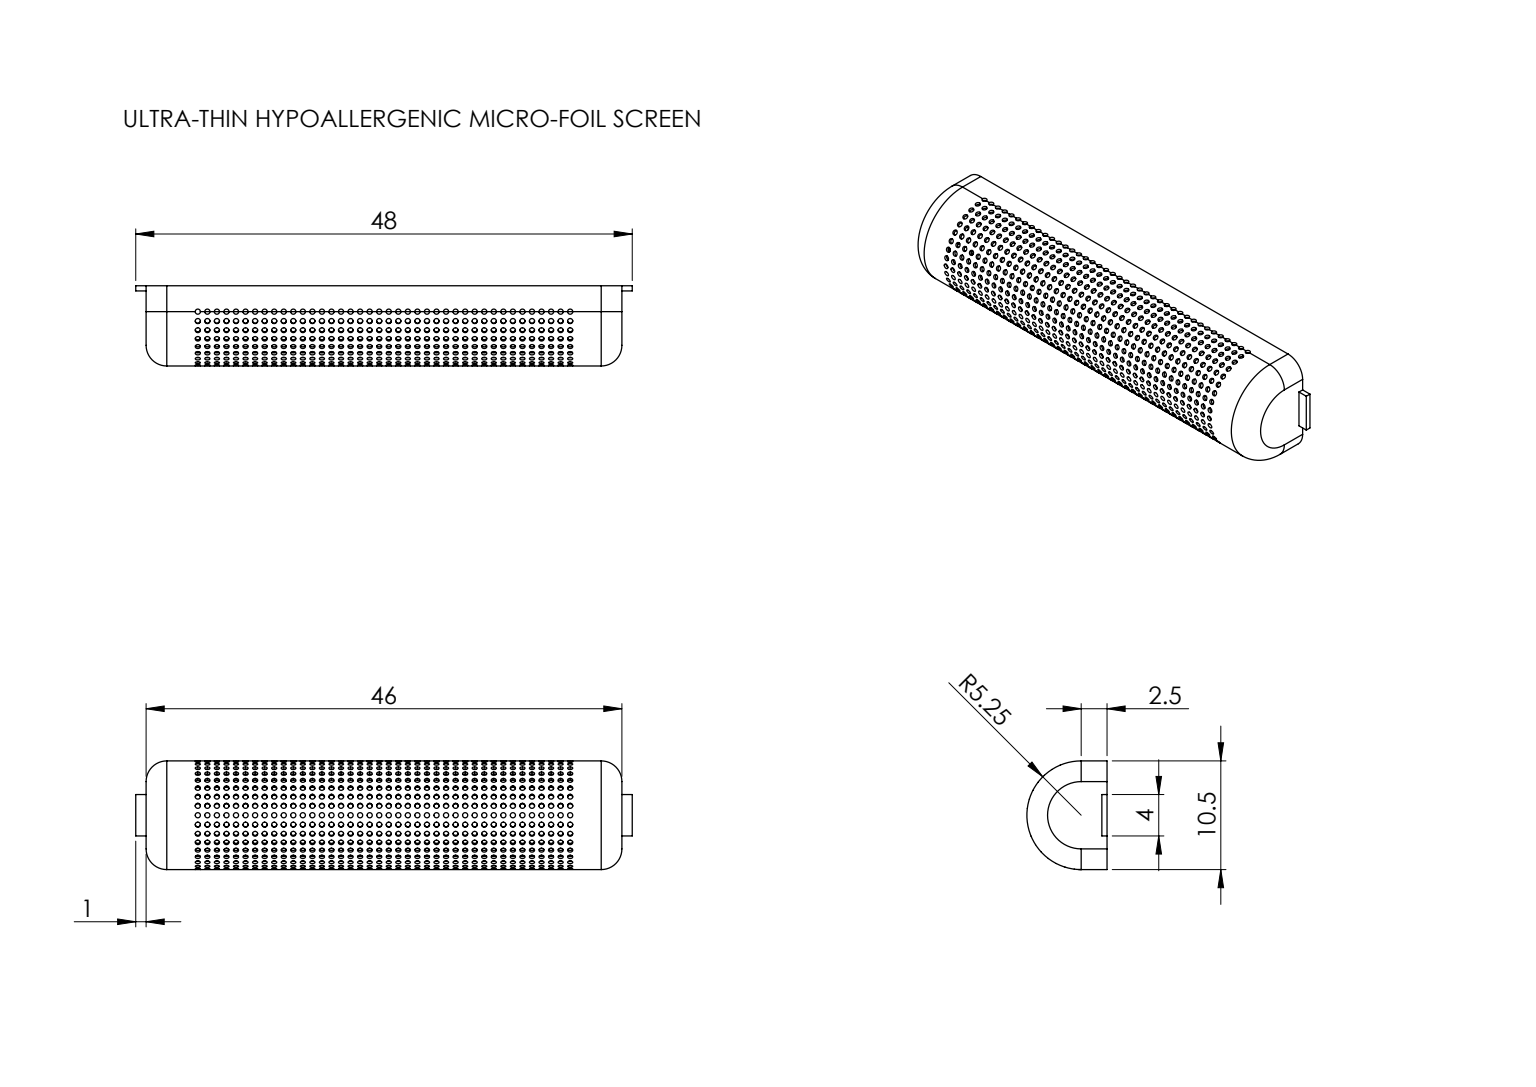
ISO-10303-21;
HEADER;
FILE_DESCRIPTION (('STEP AP214'),
    '1' );
FILE_NAME ('Ultra-Thin Hypoallergenic Micro-Foil Screen.step',
    '2026-10-05T05:16:24',
    ( '' ),
    ( '' ),
    'SwSTEP 2.0',
    'SolidWorks 2026',
    '' );
FILE_SCHEMA (( 'AUTOMOTIVE_DESIGN' ));
ENDSEC;

DATA;
#1=ORIENTED_EDGE ( 'NONE', *, *, #60678, .F. ) ;
#2=CARTESIAN_POINT ( 'NONE',  ( 7.173131342990376247, -12.65882529074907126, 30.72640787790839312 ) ) ;
#3=VERTEX_POINT ( 'NONE', #26210 ) ;
#4=CARTESIAN_POINT ( 'NONE',  ( -5.143005456283213483, -4.661471528628507777, 34.16647553114621871 ) ) ;
#5=CARTESIAN_POINT ( 'NONE',  ( -13.13461538461396394, -7.500000000000154543, 35.00000000000007105 ) ) ;
#6=CARTESIAN_POINT ( 'NONE',  ( 9.561616225640134914, -4.809359713505814149, 33.96456829005828837 ) ) ;
#7=EDGE_LOOP ( 'NONE', ( #52254, #76310 ) ) ;
#8=CARTESIAN_POINT ( 'NONE',  ( -3.230769230769352962, -3.643525952248796163, 33.31231777344771672 ) ) ;
#10=VERTEX_POINT ( 'NONE', #55017 ) ;
#11=CARTESIAN_POINT ( 'NONE',  ( 8.096099255531889582, -12.68172785388650681, 30.59649109432439218 ) ) ;
#12=ORIENTED_EDGE ( 'NONE', *, *, #66253, .T. ) ;
#13=CARTESIAN_POINT ( 'NONE',  ( -14.17690186672535901, -11.93129842949671726, 32.56571108434900452 ) ) ;
#14=ORIENTED_EDGE ( 'NONE', *, *, #40073, .T. ) ;
#15=CARTESIAN_POINT ( 'NONE',  ( 1.634669696253701288, -6.567000820036038355, 34.66262288849541306 ) ) ;
#16=AXIS2_PLACEMENT_3D ( 'NONE', #36065, #63514, #64832 ) ;
#17=CARTESIAN_POINT ( 'NONE',  ( 12.46153846153846168, -2.292212530054420494, 30.41441678777542634 ) ) ;
#18=FACE_BOUND ( 'NONE', #68088, .T. ) ;
#19=CARTESIAN_POINT ( 'NONE',  ( -17.93480601821664777, -2.506253911140446711, 29.99999999999985434 ) ) ;
#20=CARTESIAN_POINT ( 'NONE',  ( 16.08776377448601735, -3.322132147404559976, 32.92929555188719348 ) ) ;
#21=CARTESIAN_POINT ( 'NONE',  ( 9.562159722575998444, -2.373036134822904319, 30.88089517874952250 ) ) ;
#22=CARTESIAN_POINT ( 'NONE',  ( 10.36540787133602493, -10.06842814019191401, 34.32929386961144758 ) ) ;
#23=CARTESIAN_POINT ( 'NONE',  ( -3.230769230769351186, -3.300289026999228881, 32.46337939537708905 ) ) ;
#24=CARTESIAN_POINT ( 'NONE',  ( -8.096177070375302876, -9.356822207818506598, 34.66110646841856635 ) ) ;
#25=DIRECTION ( 'NONE',  ( -0.000000000000000000, 1.000000000000000000, 3.491481338843133355E-15 ) ) ;
#26=ORIENTED_EDGE ( 'NONE', *, *, #20674, .T. ) ;
#27=ORIENTED_EDGE ( 'NONE', *, *, #74196, .T. ) ;
#28=CARTESIAN_POINT ( 'NONE',  ( -17.07692307692307665, -9.780366693483667717, 34.19971097300155094 ) ) ;
#29=CYLINDRICAL_SURFACE ( 'NONE', #7462, 0.2499999999999994726 ) ;
#30=FACE_OUTER_BOUND ( 'NONE', #56324, .T. ) ;
#31=CARTESIAN_POINT ( 'NONE',  ( 3.453548772037640990, -10.81320215134717344, 33.49497208177562868 ) ) ;
#32=CARTESIAN_POINT ( 'NONE',  ( 9.019230769230707878, -7.565270000091922853, 34.99999999999999289 ) ) ;
#33=CARTESIAN_POINT ( 'NONE',  ( 11.53846153846153832, -12.09954503811598769, 35.62045528018868623 ) ) ;
#34=ORIENTED_EDGE ( 'NONE', *, *, #66033, .T. ) ;
#35=CARTESIAN_POINT ( 'NONE',  ( 2.057669070399343436, -9.271318131107980420, 34.42618302367067429 ) ) ;
#36=CARTESIAN_POINT ( 'NONE',  ( 3.453548772037639214, -11.41317474335729187, 32.86274602512330034 ) ) ;
#37=CARTESIAN_POINT ( 'NONE',  ( -14.08491263871424160, -12.47679350104403007, 31.42216943046555855 ) ) ;
#38=CARTESIAN_POINT ( 'NONE',  ( -7.053224892808619195, -6.809168938359898782, 34.95455904226513866 ) ) ;
#40=EDGE_LOOP ( 'NONE', ( #88640, #57937, #33954, #2221 ) ) ;
#41=VECTOR ( 'NONE', #83929, 1000.000000000000000 ) ;
#42=VECTOR ( 'NONE', #62583, 1000.000000000000114 ) ;
#44=CARTESIAN_POINT ( 'NONE',  ( -4.153846153846274980, -8.656820664282941280, 34.87096338111179961 ) ) ;
#45=VERTEX_POINT ( 'NONE', #81605 ) ;
#46=DIRECTION ( 'NONE',  ( -0.000000000000000000, 1.000000000000000000, 3.491481338843133355E-15 ) ) ;
#47=CARTESIAN_POINT ( 'NONE',  ( 15.45378207486262667, -4.026326845037962343, 33.68677907613344047 ) ) ;
#48=CARTESIAN_POINT ( 'NONE',  ( 4.946775867484856093, -6.852621066184267029, 34.70813303252209181 ) ) ;
#50=CIRCLE ( 'NONE', #37444, 0.2500000000000002220 ) ;
#51=CIRCLE ( 'NONE', #79120, 0.2500000000000002220 ) ;
#52=DIRECTION ( 'NONE',  ( 0.000000000000000000, 0.9848077530122072432, 0.1736481776669354937 ) ) ;
#53=VERTEX_POINT ( 'NONE', #13143 ) ;
#55=CARTESIAN_POINT ( 'NONE',  ( -15.23076923076922995, -2.486705287966279876, 31.30864560766543647 ) ) ;
#56=CARTESIAN_POINT ( 'NONE',  ( -0.5276208408985970655, -5.471508081941601986, 34.59228464037088457 ) ) ;
#57=VERTEX_POINT ( 'NONE', #40625 ) ;
#58=CARTESIAN_POINT ( 'NONE',  ( -6.923076923076922462, -2.499999999999998668, 29.50000000000001066 ) ) ;
#59=CYLINDRICAL_SURFACE ( 'NONE', #2416, 0.2500000000000002220 ) ;
#60=CARTESIAN_POINT ( 'NONE',  ( -13.60754160213153163, -4.887634598454295265, 34.01352882383564946 ) ) ;
#61=CARTESIAN_POINT ( 'NONE',  ( 11.53846153846153832, -9.905515769479276145, 34.41647553114623292 ) ) ;
#62=CARTESIAN_POINT ( 'NONE',  ( 2.438482748659261290, -2.494656445102013453, 31.33466734024120015 ) ) ;
#64=CARTESIAN_POINT ( 'NONE',  ( -3.454254174493178287, -6.760086850603068243, 34.69517049084099369 ) ) ;
#67=CARTESIAN_POINT ( 'NONE',  ( 15.00784301325308157, -8.239355502252617924, 34.69524867566427417 ) ) ;
#68=CARTESIAN_POINT ( 'NONE',  ( -14.17716686945866122, -3.625058011473228703, 33.29252011169590020 ) ) ;
#69=EDGE_CURVE ( 'NONE', #39109, #41438, #13798, .T. ) ;
#70=CARTESIAN_POINT ( 'NONE',  ( 9.692307692307695177, -10.67929555188718282, 33.92786785259544047 ) ) ;
#71=ORIENTED_EDGE ( 'NONE', *, *, #84593, .F. ) ;
#72=ORIENTED_EDGE ( 'NONE', *, *, #88944, .T. ) ;
#73=CARTESIAN_POINT ( 'NONE',  ( 20.74999999999998224, -2.499999999999999556, 27.25000000000000000 ) ) ;
#74=CARTESIAN_POINT ( 'NONE',  ( -3.100243529005668019, -6.001044277235011215, 34.52024696741798948 ) ) ;
#75=CARTESIAN_POINT ( 'NONE',  ( -16.15384615384627409, -3.835265460704628815, 33.15142922262033665 ) ) ;
#76=CARTESIAN_POINT ( 'NONE',  ( 8.769230769230768274, -1.466349020453238561, 30.81389545987213907 ) ) ;
#77=CARTESIAN_POINT ( 'NONE',  ( 17.86985203026830504, -2.647304123082329763, 31.75400227202886683 ) ) ;
#78=ORIENTED_EDGE ( 'NONE', *, *, #41184, .T. ) ;
#79=DIRECTION ( 'NONE',  ( 0.000000000000000000, 0.000000000000000000, 1.000000000000000000 ) ) ;
#81=CARTESIAN_POINT ( 'NONE',  ( -14.53117725141625094, -2.847400154188067578, 31.58180166144859058 ) ) ;
#82=LINE ( 'NONE', #529, #19231 ) ;
#83=AXIS2_PLACEMENT_3D ( 'NONE', #55221, #39954, #48454 ) ;
#84=ORIENTED_EDGE ( 'NONE', *, *, #75949, .F. ) ;
#86=EDGE_LOOP ( 'NONE', ( #15345, #5769, #84477, #70207 ) ) ;
#87=CARTESIAN_POINT ( 'NONE',  ( -16.28453762051371712, -5.582088688514999397, 34.36776431015576350 ) ) ;
#88=CYLINDRICAL_SURFACE ( 'NONE', #13871, 0.2499999999999997502 ) ;
#90=B_SPLINE_CURVE_WITH_KNOTS ( 'NONE', 3,
 ( #88183, #40422, #6186, #26896, #54800, #20574, #33653, #54355, #75089, #55682 ),
 .UNSPECIFIED., .F., .F.,
 ( 4, 2, 2, 2, 4 ),
 ( 0.000000000000000000, 0.0001954311564186868202, 0.0003908623128373736404, 0.0005862934692560604335, 0.0007817246256747472808 ),
 .UNSPECIFIED. ) ;
#91=CARTESIAN_POINT ( 'NONE',  ( 10.74591005361826035, -11.66157788607254098, 32.95092075102925833 ) ) ;
#92=CYLINDRICAL_SURFACE ( 'NONE', #79519, 0.2499999999999986955 ) ;
#93=CARTESIAN_POINT ( 'NONE',  ( 1.319344938654610333, -4.481592998940161721, 33.73612834413957984 ) ) ;
#94=CARTESIAN_POINT ( 'NONE',  ( -8.096177070375304652, -4.931416488878822335, 34.32920672191015399 ) ) ;
#95=DIRECTION ( 'NONE',  ( -0.000000000000000000, -0.7660444431189791237, -0.6427876096865379196 ) ) ;
#96=EDGE_CURVE ( 'NONE', #40194, #70315, #60434, .T. ) ;
#97=ORIENTED_EDGE ( 'NONE', *, *, #11144, .F. ) ;
#98=AXIS2_PLACEMENT_3D ( 'NONE', #21974, #77793, #7575 ) ;
#99=FACE_BOUND ( 'NONE', #31817, .T. ) ;
#100=ORIENTED_EDGE ( 'NONE', *, *, #35787, .T. ) ;
#101=CYLINDRICAL_SURFACE ( 'NONE', #51513, 0.2499999999999973355 ) ;
#102=VECTOR ( 'NONE', #77496, 999.9999999999998863 ) ;
#105=EDGE_CURVE ( 'NONE', #4412, #9551, #46022, .T. ) ;
#106=CARTESIAN_POINT ( 'NONE',  ( 4.853996859406928266, -11.76352882383564769, 32.36236540154569497 ) ) ;
#107=CARTESIAN_POINT ( 'NONE',  ( 5.999999999999878320, -5.941354392335915335, 34.76329471203413846 ) ) ;
#108=CARTESIAN_POINT ( 'NONE',  ( 7.145856464345329506, -10.11255958852956027, 34.01340905677048454 ) ) ;
#109=VECTOR ( 'NONE', #52522, 1000.000000000000227 ) ;
#110=EDGE_LOOP ( 'NONE', ( #30011, #23876 ) ) ;
#112=EDGE_LOOP ( 'NONE', ( #70272, #77319 ) ) ;
#113=FACE_OUTER_BOUND ( 'NONE', #58827, .T. ) ;
#114=ORIENTED_EDGE ( 'NONE', *, *, #66071, .T. ) ;
#115=CARTESIAN_POINT ( 'NONE',  ( 4.219913487196229163, -9.905515769479277921, 34.41647553114623292 ) ) ;
#116=B_SPLINE_CURVE_WITH_KNOTS ( 'NONE', 3,
 ( #3209, #77983, #15855, #1446, #43753, #43319, #9097, #77545, #29810, #58146 ),
 .UNSPECIFIED., .F., .F.,
 ( 4, 2, 2, 2, 4 ),
 ( 0.000000000000000000, 0.0001954311564186862239, 0.0003908623128373724478, 0.0005862934692560586988, 0.0007817246256747448956 ),
 .UNSPECIFIED. ) ;
#117=CARTESIAN_POINT ( 'NONE',  ( -11.76138849736838488, -5.582147617184174848, 34.63737895849758530 ) ) ;
#118=DIRECTION ( 'NONE',  ( 0.000000000000000000, 0.8660254037844377084, 0.5000000000000015543 ) ) ;
#119=B_SPLINE_CURVE_WITH_KNOTS ( 'NONE', 3,
 ( #65439, #64982, #64535, #3731, #23563, #51451, #79408, #16806, #85720, #17710 ),
 .UNSPECIFIED., .F., .F.,
 ( 4, 2, 2, 2, 4 ),
 ( 0.000000000000000000, 0.0001954311564186878773, 0.0003908623128373757546, 0.0005862934692560635777, 0.0007817246256747515092 ),
 .UNSPECIFIED. ) ;
#120=CARTESIAN_POINT ( 'NONE',  ( 3.361294669002876656, -9.503571793651733657, 34.60286762892837942 ) ) ;
#122=CARTESIAN_POINT ( 'NONE',  ( 5.207448778686637247, -11.46989282347013095, 32.79007818306219946 ) ) ;
#123=FACE_OUTER_BOUND ( 'NONE', #61461, .T. ) ;
#124=CARTESIAN_POINT ( 'NONE',  ( 17.29970261819148902, -2.600157965045223563, 30.74683119005207033 ) ) ;
#126=VERTEX_POINT ( 'NONE', #50456 ) ;
#127=ORIENTED_EDGE ( 'NONE', *, *, #9186, .F. ) ;
#128=CARTESIAN_POINT ( 'NONE',  ( -11.76194648218548622, -12.44517049084099725, 30.48991314939691932 ) ) ;
#129=DIRECTION ( 'NONE',  ( -0.000000000000000000, -0.1736481776669307198, -0.9848077530122080203 ) ) ;
#131=VECTOR ( 'NONE', #1295, 1000.000000000000000 ) ;
#132=CARTESIAN_POINT ( 'NONE',  ( -9.692307692307691624, -13.75783147151868846, 33.36296068462461051 ) ) ;
#133=FACE_OUTER_BOUND ( 'NONE', #80352, .T. ) ;
#134=FACE_BOUND ( 'NONE', #49727, .T. ) ;
#135=CARTESIAN_POINT ( 'NONE',  ( 7.976679547917409963, -11.46989282347013095, 32.79007818306219946 ) ) ;
#136=ORIENTED_EDGE ( 'NONE', *, *, #30561, .F. ) ;
#137=LINE ( 'NONE', #38123, #5695 ) ;
#138=LINE ( 'NONE', #88449, #37538 ) ;
#139=CARTESIAN_POINT ( 'NONE',  ( -1.515305987725692694, -3.338472653186242756, 32.95098750199972670 ) ) ;
#141=EDGE_LOOP ( 'NONE', ( #49067, #42517 ) ) ;
#142=DIRECTION ( 'NONE',  ( -1.000000000000000000, 0.000000000000000000, 0.000000000000000000 ) ) ;
#143=ORIENTED_EDGE ( 'NONE', *, *, #6318, .F. ) ;
#144=FACE_BOUND ( 'NONE', #88806, .T. ) ;
#145=CARTESIAN_POINT ( 'NONE',  ( -17.14219307747939425, -4.320704448112772766, 33.92786785259540494 ) ) ;
#146=CARTESIAN_POINT ( 'NONE',  ( -6.249999999999997335, -7.433931650972300353, 34.75000000000000711 ) ) ;
#147=CARTESIAN_POINT ( 'NONE',  ( -12.46153846153846168, -11.91647553114624181, 32.58852847137148245 ) ) ;
#148=VERTEX_POINT ( 'NONE', #49138 ) ;
#149=CARTESIAN_POINT ( 'NONE',  ( -1.384615384615383471, -12.29105614889573062, 35.45975837776705220 ) ) ;
#150=CARTESIAN_POINT ( 'NONE',  ( 4.153846153846154188, -1.367168528481310208, 33.57946703557072254 ) ) ;
#151=DIRECTION ( 'NONE',  ( -0.000000000000000000, -0.7660444431189791237, -0.6427876096865379196 ) ) ;
#152=CYLINDRICAL_SURFACE ( 'NONE', #86329, 0.2499999999999979738 ) ;
#153=ORIENTED_EDGE ( 'NONE', *, *, #56606, .F. ) ;
#154=ADVANCED_FACE ( 'NONE', ( #8609 ), #21669, .F. ) ;
#155=CARTESIAN_POINT ( 'NONE',  ( 17.99999999999987566, -5.219633306517616589, 34.19971097300220464 ) ) ;
#157=CYLINDRICAL_SURFACE ( 'NONE', #25456, 0.2499999999999997502 ) ;
#158=EDGE_LOOP ( 'NONE', ( #23871, #73123 ) ) ;
#159=DIRECTION ( 'NONE',  ( -0.000000000000000000, -0.000000000000000000, -1.000000000000000000 ) ) ;
#160=CARTESIAN_POINT ( 'NONE',  ( 0.7114838709165050012, -10.92531984108285670, 33.72920026020278073 ) ) ;
#161=CARTESIAN_POINT ( 'NONE',  ( -4.946397375159514276, -8.586989748646452369, 34.63063291749215011 ) ) ;
#162=CARTESIAN_POINT ( 'NONE',  ( -13.16183584334697265, -3.755027918224367323, 33.06320215134714857 ) ) ;
#163=LINE ( 'NONE', #28079, #50987 ) ;
#164=CARTESIAN_POINT ( 'NONE',  ( 9.019230769230768274, -2.249999999999998668, 29.75000000000000355 ) ) ;
#165=CARTESIAN_POINT ( 'NONE',  ( 6.923076923076802558, -6.026961402154118908, 34.52809138561165270 ) ) ;
#166=B_SPLINE_CURVE_WITH_KNOTS ( 'NONE', 3,
 ( #17891, #45348, #37256, #46689, #46249, #54325, #5263, #80940, #74167, #26867 ),
 .UNSPECIFIED., .F., .F.,
 ( 4, 2, 2, 2, 4 ),
 ( 0.0007817359430256306564, 0.0009771253907249969738, 0.001172514838424363291, 0.001367904286123729826, 0.001563293733823096143 ),
 .UNSPECIFIED. ) ;
#167=CARTESIAN_POINT ( 'NONE',  ( 7.976945653978636308, -4.118422570099831148, 33.43335022499816489 ) ) ;
#170=B_SPLINE_CURVE_WITH_KNOTS ( 'NONE', 3,
 ( #23736, #63848, #16993, #84585, #2145, #85454, #30936, #70611, #58864, #78697 ),
 .UNSPECIFIED., .F., .F.,
 ( 4, 2, 2, 2, 4 ),
 ( 0.000000000000000000, 0.0001954339857564080165, 0.0003908679715128160329, 0.0005863019572692240765, 0.0007817359430256320659 ),
 .UNSPECIFIED. ) ;
#171=CARTESIAN_POINT ( 'NONE',  ( -17.86947429823644029, -9.417988943895561960, 34.36773134775778260 ) ) ;
#172=ORIENTED_EDGE ( 'NONE', *, *, #13053, .F. ) ;
#173=AXIS2_PLACEMENT_3D ( 'NONE', #50512, #36570, #71672 ) ;
#174=EDGE_CURVE ( 'NONE', #81993, #52360, #48073, .T. ) ;
#175=ORIENTED_EDGE ( 'NONE', *, *, #79367, .F. ) ;
#178=CARTESIAN_POINT ( 'NONE',  ( -5.326946301144536378, -11.56360843649121861, 33.07473185843129926 ) ) ;
#180=CARTESIAN_POINT ( 'NONE',  ( 14.37376065869474751, -11.16473453929635440, 33.15142922261926373 ) ) ;
#182=CARTESIAN_POINT ( 'NONE',  ( 16.15384615384603251, -12.46129190930018460, 30.37095296980731973 ) ) ;
#183=CYLINDRICAL_SURFACE ( 'NONE', #47613, 0.2499999999999986955 ) ;
#184=AXIS2_PLACEMENT_3D ( 'NONE', #19967, #48769, #88028 ) ;
#185=DIRECTION ( 'NONE',  ( -0.000000000000000000, 0.1736481776669307198, -0.9848077530122080203 ) ) ;
#186=CARTESIAN_POINT ( 'NONE',  ( -1.384615384615383471, -4.098570777380720287, 33.41473453929634729 ) ) ;
#189=CARTESIAN_POINT ( 'NONE',  ( 10.55011416942384272, -2.625532179533445198, 30.86335684631481513 ) ) ;
#190=CARTESIAN_POINT ( 'NONE',  ( -16.94613263595612906, -10.70102852606553157, 33.91149625220312913 ) ) ;
#191=EDGE_CURVE ( 'NONE', #15565, #57014, #22554, .T. ) ;
#192=FACE_OUTER_BOUND ( 'NONE', #7478, .T. ) ;
#193=CARTESIAN_POINT ( 'NONE',  ( 11.53846153846141753, -5.219633306517616589, 34.19971097300220464 ) ) ;
#194=EDGE_CURVE ( 'NONE', #29769, #50046, #28803, .T. ) ;
#196=ORIENTED_EDGE ( 'NONE', *, *, #14784, .T. ) ;
#197=CARTESIAN_POINT ( 'NONE',  ( -7.173076923076921574, -2.249999999999998668, 29.75000000000000355 ) ) ;
#198=CARTESIAN_POINT ( 'NONE',  ( 1.515140822849032176, -3.625058011473228259, 33.29252011169590020 ) ) ;
#199=CARTESIAN_POINT ( 'NONE',  ( -6.792286482109973988, -11.93129842949671726, 32.56571108434900452 ) ) ;
#200=CARTESIAN_POINT ( 'NONE',  ( 0.3954560821783253965, -9.905515769479277921, 34.41647553114623292 ) ) ;
#202=CARTESIAN_POINT ( 'NONE',  ( 9.823098133274644539, -11.37503395064541678, 33.29242100308974273 ) ) ;
#203=FACE_OUTER_BOUND ( 'NONE', #61905, .T. ) ;
#204=AXIS2_PLACEMENT_3D ( 'NONE', #81774, #26380, #5659 ) ;
#205=CARTESIAN_POINT ( 'NONE',  ( -12.46153846153858247, -10.90142922262034020, 33.41473453929536674 ) ) ;
#206=B_SPLINE_CURVE_WITH_KNOTS ( 'NONE', 3,
 ( #5381, #32848, #40069, #18451, #4487, #53554, #45461, #67081, #59870, #45907 ),
 .UNSPECIFIED., .F., .F.,
 ( 4, 2, 2, 2, 4 ),
 ( 0.000000000000000000, 0.0001954311564186865763, 0.0003908623128373731525, 0.0005862934692560596746, 0.0007817246256747463051 ),
 .UNSPECIFIED. ) ;
#207=EDGE_CURVE ( 'NONE', #60261, #51867, #35183, .T. ) ;
#208=ORIENTED_EDGE ( 'NONE', *, *, #85819, .F. ) ;
#209=FACE_OUTER_BOUND ( 'NONE', #38454, .T. ) ;
#210=EDGE_CURVE ( 'NONE', #70883, #82406, #15810, .T. ) ;
#211=ORIENTED_EDGE ( 'NONE', *, *, #69069, .F. ) ;
#212=CARTESIAN_POINT ( 'NONE',  ( 16.15384615384603251, -9.528491918059723176, 34.59228464037033035 ) ) ;
#213=CARTESIAN_POINT ( 'NONE',  ( 8.769230769230645706, -9.528491918059723176, 34.59228464037033035 ) ) ;
#214=EDGE_CURVE ( 'NONE', #41163, #3816, #38532, .T. ) ;
#215=CARTESIAN_POINT ( 'NONE',  ( 14.05771557674995442, -4.943428324936578910, 34.04746400365624481 ) ) ;
#216=EDGE_CURVE ( 'NONE', #29227, #38893, #56032, .T. ) ;
#217=CARTESIAN_POINT ( 'NONE',  ( 16.15384615384615330, -13.63283147151868846, 33.57946703557072254 ) ) ;
#219=VERTEX_POINT ( 'NONE', #73411 ) ;
#220=ORIENTED_EDGE ( 'NONE', *, *, #40538, .F. ) ;
#221=VERTEX_POINT ( 'NONE', #52233 ) ;
#222=ORIENTED_EDGE ( 'NONE', *, *, #80830, .F. ) ;
#223=CARTESIAN_POINT ( 'NONE',  ( -10.68065461594093257, -12.51329471203370325, 31.30864560766548976 ) ) ;
#224=CARTESIAN_POINT ( 'NONE',  ( 7.596130608860882205, -3.711651800289232916, 33.01384336483936011 ) ) ;
#225=CARTESIAN_POINT ( 'NONE',  ( 4.153846153846030731, -12.16647553114689728, 32.15551576947799362 ) ) ;
#226=AXIS2_PLACEMENT_3D ( 'NONE', #60512, #52858, #32161 ) ;
#228=CARTESIAN_POINT ( 'NONE',  ( -7.846153846153844924, -4.786620604624113540, 33.94971097300155094 ) ) ;
#229=CARTESIAN_POINT ( 'NONE',  ( -15.23076923076922995, -2.486705287966279876, 31.30864560766543647 ) ) ;
#230=ORIENTED_EDGE ( 'NONE', *, *, #73529, .T. ) ;
#232=AXIS2_PLACEMENT_3D ( 'NONE', #57713, #64451, #65352 ) ;
#233=ORIENTED_EDGE ( 'NONE', *, *, #46432, .F. ) ;
#234=CARTESIAN_POINT ( 'NONE',  ( 8.769230769230647482, -9.442884908241554243, 34.35708131394783038 ) ) ;
#236=CARTESIAN_POINT ( 'NONE',  ( 17.29970274590113632, -10.97394488606063589, 33.68653795673696294 ) ) ;
#237=CARTESIAN_POINT ( 'NONE',  ( -5.010854725920638408, -11.16473453929635440, 33.15142922261926373 ) ) ;
#238=EDGE_CURVE ( 'NONE', #50121, #11896, #56698, .T. ) ;
#240=ORIENTED_EDGE ( 'NONE', *, *, #48332, .T. ) ;
#241=EDGE_CURVE ( 'NONE', #37535, #9541, #20178, .T. ) ;
#242=ORIENTED_EDGE ( 'NONE', *, *, #19023, .F. ) ;
#243=ADVANCED_FACE ( 'NONE', ( #11714 ), #66194, .F. ) ;
#244=CARTESIAN_POINT ( 'NONE',  ( 7.846153846153846700, -12.10708131394839349, 31.69288490824020244 ) ) ;
#245=FACE_BOUND ( 'NONE', #29215, .T. ) ;
#246=CARTESIAN_POINT ( 'NONE',  ( 5.076923076922953193, -5.094484230521993062, 34.41647553114689373 ) ) ;
#247=EDGE_CURVE ( 'NONE', #52855, #6141, #63243, .T. ) ;
#248=CARTESIAN_POINT ( 'NONE',  ( -4.376773112753002515, -10.01117774369187252, 34.36070679894347535 ) ) ;
#249=ORIENTED_EDGE ( 'NONE', *, *, #43935, .F. ) ;
#250=CARTESIAN_POINT ( 'NONE',  ( 8.769230769230768274, -11.91647553114624181, 32.58852847137148245 ) ) ;
#251=CARTESIAN_POINT ( 'NONE',  ( 6.923076923076800782, -12.16647553114689728, 32.15551576947799362 ) ) ;
#252=CARTESIAN_POINT ( 'NONE',  ( 16.37685750545900376, -2.554770724473668597, 30.48948780036025852 ) ) ;
#253=CARTESIAN_POINT ( 'NONE',  ( 1.384615384615386802, -10.51840700105979565, 33.73612834413961536 ) ) ;
#254=ORIENTED_EDGE ( 'NONE', *, *, #43401, .T. ) ;
#255=EDGE_CURVE ( 'NONE', #87291, #13888, #15871, .T. ) ;
#256=VECTOR ( 'NONE', #26612, 1000.000000000000227 ) ;
#257=CARTESIAN_POINT ( 'NONE',  ( -0.5268613770306369570, -7.749976743299138882, 34.99404534957040624 ) ) ;
#258=CARTESIAN_POINT ( 'NONE',  ( 1.634560902963528184, -8.433404298154336232, 34.66254593164985920 ) ) ;
#259=CARTESIAN_POINT ( 'NONE',  ( -12.68446467905460473, -12.15238873228292071, 31.58232369045353849 ) ) ;
#260=CARTESIAN_POINT ( 'NONE',  ( -2.557715544985271094, -10.76384336483936011, 33.53834819971076087 ) ) ;
#261=LINE ( 'NONE', #27723, #60185 ) ;
#262=FACE_BOUND ( 'NONE', #7058, .T. ) ;
#263=CARTESIAN_POINT ( 'NONE',  ( 17.07692307692295586, -3.835265460704628815, 33.15142922262033665 ) ) ;
#264=CARTESIAN_POINT ( 'NONE',  ( 16.82694633287448838, -2.920706130388546651, 32.31842814019191223 ) ) ;
#265=CARTESIAN_POINT ( 'NONE',  ( 5.326868486301119532, -9.357781135181031829, 34.66075350412533851 ) ) ;
#266=DIRECTION ( 'NONE',  ( 0.000000000000000000, 0.9848077530122072432, 0.1736481776669354937 ) ) ;
#267=CARTESIAN_POINT ( 'NONE',  ( -11.47239420511146513, -10.67929555188718282, 33.92786785259544757 ) ) ;
#268=AXIS2_PLACEMENT_3D ( 'NONE', #2934, #72732, #79505 ) ;
#269=CARTESIAN_POINT ( 'NONE',  ( -10.86540783960607115, -6.652501968072648708, 34.93155406624980941 ) ) ;
#271=ORIENTED_EDGE ( 'NONE', *, *, #6399, .T. ) ;
#272=DIRECTION ( 'NONE',  ( -0.000000000000000000, -0.7660444431189791237, -0.6427876096865379196 ) ) ;
#273=VERTEX_POINT ( 'NONE', #30632 ) ;
#274=CARTESIAN_POINT ( 'NONE',  ( 0.5915836243732391919, -2.504778602574659896, 29.97347330155780298 ) ) ;
#275=VERTEX_POINT ( 'NONE', #24313 ) ;
#276=CARTESIAN_POINT ( 'NONE',  ( -11.28840722682322451, -2.779044189368095275, 31.39831045268885745 ) ) ;
#277=CARTESIAN_POINT ( 'NONE',  ( -7.846153846153844924, -9.780366693483667717, 34.19971097300155094 ) ) ;
#278=CARTESIAN_POINT ( 'NONE',  ( 5.999999999999878320, -8.656820664282941280, 34.87096338111179961 ) ) ;
#279=EDGE_LOOP ( 'NONE', ( #7724, #29052, #33264, #45854 ) ) ;
#280=CARTESIAN_POINT ( 'NONE',  ( 5.299935921016470708, -11.98016756924215009, 32.48728574198911190 ) ) ;
#283=CARTESIAN_POINT ( 'NONE',  ( 3.903822916553188804, -9.271318131107980420, 34.42618302367067429 ) ) ;
#285=CARTESIAN_POINT ( 'NONE',  ( 12.21156173059611127, -2.779195860258146578, 31.39871582349836032 ) ) ;
#287=CARTESIAN_POINT ( 'NONE',  ( -0.2114841499001467451, -4.235687564193446164, 33.53795663066793509 ) ) ;
#288=CARTESIAN_POINT ( 'NONE',  ( 11.60452988946397745, -3.513871655860379306, 32.76840700105978499 ) ) ;
#290=DIRECTION ( 'NONE',  ( 0.000000000000000000, 0.9396926207859126468, 0.3420201433256571111 ) ) ;
#291=CARTESIAN_POINT ( 'NONE',  ( -1.384615384615383471, -12.78798330534102945, 29.74999999999997868 ) ) ;
#292=VERTEX_POINT ( 'NONE', #79277 ) ;
#295=AXIS2_PLACEMENT_3D ( 'NONE', #58758, #37145, #86253 ) ;
#296=LINE ( 'NONE', #12484, #72000 ) ;
#297=CARTESIAN_POINT ( 'NONE',  ( -8.769230769230892619, -3.643525952248795718, 33.31231777344771672 ) ) ;
#300=CARTESIAN_POINT ( 'NONE',  ( 17.07692307692307665, -12.78798330534102767, 29.49999999999997868 ) ) ;
#301=CARTESIAN_POINT ( 'NONE',  ( 16.15384615384603251, -2.657715359629662544, 31.77849191805970364 ) ) ;
#302=CARTESIAN_POINT ( 'NONE',  ( 4.023698184114458343, -9.504002272028875709, 34.60269587691767867 ) ) ;
#303=ORIENTED_EDGE ( 'NONE', *, *, #59543, .T. ) ;
#304=CYLINDRICAL_SURFACE ( 'NONE', #8160, 0.2500000000000009437 ) ;
#305=CARTESIAN_POINT ( 'NONE',  ( -11.53846153846153655, -2.517432740324522911, 35.29906147534542527 ) ) ;
#306=VECTOR ( 'NONE', #74624, 1000.000000000000000 ) ;
#307=MANIFOLD_SOLID_BREP ( 'Mirror3', #61571 ) ;
#308=CARTESIAN_POINT ( 'NONE',  ( 7.053867364043872712, -11.93129842949671726, 32.56571108434900452 ) ) ;
#309=CARTESIAN_POINT ( 'NONE',  ( -11.53846153846153655, -9.905515769479276145, 34.41647553114623292 ) ) ;
#310=CARTESIAN_POINT ( 'NONE',  ( -13.38461538461550582, -11.94971097300221174, 32.03036669348237098 ) ) ;
#311=ADVANCED_FACE ( 'NONE', ( #54905 ), #17579, .F. ) ;
#313=VERTEX_POINT ( 'NONE', #40952 ) ;
#314=VERTEX_POINT ( 'NONE', #12156 ) ;
#315=EDGE_CURVE ( 'NONE', #65909, #14846, #33750, .T. ) ;
#316=ORIENTED_EDGE ( 'NONE', *, *, #59548, .F. ) ;
#317=CARTESIAN_POINT ( 'NONE',  ( -16.40382289789474513, -3.436278759898155677, 33.07459398097509506 ) ) ;
#318=CARTESIAN_POINT ( 'NONE',  ( 6.673100192134572950, -2.779195860258147022, 31.39871582349836743 ) ) ;
#319=ADVANCED_FACE ( 'NONE', ( #87382 ), #67987, .F. ) ;
#320=CARTESIAN_POINT ( 'NONE',  ( -16.15384615384615330, -11.11383981884818262, 36.00935417666054406 ) ) ;
#321=CARTESIAN_POINT ( 'NONE',  ( -17.29980259366066520, -7.630690623152299956, 34.99857592706774057 ) ) ;
#322=ORIENTED_EDGE ( 'NONE', *, *, #43206, .F. ) ;
#323=ADVANCED_FACE ( 'NONE', ( #5837 ), #60772, .F. ) ;
#324=CARTESIAN_POINT ( 'NONE',  ( -18.13047670811646483, -7.276988635370451597, 34.74523720219453793 ) ) ;
#326=ORIENTED_EDGE ( 'NONE', *, *, #40277, .T. ) ;
#327=VERTEX_POINT ( 'NONE', #68417 ) ;
#328=VERTEX_POINT ( 'NONE', #87839 ) ;
#329=DIRECTION ( 'NONE',  ( 0.000000000000000000, 0.9396926207859126468, -0.3420201433256571111 ) ) ;
#330=ORIENTED_EDGE ( 'NONE', *, *, #1788, .T. ) ;
#331=CARTESIAN_POINT ( 'NONE',  ( 4.403900465484468008, -5.728107161865375829, 34.42597550085002922 ) ) ;
#333=ADVANCED_FACE ( 'NONE', ( #53570 ), #13914, .F. ) ;
#334=B_SPLINE_CURVE_WITH_KNOTS ( 'NONE', 3,
 ( #64908, #72563, #59048, #79330, #31581, #86548, #17176, #4555, #18076, #87001 ),
 .UNSPECIFIED., .F., .F.,
 ( 4, 2, 2, 2, 4 ),
 ( 0.000000000000000000, 0.0001954339857564099680, 0.0003908679715128199361, 0.0005863019572692299312, 0.0007817359430256398721 ),
 .UNSPECIFIED. ) ;
#335=B_SPLINE_CURVE_WITH_KNOTS ( 'NONE', 3,
 ( #13254, #76272, #55557, #69520, #33961, #81720, #26766, #20005, #48800, #61867 ),
 .UNSPECIFIED., .F., .F.,
 ( 4, 2, 2, 2, 4 ),
 ( 0.0007817246256747453293, 0.0009771112852218889842, 0.001172497944769032531, 0.001367884604316176294, 0.001563271263863319840 ),
 .UNSPECIFIED. ) ;
#336=LINE ( 'NONE', #27798, #62504 ) ;
#337=ADVANCED_FACE ( 'NONE', ( #33314 ), #46817, .F. ) ;
#338=CARTESIAN_POINT ( 'NONE',  ( -12.39628289026243557, -12.27809138561124591, 31.22303859784720359 ) ) ;
#340=ORIENTED_EDGE ( 'NONE', *, *, #84982, .F. ) ;
#341=EDGE_LOOP ( 'NONE', ( #3510, #61163, #15292, #57174 ) ) ;
#342=ORIENTED_EDGE ( 'NONE', *, *, #84967, .F. ) ;
#343=CARTESIAN_POINT ( 'NONE',  ( -2.242437168179467477, -3.643525952247864463, 33.31231777344670064 ) ) ;
#344=DIRECTION ( 'NONE',  ( -0.000000000000000000, -0.000000000000000000, -1.000000000000000000 ) ) ;
#346=CARTESIAN_POINT ( 'NONE',  ( 6.792385456409367528, -6.413092428213692742, 34.63065189839063152 ) ) ;
#347=ADVANCED_FACE ( 'NONE', ( #13036 ), #40520, .F. ) ;
#348=DIRECTION ( 'NONE',  ( -0.000000000000000000, 0.9848077530122085754, -0.1736481776669273613 ) ) ;
#349=EDGE_LOOP ( 'NONE', ( #49195, #32576, #79895, #88984 ) ) ;
#350=DIRECTION ( 'NONE',  ( -0.000000000000000000, -0.000000000000000000, -1.000000000000000000 ) ) ;
#352=ORIENTED_EDGE ( 'NONE', *, *, #65664, .F. ) ;
#353=FACE_BOUND ( 'NONE', #30448, .T. ) ;
#354=EDGE_CURVE ( 'NONE', #24770, #59241, #83681, .T. ) ;
#356=CARTESIAN_POINT ( 'NONE',  ( 16.02369818411445834, -2.647304123082329763, 31.75400227202886683 ) ) ;
#358=CARTESIAN_POINT ( 'NONE',  ( 7.912221179503920787, -10.67929555188718282, 33.92786785259544757 ) ) ;
#359=CARTESIAN_POINT ( 'NONE',  ( -0.4615384615384611200, -3.050289026998446396, 32.03036669348365706 ) ) ;
#360=AXIS2_PLACEMENT_3D ( 'NONE', #65343, #45520, #72546 ) ;
#361=FACE_OUTER_BOUND ( 'NONE', #8504, .T. ) ;
#363=VERTEX_POINT ( 'NONE', #29220 ) ;
#364=CARTESIAN_POINT ( 'NONE',  ( 11.53846153846153832, -5.415277668671390821, 36.20867863119892149 ) ) ;
#366=EDGE_LOOP ( 'NONE', ( #41568, #20899 ) ) ;
#367=AXIS2_PLACEMENT_3D ( 'NONE', #88511, #80411, #5626 ) ;
#368=B_SPLINE_CURVE_WITH_KNOTS ( 'NONE', 3,
 ( #9005, #62598, #77017, #71569, #35588, #35137, #64363, #36035, #36472, #2659 ),
 .UNSPECIFIED., .F., .F.,
 ( 4, 2, 2, 2, 4 ),
 ( 0.0007817246256747503166, 0.0009771112852218944052, 0.001172497944769038602, 0.001367884604316182799, 0.001563271263863326996 ),
 .UNSPECIFIED. ) ;
#370=CARTESIAN_POINT ( 'NONE',  ( -14.30769230769242917, -9.528491918059723176, 34.59228464037033035 ) ) ;
#371=CARTESIAN_POINT ( 'NONE',  ( 9.692307692307695177, -2.721908614388771852, 31.22303859784724978 ) ) ;
#372=B_SPLINE_CURVE_WITH_KNOTS ( 'NONE', 3,
 ( #22654, #8712, #16776, #20977, #9578, #2369, #77603, #30301, #37488, #70855 ),
 .UNSPECIFIED., .F., .F.,
 ( 4, 2, 2, 2, 4 ),
 ( 0.0007817246336856289524, 0.0009771112958940101571, 0.001172497958102391253, 0.001367884620310772350, 0.001563271282519153446 ),
 .UNSPECIFIED. ) ;
#373=VERTEX_POINT ( 'NONE', #845 ) ;
#374=CARTESIAN_POINT ( 'NONE',  ( -16.15384615384615330, -11.16473453929635440, 33.15142922261926373 ) ) ;
#375=CYLINDRICAL_SURFACE ( 'NONE', #76000, 0.2499999999999998890 ) ;
#376=FACE_BOUND ( 'NONE', #11299, .T. ) ;
#378=CYLINDRICAL_SURFACE ( 'NONE', #27428, 0.2500000000000002220 ) ;
#379=CARTESIAN_POINT ( 'NONE',  ( -4.087777802843714170, -8.120952969808772792, 34.71129190929999453 ) ) ;
#380=CARTESIAN_POINT ( 'NONE',  ( 7.912222197156284054, -8.973038597847271092, 34.52809138561121216 ) ) ;
#381=CARTESIAN_POINT ( 'NONE',  ( 1.450682717965462443, -12.62096338111211757, 30.90682066428152908 ) ) ;
#382=CARTESIAN_POINT ( 'NONE',  ( 0.2386122440223126528, -5.667676309546436642, 34.40238873228292249 ) ) ;
#383=FACE_OUTER_BOUND ( 'NONE', #27024, .T. ) ;
#385=ORIENTED_EDGE ( 'NONE', *, *, #9056, .F. ) ;
#386=ORIENTED_EDGE ( 'NONE', *, *, #4189, .F. ) ;
#387=CARTESIAN_POINT ( 'NONE',  ( -9.757577692864012775, -2.379036618887870436, 30.90682066428147934 ) ) ;
#388=CARTESIAN_POINT ( 'NONE',  ( 14.37294744720514572, -12.70778746994558439, 30.41441678777536595 ) ) ;
#389=CARTESIAN_POINT ( 'NONE',  ( -12.46153846153846168, -1.466349020453238561, 30.81389545987213907 ) ) ;
#390=CARTESIAN_POINT ( 'NONE',  ( -9.019207513279361876, -8.347322224742351082, 34.93158281831414058 ) ) ;
#391=CARTESIAN_POINT ( 'NONE',  ( 2.980745993476266342, -11.37209801155882971, 32.91403422569032955 ) ) ;
#394=CARTESIAN_POINT ( 'NONE',  ( -11.78846153846154010, -7.566082377512564960, 35.00000000000000711 ) ) ;
#395=CARTESIAN_POINT ( 'NONE',  ( -3.480769230769229061, -7.500000000000001776, 34.75000000000000000 ) ) ;
#396=EDGE_CURVE ( 'NONE', #70653, #65231, #6317, .T. ) ;
#397=CARTESIAN_POINT ( 'NONE',  ( 16.15384615384603251, -2.379036618888197729, 30.90682066428292885 ) ) ;
#398=CARTESIAN_POINT ( 'NONE',  ( 4.403846153847589484, -7.500000000000155431, 34.75000000000007105 ) ) ;
#399=CARTESIAN_POINT ( 'NONE',  ( -15.00798968950082291, -11.41317474335729543, 32.86274602512330034 ) ) ;
#400=CARTESIAN_POINT ( 'NONE',  ( -5.076923076923199218, -6.835583212225970762, 34.95778746994575670 ) ) ;
#401=CARTESIAN_POINT ( 'NONE',  ( 5.933916589044121004, -12.10708131394839349, 31.69288490824020244 ) ) ;
#402=CARTESIAN_POINT ( 'NONE',  ( 14.53047184896071897, -11.89424750095246175, 32.13594075562310337 ) ) ;
#403=LINE ( 'NONE', #13907, #87417 ) ;
#404=ORIENTED_EDGE ( 'NONE', *, *, #80528, .F. ) ;
#405=CARTESIAN_POINT ( 'NONE',  ( -0.2387589202700510504, -3.755027918224367767, 33.06320215134714857 ) ) ;
#406=CARTESIAN_POINT ( 'NONE',  ( 7.622668921589514923, -4.988325925672468131, 34.36044203135681130 ) ) ;
#408=LINE ( 'NONE', #82831, #54785 ) ;
#409=DIRECTION ( 'NONE',  ( -0.000000000000000000, -0.3420201433256694901, -0.9396926207859082059 ) ) ;
#410=ORIENTED_EDGE ( 'NONE', *, *, #80404, .T. ) ;
#411=DIRECTION ( 'NONE',  ( -0.000000000000000000, 1.000000000000000000, 3.491481338843133355E-15 ) ) ;
#412=DIRECTION ( 'NONE',  ( 1.000000000000000000, 0.000000000000000000, 0.000000000000000000 ) ) ;
#413=ORIENTED_EDGE ( 'NONE', *, *, #39036, .T. ) ;
#414=CARTESIAN_POINT ( 'NONE',  ( 13.38461538461538680, -13.20930481340135110, 34.54067556320372745 ) ) ;
#415=DIRECTION ( 'NONE',  ( 0.000000000000000000, 0.000000000000000000, 1.000000000000000000 ) ) ;
#416=ORIENTED_EDGE ( 'NONE', *, *, #77856, .F. ) ;
#419=ORIENTED_EDGE ( 'NONE', *, *, #191, .T. ) ;
#420=CARTESIAN_POINT ( 'NONE',  ( 16.94677586748485609, -11.47017969459903952, 32.78971311882035167 ) ) ;
#421=CARTESIAN_POINT ( 'NONE',  ( 8.096153846155281997, -7.500000000000155431, 34.75000000000007105 ) ) ;
#422=CARTESIAN_POINT ( 'NONE',  ( -15.09997742294444478, -12.38066358083363738, 30.83685684665853444 ) ) ;
#424=ORIENTED_EDGE ( 'NONE', *, *, #87981, .T. ) ;
#425=CARTESIAN_POINT ( 'NONE',  ( -10.36533019547115941, -2.318338780012835443, 30.59689888758630261 ) ) ;
#428=CARTESIAN_POINT ( 'NONE',  ( -14.98071481085577972, -4.074993327901527351, 33.72946981652012255 ) ) ;
#429=CARTESIAN_POINT ( 'NONE',  ( -1.161604033002534786, -2.554770724473667709, 30.48948780036025852 ) ) ;
#430=CARTESIAN_POINT ( 'NONE',  ( -1.384615384615506484, -11.67786785259630911, 32.92929555188603530 ) ) ;
#431=EDGE_CURVE ( 'NONE', #11896, #58120, #76950, .T. ) ;
#432=CARTESIAN_POINT ( 'NONE',  ( 0.4615384615384611200, -9.819645486525091727, 36.12317359536749706 ) ) ;
#433=CARTESIAN_POINT ( 'NONE',  ( -0.4615384615385840772, -5.941354392335915335, 34.76329471203413846 ) ) ;
#434=FACE_OUTER_BOUND ( 'NONE', #71808, .T. ) ;
#435=VECTOR ( 'NONE', #75425, 1000.000000000000000 ) ;
#436=EDGE_CURVE ( 'NONE', #46513, #56514, #28312, .T. ) ;
#437=CARTESIAN_POINT ( 'NONE',  ( 15.90382292962469180, -12.68155406624981119, 30.59749803192733708 ) ) ;
#438=ORIENTED_EDGE ( 'NONE', *, *, #56597, .F. ) ;
#440=CARTESIAN_POINT ( 'NONE',  ( -0.3954701105360236002, -12.10708131394839704, 31.69288490824020954 ) ) ;
#441=VERTEX_POINT ( 'NONE', #70189 ) ;
#443=CARTESIAN_POINT ( 'NONE',  ( -5.142193077479396912, -5.094484230520674117, 34.41647553114621161 ) ) ;
#444=ORIENTED_EDGE ( 'NONE', *, *, #26257, .F. ) ;
#445=CARTESIAN_POINT ( 'NONE',  ( 11.66925197942849302, -3.338503747796866872, 32.95102852606553512 ) ) ;
#446=CARTESIAN_POINT ( 'NONE',  ( 5.076923076922954969, -3.835265460704628371, 33.15142922262033665 ) ) ;
#447=ORIENTED_EDGE ( 'NONE', *, *, #84542, .F. ) ;
#448=DIRECTION ( 'NONE',  ( 0.000000000000000000, 0.000000000000000000, 1.000000000000000000 ) ) ;
#449=EDGE_CURVE ( 'NONE', #49542, #26693, #14245, .T. ) ;
#450=AXIS2_PLACEMENT_3D ( 'NONE', #84938, #2938, #44359 ) ;
#452=CARTESIAN_POINT ( 'NONE',  ( 7.846153846153723244, -12.70778746994576025, 30.41441678777401236 ) ) ;
#453=ORIENTED_EDGE ( 'NONE', *, *, #29446, .F. ) ;
#456=VERTEX_POINT ( 'NONE', #21105 ) ;
#457=CARTESIAN_POINT ( 'NONE',  ( 18.00000000000000000, -6.343179335718451384, 34.87096338111211935 ) ) ;
#458=CARTESIAN_POINT ( 'NONE',  ( -4.284536756956461190, -6.369640206132550553, 34.87707690430378449 ) ) ;
#459=B_SPLINE_CURVE_WITH_KNOTS ( 'NONE', 3,
 ( #38721, #52670, #86941, #51764, #3145, #31061, #37374, #10807, #11251, #64844 ),
 .UNSPECIFIED., .F., .F.,
 ( 4, 2, 2, 2, 4 ),
 ( 0.000000000000000000, 0.0001954339857564073659, 0.0003908679715128147319, 0.0005863019572692221250, 0.0007817359430256294638 ),
 .UNSPECIFIED. ) ;
#460=FACE_BOUND ( 'NONE', #10409, .T. ) ;
#461=EDGE_CURVE ( 'NONE', #35423, #73834, #49030, .T. ) ;
#462=CARTESIAN_POINT ( 'NONE',  ( 5.749976775778542937, -2.341070481393820124, 30.72580821765574299 ) ) ;
#463=CYLINDRICAL_SURFACE ( 'NONE', #51418, 0.2500000000000004996 ) ;
#464=CARTESIAN_POINT ( 'NONE',  ( 9.442330948259105128, -11.47974371597207899, 33.17467449705390692 ) ) ;
#465=CARTESIAN_POINT ( 'NONE',  ( -17.07692307692307665, -12.34228464037088635, 31.77849191805839268 ) ) ;
#466=CARTESIAN_POINT ( 'NONE',  ( -17.32689982097166492, -8.347322224742351082, 34.93158281831414058 ) ) ;
#467=CARTESIAN_POINT ( 'NONE',  ( -4.219116599806928214, -11.48612834413959582, 32.76840700105983473 ) ) ;
#468=EDGE_CURVE ( 'NONE', #6055, #84853, #21558, .T. ) ;
#470=EDGE_LOOP ( 'NONE', ( #48935, #2508, #11631, #61677 ) ) ;
#471=ORIENTED_EDGE ( 'NONE', *, *, #28570, .F. ) ;
#473=CARTESIAN_POINT ( 'NONE',  ( 15.00728428704528561, -12.24155766932282496, 31.33739205006857986 ) ) ;
#474=CARTESIAN_POINT ( 'NONE',  ( -11.66915300512909859, -11.71456829005830080, 32.44064028649416542 ) ) ;
#475=DIRECTION ( 'NONE',  ( -0.000000000000000000, 0.5000000000000011102, -0.8660254037844380415 ) ) ;
#476=CARTESIAN_POINT ( 'NONE',  ( -14.30769230769230660, -3.513871655860378418, 32.76840700105978499 ) ) ;
#477=CYLINDRICAL_SURFACE ( 'NONE', #63424, 0.2499999999999997502 ) ;
#478=EDGE_LOOP ( 'NONE', ( #50034, #54764 ) ) ;
#479=CARTESIAN_POINT ( 'NONE',  ( 13.31853197365950692, -4.786620604624113540, 33.94971097300155805 ) ) ;
#480=EDGE_CURVE ( 'NONE', #74721, #66781, #42289, .T. ) ;
#481=LINE ( 'NONE', #56306, #79055 ) ;
#482=DIRECTION ( 'NONE',  ( 0.000000000000000000, 0.000000000000000000, 1.000000000000000000 ) ) ;
#484=EDGE_LOOP ( 'NONE', ( #60123, #67289, #74118, #28070 ) ) ;
#485=VERTEX_POINT ( 'NONE', #68858 ) ;
#486=AXIS2_PLACEMENT_3D ( 'NONE', #32374, #72456, #59839 ) ;
#487=EDGE_LOOP ( 'NONE', ( #82911, #37209, #13825, #34035 ) ) ;
#488=CARTESIAN_POINT ( 'NONE',  ( -9.442362173959550020, -12.43552623307873972, 30.55307653245132826 ) ) ;
#489=ORIENTED_EDGE ( 'NONE', *, *, #55931, .T. ) ;
#490=CARTESIAN_POINT ( 'NONE',  ( -9.561517251340744039, -9.929761469519743144, 34.40412654351204225 ) ) ;
#491=CYLINDRICAL_SURFACE ( 'NONE', #21511, 0.2500000000000009437 ) ;
#492=CARTESIAN_POINT ( 'NONE',  ( 14.30769230769231015, -5.180354513474913603, 36.12317359536750416 ) ) ;
#494=ADVANCED_FACE ( 'NONE', ( #69745 ), #7164, .F. ) ;
#495=CYLINDRICAL_SURFACE ( 'NONE', #2877, 0.2499999999999986955 ) ;
#497=CARTESIAN_POINT ( 'NONE',  ( 4.403791672194295792, -4.336752205174647656, 33.62275283266504289 ) ) ;
#500=CARTESIAN_POINT ( 'NONE',  ( -9.561781990544126586, -4.459921816937791661, 33.71989282347011851 ) ) ;
#501=CARTESIAN_POINT ( 'NONE',  ( -8.992110285968356820, -7.630690623152299956, 34.99857592706774057 ) ) ;
#502=CYLINDRICAL_SURFACE ( 'NONE', #24257, 0.2500000000000002220 ) ;
#503=B_SPLINE_CURVE_WITH_KNOTS ( 'NONE', 3,
 ( #55324, #55765, #21540, #35953, #49893, #76935, #63408, #77371, #42272, #34617 ),
 .UNSPECIFIED., .F., .F.,
 ( 4, 2, 2, 2, 4 ),
 ( 0.0007817359527651090859, 0.0009771254036996478414, 0.001172514854634186489, 0.001367904305568725136, 0.001563293756503263783 ),
 .UNSPECIFIED. ) ;
#504=EDGE_CURVE ( 'NONE', #73834, #24183, #58251, .T. ) ;
#506=CARTESIAN_POINT ( 'NONE',  ( 9.822833394071261992, -10.88167719472716399, 33.43325721877153711 ) ) ;
#507=CARTESIAN_POINT ( 'NONE',  ( -9.822455662039391910, -12.50552854090298993, 31.33409797877408920 ) ) ;
#508=CARTESIAN_POINT ( 'NONE',  ( 17.32692307692451195, -7.500000000000155431, 34.75000000000007105 ) ) ;
#509=B_SPLINE_CURVE_WITH_KNOTS ( 'NONE', 3,
 ( #53464, #32756, #11153, #32322, #19251, #59784, #88619, #20134, #12059, #47600 ),
 .UNSPECIFIED., .F., .F.,
 ( 4, 2, 2, 2, 4 ),
 ( 0.000000000000000000, 0.0001954311584214071026, 0.0003908623168428142051, 0.0005862934752642213077, 0.0007817246336856284103 ),
 .UNSPECIFIED. ) ;
#510=CARTESIAN_POINT ( 'NONE',  ( -3.296852641725110722, -6.386643153685125363, 34.62446782046654903 ) ) ;
#512=ORIENTED_EDGE ( 'NONE', *, *, #29886, .T. ) ;
#513=B_SPLINE_CURVE_WITH_KNOTS ( 'NONE', 3,
 ( #47860, #40679, #88875, #68140, #13632, #69020, #14520, #28035, #82556, #69465 ),
 .UNSPECIFIED., .F., .F.,
 ( 4, 2, 2, 2, 4 ),
 ( 0.000000000000000000, 0.0001954339857564093175, 0.0003908679715128186350, 0.0005863019572692279796, 0.0007817359430256372700 ),
 .UNSPECIFIED. ) ;
#514=EDGE_CURVE ( 'NONE', #25678, #10982, #60501, .T. ) ;
#515=CARTESIAN_POINT ( 'NONE',  ( -16.94613126909828793, -10.54018710029568595, 33.71981072465678864 ) ) ;
#516=FACE_OUTER_BOUND ( 'NONE', #38907, .T. ) ;
#517=CARTESIAN_POINT ( 'NONE',  ( 8.899756207464411872, -11.04252011169590020, 33.62494198852677130 ) ) ;
#519=VERTEX_POINT ( 'NONE', #78265 ) ;
#520=CARTESIAN_POINT ( 'NONE',  ( -4.153846153846152411, -4.661471528628507777, 34.16647553114623292 ) ) ;
#521=CARTESIAN_POINT ( 'NONE',  ( 11.28848479441295005, -4.075325502946081535, 33.72974371597206300 ) ) ;
#522=CARTESIAN_POINT ( 'NONE',  ( 1.161689167099238862, -9.086856451489515152, 34.49173150075333183 ) ) ;
#524=CARTESIAN_POINT ( 'NONE',  ( -6.000000000000119904, -6.879047030192662504, 34.71129190930017927 ) ) ;
#526=ORIENTED_EDGE ( 'NONE', *, *, #76556, .F. ) ;
#527=CARTESIAN_POINT ( 'NONE',  ( 16.94623161025551639, -3.062553014421049991, 32.05460306192773601 ) ) ;
#529=CARTESIAN_POINT ( 'NONE',  ( 12.46153846153846168, -1.629998284177014645, 34.34916445242399163 ) ) ;
#530=VERTEX_POINT ( 'NONE', #79611 ) ;
#531=CARTESIAN_POINT ( 'NONE',  ( -2.557692307692305267, -7.500000000000001776, 34.75000000000000000 ) ) ;
#533=CARTESIAN_POINT ( 'NONE',  ( -2.373775718648186928, -12.10708131394839349, 31.69288490824020244 ) ) ;
#535=VERTEX_POINT ( 'NONE', #30960 ) ;
#536=DIRECTION ( 'NONE',  ( 0.000000000000000000, 0.4999999999999960032, -0.8660254037844410391 ) ) ;
#538=CARTESIAN_POINT ( 'NONE',  ( -11.78843826940389583, -6.567427716900048118, 34.66269422305636283 ) ) ;
#539=B_SPLINE_CURVE_WITH_KNOTS ( 'NONE', 3,
 ( #46049, #67220, #52352, #73535, #39310, #24434, #66766, #5067, #60006, #5518 ),
 .UNSPECIFIED., .F., .F.,
 ( 4, 2, 2, 2, 4 ),
 ( 0.0007817359430256372700, 0.0009771253907250054306, 0.001172514838424373483, 0.001367904286123741535, 0.001563293733823109804 ),
 .UNSPECIFIED. ) ;
#540=B_SPLINE_CURVE_WITH_KNOTS ( 'NONE', 3,
 ( #44835, #25469, #38544, #3854, #5198, #87634, #25913, #52038, #30880, #10621 ),
 .UNSPECIFIED., .F., .F.,
 ( 4, 2, 2, 2, 4 ),
 ( 0.0007817359430256392216, 0.0009771253907250073822, 0.001172514838424375651, 0.001367904286123743920, 0.001563293733823112189 ),
 .UNSPECIFIED. ) ;
#541=CARTESIAN_POINT ( 'NONE',  ( -0.7115384615384606759, -7.500000000000001776, 35.04278698407183867 ) ) ;
#542=CARTESIAN_POINT ( 'NONE',  ( -6.923076923076922462, -1.367168528481310208, 33.57946703557072254 ) ) ;
#543=B_SPLINE_CURVE_WITH_KNOTS ( 'NONE', 3,
 ( #64384, #38707, #65281, #4016, #4480, #31504, #58970, #2684, #57642, #86473 ),
 .UNSPECIFIED., .F., .F.,
 ( 4, 2, 2, 2, 4 ),
 ( 0.000000000000000000, 0.0001954311564186865221, 0.0003908623128373730441, 0.0005862934692560595662, 0.0007817246256747460882 ),
 .UNSPECIFIED. ) ;
#546=FACE_BOUND ( 'NONE', #34527, .T. ) ;
#547=ORIENTED_EDGE ( 'NONE', *, *, #30603, .T. ) ;
#549=VECTOR ( 'NONE', #26235, 1000.000000000000227 ) ;
#551=CARTESIAN_POINT ( 'NONE',  ( 4.826899839630111266, -11.86270091957321249, 32.19358267280087915 ) ) ;
#552=DIRECTION ( 'NONE',  ( -0.000000000000000000, -0.8660254037844397068, -0.4999999999999978906 ) ) ;
#553=CARTESIAN_POINT ( 'NONE',  ( 14.37375964104238513, -8.164416787775445883, 34.95778746994558617 ) ) ;
#554=ORIENTED_EDGE ( 'NONE', *, *, #61196, .F. ) ;
#555=ORIENTED_EDGE ( 'NONE', *, *, #60770, .T. ) ;
#556=ORIENTED_EDGE ( 'NONE', *, *, #27457, .T. ) ;
#558=VERTEX_POINT ( 'NONE', #38171 ) ;
#559=CARTESIAN_POINT ( 'NONE',  ( 4.403900573759606196, -10.06805714834173848, 34.32951233291982618 ) ) ;
#560=CARTESIAN_POINT ( 'NONE',  ( -16.82692307692307665, -2.499999999999998668, 29.75000000000000355 ) ) ;
#561=CARTESIAN_POINT ( 'NONE',  ( -18.06527000055631760, -6.835583212224500826, 34.95778746994557906 ) ) ;
#562=CARTESIAN_POINT ( 'NONE',  ( -5.076923076923197442, -10.90142922262034020, 33.41473453929536674 ) ) ;
#563=ADVANCED_FACE ( 'NONE', ( #72839 ), #85923, .F. ) ;
#564=B_SPLINE_CURVE_WITH_KNOTS ( 'NONE', 3,
 ( #69872, #41076, #87, #61323, #27112, #74871, #49153, #76634, #75736, #54575 ),
 .UNSPECIFIED., .F., .F.,
 ( 4, 2, 2, 2, 4 ),
 ( 0.000000000000000000, 0.0001954339857564075015, 0.0003908679715128150029, 0.0005863019572692224502, 0.0007817359430256300059 ),
 .UNSPECIFIED. ) ;
#565=CARTESIAN_POINT ( 'NONE',  ( 17.07692307692295586, -4.481592998941358097, 33.73612834414048933 ) ) ;
#566=CARTESIAN_POINT ( 'NONE',  ( 15.36156103859402222, -8.999086150933475636, 34.52020707165672775 ) ) ;
#567=FACE_OUTER_BOUND ( 'NONE', #79244, .T. ) ;
#568=B_SPLINE_CURVE_WITH_KNOTS ( 'NONE', 3,
 ( #50304, #64261, #58842, #19201, #52528, #86350, #31835, #17873, #30920, #12009 ),
 .UNSPECIFIED., .F., .F.,
 ( 4, 2, 2, 2, 4 ),
 ( 0.0007817246256747451124, 0.0009771112852218881168, 0.001172497944769031230, 0.001367884604316174126, 0.001563271263863317238 ),
 .UNSPECIFIED. ) ;
#569=CARTESIAN_POINT ( 'NONE',  ( -8.769230769230768274, -2.833524468853757305, 32.15551576947925838 ) ) ;
#570=ORIENTED_EDGE ( 'NONE', *, *, #5698, .T. ) ;
#571=EDGE_LOOP ( 'NONE', ( #21663, #30842, #13535, #23130 ) ) ;
#572=VERTEX_POINT ( 'NONE', #44919 ) ;
#574=VECTOR ( 'NONE', #40145, 1000.000000000000114 ) ;
#575=DIRECTION ( 'NONE',  ( 0.000000000000000000, 0.000000000000000000, 1.000000000000000000 ) ) ;
#576=CARTESIAN_POINT ( 'NONE',  ( 10.61538461538461675, -13.63283147151868846, 33.57946703557072254 ) ) ;
#577=CARTESIAN_POINT ( 'NONE',  ( 1.515405825582335497, -12.35292014791297710, 31.75344720912887198 ) ) ;
#578=CARTESIAN_POINT ( 'NONE',  ( -6.673022611438608642, -3.627508038966690496, 32.91356715214248396 ) ) ;
#579=FACE_BOUND ( 'NONE', #10836, .T. ) ;
#580=CARTESIAN_POINT ( 'NONE',  ( 16.15384615384615330, -3.050289026998446396, 32.03036669348365706 ) ) ;
#581=ORIENTED_EDGE ( 'NONE', *, *, #27829, .T. ) ;
#582=LINE ( 'NONE', #53856, #58701 ) ;
#583=EDGE_CURVE ( 'NONE', #87491, #41440, #57996, .T. ) ;
#585=CARTESIAN_POINT ( 'NONE',  ( 16.82689983963011926, -6.695914987888146541, 34.68535235679833306 ) ) ;
#586=CARTESIAN_POINT ( 'NONE',  ( 7.146089767170319185, -9.172514111537584114, 34.72667873470787470 ) ) ;
#587=ORIENTED_EDGE ( 'NONE', *, *, #4080, .T. ) ;
#588=CARTESIAN_POINT ( 'NONE',  ( 18.22301135161285046, -12.39991518177334129, 30.74647679643404530 ) ) ;
#589=EDGE_LOOP ( 'NONE', ( #40662, #68267, #42370, #16279 ) ) ;
#590=FACE_BOUND ( 'NONE', #13874, .T. ) ;
#591=CARTESIAN_POINT ( 'NONE',  ( -17.07692307692319744, -4.320704448113951379, 33.92786785259630022 ) ) ;
#592=CARTESIAN_POINT ( 'NONE',  ( -12.33101275977490197, -8.586989748646452369, 34.63063291749215011 ) ) ;
#593=CARTESIAN_POINT ( 'NONE',  ( -0.4615384615384611200, -9.584722331328613620, 36.20867863119891439 ) ) ;
#594=ORIENTED_EDGE ( 'NONE', *, *, #40606, .F. ) ;
#595=CARTESIAN_POINT ( 'NONE',  ( 0.2386122440223146512, -10.61292498521070549, 33.66303323003028680 ) ) ;
#596=CARTESIAN_POINT ( 'NONE',  ( 5.326923076924511946, -7.500000000000155431, 34.75000000000007105 ) ) ;
#597=CARTESIAN_POINT ( 'NONE',  ( 18.13052543823364360, -11.04252011169589842, 33.62494198852677840 ) ) ;
#599=ORIENTED_EDGE ( 'NONE', *, *, #70850, .F. ) ;
#600=CARTESIAN_POINT ( 'NONE',  ( 16.28463796167093847, -10.54018710029568595, 33.71981072465678864 ) ) ;
#601=ORIENTED_EDGE ( 'NONE', *, *, #47247, .T. ) ;
#602=CARTESIAN_POINT ( 'NONE',  ( -39.05038313613820122, -12.50000000000000000, 29.75000000000000355 ) ) ;
#603=VERTEX_POINT ( 'NONE', #44032 ) ;
#604=CARTESIAN_POINT ( 'NONE',  ( 15.93036122928181975, -4.225889041578354544, 33.85425143139329407 ) ) ;
#605=CARTESIAN_POINT ( 'NONE',  ( -6.792551221313358312, -11.93748526763465279, 32.05452791011430946 ) ) ;
#606=CARTESIAN_POINT ( 'NONE',  ( 13.13463865367303463, -9.148715823498378086, 34.47080413974185120 ) ) ;
#607=CARTESIAN_POINT ( 'NONE',  ( 14.08476609017615644, -9.086856451489515152, 34.49173150075333183 ) ) ;
#608=ADVANCED_FACE ( 'NONE', ( #4389 ), #80051, .F. ) ;
#609=EDGE_CURVE ( 'NONE', #36550, #75687, #65629, .T. ) ;
#610=CARTESIAN_POINT ( 'NONE',  ( -39.05038313613820122, -2.499999999999999556, 29.75000000000000355 ) ) ;
#611=CARTESIAN_POINT ( 'NONE',  ( -15.23076923076935252, -3.083524468854526912, 32.58852847137268327 ) ) ;
#613=CARTESIAN_POINT ( 'NONE',  ( 8.096208157792162297, -4.235687564193446164, 33.53795663066793509 ) ) ;
#614=B_SPLINE_CURVE_WITH_KNOTS ( 'NONE', 3,
 ( #6623, #34090, #7516, #89062, #34972, #75520, #19692, #54356, #26007, #33654 ),
 .UNSPECIFIED., .F., .F.,
 ( 4, 2, 2, 2, 4 ),
 ( 0.000000000000000000, 0.0001954339857564085315, 0.0003908679715128170629, 0.0005863019572692255944, 0.0007817359430256341259 ),
 .UNSPECIFIED. ) ;
#616=ORIENTED_EDGE ( 'NONE', *, *, #51029, .F. ) ;
#618=FACE_OUTER_BOUND ( 'NONE', #12115, .T. ) ;
#620=VECTOR ( 'NONE', #80304, 1000.000000000000000 ) ;
#621=ADVANCED_FACE ( 'NONE', ( #23757 ), #78718, .F. ) ;
#622=VERTEX_POINT ( 'NONE', #17015 ) ;
#623=CARTESIAN_POINT ( 'NONE',  ( 3.164685819813350509, -4.786620604624113540, 33.94971097300155805 ) ) ;
#624=EDGE_LOOP ( 'NONE', ( #77449, #46209, #13975, #53295 ) ) ;
#625=CARTESIAN_POINT ( 'NONE',  ( -15.23076923076922995, -2.721908614388771852, 31.22303859784724978 ) ) ;
#626=CARTESIAN_POINT ( 'NONE',  ( -8.069080805060693251, -8.282780595021769443, 34.94152052738834158 ) ) ;
#627=FACE_OUTER_BOUND ( 'NONE', #35004, .T. ) ;
#628=FACE_OUTER_BOUND ( 'NONE', #50378, .T. ) ;
#629=CARTESIAN_POINT ( 'NONE',  ( 10.83816428436268176, -6.717445702608402236, 34.94155399931962336 ) ) ;
#630=CARTESIAN_POINT ( 'NONE',  ( -8.769230769230892619, -2.657715359629662544, 31.77849191805970364 ) ) ;
#631=DIRECTION ( 'NONE',  ( -0.000000000000000000, 0.6427876096865404731, -0.7660444431189771253 ) ) ;
#632=CARTESIAN_POINT ( 'NONE',  ( 6.857806922520603976, -10.33852847137145048, 34.16647553114627556 ) ) ;
#633=CARTESIAN_POINT ( 'NONE',  ( -2.176901866725353241, -2.845873456487966635, 32.17976146951972538 ) ) ;
#635=LINE ( 'NONE', #42076, #15392 ) ;
#636=B_SPLINE_CURVE_WITH_KNOTS ( 'NONE', 3,
 ( #21746, #28510, #84351, #50094, #8244, #29406, #50962, #1034, #2345, #42918 ),
 .UNSPECIFIED., .F., .F.,
 ( 4, 2, 2, 2, 4 ),
 ( 0.0007817359430256317406, 0.0009771253907249982749, 0.001172514838424365026, 0.001367904286123731560, 0.001563293733823098094 ),
 .UNSPECIFIED. ) ;
#637=EDGE_LOOP ( 'NONE', ( #36007, #70907 ) ) ;
#638=ORIENTED_EDGE ( 'NONE', *, *, #72178, .F. ) ;
#639=CARTESIAN_POINT ( 'NONE',  ( 12.46153846153833911, -2.657715359629662544, 31.77849191805970364 ) ) ;
#640=CARTESIAN_POINT ( 'NONE',  ( 0.7114838709165033359, -12.07971442181321997, 32.31769673815850297 ) ) ;
#642=LINE ( 'NONE', #55575, #34057 ) ;
#643=CARTESIAN_POINT ( 'NONE',  ( -16.08777882049607655, -8.164416787775445883, 34.95778746994558617 ) ) ;
#644=CARTESIAN_POINT ( 'NONE',  ( -6.130691466667557599, -8.147922237126337563, 34.70805685702651999 ) ) ;
#645=AXIS2_PLACEMENT_3D ( 'NONE', #22951, #25062, #80914 ) ;
#646=DIRECTION ( 'NONE',  ( 0.000000000000000000, 0.000000000000000000, 1.000000000000000000 ) ) ;
#648=CARTESIAN_POINT ( 'NONE',  ( 6.923076923076924238, -4.945431358278436385, 36.03766855953609394 ) ) ;
#649=ORIENTED_EDGE ( 'NONE', *, *, #54191, .F. ) ;
#650=CYLINDRICAL_SURFACE ( 'NONE', #59244, 0.2500000000000002220 ) ;
#651=LINE ( 'NONE', #55589, #47066 ) ;
#652=CARTESIAN_POINT ( 'NONE',  ( -0.3307466537136748430, -6.413143153341451352, 34.63066358083362672 ) ) ;
#653=DIRECTION ( 'NONE',  ( -0.000000000000000000, -0.5000000000000009992, -0.8660254037844380415 ) ) ;
#654=CARTESIAN_POINT ( 'NONE',  ( 5.869852790561782996, -2.882441371585227063, 31.66841991370171527 ) ) ;
#655=EDGE_CURVE ( 'NONE', #29143, #16341, #58885, .T. ) ;
#656=EDGE_LOOP ( 'NONE', ( #72252, #17241 ) ) ;
#657=EDGE_LOOP ( 'NONE', ( #24562, #75991 ) ) ;
#658=EDGE_CURVE ( 'NONE', #7553, #4867, #48697, .T. ) ;
#660=ORIENTED_EDGE ( 'NONE', *, *, #52723, .T. ) ;
#661=CARTESIAN_POINT ( 'NONE',  ( -5.999999999999998224, -1.629998284177014645, 34.34916445242399163 ) ) ;
#662=CARTESIAN_POINT ( 'NONE',  ( -12.71151520558705350, -12.65889640711025521, 30.72598325615533454 ) ) ;
#663=CARTESIAN_POINT ( 'NONE',  ( 4.403900573759607084, -12.01375889529407281, 32.43194544308182969 ) ) ;
#664=VECTOR ( 'NONE', #76082, 1000.000000000000114 ) ;
#665=VECTOR ( 'NONE', #5935, 1000.000000000000000 ) ;
#666=CARTESIAN_POINT ( 'NONE',  ( 14.37283708841194318, -7.750023224968867197, 34.99404313364389907 ) ) ;
#667=EDGE_CURVE ( 'NONE', #82157, #47301, #84125, .T. ) ;
#668=CARTESIAN_POINT ( 'NONE',  ( 17.77651507543566822, -3.019605429927187501, 32.48692288466676814 ) ) ;
#669=DIRECTION ( 'NONE',  ( -0.000000000000000000, -0.9848077530122085754, -0.1736481776669273613 ) ) ;
#670=ORIENTED_EDGE ( 'NONE', *, *, #69279, .T. ) ;
#671=EDGE_CURVE ( 'NONE', #32456, #13048, #12924, .T. ) ;
#672=ORIENTED_EDGE ( 'NONE', *, *, #46655, .T. ) ;
#673=VERTEX_POINT ( 'NONE', #5723 ) ;
#674=CARTESIAN_POINT ( 'NONE',  ( 4.023698944407934519, -2.882441371585227063, 31.66841991370171527 ) ) ;
#675=ORIENTED_EDGE ( 'NONE', *, *, #8517, .T. ) ;
#676=CARTESIAN_POINT ( 'NONE',  ( 10.39245839786846837, -12.39988816332205701, 30.74660775122750778 ) ) ;
#677=DIRECTION ( 'NONE',  ( 0.000000000000000000, 1.000000000000000000, 0.000000000000000000 ) ) ;
#679=ORIENTED_EDGE ( 'NONE', *, *, #61599, .T. ) ;
#680=EDGE_CURVE ( 'NONE', #18725, #44707, #22528, .T. ) ;
#682=CARTESIAN_POINT ( 'NONE',  ( 5.142067857642707018, -7.750023224968867197, 34.99404313364389907 ) ) ;
#683=VERTEX_POINT ( 'NONE', #12485 ) ;
#684=FACE_BOUND ( 'NONE', #47971, .T. ) ;
#685=CARTESIAN_POINT ( 'NONE',  ( 3.230769230769108269, -2.657715359629662544, 31.77849191805970364 ) ) ;
#687=ORIENTED_EDGE ( 'NONE', *, *, #60462, .T. ) ;
#688=CARTESIAN_POINT ( 'NONE',  ( -6.700297381808512753, -5.114059244376869984, 34.14424750095245287 ) ) ;
#689=CARTESIAN_POINT ( 'NONE',  ( -16.02332071561251325, -12.70449254468099198, 30.44128974285582956 ) ) ;
#690=CARTESIAN_POINT ( 'NONE',  ( 8.899756207464417201, -8.630441415882550871, 34.87705825610312615 ) ) ;
#692=CARTESIAN_POINT ( 'NONE',  ( -3.453696189676080053, -9.172386477786396597, 34.72672124145550043 ) ) ;
#693=ORIENTED_EDGE ( 'NONE', *, *, #28396, .T. ) ;
#694=B_SPLINE_CURVE_WITH_KNOTS ( 'NONE', 3,
 ( #37095, #16831, #71325, #9629, #64555, #46532, #25818, #73575, #37996, #12301 ),
 .UNSPECIFIED., .F., .F.,
 ( 4, 2, 2, 2, 4 ),
 ( 0.000000000000000000, 0.0001954311564186864949, 0.0003908623128373729899, 0.0005862934692560594577, 0.0007817246256747459798 ),
 .UNSPECIFIED. ) ;
#696=CARTESIAN_POINT ( 'NONE',  ( 15.90384615384615330, -7.500000000000001776, 34.75000000000000000 ) ) ;
#697=CARTESIAN_POINT ( 'NONE',  ( -5.933932666649925025, -3.937682226553329556, 33.60647404775216529 ) ) ;
#698=CARTESIAN_POINT ( 'NONE',  ( 0.2115617305961062233, -11.79746400365624659, 32.30657167506340954 ) ) ;
#699=CYLINDRICAL_SURFACE ( 'NONE', #86069, 0.2499999999999979738 ) ;
#700=FACE_OUTER_BOUND ( 'NONE', #21142, .T. ) ;
#701=EDGE_CURVE ( 'NONE', #47506, #74563, #43282, .T. ) ;
#702=FACE_BOUND ( 'NONE', #7070, .T. ) ;
#703=CARTESIAN_POINT ( 'NONE',  ( 8.769230769230768274, -1.629998284177014645, 34.34916445242399163 ) ) ;
#704=CARTESIAN_POINT ( 'NONE',  ( 16.40384615384757439, -7.500000000000154543, 35.00000000000007105 ) ) ;
#705=CARTESIAN_POINT ( 'NONE',  ( 5.326977496836529546, -9.233818618650603938, 34.70587769442853698 ) ) ;
#707=CARTESIAN_POINT ( 'NONE',  ( -6.222926217516146608, -4.887634598454295265, 34.01352882383564946 ) ) ;
#708=ADVANCED_FACE ( 'NONE', ( #88171 ), #40412, .F. ) ;
#709=LINE ( 'NONE', #20095, #66392 ) ;
#711=EDGE_LOOP ( 'NONE', ( #17027, #50438 ) ) ;
#712=CARTESIAN_POINT ( 'NONE',  ( 1.254468175177162914, -12.27039167877662251, 31.24851455888617835 ) ) ;
#713=EDGE_LOOP ( 'NONE', ( #36866, #45226, #35384, #85177 ) ) ;
#714=CARTESIAN_POINT ( 'NONE',  ( -13.25408994638174320, -11.04252011169590020, 33.62494198852677130 ) ) ;
#715=EDGE_CURVE ( 'NONE', #45738, #29450, #27327, .T. ) ;
#716=ORIENTED_EDGE ( 'NONE', *, *, #29790, .F. ) ;
#718=CARTESIAN_POINT ( 'NONE',  ( -11.28851612908349722, -6.653508905675592722, 34.93172785388651391 ) ) ;
#719=LINE ( 'NONE', #86139, #25829 ) ;
#720=VERTEX_POINT ( 'NONE', #73297 ) ;
#721=CARTESIAN_POINT ( 'NONE',  ( -15.45425417449318317, -5.113361153441934093, 34.14387501736622710 ) ) ;
#724=DIRECTION ( 'NONE',  ( -0.000000000000000000, 0.5000000000000011102, -0.8660254037844381525 ) ) ;
#725=CARTESIAN_POINT ( 'NONE',  ( 12.46153846153846168, -2.721908614388771852, 31.22303859784724978 ) ) ;
#726=LINE ( 'NONE', #39956, #60282 ) ;
#727=DIRECTION ( 'NONE',  ( -0.000000000000000000, -0.9848077530122085754, -0.1736481776669273613 ) ) ;
#730=AXIS2_PLACEMENT_3D ( 'NONE', #16205, #11228, #78786 ) ;
#731=CARTESIAN_POINT ( 'NONE',  ( -9.822454901745913958, -3.817052484675422797, 33.13202310037935661 ) ) ;
#732=CARTESIAN_POINT ( 'NONE',  ( -14.30769230769230660, -12.48256725967547354, 35.29906147534542527 ) ) ;
#733=EDGE_LOOP ( 'NONE', ( #34474, #45884, #50430, #8739 ) ) ;
#734=CARTESIAN_POINT ( 'NONE',  ( -18.00000000000012079, -6.879047030192663392, 34.71129190930017927 ) ) ;
#736=AXIS2_PLACEMENT_3D ( 'NONE', #62957, #67314, #32632 ) ;
#737=B_SPLINE_CURVE_WITH_KNOTS ( 'NONE', 3,
 ( #7790, #54628, #21744, #13218, #6896, #62715 ),
 .UNSPECIFIED., .F., .F.,
 ( 4, 2, 4 ),
 ( 0.0003909569690057828153, 0.0005862646681846093912, 0.0007815723673634359129 ),
 .UNSPECIFIED. ) ;
#738=CARTESIAN_POINT ( 'NONE',  ( -16.15384615384627409, -12.51329471203414379, 31.30864560766407578 ) ) ;
#739=CARTESIAN_POINT ( 'NONE',  ( -15.23076923076922995, -1.367168528481310208, 33.57946703557072254 ) ) ;
#740=ORIENTED_EDGE ( 'NONE', *, *, #36232, .T. ) ;
#741=CARTESIAN_POINT ( 'NONE',  ( 14.30769230769231015, -2.538708090699994813, 30.37095296980875503 ) ) ;
#742=CARTESIAN_POINT ( 'NONE',  ( 16.40379156322419973, -2.589246495874658827, 31.60778113518102828 ) ) ;
#743=CARTESIAN_POINT ( 'NONE',  ( 4.023155550735845409, -9.084618155246140248, 34.75535874321725771 ) ) ;
#744=ORIENTED_EDGE ( 'NONE', *, *, #2317, .F. ) ;
#745=CARTESIAN_POINT ( 'NONE',  ( -39.05038313613820122, -12.75000000000000178, 29.75000000000000355 ) ) ;
#746=AXIS2_PLACEMENT_3D ( 'NONE', #34224, #7204, #34678 ) ;
#747=CARTESIAN_POINT ( 'NONE',  ( 13.51540719244017374, -2.541949514083464479, 30.39797389878540557 ) ) ;
#748=FACE_OUTER_BOUND ( 'NONE', #30218, .T. ) ;
#749=CARTESIAN_POINT ( 'NONE',  ( 4.946231610255519051, -4.118384482072085184, 33.43331474514187107 ) ) ;
#750=EDGE_CURVE ( 'NONE', #66274, #83278, #76626, .T. ) ;
#751=CARTESIAN_POINT ( 'NONE',  ( 10.36540788444226102, -3.627789207965226748, 32.91389620160131102 ) ) ;
#752=ORIENTED_EDGE ( 'NONE', *, *, #194, .T. ) ;
#754=ORIENTED_EDGE ( 'NONE', *, *, #69554, .T. ) ;
#755=CARTESIAN_POINT ( 'NONE',  ( -9.561781990544128362, -3.285477652293413264, 32.44071101563363158 ) ) ;
#757=CARTESIAN_POINT ( 'NONE',  ( -2.307692307692428724, -6.835583212225970762, 34.95778746994575670 ) ) ;
#758=CARTESIAN_POINT ( 'NONE',  ( -6.923076923076922462, -10.51840700105979565, 33.73612834413961536 ) ) ;
#759=EDGE_CURVE ( 'NONE', #21493, #48689, #46710, .T. ) ;
#760=EDGE_CURVE ( 'NONE', #41806, #15172, #56192, .T. ) ;
#761=ORIENTED_EDGE ( 'NONE', *, *, #66448, .F. ) ;
#762=CARTESIAN_POINT ( 'NONE',  ( -17.20707028636129721, -4.460286881179643004, 33.72017969459903242 ) ) ;
#763=VERTEX_POINT ( 'NONE', #78492 ) ;
#764=ORIENTED_EDGE ( 'NONE', *, *, #17336, .F. ) ;
#765=VERTEX_POINT ( 'NONE', #50578 ) ;
#766=LINE ( 'NONE', #35889, #12781 ) ;
#767=EDGE_LOOP ( 'NONE', ( #7918, #41144, #11280, #63000 ) ) ;
#768=B_SPLINE_CURVE_WITH_KNOTS ( 'NONE', 3,
 ( #36697, #64149, #2452, #84894, #23180, #71354, #17764, #72247, #80360, #18658 ),
 .UNSPECIFIED., .F., .F.,
 ( 4, 2, 2, 2, 4 ),
 ( 0.000000000000000000, 0.0001954311564186861426, 0.0003908623128373722852, 0.0005862934692560583735, 0.0007817246256747445703 ),
 .UNSPECIFIED. ) ;
#769=LINE ( 'NONE', #20160, #80481 ) ;
#770=CARTESIAN_POINT ( 'NONE',  ( 6.065255139512839122, -2.657715359629131857, 31.77849191805844242 ) ) ;
#771=EDGE_CURVE ( 'NONE', #85264, #19690, #69198, .T. ) ;
#772=CARTESIAN_POINT ( 'NONE',  ( -3.230769230769351186, -4.481592998941358097, 33.73612834414048933 ) ) ;
#773=FACE_OUTER_BOUND ( 'NONE', #14188, .T. ) ;
#776=ORIENTED_EDGE ( 'NONE', *, *, #15608, .T. ) ;
#777=ORIENTED_EDGE ( 'NONE', *, *, #70790, .T. ) ;
#778=CARTESIAN_POINT ( 'NONE',  ( -6.673022503163469565, -2.920487667080175154, 32.31805714834170828 ) ) ;
#779=CARTESIAN_POINT ( 'NONE',  ( -2.307692307692427391, -2.892918686052166066, 31.69288490824153470 ) ) ;
#781=DIRECTION ( 'NONE',  ( -0.000000000000000000, -0.8660254037844397068, -0.4999999999999978906 ) ) ;
#782=VECTOR ( 'NONE', #87590, 1000.000000000000114 ) ;
#783=CARTESIAN_POINT ( 'NONE',  ( -2.307692307692305711, -4.945431358278436385, 36.03766855953609394 ) ) ;
#784=ORIENTED_EDGE ( 'NONE', *, *, #41224, .F. ) ;
#785=EDGE_CURVE ( 'NONE', #34790, #49709, #15373, .T. ) ;
#786=CARTESIAN_POINT ( 'NONE',  ( -18.00000000000012079, -5.941354392335914447, 34.76329471203413846 ) ) ;
#787=CARTESIAN_POINT ( 'NONE',  ( -39.05038313613820122, -2.249999999999998668, 29.75000000000000355 ) ) ;
#788=ORIENTED_EDGE ( 'NONE', *, *, #10295, .T. ) ;
#789=FACE_BOUND ( 'NONE', #47609, .T. ) ;
#790=CARTESIAN_POINT ( 'NONE',  ( -11.78843828251013015, -11.47974371597208076, 33.17467449705390692 ) ) ;
#791=B_SPLINE_CURVE_WITH_KNOTS ( 'NONE', 3,
 ( #20855, #88459, #592, #54189, #81685, #19966, #34810, #40701, #68163, #62277 ),
 .UNSPECIFIED., .F., .F.,
 ( 4, 2, 2, 2, 4 ),
 ( 0.0007817359430256315238, 0.0009771253907249980580, 0.001172514838424364592, 0.001367904286123730910, 0.001563293733823097444 ),
 .UNSPECIFIED. ) ;
#793=CARTESIAN_POINT ( 'NONE',  ( -9.692307692307691624, -10.67929555188718282, 33.92786785259544047 ) ) ;
#794=DIRECTION ( 'NONE',  ( -0.000000000000000000, 0.6427876096865404731, -0.7660444431189770143 ) ) ;
#795=CARTESIAN_POINT ( 'NONE',  ( 4.853996859406926490, -9.886141570436013382, 34.14413921362392301 ) ) ;
#796=CARTESIAN_POINT ( 'NONE',  ( -3.165514091256391271, -3.643525952247864463, 33.31231777344670064 ) ) ;
#797=CARTESIAN_POINT ( 'NONE',  ( -4.219928533206287469, -10.67929555188718460, 33.92786785259543336 ) ) ;
#798=VERTEX_POINT ( 'NONE', #3277 ) ;
#799=CARTESIAN_POINT ( 'NONE',  ( 14.53047184896071542, -12.44528174975671853, 30.48912976160716681 ) ) ;
#800=VECTOR ( 'NONE', #28708, 1000.000000000000114 ) ;
#802=ORIENTED_EDGE ( 'NONE', *, *, #42651, .F. ) ;
#803=CYLINDRICAL_SURFACE ( 'NONE', #41598, 0.2499999999999994726 ) ;
#804=CARTESIAN_POINT ( 'NONE',  ( -7.623374177175779032, -2.353885683473779800, 30.79025554430704403 ) ) ;
#805=EDGE_LOOP ( 'NONE', ( #48407, #3484, #58265, #43843 ) ) ;
#806=CYLINDRICAL_SURFACE ( 'NONE', #26995, 0.2499999999999994726 ) ;
#807=CARTESIAN_POINT ( 'NONE',  ( -10.61538461538461320, -1.790695186598648903, 34.54067556320373455 ) ) ;
#808=ADVANCED_FACE ( 'NONE', ( #44245 ), #41733, .F. ) ;
#809=FACE_BOUND ( 'NONE', #1125, .T. ) ;
#810=CYLINDRICAL_SURFACE ( 'NONE', #50418, 0.2500000000000009437 ) ;
#812=CARTESIAN_POINT ( 'NONE',  ( 3.480714749117371998, -8.433404298154334455, 34.66254593164985920 ) ) ;
#813=CARTESIAN_POINT ( 'NONE',  ( -16.15384615384627409, -2.625532179533778709, 30.86335684631627174 ) ) ;
#815=CARTESIAN_POINT ( 'NONE',  ( 6.989145274079363368, -12.37446782046654192, 30.86335684631486842 ) ) ;
#816=CARTESIAN_POINT ( 'NONE',  ( -2.307692307692305711, -2.538708090699994813, 30.37095296980875503 ) ) ;
#818=EDGE_LOOP ( 'NONE', ( #13516, #54259, #65486, #44692 ) ) ;
#819=EDGE_CURVE ( 'NONE', #85855, #5133, #61991, .T. ) ;
#820=VERTEX_POINT ( 'NONE', #30316 ) ;
#821=CARTESIAN_POINT ( 'NONE',  ( -9.692307692307691624, -2.292212530054420494, 30.41441678777542634 ) ) ;
#822=VECTOR ( 'NONE', #47003, 1000.000000000000000 ) ;
#824=CARTESIAN_POINT ( 'NONE',  ( 14.55774672760575861, -12.65882529074907126, 30.72640787790839312 ) ) ;
#825=CARTESIAN_POINT ( 'NONE',  ( 14.55763771707035303, -9.357781135181031829, 34.66075350412533851 ) ) ;
#826=CARTESIAN_POINT ( 'NONE',  ( 8.519230769230768274, -2.249999999999998668, 29.75000000000000355 ) ) ;
#827=CARTESIAN_POINT ( 'NONE',  ( -13.31936024510254590, -2.657715359629131857, 31.77849191805844242 ) ) ;
#829=CARTESIAN_POINT ( 'NONE',  ( 6.856994543716785628, -2.292212530054419606, 30.41441678777542634 ) ) ;
#830=CYLINDRICAL_SURFACE ( 'NONE', #73375, 0.2499999999999973355 ) ;
#831=VECTOR ( 'NONE', #8380, 999.9999999999998863 ) ;
#833=CARTESIAN_POINT ( 'NONE',  ( -0.4615384615384611200, -10.51840700105979565, 33.73612834413961536 ) ) ;
#835=LINE ( 'NONE', #62090, #39737 ) ;
#836=CARTESIAN_POINT ( 'NONE',  ( -9.757577692864012775, -12.70778746994557551, 30.41441678777548319 ) ) ;
#837=CARTESIAN_POINT ( 'NONE',  ( -14.05774678934416499, -3.202959910592335646, 32.30730279482227019 ) ) ;
#839=EDGE_CURVE ( 'NONE', #4529, #49069, #7942, .T. ) ;
#840=ORIENTED_EDGE ( 'NONE', *, *, #396, .T. ) ;
#842=CARTESIAN_POINT ( 'NONE',  ( -0.4615384615384611200, -3.886160181151819604, 36.00935417666054406 ) ) ;
#844=CARTESIAN_POINT ( 'NONE',  ( -5.749945580086545327, -12.41089969410671223, 31.60739465890703670 ) ) ;
#845=CARTESIAN_POINT ( 'NONE',  ( -11.53846153846165912, -4.481592998941358097, 33.73612834414048933 ) ) ;
#846=ORIENTED_EDGE ( 'NONE', *, *, #33882, .T. ) ;
#847=EDGE_CURVE ( 'NONE', #31771, #32696, #72861, .T. ) ;
#848=CARTESIAN_POINT ( 'NONE',  ( 10.61538461538492406, -2.506253911140615021, 30.00000000000323297 ) ) ;
#849=CARTESIAN_POINT ( 'NONE',  ( -1.161835843346973984, -4.387253974876678342, 33.66317474335728832 ) ) ;
#850=ORIENTED_EDGE ( 'NONE', *, *, #41234, .F. ) ;
#852=CARTESIAN_POINT ( 'NONE',  ( -9.442362282929648742, -5.766571408460171355, 34.70601412856602508 ) ) ;
#853=ORIENTED_EDGE ( 'NONE', *, *, #48241, .F. ) ;
#854=CARTESIAN_POINT ( 'NONE',  ( -13.25408968285182176, -2.619367082507849442, 30.83698974864643461 ) ) ;
#858=EDGE_CURVE ( 'NONE', #40515, #5216, #48469, .T. ) ;
#861=VERTEX_POINT ( 'NONE', #2824 ) ;
#862=ORIENTED_EDGE ( 'NONE', *, *, #13935, .F. ) ;
#863=CARTESIAN_POINT ( 'NONE',  ( -6.673131513698878692, -8.476813868363244353, 34.90874843262270133 ) ) ;
#864=EDGE_CURVE ( 'NONE', #87613, #38306, #6742, .T. ) ;
#865=ORIENTED_EDGE ( 'NONE', *, *, #66693, .F. ) ;
#867=CARTESIAN_POINT ( 'NONE',  ( 4.153846153846032507, -6.879047030192662504, 34.71129190930017927 ) ) ;
#868=CARTESIAN_POINT ( 'NONE',  ( -7.173100147298380413, -2.341070481393820124, 30.72580821765574299 ) ) ;
#869=CARTESIAN_POINT ( 'NONE',  ( -5.869209559033048862, -5.496552790871117367, 34.60292014791297532 ) ) ;
#870=DIRECTION ( 'NONE',  ( -0.000000000000000000, -0.1736481776669307198, -0.9848077530122080203 ) ) ;
#871=CARTESIAN_POINT ( 'NONE',  ( 8.769230769230768274, -13.75783147151868846, 33.36296068462461051 ) ) ;
#872=B_SPLINE_CURVE_WITH_KNOTS ( 'NONE', 3,
 ( #45408, #38215, #52164, #73342, #87320, #11646, #25597, #32799, #79654, #17954 ),
 .UNSPECIFIED., .F., .F.,
 ( 4, 2, 2, 2, 4 ),
 ( 0.0007817246256747469556, 0.0009771112852218896347, 0.001172497944769032531, 0.001367884604316175427, 0.001563271263863318106 ),
 .UNSPECIFIED. ) ;
#873=CARTESIAN_POINT ( 'NONE',  ( 0.6845015958051353655, -7.369474539155827841, 34.99858011523955525 ) ) ;
#874=EDGE_CURVE ( 'NONE', #18726, #10877, #86197, .T. ) ;
#875=CARTESIAN_POINT ( 'NONE',  ( 3.165499230212911019, -10.33852847137145048, 34.16647553114627556 ) ) ;
#877=ORIENTED_EDGE ( 'NONE', *, *, #70211, .T. ) ;
#878=CARTESIAN_POINT ( 'NONE',  ( 4.153846153846154188, -8.164416787775445883, 34.95778746994557906 ) ) ;
#879=VERTEX_POINT ( 'NONE', #51895 ) ;
#880=CARTESIAN_POINT ( 'NONE',  ( 7.780071466793709867, -2.486705287966279432, 31.30864560766542937 ) ) ;
#881=ORIENTED_EDGE ( 'NONE', *, *, #4862, .F. ) ;
#883=CARTESIAN_POINT ( 'NONE',  ( -4.153846153846152411, -7.500000000000001776, 35.04278698407183867 ) ) ;
#884=CARTESIAN_POINT ( 'NONE',  ( 6.700149964170072359, -9.172386477786396597, 34.72672124145550043 ) ) ;
#886=EDGE_CURVE ( 'NONE', #67642, #25620, #63682, .T. ) ;
#887=DIRECTION ( 'NONE',  ( 0.000000000000000000, 0.3420201433256641055, -0.9396926207859100932 ) ) ;
#888=VECTOR ( 'NONE', #63429, 1000.000000000000000 ) ;
#889=ORIENTED_EDGE ( 'NONE', *, *, #12602, .F. ) ;
#890=CARTESIAN_POINT ( 'NONE',  ( -16.40386939113911779, -3.711651800289232916, 33.01384336483936011 ) ) ;
#891=ORIENTED_EDGE ( 'NONE', *, *, #87975, .T. ) ;
#892=DIRECTION ( 'NONE',  ( 0.000000000000000000, -6.938893903907222067E-15, 1.000000000000000000 ) ) ;
#893=EDGE_LOOP ( 'NONE', ( #12164, #44683, #39104, #42360 ) ) ;
#894=CARTESIAN_POINT ( 'NONE',  ( 14.98074600654777377, -2.341070481393819236, 30.72580821765574299 ) ) ;
#895=CARTESIAN_POINT ( 'NONE',  ( -4.403869378067608586, -6.652501968072646932, 34.93155406624980941 ) ) ;
#896=FACE_BOUND ( 'NONE', #56374, .T. ) ;
#897=B_SPLINE_CURVE_WITH_KNOTS ( 'NONE', 3,
 ( #11961, #39439, #33563, #60574, #74102, #68664, #12395, #60128, #5634, #88091 ),
 .UNSPECIFIED., .F., .F.,
 ( 4, 2, 2, 2, 4 ),
 ( 0.0007817359430256319575, 0.0009771253907249984917, 0.001172514838424365026, 0.001367904286123731343, 0.001563293733823097878 ),
 .UNSPECIFIED. ) ;
#898=CYLINDRICAL_SURFACE ( 'NONE', #57135, 0.2499999999999993616 ) ;
#899=DIRECTION ( 'NONE',  ( -0.000000000000000000, -0.8660254037844399289, -0.4999999999999980016 ) ) ;
#900=CARTESIAN_POINT ( 'NONE',  ( 4.153846153846032507, -12.46129190930018460, 30.37095296980731973 ) ) ;
#901=B_SPLINE_CURVE_WITH_KNOTS ( 'NONE', 3,
 ( #47578, #67414, #60646, #88158, #38609, #59318, #86825, #25091, #49794, #1167 ),
 .UNSPECIFIED., .F., .F.,
 ( 4, 2, 2, 2, 4 ),
 ( 0.0007817359430256390048, 0.0009771253907250075990, 0.001172514838424376085, 0.001367904286123744571, 0.001563293733823113056 ),
 .UNSPECIFIED. ) ;
#902=CARTESIAN_POINT ( 'NONE',  ( 0.7115384615384748868, -2.249999999999999112, 29.81603969181031033 ) ) ;
#903=CARTESIAN_POINT ( 'NONE',  ( -17.14300545628321260, -8.164416787775445883, 34.95778746994557906 ) ) ;
#904=DIRECTION ( 'NONE',  ( -0.000000000000000000, 0.5000000000000011102, -0.8660254037844380415 ) ) ;
#905=EDGE_LOOP ( 'NONE', ( #32769, #30107, #48312, #37232 ) ) ;
#906=CARTESIAN_POINT ( 'NONE',  ( -14.17716660592874334, -3.816742781228458004, 33.13167719472716044 ) ) ;
#907=ORIENTED_EDGE ( 'NONE', *, *, #15104, .T. ) ;
#908=ORIENTED_EDGE ( 'NONE', *, *, #77155, .T. ) ;
#910=DIRECTION ( 'NONE',  ( 0.000000000000000000, 0.4999999999999960032, -0.8660254037844410391 ) ) ;
#911=LINE ( 'NONE', #28379, #24043 ) ;
#912=CARTESIAN_POINT ( 'NONE',  ( -16.94613263595612906, -9.929761469519743144, 34.40412654351204225 ) ) ;
#914=CARTESIAN_POINT ( 'NONE',  ( -12.21148404162500967, -4.818054556918156983, 34.26375889529406749 ) ) ;
#915=ORIENTED_EDGE ( 'NONE', *, *, #33523, .T. ) ;
#916=AXIS2_PLACEMENT_3D ( 'NONE', #41610, #74963, #69079 ) ;
#917=CYLINDRICAL_SURFACE ( 'NONE', #15586, 0.2500000000000002220 ) ;
#918=CARTESIAN_POINT ( 'NONE',  ( 3.230769230769231726, -11.16473453929635440, 33.15142922261926373 ) ) ;
#919=CARTESIAN_POINT ( 'NONE',  ( 16.82689985270161870, -4.175268141568689195, 33.81360843649122216 ) ) ;
#920=DIRECTION ( 'NONE',  ( -0.000000000000000000, 0.6427876096865404731, -0.7660444431189770143 ) ) ;
#921=DIRECTION ( 'NONE',  ( 0.000000000000000000, 0.3420201433256641055, -0.9396926207859100932 ) ) ;
#922=VERTEX_POINT ( 'NONE', #31648 ) ;
#924=ORIENTED_EDGE ( 'NONE', *, *, #46404, .T. ) ;
#925=EDGE_CURVE ( 'NONE', #39506, #47746, #87062, .T. ) ;
#926=ORIENTED_EDGE ( 'NONE', *, *, #25814, .T. ) ;
#927=CARTESIAN_POINT ( 'NONE',  ( -6.989160334032802346, -8.120952969808774569, 34.71129190930000163 ) ) ;
#928=ADVANCED_FACE ( 'NONE', ( #44697 ), #65861, .F. ) ;
#929=ORIENTED_EDGE ( 'NONE', *, *, #6810, .F. ) ;
#930=CARTESIAN_POINT ( 'NONE',  ( -6.923076923076922462, -4.786620604624113540, 33.94971097300155094 ) ) ;
#931=CARTESIAN_POINT ( 'NONE',  ( -11.53846153846153655, -2.249999999999998668, 29.75000000000001776 ) ) ;
#932=DIRECTION ( 'NONE',  ( -0.000000000000000000, 0.9396926207859093161, -0.3420201433256662704 ) ) ;
#934=CARTESIAN_POINT ( 'NONE',  ( 9.823099500132483897, -5.582136614379148654, 34.36778462344220486 ) ) ;
#935=ORIENTED_EDGE ( 'NONE', *, *, #44196, .T. ) ;
#936=EDGE_CURVE ( 'NONE', #4757, #82729, #32582, .T. ) ;
#937=CARTESIAN_POINT ( 'NONE',  ( 4.377221639618572802, -2.251407671071270489, 29.88021292934942252 ) ) ;
#941=CARTESIAN_POINT ( 'NONE',  ( 3.100077764101673239, -12.38065189839062263, 30.83690757178629482 ) ) ;
#942=CARTESIAN_POINT ( 'NONE',  ( 16.82689983963011926, -3.711651800289232916, 33.01384336483936011 ) ) ;
#943=CARTESIAN_POINT ( 'NONE',  ( -2.557715531913763218, -12.68155406624981119, 30.59749803192733708 ) ) ;
#944=CARTESIAN_POINT ( 'NONE',  ( -9.692307692307691624, -12.34228464037088635, 31.77849191805839268 ) ) ;
#945=CARTESIAN_POINT ( 'NONE',  ( -3.453696189676077832, -10.77366814457252175, 33.85459836347579454 ) ) ;
#946=FACE_OUTER_BOUND ( 'NONE', #27174, .T. ) ;
#947=ADVANCED_FACE ( 'NONE', ( #86160 ), #59111, .F. ) ;
#950=CARTESIAN_POINT ( 'NONE',  ( -4.826923076923015365, -7.434744860731433924, 35.00000000000000711 ) ) ;
#951=CARTESIAN_POINT ( 'NONE',  ( -1.319360245102545681, -3.643525952247864463, 33.31231777344670064 ) ) ;
#952=CARTESIAN_POINT ( 'NONE',  ( 8.096099364501988305, -2.587454068350147907, 30.68340429815432202 ) ) ;
#953=VECTOR ( 'NONE', #29326, 1000.000000000000114 ) ;
#954=CARTESIAN_POINT ( 'NONE',  ( -7.780898706641007578, -3.083524468853784839, 32.58852847137153930 ) ) ;
#957=CARTESIAN_POINT ( 'NONE',  ( -3.230769230769229949, -10.51840700105979565, 33.73612834413961536 ) ) ;
#958=B_SPLINE_CURVE_WITH_KNOTS ( 'NONE', 3,
 ( #11696, #32846, #18003, #72041, #52661, #10351, #45458, #65284, #31508, #26090 ),
 .UNSPECIFIED., .F., .F.,
 ( 4, 2, 2, 2, 4 ),
 ( 0.000000000000000000, 0.0001954339857564078809, 0.0003908679715128157619, 0.0005863019572692236428, 0.0007817359430256315238 ),
 .UNSPECIFIED. ) ;
#960=CARTESIAN_POINT ( 'NONE',  ( 8.769230769230768274, -13.37000171582298513, 34.34916445242398453 ) ) ;
#961=DIRECTION ( 'NONE',  ( 0.000000000000000000, 0.9396926207859126468, -0.3420201433256571111 ) ) ;
#962=ORIENTED_EDGE ( 'NONE', *, *, #41239, .F. ) ;
#963=PRODUCT ( 'Ultra-Thin Hypoallergenic Micro-Foil Screen', 'Ultra-Thin Hypoallergenic Micro-Foil Screen', '', ( #87462 ) ) ;
#964=DIRECTION ( 'NONE',  ( -0.000000000000000000, 1.000000000000000000, 3.491481338843133355E-15 ) ) ;
#966=CARTESIAN_POINT ( 'NONE',  ( 7.846153846153725020, -6.026961402154118019, 34.52809138561165270 ) ) ;
#967=LINE ( 'NONE', #54571, #72315 ) ;
#968=ORIENTED_EDGE ( 'NONE', *, *, #4573, .F. ) ;
#969=CARTESIAN_POINT ( 'NONE',  ( -6.673022503163470454, -6.523592122091591783, 34.90882529074906415 ) ) ;
#970=EDGE_CURVE ( 'NONE', #1945, #59177, #85244, .T. ) ;
#971=EDGE_LOOP ( 'NONE', ( #65571, #72867 ) ) ;
#973=CARTESIAN_POINT ( 'NONE',  ( -3.930883250284669117, -7.369474270740069777, 34.74850911626239736 ) ) ;
#974=ORIENTED_EDGE ( 'NONE', *, *, #27473, .F. ) ;
#975=CARTESIAN_POINT ( 'NONE',  ( -17.77722033102192967, -10.23759521482555535, 34.22997729860117033 ) ) ;
#977=CARTESIAN_POINT ( 'NONE',  ( -11.66860874789976066, -6.852621066184266141, 34.70813303252209181 ) ) ;
#978=ADVANCED_FACE ( 'NONE', ( #52797 ), #80287, .F. ) ;
#979=B_SPLINE_CURVE_WITH_KNOTS ( 'NONE', 3,
 ( #36155, #56847, #63605, #84343, #22618, #70821, #15880, #43342, #64040, #2337 ),
 .UNSPECIFIED., .F., .F.,
 ( 4, 2, 2, 2, 4 ),
 ( 0.0007817359430256369448, 0.0009771253907250049969, 0.001172514838424373049, 0.001367904286123741101, 0.001563293733823109153 ),
 .UNSPECIFIED. ) ;
#980=DIRECTION ( 'NONE',  ( -0.000000000000000000, 0.6427876096865404731, -0.7660444431189770143 ) ) ;
#982=B_SPLINE_CURVE_WITH_KNOTS ( 'NONE', 3,
 ( #17469, #52571, #25998, #19248, #5727, #12489, #26450, #59334, #38175, #3935 ),
 .UNSPECIFIED., .F., .F.,
 ( 4, 2, 2, 2, 4 ),
 ( 0.0007817246256747445703, 0.0009771112852218872494, 0.001172497944769030145, 0.001367884604316172825, 0.001563271263863315504 ),
 .UNSPECIFIED. ) ;
#983=VECTOR ( 'NONE', #76955, 1000.000000000000114 ) ;
#986=EDGE_CURVE ( 'NONE', #67360, #34311, #25781, .T. ) ;
#988=FACE_BOUND ( 'NONE', #42867, .T. ) ;
#989=EDGE_LOOP ( 'NONE', ( #83458, #29915 ) ) ;
#990=DIRECTION ( 'NONE',  ( -0.000000000000000000, 0.8660254037844397068, -0.4999999999999978906 ) ) ;
#991=CARTESIAN_POINT ( 'NONE',  ( 4.403791672194296680, -11.86320923018887541, 32.19269448109604781 ) ) ;
#994=CARTESIAN_POINT ( 'NONE',  ( -16.15384615384615330, -2.708943851104267164, 35.45975837776705220 ) ) ;
#995=EDGE_CURVE ( 'NONE', #22351, #45196, #30345, .T. ) ;
#996=ORIENTED_EDGE ( 'NONE', *, *, #82380, .F. ) ;
#997=EDGE_LOOP ( 'NONE', ( #81985, #73221, #79489, #65801 ) ) ;
#998=VERTEX_POINT ( 'NONE', #41961 ) ;
#999=CYLINDRICAL_SURFACE ( 'NONE', #7439, 0.2499999999999998890 ) ;
#1000=ADVANCED_FACE ( 'NONE', ( #68534 ), #20790, .F. ) ;
#1001=EDGE_CURVE ( 'NONE', #61364, #13048, #34667, .T. ) ;
#1002=VERTEX_POINT ( 'NONE', #13154 ) ;
#1003=DIRECTION ( 'NONE',  ( -0.000000000000000000, 0.3420201433256694901, -0.9396926207859082059 ) ) ;
#1004=CARTESIAN_POINT ( 'NONE',  ( -11.78848476268299628, -5.765609946408404518, 34.70566812827425451 ) ) ;
#1005=EDGE_CURVE ( 'NONE', #29769, #31113, #19901, .T. ) ;
#1007=DIRECTION ( 'NONE',  ( -0.000000000000000000, 0.8660254037844399289, -0.4999999999999980016 ) ) ;
#1008=CARTESIAN_POINT ( 'NONE',  ( -15.23076923076935252, -3.643525952248795718, 33.31231777344771672 ) ) ;
#1009=CARTESIAN_POINT ( 'NONE',  ( 2.307692307692309264, -2.249999999999998668, 29.75000000000001776 ) ) ;
#1010=CARTESIAN_POINT ( 'NONE',  ( 11.66925334628632527, -8.147973898785416225, 34.70805048591653730 ) ) ;
#1011=ORIENTED_EDGE ( 'NONE', *, *, #79161, .T. ) ;
#1013=EDGE_LOOP ( 'NONE', ( #6290, #11618, #80010, #73134 ) ) ;
#1014=DIRECTION ( 'NONE',  ( -0.000000000000000000, -0.1736481776669307198, -0.9848077530122080203 ) ) ;
#1015=CARTESIAN_POINT ( 'NONE',  ( -3.007989561791163613, -10.23759521482555357, 34.22997729860117033 ) ) ;
#1016=CARTESIAN_POINT ( 'NONE',  ( 10.68064018666064285, -6.879047030191282275, 34.71129190930002295 ) ) ;
#1017=CARTESIAN_POINT ( 'NONE',  ( -18.00000000000000000, -5.471508081941599322, 34.59228464037088457 ) ) ;
#1018=CARTESIAN_POINT ( 'NONE',  ( -3.360916440207448286, -11.47017969459903952, 32.78971311882034456 ) ) ;
#1019=FACE_BOUND ( 'NONE', #24352, .T. ) ;
#1020=CARTESIAN_POINT ( 'NONE',  ( 8.545745844666436497, -10.97335522853832579, 33.68706563782419749 ) ) ;
#1021=ORIENTED_EDGE ( 'NONE', *, *, #63505, .T. ) ;
#1022=CARTESIAN_POINT ( 'NONE',  ( 17.07692307692295586, -10.90142922262034020, 33.41473453929536674 ) ) ;
#1025=LINE ( 'NONE', #61828, #73513 ) ;
#1026=CARTESIAN_POINT ( 'NONE',  ( 3.361559671736183752, -11.37503395064541678, 33.29242100308974983 ) ) ;
#1027=ORIENTED_EDGE ( 'NONE', *, *, #76304, .F. ) ;
#1028=CARTESIAN_POINT ( 'NONE',  ( 6.223012844093395834, -10.77377354290276301, 33.85451476688484718 ) ) ;
#1030=FACE_BOUND ( 'NONE', #47160, .T. ) ;
#1032=DIRECTION ( 'NONE',  ( -0.000000000000000000, -0.7660444431189791237, -0.6427876096865379196 ) ) ;
#1033=DIRECTION ( 'NONE',  ( -0.000000000000000000, -0.1736481776669307198, -0.9848077530122080203 ) ) ;
#1034=CARTESIAN_POINT ( 'NONE',  ( -3.099977422944443894, -8.147973898785416225, 34.70805048591653730 ) ) ;
#1035=ORIENTED_EDGE ( 'NONE', *, *, #39496, .T. ) ;
#1037=CARTESIAN_POINT ( 'NONE',  ( -5.749945580086545327, -9.233818618650603938, 34.70587769442853698 ) ) ;
#1038=CARTESIAN_POINT ( 'NONE',  ( -9.692307692307691624, -3.050289026998446396, 32.03036669348365706 ) ) ;
#1039=CARTESIAN_POINT ( 'NONE',  ( -4.826977667545033768, -5.766571408460171355, 34.70601412856602508 ) ) ;
#1040=EDGE_LOOP ( 'NONE', ( #39631, #21106 ) ) ;
#1041=B_SPLINE_CURVE_WITH_KNOTS ( 'NONE', 3,
 ( #44749, #72230, #85313, #10539, #65477, #59160, #51950, #86215, #86667, #24931 ),
 .UNSPECIFIED., .F., .F.,
 ( 4, 2, 2, 2, 4 ),
 ( 0.000000000000000000, 0.0001954311564186863323, 0.0003908623128373726646, 0.0005862934692560590241, 0.0007817246256747453293 ),
 .UNSPECIFIED. ) ;
#1042=CARTESIAN_POINT ( 'NONE',  ( 16.40379167219429490, -10.76462480002816413, 33.53768742498949962 ) ) ;
#1043=ORIENTED_EDGE ( 'NONE', *, *, #60668, .F. ) ;
#1044=ADVANCED_FACE ( 'NONE', ( #6406 ), #74411, .F. ) ;
#1045=CARTESIAN_POINT ( 'NONE',  ( -7.846153846153844924, -13.20930481340135110, 34.54067556320372745 ) ) ;
#1046=VERTEX_POINT ( 'NONE', #41070 ) ;
#1047=CARTESIAN_POINT ( 'NONE',  ( 7.715462379486291766, -10.54014554554150607, 33.71984207302941883 ) ) ;
#1048=CARTESIAN_POINT ( 'NONE',  ( -6.700297381808511865, -11.89424750095246175, 32.13594075562311758 ) ) ;
#1049=DIRECTION ( 'NONE',  ( -0.000000000000000000, 1.000000000000000000, 3.491481338843133355E-15 ) ) ;
#1052=CARTESIAN_POINT ( 'NONE',  ( 9.692307692307572609, -9.442884908241554243, 34.35708131394783038 ) ) ;
#1053=CARTESIAN_POINT ( 'NONE',  ( -5.869209559033047974, -6.369690395747422684, 34.87708834333098196 ) ) ;
#1054=CARTESIAN_POINT ( 'NONE',  ( 16.40390046548447245, -5.728107161865375829, 34.42597550085002922 ) ) ;
#1055=CARTESIAN_POINT ( 'NONE',  ( 14.08476609017615644, -3.586966769969701208, 32.86292498521069660 ) ) ;
#1058=CARTESIAN_POINT ( 'NONE',  ( 14.55769230769231015, -2.499999999999998668, 29.75000000000000355 ) ) ;
#1059=ORIENTED_EDGE ( 'NONE', *, *, #26331, .T. ) ;
#1061=DIRECTION ( 'NONE',  ( 1.000000000000000000, -0.000000000000000000, -0.000000000000000000 ) ) ;
#1062=VECTOR ( 'NONE', #67531, 1000.000000000000000 ) ;
#1063=ORIENTED_EDGE ( 'NONE', *, *, #7601, .F. ) ;
#1064=DIRECTION ( 'NONE',  ( -0.000000000000000000, 0.9848077530122085754, -0.1736481776669273613 ) ) ;
#1065=LINE ( 'NONE', #41612, #19384 ) ;
#1066=DIRECTION ( 'NONE',  ( -0.000000000000000000, 0.5000000000000011102, -0.8660254037844381525 ) ) ;
#1067=CARTESIAN_POINT ( 'NONE',  ( -7.146561847641254239, -9.417330523894424488, 34.63758898049880486 ) ) ;
#1068=CYLINDRICAL_SURFACE ( 'NONE', #27243, 0.2499999999999995559 ) ;
#1069=CARTESIAN_POINT ( 'NONE',  ( -16.37733109757010652, -3.236172620538810385, 32.36188796281389557 ) ) ;
#1070=EDGE_CURVE ( 'NONE', #51469, #4867, #82066, .T. ) ;
#1071=CARTESIAN_POINT ( 'NONE',  ( 15.90382291655318880, -11.86270091957321071, 32.19358267280088626 ) ) ;
#1073=DIRECTION ( 'NONE',  ( 0.000000000000000000, 0.9848077530122072432, -0.1736481776669354937 ) ) ;
#1074=LINE ( 'NONE', #83501, #7513 ) ;
#1075=CARTESIAN_POINT ( 'NONE',  ( 14.37288628947566593, -2.506253911140448043, 29.99999999999988631 ) ) ;
#1076=DIRECTION ( 'NONE',  ( -0.000000000000000000, 0.6427876096865404731, -0.7660444431189771253 ) ) ;
#1077=ORIENTED_EDGE ( 'NONE', *, *, #57096, .F. ) ;
#1078=EDGE_LOOP ( 'NONE', ( #31275, #76014, #59362, #29560 ) ) ;
#1079=AXIS2_PLACEMENT_3D ( 'NONE', #20945, #39913, #48415 ) ;
#1080=CARTESIAN_POINT ( 'NONE',  ( -15.00798968950081758, -8.496831190052096971, 34.64984203495476578 ) ) ;
#1081=CARTESIAN_POINT ( 'NONE',  ( -15.90384615384615330, -2.249999999999998668, 29.75000000000000355 ) ) ;
#1083=CARTESIAN_POINT ( 'NONE',  ( 9.942253101685738059, -12.07971442181322352, 32.31769673815850297 ) ) ;
#1085=ADVANCED_FACE ( 'NONE', ( #26664 ), #48258, .F. ) ;
#1087=CARTESIAN_POINT ( 'NONE',  ( 9.915087361285756629, -11.60474049983371003, 33.02348890104160262 ) ) ;
#1088=DIRECTION ( 'NONE',  ( -0.000000000000000000, 0.8660254037844399289, -0.4999999999999980016 ) ) ;
#1089=CARTESIAN_POINT ( 'NONE',  ( -3.230769230769351186, -12.27809138561165270, 31.22303859784587132 ) ) ;
#1090=EDGE_CURVE ( 'NONE', #14619, #43616, #79819, .T. ) ;
#1091=AXIS2_PLACEMENT_3D ( 'NONE', #46818, #39638, #67988 ) ;
#1093=CARTESIAN_POINT ( 'NONE',  ( -13.38461538461550582, -10.21337939537710326, 33.94971097300076224 ) ) ;
#1094=ORIENTED_EDGE ( 'NONE', *, *, #49611, .F. ) ;
#1095=CARTESIAN_POINT ( 'NONE',  ( 0.4615384615384611200, -10.51840700105979565, 33.73612834413961536 ) ) ;
#1096=CARTESIAN_POINT ( 'NONE',  ( -18.00000000000000711, -12.74702886152665471, 29.99985851721553587 ) ) ;
#1097=CARTESIAN_POINT ( 'NONE',  ( 12.33139125210024112, -8.587444163452046197, 34.63053765926554206 ) ) ;
#1099=FACE_OUTER_BOUND ( 'NONE', #19965, .T. ) ;
#1100=EDGE_LOOP ( 'NONE', ( #57674, #76067 ) ) ;
#1101=ORIENTED_EDGE ( 'NONE', *, *, #72965, .F. ) ;
#1102=AXIS2_PLACEMENT_3D ( 'NONE', #32167, #59628, #87129 ) ;
#1104=VERTEX_POINT ( 'NONE', #49597 ) ;
#1105=ORIENTED_EDGE ( 'NONE', *, *, #51314, .T. ) ;
#1106=CARTESIAN_POINT ( 'NONE',  ( 13.38461538461526601, -3.300289026999228881, 32.46337939537708905 ) ) ;
#1107=CARTESIAN_POINT ( 'NONE',  ( -2.557669051740897537, -10.06842814019191401, 34.32929386961144758 ) ) ;
#1109=B_SPLINE_CURVE_WITH_KNOTS ( 'NONE', 3,
 ( #52985, #73735, #66520, #39503, #66964, #69615, #42162, #89028, #47567, #20105 ),
 .UNSPECIFIED., .F., .F.,
 ( 4, 2, 2, 2, 4 ),
 ( 0.0007817359430256326080, 0.0009771253907250047801, 0.001172514838424369796, 0.001367904286123735030, 0.001563293733823100263 ),
 .UNSPECIFIED. ) ;
#1110=CARTESIAN_POINT ( 'NONE',  ( -4.376773112753000738, -12.38737895849757820, 31.66785238281580206 ) ) ;
#1111=CARTESIAN_POINT ( 'NONE',  ( -2.084679463598911209, -11.43677907613345113, 33.22367315496201456 ) ) ;
#1112=CARTESIAN_POINT ( 'NONE',  ( -7.596208436775802930, -4.176053281294515251, 33.81426240980091791 ) ) ;
#1113=CARTESIAN_POINT ( 'NONE',  ( 6.923076923076924238, -10.67929555188718282, 33.92786785259544047 ) ) ;
#1114=AXIS2_PLACEMENT_3D ( 'NONE', #36527, #65751, #65313 ) ;
#1115=EDGE_LOOP ( 'NONE', ( #10565, #19181, #33919, #82141 ) ) ;
#1116=ORIENTED_EDGE ( 'NONE', *, *, #74661, .T. ) ;
#1118=CARTESIAN_POINT ( 'NONE',  ( 3.930919936330007136, -2.758268499246657957, 31.33685645148949561 ) ) ;
#1119=ORIENTED_EDGE ( 'NONE', *, *, #83593, .T. ) ;
#1120=CARTESIAN_POINT ( 'NONE',  ( -17.01085472592063752, -8.973038597847269315, 34.52809138561122637 ) ) ;
#1121=CARTESIAN_POINT ( 'NONE',  ( 13.63466980452883881, -4.074993327901527351, 33.72946981652012255 ) ) ;
#1122=CARTESIAN_POINT ( 'NONE',  ( -17.07692307692307665, -12.37446782046654192, 30.86335684631486131 ) ) ;
#1123=CARTESIAN_POINT ( 'NONE',  ( 13.45068373561782593, -8.120952969808772792, 34.71129190929999453 ) ) ;
#1124=ORIENTED_EDGE ( 'NONE', *, *, #12894, .T. ) ;
#1125=EDGE_LOOP ( 'NONE', ( #67403, #51145 ) ) ;
#1126=DIRECTION ( 'NONE',  ( -0.000000000000000000, 1.000000000000000000, 3.491481338843133355E-15 ) ) ;
#1127=EDGE_LOOP ( 'NONE', ( #66624, #58900 ) ) ;
#1128=FACE_BOUND ( 'NONE', #14400, .T. ) ;
#1129=CARTESIAN_POINT ( 'NONE',  ( -1.384615384615076605, -2.506253911140615021, 30.00000000000323297 ) ) ;
#1130=AXIS2_PLACEMENT_3D ( 'NONE', #6250, #89121, #33712 ) ;
#1131=CARTESIAN_POINT ( 'NONE',  ( 7.846153846153723244, -5.941354392335915335, 34.76329471203413846 ) ) ;
#1132=ORIENTED_EDGE ( 'NONE', *, *, #59762, .F. ) ;
#1134=DIRECTION ( 'NONE',  ( -0.000000000000000000, 1.000000000000000000, 3.491481338843133355E-15 ) ) ;
#1135=LINE ( 'NONE', #35819, #16238 ) ;
#1136=CARTESIAN_POINT ( 'NONE',  ( 4.153846153846154188, -11.16473453929635440, 33.15142922261926373 ) ) ;
#1137=CARTESIAN_POINT ( 'NONE',  ( 4.284371855609720114, -3.285477652293412820, 32.44071101563363158 ) ) ;
#1138=ORIENTED_EDGE ( 'NONE', *, *, #84705, .T. ) ;
#1139=VECTOR ( 'NONE', #24290, 1000.000000000000000 ) ;
#1140=CARTESIAN_POINT ( 'NONE',  ( 6.130525701763564150, -8.586989748646452369, 34.63063291749215011 ) ) ;
#1141=CARTESIAN_POINT ( 'NONE',  ( -6.923076923076922462, -9.780366693483667717, 34.19971097300155094 ) ) ;
#1142=CARTESIAN_POINT ( 'NONE',  ( -0.4615384615384611200, -1.790695186598648903, 34.54067556320373455 ) ) ;
#1143=CARTESIAN_POINT ( 'NONE',  ( -0.7115152055870532788, -4.818429247618089661, 34.26397095200675125 ) ) ;
#1144=CARTESIAN_POINT ( 'NONE',  ( -15.23076923076935074, -11.94971097300221174, 32.03036669348237098 ) ) ;
#1145=FACE_BOUND ( 'NONE', #3062, .T. ) ;
#1146=CARTESIAN_POINT ( 'NONE',  ( 13.25392391794783009, -11.71456829005830080, 32.44064028649416542 ) ) ;
#1147=CARTESIAN_POINT ( 'NONE',  ( 17.07692307692295586, -3.083524468854526912, 32.58852847137268327 ) ) ;
#1149=CARTESIAN_POINT ( 'NONE',  ( -7.173100160369889622, -12.22074536777954989, 31.39888409691088356 ) ) ;
#1150=CARTESIAN_POINT ( 'NONE',  ( -11.28840722682322628, -11.28795663066794575, 33.01431243580653785 ) ) ;
#1151=CARTESIAN_POINT ( 'NONE',  ( -18.22348492456433178, -3.019605429927188833, 32.48692288466676104 ) ) ;
#1152=CARTESIAN_POINT ( 'NONE',  ( -18.22292621751614305, -9.886141570436018711, 34.14413921362392301 ) ) ;
#1154=ORIENTED_EDGE ( 'NONE', *, *, #4618, .F. ) ;
#1155=CARTESIAN_POINT ( 'NONE',  ( 12.46153846153846168, -2.538708090699994813, 30.37095296980875503 ) ) ;
#1156=ORIENTED_EDGE ( 'NONE', *, *, #36963, .F. ) ;
#1157=CARTESIAN_POINT ( 'NONE',  ( 8.769230769230647482, -6.026961402154118019, 34.52809138561165270 ) ) ;
#1158=VERTEX_POINT ( 'NONE', #56355 ) ;
#1159=CARTESIAN_POINT ( 'NONE',  ( -11.47239318745909920, -2.721908614388772296, 31.22303859784725333 ) ) ;
#1160=CARTESIAN_POINT ( 'NONE',  ( -18.22292621751614305, -2.554751324335734264, 30.48935550225260727 ) ) ;
#1161=VERTEX_POINT ( 'NONE', #83844 ) ;
#1162=CARTESIAN_POINT ( 'NONE',  ( -15.36146069743678844, -4.809359713505814149, 33.96456829005828837 ) ) ;
#1164=CARTESIAN_POINT ( 'NONE',  ( 2.307692307692186251, -5.941354392335915335, 34.76329471203413846 ) ) ;
#1165=CARTESIAN_POINT ( 'NONE',  ( -15.23076923076935252, -9.528491918059723176, 34.59228464037033035 ) ) ;
#1166=CARTESIAN_POINT ( 'NONE',  ( 16.02369818411445834, -8.630895178749536711, 34.87696386517710323 ) ) ;
#1167=CARTESIAN_POINT ( 'NONE',  ( 7.846153846153846700, -11.69971097300155272, 32.46337939537588113 ) ) ;
#1168=CARTESIAN_POINT ( 'NONE',  ( 11.31497659473759398, -2.847400154188068022, 31.58180166144859058 ) ) ;
#1169=DIRECTION ( 'NONE',  ( -0.000000000000000000, 0.3420201433256694901, -0.9396926207859082059 ) ) ;
#1171=CARTESIAN_POINT ( 'NONE',  ( -3.230769230769229949, -9.819645486525091727, 36.12317359536749706 ) ) ;
#1172=CARTESIAN_POINT ( 'NONE',  ( -11.53846153846165912, -11.94971097300221174, 32.03036669348237098 ) ) ;
#1173=LINE ( 'NONE', #61539, #40183 ) ;
#1175=EDGE_CURVE ( 'NONE', #60227, #41430, #46471, .T. ) ;
#1178=CARTESIAN_POINT ( 'NONE',  ( 14.53047184896071897, -2.600157965045224895, 30.74683119005207743 ) ) ;
#1179=CARTESIAN_POINT ( 'NONE',  ( 16.21910129335899597, -2.657715359629131857, 31.77849191805844242 ) ) ;
#1180=CARTESIAN_POINT ( 'NONE',  ( -16.85396017336159247, -7.369474270740072441, 34.74850911626239736 ) ) ;
#1181=DIRECTION ( 'NONE',  ( 0.000000000000000000, 0.4999999999999960032, -0.8660254037844410391 ) ) ;
#1182=EDGE_CURVE ( 'NONE', #21592, #31771, #29736, .T. ) ;
#1183=CARTESIAN_POINT ( 'NONE',  ( -16.37677237136229991, -10.61292498521070549, 33.66303323003028680 ) ) ;
#1184=CARTESIAN_POINT ( 'NONE',  ( 6.989144256427000990, -11.91647553114624358, 32.58852847137148245 ) ) ;
#1185=FACE_OUTER_BOUND ( 'NONE', #27868, .T. ) ;
#1186=CARTESIAN_POINT ( 'NONE',  ( 2.307692307692309264, -3.886160181151819604, 36.00935417666054406 ) ) ;
#1187=EDGE_CURVE ( 'NONE', #82311, #58008, #62561, .T. ) ;
#1188=ORIENTED_EDGE ( 'NONE', *, *, #40388, .F. ) ;
#1189=ORIENTED_EDGE ( 'NONE', *, *, #2614, .F. ) ;
#1190=ORIENTED_EDGE ( 'NONE', *, *, #44498, .T. ) ;
#1191=CARTESIAN_POINT ( 'NONE',  ( -16.15384615384627409, -3.643525952248796163, 33.31231777344771672 ) ) ;
#1192=CARTESIAN_POINT ( 'NONE',  ( -4.153846153846152411, -13.87047571288749737, 32.06866353760679544 ) ) ;
#1193=LINE ( 'NONE', #21916, #2914 ) ;
#1194=CARTESIAN_POINT ( 'NONE',  ( -13.13456107297707121, -12.17597550085003633, 31.52189283813461884 ) ) ;
#1195=CARTESIAN_POINT ( 'NONE',  ( 18.00000000000000000, -9.058645607665452459, 34.76329471203371924 ) ) ;
#1196=VECTOR ( 'NONE', #82084, 1000.000000000000114 ) ;
#1197=EDGE_LOOP ( 'NONE', ( #72989, #17926 ) ) ;
#1199=ORIENTED_EDGE ( 'NONE', *, *, #32116, .T. ) ;
#1200=ADVANCED_FACE ( 'NONE', ( #42410 ), #83395, .F. ) ;
#1201=EDGE_LOOP ( 'NONE', ( #63869, #3784 ) ) ;
#1202=AXIS2_PLACEMENT_3D ( 'NONE', #5534, #46941, #53707 ) ;
#1203=EDGE_LOOP ( 'NONE', ( #39780, #41369 ) ) ;
#1204=CARTESIAN_POINT ( 'NONE',  ( 13.25392478150507891, -4.684245665217972032, 34.18127051446801090 ) ) ;
#1207=LINE ( 'NONE', #62023, #64637 ) ;
#1208=EDGE_CURVE ( 'NONE', #76314, #62928, #62650, .T. ) ;
#1209=CARTESIAN_POINT ( 'NONE',  ( -3.453696189676077832, -11.98009711892699691, 32.48740034544075428 ) ) ;
#1210=EDGE_CURVE ( 'NONE', #41958, #22384, #59220, .T. ) ;
#1211=CARTESIAN_POINT ( 'NONE',  ( -9.915233909823838232, -8.239355502252617924, 34.69524867566427417 ) ) ;
#1212=CARTESIAN_POINT ( 'NONE',  ( 14.53065544195898440, -7.369474539155828730, 34.99858011523957657 ) ) ;
#1214=ORIENTED_EDGE ( 'NONE', *, *, #71167, .T. ) ;
#1215=ORIENTED_EDGE ( 'NONE', *, *, #66533, .F. ) ;
#1216=CARTESIAN_POINT ( 'NONE',  ( -6.792551484843280640, -3.068774925481847937, 32.56582465632704526 ) ) ;
#1217=CARTESIAN_POINT ( 'NONE',  ( 4.376857505459002873, -11.24521262558773671, 33.06293181088029343 ) ) ;
#1218=ORIENTED_EDGE ( 'NONE', *, *, #85820, .T. ) ;
#1219=LINE ( 'NONE', #77325, #70914 ) ;
#1220=CARTESIAN_POINT ( 'NONE',  ( -2.084680956079457026, -8.239487800360276282, 34.69522927552633718 ) ) ;
#1221=CARTESIAN_POINT ( 'NONE',  ( -0.2114840416250089172, -9.233818618650603938, 34.70587769442853698 ) ) ;
#1222=EDGE_LOOP ( 'NONE', ( #64618, #77801, #78282, #649 ) ) ;
#1223=FACE_OUTER_BOUND ( 'NONE', #27080, .T. ) ;
#1224=CARTESIAN_POINT ( 'NONE',  ( -1.384615384615383471, -2.708943851104267164, 35.45975837776705220 ) ) ;
#1225=B_SPLINE_CURVE_WITH_KNOTS ( 'NONE', 3,
 ( #80204, #18943, #39223, #58138, #58578, #86985, #25252, #72547, #31565, #52714 ),
 .UNSPECIFIED., .F., .F.,
 ( 4, 2, 2, 2, 4 ),
 ( 0.000000000000000000, 0.0001954311564186862510, 0.0003908623128373725020, 0.0005862934692560588072, 0.0007817246256747450040 ),
 .UNSPECIFIED. ) ;
#1226=AXIS2_PLACEMENT_3D ( 'NONE', #35034, #1696, #8462 ) ;
#1227=ORIENTED_EDGE ( 'NONE', *, *, #63659, .T. ) ;
#1228=FACE_BOUND ( 'NONE', #18967, .T. ) ;
#1229=CARTESIAN_POINT ( 'NONE',  ( -11.66860950819323328, -11.66186481527757302, 32.95055677023626117 ) ) ;
#1232=CARTESIAN_POINT ( 'NONE',  ( 18.13079044096695469, -2.845873456487966635, 32.17976146951972538 ) ) ;
#1233=CARTESIAN_POINT ( 'NONE',  ( 13.38461538461538680, -4.945431358278436385, 36.03766855953609394 ) ) ;
#1235=CARTESIAN_POINT ( 'NONE',  ( 18.06525557127602610, -2.892918686051626498, 31.69288490824026638 ) ) ;
#1236=ORIENTED_EDGE ( 'NONE', *, *, #29058, .T. ) ;
#1237=CARTESIAN_POINT ( 'NONE',  ( -2.307692307692428724, -4.320704448113951379, 33.92786785259630022 ) ) ;
#1238=CARTESIAN_POINT ( 'NONE',  ( -6.065270000556319374, -11.67786785259541027, 32.92929555188721480 ) ) ;
#1239=ORIENTED_EDGE ( 'NONE', *, *, #43935, .T. ) ;
#1240=CARTESIAN_POINT ( 'NONE',  ( 8.519254038288416098, -3.137211980971221781, 32.19342716148376837 ) ) ;
#1241=CARTESIAN_POINT ( 'NONE',  ( 9.469381474791543241, -2.758268499246657068, 31.33685645148948140 ) ) ;
#1242=ORIENTED_EDGE ( 'NONE', *, *, #61678, .F. ) ;
#1243=EDGE_CURVE ( 'NONE', #12426, #74753, #36094, .T. ) ;
#1244=CARTESIAN_POINT ( 'NONE',  ( -13.16183571563731647, -11.60474049983371003, 33.02348890104160262 ) ) ;
#1245=CARTESIAN_POINT ( 'NONE',  ( 4.403900465484469784, -9.943054286541403997, 34.11300777759954883 ) ) ;
#1246=FACE_BOUND ( 'NONE', #48721, .T. ) ;
#1247=CARTESIAN_POINT ( 'NONE',  ( 8.769230769230768274, -13.53365097954675988, 30.81389545987213552 ) ) ;
#1248=CARTESIAN_POINT ( 'NONE',  ( 3.930919194939304973, -12.38737895849757820, 31.66785238281580206 ) ) ;
#1249=LINE ( 'NONE', #48104, #79871 ) ;
#1251=CARTESIAN_POINT ( 'NONE',  ( -14.05769230769088729, -7.500000000000154543, 35.00000000000007105 ) ) ;
#1252=LINE ( 'NONE', #22415, #73550 ) ;
#1254=ORIENTED_EDGE ( 'NONE', *, *, #37154, .F. ) ;
#1255=EDGE_LOOP ( 'NONE', ( #1876, #5321, #78832, #65229 ) ) ;
#1256=VECTOR ( 'NONE', #85243, 1000.000000000000227 ) ;
#1257=CARTESIAN_POINT ( 'NONE',  ( 16.15384615384615330, -9.058645607665452459, 34.76329471203371924 ) ) ;
#1258=CARTESIAN_POINT ( 'NONE',  ( -15.23076923076922995, -5.471508081941601098, 34.59228464037088457 ) ) ;
#1259=CARTESIAN_POINT ( 'NONE',  ( 5.999999999999880096, -10.21337939537710326, 33.94971097300076224 ) ) ;
#1260=FACE_OUTER_BOUND ( 'NONE', #59587, .T. ) ;
#1261=CARTESIAN_POINT ( 'NONE',  ( -13.16160254052199008, -2.523321265292115534, 31.42251411153756990 ) ) ;
#1263=EDGE_CURVE ( 'NONE', #72081, #77897, #57141, .T. ) ;
#1265=CARTESIAN_POINT ( 'NONE',  ( 3.903869409797562806, -12.01397095200673881, 32.43157075238190146 ) ) ;
#1266=CARTESIAN_POINT ( 'NONE',  ( -17.07692307692319744, -5.219633306517616589, 34.19971097300220464 ) ) ;
#1267=CARTESIAN_POINT ( 'NONE',  ( 17.93474900983875386, -2.506253911140460477, 30.00000000000013856 ) ) ;
#1269=CARTESIAN_POINT ( 'NONE',  ( 16.15384615384603251, -5.219633306517616589, 34.19971097300220464 ) ) ;
#1270=VECTOR ( 'NONE', #7494, 999.9999999999998863 ) ;
#1271=CARTESIAN_POINT ( 'NONE',  ( 9.942362003946008997, -11.28795663066794575, 33.01431243580653785 ) ) ;
#1272=DIRECTION ( 'NONE',  ( -0.000000000000000000, -0.3420201433256694901, -0.9396926207859082059 ) ) ;
#1273=VECTOR ( 'NONE', #84236, 1000.000000000000000 ) ;
#1274=B_SPLINE_CURVE_WITH_KNOTS ( 'NONE', 3,
 ( #40226, #60926, #54158, #26259, #53728, #67694, #88428, #6869, #54601, #40673 ),
 .UNSPECIFIED., .F., .F.,
 ( 4, 2, 2, 2, 4 ),
 ( 0.000000000000000000, 0.0001954311564186858715, 0.0003908623128373717431, 0.0005862934692560576146, 0.0007817246256747434861 ),
 .UNSPECIFIED. ) ;
#1275=FACE_OUTER_BOUND ( 'NONE', #59675, .T. ) ;
#1276=ORIENTED_EDGE ( 'NONE', *, *, #29973, .F. ) ;
#1277=CARTESIAN_POINT ( 'NONE',  ( 4.153846153846154188, -4.786620604624113540, 33.94971097300155094 ) ) ;
#1278=CARTESIAN_POINT ( 'NONE',  ( 7.715463243043537034, -4.684245665217972032, 34.18127051446801090 ) ) ;
#1280=B_SPLINE_CURVE_WITH_KNOTS ( 'NONE', 3,
 ( #37925, #51399, #4125, #65388, #32058, #17201, #78020, #44657, #72143, #2787 ),
 .UNSPECIFIED., .F., .F.,
 ( 4, 2, 2, 2, 4 ),
 ( 0.000000000000000000, 0.0001954339857564082062, 0.0003908679715128164124, 0.0005863019572692246186, 0.0007817359430256328248 ),
 .UNSPECIFIED. ) ;
#1281=EDGE_CURVE ( 'NONE', #88074, #55385, #19492, .T. ) ;
#1282=DIRECTION ( 'NONE',  ( 0.000000000000000000, 0.3420201433256641055, -0.9396926207859100932 ) ) ;
#1283=CARTESIAN_POINT ( 'NONE',  ( 16.85399611801622655, -11.43668979543635089, 33.22377378376089752 ) ) ;
#1285=CARTESIAN_POINT ( 'NONE',  ( 10.36538461538461320, -2.499999999999999556, 29.81609845454691765 ) ) ;
#1286=CARTESIAN_POINT ( 'NONE',  ( -14.43783951713053249, -12.27039167877662251, 31.24851455888617835 ) ) ;
#1287=VERTEX_POINT ( 'NONE', #66661 ) ;
#1288=CARTESIAN_POINT ( 'NONE',  ( 6.988332494352950341, -3.835265460703683349, 33.15142922261929925 ) ) ;
#1289=CARTESIAN_POINT ( 'NONE',  ( -2.557669051740896649, -10.82459398097509684, 33.81372124010185587 ) ) ;
#1290=EDGE_CURVE ( 'NONE', #40661, #65909, #31310, .T. ) ;
#1291=ORIENTED_EDGE ( 'NONE', *, *, #48742, .T. ) ;
#1292=CARTESIAN_POINT ( 'NONE',  ( -5.326946314216042033, -11.37209801155882971, 32.91403422569032955 ) ) ;
#1293=CARTESIAN_POINT ( 'NONE',  ( 13.13459216039392885, -9.356822207818506598, 34.66110646841856635 ) ) ;
#1294=ORIENTED_EDGE ( 'NONE', *, *, #33309, .T. ) ;
#1295=DIRECTION ( 'NONE',  ( -0.000000000000000000, 1.000000000000000000, 3.491481338843133355E-15 ) ) ;
#1296=CARTESIAN_POINT ( 'NONE',  ( -11.78843828251013015, -12.41104346484419452, 31.60698883733904196 ) ) ;
#1297=CARTESIAN_POINT ( 'NONE',  ( -9.627113710524334067, -2.506253911140448487, 29.99999999999988631 ) ) ;
#1298=EDGE_CURVE ( 'NONE', #29793, #8757, #25230, .T. ) ;
#1299=ORIENTED_EDGE ( 'NONE', *, *, #42085, .F. ) ;
#1300=ORIENTED_EDGE ( 'NONE', *, *, #66318, .F. ) ;
#1301=CARTESIAN_POINT ( 'NONE',  ( -10.39237177129122003, -2.308499170217967134, 30.53291367094873721 ) ) ;
#1302=ORIENTED_EDGE ( 'NONE', *, *, #36299, .T. ) ;
#1303=EDGE_CURVE ( 'NONE', #18982, #31195, #9931, .T. ) ;
#1304=CARTESIAN_POINT ( 'NONE',  ( -1.134561072977069651, -2.564540009722895419, 30.55348353981670684 ) ) ;
#1307=CARTESIAN_POINT ( 'NONE',  ( -4.153846153846273204, -6.879047030192662504, 34.71129190930017927 ) ) ;
#1308=CARTESIAN_POINT ( 'NONE',  ( -3.903791733932699515, -12.65882529074907126, 30.72640787790839312 ) ) ;
#1309=B_SPLINE_CURVE_WITH_KNOTS ( 'NONE', 3,
 ( #63041, #54975, #49548, #7681, #21180, #1353, #28842, #15322, #82899, #34706 ),
 .UNSPECIFIED., .F., .F.,
 ( 4, 2, 2, 2, 4 ),
 ( 0.0007817359430256390048, 0.0009771253907250078159, 0.001172514838424376735, 0.001367904286123745655, 0.001563293733823114574 ),
 .UNSPECIFIED. ) ;
#1310=CARTESIAN_POINT ( 'NONE',  ( 3.100078627658922947, -9.929715669179220328, 34.40415004197138416 ) ) ;
#1311=B_SPLINE_CURVE_WITH_KNOTS ( 'NONE', 3,
 ( #45122, #64944, #30722, #31161, #58188, #29416, #56865, #51406, #78912, #58634 ),
 .UNSPECIFIED., .F., .F.,
 ( 4, 2, 2, 2, 4 ),
 ( 0.000000000000000000, 0.0001954339857564055499, 0.0003908679715128110998, 0.0005863019572692165955, 0.0007817359430256221996 ),
 .UNSPECIFIED. ) ;
#1312=EDGE_CURVE ( 'NONE', #74314, #10085, #59898, .T. ) ;
#1313=ORIENTED_EDGE ( 'NONE', *, *, #22945, .T. ) ;
#1314=ORIENTED_EDGE ( 'NONE', *, *, #41131, .F. ) ;
#1315=CARTESIAN_POINT ( 'NONE',  ( 9.561616225640136690, -4.118384482072086072, 33.43331474514187107 ) ) ;
#1316=VERTEX_POINT ( 'NONE', #37852 ) ;
#1317=CARTESIAN_POINT ( 'NONE',  ( -5.300408001487407539, -4.988325925672468131, 34.36044203135681130 ) ) ;
#1318=EDGE_LOOP ( 'NONE', ( #8769, #9636 ) ) ;
#1319=AXIS2_PLACEMENT_3D ( 'NONE', #27859, #8927, #49896 ) ;
#1320=CIRCLE ( 'NONE', #45869, 0.2500000000000002220 ) ;
#1321=ADVANCED_FACE ( 'NONE', ( #85598 ), #37400, .F. ) ;
#1322=EDGE_CURVE ( 'NONE', #60496, #33135, #52828, .T. ) ;
#1323=DIRECTION ( 'NONE',  ( -0.000000000000000000, -0.000000000000000000, -1.000000000000000000 ) ) ;
#1324=CARTESIAN_POINT ( 'NONE',  ( 6.699591998512593349, -9.417330523894424488, 34.63758898049880486 ) ) ;
#1325=ORIENTED_EDGE ( 'NONE', *, *, #58150, .T. ) ;
#1326=CARTESIAN_POINT ( 'NONE',  ( -12.21148414990014786, -5.728107161865378494, 34.42597550085002922 ) ) ;
#1328=EDGE_LOOP ( 'NONE', ( #27351, #18473, #24324, #5513 ) ) ;
#1329=CARTESIAN_POINT ( 'NONE',  ( -6.923076923076922462, -11.16473453929635440, 33.15142922261926373 ) ) ;
#1330=EDGE_LOOP ( 'NONE', ( #65690, #41436, #43338, #58463 ) ) ;
#1332=DIRECTION ( 'NONE',  ( 0.000000000000000000, 1.000000000000000000, 0.000000000000000000 ) ) ;
#1334=CARTESIAN_POINT ( 'NONE',  ( 16.15384615384615330, -12.37446782046654192, 30.86335684631486131 ) ) ;
#1335=CARTESIAN_POINT ( 'NONE',  ( -15.23076923076922995, -2.900454961884010974, 35.62045528018868623 ) ) ;
#1336=FACE_BOUND ( 'NONE', #67379, .T. ) ;
#1337=CARTESIAN_POINT ( 'NONE',  ( -11.60373198442231413, -2.625532179533444754, 30.86335684631481513 ) ) ;
#1338=CARTESIAN_POINT ( 'NONE',  ( -17.86947429823643674, -12.27024696741798770, 31.24895572276497901 ) ) ;
#1339=CARTESIAN_POINT ( 'NONE',  ( -16.15384615384627409, -5.094484230521993062, 34.41647553114689373 ) ) ;
#1340=CARTESIAN_POINT ( 'NONE',  ( 3.230769230769231726, -4.661471528628507777, 34.16647553114623292 ) ) ;
#1342=DIRECTION ( 'NONE',  ( -0.000000000000000000, 0.3420201433256694901, -0.9396926207859082059 ) ) ;
#1343=CARTESIAN_POINT ( 'NONE',  ( 10.48469401227430886, -10.70098750199973203, 33.91152734681376302 ) ) ;
#1344=VERTEX_POINT ( 'NONE', #38745 ) ;
#1345=CARTESIAN_POINT ( 'NONE',  ( -5.999999999999690914, -2.506253911140614576, 30.00000000000323297 ) ) ;
#1346=ORIENTED_EDGE ( 'NONE', *, *, #76373, .F. ) ;
#1347=ORIENTED_EDGE ( 'NONE', *, *, #86412, .F. ) ;
#1348=CARTESIAN_POINT ( 'NONE',  ( -8.769230769230768274, -13.75783147151868846, 33.36296068462461051 ) ) ;
#1349=CARTESIAN_POINT ( 'NONE',  ( 15.00784301325307979, -12.15238873228292071, 31.58232369045353849 ) ) ;
#1350=CARTESIAN_POINT ( 'NONE',  ( -11.78848477575450282, -11.86270091957321249, 32.19358267280087915 ) ) ;
#1352=CARTESIAN_POINT ( 'NONE',  ( -12.33101302330482341, -2.647132371071621471, 31.75357179365171589 ) ) ;
#1353=CARTESIAN_POINT ( 'NONE',  ( 9.942362003946010773, -2.564540009722896752, 30.55348353981670684 ) ) ;
#1354=ORIENTED_EDGE ( 'NONE', *, *, #69690, .F. ) ;
#1355=ADVANCED_FACE ( 'NONE', ( #66208 ), #78831, .F. ) ;
#1356=CARTESIAN_POINT ( 'NONE',  ( 13.31934493865461278, -5.219633306516282545, 34.19971097300152962 ) ) ;
#1357=CARTESIAN_POINT ( 'NONE',  ( -6.223484943723947893, -6.760086850603068243, 34.69517049084099369 ) ) ;
#1358=CARTESIAN_POINT ( 'NONE',  ( -10.39237326377176451, -9.886259254753566594, 34.14407573483972413 ) ) ;
#1359=CARTESIAN_POINT ( 'NONE',  ( -3.230769230769352962, -3.083524468854526912, 32.58852847137268327 ) ) ;
#1360=CYLINDRICAL_SURFACE ( 'NONE', #50617, 0.2500000000000012212 ) ;
#1361=ORIENTED_EDGE ( 'NONE', *, *, #87825, .F. ) ;
#1362=AXIS2_PLACEMENT_3D ( 'NONE', #81252, #32171, #38483 ) ;
#1363=EDGE_CURVE ( 'NONE', #62783, #21910, #30186, .T. ) ;
#1364=CARTESIAN_POINT ( 'NONE',  ( -0.7115616857599191825, -2.341070481393820124, 30.72580821765574299 ) ) ;
#1365=ORIENTED_EDGE ( 'NONE', *, *, #57441, .T. ) ;
#1366=ORIENTED_EDGE ( 'NONE', *, *, #74010, .T. ) ;
#1367=ADVANCED_FACE ( 'NONE', ( #32877 ), #46389, .F. ) ;
#1368=CARTESIAN_POINT ( 'NONE',  ( -6.065270000556318486, -4.320704448112771878, 33.92786785259540494 ) ) ;
#1371=CARTESIAN_POINT ( 'NONE',  ( 17.07692307692307665, -13.75783147151868846, 33.36296068462461051 ) ) ;
#1372=CARTESIAN_POINT ( 'NONE',  ( 14.30769230769231015, -9.905515769479276145, 34.41647553114623292 ) ) ;
#1373=CARTESIAN_POINT ( 'NONE',  ( 2.557746727605761272, -10.06805714834173848, 34.32951233291982618 ) ) ;
#1375=ADVANCED_FACE ( 'NONE', ( #33764 ), #13928, .F. ) ;
#1376=CYLINDRICAL_SURFACE ( 'NONE', #15842, 0.2499999999999979738 ) ;
#1377=ORIENTED_EDGE ( 'NONE', *, *, #68097, .T. ) ;
#1378=CARTESIAN_POINT ( 'NONE',  ( 4.403900465484468008, -4.235687564193446164, 33.53795663066793509 ) ) ;
#1379=CARTESIAN_POINT ( 'NONE',  ( -0.4615384615384611200, -5.471508081941601098, 34.59228464037088457 ) ) ;
#1380=ORIENTED_EDGE ( 'NONE', *, *, #80549, .T. ) ;
#1381=CARTESIAN_POINT ( 'NONE',  ( -9.442362173959551797, -4.336752205174649433, 33.62275283266504289 ) ) ;
#1382=FACE_OUTER_BOUND ( 'NONE', #53496, .T. ) ;
#1383=CARTESIAN_POINT ( 'NONE',  ( -0.7115152055870537229, -4.075325502946086864, 33.72974371597207721 ) ) ;
#1384=CARTESIAN_POINT ( 'NONE',  ( -3.454254174493178731, -5.113361153441932316, 34.14387501736621999 ) ) ;
#1385=CARTESIAN_POINT ( 'NONE',  ( -2.177166869458661669, -2.372941743896878286, 30.88044141588254377 ) ) ;
#1387=DIRECTION ( 'NONE',  ( -0.000000000000000000, -0.1736481776669307198, -0.9848077530122080203 ) ) ;
#1389=ORIENTED_EDGE ( 'NONE', *, *, #33394, .T. ) ;
#1390=CARTESIAN_POINT ( 'NONE',  ( -1.384615384615383471, -11.16473453929635440, 33.15142922261926373 ) ) ;
#1391=CARTESIAN_POINT ( 'NONE',  ( -1.384615384615383471, -3.322132147404559976, 32.92929555188717927 ) ) ;
#1392=VECTOR ( 'NONE', #70371, 1000.000000000000114 ) ;
#1394=CARTESIAN_POINT ( 'NONE',  ( 9.692307692307695177, -12.29105614889573062, 35.45975837776705220 ) ) ;
#1396=ORIENTED_EDGE ( 'NONE', *, *, #48193, .T. ) ;
#1398=CARTESIAN_POINT ( 'NONE',  ( -16.08777780284372128, -12.10708131394839882, 31.69288490824020954 ) ) ;
#1399=ADVANCED_FACE ( 'NONE', ( #5854 ), #67554, .F. ) ;
#1400=AXIS2_PLACEMENT_3D ( 'NONE', #83248, #42268, #48554 ) ;
#1402=CARTESIAN_POINT ( 'NONE',  ( 1.134592147322421418, -9.271318131107980420, 34.42618302367067429 ) ) ;
#1403=ADVANCED_FACE ( 'NONE', ( #73870 ), #3864, .F. ) ;
#1404=CARTESIAN_POINT ( 'NONE',  ( -0.5276208408985972875, -10.67929555188718460, 33.92786785259543336 ) ) ;
#1407=CARTESIAN_POINT ( 'NONE',  ( -15.48074596171158213, -2.779195860258146578, 31.39871582349836032 ) ) ;
#1408=CARTESIAN_POINT ( 'NONE',  ( -17.14300545628321260, -2.292212530054420050, 30.41441678777542634 ) ) ;
#1410=FACE_OUTER_BOUND ( 'NONE', #39229, .T. ) ;
#1411=ORIENTED_EDGE ( 'NONE', *, *, #7656, .F. ) ;
#1412=CARTESIAN_POINT ( 'NONE',  ( -6.923076923076922462, -6.343179335718451384, 34.87096338111211935 ) ) ;
#1413=B_SPLINE_CURVE_WITH_KNOTS ( 'NONE', 3,
 ( #19596, #45281, #74107, #4306, #66900, #39442, #88095, #86750, #59247, #52486 ),
 .UNSPECIFIED., .F., .F.,
 ( 4, 2, 2, 2, 4 ),
 ( 0.0007817246256747505334, 0.0009771112852218954894, 0.001172497944769040554, 0.001367884604316185618, 0.001563271263863330682 ),
 .UNSPECIFIED. ) ;
#1414=ORIENTED_EDGE ( 'NONE', *, *, #59284, .T. ) ;
#1416=CYLINDRICAL_SURFACE ( 'NONE', #3843, 0.2499999999999995559 ) ;
#1417=ORIENTED_EDGE ( 'NONE', *, *, #17439, .T. ) ;
#1418=FACE_OUTER_BOUND ( 'NONE', #24802, .T. ) ;
#1419=CARTESIAN_POINT ( 'NONE',  ( 4.153846153846154188, -9.058645607665452459, 34.76329471203371924 ) ) ;
#1420=CARTESIAN_POINT ( 'NONE',  ( 0.2386122440223140684, -4.186968288167447483, 33.49512374952580984 ) ) ;
#1421=CARTESIAN_POINT ( 'NONE',  ( 13.38461538461526423, -12.16647553114689728, 32.15551576947799362 ) ) ;
#1422=CARTESIAN_POINT ( 'NONE',  ( -18.22292621751614305, -4.186968288167451036, 33.49512374952581695 ) ) ;
#1423=EDGE_CURVE ( 'NONE', #25798, #52031, #74311, .T. ) ;
#1424=EDGE_CURVE ( 'NONE', #81511, #81196, #74355, .T. ) ;
#1425=ORIENTED_EDGE ( 'NONE', *, *, #59426, .F. ) ;
#1426=EDGE_LOOP ( 'NONE', ( #11958, #3521 ) ) ;
#1427=FACE_BOUND ( 'NONE', #5912, .T. ) ;
#1429=CARTESIAN_POINT ( 'NONE',  ( -7.912236225513979981, -5.471508081941602875, 34.59228464037088457 ) ) ;
#1430=VECTOR ( 'NONE', #86578, 1000.000000000000000 ) ;
#1431=B_SPLINE_CURVE_WITH_KNOTS ( 'NONE', 3,
 ( #54758, #26411, #82245, #81362, #55201, #12887, #13773, #41258, #48890, #43025 ),
 .UNSPECIFIED., .F., .F.,
 ( 4, 2, 2, 2, 4 ),
 ( 0.000000000000000000, 0.0001954339881912774070, 0.0003908679763825548140, 0.0005863019645738322752, 0.0007817359527651096280 ),
 .UNSPECIFIED. ) ;
#1432=EDGE_CURVE ( 'NONE', #22613, #47954, #51688, .T. ) ;
#1433=CARTESIAN_POINT ( 'NONE',  ( -14.08491263871423982, -11.60474049983371003, 33.02348890104160262 ) ) ;
#1435=CARTESIAN_POINT ( 'NONE',  ( 9.442284455014730682, -12.22074536777954989, 31.39888409691088356 ) ) ;
#1436=CARTESIAN_POINT ( 'NONE',  ( 0.7114838709165044461, -12.68172785388650681, 30.59649109432439573 ) ) ;
#1437=VERTEX_POINT ( 'NONE', #81079 ) ;
#1438=ORIENTED_EDGE ( 'NONE', *, *, #64153, .T. ) ;
#1439=EDGE_CURVE ( 'NONE', #28677, #64411, #73254, .T. ) ;
#1440=ORIENTED_EDGE ( 'NONE', *, *, #81732, .T. ) ;
#1441=CARTESIAN_POINT ( 'NONE',  ( 13.25400502499085675, -7.722926236386453702, 34.74524107206102030 ) ) ;
#1442=ORIENTED_EDGE ( 'NONE', *, *, #71141, .T. ) ;
#1443=VECTOR ( 'NONE', #79777, 999.9999999999998863 ) ;
#1445=EDGE_CURVE ( 'NONE', #17692, #1987, #20253, .T. ) ;
#1446=CARTESIAN_POINT ( 'NONE',  ( 14.08476534878545827, -11.98009711892699514, 32.48740034544076138 ) ) ;
#1447=CARTESIAN_POINT ( 'NONE',  ( 13.60739505359345181, -11.60474049983371003, 33.02348890104160262 ) ) ;
#1448=ORIENTED_EDGE ( 'NONE', *, *, #31385, .F. ) ;
#1449=CARTESIAN_POINT ( 'NONE',  ( -8.703975629717932705, -4.320704448112861584, 33.92786785259548310 ) ) ;
#1451=DIRECTION ( 'NONE',  ( -0.000000000000000000, 0.1736481776669307198, -0.9848077530122080203 ) ) ;
#1452=EDGE_CURVE ( 'NONE', #74112, #56593, #80776, .T. ) ;
#1453=CARTESIAN_POINT ( 'NONE',  ( -18.00000000000000000, -3.679149656540967150, 35.86790692298802696 ) ) ;
#1454=CARTESIAN_POINT ( 'NONE',  ( -11.53846153846165912, -3.300289026999228881, 32.46337939537708905 ) ) ;
#1455=ORIENTED_EDGE ( 'NONE', *, *, #59844, .F. ) ;
#1457=VECTOR ( 'NONE', #23969, 1000.000000000000000 ) ;
#1458=ORIENTED_EDGE ( 'NONE', *, *, #42077, .F. ) ;
#1459=VECTOR ( 'NONE', #50275, 1000.000000000000227 ) ;
#1460=CARTESIAN_POINT ( 'NONE',  ( 3.454195629684017277, -7.630147987733843173, 34.99859428049665411 ) ) ;
#1461=CARTESIAN_POINT ( 'NONE',  ( -8.069080063669991532, -6.503392248772476236, 34.64988816332204635 ) ) ;
#1462=CARTESIAN_POINT ( 'NONE',  ( 1.450682717965462887, -11.35647404775217595, 33.31231777344667222 ) ) ;
#1463=VECTOR ( 'NONE', #18706, 1000.000000000000227 ) ;
#1464=CARTESIAN_POINT ( 'NONE',  ( -17.74994558008654622, -5.642605341092954419, 34.66089969410670335 ) ) ;
#1465=CARTESIAN_POINT ( 'NONE',  ( 12.46153846153846168, -12.62096338111211580, 30.90682066428153263 ) ) ;
#1466=FACE_BOUND ( 'NONE', #28995, .T. ) ;
#1467=CARTESIAN_POINT ( 'NONE',  ( 8.639082799499069765, -11.04286588640298561, 33.62463336215343901 ) ) ;
#1468=EDGE_LOOP ( 'NONE', ( #13731, #4681 ) ) ;
#1469=CARTESIAN_POINT ( 'NONE',  ( 17.32686859527121470, -10.76462480002816413, 33.53768742498949962 ) ) ;
#1470=CARTESIAN_POINT ( 'NONE',  ( 9.562159722576005549, -12.15440758774515473, 32.17923288041532004 ) ) ;
#1471=CARTESIAN_POINT ( 'NONE',  ( 11.40798483034507527, -7.276988635370452485, 34.74523720219453793 ) ) ;
#1472=CARTESIAN_POINT ( 'NONE',  ( 7.053602361310569613, -9.503571793651733657, 34.60286762892837942 ) ) ;
#1474=CARTESIAN_POINT ( 'NONE',  ( -18.06527044596078113, -8.613356846314824011, 34.62446782046655613 ) ) ;
#1475=EDGE_CURVE ( 'NONE', #48420, #40198, #13133, .T. ) ;
#1476=ORIENTED_EDGE ( 'NONE', *, *, #76162, .F. ) ;
#1477=FACE_BOUND ( 'NONE', #64109, .T. ) ;
#1478=CARTESIAN_POINT ( 'NONE',  ( 6.000000000000001776, -12.62096338111211580, 30.90682066428153263 ) ) ;
#1479=DIRECTION ( 'NONE',  ( 0.000000000000000000, 0.3420201433256610524, 0.9396926207859113145 ) ) ;
#1481=ORIENTED_EDGE ( 'NONE', *, *, #32747, .T. ) ;
#1482=CARTESIAN_POINT ( 'NONE',  ( 0.3313912521002408962, -10.88202310037936194, 33.43294751532457099 ) ) ;
#1483=CARTESIAN_POINT ( 'NONE',  ( -3.453696189676078276, -2.308479472611653094, 30.53278059502174457 ) ) ;
#1484=CARTESIAN_POINT ( 'NONE',  ( 8.769230769230768274, -8.164416787775445883, 34.95778746994557906 ) ) ;
#1485=CARTESIAN_POINT ( 'NONE',  ( -16.15384615384615330, -6.435427911321262684, 35.78748833219616898 ) ) ;
#1486=VERTEX_POINT ( 'NONE', #30102 ) ;
#1487=B_SPLINE_CURVE_WITH_KNOTS ( 'NONE', 3,
 ( #50518, #16738, #43334, #70812, #72125, #30265, #71680, #3223, #30697, #9115 ),
 .UNSPECIFIED., .F., .F.,
 ( 4, 2, 2, 2, 4 ),
 ( 0.000000000000000000, 0.0001954339857564074202, 0.0003908679715128148403, 0.0005863019572692222334, 0.0007817359430256296806 ),
 .UNSPECIFIED. ) ;
#1488=B_SPLINE_CURVE_WITH_KNOTS ( 'NONE', 3,
 ( #57728, #2327, #83891, #16736, #37447, #71678 ),
 .UNSPECIFIED., .F., .F.,
 ( 4, 2, 4 ),
 ( 0.4999999999999957812, 0.7499999999999978906, 1.000000000000000000 ),
 .UNSPECIFIED. ) ;
#1489=EDGE_CURVE ( 'NONE', #37467, #53160, #71084, .T. ) ;
#1491=EDGE_LOOP ( 'NONE', ( #25827, #67846, #4888, #4081 ) ) ;
#1492=CARTESIAN_POINT ( 'NONE',  ( 4.219913487196228274, -2.833524468853757750, 32.15551576947925838 ) ) ;
#1494=CARTESIAN_POINT ( 'NONE',  ( 11.66898724022510159, -6.852161475712352789, 34.70806712695775786 ) ) ;
#1496=LINE ( 'NONE', #28982, #40056 ) ;
#1497=B_SPLINE_CURVE_WITH_KNOTS ( 'NONE', 3,
 ( #50986, #61969, #64501, #9157, #34506, #2809, #57326, #84822, #64956, #278 ),
 .UNSPECIFIED., .F., .F.,
 ( 4, 2, 2, 2, 4 ),
 ( 0.000000000000000000, 0.0001954311564186872810, 0.0003908623128373745620, 0.0005862934692560618430, 0.0007817246256747491240 ),
 .UNSPECIFIED. ) ;
#1498=CARTESIAN_POINT ( 'NONE',  ( -12.68502338610279345, -10.97335522853832579, 33.68706563782419749 ) ) ;
#1499=CARTESIAN_POINT ( 'NONE',  ( -5.869474561766354626, -6.808710257144159783, 34.95449254468098843 ) ) ;
#1500=CARTESIAN_POINT ( 'NONE',  ( 8.639082799499073317, -4.299443229763728169, 33.91186481527756058 ) ) ;
#1502=CARTESIAN_POINT ( 'NONE',  ( 8.068933387422255521, -4.387253974876678342, 33.66317474335728832 ) ) ;
#1505=ORIENTED_EDGE ( 'NONE', *, *, #84173, .T. ) ;
#1507=ORIENTED_EDGE ( 'NONE', *, *, #80002, .T. ) ;
#1508=ORIENTED_EDGE ( 'NONE', *, *, #431, .F. ) ;
#1509=CARTESIAN_POINT ( 'NONE',  ( 4.153846153846154188, -12.34228464037088635, 31.77849191805839268 ) ) ;
#1510=VERTEX_POINT ( 'NONE', #22020 ) ;
#1511=CARTESIAN_POINT ( 'NONE',  ( 16.94623161025552704, -4.809359713505814149, 33.96456829005828837 ) ) ;
#1512=EDGE_CURVE ( 'NONE', #50046, #70330, #62546, .T. ) ;
#1513=CARTESIAN_POINT ( 'NONE',  ( -5.076923076923075762, -12.62096338111211580, 30.90682066428153263 ) ) ;
#1514=CARTESIAN_POINT ( 'NONE',  ( 18.00000000000031264, -2.255955759149395501, 30.00000000000324363 ) ) ;
#1515=LINE ( 'NONE', #29000, #34445 ) ;
#1516=CARTESIAN_POINT ( 'NONE',  ( 12.46153846153833911, -10.90142922262034020, 33.41473453929536674 ) ) ;
#1518=CARTESIAN_POINT ( 'NONE',  ( 16.15384615384615330, -11.69971097300155272, 32.46337939537588113 ) ) ;
#1519=CARTESIAN_POINT ( 'NONE',  ( -15.16551409125639260, -8.656820664281605460, 34.87096338111211224 ) ) ;
#1520=EDGE_CURVE ( 'NONE', #50046, #29769, #88292, .T. ) ;
#1521=CARTESIAN_POINT ( 'NONE',  ( -18.00000000000012079, -8.613356846316285953, 34.62446782046622218 ) ) ;
#1522=CARTESIAN_POINT ( 'NONE',  ( -2.307692307692305711, -2.833524468853757305, 32.15551576947925838 ) ) ;
#1524=CARTESIAN_POINT ( 'NONE',  ( 7.846153846153846700, -2.292212530054420494, 30.41441678777542634 ) ) ;
#1525=AXIS2_PLACEMENT_3D ( 'NONE', #68477, #60388, #68918 ) ;
#1527=ORIENTED_EDGE ( 'NONE', *, *, #47274, .F. ) ;
#1528=CARTESIAN_POINT ( 'NONE',  ( 12.52679360105129724, -2.657715359629132301, 31.77849191805844242 ) ) ;
#1529=CARTESIAN_POINT ( 'NONE',  ( 3.480823650682683734, -10.82426656108011720, 33.81400080652039009 ) ) ;
#1530=CARTESIAN_POINT ( 'NONE',  ( -2.373449110206616641, -7.249945686854185389, 34.74374336980224598 ) ) ;
#1531=VERTEX_POINT ( 'NONE', #22460 ) ;
#1532=VECTOR ( 'NONE', #28097, 1000.000000000000000 ) ;
#1533=CARTESIAN_POINT ( 'NONE',  ( 12.21151522424549896, -9.271318131107980420, 34.42618302367067429 ) ) ;
#1534=AXIS2_PLACEMENT_3D ( 'NONE', #68702, #89001, #40360 ) ;
#1535=CARTESIAN_POINT ( 'NONE',  ( -10.61538461538473577, -12.70778746994576025, 30.41441678777401236 ) ) ;
#1537=CARTESIAN_POINT ( 'NONE',  ( -12.23875892027004753, -10.81320215134717344, 33.49497208177562868 ) ) ;
#1538=VERTEX_POINT ( 'NONE', #49922 ) ;
#1539=CYLINDRICAL_SURFACE ( 'NONE', #87522, 0.2499999999999993616 ) ;
#1540=EDGE_LOOP ( 'NONE', ( #24940, #19961, #33858, #62612 ) ) ;
#1541=CARTESIAN_POINT ( 'NONE',  ( 10.83816415665302380, -8.496831190052093419, 34.64984203495476578 ) ) ;
#1542=CARTESIAN_POINT ( 'NONE',  ( 8.900021210197715860, -9.084667340241226796, 34.75534355489798344 ) ) ;
#1543=CYLINDRICAL_SURFACE ( 'NONE', #7052, 0.2500000000000012212 ) ;
#1544=CARTESIAN_POINT ( 'NONE',  ( -9.822455662039388358, -8.630895178749533159, 34.87696386517710323 ) ) ;
#1545=CARTESIAN_POINT ( 'NONE',  ( -17.86947456176635640, -12.50538340440932394, 31.33453814440721885 ) ) ;
#1546=ORIENTED_EDGE ( 'NONE', *, *, #44070, .T. ) ;
#1547=EDGE_CURVE ( 'NONE', #76633, #31437, #38415, .T. ) ;
#1548=ORIENTED_EDGE ( 'NONE', *, *, #24604, .T. ) ;
#1549=ORIENTED_EDGE ( 'NONE', *, *, #14770, .F. ) ;
#1550=CARTESIAN_POINT ( 'NONE',  ( 13.38461538461538680, -3.050289026998446396, 32.03036669348365706 ) ) ;
#1551=CARTESIAN_POINT ( 'NONE',  ( 13.60762673622823726, -9.886259254753566594, 34.14407573483972413 ) ) ;
#1552=CIRCLE ( 'NONE', #4433, 0.2500000000000002220 ) ;
#1554=DIRECTION ( 'NONE',  ( 0.000000000000000000, 0.8660254037844377084, 0.5000000000000015543 ) ) ;
#1555=CARTESIAN_POINT ( 'NONE',  ( 0.3954560821783242308, -12.34228464037088280, 31.77849191805838558 ) ) ;
#1556=CARTESIAN_POINT ( 'NONE',  ( -7.846153846153844924, -3.937682226553329556, 33.60647404775216529 ) ) ;
#1558=EDGE_LOOP ( 'NONE', ( #33756, #39218 ) ) ;
#1560=ORIENTED_EDGE ( 'NONE', *, *, #74064, .F. ) ;
#1561=EDGE_CURVE ( 'NONE', #27440, #31586, #35624, .T. ) ;
#1562=LINE ( 'NONE', #56940, #28726 ) ;
#1563=ORIENTED_EDGE ( 'NONE', *, *, #50794, .F. ) ;
#1564=CARTESIAN_POINT ( 'NONE',  ( -9.822999158975250111, -8.999036380462717588, 34.52022231692819076 ) ) ;
#1566=CARTESIAN_POINT ( 'NONE',  ( -10.61538461538461320, -5.180354513474913603, 36.12317359536750416 ) ) ;
#1567=CARTESIAN_POINT ( 'NONE',  ( -10.83886955910856464, -11.89387501736622710, 32.13663884655806413 ) ) ;
#1569=VECTOR ( 'NONE', #41135, 1000.000000000000000 ) ;
#1570=EDGE_LOOP ( 'NONE', ( #71156, #18996, #23444, #80993 ) ) ;
#1571=CARTESIAN_POINT ( 'NONE',  ( 13.63456079399343146, -10.92531984108285670, 33.72920026020278073 ) ) ;
#1573=ORIENTED_EDGE ( 'NONE', *, *, #85018, .T. ) ;
#1574=FACE_BOUND ( 'NONE', #53527, .T. ) ;
#1575=CARTESIAN_POINT ( 'NONE',  ( 6.700150705560777631, -4.186968288167446595, 33.49512374952580274 ) ) ;
#1577=VECTOR ( 'NONE', #24271, 1000.000000000000114 ) ;
#1578=CARTESIAN_POINT ( 'NONE',  ( -4.284536756956462966, -9.929715669179216775, 34.40415004197138416 ) ) ;
#1579=ORIENTED_EDGE ( 'NONE', *, *, #36750, .F. ) ;
#1580=CARTESIAN_POINT ( 'NONE',  ( -14.24162497434223162, -8.164416787775445883, 34.95778746994558617 ) ) ;
#1581=ADVANCED_FACE ( 'NONE', ( #36425 ), #42744, .F. ) ;
#1585=CARTESIAN_POINT ( 'NONE',  ( -17.07692307692319744, -2.625532179533778709, 30.86335684631627174 ) ) ;
#1586=VERTEX_POINT ( 'NONE', #29669 ) ;
#1588=CARTESIAN_POINT ( 'NONE',  ( 16.37680905740764103, -7.369474270740072441, 34.74850911626239736 ) ) ;
#1589=CARTESIAN_POINT ( 'NONE',  ( -8.069638770718174925, -12.11044203135681840, 32.26167407432752299 ) ) ;
#1590=DIRECTION ( 'NONE',  ( -0.000000000000000000, -0.7660444431189791237, -0.6427876096865379196 ) ) ;
#1591=CARTESIAN_POINT ( 'NONE',  ( 13.51540582558233794, -2.295524264805589354, 30.44142389570982488 ) ) ;
#1592=CARTESIAN_POINT ( 'NONE',  ( -15.00798968950081758, -11.89424750095246175, 32.13594075562311758 ) ) ;
#1593=CARTESIAN_POINT ( 'NONE',  ( 8.992010438208833278, -4.226511098958373402, 33.85474049983370293 ) ) ;
#1594=CARTESIAN_POINT ( 'NONE',  ( 5.076923076922954969, -11.48612834414049644, 32.76840700105863391 ) ) ;
#1595=CARTESIAN_POINT ( 'NONE',  ( 11.40798635338582123, -7.276987145209184327, 34.99546412871779211 ) ) ;
#1596=EDGE_CURVE ( 'NONE', #3333, #49885, #76447, .T. ) ;
#1597=CARTESIAN_POINT ( 'NONE',  ( -0.4615384615384611200, -2.900454961884010974, 35.62045528018868623 ) ) ;
#1598=DIRECTION ( 'NONE',  ( -0.000000000000000000, -0.1736481776669307198, -0.9848077530122080203 ) ) ;
#1599=CARTESIAN_POINT ( 'NONE',  ( 2.307692307692186251, -6.835583212225970762, 34.95778746994575670 ) ) ;
#1600=CARTESIAN_POINT ( 'NONE',  ( -2.307692307692428724, -5.941354392335915335, 34.76329471203413846 ) ) ;
#1602=VERTEX_POINT ( 'NONE', #72854 ) ;
#1603=B_SPLINE_CURVE_WITH_KNOTS ( 'NONE', 3,
 ( #75818, #21762, #54650, #49240, #6915, #63185, #1937, #48342, #76714, #68621 ),
 .UNSPECIFIED., .F., .F.,
 ( 4, 2, 2, 2, 4 ),
 ( 0.000000000000000000, 0.0001954339857564054144, 0.0003908679715128108288, 0.0005863019572692162703, 0.0007817359430256216575 ),
 .UNSPECIFIED. ) ;
#1604=CARTESIAN_POINT ( 'NONE',  ( 12.68431800280687050, -2.600157965045224895, 30.74683119005207743 ) ) ;
#1605=ORIENTED_EDGE ( 'NONE', *, *, #8664, .F. ) ;
#1606=CARTESIAN_POINT ( 'NONE',  ( -13.38461538461538325, -9.058645607665452459, 34.76329471203371924 ) ) ;
#1607=ORIENTED_EDGE ( 'NONE', *, *, #49753, .T. ) ;
#1608=CARTESIAN_POINT ( 'NONE',  ( -13.16160254052199008, -2.308499170217967134, 30.53291367094873721 ) ) ;
#1609=CARTESIAN_POINT ( 'NONE',  ( 6.000000000000001776, -2.900454961884010974, 35.62045528018868623 ) ) ;
#1610=ORIENTED_EDGE ( 'NONE', *, *, #74543, .F. ) ;
#1611=CARTESIAN_POINT ( 'NONE',  ( -7.976301055592065481, -6.001485441113819874, 34.52039167877662607 ) ) ;
#1613=FACE_OUTER_BOUND ( 'NONE', #38638, .T. ) ;
#1615=CARTESIAN_POINT ( 'NONE',  ( -4.153846153845837108, -2.255955759149395501, 30.00000000000324363 ) ) ;
#1616=CARTESIAN_POINT ( 'NONE',  ( 17.07692307692295586, -9.528491918059723176, 34.59228464037033035 ) ) ;
#1617=CARTESIAN_POINT ( 'NONE',  ( 16.94623161025552704, -12.38065189839062263, 30.83690757178629482 ) ) ;
#1618=CARTESIAN_POINT ( 'NONE',  ( 15.16544521796492262, -7.749976730030849303, 34.74374725381503737 ) ) ;
#1619=CARTESIAN_POINT ( 'NONE',  ( -39.05038313613820122, -2.499999999999999556, 29.75000000000000355 ) ) ;
#1620=AXIS2_PLACEMENT_3D ( 'NONE', #26129, #39662, #54032 ) ;
#1622=EDGE_CURVE ( 'NONE', #5191, #15410, #45829, .T. ) ;
#1623=EDGE_CURVE ( 'NONE', #39944, #28593, #65207, .T. ) ;
#1624=B_SPLINE_CURVE_WITH_KNOTS ( 'NONE', 3,
 ( #85308, #86659, #71329, #78096, #3319, #51482, #79879, #58707, #17284, #57825 ),
 .UNSPECIFIED., .F., .F.,
 ( 4, 2, 2, 2, 4 ),
 ( 0.000000000000000000, 0.0001954339857564097512, 0.0003908679715128195024, 0.0005863019572692292807, 0.0007817359430256390048 ),
 .UNSPECIFIED. ) ;
#1625=CARTESIAN_POINT ( 'NONE',  ( 11.31497661389721010, -5.827078755546623690, 34.72654668319379567 ) ) ;
#1626=CARTESIAN_POINT ( 'NONE',  ( 14.53047184896071897, -10.81320215134717344, 33.49497208177562868 ) ) ;
#1628=EDGE_CURVE ( 'NONE', #21791, #14730, #87164, .T. ) ;
#1629=DIRECTION ( 'NONE',  ( 0.000000000000000000, 0.8660254037844377084, -0.5000000000000015543 ) ) ;
#1631=EDGE_CURVE ( 'NONE', #69859, #18936, #78279, .T. ) ;
#1632=B_SPLINE_CURVE_WITH_KNOTS ( 'NONE', 3,
 ( #47902, #83029, #21761, #48787, #6485, #47452, #41155, #68620, #34387, #21313 ),
 .UNSPECIFIED., .F., .F.,
 ( 4, 2, 2, 2, 4 ),
 ( 0.0007817246256747434861, 0.0009771112852218859484, 0.001172497944769028411, 0.001367884604316171090, 0.001563271263863313552 ),
 .UNSPECIFIED. ) ;
#1633=LINE ( 'NONE', #43054, #36096 ) ;
#1634=ORIENTED_EDGE ( 'NONE', *, *, #88902, .T. ) ;
#1635=FACE_OUTER_BOUND ( 'NONE', #22221, .T. ) ;
#1636=CARTESIAN_POINT ( 'NONE',  ( 16.15384615384603251, -12.27809138561165270, 31.22303859784587132 ) ) ;
#1637=CARTESIAN_POINT ( 'NONE',  ( -8.899922235898330314, -11.18331474514187995, 33.13161551792790505 ) ) ;
#1638=CARTESIAN_POINT ( 'NONE',  ( 8.769230769230645706, -5.941354392335915335, 34.76329471203413846 ) ) ;
#1639=CARTESIAN_POINT ( 'NONE',  ( -16.40386939113911779, -10.76384336483936011, 33.53834819971076087 ) ) ;
#1640=CARTESIAN_POINT ( 'NONE',  ( -3.164701897419154975, -5.471508081941601098, 34.59228464037088457 ) ) ;
#1641=CYLINDRICAL_SURFACE ( 'NONE', #77982, 0.2499999999999995559 ) ;
#1642=VECTOR ( 'NONE', #82692, 1000.000000000000114 ) ;
#1643=ORIENTED_EDGE ( 'NONE', *, *, #71969, .F. ) ;
#1644=ORIENTED_EDGE ( 'NONE', *, *, #35630, .T. ) ;
#1645=VERTEX_POINT ( 'NONE', #64756 ) ;
#1646=VECTOR ( 'NONE', #7114, 1000.000000000000227 ) ;
#1647=DIRECTION ( 'NONE',  ( -0.000000000000000000, -0.6427876096865404731, -0.7660444431189770143 ) ) ;
#1648=DIRECTION ( 'NONE',  ( 0.000000000000000000, 0.3420201433256610524, 0.9396926207859113145 ) ) ;
#1649=CARTESIAN_POINT ( 'NONE',  ( 6.699591998512590685, -3.019605429927184836, 32.48692288466676814 ) ) ;
#1650=DIRECTION ( 'NONE',  ( -0.000000000000000000, 0.3420201433256694901, -0.9396926207859082059 ) ) ;
#1651=CARTESIAN_POINT ( 'NONE',  ( 17.86930939688969033, -9.084618155246140248, 34.75535874321725771 ) ) ;
#1653=DIRECTION ( 'NONE',  ( -0.000000000000000000, -0.6427876096865404731, -0.7660444431189771253 ) ) ;
#1655=ORIENTED_EDGE ( 'NONE', *, *, #17163, .F. ) ;
#1656=ORIENTED_EDGE ( 'NONE', *, *, #23547, .T. ) ;
#1657=CARTESIAN_POINT ( 'NONE',  ( 8.703148389870630552, -12.34228464037088280, 31.77849191805838558 ) ) ;
#1658=ORIENTED_EDGE ( 'NONE', *, *, #86170, .F. ) ;
#1659=DIRECTION ( 'NONE',  ( -0.000000000000000000, -0.9848077530122085754, -0.1736481776669273613 ) ) ;
#1660=CARTESIAN_POINT ( 'NONE',  ( -10.61538461538461320, -4.786620604624113540, 33.94971097300155094 ) ) ;
#1661=CARTESIAN_POINT ( 'NONE',  ( -9.915792636031639518, -8.496056993536548418, 34.65000542017679663 ) ) ;
#1662=ORIENTED_EDGE ( 'NONE', *, *, #56806, .T. ) ;
#1663=EDGE_LOOP ( 'NONE', ( #25110, #61996, #65349, #45435 ) ) ;
#1665=CARTESIAN_POINT ( 'NONE',  ( -14.08426534583073675, -7.630147231320743018, 34.74852402298682819 ) ) ;
#1666=DIRECTION ( 'NONE',  ( -0.000000000000000000, 0.6427876096865404731, -0.7660444431189770143 ) ) ;
#1667=ORIENTED_EDGE ( 'NONE', *, *, #53635, .T. ) ;
#1668=CARTESIAN_POINT ( 'NONE',  ( -0.4615384615384611200, -1.367168528481310208, 33.57946703557072254 ) ) ;
#1670=CARTESIAN_POINT ( 'NONE',  ( -2.980714919130914353, -9.943054286541407549, 34.11300777759954883 ) ) ;
#1671=EDGE_LOOP ( 'NONE', ( #37476, #13300, #1227, #9317 ) ) ;
#1672=VECTOR ( 'NONE', #82272, 999.9999999999998863 ) ;
#1673=CARTESIAN_POINT ( 'NONE',  ( -11.40793583669797684, -5.195472089885680766, 34.18748526763464923 ) ) ;
#1674=CARTESIAN_POINT ( 'NONE',  ( -5.999999999999998224, -2.833524468853757305, 32.15551576947925838 ) ) ;
#1676=FACE_BOUND ( 'NONE', #75859, .T. ) ;
#1677=CARTESIAN_POINT ( 'NONE',  ( -10.74553258511630993, -5.070767119584671079, 34.40440758774516183 ) ) ;
#1678=CARTESIAN_POINT ( 'NONE',  ( -17.07692307692307665, -3.050289026998446396, 32.03036669348365706 ) ) ;
#1680=CYLINDRICAL_SURFACE ( 'NONE', #72480, 0.2500000000000008882 ) ;
#1681=B_SPLINE_CURVE_WITH_KNOTS ( 'NONE', 3,
 ( #73432, #31089, #24332, #45942, #18042, #11278, #45499, #87402, #66668, #38752 ),
 .UNSPECIFIED., .F., .F.,
 ( 4, 2, 2, 2, 4 ),
 ( 0.000000000000000000, 0.0001954311564186867931, 0.0003908623128373735862, 0.0005862934692560603251, 0.0007817246256747471724 ),
 .UNSPECIFIED. ) ;
#1683=CARTESIAN_POINT ( 'NONE',  ( 14.98076923076923173, -2.249999999999998668, 29.75000000000000355 ) ) ;
#1684=CARTESIAN_POINT ( 'NONE',  ( 6.923076923076924238, -2.249999999999998668, 29.50000000000001421 ) ) ;
#1685=CARTESIAN_POINT ( 'NONE',  ( 18.13052570176355971, -2.882268652242222728, 31.66798894389554064 ) ) ;
#1686=VERTEX_POINT ( 'NONE', #44482 ) ;
#1687=CARTESIAN_POINT ( 'NONE',  ( -11.28851602011339494, -12.22109172314383052, 31.39792113162168263 ) ) ;
#1688=DIRECTION ( 'NONE',  ( 0.000000000000000000, 0.4999999999999960032, -0.8660254037844410391 ) ) ;
#1689=B_SPLINE_CURVE_WITH_KNOTS ( 'NONE', 3,
 ( #61294, #52771, #87937, #88811, #46902, #80261, #18558, #12240, #54544, #47797 ),
 .UNSPECIFIED., .F., .F.,
 ( 4, 2, 2, 2, 4 ),
 ( 0.0007817246256747455461, 0.0009771112852218883336, 0.001172497944769031230, 0.001367884604316174126, 0.001563271263863317022 ),
 .UNSPECIFIED. ) ;
#1690=VERTEX_POINT ( 'NONE', #11615 ) ;
#1691=CARTESIAN_POINT ( 'NONE',  ( -16.28399412357785536, -12.70455904226513866, 30.44083106164009322 ) ) ;
#1692=CARTESIAN_POINT ( 'NONE',  ( -14.17690186672535901, -9.084667340241226796, 34.75534355489798344 ) ) ;
#1693=CARTESIAN_POINT ( 'NONE',  ( 2.980769230769232614, -7.433931650972300353, 34.75000000000000711 ) ) ;
#1694=CARTESIAN_POINT ( 'NONE',  ( 2.177001704582000485, -5.496505350115500121, 34.60290016733514307 ) ) ;
#1695=CARTESIAN_POINT ( 'NONE',  ( -0.2385271099256124072, -12.39991518177334129, 30.74647679643404530 ) ) ;
#1696=DIRECTION ( 'NONE',  ( -0.000000000000000000, 1.000000000000000000, 3.491481338843133355E-15 ) ) ;
#1697=FACE_BOUND ( 'NONE', #74741, .T. ) ;
#1698=CARTESIAN_POINT ( 'NONE',  ( 13.25392478150507891, -2.295517848115769421, 30.44137282052137294 ) ) ;
#1699=CARTESIAN_POINT ( 'NONE',  ( 15.36129493253279499, -12.27024696741798770, 31.24895572276497546 ) ) ;
#1700=EDGE_CURVE ( 'NONE', #10997, #441, #68954, .T. ) ;
#1701=CARTESIAN_POINT ( 'NONE',  ( -16.15384615384615330, -2.538708090699994813, 30.37095296980875503 ) ) ;
#1702=CARTESIAN_POINT ( 'NONE',  ( -6.700064078983529292, -10.77377354290276301, 33.85451476688484718 ) ) ;
#1703=CARTESIAN_POINT ( 'NONE',  ( -12.68446467905460828, -4.186968288167449259, 33.49512374952580274 ) ) ;
#1706=VERTEX_POINT ( 'NONE', #4864 ) ;
#1707=VECTOR ( 'NONE', #20948, 1000.000000000000114 ) ;
#1709=CARTESIAN_POINT ( 'NONE',  ( -9.692307692307812417, -11.94971097300221174, 32.03036669348237098 ) ) ;
#1710=CARTESIAN_POINT ( 'NONE',  ( -0.4615384615385826339, -2.892918686052166066, 31.69288490824153470 ) ) ;
#1711=CARTESIAN_POINT ( 'NONE',  ( -9.442362173959551797, -9.272278438253398036, 34.42582936511637115 ) ) ;
#1712=LINE ( 'NONE', #82812, #61063 ) ;
#1713=CARTESIAN_POINT ( 'NONE',  ( -17.07692307692307665, -6.386643153685126251, 34.62446782046654192 ) ) ;
#1715=VECTOR ( 'NONE', #28103, 1000.000000000000227 ) ;
#1716=CARTESIAN_POINT ( 'NONE',  ( 0.5276057948885357618, -3.937682226553329556, 33.60647404775216529 ) ) ;
#1717=CARTESIAN_POINT ( 'NONE',  ( 3.930919194939304973, -11.98009711892699691, 32.48740034544075428 ) ) ;
#1718=CARTESIAN_POINT ( 'NONE',  ( 15.48071474911737333, -11.86320923018887719, 32.19269448109604070 ) ) ;
#1719=CARTESIAN_POINT ( 'NONE',  ( 17.86930939688969033, -8.191372820521381826, 34.95448215188423546 ) ) ;
#1720=CARTESIAN_POINT ( 'NONE',  ( -3.361459833879539616, -3.957541250942359756, 33.62499894934981626 ) ) ;
#1721=DIRECTION ( 'NONE',  ( -0.000000000000000000, -0.9848077530122086864, -0.1736481776669273613 ) ) ;
#1722=ADVANCED_FACE ( 'NONE', ( #66096 ), #85492, .F. ) ;
#1723=ADVANCED_FACE ( 'NONE', ( #71972 ), #59347, .F. ) ;
#1724=CARTESIAN_POINT ( 'NONE',  ( 12.59206389977210705, -2.372941743896879174, 30.88044141588253666 ) ) ;
#1725=DIRECTION ( 'NONE',  ( 0.000000000000000000, 0.000000000000000000, 1.000000000000000000 ) ) ;
#1726=VERTEX_POINT ( 'NONE', #86402 ) ;
#1727=CARTESIAN_POINT ( 'NONE',  ( 2.177544337960614751, -3.625366637846545448, 33.29286588640298561 ) ) ;
#1728=CARTESIAN_POINT ( 'NONE',  ( 10.68145194873469173, -5.471508081941601098, 34.59228464037088457 ) ) ;
#1730=CARTESIAN_POINT ( 'NONE',  ( 4.023698184114456566, -5.070767119584671079, 34.40440758774516183 ) ) ;
#1732=EDGE_LOOP ( 'NONE', ( #67383, #34344 ) ) ;
#1735=ORIENTED_EDGE ( 'NONE', *, *, #61774, .F. ) ;
#1736=DIRECTION ( 'NONE',  ( 0.000000000000000000, 0.6427876096865368094, 0.7660444431189802339 ) ) ;
#1737=CARTESIAN_POINT ( 'NONE',  ( -2.307692307692305711, -2.499999999999998668, 29.50000000000001066 ) ) ;
#1739=ORIENTED_EDGE ( 'NONE', *, *, #13994, .F. ) ;
#1740=DIRECTION ( 'NONE',  ( 0.000000000000000000, 0.6427876096865373645, -0.7660444431189797898 ) ) ;
#1741=DIRECTION ( 'NONE',  ( -0.000000000000000000, -0.9396926207859092051, -0.3420201433256662704 ) ) ;
#1742=ORIENTED_EDGE ( 'NONE', *, *, #3228, .T. ) ;
#1743=VECTOR ( 'NONE', #59624, 1000.000000000000000 ) ;
#1744=CARTESIAN_POINT ( 'NONE',  ( 9.019176178608812933, -2.341251567377310217, 30.72681386836322659 ) ) ;
#1745=CARTESIAN_POINT ( 'NONE',  ( -11.60454391782167605, -12.34228464037088280, 31.77849191805838558 ) ) ;
#1746=CARTESIAN_POINT ( 'NONE',  ( -15.16470087976679437, -12.37446782046654192, 30.86335684631486842 ) ) ;
#1748=VECTOR ( 'NONE', #2612, 1000.000000000000227 ) ;
#1749=ORIENTED_EDGE ( 'NONE', *, *, #53727, .T. ) ;
#1750=VERTEX_POINT ( 'NONE', #88187 ) ;
#1751=CARTESIAN_POINT ( 'NONE',  ( 15.29602437028206907, -12.70778746994558439, 30.41441678777536595 ) ) ;
#1753=CARTESIAN_POINT ( 'NONE',  ( -3.100243792535585907, -8.630441415882550871, 34.87705825610312615 ) ) ;
#1754=CARTESIAN_POINT ( 'NONE',  ( -17.29984929443922681, -6.503392248772476236, 34.64988816332204635 ) ) ;
#1755=ORIENTED_EDGE ( 'NONE', *, *, #16817, .F. ) ;
#1756=EDGE_LOOP ( 'NONE', ( #66255, #3639 ) ) ;
#1757=CARTESIAN_POINT ( 'NONE',  ( -2.557692307692305711, -7.433932668274255029, 35.00000000000000711 ) ) ;
#1758=EDGE_LOOP ( 'NONE', ( #66722, #50817 ) ) ;
#1760=AXIS2_PLACEMENT_3D ( 'NONE', #26968, #48544, #74267 ) ;
#1761=ORIENTED_EDGE ( 'NONE', *, *, #17169, .F. ) ;
#1762=AXIS2_PLACEMENT_3D ( 'NONE', #5424, #67570, #87866 ) ;
#1763=CYLINDRICAL_SURFACE ( 'NONE', #47856, 0.2499999999999994726 ) ;
#1764=CARTESIAN_POINT ( 'NONE',  ( 6.923076923076924238, -9.058645607665452459, 34.76329471203371924 ) ) ;
#1765=ORIENTED_EDGE ( 'NONE', *, *, #75906, .T. ) ;
#1766=CARTESIAN_POINT ( 'NONE',  ( 7.976945653978629203, -8.147973898785416225, 34.70805048591653730 ) ) ;
#1767=VECTOR ( 'NONE', #11156, 1000.000000000000114 ) ;
#1768=EDGE_CURVE ( 'NONE', #63242, #45204, #39547, .T. ) ;
#1769=ORIENTED_EDGE ( 'NONE', *, *, #79116, .T. ) ;
#1771=VERTEX_POINT ( 'NONE', #19696 ) ;
#1772=CARTESIAN_POINT ( 'NONE',  ( -5.776988648387149539, -8.239487800360276282, 34.69522927552633718 ) ) ;
#1773=B_SPLINE_CURVE_WITH_KNOTS ( 'NONE', 3,
 ( #52051, #9740, #86313, #17843, #71431, #85852, #37206, #58357, #24135, #31801 ),
 .UNSPECIFIED., .F., .F.,
 ( 4, 2, 2, 2, 4 ),
 ( 0.000000000000000000, 0.0001954311564186862781, 0.0003908623128373725562, 0.0005862934692560588072, 0.0007817246256747451124 ),
 .UNSPECIFIED. ) ;
#1776=CARTESIAN_POINT ( 'NONE',  ( 15.48082354240754555, -3.136992222400443175, 32.19305428654138979 ) ) ;
#1777=CARTESIAN_POINT ( 'NONE',  ( 6.673100179028331524, -5.643011162660950042, 34.66104346484419096 ) ) ;
#1778=FACE_BOUND ( 'NONE', #27909, .T. ) ;
#1779=CARTESIAN_POINT ( 'NONE',  ( -9.626240358957616650, -3.937682226553329556, 33.60647404775216529 ) ) ;
#1780=FACE_OUTER_BOUND ( 'NONE', #5751, .T. ) ;
#1781=EDGE_CURVE ( 'NONE', #18284, #20058, #26459, .T. ) ;
#1782=CARTESIAN_POINT ( 'NONE',  ( 15.36129466900287177, -2.647132371071621471, 31.75357179365171589 ) ) ;
#1783=DIRECTION ( 'NONE',  ( -0.000000000000000000, -0.9396926207859093161, -0.3420201433256663259 ) ) ;
#1784=CARTESIAN_POINT ( 'NONE',  ( -11.47320596718551045, -3.300289026998473041, 32.46337939537591666 ) ) ;
#1785=CARTESIAN_POINT ( 'NONE',  ( 10.36540787133602670, -10.82459398097509329, 33.81372124010185587 ) ) ;
#1786=ORIENTED_EDGE ( 'NONE', *, *, #69158, .F. ) ;
#1787=CARTESIAN_POINT ( 'NONE',  ( 14.43848274865925774, -6.369690395747422684, 34.87708834333098196 ) ) ;
#1788=EDGE_CURVE ( 'NONE', #86079, #14268, #87289, .T. ) ;
#1789=EDGE_LOOP ( 'NONE', ( #33863, #68262, #3065, #56633 ) ) ;
#1790=VERTEX_POINT ( 'NONE', #25566 ) ;
#1791=CARTESIAN_POINT ( 'NONE',  ( 7.780070435197965928, -6.386643153685125363, 34.62446782046654903 ) ) ;
#1792=CYLINDRICAL_SURFACE ( 'NONE', #37614, 0.2500000000000008882 ) ;
#1793=VECTOR ( 'NONE', #32508, 1000.000000000000114 ) ;
#1794=CARTESIAN_POINT ( 'NONE',  ( -11.78843826940389405, -11.79746400365624659, 32.30657167506340954 ) ) ;
#1795=CARTESIAN_POINT ( 'NONE',  ( 8.068933515131911705, -3.563462043263030399, 33.22394488606062879 ) ) ;
#1796=CARTESIAN_POINT ( 'NONE',  ( -13.38461538461538325, -7.500000000000001776, 35.04278698407183867 ) ) ;
#1797=CARTESIAN_POINT ( 'NONE',  ( -0.3962828902624368488, -11.94971097300157403, 32.03036669348361443 ) ) ;
#1798=EDGE_LOOP ( 'NONE', ( #62360, #54900, #10023, #7450 ) ) ;
#1799=DIRECTION ( 'NONE',  ( -0.000000000000000000, 1.000000000000000000, 3.491481338843133355E-15 ) ) ;
#1800=CARTESIAN_POINT ( 'NONE',  ( -6.222926217516143055, -6.503392248772476236, 34.64988816332204635 ) ) ;
#1801=CARTESIAN_POINT ( 'NONE',  ( -10.55012904410859242, -10.21337939537593620, 33.94971097300152252 ) ) ;
#1803=CYLINDRICAL_SURFACE ( 'NONE', #35245, 0.2499999999999979738 ) ;
#1804=CARTESIAN_POINT ( 'NONE',  ( 13.44987052412822237, -5.941354392334607049, 34.76329471203374055 ) ) ;
#1806=ORIENTED_EDGE ( 'NONE', *, *, #680, .T. ) ;
#1807=ORIENTED_EDGE ( 'NONE', *, *, #77572, .T. ) ;
#1808=EDGE_CURVE ( 'NONE', #85122, #71718, #29245, .T. ) ;
#1809=CARTESIAN_POINT ( 'NONE',  ( -9.627052121031665521, -12.46129190930001052, 30.37095296980870174 ) ) ;
#1810=ORIENTED_EDGE ( 'NONE', *, *, #17759, .T. ) ;
#1811=CARTESIAN_POINT ( 'NONE',  ( -9.758391103263571509, -12.37446782046654192, 30.86335684631486487 ) ) ;
#1812=CARTESIAN_POINT ( 'NONE',  ( -1.254089946381739651, -10.31582465632705237, 34.18122507451815295 ) ) ;
#1814=CARTESIAN_POINT ( 'NONE',  ( 2.530705151785703322, -10.01129605718032778, 34.36064277460058491 ) ) ;
#1816=B_SPLINE_CURVE_WITH_KNOTS ( 'NONE', 3,
 ( #35621, #78701, #71487, #16997, #57977, #63069 ),
 .UNSPECIFIED., .F., .F.,
 ( 4, 2, 4 ),
 ( 0.000000000000000000, 0.0001954784845028921395, 0.0003909569690057842790 ),
 .UNSPECIFIED. ) ;
#1817=CYLINDRICAL_SURFACE ( 'NONE', #60375, 0.2499999999999973355 ) ;
#1818=EDGE_LOOP ( 'NONE', ( #71715, #13718 ) ) ;
#1819=CARTESIAN_POINT ( 'NONE',  ( -12.52680890749923570, -10.90142922261923886, 33.41473453929638993 ) ) ;
#1820=CARTESIAN_POINT ( 'NONE',  ( -16.37733109757010297, -11.89387501736623420, 32.13663884655804992 ) ) ;
#1821=ORIENTED_EDGE ( 'NONE', *, *, #64204, .F. ) ;
#1822=DIRECTION ( 'NONE',  ( -0.000000000000000000, 0.9396926207859092051, -0.3420201433256662704 ) ) ;
#1823=CARTESIAN_POINT ( 'NONE',  ( -0.7115616857599181833, -4.175268141568689195, 33.81360843649122216 ) ) ;
#1824=B_SPLINE_CURVE_WITH_KNOTS ( 'NONE', 3,
 ( #47501, #47943, #63232, #48832, #20481, #76760, #40763, #42097, #76306, #14612 ),
 .UNSPECIFIED., .F., .F.,
 ( 4, 2, 2, 2, 4 ),
 ( 0.0007817246256747434861, 0.0009771112852218861652, 0.001172497944769028844, 0.001367884604316171740, 0.001563271263863314419 ),
 .UNSPECIFIED. ) ;
#1825=CARTESIAN_POINT ( 'NONE',  ( -17.86947429823643674, -11.93748526763465279, 32.05452791011430946 ) ) ;
#1826=CARTESIAN_POINT ( 'NONE',  ( -16.15384615384615330, -2.292212530054420494, 30.41441678777542634 ) ) ;
#1827=EDGE_CURVE ( 'NONE', #50611, #13813, #56027, .T. ) ;
#1828=FACE_OUTER_BOUND ( 'NONE', #30091, .T. ) ;
#1831=VERTEX_POINT ( 'NONE', #6188 ) ;
#1833=DIRECTION ( 'NONE',  ( -0.000000000000000000, 1.000000000000000000, 3.491481338843133355E-15 ) ) ;
#1836=AXIS2_PLACEMENT_3D ( 'NONE', #49620, #77094, #64004 ) ;
#1837=EDGE_CURVE ( 'NONE', #20157, #51126, #54917, .T. ) ;
#1838=CARTESIAN_POINT ( 'NONE',  ( -13.51476259405360203, -12.45813303252208648, 30.39737893381572675 ) ) ;
#1840=EDGE_CURVE ( 'NONE', #36102, #52068, #59942, .T. ) ;
#1841=ORIENTED_EDGE ( 'NONE', *, *, #10731, .F. ) ;
#1843=CARTESIAN_POINT ( 'NONE',  ( -16.15384615384615330, -4.945431358278436385, 36.03766855953609394 ) ) ;
#1844=AXIS2_PLACEMENT_3D ( 'NONE', #65328, #85609, #43296 ) ;
#1845=ORIENTED_EDGE ( 'NONE', *, *, #82568, .T. ) ;
#1846=CARTESIAN_POINT ( 'NONE',  ( 6.923076923076924238, -2.499999999999998668, 29.50000000000001066 ) ) ;
#1847=FACE_OUTER_BOUND ( 'NONE', #20720, .T. ) ;
#1848=ORIENTED_EDGE ( 'NONE', *, *, #4862, .T. ) ;
#1849=DIRECTION ( 'NONE',  ( 0.000000000000000000, 0.9848077530122072432, 0.1736481776669354937 ) ) ;
#1850=CARTESIAN_POINT ( 'NONE',  ( -5.869954837165220596, -2.504778602574660340, 29.97347330155780298 ) ) ;
#1851=CARTESIAN_POINT ( 'NONE',  ( -12.59222906464877134, -9.929715669179220328, 34.40415004197138416 ) ) ;
#1852=CARTESIAN_POINT ( 'NONE',  ( -13.25382494364843389, -12.62708834333097663, 30.88030960425257021 ) ) ;
#1853=ORIENTED_EDGE ( 'NONE', *, *, #14845, .F. ) ;
#1854=CARTESIAN_POINT ( 'NONE',  ( -8.899790682844132661, -2.254533558242299396, 29.97296025877828285 ) ) ;
#1855=EDGE_LOOP ( 'NONE', ( #17903, #9416, #24823, #13466 ) ) ;
#1857=CARTESIAN_POINT ( 'NONE',  ( -10.68065506134539078, -2.892918686051582977, 31.69288490824015980 ) ) ;
#1858=ORIENTED_EDGE ( 'NONE', *, *, #32430, .F. ) ;
#1859=B_SPLINE_CURVE_WITH_KNOTS ( 'NONE', 3,
 ( #73875, #12173, #32884, #87859, #26125, #81084, #12618, #73265, #65162, #79134 ),
 .UNSPECIFIED., .F., .F.,
 ( 4, 2, 2, 2, 4 ),
 ( 0.000000000000000000, 0.0001954339857564081249, 0.0003908679715128162498, 0.0005863019572692244018, 0.0007817359430256324996 ),
 .UNSPECIFIED. ) ;
#1860=CARTESIAN_POINT ( 'NONE',  ( -6.066082379360134169, -10.67929555188718460, 33.92786785259543336 ) ) ;
#1862=CARTESIAN_POINT ( 'NONE',  ( 0.2115152242454955700, -4.335965774309649134, 33.62209801155880484 ) ) ;
#1864=DIRECTION ( 'NONE',  ( 0.000000000000000000, 0.7660444431189807890, 0.6427876096865361433 ) ) ;
#1866=ADVANCED_FACE ( 'NONE', ( #31277 ), #73617, .F. ) ;
#1867=VERTEX_POINT ( 'NONE', #4701 ) ;
#1868=VERTEX_POINT ( 'NONE', #59188 ) ;
#1869=FACE_BOUND ( 'NONE', #86958, .T. ) ;
#1870=VERTEX_POINT ( 'NONE', #3351 ) ;
#1871=CARTESIAN_POINT ( 'NONE',  ( 8.703147358274884837, -3.513871655860377086, 32.76840700105978499 ) ) ;
#1872=EDGE_CURVE ( 'NONE', #31746, #72998, #36661, .T. ) ;
#1873=CARTESIAN_POINT ( 'NONE',  ( 17.07692307692295586, -12.51329471203414379, 31.30864560766407578 ) ) ;
#1874=CARTESIAN_POINT ( 'NONE',  ( 6.250054419913455561, -2.920487667080175154, 32.31805714834170828 ) ) ;
#1875=CARTESIAN_POINT ( 'NONE',  ( -14.08468095607945614, -9.086983370893049639, 34.49168942202179267 ) ) ;
#1876=ORIENTED_EDGE ( 'NONE', *, *, #17283, .T. ) ;
#1879=VERTEX_POINT ( 'NONE', #4247 ) ;
#1880=CARTESIAN_POINT ( 'NONE',  ( -9.692307692307691624, -12.09954503811598769, 35.62045528018868623 ) ) ;
#1881=ORIENTED_EDGE ( 'NONE', *, *, #87497, .T. ) ;
#1882=CARTESIAN_POINT ( 'NONE',  ( 13.31934493865461278, -2.892918686051582533, 31.69288490824015980 ) ) ;
#1883=CARTESIAN_POINT ( 'NONE',  ( -2.307692307692305711, -12.34228464037088635, 31.77849191805839268 ) ) ;
#1884=B_SPLINE_CURVE_WITH_KNOTS ( 'NONE', 3,
 ( #85158, #23443, #50897, #30646, #36533, #84289, #9933, #36095, #30217, #23008 ),
 .UNSPECIFIED., .F., .F.,
 ( 4, 2, 2, 2, 4 ),
 ( 0.0007817246256747453293, 0.0009771112852218889842, 0.001172497944769032531, 0.001367884604316176294, 0.001563271263863319840 ),
 .UNSPECIFIED. ) ;
#1885=CARTESIAN_POINT ( 'NONE',  ( -17.07692307692319744, -3.083524468854526912, 32.58852847137268327 ) ) ;
#1886=ORIENTED_EDGE ( 'NONE', *, *, #25312, .F. ) ;
#1887=CARTESIAN_POINT ( 'NONE',  ( -8.769230769230768274, -3.937682226553329556, 33.60647404775216529 ) ) ;
#1889=EDGE_CURVE ( 'NONE', #12525, #14877, #53795, .T. ) ;
#1890=CARTESIAN_POINT ( 'NONE',  ( 2.557692307692308376, -2.499999999999998668, 29.75000000000000355 ) ) ;
#1891=CARTESIAN_POINT ( 'NONE',  ( -17.75000000000000355, -7.500000000000000000, 35.00000000000000000 ) ) ;
#1893=EDGE_LOOP ( 'NONE', ( #21618, #11266 ) ) ;
#1894=EDGE_CURVE ( 'NONE', #16582, #12053, #65499, .T. ) ;
#1895=EDGE_LOOP ( 'NONE', ( #86192, #47505, #21474, #23869 ) ) ;
#1896=ORIENTED_EDGE ( 'NONE', *, *, #35482, .F. ) ;
#1897=CARTESIAN_POINT ( 'NONE',  ( -3.903791842207835483, -9.943054286541407549, 34.11300777759954883 ) ) ;
#1899=CARTESIAN_POINT ( 'NONE',  ( 10.36536139116315880, -2.341070481393819236, 30.72580821765574299 ) ) ;
#1900=DIRECTION ( 'NONE',  ( -0.000000000000000000, -0.3420201433256694901, -0.9396926207859082059 ) ) ;
#1901=CARTESIAN_POINT ( 'NONE',  ( -2.241624974342231624, -2.486705287966280320, 31.30864560766543647 ) ) ;
#1902=FACE_BOUND ( 'NONE', #3198, .T. ) ;
#1903=CARTESIAN_POINT ( 'NONE',  ( 16.21910172512217585, -3.300289026998473929, 32.46337939537591666 ) ) ;
#1904=EDGE_LOOP ( 'NONE', ( #76502, #22251 ) ) ;
#1905=CARTESIAN_POINT ( 'NONE',  ( -18.00000000000012079, -12.46129190930018460, 30.37095296980731973 ) ) ;
#1906=CYLINDRICAL_SURFACE ( 'NONE', #2779, 0.2499999999999997502 ) ;
#1907=DIRECTION ( 'NONE',  ( -0.000000000000000000, -0.3420201433256694346, -0.9396926207859080948 ) ) ;
#1909=CARTESIAN_POINT ( 'NONE',  ( 3.230769230769231726, -11.35647404775217417, 33.31231777344666511 ) ) ;
#1910=ORIENTED_EDGE ( 'NONE', *, *, #27758, .F. ) ;
#1911=CARTESIAN_POINT ( 'NONE',  ( 6.130525438233645374, -11.04252011169590020, 33.62494198852677130 ) ) ;
#1912=B_SPLINE_CURVE_WITH_KNOTS ( 'NONE', 3,
 ( #25401, #38926, #65032, #3343, #72245, #18656, #10556, #24949, #32163, #79902 ),
 .UNSPECIFIED., .F., .F.,
 ( 4, 2, 2, 2, 4 ),
 ( 0.000000000000000000, 0.0001954339857564086670, 0.0003908679715128173340, 0.0005863019572692260281, 0.0007817359430256346680 ),
 .UNSPECIFIED. ) ;
#1913=VERTEX_POINT ( 'NONE', #65040 ) ;
#1914=FACE_BOUND ( 'NONE', #68021, .T. ) ;
#1915=CARTESIAN_POINT ( 'NONE',  ( 4.853438133199126980, -5.912607949931405038, 34.49155766932282319 ) ) ;
#1916=B_SPLINE_CURVE_WITH_KNOTS ( 'NONE', 3,
 ( #48411, #55613, #75019, #13747, #33586, #61924, #53848, #81335, #237, #76332 ),
 .UNSPECIFIED., .F., .F.,
 ( 4, 2, 2, 2, 4 ),
 ( 0.0007817359430256257775, 0.0009771253907249911191, 0.001172514838424356352, 0.001367904286123721586, 0.001563293733823086819 ),
 .UNSPECIFIED. ) ;
#1917=CARTESIAN_POINT ( 'NONE',  ( 4.376858997939548246, -2.523321265292115090, 31.42251411153756280 ) ) ;
#1918=CARTESIAN_POINT ( 'NONE',  ( 14.17700084102475699, -11.71456829005830080, 32.44064028649416542 ) ) ;
#1919=ORIENTED_EDGE ( 'NONE', *, *, #26185, .T. ) ;
#1920=FACE_OUTER_BOUND ( 'NONE', #21485, .T. ) ;
#1921=CARTESIAN_POINT ( 'NONE',  ( -18.00000000000012079, -2.892918686052166066, 31.69288490824153470 ) ) ;
#1922=LINE ( 'NONE', #43789, #4961 ) ;
#1923=CARTESIAN_POINT ( 'NONE',  ( -5.011667937410237528, -5.941354392334606160, 34.76329471203374055 ) ) ;
#1924=ORIENTED_EDGE ( 'NONE', *, *, #49393, .T. ) ;
#1925=CARTESIAN_POINT ( 'NONE',  ( -7.846153846153965716, -10.90142922262034020, 33.41473453929536674 ) ) ;
#1927=ORIENTED_EDGE ( 'NONE', *, *, #17655, .T. ) ;
#1928=B_SPLINE_CURVE_WITH_KNOTS ( 'NONE', 3,
 ( #77028, #48655, #42807, #84242, #29291, #56747, #9016, #36484, #76131, #63937 ),
 .UNSPECIFIED., .F., .F.,
 ( 4, 2, 2, 2, 4 ),
 ( 0.0007817246256747524850, 0.0009771112852218972241, 0.001172497944769042072, 0.001367884604316186702, 0.001563271263863331550 ),
 .UNSPECIFIED. ) ;
#1929=CARTESIAN_POINT ( 'NONE',  ( 13.51514108637895184, -12.27024696741798770, 31.24895572276497546 ) ) ;
#1930=VECTOR ( 'NONE', #5639, 999.9999999999998863 ) ;
#1931=EDGE_LOOP ( 'NONE', ( #9396, #65765, #83074, #80289 ) ) ;
#1932=CARTESIAN_POINT ( 'NONE',  ( 7.623227628637700093, -10.61292498521070549, 33.66303323003028680 ) ) ;
#1933=CARTESIAN_POINT ( 'NONE',  ( -10.61538461538473399, -12.46129190930018460, 30.37095296980731973 ) ) ;
#1934=B_SPLINE_CURVE_WITH_KNOTS ( 'NONE', 3,
 ( #45267, #12385, #24556, #39866, #66885, #31774, #11501, #5182, #72298, #72739 ),
 .UNSPECIFIED., .F., .F.,
 ( 4, 2, 2, 2, 4 ),
 ( 0.0007817246256747521597, 0.0009771112852218961399, 0.001172497944769040337, 0.001367884604316184534, 0.001563271263863328514 ),
 .UNSPECIFIED. ) ;
#1935=CARTESIAN_POINT ( 'NONE',  ( 4.153846153846154188, -11.11383981884818262, 36.00935417666054406 ) ) ;
#1936=CARTESIAN_POINT ( 'NONE',  ( -12.23852710992561477, -2.758310577978207778, 31.33698337089302299 ) ) ;
#1937=CARTESIAN_POINT ( 'NONE',  ( -8.069638789877792817, -10.81261337010820256, 33.49550067578627477 ) ) ;
#1938=CARTESIAN_POINT ( 'NONE',  ( -11.60454391782167427, -9.058645607665454236, 34.76329471203372634 ) ) ;
#1939=ADVANCED_FACE ( 'NONE', ( #85784 ), #24958, .F. ) ;
#1940=DIRECTION ( 'NONE',  ( -0.000000000000000000, 0.9396926207859092051, -0.3420201433256662704 ) ) ;
#1942=EDGE_LOOP ( 'NONE', ( #7971, #37007, #50893, #53738 ) ) ;
#1943=FACE_OUTER_BOUND ( 'NONE', #30824, .T. ) ;
#1945=VERTEX_POINT ( 'NONE', #79016 ) ;
#1946=EDGE_CURVE ( 'NONE', #68769, #43616, #52426, .T. ) ;
#1947=VERTEX_POINT ( 'NONE', #17771 ) ;
#1948=EDGE_CURVE ( 'NONE', #49139, #78712, #8756, .T. ) ;
#1949=ORIENTED_EDGE ( 'NONE', *, *, #22741, .T. ) ;
#1950=CARTESIAN_POINT ( 'NONE',  ( 10.74591005361826390, -8.630441415882550871, 34.87705825610312615 ) ) ;
#1951=CARTESIAN_POINT ( 'NONE',  ( -17.14300648787895653, -8.973038597847269315, 34.52809138561120506 ) ) ;
#1952=LINE ( 'NONE', #29437, #39934 ) ;
#1953=CARTESIAN_POINT ( 'NONE',  ( -5.076923076923197442, -3.835265460704628371, 33.15142922262033665 ) ) ;
#1954=CARTESIAN_POINT ( 'NONE',  ( -8.899378738962468560, -2.647304123082328875, 31.75400227202885972 ) ) ;
#1955=CARTESIAN_POINT ( 'NONE',  ( -8.899921372341079717, -2.845849958028613624, 32.17971566917920967 ) ) ;
#1956=FACE_OUTER_BOUND ( 'NONE', #49288, .T. ) ;
#1958=DIRECTION ( 'NONE',  ( 0.000000000000000000, 0.1736481776669267785, -0.9848077530122087975 ) ) ;
#1959=B_SPLINE_CURVE_WITH_KNOTS ( 'NONE', 3,
 ( #14843, #15279, #8522, #1754, #29244, #56697, #63889, #52146, #66104, #30114 ),
 .UNSPECIFIED., .F., .F.,
 ( 4, 2, 2, 2, 4 ),
 ( 0.000000000000000000, 0.0001954339857564075286, 0.0003908679715128150572, 0.0005863019572692225586, 0.0007817359430256301143 ),
 .UNSPECIFIED. ) ;
#1960=VECTOR ( 'NONE', #27474, 1000.000000000000000 ) ;
#1961=EDGE_CURVE ( 'NONE', #20256, #73637, #73203, .T. ) ;
#1962=CARTESIAN_POINT ( 'NONE',  ( 7.846153846153725020, -2.892918686052165622, 31.69288490824153470 ) ) ;
#1963=CARTESIAN_POINT ( 'NONE',  ( -5.076923076923075762, -1.422936976036506707, 30.56769352161908415 ) ) ;
#1965=VECTOR ( 'NONE', #10753, 1000.000000000000000 ) ;
#1966=ORIENTED_EDGE ( 'NONE', *, *, #12521, .T. ) ;
#1967=CARTESIAN_POINT ( 'NONE',  ( -17.07692307692307665, -2.486705287966279876, 31.30864560766543647 ) ) ;
#1968=CARTESIAN_POINT ( 'NONE',  ( 1.384615384615386802, -3.322132147404559976, 32.92929555188717927 ) ) ;
#1969=CARTESIAN_POINT ( 'NONE',  ( 3.361294669002873992, -11.04252011169590020, 33.62494198852677130 ) ) ;
#1971=CYLINDRICAL_SURFACE ( 'NONE', #11049, 0.2499999999999994726 ) ;
#1973=CARTESIAN_POINT ( 'NONE',  ( 12.23861224402230974, -9.086856451489515152, 34.49173150075333183 ) ) ;
#1974=DIRECTION ( 'NONE',  ( 0.000000000000000000, 1.000000000000000000, 0.000000000000000000 ) ) ;
#1975=CARTESIAN_POINT ( 'NONE',  ( -3.007989689500819352, -12.24180327182771855, 31.33663988360758168 ) ) ;
#1976=EDGE_CURVE ( 'NONE', #30954, #40782, #4423, .T. ) ;
#1977=ORIENTED_EDGE ( 'NONE', *, *, #13682, .T. ) ;
#1978=CARTESIAN_POINT ( 'NONE',  ( 0.6845498131513104711, -5.667800583137508674, 34.40243808032445827 ) ) ;
#1979=ORIENTED_EDGE ( 'NONE', *, *, #72545, .F. ) ;
#1981=CARTESIAN_POINT ( 'NONE',  ( 9.692307692307695177, -11.69971097300155272, 32.46337939537588113 ) ) ;
#1982=DIRECTION ( 'NONE',  ( -0.000000000000000000, 0.3420201433256694346, -0.9396926207859080948 ) ) ;
#1983=CARTESIAN_POINT ( 'NONE',  ( -6.249976730942354841, -2.564618984488975961, 30.55390908950641915 ) ) ;
#1984=B_SPLINE_CURVE_WITH_KNOTS ( 'NONE', 3,
 ( #56943, #77218, #15085, #14636, #42121, #8328, #29488, #76331, #77659, #15529 ),
 .UNSPECIFIED., .F., .F.,
 ( 4, 2, 2, 2, 4 ),
 ( 0.0007817246256747484735, 0.0009771112852218931041, 0.001172497944769037735, 0.001367884604316182365, 0.001563271263863326996 ),
 .UNSPECIFIED. ) ;
#1985=CARTESIAN_POINT ( 'NONE',  ( 12.46153846153846168, -1.466349020453238561, 30.81389545987213907 ) ) ;
#1986=DIRECTION ( 'NONE',  ( -0.000000000000000000, 0.9848077530122086864, -0.1736481776669273891 ) ) ;
#1987=VERTEX_POINT ( 'NONE', #88912 ) ;
#1988=EDGE_CURVE ( 'NONE', #62210, #30670, #7364, .T. ) ;
#1989=B_SPLINE_CURVE_WITH_KNOTS ( 'NONE', 3,
 ( #85951, #58027, #73326, #78743, #17045, #37755 ),
 .UNSPECIFIED., .F., .F.,
 ( 4, 2, 4 ),
 ( 0.0003909512603273880690, 0.0005862562993132132720, 0.0007815613382990384750 ),
 .UNSPECIFIED. ) ;
#1990=VECTOR ( 'NONE', #41020, 1000.000000000000227 ) ;
#1991=ORIENTED_EDGE ( 'NONE', *, *, #54747, .T. ) ;
#1993=EDGE_CURVE ( 'NONE', #27467, #75394, #77501, .T. ) ;
#1994=DIRECTION ( 'NONE',  ( -0.000000000000000000, 0.3420201433256694901, -0.9396926207859082059 ) ) ;
#1995=CYLINDRICAL_SURFACE ( 'NONE', #44502, 0.2499999999999994726 ) ;
#1996=CARTESIAN_POINT ( 'NONE',  ( 0.5267936010512989098, -6.835583212224609184, 34.95778746994559327 ) ) ;
#1997=CARTESIAN_POINT ( 'NONE',  ( -2.057746898314263273, -11.56426240980093567, 33.07394671870546432 ) ) ;
#1998=CARTESIAN_POINT ( 'NONE',  ( 7.623325748518968936, -7.369209533119140509, 34.99857337881830688 ) ) ;
#1999=CARTESIAN_POINT ( 'NONE',  ( -6.923076923077045919, -10.33852847137269571, 34.16647553114546554 ) ) ;
#2000=ORIENTED_EDGE ( 'NONE', *, *, #23568, .F. ) ;
#2001=EDGE_CURVE ( 'NONE', #45061, #56939, #12783, .T. ) ;
#2002=EDGE_LOOP ( 'NONE', ( #69498, #76017 ) ) ;
#2003=ORIENTED_EDGE ( 'NONE', *, *, #18087, .F. ) ;
#2004=CARTESIAN_POINT ( 'NONE',  ( -16.15384615384627409, -6.026961402154118908, 34.52809138561165270 ) ) ;
#2005=VERTEX_POINT ( 'NONE', #81253 ) ;
#2007=CARTESIAN_POINT ( 'NONE',  ( 8.834486340506792601, -8.613356846314928816, 34.62446782046653482 ) ) ;
#2008=CARTESIAN_POINT ( 'NONE',  ( -8.519176457592454454, -11.28795663066794575, 33.01431243580653785 ) ) ;
#2010=ORIENTED_EDGE ( 'NONE', *, *, #58469, .F. ) ;
#2011=ORIENTED_EDGE ( 'NONE', *, *, #85768, .T. ) ;
#2012=CARTESIAN_POINT ( 'NONE',  ( 5.011600161430901146, -7.749976743299137993, 34.99404534957040624 ) ) ;
#2013=VECTOR ( 'NONE', #80302, 1000.000000000000114 ) ;
#2014=ORIENTED_EDGE ( 'NONE', *, *, #10859, .F. ) ;
#2015=FACE_BOUND ( 'NONE', #70340, .T. ) ;
#2016=CARTESIAN_POINT ( 'NONE',  ( 3.480714640147272831, -2.589246495874657938, 31.60778113518102828 ) ) ;
#2017=CARTESIAN_POINT ( 'NONE',  ( -14.55769230769230660, -7.500000000000001776, 35.00000000000000000 ) ) ;
#2018=ORIENTED_EDGE ( 'NONE', *, *, #45523, .F. ) ;
#2019=CARTESIAN_POINT ( 'NONE',  ( 2.177000841024750777, -8.147922237126337563, 34.70805685702651999 ) ) ;
#2020=CARTESIAN_POINT ( 'NONE',  ( 3.480714749117372886, -3.202959910592335202, 32.30730279482227019 ) ) ;
#2021=CARTESIAN_POINT ( 'NONE',  ( -8.769230769230768274, -2.721908614388771852, 31.22303859784724978 ) ) ;
#2022=CARTESIAN_POINT ( 'NONE',  ( -11.60454494941741999, -5.557115091759785130, 34.35708131394839171 ) ) ;
#2023=CARTESIAN_POINT ( 'NONE',  ( -1.384615384615383471, -2.499999999999998668, 29.50000000000001066 ) ) ;
#2024=CARTESIAN_POINT ( 'NONE',  ( -7.053768389744480949, -11.18331474514187995, 33.13161551792790505 ) ) ;
#2025=CARTESIAN_POINT ( 'NONE',  ( -1.384615384615506484, -2.379036618888197285, 30.90682066428292885 ) ) ;
#2026=CARTESIAN_POINT ( 'NONE',  ( 0.3308469948709038544, -11.71456829005830080, 32.44064028649416542 ) ) ;
#2028=DIRECTION ( 'NONE',  ( -0.000000000000000000, -0.7660444431189791237, -0.6427876096865379196 ) ) ;
#2029=FACE_OUTER_BOUND ( 'NONE', #23695, .T. ) ;
#2030=DIRECTION ( 'NONE',  ( 0.000000000000000000, 0.1736481776669267785, -0.9848077530122087975 ) ) ;
#2031=CARTESIAN_POINT ( 'NONE',  ( 11.66925334628632882, -4.118422570099828484, 33.43335022499816489 ) ) ;
#2032=CARTESIAN_POINT ( 'NONE',  ( -1.318548051265308274, -9.058645607665452459, 34.76329471203371924 ) ) ;
#2033=CARTESIAN_POINT ( 'NONE',  ( 12.46153846153846168, -12.37446782046654192, 30.86335684631486131 ) ) ;
#2034=CARTESIAN_POINT ( 'NONE',  ( 2.372947447205147053, -6.835583212224609184, 34.95778746994559327 ) ) ;
#2035=CARTESIAN_POINT ( 'NONE',  ( 13.25400572941130584, -7.722926974430166069, 34.99546784045485737 ) ) ;
#2037=ORIENTED_EDGE ( 'NONE', *, *, #32084, .T. ) ;
#2038=B_SPLINE_CURVE_WITH_KNOTS ( 'NONE', 3,
 ( #28665, #37177, #63764, #16032, #57006, #70975, #84499, #78171, #76851, #57894 ),
 .UNSPECIFIED., .F., .F.,
 ( 4, 2, 2, 2, 4 ),
 ( 0.000000000000000000, 0.0001954311564186870913, 0.0003908623128373741825, 0.0005862934692560613009, 0.0007817246256747483650 ),
 .UNSPECIFIED. ) ;
#2040=ORIENTED_EDGE ( 'NONE', *, *, #30730, .T. ) ;
#2041=ADVANCED_FACE ( 'NONE', ( #14114 ), #67291, .F. ) ;
#2042=CARTESIAN_POINT ( 'NONE',  ( -2.557669051740897537, -2.920706130388546651, 32.31842814019191223 ) ) ;
#2043=ORIENTED_EDGE ( 'NONE', *, *, #39798, .T. ) ;
#2044=CARTESIAN_POINT ( 'NONE',  ( -10.61538461538461320, -10.89733346790207413, 36.13435417666054406 ) ) ;
#2045=EDGE_CURVE ( 'NONE', #23088, #78524, #40872, .T. ) ;
#2046=CARTESIAN_POINT ( 'NONE',  ( 14.30769230769231015, -2.292212530054420494, 30.41441678777542634 ) ) ;
#2048=CARTESIAN_POINT ( 'NONE',  ( -6.222926217516144831, -11.76352882383564769, 32.36236540154569497 ) ) ;
#2050=CARTESIAN_POINT ( 'NONE',  ( -17.93474486048716088, -9.528491918058456633, 34.59228464037085615 ) ) ;
#2051=CARTESIAN_POINT ( 'NONE',  ( -5.869474298236434961, -9.417988943895561960, 34.36773134775778260 ) ) ;
#2052=CARTESIAN_POINT ( 'NONE',  ( 15.90382292962469535, -8.475808217655753651, 34.90892951860618609 ) ) ;
#2053=AXIS2_PLACEMENT_3D ( 'NONE', #11556, #43662, #73710 ) ;
#2054=CARTESIAN_POINT ( 'NONE',  ( 15.23076923076910916, -8.656820664282941280, 34.87096338111179961 ) ) ;
#2055=CARTESIAN_POINT ( 'NONE',  ( -7.846153846153844924, -4.098570777380720287, 33.41473453929634729 ) ) ;
#2056=LINE ( 'NONE', #43928, #71280 ) ;
#2057=EDGE_CURVE ( 'NONE', #10922, #33240, #61362, .T. ) ;
#2059=CARTESIAN_POINT ( 'NONE',  ( -9.942330929600656120, -3.711651800289232028, 33.01384336483936011 ) ) ;
#2060=DIRECTION ( 'NONE',  ( 0.000000000000000000, 0.9396926207859126468, 0.3420201433256571111 ) ) ;
#2061=EDGE_CURVE ( 'NONE', #39874, #45094, #39182, .T. ) ;
#2062=CARTESIAN_POINT ( 'NONE',  ( 14.43821800945587341, -3.285477652293413264, 32.44071101563363158 ) ) ;
#2064=CARTESIAN_POINT ( 'NONE',  ( -13.38461538461538325, -2.499999999999998668, 29.75000000000001421 ) ) ;
#2065=ORIENTED_EDGE ( 'NONE', *, *, #24111, .T. ) ;
#2066=CARTESIAN_POINT ( 'NONE',  ( -17.75005448165185484, -2.824170634883621744, 31.52227843825337317 ) ) ;
#2067=CARTESIAN_POINT ( 'NONE',  ( 11.76147289007438701, -5.667800583137506010, 34.40243808032445827 ) ) ;
#2068=CARTESIAN_POINT ( 'NONE',  ( 1.254468175177166689, -12.45813303252208648, 30.39737893381572675 ) ) ;
#2069=CARTESIAN_POINT ( 'NONE',  ( 5.299702618191483694, -2.847695495035524882, 31.58253572463339509 ) ) ;
#2071=CARTESIAN_POINT ( 'NONE',  ( -9.019254006523732770, -8.432397168068783699, 34.66272746175022945 ) ) ;
#2072=DIRECTION ( 'NONE',  ( -0.000000000000000000, -0.8660254037844397068, -0.4999999999999978906 ) ) ;
#2073=VERTEX_POINT ( 'NONE', #45913 ) ;
#2075=EDGE_CURVE ( 'NONE', #42909, #68446, #37764, .T. ) ;
#2076=ORIENTED_EDGE ( 'NONE', *, *, #48961, .T. ) ;
#2077=CARTESIAN_POINT ( 'NONE',  ( 6.250000000000063949, -7.434744429011176159, 34.75000000000000711 ) ) ;
#2078=CARTESIAN_POINT ( 'NONE',  ( 6.856993512121045242, -2.721908614388772740, 31.22303859784724622 ) ) ;
#2079=CARTESIAN_POINT ( 'NONE',  ( 16.15384615384603251, -2.892918686052165622, 31.69288490824153470 ) ) ;
#2080=CARTESIAN_POINT ( 'NONE',  ( 2.057669070399342992, -5.851115903089112003, 34.47074536777953568 ) ) ;
#2081=CARTESIAN_POINT ( 'NONE',  ( 17.93472955403921887, -9.442884908240170461, 34.35708131394840592 ) ) ;
#2082=ORIENTED_EDGE ( 'NONE', *, *, #21168, .T. ) ;
#2083=EDGE_CURVE ( 'NONE', #7867, #68565, #82969, .T. ) ;
#2084=CARTESIAN_POINT ( 'NONE',  ( -17.86916158198723181, -7.277220443632451463, 34.74524770363009196 ) ) ;
#2086=ORIENTED_EDGE ( 'NONE', *, *, #40449, .T. ) ;
#2088=EDGE_CURVE ( 'NONE', #25490, #52597, #69994, .T. ) ;
#2089=CARTESIAN_POINT ( 'NONE',  ( -15.48074596171158213, -12.17611988154120972, 31.52148481390971213 ) ) ;
#2090=VERTEX_POINT ( 'NONE', #18014 ) ;
#2091=CARTESIAN_POINT ( 'NONE',  ( 8.519254038288416098, -2.779195860258146578, 31.39871582349836032 ) ) ;
#2093=FACE_OUTER_BOUND ( 'NONE', #61524, .T. ) ;
#2094=DIRECTION ( 'NONE',  ( 0.000000000000000000, 0.6427876096865373645, -0.7660444431189797898 ) ) ;
#2096=EDGE_CURVE ( 'NONE', #52736, #41563, #78509, .T. ) ;
#2097=VERTEX_POINT ( 'NONE', #18899 ) ;
#2099=AXIS2_PLACEMENT_3D ( 'NONE', #8921, #49011, #22424 ) ;
#2100=EDGE_LOOP ( 'NONE', ( #46921, #81866 ) ) ;
#2102=FACE_OUTER_BOUND ( 'NONE', #80839, .T. ) ;
#2103=EDGE_LOOP ( 'NONE', ( #22284, #27746, #22039, #53223 ) ) ;
#2104=CARTESIAN_POINT ( 'NONE',  ( 11.47319109250076430, -6.879047030191174805, 34.71129190930000163 ) ) ;
#2105=CARTESIAN_POINT ( 'NONE',  ( 13.38461538461569411, -2.506253911140615021, 30.00000000000323297 ) ) ;
#2106=EDGE_CURVE ( 'NONE', #22650, #19302, #52763, .T. ) ;
#2107=EDGE_CURVE ( 'NONE', #51215, #32941, #66641, .T. ) ;
#2108=CARTESIAN_POINT ( 'NONE',  ( -0.4615384615385840772, -9.528491918059723176, 34.59228464037033035 ) ) ;
#2109=ORIENTED_EDGE ( 'NONE', *, *, #5296, .T. ) ;
#2110=FACE_OUTER_BOUND ( 'NONE', #73589, .T. ) ;
#2111=CARTESIAN_POINT ( 'NONE',  ( 15.00728430620489995, -2.612411019501189369, 31.66733052389439962 ) ) ;
#2112=VERTEX_POINT ( 'NONE', #62960 ) ;
#2113=FACE_BOUND ( 'NONE', #58635, .T. ) ;
#2114=EDGE_CURVE ( 'NONE', #20560, #13624, #16245, .T. ) ;
#2115=CARTESIAN_POINT ( 'NONE',  ( -11.76138849736838488, -11.43668979543635089, 33.22377378376089752 ) ) ;
#2117=CARTESIAN_POINT ( 'NONE',  ( -15.00775638667583678, -2.889357225399414197, 32.26129605718031002 ) ) ;
#2118=CARTESIAN_POINT ( 'NONE',  ( 8.069166690247241647, -10.77377354290276124, 33.85451476688484718 ) ) ;
#2119=CARTESIAN_POINT ( 'NONE',  ( 4.853438133199126980, -3.236172620538810385, 32.36188796281390267 ) ) ;
#2120=CARTESIAN_POINT ( 'NONE',  ( 8.546304551714618114, -5.667676309546437530, 34.40238873228292249 ) ) ;
#2122=VERTEX_POINT ( 'NONE', #76944 ) ;
#2123=CARTESIAN_POINT ( 'NONE',  ( 10.61538461538461675, -1.790695186598648903, 34.54067556320373455 ) ) ;
#2124=CARTESIAN_POINT ( 'NONE',  ( -16.82697766754503377, -6.653508905675593610, 34.93172785388651391 ) ) ;
#2126=CARTESIAN_POINT ( 'NONE',  ( -12.21159305216042057, -3.520799739797214389, 33.17531984108286025 ) ) ;
#2127=CARTESIAN_POINT ( 'NONE',  ( 15.45378058238208219, -4.187068189119697692, 33.49521262558774026 ) ) ;
#2128=CARTESIAN_POINT ( 'NONE',  ( 3.165012428254921240, -7.249945686854185389, 34.74374336980224598 ) ) ;
#2129=CARTESIAN_POINT ( 'NONE',  ( 16.82692307692307665, -7.500000000000001776, 35.00000000000000000 ) ) ;
#2130=DIRECTION ( 'NONE',  ( -0.000000000000000000, -0.7660444431189791237, -0.6427876096865379196 ) ) ;
#2131=FACE_OUTER_BOUND ( 'NONE', #32724, .T. ) ;
#2132=FACE_BOUND ( 'NONE', #17620, .T. ) ;
#2133=CARTESIAN_POINT ( 'NONE',  ( -1.608100309179714804, -6.716662450894490100, 34.94144148231605840 ) ) ;
#2134=CARTESIAN_POINT ( 'NONE',  ( 1.515141086378949398, -2.619367082507848998, 30.83698974864644171 ) ) ;
#2135=CARTESIAN_POINT ( 'NONE',  ( -18.00000000000000000, -8.164416787775447659, 34.95778746994557906 ) ) ;
#2136=CARTESIAN_POINT ( 'NONE',  ( -7.596208436775802930, -12.68172785388650681, 30.59649109432439218 ) ) ;
#2137=CARTESIAN_POINT ( 'NONE',  ( 7.596153846153846700, -2.499999999999998668, 29.75000000000000355 ) ) ;
#2138=CYLINDRICAL_SURFACE ( 'NONE', #50494, 0.2499999999999994726 ) ;
#2140=EDGE_LOOP ( 'NONE', ( #72686, #39670, #86380, #88421 ) ) ;
#2141=ADVANCED_FACE ( 'NONE', ( #28304 ), #7155, .F. ) ;
#2142=ORIENTED_EDGE ( 'NONE', *, *, #37566, .T. ) ;
#2143=AXIS2_PLACEMENT_3D ( 'NONE', #55120, #69080, #48357 ) ;
#2145=CARTESIAN_POINT ( 'NONE',  ( -4.403822884788507253, -3.137211980971221781, 32.19342716148376837 ) ) ;
#2146=FACE_OUTER_BOUND ( 'NONE', #5200, .T. ) ;
#2147=B_SPLINE_CURVE_WITH_KNOTS ( 'NONE', 3,
 ( #73769, #12064, #39543, #60229, #87734, #26006 ),
 .UNSPECIFIED., .F., .F.,
 ( 4, 2, 4 ),
 ( 0.0003909512603273878522, 0.0005862562993132138141, 0.0007815613382990396676 ),
 .UNSPECIFIED. ) ;
#2148=CARTESIAN_POINT ( 'NONE',  ( -0.7115616857599186273, -2.985938066672154445, 32.43141759479405550 ) ) ;
#2149=VECTOR ( 'NONE', #54384, 1000.000000000000114 ) ;
#2150=CARTESIAN_POINT ( 'NONE',  ( -16.15384615384627409, -12.27809138561165270, 31.22303859784587132 ) ) ;
#2152=CARTESIAN_POINT ( 'NONE',  ( -1.253777054128622614, -7.277220318596959281, 34.99547417642776992 ) ) ;
#2153=DIRECTION ( 'NONE',  ( -0.000000000000000000, -0.8660254037844397068, -0.4999999999999978906 ) ) ;
#2154=CARTESIAN_POINT ( 'NONE',  ( -8.096177070375302876, -2.985938066672154445, 32.43141759479405550 ) ) ;
#2155=CARTESIAN_POINT ( 'NONE',  ( -1.449885830576159496, -12.46129190929999986, 30.37095296980880832 ) ) ;
#2156=CARTESIAN_POINT ( 'NONE',  ( -3.454254155333561727, -4.225889041578354544, 33.85425143139329407 ) ) ;
#2157=DIRECTION ( 'NONE',  ( 0.000000000000000000, 0.6427876096865373645, -0.7660444431189797898 ) ) ;
#2158=CARTESIAN_POINT ( 'NONE',  ( 14.37376065869474751, -11.69971097300155272, 32.46337939537588113 ) ) ;
#2159=DIRECTION ( 'NONE',  ( -0.000000000000000000, 0.3420201433256694901, -0.9396926207859082059 ) ) ;
#2161=CARTESIAN_POINT ( 'NONE',  ( 15.00784227186238162, -11.43668979543634734, 33.22377378376089752 ) ) ;
#2162=CARTESIAN_POINT ( 'NONE',  ( -17.20761454359063691, -2.729777683071817229, 31.24903638046269450 ) ) ;
#2164=CARTESIAN_POINT ( 'NONE',  ( 0.5923289025054120360, -3.338503747796865984, 32.95102852606553512 ) ) ;
#2166=VERTEX_POINT ( 'NONE', #13465 ) ;
#2167=CARTESIAN_POINT ( 'NONE',  ( 10.55013362522337239, -2.506253911140460922, 30.00000000000013856 ) ) ;
#2168=DIRECTION ( 'NONE',  ( -0.000000000000000000, -0.3420201433256694346, -0.9396926207859080948 ) ) ;
#2169=VERTEX_POINT ( 'NONE', #27429 ) ;
#2170=CARTESIAN_POINT ( 'NONE',  ( 7.976679547917411739, -3.816742781228458892, 33.13167719472716044 ) ) ;
#2171=DIRECTION ( 'NONE',  ( 0.000000000000000000, 0.8660254037844377084, -0.5000000000000015543 ) ) ;
#2172=EDGE_LOOP ( 'NONE', ( #70945, #66750, #87537, #2367 ) ) ;
#2173=CARTESIAN_POINT ( 'NONE',  ( -5.143006487878955646, -11.16473453929635440, 33.15142922261925662 ) ) ;
#2175=CARTESIAN_POINT ( 'NONE',  ( 8.992242120843618736, -4.887748414852792322, 34.01359900205216746 ) ) ;
#2176=EDGE_CURVE ( 'NONE', #63712, #74006, #46292, .T. ) ;
#2178=CARTESIAN_POINT ( 'NONE',  ( -12.52762084089859940, -2.292212530054419606, 30.41441678777542634 ) ) ;
#2180=DIRECTION ( 'NONE',  ( 0.000000000000000000, 0.9848077530122072432, 0.1736481776669354937 ) ) ;
#2181=ORIENTED_EDGE ( 'NONE', *, *, #84922, .T. ) ;
#2182=VERTEX_POINT ( 'NONE', #7603 ) ;
#2184=CARTESIAN_POINT ( 'NONE',  ( 3.230769230769108269, -2.379036618888197285, 30.90682066428292885 ) ) ;
#2185=CARTESIAN_POINT ( 'NONE',  ( 2.530471976670372936, -11.60474049983370648, 33.02348890104160262 ) ) ;
#2186=EDGE_CURVE ( 'NONE', #10414, #5178, #33471, .T. ) ;
#2187=CARTESIAN_POINT ( 'NONE',  ( -8.096153846153844924, -7.500000000000001776, 34.75000000000000000 ) ) ;
#2188=CARTESIAN_POINT ( 'NONE',  ( 2.980746006547774218, -10.18141759479407327, 34.26406193332782379 ) ) ;
#2189=VECTOR ( 'NONE', #24278, 1000.000000000000114 ) ;
#2190=ORIENTED_EDGE ( 'NONE', *, *, #70727, .F. ) ;
#2193=CARTESIAN_POINT ( 'NONE',  ( 9.692307692307572609, -4.481592998941358097, 33.73612834414048933 ) ) ;
#2195=CARTESIAN_POINT ( 'NONE',  ( 17.07692307692295586, -5.219633306517616589, 34.19971097300220464 ) ) ;
#2196=VERTEX_POINT ( 'NONE', #35514 ) ;
#2197=DIRECTION ( 'NONE',  ( -0.000000000000000000, 0.3420201433256694901, -0.9396926207859082059 ) ) ;
#2198=CARTESIAN_POINT ( 'NONE',  ( -8.519176349317316266, -12.65882529074907126, 30.72640787790839312 ) ) ;
#2201=ORIENTED_EDGE ( 'NONE', *, *, #69425, .F. ) ;
#2203=ORIENTED_EDGE ( 'NONE', *, *, #24683, .F. ) ;
#2204=CARTESIAN_POINT ( 'NONE',  ( 4.403900465484468008, -4.943051570960392382, 34.04725096376909477 ) ) ;
#2205=ADVANCED_FACE ( 'NONE', ( #1275 ), #42721, .F. ) ;
#2206=CARTESIAN_POINT ( 'NONE',  ( 14.08476534878545827, -5.582147617184174848, 34.63737895849758530 ) ) ;
#2207=EDGE_LOOP ( 'NONE', ( #10098, #41399 ) ) ;
#2208=CARTESIAN_POINT ( 'NONE',  ( 15.45378058238208041, -3.105924265160262543, 32.13625925475356127 ) ) ;
#2209=LINE ( 'NONE', #65680, #52288 ) ;
#2210=CARTESIAN_POINT ( 'NONE',  ( 17.93391762063986050, -12.34228464037088280, 31.77849191805838558 ) ) ;
#2211=FACE_BOUND ( 'NONE', #10306, .T. ) ;
#2213=CARTESIAN_POINT ( 'NONE',  ( -11.53846153846166089, -6.835583212225970762, 34.95778746994575670 ) ) ;
#2214=CARTESIAN_POINT ( 'NONE',  ( -13.38461538461538325, -1.509761064869970415, 31.06009739812519044 ) ) ;
#2215=CARTESIAN_POINT ( 'NONE',  ( 0.5915835174582330103, -2.254550872974306674, 29.97347326024527447 ) ) ;
#2216=CARTESIAN_POINT ( 'NONE',  ( -16.02332071561251681, -3.068774925481847937, 32.56582465632704526 ) ) ;
#2217=CARTESIAN_POINT ( 'NONE',  ( -7.976301055592065481, -3.285722584762969856, 32.44110544564090759 ) ) ;
#2218=CARTESIAN_POINT ( 'NONE',  ( -9.942307692307691624, -2.249999999999998668, 29.75000000000000355 ) ) ;
#2219=ORIENTED_EDGE ( 'NONE', *, *, #22671, .F. ) ;
#2220=CARTESIAN_POINT ( 'NONE',  ( -15.90379173393269596, -3.435999193479609026, 33.07426656108011542 ) ) ;
#2221=ORIENTED_EDGE ( 'NONE', *, *, #54401, .F. ) ;
#2222=ORIENTED_EDGE ( 'NONE', *, *, #70191, .T. ) ;
#2223=VECTOR ( 'NONE', #1169, 999.9999999999998863 ) ;
#2224=CARTESIAN_POINT ( 'NONE',  ( -3.230769230769229949, -3.886160181151819604, 36.00935417666054406 ) ) ;
#2226=DIRECTION ( 'NONE',  ( -0.000000000000000000, -0.1736481776669307198, -0.9848077530122080203 ) ) ;
#2227=DIRECTION ( 'NONE',  ( -0.000000000000000000, 0.9396926207859093161, -0.3420201433256663259 ) ) ;
#2228=CARTESIAN_POINT ( 'NONE',  ( -10.39237177129122003, -12.38742843783360748, 31.66772728687926985 ) ) ;
#2229=CARTESIAN_POINT ( 'NONE',  ( -0.2385271099256119354, -11.76359900205217457, 32.36225158514719880 ) ) ;
#2230=ORIENTED_EDGE ( 'NONE', *, *, #43221, .T. ) ;
#2231=CYLINDRICAL_SURFACE ( 'NONE', #37096, 0.2499999999999998890 ) ;
#2232=CARTESIAN_POINT ( 'NONE',  ( 14.17700170458200581, -12.62707690430377383, 30.88035979386743435 ) ) ;
#2233=CARTESIAN_POINT ( 'NONE',  ( -2.057692307690886846, -7.500000000000154543, 35.00000000000007105 ) ) ;
#2234=FACE_OUTER_BOUND ( 'NONE', #22715, .T. ) ;
#2238=ORIENTED_EDGE ( 'NONE', *, *, #56649, .F. ) ;
#2239=CARTESIAN_POINT ( 'NONE',  ( -7.596099426240391139, -12.01375889529407281, 32.43194544308182969 ) ) ;
#2240=ORIENTED_EDGE ( 'NONE', *, *, #29973, .T. ) ;
#2241=CYLINDRICAL_SURFACE ( 'NONE', #25393, 0.2500000000000012212 ) ;
#2242=CARTESIAN_POINT ( 'NONE',  ( 17.99999999999987566, -6.026961402154118908, 34.52809138561165270 ) ) ;
#2243=CARTESIAN_POINT ( 'NONE',  ( -6.923076923076922462, -1.242168528481310874, 33.36296068462461051 ) ) ;
#2244=CARTESIAN_POINT ( 'NONE',  ( -5.010855743573002563, -3.322132147404559976, 32.92929555188717927 ) ) ;
#2246=CARTESIAN_POINT ( 'NONE',  ( 8.519254038288414321, -6.567427716900048118, 34.66269422305636283 ) ) ;
#2247=ORIENTED_EDGE ( 'NONE', *, *, #64813, .T. ) ;
#2249=B_SPLINE_CURVE_WITH_KNOTS ( 'NONE', 3,
 ( #65012, #3320, #11419, #3766, #31697, #59155, #30792, #86661, #38904, #13631 ),
 .UNSPECIFIED., .F., .F.,
 ( 4, 2, 2, 2, 4 ),
 ( 0.0007817359430256322827, 0.0009771253907249989254, 0.001172514838424365460, 0.001367904286123731994, 0.001563293733823098745 ),
 .UNSPECIFIED. ) ;
#2250=CARTESIAN_POINT ( 'NONE',  ( -2.241623956689869246, -10.51840700105979565, 33.73612834413962247 ) ) ;
#2251=VERTEX_POINT ( 'NONE', #62523 ) ;
#2252=CARTESIAN_POINT ( 'NONE',  ( 3.100078627658924280, -12.35290016733513951, 31.75349464988449455 ) ) ;
#2253=CARTESIAN_POINT ( 'NONE',  ( -0.5276208408985965104, -3.937682226553329556, 33.60647404775217240 ) ) ;
#2254=CARTESIAN_POINT ( 'NONE',  ( -3.361460697436789324, -4.809359713505814149, 33.96456829005828837 ) ) ;
#2255=CARTESIAN_POINT ( 'NONE',  ( -12.46153846153846168, -9.780366693483667717, 34.19971097300155094 ) ) ;
#2257=CARTESIAN_POINT ( 'NONE',  ( 1.384615384615386802, -4.098570777380720287, 33.41473453929634729 ) ) ;
#2261=CARTESIAN_POINT ( 'NONE',  ( -17.01166750564705055, -10.90142922261932057, 33.41473453929631887 ) ) ;
#2262=DIRECTION ( 'NONE',  ( 0.000000000000000000, 0.7660444431189822323, -0.6427876096865344779 ) ) ;
#2264=CARTESIAN_POINT ( 'NONE',  ( -15.93083330975275658, -11.43677907613345113, 33.22367315496201456 ) ) ;
#2265=CARTESIAN_POINT ( 'NONE',  ( 2.307692307692186251, -12.16647553114689728, 32.15551576947799362 ) ) ;
#2266=VERTEX_POINT ( 'NONE', #82381 ) ;
#2268=CYLINDRICAL_SURFACE ( 'NONE', #74318, 0.2500000000000012212 ) ;
#2270=ORIENTED_EDGE ( 'NONE', *, *, #86880, .F. ) ;
#2271=DIRECTION ( 'NONE',  ( -0.000000000000000000, 0.7660444431189791237, -0.6427876096865379196 ) ) ;
#2273=EDGE_CURVE ( 'NONE', #37486, #51137, #75601, .T. ) ;
#2274=EDGE_LOOP ( 'NONE', ( #42968, #75217 ) ) ;
#2275=CARTESIAN_POINT ( 'NONE',  ( 17.77651505627605033, -6.760086850603066466, 34.69517049084099369 ) ) ;
#2276=CARTESIAN_POINT ( 'NONE',  ( -17.20707104665477161, -2.373036134822905208, 30.88089517874952250 ) ) ;
#2277=DIRECTION ( 'NONE',  ( -0.000000000000000000, -0.9848077530122085754, -0.1736481776669273613 ) ) ;
#2278=CARTESIAN_POINT ( 'NONE',  ( -16.15384615384615330, -5.415277668671390821, 36.20867863119892149 ) ) ;
#2281=EDGE_CURVE ( 'NONE', #62668, #32981, #403, .T. ) ;
#2282=EDGE_LOOP ( 'NONE', ( #39969, #10820 ) ) ;
#2283=CARTESIAN_POINT ( 'NONE',  ( -6.673076923076923350, -2.499999999999998668, 29.75000000000000355 ) ) ;
#2284=DIRECTION ( 'NONE',  ( -0.000000000000000000, 0.7660444431189791237, -0.6427876096865379196 ) ) ;
#2285=AXIS2_PLACEMENT_3D ( 'NONE', #3586, #86481, #24753 ) ;
#2286=ORIENTED_EDGE ( 'NONE', *, *, #77754, .T. ) ;
#2288=CARTESIAN_POINT ( 'NONE',  ( 11.78851595837499211, -12.65882529074907126, 30.72640787790839312 ) ) ;
#2289=DIRECTION ( 'NONE',  ( 0.000000000000000000, 0.9848077530122072432, 0.1736481776669354937 ) ) ;
#2290=CARTESIAN_POINT ( 'NONE',  ( 0.4615384615383396616, -4.481592998941358097, 33.73612834414048933 ) ) ;
#2294=B_SPLINE_CURVE_WITH_KNOTS ( 'NONE', 3,
 ( #3009, #2564, #65154, #23721, #16979, #22844, #44428, #43561, #58390, #50747 ),
 .UNSPECIFIED., .F., .F.,
 ( 4, 2, 2, 2, 4 ),
 ( 0.0007817246336856293861, 0.0009771112958940108076, 0.001172497958102392121, 0.001367884620310773434, 0.001563271282519154747 ),
 .UNSPECIFIED. ) ;
#2295=VERTEX_POINT ( 'NONE', #6278 ) ;
#2296=ORIENTED_EDGE ( 'NONE', *, *, #49343, .F. ) ;
#2297=EDGE_CURVE ( 'NONE', #69664, #33072, #42283, .T. ) ;
#2298=FACE_BOUND ( 'NONE', #32128, .T. ) ;
#2299=ORIENTED_EDGE ( 'NONE', *, *, #85061, .F. ) ;
#2300=CARTESIAN_POINT ( 'NONE',  ( 8.769230769230768274, -3.513871655860378418, 32.76840700105978499 ) ) ;
#2301=CARTESIAN_POINT ( 'NONE',  ( -18.06527000055631760, -11.06231777344663136, 33.60647404775220082 ) ) ;
#2303=CARTESIAN_POINT ( 'NONE',  ( 5.299934428535925335, -4.187068189119697692, 33.49521262558774026 ) ) ;
#2304=VERTEX_POINT ( 'NONE', #33743 ) ;
#2305=EDGE_LOOP ( 'NONE', ( #53271, #45181 ) ) ;
#2306=CARTESIAN_POINT ( 'NONE',  ( 8.769230769230768274, -4.945431358278436385, 36.03766855953609394 ) ) ;
#2308=CARTESIAN_POINT ( 'NONE',  ( -10.68065461594093435, -8.656820664281498878, 34.87096338111211935 ) ) ;
#2309=AXIS2_PLACEMENT_3D ( 'NONE', #9147, #50105, #76708 ) ;
#2310=EDGE_CURVE ( 'NONE', #42810, #46099, #9751, .T. ) ;
#2312=EDGE_CURVE ( 'NONE', #74382, #19612, #71948, .T. ) ;
#2313=CARTESIAN_POINT ( 'NONE',  ( 12.46153846153846168, -2.538708090699994813, 30.37095296980875503 ) ) ;
#2314=CARTESIAN_POINT ( 'NONE',  ( -18.24997673094235751, -11.28823185664189310, 33.01397839955799896 ) ) ;
#2316=CARTESIAN_POINT ( 'NONE',  ( 16.40390057375960708, -2.318338780012835443, 30.59689888758630616 ) ) ;
#2317=EDGE_CURVE ( 'NONE', #37303, #13779, #85916, .T. ) ;
#2318=CARTESIAN_POINT ( 'NONE',  ( -6.223484924564330001, -6.716662450894490100, 34.94144148231605840 ) ) ;
#2320=CARTESIAN_POINT ( 'NONE',  ( -7.846153846153844924, -1.466349020453238561, 30.81389545987213907 ) ) ;
#2321=CARTESIAN_POINT ( 'NONE',  ( 8.992243613324164997, -6.460100341425560444, 34.89618726649961644 ) ) ;
#2323=VECTOR ( 'NONE', #15206, 1000.000000000000114 ) ;
#2325=ORIENTED_EDGE ( 'NONE', *, *, #62800, .F. ) ;
#2326=EDGE_LOOP ( 'NONE', ( #24112, #73313, #27769, #48180 ) ) ;
#2327=CARTESIAN_POINT ( 'NONE',  ( -18.06870381900330713, -2.255952184585098053, 29.99992509483742609 ) ) ;
#2328=CARTESIAN_POINT ( 'NONE',  ( -9.469528023329624844, -8.540255544307065350, 34.89611431652622286 ) ) ;
#2329=CARTESIAN_POINT ( 'NONE',  ( -18.00000000000000000, -2.249999999999989786, 29.74999999999998579 ) ) ;
#2330=CARTESIAN_POINT ( 'NONE',  ( -2.084912638714241595, -2.612705202774697533, 31.66806509827799943 ) ) ;
#2331=LINE ( 'NONE', #21733, #24220 ) ;
#2332=DIRECTION ( 'NONE',  ( -0.000000000000000000, -0.6427876096865404731, -0.7660444431189771253 ) ) ;
#2333=ORIENTED_EDGE ( 'NONE', *, *, #66591, .F. ) ;
#2334=CARTESIAN_POINT ( 'NONE',  ( -3.230769230769351186, -2.625532179533779154, 30.86335684631627174 ) ) ;
#2335=CARTESIAN_POINT ( 'NONE',  ( 9.692307692307570832, -12.16647553114689728, 32.15551576947799362 ) ) ;
#2336=CARTESIAN_POINT ( 'NONE',  ( -9.692307692307691624, -9.819645486525091727, 36.12317359536749706 ) ) ;
#2337=CARTESIAN_POINT ( 'NONE',  ( -11.53846153846153655, -3.513871655860378418, 32.76840700105978499 ) ) ;
#2338=ORIENTED_EDGE ( 'NONE', *, *, #31520, .F. ) ;
#2339=CARTESIAN_POINT ( 'NONE',  ( 14.43848411551709887, -8.999086150933475636, 34.52020707165672775 ) ) ;
#2340=ORIENTED_EDGE ( 'NONE', *, *, #76448, .T. ) ;
#2341=FACE_BOUND ( 'NONE', #44611, .T. ) ;
#2342=B_SPLINE_CURVE_WITH_KNOTS ( 'NONE', 3,
 ( #50353, #70644, #854, #42738, #55791, #15262, #22014, #84615, #77397, #22452 ),
 .UNSPECIFIED., .F., .F.,
 ( 4, 2, 2, 2, 4 ),
 ( 0.0007817359430256392216, 0.0009771253907250080327, 0.001172514838424376952, 0.001367904286123745872, 0.001563293733823114791 ),
 .UNSPECIFIED. ) ;
#2343=CARTESIAN_POINT ( 'NONE',  ( -0.4615384615384611200, -13.75783147151868846, 33.36296068462461051 ) ) ;
#2344=DIRECTION ( 'NONE',  ( -0.000000000000000000, -0.8660254037844399289, -0.4999999999999980016 ) ) ;
#2345=CARTESIAN_POINT ( 'NONE',  ( -3.164700879766791708, -8.120952969808772792, 34.71129190929999453 ) ) ;
#2346=VERTEX_POINT ( 'NONE', #79155 ) ;
#2347=CARTESIAN_POINT ( 'NONE',  ( -14.53061852520844965, -12.39988816332205701, 30.74660775122750778 ) ) ;
#2348=CARTESIAN_POINT ( 'NONE',  ( 15.29602437028206907, -2.379036618887895305, 30.90682066428158592 ) ) ;
#2349=CARTESIAN_POINT ( 'NONE',  ( 8.703148389870634105, -8.164416787775445883, 34.95778746994557906 ) ) ;
#2350=CARTESIAN_POINT ( 'NONE',  ( -18.00000000000012079, -3.835265460704626150, 33.15142922262032954 ) ) ;
#2352=AXIS2_PLACEMENT_3D ( 'NONE', #51446, #87512, #17246 ) ;
#2353=CARTESIAN_POINT ( 'NONE',  ( 14.30769230769218581, -5.094484230521993062, 34.41647553114689373 ) ) ;
#2354=ORIENTED_EDGE ( 'NONE', *, *, #15042, .F. ) ;
#2355=CARTESIAN_POINT ( 'NONE',  ( 13.44987052412822237, -8.656820664281605460, 34.87096338111211224 ) ) ;
#2356=ORIENTED_EDGE ( 'NONE', *, *, #33390, .F. ) ;
#2357=CARTESIAN_POINT ( 'NONE',  ( 9.626224281351809964, -3.513871655860377086, 32.76840700105978499 ) ) ;
#2358=CARTESIAN_POINT ( 'NONE',  ( -1.634638608836841644, -12.45566812827425096, 31.48439005359158926 ) ) ;
#2359=CARTESIAN_POINT ( 'NONE',  ( 7.623226887246994821, -10.01117774369187252, 34.36070679894347535 ) ) ;
#2361=CARTESIAN_POINT ( 'NONE',  ( -15.36137888597331091, -7.722926974430166069, 34.99546784045485737 ) ) ;
#2363=CARTESIAN_POINT ( 'NONE',  ( 8.546303810323918171, -4.026226216239094491, 33.68668979543634379 ) ) ;
#2364=VECTOR ( 'NONE', #29528, 1000.000000000000114 ) ;
#2365=CARTESIAN_POINT ( 'NONE',  ( -9.822998295417995962, -11.93127051446799847, 32.56575433478202797 ) ) ;
#2367=ORIENTED_EDGE ( 'NONE', *, *, #77511, .F. ) ;
#2368=CARTESIAN_POINT ( 'NONE',  ( -0.4615384615385826339, -6.026961402154118908, 34.52809138561165270 ) ) ;
#2369=CARTESIAN_POINT ( 'NONE',  ( 13.31886195630205805, -7.249945578846651806, 34.99404164642496795 ) ) ;
#2370=ORIENTED_EDGE ( 'NONE', *, *, #26120, .T. ) ;
#2371=EDGE_LOOP ( 'NONE', ( #8849, #30221, #25616, #7528 ) ) ;
#2372=EDGE_LOOP ( 'NONE', ( #81677, #11518 ) ) ;
#2373=CARTESIAN_POINT ( 'NONE',  ( 4.087762742890273415, -12.10708131394839349, 31.69288490824020244 ) ) ;
#2375=CARTESIAN_POINT ( 'NONE',  ( -17.32689980786543060, -9.148715823498378086, 34.47080413974185120 ) ) ;
#2376=EDGE_CURVE ( 'NONE', #63608, #72717, #64359, .T. ) ;
#2377=LINE ( 'NONE', #22225, #38519 ) ;
#2379=CARTESIAN_POINT ( 'NONE',  ( 7.053602624840487501, -11.46989282347013095, 32.79007818306219946 ) ) ;
#2380=CARTESIAN_POINT ( 'NONE',  ( 5.750000000000003553, -7.566082377512563184, 35.00000000000000711 ) ) ;
#2381=VERTEX_POINT ( 'NONE', #36404 ) ;
#2383=CARTESIAN_POINT ( 'NONE',  ( -6.923076923076922462, -5.415277668671390821, 36.20867863119892149 ) ) ;
#2384=CARTESIAN_POINT ( 'NONE',  ( -5.076923076923075762, -8.973038597847269315, 34.52809138561121927 ) ) ;
#2385=CARTESIAN_POINT ( 'NONE',  ( -9.626239341305254271, -11.16473453929635440, 33.15142922261926373 ) ) ;
#2386=CARTESIAN_POINT ( 'NONE',  ( 5.076923076922954969, -3.300289026999228881, 32.46337939537708905 ) ) ;
#2387=B_SPLINE_CURVE_WITH_KNOTS ( 'NONE', 3,
 ( #46987, #80356, #39372, #87568, #33493, #54187, #26284, #60952, #88457, #60063 ),
 .UNSPECIFIED., .F., .F.,
 ( 4, 2, 2, 2, 4 ),
 ( 0.0007817359430256285964, 0.0009771253907249948054, 0.001172514838424360906, 0.001367904286123727223, 0.001563293733823093324 ),
 .UNSPECIFIED. ) ;
#2388=ORIENTED_EDGE ( 'NONE', *, *, #75261, .T. ) ;
#2389=DIRECTION ( 'NONE',  ( 0.000000000000000000, 0.7660444431189822323, -0.6427876096865344779 ) ) ;
#2390=B_SPLINE_CURVE_WITH_KNOTS ( 'NONE', 3,
 ( #30173, #57201, #79696, #71587, #77910, #9457, #64382, #23403, #9896, #37358 ),
 .UNSPECIFIED., .F., .F.,
 ( 4, 2, 2, 2, 4 ),
 ( 0.000000000000000000, 0.0001954339857564099951, 0.0003908679715128199903, 0.0005863019572692300396, 0.0007817359430256399806 ),
 .UNSPECIFIED. ) ;
#2391=EDGE_CURVE ( 'NONE', #59690, #29899, #8490, .T. ) ;
#2393=CARTESIAN_POINT ( 'NONE',  ( 12.33084785842815378, -9.084618155246140248, 34.75535874321725771 ) ) ;
#2394=CARTESIAN_POINT ( 'NONE',  ( -15.90384615384614264, -2.249999999999999112, 29.81603969181033165 ) ) ;
#2395=CARTESIAN_POINT ( 'NONE',  ( 3.296836564119306701, -10.67929555188718282, 33.92786785259544757 ) ) ;
#2396=CARTESIAN_POINT ( 'NONE',  ( -14.30769230769230660, -11.11383981884818262, 36.00935417666054406 ) ) ;
#2397=ORIENTED_EDGE ( 'NONE', *, *, #22673, .F. ) ;
#2398=VECTOR ( 'NONE', #12052, 1000.000000000000114 ) ;
#2399=ADVANCED_FACE ( 'NONE', ( #9805 ), #30953, .F. ) ;
#2400=CARTESIAN_POINT ( 'NONE',  ( 12.71148387091650278, -10.92531984108285670, 33.72920026020278073 ) ) ;
#2401=CARTESIAN_POINT ( 'NONE',  ( -13.38461538461550759, -11.06231777344772027, 33.60647404775119895 ) ) ;
#2402=CARTESIAN_POINT ( 'NONE',  ( 8.992010310499175318, -4.387253974876679230, 33.66317474335728832 ) ) ;
#2403=EDGE_LOOP ( 'NONE', ( #48266, #24806, #24783, #35003 ) ) ;
#2404=EDGE_CURVE ( 'NONE', #30706, #45661, #63862, .T. ) ;
#2405=CARTESIAN_POINT ( 'NONE',  ( 7.780071466793708979, -11.35647404775217595, 33.31231777344666511 ) ) ;
#2406=VERTEX_POINT ( 'NONE', #17007 ) ;
#2407=CARTESIAN_POINT ( 'NONE',  ( 9.757563263583715951, -11.94971097300157403, 32.03036669348361443 ) ) ;
#2408=EDGE_CURVE ( 'NONE', #292, #19083, #84998, .T. ) ;
#2409=CARTESIAN_POINT ( 'NONE',  ( 6.923076923076924238, -2.833524468853757305, 32.15551576947925838 ) ) ;
#2410=CIRCLE ( 'NONE', #57062, 0.2500000000000002220 ) ;
#2411=CARTESIAN_POINT ( 'NONE',  ( -7.976301815885547875, -2.647304123082328875, 31.75400227202885972 ) ) ;
#2412=EDGE_CURVE ( 'NONE', #54986, #54522, #37667, .T. ) ;
#2413=CARTESIAN_POINT ( 'NONE',  ( -14.24243673641628227, -10.21337939537593620, 33.94971097300152252 ) ) ;
#2414=CARTESIAN_POINT ( 'NONE',  ( 18.25005441991345378, -8.346898887586322147, 34.93166121998716278 ) ) ;
#2415=B_SPLINE_CURVE_WITH_KNOTS ( 'NONE', 3,
 ( #75033, #24728, #11670, #66612, #4913, #54743 ),
 .UNSPECIFIED., .F., .F.,
 ( 4, 2, 4 ),
 ( 3.252606517456513302E-19, 0.0001954784845028939284, 0.0003909569690057875316 ),
 .UNSPECIFIED. ) ;
#2416=AXIS2_PLACEMENT_3D ( 'NONE', #22539, #75706, #54998 ) ;
#2417=ORIENTED_EDGE ( 'NONE', *, *, #41255, .T. ) ;
#2418=ORIENTED_EDGE ( 'NONE', *, *, #24350, .F. ) ;
#2419=VERTEX_POINT ( 'NONE', #3038 ) ;
#2420=EDGE_CURVE ( 'NONE', #38559, #21246, #24756, .T. ) ;
#2422=CARTESIAN_POINT ( 'NONE',  ( 8.769230769230768274, -2.900454961884010974, 35.62045528018868623 ) ) ;
#2423=CARTESIAN_POINT ( 'NONE',  ( -17.01085472592063397, -3.513871655860379306, 32.76840700105978499 ) ) ;
#2424=CARTESIAN_POINT ( 'NONE',  ( 14.30769230769231015, -2.486705287966279876, 31.30864560766543647 ) ) ;
#2426=FACE_OUTER_BOUND ( 'NONE', #52785, .T. ) ;
#2427=CARTESIAN_POINT ( 'NONE',  ( 11.53846153846153832, -1.129524287112498415, 32.06866353760679544 ) ) ;
#2428=EDGE_CURVE ( 'NONE', #80371, #39612, #58183, .T. ) ;
#2429=CARTESIAN_POINT ( 'NONE',  ( 5.326977388561390470, -9.943054286541403997, 34.11300777759954883 ) ) ;
#2430=EDGE_LOOP ( 'NONE', ( #58554, #86194, #30591, #25383 ) ) ;
#2431=ORIENTED_EDGE ( 'NONE', *, *, #77572, .F. ) ;
#2433=CARTESIAN_POINT ( 'NONE',  ( 4.153846153846154188, -3.937682226553329556, 33.60647404775216529 ) ) ;
#2435=CARTESIAN_POINT ( 'NONE',  ( 0.5920641633020248262, -8.586989748646450593, 34.63063291749215011 ) ) ;
#2436=CARTESIAN_POINT ( 'NONE',  ( -5.142193077479396024, -12.70778746994557551, 30.41441678777548319 ) ) ;
#2439=VERTEX_POINT ( 'NONE', #11138 ) ;
#2440=ADVANCED_FACE ( 'NONE', ( #25986 ), #31865, .F. ) ;
#2442=CARTESIAN_POINT ( 'NONE',  ( 5.326923076923011813, -7.565270000091922853, 34.99999999999999289 ) ) ;
#2443=ORIENTED_EDGE ( 'NONE', *, *, #1263, .T. ) ;
#2444=FACE_BOUND ( 'NONE', #1100, .T. ) ;
#2445=CARTESIAN_POINT ( 'NONE',  ( 3.480823650682684622, -2.544122305571458575, 31.48381861865057729 ) ) ;
#2446=CYLINDRICAL_SURFACE ( 'NONE', #13219, 0.2499999999999994726 ) ;
#2447=ORIENTED_EDGE ( 'NONE', *, *, #6766, .T. ) ;
#2449=CARTESIAN_POINT ( 'NONE',  ( 16.15384615384615330, -11.16473453929635440, 33.15142922261926373 ) ) ;
#2450=CARTESIAN_POINT ( 'NONE',  ( -10.61538461538461320, -3.886160181151819604, 36.00935417666054406 ) ) ;
#2451=AXIS2_PLACEMENT_3D ( 'NONE', #65757, #79734, #87396 ) ;
#2452=CARTESIAN_POINT ( 'NONE',  ( 1.253924781505077801, -3.338472653186242756, 32.95098750199972670 ) ) ;
#2453=CARTESIAN_POINT ( 'NONE',  ( -11.60373198442231590, -6.026961402152685388, 34.52809138561120506 ) ) ;
#2454=CYLINDRICAL_SURFACE ( 'NONE', #75419, 0.2500000000000004996 ) ;
#2455=CARTESIAN_POINT ( 'NONE',  ( 7.846153846153723244, -11.67786785259630911, 32.92929555188603530 ) ) ;
#2456=FACE_OUTER_BOUND ( 'NONE', #34698, .T. ) ;
#2457=CARTESIAN_POINT ( 'NONE',  ( -7.976301815885538105, -12.15440758774515473, 32.17923288041532004 ) ) ;
#2458=CARTESIAN_POINT ( 'NONE',  ( -6.222926217516146608, -5.667676309546437530, 34.40238873228292249 ) ) ;
#2459=CARTESIAN_POINT ( 'NONE',  ( 16.15384615384615330, -10.67929555188718282, 33.92786785259544047 ) ) ;
#2460=CYLINDRICAL_SURFACE ( 'NONE', #84762, 0.2499999999999995559 ) ;
#2461=ADVANCED_FACE ( 'NONE', ( #39519 ), #3924, .F. ) ;
#2462=CARTESIAN_POINT ( 'NONE',  ( -13.31854805126531005, -12.34228464037088813, 31.77849191805839268 ) ) ;
#2463=CARTESIAN_POINT ( 'NONE',  ( 5.011652630962300847, -12.46129190929999986, 30.37095296980880832 ) ) ;
#2464=CARTESIAN_POINT ( 'NONE',  ( 2.372947878968333146, -10.21337939537593797, 33.94971097300152252 ) ) ;
#2465=CARTESIAN_POINT ( 'NONE',  ( -0.4615384615384611200, -8.164416787775445883, 34.95778746994557906 ) ) ;
#2466=CARTESIAN_POINT ( 'NONE',  ( 12.46153846153846168, -12.29105614889573062, 35.45975837776705220 ) ) ;
#2468=CARTESIAN_POINT ( 'NONE',  ( -5.749945688361683516, -12.41262288849542017, 30.68299917996395010 ) ) ;
#2470=ORIENTED_EDGE ( 'NONE', *, *, #2001, .T. ) ;
#2471=EDGE_CURVE ( 'NONE', #11784, #5488, #12045, .T. ) ;
#2472=LINE ( 'NONE', #65061, #49003 ) ;
#2473=ORIENTED_EDGE ( 'NONE', *, *, #80206, .T. ) ;
#2475=LINE ( 'NONE', #80266, #50704 ) ;
#2477=VERTEX_POINT ( 'NONE', #33190 ) ;
#2478=CYLINDRICAL_SURFACE ( 'NONE', #28280, 0.2499999999999994726 ) ;
#2480=CARTESIAN_POINT ( 'NONE',  ( -6.130691466667556710, -11.71456829005830080, 32.44064028649416542 ) ) ;
#2482=CARTESIAN_POINT ( 'NONE',  ( 6.065255139512838234, -6.835583212224609184, 34.95778746994559327 ) ) ;
#2483=B_SPLINE_CURVE_WITH_KNOTS ( 'NONE', 3,
 ( #28884, #36517, #35634, #23425, #36940, #77059, #63966, #15805, #56341, #43270 ),
 .UNSPECIFIED., .F., .F.,
 ( 4, 2, 2, 2, 4 ),
 ( 0.000000000000000000, 0.0001954339857564058210, 0.0003908679715128116419, 0.0005863019572692174629, 0.0007817359430256232838 ),
 .UNSPECIFIED. ) ;
#2484=CARTESIAN_POINT ( 'NONE',  ( -5.777220458731589403, -9.332535724633407526, 34.40230450496446224 ) ) ;
#2485=CARTESIAN_POINT ( 'NONE',  ( -11.53846153846122391, -2.255955759149395501, 30.00000000000324363 ) ) ;
#2486=EDGE_CURVE ( 'NONE', #7349, #76616, #3305, .T. ) ;
#2487=CARTESIAN_POINT ( 'NONE',  ( -17.07692307692307665, -12.62096338111211580, 30.90682066428153263 ) ) ;
#2488=CARTESIAN_POINT ( 'NONE',  ( -13.51530598772569292, -8.191372820521381826, 34.95448215188424967 ) ) ;
#2489=CARTESIAN_POINT ( 'NONE',  ( -13.38461538461550759, -12.16647553114689728, 32.15551576947799362 ) ) ;
#2491=FACE_OUTER_BOUND ( 'NONE', #51838, .T. ) ;
#2492=CARTESIAN_POINT ( 'NONE',  ( -15.23076923076935074, -2.625532179533778709, 30.86335684631627174 ) ) ;
#2493=VECTOR ( 'NONE', #28205, 1000.000000000000000 ) ;
#2494=CARTESIAN_POINT ( 'NONE',  ( 14.55774661933062397, -3.136992222400443175, 32.19305428654138979 ) ) ;
#2496=CARTESIAN_POINT ( 'NONE',  ( -10.48459417441766206, -5.496552790871120031, 34.60292014791297532 ) ) ;
#2497=VERTEX_POINT ( 'NONE', #32307 ) ;
#2498=CARTESIAN_POINT ( 'NONE',  ( 17.32697738856139225, -12.17597550085003633, 31.52189283813461884 ) ) ;
#2499=CARTESIAN_POINT ( 'NONE',  ( 11.66925334628632882, -5.582136614379148654, 34.36778462344220486 ) ) ;
#2500=CARTESIAN_POINT ( 'NONE',  ( 9.942253210655836781, -6.696923467548660192, 34.68552623307873972 ) ) ;
#2501=CARTESIAN_POINT ( 'NONE',  ( 5.326868595271218254, -2.824170634883622188, 31.52227843825338738 ) ) ;
#2503=CARTESIAN_POINT ( 'NONE',  ( 4.087763774486019130, -3.322132147404559976, 32.92929555188719348 ) ) ;
#2504=CARTESIAN_POINT ( 'NONE',  ( 9.561616225640134914, -11.18331474514187995, 33.13161551792790505 ) ) ;
#2505=CARTESIAN_POINT ( 'NONE',  ( 8.519254038288414321, -10.66389620160130036, 33.62221079203477103 ) ) ;
#2507=CARTESIAN_POINT ( 'NONE',  ( 17.86930853333243974, -12.38065189839062263, 30.83690757178629482 ) ) ;
#2508=ORIENTED_EDGE ( 'NONE', *, *, #42310, .T. ) ;
#2509=VECTOR ( 'NONE', #35018, 1000.000000000000000 ) ;
#2510=ORIENTED_EDGE ( 'NONE', *, *, #84358, .T. ) ;
#2511=CARTESIAN_POINT ( 'NONE',  ( -6.130690603110307890, -12.62707690430377383, 30.88035979386743435 ) ) ;
#2514=CYLINDRICAL_SURFACE ( 'NONE', #76706, 0.2499999999999995559 ) ;
#2515=CYLINDRICAL_SURFACE ( 'NONE', #82657, 0.2500000000000002220 ) ;
#2516=ORIENTED_EDGE ( 'NONE', *, *, #79009, .T. ) ;
#2518=ORIENTED_EDGE ( 'NONE', *, *, #19738, .F. ) ;
#2520=EDGE_CURVE ( 'NONE', #84646, #4955, #55947, .T. ) ;
#2521=CYLINDRICAL_SURFACE ( 'NONE', #58800, 0.2500000000000008882 ) ;
#2522=FACE_OUTER_BOUND ( 'NONE', #16135, .T. ) ;
#2523=CARTESIAN_POINT ( 'NONE',  ( -2.307692307692305711, -1.117168528481311540, 33.14645433367849847 ) ) ;
#2524=EDGE_CURVE ( 'NONE', #37993, #5737, #83944, .T. ) ;
#2525=AXIS2_PLACEMENT_3D ( 'NONE', #15439, #15882, #9127 ) ;
#2526=CARTESIAN_POINT ( 'NONE',  ( 6.923076923076924238, -13.37000171582298513, 34.34916445242398453 ) ) ;
#2527=EDGE_CURVE ( 'NONE', #88852, #39806, #37607, .T. ) ;
#2529=VERTEX_POINT ( 'NONE', #21338 ) ;
#2533=AXIS2_PLACEMENT_3D ( 'NONE', #32136, #10977, #59152 ) ;
#2535=EDGE_LOOP ( 'NONE', ( #71781, #25472 ) ) ;
#2536=EDGE_CURVE ( 'NONE', #74452, #36240, #19433, .T. ) ;
#2537=CARTESIAN_POINT ( 'NONE',  ( 1.449870955891410906, -9.442884908240271713, 34.35708131394835618 ) ) ;
#2539=B_SPLINE_CURVE_WITH_KNOTS ( 'NONE', 3,
 ( #38395, #73068, #58654, #65416, #59102, #86149, #11366, #31183, #79835, #24420 ),
 .UNSPECIFIED., .F., .F.,
 ( 4, 2, 2, 2, 4 ),
 ( 0.0007817246256747450040, 0.0009771112852218872494, 0.001172497944769029278, 0.001367884604316171523, 0.001563271263863313769 ),
 .UNSPECIFIED. ) ;
#2540=CARTESIAN_POINT ( 'NONE',  ( 7.146088274689773812, -11.76359900205217457, 32.36225158514719880 ) ) ;
#2541=VERTEX_POINT ( 'NONE', #15034 ) ;
#2542=AXIS2_PLACEMENT_3D ( 'NONE', #17138, #23447, #84293 ) ;
#2543=EDGE_CURVE ( 'NONE', #3325, #1645, #76278, .T. ) ;
#2544=CARTESIAN_POINT ( 'NONE',  ( -14.98082382139119062, -12.45601412856602686, 31.48342859153981621 ) ) ;
#2545=ORIENTED_EDGE ( 'NONE', *, *, #27219, .F. ) ;
#2546=FACE_BOUND ( 'NONE', #81293, .T. ) ;
#2547=CARTESIAN_POINT ( 'NONE',  ( 15.36129466900287532, -11.66157788607254098, 32.95092075102925833 ) ) ;
#2548=CARTESIAN_POINT ( 'NONE',  ( 10.68145296638705410, -8.973038597847271092, 34.52809138561121216 ) ) ;
#2549=B_SPLINE_CURVE_WITH_KNOTS ( 'NONE', 3,
 ( #33079, #31756, #88493, #59213, #67756, #88062, #4271, #81279, #19562, #52451 ),
 .UNSPECIFIED., .F., .F.,
 ( 4, 2, 2, 2, 4 ),
 ( 0.000000000000000000, 0.0001954339857564080707, 0.0003908679715128161414, 0.0005863019572692241849, 0.0007817359430256322827 ),
 .UNSPECIFIED. ) ;
#2550=DIRECTION ( 'NONE',  ( 0.000000000000000000, 0.6427876096865368094, 0.7660444431189802339 ) ) ;
#2551=CYLINDRICAL_SURFACE ( 'NONE', #79179, 0.2499999999999973355 ) ;
#2552=DIRECTION ( 'NONE',  ( 0.000000000000000000, 0.8660254037844377084, 0.5000000000000015543 ) ) ;
#2553=CARTESIAN_POINT ( 'NONE',  ( -1.384615384615506484, -8.656820664282941280, 34.87096338111179961 ) ) ;
#2554=CARTESIAN_POINT ( 'NONE',  ( -10.68146802634049486, -10.51840700105979387, 33.73612834413961536 ) ) ;
#2555=EDGE_LOOP ( 'NONE', ( #62347, #89031 ) ) ;
#2556=CARTESIAN_POINT ( 'NONE',  ( -11.40766973063675316, -4.118422570099827595, 33.43335022499816489 ) ) ;
#2557=CYLINDRICAL_SURFACE ( 'NONE', #47928, 0.2500000000000004996 ) ;
#2558=VERTEX_POINT ( 'NONE', #42950 ) ;
#2559=CARTESIAN_POINT ( 'NONE',  ( -12.39628332202562433, -3.643525952247864463, 33.31231777344670064 ) ) ;
#2560=CARTESIAN_POINT ( 'NONE',  ( 15.23076923076911093, -4.481592998941358097, 33.73612834414048933 ) ) ;
#2562=CARTESIAN_POINT ( 'NONE',  ( -7.715363405186894674, -10.70102852606553157, 33.91149625220312913 ) ) ;
#2563=DIRECTION ( 'NONE',  ( 0.000000000000000000, 0.6427876096865373645, -0.7660444431189797898 ) ) ;
#2564=CARTESIAN_POINT ( 'NONE',  ( -7.596153846153782752, -7.434744860731433924, 35.00000000000000711 ) ) ;
#2565=FACE_BOUND ( 'NONE', #84441, .T. ) ;
#2566=CARTESIAN_POINT ( 'NONE',  ( 12.39626801557768587, -3.300289026998414865, 32.46337939537583139 ) ) ;
#2567=CYLINDRICAL_SURFACE ( 'NONE', #24453, 0.2499999999999995559 ) ;
#2568=CARTESIAN_POINT ( 'NONE',  ( 15.90386942290380290, -3.137211980971220893, 32.19342716148376837 ) ) ;
#2569=CARTESIAN_POINT ( 'NONE',  ( -7.780086512803769949, -12.62096338111211757, 30.90682066428152908 ) ) ;
#2570=CARTESIAN_POINT ( 'NONE',  ( -12.46153846153858247, -4.481592998941358097, 33.73612834414048933 ) ) ;
#2574=VERTEX_POINT ( 'NONE', #14584 ) ;
#2575=CYLINDRICAL_SURFACE ( 'NONE', #69438, 0.2500000000000002220 ) ;
#2577=AXIS2_PLACEMENT_3D ( 'NONE', #76, #55458, #42841 ) ;
#2578=CYLINDRICAL_SURFACE ( 'NONE', #19672, 0.2499999999999997502 ) ;
#2580=CARTESIAN_POINT ( 'NONE',  ( 16.85399611801622655, -8.282780595021769443, 34.94152052738834868 ) ) ;
#2581=CARTESIAN_POINT ( 'NONE',  ( 10.68145296638705588, -12.10708131394839704, 31.69288490824020954 ) ) ;
#2583=CARTESIAN_POINT ( 'NONE',  ( -11.53846153846153655, -3.513871655860378418, 32.76840700105978499 ) ) ;
#2584=B_SPLINE_CURVE_WITH_KNOTS ( 'NONE', 3,
 ( #49743, #63700, #1564, #56509, #43873, #16847, #70912, #78991, #29487, #22279 ),
 .UNSPECIFIED., .F., .F.,
 ( 4, 2, 2, 2, 4 ),
 ( 0.000000000000000000, 0.0001954339857564073659, 0.0003908679715128147319, 0.0005863019572692221250, 0.0007817359430256294638 ),
 .UNSPECIFIED. ) ;
#2585=LINE ( 'NONE', #16552, #25870 ) ;
#2586=EDGE_CURVE ( 'NONE', #40289, #76427, #56889, .T. ) ;
#2587=CARTESIAN_POINT ( 'NONE',  ( 3.453548899747297618, -4.226511098958374291, 33.85474049983370293 ) ) ;
#2588=CARTESIAN_POINT ( 'NONE',  ( -3.007756386675836335, -11.98016756924214832, 32.48728574198911190 ) ) ;
#2589=CARTESIAN_POINT ( 'NONE',  ( -16.82686865700962286, -4.818054556918155207, 34.26375889529406749 ) ) ;
#2590=CARTESIAN_POINT ( 'NONE',  ( 12.33139049180676672, -12.70455904226513866, 30.44083106164009322 ) ) ;
#2591=B_SPLINE_CURVE_WITH_KNOTS ( 'NONE', 3,
 ( #39787, #81215, #40675, #19500, #60927, #81656, #49633, #84766, #36566, #562 ),
 .UNSPECIFIED., .F., .F.,
 ( 4, 2, 2, 2, 4 ),
 ( 0.000000000000000000, 0.0001954339857564053873, 0.0003908679715128107746, 0.0005863019572692161618, 0.0007817359430256215491 ),
 .UNSPECIFIED. ) ;
#2592=CARTESIAN_POINT ( 'NONE',  ( -14.30769230769230660, -3.886160181151819604, 36.00935417666054406 ) ) ;
#2593=ADVANCED_FACE ( 'NONE', ( #36631 ), #40405, .F. ) ;
#2594=CARTESIAN_POINT ( 'NONE',  ( 17.32697749683652688, -2.544122305571458575, 31.48381861865057729 ) ) ;
#2595=EDGE_LOOP ( 'NONE', ( #64131, #30840, #58349, #12862 ) ) ;
#2596=CARTESIAN_POINT ( 'NONE',  ( 3.480714640147273720, -12.45601412856602686, 31.48342859153981621 ) ) ;
#2597=DIRECTION ( 'NONE',  ( -0.000000000000000000, 0.9396926207859093161, -0.3420201433256663259 ) ) ;
#2599=CARTESIAN_POINT ( 'NONE',  ( 8.769230769231075584, -2.506253911140615021, 30.00000000000323297 ) ) ;
#2600=VECTOR ( 'NONE', #70934, 1000.000000000000114 ) ;
#2601=CARTESIAN_POINT ( 'NONE',  ( -17.07692307692307665, -5.471508081941601098, 34.59228464037088457 ) ) ;
#2602=VERTEX_POINT ( 'NONE', #35297 ) ;
#2603=CARTESIAN_POINT ( 'NONE',  ( -16.21911615440247090, -4.320704448112772766, 33.92786785259540494 ) ) ;
#2604=CARTESIAN_POINT ( 'NONE',  ( 12.39626801557768587, -6.026961402152685388, 34.52809138561120506 ) ) ;
#2605=ORIENTED_EDGE ( 'NONE', *, *, #45005, .F. ) ;
#2606=CARTESIAN_POINT ( 'NONE',  ( 11.76124120743959978, -4.989023458446560255, 34.36081565061822118 ) ) ;
#2607=CARTESIAN_POINT ( 'NONE',  ( -13.31854703361294590, -9.780366693483667717, 34.19971097300155805 ) ) ;
#2609=DIRECTION ( 'NONE',  ( -0.000000000000000000, -0.3420201433256694346, -0.9396926207859080948 ) ) ;
#2610=CARTESIAN_POINT ( 'NONE',  ( -0.4615384615384611200, -2.538708090699994813, 30.37095296980875503 ) ) ;
#2611=ORIENTED_EDGE ( 'NONE', *, *, #6377, .T. ) ;
#2612=DIRECTION ( 'NONE',  ( -0.000000000000000000, 0.6427876096865404731, -0.7660444431189771253 ) ) ;
#2613=EDGE_CURVE ( 'NONE', #74655, #67341, #23714, .T. ) ;
#2614=EDGE_CURVE ( 'NONE', #84921, #11924, #49411, .T. ) ;
#2615=DIRECTION ( 'NONE',  ( -0.000000000000000000, 0.9848077530122085754, -0.1736481776669273613 ) ) ;
#2617=CARTESIAN_POINT ( 'NONE',  ( 12.46153846153833911, -12.16647553114689728, 32.15551576947799362 ) ) ;
#2618=VERTEX_POINT ( 'NONE', #78050 ) ;
#2619=ORIENTED_EDGE ( 'NONE', *, *, #44342, .T. ) ;
#2621=EDGE_LOOP ( 'NONE', ( #26570, #72888 ) ) ;
#2622=FACE_OUTER_BOUND ( 'NONE', #85958, .T. ) ;
#2624=CARTESIAN_POINT ( 'NONE',  ( -7.976630554270308870, -7.276988635370452485, 34.74523720219453793 ) ) ;
#2626=EDGE_LOOP ( 'NONE', ( #14256, #1573, #31480, #28064 ) ) ;
#2627=ORIENTED_EDGE ( 'NONE', *, *, #66914, .T. ) ;
#2628=CARTESIAN_POINT ( 'NONE',  ( 9.469381474791545017, -4.186968288167450147, 33.49512374952580274 ) ) ;
#2629=EDGE_LOOP ( 'NONE', ( #45771, #11641, #56818, #22527 ) ) ;
#2632=CARTESIAN_POINT ( 'NONE',  ( -15.23076923076922995, -3.050289026998446396, 32.03036669348365706 ) ) ;
#2633=CARTESIAN_POINT ( 'NONE',  ( 15.23076923076923173, -1.129524287112498415, 32.06866353760679544 ) ) ;
#2634=CARTESIAN_POINT ( 'NONE',  ( -8.546217925137375104, -12.64618726649961289, 30.78989965857442712 ) ) ;
#2635=ORIENTED_EDGE ( 'NONE', *, *, #88523, .T. ) ;
#2636=EDGE_LOOP ( 'NONE', ( #55609, #79230, #54953, #31412 ) ) ;
#2637=CARTESIAN_POINT ( 'NONE',  ( -8.769230769230890843, -8.613356846316285953, 34.62446782046622218 ) ) ;
#2638=ORIENTED_EDGE ( 'NONE', *, *, #61565, .F. ) ;
#2639=EDGE_CURVE ( 'NONE', #38598, #75373, #12873, .T. ) ;
#2640=CARTESIAN_POINT ( 'NONE',  ( -5.999999999999998224, -8.120952969808772792, 34.71129190930000163 ) ) ;
#2641=CARTESIAN_POINT ( 'NONE',  ( -10.68065461594093435, -9.528491918058357157, 34.59228464037090589 ) ) ;
#2642=ORIENTED_EDGE ( 'NONE', *, *, #72584, .F. ) ;
#2643=CARTESIAN_POINT ( 'NONE',  ( -6.700297254098856570, -4.989023458446560255, 34.36081565061822118 ) ) ;
#2644=CARTESIAN_POINT ( 'NONE',  ( 5.326977388561388693, -11.28795663066794219, 33.01431243580653785 ) ) ;
#2645=EDGE_CURVE ( 'NONE', #63578, #81582, #76378, .T. ) ;
#2646=CARTESIAN_POINT ( 'NONE',  ( 17.77651507543566112, -12.47654668319379567, 31.42292124445336654 ) ) ;
#2647=FACE_BOUND ( 'NONE', #52747, .T. ) ;
#2648=CARTESIAN_POINT ( 'NONE',  ( -8.519176349317316266, -2.318338780012835443, 30.59689888758630261 ) ) ;
#2649=CARTESIAN_POINT ( 'NONE',  ( 4.023155550735845409, -2.295517848115769421, 30.44137282052136939 ) ) ;
#2650=CARTESIAN_POINT ( 'NONE',  ( -12.46153846153846168, -4.661471528628507777, 34.16647553114623292 ) ) ;
#2652=FACE_OUTER_BOUND ( 'NONE', #80909, .T. ) ;
#2653=DIRECTION ( 'NONE',  ( 0.000000000000000000, 1.000000000000000000, 0.000000000000000000 ) ) ;
#2654=CARTESIAN_POINT ( 'NONE',  ( -16.15384615384615330, -8.564572088678739092, 35.78748833219616898 ) ) ;
#2655=ORIENTED_EDGE ( 'NONE', *, *, #11058, .F. ) ;
#2656=CARTESIAN_POINT ( 'NONE',  ( 14.05769230769230838, -7.566083408709835645, 34.74999999999999289 ) ) ;
#2657=ORIENTED_EDGE ( 'NONE', *, *, #2937, .T. ) ;
#2658=ORIENTED_EDGE ( 'NONE', *, *, #76196, .T. ) ;
#2659=CARTESIAN_POINT ( 'NONE',  ( -1.384615384615383471, -4.661471528628507777, 34.16647553114623292 ) ) ;
#2660=CARTESIAN_POINT ( 'NONE',  ( 10.74617505635156789, -12.62708834333097663, 30.88030960425257021 ) ) ;
#2661=ADVANCED_FACE ( 'NONE', ( #24423 ), #30310, .F. ) ;
#2663=CARTESIAN_POINT ( 'NONE',  ( 13.31934538405906565, -11.67786785259540849, 32.92929555188721480 ) ) ;
#2664=FACE_OUTER_BOUND ( 'NONE', #68760, .T. ) ;
#2665=CARTESIAN_POINT ( 'NONE',  ( 2.307692307692309264, -2.292212530054420494, 30.41441678777542634 ) ) ;
#2666=CARTESIAN_POINT ( 'NONE',  ( -3.930833309752757021, -3.395485233115139057, 33.02377354290275946 ) ) ;
#2669=DIRECTION ( 'NONE',  ( -0.000000000000000000, -0.5000000000000009992, -0.8660254037844380415 ) ) ;
#2670=CARTESIAN_POINT ( 'NONE',  ( 17.14217864819909920, -6.879047030191284051, 34.71129190930002295 ) ) ;
#2671=CARTESIAN_POINT ( 'NONE',  ( 12.46153846153846168, -10.89733346790207413, 36.13435417666054406 ) ) ;
#2673=B_SPLINE_CURVE_WITH_KNOTS ( 'NONE', 3,
 ( #54549, #5499, #81161, #61300, #5939, #55005, #33411, #81600, #48238, #13573 ),
 .UNSPECIFIED., .F., .F.,
 ( 4, 2, 2, 2, 4 ),
 ( 0.0007817359430256253438, 0.0009771253907249898181, 0.001172514838424354401, 0.001367904286123718983, 0.001563293733823083566 ),
 .UNSPECIFIED. ) ;
#2675=ORIENTED_EDGE ( 'NONE', *, *, #66910, .T. ) ;
#2676=ADVANCED_FACE ( 'NONE', ( #72621 ), #10929, .F. ) ;
#2677=B_SPLINE_CURVE_WITH_KNOTS ( 'NONE', 3,
 ( #60763, #27425, #19783, #53108, #53560, #54898, #20230, #89148, #41386, #26098 ),
 .UNSPECIFIED., .F., .F.,
 ( 4, 2, 2, 2, 4 ),
 ( 0.0007817246256747444619, 0.0009771112852218868158, 0.001172497944769029061, 0.001367884604316171523, 0.001563271263863313769 ),
 .UNSPECIFIED. ) ;
#2679=CARTESIAN_POINT ( 'NONE',  ( 14.30769230769231015, -12.34228464037088635, 31.77849191805839268 ) ) ;
#2681=ORIENTED_EDGE ( 'NONE', *, *, #20197, .T. ) ;
#2682=CARTESIAN_POINT ( 'NONE',  ( -18.24999999999999645, -7.566083408709835645, 34.74999999999999289 ) ) ;
#2683=FACE_OUTER_BOUND ( 'NONE', #70992, .T. ) ;
#2684=CARTESIAN_POINT ( 'NONE',  ( 4.023698184114455678, -11.04286588640298561, 33.62463336215343901 ) ) ;
#2685=CARTESIAN_POINT ( 'NONE',  ( 17.32692307692449418, -7.500000000000154543, 35.00000000000007105 ) ) ;
#2688=ORIENTED_EDGE ( 'NONE', *, *, #11664, .T. ) ;
#2689=DIRECTION ( 'NONE',  ( -0.000000000000000000, -0.3420201433256694346, -0.9396926207859080948 ) ) ;
#2690=CYLINDRICAL_SURFACE ( 'NONE', #46803, 0.2500000000000012212 ) ;
#2691=ORIENTED_EDGE ( 'NONE', *, *, #69342, .T. ) ;
#2692=CARTESIAN_POINT ( 'NONE',  ( 7.846153846153846700, -12.78798330534102767, 29.49999999999997868 ) ) ;
#2693=CYLINDRICAL_SURFACE ( 'NONE', #8473, 0.2499999999999995559 ) ;
#2694=CARTESIAN_POINT ( 'NONE',  ( 11.28848480751918437, -4.236021600441997492, 33.53823185664189310 ) ) ;
#2695=CARTESIAN_POINT ( 'NONE',  ( 13.38461538461526423, -5.094484230521993062, 34.41647553114689373 ) ) ;
#2696=EDGE_CURVE ( 'NONE', #75758, #57723, #22604, .T. ) ;
#2697=CARTESIAN_POINT ( 'NONE',  ( -12.46153846153858247, -12.46129190930018460, 30.37095296980731973 ) ) ;
#2698=CARTESIAN_POINT ( 'NONE',  ( -8.096130577096200653, -12.41269422305637171, 30.68257228309993323 ) ) ;
#2701=CARTESIAN_POINT ( 'NONE',  ( 1.254468175177166245, -6.001485441113818986, 34.52039167877662607 ) ) ;
#2702=CARTESIAN_POINT ( 'NONE',  ( -13.45069879557126136, -8.973038597847271092, 34.52809138561120506 ) ) ;
#2704=CARTESIAN_POINT ( 'NONE',  ( -3.480745961711583902, -9.148715823498378086, 34.47080413974185120 ) ) ;
#2705=CARTESIAN_POINT ( 'NONE',  ( -0.4615384615384611200, -8.810774026931790459, 35.74407628777942847 ) ) ;
#2706=ORIENTED_EDGE ( 'NONE', *, *, #48885, .F. ) ;
#2707=CARTESIAN_POINT ( 'NONE',  ( 7.846153846153846700, -11.91647553114624181, 32.58852847137148245 ) ) ;
#2708=CARTESIAN_POINT ( 'NONE',  ( -1.384615384615505151, -10.21337939537710326, 33.94971097300076224 ) ) ;
#2709=EDGE_CURVE ( 'NONE', #24126, #59899, #50573, .T. ) ;
#2710=EDGE_LOOP ( 'NONE', ( #44549, #61475 ) ) ;
#2711=CARTESIAN_POINT ( 'NONE',  ( -4.087778820496077437, -2.486705287966279876, 31.30864560766543647 ) ) ;
#2712=ORIENTED_EDGE ( 'NONE', *, *, #58714, .F. ) ;
#2713=B_SPLINE_CURVE_WITH_KNOTS ( 'NONE', 3,
 ( #5377, #47686, #39172, #75171, #40937, #21088, #84151, #28754, #41378, #14796 ),
 .UNSPECIFIED., .F., .F.,
 ( 4, 2, 2, 2, 4 ),
 ( 0.000000000000000000, 0.0001954311564186866305, 0.0003908623128373732609, 0.0005862934692560598914, 0.0007817246256747465219 ),
 .UNSPECIFIED. ) ;
#2714=CARTESIAN_POINT ( 'NONE',  ( 14.53047184896071720, -12.24180327182771855, 31.33663988360758879 ) ) ;
#2715=ADVANCED_FACE ( 'NONE', ( #59551 ), #68098, .F. ) ;
#2717=CARTESIAN_POINT ( 'NONE',  ( 3.903822916553188360, -3.711651800289232028, 33.01384336483936011 ) ) ;
#2718=CARTESIAN_POINT ( 'NONE',  ( -6.923076923076922462, -3.669653830205710676, 35.88435417666054406 ) ) ;
#2719=CARTESIAN_POINT ( 'NONE',  ( -4.403869378067612139, -11.56360843649121861, 33.07473185843129926 ) ) ;
#2720=ORIENTED_EDGE ( 'NONE', *, *, #37888, .T. ) ;
#2721=DIRECTION ( 'NONE',  ( 0.000000000000000000, 0.1736481776669275834, 0.9848077530122086864 ) ) ;
#2722=B_SPLINE_CURVE_WITH_KNOTS ( 'NONE', 3,
 ( #41589, #47448, #6910, #88916, #46571, #60968, #34383, #54645, #88041, #39825 ),
 .UNSPECIFIED., .F., .F.,
 ( 4, 2, 2, 2, 4 ),
 ( 0.000000000000000000, 0.0001954339857564099951, 0.0003908679715128199903, 0.0005863019572692300396, 0.0007817359430256399806 ),
 .UNSPECIFIED. ) ;
#2723=B_SPLINE_CURVE_WITH_KNOTS ( 'NONE', 3,
 ( #81048, #47241, #13021, #74735, #12582, #61193, #54442, #67082, #72942, #11699 ),
 .UNSPECIFIED., .F., .F.,
 ( 4, 2, 2, 2, 4 ),
 ( 0.0007817359430256294638, 0.0009771253907249941549, 0.001172514838424358954, 0.001367904286123723754, 0.001563293733823095492 ),
 .UNSPECIFIED. ) ;
#2726=FACE_OUTER_BOUND ( 'NONE', #35318, .T. ) ;
#2727=CARTESIAN_POINT ( 'NONE',  ( -10.61538461538461320, -2.721908614388771852, 31.22303859784724978 ) ) ;
#2728=ORIENTED_EDGE ( 'NONE', *, *, #2297, .T. ) ;
#2729=CARTESIAN_POINT ( 'NONE',  ( 11.76147438255493149, -12.64618726649961289, 30.78989965857442712 ) ) ;
#2730=LINE ( 'NONE', #51339, #60800 ) ;
#2731=CARTESIAN_POINT ( 'NONE',  ( -11.76138849736838488, -2.889293201056495786, 32.26117774369186009 ) ) ;
#2733=CARTESIAN_POINT ( 'NONE',  ( -39.05038313613820122, -2.499999999999999556, 29.75000000000000355 ) ) ;
#2734=AXIS2_PLACEMENT_3D ( 'NONE', #8121, #83342, #7234 ) ;
#2735=EDGE_LOOP ( 'NONE', ( #63554, #63257 ) ) ;
#2736=ORIENTED_EDGE ( 'NONE', *, *, #87918, .T. ) ;
#2737=FACE_BOUND ( 'NONE', #6199, .T. ) ;
#2738=VERTEX_POINT ( 'NONE', #87056 ) ;
#2739=CARTESIAN_POINT ( 'NONE',  ( -8.638438961405979555, -4.118422570099831148, 33.43335022499816489 ) ) ;
#2740=FACE_OUTER_BOUND ( 'NONE', #35708, .T. ) ;
#2741=CARTESIAN_POINT ( 'NONE',  ( -14.30769230769230660, -8.973038597847269315, 34.52809138561121927 ) ) ;
#2743=ORIENTED_EDGE ( 'NONE', *, *, #84313, .T. ) ;
#2744=B_SPLINE_CURVE_WITH_KNOTS ( 'NONE', 3,
 ( #66752, #80732, #11363, #17683, #38393, #31638, #4150, #18573, #59546, #52338 ),
 .UNSPECIFIED., .F., .F.,
 ( 4, 2, 2, 2, 4 ),
 ( 0.000000000000000000, 0.0001954311564186862781, 0.0003908623128373725562, 0.0005862934692560588072, 0.0007817246256747451124 ),
 .UNSPECIFIED. ) ;
#2745=ORIENTED_EDGE ( 'NONE', *, *, #43114, .T. ) ;
#2746=CARTESIAN_POINT ( 'NONE',  ( 0.3308478584281538404, -8.191372820521381826, 34.95448215188423546 ) ) ;
#2747=EDGE_LOOP ( 'NONE', ( #44824, #22707 ) ) ;
#2748=B_SPLINE_CURVE_WITH_KNOTS ( 'NONE', 3,
 ( #48164, #34661, #62131, #35551, #27903, #62995, #14386, #47730, #54932, #54034 ),
 .UNSPECIFIED., .F., .F.,
 ( 4, 2, 2, 2, 4 ),
 ( 0.000000000000000000, 0.0001954311564186878773, 0.0003908623128373757546, 0.0005862934692560635777, 0.0007817246256747515092 ),
 .UNSPECIFIED. ) ;
#2749=CARTESIAN_POINT ( 'NONE',  ( -10.61538461538473577, -8.656820664282941280, 34.87096338111179961 ) ) ;
#2750=B_SPLINE_CURVE_WITH_KNOTS ( 'NONE', 3,
 ( #76419, #34979, #21015, #29130, #70095, #14721, #69655, #68331, #54812, #75971 ),
 .UNSPECIFIED., .F., .F.,
 ( 4, 2, 2, 2, 4 ),
 ( 0.000000000000000000, 0.0001954339857564092362, 0.0003908679715128184724, 0.0005863019572692276544, 0.0007817359430256369448 ),
 .UNSPECIFIED. ) ;
#2751=CARTESIAN_POINT ( 'NONE',  ( 2.980745993476266342, -2.823816976329320827, 31.52131813110797154 ) ) ;
#2752=VECTOR ( 'NONE', #29953, 1000.000000000000114 ) ;
#2753=CARTESIAN_POINT ( 'NONE',  ( 17.01165307636676260, -3.643525952247789856, 33.31231777344662959 ) ) ;
#2754=FACE_BOUND ( 'NONE', #11158, .T. ) ;
#2755=ORIENTED_EDGE ( 'NONE', *, *, #33766, .F. ) ;
#2756=CARTESIAN_POINT ( 'NONE',  ( 13.38461538461538680, -10.67929555188718282, 33.92786785259544047 ) ) ;
#2757=CARTESIAN_POINT ( 'NONE',  ( -15.00775638667583500, -3.395485233115139057, 33.02377354290275946 ) ) ;
#2758=DIRECTION ( 'NONE',  ( 0.000000000000000000, 0.9396926207859126468, -0.3420201433256571111 ) ) ;
#2759=CARTESIAN_POINT ( 'NONE',  ( 8.769230769230768274, -6.343179335718451384, 34.87096338111211935 ) ) ;
#2760=ORIENTED_EDGE ( 'NONE', *, *, #10928, .T. ) ;
#2761=EDGE_LOOP ( 'NONE', ( #60057, #78188, #11316, #9953 ) ) ;
#2762=ORIENTED_EDGE ( 'NONE', *, *, #79178, .F. ) ;
#2764=CARTESIAN_POINT ( 'NONE',  ( 6.923076923076924238, -5.180354513474913603, 36.12317359536750416 ) ) ;
#2765=CARTESIAN_POINT ( 'NONE',  ( -8.769230769230768274, -12.34228464037088635, 31.77849191805839268 ) ) ;
#2766=CARTESIAN_POINT ( 'NONE',  ( -13.38461538461550759, -3.083524468854526912, 32.58852847137268327 ) ) ;
#2767=CARTESIAN_POINT ( 'NONE',  ( 7.846153846153725020, -12.46129190930018460, 30.37095296980731973 ) ) ;
#2768=CARTESIAN_POINT ( 'NONE',  ( -6.988346923633241836, -3.643525952247789412, 33.31231777344662959 ) ) ;
#2769=ORIENTED_EDGE ( 'NONE', *, *, #52930, .T. ) ;
#2770=DIRECTION ( 'NONE',  ( 1.000000000000000000, 0.000000000000000000, 0.000000000000000000 ) ) ;
#2771=CARTESIAN_POINT ( 'NONE',  ( -4.153846153846152411, -8.164416787775445883, 34.95778746994557906 ) ) ;
#2772=DIRECTION ( 'NONE',  ( -0.000000000000000000, -0.7660444431189791237, -0.6427876096865379196 ) ) ;
#2773=CARTESIAN_POINT ( 'NONE',  ( -3.930834802233303282, -3.587049720035815792, 32.86302985866382897 ) ) ;
#2774=EDGE_LOOP ( 'NONE', ( #81169, #56402, #25840, #28505 ) ) ;
#2775=ORIENTED_EDGE ( 'NONE', *, *, #6683, .F. ) ;
#2776=FACE_BOUND ( 'NONE', #49924, .T. ) ;
#2777=ADVANCED_FACE ( 'NONE', ( #66757 ), #33425, .F. ) ;
#2778=B_SPLINE_CURVE_WITH_KNOTS ( 'NONE', 3,
 ( #40848, #42622, #21899, #7945, #2066, #48030, #69637, #48471, #7506, #41735 ),
 .UNSPECIFIED., .F., .F.,
 ( 4, 2, 2, 2, 4 ),
 ( 0.0007817359430256319575, 0.0009771253907250002264, 0.001172514838424368495, 0.001367904286123736764, 0.001563293733823097878 ),
 .UNSPECIFIED. ) ;
#2779=AXIS2_PLACEMENT_3D ( 'NONE', #42906, #41565, #69038 ) ;
#2780=B_SPLINE_CURVE_WITH_KNOTS ( 'NONE', 3,
 ( #55747, #35937, #84134, #22410, #43132, #84573, #64266, #27841, #76475, #14777 ),
 .UNSPECIFIED., .F., .F.,
 ( 4, 2, 2, 2, 4 ),
 ( 0.000000000000000000, 0.0001954339857564076641, 0.0003908679715128153282, 0.0005863019572692229923, 0.0007817359430256306564 ),
 .UNSPECIFIED. ) ;
#2782=CARTESIAN_POINT ( 'NONE',  ( -7.146561847641254239, -10.23692288466677880, 34.23039457007281072 ) ) ;
#2783=CARTESIAN_POINT ( 'NONE',  ( 12.39626801557768943, -12.27809138561121394, 31.22303859784730307 ) ) ;
#2784=B_SPLINE_CURVE_WITH_KNOTS ( 'NONE', 3,
 ( #65951, #37427, #70791, #37882, #36981, #43748, #64010, #51814, #23468, #58583 ),
 .UNSPECIFIED., .F., .F.,
 ( 4, 2, 2, 2, 4 ),
 ( 0.000000000000000000, 0.0001954339857564078538, 0.0003908679715128157077, 0.0005863019572692235344, 0.0007817359430256314154 ),
 .UNSPECIFIED. ) ;
#2786=B_SPLINE_CURVE_WITH_KNOTS ( 'NONE', 3,
 ( #61848, #46132, #40718, #11912, #39388, #40273, #66845, #39826, #33512, #5589 ),
 .UNSPECIFIED., .F., .F.,
 ( 4, 2, 2, 2, 4 ),
 ( 0.000000000000000000, 0.0001954311564186861697, 0.0003908623128373723394, 0.0005862934692560584820, 0.0007817246256747446788 ),
 .UNSPECIFIED. ) ;
#2787=CARTESIAN_POINT ( 'NONE',  ( -3.230769230769351186, -12.46129190930018460, 30.37095296980731973 ) ) ;
#2788=CARTESIAN_POINT ( 'NONE',  ( 6.856993512121043466, -10.51840700105979387, 33.73612834413961536 ) ) ;
#2789=CARTESIAN_POINT ( 'NONE',  ( 8.545745844666436497, -2.353723527008296568, 30.78948104536958752 ) ) ;
#2790=DIRECTION ( 'NONE',  ( 0.000000000000000000, 0.9848077530122072432, 0.1736481776669354937 ) ) ;
#2793=AXIS2_PLACEMENT_3D ( 'NONE', #16606, #50821, #77431 ) ;
#2794=CARTESIAN_POINT ( 'NONE',  ( -7.596208327805704208, -10.76462480002816235, 33.53768742498949962 ) ) ;
#2795=ORIENTED_EDGE ( 'NONE', *, *, #80548, .T. ) ;
#2798=ORIENTED_EDGE ( 'NONE', *, *, #32188, .F. ) ;
#2799=CARTESIAN_POINT ( 'NONE',  ( -8.519230769230832223, -7.565270445406050648, 34.75000000000000000 ) ) ;
#2800=CARTESIAN_POINT ( 'NONE',  ( 15.10062202133100939, -2.882441371585227508, 31.66841991370172238 ) ) ;
#2801=FACE_OUTER_BOUND ( 'NONE', #26415, .T. ) ;
#2802=CARTESIAN_POINT ( 'NONE',  ( -14.30769230769230660, -1.790695186598648903, 34.54067556320373455 ) ) ;
#2803=LINE ( 'NONE', #58194, #86523 ) ;
#2804=EDGE_CURVE ( 'NONE', #84823, #52632, #35549, .T. ) ;
#2805=CARTESIAN_POINT ( 'NONE',  ( 6.250054311638318261, -2.779044189368096163, 31.39831045268886456 ) ) ;
#2807=ORIENTED_EDGE ( 'NONE', *, *, #6581, .T. ) ;
#2808=CARTESIAN_POINT ( 'NONE',  ( 13.38461538461538680, -12.62096338111211580, 30.90682066428153263 ) ) ;
#2809=CARTESIAN_POINT ( 'NONE',  ( 5.749976775778544713, -8.475808217655753651, 34.90892951860618609 ) ) ;
#2810=VERTEX_POINT ( 'NONE', #18579 ) ;
#2811=ORIENTED_EDGE ( 'NONE', *, *, #67110, .F. ) ;
#2812=ORIENTED_EDGE ( 'NONE', *, *, #12957, .F. ) ;
#2813=CARTESIAN_POINT ( 'NONE',  ( 5.076923076923075762, -13.88283147151868846, 33.14645433367849847 ) ) ;
#2814=CARTESIAN_POINT ( 'NONE',  ( 12.46153846153833911, -4.320704448113951379, 33.92786785259630022 ) ) ;
#2815=CARTESIAN_POINT ( 'NONE',  ( -1.384615384615505151, -9.442884908241554243, 34.35708131394783038 ) ) ;
#2816=CARTESIAN_POINT ( 'NONE',  ( 9.469381474791545017, -12.39988816332205701, 30.74660775122750778 ) ) ;
#2817=CYLINDRICAL_SURFACE ( 'NONE', #76173, 0.2499999999999998890 ) ;
#2818=CARTESIAN_POINT ( 'NONE',  ( -8.899922235898328537, -11.71456829005830080, 32.44064028649416542 ) ) ;
#2819=ORIENTED_EDGE ( 'NONE', *, *, #30073, .F. ) ;
#2820=CARTESIAN_POINT ( 'NONE',  ( -12.46153846153846168, -1.044019251281081972, 31.83374038241031911 ) ) ;
#2821=CARTESIAN_POINT ( 'NONE',  ( -0.3962828902624374594, -8.613356846314930593, 34.62446782046653482 ) ) ;
#2822=EDGE_CURVE ( 'NONE', #23412, #71441, #83887, .T. ) ;
#2823=B_SPLINE_CURVE_WITH_KNOTS ( 'NONE', 3,
 ( #67906, #41318, #34994, #49404, #7974, #35441, #61133, #81871, #34559, #68345 ),
 .UNSPECIFIED., .F., .F.,
 ( 4, 2, 2, 2, 4 ),
 ( 0.0007817246256747519429, 0.0009771112852218970073, 0.001172497944769042288, 0.001367884604316187353, 0.001563271263863332417 ),
 .UNSPECIFIED. ) ;
#2824=CARTESIAN_POINT ( 'NONE',  ( 9.019230769230768274, -2.499999999999998668, 29.75000000000000355 ) ) ;
#2825=B_SPLINE_CURVE_WITH_KNOTS ( 'NONE', 3,
 ( #73146, #11445, #4694, #32165, #59626, #87126, #40703, #60516, #39813, #49107 ),
 .UNSPECIFIED., .F., .F.,
 ( 4, 2, 2, 2, 4 ),
 ( 0.000000000000000000, 0.0001954311584214072923, 0.0003908623168428145846, 0.0005862934752642218498, 0.0007817246336856291692 ),
 .UNSPECIFIED. ) ;
#2826=CARTESIAN_POINT ( 'NONE',  ( 7.911409417429871027, -2.892918686051624722, 31.69288490824025928 ) ) ;
#2829=CARTESIAN_POINT ( 'NONE',  ( 9.692307692307695177, -13.04860791097971706, 34.73218667398347037 ) ) ;
#2830=ORIENTED_EDGE ( 'NONE', *, *, #48090, .T. ) ;
#2831=EDGE_CURVE ( 'NONE', #67219, #84018, #82059, .T. ) ;
#2832=CARTESIAN_POINT ( 'NONE',  ( 12.23805353697413167, -9.417330523894424488, 34.63758898049880486 ) ) ;
#2833=DIRECTION ( 'NONE',  ( -0.000000000000000000, 0.9396926207859092051, -0.3420201433256662704 ) ) ;
#2834=CARTESIAN_POINT ( 'NONE',  ( 6.130790440966952026, -12.62708834333097663, 30.88030960425257021 ) ) ;
#2835=VERTEX_POINT ( 'NONE', #88385 ) ;
#2837=LINE ( 'NONE', #57795, #85406 ) ;
#2838=CYLINDRICAL_SURFACE ( 'NONE', #21101, 0.2499999999999997502 ) ;
#2839=CARTESIAN_POINT ( 'NONE',  ( -12.21148414990014786, -10.66356715214248396, 33.62249196103329751 ) ) ;
#2840=ORIENTED_EDGE ( 'NONE', *, *, #874, .F. ) ;
#2841=AXIS2_PLACEMENT_3D ( 'NONE', #69835, #8142, #63062 ) ;
#2842=CARTESIAN_POINT ( 'NONE',  ( -0.5276218724943421146, -8.120952969808774569, 34.71129190930000163 ) ) ;
#2844=DIRECTION ( 'NONE',  ( -0.000000000000000000, 0.3420201433256694346, -0.9396926207859080948 ) ) ;
#2845=B_SPLINE_CURVE_WITH_KNOTS ( 'NONE', 3,
 ( #70032, #43451, #71800, #30816, #16423, #44310, #29502, #78120, #10104, #84451 ),
 .UNSPECIFIED., .F., .F.,
 ( 4, 2, 2, 2, 4 ),
 ( 0.0007817359430256314154, 0.0009771253907249980580, 0.001172514838424364592, 0.001367904286123731127, 0.001563293733823097661 ),
 .UNSPECIFIED. ) ;
#2846=AXIS2_PLACEMENT_3D ( 'NONE', #87239, #18319, #88136 ) ;
#2847=AXIS2_PLACEMENT_3D ( 'NONE', #8327, #35803, #63258 ) ;
#2848=CARTESIAN_POINT ( 'NONE',  ( -16.82697766754503377, -3.520799739797214389, 33.17531984108286025 ) ) ;
#2849=CARTESIAN_POINT ( 'NONE',  ( -1.450697763975518972, -9.058645607665454236, 34.76329471203372634 ) ) ;
#2850=CARTESIAN_POINT ( 'NONE',  ( -9.942330916529147800, -8.475808217655753651, 34.90892951860618609 ) ) ;
#2851=CARTESIAN_POINT ( 'NONE',  ( 15.10007776410167679, -11.71456829005830080, 32.44064028649416542 ) ) ;
#2854=VERTEX_POINT ( 'NONE', #54118 ) ;
#2856=VERTEX_POINT ( 'NONE', #75296 ) ;
#2857=CARTESIAN_POINT ( 'NONE',  ( -10.48459280755982981, -8.147973898785416225, 34.70805048591653730 ) ) ;
#2858=CARTESIAN_POINT ( 'NONE',  ( 16.15384615384615330, -5.471508081941601098, 34.59228464037088457 ) ) ;
#2859=CARTESIAN_POINT ( 'NONE',  ( -4.023320715612507925, -6.808710257144159783, 34.95449254468098843 ) ) ;
#2860=CARTESIAN_POINT ( 'NONE',  ( -0.4615384615385840772, -4.320704448113951379, 33.92786785259630022 ) ) ;
#2861=CARTESIAN_POINT ( 'NONE',  ( 7.846153846153846700, -12.62096338111211580, 30.90682066428153263 ) ) ;
#2862=CARTESIAN_POINT ( 'NONE',  ( 11.47319109250076608, -12.27809138561121394, 31.22303859784730307 ) ) ;
#2863=CARTESIAN_POINT ( 'NONE',  ( -8.769230769230768274, -2.499999999999998668, 29.75000000000001421 ) ) ;
#2864=CARTESIAN_POINT ( 'NONE',  ( -4.087777802843715946, -10.51840700105979565, 33.73612834413962247 ) ) ;
#2865=ORIENTED_EDGE ( 'NONE', *, *, #67406, .F. ) ;
#2866=ORIENTED_EDGE ( 'NONE', *, *, #19475, .T. ) ;
#2868=ORIENTED_EDGE ( 'NONE', *, *, #61951, .T. ) ;
#2870=ORIENTED_EDGE ( 'NONE', *, *, #10012, .F. ) ;
#2871=CARTESIAN_POINT ( 'NONE',  ( -11.53846153846153655, -3.937682226553329556, 33.60647404775216529 ) ) ;
#2872=CARTESIAN_POINT ( 'NONE',  ( 10.39189967166066708, -9.331801661448606566, 34.40259984581193464 ) ) ;
#2873=CARTESIAN_POINT ( 'NONE',  ( 1.634669804528839476, -4.818054556918156983, 34.26375889529406749 ) ) ;
#2875=VERTEX_POINT ( 'NONE', #53684 ) ;
#2876=B_SPLINE_CURVE_WITH_KNOTS ( 'NONE', 3,
 ( #34488, #62826, #8801, #20962, #69165, #7470, #28169, #36272, #63284, #1594 ),
 .UNSPECIFIED., .F., .F.,
 ( 4, 2, 2, 2, 4 ),
 ( 0.000000000000000000, 0.0001954339857564064444, 0.0003908679715128128888, 0.0005863019572692193060, 0.0007817359430256257775 ),
 .UNSPECIFIED. ) ;
#2877=AXIS2_PLACEMENT_3D ( 'NONE', #82482, #82034, #13124 ) ;
#2878=ORIENTED_EDGE ( 'NONE', *, *, #4475, .T. ) ;
#2879=CARTESIAN_POINT ( 'NONE',  ( -11.60373153901785948, -12.16647553114622049, 32.15551576947930812 ) ) ;
#2880=ORIENTED_EDGE ( 'NONE', *, *, #32246, .T. ) ;
#2881=FACE_BOUND ( 'NONE', #12925, .T. ) ;
#2882=CARTESIAN_POINT ( 'NONE',  ( 3.453782074862625784, -2.523321265292116422, 31.42251411153756990 ) ) ;
#2883=ADVANCED_FACE ( 'NONE', ( #25775 ), #11824, .F. ) ;
#2884=CARTESIAN_POINT ( 'NONE',  ( 8.769230769230645706, -8.656820664282941280, 34.87096338111179961 ) ) ;
#2886=CARTESIAN_POINT ( 'NONE',  ( 16.40390046548447245, -11.28795663066794575, 33.01431243580653785 ) ) ;
#2887=DIRECTION ( 'NONE',  ( -0.000000000000000000, 0.1736481776669307198, -0.9848077530122080203 ) ) ;
#2888=LINE ( 'NONE', #77675, #65136 ) ;
#2889=ORIENTED_EDGE ( 'NONE', *, *, #40562, .T. ) ;
#2891=CARTESIAN_POINT ( 'NONE',  ( 17.74999999999999645, -7.566082377512564960, 35.00000000000000711 ) ) ;
#2892=LINE ( 'NONE', #35821, #25065 ) ;
#2893=VERTEX_POINT ( 'NONE', #80737 ) ;
#2894=CARTESIAN_POINT ( 'NONE',  ( 3.453780582382080411, -8.239487800360276282, 34.69522927552633718 ) ) ;
#2895=DIRECTION ( 'NONE',  ( -0.000000000000000000, 1.000000000000000000, 3.491481338843133355E-15 ) ) ;
#2896=CYLINDRICAL_SURFACE ( 'NONE', #31059, 0.2500000000000002220 ) ;
#2897=CARTESIAN_POINT ( 'NONE',  ( -2.437839517130525824, -2.619462340734462380, 30.83744416345203021 ) ) ;
#2898=CARTESIAN_POINT ( 'NONE',  ( 5.869852790561781219, -5.195881422630167279, 34.18770438780618548 ) ) ;
#2899=DIRECTION ( 'NONE',  ( 0.000000000000000000, -6.938893903907222067E-15, 1.000000000000000000 ) ) ;
#2900=CARTESIAN_POINT ( 'NONE',  ( 8.096099255531889582, -2.986452184633680673, 32.43230066228895225 ) ) ;
#2901=CARTESIAN_POINT ( 'NONE',  ( 4.219101725122178514, -12.27809138561124591, 31.22303859784720359 ) ) ;
#2902=DIRECTION ( 'NONE',  ( -0.000000000000000000, 0.6427876096865404731, -0.7660444431189770143 ) ) ;
#2903=AXIS2_PLACEMENT_3D ( 'NONE', #6235, #19298, #81009 ) ;
#2905=CARTESIAN_POINT ( 'NONE',  ( 18.00000000000000000, -1.629998284177014645, 34.34916445242399163 ) ) ;
#2906=CARTESIAN_POINT ( 'NONE',  ( 12.21153846153846168, -7.500000000000001776, 35.00000000000000000 ) ) ;
#2907=DIRECTION ( 'NONE',  ( 0.000000000000000000, 0.000000000000000000, 1.000000000000000000 ) ) ;
#2910=ORIENTED_EDGE ( 'NONE', *, *, #31657, .T. ) ;
#2911=DIRECTION ( 'NONE',  ( -0.000000000000000000, -0.3420201433256694346, -0.9396926207859080948 ) ) ;
#2912=ORIENTED_EDGE ( 'NONE', *, *, #70528, .T. ) ;
#2914=VECTOR ( 'NONE', #77739, 1000.000000000000114 ) ;
#2916=CARTESIAN_POINT ( 'NONE',  ( 9.627037246346919375, -6.879047030191174805, 34.71129190930000163 ) ) ;
#2917=VERTEX_POINT ( 'NONE', #60440 ) ;
#2918=CARTESIAN_POINT ( 'NONE',  ( 17.86985279056177589, -12.27039167877662251, 31.24851455888617835 ) ) ;
#2919=B_SPLINE_CURVE_WITH_KNOTS ( 'NONE', 3,
 ( #59947, #75248, #40143, #33810, #61264, #39250, #80231, #19409, #46876, #27498 ),
 .UNSPECIFIED., .F., .F.,
 ( 4, 2, 2, 2, 4 ),
 ( 0.0007817359430256219828, 0.0009771253907249863487, 0.001172514838424350498, 0.001367904286123714647, 0.001563293733823079013 ),
 .UNSPECIFIED. ) ;
#2920=EDGE_LOOP ( 'NONE', ( #70504, #51298, #18508, #75672 ) ) ;
#2921=CARTESIAN_POINT ( 'NONE',  ( -8.069080063669989755, -5.667676309546437530, 34.40238873228292249 ) ) ;
#2923=CARTESIAN_POINT ( 'NONE',  ( 7.780883845597525550, -8.656820664281498878, 34.87096338111211935 ) ) ;
#2924=VECTOR ( 'NONE', #62953, 1000.000000000000227 ) ;
#2925=CARTESIAN_POINT ( 'NONE',  ( 6.699591979352976345, -11.41268669641500466, 32.86336882939237825 ) ) ;
#2926=CARTESIAN_POINT ( 'NONE',  ( 7.145856592054988354, -10.23759521482555357, 34.22997729860117033 ) ) ;
#2927=CARTESIAN_POINT ( 'NONE',  ( -8.769230769230768274, -3.886160181151819604, 36.00935417666054406 ) ) ;
#2929=B_SPLINE_CURVE_WITH_KNOTS ( 'NONE', 3,
 ( #55591, #83080, #16380, #15948, #9197, #57364, #8753, #1097, #49284, #50151 ),
 .UNSPECIFIED., .F., .F.,
 ( 4, 2, 2, 2, 4 ),
 ( 0.000000000000000000, 0.0001954339857564079623, 0.0003908679715128159245, 0.0005863019572692238597, 0.0007817359430256318490 ),
 .UNSPECIFIED. ) ;
#2930=CARTESIAN_POINT ( 'NONE',  ( 15.16468685140909578, -8.164416787775445883, 34.95778746994557906 ) ) ;
#2931=CARTESIAN_POINT ( 'NONE',  ( -13.38461538461550759, -8.656820664282941280, 34.87096338111179961 ) ) ;
#2932=CARTESIAN_POINT ( 'NONE',  ( -2.307692307692427391, -5.219633306517616589, 34.19971097300220464 ) ) ;
#2934=CARTESIAN_POINT ( 'NONE',  ( -16.15384615384615330, -13.87047571288749737, 32.06866353760679544 ) ) ;
#2935=DIRECTION ( 'NONE',  ( -0.000000000000000000, 0.9848077530122086864, -0.1736481776669273891 ) ) ;
#2936=EDGE_CURVE ( 'NONE', #32904, #66010, #47339, .T. ) ;
#2937=EDGE_CURVE ( 'NONE', #62741, #43377, #7279, .T. ) ;
#2938=DIRECTION ( 'NONE',  ( -0.000000000000000000, -0.9396926207859093161, -0.3420201433256663259 ) ) ;
#2940=ORIENTED_EDGE ( 'NONE', *, *, #74648, .T. ) ;
#2941=EDGE_CURVE ( 'NONE', #9090, #7426, #31222, .T. ) ;
#2942=CARTESIAN_POINT ( 'NONE',  ( -13.51530598772569469, -6.369640206132551441, 34.87707690430378449 ) ) ;
#2943=FACE_OUTER_BOUND ( 'NONE', #39032, .T. ) ;
#2944=CARTESIAN_POINT ( 'NONE',  ( 1.253924781505078689, -5.496505350115500121, 34.60290016733514307 ) ) ;
#2945=CARTESIAN_POINT ( 'NONE',  ( 18.22301135161285046, -10.61302985866384141, 33.66295027996417843 ) ) ;
#2946=ADVANCED_FACE ( 'NONE', ( #1847 ), #63540, .F. ) ;
#2947=CARTESIAN_POINT ( 'NONE',  ( 15.48076923077066702, -7.500000000000155431, 34.75000000000007105 ) ) ;
#2948=CARTESIAN_POINT ( 'NONE',  ( -8.835314180186648159, -8.120952969808774569, 34.71129190930000163 ) ) ;
#2949=ORIENTED_EDGE ( 'NONE', *, *, #30482, .T. ) ;
#2950=CYLINDRICAL_SURFACE ( 'NONE', #55857, 0.2500000000000004996 ) ;
#2951=VERTEX_POINT ( 'NONE', #524 ) ;
#2952=B_SPLINE_CURVE_WITH_KNOTS ( 'NONE', 3,
 ( #22080, #49551, #15328, #7238, #36044, #34709, #22518, #41916, #56745, #29289 ),
 .UNSPECIFIED., .F., .F.,
 ( 4, 2, 2, 2, 4 ),
 ( 0.0007817359430256232838, 0.0009771253907249928539, 0.001172514838424355485, 0.001367904286123718116, 0.001563293733823080747 ),
 .UNSPECIFIED. ) ;
#2954=ORIENTED_EDGE ( 'NONE', *, *, #25673, .F. ) ;
#2955=CARTESIAN_POINT ( 'NONE',  ( -8.769230769230768274, -1.242168528481310874, 33.36296068462461051 ) ) ;
#2956=CARTESIAN_POINT ( 'NONE',  ( -16.15384615384627409, -12.51329471203414379, 31.30864560766407578 ) ) ;
#2957=CARTESIAN_POINT ( 'NONE',  ( -8.992157728137616601, -2.308479472611653094, 30.53278059502174457 ) ) ;
#2958=B_SPLINE_CURVE_WITH_KNOTS ( 'NONE', 3,
 ( #18821, #38643, #80073, #87294, #39989, #60238, #46287, #88632, #6194, #53479 ),
 .UNSPECIFIED., .F., .F.,
 ( 4, 2, 2, 2, 4 ),
 ( 0.000000000000000000, 0.0001954339857564080165, 0.0003908679715128160329, 0.0005863019572692240765, 0.0007817359430256320659 ),
 .UNSPECIFIED. ) ;
#2959=CARTESIAN_POINT ( 'NONE',  ( -6.000000000000119904, -3.300289026999228881, 32.46337939537708905 ) ) ;
#2960=LINE ( 'NONE', #30443, #61035 ) ;
#2961=ORIENTED_EDGE ( 'NONE', *, *, #9294, .F. ) ;
#2962=CARTESIAN_POINT ( 'NONE',  ( -5.999999999999998224, -5.180354513474913603, 36.12317359536750416 ) ) ;
#2963=VERTEX_POINT ( 'NONE', #28432 ) ;
#2964=ADVANCED_FACE ( 'NONE', ( #83390 ), #15371, .F. ) ;
#2965=ORIENTED_EDGE ( 'NONE', *, *, #31612, .F. ) ;
#2967=CARTESIAN_POINT ( 'NONE',  ( -6.988346923633243613, -12.16647553114622049, 32.15551576947930812 ) ) ;
#2968=CARTESIAN_POINT ( 'NONE',  ( -4.153846153846152411, -7.500000000000001776, 35.04278698407183867 ) ) ;
#2969=EDGE_CURVE ( 'NONE', #38795, #49416, #67773, .T. ) ;
#2970=FACE_OUTER_BOUND ( 'NONE', #88818, .T. ) ;
#2971=AXIS2_PLACEMENT_3D ( 'NONE', #88227, #19741, #47202 ) ;
#2973=EDGE_CURVE ( 'NONE', #71975, #46832, #35641, .T. ) ;
#2974=CARTESIAN_POINT ( 'NONE',  ( -11.76138849736838488, -8.282780595021769443, 34.94152052738834158 ) ) ;
#2975=CARTESIAN_POINT ( 'NONE',  ( -12.46153846153858424, -5.941354392335915335, 34.76329471203413846 ) ) ;
#2976=VERTEX_POINT ( 'NONE', #76172 ) ;
#2977=EDGE_LOOP ( 'NONE', ( #77447, #33383 ) ) ;
#2980=EDGE_CURVE ( 'NONE', #66580, #66677, #10823, .T. ) ;
#2981=EDGE_LOOP ( 'NONE', ( #73358, #79094, #78240, #84210 ) ) ;
#2982=CARTESIAN_POINT ( 'NONE',  ( 15.23076923076910916, -10.33852847137269571, 34.16647553114546554 ) ) ;
#2983=VERTEX_POINT ( 'NONE', #41956 ) ;
#2985=DIRECTION ( 'NONE',  ( -0.000000000000000000, -0.000000000000000000, -1.000000000000000000 ) ) ;
#2986=DIRECTION ( 'NONE',  ( -0.000000000000000000, 0.6427876096865404731, -0.7660444431189771253 ) ) ;
#2988=ORIENTED_EDGE ( 'NONE', *, *, #38854, .T. ) ;
#2989=CARTESIAN_POINT ( 'NONE',  ( 10.61538461538449418, -2.379036618888197729, 30.90682066428292885 ) ) ;
#2990=ORIENTED_EDGE ( 'NONE', *, *, #9445, .F. ) ;
#2991=CARTESIAN_POINT ( 'NONE',  ( -3.230769230769229949, -1.367168528481310208, 33.57946703557072254 ) ) ;
#2992=CARTESIAN_POINT ( 'NONE',  ( 6.923076923076924238, -5.471508081941601098, 34.59228464037088457 ) ) ;
#2993=DIRECTION ( 'NONE',  ( -0.000000000000000000, -0.9848077530122085754, -0.1736481776669273613 ) ) ;
#2994=CARTESIAN_POINT ( 'NONE',  ( 14.98076923076923173, -7.500000000000001776, 34.75000000000000000 ) ) ;
#2995=CARTESIAN_POINT ( 'NONE',  ( 5.076923076922954969, -3.300289026999228881, 32.46337939537708905 ) ) ;
#2996=CARTESIAN_POINT ( 'NONE',  ( -0.6850233861027943405, -12.47654668319379567, 31.42292124445336654 ) ) ;
#2997=DIRECTION ( 'NONE',  ( -0.000000000000000000, -0.000000000000000000, -1.000000000000000000 ) ) ;
#2998=ORIENTED_EDGE ( 'NONE', *, *, #80490, .F. ) ;
#2999=CARTESIAN_POINT ( 'NONE',  ( -11.53846153846165912, -12.27809138561165270, 31.22303859784587132 ) ) ;
#3000=LINE ( 'NONE', #16972, #69460 ) ;
#3001=B_SPLINE_CURVE_WITH_KNOTS ( 'NONE', 3,
 ( #20656, #75593, #13898, #34618, #62514, #27858 ),
 .UNSPECIFIED., .F., .F.,
 ( 4, 2, 4 ),
 ( 4.220987180333913997E-17, 0.0001954756301637161793, 0.0003909512603273901832 ),
 .UNSPECIFIED. ) ;
#3002=ADVANCED_FACE ( 'NONE', ( #20785 ), #48253, .F. ) ;
#3003=EDGE_LOOP ( 'NONE', ( #83634, #75850, #22090, #9340 ) ) ;
#3005=CARTESIAN_POINT ( 'NONE',  ( 10.54930120442873687, -6.386643153685125363, 34.62446782046654903 ) ) ;
#3006=CARTESIAN_POINT ( 'NONE',  ( -15.90390063549801347, -10.76462480002816413, 33.53768742498949962 ) ) ;
#3007=CARTESIAN_POINT ( 'NONE',  ( 2.307692307692186251, -5.941354392335915335, 34.76329471203413846 ) ) ;
#3008=DIRECTION ( 'NONE',  ( -0.000000000000000000, 0.9848077530122085754, -0.1736481776669273613 ) ) ;
#3009=CARTESIAN_POINT ( 'NONE',  ( -7.596153846152425615, -7.500000000000154543, 35.00000000000007105 ) ) ;
#3010=FACE_BOUND ( 'NONE', #2372, .T. ) ;
#3011=CARTESIAN_POINT ( 'NONE',  ( 5.076923076923075762, -5.471508081941601098, 34.59228464037088457 ) ) ;
#3012=CARTESIAN_POINT ( 'NONE',  ( 18.00000000000000000, -10.67929555188718282, 33.92786785259544047 ) ) ;
#3013=CARTESIAN_POINT ( 'NONE',  ( 4.153846153846154188, -13.53365097954675988, 30.81389545987213552 ) ) ;
#3014=CARTESIAN_POINT ( 'NONE',  ( -6.857009589726848375, -10.67929555188718282, 33.92786785259544757 ) ) ;
#3015=CARTESIAN_POINT ( 'NONE',  ( 14.17700170458200581, -10.70098750199973203, 33.91152734681376302 ) ) ;
#3017=CARTESIAN_POINT ( 'NONE',  ( 8.769230769230647482, -10.90142922262034020, 33.41473453929536674 ) ) ;
#3019=EDGE_LOOP ( 'NONE', ( #83513, #66737 ) ) ;
#3020=DIRECTION ( 'NONE',  ( 0.000000000000000000, 0.1736481776669275834, 0.9848077530122086864 ) ) ;
#3021=CARTESIAN_POINT ( 'NONE',  ( -5.076923076923197442, -3.300289026999228881, 32.46337939537708905 ) ) ;
#3022=CARTESIAN_POINT ( 'NONE',  ( -18.00000000000012079, -9.442884908241554243, 34.35708131394783038 ) ) ;
#3023=DIRECTION ( 'NONE',  ( -0.000000000000000000, 0.5000000000000011102, -0.8660254037844380415 ) ) ;
#3024=CARTESIAN_POINT ( 'NONE',  ( 10.83839596699746721, -12.15243808032445827, 31.58219941686247978 ) ) ;
#3025=LINE ( 'NONE', #76147, #16719 ) ;
#3027=CARTESIAN_POINT ( 'NONE',  ( -8.638438961405986660, -2.729792928343269587, 31.24908615093345077 ) ) ;
#3028=DIRECTION ( 'NONE',  ( 1.000000000000000000, 0.000000000000000000, 0.000000000000000000 ) ) ;
#3030=CARTESIAN_POINT ( 'NONE',  ( 17.86943940825807076, -2.504760397472873823, 29.97295953869789997 ) ) ;
#3031=B_SPLINE_CURVE_WITH_KNOTS ( 'NONE', 3,
 ( #18980, #66721, #87458, #60398, #75686, #87916, #82468, #68059, #75257, #54526 ),
 .UNSPECIFIED., .F., .F.,
 ( 4, 2, 2, 2, 4 ),
 ( 0.0007817246256747480398, 0.0009771112852218900684, 0.001172497944769032314, 0.001367884604316174559, 0.001563271263863316588 ),
 .UNSPECIFIED. ) ;
#3032=CARTESIAN_POINT ( 'NONE',  ( -17.07692307692319744, -5.094484230521993062, 34.41647553114689373 ) ) ;
#3033=CARTESIAN_POINT ( 'NONE',  ( 10.74542977821939260, -2.504778602574659896, 29.97347330155780654 ) ) ;
#3034=B_SPLINE_CURVE_WITH_KNOTS ( 'NONE', 3,
 ( #76400, #88617, #55676, #34530, #61110, #83167, #82728, #26889, #48927, #61995 ),
 .UNSPECIFIED., .F., .F.,
 ( 4, 2, 2, 2, 4 ),
 ( 0.000000000000000000, 0.0001954339857564126514, 0.0003908679715128183098, 0.0005863019572692239681, 0.0007817359430256294638 ),
 .UNSPECIFIED. ) ;
#3035=CYLINDRICAL_SURFACE ( 'NONE', #60594, 2.000000000000001776 ) ;
#3036=EDGE_CURVE ( 'NONE', #82729, #4757, #74139, .T. ) ;
#3037=ADVANCED_FACE ( 'NONE', ( #17126 ), #59001, .F. ) ;
#3038=CARTESIAN_POINT ( 'NONE',  ( -4.153846153846152411, -3.513871655860378418, 32.76840700105978499 ) ) ;
#3041=CARTESIAN_POINT ( 'NONE',  ( 7.053602624840485724, -5.195472089885680766, 34.18748526763464923 ) ) ;
#3043=EDGE_CURVE ( 'NONE', #43765, #49073, #43042, .T. ) ;
#3045=DIRECTION ( 'NONE',  ( -0.000000000000000000, -0.7660444431189791237, -0.6427876096865379196 ) ) ;
#3046=CARTESIAN_POINT ( 'NONE',  ( -16.94613263595612551, -5.496552790871120031, 34.60292014791297532 ) ) ;
#3047=ORIENTED_EDGE ( 'NONE', *, *, #34476, .F. ) ;
#3049=FACE_OUTER_BOUND ( 'NONE', #71413, .T. ) ;
#3050=EDGE_LOOP ( 'NONE', ( #74419, #33768, #65001, #74676 ) ) ;
#3051=CARTESIAN_POINT ( 'NONE',  ( -11.47326755667818077, -2.506253911140448487, 29.99999999999988631 ) ) ;
#3052=CARTESIAN_POINT ( 'NONE',  ( 17.20697051217352680, -7.723484941389743952, 34.99544897038808955 ) ) ;
#3053=EDGE_CURVE ( 'NONE', #22156, #16798, #60255, .T. ) ;
#3054=CARTESIAN_POINT ( 'NONE',  ( -6.923076923076922462, -4.945431358278436385, 36.03766855953609394 ) ) ;
#3055=VECTOR ( 'NONE', #65184, 999.9999999999998863 ) ;
#3056=FACE_OUTER_BOUND ( 'NONE', #7180, .T. ) ;
#3058=B_SPLINE_CURVE_WITH_KNOTS ( 'NONE', 3,
 ( #66267, #85218, #44647, #51387, #38358, #23498, #31141, #9545, #50954, #78444 ),
 .UNSPECIFIED., .F., .F.,
 ( 4, 2, 2, 2, 4 ),
 ( 0.000000000000000000, 0.0001954311564186862510, 0.0003908623128373725020, 0.0005862934692560588072, 0.0007817246256747450040 ),
 .UNSPECIFIED. ) ;
#3059=CARTESIAN_POINT ( 'NONE',  ( -13.38461538461538325, -12.29105614889573062, 35.45975837776705220 ) ) ;
#3061=CARTESIAN_POINT ( 'NONE',  ( 4.023154687178593925, -9.804603061927743113, 34.18744698557895845 ) ) ;
#3062=EDGE_LOOP ( 'NONE', ( #62395, #37464 ) ) ;
#3064=EDGE_CURVE ( 'NONE', #65231, #2602, #79730, .T. ) ;
#3065=ORIENTED_EDGE ( 'NONE', *, *, #78363, .F. ) ;
#3066=CARTESIAN_POINT ( 'NONE',  ( -18.06527044596078113, -3.835265460703606522, 33.15142922261924241 ) ) ;
#3067=CARTESIAN_POINT ( 'NONE',  ( -3.164701897419154530, -2.833524468853757750, 32.15551576947925838 ) ) ;
#3068=EDGE_CURVE ( 'NONE', #78512, #17646, #30111, .T. ) ;
#3069=FACE_OUTER_BOUND ( 'NONE', #47658, .T. ) ;
#3070=CARTESIAN_POINT ( 'NONE',  ( -17.75000000000000000, -7.500000000000001776, 35.00000000000000000 ) ) ;
#3071=VECTOR ( 'NONE', #44190, 1000.000000000000114 ) ;
#3072=ADVANCED_FACE ( 'NONE', ( #64412 ), #51781, .F. ) ;
#3073=ORIENTED_EDGE ( 'NONE', *, *, #9713, .T. ) ;
#3075=CARTESIAN_POINT ( 'NONE',  ( 15.23076923076911093, -5.219633306517616589, 34.19971097300220464 ) ) ;
#3076=ORIENTED_EDGE ( 'NONE', *, *, #247, .T. ) ;
#3078=ADVANCED_FACE ( 'NONE', ( #71181 ), #23000, .F. ) ;
#3079=DIRECTION ( 'NONE',  ( 0.000000000000000000, 0.1736481776669275834, 0.9848077530122086864 ) ) ;
#3080=CARTESIAN_POINT ( 'NONE',  ( 2.372947878968333146, -3.835265460703683349, 33.15142922261929925 ) ) ;
#3081=DIRECTION ( 'NONE',  ( 0.000000000000000000, 0.000000000000000000, -1.000000000000000000 ) ) ;
#3082=ORIENTED_EDGE ( 'NONE', *, *, #34856, .T. ) ;
#3083=B_SPLINE_CURVE_WITH_KNOTS ( 'NONE', 3,
 ( #77215, #42992, #62361, #7879, #77656, #70910, #9215, #48853, #36680, #2433 ),
 .UNSPECIFIED., .F., .F.,
 ( 4, 2, 2, 2, 4 ),
 ( 0.0007817246256747473893, 0.0009771112852218905021, 0.001172497944769033615, 0.001367884604316176944, 0.001563271263863320057 ),
 .UNSPECIFIED. ) ;
#3085=B_SPLINE_CURVE_WITH_KNOTS ( 'NONE', 3,
 ( #84963, #70107, #21479, #75982, #2089, #8418, #48950, #14281, #70997, #29577 ),
 .UNSPECIFIED., .F., .F.,
 ( 4, 2, 2, 2, 4 ),
 ( 0.000000000000000000, 0.0001954339857564083417, 0.0003908679715128166835, 0.0005863019572692250523, 0.0007817359430256333669 ),
 .UNSPECIFIED. ) ;
#3086=ORIENTED_EDGE ( 'NONE', *, *, #86630, .F. ) ;
#3087=CARTESIAN_POINT ( 'NONE',  ( -6.923076923077044142, -11.48612834414049644, 32.76840700105863391 ) ) ;
#3088=ORIENTED_EDGE ( 'NONE', *, *, #36649, .F. ) ;
#3090=DIRECTION ( 'NONE',  ( -0.000000000000000000, 1.000000000000000000, -0.000000000000000000 ) ) ;
#3092=EDGE_CURVE ( 'NONE', #55585, #60558, #72966, .T. ) ;
#3094=CARTESIAN_POINT ( 'NONE',  ( -14.08467946359890988, -12.64618726649961289, 30.78989965857442712 ) ) ;
#3096=FACE_BOUND ( 'NONE', #78501, .T. ) ;
#3097=CARTESIAN_POINT ( 'NONE',  ( -11.53846153846153655, -2.538708090699994813, 30.37095296980875503 ) ) ;
#3098=CARTESIAN_POINT ( 'NONE',  ( -6.857009589726848375, -9.058645607665452459, 34.76329471203371924 ) ) ;
#3100=CARTESIAN_POINT ( 'NONE',  ( -10.61538461538461320, -6.435427911321262684, 35.78748833219616898 ) ) ;
#3101=CARTESIAN_POINT ( 'NONE',  ( 3.230769230769231726, -3.322132147404559976, 32.92929555188717927 ) ) ;
#3103=CARTESIAN_POINT ( 'NONE',  ( -1.384615384615383471, -2.499999999999998668, 29.75000000000001421 ) ) ;
#3104=CARTESIAN_POINT ( 'NONE',  ( 5.326868595271218254, -2.587454068350147462, 30.68340429815432202 ) ) ;
#3105=ORIENTED_EDGE ( 'NONE', *, *, #72228, .F. ) ;
#3106=CARTESIAN_POINT ( 'NONE',  ( -5.869474298236434073, -11.93748526763465279, 32.05452791011430946 ) ) ;
#3107=ORIENTED_EDGE ( 'NONE', *, *, #61059, .F. ) ;
#3108=EDGE_CURVE ( 'NONE', #83058, #40235, #5404, .T. ) ;
#3109=ORIENTED_EDGE ( 'NONE', *, *, #59134, .F. ) ;
#3110=LINE ( 'NONE', #10770, #87836 ) ;
#3111=CARTESIAN_POINT ( 'NONE',  ( 1.449870524128225258, -5.941354392334606160, 34.76329471203374055 ) ) ;
#3112=EDGE_CURVE ( 'NONE', #44980, #72129, #11267, .T. ) ;
#3113=CARTESIAN_POINT ( 'NONE',  ( 2.438484115517094875, -2.541949514083463590, 30.39797389878540557 ) ) ;
#3114=DIRECTION ( 'NONE',  ( -0.000000000000000000, 0.9848077530122086864, -0.1736481776669273891 ) ) ;
#3115=DIRECTION ( 'NONE',  ( 0.000000000000000000, 0.7660444431189807890, 0.6427876096865361433 ) ) ;
#3116=CARTESIAN_POINT ( 'NONE',  ( 14.55774672760576394, -11.47946981652013498, 33.17500667209847620 ) ) ;
#3117=ORIENTED_EDGE ( 'NONE', *, *, #10410, .F. ) ;
#3119=CARTESIAN_POINT ( 'NONE',  ( 0.4615384615384611200, -12.62096338111211580, 30.90682066428153263 ) ) ;
#3120=CARTESIAN_POINT ( 'NONE',  ( -12.46153846153858247, -5.219633306517616589, 34.19971097300220464 ) ) ;
#3121=CARTESIAN_POINT ( 'NONE',  ( 14.30769230769218581, -3.643525952248795718, 33.31231777344771672 ) ) ;
#3123=B_SPLINE_CURVE_WITH_KNOTS ( 'NONE', 3,
 ( #31922, #38668, #66131, #4435, #59383, #40465, #27380, #81449, #7552, #6229 ),
 .UNSPECIFIED., .F., .F.,
 ( 4, 2, 2, 2, 4 ),
 ( 0.0007817359430256294638, 0.0009771253907249974075, 0.001172514838424365460, 0.001367904286123733295, 0.001563293733823094191 ),
 .UNSPECIFIED. ) ;
#3125=ORIENTED_EDGE ( 'NONE', *, *, #60449, .T. ) ;
#3126=ORIENTED_EDGE ( 'NONE', *, *, #24364, .T. ) ;
#3127=DIRECTION ( 'NONE',  ( -0.000000000000000000, 0.6427876096865404731, -0.7660444431189771253 ) ) ;
#3129=CARTESIAN_POINT ( 'NONE',  ( 17.29970274590113632, -4.226511098958373402, 33.85474049983370293 ) ) ;
#3130=CARTESIAN_POINT ( 'NONE',  ( 18.13052570176355971, -6.001044277235009439, 34.52024696741798948 ) ) ;
#3131=CYLINDRICAL_SURFACE ( 'NONE', #63952, 0.2500000000000009437 ) ;
#3132=LINE ( 'NONE', #58081, #1139 ) ;
#3134=CARTESIAN_POINT ( 'NONE',  ( 14.24160992833217065, -6.343179335718451384, 34.87096338111212646 ) ) ;
#3135=ORIENTED_EDGE ( 'NONE', *, *, #46165, .F. ) ;
#3137=CARTESIAN_POINT ( 'NONE',  ( -1.161604033002533454, -9.086983370893047862, 34.49168942202179267 ) ) ;
#3138=ORIENTED_EDGE ( 'NONE', *, *, #86303, .T. ) ;
#3139=DIRECTION ( 'NONE',  ( -0.000000000000000000, 1.000000000000000000, -0.000000000000000000 ) ) ;
#3140=CARTESIAN_POINT ( 'NONE',  ( 3.480714749117372442, -2.824170634883621744, 31.52227843825338738 ) ) ;
#3141=AXIS2_PLACEMENT_3D ( 'NONE', #53306, #32596, #73605 ) ;
#3142=CARTESIAN_POINT ( 'NONE',  ( 2.242421861731533017, -3.300289026998414865, 32.46337939537583139 ) ) ;
#3143=CARTESIAN_POINT ( 'NONE',  ( -8.769230769230768274, -2.249999999999998668, 29.75000000000001776 ) ) ;
#3144=FACE_OUTER_BOUND ( 'NONE', #55607, .T. ) ;
#3145=CARTESIAN_POINT ( 'NONE',  ( -4.403822884788507253, -9.148715823498378086, 34.47080413974185120 ) ) ;
#3146=CARTESIAN_POINT ( 'NONE',  ( -7.173053654019278191, -4.943428324936578910, 34.04746400365624481 ) ) ;
#3147=VECTOR ( 'NONE', #77172, 1000.000000000000114 ) ;
#3149=EDGE_LOOP ( 'NONE', ( #52160, #54596, #79589, #55688 ) ) ;
#3150=CARTESIAN_POINT ( 'NONE',  ( -16.15384615384615330, -9.058645607665452459, 34.76329471203371924 ) ) ;
#3151=CARTESIAN_POINT ( 'NONE',  ( -13.38461538461550759, -10.33852847137269571, 34.16647553114546554 ) ) ;
#3152=FACE_OUTER_BOUND ( 'NONE', #73334, .T. ) ;
#3155=CARTESIAN_POINT ( 'NONE',  ( -6.923076923076922462, -1.117168528481311540, 33.14645433367849847 ) ) ;
#3156=CARTESIAN_POINT ( 'NONE',  ( 15.90386940979756858, -4.818429247618089661, 34.26397095200675125 ) ) ;
#3157=ORIENTED_EDGE ( 'NONE', *, *, #17944, .F. ) ;
#3159=CARTESIAN_POINT ( 'NONE',  ( -1.384615384615506484, -12.51329471203414379, 31.30864560766407578 ) ) ;
#3160=EDGE_CURVE ( 'NONE', #47174, #67701, #53718, .T. ) ;
#3161=EDGE_LOOP ( 'NONE', ( #12682, #65661, #23637, #63398 ) ) ;
#3162=CARTESIAN_POINT ( 'NONE',  ( -4.283994123577847368, -8.630895178749536711, 34.87696386517710323 ) ) ;
#3163=EDGE_CURVE ( 'NONE', #58504, #53160, #9512, .T. ) ;
#3164=VERTEX_POINT ( 'NONE', #88289 ) ;
#3165=CARTESIAN_POINT ( 'NONE',  ( 6.923076923076924238, -3.937682226553329556, 33.60647404775216529 ) ) ;
#3166=CARTESIAN_POINT ( 'NONE',  ( 4.023154687178593036, -3.530157926970578508, 32.79014554554150607 ) ) ;
#3167=B_SPLINE_CURVE_WITH_KNOTS ( 'NONE', 3,
 ( #65046, #31733, #87139, #25415, #16874, #38040, #65504, #31282, #10118, #44323 ),
 .UNSPECIFIED., .F., .F.,
 ( 4, 2, 2, 2, 4 ),
 ( 0.0007817359527651089775, 0.0009771254036996502267, 0.001172514854634191693, 0.001367904305568727955, 0.001563293756503264216 ),
 .UNSPECIFIED. ) ;
#3168=CARTESIAN_POINT ( 'NONE',  ( 16.82694633287449193, -6.524016743844656574, 34.90889640711025521 ) ) ;
#3169=ORIENTED_EDGE ( 'NONE', *, *, #12308, .F. ) ;
#3170=CARTESIAN_POINT ( 'NONE',  ( -14.55769230769230660, -7.500000000000001776, 35.00000000000000000 ) ) ;
#3171=B_SPLINE_CURVE_WITH_KNOTS ( 'NONE', 3,
 ( #20875, #36185, #63634, #22212, #41600, #49679, #84369, #69508, #7815, #7377 ),
 .UNSPECIFIED., .F., .F.,
 ( 4, 2, 2, 2, 4 ),
 ( 0.000000000000000000, 0.0001954339881912775425, 0.0003908679763825550850, 0.0005863019645738326005, 0.0007817359527651101701 ),
 .UNSPECIFIED. ) ;
#3172=ORIENTED_EDGE ( 'NONE', *, *, #77886, .F. ) ;
#3173=EDGE_CURVE ( 'NONE', #29450, #36333, #27884, .T. ) ;
#3174=CARTESIAN_POINT ( 'NONE',  ( -5.749945580086545327, -2.318338780012835443, 30.59689888758630261 ) ) ;
#3175=B_SPLINE_CURVE_WITH_KNOTS ( 'NONE', 3,
 ( #72834, #58423, #16562, #2161, #85918, #31414, #57992, #37721, #45360, #85037 ),
 .UNSPECIFIED., .F., .F.,
 ( 4, 2, 2, 2, 4 ),
 ( 0.000000000000000000, 0.0001954311564186865763, 0.0003908623128373731525, 0.0005862934692560596746, 0.0007817246256747463051 ),
 .UNSPECIFIED. ) ;
#3176=AXIS2_PLACEMENT_3D ( 'NONE', #38592, #66048, #79133 ) ;
#3177=ORIENTED_EDGE ( 'NONE', *, *, #74398, .F. ) ;
#3179=CARTESIAN_POINT ( 'NONE',  ( -18.00000000000000000, -11.91647553114624358, 32.58852847137147535 ) ) ;
#3180=CARTESIAN_POINT ( 'NONE',  ( 12.59206416330202849, -12.27024696741798770, 31.24895572276497546 ) ) ;
#3181=ORIENTED_EDGE ( 'NONE', *, *, #60176, .T. ) ;
#3182=CARTESIAN_POINT ( 'NONE',  ( 8.519207545009313876, -4.931416488878822335, 34.32920672191015399 ) ) ;
#3183=CARTESIAN_POINT ( 'NONE',  ( -12.68502340526241312, -5.912607949931405926, 34.49155766932282319 ) ) ;
#3186=ADVANCED_FACE ( 'NONE', ( #80175 ), #39196, .F. ) ;
#3187=CARTESIAN_POINT ( 'NONE',  ( -14.17690186672535901, -9.929761469519743144, 34.40412654351204225 ) ) ;
#3189=EDGE_LOOP ( 'NONE', ( #70282, #29367 ) ) ;
#3190=ORIENTED_EDGE ( 'NONE', *, *, #858, .T. ) ;
#3191=VERTEX_POINT ( 'NONE', #18475 ) ;
#3192=CARTESIAN_POINT ( 'NONE',  ( -7.911423846710166075, -5.941354392334499579, 34.76329471203369792 ) ) ;
#3193=ORIENTED_EDGE ( 'NONE', *, *, #45330, .F. ) ;
#3194=EDGE_CURVE ( 'NONE', #16561, #39467, #55788, .T. ) ;
#3196=CARTESIAN_POINT ( 'NONE',  ( 13.38461538461538680, -10.51840700105979565, 33.73612834413961536 ) ) ;
#3197=CARTESIAN_POINT ( 'NONE',  ( -14.05763799605399278, -9.148310452688876993, 34.47095581063188519 ) ) ;
#3198=EDGE_LOOP ( 'NONE', ( #48782, #56070 ) ) ;
#3199=ORIENTED_EDGE ( 'NONE', *, *, #33265, .T. ) ;
#3201=DIRECTION ( 'NONE',  ( -0.000000000000000000, -0.3420201433256694346, -0.9396926207859080948 ) ) ;
#3202=ORIENTED_EDGE ( 'NONE', *, *, #59874, .F. ) ;
#3203=VECTOR ( 'NONE', #28287, 1000.000000000000227 ) ;
#3204=B_SPLINE_CURVE_WITH_KNOTS ( 'NONE', 3,
 ( #84488, #85369, #63754, #84051, #71392, #28651, #22763, #36730, #64184, #2489 ),
 .UNSPECIFIED., .F., .F.,
 ( 4, 2, 2, 2, 4 ),
 ( 0.000000000000000000, 0.0001954311564186861968, 0.0003908623128373723936, 0.0005862934692560585904, 0.0007817246256747447872 ),
 .UNSPECIFIED. ) ;
#3205=CARTESIAN_POINT ( 'NONE',  ( 11.76147289007438701, -11.24521262558773493, 33.06293181088029343 ) ) ;
#3206=EDGE_CURVE ( 'NONE', #79207, #29486, #51450, .T. ) ;
#3207=CARTESIAN_POINT ( 'NONE',  ( 4.153846153846030731, -12.70778746994576025, 30.41441678777401236 ) ) ;
#3209=CARTESIAN_POINT ( 'NONE',  ( 14.30769230769231015, -11.91647553114624181, 32.58852847137148245 ) ) ;
#3210=FACE_BOUND ( 'NONE', #54456, .T. ) ;
#3211=EDGE_LOOP ( 'NONE', ( #80246, #65990, #20775, #64687 ) ) ;
#3213=FACE_OUTER_BOUND ( 'NONE', #51443, .T. ) ;
#3214=CARTESIAN_POINT ( 'NONE',  ( 9.019285080869083870, -3.136992222400443175, 32.19305428654138979 ) ) ;
#3216=ORIENTED_EDGE ( 'NONE', *, *, #65232, .F. ) ;
#3217=CARTESIAN_POINT ( 'NONE',  ( 2.307692307692187583, -10.90142922262034020, 33.41473453929536674 ) ) ;
#3218=ORIENTED_EDGE ( 'NONE', *, *, #514, .F. ) ;
#3219=EDGE_CURVE ( 'NONE', #20214, #18112, #50351, .T. ) ;
#3220=ORIENTED_EDGE ( 'NONE', *, *, #87400, .T. ) ;
#3221=CARTESIAN_POINT ( 'NONE',  ( 8.769230769230768274, -13.87047571288749737, 32.06866353760679544 ) ) ;
#3222=DIRECTION ( 'NONE',  ( -0.000000000000000000, 1.000000000000000000, 3.491481338843133355E-15 ) ) ;
#3223=CARTESIAN_POINT ( 'NONE',  ( 16.02369894440793630, -6.001485441113818986, 34.52039167877662607 ) ) ;
#3224=CARTESIAN_POINT ( 'NONE',  ( -6.923076923077045919, -4.320704448113951379, 33.92786785259630022 ) ) ;
#3225=EDGE_CURVE ( 'NONE', #25408, #21841, #34246, .T. ) ;
#3226=CARTESIAN_POINT ( 'NONE',  ( -18.06608237936013950, -5.471508081941600210, 34.59228464037088457 ) ) ;
#3227=CARTESIAN_POINT ( 'NONE',  ( -12.46153846153858247, -4.481592998941358097, 33.73612834414048933 ) ) ;
#3228=EDGE_CURVE ( 'NONE', #61593, #37663, #89166, .T. ) ;
#3229=ORIENTED_EDGE ( 'NONE', *, *, #65466, .F. ) ;
#3230=CARTESIAN_POINT ( 'NONE',  ( -5.326899820971668476, -6.524016743844655686, 34.90889640711025521 ) ) ;
#3231=CARTESIAN_POINT ( 'NONE',  ( -11.66860874789975888, -10.19110544564092002, 33.96427741523702792 ) ) ;
#3232=CARTESIAN_POINT ( 'NONE',  ( 11.66929995647430118, -7.277220443632450575, 34.74524770363009196 ) ) ;
#3234=ORIENTED_EDGE ( 'NONE', *, *, #86325, .T. ) ;
#3236=ORIENTED_EDGE ( 'NONE', *, *, #16268, .T. ) ;
#3237=FACE_BOUND ( 'NONE', #74474, .T. ) ;
#3238=VECTOR ( 'NONE', #34391, 1000.000000000000000 ) ;
#3239=ORIENTED_EDGE ( 'NONE', *, *, #89142, .T. ) ;
#3240=CARTESIAN_POINT ( 'NONE',  ( 18.00000000000000000, -12.62096338111211580, 30.90682066428153263 ) ) ;
#3241=CARTESIAN_POINT ( 'NONE',  ( -1.134669975237340367, -2.341251567377310217, 30.72681386836322659 ) ) ;
#3242=EDGE_LOOP ( 'NONE', ( #68213, #74958 ) ) ;
#3243=DIRECTION ( 'NONE',  ( -0.000000000000000000, 0.5000000000000011102, -0.8660254037844381525 ) ) ;
#3244=CARTESIAN_POINT ( 'NONE',  ( -2.057637996053991447, -4.235687564193446164, 33.53795663066793509 ) ) ;
#3245=CARTESIAN_POINT ( 'NONE',  ( -8.638705067467205012, -6.852161475712352789, 34.70806712695775786 ) ) ;
#3246=DIRECTION ( 'NONE',  ( 0.000000000000000000, 0.4999999999999960032, -0.8660254037844410391 ) ) ;
#3247=ORIENTED_EDGE ( 'NONE', *, *, #45459, .T. ) ;
#3248=DIRECTION ( 'NONE',  ( -0.000000000000000000, 0.6427876096865404731, -0.7660444431189770143 ) ) ;
#3249=ORIENTED_EDGE ( 'NONE', *, *, #67110, .T. ) ;
#3250=CARTESIAN_POINT ( 'NONE',  ( 10.61538461538461675, -4.661471528628507777, 34.16647553114623292 ) ) ;
#3252=CARTESIAN_POINT ( 'NONE',  ( -7.715628144390283438, -9.417988943895561960, 34.36773134775777550 ) ) ;
#3253=CARTESIAN_POINT ( 'NONE',  ( -12.71156168575991785, -2.985938066672154445, 32.43141759479405550 ) ) ;
#3254=DIRECTION ( 'NONE',  ( -0.000000000000000000, 0.7660444431189791237, -0.6427876096865379196 ) ) ;
#3255=CARTESIAN_POINT ( 'NONE',  ( 5.750000000000002665, -7.500000000000001776, 35.00000000000000000 ) ) ;
#3256=CARTESIAN_POINT ( 'NONE',  ( 17.07692307692307665, -2.900454961884010974, 35.62045528018868623 ) ) ;
#3257=CARTESIAN_POINT ( 'NONE',  ( 5.142178648199100977, -12.46129190930001052, 30.37095296980870174 ) ) ;
#3260=CARTESIAN_POINT ( 'NONE',  ( 13.63456079399343146, -12.68172785388650681, 30.59649109432439218 ) ) ;
#3261=CARTESIAN_POINT ( 'NONE',  ( 6.065193981783355781, -2.506253911140448487, 29.99999999999988631 ) ) ;
#3263=EDGE_LOOP ( 'NONE', ( #12497, #81130 ) ) ;
#3264=CARTESIAN_POINT ( 'NONE',  ( 9.942253101685738059, -3.520799739797214389, 33.17531984108286025 ) ) ;
#3265=CARTESIAN_POINT ( 'NONE',  ( -14.05774689831426727, -2.589246495874658383, 31.60778113518102828 ) ) ;
#3266=B_SPLINE_CURVE_WITH_KNOTS ( 'NONE', 3,
 ( #51594, #79095, #20501, #81331, #34012, #74566, #61043, #41225, #46645, #33583 ),
 .UNSPECIFIED., .F., .F.,
 ( 4, 2, 2, 2, 4 ),
 ( 0.0007817359430256388964, 0.0009771253907250075990, 0.001172514838424376085, 0.001367904286123744571, 0.001563293733823113273 ),
 .UNSPECIFIED. ) ;
#3267=CARTESIAN_POINT ( 'NONE',  ( -5.076923076923199218, -12.70778746994576025, 30.41441678777401236 ) ) ;
#3268=DIRECTION ( 'NONE',  ( -1.000000000000000000, 0.000000000000000000, 0.000000000000000000 ) ) ;
#3269=CARTESIAN_POINT ( 'NONE',  ( 13.16168842570853492, -2.889293201056495786, 32.26117774369186009 ) ) ;
#3270=AXIS2_PLACEMENT_3D ( 'NONE', #14250, #42179, #1629 ) ;
#3271=CARTESIAN_POINT ( 'NONE',  ( 16.28437159207980045, -3.625058011473227815, 33.29252011169590020 ) ) ;
#3272=VECTOR ( 'NONE', #61182, 1000.000000000000227 ) ;
#3273=CARTESIAN_POINT ( 'NONE',  ( -6.923076923077044142, -11.94971097300221174, 32.03036669348237098 ) ) ;
#3274=EDGE_LOOP ( 'NONE', ( #55570, #68131 ) ) ;
#3276=CARTESIAN_POINT ( 'NONE',  ( -17.32689980786543060, -12.17611988154120795, 31.52148481390971213 ) ) ;
#3277=CARTESIAN_POINT ( 'NONE',  ( 13.38461538461538680, -12.37446782046654192, 30.86335684631486131 ) ) ;
#3278=CARTESIAN_POINT ( 'NONE',  ( 2.242421861731532573, -3.835265460703609186, 33.15142922261924241 ) ) ;
#3279=EDGE_LOOP ( 'NONE', ( #82038, #71886 ) ) ;
#3280=CARTESIAN_POINT ( 'NONE',  ( -17.32692307692307665, -2.249999999999998668, 29.75000000000000355 ) ) ;
#3281=VERTEX_POINT ( 'NONE', #42299 ) ;
#3282=CARTESIAN_POINT ( 'NONE',  ( 8.834485908743600291, -3.083524468853784839, 32.58852847137153930 ) ) ;
#3283=CARTESIAN_POINT ( 'NONE',  ( -1.514762594053604916, -9.418419913701741919, 34.36755862841477693 ) ) ;
#3284=CARTESIAN_POINT ( 'NONE',  ( -2.057692307692242650, -7.434744429011176159, 34.75000000000000711 ) ) ;
#3285=ORIENTED_EDGE ( 'NONE', *, *, #46933, .T. ) ;
#3286=CARTESIAN_POINT ( 'NONE',  ( 7.846153846153846700, -5.415277668671390821, 36.20867863119892149 ) ) ;
#3287=CARTESIAN_POINT ( 'NONE',  ( 10.55011416942384272, -3.835265460703609186, 33.15142922261924241 ) ) ;
#3288=CARTESIAN_POINT ( 'NONE',  ( -17.30040802064702987, -3.754499324213721234, 33.06261337010820256 ) ) ;
#3290=CARTESIAN_POINT ( 'NONE',  ( 8.899278375486456838, -7.723484964179501588, 34.74522123443823318 ) ) ;
#3291=CARTESIAN_POINT ( 'NONE',  ( -4.854143407945009869, -8.540255544307065350, 34.89611431652622286 ) ) ;
#3293=CARTESIAN_POINT ( 'NONE',  ( 7.846153846153723244, -11.67786785259630911, 32.92929555188603530 ) ) ;
#3295=B_SPLINE_CURVE_WITH_KNOTS ( 'NONE', 3,
 ( #45530, #4089, #26154, #72110, #72556, #60376, #37890, #53623, #32461, #87887 ),
 .UNSPECIFIED., .F., .F.,
 ( 4, 2, 2, 2, 4 ),
 ( 0.0007817246256747481482, 0.0009771112852218911526, 0.001172497944769034265, 0.001367884604316177161, 0.001563271263863320274 ),
 .UNSPECIFIED. ) ;
#3298=VECTOR ( 'NONE', #9210, 1000.000000000000000 ) ;
#3299=CARTESIAN_POINT ( 'NONE',  ( -3.230769230769229949, -12.10708131394839349, 31.69288490824020244 ) ) ;
#3300=B_SPLINE_CURVE_WITH_KNOTS ( 'NONE', 3,
 ( #24187, #29633, #16546, #64722, #31397, #44013, #85020, #77367, #84586, #3470 ),
 .UNSPECIFIED., .F., .F.,
 ( 4, 2, 2, 2, 4 ),
 ( 0.000000000000000000, 0.0001954311564186860884, 0.0003908623128373721767, 0.0005862934692560582651, 0.0007817246256747443535 ),
 .UNSPECIFIED. ) ;
#3301=CARTESIAN_POINT ( 'NONE',  ( 9.942362112221147186, -2.544122305571458575, 31.48381861865057729 ) ) ;
#3304=CARTESIAN_POINT ( 'NONE',  ( 12.71159277317677549, -9.943054286541403997, 34.11300777759954883 ) ) ;
#3305=B_SPLINE_CURVE_WITH_KNOTS ( 'NONE', 3,
 ( #60210, #52117, #53450, #73291, #58879, #87716, #26440, #72387, #12479, #80953 ),
 .UNSPECIFIED., .F., .F.,
 ( 4, 2, 2, 2, 4 ),
 ( 0.0007817246256747455461, 0.0009771112852218885505, 0.001172497944769031663, 0.001367884604316174559, 0.001563271263863317672 ),
 .UNSPECIFIED. ) ;
#3306=AXIS2_PLACEMENT_3D ( 'NONE', #72090, #58565, #59017 ) ;
#3307=ORIENTED_EDGE ( 'NONE', *, *, #7182, .T. ) ;
#3308=VERTEX_POINT ( 'NONE', #84178 ) ;
#3309=VERTEX_POINT ( 'NONE', #82399 ) ;
#3311=EDGE_CURVE ( 'NONE', #27279, #61816, #47711, .T. ) ;
#3312=CARTESIAN_POINT ( 'NONE',  ( 12.52760681254089903, -11.69971097300155272, 32.46337939537588113 ) ) ;
#3313=CYLINDRICAL_SURFACE ( 'NONE', #79056, 0.2499999999999998890 ) ;
#3314=CARTESIAN_POINT ( 'NONE',  ( -3.931066484868086075, -6.717445702608402236, 34.94155399931962336 ) ) ;
#3315=CARTESIAN_POINT ( 'NONE',  ( -12.46153846153846168, -12.34228464037088635, 31.77849191805839268 ) ) ;
#3316=B_SPLINE_CURVE_WITH_KNOTS ( 'NONE', 3,
 ( #20890, #40296, #41174, #5613, #19129, #47029, #82621, #46600, #53348, #27651 ),
 .UNSPECIFIED., .F., .F.,
 ( 4, 2, 2, 2, 4 ),
 ( 0.000000000000000000, 0.0001954311564186871184, 0.0003908623128373742367, 0.0005862934692560614093, 0.0007817246256747484735 ),
 .UNSPECIFIED. ) ;
#3317=CARTESIAN_POINT ( 'NONE',  ( -13.25382357679059986, -5.582136614379148654, 34.36778462344220486 ) ) ;
#3318=CARTESIAN_POINT ( 'NONE',  ( 8.639083559792549494, -9.418419913701741919, 34.36755862841477693 ) ) ;
#3319=CARTESIAN_POINT ( 'NONE',  ( 5.750023269057646935, -11.79746400365624659, 32.30657167506340954 ) ) ;
#3320=CARTESIAN_POINT ( 'NONE',  ( -7.780898274877821486, -3.300289026998474817, 32.46337939537591666 ) ) ;
#3321=EDGE_LOOP ( 'NONE', ( #51330, #45872, #49558, #18736 ) ) ;
#3322=VERTEX_POINT ( 'NONE', #13485 ) ;
#3323=ORIENTED_EDGE ( 'NONE', *, *, #83178, .F. ) ;
#3324=DIRECTION ( 'NONE',  ( 0.000000000000000000, 0.3420201433256641055, -0.9396926207859100932 ) ) ;
#3325=VERTEX_POINT ( 'NONE', #40962 ) ;
#3326=AXIS2_PLACEMENT_3D ( 'NONE', #84353, #69491, #7797 ) ;
#3327=CARTESIAN_POINT ( 'NONE',  ( 16.37662569511456567, -11.89424750095246175, 32.13594075562311758 ) ) ;
#3328=CARTESIAN_POINT ( 'NONE',  ( 10.39245839786846659, -9.086856451489515152, 34.49173150075333183 ) ) ;
#3329=CARTESIAN_POINT ( 'NONE',  ( 8.519230769230768274, -7.500000000000001776, 34.75000000000000000 ) ) ;
#3330=ADVANCED_FACE ( 'NONE', ( #3056 ), #23767, .F. ) ;
#3331=DIRECTION ( 'NONE',  ( -0.000000000000000000, 0.7660444431189791237, -0.6427876096865379196 ) ) ;
#3333=VERTEX_POINT ( 'NONE', #8948 ) ;
#3334=B_SPLINE_CURVE_WITH_KNOTS ( 'NONE', 3,
 ( #21528, #29625, #57526, #8909, #62939, #7580, #76922, #36380, #815, #43567 ),
 .UNSPECIFIED., .F., .F.,
 ( 4, 2, 2, 2, 4 ),
 ( 0.0007817359430256322827, 0.0009771253907249989254, 0.001172514838424365676, 0.001367904286123732428, 0.001563293733823098962 ),
 .UNSPECIFIED. ) ;
#3335=VERTEX_POINT ( 'NONE', #36848 ) ;
#3336=CARTESIAN_POINT ( 'NONE',  ( -6.923076923077045919, -6.835583212225970762, 34.95778746994575670 ) ) ;
#3337=B_SPLINE_CURVE_WITH_KNOTS ( 'NONE', 3,
 ( #83491, #74961, #74506, #14574, #75393, #48352, #42059, #41607, #27643, #12802 ),
 .UNSPECIFIED., .F., .F.,
 ( 4, 2, 2, 2, 4 ),
 ( 0.0007817246256747474977, 0.0009771112852218911526, 0.001172497944769034699, 0.001367884604316178462, 0.001563271263863322009 ),
 .UNSPECIFIED. ) ;
#3338=EDGE_LOOP ( 'NONE', ( #76233, #47912 ) ) ;
#3339=FACE_BOUND ( 'NONE', #711, .T. ) ;
#3341=CARTESIAN_POINT ( 'NONE',  ( -14.30769230769230660, -6.343179335718451384, 34.87096338111211935 ) ) ;
#3342=ORIENTED_EDGE ( 'NONE', *, *, #24027, .F. ) ;
#3343=CARTESIAN_POINT ( 'NONE',  ( 17.77707378248385339, -2.758268499246657068, 31.33685645148948851 ) ) ;
#3344=CARTESIAN_POINT ( 'NONE',  ( 9.692307692307695177, -2.900454961884010974, 35.62045528018868623 ) ) ;
#3345=CARTESIAN_POINT ( 'NONE',  ( 2.242422307135989001, -11.67786785259541027, 32.92929555188721480 ) ) ;
#3346=ORIENTED_EDGE ( 'NONE', *, *, #27533, .F. ) ;
#3347=CARTESIAN_POINT ( 'NONE',  ( -11.76194646302587010, -4.988325925672468131, 34.36044203135681130 ) ) ;
#3348=CARTESIAN_POINT ( 'NONE',  ( -18.24997673094235751, -4.943428324936578910, 34.04746400365624481 ) ) ;
#3349=VERTEX_POINT ( 'NONE', #31430 ) ;
#3350=CARTESIAN_POINT ( 'NONE',  ( 6.250000000001421085, -7.500000000000154543, 35.00000000000007105 ) ) ;
#3351=CARTESIAN_POINT ( 'NONE',  ( -9.692307692307814193, -2.379036618888197729, 30.90682066428292885 ) ) ;
#3352=ORIENTED_EDGE ( 'NONE', *, *, #71775, .T. ) ;
#3353=CARTESIAN_POINT ( 'NONE',  ( 8.519207545009310323, -11.56360843649121861, 33.07473185843129926 ) ) ;
#3354=CARTESIAN_POINT ( 'NONE',  ( 13.31853197365950514, -2.538708090699994813, 30.37095296980875148 ) ) ;
#3355=CARTESIAN_POINT ( 'NONE',  ( -8.769230769230890843, -12.46129190930018460, 30.37095296980731973 ) ) ;
#3357=CARTESIAN_POINT ( 'NONE',  ( 9.442330948259103351, -12.41104346484419452, 31.60698883733904196 ) ) ;
#3358=FACE_BOUND ( 'NONE', #81878, .T. ) ;
#3360=CARTESIAN_POINT ( 'NONE',  ( 7.173131234715237170, -3.136992222400443175, 32.19305428654138979 ) ) ;
#3361=DIRECTION ( 'NONE',  ( -0.000000000000000000, -0.7660444431189791237, -0.6427876096865379196 ) ) ;
#3362=CARTESIAN_POINT ( 'NONE',  ( 3.007902967706132191, -2.251424796025575770, 29.88072029997477586 ) ) ;
#3363=CARTESIAN_POINT ( 'NONE',  ( 12.21156171748986985, -4.818429247618089661, 34.26397095200675125 ) ) ;
#3364=CARTESIAN_POINT ( 'NONE',  ( -5.999999999999998224, -12.37446782046654192, 30.86335684631486131 ) ) ;
#3366=VERTEX_POINT ( 'NONE', #22890 ) ;
#3367=CARTESIAN_POINT ( 'NONE',  ( -15.23076923076922995, -12.34228464037088635, 31.77849191805839268 ) ) ;
#3368=VERTEX_POINT ( 'NONE', #78728 ) ;
#3369=AXIS2_PLACEMENT_3D ( 'NONE', #86885, #65241, #17512 ) ;
#3370=CARTESIAN_POINT ( 'NONE',  ( 11.53846153846153832, -11.11383981884818262, 36.00935417666054406 ) ) ;
#3371=ORIENTED_EDGE ( 'NONE', *, *, #83505, .T. ) ;
#3373=ORIENTED_EDGE ( 'NONE', *, *, #78418, .F. ) ;
#3374=CARTESIAN_POINT ( 'NONE',  ( -6.000000000000119904, -11.94971097300221174, 32.03036669348237098 ) ) ;
#3376=CARTESIAN_POINT ( 'NONE',  ( -17.86920819217521483, -5.582136614379148654, 34.36778462344220486 ) ) ;
#3377=CARTESIAN_POINT ( 'NONE',  ( -5.750054590621957118, -11.56426240980093745, 33.07394671870546432 ) ) ;
#3378=CARTESIAN_POINT ( 'NONE',  ( 13.38461538461526423, -3.083524468854526912, 32.58852847137268327 ) ) ;
#3379=B_SPLINE_CURVE_WITH_KNOTS ( 'NONE', 3,
 ( #3999, #60732, #86906, #11672, #31487, #19309, #25619, #52191, #46781, #88240 ),
 .UNSPECIFIED., .F., .F.,
 ( 4, 2, 2, 2, 4 ),
 ( 0.0007817359527651104954, 0.0009771254036996493593, 0.001172514854634188440, 0.001367904305568727304, 0.001563293756503266168 ),
 .UNSPECIFIED. ) ;
#3380=CARTESIAN_POINT ( 'NONE',  ( -6.066082379360134169, -2.486705287966279432, 31.30864560766542937 ) ) ;
#3381=CARTESIAN_POINT ( 'NONE',  ( 15.10007862765892739, -8.191372820521381826, 34.95448215188423546 ) ) ;
#3382=CARTESIAN_POINT ( 'NONE',  ( -7.623374304885436104, -2.847695495035523994, 31.58253572463339509 ) ) ;
#3383=CARTESIAN_POINT ( 'NONE',  ( 14.98076923076923173, -7.500000000000001776, 35.00000000000000000 ) ) ;
#3384=B_SPLINE_CURVE_WITH_KNOTS ( 'NONE', 3,
 ( #19609, #61917, #88981, #54270, #13739, #67803, #60591, #82207, #20496, #33579 ),
 .UNSPECIFIED., .F., .F.,
 ( 4, 2, 2, 2, 4 ),
 ( 0.000000000000000000, 0.0001954311564186860071, 0.0003908623128373720141, 0.0005862934692560580483, 0.0007817246256747440282 ),
 .UNSPECIFIED. ) ;
#3386=CARTESIAN_POINT ( 'NONE',  ( 1.384615384615265343, -3.300289026999228881, 32.46337939537708905 ) ) ;
#3388=CYLINDRICAL_SURFACE ( 'NONE', #33506, 0.2500000000000009437 ) ;
#3390=VERTEX_POINT ( 'NONE', #43606 ) ;
#3391=CARTESIAN_POINT ( 'NONE',  ( -13.60810030917971858, -6.716662450894489211, 34.94144148231605840 ) ) ;
#3392=CARTESIAN_POINT ( 'NONE',  ( 17.07692307692307665, -1.242168528481310874, 33.36296068462461051 ) ) ;
#3393=LINE ( 'NONE', #38526, #85756 ) ;
#3394=CARTESIAN_POINT ( 'NONE',  ( 18.06606835100243558, -10.51840700105979565, 33.73612834413962247 ) ) ;
#3395=CARTESIAN_POINT ( 'NONE',  ( 17.20771351789002424, -12.35292014791297710, 31.75344720912887198 ) ) ;
#3396=ADVANCED_FACE ( 'NONE', ( #64310 ), #10716, .F. ) ;
#3397=CARTESIAN_POINT ( 'NONE',  ( -3.230769230769229949, -11.35647404775217417, 33.31231777344666511 ) ) ;
#3400=CARTESIAN_POINT ( 'NONE',  ( 7.846153846153723244, -3.083524468854526912, 32.58852847137268327 ) ) ;
#3401=VERTEX_POINT ( 'NONE', #57124 ) ;
#3402=ORIENTED_EDGE ( 'NONE', *, *, #51805, .F. ) ;
#3403=CARTESIAN_POINT ( 'NONE',  ( 10.61538461538461675, -1.044019251281081972, 31.83374038241031911 ) ) ;
#3404=EDGE_CURVE ( 'NONE', #23906, #22078, #46057, .T. ) ;
#3405=CARTESIAN_POINT ( 'NONE',  ( 3.361294932532794100, -6.001044277235011215, 34.52024696741798948 ) ) ;
#3406=CARTESIAN_POINT ( 'NONE',  ( -0.2385753272717870410, -7.369474539155827841, 34.99858011523955525 ) ) ;
#3407=EDGE_CURVE ( 'NONE', #87412, #1287, #86928, .T. ) ;
#3408=CARTESIAN_POINT ( 'NONE',  ( -13.38461538461538325, -8.973038597847269315, 34.52809138561121927 ) ) ;
#3409=CARTESIAN_POINT ( 'NONE',  ( -5.076923076923075762, -8.164416787775445883, 34.95778746994557906 ) ) ;
#3410=VERTEX_POINT ( 'NONE', #2610 ) ;
#3411=EDGE_LOOP ( 'NONE', ( #7730, #87088 ) ) ;
#3412=AXIS2_PLACEMENT_3D ( 'NONE', #23863, #24768, #31979 ) ;
#3415=EDGE_CURVE ( 'NONE', #14630, #80116, #66472, .T. ) ;
#3416=CARTESIAN_POINT ( 'NONE',  ( 1.319344938654611887, -11.48612834413959582, 32.76840700105983473 ) ) ;
#3417=CARTESIAN_POINT ( 'NONE',  ( 16.28463796167094557, -12.38066358083363738, 30.83685684665853444 ) ) ;
#3418=DIRECTION ( 'NONE',  ( -0.000000000000000000, -0.8660254037844397068, -0.4999999999999980016 ) ) ;
#3421=CARTESIAN_POINT ( 'NONE',  ( -15.23076923076935074, -3.300289026999228881, 32.46337939537708905 ) ) ;
#3422=CARTESIAN_POINT ( 'NONE',  ( -4.153846153846152411, -8.120952969808772792, 34.71129190930000163 ) ) ;
#3423=CARTESIAN_POINT ( 'NONE',  ( 17.86985279056177944, -8.587444163452046197, 34.63053765926554206 ) ) ;
#3424=ORIENTED_EDGE ( 'NONE', *, *, #26826, .T. ) ;
#3425=ORIENTED_EDGE ( 'NONE', *, *, #17387, .F. ) ;
#3426=B_SPLINE_CURVE_WITH_KNOTS ( 'NONE', 3,
 ( #16830, #72211, #84865, #3757, #36668, #59146, #65896, #85302, #24469, #44279 ),
 .UNSPECIFIED., .F., .F.,
 ( 4, 2, 2, 2, 4 ),
 ( 0.0007817359430256324996, 0.0009771253907249991422, 0.001172514838424365676, 0.001367904286123732428, 0.001563293733823098962 ),
 .UNSPECIFIED. ) ;
#3428=ORIENTED_EDGE ( 'NONE', *, *, #51871, .F. ) ;
#3429=CARTESIAN_POINT ( 'NONE',  ( -5.869208192175213945, -3.062576670634119758, 32.05464942895959979 ) ) ;
#3430=ORIENTED_EDGE ( 'NONE', *, *, #69548, .T. ) ;
#3431=CARTESIAN_POINT ( 'NONE',  ( -10.39260494640654464, -4.226511098958373402, 33.85474049983370293 ) ) ;
#3432=CARTESIAN_POINT ( 'NONE',  ( 6.250054311638314708, -12.41262288849542017, 30.68299917996395010 ) ) ;
#3434=ADVANCED_FACE ( 'NONE', ( #50788 ), #10275, .F. ) ;
#3435=ORIENTED_EDGE ( 'NONE', *, *, #19569, .F. ) ;
#3436=EDGE_CURVE ( 'NONE', #53046, #51788, #42874, .T. ) ;
#3437=CARTESIAN_POINT ( 'NONE',  ( -14.30769230769230660, -12.34228464037088635, 31.77849191805839268 ) ) ;
#3439=CARTESIAN_POINT ( 'NONE',  ( -8.992715693795101828, -4.988325925672468131, 34.36044203135681130 ) ) ;
#3440=CARTESIAN_POINT ( 'NONE',  ( 17.07692307692307665, -13.88283147151868846, 33.14645433367849847 ) ) ;
#3441=CARTESIAN_POINT ( 'NONE',  ( 2.177001704582003150, -12.35290016733513951, 31.75349464988449455 ) ) ;
#3442=CARTESIAN_POINT ( 'NONE',  ( 5.750023255951411727, -12.41104346484419452, 31.60698883733904196 ) ) ;
#3443=LINE ( 'NONE', #37677, #56986 ) ;
#3444=EDGE_CURVE ( 'NONE', #50148, #24402, #75102, .T. ) ;
#3445=CARTESIAN_POINT ( 'NONE',  ( 8.519254038288416098, -5.728515186090277211, 34.42611988154120439 ) ) ;
#3446=LINE ( 'NONE', #58380, #53455 ) ;
#3447=EDGE_LOOP ( 'NONE', ( #37992, #2627, #21349, #15975 ) ) ;
#3449=CYLINDRICAL_SURFACE ( 'NONE', #56164, 0.2499999999999998890 ) ;
#3450=DIRECTION ( 'NONE',  ( -0.000000000000000000, 1.000000000000000000, -0.000000000000000000 ) ) ;
#3451=ORIENTED_EDGE ( 'NONE', *, *, #5763, .F. ) ;
#3452=DIRECTION ( 'NONE',  ( 0.000000000000000000, 0.4999999999999960032, -0.8660254037844410391 ) ) ;
#3453=CARTESIAN_POINT ( 'NONE',  ( -4.826977558574935045, -5.852078868378311149, 34.47109172314383585 ) ) ;
#3454=CARTESIAN_POINT ( 'NONE',  ( 10.48469401227430886, -8.191372820521381826, 34.95448215188423546 ) ) ;
#3455=FACE_OUTER_BOUND ( 'NONE', #34753, .T. ) ;
#3457=FACE_BOUND ( 'NONE', #21369, .T. ) ;
#3458=CARTESIAN_POINT ( 'NONE',  ( 12.39545608217832395, -9.905515769479276145, 34.41647553114623292 ) ) ;
#3459=CARTESIAN_POINT ( 'NONE',  ( 1.607626736228235487, -2.554770724473667709, 30.48948780036025852 ) ) ;
#3460=CYLINDRICAL_SURFACE ( 'NONE', #20960, 0.2499999999999993616 ) ;
#3461=CARTESIAN_POINT ( 'NONE',  ( 3.007284287045282500, -4.386631170607603991, 33.66268669641500111 ) ) ;
#3462=CARTESIAN_POINT ( 'NONE',  ( 9.915319043920545639, -4.187068189119697692, 33.49521262558774026 ) ) ;
#3463=CYLINDRICAL_SURFACE ( 'NONE', #48393, 0.2500000000000004996 ) ;
#3464=CARTESIAN_POINT ( 'NONE',  ( 17.07692307692307665, -1.509761064869970415, 31.06009739812519044 ) ) ;
#3467=CARTESIAN_POINT ( 'NONE',  ( -9.692307692307814193, -3.083524468854526912, 32.58852847137268327 ) ) ;
#3468=B_SPLINE_CURVE_WITH_KNOTS ( 'NONE', 3,
 ( #40600, #25300, #6797, #27073, #81146, #13120, #87468, #33827, #61285, #39718 ),
 .UNSPECIFIED., .F., .F.,
 ( 4, 2, 2, 2, 4 ),
 ( 0.000000000000000000, 0.0001954339857564073659, 0.0003908679715128147319, 0.0005863019572692221250, 0.0007817359430256294638 ),
 .UNSPECIFIED. ) ;
#3469=CARTESIAN_POINT ( 'NONE',  ( -14.43838377435986864, -6.413092428213692742, 34.63065189839063152 ) ) ;
#3470=CARTESIAN_POINT ( 'NONE',  ( -0.4615384615385840772, -3.643525952248795718, 33.31231777344771672 ) ) ;
#3471=CARTESIAN_POINT ( 'NONE',  ( 2.557692307692308376, -2.249999999999998668, 29.75000000000000355 ) ) ;
#3472=CARTESIAN_POINT ( 'NONE',  ( 6.792928953345226617, -12.70455904226513866, 30.44083106164009322 ) ) ;
#3473=DIRECTION ( 'NONE',  ( -0.000000000000000000, 0.5000000000000011102, -0.8660254037844381525 ) ) ;
#3475=CARTESIAN_POINT ( 'NONE',  ( -1.134615384613964384, -7.500000000000154543, 35.00000000000007105 ) ) ;
#3476=CARTESIAN_POINT ( 'NONE',  ( 0.4615384615384611200, -3.513871655860378418, 32.76840700105978499 ) ) ;
#3477=CARTESIAN_POINT ( 'NONE',  ( 11.28846153846154188, -7.566082377512564960, 35.00000000000000711 ) ) ;
#3478=DIRECTION ( 'NONE',  ( 0.000000000000000000, -6.938893903907222067E-15, 1.000000000000000000 ) ) ;
#3479=CARTESIAN_POINT ( 'NONE',  ( 0.3962680155776860391, -11.48612834413959582, 32.76840700105983473 ) ) ;
#3480=CARTESIAN_POINT ( 'NONE',  ( 15.23076923076923173, -11.11383981884818262, 36.00935417666054406 ) ) ;
#3481=EDGE_CURVE ( 'NONE', #46107, #77857, #82617, .T. ) ;
#3482=FACE_OUTER_BOUND ( 'NONE', #38746, .T. ) ;
#3483=CARTESIAN_POINT ( 'NONE',  ( 17.07692307692295586, -2.657715359629662544, 31.77849191805970364 ) ) ;
#3484=ORIENTED_EDGE ( 'NONE', *, *, #73546, .F. ) ;
#3485=CARTESIAN_POINT ( 'NONE',  ( 3.230769230769108269, -12.51329471203414379, 31.30864560766407578 ) ) ;
#3486=CARTESIAN_POINT ( 'NONE',  ( 3.230769230769231726, -13.87047571288749737, 32.06866353760679544 ) ) ;
#3490=CARTESIAN_POINT ( 'NONE',  ( 2.084766090176161324, -4.186968288167446595, 33.49512374952580274 ) ) ;
#3491=CARTESIAN_POINT ( 'NONE',  ( -16.82686865700962642, -5.642605341092955307, 34.66089969410670335 ) ) ;
#3493=CARTESIAN_POINT ( 'NONE',  ( -18.13014720943822056, -9.418419913701741919, 34.36755862841476272 ) ) ;
#3494=CARTESIAN_POINT ( 'NONE',  ( 2.307692307692309264, -10.67929555188718282, 33.92786785259544047 ) ) ;
#3495=DIRECTION ( 'NONE',  ( 0.000000000000000000, 0.000000000000000000, -1.000000000000000000 ) ) ;
#3496=EDGE_LOOP ( 'NONE', ( #69343, #672 ) ) ;
#3498=CARTESIAN_POINT ( 'NONE',  ( -17.07692307692307665, -2.486705287966279876, 31.30864560766543647 ) ) ;
#3499=DIRECTION ( 'NONE',  ( -0.000000000000000000, 0.7660444431189791237, -0.6427876096865379196 ) ) ;
#3500=EDGE_CURVE ( 'NONE', #62030, #70013, #60673, .T. ) ;
#3501=CARTESIAN_POINT ( 'NONE',  ( -14.08491276642389955, -11.41317474335729543, 32.86274602512330034 ) ) ;
#3502=ORIENTED_EDGE ( 'NONE', *, *, #75844, .T. ) ;
#3503=CARTESIAN_POINT ( 'NONE',  ( 3.230769230769231726, -2.486705287966279876, 31.30864560766543647 ) ) ;
#3505=B_SPLINE_CURVE_WITH_KNOTS ( 'NONE', 3,
 ( #72936, #4481, #11238, #31958, #59422, #78797, #64386, #3578, #79253, #86929 ),
 .UNSPECIFIED., .F., .F.,
 ( 4, 2, 2, 2, 4 ),
 ( 0.0007817359527651096280, 0.0009771254036996484919, 0.001172514854634187573, 0.001367904305568726653, 0.001563293756503265517 ),
 .UNSPECIFIED. ) ;
#3506=CARTESIAN_POINT ( 'NONE',  ( 15.10062126103753499, -10.31621877034669588, 34.18098118002070152 ) ) ;
#3507=ORIENTED_EDGE ( 'NONE', *, *, #68893, .T. ) ;
#3508=ORIENTED_EDGE ( 'NONE', *, *, #3043, .T. ) ;
#3509=B_SPLINE_CURVE_WITH_KNOTS ( 'NONE', 3,
 ( #87434, #11761, #67149, #59936, #53173, #36027 ),
 .UNSPECIFIED., .F., .F.,
 ( 4, 2, 4 ),
 ( 0.000000000000000000, 0.0001954784845028934947, 0.0003909569690057869895 ),
 .UNSPECIFIED. ) ;
#3510=ORIENTED_EDGE ( 'NONE', *, *, #50763, .T. ) ;
#3511=ADVANCED_FACE ( 'NONE', ( #87732 ), #12495, .F. ) ;
#3512=DIRECTION ( 'NONE',  ( 0.000000000000000000, 0.9848077530122072432, -0.1736481776669354937 ) ) ;
#3513=CARTESIAN_POINT ( 'NONE',  ( -7.846153846153844924, -13.75783147151868846, 33.36296068462461051 ) ) ;
#3514=EDGE_CURVE ( 'NONE', #7867, #87048, #88180, .T. ) ;
#3515=CARTESIAN_POINT ( 'NONE',  ( 13.25392391794782654, -11.18331474514187995, 33.13161551792790505 ) ) ;
#3516=CARTESIAN_POINT ( 'NONE',  ( 7.846153846153846700, -8.120952969808772792, 34.71129190930000163 ) ) ;
#3517=VERTEX_POINT ( 'NONE', #47153 ) ;
#3520=CARTESIAN_POINT ( 'NONE',  ( -11.53846153846153655, -2.538708090699994813, 30.37095296980875503 ) ) ;
#3521=ORIENTED_EDGE ( 'NONE', *, *, #76748, .T. ) ;
#3522=LINE ( 'NONE', #64334, #19383 ) ;
#3523=EDGE_CURVE ( 'NONE', #59454, #38026, #68704, .T. ) ;
#3524=CARTESIAN_POINT ( 'NONE',  ( 10.48523740594639442, -11.47017969459903952, 32.78971311882035167 ) ) ;
#3525=FACE_OUTER_BOUND ( 'NONE', #75446, .T. ) ;
#3526=EDGE_CURVE ( 'NONE', #60787, #58112, #6351, .T. ) ;
#3527=EDGE_LOOP ( 'NONE', ( #70212, #78672 ) ) ;
#3528=ORIENTED_EDGE ( 'NONE', *, *, #25050, .F. ) ;
#3530=CARTESIAN_POINT ( 'NONE',  ( 9.019176287578909879, -2.587454068350148351, 30.68340429815432202 ) ) ;
#3531=ORIENTED_EDGE ( 'NONE', *, *, #8095, .F. ) ;
#3532=CARTESIAN_POINT ( 'NONE',  ( -0.5916856709766812328, -10.88202310037936194, 33.43294751532457099 ) ) ;
#3533=B_SPLINE_CURVE_WITH_KNOTS ( 'NONE', 3,
 ( #1379, #56, #20764, #62626, #6803, #83816, #69401, #54995, #40608, #7708 ),
 .UNSPECIFIED., .F., .F.,
 ( 4, 2, 2, 2, 4 ),
 ( 0.000000000000000000, 0.0001954311564186865221, 0.0003908623128373730441, 0.0005862934692560595662, 0.0007817246256747460882 ),
 .UNSPECIFIED. ) ;
#3534=VECTOR ( 'NONE', #27048, 1000.000000000000227 ) ;
#3535=CARTESIAN_POINT ( 'NONE',  ( -10.86536135943320502, -9.234221910056348293, 34.70572697212741531 ) ) ;
#3536=EDGE_CURVE ( 'NONE', #87771, #4656, #47150, .T. ) ;
#3537=ORIENTED_EDGE ( 'NONE', *, *, #16422, .T. ) ;
#3538=CARTESIAN_POINT ( 'NONE',  ( 6.923076923077231548, -2.506253911140614576, 30.00000000000323297 ) ) ;
#3539=CARTESIAN_POINT ( 'NONE',  ( -17.07692307692307665, -4.786620604624113540, 33.94971097300155094 ) ) ;
#3540=CARTESIAN_POINT ( 'NONE',  ( -5.750054590621955342, -3.520799739797213501, 33.17531984108286025 ) ) ;
#3541=FACE_BOUND ( 'NONE', #33905, .T. ) ;
#3542=AXIS2_PLACEMENT_3D ( 'NONE', #21368, #42537, #23139 ) ;
#3543=CARTESIAN_POINT ( 'NONE',  ( 15.16549878480845770, -6.026961402152685388, 34.52809138561120506 ) ) ;
#3544=CARTESIAN_POINT ( 'NONE',  ( 11.28848480751918437, -8.303909089506435137, 34.68538101551103381 ) ) ;
#3545=EDGE_CURVE ( 'NONE', #148, #38452, #20572, .T. ) ;
#3546=VECTOR ( 'NONE', #50538, 1000.000000000000114 ) ;
#3547=DIRECTION ( 'NONE',  ( 0.000000000000000000, 0.9848077530122072432, -0.1736481776669354937 ) ) ;
#3548=CARTESIAN_POINT ( 'NONE',  ( -12.46153846153858247, -4.481592998941358097, 33.73612834414048933 ) ) ;
#3549=CARTESIAN_POINT ( 'NONE',  ( -5.999999999999998224, -10.51840700105979565, 33.73612834413961536 ) ) ;
#3550=CARTESIAN_POINT ( 'NONE',  ( -7.911424292114620727, -3.300289026998414865, 32.46337939537583139 ) ) ;
#3551=CARTESIAN_POINT ( 'NONE',  ( 1.449870524128225036, -2.379036618887895305, 30.90682066428159303 ) ) ;
#3552=ORIENTED_EDGE ( 'NONE', *, *, #82172, .F. ) ;
#3553=EDGE_CURVE ( 'NONE', #81210, #35763, #61114, .T. ) ;
#3554=CARTESIAN_POINT ( 'NONE',  ( 10.39189967166066708, -10.81261337010820256, 33.49550067578627477 ) ) ;
#3555=EDGE_LOOP ( 'NONE', ( #25277, #67546, #29792, #69570 ) ) ;
#3556=EDGE_LOOP ( 'NONE', ( #16356, #50702, #32472, #87338 ) ) ;
#3557=CARTESIAN_POINT ( 'NONE',  ( -6.857821351800899023, -8.613356846314928816, 34.62446782046653482 ) ) ;
#3558=CARTESIAN_POINT ( 'NONE',  ( 1.161689167099240194, -10.61292498521070549, 33.66303323003028680 ) ) ;
#3559=CARTESIAN_POINT ( 'NONE',  ( 11.31497661389720832, -8.539481045369596401, 34.89627647299170832 ) ) ;
#3560=CYLINDRICAL_SURFACE ( 'NONE', #84747, 0.2499999999999998890 ) ;
#3561=CARTESIAN_POINT ( 'NONE',  ( -2.530619266599154038, -11.43668979543635089, 33.22377378376089752 ) ) ;
#3562=ORIENTED_EDGE ( 'NONE', *, *, #35933, .T. ) ;
#3564=CARTESIAN_POINT ( 'NONE',  ( 6.856993512121043466, -3.513871655860377086, 32.76840700105978499 ) ) ;
#3565=CARTESIAN_POINT ( 'NONE',  ( -12.59168567097668401, -5.195881422630166391, 34.18770438780619259 ) ) ;
#3566=CARTESIAN_POINT ( 'NONE',  ( 5.076923076923075762, -2.499999999999998668, 29.75000000000001421 ) ) ;
#3567=CARTESIAN_POINT ( 'NONE',  ( 4.153846153846154188, -13.87047571288749737, 32.06866353760679544 ) ) ;
#3568=ADVANCED_FACE ( 'NONE', ( #56134 ), #48931, .F. ) ;
#3570=ORIENTED_EDGE ( 'NONE', *, *, #76304, .T. ) ;
#3571=ORIENTED_EDGE ( 'NONE', *, *, #23831, .F. ) ;
#3572=CARTESIAN_POINT ( 'NONE',  ( -5.076923076923075762, -2.499999999999998668, 29.75000000000001421 ) ) ;
#3573=EDGE_CURVE ( 'NONE', #32448, #64799, #80532, .T. ) ;
#3574=ORIENTED_EDGE ( 'NONE', *, *, #36519, .T. ) ;
#3575=CARTESIAN_POINT ( 'NONE',  ( -0.4615384615385840772, -12.16647553114689728, 32.15551576947799362 ) ) ;
#3576=CARTESIAN_POINT ( 'NONE',  ( -12.39628289026243557, -10.21337939537593620, 33.94971097300152252 ) ) ;
#3578=CARTESIAN_POINT ( 'NONE',  ( 2.084865615213304491, -7.369208160676173236, 34.74850200257122879 ) ) ;
#3580=DIRECTION ( 'NONE',  ( -0.000000000000000000, 0.9396926207859093161, -0.3420201433256663259 ) ) ;
#3581=AXIS2_PLACEMENT_3D ( 'NONE', #55321, #76932, #63404 ) ;
#3582=EDGE_LOOP ( 'NONE', ( #8943, #44814, #13659, #18476 ) ) ;
#3583=CARTESIAN_POINT ( 'NONE',  ( -1.384615384615383471, -1.129524287112498415, 32.06866353760679544 ) ) ;
#3584=CARTESIAN_POINT ( 'NONE',  ( -1.384615384615383471, -8.973038597847269315, 34.52809138561121927 ) ) ;
#3585=EDGE_LOOP ( 'NONE', ( #22965, #230 ) ) ;
#3586=CARTESIAN_POINT ( 'NONE',  ( 8.769230769230768274, -13.75783147151868846, 33.36296068462461051 ) ) ;
#3587=CARTESIAN_POINT ( 'NONE',  ( 18.00000000000000000, -13.04860791097971706, 34.73218667398347037 ) ) ;
#3588=CARTESIAN_POINT ( 'NONE',  ( -12.59222906464877134, -8.191372820521381826, 34.95448215188424967 ) ) ;
#3589=EDGE_CURVE ( 'NONE', #88590, #78118, #24681, .T. ) ;
#3590=CYLINDRICAL_SURFACE ( 'NONE', #6993, 0.2500000000000009437 ) ;
#3591=LINE ( 'NONE', #17566, #8917 ) ;
#3592=DIRECTION ( 'NONE',  ( 0.000000000000000000, 0.9848077530122072432, 0.1736481776669354937 ) ) ;
#3595=ORIENTED_EDGE ( 'NONE', *, *, #77455, .T. ) ;
#3596=CARTESIAN_POINT ( 'NONE',  ( -4.376772371362299907, -4.887634598454295265, 34.01352882383564946 ) ) ;
#3597=ADVANCED_FACE ( 'NONE', ( #41300 ), #13373, .F. ) ;
#3598=CARTESIAN_POINT ( 'NONE',  ( -13.25382494364843389, -9.929761469519743144, 34.40412654351204225 ) ) ;
#3599=LINE ( 'NONE', #72503, #8832 ) ;
#3602=CARTESIAN_POINT ( 'NONE',  ( -3.361460697436788436, -8.999036380462717588, 34.52022231692819076 ) ) ;
#3603=CARTESIAN_POINT ( 'NONE',  ( -17.30040802064702987, -2.599994579823202923, 30.74605699353653776 ) ) ;
#3604=CARTESIAN_POINT ( 'NONE',  ( 8.519207531937805555, -11.37209801155882793, 32.91403422569033665 ) ) ;
#3605=ORIENTED_EDGE ( 'NONE', *, *, #64105, .F. ) ;
#3607=CARTESIAN_POINT ( 'NONE',  ( -1.514762594053607581, -10.19110544564091825, 33.96427741523702792 ) ) ;
#3608=EDGE_LOOP ( 'NONE', ( #22359, #1291, #31792, #24930 ) ) ;
#3609=EDGE_CURVE ( 'NONE', #12402, #39715, #52591, .T. ) ;
#3610=CARTESIAN_POINT ( 'NONE',  ( -4.023055712879203938, -2.494656445102013453, 31.33466734024120015 ) ) ;
#3611=ORIENTED_EDGE ( 'NONE', *, *, #82733, .T. ) ;
#3612=CARTESIAN_POINT ( 'NONE',  ( 14.53070365930516061, -12.15243808032445827, 31.58219941686247978 ) ) ;
#3613=CARTESIAN_POINT ( 'NONE',  ( -7.846153846153844924, -11.69971097300155272, 32.46337939537588113 ) ) ;
#3615=CARTESIAN_POINT ( 'NONE',  ( -1.634638621908348632, -4.335965774309649134, 33.62209801155881905 ) ) ;
#3616=VERTEX_POINT ( 'NONE', #62431 ) ;
#3617=CARTESIAN_POINT ( 'NONE',  ( 0.2380535369741292595, -4.988325925672468131, 34.36044203135681130 ) ) ;
#3618=ORIENTED_EDGE ( 'NONE', *, *, #4431, .F. ) ;
#3619=DIRECTION ( 'NONE',  ( -0.000000000000000000, 0.7660444431189791237, -0.6427876096865379196 ) ) ;
#3620=EDGE_LOOP ( 'NONE', ( #78325, #40008 ) ) ;
#3621=CARTESIAN_POINT ( 'NONE',  ( -6.673076923076920686, -2.499999999999999112, 29.81604066197450109 ) ) ;
#3622=CARTESIAN_POINT ( 'NONE',  ( 12.46153846153833911, -12.27809138561165270, 31.22303859784587132 ) ) ;
#3623=ORIENTED_EDGE ( 'NONE', *, *, #22161, .T. ) ;
#3625=CARTESIAN_POINT ( 'NONE',  ( -5.750054481651856619, -11.37275283266503756, 32.91324779482534524 ) ) ;
#3626=CARTESIAN_POINT ( 'NONE',  ( -12.46153846153846168, -5.557115091759785130, 34.35708131394839171 ) ) ;
#3627=ADVANCED_FACE ( 'NONE', ( #748 ), #14710, .F. ) ;
#3630=CARTESIAN_POINT ( 'NONE',  ( -13.31936024510254590, -12.16647553114626490, 32.15551576947920864 ) ) ;
#3631=ORIENTED_EDGE ( 'NONE', *, *, #64025, .F. ) ;
#3632=ORIENTED_EDGE ( 'NONE', *, *, #85186, .T. ) ;
#3636=CARTESIAN_POINT ( 'NONE',  ( -8.992156986746914882, -9.886141570436013382, 34.14413921362392301 ) ) ;
#3637=CARTESIAN_POINT ( 'NONE',  ( 1.449870955891410906, -2.892918686051626498, 31.69288490824025928 ) ) ;
#3639=ORIENTED_EDGE ( 'NONE', *, *, #30452, .T. ) ;
#3640=EDGE_LOOP ( 'NONE', ( #61494, #14865 ) ) ;
#3641=CARTESIAN_POINT ( 'NONE',  ( -18.00000000000000000, -11.91647553114624358, 32.58852847137147535 ) ) ;
#3642=VERTEX_POINT ( 'NONE', #83173 ) ;
#3643=CARTESIAN_POINT ( 'NONE',  ( 2.557746619330623528, -4.235687564193446164, 33.53795663066793509 ) ) ;
#3644=FACE_OUTER_BOUND ( 'NONE', #80112, .T. ) ;
#3645=CARTESIAN_POINT ( 'NONE',  ( -9.822782877383410494, -7.276987145209185215, 34.99546412871779211 ) ) ;
#3646=FACE_BOUND ( 'NONE', #42577, .T. ) ;
#3648=CARTESIAN_POINT ( 'NONE',  ( 2.177081948067780104, -7.722926236386453702, 34.74524107206102030 ) ) ;
#3649=CARTESIAN_POINT ( 'NONE',  ( 12.52760681254089903, -5.557115091759786019, 34.35708131394839882 ) ) ;
#3650=ADVANCED_FACE ( 'NONE', ( #20136 ), #6621, .F. ) ;
#3651=DIRECTION ( 'NONE',  ( 0.000000000000000000, 0.9848077530122072432, 0.1736481776669354937 ) ) ;
#3652=CARTESIAN_POINT ( 'NONE',  ( 8.992242120843616959, -3.105924265160262543, 32.13625925475356127 ) ) ;
#3653=CARTESIAN_POINT ( 'NONE',  ( 17.20771488474786892, -8.999086150933472084, 34.52020707165672064 ) ) ;
#3654=EDGE_LOOP ( 'NONE', ( #47561, #62986, #5738, #74868 ) ) ;
#3655=EDGE_CURVE ( 'NONE', #32155, #88566, #56903, .T. ) ;
#3656=CARTESIAN_POINT ( 'NONE',  ( -7.053768389744480949, -6.413092428213692742, 34.63065189839063152 ) ) ;
#3657=VERTEX_POINT ( 'NONE', #9712 ) ;
#3659=CARTESIAN_POINT ( 'NONE',  ( 2.307692307692309264, -6.681629849574314051, 35.83090037661290239 ) ) ;
#3660=CARTESIAN_POINT ( 'NONE',  ( -9.626240358957616650, -8.164416787775445883, 34.95778746994558617 ) ) ;
#3661=EDGE_CURVE ( 'NONE', #68446, #72207, #77728, .T. ) ;
#3662=CARTESIAN_POINT ( 'NONE',  ( -10.74553182482283908, -12.27039167877662251, 31.24851455888617835 ) ) ;
#3663=CARTESIAN_POINT ( 'NONE',  ( 12.46153846153846168, -13.75783147151868846, 33.36296068462461051 ) ) ;
#3665=FACE_OUTER_BOUND ( 'NONE', #20317, .T. ) ;
#3666=ORIENTED_EDGE ( 'NONE', *, *, #70394, .T. ) ;
#3667=B_SPLINE_CURVE_WITH_KNOTS ( 'NONE', 3,
 ( #35911, #63366, #1673, #70128, #29595, #29161, #64239, #15197, #28252, #84105 ),
 .UNSPECIFIED., .F., .F.,
 ( 4, 2, 2, 2, 4 ),
 ( 0.0007817359430256287049, 0.0009771253907249945886, 0.001172514838424360255, 0.001367904286123725922, 0.001563293733823091806 ),
 .UNSPECIFIED. ) ;
#3668=VECTOR ( 'NONE', #4082, 1000.000000000000000 ) ;
#3669=CARTESIAN_POINT ( 'NONE',  ( 6.857806922520603976, -2.657715359629089225, 31.77849191805834295 ) ) ;
#3670=CARTESIAN_POINT ( 'NONE',  ( -5.999999999999998224, -2.249999999999998668, 29.75000000000001776 ) ) ;
#3671=CARTESIAN_POINT ( 'NONE',  ( 4.153846153846468603, -2.255955759149395501, 30.00000000000324363 ) ) ;
#3672=CARTESIAN_POINT ( 'NONE',  ( -3.903791842207838148, -3.627508038966689607, 32.91356715214248396 ) ) ;
#3673=VERTEX_POINT ( 'NONE', #50244 ) ;
#3674=EDGE_CURVE ( 'NONE', #63787, #17157, #7458, .T. ) ;
#3675=VERTEX_POINT ( 'NONE', #70536 ) ;
#3676=FACE_BOUND ( 'NONE', #83568, .T. ) ;
#3677=ORIENTED_EDGE ( 'NONE', *, *, #71444, .F. ) ;
#3678=CARTESIAN_POINT ( 'NONE',  ( 11.60371667797437922, -12.51329471203373345, 31.30864560766537963 ) ) ;
#3679=DIRECTION ( 'NONE',  ( -0.000000000000000000, -0.3420201433256694346, -0.9396926207859080948 ) ) ;
#3680=VERTEX_POINT ( 'NONE', #37182 ) ;
#3681=AXIS2_PLACEMENT_3D ( 'NONE', #35574, #49529, #56280 ) ;
#3682=CARTESIAN_POINT ( 'NONE',  ( -16.37677311275299985, -11.43668979543635089, 33.22377378376089752 ) ) ;
#3683=CARTESIAN_POINT ( 'NONE',  ( -10.74553182482283198, -6.852621066184266141, 34.70813303252209181 ) ) ;
#3684=CARTESIAN_POINT ( 'NONE',  ( 16.08857570788537572, -8.613356846314824011, 34.62446782046655613 ) ) ;
#3685=CARTESIAN_POINT ( 'NONE',  ( -6.792285115252136407, -3.062576670634119758, 32.05464942895959979 ) ) ;
#3687=CARTESIAN_POINT ( 'NONE',  ( -3.903791842207838148, -6.567000820036038355, 34.66262288849541306 ) ) ;
#3689=DIRECTION ( 'NONE',  ( 1.000000000000000000, 0.000000000000000000, 0.000000000000000000 ) ) ;
#3690=VERTEX_POINT ( 'NONE', #3397 ) ;
#3691=DIRECTION ( 'NONE',  ( 0.000000000000000000, 0.9396926207859126468, -0.3420201433256571111 ) ) ;
#3693=DIRECTION ( 'NONE',  ( -0.000000000000000000, -0.8660254037844397068, -0.4999999999999978906 ) ) ;
#3694=CARTESIAN_POINT ( 'NONE',  ( 15.29683758177167086, -12.37446782046654192, 30.86335684631486842 ) ) ;
#3695=CARTESIAN_POINT ( 'NONE',  ( -14.37377468705243899, -8.164416787775445883, 34.95778746994557906 ) ) ;
#3696=DIRECTION ( 'NONE',  ( -0.000000000000000000, -0.9848077530122086864, -0.1736481776669273613 ) ) ;
#3699=EDGE_CURVE ( 'NONE', #62418, #41186, #32201, .T. ) ;
#3700=CARTESIAN_POINT ( 'NONE',  ( 4.946232473812769648, -11.93127051446800024, 32.56575433478200665 ) ) ;
#3702=CARTESIAN_POINT ( 'NONE',  ( 7.846153846153846700, -2.249999999999998668, 29.50000000000001421 ) ) ;
#3703=VECTOR ( 'NONE', #30517, 1000.000000000000114 ) ;
#3704=EDGE_LOOP ( 'NONE', ( #35032, #33615, #14508, #211 ) ) ;
#3705=ORIENTED_EDGE ( 'NONE', *, *, #12894, .F. ) ;
#3706=CARTESIAN_POINT ( 'NONE',  ( -1.449866374776626055, -2.506253911140460922, 30.00000000000013856 ) ) ;
#3707=CARTESIAN_POINT ( 'NONE',  ( -7.715628407920200438, -5.915461855592780260, 34.75538340440931506 ) ) ;
#3708=CARTESIAN_POINT ( 'NONE',  ( -0.6850233861027920090, -9.417330523894424488, 34.63758898049880486 ) ) ;
#3709=B_SPLINE_CURVE_WITH_KNOTS ( 'NONE', 3,
 ( #45821, #3051, #4395, #17471, #36845, #44925 ),
 .UNSPECIFIED., .F., .F.,
 ( 4, 2, 4 ),
 ( 0.0003909569690057817311, 0.0005862646681846062470, 0.0007815723673634307088 ),
 .UNSPECIFIED. ) ;
#3710=CARTESIAN_POINT ( 'NONE',  ( 10.48523740594639619, -6.001485441113819874, 34.52039167877662607 ) ) ;
#3711=CARTESIAN_POINT ( 'NONE',  ( 16.08776377448601735, -9.905515769479276145, 34.41647553114623292 ) ) ;
#3713=CARTESIAN_POINT ( 'NONE',  ( -8.834501215191545853, -11.94971097300153140, 32.03036669348370680 ) ) ;
#3714=B_SPLINE_CURVE_WITH_KNOTS ( 'NONE', 3,
 ( #70659, #71090, #1753, #77850, #8965, #71979, #22031, #36864, #85066, #29677 ),
 .UNSPECIFIED., .F., .F.,
 ( 4, 2, 2, 2, 4 ),
 ( 0.0007817246256747494492, 0.0009771112852218935378, 0.001172497944769037518, 0.001367884604316181498, 0.001563271263863325695 ),
 .UNSPECIFIED. ) ;
#3715=DIRECTION ( 'NONE',  ( 0.000000000000000000, 0.6427876096865368094, 0.7660444431189802339 ) ) ;
#3716=EDGE_LOOP ( 'NONE', ( #58715, #36906, #26630, #962 ) ) ;
#3717=B_SPLINE_CURVE_WITH_KNOTS ( 'NONE', 3,
 ( #3763, #59153, #23590, #10531, #51941, #51481, #38902, #66360, #65903, #18626 ),
 .UNSPECIFIED., .F., .F.,
 ( 4, 2, 2, 2, 4 ),
 ( 0.000000000000000000, 0.0001954311564186882568, 0.0003908623128373765136, 0.0005862934692560647703, 0.0007817246256747530271 ),
 .UNSPECIFIED. ) ;
#3718=B_SPLINE_CURVE_WITH_KNOTS ( 'NONE', 3,
 ( #73044, #85672, #17663, #23949, #72593, #10901, #59524, #11340, #59078, #87028 ),
 .UNSPECIFIED., .F., .F.,
 ( 4, 2, 2, 2, 4 ),
 ( 0.000000000000000000, 0.0001954339857564126514, 0.0003908679715128183098, 0.0005863019572692239681, 0.0007817359430256294638 ),
 .UNSPECIFIED. ) ;
#3719=CARTESIAN_POINT ( 'NONE',  ( 6.066068351002440018, -10.51840700105979565, 33.73612834413962247 ) ) ;
#3720=CARTESIAN_POINT ( 'NONE',  ( 16.15384615384615330, -1.466349020453238561, 30.81389545987213907 ) ) ;
#3721=EDGE_CURVE ( 'NONE', #10587, #59888, #23562, .T. ) ;
#3722=CARTESIAN_POINT ( 'NONE',  ( 6.923076923076924238, -6.343179335718451384, 34.87096338111211935 ) ) ;
#3723=CARTESIAN_POINT ( 'NONE',  ( 9.561617089197389063, -2.494641256782728966, 31.33461815524612959 ) ) ;
#3725=CARTESIAN_POINT ( 'NONE',  ( 13.63466969625370062, -6.567000820036036579, 34.66262288849541306 ) ) ;
#3727=CARTESIAN_POINT ( 'NONE',  ( 12.46153846153833911, -9.528491918059723176, 34.59228464037033035 ) ) ;
#3728=CARTESIAN_POINT ( 'NONE',  ( 10.36536139116316058, -3.520140089381495585, 33.17453946501458262 ) ) ;
#3729=FACE_OUTER_BOUND ( 'NONE', #37395, .T. ) ;
#3730=VERTEX_POINT ( 'NONE', #57456 ) ;
#3731=CARTESIAN_POINT ( 'NONE',  ( -1.607542343522232686, -12.64616026154729411, 30.79003144601913533 ) ) ;
#3732=EDGE_CURVE ( 'NONE', #68579, #66377, #30432, .T. ) ;
#3733=DIRECTION ( 'NONE',  ( 0.000000000000000000, 0.1736481776669267785, -0.9848077530122087975 ) ) ;
#3734=CARTESIAN_POINT ( 'NONE',  ( 9.019230769232203571, -7.500000000000155431, 34.75000000000007105 ) ) ;
#3735=CARTESIAN_POINT ( 'NONE',  ( -4.826868657009623753, -10.82426656108011720, 33.81400080652039009 ) ) ;
#3736=EDGE_CURVE ( 'NONE', #88905, #54183, #64385, .T. ) ;
#3737=EDGE_CURVE ( 'NONE', #52906, #5237, #35362, .T. ) ;
#3738=VECTOR ( 'NONE', #79914, 1000.000000000000114 ) ;
#3739=ORIENTED_EDGE ( 'NONE', *, *, #70719, .T. ) ;
#3741=ORIENTED_EDGE ( 'NONE', *, *, #1512, .T. ) ;
#3742=CARTESIAN_POINT ( 'NONE',  ( -2.557715531913765439, -2.588893531581426544, 31.60682220781847818 ) ) ;
#3743=ADVANCED_FACE ( 'NONE', ( #52912 ), #38077, .F. ) ;
#3744=CARTESIAN_POINT ( 'NONE',  ( 4.853438133199126092, -12.24155766932282496, 31.33739205006857986 ) ) ;
#3745=B_SPLINE_CURVE_WITH_KNOTS ( 'NONE', 3,
 ( #75209, #68876, #27459, #6306, #82413, #47276, #34206, #83292, #75630, #35091 ),
 .UNSPECIFIED., .F., .F.,
 ( 4, 2, 2, 2, 4 ),
 ( 0.000000000000000000, 0.0001954311564186866034, 0.0003908623128373732067, 0.0005862934692560597830, 0.0007817246256747464135 ),
 .UNSPECIFIED. ) ;
#3746=CARTESIAN_POINT ( 'NONE',  ( -3.480769230769229061, -7.566083408709834757, 34.74999999999999289 ) ) ;
#3747=CARTESIAN_POINT ( 'NONE',  ( 7.846153846153846700, -13.20930481340135110, 34.54067556320372745 ) ) ;
#3748=B_SPLINE_CURVE_WITH_KNOTS ( 'NONE', 3,
 ( #26844, #81353, #34038, #61502, #20956, #40807, #67385, #27720, #33155, #19638 ),
 .UNSPECIFIED., .F., .F.,
 ( 4, 2, 2, 2, 4 ),
 ( 0.0007817359430256252354, 0.0009771253907249898181, 0.001172514838424354618, 0.001367904286123719200, 0.001563293733823083783 ),
 .UNSPECIFIED. ) ;
#3749=AXIS2_PLACEMENT_3D ( 'NONE', #5078, #73991, #18600 ) ;
#3751=CARTESIAN_POINT ( 'NONE',  ( 14.98074599347626368, -11.86270091957321249, 32.19358267280087915 ) ) ;
#3753=ORIENTED_EDGE ( 'NONE', *, *, #10731, .T. ) ;
#3754=ORIENTED_EDGE ( 'NONE', *, *, #50268, .T. ) ;
#3755=ORIENTED_EDGE ( 'NONE', *, *, #62683, .T. ) ;
#3757=CARTESIAN_POINT ( 'NONE',  ( -1.161835843346973096, -3.236590943229498585, 32.36255958852954251 ) ) ;
#3758=CARTESIAN_POINT ( 'NONE',  ( -1.253823576790598304, -12.38066358083363738, 30.83685684665853444 ) ) ;
#3759=CARTESIAN_POINT ( 'NONE',  ( -6.988327913238165934, -2.506253911140460477, 30.00000000000013856 ) ) ;
#3760=DIRECTION ( 'NONE',  ( 0.000000000000000000, 0.1736481776669267785, -0.9848077530122087975 ) ) ;
#3761=CARTESIAN_POINT ( 'NONE',  ( -13.63459212866397685, -3.436278759898153901, 33.07459398097509506 ) ) ;
#3762=EDGE_CURVE ( 'NONE', #14846, #32458, #14960, .T. ) ;
#3763=CARTESIAN_POINT ( 'NONE',  ( -12.46153846153846168, -12.34228464037088635, 31.77849191805839268 ) ) ;
#3765=CARTESIAN_POINT ( 'NONE',  ( -24.00000000000000000, -9.499999999999982236, 27.74999999999999645 ) ) ;
#3766=CARTESIAN_POINT ( 'NONE',  ( -7.623374304885432551, -3.236590943229497253, 32.36255958852954251 ) ) ;
#3767=CARTESIAN_POINT ( 'NONE',  ( -4.376772371362299907, -9.886141570436013382, 34.14413921362392301 ) ) ;
#3769=ORIENTED_EDGE ( 'NONE', *, *, #42615, .T. ) ;
#3771=AXIS2_PLACEMENT_3D ( 'NONE', #57117, #30530, #3495 ) ;
#3772=EDGE_LOOP ( 'NONE', ( #75303, #84039, #61919, #19823 ) ) ;
#3774=EDGE_LOOP ( 'NONE', ( #10199, #84548, #42447, #64543 ) ) ;
#3775=CARTESIAN_POINT ( 'NONE',  ( 6.673053698855464511, -11.56360843649121861, 33.07473185843129926 ) ) ;
#3776=CARTESIAN_POINT ( 'NONE',  ( 10.48523740594639619, -9.418419913701741919, 34.36755862841477693 ) ) ;
#3777=ADVANCED_FACE ( 'NONE', ( #65986 ), #45270, .F. ) ;
#3779=CARTESIAN_POINT ( 'NONE',  ( -14.43838377435986864, -9.804603061927743113, 34.18744698557895845 ) ) ;
#3780=ORIENTED_EDGE ( 'NONE', *, *, #63579, .F. ) ;
#3781=ORIENTED_EDGE ( 'NONE', *, *, #80505, .F. ) ;
#3782=ADVANCED_FACE ( 'NONE', ( #25457 ), #46177, .F. ) ;
#3783=CARTESIAN_POINT ( 'NONE',  ( -2.372962753653082402, -12.46129190929999986, 30.37095296980880832 ) ) ;
#3784=ORIENTED_EDGE ( 'NONE', *, *, #20149, .T. ) ;
#3785=FACE_BOUND ( 'NONE', #28868, .T. ) ;
#3786=CARTESIAN_POINT ( 'NONE',  ( 15.00784301325308157, -9.886141570436013382, 34.14413921362392301 ) ) ;
#3787=CARTESIAN_POINT ( 'NONE',  ( -3.930834802233303282, -11.76359900205217457, 32.36225158514719880 ) ) ;
#3788=ORIENTED_EDGE ( 'NONE', *, *, #26692, .T. ) ;
#3790=CARTESIAN_POINT ( 'NONE',  ( -6.923076923076922462, -2.292212530054420494, 30.41441678777542634 ) ) ;
#3791=CARTESIAN_POINT ( 'NONE',  ( 2.177544337960611642, -11.66186481527757479, 32.95055677023626117 ) ) ;
#3792=VERTEX_POINT ( 'NONE', #72743 ) ;
#3793=LINE ( 'NONE', #59183, #35643 ) ;
#3794=DIRECTION ( 'NONE',  ( 0.000000000000000000, -6.938893903907222067E-15, 1.000000000000000000 ) ) ;
#3795=ORIENTED_EDGE ( 'NONE', *, *, #26653, .T. ) ;
#3796=ADVANCED_FACE ( 'NONE', ( #5187 ), #52027, .F. ) ;
#3797=CARTESIAN_POINT ( 'NONE',  ( -5.076923076923075762, -13.75783147151868846, 33.36296068462461051 ) ) ;
#3799=ORIENTED_EDGE ( 'NONE', *, *, #51457, .F. ) ;
#3800=CARTESIAN_POINT ( 'NONE',  ( 7.146089767170318297, -2.523321265292115090, 31.42251411153756280 ) ) ;
#3801=CARTESIAN_POINT ( 'NONE',  ( -12.39547011053602432, -2.538708090699994813, 30.37095296980875503 ) ) ;
#3802=CYLINDRICAL_SURFACE ( 'NONE', #28339, 0.2499999999999979738 ) ;
#3803=CARTESIAN_POINT ( 'NONE',  ( -8.519285250882628446, -9.272278438253398036, 34.42582936511637115 ) ) ;
#3804=CARTESIAN_POINT ( 'NONE',  ( -18.25002323729296450, -6.695914987888146541, 34.68535235679833306 ) ) ;
#3806=CARTESIAN_POINT ( 'NONE',  ( -0.2115384615384616196, -2.249999999999998668, 29.75000000000000355 ) ) ;
#3807=CARTESIAN_POINT ( 'NONE',  ( -1.384615384615505151, -2.892918686052166066, 31.69288490824153470 ) ) ;
#3808=CARTESIAN_POINT ( 'NONE',  ( 9.915087361285756629, -4.989023458446560255, 34.36081565061822118 ) ) ;
#3809=DIRECTION ( 'NONE',  ( 0.000000000000000000, 0.9848077530122072432, 0.1736481776669354937 ) ) ;
#3810=CARTESIAN_POINT ( 'NONE',  ( 2.980769230769232170, -2.249999999999998668, 29.75000000000000355 ) ) ;
#3811=CARTESIAN_POINT ( 'NONE',  ( -5.076923076923199218, -2.657715359629662988, 31.77849191805970364 ) ) ;
#3813=ORIENTED_EDGE ( 'NONE', *, *, #74543, .T. ) ;
#3814=CARTESIAN_POINT ( 'NONE',  ( 0.3308469948709023556, -12.38065189839062263, 30.83690757178629482 ) ) ;
#3815=ORIENTED_EDGE ( 'NONE', *, *, #58445, .F. ) ;
#3816=VERTEX_POINT ( 'NONE', #4293 ) ;
#3817=EDGE_CURVE ( 'NONE', #44275, #69035, #53547, .T. ) ;
#3818=FACE_OUTER_BOUND ( 'NONE', #11087, .T. ) ;
#3820=ORIENTED_EDGE ( 'NONE', *, *, #78843, .F. ) ;
#3821=CARTESIAN_POINT ( 'NONE',  ( 3.453548772037639214, -10.11255958852955850, 34.01340905677048454 ) ) ;
#3823=CARTESIAN_POINT ( 'NONE',  ( -11.53846153846153655, -1.242168528481310874, 33.36296068462461051 ) ) ;
#3824=EDGE_CURVE ( 'NONE', #48826, #63003, #39538, .T. ) ;
#3825=CARTESIAN_POINT ( 'NONE',  ( -4.826868765284761942, -2.779044189368096163, 31.39831045268886456 ) ) ;
#3827=CARTESIAN_POINT ( 'NONE',  ( 17.93472999944368240, -2.379036618887870436, 30.90682066428148644 ) ) ;
#3828=CARTESIAN_POINT ( 'NONE',  ( -8.638705067467206788, -5.195472089885680766, 34.18748526763464923 ) ) ;
#3829=DIRECTION ( 'NONE',  ( 0.000000000000000000, 0.7660444431189807890, 0.6427876096865361433 ) ) ;
#3830=CARTESIAN_POINT ( 'NONE',  ( -7.846153846153844924, -12.10708131394839349, 31.69288490824020244 ) ) ;
#3832=CARTESIAN_POINT ( 'NONE',  ( 1.607394925883797177, -3.236590943229498585, 32.36255958852954251 ) ) ;
#3833=CARTESIAN_POINT ( 'NONE',  ( 13.13459216039393240, -3.520140089381495585, 33.17453946501458262 ) ) ;
#3835=CARTESIAN_POINT ( 'NONE',  ( 14.43848411551709177, -3.062576670634119758, 32.05464942895959979 ) ) ;
#3836=ORIENTED_EDGE ( 'NONE', *, *, #73095, .T. ) ;
#3838=CARTESIAN_POINT ( 'NONE',  ( -6.673076923076923350, -7.500000000000001776, 35.04278698407183867 ) ) ;
#3840=CARTESIAN_POINT ( 'NONE',  ( -17.07692307692307665, -8.810774026931790459, 35.74407628777942847 ) ) ;
#3842=CARTESIAN_POINT ( 'NONE',  ( 14.08476534878545827, -3.395401636524185474, 33.02366814457250399 ) ) ;
#3843=AXIS2_PLACEMENT_3D ( 'NONE', #83402, #21684, #28908 ) ;
#3844=CARTESIAN_POINT ( 'NONE',  ( -16.15384615384615330, -8.973038597847269315, 34.52809138561121927 ) ) ;
#3845=EDGE_CURVE ( 'NONE', #12325, #44606, #81486, .T. ) ;
#3846=ORIENTED_EDGE ( 'NONE', *, *, #42171, .F. ) ;
#3847=CARTESIAN_POINT ( 'NONE',  ( -1.384615384615383471, -9.780366693483667717, 34.19971097300155094 ) ) ;
#3848=EDGE_LOOP ( 'NONE', ( #9958, #53180 ) ) ;
#3849=ORIENTED_EDGE ( 'NONE', *, *, #73890, .F. ) ;
#3850=CARTESIAN_POINT ( 'NONE',  ( -5.776988648387149539, -5.667800583137508674, 34.40243808032445827 ) ) ;
#3851=CARTESIAN_POINT ( 'NONE',  ( 12.46153846153846168, -2.249999999999998668, 29.50000000000001421 ) ) ;
#3852=CARTESIAN_POINT ( 'NONE',  ( -4.219116154402472674, -12.70778746994557551, 30.41441678777548319 ) ) ;
#3854=CARTESIAN_POINT ( 'NONE',  ( -2.084912766423895558, -11.89424750095246175, 32.13594075562311758 ) ) ;
#3855=ORIENTED_EDGE ( 'NONE', *, *, #77944, .T. ) ;
#3857=ORIENTED_EDGE ( 'NONE', *, *, #30161, .T. ) ;
#3858=CARTESIAN_POINT ( 'NONE',  ( -6.923076923077045919, -12.16647553114689728, 32.15551576947799362 ) ) ;
#3859=CARTESIAN_POINT ( 'NONE',  ( -6.000000000000121680, -9.528491918059723176, 34.59228464037033035 ) ) ;
#3861=CARTESIAN_POINT ( 'NONE',  ( 10.36540787133602493, -4.818429247618089661, 34.26397095200675125 ) ) ;
#3862=CARTESIAN_POINT ( 'NONE',  ( -4.377331097570101193, -8.496056993536548418, 34.65000542017679663 ) ) ;
#3863=CARTESIAN_POINT ( 'NONE',  ( -15.90390063549801347, -2.824170634883621744, 31.52227843825337317 ) ) ;
#3864=TOROIDAL_SURFACE ( 'NONE', #28319, 3.000000000000000888, 2.000000000000000000 ) ;
#3865=ORIENTED_EDGE ( 'NONE', *, *, #23777, .F. ) ;
#3866=ORIENTED_EDGE ( 'NONE', *, *, #468, .T. ) ;
#3868=B_SPLINE_CURVE_WITH_KNOTS ( 'NONE', 3,
 ( #46035, #73066, #37491, #44684, #52787, #11819, #38845, #58207, #5053, #32517 ),
 .UNSPECIFIED., .F., .F.,
 ( 4, 2, 2, 2, 4 ),
 ( 0.000000000000000000, 0.0001954339857564054144, 0.0003908679715128108288, 0.0005863019572692162703, 0.0007817359430256216575 ),
 .UNSPECIFIED. ) ;
#3869=ORIENTED_EDGE ( 'NONE', *, *, #38115, .F. ) ;
#3870=CARTESIAN_POINT ( 'NONE',  ( 15.48071474911737333, -5.852078868378309373, 34.47109172314383585 ) ) ;
#3872=CARTESIAN_POINT ( 'NONE',  ( 7.911409417429871027, -12.46129190930001052, 30.37095296980870174 ) ) ;
#3873=DIRECTION ( 'NONE',  ( 0.000000000000000000, 0.6427876096865368094, 0.7660444431189802339 ) ) ;
#3874=B_SPLINE_CURVE_WITH_KNOTS ( 'NONE', 3,
 ( #3299, #22691, #83973, #15947, #72201, #77194, #64545, #70447, #10516, #29904 ),
 .UNSPECIFIED., .F., .F.,
 ( 4, 2, 2, 2, 4 ),
 ( 0.000000000000000000, 0.0001954339857564083146, 0.0003908679715128166293, 0.0005863019572692249439, 0.0007817359430256332585 ),
 .UNSPECIFIED. ) ;
#3877=CARTESIAN_POINT ( 'NONE',  ( -1.254089946381741871, -2.647132371071621471, 31.75357179365173010 ) ) ;
#3879=DIRECTION ( 'NONE',  ( 0.000000000000000000, 0.1736481776669275834, 0.9848077530122086864 ) ) ;
#3880=CYLINDRICAL_SURFACE ( 'NONE', #68751, 0.2500000000000009437 ) ;
#3881=FACE_BOUND ( 'NONE', #28778, .T. ) ;
#3882=CARTESIAN_POINT ( 'NONE',  ( -16.15384615384615330, -12.29105614889573062, 35.45975837776705220 ) ) ;
#3883=DIRECTION ( 'NONE',  ( -0.000000000000000000, -0.5000000000000009992, -0.8660254037844380415 ) ) ;
#3890=ORIENTED_EDGE ( 'NONE', *, *, #17597, .F. ) ;
#3891=CARTESIAN_POINT ( 'NONE',  ( -8.638705330997124676, -3.625058011473228703, 33.29252011169590020 ) ) ;
#3892=CARTESIAN_POINT ( 'NONE',  ( -5.011667505647053211, -6.026961402152789304, 34.52809138561124769 ) ) ;
#3893=CARTESIAN_POINT ( 'NONE',  ( 10.36536139116316235, -8.475808217655753651, 34.90892951860618609 ) ) ;
#3895=CARTESIAN_POINT ( 'NONE',  ( -22.75000000000000000, -10.50000000000000000, 29.75000000000000355 ) ) ;
#3896=FACE_BOUND ( 'NONE', #17016, .T. ) ;
#3897=CARTESIAN_POINT ( 'NONE',  ( -2.557692307692305267, -2.499999999999998668, 29.75000000000000355 ) ) ;
#3899=AXIS2_PLACEMENT_3D ( 'NONE', #7605, #49903, #68854 ) ;
#3900=CYLINDRICAL_SURFACE ( 'NONE', #75550, 0.2499999999999997502 ) ;
#3901=CARTESIAN_POINT ( 'NONE',  ( 18.00000000000000000, -11.16473453929635440, 33.15142922261926373 ) ) ;
#3902=CARTESIAN_POINT ( 'NONE',  ( 0.5923289025054107038, -2.845873456487965747, 32.17976146951972538 ) ) ;
#3903=CARTESIAN_POINT ( 'NONE',  ( -4.153846153846274980, -11.06231777344772027, 33.60647404775119895 ) ) ;
#3904=CARTESIAN_POINT ( 'NONE',  ( 8.834486340506792601, -10.90142922261932057, 33.41473453929631887 ) ) ;
#3906=ORIENTED_EDGE ( 'NONE', *, *, #40114, .T. ) ;
#3907=EDGE_CURVE ( 'NONE', #77663, #76807, #19095, .T. ) ;
#3908=B_SPLINE_CURVE_WITH_KNOTS ( 'NONE', 3,
 ( #9131, #10779, #66155, #66618, #58956, #59409, #84348, #42916, #4920, #32385 ),
 .UNSPECIFIED., .F., .F.,
 ( 4, 2, 2, 2, 4 ),
 ( 0.0007817359430256374869, 0.0009771253907250054306, 0.001172514838424373266, 0.001367904286123741101, 0.001563293733823109153 ),
 .UNSPECIFIED. ) ;
#3909=CARTESIAN_POINT ( 'NONE',  ( -8.096130577096200653, -11.28823185664190376, 33.01397839955799896 ) ) ;
#3910=CARTESIAN_POINT ( 'NONE',  ( 5.076923076923075762, -13.20930481340135110, 34.54067556320372745 ) ) ;
#3911=CARTESIAN_POINT ( 'NONE',  ( 5.869309396889694774, -5.496505350115500121, 34.60290016733514307 ) ) ;
#3913=CARTESIAN_POINT ( 'NONE',  ( 2.307692307692309264, -13.87047571288749737, 32.06866353760679544 ) ) ;
#3914=CARTESIAN_POINT ( 'NONE',  ( -12.46153846153858424, -6.835583212225970762, 34.95778746994575670 ) ) ;
#3916=CARTESIAN_POINT ( 'NONE',  ( -15.29685161012936767, -12.62096338111211580, 30.90682066428152908 ) ) ;
#3917=DIRECTION ( 'NONE',  ( 0.000000000000000000, 0.6427876096865368094, 0.7660444431189802339 ) ) ;
#3918=CARTESIAN_POINT ( 'NONE',  ( -7.715363405186896451, -9.929761469519743144, 34.40412654351204225 ) ) ;
#3919=FACE_OUTER_BOUND ( 'NONE', #55815, .T. ) ;
#3920=CARTESIAN_POINT ( 'NONE',  ( -6.989160334032802346, -4.098570777380720287, 33.41473453929634729 ) ) ;
#3921=CARTESIAN_POINT ( 'NONE',  ( 5.207713517890025123, -8.191423895709842640, 34.95447573519442130 ) ) ;
#3922=LINE ( 'NONE', #72385, #16048 ) ;
#3923=ADVANCED_FACE ( 'NONE', ( #47936 ), #28113, .F. ) ;
#3924=CYLINDRICAL_SURFACE ( 'NONE', #78726, 0.2499999999999994726 ) ;
#3926=DIRECTION ( 'NONE',  ( -0.000000000000000000, 0.7660444431189791237, -0.6427876096865379196 ) ) ;
#3927=CARTESIAN_POINT ( 'NONE',  ( -5.750054590621957118, -2.589246495874657938, 31.60778113518102828 ) ) ;
#3930=CARTESIAN_POINT ( 'NONE',  ( -10.86536135943320502, -2.544273027872575366, 31.48422191005632342 ) ) ;
#3931=CARTESIAN_POINT ( 'NONE',  ( -39.05038313613820122, -2.249999999999998668, 29.75000000000000355 ) ) ;
#3932=ORIENTED_EDGE ( 'NONE', *, *, #27797, .T. ) ;
#3933=CARTESIAN_POINT ( 'NONE',  ( 10.61538461538461675, -6.386643153685126251, 34.62446782046654192 ) ) ;
#3934=CYLINDRICAL_SURFACE ( 'NONE', #28728, 0.2500000000000012212 ) ;
#3935=CARTESIAN_POINT ( 'NONE',  ( 8.769230769230768274, -2.486705287966279876, 31.30864560766543647 ) ) ;
#3936=VERTEX_POINT ( 'NONE', #68220 ) ;
#3937=CARTESIAN_POINT ( 'NONE',  ( -13.63459212866397685, -10.06842814019191401, 34.32929386961144758 ) ) ;
#3938=CARTESIAN_POINT ( 'NONE',  ( 15.23076923076923173, -6.435427911321262684, 35.78748833219616898 ) ) ;
#3940=DIRECTION ( 'NONE',  ( -0.000000000000000000, -0.3420201433256694346, -0.9396926207859080948 ) ) ;
#3941=CARTESIAN_POINT ( 'NONE',  ( -13.38461538461538325, -3.050289026998446396, 32.03036669348365706 ) ) ;
#3942=EDGE_LOOP ( 'NONE', ( #35822, #28676, #75035, #62032 ) ) ;
#3943=DIRECTION ( 'NONE',  ( -0.000000000000000000, 0.3420201433256694346, -0.9396926207859080948 ) ) ;
#3946=DIRECTION ( 'NONE',  ( -0.000000000000000000, 0.8660254037844397068, -0.4999999999999978906 ) ) ;
#3947=ORIENTED_EDGE ( 'NONE', *, *, #60976, .F. ) ;
#3949=EDGE_CURVE ( 'NONE', #43000, #60966, #41755, .T. ) ;
#3950=ORIENTED_EDGE ( 'NONE', *, *, #9686, .T. ) ;
#3951=ADVANCED_FACE ( 'NONE', ( #203 ), #83069, .F. ) ;
#3954=CARTESIAN_POINT ( 'NONE',  ( 6.130525438233648039, -2.372941743896878286, 30.88044141588254377 ) ) ;
#3955=CARTESIAN_POINT ( 'NONE',  ( -9.469294848214296678, -12.64618726649961289, 30.78989965857442712 ) ) ;
#3958=AXIS2_PLACEMENT_3D ( 'NONE', #26557, #26996, #54011 ) ;
#3959=ORIENTED_EDGE ( 'NONE', *, *, #37262, .T. ) ;
#3960=CARTESIAN_POINT ( 'NONE',  ( 15.36129493253279499, -5.195472089885680766, 34.18748526763464923 ) ) ;
#3961=VERTEX_POINT ( 'NONE', #6522 ) ;
#3962=CARTESIAN_POINT ( 'NONE',  ( -5.207613680033381875, -2.494641256782728966, 31.33461815524612959 ) ) ;
#3963=B_SPLINE_CURVE_WITH_KNOTS ( 'NONE', 3,
 ( #63054, #77471, #69392, #63944, #83354, #21639, #22089, #69829, #1368, #8136 ),
 .UNSPECIFIED., .F., .F.,
 ( 4, 2, 2, 2, 4 ),
 ( 0.000000000000000000, 0.0001954311564186868473, 0.0003908623128373736946, 0.0005862934692560605419, 0.0007817246256747473893 ),
 .UNSPECIFIED. ) ;
#3964=CARTESIAN_POINT ( 'NONE',  ( 12.46153846153846168, -11.35647404775217417, 33.31231777344666511 ) ) ;
#3965=CARTESIAN_POINT ( 'NONE',  ( 2.530703659305158393, -3.587049720035815348, 32.86302985866382897 ) ) ;
#3966=CARTESIAN_POINT ( 'NONE',  ( -1.134669975237340367, -12.68172785388650681, 30.59649109432439573 ) ) ;
#3967=ORIENTED_EDGE ( 'NONE', *, *, #75764, .F. ) ;
#3968=ORIENTED_EDGE ( 'NONE', *, *, #34909, .F. ) ;
#3969=ORIENTED_EDGE ( 'NONE', *, *, #48301, .F. ) ;
#3970=CARTESIAN_POINT ( 'NONE',  ( 5.326977388561390470, -4.943051570960391494, 34.04725096376909477 ) ) ;
#3971=ORIENTED_EDGE ( 'NONE', *, *, #76726, .T. ) ;
#3973=ADVANCED_FACE ( 'NONE', ( #67775 ), #83519, .F. ) ;
#3974=VECTOR ( 'NONE', #64826, 1000.000000000000000 ) ;
#3975=CARTESIAN_POINT ( 'NONE',  ( -13.51530685128294351, -6.413092428213692742, 34.63065189839063152 ) ) ;
#3977=CARTESIAN_POINT ( 'NONE',  ( 12.46153846153833911, -6.835583212225970762, 34.95778746994575670 ) ) ;
#3978=CARTESIAN_POINT ( 'NONE',  ( -2.307692307692305711, -12.29105614889573062, 35.45975837776705220 ) ) ;
#3979=DIRECTION ( 'NONE',  ( 1.000000000000000000, 0.000000000000000000, 0.000000000000000000 ) ) ;
#3980=VECTOR ( 'NONE', #70242, 1000.000000000000000 ) ;
#3981=FACE_BOUND ( 'NONE', #25485, .T. ) ;
#3982=CARTESIAN_POINT ( 'NONE',  ( -0.6844646790546080606, -4.186968288167446595, 33.49512374952580274 ) ) ;
#3983=CARTESIAN_POINT ( 'NONE',  ( 9.469480999828689960, -7.369208160676172348, 34.74850200257122879 ) ) ;
#3984=LINE ( 'NONE', #2214, #62440 ) ;
#3985=DIRECTION ( 'NONE',  ( -0.000000000000000000, 0.6427876096865404731, -0.7660444431189770143 ) ) ;
#3986=CARTESIAN_POINT ( 'NONE',  ( -5.869474298236436738, -2.882268652242224505, 31.66798894389554064 ) ) ;
#3987=CARTESIAN_POINT ( 'NONE',  ( -11.47239318745910097, -3.050289026998446840, 32.03036669348366416 ) ) ;
#3989=ORIENTED_EDGE ( 'NONE', *, *, #57321, .T. ) ;
#3990=CARTESIAN_POINT ( 'NONE',  ( -16.15384615384627409, -3.643525952248796163, 33.31231777344771672 ) ) ;
#3991=CARTESIAN_POINT ( 'NONE',  ( -7.596208327805703320, -2.587454068350147462, 30.68340429815432202 ) ) ;
#3994=EDGE_CURVE ( 'NONE', #78946, #64675, #15916, .T. ) ;
#3995=CARTESIAN_POINT ( 'NONE',  ( -11.60454391782167605, -12.62096338111211580, 30.90682066428152908 ) ) ;
#3996=CARTESIAN_POINT ( 'NONE',  ( -5.869208192175212169, -12.11778462344220841, 31.66786338562085135 ) ) ;
#3997=CARTESIAN_POINT ( 'NONE',  ( -6.857821351800898135, -6.879047030191282275, 34.71129190930002295 ) ) ;
#3999=CARTESIAN_POINT ( 'NONE',  ( -14.98076923076779465, -7.500000000000155431, 34.75000000000007105 ) ) ;
#4000=EDGE_LOOP ( 'NONE', ( #72568, #88952 ) ) ;
#4001=CARTESIAN_POINT ( 'NONE',  ( 5.326923076923075762, -7.500000000000001776, 35.04278698407183867 ) ) ;
#4002=CARTESIAN_POINT ( 'NONE',  ( -1.384615384615506484, -12.16647553114689728, 32.15551576947799362 ) ) ;
#4004=CYLINDRICAL_SURFACE ( 'NONE', #61751, 0.2499999999999998890 ) ;
#4005=CARTESIAN_POINT ( 'NONE',  ( -1.634638608836840756, -10.18141759479407327, 34.26406193332782379 ) ) ;
#4006=CARTESIAN_POINT ( 'NONE',  ( 0.2115152373170040290, -3.520140089381497361, 33.17453946501458262 ) ) ;
#4007=CARTESIAN_POINT ( 'NONE',  ( -17.01166793741023042, -2.657715359629131857, 31.77849191805844242 ) ) ;
#4009=ORIENTED_EDGE ( 'NONE', *, *, #36789, .T. ) ;
#4010=VERTEX_POINT ( 'NONE', #57796 ) ;
#4013=LINE ( 'NONE', #31954, #31966 ) ;
#4014=CARTESIAN_POINT ( 'NONE',  ( 17.07692307692295586, -4.320704448113951379, 33.92786785259630022 ) ) ;
#4015=DIRECTION ( 'NONE',  ( -0.000000000000000000, -0.5000000000000009992, -0.8660254037844380415 ) ) ;
#4016=CARTESIAN_POINT ( 'NONE',  ( 3.930919194939304973, -10.77366814457252175, 33.85459836347579454 ) ) ;
#4017=EDGE_CURVE ( 'NONE', #65065, #26721, #85722, .T. ) ;
#4018=CYLINDRICAL_SURFACE ( 'NONE', #57208, 0.2500000000000008882 ) ;
#4020=CARTESIAN_POINT ( 'NONE',  ( -11.76194646302586655, -9.417330523894424488, 34.63758898049880486 ) ) ;
#4021=LINE ( 'NONE', #32402, #50337 ) ;
#4023=CYLINDRICAL_SURFACE ( 'NONE', #44457, 0.2500000000000009437 ) ;
#4024=DIRECTION ( 'NONE',  ( -0.000000000000000000, -0.7660444431189791237, -0.6427876096865379196 ) ) ;
#4026=CARTESIAN_POINT ( 'NONE',  ( 3.361294932532794100, -2.882268652242222284, 31.66798894389554064 ) ) ;
#4027=CARTESIAN_POINT ( 'NONE',  ( -18.00000000000000000, -5.184797716151534175, 36.11096599634342397 ) ) ;
#4028=CARTESIAN_POINT ( 'NONE',  ( 17.32692307692307665, -2.499999999999998668, 29.75000000000000355 ) ) ;
#4029=CARTESIAN_POINT ( 'NONE',  ( 10.83839596699746366, -2.758310577978208666, 31.33698337089302299 ) ) ;
#4030=ADVANCED_FACE ( 'NONE', ( #35772 ), #2838, .F. ) ;
#4031=CARTESIAN_POINT ( 'NONE',  ( 7.780071466793711643, -3.322132147404559532, 32.92929555188719348 ) ) ;
#4032=CARTESIAN_POINT ( 'NONE',  ( -15.23076923076935074, -3.300289026999228881, 32.46337939537708905 ) ) ;
#4033=ORIENTED_EDGE ( 'NONE', *, *, #88681, .F. ) ;
#4035=CARTESIAN_POINT ( 'NONE',  ( -5.326923076923075762, -7.500000000000001776, 35.00000000000000000 ) ) ;
#4038=EDGE_CURVE ( 'NONE', #56240, #51377, #5212, .T. ) ;
#4039=CARTESIAN_POINT ( 'NONE',  ( -14.24162395668986747, -4.786620604624113540, 33.94971097300155805 ) ) ;
#4040=CARTESIAN_POINT ( 'NONE',  ( 2.530705151785703322, -11.98016756924214832, 32.48728574198911190 ) ) ;
#4041=CARTESIAN_POINT ( 'NONE',  ( 10.39255651774974076, -7.369209533119137845, 34.99857337881830688 ) ) ;
#4044=DIRECTION ( 'NONE',  ( -0.000000000000000000, 0.5000000000000011102, -0.8660254037844381525 ) ) ;
#4045=EDGE_CURVE ( 'NONE', #41861, #52419, #8406, .T. ) ;
#4046=B_SPLINE_CURVE_WITH_KNOTS ( 'NONE', 3,
 ( #60153, #38564, #66018, #73236, #25492, #66479 ),
 .UNSPECIFIED., .F., .F.,
 ( 4, 2, 4 ),
 ( 4.220987180333913997E-17, 0.0001954756301637156914, 0.0003909512603273892074 ),
 .UNSPECIFIED. ) ;
#4047=VERTEX_POINT ( 'NONE', #8743 ) ;
#4048=CARTESIAN_POINT ( 'NONE',  ( 6.673053698855467175, -6.652501968072646932, 34.93155406624980941 ) ) ;
#4050=CARTESIAN_POINT ( 'NONE',  ( 3.230769230769231726, -1.466349020453238561, 30.81389545987213907 ) ) ;
#4051=CARTESIAN_POINT ( 'NONE',  ( -1.515305987725691361, -11.93127051446800024, 32.56575433478200665 ) ) ;
#4052=EDGE_CURVE ( 'NONE', #15474, #19611, #80362, .T. ) ;
#4053=CARTESIAN_POINT ( 'NONE',  ( 17.07692307692295586, -6.835583212225970762, 34.95778746994575670 ) ) ;
#4054=VERTEX_POINT ( 'NONE', #37520 ) ;
#4055=CARTESIAN_POINT ( 'NONE',  ( -10.48459280755982981, -12.38066358083363738, 30.83685684665853444 ) ) ;
#4056=ORIENTED_EDGE ( 'NONE', *, *, #50291, .T. ) ;
#4057=CARTESIAN_POINT ( 'NONE',  ( -6.000000000000121680, -2.379036618888197729, 30.90682066428292885 ) ) ;
#4059=EDGE_LOOP ( 'NONE', ( #64446, #17971, #7795, #35113 ) ) ;
#4060=CARTESIAN_POINT ( 'NONE',  ( -0.4615384615385826339, -3.300289026999228881, 32.46337939537708905 ) ) ;
#4061=FACE_OUTER_BOUND ( 'NONE', #78141, .T. ) ;
#4062=EDGE_CURVE ( 'NONE', #63180, #2976, #24504, .T. ) ;
#4064=EDGE_CURVE ( 'NONE', #85264, #74870, #71429, .T. ) ;
#4065=LINE ( 'NONE', #45945, #46226 ) ;
#4066=CARTESIAN_POINT ( 'NONE',  ( 10.61538461538461675, -12.78798330534103123, 29.99999999999997868 ) ) ;
#4067=DIRECTION ( 'NONE',  ( -0.000000000000000000, -0.1736481776669307198, -0.9848077530122080203 ) ) ;
#4068=DIRECTION ( 'NONE',  ( 0.000000000000000000, 0.4999999999999985567, 0.8660254037844395958 ) ) ;
#4069=CARTESIAN_POINT ( 'NONE',  ( -18.00000000000000000, -5.557115091759784242, 34.35708131394839171 ) ) ;
#4070=ORIENTED_EDGE ( 'NONE', *, *, #77427, .T. ) ;
#4071=ORIENTED_EDGE ( 'NONE', *, *, #18028, .T. ) ;
#4072=EDGE_LOOP ( 'NONE', ( #78909, #62436, #43868, #71226 ) ) ;
#4073=CARTESIAN_POINT ( 'NONE',  ( 15.23076923076923173, -2.538708090699994813, 30.37095296980875503 ) ) ;
#4075=B_SPLINE_CURVE_WITH_KNOTS ( 'NONE', 3,
 ( #75609, #1285, #14358, #22882, #2167, #848 ),
 .UNSPECIFIED., .F., .F.,
 ( 4, 2, 4 ),
 ( 0.000000000000000000, 0.0001954784845028902692, 0.0003909569690057805385 ),
 .UNSPECIFIED. ) ;
#4076=CARTESIAN_POINT ( 'NONE',  ( -6.923076923076922462, -8.120952969808772792, 34.71129190930000163 ) ) ;
#4077=CARTESIAN_POINT ( 'NONE',  ( 6.250054419913455561, -10.06805714834173848, 34.32951233291982618 ) ) ;
#4078=B_SPLINE_CURVE_WITH_KNOTS ( 'NONE', 3,
 ( #30981, #31440, #36859, #30548, #64321, #24225, #57576, #79632, #79185, #17486 ),
 .UNSPECIFIED., .F., .F.,
 ( 4, 2, 2, 2, 4 ),
 ( 0.000000000000000000, 0.0001954339857564090194, 0.0003908679715128180387, 0.0005863019572692270039, 0.0007817359430256360774 ),
 .UNSPECIFIED. ) ;
#4079=ORIENTED_EDGE ( 'NONE', *, *, #62537, .T. ) ;
#4080=EDGE_CURVE ( 'NONE', #62746, #27408, #42707, .T. ) ;
#4081=ORIENTED_EDGE ( 'NONE', *, *, #16703, .F. ) ;
#4082=DIRECTION ( 'NONE',  ( -0.000000000000000000, -0.5000000000000009992, -0.8660254037844380415 ) ) ;
#4083=ORIENTED_EDGE ( 'NONE', *, *, #3436, .F. ) ;
#4085=CARTESIAN_POINT ( 'NONE',  ( 11.60452988946397745, -11.16473453929635440, 33.15142922261926373 ) ) ;
#4086=ADVANCED_FACE ( 'NONE', ( #88735 ), #67121, .F. ) ;
#4087=CARTESIAN_POINT ( 'NONE',  ( 17.01084069756293715, -12.34228464037088280, 31.77849191805838558 ) ) ;
#4088=ADVANCED_FACE ( 'NONE', ( #19368 ), #12174, .F. ) ;
#4089=CARTESIAN_POINT ( 'NONE',  ( -16.08859101433330707, -11.06231777344670775, 33.60647404775212266 ) ) ;
#4090=ADVANCED_FACE ( 'NONE', ( #12619 ), #59906, .F. ) ;
#4091=FACE_BOUND ( 'NONE', #82233, .T. ) ;
#4092=EDGE_LOOP ( 'NONE', ( #69559, #18044 ) ) ;
#4093=CARTESIAN_POINT ( 'NONE',  ( -7.846153846153844924, -2.499999999999998668, 29.75000000000001421 ) ) ;
#4094=DIRECTION ( 'NONE',  ( 0.000000000000000000, 0.7660444431189807890, 0.6427876096865361433 ) ) ;
#4095=EDGE_CURVE ( 'NONE', #56825, #33571, #11733, .T. ) ;
#4096=CARTESIAN_POINT ( 'NONE',  ( -13.38461538461538325, -12.62096338111211580, 30.90682066428153263 ) ) ;
#4097=CARTESIAN_POINT ( 'NONE',  ( -14.37296275365308418, -9.442884908240170461, 34.35708131394840592 ) ) ;
#4099=ORIENTED_EDGE ( 'NONE', *, *, #75056, .F. ) ;
#4100=CARTESIAN_POINT ( 'NONE',  ( -7.146561866800870355, -6.760086850603068243, 34.69517049084099369 ) ) ;
#4102=ORIENTED_EDGE ( 'NONE', *, *, #37745, .F. ) ;
#4104=CARTESIAN_POINT ( 'NONE',  ( -7.146561847641255127, -4.225889041578354544, 33.85425143139329407 ) ) ;
#4105=CARTESIAN_POINT ( 'NONE',  ( -1.449885385171703289, -5.941354392334500467, 34.76329471203369792 ) ) ;
#4106=CARTESIAN_POINT ( 'NONE',  ( -8.519285359852727169, -12.45601412856602686, 31.48342859153981621 ) ) ;
#4108=CARTESIAN_POINT ( 'NONE',  ( 1.515407192440173301, -9.804649428959606894, 34.18742332936588468 ) ) ;
#4109=CARTESIAN_POINT ( 'NONE',  ( -11.60454391782167427, -2.292212530054419606, 30.41441678777542634 ) ) ;
#4110=ORIENTED_EDGE ( 'NONE', *, *, #23019, .T. ) ;
#4111=CARTESIAN_POINT ( 'NONE',  ( 6.699591998512590685, -2.612411019501189813, 31.66733052389439962 ) ) ;
#4112=DIRECTION ( 'NONE',  ( -0.000000000000000000, -0.5000000000000009992, -0.8660254037844380415 ) ) ;
#4113=CARTESIAN_POINT ( 'NONE',  ( 2.307692307692186251, -12.70778746994576025, 30.41441678777401236 ) ) ;
#4114=CARTESIAN_POINT ( 'NONE',  ( 10.86533013373275836, -11.86320923018887719, 32.19269448109604070 ) ) ;
#4115=VERTEX_POINT ( 'NONE', #13058 ) ;
#4116=VECTOR ( 'NONE', #46671, 1000.000000000000000 ) ;
#4117=B_SPLINE_CURVE_WITH_KNOTS ( 'NONE', 3,
 ( #88072, #25892, #81291, #74522, #12817, #73651 ),
 .UNSPECIFIED., .F., .F.,
 ( 4, 2, 4 ),
 ( 0.0003909569690057827069, 0.0005862646681846092828, 0.0007815723673634358045 ),
 .UNSPECIFIED. ) ;
#4118=ORIENTED_EDGE ( 'NONE', *, *, #24235, .F. ) ;
#4119=FACE_BOUND ( 'NONE', #73231, .T. ) ;
#4121=VERTEX_POINT ( 'NONE', #20260 ) ;
#4122=CARTESIAN_POINT ( 'NONE',  ( 18.24994540937804643, -12.68172785388650681, 30.59649109432439573 ) ) ;
#4123=CARTESIAN_POINT ( 'NONE',  ( 6.923076923076924238, -12.10708131394839349, 31.69288490824020244 ) ) ;
#4124=ORIENTED_EDGE ( 'NONE', *, *, #20014, .T. ) ;
#4125=CARTESIAN_POINT ( 'NONE',  ( -3.361460697436789324, -12.38065189839062263, 30.83690757178629482 ) ) ;
#4126=FACE_OUTER_BOUND ( 'NONE', #733, .T. ) ;
#4127=CYLINDRICAL_SURFACE ( 'NONE', #16458, 0.2499999999999997502 ) ;
#4129=CARTESIAN_POINT ( 'NONE',  ( -1.384615384615383471, -3.937682226553329556, 33.60647404775216529 ) ) ;
#4130=EDGE_CURVE ( 'NONE', #20820, #6804, #87878, .T. ) ;
#4131=CARTESIAN_POINT ( 'NONE',  ( -0.4615384615384611200, -1.629998284177014645, 34.34916445242399163 ) ) ;
#4133=CARTESIAN_POINT ( 'NONE',  ( -15.10024379253558635, -2.372941743896879174, 30.88044141588253666 ) ) ;
#4134=ORIENTED_EDGE ( 'NONE', *, *, #49668, .F. ) ;
#4135=CARTESIAN_POINT ( 'NONE',  ( -16.15384615384615330, -2.499999999999998668, 29.75000000000001421 ) ) ;
#4136=CARTESIAN_POINT ( 'NONE',  ( 15.23076923076910916, -5.094484230521993062, 34.41647553114689373 ) ) ;
#4137=LINE ( 'NONE', #37479, #81837 ) ;
#4138=CARTESIAN_POINT ( 'NONE',  ( 18.25005431163831204, -8.303483539816726378, 34.68545999027711702 ) ) ;
#4139=CARTESIAN_POINT ( 'NONE',  ( -5.999999999999683808, -2.255955759149395501, 30.00000000000324363 ) ) ;
#4140=CARTESIAN_POINT ( 'NONE',  ( 5.326977388561390470, -12.41262288849542017, 30.68299917996395010 ) ) ;
#4142=ORIENTED_EDGE ( 'NONE', *, *, #16662, .F. ) ;
#4143=DIRECTION ( 'NONE',  ( -0.000000000000000000, 0.3420201433256694346, -0.9396926207859080948 ) ) ;
#4144=LINE ( 'NONE', #39735, #21807 ) ;
#4145=FACE_OUTER_BOUND ( 'NONE', #47836, .T. ) ;
#4146=B_SPLINE_CURVE_WITH_KNOTS ( 'NONE', 3,
 ( #59943, #75244, #13974, #77013, #69805, #83779, #63485, #48199, #56293, #41904 ),
 .UNSPECIFIED., .F., .F.,
 ( 4, 2, 2, 2, 4 ),
 ( 0.000000000000000000, 0.0001954339857564091007, 0.0003908679715128182013, 0.0005863019572692273291, 0.0007817359430256364027 ),
 .UNSPECIFIED. ) ;
#4147=AXIS2_PLACEMENT_3D ( 'NONE', #88267, #13459, #32850 ) ;
#4148=ORIENTED_EDGE ( 'NONE', *, *, #48127, .F. ) ;
#4150=CARTESIAN_POINT ( 'NONE',  ( -8.992715693795100051, -5.827078755546623690, 34.72654668319379567 ) ) ;
#4151=CARTESIAN_POINT ( 'NONE',  ( -7.846153846153967493, -5.941354392335915335, 34.76329471203413846 ) ) ;
#4152=CARTESIAN_POINT ( 'NONE',  ( -0.7115152055870527237, -9.234221910056348293, 34.70572697212741531 ) ) ;
#4153=B_SPLINE_CURVE_WITH_KNOTS ( 'NONE', 3,
 ( #81455, #75138, #87783, #26500, #19740, #26056, #53963, #27386, #87331, #74693 ),
 .UNSPECIFIED., .F., .F.,
 ( 4, 2, 2, 2, 4 ),
 ( 0.000000000000000000, 0.0001954311564186868202, 0.0003908623128373735320, 0.0005862934692560603251, 0.0007817246256747470640 ),
 .UNSPECIFIED. ) ;
#4154=VECTOR ( 'NONE', #80200, 1000.000000000000000 ) ;
#4155=CARTESIAN_POINT ( 'NONE',  ( 13.31853300525525086, -2.833524468853757305, 32.15551576947924417 ) ) ;
#4156=B_SPLINE_CURVE_WITH_KNOTS ( 'NONE', 3,
 ( #32813, #81457, #74696, #12986, #28718, #7562, #62052, #70138, #8449, #35921 ),
 .UNSPECIFIED., .F., .F.,
 ( 4, 2, 2, 2, 4 ),
 ( 0.0007817359430256215491, 0.0009771253907249856981, 0.001172514838424349847, 0.001367904286123713779, 0.001563293733823077928 ),
 .UNSPECIFIED. ) ;
#4158=AXIS2_PLACEMENT_3D ( 'NONE', #66634, #18450, #74282 ) ;
#4159=CARTESIAN_POINT ( 'NONE',  ( -7.146003140593069958, -11.76352882383564769, 32.36236540154569497 ) ) ;
#4160=B_SPLINE_CURVE_WITH_KNOTS ( 'NONE', 3,
 ( #55784, #82835, #22009, #75610, #35075, #14359, #76953, #20676, #40523, #7167 ),
 .UNSPECIFIED., .F., .F.,
 ( 4, 2, 2, 2, 4 ),
 ( 0.000000000000000000, 0.0001954311584214072923, 0.0003908623168428145846, 0.0005862934752642218498, 0.0007817246336856291692 ),
 .UNSPECIFIED. ) ;
#4161=ORIENTED_EDGE ( 'NONE', *, *, #42753, .F. ) ;
#4162=CARTESIAN_POINT ( 'NONE',  ( -3.230769230769352962, -12.70778746994576025, 30.41441678777401236 ) ) ;
#4164=EDGE_CURVE ( 'NONE', #22486, #11909, #49253, .T. ) ;
#4166=EDGE_CURVE ( 'NONE', #40441, #40827, #64213, .T. ) ;
#4167=CARTESIAN_POINT ( 'NONE',  ( 7.053602361310569613, -6.808710257144159783, 34.95449254468098843 ) ) ;
#4168=CARTESIAN_POINT ( 'NONE',  ( 17.07692307692339284, -2.255955759149395501, 30.00000000000324363 ) ) ;
#4169=ORIENTED_EDGE ( 'NONE', *, *, #50814, .F. ) ;
#4171=ADVANCED_FACE ( 'NONE', ( #18928 ), #46397, .F. ) ;
#4172=EDGE_LOOP ( 'NONE', ( #11667, #17271 ) ) ;
#4173=CARTESIAN_POINT ( 'NONE',  ( 1.634615384615450084, -7.434744429011176159, 34.75000000000000711 ) ) ;
#4175=CARTESIAN_POINT ( 'NONE',  ( 16.40384615384617462, -2.249999999999997780, 29.81603969181029257 ) ) ;
#4176=CARTESIAN_POINT ( 'NONE',  ( -0.4615384615384611200, -4.661471528628507777, 34.16647553114623292 ) ) ;
#4177=ORIENTED_EDGE ( 'NONE', *, *, #5225, .F. ) ;
#4178=ADVANCED_FACE ( 'NONE', ( #8518 ), #7634, .F. ) ;
#4180=CARTESIAN_POINT ( 'NONE',  ( 5.869308533332442401, -9.804603061927743113, 34.18744698557895845 ) ) ;
#4181=CARTESIAN_POINT ( 'NONE',  ( -6.792551484843277976, -12.50538340440932217, 31.33453814440721885 ) ) ;
#4182=EDGE_CURVE ( 'NONE', #29819, #65895, #7294, .T. ) ;
#4185=ORIENTED_EDGE ( 'NONE', *, *, #52252, .F. ) ;
#4186=CARTESIAN_POINT ( 'NONE',  ( 7.596177102105255763, -11.47974371597207899, 33.17467449705390692 ) ) ;
#4187=ORIENTED_EDGE ( 'NONE', *, *, #69668, .F. ) ;
#4188=CARTESIAN_POINT ( 'NONE',  ( 5.207713517890026900, -11.37503395064541678, 33.29242100308974983 ) ) ;
#4189=EDGE_CURVE ( 'NONE', #4777, #84330, #21330, .T. ) ;
#4190=AXIS2_PLACEMENT_3D ( 'NONE', #16875, #79022, #17322 ) ;
#4191=FACE_OUTER_BOUND ( 'NONE', #38214, .T. ) ;
#4192=CARTESIAN_POINT ( 'NONE',  ( -0.3310130233048198534, -2.647132371071621915, 31.75357179365173010 ) ) ;
#4193=CARTESIAN_POINT ( 'NONE',  ( 7.715463243043540587, -12.35290016733513951, 31.75349464988449455 ) ) ;
#4194=EDGE_CURVE ( 'NONE', #25778, #5919, #83546, .T. ) ;
#4195=CARTESIAN_POINT ( 'NONE',  ( -5.999999999999998224, -4.098570777380720287, 33.41473453929634729 ) ) ;
#4197=ORIENTED_EDGE ( 'NONE', *, *, #16463, .T. ) ;
#4198=VERTEX_POINT ( 'NONE', #22027 ) ;
#4199=ORIENTED_EDGE ( 'NONE', *, *, #46404, .F. ) ;
#4200=B_SPLINE_CURVE_WITH_KNOTS ( 'NONE', 3,
 ( #62067, #60294, #81917, #74265, #89126, #14327, #6255, #34601, #21073, #53533 ),
 .UNSPECIFIED., .F., .F.,
 ( 4, 2, 2, 2, 4 ),
 ( 0.000000000000000000, 0.0001954339857564074473, 0.0003908679715128148945, 0.0005863019572692223418, 0.0007817359430256297891 ),
 .UNSPECIFIED. ) ;
#4201=ORIENTED_EDGE ( 'NONE', *, *, #73939, .T. ) ;
#4202=EDGE_CURVE ( 'NONE', #79454, #65351, #52420, .T. ) ;
#4203=VERTEX_POINT ( 'NONE', #28333 ) ;
#4205=CYLINDRICAL_SURFACE ( 'NONE', #54603, 0.2500000000000004996 ) ;
#4206=CARTESIAN_POINT ( 'NONE',  ( -10.39260494640654819, -4.989023458446560255, 34.36081565061822118 ) ) ;
#4207=EDGE_CURVE ( 'NONE', #80539, #64011, #78272, .T. ) ;
#4208=CARTESIAN_POINT ( 'NONE',  ( -7.053768389744483613, -3.062553014421049546, 32.05460306192773601 ) ) ;
#4209=CARTESIAN_POINT ( 'NONE',  ( 13.31853197365950692, -8.120952969808774569, 34.71129190930000163 ) ) ;
#4210=CARTESIAN_POINT ( 'NONE',  ( 0.6843180028068696075, -5.114059244376869984, 34.14424750095245287 ) ) ;
#4211=VECTOR ( 'NONE', #14778, 1000.000000000000000 ) ;
#4212=DIRECTION ( 'NONE',  ( 1.000000000000000000, -0.000000000000000000, -0.000000000000000000 ) ) ;
#4214=LINE ( 'NONE', #66811, #56233 ) ;
#4215=EDGE_LOOP ( 'NONE', ( #60600, #50026 ) ) ;
#4217=B_SPLINE_CURVE_WITH_KNOTS ( 'NONE', 3,
 ( #69911, #49198, #56403, #14977, #20837, #83890, #82562, #7772, #76677, #28486 ),
 .UNSPECIFIED., .F., .F.,
 ( 4, 2, 2, 2, 4 ),
 ( 0.000000000000000000, 0.0001954311564186862239, 0.0003908623128373724478, 0.0005862934692560586988, 0.0007817246256747448956 ),
 .UNSPECIFIED. ) ;
#4218=EDGE_LOOP ( 'NONE', ( #49024, #33790, #37115, #25724 ) ) ;
#4220=CARTESIAN_POINT ( 'NONE',  ( 0.3962684609821406356, -12.16647553114622049, 32.15551576947930812 ) ) ;
#4221=EDGE_CURVE ( 'NONE', #65186, #28534, #36325, .T. ) ;
#4222=ORIENTED_EDGE ( 'NONE', *, *, #28490, .T. ) ;
#4223=CARTESIAN_POINT ( 'NONE',  ( -16.15384615384627409, -6.879047030192662504, 34.71129190930017927 ) ) ;
#4224=CARTESIAN_POINT ( 'NONE',  ( -0.4615384615384611200, -1.215029322943914858, 32.30358669280327177 ) ) ;
#4225=DIRECTION ( 'NONE',  ( -0.000000000000000000, 0.3420201433256694346, -0.9396926207859080948 ) ) ;
#4226=CARTESIAN_POINT ( 'NONE',  ( -10.61538461538473399, -11.94971097300221174, 32.03036669348237098 ) ) ;
#4227=FACE_BOUND ( 'NONE', #25106, .T. ) ;
#4228=ORIENTED_EDGE ( 'NONE', *, *, #72896, .T. ) ;
#4229=EDGE_CURVE ( 'NONE', #18188, #20537, #68544, .T. ) ;
#4231=CARTESIAN_POINT ( 'NONE',  ( -6.923076923077045919, -5.094484230521993062, 34.41647553114689373 ) ) ;
#4232=ORIENTED_EDGE ( 'NONE', *, *, #30406, .F. ) ;
#4233=FACE_BOUND ( 'NONE', #70260, .T. ) ;
#4234=CARTESIAN_POINT ( 'NONE',  ( -9.561517251340744039, -2.295524264805589354, 30.44142389570982488 ) ) ;
#4235=FACE_OUTER_BOUND ( 'NONE', #14357, .T. ) ;
#4236=ORIENTED_EDGE ( 'NONE', *, *, #43509, .T. ) ;
#4237=LINE ( 'NONE', #11443, #1743 ) ;
#4238=CYLINDRICAL_SURFACE ( 'NONE', #82165, 0.2500000000000004996 ) ;
#4239=CARTESIAN_POINT ( 'NONE',  ( 2.307692307692309264, -11.35647404775217417, 33.31231777344666511 ) ) ;
#4241=CARTESIAN_POINT ( 'NONE',  ( 12.39545505058258179, -4.786620604624113540, 33.94971097300155805 ) ) ;
#4242=CARTESIAN_POINT ( 'NONE',  ( 3.165498784808456367, -12.27809138561121394, 31.22303859784730307 ) ) ;
#4243=EDGE_CURVE ( 'NONE', #40235, #83058, #10484, .T. ) ;
#4244=ORIENTED_EDGE ( 'NONE', *, *, #41762, .T. ) ;
#4245=ADVANCED_FACE ( 'NONE', ( #30108 ), #10283, .F. ) ;
#4247=CARTESIAN_POINT ( 'NONE',  ( 13.38461538461538680, -9.780366693483667717, 34.19971097300155094 ) ) ;
#4248=ORIENTED_EDGE ( 'NONE', *, *, #80438, .T. ) ;
#4249=CARTESIAN_POINT ( 'NONE',  ( -12.59168643127016196, -5.915902021225889484, 34.75552854090298638 ) ) ;
#4250=CARTESIAN_POINT ( 'NONE',  ( -12.21148414990014963, -2.564540009722895419, 30.55348353981670684 ) ) ;
#4251=CARTESIAN_POINT ( 'NONE',  ( -15.90390063549801347, -8.433404298154332679, 34.66254593164985920 ) ) ;
#4252=CARTESIAN_POINT ( 'NONE',  ( -10.39260507411620260, -5.913360116392397892, 34.49180327182771322 ) ) ;
#4253=CARTESIAN_POINT ( 'NONE',  ( 0.2115617174898712927, -2.544273027872575366, 31.48422191005632342 ) ) ;
#4254=DIRECTION ( 'NONE',  ( 0.000000000000000000, 0.000000000000000000, 1.000000000000000000 ) ) ;
#4255=CARTESIAN_POINT ( 'NONE',  ( -13.45069776397551564, -3.937682226553330445, 33.60647404775217240 ) ) ;
#4256=DIRECTION ( 'NONE',  ( -0.000000000000000000, -0.1736481776669307198, -0.9848077530122080203 ) ) ;
#4257=CARTESIAN_POINT ( 'NONE',  ( 10.83816428436268176, -9.418065098278013636, 34.63729479722530158 ) ) ;
#4258=CARTESIAN_POINT ( 'NONE',  ( 12.23865894480087846, -7.630690623152299956, 34.99857592706774057 ) ) ;
#4259=CARTESIAN_POINT ( 'NONE',  ( -6.673076923075486278, -7.500000000000155431, 34.75000000000007105 ) ) ;
#4262=VERTEX_POINT ( 'NONE', #77847 ) ;
#4263=CARTESIAN_POINT ( 'NONE',  ( -4.023055712879203938, -5.496552790871117367, 34.60292014791297532 ) ) ;
#4264=ORIENTED_EDGE ( 'NONE', *, *, #18566, .F. ) ;
#4265=ORIENTED_EDGE ( 'NONE', *, *, #77504, .F. ) ;
#4266=CARTESIAN_POINT ( 'NONE',  ( -7.623141002060450866, -2.523321265292116422, 31.42251411153756990 ) ) ;
#4267=VERTEX_POINT ( 'NONE', #44048 ) ;
#4268=CARTESIAN_POINT ( 'NONE',  ( -39.05038313613820122, -2.499999999999999556, 29.75000000000000355 ) ) ;
#4270=CARTESIAN_POINT ( 'NONE',  ( -13.31854805126531005, -5.471508081941601098, 34.59228464037088457 ) ) ;
#4271=CARTESIAN_POINT ( 'NONE',  ( -8.992715712954719720, -3.236172620538810385, 32.36188796281390267 ) ) ;
#4273=DIRECTION ( 'NONE',  ( -0.000000000000000000, -0.5000000000000009992, -0.8660254037844380415 ) ) ;
#4274=CARTESIAN_POINT ( 'NONE',  ( -4.853910232829681703, -2.523321265292115090, 31.42251411153756280 ) ) ;
#4275=CYLINDRICAL_SURFACE ( 'NONE', #87637, 0.2499999999999973355 ) ;
#4276=CARTESIAN_POINT ( 'NONE',  ( 5.749976762707035505, -4.335965774309649134, 33.62209801155881905 ) ) ;
#4278=CARTESIAN_POINT ( 'NONE',  ( 1.450683735617824821, -3.050289026998446840, 32.03036669348366416 ) ) ;
#4279=DIRECTION ( 'NONE',  ( 0.000000000000000000, 0.8660254037844377084, -0.5000000000000015543 ) ) ;
#4280=VECTOR ( 'NONE', #42004, 1000.000000000000227 ) ;
#4281=FACE_OUTER_BOUND ( 'NONE', #57087, .T. ) ;
#4282=AXIS2_PLACEMENT_3D ( 'NONE', #37203, #1659, #70557 ) ;
#4283=ORIENTED_EDGE ( 'NONE', *, *, #55584, .T. ) ;
#4284=EDGE_LOOP ( 'NONE', ( #69640, #81347 ) ) ;
#4286=CARTESIAN_POINT ( 'NONE',  ( -17.07692307692319744, -8.613356846316285953, 34.62446782046622218 ) ) ;
#4287=DIRECTION ( 'NONE',  ( 0.000000000000000000, 0.000000000000000000, 1.000000000000000000 ) ) ;
#4288=CARTESIAN_POINT ( 'NONE',  ( -6.988346923633241836, -5.941354392334500467, 34.76329471203369792 ) ) ;
#4289=ADVANCED_FACE ( 'NONE', ( #24679 ), #51228, .F. ) ;
#4290=AXIS2_PLACEMENT_3D ( 'NONE', #16216, #30174, #45001 ) ;
#4292=AXIS2_PLACEMENT_3D ( 'NONE', #78754, #24243, #36017 ) ;
#4293=CARTESIAN_POINT ( 'NONE',  ( 2.307692307692309264, -11.91647553114624181, 32.58852847137148245 ) ) ;
#4295=AXIS2_PLACEMENT_3D ( 'NONE', #3392, #60117, #86737 ) ;
#4296=B_SPLINE_CURVE_WITH_KNOTS ( 'NONE', 3,
 ( #57961, #85441, #62932, #1244, #56197, #21971, #32275, #86797, #58843, #4351 ),
 .UNSPECIFIED., .F., .F.,
 ( 4, 2, 2, 2, 4 ),
 ( 0.0007817246256747463051, 0.0009771112852218896347, 0.001172497944769032747, 0.001367884604316176077, 0.001563271263863319407 ),
 .UNSPECIFIED. ) ;
#4297=ORIENTED_EDGE ( 'NONE', *, *, #15295, .F. ) ;
#4298=CARTESIAN_POINT ( 'NONE',  ( 7.596177102105254875, -2.920706130388546651, 32.31842814019191223 ) ) ;
#4299=VERTEX_POINT ( 'NONE', #9833 ) ;
#4300=B_SPLINE_CURVE_WITH_KNOTS ( 'NONE', 3,
 ( #47224, #75580, #68387, #88690, #82360, #46791, #81919, #27405, #26077, #61624 ),
 .UNSPECIFIED., .F., .F.,
 ( 4, 2, 2, 2, 4 ),
 ( 0.000000000000000000, 0.0001954311564186864949, 0.0003908623128373729899, 0.0005862934692560594577, 0.0007817246256747459798 ),
 .UNSPECIFIED. ) ;
#4301=ADVANCED_FACE ( 'NONE', ( #2622 ), #51682, .F. ) ;
#4302=VERTEX_POINT ( 'NONE', #9399 ) ;
#4303=CARTESIAN_POINT ( 'NONE',  ( -9.561782254074051579, -3.068774925481847493, 32.56582465632704526 ) ) ;
#4304=CARTESIAN_POINT ( 'NONE',  ( 5.869523291883536054, -7.276988635370452485, 34.74523720219453793 ) ) ;
#4305=CARTESIAN_POINT ( 'NONE',  ( -0.5272918898517936492, -7.249945578846653582, 34.99404164642496795 ) ) ;
#4306=CARTESIAN_POINT ( 'NONE',  ( 11.76124120743960333, -2.353885683473779800, 30.79025554430704403 ) ) ;
#4308=ORIENTED_EDGE ( 'NONE', *, *, #85512, .F. ) ;
#4309=EDGE_CURVE ( 'NONE', #6804, #20820, #4078, .T. ) ;
#4310=VERTEX_POINT ( 'NONE', #44938 ) ;
#4311=ORIENTED_EDGE ( 'NONE', *, *, #31894, .F. ) ;
#4312=CARTESIAN_POINT ( 'NONE',  ( -4.023320715612509701, -12.15418822224088657, 32.17964115625579069 ) ) ;
#4313=CARTESIAN_POINT ( 'NONE',  ( -1.384615384615506484, -5.094484230521993062, 34.41647553114689373 ) ) ;
#4314=EDGE_CURVE ( 'NONE', #81411, #2917, #72416, .T. ) ;
#4315=DIRECTION ( 'NONE',  ( 0.000000000000000000, 0.4999999999999985567, 0.8660254037844395958 ) ) ;
#4316=CARTESIAN_POINT ( 'NONE',  ( 2.307692307692309264, -11.16473453929635440, 33.15142922261926373 ) ) ;
#4317=CARTESIAN_POINT ( 'NONE',  ( -11.66860950819323328, -8.630895178749533159, 34.87696386517710323 ) ) ;
#4318=EDGE_CURVE ( 'NONE', #1947, #21625, #27695, .T. ) ;
#4319=CARTESIAN_POINT ( 'NONE',  ( 9.692307692307695177, -8.564572088678739092, 35.78748833219616898 ) ) ;
#4320=ORIENTED_EDGE ( 'NONE', *, *, #28448, .F. ) ;
#4321=ORIENTED_EDGE ( 'NONE', *, *, #25774, .F. ) ;
#4322=DIRECTION ( 'NONE',  ( 0.000000000000000000, 0.9396926207859126468, 0.3420201433256571111 ) ) ;
#4323=EDGE_LOOP ( 'NONE', ( #39501, #2728, #18523, #49780 ) ) ;
#4324=CARTESIAN_POINT ( 'NONE',  ( -5.749945688361685292, -3.136992222400443175, 32.19305428654138979 ) ) ;
#4326=CARTESIAN_POINT ( 'NONE',  ( -10.54931728203453822, -3.937682226553329556, 33.60647404775216529 ) ) ;
#4327=CARTESIAN_POINT ( 'NONE',  ( 8.096153846153846700, -2.499999999999998668, 29.75000000000000355 ) ) ;
#4329=ORIENTED_EDGE ( 'NONE', *, *, #31031, .T. ) ;
#4330=EDGE_CURVE ( 'NONE', #31749, #31146, #2958, .T. ) ;
#4332=CARTESIAN_POINT ( 'NONE',  ( -13.60810032833933292, -12.24155766932282496, 31.33739205006857986 ) ) ;
#4333=VERTEX_POINT ( 'NONE', #46730 ) ;
#4334=CARTESIAN_POINT ( 'NONE',  ( 11.53846153846141753, -2.892918686052165622, 31.69288490824153470 ) ) ;
#4335=CARTESIAN_POINT ( 'NONE',  ( 14.43821774592595197, -12.50538340440932394, 31.33453814440721885 ) ) ;
#4336=FACE_BOUND ( 'NONE', #39804, .T. ) ;
#4337=CARTESIAN_POINT ( 'NONE',  ( -6.923076923076922462, -5.471508081941601098, 34.59228464037088457 ) ) ;
#4338=DIRECTION ( 'NONE',  ( -0.000000000000000000, 0.1736481776669307198, -0.9848077530122080203 ) ) ;
#4340=CARTESIAN_POINT ( 'NONE',  ( -1.514763354347077540, -3.625366637846545448, 33.29286588640298561 ) ) ;
#4341=FACE_OUTER_BOUND ( 'NONE', #61544, .T. ) ;
#4342=EDGE_LOOP ( 'NONE', ( #33568, #63033 ) ) ;
#4343=CYLINDRICAL_SURFACE ( 'NONE', #67685, 0.2500000000000004996 ) ;
#4344=CARTESIAN_POINT ( 'NONE',  ( 15.00728428704528561, -4.386631170607603991, 33.66268669641500111 ) ) ;
#4345=ADVANCED_FACE ( 'NONE', ( #19702 ), #67450, .F. ) ;
#4348=CARTESIAN_POINT ( 'NONE',  ( -8.638440328263817136, -3.338503747796866872, 32.95102852606553512 ) ) ;
#4350=CARTESIAN_POINT ( 'NONE',  ( 14.53047197667037516, -10.23759521482555357, 34.22997729860117033 ) ) ;
#4351=CARTESIAN_POINT ( 'NONE',  ( -13.38461538461538325, -11.35647404775217417, 33.31231777344666511 ) ) ;
#4352=ADVANCED_FACE ( 'NONE', ( #59352 ), #18375, .F. ) ;
#4353=CARTESIAN_POINT ( 'NONE',  ( 12.46153846153833911, -4.320704448113951379, 33.92786785259630022 ) ) ;
#4354=EDGE_CURVE ( 'NONE', #21191, #52651, #15398, .T. ) ;
#4355=FACE_BOUND ( 'NONE', #88030, .T. ) ;
#4356=DIRECTION ( 'NONE',  ( -1.000000000000000000, 0.000000000000000000, 0.000000000000000000 ) ) ;
#4358=LINE ( 'NONE', #59296, #82768 ) ;
#4359=CARTESIAN_POINT ( 'NONE',  ( 18.25005431163831204, -11.28795663066794575, 33.01431243580653785 ) ) ;
#4360=CARTESIAN_POINT ( 'NONE',  ( 9.822833394071258439, -4.459921816937791661, 33.71989282347011851 ) ) ;
#4361=DIRECTION ( 'NONE',  ( -0.000000000000000000, -0.8660254037844399289, -0.4999999999999980016 ) ) ;
#4362=EDGE_CURVE ( 'NONE', #33850, #61846, #12719, .T. ) ;
#4365=EDGE_CURVE ( 'NONE', #82116, #24019, #22274, .T. ) ;
#4366=CARTESIAN_POINT ( 'NONE',  ( -12.71153846153846168, -7.500000000000001776, 35.00000000000000000 ) ) ;
#4367=EDGE_LOOP ( 'NONE', ( #49499, #6334, #67461, #28804 ) ) ;
#4368=CARTESIAN_POINT ( 'NONE',  ( -4.219929564802034072, -11.69971097300155272, 32.46337939537587403 ) ) ;
#4369=CARTESIAN_POINT ( 'NONE',  ( -3.230769230769229949, -1.242168528481310874, 33.36296068462461051 ) ) ;
#4370=CARTESIAN_POINT ( 'NONE',  ( -1.161835843346973762, -10.81320215134717344, 33.49497208177562868 ) ) ;
#4371=CARTESIAN_POINT ( 'NONE',  ( -9.822999158975248335, -10.54014554554150607, 33.71984207302941883 ) ) ;
#4372=CARTESIAN_POINT ( 'NONE',  ( 6.673100179028333301, -12.65889640711025521, 30.72598325615533454 ) ) ;
#4373=CARTESIAN_POINT ( 'NONE',  ( -10.61538461538461320, -1.129524287112498415, 32.06866353760679544 ) ) ;
#4375=DIRECTION ( 'NONE',  ( -0.000000000000000000, 0.9396926207859093161, -0.3420201433256663259 ) ) ;
#4376=LINE ( 'NONE', #17895, #8707 ) ;
#4378=CARTESIAN_POINT ( 'NONE',  ( 8.769230769230768274, -12.78798330534102945, 29.74999999999997868 ) ) ;
#4379=CARTESIAN_POINT ( 'NONE',  ( 14.30769230769218581, -3.083524468854526912, 32.58852847137268327 ) ) ;
#4380=CARTESIAN_POINT ( 'NONE',  ( 1.515405825582336163, -9.929761469519744921, 34.40412654351204225 ) ) ;
#4381=CARTESIAN_POINT ( 'NONE',  ( -12.46153846153846168, -12.29105614889573062, 35.45975837776705220 ) ) ;
#4383=ORIENTED_EDGE ( 'NONE', *, *, #85167, .F. ) ;
#4384=AXIS2_PLACEMENT_3D ( 'NONE', #83254, #31858, #78704 ) ;
#4385=CARTESIAN_POINT ( 'NONE',  ( 16.21991348719623360, -4.661471528628508665, 34.16647553114624003 ) ) ;
#4386=CARTESIAN_POINT ( 'NONE',  ( -12.46153846153846168, -1.242168528481310874, 33.36296068462461051 ) ) ;
#4388=DIRECTION ( 'NONE',  ( -0.000000000000000000, 0.9848077530122085754, -0.1736481776669273613 ) ) ;
#4389=FACE_OUTER_BOUND ( 'NONE', #33317, .T. ) ;
#4390=VERTEX_POINT ( 'NONE', #12073 ) ;
#4391=CARTESIAN_POINT ( 'NONE',  ( 1.384615384615386802, -4.098570777380720287, 33.41473453929634729 ) ) ;
#4392=CARTESIAN_POINT ( 'NONE',  ( -17.07692307692319744, -9.528491918059723176, 34.59228464037033035 ) ) ;
#4393=CARTESIAN_POINT ( 'NONE',  ( 4.826946332874485712, -12.41104346484419452, 31.60698883733904196 ) ) ;
#4394=ORIENTED_EDGE ( 'NONE', *, *, #86524, .T. ) ;
#4395=CARTESIAN_POINT ( 'NONE',  ( -11.40841637562676070, -2.504778602574660340, 29.97347330155780654 ) ) ;
#4396=CARTESIAN_POINT ( 'NONE',  ( -3.007989689500820241, -3.755027918224367767, 33.06320215134714857 ) ) ;
#4397=CARTESIAN_POINT ( 'NONE',  ( -12.46153846153846168, -8.564572088678739092, 35.78748833219616898 ) ) ;
#4398=CARTESIAN_POINT ( 'NONE',  ( -11.66860950819324039, -2.647304123082328875, 31.75400227202885972 ) ) ;
#4399=ORIENTED_EDGE ( 'NONE', *, *, #46738, .F. ) ;
#4400=CARTESIAN_POINT ( 'NONE',  ( -11.53846153846153655, -8.120952969808772792, 34.71129190930000163 ) ) ;
#4401=LINE ( 'NONE', #25117, #46585 ) ;
#4403=ORIENTED_EDGE ( 'NONE', *, *, #35968, .F. ) ;
#4404=EDGE_LOOP ( 'NONE', ( #84042, #53048, #56399, #85782 ) ) ;
#4405=ORIENTED_EDGE ( 'NONE', *, *, #53561, .T. ) ;
#4407=DIRECTION ( 'NONE',  ( -0.000000000000000000, 0.7660444431189791237, -0.6427876096865379196 ) ) ;
#4408=FACE_OUTER_BOUND ( 'NONE', #79355, .T. ) ;
#4409=CARTESIAN_POINT ( 'NONE',  ( 2.530703659305158837, -5.667800583137508674, 34.40243808032445827 ) ) ;
#4410=EDGE_CURVE ( 'NONE', #13301, #6878, #35382, .T. ) ;
#4411=LINE ( 'NONE', #64770, #26209 ) ;
#4412=VERTEX_POINT ( 'NONE', #39551 ) ;
#4413=ORIENTED_EDGE ( 'NONE', *, *, #43709, .T. ) ;
#4414=DIRECTION ( 'NONE',  ( -0.000000000000000000, 1.000000000000000000, -0.000000000000000000 ) ) ;
#4415=ORIENTED_EDGE ( 'NONE', *, *, #43726, .F. ) ;
#4416=CARTESIAN_POINT ( 'NONE',  ( -6.673131513698878692, -4.176053281294514363, 33.81426240980091791 ) ) ;
#4417=B_SPLINE_CURVE_WITH_KNOTS ( 'NONE', 3,
 ( #62459, #70114, #14739, #65005, #42218, #7979, #58257, #57819, #17279, #42655 ),
 .UNSPECIFIED., .F., .F.,
 ( 4, 2, 2, 2, 4 ),
 ( 0.0007817359527651090859, 0.0009771254036996478414, 0.001172514854634186489, 0.001367904305568725136, 0.001563293756503263783 ),
 .UNSPECIFIED. ) ;
#4418=CARTESIAN_POINT ( 'NONE',  ( 15.23076923076911093, -3.300289026999228881, 32.46337939537708905 ) ) ;
#4419=EDGE_CURVE ( 'NONE', #52360, #49441, #4868, .T. ) ;
#4420=CARTESIAN_POINT ( 'NONE',  ( 6.000000000000001776, -3.937682226553329556, 33.60647404775216529 ) ) ;
#4421=CARTESIAN_POINT ( 'NONE',  ( -1.318548051265307830, -12.62096338111211757, 30.90682066428152908 ) ) ;
#4422=EDGE_LOOP ( 'NONE', ( #14875, #83873, #69204, #25680 ) ) ;
#4423=B_SPLINE_CURVE_WITH_KNOTS ( 'NONE', 3,
 ( #74052, #48334, #33056, #88038, #41585, #82139, #13233, #6477, #27626, #19978 ),
 .UNSPECIFIED., .F., .F.,
 ( 4, 2, 2, 2, 4 ),
 ( 0.000000000000000000, 0.0001954311564186865221, 0.0003908623128373730441, 0.0005862934692560595662, 0.0007817246256747460882 ),
 .UNSPECIFIED. ) ;
#4424=ORIENTED_EDGE ( 'NONE', *, *, #31815, .F. ) ;
#4425=VERTEX_POINT ( 'NONE', #40434 ) ;
#4426=CARTESIAN_POINT ( 'NONE',  ( 9.692307692307572609, -11.94971097300221174, 32.03036669348237098 ) ) ;
#4427=EDGE_LOOP ( 'NONE', ( #53587, #66227 ) ) ;
#4428=CARTESIAN_POINT ( 'NONE',  ( 16.82689985270161870, -5.765609946408405406, 34.70566812827424741 ) ) ;
#4429=CARTESIAN_POINT ( 'NONE',  ( -0.2115930521604186265, -4.932303261841488151, 34.32971442181322885 ) ) ;
#4431=EDGE_CURVE ( 'NONE', #59397, #30893, #54491, .T. ) ;
#4433=AXIS2_PLACEMENT_3D ( 'NONE', #2064, #84060, #29548 ) ;
#4434=DIRECTION ( 'NONE',  ( 0.000000000000000000, 0.000000000000000000, -1.000000000000000000 ) ) ;
#4435=CARTESIAN_POINT ( 'NONE',  ( 4.376625695114563008, -2.847695495035524882, 31.58253572463339509 ) ) ;
#4436=FACE_BOUND ( 'NONE', #41964, .T. ) ;
#4437=B_SPLINE_CURVE_WITH_KNOTS ( 'NONE', 3,
 ( #45803, #65181, #72382, #73285, #58415, #66530, #59766, #87261, #25541, #52994 ),
 .UNSPECIFIED., .F., .F.,
 ( 4, 2, 2, 2, 4 ),
 ( 0.000000000000000000, 0.0001954311564186868202, 0.0003908623128373736404, 0.0005862934692560604335, 0.0007817246256747472808 ),
 .UNSPECIFIED. ) ;
#4438=CARTESIAN_POINT ( 'NONE',  ( -0.7115151924808161832, -4.236021600441998380, 33.53823185664189310 ) ) ;
#4439=CARTESIAN_POINT ( 'NONE',  ( 11.53846153846141753, -8.613356846316285953, 34.62446782046622218 ) ) ;
#4440=DIRECTION ( 'NONE',  ( 0.000000000000000000, 0.7660444431189822323, -0.6427876096865344779 ) ) ;
#4441=CARTESIAN_POINT ( 'NONE',  ( 16.94677510719138169, -9.504002272028873932, 34.60269587691767867 ) ) ;
#4442=CARTESIAN_POINT ( 'NONE',  ( 6.792928953345223064, -11.04286588640298561, 33.62463336215343901 ) ) ;
#4443=CARTESIAN_POINT ( 'NONE',  ( 5.076923076923075762, -13.53365097954675988, 30.81389545987213552 ) ) ;
#4444=CARTESIAN_POINT ( 'NONE',  ( 1.607628228708780638, -2.308499170217967134, 30.53291367094873721 ) ) ;
#4445=EDGE_LOOP ( 'NONE', ( #50104, #31752 ) ) ;
#4446=CARTESIAN_POINT ( 'NONE',  ( -15.90384615384471800, -7.500000000000155431, 34.75000000000007105 ) ) ;
#4447=CYLINDRICAL_SURFACE ( 'NONE', #11997, 0.2499999999999995559 ) ;
#4448=ORIENTED_EDGE ( 'NONE', *, *, #36636, .F. ) ;
#4449=EDGE_LOOP ( 'NONE', ( #5427, #34764, #48947, #61517 ) ) ;
#4450=CARTESIAN_POINT ( 'NONE',  ( 16.15384615384615330, -2.708943851104267164, 35.45975837776705220 ) ) ;
#4451=CARTESIAN_POINT ( 'NONE',  ( 0.4615384615383382183, -8.656820664282941280, 34.87096338111179961 ) ) ;
#4452=CARTESIAN_POINT ( 'NONE',  ( 16.21991450484859953, -2.538708090699994813, 30.37095296980875503 ) ) ;
#4453=CARTESIAN_POINT ( 'NONE',  ( 2.530471976670374268, -2.353885683473778023, 30.79025554430704759 ) ) ;
#4454=DIRECTION ( 'NONE',  ( -0.000000000000000000, -0.3420201433256694346, -0.9396926207859080948 ) ) ;
#4455=ORIENTED_EDGE ( 'NONE', *, *, #14588, .F. ) ;
#4457=EDGE_CURVE ( 'NONE', #28781, #69896, #74933, .T. ) ;
#4459=CARTESIAN_POINT ( 'NONE',  ( 18.22301284409340028, -2.523321265292116866, 31.42251411153756990 ) ) ;
#4460=B_SPLINE_CURVE_WITH_KNOTS ( 'NONE', 3,
 ( #75589, #76037, #7590, #41376, #55322, #391, #35051, #63851, #22859, #15236 ),
 .UNSPECIFIED., .F., .F.,
 ( 4, 2, 2, 2, 4 ),
 ( 0.000000000000000000, 0.0001954339857564065528, 0.0003908679715128131056, 0.0005863019572692196313, 0.0007817359430256262112 ),
 .UNSPECIFIED. ) ;
#4461=CARTESIAN_POINT ( 'NONE',  ( 11.53846153846141576, -3.083524468854526912, 32.58852847137268327 ) ) ;
#4462=DIRECTION ( 'NONE',  ( -0.000000000000000000, -0.6427876096865404731, -0.7660444431189770143 ) ) ;
#4463=B_SPLINE_CURVE_WITH_KNOTS ( 'NONE', 3,
 ( #8683, #35709, #55081, #22620, #48319, #43346, #22189, #69042, #1474, #36158 ),
 .UNSPECIFIED., .F., .F.,
 ( 4, 2, 2, 2, 4 ),
 ( 0.000000000000000000, 0.0001954339857564082062, 0.0003908679715128164124, 0.0005863019572692246186, 0.0007817359430256328248 ),
 .UNSPECIFIED. ) ;
#4464=CARTESIAN_POINT ( 'NONE',  ( 7.846153846153725020, -6.026961402154118019, 34.52809138561165270 ) ) ;
#4465=VECTOR ( 'NONE', #62632, 1000.000000000000000 ) ;
#4466=CARTESIAN_POINT ( 'NONE',  ( -1.384615384615383471, -13.04860791097971706, 34.73218667398347037 ) ) ;
#4467=CARTESIAN_POINT ( 'NONE',  ( -15.16551409125639260, -11.06231777344671130, 33.60647404775212976 ) ) ;
#4468=B_SPLINE_CURVE_WITH_KNOTS ( 'NONE', 3,
 ( #1131, #21403, #84448, #34473, #21846, #8339, #14649, #63269, #7453, #42132 ),
 .UNSPECIFIED., .F., .F.,
 ( 4, 2, 2, 2, 4 ),
 ( 0.0007817246256747453293, 0.0009771112852218885505, 0.001172497944769031663, 0.001367884604316174993, 0.001563271263863318106 ),
 .UNSPECIFIED. ) ;
#4470=EDGE_LOOP ( 'NONE', ( #55949, #42737, #52267, #78416 ) ) ;
#4471=B_SPLINE_CURVE_WITH_KNOTS ( 'NONE', 3,
 ( #14900, #22529, #28859, #75695, #35609, #56318, #20755, #69831, #49561, #77037 ),
 .UNSPECIFIED., .F., .F.,
 ( 4, 2, 2, 2, 4 ),
 ( 0.0007817359430256318490, 0.0009771253907249984917, 0.001172514838424365026, 0.001367904286123731560, 0.001563293733823098311 ),
 .UNSPECIFIED. ) ;
#4472=VECTOR ( 'NONE', #37440, 1000.000000000000227 ) ;
#4473=VECTOR ( 'NONE', #74483, 1000.000000000000000 ) ;
#4474=ORIENTED_EDGE ( 'NONE', *, *, #28725, .T. ) ;
#4475=EDGE_CURVE ( 'NONE', #85765, #3642, #49820, .T. ) ;
#4477=CYLINDRICAL_SURFACE ( 'NONE', #29701, 0.2500000000000008882 ) ;
#4478=CARTESIAN_POINT ( 'NONE',  ( 4.403846153846153300, -2.499999999999998668, 29.75000000000000355 ) ) ;
#4479=EDGE_CURVE ( 'NONE', #80242, #45697, #48490, .T. ) ;
#4480=CARTESIAN_POINT ( 'NONE',  ( 3.903869409797563250, -10.82459398097509684, 33.81372124010185587 ) ) ;
#4481=CARTESIAN_POINT ( 'NONE',  ( 2.557692307692372768, -7.434744429011176159, 34.75000000000000711 ) ) ;
#4483=AXIS2_PLACEMENT_3D ( 'NONE', #46990, #40258, #13658 ) ;
#4484=CARTESIAN_POINT ( 'NONE',  ( 13.38461538461538680, -1.629998284177014645, 34.34916445242399163 ) ) ;
#4485=CARTESIAN_POINT ( 'NONE',  ( -13.38461538461538325, -12.10708131394839349, 31.69288490824020244 ) ) ;
#4486=CARTESIAN_POINT ( 'NONE',  ( -8.899378738962466784, -12.70455904226513866, 30.44083106164009322 ) ) ;
#4487=CARTESIAN_POINT ( 'NONE',  ( 12.21156171748987163, -11.47974371597207899, 33.17467449705390692 ) ) ;
#4489=CARTESIAN_POINT ( 'NONE',  ( 14.17754509825408604, -12.27039167877662251, 31.24851455888617835 ) ) ;
#4490=CYLINDRICAL_SURFACE ( 'NONE', #81182, 0.2500000000000012212 ) ;
#4491=CARTESIAN_POINT ( 'NONE',  ( 8.069166690247241647, -8.282913670948747864, 34.94150082978203642 ) ) ;
#4492=CARTESIAN_POINT ( 'NONE',  ( -5.869209559033049750, -4.684288915650984819, 34.18129842949671371 ) ) ;
#4493=CARTESIAN_POINT ( 'NONE',  ( 9.627037691751372250, -5.094484230520674117, 34.41647553114621161 ) ) ;
#4494=CARTESIAN_POINT ( 'NONE',  ( -15.45369544828537656, -8.239355502252617924, 34.69524867566427417 ) ) ;
#4496=CARTESIAN_POINT ( 'NONE',  ( -16.40382289789473802, -9.234221910056350069, 34.70572697212741531 ) ) ;
#4497=CARTESIAN_POINT ( 'NONE',  ( 1.318531973659506029, -5.557115091759785130, 34.35708131394839171 ) ) ;
#4498=CARTESIAN_POINT ( 'NONE',  ( -4.376773112752999850, -5.582147617184174848, 34.63737895849758530 ) ) ;
#4500=CARTESIAN_POINT ( 'NONE',  ( 17.07692307692307665, -6.386643153685126251, 34.62446782046654192 ) ) ;
#4501=DIRECTION ( 'NONE',  ( 0.000000000000000000, 1.000000000000000000, 0.000000000000000000 ) ) ;
#4502=CARTESIAN_POINT ( 'NONE',  ( 10.86538461538603606, -7.500000000000154543, 35.00000000000007105 ) ) ;
#4503=ORIENTED_EDGE ( 'NONE', *, *, #19598, .F. ) ;
#4505=CARTESIAN_POINT ( 'NONE',  ( -1.515306851282943734, -9.804603061927743113, 34.18744698557895845 ) ) ;
#4506=ORIENTED_EDGE ( 'NONE', *, *, #64092, .F. ) ;
#4507=B_SPLINE_CURVE_WITH_KNOTS ( 'NONE', 3,
 ( #69380, #83791, #22077, #42801, #55853, #83343, #33814, #76578, #54521, #82014 ),
 .UNSPECIFIED., .F., .F.,
 ( 4, 2, 2, 2, 4 ),
 ( 0.0007817359430256253438, 0.0009771253907249898181, 0.001172514838424354401, 0.001367904286123718983, 0.001563293733823083566 ),
 .UNSPECIFIED. ) ;
#4508=CARTESIAN_POINT ( 'NONE',  ( -17.77722045873158763, -3.755027918224366879, 33.06320215134716278 ) ) ;
#4509=ORIENTED_EDGE ( 'NONE', *, *, #16269, .T. ) ;
#4510=AXIS2_PLACEMENT_3D ( 'NONE', #432, #6736, #14838 ) ;
#4511=B_SPLINE_CURVE_WITH_KNOTS ( 'NONE', 3,
 ( #50003, #77918, #15347, #23844, #31053, #37366, #43689, #9465, #64835, #78802 ),
 .UNSPECIFIED., .F., .F.,
 ( 4, 2, 2, 2, 4 ),
 ( 0.0007817246256747511840, 0.0009771112852218952725, 0.001172497944769039470, 0.001367884604316183667, 0.001563271263863327864 ),
 .UNSPECIFIED. ) ;
#4512=CYLINDRICAL_SURFACE ( 'NONE', #46369, 0.2499999999999998890 ) ;
#4513=LINE ( 'NONE', #87394, #83999 ) ;
#4514=CARTESIAN_POINT ( 'NONE',  ( -18.00000000000000000, -12.75000000000001066, 29.99999999999997868 ) ) ;
#4515=ORIENTED_EDGE ( 'NONE', *, *, #36042, .T. ) ;
#4516=CARTESIAN_POINT ( 'NONE',  ( -10.61538461538473399, -12.46129190930018460, 30.37095296980731973 ) ) ;
#4518=ORIENTED_EDGE ( 'NONE', *, *, #29798, .F. ) ;
#4519=CARTESIAN_POINT ( 'NONE',  ( -5.933932666649922361, -2.292212530054420494, 30.41441678777542990 ) ) ;
#4520=EDGE_LOOP ( 'NONE', ( #13365, #70301 ) ) ;
#4521=CARTESIAN_POINT ( 'NONE',  ( 11.53846153846153832, -3.937682226553329556, 33.60647404775216529 ) ) ;
#4522=CARTESIAN_POINT ( 'NONE',  ( -16.15384615384627409, -9.528491918059723176, 34.59228464037033035 ) ) ;
#4523=CARTESIAN_POINT ( 'NONE',  ( -10.83886953994894320, -12.11044203135681840, 32.26167407432752299 ) ) ;
#4524=CARTESIAN_POINT ( 'NONE',  ( -3.165514091256391715, -5.094484230520773593, 34.41647553114626845 ) ) ;
#4525=CARTESIAN_POINT ( 'NONE',  ( 11.47319109250076075, -11.94971097300153140, 32.03036669348370680 ) ) ;
#4527=CARTESIAN_POINT ( 'NONE',  ( 13.38461538461538680, -13.75783147151868846, 33.36296068462461051 ) ) ;
#4529=VERTEX_POINT ( 'NONE', #27346 ) ;
#4530=ORIENTED_EDGE ( 'NONE', *, *, #87060, .T. ) ;
#4531=CARTESIAN_POINT ( 'NONE',  ( 3.361294669002873547, -12.70449254468099198, 30.44128974285582956 ) ) ;
#4532=VERTEX_POINT ( 'NONE', #83183 ) ;
#4534=ADVANCED_FACE ( 'NONE', ( #48939 ), #35878, .F. ) ;
#4535=CARTESIAN_POINT ( 'NONE',  ( 4.153846153846154188, -8.810774026931790459, 35.74407628777942847 ) ) ;
#4536=CARTESIAN_POINT ( 'NONE',  ( -10.86540785267757947, -9.271318131107980420, 34.42618302367067429 ) ) ;
#4537=EDGE_CURVE ( 'NONE', #54993, #2251, #2750, .T. ) ;
#4538=EDGE_LOOP ( 'NONE', ( #25366, #23644 ) ) ;
#4539=CARTESIAN_POINT ( 'NONE',  ( -17.07692307692307665, -8.318370150425687726, 35.83090037661290239 ) ) ;
#4542=CARTESIAN_POINT ( 'NONE',  ( -10.68065506134539078, -3.300289026998414865, 32.46337939537583139 ) ) ;
#4544=CARTESIAN_POINT ( 'NONE',  ( -12.71153846153846168, -7.500000000000001776, 35.00000000000000000 ) ) ;
#4545=EDGE_CURVE ( 'NONE', #83475, #66483, #49905, .T. ) ;
#4546=LINE ( 'NONE', #59487, #5762 ) ;
#4548=FACE_BOUND ( 'NONE', #49176, .T. ) ;
#4549=DIRECTION ( 'NONE',  ( -1.000000000000000000, 0.000000000000000000, 0.000000000000000000 ) ) ;
#4550=CARTESIAN_POINT ( 'NONE',  ( 12.59206416330202671, -6.001044277235009439, 34.52024696741798948 ) ) ;
#4552=CARTESIAN_POINT ( 'NONE',  ( 13.63456079399342791, -4.932303261841489928, 34.32971442181322885 ) ) ;
#4554=LINE ( 'NONE', #24818, #45205 ) ;
#4555=CARTESIAN_POINT ( 'NONE',  ( -1.514762594053604250, -2.619462340734462380, 30.83744416345203021 ) ) ;
#4557=CARTESIAN_POINT ( 'NONE',  ( 8.769230769230768274, -1.466349020453238561, 30.81389545987213907 ) ) ;
#4558=B_SPLINE_CURVE_WITH_KNOTS ( 'NONE', 3,
 ( #59667, #54232, #25445, #52901, #32639, #45709, #79946, #26332, #53798, #18247 ),
 .UNSPECIFIED., .F., .F.,
 ( 4, 2, 2, 2, 4 ),
 ( 0.0007817246256747447872, 0.0009771112852218874663, 0.001172497944769030362, 0.001367884604316173258, 0.001563271263863315937 ),
 .UNSPECIFIED. ) ;
#4559=ORIENTED_EDGE ( 'NONE', *, *, #44696, .T. ) ;
#4560=B_SPLINE_CURVE_WITH_KNOTS ( 'NONE', 3,
 ( #53511, #25158, #40469, #26055, #73350, #58936, #81008, #88225, #25606, #40026 ),
 .UNSPECIFIED., .F., .F.,
 ( 4, 2, 2, 2, 4 ),
 ( 0.0007817246256747453293, 0.0009771112852218889842, 0.001172497944769032531, 0.001367884604316176294, 0.001563271263863319840 ),
 .UNSPECIFIED. ) ;
#4562=CARTESIAN_POINT ( 'NONE',  ( 5.999999999999878320, -12.16647553114689728, 32.15551576947799362 ) ) ;
#4563=CYLINDRICAL_SURFACE ( 'NONE', #50593, 0.2499999999999986955 ) ;
#4564=CARTESIAN_POINT ( 'NONE',  ( 16.37662582282421653, -11.60474049983370648, 33.02348890104160262 ) ) ;
#4565=CARTESIAN_POINT ( 'NONE',  ( -4.153846153846273204, -4.481592998941358097, 33.73612834414048933 ) ) ;
#4567=CARTESIAN_POINT ( 'NONE',  ( -15.36146069743679199, -3.530157926970578952, 32.79014554554150607 ) ) ;
#4569=ADVANCED_FACE ( 'NONE', ( #28679 ), #7961, .F. ) ;
#4570=CARTESIAN_POINT ( 'NONE',  ( 16.85343813319912698, -5.912607949931405038, 34.49155766932282319 ) ) ;
#4571=CARTESIAN_POINT ( 'NONE',  ( -11.78843826940389583, -9.943427161483782584, 34.11278801902876978 ) ) ;
#4572=CARTESIAN_POINT ( 'NONE',  ( 2.557746727605760384, -12.65882529074907126, 30.72640787790839312 ) ) ;
#4573=EDGE_CURVE ( 'NONE', #31319, #26024, #65127, .T. ) ;
#4574=CARTESIAN_POINT ( 'NONE',  ( 4.946312717298547490, -7.722926236386453702, 34.74524107206102030 ) ) ;
#4575=VECTOR ( 'NONE', #84387, 1000.000000000000000 ) ;
#4577=ORIENTED_EDGE ( 'NONE', *, *, #61961, .T. ) ;
#4579=VERTEX_POINT ( 'NONE', #36753 ) ;
#4580=EDGE_CURVE ( 'NONE', #48470, #58457, #30440, .T. ) ;
#4581=CARTESIAN_POINT ( 'NONE',  ( 17.93424319748568507, -7.249945686854186278, 34.74374336980224598 ) ) ;
#4582=CARTESIAN_POINT ( 'NONE',  ( -7.780085495151405794, -4.786620604624114428, 33.94971097300155805 ) ) ;
#4583=EDGE_CURVE ( 'NONE', #36979, #84371, #55411, .T. ) ;
#4584=VERTEX_POINT ( 'NONE', #70544 ) ;
#4585=CARTESIAN_POINT ( 'NONE',  ( 8.769230769230768274, -2.721908614388771852, 31.22303859784724978 ) ) ;
#4586=CARTESIAN_POINT ( 'NONE',  ( 6.065255139512839122, -11.67786785259547777, 32.92929555188713664 ) ) ;
#4587=CARTESIAN_POINT ( 'NONE',  ( 0.4615384615384611200, -12.10708131394839349, 31.69288490824020244 ) ) ;
#4588=CARTESIAN_POINT ( 'NONE',  ( 14.08486561521330493, -7.369208160676172348, 34.74850200257122879 ) ) ;
#4589=CARTESIAN_POINT ( 'NONE',  ( -2.307692307692305711, -1.129524287112498415, 32.06866353760679544 ) ) ;
#4590=ORIENTED_EDGE ( 'NONE', *, *, #50857, .T. ) ;
#4591=CARTESIAN_POINT ( 'NONE',  ( -15.23076923076935252, -12.16647553114689728, 32.15551576947799362 ) ) ;
#4592=EDGE_LOOP ( 'NONE', ( #10183, #18232, #36716, #50559 ) ) ;
#4593=DIRECTION ( 'NONE',  ( 0.000000000000000000, 0.8660254037844377084, -0.5000000000000015543 ) ) ;
#4594=LINE ( 'NONE', #78915, #51129 ) ;
#4595=CARTESIAN_POINT ( 'NONE',  ( -7.846153846153967493, -3.643525952248795718, 33.31231777344771672 ) ) ;
#4596=CARTESIAN_POINT ( 'NONE',  ( -4.087777802843713282, -12.37446782046654192, 30.86335684631486842 ) ) ;
#4597=CARTESIAN_POINT ( 'NONE',  ( 13.25446741488368829, -4.299443229763728169, 33.91186481527756058 ) ) ;
#4598=CARTESIAN_POINT ( 'NONE',  ( 18.00000000000000000, -2.538708090699994813, 30.37095296980875503 ) ) ;
#4600=ORIENTED_EDGE ( 'NONE', *, *, #85508, .T. ) ;
#4601=B_SPLINE_CURVE_WITH_KNOTS ( 'NONE', 3,
 ( #4195, #79863, #31220, #58691, #18164, #80317, #72203, #25808, #18613, #11401 ),
 .UNSPECIFIED., .F., .F.,
 ( 4, 2, 2, 2, 4 ),
 ( 0.000000000000000000, 0.0001954339857564075828, 0.0003908679715128151656, 0.0005863019572692227755, 0.0007817359430256303312 ),
 .UNSPECIFIED. ) ;
#4602=CARTESIAN_POINT ( 'NONE',  ( 17.20744851515671670, -3.068774925481847937, 32.56582465632704526 ) ) ;
#4605=B_SPLINE_CURVE_WITH_KNOTS ( 'NONE', 3,
 ( #36420, #14364, #35080, #7618, #63434, #23329, #76959, #70198, #83279, #35532 ),
 .UNSPECIFIED., .F., .F.,
 ( 4, 2, 2, 2, 4 ),
 ( 0.000000000000000000, 0.0001954339857564081520, 0.0003908679715128163040, 0.0005863019572692244018, 0.0007817359430256326080 ),
 .UNSPECIFIED. ) ;
#4606=AXIS2_PLACEMENT_3D ( 'NONE', #9450, #30166, #63938 ) ;
#4608=ORIENTED_EDGE ( 'NONE', *, *, #75949, .T. ) ;
#4609=VERTEX_POINT ( 'NONE', #78624 ) ;
#4610=CARTESIAN_POINT ( 'NONE',  ( 8.769230769230768274, -8.564572088678739092, 35.78748833219616898 ) ) ;
#4611=CARTESIAN_POINT ( 'NONE',  ( 12.59232890250541281, -3.957578996910242619, 33.62503395064540257 ) ) ;
#4612=CARTESIAN_POINT ( 'NONE',  ( -4.153846153846273204, -9.442884908241554243, 34.35708131394783038 ) ) ;
#4614=CARTESIAN_POINT ( 'NONE',  ( 9.019230769230768274, -2.249999999999998668, 29.75000000000000355 ) ) ;
#4615=CARTESIAN_POINT ( 'NONE',  ( -8.992156986746916658, -11.76352882383564769, 32.36236540154569497 ) ) ;
#4616=CARTESIAN_POINT ( 'NONE',  ( -15.23076923076922995, -8.164416787775445883, 34.95778746994557906 ) ) ;
#4617=EDGE_LOOP ( 'NONE', ( #3754, #23959, #69110, #80274 ) ) ;
#4618=EDGE_CURVE ( 'NONE', #24436, #80960, #53352, .T. ) ;
#4619=CARTESIAN_POINT ( 'NONE',  ( -3.165514091256391271, -12.70778746994558439, 30.41441678777536595 ) ) ;
#4620=CARTESIAN_POINT ( 'NONE',  ( -2.084680956079456582, -9.886259254753566594, 34.14407573483972413 ) ) ;
#4621=CARTESIAN_POINT ( 'NONE',  ( 9.442284468086237226, -2.588893531581426988, 31.60682220781847818 ) ) ;
#4622=ORIENTED_EDGE ( 'NONE', *, *, #23777, .T. ) ;
#4623=CARTESIAN_POINT ( 'NONE',  ( 10.36540787133602670, -9.234221910056348293, 34.70572697212741531 ) ) ;
#4624=EDGE_LOOP ( 'NONE', ( #41223, #51347, #56237, #68123 ) ) ;
#4625=CARTESIAN_POINT ( 'NONE',  ( 1.318858582101077204, -7.249945686854186278, 34.74374336980224598 ) ) ;
#4626=CARTESIAN_POINT ( 'NONE',  ( 6.923076923076924238, -5.557115091759785130, 34.35708131394839171 ) ) ;
#4627=CARTESIAN_POINT ( 'NONE',  ( 3.100078627658922503, -2.845849958028613624, 32.17971566917920967 ) ) ;
#4628=EDGE_LOOP ( 'NONE', ( #32446, #19660, #65413, #36113 ) ) ;
#4630=CARTESIAN_POINT ( 'NONE',  ( 17.07692307692307665, -9.819645486525091727, 36.12317359536749706 ) ) ;
#4631=EDGE_CURVE ( 'NONE', #11542, #66197, #56532, .T. ) ;
#4632=DIRECTION ( 'NONE',  ( -0.000000000000000000, -0.6427876096865404731, -0.7660444431189771253 ) ) ;
#4634=AXIS2_PLACEMENT_3D ( 'NONE', #3572, #52653, #31042 ) ;
#4635=CARTESIAN_POINT ( 'NONE',  ( -7.846153846153967493, -5.094484230521993062, 34.41647553114689373 ) ) ;
#4636=CARTESIAN_POINT ( 'NONE',  ( -2.057637887778853703, -10.82426656108011720, 33.81400080652039009 ) ) ;
#4637=ORIENTED_EDGE ( 'NONE', *, *, #32326, .T. ) ;
#4638=B_SPLINE_CURVE_WITH_KNOTS ( 'NONE', 3,
 ( #29740, #33942, #27186, #84253, #54644, #1373, #1814, #57204, #29304, #49117 ),
 .UNSPECIFIED., .F., .F.,
 ( 4, 2, 2, 2, 4 ),
 ( 0.0007817246256747461966, 0.0009771112852218892010, 0.001172497944769032314, 0.001367884604316175427, 0.001563271263863318323 ),
 .UNSPECIFIED. ) ;
#4639=CYLINDRICAL_SURFACE ( 'NONE', #78865, 0.2500000000000008882 ) ;
#4640=ORIENTED_EDGE ( 'NONE', *, *, #9256, .T. ) ;
#4642=CARTESIAN_POINT ( 'NONE',  ( 7.596153846153846700, -2.499999999999998668, 29.75000000000000355 ) ) ;
#4643=B_SPLINE_CURVE_WITH_KNOTS ( 'NONE', 3,
 ( #67973, #401, #67084, #54897, #89147, #48126, #26544, #82821, #47692, #60315 ),
 .UNSPECIFIED., .F., .F.,
 ( 4, 2, 2, 2, 4 ),
 ( 0.000000000000000000, 0.0001954339857564081520, 0.0003908679715128163040, 0.0005863019572692244018, 0.0007817359430256326080 ),
 .UNSPECIFIED. ) ;
#4644=CARTESIAN_POINT ( 'NONE',  ( -9.469528151039279251, -12.24180327182772388, 31.33663988360758168 ) ) ;
#4645=CARTESIAN_POINT ( 'NONE',  ( -0.3962833220256236078, -2.657715359629131857, 31.77849191805844242 ) ) ;
#4646=EDGE_CURVE ( 'NONE', #69108, #65429, #73780, .T. ) ;
#4648=CARTESIAN_POINT ( 'NONE',  ( 9.019285080869083870, -3.627508038966690496, 32.91356715214248396 ) ) ;
#4649=LINE ( 'NONE', #53267, #36451 ) ;
#4650=CARTESIAN_POINT ( 'NONE',  ( 16.02315555073584008, -11.93127051446800380, 32.56575433478200665 ) ) ;
#4651=EDGE_CURVE ( 'NONE', #28571, #16403, #9297, .T. ) ;
#4653=ORIENTED_EDGE ( 'NONE', *, *, #14276, .F. ) ;
#4654=VERTEX_POINT ( 'NONE', #2956 ) ;
#4655=EDGE_LOOP ( 'NONE', ( #57573, #71400 ) ) ;
#4656=VERTEX_POINT ( 'NONE', #3851 ) ;
#4657=CARTESIAN_POINT ( 'NONE',  ( -4.403846153846151523, -2.499999999999998668, 29.75000000000000355 ) ) ;
#4658=EDGE_CURVE ( 'NONE', #13650, #84346, #86728, .T. ) ;
#4659=CARTESIAN_POINT ( 'NONE',  ( -2.084680956079457914, -3.105924265160262543, 32.13625925475356127 ) ) ;
#4660=LINE ( 'NONE', #52834, #76990 ) ;
#4661=CARTESIAN_POINT ( 'NONE',  ( -6.923076923077044142, -3.300289026999228881, 32.46337939537708905 ) ) ;
#4662=CARTESIAN_POINT ( 'NONE',  ( 7.622668921589514923, -12.69144148231606017, 30.53333754910549303 ) ) ;
#4664=CARTESIAN_POINT ( 'NONE',  ( 3.164685819813350509, -5.557115091759785130, 34.35708131394839171 ) ) ;
#4666=CARTESIAN_POINT ( 'NONE',  ( 17.07692307692295586, -6.835583212225970762, 34.95778746994575670 ) ) ;
#4667=CARTESIAN_POINT ( 'NONE',  ( 8.069166690247241647, -4.762714258010882773, 34.23016756924214832 ) ) ;
#4668=VERTEX_POINT ( 'NONE', #39440 ) ;
#4669=ORIENTED_EDGE ( 'NONE', *, *, #82770, .F. ) ;
#4671=B_SPLINE_CURVE_WITH_KNOTS ( 'NONE', 3,
 ( #45430, #3995, #52184, #59399, #25169, #78775, #72908, #11214, #39146, #86901 ),
 .UNSPECIFIED., .F., .F.,
 ( 4, 2, 2, 2, 4 ),
 ( 0.000000000000000000, 0.0001954311564186876876, 0.0003908623128373753751, 0.0005862934692560630356, 0.0007817246256747507503 ),
 .UNSPECIFIED. ) ;
#4672=VERTEX_POINT ( 'NONE', #46186 ) ;
#4673=CARTESIAN_POINT ( 'NONE',  ( 0.3308478584281537849, -11.93127051446800024, 32.56575433478200665 ) ) ;
#4675=DIRECTION ( 'NONE',  ( 0.000000000000000000, 1.000000000000000000, 0.000000000000000000 ) ) ;
#4676=CARTESIAN_POINT ( 'NONE',  ( -17.93474486048716088, -11.67786785259547777, 32.92929555188713664 ) ) ;
#4677=B_SPLINE_CURVE_WITH_KNOTS ( 'NONE', 3,
 ( #42764, #63458, #71099, #70224, #8528, #30557 ),
 .UNSPECIFIED., .F., .F.,
 ( 4, 2, 4 ),
 ( 0.0003909569690057827069, 0.0005862646681846092828, 0.0007815723673634358045 ),
 .UNSPECIFIED. ) ;
#4678=CYLINDRICAL_SURFACE ( 'NONE', #34147, 0.2500000000000012212 ) ;
#4679=CARTESIAN_POINT ( 'NONE',  ( -14.53117725141625627, -10.11188796281391511, 34.01382737946119050 ) ) ;
#4680=FACE_BOUND ( 'NONE', #38021, .T. ) ;
#4681=ORIENTED_EDGE ( 'NONE', *, *, #42842, .T. ) ;
#4682=EDGE_CURVE ( 'NONE', #20422, #68899, #44713, .T. ) ;
#4683=ORIENTED_EDGE ( 'NONE', *, *, #5175, .T. ) ;
#4684=CARTESIAN_POINT ( 'NONE',  ( -11.53846153846153655, -11.91647553114624181, 32.58852847137148245 ) ) ;
#4685=EDGE_LOOP ( 'NONE', ( #33890, #60463 ) ) ;
#4687=FACE_BOUND ( 'NONE', #32223, .T. ) ;
#4688=CARTESIAN_POINT ( 'NONE',  ( -9.692307692307814193, -2.379036618888197729, 30.90682066428292885 ) ) ;
#4689=FACE_OUTER_BOUND ( 'NONE', #67138, .T. ) ;
#4691=CARTESIAN_POINT ( 'NONE',  ( 12.46153846153846168, -9.780366693483667717, 34.19971097300155094 ) ) ;
#4692=CARTESIAN_POINT ( 'NONE',  ( -1.514763354347078872, -8.630895178749536711, 34.87696386517710323 ) ) ;
#4694=CARTESIAN_POINT ( 'NONE',  ( -5.299802593660662531, -7.630690623152302621, 34.99857592706774057 ) ) ;
#4696=FACE_OUTER_BOUND ( 'NONE', #16049, .T. ) ;
#4697=CARTESIAN_POINT ( 'NONE',  ( 3.230769230769231726, -12.10708131394839349, 31.69288490824020244 ) ) ;
#4698=CARTESIAN_POINT ( 'NONE',  ( -0.4615384615384611200, -2.517432740324522911, 35.29906147534542527 ) ) ;
#4699=VERTEX_POINT ( 'NONE', #5194 ) ;
#4700=CARTESIAN_POINT ( 'NONE',  ( -1.608100328339332030, -5.912607949931405038, 34.49155766932282319 ) ) ;
#4701=CARTESIAN_POINT ( 'NONE',  ( -9.692307692307691624, -11.35647404775217417, 33.31231777344666511 ) ) ;
#4702=CIRCLE ( 'NONE', #86692, 0.2500000000000002220 ) ;
#4703=ORIENTED_EDGE ( 'NONE', *, *, #12062, .T. ) ;
#4704=FACE_OUTER_BOUND ( 'NONE', #40079, .T. ) ;
#4705=CARTESIAN_POINT ( 'NONE',  ( -10.61538461538473399, -5.219633306517616589, 34.19971097300220464 ) ) ;
#4706=CARTESIAN_POINT ( 'NONE',  ( 21.00000000000000355, -7.500000000000000000, 29.75000000000000355 ) ) ;
#4708=CYLINDRICAL_SURFACE ( 'NONE', #51604, 0.2500000000000002220 ) ;
#4709=CARTESIAN_POINT ( 'NONE',  ( 17.29970274590113632, -4.989023458446561143, 34.36081565061822118 ) ) ;
#4710=DIRECTION ( 'NONE',  ( -0.000000000000000000, 0.6427876096865404731, -0.7660444431189770143 ) ) ;
#4711=CARTESIAN_POINT ( 'NONE',  ( -17.01166750564705055, -8.613356846314930593, 34.62446782046653482 ) ) ;
#4712=CARTESIAN_POINT ( 'NONE',  ( 10.74617505635156789, -9.084667340241226796, 34.75534355489798344 ) ) ;
#4713=LINE ( 'NONE', #41159, #37759 ) ;
#4714=EDGE_CURVE ( 'NONE', #50483, #65254, #57654, .T. ) ;
#4718=EDGE_LOOP ( 'NONE', ( #4907, #42635, #22946, #57955 ) ) ;
#4719=B_SPLINE_CURVE_WITH_KNOTS ( 'NONE', 3,
 ( #74987, #12831, #53815, #88517, #59687, #73663, #87184, #80415, #12392, #5190 ),
 .UNSPECIFIED., .F., .F.,
 ( 4, 2, 2, 2, 4 ),
 ( 0.0007817359430256322827, 0.0009771253907249989254, 0.001172514838424365676, 0.001367904286123732428, 0.001563293733823098962 ),
 .UNSPECIFIED. ) ;
#4721=EDGE_LOOP ( 'NONE', ( #4265, #20171, #85178, #4177 ) ) ;
#4722=DIRECTION ( 'NONE',  ( -0.000000000000000000, -0.9848077530122085754, -0.1736481776669273613 ) ) ;
#4723=ORIENTED_EDGE ( 'NONE', *, *, #24111, .F. ) ;
#4724=CARTESIAN_POINT ( 'NONE',  ( 11.53846153846141576, -2.657715359629662544, 31.77849191805970364 ) ) ;
#4726=CARTESIAN_POINT ( 'NONE',  ( 2.307692307692309264, -4.661471528628507777, 34.16647553114623292 ) ) ;
#4727=CARTESIAN_POINT ( 'NONE',  ( -15.45425415533356528, -12.47654668319379567, 31.42292124445336654 ) ) ;
#4728=CARTESIAN_POINT ( 'NONE',  ( -0.3307466537136744544, -5.582136614379148654, 34.36778462344220486 ) ) ;
#4729=CARTESIAN_POINT ( 'NONE',  ( -14.43838291080261449, -10.70098750199973203, 33.91152734681376302 ) ) ;
#4730=CARTESIAN_POINT ( 'NONE',  ( -10.61538461538461320, -3.322132147404559976, 32.92929555188717927 ) ) ;
#4731=CARTESIAN_POINT ( 'NONE',  ( -10.74607608205217346, -4.118384482072085184, 33.43331474514187107 ) ) ;
#4732=FACE_OUTER_BOUND ( 'NONE', #13536, .T. ) ;
#4734=B_SPLINE_CURVE_WITH_KNOTS ( 'NONE', 3,
 ( #42398, #76613, #60877, #19890, #27540, #6394, #62638, #75288, #14920, #33849 ),
 .UNSPECIFIED., .F., .F.,
 ( 4, 2, 2, 2, 4 ),
 ( 0.0007817246256747484735, 0.0009771112852218931041, 0.001172497944769037735, 0.001367884604316182365, 0.001563271263863326996 ),
 .UNSPECIFIED. ) ;
#4736=CARTESIAN_POINT ( 'NONE',  ( -7.173053667125516064, -4.818429247618089661, 34.26397095200675125 ) ) ;
#4737=DIRECTION ( 'NONE',  ( 0.000000000000000000, 0.000000000000000000, 1.000000000000000000 ) ) ;
#4738=CARTESIAN_POINT ( 'NONE',  ( 5.869852030268307708, -3.625366637846544560, 33.29286588640298561 ) ) ;
#4739=EDGE_CURVE ( 'NONE', #87539, #46286, #32931, .T. ) ;
#4741=EDGE_CURVE ( 'NONE', #22687, #56815, #74542, .T. ) ;
#4742=CIRCLE ( 'NONE', #88146, 0.2500000000000002220 ) ;
#4743=VERTEX_POINT ( 'NONE', #33564 ) ;
#4744=ORIENTED_EDGE ( 'NONE', *, *, #27598, .T. ) ;
#4745=CARTESIAN_POINT ( 'NONE',  ( 6.673100192134568509, -2.564618984488975961, 30.55390908950641915 ) ) ;
#4746=CARTESIAN_POINT ( 'NONE',  ( -14.05774678934416499, -8.433404298154334455, 34.66254593164985920 ) ) ;
#4747=LINE ( 'NONE', #53362, #31095 ) ;
#4748=CARTESIAN_POINT ( 'NONE',  ( 2.307692307692309264, -2.292212530054420494, 30.41441678777542634 ) ) ;
#4750=VECTOR ( 'NONE', #41521, 1000.000000000000114 ) ;
#4751=CARTESIAN_POINT ( 'NONE',  ( -16.28453762051371712, -8.999036380462719364, 34.52022231692819076 ) ) ;
#4752=ADVANCED_FACE ( 'NONE', ( #52035 ), #72752, .F. ) ;
#4753=EDGE_CURVE ( 'NONE', #70987, #76146, #41643, .T. ) ;
#4754=ORIENTED_EDGE ( 'NONE', *, *, #35336, .F. ) ;
#4755=LINE ( 'NONE', #19150, #73167 ) ;
#4756=ORIENTED_EDGE ( 'NONE', *, *, #14798, .F. ) ;
#4757=VERTEX_POINT ( 'NONE', #62340 ) ;
#4758=CARTESIAN_POINT ( 'NONE',  ( 7.716005876422148191, -11.04286588640298561, 33.62463336215343901 ) ) ;
#4759=CARTESIAN_POINT ( 'NONE',  ( -2.307692307692428724, -9.528491918059723176, 34.59228464037033035 ) ) ;
#4760=CARTESIAN_POINT ( 'NONE',  ( -4.153846153846152411, -12.62096338111211580, 30.90682066428153263 ) ) ;
#4761=CARTESIAN_POINT ( 'NONE',  ( -4.153846153846152411, -6.435427911321262684, 35.78748833219616898 ) ) ;
#4762=CARTESIAN_POINT ( 'NONE',  ( 13.31934538405906565, -5.941354392334499579, 34.76329471203369792 ) ) ;
#4765=CIRCLE ( 'NONE', #76641, 3.249999999999999556 ) ;
#4767=EDGE_LOOP ( 'NONE', ( #78259, #70125, #69660, #69925 ) ) ;
#4768=VERTEX_POINT ( 'NONE', #21364 ) ;
#4769=CARTESIAN_POINT ( 'NONE',  ( 17.07692307692307665, -2.499999999999998668, 29.75000000000001421 ) ) ;
#4770=CARTESIAN_POINT ( 'NONE',  ( -0.2387587925603949501, -10.23759521482555357, 34.22997729860117033 ) ) ;
#4771=B_SPLINE_CURVE_WITH_KNOTS ( 'NONE', 3,
 ( #42664, #2537, #57489, #56612, #70122, #43097, #84978, #8430, #50720, #22380 ),
 .UNSPECIFIED., .F., .F.,
 ( 4, 2, 2, 2, 4 ),
 ( 0.0007817359430256293554, 0.0009771253907249950223, 0.001172514838424360906, 0.001367904286123726790, 0.001563293733823092457 ),
 .UNSPECIFIED. ) ;
#4772=DIRECTION ( 'NONE',  ( 0.000000000000000000, 0.7660444431189822323, -0.6427876096865344779 ) ) ;
#4773=DIRECTION ( 'NONE',  ( 0.000000000000000000, 0.8660254037844377084, -0.5000000000000015543 ) ) ;
#4774=CARTESIAN_POINT ( 'NONE',  ( -4.283993363284373856, -8.587444163452046197, 34.63053765926554206 ) ) ;
#4775=CARTESIAN_POINT ( 'NONE',  ( 5.999999999999880096, -12.46129190930018460, 30.37095296980731973 ) ) ;
#4776=EDGE_LOOP ( 'NONE', ( #22085, #4916 ) ) ;
#4777=VERTEX_POINT ( 'NONE', #54254 ) ;
#4778=CARTESIAN_POINT ( 'NONE',  ( 0.5267940328144856688, -11.94971097300157403, 32.03036669348361443 ) ) ;
#4779=CARTESIAN_POINT ( 'NONE',  ( -5.999999999999998224, -3.050289026998446396, 32.03036669348365706 ) ) ;
#4780=EDGE_LOOP ( 'NONE', ( #63878, #80858, #78523, #73454 ) ) ;
#4781=CARTESIAN_POINT ( 'NONE',  ( -39.05038313613820122, -2.249999999999998668, 29.75000000000000355 ) ) ;
#4782=CARTESIAN_POINT ( 'NONE',  ( -9.758391103263571509, -11.69971097300155272, 32.46337939537587403 ) ) ;
#4784=VERTEX_POINT ( 'NONE', #28120 ) ;
#4785=DIRECTION ( 'NONE',  ( 1.000000000000000000, 0.000000000000000000, 0.000000000000000000 ) ) ;
#4786=ORIENTED_EDGE ( 'NONE', *, *, #34339, .T. ) ;
#4787=FACE_OUTER_BOUND ( 'NONE', #88658, .T. ) ;
#4788=CARTESIAN_POINT ( 'NONE',  ( -5.076923076923075762, -6.386643153685126251, 34.62446782046654192 ) ) ;
#4791=FACE_BOUND ( 'NONE', #4092, .T. ) ;
#4792=CARTESIAN_POINT ( 'NONE',  ( 11.53846153846153832, -12.29105614889573062, 35.45975837776705220 ) ) ;
#4793=CARTESIAN_POINT ( 'NONE',  ( 7.976944287120795174, -2.295524264805589354, 30.44142389570982488 ) ) ;
#4794=CIRCLE ( 'NONE', #86786, 0.2500000000000002220 ) ;
#4795=DIRECTION ( 'NONE',  ( -0.000000000000000000, 0.5000000000000011102, -0.8660254037844381525 ) ) ;
#4796=EDGE_LOOP ( 'NONE', ( #59463, #14742 ) ) ;
#4797=CARTESIAN_POINT ( 'NONE',  ( -11.53846153846166089, -8.656820664282941280, 34.87096338111179961 ) ) ;
#4798=EDGE_CURVE ( 'NONE', #59654, #76676, #651, .T. ) ;
#4799=CARTESIAN_POINT ( 'NONE',  ( 11.53846153846185274, -2.255955759149395501, 30.00000000000324363 ) ) ;
#4800=CARTESIAN_POINT ( 'NONE',  ( 16.15384615384603251, -5.941354392335915335, 34.76329471203413846 ) ) ;
#4801=VERTEX_POINT ( 'NONE', #35780 ) ;
#4802=EDGE_CURVE ( 'NONE', #12672, #87474, #1824, .T. ) ;
#4803=B_SPLINE_CURVE_WITH_KNOTS ( 'NONE', 3,
 ( #3378, #57880, #24538, #29974, #10146, #23650, #56991, #8820, #84484, #43485 ),
 .UNSPECIFIED., .F., .F.,
 ( 4, 2, 2, 2, 4 ),
 ( 0.0007817246256747440282, 0.0009771112852218863821, 0.001172497944769028844, 0.001367884604316171307, 0.001563271263863313769 ),
 .UNSPECIFIED. ) ;
#4804=LINE ( 'NONE', #18761, #54503 ) ;
#4805=CARTESIAN_POINT ( 'NONE',  ( -8.769230769230892619, -3.083524468854526912, 32.58852847137268327 ) ) ;
#4806=CARTESIAN_POINT ( 'NONE',  ( -16.21992853320628925, -11.91647553114624181, 32.58852847137148245 ) ) ;
#4807=CARTESIAN_POINT ( 'NONE',  ( 7.976679547917411739, -3.285477652293412820, 32.44071101563363158 ) ) ;
#4808=FACE_BOUND ( 'NONE', #13389, .T. ) ;
#4810=DIRECTION ( 'NONE',  ( -0.000000000000000000, 0.8660254037844397068, -0.4999999999999978906 ) ) ;
#4811=CARTESIAN_POINT ( 'NONE',  ( 4.153846153846032507, -2.892918686052165622, 31.69288490824153470 ) ) ;
#4812=CARTESIAN_POINT ( 'NONE',  ( 17.99999999999987566, -11.48612834414049644, 32.76840700105863391 ) ) ;
#4813=CARTESIAN_POINT ( 'NONE',  ( -4.087778820496076548, -10.67929555188718282, 33.92786785259544757 ) ) ;
#4815=CARTESIAN_POINT ( 'NONE',  ( 13.38461538461526423, -2.657715359629662544, 31.77849191805970364 ) ) ;
#4817=B_SPLINE_CURVE_WITH_KNOTS ( 'NONE', 3,
 ( #54102, #81596, #19883, #47349, #74845, #943, #77051, #23415, #35626, #69847 ),
 .UNSPECIFIED., .F., .F.,
 ( 4, 2, 2, 2, 4 ),
 ( 0.000000000000000000, 0.0001954311564186877960, 0.0003908623128373755920, 0.0005862934692560633609, 0.0007817246256747511840 ),
 .UNSPECIFIED. ) ;
#4818=DIRECTION ( 'NONE',  ( -0.000000000000000000, -0.7660444431189791237, -0.6427876096865379196 ) ) ;
#4819=ORIENTED_EDGE ( 'NONE', *, *, #6488, .F. ) ;
#4820=CARTESIAN_POINT ( 'NONE',  ( -4.153846153846273204, -11.94971097300221174, 32.03036669348237098 ) ) ;
#4821=CARTESIAN_POINT ( 'NONE',  ( 2.057669083470851756, -2.341070481393819236, 30.72580821765574299 ) ) ;
#4822=CARTESIAN_POINT ( 'NONE',  ( -1.134561072977068985, -10.66356715214248396, 33.62249196103329751 ) ) ;
#4823=DIRECTION ( 'NONE',  ( 0.000000000000000000, 0.4999999999999960032, -0.8660254037844410391 ) ) ;
#4824=CARTESIAN_POINT ( 'NONE',  ( -10.48485917715097315, -12.15418822224088835, 32.17964115625579069 ) ) ;
#4825=CARTESIAN_POINT ( 'NONE',  ( -12.59222906464877134, -6.369640206132551441, 34.87707690430378449 ) ) ;
#4827=CARTESIAN_POINT ( 'NONE',  ( 14.17754509825408960, -10.88202310037935661, 33.43294751532457099 ) ) ;
#4828=LINE ( 'NONE', #46253, #87807 ) ;
#4829=VECTOR ( 'NONE', #63096, 1000.000000000000227 ) ;
#4830=CARTESIAN_POINT ( 'NONE',  ( -4.946132635956128176, -11.93129842949671726, 32.56571108434900452 ) ) ;
#4831=CARTESIAN_POINT ( 'NONE',  ( 9.442284468086237226, -4.175268141568685643, 33.81360843649122216 ) ) ;
#4832=LINE ( 'NONE', #31406, #62664 ) ;
#4833=DIRECTION ( 'NONE',  ( -0.000000000000000000, 0.3420201433256694346, -0.9396926207859080948 ) ) ;
#4834=CARTESIAN_POINT ( 'NONE',  ( 14.17754509825408960, -6.001485441113819874, 34.52039167877662607 ) ) ;
#4835=CARTESIAN_POINT ( 'NONE',  ( -11.40793583669797506, -10.88167719472716399, 33.43325721877153711 ) ) ;
#4836=ORIENTED_EDGE ( 'NONE', *, *, #71660, .T. ) ;
#4837=CARTESIAN_POINT ( 'NONE',  ( 17.07692307692307665, -2.721908614388771852, 31.22303859784724978 ) ) ;
#4840=EDGE_CURVE ( 'NONE', #28639, #43192, #82192, .T. ) ;
#4841=LINE ( 'NONE', #60215, #74920 ) ;
#4842=CARTESIAN_POINT ( 'NONE',  ( 5.076923076922953193, -6.835583212225970762, 34.95778746994575670 ) ) ;
#4843=ORIENTED_EDGE ( 'NONE', *, *, #1547, .F. ) ;
#4844=CARTESIAN_POINT ( 'NONE',  ( 6.923076923076924238, -8.120952969808772792, 34.71129190930000163 ) ) ;
#4845=CARTESIAN_POINT ( 'NONE',  ( 5.999999999999880096, -11.48612834414049644, 32.76840700105863391 ) ) ;
#4846=CARTESIAN_POINT ( 'NONE',  ( 11.78846153846154010, -2.249999999999998668, 29.75000000000000355 ) ) ;
#4847=ORIENTED_EDGE ( 'NONE', *, *, #6096, .T. ) ;
#4848=CARTESIAN_POINT ( 'NONE',  ( 11.78851585009985570, -4.943051570960394159, 34.04725096376909477 ) ) ;
#4849=CARTESIAN_POINT ( 'NONE',  ( -3.230769230769351186, -3.835265460704628371, 33.15142922262033665 ) ) ;
#4850=DIRECTION ( 'NONE',  ( 0.000000000000000000, 0.8660254037844377084, 0.5000000000000015543 ) ) ;
#4851=B_SPLINE_CURVE_WITH_KNOTS ( 'NONE', 3,
 ( #3280, #64527, #23552, #35761, #83951, #51005 ),
 .UNSPECIFIED., .F., .F.,
 ( 4, 2, 4 ),
 ( 1.769077770938648657E-17, 0.0001954756301636913782, 0.0003909512603273650297 ),
 .UNSPECIFIED. ) ;
#4852=CARTESIAN_POINT ( 'NONE',  ( -16.37667425148103106, -7.369209533119136069, 34.99857337881830688 ) ) ;
#4854=ORIENTED_EDGE ( 'NONE', *, *, #36509, .F. ) ;
#4855=B_SPLINE_CURVE_WITH_KNOTS ( 'NONE', 3,
 ( #69659, #7965, #35428, #56146, #70100, #8409, #35882, #72757, #32231, #86301 ),
 .UNSPECIFIED., .F., .F.,
 ( 4, 2, 2, 2, 4 ),
 ( 0.000000000000000000, 0.0001954311564186870913, 0.0003908623128373741825, 0.0005862934692560613009, 0.0007817246256747483650 ),
 .UNSPECIFIED. ) ;
#4856=CYLINDRICAL_SURFACE ( 'NONE', #61980, 0.2499999999999986955 ) ;
#4857=B_SPLINE_CURVE_WITH_KNOTS ( 'NONE', 3,
 ( #64845, #31062, #44125, #58529, #3146, #10364, #9472, #65735, #63962, #71166 ),
 .UNSPECIFIED., .F., .F.,
 ( 4, 2, 2, 2, 4 ),
 ( 0.000000000000000000, 0.0001954339857564070678, 0.0003908679715128141356, 0.0005863019572692211492, 0.0007817359430256282712 ),
 .UNSPECIFIED. ) ;
#4858=B_SPLINE_CURVE_WITH_KNOTS ( 'NONE', 3,
 ( #73499, #86576, #38822, #32496, #10459, #44213, #66282, #25301, #37927, #4587 ),
 .UNSPECIFIED., .F., .F.,
 ( 4, 2, 2, 2, 4 ),
 ( 0.0007817359430256235007, 0.0009771253907249932875, 0.001172514838424355919, 0.001367904286123718983, 0.001563293733823081615 ),
 .UNSPECIFIED. ) ;
#4859=LINE ( 'NONE', #32329, #22149 ) ;
#4861=VECTOR ( 'NONE', #24583, 1000.000000000000000 ) ;
#4862=EDGE_CURVE ( 'NONE', #10877, #18726, #8205, .T. ) ;
#4863=EDGE_CURVE ( 'NONE', #63786, #29793, #64013, .T. ) ;
#4864=CARTESIAN_POINT ( 'NONE',  ( -15.23076923076922995, -6.343179335718451384, 34.87096338111211935 ) ) ;
#4865=VERTEX_POINT ( 'NONE', #34437 ) ;
#4867=VERTEX_POINT ( 'NONE', #61900 ) ;
#4868=LINE ( 'NONE', #67009, #23991 ) ;
#4869=FACE_OUTER_BOUND ( 'NONE', #47292, .T. ) ;
#4870=CARTESIAN_POINT ( 'NONE',  ( -9.692307692307691624, -5.180354513474913603, 36.12317359536750416 ) ) ;
#4871=EDGE_CURVE ( 'NONE', #64358, #47735, #18894, .T. ) ;
#4872=CARTESIAN_POINT ( 'NONE',  ( -18.12834546406995528, -7.274827144381421640, 34.99539338292708379 ) ) ;
#4875=ADVANCED_FACE ( 'NONE', ( #49720 ), #77637, .F. ) ;
#4876=ORIENTED_EDGE ( 'NONE', *, *, #85167, .T. ) ;
#4877=ORIENTED_EDGE ( 'NONE', *, *, #6370, .F. ) ;
#4878=CARTESIAN_POINT ( 'NONE',  ( 11.66925197942848946, -11.37503395064541678, 33.29242100308974273 ) ) ;
#4879=ORIENTED_EDGE ( 'NONE', *, *, #17863, .T. ) ;
#4880=DIRECTION ( 'NONE',  ( -0.000000000000000000, -0.9848077530122085754, -0.1736481776669273891 ) ) ;
#4881=EDGE_CURVE ( 'NONE', #64027, #72207, #3874, .T. ) ;
#4882=CARTESIAN_POINT ( 'NONE',  ( -3.480792454990687457, -4.931416488878823223, 34.32920672191015399 ) ) ;
#4883=B_SPLINE_CURVE_WITH_KNOTS ( 'NONE', 3,
 ( #44825, #44373, #2507, #79071, #25010, #72306, #79523, #38536, #52478, #79962 ),
 .UNSPECIFIED., .F., .F.,
 ( 4, 2, 2, 2, 4 ),
 ( 0.000000000000000000, 0.0001954339857564080978, 0.0003908679715128161956, 0.0005863019572692242934, 0.0007817359430256323911 ),
 .UNSPECIFIED. ) ;
#4884=CARTESIAN_POINT ( 'NONE',  ( 10.55011416942384095, -11.48612834413959582, 32.76840700105983473 ) ) ;
#4885=CARTESIAN_POINT ( 'NONE',  ( -1.134560964701931463, -12.65882529074907126, 30.72640787790839312 ) ) ;
#4887=B_SPLINE_CURVE_WITH_KNOTS ( 'NONE', 3,
 ( #38941, #23626, #24513, #79915, #45229, #71362, #66398, #2897, #59638, #65942 ),
 .UNSPECIFIED., .F., .F.,
 ( 4, 2, 2, 2, 4 ),
 ( 0.000000000000000000, 0.0001954339857564100222, 0.0003908679715128200445, 0.0005863019572692300396, 0.0007817359430256400890 ),
 .UNSPECIFIED. ) ;
#4888=ORIENTED_EDGE ( 'NONE', *, *, #15569, .T. ) ;
#4890=CARTESIAN_POINT ( 'NONE',  ( 14.30769230769231015, -10.67929555188718282, 33.92786785259544047 ) ) ;
#4892=ORIENTED_EDGE ( 'NONE', *, *, #701, .T. ) ;
#4893=CARTESIAN_POINT ( 'NONE',  ( 3.007843013253083786, -11.76352882383564769, 32.36236540154569497 ) ) ;
#4894=CARTESIAN_POINT ( 'NONE',  ( -13.38461538461538325, -6.386643153685126251, 34.62446782046654192 ) ) ;
#4895=CARTESIAN_POINT ( 'NONE',  ( 12.68431813051652846, -6.717445702608402236, 34.94155399931962336 ) ) ;
#4896=CARTESIAN_POINT ( 'NONE',  ( -1.384615384615383471, -8.120952969808772792, 34.71129190930000163 ) ) ;
#4897=CARTESIAN_POINT ( 'NONE',  ( -2.176900499867519212, -11.18335022499818621, 33.13157742990016885 ) ) ;
#4898=FACE_BOUND ( 'NONE', #84623, .T. ) ;
#4899=CARTESIAN_POINT ( 'NONE',  ( 18.00000000000000000, -11.91647553114624181, 32.58852847137148245 ) ) ;
#4900=CARTESIAN_POINT ( 'NONE',  ( 10.61538461538461675, -1.367168528481310208, 33.57946703557072254 ) ) ;
#4901=EDGE_CURVE ( 'NONE', #20256, #69595, #8752, .T. ) ;
#4902=CARTESIAN_POINT ( 'NONE',  ( -8.992156986746914882, -4.186968288167449259, 33.49512374952580274 ) ) ;
#4903=CARTESIAN_POINT ( 'NONE',  ( 9.561616225640133138, -3.062553014421049546, 32.05460306192773601 ) ) ;
#4904=CARTESIAN_POINT ( 'NONE',  ( 6.856994543716785628, -10.67929555188718460, 33.92786785259543336 ) ) ;
#4905=CARTESIAN_POINT ( 'NONE',  ( 0.2115152242454951537, -12.22074536777954989, 31.39888409691088356 ) ) ;
#4906=CARTESIAN_POINT ( 'NONE',  ( 7.846153846153725020, -11.48612834414049644, 32.76840700105863391 ) ) ;
#4907=ORIENTED_EDGE ( 'NONE', *, *, #2075, .T. ) ;
#4908=DIRECTION ( 'NONE',  ( -0.000000000000000000, -0.6427876096865404731, -0.7660444431189770143 ) ) ;
#4909=CARTESIAN_POINT ( 'NONE',  ( 12.46153846153846168, -3.322132147404559976, 32.92929555188717927 ) ) ;
#4910=ORIENTED_EDGE ( 'NONE', *, *, #42355, .F. ) ;
#4911=EDGE_LOOP ( 'NONE', ( #28871, #3047 ) ) ;
#4912=CARTESIAN_POINT ( 'NONE',  ( 8.769230769230645706, -11.67786785259630911, 32.92929555188603530 ) ) ;
#4913=CARTESIAN_POINT ( 'NONE',  ( -0.5267894516997033705, -2.506253911140460922, 30.00000000000013856 ) ) ;
#4914=DIRECTION ( 'NONE',  ( -0.000000000000000000, 0.5000000000000011102, -0.8660254037844380415 ) ) ;
#4915=CARTESIAN_POINT ( 'NONE',  ( 12.21156171748987163, -10.82459398097509329, 33.81372124010185587 ) ) ;
#4916=ORIENTED_EDGE ( 'NONE', *, *, #4362, .T. ) ;
#4917=CARTESIAN_POINT ( 'NONE',  ( 14.53047184896071542, -9.332535724633409302, 34.40230450496446934 ) ) ;
#4918=CARTESIAN_POINT ( 'NONE',  ( -4.376773112753001627, -9.172386477786396597, 34.72672124145550043 ) ) ;
#4919=AXIS2_PLACEMENT_3D ( 'NONE', #2320, #10872, #23048 ) ;
#4920=CARTESIAN_POINT ( 'NONE',  ( 18.06606835100244268, -3.513871655860379306, 32.76840700105978499 ) ) ;
#4921=CARTESIAN_POINT ( 'NONE',  ( 5.777073041093150785, -6.459968553980839800, 34.89616026154728701 ) ) ;
#4922=CARTESIAN_POINT ( 'NONE',  ( 9.692307692307695177, -1.367168528481310208, 33.57946703557072254 ) ) ;
#4923=CARTESIAN_POINT ( 'NONE',  ( -5.076923076923075762, -8.973038597847269315, 34.52809138561121927 ) ) ;
#4925=B_SPLINE_CURVE_WITH_KNOTS ( 'NONE', 3,
 ( #32040, #23932, #64919, #51843, #37907, #18086, #79339, #80233, #17184, #2766 ),
 .UNSPECIFIED., .F., .F.,
 ( 4, 2, 2, 2, 4 ),
 ( 0.000000000000000000, 0.0001954311564186860613, 0.0003908623128373721225, 0.0005862934692560581567, 0.0007817246256747442451 ),
 .UNSPECIFIED. ) ;
#4927=EDGE_LOOP ( 'NONE', ( #16053, #57932, #79017, #52065 ) ) ;
#4929=EDGE_LOOP ( 'NONE', ( #67408, #77553 ) ) ;
#4930=LINE ( 'NONE', #53991, #75177 ) ;
#4931=CARTESIAN_POINT ( 'NONE',  ( 12.39578165902414852, -7.249945686854186278, 34.74374336980224598 ) ) ;
#4933=CARTESIAN_POINT ( 'NONE',  ( 20.99999999999998934, -2.249999999999998668, 29.75000000000000355 ) ) ;
#4934=DIRECTION ( 'NONE',  ( -0.000000000000000000, 0.7660444431189791237, -0.6427876096865379196 ) ) ;
#4937=CARTESIAN_POINT ( 'NONE',  ( -12.46153846153846168, -6.386643153685126251, 34.62446782046654192 ) ) ;
#4938=EDGE_CURVE ( 'NONE', #39482, #83084, #36126, .T. ) ;
#4939=CARTESIAN_POINT ( 'NONE',  ( 17.01083966596719321, -12.10708131394839349, 31.69288490824020244 ) ) ;
#4940=CARTESIAN_POINT ( 'NONE',  ( 6.000000000000001776, -9.905515769479276145, 34.41647553114623292 ) ) ;
#4941=CARTESIAN_POINT ( 'NONE',  ( 4.153846153846154188, -13.78497067705608181, 32.30358669280327177 ) ) ;
#4942=CARTESIAN_POINT ( 'NONE',  ( 8.545745825506822158, -12.24155766932282496, 31.33739205006857986 ) ) ;
#4944=CARTESIAN_POINT ( 'NONE',  ( 3.903822916553188804, -12.43535235679832596, 30.55408501211184813 ) ) ;
#4945=CARTESIAN_POINT ( 'NONE',  ( 10.68064018666064285, -2.892918686051625166, 31.69288490824026638 ) ) ;
#4946=CARTESIAN_POINT ( 'NONE',  ( 8.519230769230768274, -7.500000000000001776, 35.04278698407183867 ) ) ;
#4947=ORIENTED_EDGE ( 'NONE', *, *, #68117, .F. ) ;
#4948=CARTESIAN_POINT ( 'NONE',  ( -1.384615384615383471, -2.538708090699994813, 30.37095296980875503 ) ) ;
#4949=DIRECTION ( 'NONE',  ( -0.000000000000000000, -0.3420201433256694901, -0.9396926207859082059 ) ) ;
#4950=DIRECTION ( 'NONE',  ( 0.000000000000000000, 0.3420201433256641055, -0.9396926207859100932 ) ) ;
#4952=CARTESIAN_POINT ( 'NONE',  ( 5.326868486301119532, -10.18230066228895758, 34.26354781536631577 ) ) ;
#4953=CARTESIAN_POINT ( 'NONE',  ( -0.4615384615384611200, -6.189225973068211317, 35.74407628777942847 ) ) ;
#4954=CARTESIAN_POINT ( 'NONE',  ( 11.53846153846153832, -2.249999999999998668, 29.75000000000001776 ) ) ;
#4955=VERTEX_POINT ( 'NONE', #23136 ) ;
#4957=EDGE_CURVE ( 'NONE', #27791, #58249, #60838, .T. ) ;
#4961=VECTOR ( 'NONE', #42035, 1000.000000000000227 ) ;
#4962=CARTESIAN_POINT ( 'NONE',  ( 18.22301135161285046, -9.086983370893049639, 34.49168942202179267 ) ) ;
#4963=ORIENTED_EDGE ( 'NONE', *, *, #16281, .T. ) ;
#4964=CARTESIAN_POINT ( 'NONE',  ( -7.596099426240392027, -6.523592122091590895, 34.90882529074906415 ) ) ;
#4965=CARTESIAN_POINT ( 'NONE',  ( 13.25392391794783187, -9.804603061927743113, 34.18744698557895845 ) ) ;
#4966=EDGE_CURVE ( 'NONE', #49902, #86068, #51022, .T. ) ;
#4967=CARTESIAN_POINT ( 'NONE',  ( -1.384615384615505151, -4.481592998941358097, 33.73612834414048933 ) ) ;
#4968=EDGE_LOOP ( 'NONE', ( #31152, #88726 ) ) ;
#4969=CARTESIAN_POINT ( 'NONE',  ( -10.39237326377176451, -12.39991518177334129, 30.74647679643404530 ) ) ;
#4970=EDGE_LOOP ( 'NONE', ( #62096, #9225, #36111, #48053 ) ) ;
#4971=ORIENTED_EDGE ( 'NONE', *, *, #63299, .F. ) ;
#4973=CARTESIAN_POINT ( 'NONE',  ( -0.4615384615385826339, -10.90142922262034020, 33.41473453929536674 ) ) ;
#4974=CARTESIAN_POINT ( 'NONE',  ( -10.54931626438217585, -6.386643153685127139, 34.62446782046654192 ) ) ;
#4975=CARTESIAN_POINT ( 'NONE',  ( 9.561616225640136690, -8.999036380462717588, 34.52022231692819076 ) ) ;
#4976=CARTESIAN_POINT ( 'NONE',  ( -3.100243792535585907, -5.070358843744209310, 34.40418822224088302 ) ) ;
#4978=DIRECTION ( 'NONE',  ( 0.000000000000000000, 0.000000000000000000, 1.000000000000000000 ) ) ;
#4979=B_SPLINE_CURVE_WITH_KNOTS ( 'NONE', 3,
 ( #75592, #829, #8925, #28294, #7146, #21989, #43147, #56657, #83253, #49462 ),
 .UNSPECIFIED., .F., .F.,
 ( 4, 2, 2, 2, 4 ),
 ( 0.000000000000000000, 0.0001954311564186879044, 0.0003908623128373758088, 0.0005862934692560636861, 0.0007817246256747516176 ),
 .UNSPECIFIED. ) ;
#4980=EDGE_CURVE ( 'NONE', #31594, #15866, #17937, .T. ) ;
#4982=ORIENTED_EDGE ( 'NONE', *, *, #6426, .F. ) ;
#4983=VERTEX_POINT ( 'NONE', #72649 ) ;
#4986=VERTEX_POINT ( 'NONE', #65885 ) ;
#4988=B_SPLINE_CURVE_WITH_KNOTS ( 'NONE', 3,
 ( #76045, #68848, #75598, #41383, #9803, #79153, #17454, #3921, #71494, #23311 ),
 .UNSPECIFIED., .F., .F.,
 ( 4, 2, 2, 2, 4 ),
 ( 0.0007817246256747491240, 0.0009771112852218931041, 0.001172497944769036867, 0.001367884604316180631, 0.001563271263863324611 ),
 .UNSPECIFIED. ) ;
#4989=VECTOR ( 'NONE', #41050, 1000.000000000000114 ) ;
#4990=CARTESIAN_POINT ( 'NONE',  ( -8.769230769230768274, -9.780366693483667717, 34.19971097300155094 ) ) ;
#4991=CARTESIAN_POINT ( 'NONE',  ( -10.86536134632696715, -9.148715823498378086, 34.47080413974185120 ) ) ;
#4992=ORIENTED_EDGE ( 'NONE', *, *, #58669, .T. ) ;
#4994=VERTEX_POINT ( 'NONE', #52817 ) ;
#4995=CARTESIAN_POINT ( 'NONE',  ( 16.15384615384615330, -13.37000171582298513, 34.34916445242398453 ) ) ;
#4996=ORIENTED_EDGE ( 'NONE', *, *, #28211, .F. ) ;
#4997=CARTESIAN_POINT ( 'NONE',  ( -18.06608237936013595, -9.058645607665454236, 34.76329471203372634 ) ) ;
#4998=CARTESIAN_POINT ( 'NONE',  ( -11.60454494941741999, -3.513871655860377086, 32.76840700105978499 ) ) ;
#4999=CARTESIAN_POINT ( 'NONE',  ( -11.28851612908349722, -12.07971442181322175, 32.31769673815850297 ) ) ;
#5000=FACE_BOUND ( 'NONE', #16448, .T. ) ;
#5001=CARTESIAN_POINT ( 'NONE',  ( 17.07692307692307665, -6.343179335718451384, 34.87096338111211935 ) ) ;
#5002=DIRECTION ( 'NONE',  ( 0.000000000000000000, 0.8660254037844377084, 0.5000000000000015543 ) ) ;
#5003=CARTESIAN_POINT ( 'NONE',  ( 13.60739505359345181, -4.989023458446560255, 34.36081565061822118 ) ) ;
#5004=FACE_OUTER_BOUND ( 'NONE', #51269, .T. ) ;
#5006=CARTESIAN_POINT ( 'NONE',  ( 2.307692307692309264, -1.790695186598648903, 34.54067556320373455 ) ) ;
#5007=ORIENTED_EDGE ( 'NONE', *, *, #83665, .F. ) ;
#5008=CARTESIAN_POINT ( 'NONE',  ( 2.307692307692309264, -12.48256725967547354, 35.29906147534542527 ) ) ;
#5009=ORIENTED_EDGE ( 'NONE', *, *, #64284, .T. ) ;
#5010=VERTEX_POINT ( 'NONE', #5538 ) ;
#5011=CARTESIAN_POINT ( 'NONE',  ( -6.923076923076922462, -3.937682226553329556, 33.60647404775216529 ) ) ;
#5012=CARTESIAN_POINT ( 'NONE',  ( -14.17690049986752143, -12.38066358083363738, 30.83685684665853444 ) ) ;
#5013=DIRECTION ( 'NONE',  ( -0.000000000000000000, -0.3420201433256694901, -0.9396926207859082059 ) ) ;
#5014=CARTESIAN_POINT ( 'NONE',  ( -14.55766905174089665, -12.01397095200674059, 32.43157075238190146 ) ) ;
#5017=ORIENTED_EDGE ( 'NONE', *, *, #40433, .T. ) ;
#5020=CARTESIAN_POINT ( 'NONE',  ( 10.36536137809165403, -3.202444869320336451, 32.30641848906366675 ) ) ;
#5021=CARTESIAN_POINT ( 'NONE',  ( -3.296851610129365451, -12.62096338111211580, 30.90682066428152197 ) ) ;
#5022=ORIENTED_EDGE ( 'NONE', *, *, #32219, .F. ) ;
#5024=VERTEX_POINT ( 'NONE', #24905 ) ;
#5026=CARTESIAN_POINT ( 'NONE',  ( 4.826946332874483936, -2.920706130388546651, 32.31842814019191223 ) ) ;
#5027=ORIENTED_EDGE ( 'NONE', *, *, #61538, .T. ) ;
#5028=CARTESIAN_POINT ( 'NONE',  ( 3.007842271862382066, -12.64616026154729411, 30.79003144601913533 ) ) ;
#5029=DIRECTION ( 'NONE',  ( 0.000000000000000000, 0.000000000000000000, 1.000000000000000000 ) ) ;
#5030=CARTESIAN_POINT ( 'NONE',  ( -7.911424292114622503, -11.94971097300153140, 32.03036669348370680 ) ) ;
#5031=LINE ( 'NONE', #5485, #21571 ) ;
#5032=CARTESIAN_POINT ( 'NONE',  ( -11.53846153846165912, -9.442884908241554243, 34.35708131394783038 ) ) ;
#5033=EDGE_LOOP ( 'NONE', ( #80228, #50565 ) ) ;
#5034=CARTESIAN_POINT ( 'NONE',  ( -15.23076923076922995, -2.292212530054420494, 30.41441678777542634 ) ) ;
#5035=VERTEX_POINT ( 'NONE', #53264 ) ;
#5037=CARTESIAN_POINT ( 'NONE',  ( 8.519230769230768274, -2.499999999999998668, 29.75000000000000355 ) ) ;
#5038=CARTESIAN_POINT ( 'NONE',  ( -11.78843828251013015, -10.82459398097509329, 33.81372124010185587 ) ) ;
#5039=LINE ( 'NONE', #10471, #48112 ) ;
#5040=CARTESIAN_POINT ( 'NONE',  ( -3.903900744468109529, -4.932303261841489039, 34.32971442181322885 ) ) ;
#5042=CARTESIAN_POINT ( 'NONE',  ( 5.076923076923075762, -8.564572088678739092, 35.78748833219616898 ) ) ;
#5044=ORIENTED_EDGE ( 'NONE', *, *, #6399, .F. ) ;
#5045=CARTESIAN_POINT ( 'NONE',  ( 11.66898724022509981, -2.882268652242222284, 31.66798894389554064 ) ) ;
#5046=LINE ( 'NONE', #19450, #64928 ) ;
#5047=CARTESIAN_POINT ( 'NONE',  ( -8.769230769230768274, -9.819645486525091727, 36.12317359536749706 ) ) ;
#5048=VECTOR ( 'NONE', #59966, 1000.000000000000227 ) ;
#5049=EDGE_CURVE ( 'NONE', #87441, #39364, #15710, .T. ) ;
#5050=B_SPLINE_CURVE_WITH_KNOTS ( 'NONE', 3,
 ( #73704, #60163, #81785, #20075, #68260, #87667, #53406, #19190, #46660, #74133 ),
 .UNSPECIFIED., .F., .F.,
 ( 4, 2, 2, 2, 4 ),
 ( 0.0007817359430256326080, 0.0009771253907250047801, 0.001172514838424369796, 0.001367904286123735030, 0.001563293733823100046 ),
 .UNSPECIFIED. ) ;
#5051=ORIENTED_EDGE ( 'NONE', *, *, #3404, .F. ) ;
#5052=EDGE_LOOP ( 'NONE', ( #56781, #1021, #42484, #31637 ) ) ;
#5053=CARTESIAN_POINT ( 'NONE',  ( -11.60373198442231590, -10.90142922261923886, 33.41473453929638993 ) ) ;
#5054=CYLINDRICAL_SURFACE ( 'NONE', #54110, 0.2500000000000002220 ) ;
#5056=FACE_OUTER_BOUND ( 'NONE', #64063, .T. ) ;
#5057=CARTESIAN_POINT ( 'NONE',  ( 10.61538461538449418, -5.094484230521993062, 34.41647553114689373 ) ) ;
#5059=CARTESIAN_POINT ( 'NONE',  ( -7.173053654019277303, -11.79746400365624659, 32.30657167506340954 ) ) ;
#5061=B_SPLINE_CURVE_WITH_KNOTS ( 'NONE', 3,
 ( #76614, #8159, #517, #55891, #83380, #83830, #28886, #7722, #5167, #46158 ),
 .UNSPECIFIED., .F., .F.,
 ( 4, 2, 2, 2, 4 ),
 ( 0.0007817246256747451124, 0.0009771112852218885505, 0.001172497944769032097, 0.001367884604316175427, 0.001563271263863318973 ),
 .UNSPECIFIED. ) ;
#5062=CYLINDRICAL_SURFACE ( 'NONE', #86565, 0.2500000000000009437 ) ;
#5063=EDGE_CURVE ( 'NONE', #33483, #66604, #75842, .T. ) ;
#5064=CARTESIAN_POINT ( 'NONE',  ( -2.176900499867519212, -9.804649428959608670, 34.18742332936588468 ) ) ;
#5065=LINE ( 'NONE', #60004, #57982 ) ;
#5066=ORIENTED_EDGE ( 'NONE', *, *, #12826, .F. ) ;
#5067=CARTESIAN_POINT ( 'NONE',  ( 12.59233026936324684, -3.530189275343204702, 32.79018710029569661 ) ) ;
#5069=CARTESIAN_POINT ( 'NONE',  ( -0.3307466537136773965, -2.729792928343270031, 31.24908615093345432 ) ) ;
#5070=CARTESIAN_POINT ( 'NONE',  ( -13.63461538461538147, -7.566082377512564960, 35.00000000000000711 ) ) ;
#5071=CYLINDRICAL_SURFACE ( 'NONE', #62838, 0.2500000000000012212 ) ;
#5072=ORIENTED_EDGE ( 'NONE', *, *, #52468, .T. ) ;
#5073=CARTESIAN_POINT ( 'NONE',  ( -13.25382494364843389, -4.684288915650983043, 34.18129842949671371 ) ) ;
#5074=CARTESIAN_POINT ( 'NONE',  ( -11.47320596718551045, -12.46129190930001052, 30.37095296980870174 ) ) ;
#5077=CARTESIAN_POINT ( 'NONE',  ( 11.78846153846154010, -2.249999999999998668, 29.75000000000000355 ) ) ;
#5078=CARTESIAN_POINT ( 'NONE',  ( -0.4615384615384611200, -13.87047571288749737, 32.06866353760679544 ) ) ;
#5079=ADVANCED_FACE ( 'NONE', ( #38882 ), #32117, .F. ) ;
#5080=B_SPLINE_CURVE_WITH_KNOTS ( 'NONE', 3,
 ( #74966, #53789, #41169, #74510, #40292, #6932, #25017, #45280, #11066, #44832 ),
 .UNSPECIFIED., .F., .F.,
 ( 4, 2, 2, 2, 4 ),
 ( 0.0007817246256747442451, 0.0009771112852218865989, 0.001172497944769029061, 0.001367884604316171523, 0.001563271263863313986 ),
 .UNSPECIFIED. ) ;
#5081=ORIENTED_EDGE ( 'NONE', *, *, #82787, .F. ) ;
#5083=ADVANCED_FACE ( 'NONE', ( #11398 ), #59580, .F. ) ;
#5084=VERTEX_POINT ( 'NONE', #66788 ) ;
#5085=CARTESIAN_POINT ( 'NONE',  ( 5.326977496836529546, -11.47946981652013498, 33.17500667209846910 ) ) ;
#5086=B_SPLINE_CURVE_WITH_KNOTS ( 'NONE', 3,
 ( #30918, #2559, #58386, #17422, #2126, #43125, #30050, #85881, #50302, #70592 ),
 .UNSPECIFIED., .F., .F.,
 ( 4, 2, 2, 2, 4 ),
 ( 0.0007817246256747434861, 0.0009771112852218859484, 0.001172497944769028411, 0.001367884604316171090, 0.001563271263863313552 ),
 .UNSPECIFIED. ) ;
#5088=CARTESIAN_POINT ( 'NONE',  ( -3.480769230769229061, -7.500000000000001776, 34.75000000000000000 ) ) ;
#5089=EDGE_CURVE ( 'NONE', #10170, #67262, #80155, .T. ) ;
#5090=CARTESIAN_POINT ( 'NONE',  ( 11.53846153846153832, -4.786620604624113540, 33.94971097300155094 ) ) ;
#5092=CARTESIAN_POINT ( 'NONE',  ( -14.30769230769230660, -12.10708131394839349, 31.69288490824020244 ) ) ;
#5093=CARTESIAN_POINT ( 'NONE',  ( 3.230769230769231726, -13.04860791097971706, 34.73218667398347037 ) ) ;
#5094=DIRECTION ( 'NONE',  ( 0.000000000000000000, 0.000000000000000000, -1.000000000000000000 ) ) ;
#5095=ORIENTED_EDGE ( 'NONE', *, *, #63450, .T. ) ;
#5096=ORIENTED_EDGE ( 'NONE', *, *, #14503, .F. ) ;
#5097=EDGE_LOOP ( 'NONE', ( #57875, #7750 ) ) ;
#5098=EDGE_LOOP ( 'NONE', ( #10810, #53051, #45393, #64566 ) ) ;
#5099=AXIS2_PLACEMENT_3D ( 'NONE', #24175, #65159, #36810 ) ;
#5100=CARTESIAN_POINT ( 'NONE',  ( -5.207613680033385428, -3.957541250942359756, 33.62499894934981626 ) ) ;
#5102=CARTESIAN_POINT ( 'NONE',  ( -2.557692307692304823, -7.566083408709834757, 34.74999999999999289 ) ) ;
#5103=CARTESIAN_POINT ( 'NONE',  ( 6.250054311638317373, -12.17597550085003633, 31.52189283813461884 ) ) ;
#5104=CARTESIAN_POINT ( 'NONE',  ( 11.31497659473759043, -2.599994579823202923, 30.74605699353653776 ) ) ;
#5105=B_SPLINE_CURVE_WITH_KNOTS ( 'NONE', 3,
 ( #40801, #13757, #69151, #28613, #68263, #27713, #41240, #7456, #61495, #21849 ),
 .UNSPECIFIED., .F., .F.,
 ( 4, 2, 2, 2, 4 ),
 ( 0.000000000000000000, 0.0001954311564186871184, 0.0003908623128373742367, 0.0005862934692560614093, 0.0007817246256747484735 ),
 .UNSPECIFIED. ) ;
#5106=DIRECTION ( 'NONE',  ( -0.000000000000000000, 0.9396926207859092051, -0.3420201433256662704 ) ) ;
#5107=CARTESIAN_POINT ( 'NONE',  ( -4.854143535654664277, -4.387253974876676565, 33.66317474335728832 ) ) ;
#5108=CARTESIAN_POINT ( 'NONE',  ( 10.61538461538461675, -13.88283147151868846, 33.14645433367849847 ) ) ;
#5109=ORIENTED_EDGE ( 'NONE', *, *, #21698, .F. ) ;
#5111=ORIENTED_EDGE ( 'NONE', *, *, #65230, .T. ) ;
#5112=ORIENTED_EDGE ( 'NONE', *, *, #11291, .F. ) ;
#5113=CARTESIAN_POINT ( 'NONE',  ( 5.076923076923075762, -6.681629849574314051, 35.83090037661290239 ) ) ;
#5114=EDGE_LOOP ( 'NONE', ( #51373, #19888, #35046, #71300 ) ) ;
#5115=CARTESIAN_POINT ( 'NONE',  ( -16.15384615384615330, -6.386643153685126251, 34.62446782046654192 ) ) ;
#5116=CARTESIAN_POINT ( 'NONE',  ( 17.07692307692307665, -11.33034616979429110, 35.88435417666054406 ) ) ;
#5117=EDGE_CURVE ( 'NONE', #52597, #25490, #61948, .T. ) ;
#5118=CARTESIAN_POINT ( 'NONE',  ( -0.2115930521604179326, -2.341251567377309772, 30.72681386836322659 ) ) ;
#5119=CARTESIAN_POINT ( 'NONE',  ( 4.219914504848593317, -2.538708090699994813, 30.37095296980875503 ) ) ;
#5120=FACE_BOUND ( 'NONE', #37417, .T. ) ;
#5121=EDGE_LOOP ( 'NONE', ( #8371, #25842 ) ) ;
#5122=ORIENTED_EDGE ( 'NONE', *, *, #80185, .F. ) ;
#5123=CARTESIAN_POINT ( 'NONE',  ( 4.946775107191380805, -2.373036134822904319, 30.88089517874952250 ) ) ;
#5125=FACE_BOUND ( 'NONE', #4342, .T. ) ;
#5126=LINE ( 'NONE', #38472, #13082 ) ;
#5127=LINE ( 'NONE', #73142, #82204 ) ;
#5129=AXIS2_PLACEMENT_3D ( 'NONE', #50549, #10909, #38379 ) ;
#5130=CARTESIAN_POINT ( 'NONE',  ( 10.61538461538461675, -11.69971097300155272, 32.46337939537588113 ) ) ;
#5131=CARTESIAN_POINT ( 'NONE',  ( -15.23076923076922995, -2.249999999999998668, 29.50000000000001421 ) ) ;
#5132=CARTESIAN_POINT ( 'NONE',  ( -18.24997674404858827, -4.075325502946086864, 33.72974371597207721 ) ) ;
#5133=VERTEX_POINT ( 'NONE', #4032 ) ;
#5135=CARTESIAN_POINT ( 'NONE',  ( -18.22348494372394967, -5.113361153441933205, 34.14387501736621999 ) ) ;
#5136=CARTESIAN_POINT ( 'NONE',  ( -9.442362173959550020, -2.587454068350147018, 30.68340429815432202 ) ) ;
#5137=ORIENTED_EDGE ( 'NONE', *, *, #13606, .F. ) ;
#5138=EDGE_CURVE ( 'NONE', #2097, #33427, #59718, .T. ) ;
#5140=CARTESIAN_POINT ( 'NONE',  ( -1.449885830576159274, -6.026961402152685388, 34.52809138561120506 ) ) ;
#5141=CARTESIAN_POINT ( 'NONE',  ( 12.46153846153846168, -1.367168528481310208, 33.57946703557072254 ) ) ;
#5142=ORIENTED_EDGE ( 'NONE', *, *, #78791, .F. ) ;
#5143=CARTESIAN_POINT ( 'NONE',  ( 0.3962680155776848734, -9.442884908240170461, 34.35708131394840592 ) ) ;
#5144=LINE ( 'NONE', #10116, #39705 ) ;
#5145=CARTESIAN_POINT ( 'NONE',  ( -7.976844449264153702, -12.35290016733513951, 31.75349464988449455 ) ) ;
#5146=CARTESIAN_POINT ( 'NONE',  ( -0.4615384615385826339, -9.442884908241554243, 34.35708131394783038 ) ) ;
#5147=CARTESIAN_POINT ( 'NONE',  ( -9.692307692307691624, -6.386643153685126251, 34.62446782046654192 ) ) ;
#5148=FACE_OUTER_BOUND ( 'NONE', #54609, .T. ) ;
#5149=CARTESIAN_POINT ( 'NONE',  ( 14.08482688548867223, -2.501496062324912284, 29.88072118266895671 ) ) ;
#5150=CARTESIAN_POINT ( 'NONE',  ( -15.36091644020745051, -12.45813303252208648, 30.39737893381572675 ) ) ;
#5151=DIRECTION ( 'NONE',  ( 1.000000000000000000, 0.000000000000000000, 0.000000000000000000 ) ) ;
#5156=ORIENTED_EDGE ( 'NONE', *, *, #26506, .T. ) ;
#5158=ORIENTED_EDGE ( 'NONE', *, *, #49477, .F. ) ;
#5159=CARTESIAN_POINT ( 'NONE',  ( -7.780898706641008467, -2.657715359629131857, 31.77849191805844242 ) ) ;
#5160=EDGE_LOOP ( 'NONE', ( #49037, #87439, #51459, #27698 ) ) ;
#5161=CARTESIAN_POINT ( 'NONE',  ( 3.296837581771670411, -9.780366693483667717, 34.19971097300155805 ) ) ;
#5163=CARTESIAN_POINT ( 'NONE',  ( -13.13456096470193124, -5.642605341092957971, 34.66089969410670335 ) ) ;
#5164=EDGE_CURVE ( 'NONE', #62928, #27137, #4857, .T. ) ;
#5165=CARTESIAN_POINT ( 'NONE',  ( -15.48079245499068612, -12.45566812827425451, 31.48439005359158926 ) ) ;
#5166=CARTESIAN_POINT ( 'NONE',  ( -9.942307692307691624, -7.500000000000001776, 35.04278698407183867 ) ) ;
#5167=CARTESIAN_POINT ( 'NONE',  ( 8.835298102580845025, -10.67929555188718282, 33.92786785259544757 ) ) ;
#5168=CARTESIAN_POINT ( 'NONE',  ( -8.703162418228330921, -4.786620604624113540, 33.94971097300155805 ) ) ;
#5169=DIRECTION ( 'NONE',  ( -0.000000000000000000, 0.8660254037844397068, -0.4999999999999978906 ) ) ;
#5170=CARTESIAN_POINT ( 'NONE',  ( -7.623374304885432551, -12.24180327182771855, 31.33663988360758168 ) ) ;
#5173=DIRECTION ( 'NONE',  ( -0.000000000000000000, 0.1736481776669307198, -0.9848077530122080203 ) ) ;
#5174=CARTESIAN_POINT ( 'NONE',  ( -13.31935981333935537, -6.879047030191282275, 34.71129190930002295 ) ) ;
#5175=EDGE_CURVE ( 'NONE', #46048, #75057, #45020, .T. ) ;
#5176=CARTESIAN_POINT ( 'NONE',  ( -2.557715544985271094, -4.335965774309649134, 33.62209801155881905 ) ) ;
#5177=EDGE_CURVE ( 'NONE', #79680, #87031, #5977, .T. ) ;
#5178=VERTEX_POINT ( 'NONE', #16231 ) ;
#5179=ORIENTED_EDGE ( 'NONE', *, *, #24235, .T. ) ;
#5180=CARTESIAN_POINT ( 'NONE',  ( 14.05771556364371655, -8.347322224742351082, 34.93158281831414769 ) ) ;
#5181=CARTESIAN_POINT ( 'NONE',  ( 6.000000000000001776, -4.945431358278436385, 36.03766855953609394 ) ) ;
#5182=CARTESIAN_POINT ( 'NONE',  ( 16.28463659481310444, -12.35292014791297710, 31.75344720912887198 ) ) ;
#5183=CARTESIAN_POINT ( 'NONE',  ( -16.15384615384627409, -12.46129190930018460, 30.37095296980731973 ) ) ;
#5186=CARTESIAN_POINT ( 'NONE',  ( 8.519207531937803779, -4.335965774309649134, 33.62209801155881905 ) ) ;
#5187=FACE_OUTER_BOUND ( 'NONE', #24799, .T. ) ;
#5188=ADVANCED_FACE ( 'NONE', ( #85579 ), #50878, .F. ) ;
#5189=EDGE_LOOP ( 'NONE', ( #37507, #59341 ) ) ;
#5190=CARTESIAN_POINT ( 'NONE',  ( -5.076923076923075762, -12.37446782046654192, 30.86335684631486131 ) ) ;
#5191=VERTEX_POINT ( 'NONE', #40995 ) ;
#5192=ORIENTED_EDGE ( 'NONE', *, *, #53688, .T. ) ;
#5193=CARTESIAN_POINT ( 'NONE',  ( -14.55769230769230660, -7.500000000000001776, 34.75000000000000000 ) ) ;
#5194=CARTESIAN_POINT ( 'NONE',  ( -7.846153846153965716, -10.90142922262034020, 33.41473453929536674 ) ) ;
#5195=CARTESIAN_POINT ( 'NONE',  ( -9.692307692307691624, -6.386643153685126251, 34.62446782046654192 ) ) ;
#5196=EDGE_CURVE ( 'NONE', #8026, #57991, #12349, .T. ) ;
#5197=DIRECTION ( 'NONE',  ( -0.000000000000000000, -0.000000000000000000, 1.000000000000000000 ) ) ;
#5198=CARTESIAN_POINT ( 'NONE',  ( -2.057746789344163219, -11.86320923018887719, 32.19269448109604781 ) ) ;
#5199=VECTOR ( 'NONE', #60118, 1000.000000000000000 ) ;
#5200=EDGE_LOOP ( 'NONE', ( #9204, #61459, #36948, #14172 ) ) ;
#5201=VERTEX_POINT ( 'NONE', #76549 ) ;
#5202=VERTEX_POINT ( 'NONE', #8 ) ;
#5204=CARTESIAN_POINT ( 'NONE',  ( 10.39245765647776842, -11.43668979543634734, 33.22377378376089752 ) ) ;
#5205=EDGE_CURVE ( 'NONE', #81424, #20877, #55827, .T. ) ;
#5206=CARTESIAN_POINT ( 'NONE',  ( 16.37662582282421653, -5.827830569534415694, 34.72679350104403539 ) ) ;
#5207=CARTESIAN_POINT ( 'NONE',  ( -8.519285359852727169, -10.18230066228895758, 34.26354781536631577 ) ) ;
#5208=EDGE_CURVE ( 'NONE', #41231, #30159, #28813, .T. ) ;
#5209=CARTESIAN_POINT ( 'NONE',  ( 17.77707378248385339, -4.887634598454295265, 34.01352882383564946 ) ) ;
#5210=DIRECTION ( 'NONE',  ( 0.000000000000000000, 0.9848077530122072432, 0.1736481776669354937 ) ) ;
#5211=ORIENTED_EDGE ( 'NONE', *, *, #73596, .T. ) ;
#5212=B_SPLINE_CURVE_WITH_KNOTS ( 'NONE', 3,
 ( #8296, #9610, #23566, #30330, #9188, #22244 ),
 .UNSPECIFIED., .F., .F.,
 ( 4, 2, 4 ),
 ( 0.000000000000000000, 0.0001954784845028914076, 0.0003909569690057828153 ),
 .UNSPECIFIED. ) ;
#5213=EDGE_LOOP ( 'NONE', ( #2736, #63189, #16064, #60573 ) ) ;
#5215=CARTESIAN_POINT ( 'NONE',  ( -11.53846153846153655, -13.20930481340135110, 34.54067556320372745 ) ) ;
#5216=VERTEX_POINT ( 'NONE', #27478 ) ;
#5217=CARTESIAN_POINT ( 'NONE',  ( 1.384615384615386802, -3.886160181151819604, 36.00935417666054406 ) ) ;
#5218=CARTESIAN_POINT ( 'NONE',  ( 12.71159288145191013, -8.346898887586323923, 34.93166121998716278 ) ) ;
#5220=AXIS2_PLACEMENT_3D ( 'NONE', #4373, #26427, #59760 ) ;
#5221=CARTESIAN_POINT ( 'NONE',  ( 13.13461538461538680, -7.500000000000001776, 35.04278698407183867 ) ) ;
#5222=ORIENTED_EDGE ( 'NONE', *, *, #18541, .T. ) ;
#5223=CARTESIAN_POINT ( 'NONE',  ( 23.00000000000000000, -2.249999999999999556, 27.25000000000000000 ) ) ;
#5224=VERTEX_POINT ( 'NONE', #29257 ) ;
#5225=EDGE_CURVE ( 'NONE', #15004, #25632, #67234, .T. ) ;
#5229=CARTESIAN_POINT ( 'NONE',  ( -7.173053654019278191, -3.627789207965226748, 32.91389620160131102 ) ) ;
#5230=CARTESIAN_POINT ( 'NONE',  ( 8.096099255531889582, -2.341251567377310217, 30.72681386836322659 ) ) ;
#5231=ADVANCED_FACE ( 'NONE', ( #28350 ), #15293, .F. ) ;
#5232=DIRECTION ( 'NONE',  ( 0.000000000000000000, 0.000000000000000000, 1.000000000000000000 ) ) ;
#5233=EDGE_LOOP ( 'NONE', ( #25318, #57800, #17857, #64875 ) ) ;
#5234=CARTESIAN_POINT ( 'NONE',  ( -11.40793610022789650, -8.630441415882550871, 34.87705825610312615 ) ) ;
#5235=CARTESIAN_POINT ( 'NONE',  ( 8.900022577055556994, -6.413143153341454017, 34.63066358083362672 ) ) ;
#5236=CARTESIAN_POINT ( 'NONE',  ( -14.17716660592874867, -2.882268652242222284, 31.66798894389554064 ) ) ;
#5237=VERTEX_POINT ( 'NONE', #42769 ) ;
#5238=ADVANCED_FACE ( 'NONE', ( #62144 ), #82434, .F. ) ;
#5239=CARTESIAN_POINT ( 'NONE',  ( -9.627052552794857831, -5.094484230520773593, 34.41647553114626845 ) ) ;
#5240=DIRECTION ( 'NONE',  ( 0.000000000000000000, 0.8660254037844377084, 0.5000000000000015543 ) ) ;
#5241=DIRECTION ( 'NONE',  ( -0.000000000000000000, 0.6427876096865404731, -0.7660444431189771253 ) ) ;
#5242=CARTESIAN_POINT ( 'NONE',  ( 4.153846153846030731, -8.656820664282941280, 34.87096338111179961 ) ) ;
#5243=DIRECTION ( 'NONE',  ( -0.000000000000000000, 0.5000000000000011102, -0.8660254037844381525 ) ) ;
#5244=FACE_BOUND ( 'NONE', #86644, .T. ) ;
#5247=DIRECTION ( 'NONE',  ( -0.000000000000000000, -0.8660254037844397068, -0.4999999999999978906 ) ) ;
#5248=CARTESIAN_POINT ( 'NONE',  ( -17.93393164899756087, -11.16473453929635440, 33.15142922261927083 ) ) ;
#5249=CARTESIAN_POINT ( 'NONE',  ( 14.30769230769231015, -1.466349020453238561, 30.81389545987213907 ) ) ;
#5250=B_SPLINE_CURVE_WITH_KNOTS ( 'NONE', 3,
 ( #81707, #20443, #69951, #1055, #83930, #48344, #55993, #14124, #29426, #55548 ),
 .UNSPECIFIED., .F., .F.,
 ( 4, 2, 2, 2, 4 ),
 ( 0.000000000000000000, 0.0001954339857564093175, 0.0003908679715128186350, 0.0005863019572692279796, 0.0007817359430256372700 ),
 .UNSPECIFIED. ) ;
#5251=DIRECTION ( 'NONE',  ( -0.000000000000000000, -0.8660254037844397068, -0.4999999999999978906 ) ) ;
#5253=ORIENTED_EDGE ( 'NONE', *, *, #61708, .F. ) ;
#5255=ORIENTED_EDGE ( 'NONE', *, *, #39907, .F. ) ;
#5256=DIRECTION ( 'NONE',  ( 1.000000000000000000, 0.000000000000000000, 0.000000000000000000 ) ) ;
#5257=VECTOR ( 'NONE', #18911, 1000.000000000000000 ) ;
#5258=EDGE_LOOP ( 'NONE', ( #63900, #27367 ) ) ;
#5259=CARTESIAN_POINT ( 'NONE',  ( 7.622668902429897919, -9.331801661448606566, 34.40259984581193464 ) ) ;
#5262=ORIENTED_EDGE ( 'NONE', *, *, #42796, .T. ) ;
#5263=CARTESIAN_POINT ( 'NONE',  ( 3.453780582382080855, -6.503523203565942268, 34.64991518177335195 ) ) ;
#5264=CARTESIAN_POINT ( 'NONE',  ( 6.000000000000001776, -3.322132147404559976, 32.92929555188717927 ) ) ;
#5266=EDGE_CURVE ( 'NONE', #54936, #19690, #64296, .T. ) ;
#5267=CARTESIAN_POINT ( 'NONE',  ( 4.153846153846032507, -10.90142922262034020, 33.41473453929536674 ) ) ;
#5268=CARTESIAN_POINT ( 'NONE',  ( -14.55766905174089665, -11.47974371597208076, 33.17467449705390692 ) ) ;
#5269=AXIS2_PLACEMENT_3D ( 'NONE', #43724, #49154, #42417 ) ;
#5270=DIRECTION ( 'NONE',  ( -0.000000000000000000, -0.8660254037844397068, -0.4999999999999978906 ) ) ;
#5272=CARTESIAN_POINT ( 'NONE',  ( 0.3313912521002431166, -11.47017969459903952, 32.78971311882034456 ) ) ;
#5273=CARTESIAN_POINT ( 'NONE',  ( 1.515140822849031066, -10.31582465632705237, 34.18122507451815295 ) ) ;
#5275=DIRECTION ( 'NONE',  ( 0.000000000000000000, 0.1736481776669267785, -0.9848077530122087975 ) ) ;
#5276=CARTESIAN_POINT ( 'NONE',  ( 3.230769230769231726, -11.11383981884818262, 36.00935417666054406 ) ) ;
#5277=ORIENTED_EDGE ( 'NONE', *, *, #44723, .F. ) ;
#5278=CARTESIAN_POINT ( 'NONE',  ( 6.000000000000001776, -12.29105614889573062, 35.45975837776705220 ) ) ;
#5279=LINE ( 'NONE', #52563, #73335 ) ;
#5281=CARTESIAN_POINT ( 'NONE',  ( 2.177545098254088707, -4.460286881179643004, 33.72017969459903242 ) ) ;
#5282=DIRECTION ( 'NONE',  ( 0.000000000000000000, 1.000000000000000000, 0.000000000000000000 ) ) ;
#5283=VERTEX_POINT ( 'NONE', #84207 ) ;
#5284=CARTESIAN_POINT ( 'NONE',  ( -2.307692307692305711, -6.435427911321262684, 35.78748833219616898 ) ) ;
#5285=CARTESIAN_POINT ( 'NONE',  ( -6.923076923077045919, -12.16647553114689728, 32.15551576947799362 ) ) ;
#5286=CARTESIAN_POINT ( 'NONE',  ( 11.47237915910140771, -2.833524468853757305, 32.15551576947924417 ) ) ;
#5287=ORIENTED_EDGE ( 'NONE', *, *, #60360, .F. ) ;
#5288=LINE ( 'NONE', #32755, #48480 ) ;
#5289=CARTESIAN_POINT ( 'NONE',  ( -8.769230769230768274, -2.833524468853757305, 32.15551576947925838 ) ) ;
#5290=B_SPLINE_CURVE_WITH_KNOTS ( 'NONE', 3,
 ( #56758, #35159, #76141, #77041, #62622, #29305, #47790, #84254, #68500, #41039 ),
 .UNSPECIFIED., .F., .F.,
 ( 4, 2, 2, 2, 4 ),
 ( 0.0007817359430256283796, 0.0009771253907249943717, 0.001172514838424360255, 0.001367904286123726356, 0.001563293733823092240 ),
 .UNSPECIFIED. ) ;
#5291=CYLINDRICAL_SURFACE ( 'NONE', #36316, 0.2499999999999995559 ) ;
#5292=CARTESIAN_POINT ( 'NONE',  ( -16.40384615384615330, -7.433932668274255917, 35.00000000000000711 ) ) ;
#5293=ORIENTED_EDGE ( 'NONE', *, *, #80713, .T. ) ;
#5296=EDGE_CURVE ( 'NONE', #36772, #54237, #51141, .T. ) ;
#5297=CARTESIAN_POINT ( 'NONE',  ( 1.134638640566794754, -2.920706130388546651, 32.31842814019191223 ) ) ;
#5299=VERTEX_POINT ( 'NONE', #41434 ) ;
#5300=AXIS2_PLACEMENT_3D ( 'NONE', #20580, #48046, #41307 ) ;
#5301=EDGE_CURVE ( 'NONE', #29766, #27440, #22075, .T. ) ;
#5303=DIRECTION ( 'NONE',  ( -0.000000000000000000, 0.6427876096865404731, -0.7660444431189771253 ) ) ;
#5304=CARTESIAN_POINT ( 'NONE',  ( -6.923076923077044142, -4.481592998941358097, 33.73612834414048933 ) ) ;
#5305=ADVANCED_FACE ( 'NONE', ( #11977 ), #32244, .F. ) ;
#5307=CARTESIAN_POINT ( 'NONE',  ( 9.692307692307695177, -12.78798330534103123, 29.99999999999997868 ) ) ;
#5308=EDGE_CURVE ( 'NONE', #12209, #19490, #62887, .T. ) ;
#5309=CARTESIAN_POINT ( 'NONE',  ( -17.77451305701315221, -7.371803252071508439, 34.99865873832523278 ) ) ;
#5310=VERTEX_POINT ( 'NONE', #18733 ) ;
#5311=ORIENTED_EDGE ( 'NONE', *, *, #4739, .T. ) ;
#5312=VERTEX_POINT ( 'NONE', #32674 ) ;
#5313=CARTESIAN_POINT ( 'NONE',  ( -7.846153846153844924, -4.786620604624113540, 33.94971097300155094 ) ) ;
#5315=CARTESIAN_POINT ( 'NONE',  ( -6.792286482109971324, -3.957578996910242619, 33.62503395064540257 ) ) ;
#5317=CYLINDRICAL_SURFACE ( 'NONE', #52279, 0.2500000000000009437 ) ;
#5318=AXIS2_PLACEMENT_3D ( 'NONE', #11306, #25715, #26156 ) ;
#5319=CARTESIAN_POINT ( 'NONE',  ( 5.750023255951409951, -4.075325502946086864, 33.72974371597207721 ) ) ;
#5320=CARTESIAN_POINT ( 'NONE',  ( 3.230769230769110045, -8.613356846316285953, 34.62446782046622218 ) ) ;
#5321=ORIENTED_EDGE ( 'NONE', *, *, #10065, .T. ) ;
#5322=ORIENTED_EDGE ( 'NONE', *, *, #38640, .F. ) ;
#5323=AXIS2_PLACEMENT_3D ( 'NONE', #16986, #44435, #10238 ) ;
#5324=VERTEX_POINT ( 'NONE', #79543 ) ;
#5325=CARTESIAN_POINT ( 'NONE',  ( 10.68145296638705410, -10.51840700105979565, 33.73612834413962247 ) ) ;
#5326=CARTESIAN_POINT ( 'NONE',  ( 8.992242120843616959, -2.554770724473668153, 30.48948780036025852 ) ) ;
#5327=ORIENTED_EDGE ( 'NONE', *, *, #62910, .T. ) ;
#5328=B_SPLINE_CURVE_WITH_KNOTS ( 'NONE', 3,
 ( #48654, #46885, #68487, #60845, #75685, #919, #54525, #82903, #69384, #74368 ),
 .UNSPECIFIED., .F., .F.,
 ( 4, 2, 2, 2, 4 ),
 ( 0.000000000000000000, 0.0001954311564186869015, 0.0003908623128373738030, 0.0005862934692560607588, 0.0007817246256747476061 ),
 .UNSPECIFIED. ) ;
#5329=CARTESIAN_POINT ( 'NONE',  ( 17.01165307636676260, -5.941354392334501355, 34.76329471203369792 ) ) ;
#5332=CARTESIAN_POINT ( 'NONE',  ( 16.28463796167094557, -8.147973898785416225, 34.70805048591653730 ) ) ;
#5333=CARTESIAN_POINT ( 'NONE',  ( -24.00000000000000000, -9.499999999999982236, 27.74999999999999645 ) ) ;
#5334=CARTESIAN_POINT ( 'NONE',  ( 8.835299120233207404, -5.557115091759786019, 34.35708131394839882 ) ) ;
#5335=FACE_BOUND ( 'NONE', #64145, .T. ) ;
#5336=EDGE_CURVE ( 'NONE', #88472, #5216, #57472, .T. ) ;
#5337=CARTESIAN_POINT ( 'NONE',  ( -0.5268089074992376997, -4.481592998940161721, 33.73612834413957984 ) ) ;
#5338=DIRECTION ( 'NONE',  ( -0.000000000000000000, -1.000000000000000000, 3.491481338843133355E-15 ) ) ;
#5339=CARTESIAN_POINT ( 'NONE',  ( 11.78851585009985214, -12.41262288849542017, 30.68299917996395010 ) ) ;
#5340=CARTESIAN_POINT ( 'NONE',  ( 9.468822748583747284, -3.236172620538810385, 32.36188796281390267 ) ) ;
#5341=CARTESIAN_POINT ( 'NONE',  ( -5.143006487878955646, -3.050289026998445951, 32.03036669348365706 ) ) ;
#5343=CARTESIAN_POINT ( 'NONE',  ( 0.3954550505825807361, -12.10708131394839349, 31.69288490824020244 ) ) ;
#5344=CARTESIAN_POINT ( 'NONE',  ( 12.71159288145191368, -2.920487667080175598, 32.31805714834170828 ) ) ;
#5345=ORIENTED_EDGE ( 'NONE', *, *, #64657, .T. ) ;
#5346=CARTESIAN_POINT ( 'NONE',  ( -17.14300545628320904, -5.471508081941601986, 34.59228464037088457 ) ) ;
#5347=DIRECTION ( 'NONE',  ( 0.000000000000000000, 0.9848077530122072432, -0.1736481776669354937 ) ) ;
#5349=ORIENTED_EDGE ( 'NONE', *, *, #61432, .F. ) ;
#5350=CARTESIAN_POINT ( 'NONE',  ( -17.20707028636130076, -11.47017969459903952, 32.78971311882035167 ) ) ;
#5351=EDGE_CURVE ( 'NONE', #68924, #33447, #33877, .T. ) ;
#5352=CARTESIAN_POINT ( 'NONE',  ( 15.90382291655318880, -3.711651800289232916, 33.01384336483936011 ) ) ;
#5354=VERTEX_POINT ( 'NONE', #25922 ) ;
#5358=EDGE_CURVE ( 'NONE', #5133, #31652, #73624, .T. ) ;
#5359=CARTESIAN_POINT ( 'NONE',  ( -14.37296230824862775, -4.320704448112771878, 33.92786785259540494 ) ) ;
#5360=CARTESIAN_POINT ( 'NONE',  ( -16.85354759115065448, -2.251407671071268712, 29.88021292934942963 ) ) ;
#5361=DIRECTION ( 'NONE',  ( 0.000000000000000000, 0.000000000000000000, 1.000000000000000000 ) ) ;
#5364=CARTESIAN_POINT ( 'NONE',  ( -10.48485917715097138, -11.66157788607254098, 32.95092075102925833 ) ) ;
#5365=AXIS2_PLACEMENT_3D ( 'NONE', #34227, #21152, #887 ) ;
#5368=ORIENTED_EDGE ( 'NONE', *, *, #25211, .F. ) ;
#5369=CARTESIAN_POINT ( 'NONE',  ( -9.757577692864012775, -2.657715359629089225, 31.77849191805832874 ) ) ;
#5371=FACE_OUTER_BOUND ( 'NONE', #47563, .T. ) ;
#5372=DIRECTION ( 'NONE',  ( -0.000000000000000000, 0.3420201433256694346, -0.9396926207859080948 ) ) ;
#5373=CARTESIAN_POINT ( 'NONE',  ( -0.2385755579769766321, -7.369474270740072441, 34.74850911626239736 ) ) ;
#5374=CARTESIAN_POINT ( 'NONE',  ( -3.296039676730006196, -6.026961402152685388, 34.52809138561120506 ) ) ;
#5377=CARTESIAN_POINT ( 'NONE',  ( -12.46153846153846168, -3.937682226553329556, 33.60647404775216529 ) ) ;
#5378=DIRECTION ( 'NONE',  ( 0.000000000000000000, 0.3420201433256641055, -0.9396926207859100932 ) ) ;
#5379=EDGE_CURVE ( 'NONE', #12293, #81839, #14586, .T. ) ;
#5380=CARTESIAN_POINT ( 'NONE',  ( -13.13461538461394973, -7.500000000000155431, 34.75000000000007105 ) ) ;
#5381=CARTESIAN_POINT ( 'NONE',  ( 12.46153846153846168, -11.35647404775217417, 33.31231777344666511 ) ) ;
#5382=CYLINDRICAL_SURFACE ( 'NONE', #79967, 0.2499999999999986955 ) ;
#5383=CYLINDRICAL_SURFACE ( 'NONE', #4147, 0.2500000000000008882 ) ;
#5386=CARTESIAN_POINT ( 'NONE',  ( 7.053867364043878929, -3.338503747796866872, 32.95102852606553512 ) ) ;
#5387=CARTESIAN_POINT ( 'NONE',  ( 3.930361210122206295, -12.44517049084099725, 30.48991314939691932 ) ) ;
#5388=CARTESIAN_POINT ( 'NONE',  ( -8.703975629717932705, -11.67786785259547777, 32.92929555188713664 ) ) ;
#5389=CARTESIAN_POINT ( 'NONE',  ( -7.623142494540996239, -12.39991518177334129, 30.74647679643404530 ) ) ;
#5390=ORIENTED_EDGE ( 'NONE', *, *, #72138, .F. ) ;
#5391=EDGE_CURVE ( 'NONE', #41035, #83912, #24127, .T. ) ;
#5392=CARTESIAN_POINT ( 'NONE',  ( -4.853911725310226188, -11.76359900205217457, 32.36225158514719880 ) ) ;
#5393=CARTESIAN_POINT ( 'NONE',  ( -17.14219307747939425, -6.835583212224499938, 34.95778746994557906 ) ) ;
#5394=CARTESIAN_POINT ( 'NONE',  ( 5.750023255951412615, -2.544273027872574922, 31.48422191005632342 ) ) ;
#5396=CARTESIAN_POINT ( 'NONE',  ( -17.99999999999969447, -2.506253911140613244, 30.00000000000320455 ) ) ;
#5397=CIRCLE ( 'NONE', #65743, 0.2500000000000002220 ) ;
#5398=DIRECTION ( 'NONE',  ( 0.000000000000000000, 0.9848077530122072432, -0.1736481776669354937 ) ) ;
#5399=CARTESIAN_POINT ( 'NONE',  ( -11.31568186948346977, -4.989023458446560255, 34.36081565061822118 ) ) ;
#5400=CYLINDRICAL_SURFACE ( 'NONE', #55474, 0.2499999999999994726 ) ;
#5401=ORIENTED_EDGE ( 'NONE', *, *, #72516, .T. ) ;
#5403=CARTESIAN_POINT ( 'NONE',  ( -14.43838291080261627, -5.496505350115501010, 34.60290016733514307 ) ) ;
#5404=B_SPLINE_CURVE_WITH_KNOTS ( 'NONE', 3,
 ( #60333, #66657, #40092, #4508, #54019, #32872, #20248, #19358, #46825, #66203 ),
 .UNSPECIFIED., .F., .F.,
 ( 4, 2, 2, 2, 4 ),
 ( 0.0007817359430256385711, 0.0009771253907250075990, 0.001172514838424376735, 0.001367904286123745872, 0.001563293733823115008 ),
 .UNSPECIFIED. ) ;
#5405=VERTEX_POINT ( 'NONE', #33124 ) ;
#5406=CARTESIAN_POINT ( 'NONE',  ( 0.2386122440223136243, -2.758268499246656180, 31.33685645148946719 ) ) ;
#5407=ORIENTED_EDGE ( 'NONE', *, *, #42903, .T. ) ;
#5408=CARTESIAN_POINT ( 'NONE',  ( 3.165499230212912352, -5.094484230520674117, 34.41647553114621161 ) ) ;
#5409=CARTESIAN_POINT ( 'NONE',  ( -9.442362173959551797, -2.824170634883621744, 31.52227843825338738 ) ) ;
#5410=VECTOR ( 'NONE', #25554, 1000.000000000000000 ) ;
#5411=CARTESIAN_POINT ( 'NONE',  ( -7.912237257109728361, -3.513871655860377086, 32.76840700105978499 ) ) ;
#5412=ORIENTED_EDGE ( 'NONE', *, *, #51691, .T. ) ;
#5414=B_SPLINE_CURVE_WITH_KNOTS ( 'NONE', 3,
 ( #55897, #28893, #58430, #522, #77067, #1402, #24209, #57999, #14474, #41506 ),
 .UNSPECIFIED., .F., .F.,
 ( 4, 2, 2, 2, 4 ),
 ( 0.000000000000000000, 0.0001954339857564073388, 0.0003908679715128146777, 0.0005863019572692220165, 0.0007817359430256293554 ),
 .UNSPECIFIED. ) ;
#5415=EDGE_LOOP ( 'NONE', ( #81856, #81074 ) ) ;
#5416=CARTESIAN_POINT ( 'NONE',  ( -16.08777882049607655, -2.292212530054420494, 30.41441678777542990 ) ) ;
#5417=CARTESIAN_POINT ( 'NONE',  ( -2.307692307692427391, -9.442884908241554243, 34.35708131394783038 ) ) ;
#5418=CARTESIAN_POINT ( 'NONE',  ( -9.469528151039281028, -10.11255958852956027, 34.01340905677048454 ) ) ;
#5420=CARTESIAN_POINT ( 'NONE',  ( 9.442284455014730682, -9.271318131107980420, 34.42618302367067429 ) ) ;
#5422=CARTESIAN_POINT ( 'NONE',  ( -12.46153846153846168, -4.098570777380720287, 33.41473453929634729 ) ) ;
#5424=CARTESIAN_POINT ( 'NONE',  ( -17.07692307692307665, -7.500000000000001776, 35.04278698407183867 ) ) ;
#5426=EDGE_LOOP ( 'NONE', ( #41313, #37789, #11722, #54633 ) ) ;
#5427=ORIENTED_EDGE ( 'NONE', *, *, #55798, .F. ) ;
#5428=VERTEX_POINT ( 'NONE', #13297 ) ;
#5429=CARTESIAN_POINT ( 'NONE',  ( -4.087778820496076548, -8.164416787775445883, 34.95778746994558617 ) ) ;
#5430=ORIENTED_EDGE ( 'NONE', *, *, #82470, .F. ) ;
#5431=EDGE_CURVE ( 'NONE', #22911, #17317, #28456, .T. ) ;
#5432=CIRCLE ( 'NONE', #45730, 2.000000000000001776 ) ;
#5433=B_SPLINE_CURVE_WITH_KNOTS ( 'NONE', 3,
 ( #33074, #38054, #87153, #59653, #26318, #17794, #45246, #18685, #79933, #87598 ),
 .UNSPECIFIED., .F., .F.,
 ( 4, 2, 2, 2, 4 ),
 ( 0.0007817246256747480398, 0.0009771112852218900684, 0.001172497944769032314, 0.001367884604316174559, 0.001563271263863316588 ),
 .UNSPECIFIED. ) ;
#5434=AXIS2_PLACEMENT_3D ( 'NONE', #17025, #44040, #84617 ) ;
#5435=CARTESIAN_POINT ( 'NONE',  ( 10.36538461538461675, -2.249999999999998668, 29.75000000000000355 ) ) ;
#5436=CARTESIAN_POINT ( 'NONE',  ( 12.52679403281448600, -3.300289026998473041, 32.46337939537591666 ) ) ;
#5437=ORIENTED_EDGE ( 'NONE', *, *, #61784, .F. ) ;
#5438=LINE ( 'NONE', #32901, #44408 ) ;
#5439=EDGE_CURVE ( 'NONE', #54976, #84095, #85398, .T. ) ;
#5440=ORIENTED_EDGE ( 'NONE', *, *, #72392, .F. ) ;
#5441=CARTESIAN_POINT ( 'NONE',  ( 0.4615384615384611200, -5.180354513474913603, 36.12317359536750416 ) ) ;
#5442=ORIENTED_EDGE ( 'NONE', *, *, #56930, .T. ) ;
#5443=CARTESIAN_POINT ( 'NONE',  ( -12.21153846153704237, -7.500000000000154543, 35.00000000000007105 ) ) ;
#5444=CARTESIAN_POINT ( 'NONE',  ( -2.307692307692305711, -11.33034616979429110, 35.88435417666054406 ) ) ;
#5445=CARTESIAN_POINT ( 'NONE',  ( -14.30769230769242917, -12.16647553114689728, 32.15551576947799362 ) ) ;
#5446=FACE_BOUND ( 'NONE', #34330, .T. ) ;
#5447=ADVANCED_FACE ( 'NONE', ( #41659 ), #33577, .F. ) ;
#5448=CARTESIAN_POINT ( 'NONE',  ( 2.057692307692309708, -7.500000000000001776, 34.75000000000000000 ) ) ;
#5449=CARTESIAN_POINT ( 'NONE',  ( 12.46153846153846168, -8.564572088678739092, 35.78748833219616898 ) ) ;
#5450=FACE_OUTER_BOUND ( 'NONE', #47522, .T. ) ;
#5451=CARTESIAN_POINT ( 'NONE',  ( 3.230769230769108269, -5.094484230521993062, 34.41647553114689373 ) ) ;
#5452=AXIS2_PLACEMENT_3D ( 'NONE', #47666, #75151, #34596 ) ;
#5453=DIRECTION ( 'NONE',  ( 0.000000000000000000, 0.9848077530122072432, 0.1736481776669354937 ) ) ;
#5454=CARTESIAN_POINT ( 'NONE',  ( 16.08857570788537572, -4.481592998940161721, 33.73612834413957984 ) ) ;
#5455=VERTEX_POINT ( 'NONE', #82659 ) ;
#5456=EDGE_CURVE ( 'NONE', #86258, #65223, #56371, .T. ) ;
#5457=DIRECTION ( 'NONE',  ( 0.000000000000000000, 0.3420201433256641055, -0.9396926207859100932 ) ) ;
#5458=VERTEX_POINT ( 'NONE', #47514 ) ;
#5459=B_SPLINE_CURVE_WITH_KNOTS ( 'NONE', 3,
 ( #19752, #40480, #12995, #804, #27836, #61613, #7124, #33710, #28272, #55299 ),
 .UNSPECIFIED., .F., .F.,
 ( 4, 2, 2, 2, 4 ),
 ( 0.0007817246256747504250, 0.0009771112852218954894, 0.001172497944769040554, 0.001367884604316185401, 0.001563271263863330466 ),
 .UNSPECIFIED. ) ;
#5460=ORIENTED_EDGE ( 'NONE', *, *, #83293, .T. ) ;
#5462=CYLINDRICAL_SURFACE ( 'NONE', #73408, 0.2499999999999994726 ) ;
#5463=DIRECTION ( 'NONE',  ( -0.000000000000000000, 0.1736481776669307198, -0.9848077530122080203 ) ) ;
#5464=B_SPLINE_CURVE_WITH_KNOTS ( 'NONE', 3,
 ( #81217, #53282, #47859, #5107, #25825, #74450, #19067, #33468, #60930, #12747 ),
 .UNSPECIFIED., .F., .F.,
 ( 4, 2, 2, 2, 4 ),
 ( 0.0007817359430256303312, 0.0009771253907249965402, 0.001172514838424362641, 0.001367904286123728958, 0.001563293733823095059 ),
 .UNSPECIFIED. ) ;
#5465=B_SPLINE_CURVE_WITH_KNOTS ( 'NONE', 3,
 ( #55769, #26541, #54000, #13456, #27422, #40940, #83258, #81492, #47689, #68847 ),
 .UNSPECIFIED., .F., .F.,
 ( 4, 2, 2, 2, 4 ),
 ( 0.0007817246256747434861, 0.0009771112852218861652, 0.001172497944769028844, 0.001367884604316171740, 0.001563271263863314419 ),
 .UNSPECIFIED. ) ;
#5466=FACE_OUTER_BOUND ( 'NONE', #6093, .T. ) ;
#5467=CARTESIAN_POINT ( 'NONE',  ( 3.453780582382079523, -10.61302985866383963, 33.66295027996417843 ) ) ;
#5469=DIRECTION ( 'NONE',  ( -0.000000000000000000, 0.9396926207859092051, -0.3420201433256662704 ) ) ;
#5470=ORIENTED_EDGE ( 'NONE', *, *, #48090, .F. ) ;
#5471=CARTESIAN_POINT ( 'NONE',  ( 2.177000841024750777, -8.999036380462717588, 34.52022231692819076 ) ) ;
#5472=EDGE_CURVE ( 'NONE', #69315, #83335, #44535, .T. ) ;
#5473=CARTESIAN_POINT ( 'NONE',  ( 15.16549923021291058, -4.320704448112771878, 33.92786785259540494 ) ) ;
#5475=CARTESIAN_POINT ( 'NONE',  ( -3.230769230769351186, -11.94971097300221174, 32.03036669348237098 ) ) ;
#5477=VERTEX_POINT ( 'NONE', #62789 ) ;
#5478=ORIENTED_EDGE ( 'NONE', *, *, #67436, .F. ) ;
#5479=FACE_OUTER_BOUND ( 'NONE', #37572, .T. ) ;
#5481=EDGE_LOOP ( 'NONE', ( #44732, #24211 ) ) ;
#5482=CARTESIAN_POINT ( 'NONE',  ( 9.692307692307695177, -2.833524468853757305, 32.15551576947925838 ) ) ;
#5483=CARTESIAN_POINT ( 'NONE',  ( 14.37375964104238335, -5.471508081941601098, 34.59228464037088457 ) ) ;
#5485=CARTESIAN_POINT ( 'NONE',  ( 17.07692307692307665, -1.951392089020283160, 34.73218667398347748 ) ) ;
#5487=CARTESIAN_POINT ( 'NONE',  ( -0.5268089074992364784, -11.48612834413959582, 32.76840700105983473 ) ) ;
#5488=VERTEX_POINT ( 'NONE', #55604 ) ;
#5489=CARTESIAN_POINT ( 'NONE',  ( -5.076923076923075762, -2.833524468853757305, 32.15551576947925838 ) ) ;
#5492=FACE_OUTER_BOUND ( 'NONE', #50613, .T. ) ;
#5493=CARTESIAN_POINT ( 'NONE',  ( 11.53846153846153832, -9.905515769479276145, 34.41647553114623292 ) ) ;
#5495=EDGE_CURVE ( 'NONE', #74234, #82533, #8041, .T. ) ;
#5497=CARTESIAN_POINT ( 'NONE',  ( 15.48071474911737333, -12.43552623307873972, 30.55307653245132826 ) ) ;
#5498=CARTESIAN_POINT ( 'NONE',  ( 2.530471976670372936, -2.612705202774697533, 31.66806509827799943 ) ) ;
#5499=CARTESIAN_POINT ( 'NONE',  ( 12.52679403281448245, -11.48612834413965977, 32.76840700105972815 ) ) ;
#5502=CARTESIAN_POINT ( 'NONE',  ( -6.923076923076922462, -10.67929555188718282, 33.92786785259544047 ) ) ;
#5503=CARTESIAN_POINT ( 'NONE',  ( 2.373759641042384239, -3.937682226553329556, 33.60647404775216529 ) ) ;
#5505=VECTOR ( 'NONE', #27782, 1000.000000000000114 ) ;
#5507=CARTESIAN_POINT ( 'NONE',  ( 2.438530638179069232, -7.277220318596959281, 34.99547417642776992 ) ) ;
#5508=CARTESIAN_POINT ( 'NONE',  ( -12.59168567097668401, -3.285722584762969856, 32.44110544564090759 ) ) ;
#5509=CARTESIAN_POINT ( 'NONE',  ( -0.5922290646487698984, -9.084618155246140248, 34.75535874321725771 ) ) ;
#5510=DIRECTION ( 'NONE',  ( -0.000000000000000000, 0.1736481776669307198, -0.9848077530122080203 ) ) ;
#5512=CARTESIAN_POINT ( 'NONE',  ( -14.43838291080261627, -2.845849958028613624, 32.17971566917920967 ) ) ;
#5513=ORIENTED_EDGE ( 'NONE', *, *, #26133, .F. ) ;
#5514=CARTESIAN_POINT ( 'NONE',  ( -3.007989561791164945, -12.69155399931963046, 30.53255429739157734 ) ) ;
#5515=CARTESIAN_POINT ( 'NONE',  ( -2.307692307692427391, -10.21337939537710326, 33.94971097300076224 ) ) ;
#5516=DIRECTION ( 'NONE',  ( -0.000000000000000000, 0.5000000000000011102, -0.8660254037844380415 ) ) ;
#5517=ORIENTED_EDGE ( 'NONE', *, *, #21257, .T. ) ;
#5518=CARTESIAN_POINT ( 'NONE',  ( 12.46153846153846168, -3.513871655860378418, 32.76840700105978499 ) ) ;
#5520=VECTOR ( 'NONE', #87585, 1000.000000000000227 ) ;
#5523=CARTESIAN_POINT ( 'NONE',  ( 5.750000000000002665, -7.500000000000001776, 34.75000000000000000 ) ) ;
#5524=ORIENTED_EDGE ( 'NONE', *, *, #8488, .T. ) ;
#5525=B_SPLINE_CURVE_WITH_KNOTS ( 'NONE', 3,
 ( #68102, #27103, #527, #21228, #74863, #6404, #75729, #13152, #28434, #48699 ),
 .UNSPECIFIED., .F., .F.,
 ( 4, 2, 2, 2, 4 ),
 ( 0.000000000000000000, 0.0001954339857564079352, 0.0003908679715128158703, 0.0005863019572692237513, 0.0007817359430256317406 ),
 .UNSPECIFIED. ) ;
#5526=CARTESIAN_POINT ( 'NONE',  ( -13.13466997523734214, -4.932303261841489928, 34.32971442181322885 ) ) ;
#5527=CARTESIAN_POINT ( 'NONE',  ( 5.776515056276053883, -10.11188796281391511, 34.01382737946119050 ) ) ;
#5528=B_SPLINE_CURVE_WITH_KNOTS ( 'NONE', 3,
 ( #62786, #8314, #49293, #15512, #15958, #55601, #42982, #70002, #9205, #48399 ),
 .UNSPECIFIED., .F., .F.,
 ( 4, 2, 2, 2, 4 ),
 ( 0.000000000000000000, 0.0001954339857564064444, 0.0003908679715128128888, 0.0005863019572692193060, 0.0007817359430256257775 ),
 .UNSPECIFIED. ) ;
#5529=DIRECTION ( 'NONE',  ( 0.000000000000000000, 0.4999999999999960032, -0.8660254037844410391 ) ) ;
#5530=CARTESIAN_POINT ( 'NONE',  ( 6.989144256427000990, -12.34228464037088813, 31.77849191805839268 ) ) ;
#5531=CARTESIAN_POINT ( 'NONE',  ( 16.15384615384615330, -4.098570777380720287, 33.41473453929634729 ) ) ;
#5533=ORIENTED_EDGE ( 'NONE', *, *, #41239, .T. ) ;
#5534=CARTESIAN_POINT ( 'NONE',  ( 4.153846153846154188, -1.790695186598648903, 34.54067556320373455 ) ) ;
#5535=VERTEX_POINT ( 'NONE', #14627 ) ;
#5536=CARTESIAN_POINT ( 'NONE',  ( 8.769230769230768274, -12.37446782046654192, 30.86335684631486131 ) ) ;
#5537=FACE_OUTER_BOUND ( 'NONE', #88731, .T. ) ;
#5538=CARTESIAN_POINT ( 'NONE',  ( 2.307692307692187583, -4.481592998941358097, 33.73612834414048933 ) ) ;
#5539=DIRECTION ( 'NONE',  ( -0.000000000000000000, -0.6427876096865404731, -0.7660444431189770143 ) ) ;
#5540=CARTESIAN_POINT ( 'NONE',  ( -14.24243673641627872, -12.27809138561124591, 31.22303859784720359 ) ) ;
#5541=CARTESIAN_POINT ( 'NONE',  ( -10.61538461538473399, -9.442884908241554243, 34.35708131394783038 ) ) ;
#5542=ORIENTED_EDGE ( 'NONE', *, *, #42232, .F. ) ;
#5543=ORIENTED_EDGE ( 'NONE', *, *, #50372, .T. ) ;
#5544=EDGE_LOOP ( 'NONE', ( #73729, #82208, #42243, #74709 ) ) ;
#5545=ORIENTED_EDGE ( 'NONE', *, *, #12553, .F. ) ;
#5546=CARTESIAN_POINT ( 'NONE',  ( 2.084207363968360038, -5.113361153441932316, 34.14387501736621999 ) ) ;
#5547=CARTESIAN_POINT ( 'NONE',  ( 4.403791563224197070, -10.18230066228895758, 34.26354781536631577 ) ) ;
#5548=CARTESIAN_POINT ( 'NONE',  ( -2.530570990120954100, -7.630691491037286056, 34.74850469731152458 ) ) ;
#5549=LINE ( 'NONE', #80333, #86014 ) ;
#5550=LINE ( 'NONE', #61804, #70093 ) ;
#5551=EDGE_CURVE ( 'NONE', #30008, #45585, #26382, .T. ) ;
#5552=CARTESIAN_POINT ( 'NONE',  ( 5.076923076923075762, -2.499999999999998668, 29.75000000000001421 ) ) ;
#5553=CARTESIAN_POINT ( 'NONE',  ( -2.307692307692427391, -3.835265460704628371, 33.15142922262033665 ) ) ;
#5555=VERTEX_POINT ( 'NONE', #56931 ) ;
#5556=EDGE_LOOP ( 'NONE', ( #38375, #63616, #22591, #39013 ) ) ;
#5557=EDGE_LOOP ( 'NONE', ( #670, #43528, #17289, #50294 ) ) ;
#5558=CARTESIAN_POINT ( 'NONE',  ( 2.084766090176160436, -2.554751324335734264, 30.48935550225260727 ) ) ;
#5560=CARTESIAN_POINT ( 'NONE',  ( 16.15384615384615330, -11.69971097300155272, 32.46337939537588113 ) ) ;
#5561=CARTESIAN_POINT ( 'NONE',  ( -7.912237257109724808, -4.098570777380719399, 33.41473453929634729 ) ) ;
#5562=CARTESIAN_POINT ( 'NONE',  ( 16.37727311570772670, -7.630147231320743018, 34.74852402298682819 ) ) ;
#5563=CARTESIAN_POINT ( 'NONE',  ( -9.942284423250047354, -6.567427716900048118, 34.66269422305636283 ) ) ;
#5564=FACE_BOUND ( 'NONE', #6462, .T. ) ;
#5566=EDGE_CURVE ( 'NONE', #3333, #58130, #35793, .T. ) ;
#5567=EDGE_LOOP ( 'NONE', ( #82605, #51474, #60399, #9534 ) ) ;
#5568=CARTESIAN_POINT ( 'NONE',  ( -1.384615384615383471, -11.91647553114624181, 32.58852847137148245 ) ) ;
#5569=ORIENTED_EDGE ( 'NONE', *, *, #18028, .F. ) ;
#5570=FACE_BOUND ( 'NONE', #38233, .T. ) ;
#5571=CARTESIAN_POINT ( 'NONE',  ( 9.915320536401090123, -5.582272713120729257, 34.63742843783360570 ) ) ;
#5572=VECTOR ( 'NONE', #63305, 1000.000000000000227 ) ;
#5573=CARTESIAN_POINT ( 'NONE',  ( 15.10062126103753855, -6.809168938359901446, 34.95455904226513866 ) ) ;
#5574=VERTEX_POINT ( 'NONE', #23152 ) ;
#5575=CARTESIAN_POINT ( 'NONE',  ( -5.933830859037342975, -7.250054483168843156, 34.74374881642865631 ) ) ;
#5576=CARTESIAN_POINT ( 'NONE',  ( 4.153846153846154188, -1.242168528481310874, 33.36296068462461051 ) ) ;
#5577=CARTESIAN_POINT ( 'NONE',  ( 17.07692307692307665, -12.29105614889573062, 35.45975837776705220 ) ) ;
#5579=CYLINDRICAL_SURFACE ( 'NONE', #74461, 0.2500000000000008882 ) ;
#5580=CARTESIAN_POINT ( 'NONE',  ( 6.700150705560775855, -12.39988816332205701, 30.74660775122750778 ) ) ;
#5581=CARTESIAN_POINT ( 'NONE',  ( -39.05038313613820122, -2.249999999999999556, 27.25000000000000000 ) ) ;
#5583=CARTESIAN_POINT ( 'NONE',  ( 18.00000000000000000, -10.51840700105979565, 33.73612834413961536 ) ) ;
#5584=CARTESIAN_POINT ( 'NONE',  ( 2.557746727605761272, -3.435999193479609470, 33.07426656108011542 ) ) ;
#5585=AXIS2_PLACEMENT_3D ( 'NONE', #3143, #58092, #36073 ) ;
#5586=ORIENTED_EDGE ( 'NONE', *, *, #25752, .T. ) ;
#5587=CARTESIAN_POINT ( 'NONE',  ( 3.480823650682684178, -6.523592122091589118, 34.90882529074906415 ) ) ;
#5589=CARTESIAN_POINT ( 'NONE',  ( -14.30769230769242917, -2.657715359629662544, 31.77849191805970364 ) ) ;
#5590=CARTESIAN_POINT ( 'NONE',  ( -11.66860874789975888, -8.587444163452046197, 34.63053765926554206 ) ) ;
#5591=CARTESIAN_POINT ( 'NONE',  ( 0.4615384615383382183, -2.657715359629662544, 31.77849191805970364 ) ) ;
#5592=EDGE_CURVE ( 'NONE', #29939, #63009, #13460, .T. ) ;
#5593=ADVANCED_FACE ( 'NONE', ( #2426 ), #29919, .F. ) ;
#5594=CARTESIAN_POINT ( 'NONE',  ( 17.14217821643591932, -5.094484230520771817, 34.41647553114626845 ) ) ;
#5595=CARTESIAN_POINT ( 'NONE',  ( 14.05769230769230838, -2.499999999999998668, 29.75000000000000355 ) ) ;
#5596=CARTESIAN_POINT ( 'NONE',  ( -15.29603967673000575, -12.46129190929999986, 30.37095296980880832 ) ) ;
#5597=CARTESIAN_POINT ( 'NONE',  ( -3.230769230769351186, -2.625532179533779154, 30.86335684631627174 ) ) ;
#5598=CARTESIAN_POINT ( 'NONE',  ( -6.673022611438607754, -2.779044189368096163, 31.39831045268886456 ) ) ;
#5600=EDGE_LOOP ( 'NONE', ( #35797, #28180, #48878, #80964 ) ) ;
#5601=CARTESIAN_POINT ( 'NONE',  ( 6.923076923076924238, -7.500000000000001776, 35.04278698407183867 ) ) ;
#5603=ADVANCED_FACE ( 'NONE', ( #43862 ), #71328, .F. ) ;
#5605=CARTESIAN_POINT ( 'NONE',  ( 11.53846153846153832, -4.661471528628507777, 34.16647553114623292 ) ) ;
#5606=VERTEX_POINT ( 'NONE', #58261 ) ;
#5607=CARTESIAN_POINT ( 'NONE',  ( -5.933932666649923249, -9.905515769479277921, 34.41647553114623292 ) ) ;
#5609=CARTESIAN_POINT ( 'NONE',  ( 14.53047184896071542, -11.41317474335729543, 32.86274602512330034 ) ) ;
#5610=CARTESIAN_POINT ( 'NONE',  ( -18.00000000000000000, -11.91647553114624358, 32.58852847137147535 ) ) ;
#5611=CARTESIAN_POINT ( 'NONE',  ( -7.780898274877820597, -6.026961402152789304, 34.52809138561124769 ) ) ;
#5612=CARTESIAN_POINT ( 'NONE',  ( -12.46153846153846168, -11.91647553114624181, 32.58852847137148245 ) ) ;
#5613=CARTESIAN_POINT ( 'NONE',  ( -15.45369618967607828, -4.762599654559228846, 34.23009711892697737 ) ) ;
#5614=CARTESIAN_POINT ( 'NONE',  ( 2.057715576749954867, -9.943427161483782584, 34.11278801902876978 ) ) ;
#5616=CARTESIAN_POINT ( 'NONE',  ( -7.146003881983771677, -4.762599654559228846, 34.23009711892697737 ) ) ;
#5617=CARTESIAN_POINT ( 'NONE',  ( -17.77722033102193322, -2.353885683473780244, 30.79025554430704759 ) ) ;
#5618=CYLINDRICAL_SURFACE ( 'NONE', #6183, 0.2500000000000009437 ) ;
#5620=EDGE_LOOP ( 'NONE', ( #14694, #50528 ) ) ;
#5621=ORIENTED_EDGE ( 'NONE', *, *, #87981, .F. ) ;
#5622=CYLINDRICAL_SURFACE ( 'NONE', #42882, 0.2500000000000009437 ) ;
#5623=CARTESIAN_POINT ( 'NONE',  ( -3.230769230769229949, -13.75783147151868846, 33.36296068462461051 ) ) ;
#5624=CARTESIAN_POINT ( 'NONE',  ( 2.307692307692309264, -12.78798330534102945, 29.74999999999997868 ) ) ;
#5625=CARTESIAN_POINT ( 'NONE',  ( -7.146561847641253351, -5.827078755546623690, 34.72654668319379567 ) ) ;
#5626=DIRECTION ( 'NONE',  ( 0.000000000000000000, 0.1736481776669275834, 0.9848077530122086864 ) ) ;
#5627=B_SPLINE_CURVE_WITH_KNOTS ( 'NONE', 3,
 ( #25405, #4241, #71356, #66388, #58736, #72250, #11007, #58287, #24061, #51971 ),
 .UNSPECIFIED., .F., .F.,
 ( 4, 2, 2, 2, 4 ),
 ( 0.000000000000000000, 0.0001954339857564072033, 0.0003908679715128144066, 0.0005863019572692215828, 0.0007817359430256288133 ),
 .UNSPECIFIED. ) ;
#5628=CARTESIAN_POINT ( 'NONE',  ( -0.5276218724943421146, -6.386643153685125363, 34.62446782046654903 ) ) ;
#5629=B_SPLINE_CURVE_WITH_KNOTS ( 'NONE', 3,
 ( #23363, #36882, #78756, #17058, #3535, #71109, #22927, #30567, #2641, #31006 ),
 .UNSPECIFIED., .F., .F.,
 ( 4, 2, 2, 2, 4 ),
 ( 0.000000000000000000, 0.0001954311564186865221, 0.0003908623128373730441, 0.0005862934692560595662, 0.0007817246256747460882 ),
 .UNSPECIFIED. ) ;
#5632=VERTEX_POINT ( 'NONE', #32137 ) ;
#5634=CARTESIAN_POINT ( 'NONE',  ( 5.142991427925513115, -8.120952969808772792, 34.71129190929999453 ) ) ;
#5635=AXIS2_PLACEMENT_3D ( 'NONE', #15136, #20553, #7493 ) ;
#5636=VECTOR ( 'NONE', #83417, 1000.000000000000000 ) ;
#5637=CARTESIAN_POINT ( 'NONE',  ( -2.372962308248625085, -9.528491918058357157, 34.59228464037090589 ) ) ;
#5638=CARTESIAN_POINT ( 'NONE',  ( -4.283993363284373856, -4.460286881179643004, 33.72017969459903242 ) ) ;
#5639=DIRECTION ( 'NONE',  ( -0.000000000000000000, 0.3420201433256694901, -0.9396926207859082059 ) ) ;
#5640=CARTESIAN_POINT ( 'NONE',  ( -13.51476335434708709, -2.647304123082328875, 31.75400227202885972 ) ) ;
#5641=EDGE_CURVE ( 'NONE', #66197, #11542, #66093, .T. ) ;
#5643=VECTOR ( 'NONE', #45009, 1000.000000000000000 ) ;
#5645=ORIENTED_EDGE ( 'NONE', *, *, #3053, .F. ) ;
#5647=DIRECTION ( 'NONE',  ( 0.000000000000000000, 0.7660444431189822323, -0.6427876096865344779 ) ) ;
#5648=CARTESIAN_POINT ( 'NONE',  ( 10.48523664565292002, -11.66186481527757302, 32.95055677023626117 ) ) ;
#5650=CARTESIAN_POINT ( 'NONE',  ( -15.36146069743678844, -11.18331474514187995, 33.13161551792790505 ) ) ;
#5651=EDGE_CURVE ( 'NONE', #18982, #558, #3717, .T. ) ;
#5652=CARTESIAN_POINT ( 'NONE',  ( 17.75002326905764605, -4.943428324936578910, 34.04746400365624481 ) ) ;
#5653=CARTESIAN_POINT ( 'NONE',  ( -10.36543909703647337, -12.22109172314383052, 31.39792113162168263 ) ) ;
#5654=VERTEX_POINT ( 'NONE', #85307 ) ;
#5655=EDGE_CURVE ( 'NONE', #21025, #26289, #71520, .T. ) ;
#5657=CARTESIAN_POINT ( 'NONE',  ( 17.14217864819910275, -12.46129190930001052, 30.37095296980869819 ) ) ;
#5659=DIRECTION ( 'NONE',  ( 0.000000000000000000, 0.000000000000000000, 1.000000000000000000 ) ) ;
#5660=CARTESIAN_POINT ( 'NONE',  ( 12.71148387091650278, -8.476813868363244353, 34.90874843262270133 ) ) ;
#5662=VERTEX_POINT ( 'NONE', #11872 ) ;
#5663=EDGE_CURVE ( 'NONE', #86404, #60435, #24924, .T. ) ;
#5664=CARTESIAN_POINT ( 'NONE',  ( -1.134669975237341921, -2.589246495874657938, 31.60778113518102828 ) ) ;
#5665=ORIENTED_EDGE ( 'NONE', *, *, #4431, .T. ) ;
#5666=CARTESIAN_POINT ( 'NONE',  ( -5.999999999999998224, -12.29105614889573062, 35.45975837776705220 ) ) ;
#5669=CARTESIAN_POINT ( 'NONE',  ( -5.934744860487159990, -3.083524468853784839, 32.58852847137153930 ) ) ;
#5670=EDGE_CURVE ( 'NONE', #32572, #67440, #61781, .T. ) ;
#5671=CARTESIAN_POINT ( 'NONE',  ( 8.519254038288414321, -4.943428324936578910, 34.04746400365624481 ) ) ;
#5672=ORIENTED_EDGE ( 'NONE', *, *, #5914, .T. ) ;
#5673=DIRECTION ( 'NONE',  ( 0.000000000000000000, 0.3420201433256610524, 0.9396926207859113145 ) ) ;
#5675=CARTESIAN_POINT ( 'NONE',  ( -14.08468095607945969, -2.758310577978207778, 31.33698337089302299 ) ) ;
#5676=ORIENTED_EDGE ( 'NONE', *, *, #60848, .F. ) ;
#5677=CARTESIAN_POINT ( 'NONE',  ( -9.442253272394237840, -4.818054556918156983, 34.26375889529406749 ) ) ;
#5678=CARTESIAN_POINT ( 'NONE',  ( -4.023320715612507925, -10.31582465632705237, 34.18122507451815295 ) ) ;
#5679=CARTESIAN_POINT ( 'NONE',  ( -16.40384615384616041, -2.250000000000000000, 29.81609741502490607 ) ) ;
#5680=CARTESIAN_POINT ( 'NONE',  ( -9.692307692307691624, -1.790695186598648903, 34.54067556320373455 ) ) ;
#5681=CARTESIAN_POINT ( 'NONE',  ( 8.899756207464413649, -10.31582465632705237, 34.18122507451815295 ) ) ;
#5683=FACE_BOUND ( 'NONE', #62574, .T. ) ;
#5684=CARTESIAN_POINT ( 'NONE',  ( 1.319292469123210854, -7.749976743299137993, 34.99404534957040624 ) ) ;
#5686=CARTESIAN_POINT ( 'NONE',  ( 2.084765348785458272, -10.01117774369187252, 34.36070679894347535 ) ) ;
#5688=CARTESIAN_POINT ( 'NONE',  ( -2.057692307692306599, -2.499999999999998668, 29.75000000000000355 ) ) ;
#5689=EDGE_CURVE ( 'NONE', #66615, #50015, #42509, .T. ) ;
#5690=CARTESIAN_POINT ( 'NONE',  ( 6.130790440966950250, -4.684288915650984819, 34.18129842949671371 ) ) ;
#5692=ORIENTED_EDGE ( 'NONE', *, *, #3407, .T. ) ;
#5693=CARTESIAN_POINT ( 'NONE',  ( 10.48523664565292357, -12.15440758774515473, 32.17923288041532004 ) ) ;
#5695=VECTOR ( 'NONE', #68592, 1000.000000000000000 ) ;
#5697=DIRECTION ( 'NONE',  ( 0.000000000000000000, 0.3420201433256641055, -0.9396926207859100932 ) ) ;
#5698=EDGE_CURVE ( 'NONE', #72772, #12820, #25263, .T. ) ;
#5700=ADVANCED_FACE ( 'NONE', ( #74902 ), #54160, .F. ) ;
#5701=CARTESIAN_POINT ( 'NONE',  ( 7.846153846153725020, -9.442884908241554243, 34.35708131394783038 ) ) ;
#5703=CARTESIAN_POINT ( 'NONE',  ( -10.68065461594093435, -11.67786785259540849, 32.92929555188721480 ) ) ;
#5704=ORIENTED_EDGE ( 'NONE', *, *, #42159, .T. ) ;
#5705=CARTESIAN_POINT ( 'NONE',  ( 7.846153846153725020, -9.442884908241554243, 34.35708131394783038 ) ) ;
#5706=DIRECTION ( 'NONE',  ( -0.000000000000000000, 0.9396926207859092051, -0.3420201433256662704 ) ) ;
#5708=CARTESIAN_POINT ( 'NONE',  ( 4.219101725122178514, -10.90142922261932057, 33.41473453929631887 ) ) ;
#5709=CARTESIAN_POINT ( 'NONE',  ( 8.639082799499067988, -2.647304123082328875, 31.75400227202885972 ) ) ;
#5711=CARTESIAN_POINT ( 'NONE',  ( 4.023698944407932743, -11.93770438780619259, 32.05411857736982029 ) ) ;
#5712=CARTESIAN_POINT ( 'NONE',  ( -1.134560964701931018, -6.523592122091591783, 34.90882529074906415 ) ) ;
#5713=CARTESIAN_POINT ( 'NONE',  ( 1.450682717965462221, -9.905515769479277921, 34.41647553114623292 ) ) ;
#5716=CARTESIAN_POINT ( 'NONE',  ( -4.219928533206289245, -2.833524468853757305, 32.15551576947924417 ) ) ;
#5717=CARTESIAN_POINT ( 'NONE',  ( -11.53846153846165912, -10.90142922262034020, 33.41473453929536674 ) ) ;
#5718=EDGE_LOOP ( 'NONE', ( #35076, #3105 ) ) ;
#5720=DIRECTION ( 'NONE',  ( 0.000000000000000000, 0.4999999999999960032, -0.8660254037844410391 ) ) ;
#5722=CARTESIAN_POINT ( 'NONE',  ( 2.177544337960612086, -5.070767119584671967, 34.40440758774516183 ) ) ;
#5723=CARTESIAN_POINT ( 'NONE',  ( 6.923076923077231548, -2.506253911140614576, 30.00000000000323297 ) ) ;
#5724=ORIENTED_EDGE ( 'NONE', *, *, #78900, .T. ) ;
#5725=DIRECTION ( 'NONE',  ( -0.000000000000000000, -0.1736481776669307198, -0.9848077530122080203 ) ) ;
#5726=DIRECTION ( 'NONE',  ( -0.000000000000000000, -0.3420201433256694346, -0.9396926207859080948 ) ) ;
#5727=CARTESIAN_POINT ( 'NONE',  ( 9.019176178608811156, -2.589246495874658383, 31.60778113518102828 ) ) ;
#5728=ORIENTED_EDGE ( 'NONE', *, *, #44247, .F. ) ;
#5730=CARTESIAN_POINT ( 'NONE',  ( -15.00775638667583678, -11.98016756924215009, 32.48728574198911190 ) ) ;
#5732=ORIENTED_EDGE ( 'NONE', *, *, #5813, .F. ) ;
#5733=CARTESIAN_POINT ( 'NONE',  ( 5.011652630962299959, -4.481592998940161721, 33.73612834413957984 ) ) ;
#5734=EDGE_CURVE ( 'NONE', #31351, #1868, #5550, .T. ) ;
#5736=CARTESIAN_POINT ( 'NONE',  ( 1.384615384615386802, -2.833524468853757305, 32.15551576947925838 ) ) ;
#5737=VERTEX_POINT ( 'NONE', #46535 ) ;
#5738=ORIENTED_EDGE ( 'NONE', *, *, #4753, .T. ) ;
#5740=EDGE_CURVE ( 'NONE', #72102, #87523, #45511, .T. ) ;
#5741=VECTOR ( 'NONE', #58632, 1000.000000000000114 ) ;
#5742=ORIENTED_EDGE ( 'NONE', *, *, #88799, .T. ) ;
#5744=CARTESIAN_POINT ( 'NONE',  ( 5.326868595271218254, -12.22109172314383052, 31.39792113162168263 ) ) ;
#5745=CARTESIAN_POINT ( 'NONE',  ( -2.307692307692427391, -6.026961402154118908, 34.52809138561165270 ) ) ;
#5746=DIRECTION ( 'NONE',  ( -0.000000000000000000, 1.000000000000000000, -0.000000000000000000 ) ) ;
#5748=EDGE_CURVE ( 'NONE', #18634, #26348, #21908, .T. ) ;
#5750=ORIENTED_EDGE ( 'NONE', *, *, #34917, .F. ) ;
#5751=EDGE_LOOP ( 'NONE', ( #41470, #31607, #88440, #45608 ) ) ;
#5752=B_SPLINE_CURVE_WITH_KNOTS ( 'NONE', 3,
 ( #47989, #5679, #26845, #60618, #61503, #34484 ),
 .UNSPECIFIED., .F., .F.,
 ( 4, 2, 4 ),
 ( 1.769077770938648657E-17, 0.0001954756301636913782, 0.0003909512603273650297 ),
 .UNSPECIFIED. ) ;
#5754=ORIENTED_EDGE ( 'NONE', *, *, #21698, .T. ) ;
#5755=CARTESIAN_POINT ( 'NONE',  ( -2.980769230769230393, -2.499999999999998668, 29.75000000000000355 ) ) ;
#5756=ORIENTED_EDGE ( 'NONE', *, *, #71480, .F. ) ;
#5757=CARTESIAN_POINT ( 'NONE',  ( -16.37677311275299985, -12.38737895849757820, 31.66785238281580206 ) ) ;
#5758=B_SPLINE_CURVE_WITH_KNOTS ( 'NONE', 3,
 ( #46772, #39590, #33702, #33263, #34587, #12111, #88670, #75142, #53966, #13425 ),
 .UNSPECIFIED., .F., .F.,
 ( 4, 2, 2, 2, 4 ),
 ( 0.000000000000000000, 0.0001954339857564092904, 0.0003908679715128185808, 0.0005863019572692278712, 0.0007817359430256371616 ),
 .UNSPECIFIED. ) ;
#5759=B_SPLINE_CURVE_WITH_KNOTS ( 'NONE', 3,
 ( #59495, #39690, #25717, #88332, #46867, #47308, #74800, #13091, #73470, #86998 ),
 .UNSPECIFIED., .F., .F.,
 ( 4, 2, 2, 2, 4 ),
 ( 0.000000000000000000, 0.0001954311564186878773, 0.0003908623128373757546, 0.0005862934692560635777, 0.0007817246256747515092 ),
 .UNSPECIFIED. ) ;
#5760=DIRECTION ( 'NONE',  ( 0.000000000000000000, 0.7660444431189807890, 0.6427876096865361433 ) ) ;
#5762=VECTOR ( 'NONE', #80214, 1000.000000000000227 ) ;
#5763=EDGE_CURVE ( 'NONE', #10580, #58351, #13290, .T. ) ;
#5767=ADVANCED_FACE ( 'NONE', ( #60039 ), #87546, .F. ) ;
#5768=ORIENTED_EDGE ( 'NONE', *, *, #63089, .F. ) ;
#5769=ORIENTED_EDGE ( 'NONE', *, *, #39546, .T. ) ;
#5770=CARTESIAN_POINT ( 'NONE',  ( 10.68064018666063930, -10.90142922261932057, 33.41473453929631887 ) ) ;
#5771=CYLINDRICAL_SURFACE ( 'NONE', #61688, 0.2499999999999995559 ) ;
#5772=EDGE_LOOP ( 'NONE', ( #62273, #26038, #23597, #37806 ) ) ;
#5773=DIRECTION ( 'NONE',  ( -0.000000000000000000, -0.3420201433256694901, -0.9396926207859082059 ) ) ;
#5775=ORIENTED_EDGE ( 'NONE', *, *, #9846, .T. ) ;
#5776=FACE_OUTER_BOUND ( 'NONE', #2140, .T. ) ;
#5777=DIRECTION ( 'NONE',  ( -1.000000000000000000, 0.000000000000000000, 0.000000000000000000 ) ) ;
#5778=FACE_OUTER_BOUND ( 'NONE', #8619, .T. ) ;
#5779=FACE_BOUND ( 'NONE', #66797, .T. ) ;
#5780=CARTESIAN_POINT ( 'NONE',  ( -15.23076923076935252, -8.656820664282941280, 34.87096338111179961 ) ) ;
#5781=CARTESIAN_POINT ( 'NONE',  ( -1.318547033612944563, -11.69971097300155272, 32.46337939537588113 ) ) ;
#5782=DIRECTION ( 'NONE',  ( -0.000000000000000000, -0.3420201433256694901, -0.9396926207859082059 ) ) ;
#5783=DIRECTION ( 'NONE',  ( -0.000000000000000000, -0.1736481776669307198, -0.9848077530122080203 ) ) ;
#5784=CARTESIAN_POINT ( 'NONE',  ( 15.36155967173618286, -9.929761469519743144, 34.40412654351204225 ) ) ;
#5785=CYLINDRICAL_SURFACE ( 'NONE', #50979, 0.2499999999999995559 ) ;
#5786=CARTESIAN_POINT ( 'NONE',  ( 12.46153846153833911, -3.083524468854526912, 32.58852847137268327 ) ) ;
#5787=ORIENTED_EDGE ( 'NONE', *, *, #83805, .T. ) ;
#5788=CARTESIAN_POINT ( 'NONE',  ( -17.20761368003338276, -5.496505350115500121, 34.60290016733514307 ) ) ;
#5789=CARTESIAN_POINT ( 'NONE',  ( 10.61538461538449596, -3.835265460704628371, 33.15142922262033665 ) ) ;
#5790=ORIENTED_EDGE ( 'NONE', *, *, #37887, .F. ) ;
#5792=CARTESIAN_POINT ( 'NONE',  ( -17.14219352288385423, -11.48612834413959582, 32.76840700105983473 ) ) ;
#5793=CARTESIAN_POINT ( 'NONE',  ( -15.45425417449317784, -2.599994579823203367, 30.74605699353653776 ) ) ;
#5794=CARTESIAN_POINT ( 'NONE',  ( -11.76194646302586655, -10.23692288466677880, 34.23039457007281072 ) ) ;
#5795=ORIENTED_EDGE ( 'NONE', *, *, #43074, .F. ) ;
#5796=CARTESIAN_POINT ( 'NONE',  ( -16.15384615384627409, -11.48612834414049644, 32.76840700105863391 ) ) ;
#5797=CARTESIAN_POINT ( 'NONE',  ( -4.284536756956460302, -9.084618155246140248, 34.75535874321725771 ) ) ;
#5798=EDGE_CURVE ( 'NONE', #42433, #17811, #2591, .T. ) ;
#5799=EDGE_CURVE ( 'NONE', #60703, #10963, #14405, .T. ) ;
#5800=FACE_BOUND ( 'NONE', #9323, .T. ) ;
#5801=DIRECTION ( 'NONE',  ( -0.000000000000000000, 0.9848077530122085754, -0.1736481776669273613 ) ) ;
#5802=CARTESIAN_POINT ( 'NONE',  ( -9.915792636031639518, -4.386631170607603991, 33.66268669641500111 ) ) ;
#5803=CARTESIAN_POINT ( 'NONE',  ( -13.51530598772569292, -2.295517848115769421, 30.44137282052137294 ) ) ;
#5806=DIRECTION ( 'NONE',  ( -0.000000000000000000, -0.7660444431189791237, -0.6427876096865379196 ) ) ;
#5807=AXIS2_PLACEMENT_3D ( 'NONE', #14922, #54557, #75716 ) ;
#5810=ADVANCED_FACE ( 'NONE', ( #9102 ), #50508, .F. ) ;
#5812=CARTESIAN_POINT ( 'NONE',  ( -12.39547112818838670, -5.471508081941601098, 34.59228464037088457 ) ) ;
#5813=EDGE_CURVE ( 'NONE', #50015, #66615, #59554, .T. ) ;
#5814=CARTESIAN_POINT ( 'NONE',  ( -4.153846153846273204, -12.46129190930018460, 30.37095296980731973 ) ) ;
#5815=CARTESIAN_POINT ( 'NONE',  ( -10.61538461538461320, -2.292212530054420494, 30.41441678777542634 ) ) ;
#5817=CARTESIAN_POINT ( 'NONE',  ( -7.716108790234073034, -2.254550872974305342, 29.97347326024527447 ) ) ;
#5819=CARTESIAN_POINT ( 'NONE',  ( -8.899378738962465007, -10.31621877034669588, 34.18098118002070152 ) ) ;
#5820=CARTESIAN_POINT ( 'NONE',  ( 5.869309396889694774, -2.845849958028613624, 32.17971566917920967 ) ) ;
#5822=CARTESIAN_POINT ( 'NONE',  ( 13.25392478150507891, -9.929715669179220328, 34.40415004197138416 ) ) ;
#5823=DIRECTION ( 'NONE',  ( -0.000000000000000000, -0.3420201433256694901, -0.9396926207859082059 ) ) ;
#5824=CARTESIAN_POINT ( 'NONE',  ( 13.31853197365950514, -4.098570777380720287, 33.41473453929634729 ) ) ;
#5825=DIRECTION ( 'NONE',  ( -0.000000000000000000, -0.000000000000000000, -1.000000000000000000 ) ) ;
#5827=AXIS2_PLACEMENT_3D ( 'NONE', #12108, #39134, #39587 ) ;
#5828=CARTESIAN_POINT ( 'NONE',  ( -15.23076923076935074, -10.21337939537710326, 33.94971097300076224 ) ) ;
#5829=ADVANCED_FACE ( 'NONE', ( #69902 ), #56826, .F. ) ;
#5830=VERTEX_POINT ( 'NONE', #42887 ) ;
#5831=CARTESIAN_POINT ( 'NONE',  ( -7.846153846153844924, -12.78798330534102767, 29.49999999999997868 ) ) ;
#5832=CARTESIAN_POINT ( 'NONE',  ( 18.22301284409339672, -4.762714258010882773, 34.23016756924214832 ) ) ;
#5835=AXIS2_PLACEMENT_3D ( 'NONE', #84338, #84781, #85215 ) ;
#5836=CARTESIAN_POINT ( 'NONE',  ( -18.25000000000000000, -2.499999999999999556, 29.75000000000000355 ) ) ;
#5837=FACE_OUTER_BOUND ( 'NONE', #87459, .T. ) ;
#5838=EDGE_CURVE ( 'NONE', #23792, #13144, #35689, .T. ) ;
#5839=CARTESIAN_POINT ( 'NONE',  ( -1.384615384615383471, -13.88283147151868846, 33.14645433367849847 ) ) ;
#5840=CARTESIAN_POINT ( 'NONE',  ( 10.68155122197626028, -7.250054591869670162, 34.99404684341514127 ) ) ;
#5841=ORIENTED_EDGE ( 'NONE', *, *, #66428, .T. ) ;
#5843=CARTESIAN_POINT ( 'NONE',  ( 17.07692307692307665, -8.810774026931790459, 35.74407628777942847 ) ) ;
#5844=CIRCLE ( 'NONE', #71980, 0.2500000000000002220 ) ;
#5845=EDGE_LOOP ( 'NONE', ( #59574, #30913, #65334, #72865 ) ) ;
#5846=CARTESIAN_POINT ( 'NONE',  ( -5.076923076923197442, -11.94971097300221174, 32.03036669348237098 ) ) ;
#5847=AXIS2_PLACEMENT_3D ( 'NONE', #71910, #10220, #36364 ) ;
#5848=CARTESIAN_POINT ( 'NONE',  ( 18.13079180782478872, -8.999086150933472084, 34.52020707165672064 ) ) ;
#5850=ORIENTED_EDGE ( 'NONE', *, *, #87416, .F. ) ;
#5851=CARTESIAN_POINT ( 'NONE',  ( 3.007842271862381622, -4.762599654559228846, 34.23009711892697737 ) ) ;
#5852=EDGE_CURVE ( 'NONE', #8365, #47121, #67056, .T. ) ;
#5853=CARTESIAN_POINT ( 'NONE',  ( -16.21917016665046418, -7.749976730030849303, 34.74374725381503737 ) ) ;
#5854=FACE_OUTER_BOUND ( 'NONE', #63365, .T. ) ;
#5855=ORIENTED_EDGE ( 'NONE', *, *, #84982, .T. ) ;
#5856=VERTEX_POINT ( 'NONE', #56394 ) ;
#5857=EDGE_CURVE ( 'NONE', #42328, #65392, #69119, .T. ) ;
#5858=ORIENTED_EDGE ( 'NONE', *, *, #46650, .T. ) ;
#5859=DIRECTION ( 'NONE',  ( -0.000000000000000000, 0.8660254037844399289, -0.4999999999999980016 ) ) ;
#5860=CARTESIAN_POINT ( 'NONE',  ( 15.90384615384615330, -2.499999999999998668, 29.75000000000000355 ) ) ;
#5862=CARTESIAN_POINT ( 'NONE',  ( -15.45369618967607828, -2.308479472611653094, 30.53278059502174457 ) ) ;
#5863=DIRECTION ( 'NONE',  ( 1.000000000000000000, 0.000000000000000000, 0.000000000000000000 ) ) ;
#5865=CARTESIAN_POINT ( 'NONE',  ( 12.46153846153833911, -5.219633306517616589, 34.19971097300220464 ) ) ;
#5866=EDGE_CURVE ( 'NONE', #314, #32867, #23022, .T. ) ;
#5867=CARTESIAN_POINT ( 'NONE',  ( 16.02315555073584363, -12.62707690430377383, 30.88035979386743435 ) ) ;
#5868=ORIENTED_EDGE ( 'NONE', *, *, #48932, .T. ) ;
#5869=EDGE_LOOP ( 'NONE', ( #49224, #63503 ) ) ;
#5871=VERTEX_POINT ( 'NONE', #44180 ) ;
#5873=ORIENTED_EDGE ( 'NONE', *, *, #22145, .T. ) ;
#5874=AXIS2_PLACEMENT_3D ( 'NONE', #8938, #3045, #70634 ) ;
#5875=DIRECTION ( 'NONE',  ( 0.000000000000000000, -6.938893903907222067E-15, 1.000000000000000000 ) ) ;
#5876=CARTESIAN_POINT ( 'NONE',  ( 11.78840705680967993, -12.22109172314383052, 31.39792113162168263 ) ) ;
#5877=VERTEX_POINT ( 'NONE', #18072 ) ;
#5878=EDGE_CURVE ( 'NONE', #70194, #48033, #55245, .T. ) ;
#5879=CARTESIAN_POINT ( 'NONE',  ( -12.46153846153858424, -11.67786785259630911, 32.92929555188603530 ) ) ;
#5880=ADVANCED_FACE ( 'NONE', ( #86997 ), #85640, .F. ) ;
#5881=ORIENTED_EDGE ( 'NONE', *, *, #69342, .F. ) ;
#5882=CARTESIAN_POINT ( 'NONE',  ( 16.94623161025551639, -9.804603061927743113, 34.18744698557895845 ) ) ;
#5883=EDGE_LOOP ( 'NONE', ( #61223, #1848, #48991, #19306 ) ) ;
#5884=LINE ( 'NONE', #67141, #17206 ) ;
#5885=CARTESIAN_POINT ( 'NONE',  ( 1.607626736228236819, -6.503523203565942268, 34.64991518177335195 ) ) ;
#5886=CARTESIAN_POINT ( 'NONE',  ( 16.94677586748486320, -2.882441371585227508, 31.66841991370172238 ) ) ;
#5887=B_SPLINE_CURVE_WITH_KNOTS ( 'NONE', 3,
 ( #65572, #31358, #65125, #3431, #58819, #52507, #44402, #11536, #4326, #86322 ),
 .UNSPECIFIED., .F., .F.,
 ( 4, 2, 2, 2, 4 ),
 ( 0.0007817246256747465219, 0.0009771112852218900684, 0.001172497944769033615, 0.001367884604316177378, 0.001563271263863320925 ),
 .UNSPECIFIED. ) ;
#5888=FACE_BOUND ( 'NONE', #82907, .T. ) ;
#5889=CARTESIAN_POINT ( 'NONE',  ( -14.43784027742400156, -9.504002272028875709, 34.60269587691767867 ) ) ;
#5890=CARTESIAN_POINT ( 'NONE',  ( 8.769230769230645706, -5.941354392335915335, 34.76329471203413846 ) ) ;
#5891=VECTOR ( 'NONE', #53283, 1000.000000000000227 ) ;
#5896=CYLINDRICAL_SURFACE ( 'NONE', #13159, 0.2500000000000012212 ) ;
#5897=CYLINDRICAL_SURFACE ( 'NONE', #87767, 0.2499999999999979738 ) ;
#5898=EDGE_LOOP ( 'NONE', ( #50989, #37839, #11867, #56311 ) ) ;
#5899=EDGE_LOOP ( 'NONE', ( #67957, #38556 ) ) ;
#5901=CARTESIAN_POINT ( 'NONE',  ( -3.230769230769229949, -2.538708090699994813, 30.37095296980875503 ) ) ;
#5902=DIRECTION ( 'NONE',  ( 0.000000000000000000, 0.8660254037844377084, -0.5000000000000015543 ) ) ;
#5903=FACE_OUTER_BOUND ( 'NONE', #86304, .T. ) ;
#5904=CARTESIAN_POINT ( 'NONE',  ( -13.38461538461538325, -13.57706302396349152, 30.56769352161908060 ) ) ;
#5906=CARTESIAN_POINT ( 'NONE',  ( -2.242436736416282717, -2.892918686051626498, 31.69288490824026638 ) ) ;
#5907=ORIENTED_EDGE ( 'NONE', *, *, #78893, .F. ) ;
#5908=CARTESIAN_POINT ( 'NONE',  ( -5.076923076923075762, -5.471508081941601098, 34.59228464037088457 ) ) ;
#5909=CARTESIAN_POINT ( 'NONE',  ( 14.08476609017615644, -11.24512374952581872, 33.06303171183252942 ) ) ;
#5911=CARTESIAN_POINT ( 'NONE',  ( 6.923076923076924238, -2.499999999999998668, 29.75000000000001421 ) ) ;
#5912=EDGE_LOOP ( 'NONE', ( #17761, #34670 ) ) ;
#5913=ORIENTED_EDGE ( 'NONE', *, *, #36418, .F. ) ;
#5914=EDGE_CURVE ( 'NONE', #34591, #52302, #64905, .T. ) ;
#5916=ORIENTED_EDGE ( 'NONE', *, *, #58604, .T. ) ;
#5917=CARTESIAN_POINT ( 'NONE',  ( 0.3310617534219970626, -7.276988635370452485, 34.74523720219453793 ) ) ;
#5918=ADVANCED_FACE ( 'NONE', ( #52287 ), #85201, .F. ) ;
#5919=VERTEX_POINT ( 'NONE', #45533 ) ;
#5921=CARTESIAN_POINT ( 'NONE',  ( 14.43821774592595553, -5.915461855592780260, 34.75538340440931506 ) ) ;
#5922=CARTESIAN_POINT ( 'NONE',  ( 3.230769230769108269, -10.33852847137269571, 34.16647553114546554 ) ) ;
#5923=DIRECTION ( 'NONE',  ( -0.000000000000000000, -0.7660444431189791237, -0.6427876096865379196 ) ) ;
#5924=CARTESIAN_POINT ( 'NONE',  ( 8.546304551714619890, -6.503392248772476236, 34.64988816332204635 ) ) ;
#5925=ORIENTED_EDGE ( 'NONE', *, *, #55195, .F. ) ;
#5926=EDGE_CURVE ( 'NONE', #74684, #52843, #75658, .T. ) ;
#5927=CARTESIAN_POINT ( 'NONE',  ( -15.00775638667583500, -2.523321265292115534, 31.42251411153756990 ) ) ;
#5928=CARTESIAN_POINT ( 'NONE',  ( -15.48079245499068435, -12.07920672191015221, 32.31858351112116168 ) ) ;
#5929=VERTEX_POINT ( 'NONE', #52728 ) ;
#5930=DIRECTION ( 'NONE',  ( -0.000000000000000000, -0.8660254037844399289, -0.4999999999999980016 ) ) ;
#5931=CARTESIAN_POINT ( 'NONE',  ( -2.531177251416254936, -9.331801661448606566, 34.40259984581193464 ) ) ;
#5932=CARTESIAN_POINT ( 'NONE',  ( -11.53846153846166089, -11.06231777344772027, 33.60647404775119895 ) ) ;
#5933=B_SPLINE_CURVE_WITH_KNOTS ( 'NONE', 3,
 ( #5267, #5708, #6155, #12906, #67854, #88156, #19229, #75065, #80491, #60644 ),
 .UNSPECIFIED., .F., .F.,
 ( 4, 2, 2, 2, 4 ),
 ( 0.0007817359430256215491, 0.0009771253907249856981, 0.001172514838424349847, 0.001367904286123713779, 0.001563293733823077928 ),
 .UNSPECIFIED. ) ;
#5935=DIRECTION ( 'NONE',  ( -0.000000000000000000, 1.000000000000000000, 3.491481338843133355E-15 ) ) ;
#5936=FACE_OUTER_BOUND ( 'NONE', #18233, .T. ) ;
#5937=CARTESIAN_POINT ( 'NONE',  ( -8.519285359852727169, -9.357781135181031829, 34.66075350412533851 ) ) ;
#5938=B_SPLINE_CURVE_WITH_KNOTS ( 'NONE', 3,
 ( #12825, #33097, #79956, #40310, #67772, #45268 ),
 .UNSPECIFIED., .F., .F.,
 ( 4, 2, 4 ),
 ( 0.0003909512603273932732, 0.0005862562993132219456, 0.0007815613382990506180 ),
 .UNSPECIFIED. ) ;
#5939=CARTESIAN_POINT ( 'NONE',  ( 12.71148397988660328, -11.37275283266504111, 32.91324779482534524 ) ) ;
#5940=AXIS2_PLACEMENT_3D ( 'NONE', #42833, #9476, #2262 ) ;
#5943=ORIENTED_EDGE ( 'NONE', *, *, #37165, .F. ) ;
#5944=B_SPLINE_CURVE_WITH_KNOTS ( 'NONE', 3,
 ( #29509, #76809, #8796, #36267, #84459, #49764, #1589, #2457, #22734, #51076 ),
 .UNSPECIFIED., .F., .F.,
 ( 4, 2, 2, 2, 4 ),
 ( 0.000000000000000000, 0.0001954311564186861968, 0.0003908623128373723936, 0.0005862934692560585904, 0.0007817246256747447872 ),
 .UNSPECIFIED. ) ;
#5945=CARTESIAN_POINT ( 'NONE',  ( -6.989159302437059296, -10.67929555188718460, 33.92786785259543336 ) ) ;
#5946=CARTESIAN_POINT ( 'NONE',  ( -1.161835715637316913, -3.563462043263030399, 33.22394488606062879 ) ) ;
#5947=B_SPLINE_CURVE_WITH_KNOTS ( 'NONE', 3,
 ( #55882, #83369, #15353, #16659, #63072, #8151, #84263, #15796, #71600, #84706 ),
 .UNSPECIFIED., .F., .F.,
 ( 4, 2, 2, 2, 4 ),
 ( 0.0007817246256747440282, 0.0009771112852218863821, 0.001172497944769028844, 0.001367884604316171307, 0.001563271263863313769 ),
 .UNSPECIFIED. ) ;
#5948=EDGE_CURVE ( 'NONE', #59502, #20820, #9525, .T. ) ;
#5949=ORIENTED_EDGE ( 'NONE', *, *, #3036, .F. ) ;
#5950=CARTESIAN_POINT ( 'NONE',  ( -1.384615384615383471, -11.69971097300155272, 32.46337939537588113 ) ) ;
#5951=CARTESIAN_POINT ( 'NONE',  ( -3.230769230769229949, -5.557115091759785130, 34.35708131394839171 ) ) ;
#5953=EDGE_CURVE ( 'NONE', #8955, #37810, #11217, .T. ) ;
#5954=CARTESIAN_POINT ( 'NONE',  ( 6.923076923076924238, -5.557115091759785130, 34.35708131394839171 ) ) ;
#5955=CARTESIAN_POINT ( 'NONE',  ( 17.93391762063986761, -2.486705287966279432, 31.30864560766543647 ) ) ;
#5956=ORIENTED_EDGE ( 'NONE', *, *, #81788, .F. ) ;
#5957=CYLINDRICAL_SURFACE ( 'NONE', #64990, 0.2499999999999995559 ) ;
#5960=CARTESIAN_POINT ( 'NONE',  ( 18.13079044096694759, -12.35292014791297710, 31.75344720912887198 ) ) ;
#5962=CARTESIAN_POINT ( 'NONE',  ( -17.01166793741023042, -12.16647553114626490, 32.15551576947920864 ) ) ;
#5963=EDGE_CURVE ( 'NONE', #44313, #87990, #31577, .T. ) ;
#5965=CARTESIAN_POINT ( 'NONE',  ( 13.60762673622823549, -3.587049720035815348, 32.86302985866382897 ) ) ;
#5966=CARTESIAN_POINT ( 'NONE',  ( 15.23076923076923173, -1.790695186598648903, 34.54067556320373455 ) ) ;
#5967=VERTEX_POINT ( 'NONE', #75239 ) ;
#5968=ADVANCED_FACE ( 'NONE', ( #39238 ), #46424, .F. ) ;
#5970=CARTESIAN_POINT ( 'NONE',  ( -6.130147969731694069, -2.373036134822904319, 30.88089517874952250 ) ) ;
#5971=CARTESIAN_POINT ( 'NONE',  ( -9.942284423250045577, -2.564618984488975073, 30.55390908950641915 ) ) ;
#5972=VECTOR ( 'NONE', #50658, 1000.000000000000000 ) ;
#5973=B_SPLINE_CURVE_WITH_KNOTS ( 'NONE', 3,
 ( #69316, #1288, #63873, #63431, #57119, #8058, #84172, #15259, #71077, #76512 ),
 .UNSPECIFIED., .F., .F.,
 ( 4, 2, 2, 2, 4 ),
 ( 0.0007817359430256372700, 0.0009771253907250052138, 0.001172514838424373266, 0.001367904286123741101, 0.001563293733823109153 ),
 .UNSPECIFIED. ) ;
#5974=B_SPLINE_CURVE_WITH_KNOTS ( 'NONE', 3,
 ( #6335, #61697, #54054, #75235, #61250, #47303, #26152, #60820, #74793, #34686 ),
 .UNSPECIFIED., .F., .F.,
 ( 4, 2, 2, 2, 4 ),
 ( 0.0007817246256747453293, 0.0009771112852218889842, 0.001172497944769032531, 0.001367884604316176294, 0.001563271263863319840 ),
 .UNSPECIFIED. ) ;
#5975=CARTESIAN_POINT ( 'NONE',  ( -14.30769230769230660, -4.786620604624113540, 33.94971097300155094 ) ) ;
#5976=CARTESIAN_POINT ( 'NONE',  ( -1.514763354347082647, -11.04286588640298561, 33.62463336215343901 ) ) ;
#5977=B_SPLINE_CURVE_WITH_KNOTS ( 'NONE', 3,
 ( #86025, #72499, #58095, #78812, #70739, #57220, #10808, #17112, #44567, #56769 ),
 .UNSPECIFIED., .F., .F.,
 ( 4, 2, 2, 2, 4 ),
 ( 0.0007817359430256253438, 0.0009771253907249898181, 0.001172514838424354401, 0.001367904286123718983, 0.001563293733823083566 ),
 .UNSPECIFIED. ) ;
#5978=EDGE_CURVE ( 'NONE', #67015, #76205, #39689, .T. ) ;
#5981=FACE_BOUND ( 'NONE', #40325, .T. ) ;
#5982=ORIENTED_EDGE ( 'NONE', *, *, #36049, .T. ) ;
#5983=CARTESIAN_POINT ( 'NONE',  ( -9.692307692307691624, -2.499999999999998668, 29.75000000000001421 ) ) ;
#5984=DIRECTION ( 'NONE',  ( 0.000000000000000000, 0.000000000000000000, 1.000000000000000000 ) ) ;
#5985=CARTESIAN_POINT ( 'NONE',  ( -13.38461538461538325, -13.88283147151868846, 33.14645433367849847 ) ) ;
#5986=LINE ( 'NONE', #40217, #62207 ) ;
#5987=CARTESIAN_POINT ( 'NONE',  ( -11.28851602011339672, -2.587454068350147018, 30.68340429815432202 ) ) ;
#5988=EDGE_CURVE ( 'NONE', #68238, #35285, #74469, .T. ) ;
#5991=VERTEX_POINT ( 'NONE', #87433 ) ;
#5992=VECTOR ( 'NONE', #26273, 1000.000000000000227 ) ;
#5993=EDGE_CURVE ( 'NONE', #88630, #88864, #8984, .T. ) ;
#5994=EDGE_CURVE ( 'NONE', #11924, #84921, #61611, .T. ) ;
#5995=EDGE_LOOP ( 'NONE', ( #73917, #38811 ) ) ;
#5996=CARTESIAN_POINT ( 'NONE',  ( 2.241608896736428047, -4.786620604624113540, 33.94971097300155805 ) ) ;
#5997=CARTESIAN_POINT ( 'NONE',  ( -6.130147209438218781, -12.45813303252208648, 30.39737893381572675 ) ) ;
#5999=CARTESIAN_POINT ( 'NONE',  ( 15.23076923076911093, -5.219633306517616589, 34.19971097300220464 ) ) ;
#6000=ADVANCED_FACE ( 'NONE', ( #18517 ), #40133, .F. ) ;
#6001=CARTESIAN_POINT ( 'NONE',  ( 6.222779541268411485, -12.24180327182771855, 31.33663988360758168 ) ) ;
#6002=CARTESIAN_POINT ( 'NONE',  ( 1.384615384615386802, -8.564572088678739092, 35.78748833219616898 ) ) ;
#6003=CYLINDRICAL_SURFACE ( 'NONE', #69535, 0.2499999999999997502 ) ;
#6004=CYLINDRICAL_SURFACE ( 'NONE', #72537, 0.2499999999999979738 ) ;
#6005=CARTESIAN_POINT ( 'NONE',  ( -4.854143407945010757, -11.60474049983371003, 33.02348890104160262 ) ) ;
#6006=ORIENTED_EDGE ( 'NONE', *, *, #69682, .T. ) ;
#6007=VERTEX_POINT ( 'NONE', #5890 ) ;
#6008=EDGE_LOOP ( 'NONE', ( #11268, #77406 ) ) ;
#6009=CARTESIAN_POINT ( 'NONE',  ( -11.78848477575450282, -12.43535235679832596, 30.55408501211184813 ) ) ;
#6011=CARTESIAN_POINT ( 'NONE',  ( -3.100243792535585907, -10.31582465632705237, 34.18122507451815295 ) ) ;
#6012=CARTESIAN_POINT ( 'NONE',  ( -5.776988648387149539, -3.587049720035815348, 32.86302985866382897 ) ) ;
#6013=CARTESIAN_POINT ( 'NONE',  ( -13.38461538461550582, -8.613356846316285953, 34.62446782046622218 ) ) ;
#6015=FACE_BOUND ( 'NONE', #82561, .T. ) ;
#6016=VERTEX_POINT ( 'NONE', #41007 ) ;
#6017=CYLINDRICAL_SURFACE ( 'NONE', #63395, 0.2500000000000009437 ) ;
#6018=CARTESIAN_POINT ( 'NONE',  ( -3.296039231325550212, -3.643525952247789412, 33.31231777344662959 ) ) ;
#6019=EDGE_LOOP ( 'NONE', ( #27780, #74664, #15185, #9682 ) ) ;
#6020=CARTESIAN_POINT ( 'NONE',  ( 17.32697749683652688, -5.642605341092955307, 34.66089969410670335 ) ) ;
#6021=ORIENTED_EDGE ( 'NONE', *, *, #44175, .T. ) ;
#6022=FACE_BOUND ( 'NONE', #13822, .T. ) ;
#6023=CARTESIAN_POINT ( 'NONE',  ( -10.61538461538461320, -2.833524468853757305, 32.15551576947925838 ) ) ;
#6026=EDGE_LOOP ( 'NONE', ( #81850, #78827 ) ) ;
#6028=CARTESIAN_POINT ( 'NONE',  ( -12.52762084089859584, -11.91647553114624181, 32.58852847137148245 ) ) ;
#6029=CYLINDRICAL_SURFACE ( 'NONE', #52230, 0.2500000000000008882 ) ;
#6030=ORIENTED_EDGE ( 'NONE', *, *, #46375, .T. ) ;
#6031=CARTESIAN_POINT ( 'NONE',  ( 6.673100192134570285, -9.943427161483782584, 34.11278801902876978 ) ) ;
#6032=CARTESIAN_POINT ( 'NONE',  ( -7.715363405186894674, -8.191423895709840863, 34.95447573519442130 ) ) ;
#6033=CARTESIAN_POINT ( 'NONE',  ( 12.59233026936325039, -6.413143153341454017, 34.63066358083362672 ) ) ;
#6034=CARTESIAN_POINT ( 'NONE',  ( -8.096130577096197101, -2.779195860258146578, 31.39871582349836032 ) ) ;
#6035=ORIENTED_EDGE ( 'NONE', *, *, #74689, .T. ) ;
#6037=CARTESIAN_POINT ( 'NONE',  ( 4.826923076923076650, -7.500000000000001776, 35.04278698407183867 ) ) ;
#6038=CARTESIAN_POINT ( 'NONE',  ( 5.076923076923075762, -1.242168528481310874, 33.36296068462461051 ) ) ;
#6040=CARTESIAN_POINT ( 'NONE',  ( 18.24994551834813805, -6.696923467548659303, 34.68552623307873972 ) ) ;
#6042=CARTESIAN_POINT ( 'NONE',  ( 0.5267936010512995759, -11.06231777344671130, 33.60647404775212976 ) ) ;
#6043=FACE_OUTER_BOUND ( 'NONE', #22470, .T. ) ;
#6044=CARTESIAN_POINT ( 'NONE',  ( -15.90390063549801347, -4.336752205174650321, 33.62275283266504289 ) ) ;
#6045=CARTESIAN_POINT ( 'NONE',  ( 15.10007862765892206, -5.496505350115501010, 34.60290016733514307 ) ) ;
#6046=CARTESIAN_POINT ( 'NONE',  ( 0.7114838709165038910, -11.56426240980093567, 33.07394671870546432 ) ) ;
#6047=CARTESIAN_POINT ( 'NONE',  ( -2.307692307691999289, -2.506253911140615021, 30.00000000000323297 ) ) ;
#6050=VERTEX_POINT ( 'NONE', #81556 ) ;
#6051=CARTESIAN_POINT ( 'NONE',  ( 4.853996118016224770, -6.459968553980839800, 34.89616026154728701 ) ) ;
#6052=VERTEX_POINT ( 'NONE', #13088 ) ;
#6053=ORIENTED_EDGE ( 'NONE', *, *, #22052, .F. ) ;
#6054=CARTESIAN_POINT ( 'NONE',  ( 3.230769230769231726, -2.708943851104267164, 35.45975837776705220 ) ) ;
#6055=VERTEX_POINT ( 'NONE', #19842 ) ;
#6056=CARTESIAN_POINT ( 'NONE',  ( -1.384615384615506484, -2.657715359629662544, 31.77849191805970364 ) ) ;
#6059=CARTESIAN_POINT ( 'NONE',  ( 5.869308533332445066, -11.18331474514187995, 33.13161551792790505 ) ) ;
#6060=CARTESIAN_POINT ( 'NONE',  ( -3.099977422944443006, -8.999086150933472084, 34.52020707165672064 ) ) ;
#6061=DIRECTION ( 'NONE',  ( -0.000000000000000000, -0.6427876096865404731, -0.7660444431189770143 ) ) ;
#6063=CARTESIAN_POINT ( 'NONE',  ( -11.60454494941741999, -4.786620604624113540, 33.94971097300155805 ) ) ;
#6068=LINE ( 'NONE', #88069, #1715 ) ;
#6070=CARTESIAN_POINT ( 'NONE',  ( 5.933917620639865831, -3.322132147404559976, 32.92929555188719348 ) ) ;
#6071=ORIENTED_EDGE ( 'NONE', *, *, #67894, .T. ) ;
#6072=VERTEX_POINT ( 'NONE', #13526 ) ;
#6073=CARTESIAN_POINT ( 'NONE',  ( -9.692307692307691624, -3.513871655860378418, 32.76840700105978499 ) ) ;
#6074=CARTESIAN_POINT ( 'NONE',  ( 15.29602437028206907, -12.16647553114626490, 32.15551576947920864 ) ) ;
#6075=CARTESIAN_POINT ( 'NONE',  ( -6.792551484843279752, -12.15418822224088657, 32.17964115625579069 ) ) ;
#6076=CARTESIAN_POINT ( 'NONE',  ( -15.90379184220783948, -12.41262288849542017, 30.68299917996395010 ) ) ;
#6077=ADVANCED_FACE ( 'NONE', ( #32464 ), #25716, .F. ) ;
#6078=CARTESIAN_POINT ( 'NONE',  ( -24.00000000000000000, -5.499999999999981348, 27.25000000000000000 ) ) ;
#6079=CARTESIAN_POINT ( 'NONE',  ( 24.00000000000000000, -9.499999999999982236, 27.74999999999999645 ) ) ;
#6080=DIRECTION ( 'NONE',  ( 1.000000000000000000, 0.000000000000000000, 0.000000000000000000 ) ) ;
#6081=ADVANCED_FACE ( 'NONE', ( #82000 ), #20293, .F. ) ;
#6082=ORIENTED_EDGE ( 'NONE', *, *, #88861, .F. ) ;
#6083=CARTESIAN_POINT ( 'NONE',  ( 17.07692307692295586, -3.835265460704628815, 33.15142922262033665 ) ) ;
#6084=ORIENTED_EDGE ( 'NONE', *, *, #66703, .T. ) ;
#6085=ORIENTED_EDGE ( 'NONE', *, *, #46754, .F. ) ;
#6086=AXIS2_PLACEMENT_3D ( 'NONE', #32389, #59414, #73374 ) ;
#6087=CARTESIAN_POINT ( 'NONE',  ( 7.846153846153846700, -13.57706302396349152, 30.56769352161908060 ) ) ;
#6088=DIRECTION ( 'NONE',  ( -0.000000000000000000, 0.6427876096865404731, -0.7660444431189771253 ) ) ;
#6089=CARTESIAN_POINT ( 'NONE',  ( 11.66925334628632527, -10.54018710029568595, 33.71981072465678864 ) ) ;
#6090=CARTESIAN_POINT ( 'NONE',  ( 4.087763774486018242, -6.343179335718451384, 34.87096338111212646 ) ) ;
#6091=CARTESIAN_POINT ( 'NONE',  ( 11.53846153846153832, -13.75783147151868846, 33.36296068462461051 ) ) ;
#6092=AXIS2_PLACEMENT_3D ( 'NONE', #84847, #51012, #50589 ) ;
#6093=EDGE_LOOP ( 'NONE', ( #1858, #68731, #53604, #13435 ) ) ;
#6094=EDGE_LOOP ( 'NONE', ( #72840, #31198 ) ) ;
#6095=B_SPLINE_CURVE_WITH_KNOTS ( 'NONE', 3,
 ( #40375, #19209, #39047, #80018, #33161, #52091, #45333, #53875, #32710, #67391 ),
 .UNSPECIFIED., .F., .F.,
 ( 4, 2, 2, 2, 4 ),
 ( 0.0007817246256747517261, 0.0009771112852218961399, 0.001172497944769040771, 0.001367884604316185401, 0.001563271263863329815 ),
 .UNSPECIFIED. ) ;
#6096=EDGE_CURVE ( 'NONE', #12296, #43958, #55397, .T. ) ;
#6097=EDGE_CURVE ( 'NONE', #58471, #7620, #5432, .T. ) ;
#6098=ORIENTED_EDGE ( 'NONE', *, *, #39397, .F. ) ;
#6099=ORIENTED_EDGE ( 'NONE', *, *, #77450, .T. ) ;
#6100=LINE ( 'NONE', #26809, #6987 ) ;
#6102=CARTESIAN_POINT ( 'NONE',  ( 14.24242230713598723, -2.657715359629088780, 31.77849191805832874 ) ) ;
#6103=CARTESIAN_POINT ( 'NONE',  ( 16.28437185560971656, -10.19071101563364401, 33.96452234770658407 ) ) ;
#6104=CARTESIAN_POINT ( 'NONE',  ( -16.15384615384615330, -3.322132147404559976, 32.92929555188717927 ) ) ;
#6105=CARTESIAN_POINT ( 'NONE',  ( 14.30769230769231015, -12.37446782046654192, 30.86335684631486131 ) ) ;
#6106=ORIENTED_EDGE ( 'NONE', *, *, #20185, .T. ) ;
#6107=ORIENTED_EDGE ( 'NONE', *, *, #34999, .F. ) ;
#6108=EDGE_LOOP ( 'NONE', ( #82918, #3739, #85509, #73785 ) ) ;
#6109=CARTESIAN_POINT ( 'NONE',  ( 17.14299142792551578, -12.37446782046654192, 30.86335684631486842 ) ) ;
#6110=EDGE_LOOP ( 'NONE', ( #57144, #47599, #41354, #18356 ) ) ;
#6111=DIRECTION ( 'NONE',  ( 0.000000000000000000, 0.8660254037844377084, 0.5000000000000015543 ) ) ;
#6113=AXIS2_PLACEMENT_3D ( 'NONE', #20540, #35840, #75932 ) ;
#6116=CARTESIAN_POINT ( 'NONE',  ( -2.980823712421087901, -12.43552623307873972, 30.55307653245132826 ) ) ;
#6117=ORIENTED_EDGE ( 'NONE', *, *, #74086, .F. ) ;
#6118=CYLINDRICAL_SURFACE ( 'NONE', #41320, 0.2499999999999973355 ) ;
#6119=FACE_BOUND ( 'NONE', #67032, .T. ) ;
#6120=CYLINDRICAL_SURFACE ( 'NONE', #66181, 0.2499999999999979738 ) ;
#6122=EDGE_LOOP ( 'NONE', ( #15540, #30793, #86613, #83352 ) ) ;
#6123=CARTESIAN_POINT ( 'NONE',  ( 5.076923076923075762, -13.75783147151868846, 33.36296068462461051 ) ) ;
#6124=B_SPLINE_CURVE_WITH_KNOTS ( 'NONE', 3,
 ( #4451, #26510, #66609, #53524, #67500, #28156, #59400, #86902, #48872, #53973 ),
 .UNSPECIFIED., .F., .F.,
 ( 4, 2, 2, 2, 4 ),
 ( 0.0007817246256747495577, 0.0009771112852218935378, 0.001172497944769037518, 0.001367884604316181715, 0.001563271263863325695 ),
 .UNSPECIFIED. ) ;
#6125=CARTESIAN_POINT ( 'NONE',  ( 15.23076923076923173, -6.343179335718451384, 34.87096338111211935 ) ) ;
#6126=EDGE_LOOP ( 'NONE', ( #69156, #87071, #7183, #82131 ) ) ;
#6127=B_SPLINE_CURVE_WITH_KNOTS ( 'NONE', 3,
 ( #67250, #31691, #58256, #65464, #38443, #79433, #74011, #32132, #59594, #53276 ),
 .UNSPECIFIED., .F., .F.,
 ( 4, 2, 2, 2, 4 ),
 ( 0.000000000000000000, 0.0001954311564186867389, 0.0003908623128373734778, 0.0005862934692560602167, 0.0007817246256747469556 ),
 .UNSPECIFIED. ) ;
#6128=LINE ( 'NONE', #73713, #57389 ) ;
#6129=CARTESIAN_POINT ( 'NONE',  ( 1.384615384615386802, -8.120952969808772792, 34.71129190930000163 ) ) ;
#6130=CARTESIAN_POINT ( 'NONE',  ( -6.923076923076922462, -6.343179335718451384, 34.87096338111211935 ) ) ;
#6131=DIRECTION ( 'NONE',  ( -0.000000000000000000, -0.7660444431189791237, -0.6427876096865379196 ) ) ;
#6132=DIRECTION ( 'NONE',  ( -0.000000000000000000, -0.5000000000000009992, -0.8660254037844380415 ) ) ;
#6133=FACE_BOUND ( 'NONE', #13512, .T. ) ;
#6136=DIRECTION ( 'NONE',  ( -0.000000000000000000, -0.5000000000000009992, -0.8660254037844380415 ) ) ;
#6137=CARTESIAN_POINT ( 'NONE',  ( -5.999999999999998224, -9.780366693483667717, 34.19971097300155094 ) ) ;
#6138=CARTESIAN_POINT ( 'NONE',  ( -2.176901866725356349, -8.191423895709840863, 34.95447573519442130 ) ) ;
#6139=CARTESIAN_POINT ( 'NONE',  ( 9.019176178608812933, -12.68172785388650681, 30.59649109432439218 ) ) ;
#6141=VERTEX_POINT ( 'NONE', #77440 ) ;
#6142=AXIS2_PLACEMENT_3D ( 'NONE', #69408, #49129, #28415 ) ;
#6143=CARTESIAN_POINT ( 'NONE',  ( -8.519176457592452678, -5.728107161865378494, 34.42597550085002922 ) ) ;
#6144=ORIENTED_EDGE ( 'NONE', *, *, #74043, .F. ) ;
#6145=VECTOR ( 'NONE', #64443, 1000.000000000000227 ) ;
#6146=CARTESIAN_POINT ( 'NONE',  ( 1.319364394454144440, -2.506253911140460922, 30.00000000000013856 ) ) ;
#6149=CARTESIAN_POINT ( 'NONE',  ( -2.057692307692306599, -7.500000000000001776, 35.04278698407183867 ) ) ;
#6150=CARTESIAN_POINT ( 'NONE',  ( -9.692307692307691624, -12.37446782046654192, 30.86335684631486131 ) ) ;
#6151=ORIENTED_EDGE ( 'NONE', *, *, #64435, .T. ) ;
#6152=CARTESIAN_POINT ( 'NONE',  ( -11.53846153846153655, -2.721908614388771852, 31.22303859784724978 ) ) ;
#6153=CARTESIAN_POINT ( 'NONE',  ( 0.4615384615384611200, -12.62096338111211580, 30.90682066428153263 ) ) ;
#6155=CARTESIAN_POINT ( 'NONE',  ( 4.284371855609718338, -10.88167719472716399, 33.43325721877153711 ) ) ;
#6156=CARTESIAN_POINT ( 'NONE',  ( 4.946231610255517275, -4.809359713505814149, 33.96456829005828837 ) ) ;
#6157=CARTESIAN_POINT ( 'NONE',  ( 2.307692307692309264, -2.486705287966279876, 31.30864560766543647 ) ) ;
#6158=CARTESIAN_POINT ( 'NONE',  ( 1.253924781505077801, -4.684245665217972032, 34.18127051446801090 ) ) ;
#6159=CYLINDRICAL_SURFACE ( 'NONE', #38239, 0.2500000000000008882 ) ;
#6160=ADVANCED_FACE ( 'NONE', ( #14412 ), #463, .F. ) ;
#6161=CARTESIAN_POINT ( 'NONE',  ( 9.561617089197383734, -3.338472653186243644, 32.95098750199972670 ) ) ;
#6162=EDGE_CURVE ( 'NONE', #59859, #33344, #50909, .T. ) ;
#6164=CARTESIAN_POINT ( 'NONE',  ( 9.442307692307693401, -7.566083408709835645, 34.74999999999999289 ) ) ;
#6165=DIRECTION ( 'NONE',  ( 0.000000000000000000, 0.8660254037844377084, 0.5000000000000015543 ) ) ;
#6166=ORIENTED_EDGE ( 'NONE', *, *, #15177, .T. ) ;
#6167=CARTESIAN_POINT ( 'NONE',  ( 7.146503321991712454, -7.630147987733840509, 34.99859428049665411 ) ) ;
#6170=B_SPLINE_CURVE_WITH_KNOTS ( 'NONE', 3,
 ( #16570, #44034, #71074, #10267, #58887, #9382, #71507, #64302, #2603, #51212 ),
 .UNSPECIFIED., .F., .F.,
 ( 4, 2, 2, 2, 4 ),
 ( 0.000000000000000000, 0.0001954311564186870099, 0.0003908623128373740199, 0.0005862934692560609756, 0.0007817246256747480398 ),
 .UNSPECIFIED. ) ;
#6171=DIRECTION ( 'NONE',  ( -0.000000000000000000, -0.1736481776669307198, -0.9848077530122080203 ) ) ;
#6172=CARTESIAN_POINT ( 'NONE',  ( 17.29993442853592711, -11.76359900205217457, 32.36225158514719880 ) ) ;
#6173=VERTEX_POINT ( 'NONE', #84220 ) ;
#6174=CYLINDRICAL_SURFACE ( 'NONE', #85949, 0.2500000000000002220 ) ;
#6175=CARTESIAN_POINT ( 'NONE',  ( -17.01085574357299990, -9.058645607665452459, 34.76329471203371924 ) ) ;
#6176=CARTESIAN_POINT ( 'NONE',  ( 10.36538461538461675, -7.500000000000001776, 35.00000000000000000 ) ) ;
#6177=EDGE_LOOP ( 'NONE', ( #79473, #64330 ) ) ;
#6178=FACE_OUTER_BOUND ( 'NONE', #49006, .T. ) ;
#6179=ADVANCED_FACE ( 'NONE', ( #62587 ), #35578, .F. ) ;
#6180=B_SPLINE_CURVE_WITH_KNOTS ( 'NONE', 3,
 ( #2727, #84738, #83850, #63553, #23014, #62658, #35654, #8629, #1857, #29341 ),
 .UNSPECIFIED., .F., .F.,
 ( 4, 2, 2, 2, 4 ),
 ( 0.000000000000000000, 0.0001954339857564073388, 0.0003908679715128146777, 0.0005863019572692220165, 0.0007817359430256293554 ),
 .UNSPECIFIED. ) ;
#6181=CARTESIAN_POINT ( 'NONE',  ( 5.011169648609741678, -7.249945578846651806, 34.99404164642496795 ) ) ;
#6182=CARTESIAN_POINT ( 'NONE',  ( -12.68502338610279523, -4.988325925672468131, 34.36044203135681130 ) ) ;
#6183=AXIS2_PLACEMENT_3D ( 'NONE', #60113, #46168, #80856 ) ;
#6184=ORIENTED_EDGE ( 'NONE', *, *, #63808, .T. ) ;
#6185=VECTOR ( 'NONE', #83185, 1000.000000000000000 ) ;
#6186=CARTESIAN_POINT ( 'NONE',  ( 2.177001704581999153, -3.957541250942359756, 33.62499894934981626 ) ) ;
#6187=CARTESIAN_POINT ( 'NONE',  ( -13.38461538461538325, -11.69971097300155272, 32.46337939537588113 ) ) ;
#6188=CARTESIAN_POINT ( 'NONE',  ( 2.307692307692309264, -8.164416787775445883, 34.95778746994557906 ) ) ;
#6189=ADVANCED_FACE ( 'NONE', ( #1780 ), #55837, .F. ) ;
#6190=EDGE_LOOP ( 'NONE', ( #65881, #37152 ) ) ;
#6191=ORIENTED_EDGE ( 'NONE', *, *, #10250, .F. ) ;
#6192=ORIENTED_EDGE ( 'NONE', *, *, #17038, .F. ) ;
#6193=ORIENTED_EDGE ( 'NONE', *, *, #59556, .F. ) ;
#6194=CARTESIAN_POINT ( 'NONE',  ( 0.3962680155776852065, -8.613356846314824011, 34.62446782046655613 ) ) ;
#6195=CARTESIAN_POINT ( 'NONE',  ( 14.24160889673642849, -4.098570777380720287, 33.41473453929634729 ) ) ;
#6196=CARTESIAN_POINT ( 'NONE',  ( -16.37733107841048508, -3.019605429927187501, 32.48692288466676814 ) ) ;
#6198=CARTESIAN_POINT ( 'NONE',  ( -18.25000000000000355, -7.500000000000000000, 35.00000000000000000 ) ) ;
#6199=EDGE_LOOP ( 'NONE', ( #31704, #58187 ) ) ;
#6200=EDGE_CURVE ( 'NONE', #3325, #1602, #52997, .T. ) ;
#6201=EDGE_LOOP ( 'NONE', ( #68130, #39645, #7697, #46448 ) ) ;
#6202=B_SPLINE_CURVE_WITH_KNOTS ( 'NONE', 3,
 ( #60314, #47243, #20228, #67971, #81049, #39626, #4942, #67083, #40072, #26094 ),
 .UNSPECIFIED., .F., .F.,
 ( 4, 2, 2, 2, 4 ),
 ( 0.000000000000000000, 0.0001954339857564083688, 0.0003908679715128167377, 0.0005863019572692250523, 0.0007817359430256334753 ),
 .UNSPECIFIED. ) ;
#6203=ORIENTED_EDGE ( 'NONE', *, *, #53113, .F. ) ;
#6204=CYLINDRICAL_SURFACE ( 'NONE', #19976, 0.2500000000000008882 ) ;
#6205=EDGE_CURVE ( 'NONE', #30718, #38938, #16478, .T. ) ;
#6207=B_SPLINE_CURVE_WITH_KNOTS ( 'NONE', 3,
 ( #68958, #35628, #35175, #945, #34284, #62633, #55443, #82928, #21659, #7266 ),
 .UNSPECIFIED., .F., .F.,
 ( 4, 2, 2, 2, 4 ),
 ( 0.000000000000000000, 0.0001954311564186864949, 0.0003908623128373729899, 0.0005862934692560594577, 0.0007817246256747459798 ),
 .UNSPECIFIED. ) ;
#6208=CARTESIAN_POINT ( 'NONE',  ( 4.219914504848592429, -5.557115091759786019, 34.35708131394839882 ) ) ;
#6209=B_SPLINE_CURVE_WITH_KNOTS ( 'NONE', 3,
 ( #28248, #14297, #21492, #6225, #27376, #55280, #54842, #82769, #21044, #53953 ),
 .UNSPECIFIED., .F., .F.,
 ( 4, 2, 2, 2, 4 ),
 ( 0.000000000000000000, 0.0001954311564186867660, 0.0003908623128373735320, 0.0005862934692560603251, 0.0007817246256747470640 ),
 .UNSPECIFIED. ) ;
#6210=DIRECTION ( 'NONE',  ( 0.000000000000000000, 1.000000000000000000, 0.000000000000000000 ) ) ;
#6211=AXIS2_PLACEMENT_3D ( 'NONE', #29179, #84561, #8007 ) ;
#6213=EDGE_CURVE ( 'NONE', #7402, #39647, #18727, .T. ) ;
#6214=EDGE_CURVE ( 'NONE', #7653, #37364, #52042, .T. ) ;
#6217=ORIENTED_EDGE ( 'NONE', *, *, #7602, .T. ) ;
#6218=VECTOR ( 'NONE', #33444, 1000.000000000000000 ) ;
#6219=ORIENTED_EDGE ( 'NONE', *, *, #31118, .F. ) ;
#6221=LINE ( 'NONE', #25594, #20237 ) ;
#6222=DIRECTION ( 'NONE',  ( -0.000000000000000000, 0.8660254037844399289, -0.4999999999999980016 ) ) ;
#6223=ORIENTED_EDGE ( 'NONE', *, *, #72660, .F. ) ;
#6224=CARTESIAN_POINT ( 'NONE',  ( 9.627037246346915822, -11.94971097300153140, 32.03036669348370680 ) ) ;
#6225=CARTESIAN_POINT ( 'NONE',  ( -0.6844654204453101132, -6.459968553980839800, 34.89616026154728701 ) ) ;
#6227=CYLINDRICAL_SURFACE ( 'NONE', #79111, 0.2499999999999995559 ) ;
#6228=CARTESIAN_POINT ( 'NONE',  ( 16.40390046548447245, -3.627508038966690496, 32.91356715214248396 ) ) ;
#6229=CARTESIAN_POINT ( 'NONE',  ( 4.153846153846154188, -2.721908614388771852, 31.22303859784724978 ) ) ;
#6230=FACE_BOUND ( 'NONE', #4445, .T. ) ;
#6231=CARTESIAN_POINT ( 'NONE',  ( -17.74994568836168440, -8.303483539816726378, 34.68545999027711702 ) ) ;
#6232=B_SPLINE_CURVE_WITH_KNOTS ( 'NONE', 3,
 ( #63713, #28612, #56075, #83569, #76802, #42571, #56521, #70031, #43009, #8341 ),
 .UNSPECIFIED., .F., .F.,
 ( 4, 2, 2, 2, 4 ),
 ( 0.0007817246336856289524, 0.0009771112958940101571, 0.001172497958102391253, 0.001367884620310772350, 0.001563271282519153446 ),
 .UNSPECIFIED. ) ;
#6233=CARTESIAN_POINT ( 'NONE',  ( -1.161604033002534120, -11.76359900205217457, 32.36225158514719880 ) ) ;
#6234=CARTESIAN_POINT ( 'NONE',  ( 12.23861150263161157, -6.459968553980841577, 34.89616026154728701 ) ) ;
#6235=CARTESIAN_POINT ( 'NONE',  ( -23.00000000000000000, -7.500000000000000000, 29.75000000000000355 ) ) ;
#6236=CARTESIAN_POINT ( 'NONE',  ( -0.5922299282060162762, -12.11776431015575994, 31.66791131148498906 ) ) ;
#6238=CARTESIAN_POINT ( 'NONE',  ( -4.153846153846274980, -11.67786785259630911, 32.92929555188603530 ) ) ;
#6239=EDGE_LOOP ( 'NONE', ( #53272, #79400, #16735, #4877 ) ) ;
#6240=CARTESIAN_POINT ( 'NONE',  ( 2.307692307692187583, -6.879047030192662504, 34.71129190930017927 ) ) ;
#6241=CARTESIAN_POINT ( 'NONE',  ( -7.846153846153537614, -2.506253911140614576, 30.00000000000323297 ) ) ;
#6243=CARTESIAN_POINT ( 'NONE',  ( -6.792285115252136407, -4.809403383903225304, 33.96459661697924304 ) ) ;
#6246=CARTESIAN_POINT ( 'NONE',  ( -13.63463860883683942, -4.931416488878822335, 34.32920672191015399 ) ) ;
#6247=DIRECTION ( 'NONE',  ( 0.000000000000000000, 0.3420201433256641055, -0.9396926207859100932 ) ) ;
#6248=VERTEX_POINT ( 'NONE', #57168 ) ;
#6249=ADVANCED_FACE ( 'NONE', ( #57608 ), #72895, .F. ) ;
#6250=CARTESIAN_POINT ( 'NONE',  ( -11.53846153846153655, -12.29105614889573062, 35.45975837776705220 ) ) ;
#6251=CARTESIAN_POINT ( 'NONE',  ( 6.923076923076800782, -8.656820664282941280, 34.87096338111179961 ) ) ;
#6252=FACE_BOUND ( 'NONE', #38843, .T. ) ;
#6253=CARTESIAN_POINT ( 'NONE',  ( 11.53846153846184563, -2.506253911140615021, 30.00000000000323297 ) ) ;
#6254=CARTESIAN_POINT ( 'NONE',  ( -16.82692307692307665, -2.249999999999998668, 29.75000000000000355 ) ) ;
#6255=CARTESIAN_POINT ( 'NONE',  ( -8.992715712954719720, -6.760086850603066466, 34.69517049084099369 ) ) ;
#6256=CARTESIAN_POINT ( 'NONE',  ( -5.143006487878955646, -8.973038597847269315, 34.52809138561120506 ) ) ;
#6258=CARTESIAN_POINT ( 'NONE',  ( -8.546219417617917813, -12.15243808032446005, 31.58219941686247978 ) ) ;
#6260=ORIENTED_EDGE ( 'NONE', *, *, #59532, .F. ) ;
#6263=CARTESIAN_POINT ( 'NONE',  ( -4.219116599806928214, -12.46129190929999986, 30.37095296980880832 ) ) ;
#6264=CARTESIAN_POINT ( 'NONE',  ( 16.40379156322419973, -2.986452184633680229, 32.43230066228895225 ) ) ;
#6265=CARTESIAN_POINT ( 'NONE',  ( -0.5272952640527707180, -7.249945686854186278, 34.74374336980224598 ) ) ;
#6266=CARTESIAN_POINT ( 'NONE',  ( -3.360916440207450506, -6.001485441113818986, 34.52039167877662607 ) ) ;
#6268=EDGE_CURVE ( 'NONE', #28219, #23488, #34828, .T. ) ;
#6270=CARTESIAN_POINT ( 'NONE',  ( 8.769230769230768274, -2.833524468853757305, 32.15551576947925838 ) ) ;
#6271=CARTESIAN_POINT ( 'NONE',  ( 17.93391762063986405, -3.937682226553330445, 33.60647404775217240 ) ) ;
#6272=CARTESIAN_POINT ( 'NONE',  ( -15.09997742294444301, -11.18335022499818621, 33.13157742990016885 ) ) ;
#6273=DIRECTION ( 'NONE',  ( -0.000000000000000000, 0.9396926207859092051, -0.3420201433256662704 ) ) ;
#6274=CARTESIAN_POINT ( 'NONE',  ( 13.38461538461526601, -4.481592998941358097, 33.73612834414048933 ) ) ;
#6275=LINE ( 'NONE', #54445, #45213 ) ;
#6276=B_SPLINE_CURVE_WITH_KNOTS ( 'NONE', 3,
 ( #80980, #39556, #88196, #53933, #74662, #12948, #40440, #13388, #67898, #48051 ),
 .UNSPECIFIED., .F., .F.,
 ( 4, 2, 2, 2, 4 ),
 ( 0.0007817359430256282712, 0.0009771253907249941549, 0.001172514838424359822, 0.001367904286123725489, 0.001563293733823091372 ),
 .UNSPECIFIED. ) ;
#6277=CARTESIAN_POINT ( 'NONE',  ( -8.769230769230768274, -13.95598074871891292, 31.83374038241031911 ) ) ;
#6278=CARTESIAN_POINT ( 'NONE',  ( 4.403846153846153300, -2.249999999999998668, 29.75000000000000355 ) ) ;
#6279=ORIENTED_EDGE ( 'NONE', *, *, #33882, .F. ) ;
#6280=CARTESIAN_POINT ( 'NONE',  ( 1.134592147322422084, -2.587272538249755449, 30.68239716806877837 ) ) ;
#6285=EDGE_CURVE ( 'NONE', #9213, #27850, #87501, .T. ) ;
#6286=CARTESIAN_POINT ( 'NONE',  ( 3.930361229281821966, -4.988325925672468131, 34.36044203135681130 ) ) ;
#6287=CARTESIAN_POINT ( 'NONE',  ( -12.46153846153846168, -11.11383981884818262, 36.00935417666054406 ) ) ;
#6288=CYLINDRICAL_SURFACE ( 'NONE', #3958, 0.2500000000000008882 ) ;
#6289=CARTESIAN_POINT ( 'NONE',  ( -1.134669866267242311, -4.336752205174647656, 33.62275283266504289 ) ) ;
#6290=ORIENTED_EDGE ( 'NONE', *, *, #82822, .T. ) ;
#6292=CARTESIAN_POINT ( 'NONE',  ( -1.384615384615383471, -9.819645486525091727, 36.12317359536749706 ) ) ;
#6293=EDGE_CURVE ( 'NONE', #66691, #54559, #26222, .T. ) ;
#6294=ORIENTED_EDGE ( 'NONE', *, *, #81115, .T. ) ;
#6295=CARTESIAN_POINT ( 'NONE',  ( -15.90379184220783948, -9.943054286541403997, 34.11300777759954883 ) ) ;
#6296=CARTESIAN_POINT ( 'NONE',  ( -2.307692307692427391, -2.625532179533779154, 30.86335684631627174 ) ) ;
#6297=ORIENTED_EDGE ( 'NONE', *, *, #14711, .T. ) ;
#6298=CARTESIAN_POINT ( 'NONE',  ( 7.715462379486291766, -4.118384482072085184, 33.43331474514187107 ) ) ;
#6299=CARTESIAN_POINT ( 'NONE',  ( -15.09993090028246954, -7.277220318596961057, 34.99547417642776992 ) ) ;
#6300=CARTESIAN_POINT ( 'NONE',  ( -8.069638789877796370, -3.754499324213721234, 33.06261337010820256 ) ) ;
#6301=EDGE_CURVE ( 'NONE', #19438, #79333, #46632, .T. ) ;
#6302=ORIENTED_EDGE ( 'NONE', *, *, #68492, .T. ) ;
#6303=VERTEX_POINT ( 'NONE', #24712 ) ;
#6304=ORIENTED_EDGE ( 'NONE', *, *, #81061, .F. ) ;
#6305=EDGE_CURVE ( 'NONE', #56065, #57354, #11655, .T. ) ;
#6306=CARTESIAN_POINT ( 'NONE',  ( 7.623226887246995709, -9.172386477786396597, 34.72672124145550043 ) ) ;
#6307=CARTESIAN_POINT ( 'NONE',  ( 7.145856592054987466, -11.60474049983371003, 33.02348890104160262 ) ) ;
#6308=CARTESIAN_POINT ( 'NONE',  ( 0.4615384615384611200, -13.87047571288749737, 32.06866353760679544 ) ) ;
#6309=CARTESIAN_POINT ( 'NONE',  ( -12.46153846153858247, -3.300289026999228881, 32.46337939537708905 ) ) ;
#6310=ADVANCED_FACE ( 'NONE', ( #25156 ), #67486, .F. ) ;
#6311=CARTESIAN_POINT ( 'NONE',  ( -2.307692307692305711, -4.098570777380720287, 33.41473453929634729 ) ) ;
#6312=CYLINDRICAL_SURFACE ( 'NONE', #16247, 0.2499999999999973355 ) ;
#6313=CARTESIAN_POINT ( 'NONE',  ( 13.38461538461526601, -3.300289026999228881, 32.46337939537708905 ) ) ;
#6314=B_SPLINE_CURVE_WITH_KNOTS ( 'NONE', 3,
 ( #19825, #26137, #53606, #68885, #81096, #19381, #46849, #7199, #74780, #68020 ),
 .UNSPECIFIED., .F., .F.,
 ( 4, 2, 2, 2, 4 ),
 ( 0.0007817246256747484735, 0.0009771112852218915863, 0.001172497944769034916, 0.001367884604316178029, 0.001563271263863321141 ),
 .UNSPECIFIED. ) ;
#6315=VECTOR ( 'NONE', #34704, 999.9999999999998863 ) ;
#6316=CARTESIAN_POINT ( 'NONE',  ( -0.3310130233048143023, -12.50538340440932217, 31.33453814440721885 ) ) ;
#6317=B_SPLINE_CURVE_WITH_KNOTS ( 'NONE', 3,
 ( #50343, #14814, #41844, #1283, #28771, #76507, #56236, #83721, #34635, #22880 ),
 .UNSPECIFIED., .F., .F.,
 ( 4, 2, 2, 2, 4 ),
 ( 0.000000000000000000, 0.0001954311564186872268, 0.0003908623128373744536, 0.0005862934692560616261, 0.0007817246256747489071 ),
 .UNSPECIFIED. ) ;
#6318=EDGE_CURVE ( 'NONE', #7411, #38055, #78846, .T. ) ;
#6321=CARTESIAN_POINT ( 'NONE',  ( -1.634615384615383027, -7.500000000000001776, 34.75000000000000000 ) ) ;
#6325=LINE ( 'NONE', #68891, #21959 ) ;
#6326=CARTESIAN_POINT ( 'NONE',  ( 11.60452988946398101, -12.10708131394839704, 31.69288490824020954 ) ) ;
#6327=ORIENTED_EDGE ( 'NONE', *, *, #64020, .T. ) ;
#6328=CARTESIAN_POINT ( 'NONE',  ( 15.29683656411930848, -9.058645607665452459, 34.76329471203371924 ) ) ;
#6329=ORIENTED_EDGE ( 'NONE', *, *, #46955, .F. ) ;
#6330=CARTESIAN_POINT ( 'NONE',  ( 17.20744851515672025, -9.503571793651730104, 34.60286762892837942 ) ) ;
#6331=ORIENTED_EDGE ( 'NONE', *, *, #74672, .F. ) ;
#6332=CARTESIAN_POINT ( 'NONE',  ( -6.923076923076922462, -2.833524468853757305, 32.15551576947925838 ) ) ;
#6333=AXIS2_PLACEMENT_3D ( 'NONE', #9309, #16941, #16058 ) ;
#6334=ORIENTED_EDGE ( 'NONE', *, *, #66448, .T. ) ;
#6335=CARTESIAN_POINT ( 'NONE',  ( -12.46153846153858424, -10.33852847137269571, 34.16647553114546554 ) ) ;
#6336=EDGE_CURVE ( 'NONE', #43656, #27369, #8316, .T. ) ;
#6337=B_SPLINE_CURVE_WITH_KNOTS ( 'NONE', 3,
 ( #16180, #43645, #57605, #23368, #50826, #78311, #16611, #32361, #10754, #17961 ),
 .UNSPECIFIED., .F., .F.,
 ( 4, 2, 2, 2, 4 ),
 ( 0.0007817359430256372700, 0.0009771253907250054306, 0.001172514838424373483, 0.001367904286123741535, 0.001563293733823109804 ),
 .UNSPECIFIED. ) ;
#6338=CARTESIAN_POINT ( 'NONE',  ( 12.23805353697412812, -2.353723527008296568, 30.78948104536958752 ) ) ;
#6339=FACE_BOUND ( 'NONE', #60342, .T. ) ;
#6340=B_SPLINE_CURVE_WITH_KNOTS ( 'NONE', 3,
 ( #31969, #16663, #51763, #58981, #44565, #59433, #24759, #10806, #52221, #80158 ),
 .UNSPECIFIED., .F., .F.,
 ( 4, 2, 2, 2, 4 ),
 ( 0.0007817359430256257775, 0.0009771253907249906855, 0.001172514838424355485, 0.001367904286123720285, 0.001563293733823085301 ),
 .UNSPECIFIED. ) ;
#6342=CARTESIAN_POINT ( 'NONE',  ( 5.869309396889694774, -2.295517848115769421, 30.44137282052136939 ) ) ;
#6343=DIRECTION ( 'NONE',  ( -0.000000000000000000, -0.6427876096865404731, -0.7660444431189771253 ) ) ;
#6344=AXIS2_PLACEMENT_3D ( 'NONE', #18151, #51914, #51455 ) ;
#6346=CARTESIAN_POINT ( 'NONE',  ( 10.48523664565292179, -10.31621877034669588, 34.18098118002070152 ) ) ;
#6347=EDGE_CURVE ( 'NONE', #68662, #84581, #66924, .T. ) ;
#6348=DIRECTION ( 'NONE',  ( -0.000000000000000000, 0.1736481776669307198, -0.9848077530122080203 ) ) ;
#6350=CARTESIAN_POINT ( 'NONE',  ( -11.76138849736838488, -3.395401636524185474, 33.02366814457250399 ) ) ;
#6351=B_SPLINE_CURVE_WITH_KNOTS ( 'NONE', 3,
 ( #32325, #53917, #40420, #81405, #19688, #67880, #6182, #24668, #33651, #86396 ),
 .UNSPECIFIED., .F., .F.,
 ( 4, 2, 2, 2, 4 ),
 ( 0.000000000000000000, 0.0001954311564186871184, 0.0003908623128373742367, 0.0005862934692560614093, 0.0007817246256747484735 ),
 .UNSPECIFIED. ) ;
#6352=VERTEX_POINT ( 'NONE', #52622 ) ;
#6353=EDGE_LOOP ( 'NONE', ( #24009, #63196, #2003, #1314 ) ) ;
#6354=CARTESIAN_POINT ( 'NONE',  ( -17.01085472592063397, -9.780366693483667717, 34.19971097300155805 ) ) ;
#6355=CARTESIAN_POINT ( 'NONE',  ( 10.61538461538461675, -5.557115091759785130, 34.35708131394839171 ) ) ;
#6356=CARTESIAN_POINT ( 'NONE',  ( 16.40390057375960708, -11.47946981652013498, 33.17500667209846910 ) ) ;
#6357=CARTESIAN_POINT ( 'NONE',  ( -3.931066484868084299, -9.418065098278011860, 34.63729479722530158 ) ) ;
#6358=CARTESIAN_POINT ( 'NONE',  ( -17.32689982097166492, -12.41104346484419452, 31.60698883733904196 ) ) ;
#6360=EDGE_LOOP ( 'NONE', ( #254, #44849, #64413, #29279 ) ) ;
#6361=EDGE_CURVE ( 'NONE', #45648, #53485, #81895, .T. ) ;
#6362=CARTESIAN_POINT ( 'NONE',  ( -5.777220331021931443, -8.540255544307065350, 34.89611431652622286 ) ) ;
#6363=CARTESIAN_POINT ( 'NONE',  ( 14.05766907039934210, -11.37209801155882793, 32.91403422569033665 ) ) ;
#6364=CARTESIAN_POINT ( 'NONE',  ( -3.480745974817820887, -11.47974371597207899, 33.17467449705390692 ) ) ;
#6365=FACE_OUTER_BOUND ( 'NONE', #50860, .T. ) ;
#6366=EDGE_LOOP ( 'NONE', ( #3618, #3428 ) ) ;
#6367=EDGE_CURVE ( 'NONE', #76991, #72654, #40025, .T. ) ;
#6368=ORIENTED_EDGE ( 'NONE', *, *, #17546, .T. ) ;
#6370=EDGE_CURVE ( 'NONE', #50376, #23593, #19296, .T. ) ;
#6371=CARTESIAN_POINT ( 'NONE',  ( 10.61538461538449418, -4.320704448113951379, 33.92786785259630022 ) ) ;
#6372=ORIENTED_EDGE ( 'NONE', *, *, #31261, .T. ) ;
#6373=CARTESIAN_POINT ( 'NONE',  ( 17.07692307692307665, -12.78798330534102945, 29.74999999999997868 ) ) ;
#6374=CARTESIAN_POINT ( 'NONE',  ( -6.923076923077044142, -2.625532179533778709, 30.86335684631627174 ) ) ;
#6375=CARTESIAN_POINT ( 'NONE',  ( 3.453782074862625784, -5.582272713120728369, 34.63742843783360570 ) ) ;
#6377=EDGE_CURVE ( 'NONE', #219, #62136, #15408, .T. ) ;
#6378=CARTESIAN_POINT ( 'NONE',  ( -11.40766973063675316, -6.413143153341454017, 34.63066358083362672 ) ) ;
#6380=VERTEX_POINT ( 'NONE', #73805 ) ;
#6381=CARTESIAN_POINT ( 'NONE',  ( -11.66893672353726075, -7.276987145209185215, 34.99546412871779211 ) ) ;
#6382=CARTESIAN_POINT ( 'NONE',  ( -12.46153846153846168, -11.69971097300155272, 32.46337939537588113 ) ) ;
#6383=EDGE_LOOP ( 'NONE', ( #48624, #12280 ) ) ;
#6385=DIRECTION ( 'NONE',  ( -0.000000000000000000, -0.9848077530122086864, -0.1736481776669273613 ) ) ;
#6386=FACE_OUTER_BOUND ( 'NONE', #28320, .T. ) ;
#6387=CARTESIAN_POINT ( 'NONE',  ( 11.60371667797437567, -10.33852847137154107, 34.16647553114620450 ) ) ;
#6388=CARTESIAN_POINT ( 'NONE',  ( -9.692307692307814193, -12.51329471203414379, 31.30864560766407578 ) ) ;
#6389=B_SPLINE_CURVE_WITH_KNOTS ( 'NONE', 3,
 ( #72494, #72943, #4026, #17107, #3140, #30185, #30617, #65291, #51300, #86019 ),
 .UNSPECIFIED., .F., .F.,
 ( 4, 2, 2, 2, 4 ),
 ( 0.0007817359430256294638, 0.0009771253907249937212, 0.001172514838424358087, 0.001367904286123722453, 0.001563293733823093758 ),
 .UNSPECIFIED. ) ;
#6392=ORIENTED_EDGE ( 'NONE', *, *, #62889, .T. ) ;
#6393=CARTESIAN_POINT ( 'NONE',  ( -16.40384615384615330, -7.500000000000001776, 35.04278698407183867 ) ) ;
#6394=CARTESIAN_POINT ( 'NONE',  ( 12.71159288145191368, -4.818054556918156983, 34.26375889529406749 ) ) ;
#6397=CARTESIAN_POINT ( 'NONE',  ( 2.557692307693728129, -7.500000000000154543, 35.00000000000007105 ) ) ;
#6398=CARTESIAN_POINT ( 'NONE',  ( -5.143006487878956534, -6.386643153685125363, 34.62446782046654903 ) ) ;
#6399=EDGE_CURVE ( 'NONE', #81961, #24104, #53033, .T. ) ;
#6400=CARTESIAN_POINT ( 'NONE',  ( -10.61538461538461320, -2.292212530054420494, 30.41441678777542634 ) ) ;
#6401=CARTESIAN_POINT ( 'NONE',  ( -4.853547136224893421, -2.501478030877322567, 29.88021232661720816 ) ) ;
#6403=ORIENTED_EDGE ( 'NONE', *, *, #25235, .F. ) ;
#6404=CARTESIAN_POINT ( 'NONE',  ( 16.82689983963010860, -3.202444869320336451, 32.30641848906366675 ) ) ;
#6405=VECTOR ( 'NONE', #55502, 1000.000000000000000 ) ;
#6406=FACE_OUTER_BOUND ( 'NONE', #65035, .T. ) ;
#6407=CARTESIAN_POINT ( 'NONE',  ( 18.24994540937804643, -12.45601412856602686, 31.48342859153981621 ) ) ;
#6408=ORIENTED_EDGE ( 'NONE', *, *, #25530, .F. ) ;
#6409=CARTESIAN_POINT ( 'NONE',  ( -16.82686865700962286, -12.01375889529407992, 32.43194544308182969 ) ) ;
#6410=VECTOR ( 'NONE', #82418, 1000.000000000000227 ) ;
#6411=EDGE_LOOP ( 'NONE', ( #81329, #29247 ) ) ;
#6413=FACE_OUTER_BOUND ( 'NONE', #58921, .T. ) ;
#6414=ORIENTED_EDGE ( 'NONE', *, *, #17597, .T. ) ;
#6415=CARTESIAN_POINT ( 'NONE',  ( 12.46153846153846168, -3.513871655860378418, 32.76840700105978499 ) ) ;
#6416=CARTESIAN_POINT ( 'NONE',  ( 5.869852790561781219, -10.19110544564092002, 33.96427741523702792 ) ) ;
#6417=CARTESIAN_POINT ( 'NONE',  ( -11.76138775597768138, -6.503392248772476236, 34.64988816332204635 ) ) ;
#6418=CARTESIAN_POINT ( 'NONE',  ( 2.307692307692309264, -3.050289026998446396, 32.03036669348365706 ) ) ;
#6421=VERTEX_POINT ( 'NONE', #14757 ) ;
#6422=FACE_OUTER_BOUND ( 'NONE', #7079, .T. ) ;
#6423=EDGE_LOOP ( 'NONE', ( #70553, #59602, #31130, #64987 ) ) ;
#6424=CARTESIAN_POINT ( 'NONE',  ( 5.999999999999880096, -2.892918686052165622, 31.69288490824153470 ) ) ;
#6426=EDGE_CURVE ( 'NONE', #14948, #87491, #22893, .T. ) ;
#6427=CARTESIAN_POINT ( 'NONE',  ( 18.25005431163831915, -12.17597550085003633, 31.52189283813461884 ) ) ;
#6429=LINE ( 'NONE', #33453, #7561 ) ;
#6430=CARTESIAN_POINT ( 'NONE',  ( 7.053868730901709405, -9.804649428959608670, 34.18742332936588468 ) ) ;
#6431=ORIENTED_EDGE ( 'NONE', *, *, #81941, .F. ) ;
#6432=VERTEX_POINT ( 'NONE', #1678 ) ;
#6434=VERTEX_POINT ( 'NONE', #61601 ) ;
#6435=VERTEX_POINT ( 'NONE', #34132 ) ;
#6436=CARTESIAN_POINT ( 'NONE',  ( -5.076923076923197442, -5.219633306517616589, 34.19971097300220464 ) ) ;
#6437=EDGE_CURVE ( 'NONE', #26337, #67575, #82779, .T. ) ;
#6438=CARTESIAN_POINT ( 'NONE',  ( -9.626138551345036376, -7.250054483168843156, 34.74374881642865631 ) ) ;
#6439=LINE ( 'NONE', #13194, #81723 ) ;
#6440=ORIENTED_EDGE ( 'NONE', *, *, #67406, .T. ) ;
#6441=CARTESIAN_POINT ( 'NONE',  ( 11.31553532094538994, -2.554751324335735152, 30.48935550225260727 ) ) ;
#6442=CARTESIAN_POINT ( 'NONE',  ( -2.438383774359865974, -4.809359713505814149, 33.96456829005828837 ) ) ;
#6443=CARTESIAN_POINT ( 'NONE',  ( -2.242436736416281384, -3.835265460703683349, 33.15142922261929925 ) ) ;
#6444=CARTESIAN_POINT ( 'NONE',  ( -4.946397638689434828, -11.66157788607254275, 32.95092075102925833 ) ) ;
#6445=VERTEX_POINT ( 'NONE', #22391 ) ;
#6446=ORIENTED_EDGE ( 'NONE', *, *, #86777, .F. ) ;
#6447=ORIENTED_EDGE ( 'NONE', *, *, #468, .F. ) ;
#6448=DIRECTION ( 'NONE',  ( -0.000000000000000000, 0.1736481776669307198, -0.9848077530122080203 ) ) ;
#6449=CARTESIAN_POINT ( 'NONE',  ( 1.634669696253701288, -5.728107161865378494, 34.42597550085002922 ) ) ;
#6450=CARTESIAN_POINT ( 'NONE',  ( -7.715628407920200438, -9.503571793651731880, 34.60286762892837942 ) ) ;
#6451=B_SPLINE_CURVE_WITH_KNOTS ( 'NONE', 3,
 ( #47325, #27952, #34710, #37, #21186, #81133, #76129, #40589, #54980, #14431 ),
 .UNSPECIFIED., .F., .F.,
 ( 4, 2, 2, 2, 4 ),
 ( 0.0007817246256747530271, 0.0009771112852218978746, 0.001172497944769042939, 0.001367884604316188003, 0.001563271263863332851 ),
 .UNSPECIFIED. ) ;
#6452=LINE ( 'NONE', #33911, #78709 ) ;
#6453=CARTESIAN_POINT ( 'NONE',  ( -10.83831083290076158, -3.586966769969701208, 32.86292498521069660 ) ) ;
#6454=FACE_BOUND ( 'NONE', #70472, .T. ) ;
#6455=ORIENTED_EDGE ( 'NONE', *, *, #11182, .T. ) ;
#6456=VECTOR ( 'NONE', #40249, 1000.000000000000227 ) ;
#6457=CARTESIAN_POINT ( 'NONE',  ( -1.253823576790599637, -2.729792928343270031, 31.24908615093345432 ) ) ;
#6458=CARTESIAN_POINT ( 'NONE',  ( 3.100077764101675459, -10.54014554554150607, 33.71984207302941883 ) ) ;
#6460=CARTESIAN_POINT ( 'NONE',  ( 5.076923076923075762, -2.292212530054420494, 30.41441678777542634 ) ) ;
#6462=EDGE_LOOP ( 'NONE', ( #32561, #67551 ) ) ;
#6463=FACE_BOUND ( 'NONE', #34588, .T. ) ;
#6466=CARTESIAN_POINT ( 'NONE',  ( -2.307692307692305711, -2.249999999999998668, 29.50000000000001421 ) ) ;
#6468=CARTESIAN_POINT ( 'NONE',  ( 1.384615384615386802, -3.050289026998446396, 32.03036669348365706 ) ) ;
#6469=ORIENTED_EDGE ( 'NONE', *, *, #81443, .F. ) ;
#6470=CARTESIAN_POINT ( 'NONE',  ( 6.856993512121041690, -9.780366693483667717, 34.19971097300155805 ) ) ;
#6471=CARTESIAN_POINT ( 'NONE',  ( 14.55774672760576394, -3.435999193479609914, 33.07426656108010832 ) ) ;
#6472=CARTESIAN_POINT ( 'NONE',  ( -16.28453762051371356, -12.38065189839062263, 30.83690757178629482 ) ) ;
#6473=CYLINDRICAL_SURFACE ( 'NONE', #21700, 0.2499999999999995559 ) ;
#6474=ORIENTED_EDGE ( 'NONE', *, *, #52098, .F. ) ;
#6475=EDGE_CURVE ( 'NONE', #6435, #2497, #9963, .T. ) ;
#6476=CARTESIAN_POINT ( 'NONE',  ( -12.23875892027004930, -3.236590943229499029, 32.36255958852954251 ) ) ;
#6477=CARTESIAN_POINT ( 'NONE',  ( 4.023698184114458343, -10.31621877034669588, 34.18098118002070152 ) ) ;
#6478=CARTESIAN_POINT ( 'NONE',  ( 1.515405825582336607, -2.845873456487965747, 32.17976146951972538 ) ) ;
#6480=CARTESIAN_POINT ( 'NONE',  ( -8.769230769230890843, -10.90142922262034020, 33.41473453929536674 ) ) ;
#6482=CARTESIAN_POINT ( 'NONE',  ( -13.16160403300253279, -4.887748414852792322, 34.01359900205216746 ) ) ;
#6484=CARTESIAN_POINT ( 'NONE',  ( -10.36533030374629938, -2.564540009722895419, 30.55348353981670684 ) ) ;
#6485=CARTESIAN_POINT ( 'NONE',  ( -13.13466997523734037, -3.520799739797214389, 33.17531984108286025 ) ) ;
#6488=EDGE_CURVE ( 'NONE', #62563, #80983, #41793, .T. ) ;
#6489=CARTESIAN_POINT ( 'NONE',  ( -12.33101275977490197, -11.46989282347013095, 32.79007818306219946 ) ) ;
#6491=ORIENTED_EDGE ( 'NONE', *, *, #46945, .F. ) ;
#6492=CARTESIAN_POINT ( 'NONE',  ( 14.30769230769231015, -1.790695186598648903, 34.54067556320373455 ) ) ;
#6493=EDGE_LOOP ( 'NONE', ( #87279, #33703, #64868, #42133 ) ) ;
#6494=ORIENTED_EDGE ( 'NONE', *, *, #2391, .F. ) ;
#6499=CARTESIAN_POINT ( 'NONE',  ( 17.93472999944368240, -5.094484230520675894, 34.41647553114621161 ) ) ;
#6500=ADVANCED_FACE ( 'NONE', ( #28257 ), #83217, .F. ) ;
#6502=CARTESIAN_POINT ( 'NONE',  ( -1.384615384615383471, -9.819645486525091727, 36.12317359536749706 ) ) ;
#6504=CARTESIAN_POINT ( 'NONE',  ( 13.38461538461538680, -2.499999999999998668, 29.75000000000001421 ) ) ;
#6505=CYLINDRICAL_SURFACE ( 'NONE', #73288, 0.2499999999999998890 ) ;
#6506=CARTESIAN_POINT ( 'NONE',  ( 10.61538461538461675, -2.517432740324522911, 35.29906147534542527 ) ) ;
#6508=EDGE_CURVE ( 'NONE', #54081, #56507, #21954, .T. ) ;
#6509=EDGE_CURVE ( 'NONE', #13749, #83195, #15203, .T. ) ;
#6510=CARTESIAN_POINT ( 'NONE',  ( -7.053224892808620083, -5.070767119584671079, 34.40440758774516183 ) ) ;
#6511=CARTESIAN_POINT ( 'NONE',  ( -13.13456107297706943, -6.567000820036036579, 34.66262288849541306 ) ) ;
#6512=CARTESIAN_POINT ( 'NONE',  ( 5.934729999443681514, -11.67786785259541027, 32.92929555188721480 ) ) ;
#6513=B_SPLINE_CURVE_WITH_KNOTS ( 'NONE', 3,
 ( #46302, #73789, #19721, #47179, #74674, #12963, #37097, #10077, #30351, #78528 ),
 .UNSPECIFIED., .F., .F.,
 ( 4, 2, 2, 2, 4 ),
 ( 0.0007817359430256294638, 0.0009771253907249948054, 0.001172514838424360255, 0.001367904286123725489, 0.001563293733823090939 ),
 .UNSPECIFIED. ) ;
#6514=ADVANCED_FACE ( 'NONE', ( #43982 ), #3880, .F. ) ;
#6515=ORIENTED_EDGE ( 'NONE', *, *, #7975, .T. ) ;
#6516=EDGE_LOOP ( 'NONE', ( #55360, #30269, #63798, #1254 ) ) ;
#6517=CARTESIAN_POINT ( 'NONE',  ( 2.980792486720641232, -10.82459398097509684, 33.81372124010185587 ) ) ;
#6518=CARTESIAN_POINT ( 'NONE',  ( 0.4615384615383382183, -12.16647553114689728, 32.15551576947799362 ) ) ;
#6519=CARTESIAN_POINT ( 'NONE',  ( 10.61538461538461675, -1.509761064869970415, 31.06009739812519044 ) ) ;
#6520=CARTESIAN_POINT ( 'NONE',  ( 9.823098133274644539, -11.93129842949671726, 32.56571108434900452 ) ) ;
#6521=CARTESIAN_POINT ( 'NONE',  ( 6.250054311638316484, -4.943051570960391494, 34.04725096376909477 ) ) ;
#6522=CARTESIAN_POINT ( 'NONE',  ( -3.230769230769352962, -11.67786785259630911, 32.92929555188603530 ) ) ;
#6524=AXIS2_PLACEMENT_3D ( 'NONE', #26178, #27510, #32484 ) ;
#6525=ORIENTED_EDGE ( 'NONE', *, *, #27829, .F. ) ;
#6526=DIRECTION ( 'NONE',  ( -0.000000000000000000, -0.5000000000000009992, -0.8660254037844380415 ) ) ;
#6527=ORIENTED_EDGE ( 'NONE', *, *, #34266, .T. ) ;
#6528=B_SPLINE_CURVE_WITH_KNOTS ( 'NONE', 3,
 ( #73069, #11367, #20784, #48251, #67209, #32977, #33423, #68096, #34297, #53682 ),
 .UNSPECIFIED., .F., .F.,
 ( 4, 2, 2, 2, 4 ),
 ( 0.000000000000000000, 0.0001954311564186863323, 0.0003908623128373726646, 0.0005862934692560590241, 0.0007817246256747453293 ),
 .UNSPECIFIED. ) ;
#6530=CARTESIAN_POINT ( 'NONE',  ( -8.703975629717932705, -5.094484230520773593, 34.41647553114626845 ) ) ;
#6532=CARTESIAN_POINT ( 'NONE',  ( -7.145956439814507455, -7.630690623152302621, 34.99857592706774057 ) ) ;
#6533=AXIS2_PLACEMENT_3D ( 'NONE', #20167, #67910, #34116 ) ;
#6534=CARTESIAN_POINT ( 'NONE',  ( 2.980746006547773774, -8.475808217655753651, 34.90892951860618609 ) ) ;
#6535=DIRECTION ( 'NONE',  ( -0.000000000000000000, 0.8660254037844399289, -0.4999999999999980016 ) ) ;
#6536=ORIENTED_EDGE ( 'NONE', *, *, #69796, .T. ) ;
#6537=EDGE_CURVE ( 'NONE', #2738, #76676, #26095, .T. ) ;
#6538=ORIENTED_EDGE ( 'NONE', *, *, #41649, .T. ) ;
#6539=EDGE_LOOP ( 'NONE', ( #20938, #55997, #49401, #4683, #29417, #46971 ) ) ;
#6541=CARTESIAN_POINT ( 'NONE',  ( -6.130147969731695845, -5.070767119584671079, 34.40440758774516183 ) ) ;
#6542=CARTESIAN_POINT ( 'NONE',  ( 4.826899839630110378, -10.76384336483936011, 33.53834819971076087 ) ) ;
#6543=EDGE_CURVE ( 'NONE', #79083, #69664, #46508, .T. ) ;
#6544=CARTESIAN_POINT ( 'NONE',  ( 16.02328624023278891, -2.254533558242299396, 29.97296025877828640 ) ) ;
#6545=CARTESIAN_POINT ( 'NONE',  ( 14.55769230769224798, -7.565270000091922853, 34.99999999999999289 ) ) ;
#6549=EDGE_LOOP ( 'NONE', ( #29578, #77211 ) ) ;
#6550=EDGE_LOOP ( 'NONE', ( #71703, #86951, #74443, #40159 ) ) ;
#6551=ADVANCED_FACE ( 'NONE', ( #65135 ), #51159, .F. ) ;
#6552=DIRECTION ( 'NONE',  ( 0.000000000000000000, 0.7660444431189807890, 0.6427876096865361433 ) ) ;
#6553=ORIENTED_EDGE ( 'NONE', *, *, #1976, .T. ) ;
#6554=CARTESIAN_POINT ( 'NONE',  ( 8.769230769230768274, -9.819645486525091727, 36.12317359536749706 ) ) ;
#6555=CARTESIAN_POINT ( 'NONE',  ( 6.923076923076924238, -11.11383981884818262, 36.00935417666054406 ) ) ;
#6557=ORIENTED_EDGE ( 'NONE', *, *, #36159, .F. ) ;
#6558=CARTESIAN_POINT ( 'NONE',  ( -5.999999999999998224, -9.058645607665452459, 34.76329471203371924 ) ) ;
#6559=ORIENTED_EDGE ( 'NONE', *, *, #18862, .T. ) ;
#6560=CARTESIAN_POINT ( 'NONE',  ( 2.057669070399342992, -6.695914987888143877, 34.68535235679833306 ) ) ;
#6561=FACE_BOUND ( 'NONE', #5620, .T. ) ;
#6563=CARTESIAN_POINT ( 'NONE',  ( 5.999999999999878320, -3.083524468854526912, 32.58852847137268327 ) ) ;
#6564=VERTEX_POINT ( 'NONE', #2992 ) ;
#6567=CARTESIAN_POINT ( 'NONE',  ( 8.992243613324164997, -8.282913670948747864, 34.94150082978203642 ) ) ;
#6568=CARTESIAN_POINT ( 'NONE',  ( 16.21910172512217585, -2.625532179533470512, 30.86335684631491105 ) ) ;
#6569=LINE ( 'NONE', #21410, #7852 ) ;
#6570=ORIENTED_EDGE ( 'NONE', *, *, #88271, .T. ) ;
#6571=CARTESIAN_POINT ( 'NONE',  ( 11.60371710973756620, -3.300289026998473041, 32.46337939537591666 ) ) ;
#6572=CARTESIAN_POINT ( 'NONE',  ( -6.000000000000121680, -4.320704448113951379, 33.92786785259630022 ) ) ;
#6573=CARTESIAN_POINT ( 'NONE',  ( 17.29970261819148192, -10.11255958852955672, 34.01340905677048454 ) ) ;
#6574=LINE ( 'NONE', #33605, #21325 ) ;
#6575=CARTESIAN_POINT ( 'NONE',  ( -13.38461538461550582, -10.90142922262034020, 33.41473453929536674 ) ) ;
#6576=AXIS2_PLACEMENT_3D ( 'NONE', #65152, #37235, #15656 ) ;
#6577=FACE_BOUND ( 'NONE', #2305, .T. ) ;
#6578=CARTESIAN_POINT ( 'NONE',  ( -3.230769230769229949, -11.91647553114624181, 32.58852847137148245 ) ) ;
#6579=CARTESIAN_POINT ( 'NONE',  ( 11.28843830116857383, -12.43535235679832596, 30.55408501211184813 ) ) ;
#6581=EDGE_CURVE ( 'NONE', #49750, #47506, #30472, .T. ) ;
#6582=DIRECTION ( 'NONE',  ( 0.000000000000000000, 0.4999999999999960032, -0.8660254037844410391 ) ) ;
#6583=CARTESIAN_POINT ( 'NONE',  ( -8.638705067467203236, -11.93748526763465279, 32.05452791011430946 ) ) ;
#6584=CARTESIAN_POINT ( 'NONE',  ( -2.084912638714241595, -12.47679350104403007, 31.42216943046555855 ) ) ;
#6585=CARTESIAN_POINT ( 'NONE',  ( -5.326946301144534601, -12.45566812827425096, 31.48439005359158926 ) ) ;
#6587=ORIENTED_EDGE ( 'NONE', *, *, #63531, .F. ) ;
#6588=CARTESIAN_POINT ( 'NONE',  ( -8.519230769230704325, -7.434744429011176159, 34.75000000000000711 ) ) ;
#6590=CARTESIAN_POINT ( 'NONE',  ( -18.13014796973169851, -3.625366637846541007, 33.29286588640297850 ) ) ;
#6591=ORIENTED_EDGE ( 'NONE', *, *, #9553, .F. ) ;
#6592=DIRECTION ( 'NONE',  ( 0.000000000000000000, 1.000000000000000000, 0.000000000000000000 ) ) ;
#6593=CARTESIAN_POINT ( 'NONE',  ( -16.02332071561251325, -12.15418822224088657, 32.17964115625579069 ) ) ;
#6594=DIRECTION ( 'NONE',  ( -0.000000000000000000, -0.5000000000000009992, -0.8660254037844380415 ) ) ;
#6596=ORIENTED_EDGE ( 'NONE', *, *, #50969, .T. ) ;
#6597=CARTESIAN_POINT ( 'NONE',  ( -15.29603967673000575, -5.219633306516282545, 34.19971097300152962 ) ) ;
#6599=DIRECTION ( 'NONE',  ( 0.000000000000000000, 1.000000000000000000, 0.000000000000000000 ) ) ;
#6601=CARTESIAN_POINT ( 'NONE',  ( -9.692307692307812417, -10.90142922262034020, 33.41473453929536674 ) ) ;
#6603=FACE_OUTER_BOUND ( 'NONE', #73604, .T. ) ;
#6606=EDGE_CURVE ( 'NONE', #20850, #78839, #85868, .T. ) ;
#6607=CARTESIAN_POINT ( 'NONE',  ( 3.100294045693512857, -7.276987145209184327, 34.99546412871779211 ) ) ;
#6608=ORIENTED_EDGE ( 'NONE', *, *, #10778, .T. ) ;
#6612=CARTESIAN_POINT ( 'NONE',  ( -20.99999999999999645, -12.75000000000000178, 27.25000000000000000 ) ) ;
#6613=ORIENTED_EDGE ( 'NONE', *, *, #18377, .T. ) ;
#6614=CARTESIAN_POINT ( 'NONE',  ( 6.673076923076925127, -7.500000000000001776, 35.04278698407183867 ) ) ;
#6615=CARTESIAN_POINT ( 'NONE',  ( -0.3310127597748996342, -10.19071101563364401, 33.96452234770657697 ) ) ;
#6616=CARTESIAN_POINT ( 'NONE',  ( -20.74999999999999645, -10.50000000000000000, 27.25000000000000000 ) ) ;
#6617=ORIENTED_EDGE ( 'NONE', *, *, #72018, .F. ) ;
#6618=CARTESIAN_POINT ( 'NONE',  ( 0.4615384615384611200, -1.129524287112498415, 32.06866353760679544 ) ) ;
#6619=CARTESIAN_POINT ( 'NONE',  ( -16.82692307692165556, -7.500000000000154543, 35.00000000000007105 ) ) ;
#6621=CYLINDRICAL_SURFACE ( 'NONE', #35656, 0.2500000000000002220 ) ;
#6622=CARTESIAN_POINT ( 'NONE',  ( 3.165499230212911463, -2.657715359629089225, 31.77849191805834295 ) ) ;
#6623=CARTESIAN_POINT ( 'NONE',  ( -18.00000000000000000, -12.10708131394839349, 31.69288490824020244 ) ) ;
#6624=DIRECTION ( 'NONE',  ( 0.000000000000000000, 0.000000000000000000, 1.000000000000000000 ) ) ;
#6625=ORIENTED_EDGE ( 'NONE', *, *, #70339, .F. ) ;
#6626=EDGE_LOOP ( 'NONE', ( #78773, #26281, #23100, #22709 ) ) ;
#6627=ORIENTED_EDGE ( 'NONE', *, *, #42062, .F. ) ;
#6629=CARTESIAN_POINT ( 'NONE',  ( 0.4615384615384611755, -11.33034616979429110, 35.88435417666054406 ) ) ;
#6630=CARTESIAN_POINT ( 'NONE',  ( 14.05771557674995442, -4.236021600441997492, 33.53823185664189310 ) ) ;
#6631=B_SPLINE_CURVE_WITH_KNOTS ( 'NONE', 3,
 ( #36530, #23439, #56786, #16686, #36951, #9060, #22562, #43283, #78829, #3165 ),
 .UNSPECIFIED., .F., .F.,
 ( 4, 2, 2, 2, 4 ),
 ( 0.0007817246256747473893, 0.0009771112852218905021, 0.001172497944769033615, 0.001367884604316176944, 0.001563271263863320057 ),
 .UNSPECIFIED. ) ;
#6633=CARTESIAN_POINT ( 'NONE',  ( -17.20753273212715939, -7.722926974430166069, 34.99546784045485737 ) ) ;
#6634=B_SPLINE_CURVE_WITH_KNOTS ( 'NONE', 3,
 ( #35439, #62891, #1204, #30449, #17384, #65559, #32238, #44841, #37648, #78194 ),
 .UNSPECIFIED., .F., .F.,
 ( 4, 2, 2, 2, 4 ),
 ( 0.000000000000000000, 0.0001954311564186871184, 0.0003908623128373742367, 0.0005862934692560614093, 0.0007817246256747484735 ),
 .UNSPECIFIED. ) ;
#6635=CARTESIAN_POINT ( 'NONE',  ( 17.99999999999987566, -11.94971097300221174, 32.03036669348237098 ) ) ;
#6636=ORIENTED_EDGE ( 'NONE', *, *, #33792, .T. ) ;
#6638=ORIENTED_EDGE ( 'NONE', *, *, #46515, .F. ) ;
#6639=ORIENTED_EDGE ( 'NONE', *, *, #30742, .F. ) ;
#6640=CARTESIAN_POINT ( 'NONE',  ( -6.923076923077045919, -8.656820664282941280, 34.87096338111179961 ) ) ;
#6642=CARTESIAN_POINT ( 'NONE',  ( -0.7115151924808164052, -4.943428324936578910, 34.04746400365624481 ) ) ;
#6643=CARTESIAN_POINT ( 'NONE',  ( 5.749976775778542937, -12.68155406624981119, 30.59749803192733708 ) ) ;
#6644=DIRECTION ( 'NONE',  ( -0.000000000000000000, 0.5000000000000011102, -0.8660254037844380415 ) ) ;
#6646=AXIS2_PLACEMENT_3D ( 'NONE', #7560, #21054, #48982 ) ;
#6648=VERTEX_POINT ( 'NONE', #24603 ) ;
#6649=ORIENTED_EDGE ( 'NONE', *, *, #86961, .F. ) ;
#6650=CARTESIAN_POINT ( 'NONE',  ( -5.142247089727384868, -7.749976730030849303, 34.74374725381503737 ) ) ;
#6651=CARTESIAN_POINT ( 'NONE',  ( -10.39237177129122003, -2.523321265292115534, 31.42251411153756990 ) ) ;
#6652=ORIENTED_EDGE ( 'NONE', *, *, #18647, .T. ) ;
#6653=CARTESIAN_POINT ( 'NONE',  ( -11.53846153846153655, -12.62096338111211580, 30.90682066428153263 ) ) ;
#6654=CYLINDRICAL_SURFACE ( 'NONE', #14858, 0.2500000000000014988 ) ;
#6655=ORIENTED_EDGE ( 'NONE', *, *, #65346, .F. ) ;
#6656=CARTESIAN_POINT ( 'NONE',  ( 16.37662569511456567, -3.755027918224367767, 33.06320215134714857 ) ) ;
#6657=DIRECTION ( 'NONE',  ( -0.000000000000000000, 0.5000000000000011102, -0.8660254037844381525 ) ) ;
#6658=FACE_BOUND ( 'NONE', #30601, .T. ) ;
#6659=CARTESIAN_POINT ( 'NONE',  ( 10.83816415665302380, -10.11255958852956027, 34.01340905677048454 ) ) ;
#6660=CARTESIAN_POINT ( 'NONE',  ( 13.63456079399342791, -6.653508905675592722, 34.93172785388651391 ) ) ;
#6661=EDGE_CURVE ( 'NONE', #72951, #35434, #9331, .T. ) ;
#6662=CARTESIAN_POINT ( 'NONE',  ( 15.23076923076923173, -8.318370150425687726, 35.83090037661290239 ) ) ;
#6663=CARTESIAN_POINT ( 'NONE',  ( -10.61538461538461320, -9.584722331328613620, 36.20867863119891439 ) ) ;
#6664=CARTESIAN_POINT ( 'NONE',  ( -0.5268089074992368115, -12.27809138561121394, 31.22303859784730307 ) ) ;
#6666=CARTESIAN_POINT ( 'NONE',  ( -4.087777802843714170, -2.721908614388772296, 31.22303859784725333 ) ) ;
#6667=CARTESIAN_POINT ( 'NONE',  ( -3.903900744468110418, -11.56426240980093745, 33.07394671870546432 ) ) ;
#6669=CARTESIAN_POINT ( 'NONE',  ( -7.976844449264153702, -6.369640206132551441, 34.87707690430378449 ) ) ;
#6670=CARTESIAN_POINT ( 'NONE',  ( -7.976714437895769727, -2.504760397472875155, 29.97295953869789997 ) ) ;
#6671=VERTEX_POINT ( 'NONE', #17411 ) ;
#6672=AXIS2_PLACEMENT_3D ( 'NONE', #53142, #80646, #46836 ) ;
#6673=LINE ( 'NONE', #18864, #41528 ) ;
#6675=CARTESIAN_POINT ( 'NONE',  ( -4.376773112753001627, -3.395401636524186362, 33.02366814457250399 ) ) ;
#6676=EDGE_LOOP ( 'NONE', ( #15043, #40540 ) ) ;
#6677=DIRECTION ( 'NONE',  ( 0.000000000000000000, 0.8660254037844377084, -0.5000000000000015543 ) ) ;
#6678=DIRECTION ( 'NONE',  ( 0.000000000000000000, -6.938893903907222067E-15, 1.000000000000000000 ) ) ;
#6679=FACE_BOUND ( 'NONE', #80386, .T. ) ;
#6680=FACE_OUTER_BOUND ( 'NONE', #20603, .T. ) ;
#6681=CARTESIAN_POINT ( 'NONE',  ( 15.45354877203763877, -12.24180327182771855, 31.33663988360758879 ) ) ;
#6682=CARTESIAN_POINT ( 'NONE',  ( 7.976679547917409963, -9.417988943895561960, 34.36773134775777550 ) ) ;
#6683=EDGE_CURVE ( 'NONE', #9491, #40013, #42206, .T. ) ;
#6684=VECTOR ( 'NONE', #54321, 1000.000000000000000 ) ;
#6685=CARTESIAN_POINT ( 'NONE',  ( 2.372947878968333590, -5.219633306516380244, 34.19971097300157936 ) ) ;
#6687=CARTESIAN_POINT ( 'NONE',  ( -0.4615384615384611200, -1.951392089020283160, 34.73218667398347748 ) ) ;
#6689=ORIENTED_EDGE ( 'NONE', *, *, #58662, .T. ) ;
#6690=ORIENTED_EDGE ( 'NONE', *, *, #44095, .T. ) ;
#6691=CARTESIAN_POINT ( 'NONE',  ( -15.23076923076922995, -11.69971097300155272, 32.46337939537588113 ) ) ;
#6692=CARTESIAN_POINT ( 'NONE',  ( -10.36533019547115941, -8.346898887586323923, 34.93166121998716278 ) ) ;
#6693=DIRECTION ( 'NONE',  ( -0.000000000000000000, -0.6427876096865404731, -0.7660444431189770143 ) ) ;
#6694=CARTESIAN_POINT ( 'NONE',  ( 6.857806477116148436, -12.27809138561121394, 31.22303859784730307 ) ) ;
#6695=CARTESIAN_POINT ( 'NONE',  ( 5.207713517890028676, -3.338503747796866872, 32.95102852606553512 ) ) ;
#6697=CARTESIAN_POINT ( 'NONE',  ( 0.5915860677941437995, -7.723484964179500700, 34.74522123443823318 ) ) ;
#6698=CARTESIAN_POINT ( 'NONE',  ( 1.161130460051056357, -10.23692288466677880, 34.23039457007281072 ) ) ;
#6699=CARTESIAN_POINT ( 'NONE',  ( 17.75002325595140817, -4.075325502946085976, 33.72974371597207721 ) ) ;
#6701=CARTESIAN_POINT ( 'NONE',  ( 18.25005431163831204, -9.943054286541403997, 34.11300777759954883 ) ) ;
#6702=CARTESIAN_POINT ( 'NONE',  ( 6.250054419913455561, -6.523592122091591783, 34.90882529074906415 ) ) ;
#6703=CARTESIAN_POINT ( 'NONE',  ( 6.988332062589760696, -3.643525952247864463, 33.31231777344670064 ) ) ;
#6704=ADVANCED_FACE ( 'NONE', ( #57058 ), #32690, .F. ) ;
#6705=DIRECTION ( 'NONE',  ( 0.000000000000000000, 0.3420201433256610524, 0.9396926207859113145 ) ) ;
#6706=CARTESIAN_POINT ( 'NONE',  ( -12.59209905328038026, -2.504760397472875155, 29.97295953869789997 ) ) ;
#6708=B_SPLINE_CURVE_WITH_KNOTS ( 'NONE', 3,
 ( #16728, #44184, #28481, #83437, #21720, #69905, #49191, #8215, #63139, #1454 ),
 .UNSPECIFIED., .F., .F.,
 ( 4, 2, 2, 2, 4 ),
 ( 0.000000000000000000, 0.0001954339857564080707, 0.0003908679715128161414, 0.0005863019572692241849, 0.0007817359430256322827 ),
 .UNSPECIFIED. ) ;
#6709=CARTESIAN_POINT ( 'NONE',  ( 0.4615384615384611200, -8.564572088678739092, 35.78748833219616898 ) ) ;
#6710=CARTESIAN_POINT ( 'NONE',  ( -17.30040800148741198, -6.716662450894490100, 34.94144148231605840 ) ) ;
#6712=ADVANCED_FACE ( 'NONE', ( #66489 ), #86781, .F. ) ;
#6713=EDGE_CURVE ( 'NONE', #84305, #59182, #63722, .T. ) ;
#6715=DIRECTION ( 'NONE',  ( 0.000000000000000000, 0.9396926207859126468, 0.3420201433256571111 ) ) ;
#6716=CARTESIAN_POINT ( 'NONE',  ( -11.53846153846153655, -4.661471528628507777, 34.16647553114623292 ) ) ;
#6717=DIRECTION ( 'NONE',  ( -0.000000000000000000, -0.9848077530122086864, -0.1736481776669273613 ) ) ;
#6718=EDGE_LOOP ( 'NONE', ( #71439, #24664, #38934, #23582 ) ) ;
#6720=CARTESIAN_POINT ( 'NONE',  ( -14.30769230769242917, -5.941354392335915335, 34.76329471203413846 ) ) ;
#6722=VERTEX_POINT ( 'NONE', #4788 ) ;
#6723=CARTESIAN_POINT ( 'NONE',  ( 11.66925197942848769, -9.084667340241226796, 34.75534355489798344 ) ) ;
#6724=CARTESIAN_POINT ( 'NONE',  ( 10.83839745947800992, -10.77377354290276124, 33.85451476688484718 ) ) ;
#6725=ORIENTED_EDGE ( 'NONE', *, *, #29681, .T. ) ;
#6726=CARTESIAN_POINT ( 'NONE',  ( 16.82689983963011215, -11.37209801155882793, 32.91403422569033665 ) ) ;
#6727=LINE ( 'NONE', #34200, #7691 ) ;
#6728=CARTESIAN_POINT ( 'NONE',  ( 2.177001704582001818, -12.62707690430377383, 30.88035979386743435 ) ) ;
#6729=EDGE_LOOP ( 'NONE', ( #27355, #62874 ) ) ;
#6730=VERTEX_POINT ( 'NONE', #32263 ) ;
#6731=CARTESIAN_POINT ( 'NONE',  ( 15.45378207486262667, -4.762714258010881885, 34.23016756924214832 ) ) ;
#6733=CARTESIAN_POINT ( 'NONE',  ( 3.296836564119306701, -11.91647553114624358, 32.58852847137148245 ) ) ;
#6734=CARTESIAN_POINT ( 'NONE',  ( -9.469296340694841163, -9.886259254753566594, 34.14407573483972413 ) ) ;
#6735=CARTESIAN_POINT ( 'NONE',  ( 9.692307692307695177, -9.058645607665452459, 34.76329471203371924 ) ) ;
#6736=DIRECTION ( 'NONE',  ( -0.000000000000000000, 0.3420201433256694346, -0.9396926207859080948 ) ) ;
#6737=CARTESIAN_POINT ( 'NONE',  ( 1.384615384615265343, -4.481592998941358097, 33.73612834414048933 ) ) ;
#6738=CARTESIAN_POINT ( 'NONE',  ( -2.438252221305670542, -2.254533558242299396, 29.97296025877828285 ) ) ;
#6739=AXIS2_PLACEMENT_3D ( 'NONE', #13130, #82040, #54100 ) ;
#6740=B_SPLINE_CURVE_WITH_KNOTS ( 'NONE', 3,
 ( #22564, #1408, #57240, #29333, #36531, #63978, #15376, #2276, #64416, #56787 ),
 .UNSPECIFIED., .F., .F.,
 ( 4, 2, 2, 2, 4 ),
 ( 0.000000000000000000, 0.0001954311564186882026, 0.0003908623128373764051, 0.0005862934692560646619, 0.0007817246256747528103 ),
 .UNSPECIFIED. ) ;
#6741=CARTESIAN_POINT ( 'NONE',  ( -12.68502340526241312, -6.760086850603066466, 34.69517049084099369 ) ) ;
#6742=B_SPLINE_CURVE_WITH_KNOTS ( 'NONE', 3,
 ( #35407, #23115, #57784, #16359, #83163, #21454, #48923, #85267, #2385, #23548 ),
 .UNSPECIFIED., .F., .F.,
 ( 4, 2, 2, 2, 4 ),
 ( 0.0007817359430256252354, 0.0009771253907249898181, 0.001172514838424354401, 0.001367904286123718983, 0.001563293733823083566 ),
 .UNSPECIFIED. ) ;
#6743=ADVANCED_FACE ( 'NONE', ( #18299 ), #66025, .F. ) ;
#6744=ORIENTED_EDGE ( 'NONE', *, *, #63330, .T. ) ;
#6745=ORIENTED_EDGE ( 'NONE', *, *, #14433, .F. ) ;
#6746=CARTESIAN_POINT ( 'NONE',  ( 6.988332062589761584, -12.70778746994558439, 30.41441678777537305 ) ) ;
#6747=ORIENTED_EDGE ( 'NONE', *, *, #86116, .T. ) ;
#6748=CARTESIAN_POINT ( 'NONE',  ( 2.307692307692309264, -13.37000171582298513, 34.34916445242398453 ) ) ;
#6749=CARTESIAN_POINT ( 'NONE',  ( -13.63461538461538503, -7.433932668274256805, 35.00000000000000711 ) ) ;
#6750=CARTESIAN_POINT ( 'NONE',  ( 11.66925334628632704, -12.11778462344221019, 31.66786338562085135 ) ) ;
#6751=VERTEX_POINT ( 'NONE', #69037 ) ;
#6752=CARTESIAN_POINT ( 'NONE',  ( -12.46153846153846168, -5.557115091759785130, 34.35708131394839171 ) ) ;
#6753=ADVANCED_FACE ( 'NONE', ( #34799 ), #62267, .F. ) ;
#6754=ORIENTED_EDGE ( 'NONE', *, *, #75629, .T. ) ;
#6755=CARTESIAN_POINT ( 'NONE',  ( -9.692307692307691624, -7.500000000000001776, 35.04278698407183867 ) ) ;
#6756=ORIENTED_EDGE ( 'NONE', *, *, #4583, .F. ) ;
#6757=LINE ( 'NONE', #7210, #21513 ) ;
#6758=VECTOR ( 'NONE', #42515, 1000.000000000000000 ) ;
#6759=ORIENTED_EDGE ( 'NONE', *, *, #22364, .T. ) ;
#6760=CARTESIAN_POINT ( 'NONE',  ( 12.46153846153833911, -2.379036618888197729, 30.90682066428292885 ) ) ;
#6761=CARTESIAN_POINT ( 'NONE',  ( 3.230769230769231726, -2.292212530054420494, 30.41441678777542634 ) ) ;
#6762=FACE_BOUND ( 'NONE', #39766, .T. ) ;
#6763=CARTESIAN_POINT ( 'NONE',  ( 14.30769230769231015, -1.129524287112498415, 32.06866353760679544 ) ) ;
#6765=B_SPLINE_CURVE_WITH_KNOTS ( 'NONE', 3,
 ( #2560, #44425, #51620, #58387, #51172, #8898, #2127, #23717, #30051, #50743 ),
 .UNSPECIFIED., .F., .F.,
 ( 4, 2, 2, 2, 4 ),
 ( 0.0007817359430256315238, 0.0009771253907249976244, 0.001172514838424363508, 0.001367904286123729392, 0.001563293733823095492 ),
 .UNSPECIFIED. ) ;
#6766=EDGE_CURVE ( 'NONE', #50121, #70789, #582, .T. ) ;
#6767=CARTESIAN_POINT ( 'NONE',  ( -24.00000000000000000, -5.499999999999981348, 27.25000000000000000 ) ) ;
#6768=CARTESIAN_POINT ( 'NONE',  ( 4.403900465484468896, -8.303483539816728154, 34.68545999027711702 ) ) ;
#6769=CARTESIAN_POINT ( 'NONE',  ( -4.946397638689432164, -4.299079248970732792, 33.91157788607253565 ) ) ;
#6770=FACE_OUTER_BOUND ( 'NONE', #47897, .T. ) ;
#6772=CARTESIAN_POINT ( 'NONE',  ( 14.37294744720514572, -6.835583212224610072, 34.95778746994559327 ) ) ;
#6775=VERTEX_POINT ( 'NONE', #55516 ) ;
#6776=CARTESIAN_POINT ( 'NONE',  ( -16.94613126909828793, -9.804649428959608670, 34.18742332936588468 ) ) ;
#6777=DIRECTION ( 'NONE',  ( -0.000000000000000000, -0.9848077530122085754, -0.1736481776669273613 ) ) ;
#6778=CARTESIAN_POINT ( 'NONE',  ( -9.692307692307814193, -12.51329471203414379, 31.30864560766407578 ) ) ;
#6779=CARTESIAN_POINT ( 'NONE',  ( -14.30769230769230660, -11.91647553114624181, 32.58852847137148245 ) ) ;
#6780=CARTESIAN_POINT ( 'NONE',  ( -17.20707104665477516, -12.50552854090298638, 31.33409797877408920 ) ) ;
#6781=CARTESIAN_POINT ( 'NONE',  ( -12.21159305216042057, -4.932303261841489928, 34.32971442181322885 ) ) ;
#6782=EDGE_LOOP ( 'NONE', ( #51489, #20979, #54498, #61337 ) ) ;
#6785=CARTESIAN_POINT ( 'NONE',  ( -3.296851610129365895, -11.35647404775217595, 33.31231777344666511 ) ) ;
#6786=EDGE_CURVE ( 'NONE', #70777, #48900, #73243, .T. ) ;
#6788=VERTEX_POINT ( 'NONE', #75786 ) ;
#6790=ORIENTED_EDGE ( 'NONE', *, *, #8197, .F. ) ;
#6791=EDGE_CURVE ( 'NONE', #84846, #34142, #44404, .T. ) ;
#6793=FACE_OUTER_BOUND ( 'NONE', #60416, .T. ) ;
#6796=DIRECTION ( 'NONE',  ( 0.000000000000000000, -6.938893903907222067E-15, 1.000000000000000000 ) ) ;
#6797=CARTESIAN_POINT ( 'NONE',  ( 15.10007776410167679, -8.999036380462717588, 34.52022231692819076 ) ) ;
#6798=CARTESIAN_POINT ( 'NONE',  ( 18.00000000000000000, -8.120952969808772792, 34.71129190930000163 ) ) ;
#6799=CARTESIAN_POINT ( 'NONE',  ( -17.20707104665477161, -9.504002272028873932, 34.60269587691767867 ) ) ;
#6800=CARTESIAN_POINT ( 'NONE',  ( 9.915319043920545639, -5.667800583137506010, 34.40243808032445827 ) ) ;
#6801=VERTEX_POINT ( 'NONE', #60161 ) ;
#6802=CARTESIAN_POINT ( 'NONE',  ( -15.16470189741915320, -2.486705287966280320, 31.30864560766543647 ) ) ;
#6803=CARTESIAN_POINT ( 'NONE',  ( -0.7115152055870527237, -5.643011162660950042, 34.66104346484419096 ) ) ;
#6804=VERTEX_POINT ( 'NONE', #26388 ) ;
#6805=CYLINDRICAL_SURFACE ( 'NONE', #18222, 0.2499999999999986955 ) ;
#6806=CARTESIAN_POINT ( 'NONE',  ( -3.230769230769229949, -2.708943851104267164, 35.45975837776705220 ) ) ;
#6807=DIRECTION ( 'NONE',  ( -1.000000000000000000, 0.000000000000000000, 0.000000000000000000 ) ) ;
#6809=CARTESIAN_POINT ( 'NONE',  ( 6.000000000000001776, -1.242168528481310874, 33.36296068462461051 ) ) ;
#6810=EDGE_CURVE ( 'NONE', #49750, #33268, #48732, .T. ) ;
#6811=LINE ( 'NONE', #41941, #40674 ) ;
#6814=ORIENTED_EDGE ( 'NONE', *, *, #74797, .T. ) ;
#6816=CARTESIAN_POINT ( 'NONE',  ( 0.6845498131513094719, -3.105924265160262543, 32.13625925475356127 ) ) ;
#6818=CARTESIAN_POINT ( 'NONE',  ( 9.758375025657770152, -10.67929555188718282, 33.92786785259544757 ) ) ;
#6819=ORIENTED_EDGE ( 'NONE', *, *, #82316, .T. ) ;
#6820=EDGE_CURVE ( 'NONE', #41209, #57354, #76657, .T. ) ;
#6821=ORIENTED_EDGE ( 'NONE', *, *, #43391, .F. ) ;
#6822=CARTESIAN_POINT ( 'NONE',  ( -5.869208192175211281, -2.541949514083464479, 30.39797389878540557 ) ) ;
#6823=CARTESIAN_POINT ( 'NONE',  ( -3.230769230769352962, -5.094484230521993062, 34.41647553114689373 ) ) ;
#6824=CARTESIAN_POINT ( 'NONE',  ( 10.74591005361826035, -5.070358843744210198, 34.40418822224088302 ) ) ;
#6825=CARTESIAN_POINT ( 'NONE',  ( 6.989145274079363368, -5.557115091759786019, 34.35708131394839882 ) ) ;
#6826=CARTESIAN_POINT ( 'NONE',  ( 18.00000000000000000, -2.486705287966279876, 31.30864560766543647 ) ) ;
#6827=ORIENTED_EDGE ( 'NONE', *, *, #32526, .F. ) ;
#6828=AXIS2_PLACEMENT_3D ( 'NONE', #2329, #59056, #86556 ) ;
#6829=CARTESIAN_POINT ( 'NONE',  ( 6.250054311638314708, -5.728107161865375829, 34.42597550085002922 ) ) ;
#6830=CARTESIAN_POINT ( 'NONE',  ( 3.296024802045256052, -12.27809138561124591, 31.22303859784720359 ) ) ;
#6831=CARTESIAN_POINT ( 'NONE',  ( 5.142178216435913107, -12.51329471203373700, 31.30864560766537963 ) ) ;
#6832=ORIENTED_EDGE ( 'NONE', *, *, #62487, .T. ) ;
#6833=CARTESIAN_POINT ( 'NONE',  ( 7.846153846153846700, -1.790695186598648903, 34.54067556320373455 ) ) ;
#6834=B_SPLINE_CURVE_WITH_KNOTS ( 'NONE', 3,
 ( #88968, #49285, #67788, #68233, #76763, #6534, #27238, #48834, #54704, #14615 ),
 .UNSPECIFIED., .F., .F.,
 ( 4, 2, 2, 2, 4 ),
 ( 0.000000000000000000, 0.0001954311564186873623, 0.0003908623128373747246, 0.0005862934692560620598, 0.0007817246256747494492 ),
 .UNSPECIFIED. ) ;
#6835=VECTOR ( 'NONE', #62575, 1000.000000000000227 ) ;
#6837=CARTESIAN_POINT ( 'NONE',  ( 1.161788692136382695, -7.369208160676172348, 34.74850200257122879 ) ) ;
#6838=CARTESIAN_POINT ( 'NONE',  ( 11.28843831424007860, -2.588893531581426988, 31.60682220781847818 ) ) ;
#6839=EDGE_LOOP ( 'NONE', ( #60946, #27921, #43809, #23205 ) ) ;
#6840=VECTOR ( 'NONE', #49258, 1000.000000000000000 ) ;
#6841=CARTESIAN_POINT ( 'NONE',  ( -17.77698715590660328, -10.01129605718032956, 34.36064277460058491 ) ) ;
#6842=CARTESIAN_POINT ( 'NONE',  ( 4.376625822824220080, -9.418065098278011860, 34.63729479722530158 ) ) ;
#6843=FACE_OUTER_BOUND ( 'NONE', #15745, .T. ) ;
#6844=CARTESIAN_POINT ( 'NONE',  ( 11.53846153846141576, -12.51329471203414379, 31.30864560766407578 ) ) ;
#6845=CARTESIAN_POINT ( 'NONE',  ( 3.480714749117373330, -12.43552623307873972, 30.55307653245132826 ) ) ;
#6847=ORIENTED_EDGE ( 'NONE', *, *, #22304, .T. ) ;
#6848=FACE_BOUND ( 'NONE', #17152, .T. ) ;
#6850=DIRECTION ( 'NONE',  ( -0.000000000000000000, -0.9848077530122086864, -0.1736481776669273613 ) ) ;
#6851=EDGE_CURVE ( 'NONE', #7007, #31488, #34702, .T. ) ;
#6852=EDGE_CURVE ( 'NONE', #11900, #77704, #83899, .T. ) ;
#6854=EDGE_CURVE ( 'NONE', #79445, #81564, #36932, .T. ) ;
#6855=VECTOR ( 'NONE', #3008, 1000.000000000000114 ) ;
#6856=FACE_OUTER_BOUND ( 'NONE', #79271, .T. ) ;
#6857=CARTESIAN_POINT ( 'NONE',  ( 2.980746006547773330, -11.56360843649121861, 33.07473185843129926 ) ) ;
#6859=ORIENTED_EDGE ( 'NONE', *, *, #50072, .F. ) ;
#6861=VECTOR ( 'NONE', #36062, 1000.000000000000000 ) ;
#6862=ORIENTED_EDGE ( 'NONE', *, *, #1298, .F. ) ;
#6863=ORIENTED_EDGE ( 'NONE', *, *, #79994, .F. ) ;
#6864=CARTESIAN_POINT ( 'NONE',  ( -3.007989561791164945, -11.60474049983370648, 33.02348890104160262 ) ) ;
#6865=EDGE_LOOP ( 'NONE', ( #18169, #87912 ) ) ;
#6866=VECTOR ( 'NONE', #88282, 1000.000000000000227 ) ;
#6867=CARTESIAN_POINT ( 'NONE',  ( 15.10007862765892206, -3.338472653186243644, 32.95098750199972670 ) ) ;
#6868=DIRECTION ( 'NONE',  ( -0.000000000000000000, 0.3420201433256694346, -0.9396926207859080948 ) ) ;
#6869=CARTESIAN_POINT ( 'NONE',  ( -7.976301815885543434, -3.625366637846544116, 33.29286588640298561 ) ) ;
#6870=CARTESIAN_POINT ( 'NONE',  ( 3.903846153846154632, -2.499999999999998668, 29.75000000000000355 ) ) ;
#6872=CARTESIAN_POINT ( 'NONE',  ( -2.531177251416254936, -5.113361153441932316, 34.14387501736621999 ) ) ;
#6873=CARTESIAN_POINT ( 'NONE',  ( -6.923076923076922462, -12.29105614889573062, 35.45975837776705220 ) ) ;
#6874=CARTESIAN_POINT ( 'NONE',  ( -8.519285359852727169, -2.986452184633680229, 32.43230066228895225 ) ) ;
#6875=VERTEX_POINT ( 'NONE', #1905 ) ;
#6876=ADVANCED_FACE ( 'NONE', ( #16310 ), #57290, .F. ) ;
#6878=VERTEX_POINT ( 'NONE', #23066 ) ;
#6879=CARTESIAN_POINT ( 'NONE',  ( -11.53846153846165912, -12.46129190930018460, 30.37095296980731973 ) ) ;
#6880=CARTESIAN_POINT ( 'NONE',  ( 1.515407192440173745, -5.582136614379148654, 34.36778462344220486 ) ) ;
#6881=CARTESIAN_POINT ( 'NONE',  ( -0.4615384615385840772, -8.656820664282941280, 34.87096338111179961 ) ) ;
#6882=CARTESIAN_POINT ( 'NONE',  ( 11.53846153846153832, -2.292212530054420494, 30.41441678777542634 ) ) ;
#6883=AXIS2_PLACEMENT_3D ( 'NONE', #86575, #24845, #18107 ) ;
#6884=CARTESIAN_POINT ( 'NONE',  ( -10.86540785267757947, -3.711651800289232028, 33.01384336483936011 ) ) ;
#6885=FACE_BOUND ( 'NONE', #9734, .T. ) ;
#6886=CARTESIAN_POINT ( 'NONE',  ( -7.173100147298380413, -3.520140089381497361, 33.17453946501458262 ) ) ;
#6887=VERTEX_POINT ( 'NONE', #50523 ) ;
#6888=CARTESIAN_POINT ( 'NONE',  ( 7.911408985666682270, -2.379036618887895305, 30.90682066428158592 ) ) ;
#6889=CARTESIAN_POINT ( 'NONE',  ( -1.254089682851821541, -2.882268652242222728, 31.66798894389554064 ) ) ;
#6890=CARTESIAN_POINT ( 'NONE',  ( -17.07692307692307665, -3.886160181151819604, 36.00935417666054406 ) ) ;
#6891=ORIENTED_EDGE ( 'NONE', *, *, #29407, .T. ) ;
#6892=CARTESIAN_POINT ( 'NONE',  ( -13.38461538461538325, -4.786620604624113540, 33.94971097300155094 ) ) ;
#6893=VECTOR ( 'NONE', #6343, 1000.000000000000227 ) ;
#6894=ORIENTED_EDGE ( 'NONE', *, *, #65779, .T. ) ;
#6895=FACE_BOUND ( 'NONE', #41773, .T. ) ;
#6896=CARTESIAN_POINT ( 'NONE',  ( -15.90384615384615330, -2.499999999999999112, 29.81604066197449754 ) ) ;
#6897=CARTESIAN_POINT ( 'NONE',  ( 15.23076923076923173, -13.49023893513002648, 31.06009739812518688 ) ) ;
#6898=DIRECTION ( 'NONE',  ( 0.000000000000000000, 1.000000000000000000, 0.000000000000000000 ) ) ;
#6899=VECTOR ( 'NONE', #1741, 1000.000000000000114 ) ;
#6900=ORIENTED_EDGE ( 'NONE', *, *, #80438, .F. ) ;
#6901=DIRECTION ( 'NONE',  ( -0.000000000000000000, 0.9396926207859093161, -0.3420201433256663259 ) ) ;
#6903=CARTESIAN_POINT ( 'NONE',  ( 12.46153846153846168, -6.386643153685126251, 34.62446782046654192 ) ) ;
#6904=CARTESIAN_POINT ( 'NONE',  ( 1.384615384615265343, -6.879047030192662504, 34.71129190930017927 ) ) ;
#6907=CARTESIAN_POINT ( 'NONE',  ( -16.08859101433330707, -10.33852847137154107, 34.16647553114620450 ) ) ;
#6910=CARTESIAN_POINT ( 'NONE',  ( -4.284537620513712675, -2.541943142973490666, 30.39792223712631980 ) ) ;
#6913=CARTESIAN_POINT ( 'NONE',  ( 14.17700084102475522, -8.999036380462717588, 34.52022231692819076 ) ) ;
#6915=CARTESIAN_POINT ( 'NONE',  ( -8.096130577096200653, -10.66389620160130036, 33.62221079203477103 ) ) ;
#6917=EDGE_CURVE ( 'NONE', #68189, #15487, #37008, .T. ) ;
#6919=CARTESIAN_POINT ( 'NONE',  ( 9.692307692307695177, -8.973038597847269315, 34.52809138561121927 ) ) ;
#6921=ORIENTED_EDGE ( 'NONE', *, *, #29572, .F. ) ;
#6922=DIRECTION ( 'NONE',  ( -0.000000000000000000, -0.9848077530122086864, -0.1736481776669273613 ) ) ;
#6923=ORIENTED_EDGE ( 'NONE', *, *, #13682, .F. ) ;
#6926=ORIENTED_EDGE ( 'NONE', *, *, #47745, .T. ) ;
#6928=EDGE_CURVE ( 'NONE', #85149, #35421, #44646, .T. ) ;
#6929=ORIENTED_EDGE ( 'NONE', *, *, #2543, .F. ) ;
#6930=CARTESIAN_POINT ( 'NONE',  ( -12.46153846153846168, -4.102666532097928531, 36.13435417666054406 ) ) ;
#6932=CARTESIAN_POINT ( 'NONE',  ( -14.05763788777885637, -2.920487667080175598, 32.31805714834170828 ) ) ;
#6933=DIRECTION ( 'NONE',  ( -0.000000000000000000, 0.3420201433256694901, -0.9396926207859082059 ) ) ;
#6934=DIRECTION ( 'NONE',  ( 0.000000000000000000, 0.9396926207859126468, 0.3420201433256571111 ) ) ;
#6935=AXIS2_PLACEMENT_3D ( 'NONE', #14383, #15274, #16154 ) ;
#6936=CARTESIAN_POINT ( 'NONE',  ( -6.988346923633242724, -9.528491918058357157, 34.59228464037090589 ) ) ;
#6938=DIRECTION ( 'NONE',  ( 0.000000000000000000, -6.938893903907222067E-15, 1.000000000000000000 ) ) ;
#6940=DIRECTION ( 'NONE',  ( -0.000000000000000000, -0.9848077530122086864, -0.1736481776669273613 ) ) ;
#6941=CARTESIAN_POINT ( 'NONE',  ( 6.673100179028332413, -10.06842814019191401, 34.32929386961144758 ) ) ;
#6942=CARTESIAN_POINT ( 'NONE',  ( 15.23076923076910916, -9.528491918059723176, 34.59228464037033035 ) ) ;
#6943=AXIS2_PLACEMENT_3D ( 'NONE', #84942, #24554, #52021 ) ;
#6945=DIRECTION ( 'NONE',  ( -0.000000000000000000, -0.3420201433256694901, -0.9396926207859082059 ) ) ;
#6946=CARTESIAN_POINT ( 'NONE',  ( -9.942330916529147800, -3.520140089381495585, 33.17453946501458262 ) ) ;
#6947=B_SPLINE_CURVE_WITH_KNOTS ( 'NONE', 3,
 ( #23232, #18263, #52030, #64207, #72747, #8074, #16921, #38082, #71862, #78619 ),
 .UNSPECIFIED., .F., .F.,
 ( 4, 2, 2, 2, 4 ),
 ( 0.000000000000000000, 0.0001954311584214072923, 0.0003908623168428145846, 0.0005862934752642218498, 0.0007817246336856291692 ),
 .UNSPECIFIED. ) ;
#6948=ORIENTED_EDGE ( 'NONE', *, *, #25515, .T. ) ;
#6950=LINE ( 'NONE', #44704, #68720 ) ;
#6951=CARTESIAN_POINT ( 'NONE',  ( 5.299934428535925335, -9.086983370893049639, 34.49168942202179267 ) ) ;
#6952=CARTESIAN_POINT ( 'NONE',  ( -0.4615384615384611200, -6.681629849574314051, 35.83090037661290239 ) ) ;
#6953=ADVANCED_FACE ( 'NONE', ( #78890 ), #16743, .F. ) ;
#6954=CARTESIAN_POINT ( 'NONE',  ( 9.942362112221147186, -12.01375889529407281, 32.43194544308182969 ) ) ;
#6955=B_SPLINE_CURVE_WITH_KNOTS ( 'NONE', 3,
 ( #4705, #32175, #86695, #18218, #25861, #79019, #31731, #59191, #10567, #45228 ),
 .UNSPECIFIED., .F., .F.,
 ( 4, 2, 2, 2, 4 ),
 ( 0.0007817359430256287049, 0.0009771253907249945886, 0.001172514838424360255, 0.001367904286123725922, 0.001563293733823091806 ),
 .UNSPECIFIED. ) ;
#6956=CARTESIAN_POINT ( 'NONE',  ( 9.692307692307570832, -11.67786785259630911, 32.92929555188603530 ) ) ;
#6959=ADVANCED_FACE ( 'NONE', ( #73486 ), #17188, .F. ) ;
#6960=ORIENTED_EDGE ( 'NONE', *, *, #37205, .F. ) ;
#6961=CARTESIAN_POINT ( 'NONE',  ( -14.53117723225664015, -12.69144148231606017, 30.53333754910549303 ) ) ;
#6962=ORIENTED_EDGE ( 'NONE', *, *, #55480, .F. ) ;
#6964=EDGE_CURVE ( 'NONE', #64638, #27377, #31513, .T. ) ;
#6965=CARTESIAN_POINT ( 'NONE',  ( 0.4615384615383382183, -5.094484230521993062, 34.41647553114689373 ) ) ;
#6967=CARTESIAN_POINT ( 'NONE',  ( -7.173076923076921574, -7.500000000000001776, 35.00000000000000000 ) ) ;
#6968=CARTESIAN_POINT ( 'NONE',  ( -15.48079246806219267, -3.202444869320336451, 32.30641848906366675 ) ) ;
#6971=ADVANCED_FACE ( 'NONE', ( #79343 ), #86105, .F. ) ;
#6972=ORIENTED_EDGE ( 'NONE', *, *, #63381, .F. ) ;
#6973=EDGE_LOOP ( 'NONE', ( #85060, #43370 ) ) ;
#6975=EDGE_CURVE ( 'NONE', #45215, #47964, #47624, .T. ) ;
#6976=CARTESIAN_POINT ( 'NONE',  ( 17.07692307692307665, -9.905515769479276145, 34.41647553114623292 ) ) ;
#6977=CARTESIAN_POINT ( 'NONE',  ( -12.52762084089859584, -12.62096338111211580, 30.90682066428152908 ) ) ;
#6978=CARTESIAN_POINT ( 'NONE',  ( -3.480745961711584346, -9.943427161483782584, 34.11278801902876978 ) ) ;
#6979=CARTESIAN_POINT ( 'NONE',  ( 16.28463796167094202, -9.804649428959608670, 34.18742332936588468 ) ) ;
#6980=VECTOR ( 'NONE', #12241, 1000.000000000000227 ) ;
#6981=CARTESIAN_POINT ( 'NONE',  ( -7.715363405186896451, -3.957578996910242619, 33.62503395064540257 ) ) ;
#6982=CARTESIAN_POINT ( 'NONE',  ( -10.48485891362104816, -12.27024696741798948, 31.24895572276497546 ) ) ;
#6984=EDGE_CURVE ( 'NONE', #13048, #61364, #51916, .T. ) ;
#6987=VECTOR ( 'NONE', #73678, 1000.000000000000227 ) ;
#6988=CARTESIAN_POINT ( 'NONE',  ( 9.692307692307570832, -6.835583212225970762, 34.95778746994575670 ) ) ;
#6989=ORIENTED_EDGE ( 'NONE', *, *, #785, .F. ) ;
#6991=CARTESIAN_POINT ( 'NONE',  ( 17.14299041027315695, -10.67929555188718282, 33.92786785259544757 ) ) ;
#6992=CARTESIAN_POINT ( 'NONE',  ( -12.39547112818838492, -11.91647553114624358, 32.58852847137148245 ) ) ;
#6993=AXIS2_PLACEMENT_3D ( 'NONE', #58525, #42828, #86021 ) ;
#6995=ORIENTED_EDGE ( 'NONE', *, *, #82028, .F. ) ;
#6997=ORIENTED_EDGE ( 'NONE', *, *, #38899, .T. ) ;
#6999=FACE_BOUND ( 'NONE', #66921, .T. ) ;
#7000=CARTESIAN_POINT ( 'NONE',  ( 4.826946332874483936, -4.818429247618089661, 34.26397095200675125 ) ) ;
#7001=CARTESIAN_POINT ( 'NONE',  ( 4.153846153846154188, -2.249999999999998668, 29.50000000000001421 ) ) ;
#7002=ORIENTED_EDGE ( 'NONE', *, *, #60808, .F. ) ;
#7003=CARTESIAN_POINT ( 'NONE',  ( 3.230769230769231726, -12.78798330534102767, 29.49999999999997868 ) ) ;
#7004=CARTESIAN_POINT ( 'NONE',  ( 6.673053698855464511, -12.07920672191015221, 32.31858351112116168 ) ) ;
#7005=DIRECTION ( 'NONE',  ( -0.000000000000000000, -0.9848077530122085754, -0.1736481776669273613 ) ) ;
#7006=LINE ( 'NONE', #69594, #82636 ) ;
#7007=VERTEX_POINT ( 'NONE', #67165 ) ;
#7008=CARTESIAN_POINT ( 'NONE',  ( 6.065255571276024327, -8.613356846314928816, 34.62446782046653482 ) ) ;
#7009=CARTESIAN_POINT ( 'NONE',  ( -4.088591014333315066, -10.33852847137154107, 34.16647553114620450 ) ) ;
#7011=DIRECTION ( 'NONE',  ( -0.000000000000000000, 0.5000000000000011102, -0.8660254037844381525 ) ) ;
#7012=DIRECTION ( 'NONE',  ( 0.000000000000000000, 1.000000000000000000, 0.000000000000000000 ) ) ;
#7013=FACE_BOUND ( 'NONE', #15182, .T. ) ;
#7014=CARTESIAN_POINT ( 'NONE',  ( -9.019230769230768274, -2.499999999999998668, 29.75000000000000355 ) ) ;
#7015=CARTESIAN_POINT ( 'NONE',  ( -17.20707104665477516, -11.04286588640298561, 33.62463336215343901 ) ) ;
#7016=FACE_OUTER_BOUND ( 'NONE', #84005, .T. ) ;
#7017=CARTESIAN_POINT ( 'NONE',  ( -18.24997674404858827, -2.318417181685855422, 30.59732222474233865 ) ) ;
#7018=CARTESIAN_POINT ( 'NONE',  ( 15.48071474911737333, -10.05730279482229683, 34.04704008940765902 ) ) ;
#7019=CARTESIAN_POINT ( 'NONE',  ( -1.384615384615383471, -13.53365097954675988, 30.81389545987213552 ) ) ;
#7022=ORIENTED_EDGE ( 'NONE', *, *, #8986, .F. ) ;
#7023=CARTESIAN_POINT ( 'NONE',  ( -5.869474561766357290, -11.04252011169590020, 33.62494198852677130 ) ) ;
#7024=ORIENTED_EDGE ( 'NONE', *, *, #49260, .T. ) ;
#7025=DIRECTION ( 'NONE',  ( -0.000000000000000000, 0.6427876096865404731, -0.7660444431189771253 ) ) ;
#7027=DIRECTION ( 'NONE',  ( 0.000000000000000000, 0.000000000000000000, 1.000000000000000000 ) ) ;
#7028=ADVANCED_FACE ( 'NONE', ( #25732 ), #19859, .F. ) ;
#7029=LINE ( 'NONE', #88592, #15737 ) ;
#7030=CARTESIAN_POINT ( 'NONE',  ( -9.561782254074051579, -11.66157788607254098, 32.95092075102925833 ) ) ;
#7031=ORIENTED_EDGE ( 'NONE', *, *, #38234, .T. ) ;
#7032=CARTESIAN_POINT ( 'NONE',  ( 17.77717190236512224, -7.369209533119136069, 34.99857337881830688 ) ) ;
#7034=DIRECTION ( 'NONE',  ( -0.000000000000000000, -0.6427876096865404731, -0.7660444431189770143 ) ) ;
#7038=CARTESIAN_POINT ( 'NONE',  ( 6.923076923076924238, -4.098570777380720287, 33.41473453929634729 ) ) ;
#7039=CARTESIAN_POINT ( 'NONE',  ( 7.846153846153846700, -6.343179335718451384, 34.87096338111211935 ) ) ;
#7040=EDGE_CURVE ( 'NONE', #42225, #2251, #81131, .T. ) ;
#7041=B_SPLINE_CURVE_WITH_KNOTS ( 'NONE', 3,
 ( #34169, #13453, #87364, #80604, #32845, #18888, #53551, #19334, #46356, #25196 ),
 .UNSPECIFIED., .F., .F.,
 ( 4, 2, 2, 2, 4 ),
 ( 0.0007817359430256315238, 0.0009771253907249980580, 0.001172514838424364592, 0.001367904286123730910, 0.001563293733823097444 ),
 .UNSPECIFIED. ) ;
#7043=CARTESIAN_POINT ( 'NONE',  ( -18.00000000000012079, -11.67786785259630733, 32.92929555188604240 ) ) ;
#7044=DIRECTION ( 'NONE',  ( -0.000000000000000000, 1.000000000000000000, -0.000000000000000000 ) ) ;
#7045=B_SPLINE_CURVE_WITH_KNOTS ( 'NONE', 3,
 ( #42625, #68761, #7059, #28209, #83169, #21460, #13370, #21004, #56575, #13814 ),
 .UNSPECIFIED., .F., .F.,
 ( 4, 2, 2, 2, 4 ),
 ( 0.000000000000000000, 0.0001954339881912763499, 0.0003908679763825526998, 0.0005863019645738316247, 0.0007817359527651106038 ),
 .UNSPECIFIED. ) ;
#7046=EDGE_LOOP ( 'NONE', ( #36217, #44593, #5072, #64822, #89091, #69780 ) ) ;
#7047=EDGE_CURVE ( 'NONE', #535, #10551, #71215, .T. ) ;
#7048=CARTESIAN_POINT ( 'NONE',  ( 9.019176287578908102, -10.05730279482229683, 34.04704008940765902 ) ) ;
#7049=B_SPLINE_CURVE_WITH_KNOTS ( 'NONE', 3,
 ( #62821, #56529, #37134, #23625, #70932, #8350, #43017, #84021, #9242, #85339 ),
 .UNSPECIFIED., .F., .F.,
 ( 4, 2, 2, 2, 4 ),
 ( 0.0007817359430256304396, 0.0009771253907249963233, 0.001172514838424362424, 0.001367904286123728524, 0.001563293733823094408 ),
 .UNSPECIFIED. ) ;
#7051=CARTESIAN_POINT ( 'NONE',  ( 2.307692307692309264, -4.661471528628507777, 34.16647553114623292 ) ) ;
#7052=AXIS2_PLACEMENT_3D ( 'NONE', #49722, #56486, #85291 ) ;
#7053=CARTESIAN_POINT ( 'NONE',  ( 4.088523238353977796, -7.749976743299137993, 34.99404534957040624 ) ) ;
#7055=CARTESIAN_POINT ( 'NONE',  ( -4.153846153846274980, -2.657715359629662988, 31.77849191805970364 ) ) ;
#7056=CARTESIAN_POINT ( 'NONE',  ( -14.53061852520844965, -11.24512374952581872, 33.06303171183252942 ) ) ;
#7057=CARTESIAN_POINT ( 'NONE',  ( 8.769230769230768274, -1.215029322943914858, 32.30358669280327177 ) ) ;
#7058=EDGE_LOOP ( 'NONE', ( #32320, #9191 ) ) ;
#7059=CARTESIAN_POINT ( 'NONE',  ( -8.069032528582491537, -7.630691491037285168, 34.74850469731151748 ) ) ;
#7060=CARTESIAN_POINT ( 'NONE',  ( -17.14267650523641251, -7.249945578846654470, 34.99404164642496795 ) ) ;
#7061=VECTOR ( 'NONE', #54276, 1000.000000000000227 ) ;
#7062=CARTESIAN_POINT ( 'NONE',  ( -10.54931728203453822, -9.058645607665452459, 34.76329471203371924 ) ) ;
#7063=ADVANCED_FACE ( 'NONE', ( #75683 ), #88348, .F. ) ;
#7064=VECTOR ( 'NONE', #82267, 1000.000000000000227 ) ;
#7065=CARTESIAN_POINT ( 'NONE',  ( 5.010839665967194989, -4.098570777380720287, 33.41473453929634729 ) ) ;
#7066=CARTESIAN_POINT ( 'NONE',  ( -13.51476259405360203, -11.93770438780619259, 32.05411857736982029 ) ) ;
#7068=ORIENTED_EDGE ( 'NONE', *, *, #75334, .T. ) ;
#7069=EDGE_CURVE ( 'NONE', #75335, #83859, #64663, .T. ) ;
#7070=EDGE_LOOP ( 'NONE', ( #54166, #66474 ) ) ;
#7073=EDGE_CURVE ( 'NONE', #11434, #5312, #13171, .T. ) ;
#7075=CARTESIAN_POINT ( 'NONE',  ( -17.32692307692308020, -7.566082377512564960, 35.00000000000000711 ) ) ;
#7076=CARTESIAN_POINT ( 'NONE',  ( 17.20744851515671670, -11.66157788607254275, 32.95092075102925833 ) ) ;
#7077=B_SPLINE_CURVE_WITH_KNOTS ( 'NONE', 3,
 ( #86059, #50906, #84299, #2731, #22576, #37865, #57253, #10398, #30227, #24337 ),
 .UNSPECIFIED., .F., .F.,
 ( 4, 2, 2, 2, 4 ),
 ( 0.000000000000000000, 0.0001954311564186860613, 0.0003908623128373721225, 0.0005862934692560581567, 0.0007817246256747442451 ),
 .UNSPECIFIED. ) ;
#7078=ORIENTED_EDGE ( 'NONE', *, *, #4318, .F. ) ;
#7079=EDGE_LOOP ( 'NONE', ( #35890, #9296, #56081, #20142 ) ) ;
#7080=EDGE_CURVE ( 'NONE', #29264, #39978, #24963, .T. ) ;
#7081=ORIENTED_EDGE ( 'NONE', *, *, #44105, .T. ) ;
#7082=CARTESIAN_POINT ( 'NONE',  ( -7.146561847641254239, -8.539481045369598178, 34.89627647299170832 ) ) ;
#7083=VERTEX_POINT ( 'NONE', #74366 ) ;
#7084=CARTESIAN_POINT ( 'NONE',  ( -14.30769230769230660, -8.810774026931790459, 35.74407628777942847 ) ) ;
#7085=VECTOR ( 'NONE', #67739, 1000.000000000000114 ) ;
#7086=CARTESIAN_POINT ( 'NONE',  ( -2.307692307692305711, -2.486705287966279876, 31.30864560766543647 ) ) ;
#7087=CARTESIAN_POINT ( 'NONE',  ( 6.988332062589761584, -5.094484230520773593, 34.41647553114626845 ) ) ;
#7088=DIRECTION ( 'NONE',  ( -0.000000000000000000, 0.8660254037844397068, -0.4999999999999978906 ) ) ;
#7089=ORIENTED_EDGE ( 'NONE', *, *, #10205, .T. ) ;
#7090=EDGE_CURVE ( 'NONE', #4584, #45693, #57182, .T. ) ;
#7091=ORIENTED_EDGE ( 'NONE', *, *, #28640, .F. ) ;
#7092=ORIENTED_EDGE ( 'NONE', *, *, #85130, .T. ) ;
#7094=LINE ( 'NONE', #12527, #34376 ) ;
#7095=ORIENTED_EDGE ( 'NONE', *, *, #38218, .F. ) ;
#7096=CARTESIAN_POINT ( 'NONE',  ( -11.31544869436814338, -12.64618726649961289, 30.78989965857442712 ) ) ;
#7097=ADVANCED_FACE ( 'NONE', ( #70261 ), #917, .F. ) ;
#7098=EDGE_CURVE ( 'NONE', #7083, #44733, #55416, .T. ) ;
#7099=FACE_OUTER_BOUND ( 'NONE', #54374, .T. ) ;
#7100=VERTEX_POINT ( 'NONE', #28844 ) ;
#7101=CARTESIAN_POINT ( 'NONE',  ( 16.28437185560972011, -3.816742781228458448, 33.13167719472716044 ) ) ;
#7102=CARTESIAN_POINT ( 'NONE',  ( 12.52760579488853665, -9.058645607665452459, 34.76329471203371924 ) ) ;
#7103=ORIENTED_EDGE ( 'NONE', *, *, #44196, .F. ) ;
#7104=FACE_BOUND ( 'NONE', #40317, .T. ) ;
#7106=DIRECTION ( 'NONE',  ( -0.000000000000000000, 1.000000000000000000, 3.491481338843133355E-15 ) ) ;
#7107=CARTESIAN_POINT ( 'NONE',  ( 13.63466980452883881, -6.523592122091592671, 34.90882529074906415 ) ) ;
#7108=CYLINDRICAL_SURFACE ( 'NONE', #27931, 0.2499999999999994726 ) ;
#7109=CARTESIAN_POINT ( 'NONE',  ( 18.06606733335007675, -2.833524468853757750, 32.15551576947925838 ) ) ;
#7110=VECTOR ( 'NONE', #52517, 1000.000000000000114 ) ;
#7111=CARTESIAN_POINT ( 'NONE',  ( 4.826899839630108602, -10.05641848906368097, 34.04755513067966177 ) ) ;
#7113=CYLINDRICAL_SURFACE ( 'NONE', #29474, 0.2500000000000002220 ) ;
#7114=DIRECTION ( 'NONE',  ( -0.000000000000000000, 0.6427876096865404731, -0.7660444431189771253 ) ) ;
#7115=EDGE_LOOP ( 'NONE', ( #80553, #1662 ) ) ;
#7116=CARTESIAN_POINT ( 'NONE',  ( 14.55774661933062042, -12.41262288849542017, 30.68299917996395010 ) ) ;
#7118=B_SPLINE_CURVE_WITH_KNOTS ( 'NONE', 3,
 ( #33060, #12788, #5145, #60527, #53770, #60969, #26744, #54204, #32610, #81257 ),
 .UNSPECIFIED., .F., .F.,
 ( 4, 2, 2, 2, 4 ),
 ( 0.000000000000000000, 0.0001954311564186879044, 0.0003908623128373758088, 0.0005862934692560636861, 0.0007817246256747516176 ),
 .UNSPECIFIED. ) ;
#7119=AXIS2_PLACEMENT_3D ( 'NONE', #389, #13449, #55760 ) ;
#7120=EDGE_LOOP ( 'NONE', ( #75564, #24034 ) ) ;
#7121=CIRCLE ( 'NONE', #43123, 0.2500000000000002220 ) ;
#7123=LINE ( 'NONE', #35477, #25711 ) ;
#7124=CARTESIAN_POINT ( 'NONE',  ( -7.623141002060451754, -2.308499170217967134, 30.53291367094873721 ) ) ;
#7125=B_SPLINE_CURVE_WITH_KNOTS ( 'NONE', 3,
 ( #26719, #54179, #54622, #41566, #60944, #585, #55078, #20412, #47424, #61377 ),
 .UNSPECIFIED., .F., .F.,
 ( 4, 2, 2, 2, 4 ),
 ( 0.000000000000000000, 0.0001954339857564075286, 0.0003908679715128150572, 0.0005863019572692225586, 0.0007817359430256301143 ),
 .UNSPECIFIED. ) ;
#7128=CARTESIAN_POINT ( 'NONE',  ( -9.019254006523732770, -5.851115903089112003, 34.47074536777953568 ) ) ;
#7129=FACE_BOUND ( 'NONE', #24342, .T. ) ;
#7130=CARTESIAN_POINT ( 'NONE',  ( -18.00000000000012079, -3.300289026999231545, 32.46337939537709616 ) ) ;
#7131=CARTESIAN_POINT ( 'NONE',  ( 15.29683758177167441, -12.10708131394839704, 31.69288490824020954 ) ) ;
#7132=CARTESIAN_POINT ( 'NONE',  ( -13.51476335434707821, -2.373036134822904319, 30.88089517874952250 ) ) ;
#7133=CARTESIAN_POINT ( 'NONE',  ( 1.449870524128224814, -12.70778746994558439, 30.41441678777537305 ) ) ;
#7135=CARTESIAN_POINT ( 'NONE',  ( 2.307692307692187583, -3.300289026999228881, 32.46337939537708905 ) ) ;
#7138=ORIENTED_EDGE ( 'NONE', *, *, #64704, .F. ) ;
#7140=CARTESIAN_POINT ( 'NONE',  ( 5.142991427925513115, -6.386643153685127139, 34.62446782046654192 ) ) ;
#7141=CARTESIAN_POINT ( 'NONE',  ( -15.48079245499068612, -5.765609946408404518, 34.70566812827425451 ) ) ;
#7142=CARTESIAN_POINT ( 'NONE',  ( 16.21991348719623360, -2.833524468853757750, 32.15551576947925838 ) ) ;
#7143=CARTESIAN_POINT ( 'NONE',  ( -8.835313148590902443, -8.164416787775445883, 34.95778746994557906 ) ) ;
#7144=CARTESIAN_POINT ( 'NONE',  ( -16.37733109757011007, -12.24155766932282496, 31.33739205006857986 ) ) ;
#7146=CARTESIAN_POINT ( 'NONE',  ( 6.673100179028331524, -2.318417181685854978, 30.59732222474233865 ) ) ;
#7148=CARTESIAN_POINT ( 'NONE',  ( 3.230769230769108269, -4.320704448113951379, 33.92786785259630022 ) ) ;
#7149=CARTESIAN_POINT ( 'NONE',  ( 1.384615384615386802, -5.557115091759785130, 34.35708131394839171 ) ) ;
#7150=CARTESIAN_POINT ( 'NONE',  ( -15.16551365949320562, -11.48612834413965977, 32.76840700105972815 ) ) ;
#7151=CARTESIAN_POINT ( 'NONE',  ( 16.15384615384615330, -4.786620604624113540, 33.94971097300155094 ) ) ;
#7152=CARTESIAN_POINT ( 'NONE',  ( -3.480792454990687013, -10.18141759479407327, 34.26406193332782379 ) ) ;
#7153=B_SPLINE_CURVE_WITH_KNOTS ( 'NONE', 3,
 ( #67679, #60913, #26688, #61343, #54145, #88858, #38203, #77093, #2301, #36116 ),
 .UNSPECIFIED., .F., .F.,
 ( 4, 2, 2, 2, 4 ),
 ( 0.000000000000000000, 0.0001954311564186854107, 0.0003908623128373708215, 0.0005862934692560562051, 0.0007817246256747416430 ),
 .UNSPECIFIED. ) ;
#7155=CYLINDRICAL_SURFACE ( 'NONE', #52862, 0.2500000000000008882 ) ;
#7156=B_SPLINE_CURVE_WITH_KNOTS ( 'NONE', 3,
 ( #11825, #39303, #12259, #4159, #5059, #32523, #65423, #23980, #31644, #3273 ),
 .UNSPECIFIED., .F., .F.,
 ( 4, 2, 2, 2, 4 ),
 ( 0.000000000000000000, 0.0001954339857564097512, 0.0003908679715128195024, 0.0005863019572692292807, 0.0007817359430256390048 ),
 .UNSPECIFIED. ) ;
#7157=ORIENTED_EDGE ( 'NONE', *, *, #86706, .T. ) ;
#7158=AXIS2_PLACEMENT_3D ( 'NONE', #11010, #72700, #33055 ) ;
#7159=B_SPLINE_CURVE_WITH_KNOTS ( 'NONE', 3,
 ( #10991, #66820, #85320, #10546, #73132, #18643, #65482, #51495, #23602, #58719 ),
 .UNSPECIFIED., .F., .F.,
 ( 4, 2, 2, 2, 4 ),
 ( 0.0007817246256747460882, 0.0009771112852218900684, 0.001172497944769033832, 0.001367884604316177595, 0.001563271263863321575 ),
 .UNSPECIFIED. ) ;
#7160=CARTESIAN_POINT ( 'NONE',  ( -0.3310127597748955264, -3.816742781228458448, 33.13167719472716044 ) ) ;
#7161=CARTESIAN_POINT ( 'NONE',  ( 7.623226887246995709, -4.762599654559228846, 34.23009711892697737 ) ) ;
#7164=CYLINDRICAL_SURFACE ( 'NONE', #80075, 0.2499999999999986955 ) ;
#7165=VERTEX_POINT ( 'NONE', #55856 ) ;
#7166=CARTESIAN_POINT ( 'NONE',  ( -9.692307692307691624, -5.471508081941601098, 34.59228464037088457 ) ) ;
#7167=CARTESIAN_POINT ( 'NONE',  ( -5.749999999998578915, -7.500000000000154543, 35.00000000000007105 ) ) ;
#7170=CARTESIAN_POINT ( 'NONE',  ( -5.011667505647053211, -10.21337939537593620, 33.94971097300152252 ) ) ;
#7171=VERTEX_POINT ( 'NONE', #49550 ) ;
#7174=ORIENTED_EDGE ( 'NONE', *, *, #88331, .T. ) ;
#7175=CARTESIAN_POINT ( 'NONE',  ( 6.923076923076924238, -1.951392089020283160, 34.73218667398347748 ) ) ;
#7176=CARTESIAN_POINT ( 'NONE',  ( 2.530705151785704210, -8.282913670948747864, 34.94150082978203642 ) ) ;
#7178=CARTESIAN_POINT ( 'NONE',  ( 2.057715563643717882, -12.65889640711025521, 30.72598325615533454 ) ) ;
#7179=ORIENTED_EDGE ( 'NONE', *, *, #39305, .T. ) ;
#7180=EDGE_LOOP ( 'NONE', ( #43433, #77292, #3193, #88759 ) ) ;
#7181=CARTESIAN_POINT ( 'NONE',  ( -6.857009589726848375, -8.164416787775445883, 34.95778746994558617 ) ) ;
#7182=EDGE_CURVE ( 'NONE', #68002, #14815, #50414, .T. ) ;
#7183=ORIENTED_EDGE ( 'NONE', *, *, #62280, .T. ) ;
#7185=AXIS2_PLACEMENT_3D ( 'NONE', #85524, #86436, #17959 ) ;
#7186=DIRECTION ( 'NONE',  ( -0.000000000000000000, 0.6427876096865404731, -0.7660444431189771253 ) ) ;
#7187=CARTESIAN_POINT ( 'NONE',  ( 12.52679403281448600, -9.442884908240273489, 34.35708131394835618 ) ) ;
#7188=CARTESIAN_POINT ( 'NONE',  ( -1.607542343522232464, -11.43668979543635089, 33.22377378376089752 ) ) ;
#7191=CARTESIAN_POINT ( 'NONE',  ( -2.307692307691991296, -2.255955759149395501, 30.00000000000324363 ) ) ;
#7192=VECTOR ( 'NONE', #52780, 1000.000000000000227 ) ;
#7194=AXIS2_PLACEMENT_3D ( 'NONE', #5623, #12823, #20901 ) ;
#7195=CARTESIAN_POINT ( 'NONE',  ( 10.39245839786846659, -12.15238873228292071, 31.58232369045353849 ) ) ;
#7197=EDGE_CURVE ( 'NONE', #49278, #78341, #42361, .T. ) ;
#7198=VERTEX_POINT ( 'NONE', #29726 ) ;
#7199=CARTESIAN_POINT ( 'NONE',  ( 18.13079044096694759, -9.084667340241228572, 34.75534355489798344 ) ) ;
#7200=ORIENTED_EDGE ( 'NONE', *, *, #8617, .F. ) ;
#7201=CARTESIAN_POINT ( 'NONE',  ( -5.076923076923075762, -4.661471528628507777, 34.16647553114623292 ) ) ;
#7202=ORIENTED_EDGE ( 'NONE', *, *, #15942, .T. ) ;
#7203=CARTESIAN_POINT ( 'NONE',  ( -13.25377705412862106, -7.277220318596961057, 34.99547417642776992 ) ) ;
#7204=DIRECTION ( 'NONE',  ( -0.000000000000000000, 0.8660254037844399289, -0.4999999999999980016 ) ) ;
#7205=ORIENTED_EDGE ( 'NONE', *, *, #69818, .T. ) ;
#7206=CARTESIAN_POINT ( 'NONE',  ( -9.942307692307691624, -2.499999999999998668, 29.75000000000000355 ) ) ;
#7208=CARTESIAN_POINT ( 'NONE',  ( -16.08859101433330707, -5.941354392334603496, 34.76329471203374055 ) ) ;
#7209=EDGE_LOOP ( 'NONE', ( #36281, #17636, #10798, #64824 ) ) ;
#7210=CARTESIAN_POINT ( 'NONE',  ( -22.75000000000000000, -2.249999999999999556, 27.25000000000000000 ) ) ;
#7211=B_SPLINE_CURVE_WITH_KNOTS ( 'NONE', 3,
 ( #3012, #85009, #10233, #15663, #57965, #30925, #23290, #23725, #58393, #85889 ),
 .UNSPECIFIED., .F., .F.,
 ( 4, 2, 2, 2, 4 ),
 ( 0.000000000000000000, 0.0001954311564186871455, 0.0003908623128373742909, 0.0005862934692560614093, 0.0007817246256747485819 ),
 .UNSPECIFIED. ) ;
#7212=EDGE_CURVE ( 'NONE', #18418, #51867, #48565, .T. ) ;
#7213=EDGE_CURVE ( 'NONE', #60134, #54717, #27036, .T. ) ;
#7215=CARTESIAN_POINT ( 'NONE',  ( -6.857821783564084228, -5.094484230520773593, 34.41647553114626845 ) ) ;
#7216=B_SPLINE_CURVE_WITH_KNOTS ( 'NONE', 3,
 ( #18766, #20090, #75044, #88577, #12883, #13770, #40374, #89014, #67390, #33160 ),
 .UNSPECIFIED., .F., .F.,
 ( 4, 2, 2, 2, 4 ),
 ( 0.000000000000000000, 0.0001954311564186875792, 0.0003908623128373751583, 0.0005862934692560627103, 0.0007817246256747503166 ),
 .UNSPECIFIED. ) ;
#7218=CARTESIAN_POINT ( 'NONE',  ( 16.85399685940693004, -2.758268499246657068, 31.33685645148948851 ) ) ;
#7219=FACE_BOUND ( 'NONE', #83397, .T. ) ;
#7220=CARTESIAN_POINT ( 'NONE',  ( -3.230769230769229949, -7.500000000000001776, 35.04278698407183867 ) ) ;
#7221=DIRECTION ( 'NONE',  ( 0.000000000000000000, 0.8660254037844377084, -0.5000000000000015543 ) ) ;
#7222=CARTESIAN_POINT ( 'NONE',  ( -15.93106648486808119, -4.989023458446560255, 34.36081565061822118 ) ) ;
#7223=CARTESIAN_POINT ( 'NONE',  ( 10.61538461538461675, -9.905515769479276145, 34.41647553114623292 ) ) ;
#7224=EDGE_CURVE ( 'NONE', #48794, #53001, #68992, .T. ) ;
#7225=CARTESIAN_POINT ( 'NONE',  ( 18.00000000000000000, -6.386643153685126251, 34.62446782046654192 ) ) ;
#7227=CYLINDRICAL_SURFACE ( 'NONE', #74890, 0.2499999999999997502 ) ;
#7228=ORIENTED_EDGE ( 'NONE', *, *, #72529, .T. ) ;
#7229=ORIENTED_EDGE ( 'NONE', *, *, #44604, .T. ) ;
#7230=CARTESIAN_POINT ( 'NONE',  ( -17.07692307692319744, -10.21337939537710326, 33.94971097300076224 ) ) ;
#7232=CARTESIAN_POINT ( 'NONE',  ( -11.60454494941741999, -11.69971097300155272, 32.46337939537587403 ) ) ;
#7233=FACE_OUTER_BOUND ( 'NONE', #4059, .T. ) ;
#7234=DIRECTION ( 'NONE',  ( 0.000000000000000000, 0.9396926207859126468, -0.3420201433256571111 ) ) ;
#7236=EDGE_LOOP ( 'NONE', ( #23234, #40364, #3451, #87851 ) ) ;
#7237=CARTESIAN_POINT ( 'NONE',  ( -5.300408001487404874, -5.827078755546623690, 34.72654668319379567 ) ) ;
#7238=CARTESIAN_POINT ( 'NONE',  ( 1.607394925883796510, -12.24180327182771855, 31.33663988360758168 ) ) ;
#7239=CARTESIAN_POINT ( 'NONE',  ( -8.834501215191544077, -12.27809138561121394, 31.22303859784730307 ) ) ;
#7240=VECTOR ( 'NONE', #63373, 1000.000000000000114 ) ;
#7241=CARTESIAN_POINT ( 'NONE',  ( 3.100622021331011169, -3.285722584762969856, 32.44110544564090759 ) ) ;
#7242=VERTEX_POINT ( 'NONE', #9013 ) ;
#7243=ORIENTED_EDGE ( 'NONE', *, *, #4840, .T. ) ;
#7245=VERTEX_POINT ( 'NONE', #49980 ) ;
#7246=CARTESIAN_POINT ( 'NONE',  ( -9.692307692307691624, -12.37446782046654192, 30.86335684631486131 ) ) ;
#7247=ORIENTED_EDGE ( 'NONE', *, *, #50545, .T. ) ;
#7248=B_SPLINE_CURVE_WITH_KNOTS ( 'NONE', 3,
 ( #26167, #33375, #66712, #25726, #60835, #81567, #18529, #5012, #74360, #18971 ),
 .UNSPECIFIED., .F., .F.,
 ( 4, 2, 2, 2, 4 ),
 ( 0.0007817359430256326080, 0.0009771253907249993591, 0.001172514838424366327, 0.001367904286123733078, 0.001563293733823099829 ),
 .UNSPECIFIED. ) ;
#7249=CARTESIAN_POINT ( 'NONE',  ( -9.822999158975250111, -12.38065189839062263, 30.83690757178629482 ) ) ;
#7250=CARTESIAN_POINT ( 'NONE',  ( 15.36155967173618286, -3.957578996910242619, 33.62503395064540257 ) ) ;
#7251=DIRECTION ( 'NONE',  ( -0.000000000000000000, -0.9848077530122085754, -0.1736481776669273613 ) ) ;
#7254=VECTOR ( 'NONE', #55735, 1000.000000000000227 ) ;
#7255=CARTESIAN_POINT ( 'NONE',  ( 9.692307692307695177, -5.557115091759785130, 34.35708131394839171 ) ) ;
#7256=ORIENTED_EDGE ( 'NONE', *, *, #66349, .F. ) ;
#7258=CARTESIAN_POINT ( 'NONE',  ( 4.283891209765926966, -2.254550872974306674, 29.97347326024527447 ) ) ;
#7259=CARTESIAN_POINT ( 'NONE',  ( -11.53846153846166089, -11.67786785259630911, 32.92929555188603530 ) ) ;
#7260=ORIENTED_EDGE ( 'NONE', *, *, #27981, .F. ) ;
#7261=CARTESIAN_POINT ( 'NONE',  ( -17.01085574357300345, -8.164416787775445883, 34.95778746994558617 ) ) ;
#7262=CYLINDRICAL_SURFACE ( 'NONE', #9622, 0.2499999999999995559 ) ;
#7264=CARTESIAN_POINT ( 'NONE',  ( -6.923076923076922462, -12.78798330534102767, 29.49999999999997868 ) ) ;
#7265=CARTESIAN_POINT ( 'NONE',  ( 2.307692307692309264, -2.486705287966279876, 31.30864560766543647 ) ) ;
#7266=CARTESIAN_POINT ( 'NONE',  ( -3.230769230769352962, -11.06231777344772027, 33.60647404775119895 ) ) ;
#7267=CARTESIAN_POINT ( 'NONE',  ( -0.6850233861027952287, -2.612411019501189369, 31.66733052389439962 ) ) ;
#7270=CARTESIAN_POINT ( 'NONE',  ( -3.164701897419154975, -6.343179335718452272, 34.87096338111212646 ) ) ;
#7272=CARTESIAN_POINT ( 'NONE',  ( 8.068933387422251968, -2.600157965045225783, 30.74683119005207743 ) ) ;
#7273=CARTESIAN_POINT ( 'NONE',  ( -13.31854703361294767, -8.120952969808772792, 34.71129190929999453 ) ) ;
#7274=ORIENTED_EDGE ( 'NONE', *, *, #45958, .F. ) ;
#7275=CARTESIAN_POINT ( 'NONE',  ( 2.373858914283949240, -7.250054591869667497, 34.99404684341514127 ) ) ;
#7276=CARTESIAN_POINT ( 'NONE',  ( 11.47237915910140771, -3.937682226553330445, 33.60647404775217240 ) ) ;
#7277=ADVANCED_FACE ( 'NONE', ( #15768 ), #62172, .F. ) ;
#7278=CARTESIAN_POINT ( 'NONE',  ( -1.161604033002533454, -6.503523203565942268, 34.64991518177335195 ) ) ;
#7279=LINE ( 'NONE', #49143, #84516 ) ;
#7280=CARTESIAN_POINT ( 'NONE',  ( -14.30769230769230660, -2.833524468853757305, 32.15551576947925838 ) ) ;
#7281=ORIENTED_EDGE ( 'NONE', *, *, #39271, .F. ) ;
#7282=CARTESIAN_POINT ( 'NONE',  ( -12.23852710992561121, -9.086983370893049639, 34.49168942202179267 ) ) ;
#7283=CARTESIAN_POINT ( 'NONE',  ( 3.361561038594018669, -12.11778462344221019, 31.66786338562085135 ) ) ;
#7284=CYLINDRICAL_SURFACE ( 'NONE', #30659, 0.2499999999999994726 ) ;
#7288=ADVANCED_FACE ( 'NONE', ( #63934 ), #2231, .F. ) ;
#7289=ORIENTED_EDGE ( 'NONE', *, *, #38087, .T. ) ;
#7290=B_SPLINE_CURVE_WITH_KNOTS ( 'NONE', 3,
 ( #67759, #80396, #39414, #18693, #60106, #88064, #4274, #86724, #40295, #17802 ),
 .UNSPECIFIED., .F., .F.,
 ( 4, 2, 2, 2, 4 ),
 ( 0.0007817246256747457630, 0.0009771112852218887673, 0.001172497944769031880, 0.001367884604316174993, 0.001563271263863318106 ),
 .UNSPECIFIED. ) ;
#7291=CARTESIAN_POINT ( 'NONE',  ( -2.307692307692305711, -12.10708131394839349, 31.69288490824020244 ) ) ;
#7292=CARTESIAN_POINT ( 'NONE',  ( 11.60371667797437567, -6.835583212224610072, 34.95778746994559327 ) ) ;
#7293=VERTEX_POINT ( 'NONE', #31032 ) ;
#7294=B_SPLINE_CURVE_WITH_KNOTS ( 'NONE', 3,
 ( #55805, #1751, #13936, #42751, #41865, #15720, #83294, #28794, #69333, #87907 ),
 .UNSPECIFIED., .F., .F.,
 ( 4, 2, 2, 2, 4 ),
 ( 0.0007817246256747507503, 0.0009771112852218959231, 0.001172497944769040987, 0.001367884604316186052, 0.001563271263863331116 ),
 .UNSPECIFIED. ) ;
#7295=ADVANCED_FACE ( 'NONE', ( #85549 ), #58955, .F. ) ;
#7296=CARTESIAN_POINT ( 'NONE',  ( 7.622668902429896143, -12.24155766932282496, 31.33739205006857986 ) ) ;
#7297=CARTESIAN_POINT ( 'NONE',  ( 4.403791563224197070, -9.357781135181031829, 34.66075350412533851 ) ) ;
#7298=CARTESIAN_POINT ( 'NONE',  ( 13.31853197365950692, -6.386643153685125363, 34.62446782046654903 ) ) ;
#7299=CARTESIAN_POINT ( 'NONE',  ( 4.826923076923076650, -2.499999999999998668, 29.75000000000000355 ) ) ;
#7300=CARTESIAN_POINT ( 'NONE',  ( 3.361561038594017781, -12.38066358083363738, 30.83685684665853444 ) ) ;
#7301=EDGE_LOOP ( 'NONE', ( #88865, #12964, #41411, #27718 ) ) ;
#7304=FACE_BOUND ( 'NONE', #4685, .T. ) ;
#7305=ORIENTED_EDGE ( 'NONE', *, *, #41393, .T. ) ;
#7306=CARTESIAN_POINT ( 'NONE',  ( -8.769230769230768274, -12.34228464037088635, 31.77849191805839268 ) ) ;
#7307=VECTOR ( 'NONE', #27504, 1000.000000000000227 ) ;
#7308=EDGE_CURVE ( 'NONE', #53380, #12502, #85104, .T. ) ;
#7309=CARTESIAN_POINT ( 'NONE',  ( 18.22301135161285046, -12.15243808032446005, 31.58219941686247978 ) ) ;
#7310=LINE ( 'NONE', #41987, #10453 ) ;
#7313=ORIENTED_EDGE ( 'NONE', *, *, #17589, .F. ) ;
#7314=ORIENTED_EDGE ( 'NONE', *, *, #4130, .F. ) ;
#7315=VERTEX_POINT ( 'NONE', #9882 ) ;
#7316=CARTESIAN_POINT ( 'NONE',  ( -10.83886953994894675, -8.539481045369596401, 34.89627647299170832 ) ) ;
#7319=B_SPLINE_CURVE_WITH_KNOTS ( 'NONE', 3,
 ( #17342, #53342, #46154, #52450, #31302, #39410, #65070, #3376, #86266, #11035 ),
 .UNSPECIFIED., .F., .F.,
 ( 4, 2, 2, 2, 4 ),
 ( 0.0007817359430256278375, 0.0009771253907249935044, 0.001172514838424359171, 0.001367904286123724838, 0.001563293733823090505 ),
 .UNSPECIFIED. ) ;
#7320=CARTESIAN_POINT ( 'NONE',  ( 15.23076923076923173, -3.322132147404559976, 32.92929555188717927 ) ) ;
#7322=CARTESIAN_POINT ( 'NONE',  ( -6.857883934782265989, -2.255955759149235629, 29.99999999999988631 ) ) ;
#7323=CARTESIAN_POINT ( 'NONE',  ( -1.384615384615383471, -9.905515769479276145, 34.41647553114623292 ) ) ;
#7324=CARTESIAN_POINT ( 'NONE',  ( 16.37685899793955357, -2.308499170217968022, 30.53291367094874076 ) ) ;
#7325=ADVANCED_FACE ( 'NONE', ( #51277 ), #24275, .F. ) ;
#7327=CARTESIAN_POINT ( 'NONE',  ( -14.17716686945866655, -12.70449254468099198, 30.44128974285582956 ) ) ;
#7328=EDGE_CURVE ( 'NONE', #63430, #31770, #67882, .T. ) ;
#7329=CARTESIAN_POINT ( 'NONE',  ( 4.023698184114453014, -2.647304123082328875, 31.75400227202885262 ) ) ;
#7330=CARTESIAN_POINT ( 'NONE',  ( 17.29993442853592711, -2.554770724473668597, 30.48948780036025852 ) ) ;
#7331=ORIENTED_EDGE ( 'NONE', *, *, #54372, .F. ) ;
#7332=B_SPLINE_CURVE_WITH_KNOTS ( 'NONE', 3,
 ( #67523, #74731, #88263, #12579, #33298, #13454, #53998, #48121, #40065, #54437 ),
 .UNSPECIFIED., .F., .F.,
 ( 4, 2, 2, 2, 4 ),
 ( 0.000000000000000000, 0.0001954311564186872810, 0.0003908623128373745620, 0.0005862934692560618430, 0.0007817246256747491240 ),
 .UNSPECIFIED. ) ;
#7333=ORIENTED_EDGE ( 'NONE', *, *, #49393, .F. ) ;
#7334=ORIENTED_EDGE ( 'NONE', *, *, #88402, .F. ) ;
#7335=CYLINDRICAL_SURFACE ( 'NONE', #56041, 0.2499999999999997502 ) ;
#7337=CARTESIAN_POINT ( 'NONE',  ( -13.44988583057615905, -6.026961402152685388, 34.52809138561120506 ) ) ;
#7338=AXIS2_PLACEMENT_3D ( 'NONE', #12274, #12720, #39759 ) ;
#7339=FACE_OUTER_BOUND ( 'NONE', #40458, .T. ) ;
#7340=DIRECTION ( 'NONE',  ( -0.000000000000000000, -0.9396926207859092051, -0.3420201433256662704 ) ) ;
#7341=LINE ( 'NONE', #70814, #81779 ) ;
#7342=LINE ( 'NONE', #82115, #24528 ) ;
#7343=EDGE_LOOP ( 'NONE', ( #69651, #78962, #11450, #67844 ) ) ;
#7344=DIRECTION ( 'NONE',  ( 0.000000000000000000, 0.6427876096865373645, -0.7660444431189797898 ) ) ;
#7346=FACE_OUTER_BOUND ( 'NONE', #50999, .T. ) ;
#7347=CARTESIAN_POINT ( 'NONE',  ( -3.230769230769352962, -3.643525952248796163, 33.31231777344771672 ) ) ;
#7349=VERTEX_POINT ( 'NONE', #4002 ) ;
#7350=CARTESIAN_POINT ( 'NONE',  ( 18.13052570176356326, -12.45806712695776319, 30.39783852428763566 ) ) ;
#7352=FACE_BOUND ( 'NONE', #45153, .T. ) ;
#7354=B_SPLINE_CURVE_WITH_KNOTS ( 'NONE', 3,
 ( #1122, #35805, #85646, #52293, #23925, #57724, #51835, #71674, #18078, #79782 ),
 .UNSPECIFIED., .F., .F.,
 ( 4, 2, 2, 2, 4 ),
 ( 0.000000000000000000, 0.0001954339857564082062, 0.0003908679715128164124, 0.0005863019572692246186, 0.0007817359430256328248 ),
 .UNSPECIFIED. ) ;
#7355=LINE ( 'NONE', #55085, #14659 ) ;
#7356=CARTESIAN_POINT ( 'NONE',  ( 17.01165307636676260, -12.16647553114622049, 32.15551576947930812 ) ) ;
#7357=ORIENTED_EDGE ( 'NONE', *, *, #63784, .T. ) ;
#7359=CARTESIAN_POINT ( 'NONE',  ( -17.86947456176635640, -4.299079248970731904, 33.91157788607253565 ) ) ;
#7360=CARTESIAN_POINT ( 'NONE',  ( 6.792385456409367528, -12.38065189839062263, 30.83690757178629482 ) ) ;
#7361=CYLINDRICAL_SURFACE ( 'NONE', #67614, 0.2499999999999998890 ) ;
#7363=CARTESIAN_POINT ( 'NONE',  ( -12.33074665371367651, -3.062576670634119758, 32.05464942895959979 ) ) ;
#7364=LINE ( 'NONE', #34822, #54220 ) ;
#7365=DIRECTION ( 'NONE',  ( 0.000000000000000000, 0.6427876096865368094, 0.7660444431189802339 ) ) ;
#7368=DIRECTION ( 'NONE',  ( 0.000000000000000000, 0.4999999999999985567, 0.8660254037844395958 ) ) ;
#7369=B_SPLINE_CURVE_WITH_KNOTS ( 'NONE', 3,
 ( #76060, #88719, #42292, #83274, #62973, #75190, #69748, #21108, #13478, #8056 ),
 .UNSPECIFIED., .F., .F.,
 ( 4, 2, 2, 2, 4 ),
 ( 0.0007817359430256287049, 0.0009771253907249945886, 0.001172514838424360255, 0.001367904286123725922, 0.001563293733823091806 ),
 .UNSPECIFIED. ) ;
#7370=CARTESIAN_POINT ( 'NONE',  ( 4.826899852701616034, -2.588893531581426544, 31.60682220781847818 ) ) ;
#7371=CARTESIAN_POINT ( 'NONE',  ( -13.13456107297707121, -3.627508038966690496, 32.91356715214248396 ) ) ;
#7372=EDGE_CURVE ( 'NONE', #7245, #45245, #17538, .T. ) ;
#7373=CARTESIAN_POINT ( 'NONE',  ( 16.85399611801622655, -4.762599654559227069, 34.23009711892697737 ) ) ;
#7374=CARTESIAN_POINT ( 'NONE',  ( -2.980714810855777053, -4.074993327901525575, 33.72946981652012255 ) ) ;
#7375=CARTESIAN_POINT ( 'NONE',  ( -16.82686876528476105, -8.303483539816726378, 34.68545999027711702 ) ) ;
#7376=CIRCLE ( 'NONE', #5585, 0.2500000000000002220 ) ;
#7377=CARTESIAN_POINT ( 'NONE',  ( 12.71153846153989697, -7.500000000000155431, 34.75000000000007105 ) ) ;
#7380=CARTESIAN_POINT ( 'NONE',  ( 17.99999999999987566, -4.481592998941358097, 33.73612834414048933 ) ) ;
#7382=VECTOR ( 'NONE', #7670, 1000.000000000000000 ) ;
#7383=ORIENTED_EDGE ( 'NONE', *, *, #11988, .T. ) ;
#7384=DIRECTION ( 'NONE',  ( -0.000000000000000000, -0.6427876096865404731, -0.7660444431189770143 ) ) ;
#7385=ORIENTED_EDGE ( 'NONE', *, *, #61279, .T. ) ;
#7386=CARTESIAN_POINT ( 'NONE',  ( -5.142193077479396912, -11.67786785259541027, 32.92929555188721480 ) ) ;
#7387=EDGE_CURVE ( 'NONE', #86865, #75988, #59253, .T. ) ;
#7389=CARTESIAN_POINT ( 'NONE',  ( 6.066068351002440906, -3.050289026998446840, 32.03036669348366416 ) ) ;
#7392=CYLINDRICAL_SURFACE ( 'NONE', #55968, 0.2499999999999998890 ) ;
#7393=LINE ( 'NONE', #20459, #83318 ) ;
#7394=CARTESIAN_POINT ( 'NONE',  ( 1.384615384615386802, -8.564572088678739092, 35.78748833219616898 ) ) ;
#7396=CARTESIAN_POINT ( 'NONE',  ( -12.46153846153846168, -6.435427911321262684, 35.78748833219616898 ) ) ;
#7397=CARTESIAN_POINT ( 'NONE',  ( 15.16468685140909400, -9.058645607665454236, 34.76329471203372634 ) ) ;
#7398=CARTESIAN_POINT ( 'NONE',  ( 5.326868486301119532, -10.92531984108285670, 33.72920026020278073 ) ) ;
#7399=CARTESIAN_POINT ( 'NONE',  ( -7.976301055592065481, -8.587444163452046197, 34.63053765926554206 ) ) ;
#7401=EDGE_LOOP ( 'NONE', ( #39382, #63078 ) ) ;
#7402=VERTEX_POINT ( 'NONE', #40044 ) ;
#7403=CARTESIAN_POINT ( 'NONE',  ( -15.09997742294444478, -8.147973898785416225, 34.70805048591653730 ) ) ;
#7404=CARTESIAN_POINT ( 'NONE',  ( 5.326977388561390470, -9.148310452688871663, 34.47095581063188519 ) ) ;
#7406=CARTESIAN_POINT ( 'NONE',  ( 9.692307692307695177, -11.91647553114624181, 32.58852847137148245 ) ) ;
#7407=EDGE_CURVE ( 'NONE', #43255, #47148, #73308, .T. ) ;
#7409=CARTESIAN_POINT ( 'NONE',  ( 11.78840694783958298, -4.176053281294518804, 33.81426240980091791 ) ) ;
#7410=LINE ( 'NONE', #13273, #39455 ) ;
#7411=VERTEX_POINT ( 'NONE', #53079 ) ;
#7412=ADVANCED_FACE ( 'NONE', ( #89122 ), #53529, .F. ) ;
#7413=DIRECTION ( 'NONE',  ( -0.000000000000000000, -0.3420201433256694346, -0.9396926207859080948 ) ) ;
#7414=ORIENTED_EDGE ( 'NONE', *, *, #86184, .F. ) ;
#7415=AXIS2_PLACEMENT_3D ( 'NONE', #77933, #71171, #77493 ) ;
#7416=CARTESIAN_POINT ( 'NONE',  ( 13.31934538405906565, -12.51329471203370325, 31.30864560766548976 ) ) ;
#7418=DIRECTION ( 'NONE',  ( -1.000000000000000000, 0.000000000000000000, 0.000000000000000000 ) ) ;
#7419=B_SPLINE_CURVE_WITH_KNOTS ( 'NONE', 3,
 ( #36964, #16697, #63991, #31092, #36540, #2288, #2729, #50041, #56799, #30655 ),
 .UNSPECIFIED., .F., .F.,
 ( 4, 2, 2, 2, 4 ),
 ( 0.0007817246256747507503, 0.0009771112852218959231, 0.001172497944769040987, 0.001367884604316186052, 0.001563271263863331116 ),
 .UNSPECIFIED. ) ;
#7420=CARTESIAN_POINT ( 'NONE',  ( -15.29603967673000575, -3.300289026998414865, 32.46337939537583139 ) ) ;
#7421=CARTESIAN_POINT ( 'NONE',  ( -18.00000000000012079, -12.51329471203414379, 31.30864560766407578 ) ) ;
#7422=VERTEX_POINT ( 'NONE', #19314 ) ;
#7423=EDGE_LOOP ( 'NONE', ( #42089, #34458, #9044, #97 ) ) ;
#7425=ORIENTED_EDGE ( 'NONE', *, *, #74183, .T. ) ;
#7426=VERTEX_POINT ( 'NONE', #80585 ) ;
#7427=EDGE_CURVE ( 'NONE', #33889, #53025, #20202, .T. ) ;
#7428=CARTESIAN_POINT ( 'NONE',  ( -10.86540783960607115, -12.45566812827425451, 31.48439005359158926 ) ) ;
#7429=CARTESIAN_POINT ( 'NONE',  ( -12.46153846153846168, -12.62096338111211580, 30.90682066428153263 ) ) ;
#7430=CARTESIAN_POINT ( 'NONE',  ( 14.05771556364371833, -2.544273027872575366, 31.48422191005632342 ) ) ;
#7431=ADVANCED_FACE ( 'NONE', ( #87347 ), #68380, .F. ) ;
#7432=CIRCLE ( 'NONE', #54881, 0.2500000000000002220 ) ;
#7433=DIRECTION ( 'NONE',  ( 0.000000000000000000, 0.6427876096865368094, 0.7660444431189802339 ) ) ;
#7434=CARTESIAN_POINT ( 'NONE',  ( 4.403900465484468008, -6.567000820036038355, 34.66262288849541306 ) ) ;
#7436=CYLINDRICAL_SURFACE ( 'NONE', #55248, 0.2499999999999995559 ) ;
#7438=VERTEX_POINT ( 'NONE', #33276 ) ;
#7439=AXIS2_PLACEMENT_3D ( 'NONE', #27581, #76658, #13623 ) ;
#7440=EDGE_LOOP ( 'NONE', ( #71409, #11511, #30035, #24478 ) ) ;
#7441=CARTESIAN_POINT ( 'NONE',  ( 12.68431800280687050, -8.496831190052093419, 34.64984203495476578 ) ) ;
#7442=ORIENTED_EDGE ( 'NONE', *, *, #18711, .F. ) ;
#7443=CARTESIAN_POINT ( 'NONE',  ( 10.54930120442873331, -12.37446782046654192, 30.86335684631486487 ) ) ;
#7444=CARTESIAN_POINT ( 'NONE',  ( -12.46153846153858424, -12.16647553114689728, 32.15551576947799362 ) ) ;
#7447=EDGE_CURVE ( 'NONE', #36450, #81317, #61484, .T. ) ;
#7448=EDGE_LOOP ( 'NONE', ( #31981, #7843, #8982, #37425 ) ) ;
#7449=CYLINDRICAL_SURFACE ( 'NONE', #49990, 0.2500000000000004996 ) ;
#7450=ORIENTED_EDGE ( 'NONE', *, *, #32378, .F. ) ;
#7451=FACE_BOUND ( 'NONE', #42332, .T. ) ;
#7452=CARTESIAN_POINT ( 'NONE',  ( -2.057637887778852814, -4.818054556918156983, 34.26375889529406749 ) ) ;
#7453=CARTESIAN_POINT ( 'NONE',  ( 7.912221179503920787, -5.471508081941601098, 34.59228464037088457 ) ) ;
#7454=EDGE_LOOP ( 'NONE', ( #21254, #47428, #8860, #67117 ) ) ;
#7455=EDGE_CURVE ( 'NONE', #86041, #59263, #37884, .T. ) ;
#7456=CARTESIAN_POINT ( 'NONE',  ( -9.822455662039388358, -5.070767119584671079, 34.40440758774516183 ) ) ;
#7457=CARTESIAN_POINT ( 'NONE',  ( 8.769230769230645706, -8.656820664282941280, 34.87096338111179961 ) ) ;
#7458=B_SPLINE_CURVE_WITH_KNOTS ( 'NONE', 3,
 ( #44369, #35871, #71859, #51122, #71407, #49812, #57012, #16918, #65090, #36746 ),
 .UNSPECIFIED., .F., .F.,
 ( 4, 2, 2, 2, 4 ),
 ( 0.000000000000000000, 0.0001954339857564083146, 0.0003908679715128166293, 0.0005863019572692249439, 0.0007817359430256332585 ),
 .UNSPECIFIED. ) ;
#7459=CARTESIAN_POINT ( 'NONE',  ( 0.5920641633020244932, -6.852161475712352789, 34.70806712695775786 ) ) ;
#7460=CARTESIAN_POINT ( 'NONE',  ( 15.36129466900287532, -6.808710257144161559, 34.95449254468098843 ) ) ;
#7461=EDGE_LOOP ( 'NONE', ( #39097, #38410 ) ) ;
#7462=AXIS2_PLACEMENT_3D ( 'NONE', #11772, #73480, #45985 ) ;
#7463=CARTESIAN_POINT ( 'NONE',  ( -0.7115384615384606759, -7.566082377512564960, 35.00000000000000711 ) ) ;
#7464=CARTESIAN_POINT ( 'NONE',  ( -5.777220331021931443, -4.226511098958374291, 33.85474049983370293 ) ) ;
#7466=FACE_OUTER_BOUND ( 'NONE', #80389, .T. ) ;
#7467=CYLINDRICAL_SURFACE ( 'NONE', #87543, 0.2499999999999995559 ) ;
#7468=EDGE_CURVE ( 'NONE', #41734, #62713, #86244, .T. ) ;
#7469=FACE_BOUND ( 'NONE', #14445, .T. ) ;
#7470=CARTESIAN_POINT ( 'NONE',  ( 4.826899839630110378, -11.37209801155882971, 32.91403422569032955 ) ) ;
#7471=CARTESIAN_POINT ( 'NONE',  ( 11.31497659473759043, -12.44517049084099725, 30.48991314939691932 ) ) ;
#7472=CARTESIAN_POINT ( 'NONE',  ( -6.923076923076922462, -12.10708131394839349, 31.69288490824020244 ) ) ;
#7473=CARTESIAN_POINT ( 'NONE',  ( -18.00000000000012079, -2.379036618888197285, 30.90682066428292885 ) ) ;
#7474=CARTESIAN_POINT ( 'NONE',  ( 2.307692307692309264, -6.343179335718451384, 34.87096338111211935 ) ) ;
#7475=AXIS2_PLACEMENT_3D ( 'NONE', #56460, #55566, #68642 ) ;
#7476=CARTESIAN_POINT ( 'NONE',  ( -18.25002323729296450, -10.05641848906368629, 34.04755513067964756 ) ) ;
#7478=EDGE_LOOP ( 'NONE', ( #42084, #46511, #70092, #34398 ) ) ;
#7480=CARTESIAN_POINT ( 'NONE',  ( 1.134638653673032627, -12.17611988154120972, 31.52148481390971213 ) ) ;
#7482=ADVANCED_FACE ( 'NONE', ( #41808 ), #375, .F. ) ;
#7483=CYLINDRICAL_SURFACE ( 'NONE', #6113, 0.2500000000000002220 ) ;
#7484=ORIENTED_EDGE ( 'NONE', *, *, #42372, .T. ) ;
#7486=CARTESIAN_POINT ( 'NONE',  ( 14.05771556364371833, -4.075325502946081535, 33.72974371597206300 ) ) ;
#7488=DIRECTION ( 'NONE',  ( 0.000000000000000000, 0.1736481776669267785, -0.9848077530122087975 ) ) ;
#7490=CARTESIAN_POINT ( 'NONE',  ( 4.153846153846154188, -8.973038597847269315, 34.52809138561121927 ) ) ;
#7491=CARTESIAN_POINT ( 'NONE',  ( 16.02315555073584363, -8.191372820521381826, 34.95448215188423546 ) ) ;
#7492=EDGE_CURVE ( 'NONE', #27260, #78559, #83996, .T. ) ;
#7493=DIRECTION ( 'NONE',  ( 0.000000000000000000, 0.7660444431189807890, 0.6427876096865361433 ) ) ;
#7494=DIRECTION ( 'NONE',  ( -0.000000000000000000, 0.3420201433256694901, -0.9396926207859082059 ) ) ;
#7495=CARTESIAN_POINT ( 'NONE',  ( 2.557746619330623972, -2.779044189368095719, 31.39831045268885745 ) ) ;
#7498=DIRECTION ( 'NONE',  ( -0.000000000000000000, -0.6427876096865404731, -0.7660444431189771253 ) ) ;
#7499=CARTESIAN_POINT ( 'NONE',  ( -14.30769230769230660, -9.819645486525091727, 36.12317359536749706 ) ) ;
#7500=ORIENTED_EDGE ( 'NONE', *, *, #77421, .T. ) ;
#7501=DIRECTION ( 'NONE',  ( -0.000000000000000000, 1.000000000000000000, -0.000000000000000000 ) ) ;
#7503=CARTESIAN_POINT ( 'NONE',  ( 2.241609928332172874, -4.661471528628506888, 34.16647553114621871 ) ) ;
#7504=DIRECTION ( 'NONE',  ( 1.000000000000000000, 0.000000000000000000, 0.000000000000000000 ) ) ;
#7505=EDGE_LOOP ( 'NONE', ( #32192, #50257 ) ) ;
#7506=CARTESIAN_POINT ( 'NONE',  ( -17.93393164899756442, -2.721908614388772296, 31.22303859784725333 ) ) ;
#7507=CARTESIAN_POINT ( 'NONE',  ( -0.4615384615385826339, -10.21337939537710326, 33.94971097300076224 ) ) ;
#7509=ORIENTED_EDGE ( 'NONE', *, *, #30019, .T. ) ;
#7510=CARTESIAN_POINT ( 'NONE',  ( 8.638540166120458608, -5.496505350115501010, 34.60290016733514307 ) ) ;
#7511=EDGE_CURVE ( 'NONE', #45323, #52135, #77615, .T. ) ;
#7513=VECTOR ( 'NONE', #20895, 1000.000000000000114 ) ;
#7514=CARTESIAN_POINT ( 'NONE',  ( -10.36543920600657209, -9.357781135181031829, 34.66075350412533851 ) ) ;
#7515=CARTESIAN_POINT ( 'NONE',  ( -9.561517251340742263, -2.494656445102012565, 31.33466734024120015 ) ) ;
#7516=CARTESIAN_POINT ( 'NONE',  ( -18.13069146666756382, -12.11776431015576172, 31.66791131148498906 ) ) ;
#7517=ORIENTED_EDGE ( 'NONE', *, *, #54217, .T. ) ;
#7518=ORIENTED_EDGE ( 'NONE', *, *, #67285, .T. ) ;
#7519=EDGE_LOOP ( 'NONE', ( #24928, #18571 ) ) ;
#7520=DIRECTION ( 'NONE',  ( 0.000000000000000000, 0.7660444431189822323, -0.6427876096865344779 ) ) ;
#7521=FACE_OUTER_BOUND ( 'NONE', #13956, .T. ) ;
#7522=CARTESIAN_POINT ( 'NONE',  ( -13.13466986626724164, -12.22109172314383052, 31.39792113162168263 ) ) ;
#7523=CARTESIAN_POINT ( 'NONE',  ( -5.076923076923075762, -13.75783147151868846, 33.36296068462461051 ) ) ;
#7524=ORIENTED_EDGE ( 'NONE', *, *, #69729, .F. ) ;
#7525=B_SPLINE_CURVE_WITH_KNOTS ( 'NONE', 3,
 ( #43652, #24258, #45422, #84664, #57613, #72900, #85535, #51264, #71562, #10761 ),
 .UNSPECIFIED., .F., .F.,
 ( 4, 2, 2, 2, 4 ),
 ( 0.000000000000000000, 0.0001954311564186864949, 0.0003908623128373729899, 0.0005862934692560594577, 0.0007817246256747459798 ),
 .UNSPECIFIED. ) ;
#7528=ORIENTED_EDGE ( 'NONE', *, *, #37619, .F. ) ;
#7529=ORIENTED_EDGE ( 'NONE', *, *, #11272, .F. ) ;
#7530=ORIENTED_EDGE ( 'NONE', *, *, #67351, .F. ) ;
#7531=DIRECTION ( 'NONE',  ( -0.000000000000000000, -0.8660254037844397068, -0.4999999999999978906 ) ) ;
#7533=CARTESIAN_POINT ( 'NONE',  ( -0.5916856709766811218, -5.195881422630166391, 34.18770438780619259 ) ) ;
#7535=CARTESIAN_POINT ( 'NONE',  ( -3.296039231325550656, -12.16647553114622049, 32.15551576947930812 ) ) ;
#7536=ADVANCED_FACE ( 'NONE', ( #76473 ), #68823, .F. ) ;
#7537=CARTESIAN_POINT ( 'NONE',  ( -3.100243529005666687, -4.459921816937789885, 33.71989282347011851 ) ) ;
#7538=CARTESIAN_POINT ( 'NONE',  ( 8.769230769230647482, -2.625532179533778709, 30.86335684631627174 ) ) ;
#7539=ADVANCED_FACE ( 'NONE', ( #29619 ), #77353, .F. ) ;
#7540=ORIENTED_EDGE ( 'NONE', *, *, #86846, .F. ) ;
#7541=ORIENTED_EDGE ( 'NONE', *, *, #82198, .F. ) ;
#7542=ORIENTED_EDGE ( 'NONE', *, *, #63795, .T. ) ;
#7544=DIRECTION ( 'NONE',  ( 0.000000000000000000, 0.4999999999999985567, 0.8660254037844395958 ) ) ;
#7545=ORIENTED_EDGE ( 'NONE', *, *, #22235, .F. ) ;
#7546=EDGE_CURVE ( 'NONE', #441, #10997, #41086, .T. ) ;
#7547=CARTESIAN_POINT ( 'NONE',  ( -2.084912766423896446, -8.496831190052096971, 34.64984203495476578 ) ) ;
#7548=CARTESIAN_POINT ( 'NONE',  ( 7.846153846153846700, -8.564572088678739092, 35.78748833219616898 ) ) ;
#7549=EDGE_LOOP ( 'NONE', ( #59106, #80811 ) ) ;
#7550=CARTESIAN_POINT ( 'NONE',  ( -4.153846153846152411, -4.786620604624113540, 33.94971097300155094 ) ) ;
#7552=CARTESIAN_POINT ( 'NONE',  ( 4.219914504848593317, -2.721908614388772296, 31.22303859784725333 ) ) ;
#7553=VERTEX_POINT ( 'NONE', #63836 ) ;
#7554=FACE_BOUND ( 'NONE', #3848, .T. ) ;
#7557=AXIS2_PLACEMENT_3D ( 'NONE', #73630, #19549, #39396 ) ;
#7559=CARTESIAN_POINT ( 'NONE',  ( -6.673076923075486278, -7.500000000000155431, 34.75000000000007105 ) ) ;
#7560=CARTESIAN_POINT ( 'NONE',  ( -5.076923076923075762, -12.29105614889573062, 35.45975837776705220 ) ) ;
#7561=VECTOR ( 'NONE', #20381, 1000.000000000000114 ) ;
#7562=CARTESIAN_POINT ( 'NONE',  ( -4.826868765284761942, -10.66356715214248396, 33.62249196103329751 ) ) ;
#7563=CARTESIAN_POINT ( 'NONE',  ( -2.557669038634660996, -3.627789207965226748, 32.91389620160131102 ) ) ;
#7564=ORIENTED_EDGE ( 'NONE', *, *, #9056, .T. ) ;
#7565=CARTESIAN_POINT ( 'NONE',  ( -7.846153846153844924, -6.343179335718451384, 34.87096338111211935 ) ) ;
#7566=CARTESIAN_POINT ( 'NONE',  ( 13.13461538461538680, -7.433931650972300353, 34.75000000000000711 ) ) ;
#7567=ORIENTED_EDGE ( 'NONE', *, *, #63726, .T. ) ;
#7569=CARTESIAN_POINT ( 'NONE',  ( 8.769230769230768274, -3.050289026998446396, 32.03036669348365706 ) ) ;
#7570=CARTESIAN_POINT ( 'NONE',  ( 9.468822748583749060, -2.847400154188068022, 31.58180166144859058 ) ) ;
#7571=EDGE_LOOP ( 'NONE', ( #65774, #12763, #56591, #14116 ) ) ;
#7572=CARTESIAN_POINT ( 'NONE',  ( 17.75002326905764960, -5.728515186090277211, 34.42611988154120439 ) ) ;
#7573=CARTESIAN_POINT ( 'NONE',  ( -4.376773112752999850, -2.308479472611653094, 30.53278059502174457 ) ) ;
#7574=FACE_BOUND ( 'NONE', #72500, .T. ) ;
#7575=DIRECTION ( 'NONE',  ( 0.000000000000000000, 0.6427876096865373645, -0.7660444431189797898 ) ) ;
#7576=LINE ( 'NONE', #35038, #34435 ) ;
#7577=CARTESIAN_POINT ( 'NONE',  ( 10.55011416942384095, -8.613356846314824011, 34.62446782046655613 ) ) ;
#7578=CARTESIAN_POINT ( 'NONE',  ( -15.48074596171158213, -9.148715823498378086, 34.47080413974185120 ) ) ;
#7580=CARTESIAN_POINT ( 'NONE',  ( 7.173131234715237170, -12.41262288849542017, 30.68299917996395010 ) ) ;
#7583=ORIENTED_EDGE ( 'NONE', *, *, #52444, .F. ) ;
#7585=EDGE_LOOP ( 'NONE', ( #10787, #24479, #49614, #27170 ) ) ;
#7588=CARTESIAN_POINT ( 'NONE',  ( 6.792601738001206257, -7.276987145209185215, 34.99546412871779211 ) ) ;
#7590=CARTESIAN_POINT ( 'NONE',  ( 3.100077764101674127, -11.18331474514187995, 33.13161551792790505 ) ) ;
#7592=PLANE ( 'NONE',  #58990 ) ;
#7593=DIRECTION ( 'NONE',  ( -0.000000000000000000, 0.7660444431189791237, -0.6427876096865379196 ) ) ;
#7594=ADVANCED_FACE ( 'NONE', ( #2131 ), #76019, .F. ) ;
#7595=CARTESIAN_POINT ( 'NONE',  ( -3.230769230769351186, -6.026961402154118908, 34.52809138561165270 ) ) ;
#7596=CARTESIAN_POINT ( 'NONE',  ( -5.076923076923075762, -2.292212530054420494, 30.41441678777542634 ) ) ;
#7597=CARTESIAN_POINT ( 'NONE',  ( 4.153846153846154188, -1.117168528481311540, 33.14645433367849847 ) ) ;
#7599=CARTESIAN_POINT ( 'NONE',  ( -4.826977558574936822, -2.824170634883622188, 31.52227843825338738 ) ) ;
#7600=CARTESIAN_POINT ( 'NONE',  ( 14.30769230769218758, -11.94971097300221174, 32.03036669348237098 ) ) ;
#7601=EDGE_CURVE ( 'NONE', #47075, #28663, #36761, .T. ) ;
#7602=EDGE_CURVE ( 'NONE', #31488, #7007, #2294, .T. ) ;
#7603=CARTESIAN_POINT ( 'NONE',  ( -13.38461538461550759, -6.835583212225970762, 34.95778746994575670 ) ) ;
#7604=ORIENTED_EDGE ( 'NONE', *, *, #48463, .T. ) ;
#7605=CARTESIAN_POINT ( 'NONE',  ( 8.769230769230768274, -6.435427911321262684, 35.78748833219616898 ) ) ;
#7606=CARTESIAN_POINT ( 'NONE',  ( 0.4615384615384611200, -2.538708090699994813, 30.37095296980875503 ) ) ;
#7608=CARTESIAN_POINT ( 'NONE',  ( -5.869474561766353737, -12.50538340440932217, 31.33453814440721885 ) ) ;
#7609=CARTESIAN_POINT ( 'NONE',  ( -15.93083330975275658, -2.523321265292116866, 31.42251411153756990 ) ) ;
#7610=ORIENTED_EDGE ( 'NONE', *, *, #62332, .T. ) ;
#7611=CARTESIAN_POINT ( 'NONE',  ( -9.692307692307814193, -5.941354392335915335, 34.76329471203413846 ) ) ;
#7612=LINE ( 'NONE', #20242, #18059 ) ;
#7613=EDGE_LOOP ( 'NONE', ( #85569, #33522, #7981, #87550 ) ) ;
#7615=DIRECTION ( 'NONE',  ( -0.000000000000000000, 0.9848077530122085754, -0.1736481776669273613 ) ) ;
#7616=EDGE_CURVE ( 'NONE', #10070, #62944, #49697, .T. ) ;
#7617=EDGE_LOOP ( 'NONE', ( #1667, #5858, #26804, #65192 ) ) ;
#7618=CARTESIAN_POINT ( 'NONE',  ( -5.299849294439222369, -12.15238873228292071, 31.58232369045353849 ) ) ;
#7620=VERTEX_POINT ( 'NONE', #3895 ) ;
#7621=CARTESIAN_POINT ( 'NONE',  ( -10.68065461594093435, -4.320704448112771878, 33.92786785259540494 ) ) ;
#7622=EDGE_CURVE ( 'NONE', #57991, #8026, #31342, .T. ) ;
#7624=CARTESIAN_POINT ( 'NONE',  ( -15.16460262417758820, -7.250054591869670162, 34.99404684341514127 ) ) ;
#7625=CARTESIAN_POINT ( 'NONE',  ( 9.692307692307695177, -6.681629849574314051, 35.83090037661290239 ) ) ;
#7627=ORIENTED_EDGE ( 'NONE', *, *, #67473, .T. ) ;
#7628=CARTESIAN_POINT ( 'NONE',  ( 15.29683758177167086, -10.51840700105979565, 33.73612834413962247 ) ) ;
#7629=ADVANCED_FACE ( 'NONE', ( #30490 ), #35778, .T. ) ;
#7630=B_SPLINE_CURVE_WITH_KNOTS ( 'NONE', 3,
 ( #37973, #36645, #51911, #64103, #2400, #23126, #85280, #31205, #24001, #10048 ),
 .UNSPECIFIED., .F., .F.,
 ( 4, 2, 2, 2, 4 ),
 ( 0.0007817246256747451124, 0.0009771112852218885505, 0.001172497944769032097, 0.001367884604316175427, 0.001563271263863318973 ),
 .UNSPECIFIED. ) ;
#7632=EDGE_LOOP ( 'NONE', ( #65336, #75891, #43852, #62695 ) ) ;
#7633=CARTESIAN_POINT ( 'NONE',  ( 3.361559671736180199, -11.93129842949671726, 32.56571108434900452 ) ) ;
#7634=CYLINDRICAL_SURFACE ( 'NONE', #62807, 0.2499999999999997502 ) ;
#7635=CARTESIAN_POINT ( 'NONE',  ( 13.51540582558234149, -3.338503747796866872, 32.95102852606553512 ) ) ;
#7636=CARTESIAN_POINT ( 'NONE',  ( -6.792286482109970436, -11.37503395064541678, 33.29242100308974983 ) ) ;
#7637=FACE_OUTER_BOUND ( 'NONE', #54344, .T. ) ;
#7638=CARTESIAN_POINT ( 'NONE',  ( -2.530558570755406134, -2.251424796025575770, 29.88072029997477586 ) ) ;
#7639=VECTOR ( 'NONE', #65098, 1000.000000000000000 ) ;
#7640=CYLINDRICAL_SURFACE ( 'NONE', #27614, 0.2500000000000008882 ) ;
#7641=ORIENTED_EDGE ( 'NONE', *, *, #13372, .F. ) ;
#7642=ORIENTED_EDGE ( 'NONE', *, *, #32646, .T. ) ;
#7643=CARTESIAN_POINT ( 'NONE',  ( -0.3307466537136750095, -12.11778462344221019, 31.66786338562085135 ) ) ;
#7646=CARTESIAN_POINT ( 'NONE',  ( 16.94623247381277054, -2.295517848115769421, 30.44137282052136939 ) ) ;
#7647=EDGE_LOOP ( 'NONE', ( #51745, #86403, #38735, #36858 ) ) ;
#7649=CARTESIAN_POINT ( 'NONE',  ( -8.069080805060693251, -10.01117774369187252, 34.36070679894347535 ) ) ;
#7650=ORIENTED_EDGE ( 'NONE', *, *, #80851, .T. ) ;
#7651=CARTESIAN_POINT ( 'NONE',  ( -15.23076923076922995, -1.951392089020283160, 34.73218667398347748 ) ) ;
#7653=VERTEX_POINT ( 'NONE', #16531 ) ;
#7654=CARTESIAN_POINT ( 'NONE',  ( -16.28453762051371712, -3.530157926970578508, 32.79014554554150607 ) ) ;
#7655=ORIENTED_EDGE ( 'NONE', *, *, #63111, .T. ) ;
#7656=EDGE_CURVE ( 'NONE', #85495, #74960, #38137, .T. ) ;
#7657=AXIS2_PLACEMENT_3D ( 'NONE', #55885, #36510, #63961 ) ;
#7658=CARTESIAN_POINT ( 'NONE',  ( 17.99999999999987566, -9.528491918059723176, 34.59228464037033035 ) ) ;
#7659=VERTEX_POINT ( 'NONE', #9777 ) ;
#7660=B_SPLINE_CURVE_WITH_KNOTS ( 'NONE', 3,
 ( #67409, #81378, #4824, #52988, #18333, #11581, #67851, #18782, #26426, #33178 ),
 .UNSPECIFIED., .F., .F.,
 ( 4, 2, 2, 2, 4 ),
 ( 0.0007817246256747447872, 0.0009771112852218876831, 0.001172497944769030579, 0.001367884604316173475, 0.001563271263863316371 ),
 .UNSPECIFIED. ) ;
#7661=CARTESIAN_POINT ( 'NONE',  ( 17.77651505627605033, -10.81261337010820256, 33.49550067578627477 ) ) ;
#7662=CARTESIAN_POINT ( 'NONE',  ( -8.992715712954716167, -2.847400154188067578, 31.58180166144859058 ) ) ;
#7663=FACE_BOUND ( 'NONE', #21652, .T. ) ;
#7664=B_SPLINE_CURVE_WITH_KNOTS ( 'NONE', 3,
 ( #60986, #33528, #82612, #88932, #62306, #7823, #27203, #55115, #19999, #75828 ),
 .UNSPECIFIED., .F., .F.,
 ( 4, 2, 2, 2, 4 ),
 ( 0.0007817246256747504250, 0.0009771112852218954894, 0.001172497944769040554, 0.001367884604316185401, 0.001563271263863330466 ),
 .UNSPECIFIED. ) ;
#7665=CARTESIAN_POINT ( 'NONE',  ( -14.30769230769230660, -9.058645607665452459, 34.76329471203371924 ) ) ;
#7667=CARTESIAN_POINT ( 'NONE',  ( 4.153846153846154188, -12.37446782046654192, 30.86335684631486131 ) ) ;
#7669=CARTESIAN_POINT ( 'NONE',  ( 5.142178648199100088, -10.90142922261932057, 33.41473453929631887 ) ) ;
#7670=DIRECTION ( 'NONE',  ( 1.000000000000000000, 0.000000000000000000, 0.000000000000000000 ) ) ;
#7671=EDGE_LOOP ( 'NONE', ( #19042, #25972 ) ) ;
#7672=CARTESIAN_POINT ( 'NONE',  ( -14.05774678934416499, -3.712312575010499049, 33.01462480002815170 ) ) ;
#7673=EDGE_LOOP ( 'NONE', ( #59250, #10074 ) ) ;
#7674=EDGE_LOOP ( 'NONE', ( #8253, #50348 ) ) ;
#7675=CARTESIAN_POINT ( 'NONE',  ( 2.242421861731532573, -10.90142922261923886, 33.41473453929638993 ) ) ;
#7676=DIRECTION ( 'NONE',  ( -0.000000000000000000, -0.8660254037844399289, -0.4999999999999980016 ) ) ;
#7678=CARTESIAN_POINT ( 'NONE',  ( -12.59222992820602194, -2.541943142973491554, 30.39792223712631980 ) ) ;
#7679=CARTESIAN_POINT ( 'NONE',  ( -16.85414340794500276, -10.23759521482555357, 34.22997729860117033 ) ) ;
#7680=CYLINDRICAL_SURFACE ( 'NONE', #14195, 0.2499999999999998890 ) ;
#7681=CARTESIAN_POINT ( 'NONE',  ( 9.915087233576102221, -2.600157965045224895, 30.74683119005207743 ) ) ;
#7682=ORIENTED_EDGE ( 'NONE', *, *, #1322, .F. ) ;
#7683=CARTESIAN_POINT ( 'NONE',  ( 11.53846153846153832, -3.322132147404559976, 32.92929555188717927 ) ) ;
#7684=VECTOR ( 'NONE', #15729, 1000.000000000000114 ) ;
#7685=CARTESIAN_POINT ( 'NONE',  ( -14.53061926659915315, -10.01117774369187252, 34.36070679894347535 ) ) ;
#7686=CARTESIAN_POINT ( 'NONE',  ( -3.230769230769229949, -11.35647404775217417, 33.31231777344666511 ) ) ;
#7688=CARTESIAN_POINT ( 'NONE',  ( -13.60754160213152808, -10.61292498521070549, 33.66303323003028680 ) ) ;
#7689=VERTEX_POINT ( 'NONE', #4353 ) ;
#7691=VECTOR ( 'NONE', #54919, 1000.000000000000227 ) ;
#7693=ORIENTED_EDGE ( 'NONE', *, *, #16052, .F. ) ;
#7694=AXIS2_PLACEMENT_3D ( 'NONE', #60929, #88430, #53730 ) ;
#7695=LINE ( 'NONE', #42371, #86626 ) ;
#7696=ADVANCED_FACE ( 'NONE', ( #85442 ), #65595, .F. ) ;
#7697=ORIENTED_EDGE ( 'NONE', *, *, #17808, .T. ) ;
#7698=CARTESIAN_POINT ( 'NONE',  ( -9.469528023329623068, -10.23759521482555357, 34.22997729860117033 ) ) ;
#7699=CARTESIAN_POINT ( 'NONE',  ( -12.46153846153858247, -6.879047030192662504, 34.71129190930017927 ) ) ;
#7700=CYLINDRICAL_SURFACE ( 'NONE', #72569, 0.2500000000000004996 ) ;
#7702=ADVANCED_FACE ( 'NONE', ( #31837 ), #59292, .F. ) ;
#7703=B_SPLINE_CURVE_WITH_KNOTS ( 'NONE', 3,
 ( #21734, #22182, #77122, #41124, #68588, #6886, #34354, #61825, #2768, #44644 ),
 .UNSPECIFIED., .F., .F.,
 ( 4, 2, 2, 2, 4 ),
 ( 0.000000000000000000, 0.0001954311564186861155, 0.0003908623128373722310, 0.0005862934692560583735, 0.0007817246256747444619 ),
 .UNSPECIFIED. ) ;
#7704=CARTESIAN_POINT ( 'NONE',  ( 12.39626801557768587, -10.21337939537584383, 33.94971097300158647 ) ) ;
#7705=ORIENTED_EDGE ( 'NONE', *, *, #84527, .F. ) ;
#7706=CARTESIAN_POINT ( 'NONE',  ( 8.519230769230768274, -2.249999999999998668, 29.75000000000000355 ) ) ;
#7707=B_SPLINE_CURVE_WITH_KNOTS ( 'NONE', 3,
 ( #24476, #87100, #25376, #9635, #86208, #66362, #23592, #78984, #18181, #37103 ),
 .UNSPECIFIED., .F., .F.,
 ( 4, 2, 2, 2, 4 ),
 ( 0.000000000000000000, 0.0001954311564186863052, 0.0003908623128373726104, 0.0005862934692560589156, 0.0007817246256747452209 ),
 .UNSPECIFIED. ) ;
#7708=CARTESIAN_POINT ( 'NONE',  ( -0.4615384615385840772, -5.941354392335915335, 34.76329471203413846 ) ) ;
#7710=CARTESIAN_POINT ( 'NONE',  ( -3.361329822511150311, -2.504760397472875155, 29.97295953869789997 ) ) ;
#7711=CARTESIAN_POINT ( 'NONE',  ( 3.230769230769231726, -12.37446782046654192, 30.86335684631486131 ) ) ;
#7712=CARTESIAN_POINT ( 'NONE',  ( 17.20771488474786892, -11.18335022499818621, 33.13157742990016885 ) ) ;
#7713=LINE ( 'NONE', #13569, #4989 ) ;
#7714=CARTESIAN_POINT ( 'NONE',  ( -17.93474486048716088, -11.06231777344670952, 33.60647404775212266 ) ) ;
#7716=FACE_OUTER_BOUND ( 'NONE', #35899, .T. ) ;
#7717=CARTESIAN_POINT ( 'NONE',  ( 6.923076923076800782, -11.67786785259630911, 32.92929555188603530 ) ) ;
#7719=ORIENTED_EDGE ( 'NONE', *, *, #15620, .T. ) ;
#7720=CARTESIAN_POINT ( 'NONE',  ( -4.826923076921656452, -7.500000000000154543, 35.00000000000007105 ) ) ;
#7721=CARTESIAN_POINT ( 'NONE',  ( -14.05774689831426372, -3.520799739797214389, 33.17531984108286025 ) ) ;
#7722=CARTESIAN_POINT ( 'NONE',  ( 8.900021210197715860, -10.70102852606553157, 33.91149625220312913 ) ) ;
#7723=CARTESIAN_POINT ( 'NONE',  ( 9.692307692307570832, -6.835583212225970762, 34.95778746994575670 ) ) ;
#7724=ORIENTED_EDGE ( 'NONE', *, *, #4901, .F. ) ;
#7727=CARTESIAN_POINT ( 'NONE',  ( -1.318547033612945452, -6.386643153685127139, 34.62446782046654192 ) ) ;
#7728=VECTOR ( 'NONE', #23716, 1000.000000000000000 ) ;
#7729=CARTESIAN_POINT ( 'NONE',  ( 14.17754509825408960, -3.285722584762969856, 32.44110544564090759 ) ) ;
#7730=ORIENTED_EDGE ( 'NONE', *, *, #30780, .T. ) ;
#7731=CARTESIAN_POINT ( 'NONE',  ( 15.23076923076911093, -4.481592998941358097, 33.73612834414048933 ) ) ;
#7732=EDGE_CURVE ( 'NONE', #31209, #65326, #52875, .T. ) ;
#7733=CARTESIAN_POINT ( 'NONE',  ( -0.5268084620947813823, -10.33852847137145048, 34.16647553114627556 ) ) ;
#7734=CARTESIAN_POINT ( 'NONE',  ( -14.08472917342563591, -7.369474539155828730, 34.99858011523957657 ) ) ;
#7735=VERTEX_POINT ( 'NONE', #87236 ) ;
#7736=DIRECTION ( 'NONE',  ( -0.000000000000000000, 0.3420201433256694346, -0.9396926207859080948 ) ) ;
#7737=ORIENTED_EDGE ( 'NONE', *, *, #51029, .T. ) ;
#7738=CARTESIAN_POINT ( 'NONE',  ( -2.530618525208453651, -12.15238873228292071, 31.58232369045353849 ) ) ;
#7739=CARTESIAN_POINT ( 'NONE',  ( 4.853438152358745761, -5.827078755546623690, 34.72654668319379567 ) ) ;
#7741=DIRECTION ( 'NONE',  ( -0.000000000000000000, -0.8660254037844399289, -0.4999999999999980016 ) ) ;
#7742=CARTESIAN_POINT ( 'NONE',  ( 7.846153846153846700, -3.886160181151819604, 36.00935417666054406 ) ) ;
#7743=CARTESIAN_POINT ( 'NONE',  ( 10.61538461538461675, -1.422936976036506707, 30.56769352161908415 ) ) ;
#7744=CARTESIAN_POINT ( 'NONE',  ( -11.47320639894870276, -5.941354392334607049, 34.76329471203374055 ) ) ;
#7745=CARTESIAN_POINT ( 'NONE',  ( -0.4615384615384611200, -1.466349020453238561, 30.81389545987213907 ) ) ;
#7747=ORIENTED_EDGE ( 'NONE', *, *, #79413, .F. ) ;
#7748=EDGE_LOOP ( 'NONE', ( #57149, #6414 ) ) ;
#7749=FACE_BOUND ( 'NONE', #69583, .T. ) ;
#7750=ORIENTED_EDGE ( 'NONE', *, *, #4229, .F. ) ;
#7751=CARTESIAN_POINT ( 'NONE',  ( -5.076923076923075762, -8.318370150425687726, 35.83090037661290239 ) ) ;
#7752=VECTOR ( 'NONE', #80972, 1000.000000000000000 ) ;
#7754=CARTESIAN_POINT ( 'NONE',  ( 6.222779668978068557, -5.827830569534416583, 34.72679350104403539 ) ) ;
#7755=CARTESIAN_POINT ( 'NONE',  ( 14.53070515178570332, -8.282913670948747864, 34.94150082978203642 ) ) ;
#7756=B_SPLINE_CURVE_WITH_KNOTS ( 'NONE', 3,
 ( #27655, #29004, #15037, #28551, #54672, #82170, #61874, #8281, #189, #76281 ),
 .UNSPECIFIED., .F., .F.,
 ( 4, 2, 2, 2, 4 ),
 ( 0.000000000000000000, 0.0001954339857564097512, 0.0003908679715128195024, 0.0005863019572692292807, 0.0007817359430256390048 ),
 .UNSPECIFIED. ) ;
#7757=ORIENTED_EDGE ( 'NONE', *, *, #56503, .T. ) ;
#7758=ORIENTED_EDGE ( 'NONE', *, *, #70785, .F. ) ;
#7759=VERTEX_POINT ( 'NONE', #12012 ) ;
#7761=EDGE_LOOP ( 'NONE', ( #59539, #13844 ) ) ;
#7763=CARTESIAN_POINT ( 'NONE',  ( -11.66860950819323328, -5.915902021225889484, 34.75552854090298638 ) ) ;
#7764=CARTESIAN_POINT ( 'NONE',  ( -18.06527044596078113, -11.48612834413959405, 32.76840700105983473 ) ) ;
#7765=CARTESIAN_POINT ( 'NONE',  ( -1.253776966602621057, -7.277220443632450575, 34.74524770363009196 ) ) ;
#7766=DIRECTION ( 'NONE',  ( 0.000000000000000000, 0.000000000000000000, 1.000000000000000000 ) ) ;
#7767=CARTESIAN_POINT ( 'NONE',  ( -17.75000000000000711, -12.75000000000000178, 29.75000000000000355 ) ) ;
#7768=CARTESIAN_POINT ( 'NONE',  ( 17.20771488474786537, -2.541949514083464479, 30.39797389878540557 ) ) ;
#7769=ORIENTED_EDGE ( 'NONE', *, *, #8010, .F. ) ;
#7770=ORIENTED_EDGE ( 'NONE', *, *, #28128, .F. ) ;
#7771=ORIENTED_EDGE ( 'NONE', *, *, #62359, .F. ) ;
#7772=CARTESIAN_POINT ( 'NONE',  ( 4.023698184114455678, -3.069018819979302926, 32.56621877034667278 ) ) ;
#7773=VECTOR ( 'NONE', #48648, 1000.000000000000114 ) ;
#7775=CARTESIAN_POINT ( 'NONE',  ( -13.60810032833933469, -5.912607949931405926, 34.49155766932282319 ) ) ;
#7776=CARTESIAN_POINT ( 'NONE',  ( 11.40777093535123221, -2.295517848115769421, 30.44137282052137294 ) ) ;
#7777=DIRECTION ( 'NONE',  ( -0.000000000000000000, 0.3420201433256694901, -0.9396926207859082059 ) ) ;
#7778=FACE_BOUND ( 'NONE', #23111, .T. ) ;
#7779=DIRECTION ( 'NONE',  ( -0.000000000000000000, -0.3420201433256694901, -0.9396926207859082059 ) ) ;
#7780=ORIENTED_EDGE ( 'NONE', *, *, #7492, .F. ) ;
#7781=CARTESIAN_POINT ( 'NONE',  ( 17.32697749683652688, -12.01375889529407992, 32.43194544308182969 ) ) ;
#7782=LINE ( 'NONE', #36153, #1392 ) ;
#7783=CARTESIAN_POINT ( 'NONE',  ( -10.61538461538473577, -3.083524468854526912, 32.58852847137268327 ) ) ;
#7785=VERTEX_POINT ( 'NONE', #52530 ) ;
#7786=CARTESIAN_POINT ( 'NONE',  ( 8.769230769230768274, -12.62096338111211580, 30.90682066428153263 ) ) ;
#7787=ORIENTED_EDGE ( 'NONE', *, *, #8596, .F. ) ;
#7788=FACE_BOUND ( 'NONE', #30256, .T. ) ;
#7789=B_SPLINE_CURVE_WITH_KNOTS ( 'NONE', 3,
 ( #6619, #82289, #13815, #74193, #68763, #7060, #53014, #12494, #39976, #82732 ),
 .UNSPECIFIED., .F., .F.,
 ( 4, 2, 2, 2, 4 ),
 ( 0.0007817246336856291692, 0.0009771112958940103739, 0.001172497958102391470, 0.001367884620310772566, 0.001563271282519153663 ),
 .UNSPECIFIED. ) ;
#7790=CARTESIAN_POINT ( 'NONE',  ( -16.15384615384584777, -2.506253911140615021, 30.00000000000323297 ) ) ;
#7791=EDGE_CURVE ( 'NONE', #6141, #52855, #71059, .T. ) ;
#7792=B_SPLINE_CURVE_WITH_KNOTS ( 'NONE', 3,
 ( #18991, #12232, #5921, #88359, #54091, #67180, #81584, #19872, #5483, #82031 ),
 .UNSPECIFIED., .F., .F.,
 ( 4, 2, 2, 2, 4 ),
 ( 0.0007817246256747450040, 0.0009771112852218881168, 0.001172497944769031230, 0.001367884604316174342, 0.001563271263863317455 ),
 .UNSPECIFIED. ) ;
#7793=CARTESIAN_POINT ( 'NONE',  ( 17.01083966596718611, -11.69971097300155272, 32.46337939537587403 ) ) ;
#7795=ORIENTED_EDGE ( 'NONE', *, *, #37270, .T. ) ;
#7796=EDGE_CURVE ( 'NONE', #16308, #1913, #82875, .T. ) ;
#7797=DIRECTION ( 'NONE',  ( 0.000000000000000000, 0.7660444431189807890, 0.6427876096865361433 ) ) ;
#7798=CARTESIAN_POINT ( 'NONE',  ( -5.776987155906603277, -9.172514111537584114, 34.72667873470787470 ) ) ;
#7799=CARTESIAN_POINT ( 'NONE',  ( 8.703960768674447124, -8.656820664281498878, 34.87096338111211935 ) ) ;
#7800=CARTESIAN_POINT ( 'NONE',  ( 6.222779541268413261, -3.755027918224367767, 33.06320215134714857 ) ) ;
#7801=ORIENTED_EDGE ( 'NONE', *, *, #60754, .F. ) ;
#7802=CARTESIAN_POINT ( 'NONE',  ( 16.40390046548447245, -10.66356715214248574, 33.62249196103329751 ) ) ;
#7803=VERTEX_POINT ( 'NONE', #60175 ) ;
#7804=CARTESIAN_POINT ( 'NONE',  ( 4.284636594813106214, -2.845873456487966635, 32.17976146951972538 ) ) ;
#7805=ORIENTED_EDGE ( 'NONE', *, *, #54149, .F. ) ;
#7806=CARTESIAN_POINT ( 'NONE',  ( 7.596130608860880429, -10.76384336483936011, 33.53834819971076087 ) ) ;
#7807=CARTESIAN_POINT ( 'NONE',  ( -4.377331097570098528, -2.847400154188068022, 31.58180166144859058 ) ) ;
#7808=LINE ( 'NONE', #62734, #78854 ) ;
#7809=LINE ( 'NONE', #35275, #28633 ) ;
#7810=CARTESIAN_POINT ( 'NONE',  ( -8.769230769230768274, -12.78798330534102767, 29.49999999999997868 ) ) ;
#7811=CARTESIAN_POINT ( 'NONE',  ( -3.230769230769352962, -4.320704448113951379, 33.92786785259630022 ) ) ;
#7813=CARTESIAN_POINT ( 'NONE',  ( 16.28437185560972011, -6.001044277235009439, 34.52024696741798948 ) ) ;
#7814=EDGE_CURVE ( 'NONE', #78459, #28559, #40810, .T. ) ;
#7815=CARTESIAN_POINT ( 'NONE',  ( 12.71153846153839950, -7.565270445406050648, 34.75000000000000000 ) ) ;
#7818=CIRCLE ( 'NONE', #38020, 0.2500000000000002220 ) ;
#7819=CARTESIAN_POINT ( 'NONE',  ( 5.076923076923075762, -1.422936976036506707, 30.56769352161908415 ) ) ;
#7820=VERTEX_POINT ( 'NONE', #81356 ) ;
#7821=VECTOR ( 'NONE', #46135, 1000.000000000000227 ) ;
#7822=ORIENTED_EDGE ( 'NONE', *, *, #9348, .F. ) ;
#7823=CARTESIAN_POINT ( 'NONE',  ( -11.28840711854808632, -2.318338780012835443, 30.59689888758630261 ) ) ;
#7824=ORIENTED_EDGE ( 'NONE', *, *, #55980, .F. ) ;
#7825=CARTESIAN_POINT ( 'NONE',  ( 4.088575707885377497, -12.27809138561121394, 31.22303859784730307 ) ) ;
#7826=CARTESIAN_POINT ( 'NONE',  ( -7.976301815885541657, -8.630895178749533159, 34.87696386517710323 ) ) ;
#7827=CYLINDRICAL_SURFACE ( 'NONE', #33218, 0.2499999999999994726 ) ;
#7828=CARTESIAN_POINT ( 'NONE',  ( 1.161688425708538031, -2.523278758544489353, 31.42238647778637528 ) ) ;
#7829=CARTESIAN_POINT ( 'NONE',  ( 10.83839745947800992, -6.460100341425560444, 34.89618726649961644 ) ) ;
#7830=CARTESIAN_POINT ( 'NONE',  ( 12.39626801557768587, -10.90142922261923886, 33.41473453929638993 ) ) ;
#7831=CARTESIAN_POINT ( 'NONE',  ( 17.07692307692307665, -8.164416787775445883, 34.95778746994557906 ) ) ;
#7833=CYLINDRICAL_SURFACE ( 'NONE', #7475, 0.2500000000000009437 ) ;
#7834=CARTESIAN_POINT ( 'NONE',  ( 18.00000000000000000, -11.69971097300155272, 32.46337939537588113 ) ) ;
#7835=EDGE_CURVE ( 'NONE', #88017, #89081, #47101, .T. ) ;
#7836=EDGE_CURVE ( 'NONE', #16729, #66445, #19205, .T. ) ;
#7837=LINE ( 'NONE', #63208, #86753 ) ;
#7838=B_SPLINE_CURVE_WITH_KNOTS ( 'NONE', 3,
 ( #72453, #31931, #23811, #24720, #3104, #78770, #17071, #17970, #30579, #52178 ),
 .UNSPECIFIED., .F., .F.,
 ( 4, 2, 2, 2, 4 ),
 ( 0.0007817359430256399806, 0.0009771253907250089001, 0.001172514838424378036, 0.001367904286123746956, 0.001563293733823115875 ),
 .UNSPECIFIED. ) ;
#7839=CARTESIAN_POINT ( 'NONE',  ( 11.66925334628632882, -4.809403383903225304, 33.96459661697924304 ) ) ;
#7840=B_SPLINE_CURVE_WITH_KNOTS ( 'NONE', 3,
 ( #46597, #24986, #87158, #53790, #59659, #25436, #53343, #19126, #80844, #74076 ),
 .UNSPECIFIED., .F., .F.,
 ( 4, 2, 2, 2, 4 ),
 ( 0.0007817246256747445703, 0.0009771112852218872494, 0.001172497944769030145, 0.001367884604316172825, 0.001563271263863315504 ),
 .UNSPECIFIED. ) ;
#7841=EDGE_CURVE ( 'NONE', #67170, #38356, #73195, .T. ) ;
#7842=EDGE_LOOP ( 'NONE', ( #76539, #32485, #86213, #29033 ) ) ;
#7843=ORIENTED_EDGE ( 'NONE', *, *, #8207, .T. ) ;
#7844=EDGE_CURVE ( 'NONE', #72978, #82350, #39043, .T. ) ;
#7845=DIRECTION ( 'NONE',  ( 1.000000000000000000, 0.000000000000000000, 0.000000000000000000 ) ) ;
#7846=LINE ( 'NONE', #15046, #20121 ) ;
#7847=CARTESIAN_POINT ( 'NONE',  ( 3.230769230769231726, -10.67929555188718282, 33.92786785259544047 ) ) ;
#7848=DIRECTION ( 'NONE',  ( -0.000000000000000000, 0.6427876096865404731, -0.7660444431189771253 ) ) ;
#7849=EDGE_LOOP ( 'NONE', ( #58330, #72961, #23904, #18650 ) ) ;
#7851=CARTESIAN_POINT ( 'NONE',  ( 11.53846153846141576, -4.320704448113951379, 33.92786785259630022 ) ) ;
#7852=VECTOR ( 'NONE', #74586, 1000.000000000000227 ) ;
#7853=FACE_OUTER_BOUND ( 'NONE', #1895, .T. ) ;
#7854=ORIENTED_EDGE ( 'NONE', *, *, #6336, .F. ) ;
#7855=CARTESIAN_POINT ( 'NONE',  ( -14.53061926659915315, -12.64616026154729411, 30.79003144601914244 ) ) ;
#7856=ORIENTED_EDGE ( 'NONE', *, *, #23569, .T. ) ;
#7857=CARTESIAN_POINT ( 'NONE',  ( -8.769230769230768274, -7.500000000000001776, 35.04278698407183867 ) ) ;
#7858=CARTESIAN_POINT ( 'NONE',  ( 4.403846153847572609, -7.500000000000154543, 35.00000000000007105 ) ) ;
#7859=CARTESIAN_POINT ( 'NONE',  ( -1.608100309179714360, -9.417330523894424488, 34.63758898049880486 ) ) ;
#7860=CARTESIAN_POINT ( 'NONE',  ( -2.307692307692305711, -11.69971097300155272, 32.46337939537588113 ) ) ;
#7861=CARTESIAN_POINT ( 'NONE',  ( -2.980769230767811084, -7.500000000000154543, 35.00000000000007105 ) ) ;
#7862=ORIENTED_EDGE ( 'NONE', *, *, #85061, .T. ) ;
#7863=VERTEX_POINT ( 'NONE', #6575 ) ;
#7864=B_SPLINE_CURVE_WITH_KNOTS ( 'NONE', 3,
 ( #47120, #67407, #47570, #32727, #34061, #19223, #68291, #12029, #87697, #40391 ),
 .UNSPECIFIED., .F., .F.,
 ( 4, 2, 2, 2, 4 ),
 ( 0.0007817246256747472808, 0.0009771112852218907189, 0.001172497944769034265, 0.001367884604316177595, 0.001563271263863321141 ),
 .UNSPECIFIED. ) ;
#7865=EDGE_CURVE ( 'NONE', #43710, #77653, #86062, .T. ) ;
#7866=ORIENTED_EDGE ( 'NONE', *, *, #13576, .F. ) ;
#7867=VERTEX_POINT ( 'NONE', #13767 ) ;
#7868=CARTESIAN_POINT ( 'NONE',  ( 13.16168916709923664, -3.105860786376062332, 32.13614157043599562 ) ) ;
#7869=CARTESIAN_POINT ( 'NONE',  ( -12.71156168575991785, -12.68155406624981119, 30.59749803192733708 ) ) ;
#7870=CARTESIAN_POINT ( 'NONE',  ( -4.219116154402471786, -12.51329471203370325, 31.30864560766548976 ) ) ;
#7871=AXIS2_PLACEMENT_3D ( 'NONE', #9847, #64776, #3079 ) ;
#7872=CARTESIAN_POINT ( 'NONE',  ( 16.85399611801622299, -10.01117774369187252, 34.36070679894347535 ) ) ;
#7874=CARTESIAN_POINT ( 'NONE',  ( 14.43821800945587341, -10.19071101563364756, 33.96452234770658407 ) ) ;
#7875=VERTEX_POINT ( 'NONE', #7906 ) ;
#7877=ADVANCED_FACE ( 'NONE', ( #69163 ), #7467, .F. ) ;
#7878=EDGE_LOOP ( 'NONE', ( #31110, #78542, #65387, #46441 ) ) ;
#7879=CARTESIAN_POINT ( 'NONE',  ( 4.376625822824220080, -4.226511098958374291, 33.85474049983370293 ) ) ;
#7881=CARTESIAN_POINT ( 'NONE',  ( -16.94639737515951339, -9.417988943895561960, 34.36773134775778260 ) ) ;
#7882=CARTESIAN_POINT ( 'NONE',  ( 13.44987052412822237, -4.320704448112861584, 33.92786785259548310 ) ) ;
#7884=CARTESIAN_POINT ( 'NONE',  ( 13.51514108637895006, -8.586989748646452369, 34.63063291749215011 ) ) ;
#7885=ORIENTED_EDGE ( 'NONE', *, *, #34867, .T. ) ;
#7886=ORIENTED_EDGE ( 'NONE', *, *, #75416, .T. ) ;
#7887=CARTESIAN_POINT ( 'NONE',  ( 3.930919194939302308, -4.026226216239095379, 33.68668979543632958 ) ) ;
#7888=ORIENTED_EDGE ( 'NONE', *, *, #59827, .T. ) ;
#7889=FACE_BOUND ( 'NONE', #48450, .T. ) ;
#7890=CARTESIAN_POINT ( 'NONE',  ( 6.673053685783957967, -4.335965774309649134, 33.62209801155881905 ) ) ;
#7891=ADVANCED_FACE ( 'NONE', ( #700 ), #69601, .F. ) ;
#7892=LINE ( 'NONE', #83567, #34752 ) ;
#7895=CARTESIAN_POINT ( 'NONE',  ( -16.15384615384615330, -12.62096338111211580, 30.90682066428153263 ) ) ;
#7896=DIRECTION ( 'NONE',  ( 0.000000000000000000, 1.000000000000000000, 0.000000000000000000 ) ) ;
#7897=EDGE_CURVE ( 'NONE', #80982, #4310, #15110, .T. ) ;
#7898=CARTESIAN_POINT ( 'NONE',  ( 0.5276068125408991394, -6.386643153685127139, 34.62446782046654192 ) ) ;
#7899=CARTESIAN_POINT ( 'NONE',  ( 15.48071464014727283, -6.653508905675592722, 34.93172785388651391 ) ) ;
#7900=ORIENTED_EDGE ( 'NONE', *, *, #4457, .F. ) ;
#7902=CARTESIAN_POINT ( 'NONE',  ( -11.28851612908349722, -12.45601412856602686, 31.48342859153981621 ) ) ;
#7903=LINE ( 'NONE', #83577, #12377 ) ;
#7905=CARTESIAN_POINT ( 'NONE',  ( 6.000000000000001776, -4.786620604624113540, 33.94971097300155094 ) ) ;
#7906=CARTESIAN_POINT ( 'NONE',  ( -8.769230769230890843, -2.625532179533778709, 30.86335684631627174 ) ) ;
#7907=FACE_BOUND ( 'NONE', #19903, .T. ) ;
#7908=CARTESIAN_POINT ( 'NONE',  ( -6.923076923076922462, -12.62096338111211580, 30.90682066428153263 ) ) ;
#7909=DIRECTION ( 'NONE',  ( -1.000000000000000000, 0.000000000000000000, 0.000000000000000000 ) ) ;
#7910=EDGE_CURVE ( 'NONE', #16403, #59207, #12742, .T. ) ;
#7911=CARTESIAN_POINT ( 'NONE',  ( -14.43838291080261627, -3.338472653186243644, 32.95098750199972670 ) ) ;
#7912=CARTESIAN_POINT ( 'NONE',  ( -11.31545018684868964, -11.24521262558773493, 33.06293181088029343 ) ) ;
#7913=CARTESIAN_POINT ( 'NONE',  ( 5.999999999999880096, -10.90142922262034020, 33.41473453929536674 ) ) ;
#7914=DIRECTION ( 'NONE',  ( 0.000000000000000000, 0.8660254037844377084, -0.5000000000000015543 ) ) ;
#7916=ORIENTED_EDGE ( 'NONE', *, *, #5049, .T. ) ;
#7917=CARTESIAN_POINT ( 'NONE',  ( -8.899707477347234885, -7.276988635370452485, 34.74523720219453793 ) ) ;
#7918=ORIENTED_EDGE ( 'NONE', *, *, #58239, .F. ) ;
#7919=ADVANCED_FACE ( 'NONE', ( #49335 ), #61949, .F. ) ;
#7920=CARTESIAN_POINT ( 'NONE',  ( -18.00000000000000000, -6.386643153685127139, 34.62446782046654192 ) ) ;
#7922=CARTESIAN_POINT ( 'NONE',  ( -11.28840711854808632, -6.523592122091592671, 34.90882529074906415 ) ) ;
#7923=CARTESIAN_POINT ( 'NONE',  ( 14.05766908347084865, -4.175268141568685643, 33.81360843649122216 ) ) ;
#7924=EDGE_CURVE ( 'NONE', #27570, #17114, #11885, .T. ) ;
#7925=VERTEX_POINT ( 'NONE', #34922 ) ;
#7926=CARTESIAN_POINT ( 'NONE',  ( -9.942307692307691624, -7.566083408709835645, 34.74999999999999289 ) ) ;
#7928=CARTESIAN_POINT ( 'NONE',  ( -10.36533019547115941, -12.65882529074907126, 30.72640787790839312 ) ) ;
#7929=CARTESIAN_POINT ( 'NONE',  ( 6.989145274079363368, -8.973038597847269315, 34.52809138561122637 ) ) ;
#7930=CARTESIAN_POINT ( 'NONE',  ( 5.076923076922954969, -6.879047030192662504, 34.71129190930017927 ) ) ;
#7931=DIRECTION ( 'NONE',  ( -1.000000000000000000, 0.000000000000000000, 0.000000000000000000 ) ) ;
#7933=CARTESIAN_POINT ( 'NONE',  ( -6.000000000000119904, -10.90142922262034020, 33.41473453929536674 ) ) ;
#7935=VECTOR ( 'NONE', #43237, 1000.000000000000114 ) ;
#7936=DIRECTION ( 'NONE',  ( -0.000000000000000000, 0.7660444431189791237, -0.6427876096865379196 ) ) ;
#7937=CARTESIAN_POINT ( 'NONE',  ( 10.86533013373275658, -11.37275283266504111, 32.91324779482534524 ) ) ;
#7938=EDGE_CURVE ( 'NONE', #14112, #37020, #18542, .T. ) ;
#7941=CARTESIAN_POINT ( 'NONE',  ( -17.32692307692307665, -7.500000000000001776, 34.75000000000000000 ) ) ;
#7942=LINE ( 'NONE', #75956, #39776 ) ;
#7943=ORIENTED_EDGE ( 'NONE', *, *, #17262, .T. ) ;
#7944=ADVANCED_FACE ( 'NONE', ( #42582 ), #34486, .F. ) ;
#7945=CARTESIAN_POINT ( 'NONE',  ( -17.77722045873158763, -2.847695495035523106, 31.58253572463339154 ) ) ;
#7946=CARTESIAN_POINT ( 'NONE',  ( 16.21991348719623360, -2.486705287966280320, 31.30864560766543647 ) ) ;
#7947=CARTESIAN_POINT ( 'NONE',  ( -0.4615384615384611200, -4.102666532097928531, 36.13435417666054406 ) ) ;
#7949=CARTESIAN_POINT ( 'NONE',  ( -14.53061852520845498, -11.76352882383564769, 32.36236540154569497 ) ) ;
#7950=EDGE_CURVE ( 'NONE', #62974, #19083, #28166, .T. ) ;
#7951=CARTESIAN_POINT ( 'NONE',  ( -1.449885830576159940, -10.90142922261923886, 33.41473453929638993 ) ) ;
#7953=CARTESIAN_POINT ( 'NONE',  ( -39.05038313613820122, -2.499999999999999556, 29.75000000000000355 ) ) ;
#7954=CARTESIAN_POINT ( 'NONE',  ( -10.39260507411620260, -10.81320215134717344, 33.49497208177562868 ) ) ;
#7955=ORIENTED_EDGE ( 'NONE', *, *, #88303, .T. ) ;
#7956=CARTESIAN_POINT ( 'NONE',  ( 7.053602361310566948, -11.66157788607254275, 32.95092075102925833 ) ) ;
#7957=VERTEX_POINT ( 'NONE', #8799 ) ;
#7958=B_SPLINE_CURVE_WITH_KNOTS ( 'NONE', 3,
 ( #45510, #37869, #65332, #74208, #12507, #58568, #86061, #24341, #60685, #81419 ),
 .UNSPECIFIED., .F., .F.,
 ( 4, 2, 2, 2, 4 ),
 ( 0.000000000000000000, 0.0001954311564186877418, 0.0003908623128373754836, 0.0005862934692560632524, 0.0007817246256747509671 ),
 .UNSPECIFIED. ) ;
#7959=B_SPLINE_CURVE_WITH_KNOTS ( 'NONE', 3,
 ( #7834, #69970, #77173, #54673, #48808, #20464, #83054, #22231, #70424, #56013 ),
 .UNSPECIFIED., .F., .F.,
 ( 4, 2, 2, 2, 4 ),
 ( 0.000000000000000000, 0.0001954339857564096699, 0.0003908679715128193398, 0.0005863019572692289554, 0.0007817359430256386795 ),
 .UNSPECIFIED. ) ;
#7960=EDGE_LOOP ( 'NONE', ( #80731, #3323 ) ) ;
#7961=CYLINDRICAL_SURFACE ( 'NONE', #34096, 0.2499999999999979738 ) ;
#7962=CARTESIAN_POINT ( 'NONE',  ( 6.857806477116149324, -2.892918686051582089, 31.69288490824015270 ) ) ;
#7963=EDGE_CURVE ( 'NONE', #23024, #87173, #261, .T. ) ;
#7964=CARTESIAN_POINT ( 'NONE',  ( 9.942362003946010773, -4.943051570960394159, 34.04725096376909477 ) ) ;
#7965=CARTESIAN_POINT ( 'NONE',  ( 13.31853300525524908, -8.164416787775445883, 34.95778746994557906 ) ) ;
#7966=ORIENTED_EDGE ( 'NONE', *, *, #14932, .F. ) ;
#7967=CARTESIAN_POINT ( 'NONE',  ( -17.29984929443921970, -4.186968288167451036, 33.49512374952580274 ) ) ;
#7968=EDGE_LOOP ( 'NONE', ( #38906, #47783, #15264, #4169 ) ) ;
#7970=EDGE_LOOP ( 'NONE', ( #62182, #86002, #35987, #14720 ) ) ;
#7971=ORIENTED_EDGE ( 'NONE', *, *, #65140, .T. ) ;
#7974=CARTESIAN_POINT ( 'NONE',  ( -4.826977667545032880, -12.45601412856602863, 31.48342859153981621 ) ) ;
#7975=EDGE_CURVE ( 'NONE', #42322, #16211, #70491, .T. ) ;
#7976=CARTESIAN_POINT ( 'NONE',  ( -3.230769230769352962, -12.16647553114689728, 32.15551576947799362 ) ) ;
#7977=ADVANCED_FACE ( 'NONE', ( #41690 ), #77683, .F. ) ;
#7978=DIRECTION ( 'NONE',  ( 0.000000000000000000, 0.9396926207859126468, -0.3420201433256571111 ) ) ;
#7979=CARTESIAN_POINT ( 'NONE',  ( -5.142679879437387136, -7.249945686854186278, 34.74374336980224598 ) ) ;
#7980=ORIENTED_EDGE ( 'NONE', *, *, #74850, .T. ) ;
#7981=ORIENTED_EDGE ( 'NONE', *, *, #62093, .T. ) ;
#7982=EDGE_CURVE ( 'NONE', #41734, #74112, #44324, .T. ) ;
#7984=CARTESIAN_POINT ( 'NONE',  ( -2.084679463598910765, -3.395485233115138168, 33.02377354290276656 ) ) ;
#7985=CARTESIAN_POINT ( 'NONE',  ( 4.403900465484468008, -11.28795663066794219, 33.01431243580653785 ) ) ;
#7986=ORIENTED_EDGE ( 'NONE', *, *, #61460, .T. ) ;
#7987=LINE ( 'NONE', #1668, #19163 ) ;
#7989=B_SPLINE_CURVE_WITH_KNOTS ( 'NONE', 3,
 ( #42711, #394, #70617, #43580, #37710, #58411, #85024, #71053, #37259, #10251 ),
 .UNSPECIFIED., .F., .F.,
 ( 4, 2, 2, 2, 4 ),
 ( 0.000000000000000000, 0.0001954311584214072923, 0.0003908623168428145846, 0.0005862934752642218498, 0.0007817246336856291692 ),
 .UNSPECIFIED. ) ;
#7990=VECTOR ( 'NONE', #5151, 1000.000000000000000 ) ;
#7991=CARTESIAN_POINT ( 'NONE',  ( -0.3307480205715107036, -9.084667340241226796, 34.75534355489798344 ) ) ;
#7992=ORIENTED_EDGE ( 'NONE', *, *, #61695, .F. ) ;
#7993=DIRECTION ( 'NONE',  ( 0.000000000000000000, 0.6427876096865368094, 0.7660444431189802339 ) ) ;
#7994=CARTESIAN_POINT ( 'NONE',  ( 15.16468685140909400, -2.486705287966279432, 31.30864560766542937 ) ) ;
#7996=FACE_BOUND ( 'NONE', #11816, .T. ) ;
#7997=CARTESIAN_POINT ( 'NONE',  ( -18.00000000000000000, -12.50000000000000000, 29.74999999999997868 ) ) ;
#7998=CARTESIAN_POINT ( 'NONE',  ( 13.38461538461526423, -6.835583212225970762, 34.95778746994575670 ) ) ;
#7999=B_SPLINE_CURVE_WITH_KNOTS ( 'NONE', 3,
 ( #49676, #77152, #71262, #85245, #64495, #43365, #70847, #64950, #15461, #76713 ),
 .UNSPECIFIED., .F., .F.,
 ( 4, 2, 2, 2, 4 ),
 ( 0.0007817359430256315238, 0.0009771253907249976244, 0.001172514838424363508, 0.001367904286123729392, 0.001563293733823095492 ),
 .UNSPECIFIED. ) ;
#8000=CYLINDRICAL_SURFACE ( 'NONE', #52354, 2.000000000000001776 ) ;
#8002=CARTESIAN_POINT ( 'NONE',  ( 18.22301135161285046, -4.187068189119696804, 33.49521262558774026 ) ) ;
#8003=CARTESIAN_POINT ( 'NONE',  ( -11.53846153846166089, -10.33852847137269571, 34.16647553114546554 ) ) ;
#8004=CARTESIAN_POINT ( 'NONE',  ( -2.372962753653082402, -3.835265460703609186, 33.15142922261924241 ) ) ;
#8006=DIRECTION ( 'NONE',  ( 0.000000000000000000, 0.6427876096865368094, 0.7660444431189802339 ) ) ;
#8007=DIRECTION ( 'NONE',  ( 0.000000000000000000, 0.3420201433256610524, 0.9396926207859113145 ) ) ;
#8008=EDGE_CURVE ( 'NONE', #17545, #64477, #74256, .T. ) ;
#8009=ORIENTED_EDGE ( 'NONE', *, *, #19204, .T. ) ;
#8010=EDGE_CURVE ( 'NONE', #5191, #47721, #52706, .T. ) ;
#8012=CARTESIAN_POINT ( 'NONE',  ( 9.562160482869474620, -2.882441371585227508, 31.66841991370172238 ) ) ;
#8014=CARTESIAN_POINT ( 'NONE',  ( -0.2387589202700529378, -12.44528174975671853, 30.48912976160716681 ) ) ;
#8015=DIRECTION ( 'NONE',  ( -0.000000000000000000, -0.7660444431189791237, -0.6427876096865379196 ) ) ;
#8016=FACE_BOUND ( 'NONE', #31257, .T. ) ;
#8017=CARTESIAN_POINT ( 'NONE',  ( -5.076923076923197442, -2.892918686052165622, 31.69288490824153470 ) ) ;
#8018=CARTESIAN_POINT ( 'NONE',  ( 15.23076923076923173, -12.10708131394839349, 31.69288490824020244 ) ) ;
#8020=CARTESIAN_POINT ( 'NONE',  ( 12.21156171748987163, -12.41104346484419452, 31.60698883733904196 ) ) ;
#8021=CARTESIAN_POINT ( 'NONE',  ( -3.099977422944444783, -11.71459661697925903, 32.44059661609676937 ) ) ;
#8022=CARTESIAN_POINT ( 'NONE',  ( 7.780902855992604117, -2.506253911140460922, 30.00000000000013856 ) ) ;
#8023=CARTESIAN_POINT ( 'NONE',  ( -14.17690186672535901, -5.496552790871120031, 34.60292014791297532 ) ) ;
#8025=ORIENTED_EDGE ( 'NONE', *, *, #44155, .F. ) ;
#8026=VERTEX_POINT ( 'NONE', #58299 ) ;
#8028=VECTOR ( 'NONE', #69628, 1000.000000000000227 ) ;
#8029=CARTESIAN_POINT ( 'NONE',  ( -10.48485917715096782, -8.630441415882550871, 34.87705825610312615 ) ) ;
#8030=CARTESIAN_POINT ( 'NONE',  ( 1.607395053593452694, -9.418065098278011860, 34.63729479722530158 ) ) ;
#8031=CARTESIAN_POINT ( 'NONE',  ( -0.4615384615385840772, -3.083524468854526912, 32.58852847137268327 ) ) ;
#8032=CARTESIAN_POINT ( 'NONE',  ( -13.38461538461550759, -2.657715359629662544, 31.77849191805970364 ) ) ;
#8035=DIRECTION ( 'NONE',  ( -1.000000000000000000, 0.000000000000000000, 0.000000000000000000 ) ) ;
#8037=CYLINDRICAL_SURFACE ( 'NONE', #1319, 0.2499999999999997502 ) ;
#8038=CARTESIAN_POINT ( 'NONE',  ( 7.623226887246997485, -5.582147617184174848, 34.63737895849758530 ) ) ;
#8039=DIRECTION ( 'NONE',  ( -0.000000000000000000, 1.000000000000000000, 3.491481338843133355E-15 ) ) ;
#8040=CARTESIAN_POINT ( 'NONE',  ( -17.07692307692307665, -2.249999999999998668, 29.75000000000001776 ) ) ;
#8041=B_SPLINE_CURVE_WITH_KNOTS ( 'NONE', 3,
 ( #28589, #70461, #43429, #83092, #1997, #77207, #1111, #42985, #70005, #22703 ),
 .UNSPECIFIED., .F., .F.,
 ( 4, 2, 2, 2, 4 ),
 ( 0.0007817246256747478229, 0.0009771112852218913694, 0.001172497944769034916, 0.001367884604316178679, 0.001563271263863322226 ),
 .UNSPECIFIED. ) ;
#8042=CARTESIAN_POINT ( 'NONE',  ( -9.692307692307814193, -12.70778746994576025, 30.41441678777401236 ) ) ;
#8043=DIRECTION ( 'NONE',  ( -0.000000000000000000, 0.9396926207859092051, -0.3420201433256662704 ) ) ;
#8044=ADVANCED_FACE ( 'NONE', ( #45231 ), #64158, .F. ) ;
#8045=ADVANCED_FACE ( 'NONE', ( #65505 ), #43461, .F. ) ;
#8046=CARTESIAN_POINT ( 'NONE',  ( -12.71153846153846168, -2.499999999999998668, 29.75000000000000355 ) ) ;
#8047=EDGE_LOOP ( 'NONE', ( #555, #12318, #44257, #88757 ) ) ;
#8048=CARTESIAN_POINT ( 'NONE',  ( -14.37377571864818293, -3.513871655860377086, 32.76840700105978499 ) ) ;
#8049=CARTESIAN_POINT ( 'NONE',  ( 7.846153846153846700, -4.661471528628507777, 34.16647553114623292 ) ) ;
#8051=ADVANCED_FACE ( 'NONE', ( #72260 ), #2460, .F. ) ;
#8052=DIRECTION ( 'NONE',  ( -0.000000000000000000, 0.7660444431189791237, -0.6427876096865379196 ) ) ;
#8054=ORIENTED_EDGE ( 'NONE', *, *, #54675, .F. ) ;
#8055=CARTESIAN_POINT ( 'NONE',  ( -9.758390071667825794, -5.471508081941602875, 34.59228464037088457 ) ) ;
#8056=CARTESIAN_POINT ( 'NONE',  ( -9.692307692307691624, -4.786620604624113540, 33.94971097300155094 ) ) ;
#8057=VERTEX_POINT ( 'NONE', #57410 ) ;
#8058=CARTESIAN_POINT ( 'NONE',  ( 7.173131234715237170, -3.627508038966690496, 32.91356715214248396 ) ) ;
#8059=CARTESIAN_POINT ( 'NONE',  ( -2.438382910802613157, -10.70098750199973203, 33.91152734681376302 ) ) ;
#8060=EDGE_CURVE ( 'NONE', #24465, #37632, #85790, .T. ) ;
#8061=EDGE_LOOP ( 'NONE', ( #80915, #38701, #80256, #24488 ) ) ;
#8062=DIRECTION ( 'NONE',  ( 0.000000000000000000, -1.000000000000000000, 0.000000000000000000 ) ) ;
#8063=CARTESIAN_POINT ( 'NONE',  ( 13.38461538461538680, -9.058645607665452459, 34.76329471203371924 ) ) ;
#8064=EDGE_CURVE ( 'NONE', #23956, #32626, #76075, .T. ) ;
#8066=CARTESIAN_POINT ( 'NONE',  ( 17.01165263096230262, -11.48612834413959582, 32.76840700105983473 ) ) ;
#8069=VERTEX_POINT ( 'NONE', #72707 ) ;
#8070=EDGE_LOOP ( 'NONE', ( #71863, #42234 ) ) ;
#8071=ADVANCED_FACE ( 'NONE', ( #10570 ), #37137, .F. ) ;
#8072=CARTESIAN_POINT ( 'NONE',  ( -10.55012947587177941, -2.379036618887895305, 30.90682066428158592 ) ) ;
#8073=ORIENTED_EDGE ( 'NONE', *, *, #79413, .T. ) ;
#8074=CARTESIAN_POINT ( 'NONE',  ( -10.55023983466498017, -7.750023224968867197, 34.99404313364389907 ) ) ;
#8075=CARTESIAN_POINT ( 'NONE',  ( 5.326977496836529546, -4.818054556918156095, 34.26375889529406749 ) ) ;
#8076=CARTESIAN_POINT ( 'NONE',  ( -14.37377571864818293, -3.050289026998445951, 32.03036669348365706 ) ) ;
#8077=ADVANCED_FACE ( 'NONE', ( #23628 ), #78572, .F. ) ;
#8079=CARTESIAN_POINT ( 'NONE',  ( -5.076923076923197442, -12.27809138561165270, 31.22303859784587132 ) ) ;
#8080=CARTESIAN_POINT ( 'NONE',  ( 11.53846153846153832, -1.629998284177014645, 34.34916445242399163 ) ) ;
#8081=CARTESIAN_POINT ( 'NONE',  ( 15.48076923076923705, -2.499999999999999556, 29.81604066197449754 ) ) ;
#8082=ORIENTED_EDGE ( 'NONE', *, *, #10857, .F. ) ;
#8083=ORIENTED_EDGE ( 'NONE', *, *, #30057, .F. ) ;
#8084=DIRECTION ( 'NONE',  ( -0.000000000000000000, 0.5000000000000011102, -0.8660254037844381525 ) ) ;
#8085=ORIENTED_EDGE ( 'NONE', *, *, #65230, .F. ) ;
#8087=CARTESIAN_POINT ( 'NONE',  ( 7.622668921589513147, -2.612411019501189369, 31.66733052389439962 ) ) ;
#8088=ORIENTED_EDGE ( 'NONE', *, *, #59355, .F. ) ;
#8089=AXIS2_PLACEMENT_3D ( 'NONE', #20353, #54114, #80733 ) ;
#8090=CARTESIAN_POINT ( 'NONE',  ( 9.692307692307695177, -12.48256725967547354, 35.29906147534542527 ) ) ;
#8091=CARTESIAN_POINT ( 'NONE',  ( 8.096208157792160520, -4.943051570960394159, 34.04725096376909477 ) ) ;
#8092=ORIENTED_EDGE ( 'NONE', *, *, #86036, .F. ) ;
#8093=CARTESIAN_POINT ( 'NONE',  ( -12.46153846153858247, -6.026961402154118019, 34.52809138561165270 ) ) ;
#8094=AXIS2_PLACEMENT_3D ( 'NONE', #49374, #78611, #70084 ) ;
#8095=EDGE_CURVE ( 'NONE', #62614, #4262, #87196, .T. ) ;
#8097=CARTESIAN_POINT ( 'NONE',  ( -8.546451227962359454, -8.496831190052096971, 34.64984203495476578 ) ) ;
#8099=CARTESIAN_POINT ( 'NONE',  ( -14.24243716817946925, -12.16647553114626490, 32.15551576947920864 ) ) ;
#8100=VERTEX_POINT ( 'NONE', #26746 ) ;
#8101=EDGE_CURVE ( 'NONE', #45738, #41484, #66759, .T. ) ;
#8102=CARTESIAN_POINT ( 'NONE',  ( 14.30769230769231015, -2.499999999999998668, 29.75000000000001421 ) ) ;
#8103=CARTESIAN_POINT ( 'NONE',  ( 17.93472999944368240, -12.51329471203370325, 31.30864560766548976 ) ) ;
#8104=FACE_BOUND ( 'NONE', #85866, .T. ) ;
#8105=CARTESIAN_POINT ( 'NONE',  ( 1.634560902963529072, -12.43552623307873972, 30.55307653245132826 ) ) ;
#8106=CARTESIAN_POINT ( 'NONE',  ( -18.00000000000000000, -12.10708131394839349, 31.69288490824020244 ) ) ;
#8107=CARTESIAN_POINT ( 'NONE',  ( 9.469380733400843297, -11.43668979543634734, 33.22377378376089752 ) ) ;
#8108=CARTESIAN_POINT ( 'NONE',  ( 12.39626846098214230, -3.643525952247789412, 33.31231777344662959 ) ) ;
#8109=CARTESIAN_POINT ( 'NONE',  ( 6.000000000000001776, -12.37446782046654192, 30.86335684631486131 ) ) ;
#8110=CARTESIAN_POINT ( 'NONE',  ( -16.28453762051371356, -8.147922237126337563, 34.70805685702651999 ) ) ;
#8111=ORIENTED_EDGE ( 'NONE', *, *, #69050, .T. ) ;
#8112=CYLINDRICAL_SURFACE ( 'NONE', #33152, 0.2500000000000002220 ) ;
#8114=EDGE_CURVE ( 'NONE', #32882, #3366, #81702, .T. ) ;
#8115=ORIENTED_EDGE ( 'NONE', *, *, #42048, .T. ) ;
#8116=CARTESIAN_POINT ( 'NONE',  ( 9.692307692308007816, -2.255955759149395501, 30.00000000000324363 ) ) ;
#8117=DIRECTION ( 'NONE',  ( 0.000000000000000000, 0.3420201433256610524, 0.9396926207859113145 ) ) ;
#8118=EDGE_CURVE ( 'NONE', #21774, #75150, #12350, .T. ) ;
#8119=DIRECTION ( 'NONE',  ( -0.000000000000000000, -0.8660254037844399289, -0.4999999999999980016 ) ) ;
#8120=CARTESIAN_POINT ( 'NONE',  ( -16.82697766754503377, -10.18230066228895758, 34.26354781536631577 ) ) ;
#8121=CARTESIAN_POINT ( 'NONE',  ( 5.076923076923075762, -5.180354513474913603, 36.12317359536750416 ) ) ;
#8122=CARTESIAN_POINT ( 'NONE',  ( -12.39547112818838492, -4.661471528628508665, 34.16647553114624003 ) ) ;
#8123=ADVANCED_FACE ( 'NONE', ( #60080 ), #4708, .F. ) ;
#8125=VECTOR ( 'NONE', #1064, 1000.000000000000114 ) ;
#8126=CARTESIAN_POINT ( 'NONE',  ( 11.53846153846141576, -3.643525952248795718, 33.31231777344771672 ) ) ;
#8127=CARTESIAN_POINT ( 'NONE',  ( -6.065270445960775803, -6.879047030191174805, 34.71129190930000163 ) ) ;
#8129=CARTESIAN_POINT ( 'NONE',  ( 10.61538461538461675, -8.120952969808772792, 34.71129190930000163 ) ) ;
#8130=CARTESIAN_POINT ( 'NONE',  ( 2.372947447205147942, -5.941354392334606160, 34.76329471203374055 ) ) ;
#8131=VERTEX_POINT ( 'NONE', #53322 ) ;
#8132=CARTESIAN_POINT ( 'NONE',  ( -0.5276208408985981757, -2.292212530054419606, 30.41441678777542634 ) ) ;
#8133=VERTEX_POINT ( 'NONE', #5147 ) ;
#8135=ORIENTED_EDGE ( 'NONE', *, *, #69016, .T. ) ;
#8136=CARTESIAN_POINT ( 'NONE',  ( -6.000000000000121680, -4.320704448113951379, 33.92786785259630022 ) ) ;
#8137=EDGE_LOOP ( 'NONE', ( #55390, #48515 ) ) ;
#8141=CARTESIAN_POINT ( 'NONE',  ( -17.14219307747939069, -12.70778746994557551, 30.41441678777548319 ) ) ;
#8142=DIRECTION ( 'NONE',  ( -0.000000000000000000, 1.000000000000000000, 3.491481338843133355E-15 ) ) ;
#8143=CARTESIAN_POINT ( 'NONE',  ( 8.703960323269994248, -6.879047030191174805, 34.71129190930000163 ) ) ;
#8145=CARTESIAN_POINT ( 'NONE',  ( -11.40762320797477614, -7.277220318596961057, 34.99547417642776992 ) ) ;
#8146=CARTESIAN_POINT ( 'NONE',  ( -17.07692307692319744, -4.481592998941358097, 33.73612834414048933 ) ) ;
#8147=ORIENTED_EDGE ( 'NONE', *, *, #57036, .T. ) ;
#8148=CARTESIAN_POINT ( 'NONE',  ( -6.000000000000121680, -3.643525952248796163, 33.31231777344771672 ) ) ;
#8149=LINE ( 'NONE', #63070, #71463 ) ;
#8150=CARTESIAN_POINT ( 'NONE',  ( -17.32689982097166492, -12.01397095200673881, 32.43157075238190146 ) ) ;
#8151=CARTESIAN_POINT ( 'NONE',  ( 15.48082365068267841, -2.920487667080175598, 32.31805714834170828 ) ) ;
#8152=CARTESIAN_POINT ( 'NONE',  ( -9.915234651214539952, -12.38737895849757820, 31.66785238281580206 ) ) ;
#8154=DIRECTION ( 'NONE',  ( 0.000000000000000000, 0.6427876096865368094, 0.7660444431189802339 ) ) ;
#8156=ORIENTED_EDGE ( 'NONE', *, *, #39642, .T. ) ;
#8157=CARTESIAN_POINT ( 'NONE',  ( -16.94639737515951339, -10.88167719472716399, 33.43325721877153711 ) ) ;
#8158=CARTESIAN_POINT ( 'NONE',  ( -13.51476259405360203, -9.418419913701741919, 34.36755862841477693 ) ) ;
#8159=CARTESIAN_POINT ( 'NONE',  ( 8.834485908743605620, -11.06231777344671130, 33.60647404775212976 ) ) ;
#8160=AXIS2_PLACEMENT_3D ( 'NONE', #14261, #48475, #70085 ) ;
#8161=CARTESIAN_POINT ( 'NONE',  ( 9.626225312947559232, -6.343179335718451384, 34.87096338111212646 ) ) ;
#8162=EDGE_LOOP ( 'NONE', ( #5322, #67100 ) ) ;
#8163=DIRECTION ( 'NONE',  ( -0.000000000000000000, 0.9848077530122085754, -0.1736481776669273613 ) ) ;
#8164=CARTESIAN_POINT ( 'NONE',  ( -15.90379184220783948, -12.17597550085003633, 31.52189283813461884 ) ) ;
#8166=CARTESIAN_POINT ( 'NONE',  ( 14.05769230769230838, -2.249999999999998668, 29.75000000000000355 ) ) ;
#8167=DIRECTION ( 'NONE',  ( -0.000000000000000000, -0.3420201433256694901, -0.9396926207859082059 ) ) ;
#8168=EDGE_CURVE ( 'NONE', #15450, #38452, #9915, .T. ) ;
#8169=VERTEX_POINT ( 'NONE', #45682 ) ;
#8170=B_SPLINE_CURVE_WITH_KNOTS ( 'NONE', 3,
 ( #11241, #36182, #72938, #2363, #49241, #42934, #79703, #1500, #70403, #29425 ),
 .UNSPECIFIED., .F., .F.,
 ( 4, 2, 2, 2, 4 ),
 ( 0.000000000000000000, 0.0001954311564186866034, 0.0003908623128373732067, 0.0005862934692560597830, 0.0007817246256747464135 ),
 .UNSPECIFIED. ) ;
#8171=CARTESIAN_POINT ( 'NONE',  ( -12.21148414990014963, -9.148310452688876993, 34.47095581063188519 ) ) ;
#8172=B_SPLINE_CURVE_WITH_KNOTS ( 'NONE', 3,
 ( #12413, #41219, #88106, #34007, #32245, #75443, #54269, #88538, #33578, #11978 ),
 .UNSPECIFIED., .F., .F.,
 ( 4, 2, 2, 2, 4 ),
 ( 0.0007817246256747460882, 0.0009771112852218900684, 0.001172497944769033832, 0.001367884604316177595, 0.001563271263863321575 ),
 .UNSPECIFIED. ) ;
#8173=AXIS2_PLACEMENT_3D ( 'NONE', #81816, #21432, #76372 ) ;
#8174=CARTESIAN_POINT ( 'NONE',  ( -0.6850233861027921201, -10.23692288466677880, 34.23039457007281072 ) ) ;
#8175=CARTESIAN_POINT ( 'NONE',  ( -13.25408994638174320, -12.70449254468099198, 30.44128974285582956 ) ) ;
#8176=VERTEX_POINT ( 'NONE', #88044 ) ;
#8177=ADVANCED_FACE ( 'NONE', ( #59194 ), #47451, .F. ) ;
#8178=CARTESIAN_POINT ( 'NONE',  ( 9.692307692307695177, -12.09954503811598769, 35.62045528018868623 ) ) ;
#8179=VERTEX_POINT ( 'NONE', #32178 ) ;
#8180=CARTESIAN_POINT ( 'NONE',  ( -2.531177251416256713, -12.24155766932282496, 31.33739205006857986 ) ) ;
#8181=CARTESIAN_POINT ( 'NONE',  ( 6.223426961861570739, -7.630147231320743018, 34.74852402298682819 ) ) ;
#8182=ORIENTED_EDGE ( 'NONE', *, *, #44950, .F. ) ;
#8184=CARTESIAN_POINT ( 'NONE',  ( -8.992715712954716167, -2.599994579823203367, 30.74605699353653776 ) ) ;
#8185=CARTESIAN_POINT ( 'NONE',  ( 1.161130440891438687, -4.386631170607604879, 33.66268669641500111 ) ) ;
#8186=EDGE_CURVE ( 'NONE', #57379, #66205, #17295, .T. ) ;
#8187=DIRECTION ( 'NONE',  ( -0.000000000000000000, -0.9848077530122085754, -0.1736481776669273613 ) ) ;
#8188=FACE_OUTER_BOUND ( 'NONE', #73969, .T. ) ;
#8189=ORIENTED_EDGE ( 'NONE', *, *, #22291, .F. ) ;
#8191=FACE_BOUND ( 'NONE', #53229, .T. ) ;
#8192=ORIENTED_EDGE ( 'NONE', *, *, #73661, .T. ) ;
#8195=ADVANCED_FACE ( 'NONE', ( #59640 ), #87140, .F. ) ;
#8197=EDGE_CURVE ( 'NONE', #28285, #14918, #42045, .T. ) ;
#8198=CYLINDRICAL_SURFACE ( 'NONE', #73733, 0.2500000000000004996 ) ;
#8200=VERTEX_POINT ( 'NONE', #83479 ) ;
#8201=B_SPLINE_CURVE_WITH_KNOTS ( 'NONE', 3,
 ( #65850, #10482, #65414, #72616, #3706, #59098 ),
 .UNSPECIFIED., .F., .F.,
 ( 4, 2, 4 ),
 ( 0.000000000000000000, 0.0001954784845028911366, 0.0003909569690057822732 ),
 .UNSPECIFIED. ) ;
#8202=ORIENTED_EDGE ( 'NONE', *, *, #70714, .F. ) ;
#8203=ORIENTED_EDGE ( 'NONE', *, *, #34977, .F. ) ;
#8204=CARTESIAN_POINT ( 'NONE',  ( -0.2385271099256131566, -3.105924265160262543, 32.13625925475356127 ) ) ;
#8205=B_SPLINE_CURVE_WITH_KNOTS ( 'NONE', 3,
 ( #7858, #81749, #35320, #62776, #28577, #13726, #74993, #41200, #13281, #33991 ),
 .UNSPECIFIED., .F., .F.,
 ( 4, 2, 2, 2, 4 ),
 ( 0.0007817246336856291692, 0.0009771112958940103739, 0.001172497958102391470, 0.001367884620310772566, 0.001563271282519153879 ),
 .UNSPECIFIED. ) ;
#8206=VERTEX_POINT ( 'NONE', #27190 ) ;
#8207=EDGE_CURVE ( 'NONE', #42366, #55800, #54648, .T. ) ;
#8208=CARTESIAN_POINT ( 'NONE',  ( -14.30769230769242739, -3.300289026999228881, 32.46337939537708905 ) ) ;
#8209=CARTESIAN_POINT ( 'NONE',  ( 1.384615384615264011, -6.835583212225970762, 34.95778746994575670 ) ) ;
#8210=CARTESIAN_POINT ( 'NONE',  ( 13.38461538461538680, -11.35647404775217417, 33.31231777344666511 ) ) ;
#8211=DIRECTION ( 'NONE',  ( 0.000000000000000000, 0.4999999999999960032, -0.8660254037844410391 ) ) ;
#8212=CARTESIAN_POINT ( 'NONE',  ( -6.130690603110307002, -6.369640206132550553, 34.87707690430378449 ) ) ;
#8213=AXIS2_PLACEMENT_3D ( 'NONE', #11952, #39867, #60563 ) ;
#8214=LINE ( 'NONE', #28942, #15016 ) ;
#8215=CARTESIAN_POINT ( 'NONE',  ( -11.66860874789975888, -3.285722584762969856, 32.44110544564090759 ) ) ;
#8217=ORIENTED_EDGE ( 'NONE', *, *, #86095, .F. ) ;
#8220=CARTESIAN_POINT ( 'NONE',  ( -4.023320452082591814, -10.19071101563364756, 33.96452234770658407 ) ) ;
#8222=CARTESIAN_POINT ( 'NONE',  ( 10.36540787133602670, -2.318417181685855422, 30.59732222474233865 ) ) ;
#8223=CARTESIAN_POINT ( 'NONE',  ( 1.607628228708780860, -12.38742843783360748, 31.66772728687926985 ) ) ;
#8224=CARTESIAN_POINT ( 'NONE',  ( 12.46153846153833911, -12.70778746994576025, 30.41441678777401236 ) ) ;
#8225=ADVANCED_FACE ( 'NONE', ( #55102 ), #68618, .F. ) ;
#8226=FACE_BOUND ( 'NONE', #38844, .T. ) ;
#8227=CARTESIAN_POINT ( 'NONE',  ( 7.912222197156282277, -11.16473453929635440, 33.15142922261926373 ) ) ;
#8228=EDGE_CURVE ( 'NONE', #2251, #54993, #60207, .T. ) ;
#8229=VERTEX_POINT ( 'NONE', #48786 ) ;
#8231=VECTOR ( 'NONE', #32857, 1000.000000000000227 ) ;
#8233=CARTESIAN_POINT ( 'NONE',  ( -17.29984929443922681, -11.76352882383564769, 32.36236540154569497 ) ) ;
#8234=CYLINDRICAL_SURFACE ( 'NONE', #28050, 0.2499999999999995559 ) ;
#8235=VERTEX_POINT ( 'NONE', #76711 ) ;
#8236=CARTESIAN_POINT ( 'NONE',  ( 2.530471848960718084, -11.89424750095246175, 32.13594075562311758 ) ) ;
#8237=EDGE_CURVE ( 'NONE', #81196, #16341, #66022, .T. ) ;
#8238=ORIENTED_EDGE ( 'NONE', *, *, #52947, .F. ) ;
#8239=FACE_BOUND ( 'NONE', #70342, .T. ) ;
#8241=B_SPLINE_CURVE_WITH_KNOTS ( 'NONE', 3,
 ( #35410, #62863, #28664, #61993, #76398, #56129, #55236, #77282, #70531, #83165 ),
 .UNSPECIFIED., .F., .F.,
 ( 4, 2, 2, 2, 4 ),
 ( 0.000000000000000000, 0.0001954339881912772715, 0.0003908679763825545429, 0.0005863019645738318415, 0.0007817359527651090859 ),
 .UNSPECIFIED. ) ;
#8242=B_SPLINE_CURVE_WITH_KNOTS ( 'NONE', 3,
 ( #83127, #48433, #1146, #21860, #75919, #29082, #22306, #56970, #84464, #50200 ),
 .UNSPECIFIED., .F., .F.,
 ( 4, 2, 2, 2, 4 ),
 ( 0.000000000000000000, 0.0001954339857564097241, 0.0003908679715128194482, 0.0005863019572692291723, 0.0007817359430256388964 ),
 .UNSPECIFIED. ) ;
#8243=CARTESIAN_POINT ( 'NONE',  ( 4.219101293358989757, -2.657715359629131857, 31.77849191805844242 ) ) ;
#8244=CARTESIAN_POINT ( 'NONE',  ( -2.980823712421088789, -8.433404298154334455, 34.66254593164985920 ) ) ;
#8245=B_SPLINE_CURVE_WITH_KNOTS ( 'NONE', 3,
 ( #11022, #88048, #46580, #4257, #53327, #32618, #18226, #4712, #38949, #60086 ),
 .UNSPECIFIED., .F., .F.,
 ( 4, 2, 2, 2, 4 ),
 ( 0.0007817246256747459798, 0.0009771112852218896347, 0.001172497944769033398, 0.001367884604316177161, 0.001563271263863320708 ),
 .UNSPECIFIED. ) ;
#8246=EDGE_LOOP ( 'NONE', ( #16076, #72558 ) ) ;
#8247=CARTESIAN_POINT ( 'NONE',  ( 0.3308469948709041319, -10.54014554554150607, 33.71984207302941883 ) ) ;
#8248=CARTESIAN_POINT ( 'NONE',  ( -18.00000000000012079, -4.320704448113953156, 33.92786785259630022 ) ) ;
#8249=CARTESIAN_POINT ( 'NONE',  ( 8.639082799499073317, -2.373036134822904319, 30.88089517874952250 ) ) ;
#8250=CARTESIAN_POINT ( 'NONE',  ( -6.923076923077044142, -10.90142922262034020, 33.41473453929536674 ) ) ;
#8251=ORIENTED_EDGE ( 'NONE', *, *, #43621, .T. ) ;
#8253=ORIENTED_EDGE ( 'NONE', *, *, #42719, .T. ) ;
#8254=CARTESIAN_POINT ( 'NONE',  ( -8.835314180186649935, -3.513871655860377086, 32.76840700105978499 ) ) ;
#8255=VERTEX_POINT ( 'NONE', #47901 ) ;
#8256=CARTESIAN_POINT ( 'NONE',  ( -8.519230769229334754, -7.500000000000155431, 34.75000000000007105 ) ) ;
#8258=CARTESIAN_POINT ( 'NONE',  ( 7.716005876422150855, -10.31621877034669588, 34.18098118002070152 ) ) ;
#8259=B_SPLINE_CURVE_WITH_KNOTS ( 'NONE', 3,
 ( #52005, #24539, #79500, #44803, #24988, #17801, #30850, #79940, #37610, #58321 ),
 .UNSPECIFIED., .F., .F.,
 ( 4, 2, 2, 2, 4 ),
 ( 0.0007817246256747465219, 0.0009771112852218900684, 0.001172497944769033615, 0.001367884604316177378, 0.001563271263863320925 ),
 .UNSPECIFIED. ) ;
#8261=CARTESIAN_POINT ( 'NONE',  ( -12.21159294319032362, -2.824170634883621744, 31.52227843825338738 ) ) ;
#8262=CARTESIAN_POINT ( 'NONE',  ( 8.834423757525421195, -2.255955759149236073, 29.99999999999988631 ) ) ;
#8263=CARTESIAN_POINT ( 'NONE',  ( 2.307692307692309264, -10.05456864172156806, 36.03766855953608683 ) ) ;
#8264=CARTESIAN_POINT ( 'NONE',  ( 7.846153846153725020, -4.481592998941358097, 33.73612834414048933 ) ) ;
#8268=CARTESIAN_POINT ( 'NONE',  ( -16.40386937806761125, -4.931416488878823223, 34.32920672191015399 ) ) ;
#8269=ORIENTED_EDGE ( 'NONE', *, *, #79918, .F. ) ;
#8270=ORIENTED_EDGE ( 'NONE', *, *, #15736, .T. ) ;
#8271=CARTESIAN_POINT ( 'NONE',  ( -15.93083330975275658, -6.460100341425561332, 34.89618726649961644 ) ) ;
#8272=VECTOR ( 'NONE', #71064, 1000.000000000000114 ) ;
#8273=ORIENTED_EDGE ( 'NONE', *, *, #29370, .T. ) ;
#8274=CARTESIAN_POINT ( 'NONE',  ( 10.83816428436267820, -8.540255544307065350, 34.89611431652622286 ) ) ;
#8275=CARTESIAN_POINT ( 'NONE',  ( 2.980792499826876440, -8.303909089506435137, 34.68538101551103381 ) ) ;
#8276=CARTESIAN_POINT ( 'NONE',  ( -11.76194648218548267, -11.41268669641500466, 32.86336882939237825 ) ) ;
#8278=CARTESIAN_POINT ( 'NONE',  ( 13.38461538461526423, -2.657715359629662544, 31.77849191805970364 ) ) ;
#8279=CARTESIAN_POINT ( 'NONE',  ( 6.988332494352946789, -11.48612834413965977, 32.76840700105972815 ) ) ;
#8280=CARTESIAN_POINT ( 'NONE',  ( 13.38461538461538680, -8.318370150425687726, 35.83090037661290239 ) ) ;
#8281=CARTESIAN_POINT ( 'NONE',  ( 10.48523740594639442, -2.619462340734462380, 30.83744416345203021 ) ) ;
#8282=CARTESIAN_POINT ( 'NONE',  ( 15.10007862765892206, -9.084618155246140248, 34.75535874321725771 ) ) ;
#8283=B_SPLINE_CURVE_WITH_KNOTS ( 'NONE', 3,
 ( #7280, #26661, #5512, #47818, #41067, #67654, #68528, #33857, #61315, #61762 ),
 .UNSPECIFIED., .F., .F.,
 ( 4, 2, 2, 2, 4 ),
 ( 0.000000000000000000, 0.0001954311564186860613, 0.0003908623128373721225, 0.0005862934692560581567, 0.0007817246256747442451 ),
 .UNSPECIFIED. ) ;
#8284=CARTESIAN_POINT ( 'NONE',  ( 14.55769230769231370, -2.499999999999999556, 29.81604066197449754 ) ) ;
#8286=B_SPLINE_CURVE_WITH_KNOTS ( 'NONE', 3,
 ( #62281, #36597, #21748, #57305, #15000, #50096, #75802, #64055, #42920, #42033 ),
 .UNSPECIFIED., .F., .F.,
 ( 4, 2, 2, 2, 4 ),
 ( 0.0007817359430256320659, 0.0009771253907249987086, 0.001172514838424365460, 0.001367904286123731994, 0.001563293733823098745 ),
 .UNSPECIFIED. ) ;
#8288=VERTEX_POINT ( 'NONE', #82596 ) ;
#8289=VECTOR ( 'NONE', #30906, 1000.000000000000000 ) ;
#8290=CARTESIAN_POINT ( 'NONE',  ( -15.23076923076935074, -8.613356846316285953, 34.62446782046622218 ) ) ;
#8291=DIRECTION ( 'NONE',  ( 0.000000000000000000, 1.000000000000000000, 0.000000000000000000 ) ) ;
#8292=CARTESIAN_POINT ( 'NONE',  ( -2.980823712421089233, -2.824170634883621744, 31.52227843825338738 ) ) ;
#8293=CARTESIAN_POINT ( 'NONE',  ( 0.2380535369741302587, -10.23692288466677702, 34.23039457007281072 ) ) ;
#8294=ORIENTED_EDGE ( 'NONE', *, *, #87040, .F. ) ;
#8295=CARTESIAN_POINT ( 'NONE',  ( 6.000000000000001776, -4.786620604624113540, 33.94971097300155094 ) ) ;
#8296=CARTESIAN_POINT ( 'NONE',  ( -17.32692307692307665, -2.499999999999998668, 29.75000000000000355 ) ) ;
#8297=CARTESIAN_POINT ( 'NONE',  ( -3.099977422944442562, -12.11778462344221019, 31.66786338562085135 ) ) ;
#8300=CARTESIAN_POINT ( 'NONE',  ( 18.22277966897806678, -3.563462043263029955, 33.22394488606062879 ) ) ;
#8301=ORIENTED_EDGE ( 'NONE', *, *, #50058, .F. ) ;
#8303=EDGE_CURVE ( 'NONE', #83509, #60361, #27989, .T. ) ;
#8304=DIRECTION ( 'NONE',  ( -0.000000000000000000, -0.9848077530122085754, -0.1736481776669273613 ) ) ;
#8305=CARTESIAN_POINT ( 'NONE',  ( -6.130691466667558487, -2.541943142973490666, 30.39792223712631980 ) ) ;
#8306=CARTESIAN_POINT ( 'NONE',  ( -14.24162395668986747, -11.69971097300155272, 32.46337939537588113 ) ) ;
#8307=CARTESIAN_POINT ( 'NONE',  ( 18.13052543823364360, -8.630441415882549094, 34.87705825610312615 ) ) ;
#8308=ORIENTED_EDGE ( 'NONE', *, *, #46456, .T. ) ;
#8311=ORIENTED_EDGE ( 'NONE', *, *, #27265, .F. ) ;
#8313=EDGE_CURVE ( 'NONE', #861, #60596, #7809, .T. ) ;
#8314=CARTESIAN_POINT ( 'NONE',  ( -6.066083410955878996, -11.16473453929635440, 33.15142922261925662 ) ) ;
#8315=FACE_OUTER_BOUND ( 'NONE', #87004, .T. ) ;
#8316=CIRCLE ( 'NONE', #19827, 0.2500000000000002220 ) ;
#8317=DIRECTION ( 'NONE',  ( -0.000000000000000000, 0.5000000000000011102, -0.8660254037844381525 ) ) ;
#8318=CARTESIAN_POINT ( 'NONE',  ( 16.94677510719138169, -10.31621877034669588, 34.18098118002070152 ) ) ;
#8319=CARTESIAN_POINT ( 'NONE',  ( 4.284637961670941131, -6.413143153341454017, 34.63066358083362672 ) ) ;
#8321=AXIS2_PLACEMENT_3D ( 'NONE', #88622, #48477, #42629 ) ;
#8322=ORIENTED_EDGE ( 'NONE', *, *, #33933, .F. ) ;
#8323=ORIENTED_EDGE ( 'NONE', *, *, #7372, .F. ) ;
#8324=VERTEX_POINT ( 'NONE', #25254 ) ;
#8325=CARTESIAN_POINT ( 'NONE',  ( -3.007757879156381264, -10.61302985866383963, 33.66295027996417843 ) ) ;
#8327=CARTESIAN_POINT ( 'NONE',  ( -13.38461538461538325, -13.75783147151868846, 33.36296068462461051 ) ) ;
#8328=CARTESIAN_POINT ( 'NONE',  ( 14.55774672760575861, -4.818054556918156983, 34.26375889529406749 ) ) ;
#8329=CYLINDRICAL_SURFACE ( 'NONE', #46013, 0.2499999999999973355 ) ;
#8331=CARTESIAN_POINT ( 'NONE',  ( 13.44987095589141113, -8.613356846314928816, 34.62446782046653482 ) ) ;
#8332=EDGE_CURVE ( 'NONE', #79011, #30706, #44066, .T. ) ;
#8333=VERTEX_POINT ( 'NONE', #26590 ) ;
#8334=ORIENTED_EDGE ( 'NONE', *, *, #78010, .F. ) ;
#8335=CARTESIAN_POINT ( 'NONE',  ( 4.023155550735844521, -3.957541250942359756, 33.62499894934981626 ) ) ;
#8337=FACE_BOUND ( 'NONE', #40593, .T. ) ;
#8338=DIRECTION ( 'NONE',  ( 0.000000000000000000, 0.3420201433256610524, 0.9396926207859113145 ) ) ;
#8339=CARTESIAN_POINT ( 'NONE',  ( 8.096208266067300485, -5.642605341092957971, 34.66089969410670335 ) ) ;
#8340=ORIENTED_EDGE ( 'NONE', *, *, #46518, .F. ) ;
#8341=CARTESIAN_POINT ( 'NONE',  ( 14.98076923076923173, -7.500000000000001776, 35.00000000000000000 ) ) ;
#8342=CARTESIAN_POINT ( 'NONE',  ( 11.31497661389720832, -6.716662450894489211, 34.94144148231605840 ) ) ;
#8343=DIRECTION ( 'NONE',  ( -0.000000000000000000, -0.5000000000000009992, -0.8660254037844380415 ) ) ;
#8344=EDGE_CURVE ( 'NONE', #18328, #37947, #19376, .T. ) ;
#8345=CARTESIAN_POINT ( 'NONE',  ( 0.6845498131513110263, -6.503523203565942268, 34.64991518177335195 ) ) ;
#8347=ORIENTED_EDGE ( 'NONE', *, *, #67920, .F. ) ;
#8348=VECTOR ( 'NONE', #20433, 1000.000000000000227 ) ;
#8349=CARTESIAN_POINT ( 'NONE',  ( 11.78851585009985570, -3.136992222400443175, 32.19305428654138979 ) ) ;
#8350=CARTESIAN_POINT ( 'NONE',  ( 3.480823542407545546, -4.235687564193446164, 33.53795663066793509 ) ) ;
#8351=CARTESIAN_POINT ( 'NONE',  ( 16.28437185560972011, -9.417988943895561960, 34.36773134775778260 ) ) ;
#8353=CARTESIAN_POINT ( 'NONE',  ( -5.999999999999998224, -1.129524287112498415, 32.06866353760679544 ) ) ;
#8354=FACE_BOUND ( 'NONE', #52019, .T. ) ;
#8355=CARTESIAN_POINT ( 'NONE',  ( -6.673131513698879580, -12.68172785388650681, 30.59649109432439573 ) ) ;
#8356=CARTESIAN_POINT ( 'NONE',  ( -8.769230769230892619, -9.528491918059723176, 34.59228464037033035 ) ) ;
#8358=LINE ( 'NONE', #1597, #19494 ) ;
#8359=CARTESIAN_POINT ( 'NONE',  ( -3.296039231325550212, -3.083524468853724443, 32.58852847137143272 ) ) ;
#8360=CARTESIAN_POINT ( 'NONE',  ( -18.24997674404859183, -2.920706130388549759, 32.31842814019191223 ) ) ;
#8361=FACE_OUTER_BOUND ( 'NONE', #59475, .T. ) ;
#8365=VERTEX_POINT ( 'NONE', #81544 ) ;
#8366=CARTESIAN_POINT ( 'NONE',  ( -11.53846153846166089, -12.51329471203414379, 31.30864560766407578 ) ) ;
#8368=CARTESIAN_POINT ( 'NONE',  ( -11.31545018684869142, -2.758310577978207778, 31.33698337089302299 ) ) ;
#8369=CARTESIAN_POINT ( 'NONE',  ( -18.25002323729296450, -2.587272538249755005, 30.68239716806877837 ) ) ;
#8370=B_SPLINE_CURVE_WITH_KNOTS ( 'NONE', 3,
 ( #70701, #9006, #22071, #63491, #29281, #62599, #55407, #36473, #49544, #36036 ),
 .UNSPECIFIED., .F., .F.,
 ( 4, 2, 2, 2, 4 ),
 ( 0.0007817359430256339090, 0.0009771253907250065148, 0.001172514838424371965, 0.001367904286123737632, 0.001563293733823103299 ),
 .UNSPECIFIED. ) ;
#8371=ORIENTED_EDGE ( 'NONE', *, *, #47317, .F. ) ;
#8372=CARTESIAN_POINT ( 'NONE',  ( -18.13069146666755671, -12.38065189839062263, 30.83690757178629482 ) ) ;
#8374=LINE ( 'NONE', #35847, #5572 ) ;
#8375=CARTESIAN_POINT ( 'NONE',  ( -15.29603923132555110, -9.528491918058357157, 34.59228464037090589 ) ) ;
#8376=CARTESIAN_POINT ( 'NONE',  ( 16.15384615384615330, -8.164416787775445883, 34.95778746994557906 ) ) ;
#8377=B_SPLINE_CURVE_WITH_KNOTS ( 'NONE', 3,
 ( #42321, #56264, #1315, #2628, #16593, #78294, #84636, #62565, #8526, #2193 ),
 .UNSPECIFIED., .F., .F.,
 ( 4, 2, 2, 2, 4 ),
 ( 0.000000000000000000, 0.0001954339857564078809, 0.0003908679715128157619, 0.0005863019572692236428, 0.0007817359430256315238 ),
 .UNSPECIFIED. ) ;
#8378=CARTESIAN_POINT ( 'NONE',  ( -3.007393744996809115, -2.251407671071270489, 29.88021292934942252 ) ) ;
#8379=CYLINDRICAL_SURFACE ( 'NONE', #12784, 0.2499999999999993616 ) ;
#8380=DIRECTION ( 'NONE',  ( -0.000000000000000000, -0.9848077530122086864, -0.1736481776669273613 ) ) ;
#8382=CARTESIAN_POINT ( 'NONE',  ( -18.25002322422145440, -11.56360843649121861, 33.07473185843129926 ) ) ;
#8383=DIRECTION ( 'NONE',  ( 0.000000000000000000, 0.7660444431189807890, 0.6427876096865361433 ) ) ;
#8387=CARTESIAN_POINT ( 'NONE',  ( -14.08468095607945791, -10.61302985866383963, 33.66295027996417843 ) ) ;
#8388=VERTEX_POINT ( 'NONE', #52716 ) ;
#8389=CYLINDRICAL_SURFACE ( 'NONE', #71603, 0.2499999999999995559 ) ;
#8391=CARTESIAN_POINT ( 'NONE',  ( 1.384615384615386802, -12.37446782046654192, 30.86335684631486131 ) ) ;
#8392=CARTESIAN_POINT ( 'NONE',  ( -5.142193522883852452, -6.026961402152685388, 34.52809138561120506 ) ) ;
#8394=EDGE_CURVE ( 'NONE', #22482, #72792, #40560, .T. ) ;
#8395=DIRECTION ( 'NONE',  ( -0.000000000000000000, 1.000000000000000000, 3.491481338843133355E-15 ) ) ;
#8396=CARTESIAN_POINT ( 'NONE',  ( -5.999999999999998224, -2.499999999999998668, 29.50000000000001066 ) ) ;
#8397=ORIENTED_EDGE ( 'NONE', *, *, #50545, .F. ) ;
#8398=ORIENTED_EDGE ( 'NONE', *, *, #41539, .T. ) ;
#8400=ORIENTED_EDGE ( 'NONE', *, *, #57473, .T. ) ;
#8404=CARTESIAN_POINT ( 'NONE',  ( -6.792285115252135519, -4.118422570099827595, 33.43335022499816489 ) ) ;
#8405=CARTESIAN_POINT ( 'NONE',  ( -15.36091720050093024, -11.04286588640298561, 33.62463336215343901 ) ) ;
#8406=B_SPLINE_CURVE_WITH_KNOTS ( 'NONE', 3,
 ( #43838, #71303, #70881, #56906, #77187, #50591, #43402, #76750, #49711, #64537 ),
 .UNSPECIFIED., .F., .F.,
 ( 4, 2, 2, 2, 4 ),
 ( 0.0007817359527651104954, 0.0009771254036996493593, 0.001172514854634188223, 0.001367904305568727087, 0.001563293756503265951 ),
 .UNSPECIFIED. ) ;
#8407=EDGE_CURVE ( 'NONE', #52040, #82649, #35476, .T. ) ;
#8409=CARTESIAN_POINT ( 'NONE',  ( 13.13459216039393240, -8.475808217655753651, 34.90892951860618609 ) ) ;
#8410=VECTOR ( 'NONE', #6850, 999.9999999999998863 ) ;
#8412=CYLINDRICAL_SURFACE ( 'NONE', #56421, 0.2500000000000004996 ) ;
#8413=ORIENTED_EDGE ( 'NONE', *, *, #63582, .T. ) ;
#8414=ORIENTED_EDGE ( 'NONE', *, *, #84070, .T. ) ;
#8416=EDGE_CURVE ( 'NONE', #64954, #4054, #50629, .T. ) ;
#8417=ORIENTED_EDGE ( 'NONE', *, *, #57440, .T. ) ;
#8418=CARTESIAN_POINT ( 'NONE',  ( -15.48079246806219800, -12.22074536777954989, 31.39888409691088356 ) ) ;
#8419=ORIENTED_EDGE ( 'NONE', *, *, #89077, .T. ) ;
#8420=DIRECTION ( 'NONE',  ( -0.000000000000000000, -0.8660254037844397068, -0.4999999999999978906 ) ) ;
#8422=ADVANCED_FACE ( 'NONE', ( #66232 ), #32454, .F. ) ;
#8423=CARTESIAN_POINT ( 'NONE',  ( -9.942284423250047354, -8.303909089506435137, 34.68538101551103381 ) ) ;
#8424=VERTEX_POINT ( 'NONE', #12192 ) ;
#8425=ORIENTED_EDGE ( 'NONE', *, *, #37773, .F. ) ;
#8426=EDGE_LOOP ( 'NONE', ( #32679, #30335, #71228, #4033 ) ) ;
#8427=CARTESIAN_POINT ( 'NONE',  ( 14.30769230769231015, -8.810774026931790459, 35.74407628777942847 ) ) ;
#8428=CARTESIAN_POINT ( 'NONE',  ( 10.61538461538461675, -1.629998284177014645, 34.34916445242399163 ) ) ;
#8429=VERTEX_POINT ( 'NONE', #39677 ) ;
#8430=CARTESIAN_POINT ( 'NONE',  ( 1.515407192440174189, -8.999086150933472084, 34.52020707165672064 ) ) ;
#8431=CARTESIAN_POINT ( 'NONE',  ( 6.923076923076800782, -12.51329471203414379, 31.30864560766407578 ) ) ;
#8432=CARTESIAN_POINT ( 'NONE',  ( -2.980823712421090121, -10.05730279482229683, 34.04704008940765902 ) ) ;
#8433=EDGE_CURVE ( 'NONE', #70653, #80357, #5438, .T. ) ;
#8435=EDGE_CURVE ( 'NONE', #126, #24282, #23499, .T. ) ;
#8436=B_SPLINE_CURVE_WITH_KNOTS ( 'NONE', 3,
 ( #87229, #25508, #80461, #30915, #46222, #73709, #58384, #51617, #79117, #17420 ),
 .UNSPECIFIED., .F., .F.,
 ( 4, 2, 2, 2, 4 ),
 ( 0.000000000000000000, 0.0001954311564186866305, 0.0003908623128373732609, 0.0005862934692560598914, 0.0007817246256747465219 ),
 .UNSPECIFIED. ) ;
#8437=CARTESIAN_POINT ( 'NONE',  ( 14.98079249982687777, -10.66389620160130036, 33.62221079203477103 ) ) ;
#8438=CYLINDRICAL_SURFACE ( 'NONE', #52605, 0.2499999999999979738 ) ;
#8439=VECTOR ( 'NONE', #57628, 1000.000000000000114 ) ;
#8440=ORIENTED_EDGE ( 'NONE', *, *, #32237, .T. ) ;
#8441=FACE_BOUND ( 'NONE', #74790, .T. ) ;
#8442=B_SPLINE_CURVE_WITH_KNOTS ( 'NONE', 3,
 ( #86612, #24882, #52798, #11830, #46045, #52350, #80288, #73533, #39308, #66764 ),
 .UNSPECIFIED., .F., .F.,
 ( 4, 2, 2, 2, 4 ),
 ( 0.000000000000000000, 0.0001954311564186872810, 0.0003908623128373745620, 0.0005862934692560618430, 0.0007817246256747491240 ),
 .UNSPECIFIED. ) ;
#8444=CARTESIAN_POINT ( 'NONE',  ( -18.22348492456433178, -12.47654668319379567, 31.42292124445336654 ) ) ;
#8445=CARTESIAN_POINT ( 'NONE',  ( 9.692307692307695177, -1.466349020453238561, 30.81389545987213907 ) ) ;
#8446=CARTESIAN_POINT ( 'NONE',  ( -7.846153846153844924, -10.89733346790207413, 36.13435417666054406 ) ) ;
#8447=DIRECTION ( 'NONE',  ( -0.000000000000000000, -0.5000000000000009992, -0.8660254037844380415 ) ) ;
#8448=EDGE_CURVE ( 'NONE', #85898, #17034, #44200, .T. ) ;
#8449=CARTESIAN_POINT ( 'NONE',  ( -5.010854725920639297, -10.51840700105979565, 33.73612834413962247 ) ) ;
#8450=CARTESIAN_POINT ( 'NONE',  ( -4.219116154402473562, -11.06231777344662781, 33.60647404775220082 ) ) ;
#8451=ORIENTED_EDGE ( 'NONE', *, *, #49791, .F. ) ;
#8452=EDGE_CURVE ( 'NONE', #78712, #49139, #81755, .T. ) ;
#8453=CARTESIAN_POINT ( 'NONE',  ( 14.53070365930516239, -12.39991518177334129, 30.74647679643404530 ) ) ;
#8454=CARTESIAN_POINT ( 'NONE',  ( -17.07692307692307665, -6.343179335718451384, 34.87096338111211935 ) ) ;
#8455=B_SPLINE_CURVE_WITH_KNOTS ( 'NONE', 3,
 ( #69731, #9798, #23307, #1717, #1265, #16118, #84592, #28755, #49015, #21990 ),
 .UNSPECIFIED., .F., .F.,
 ( 4, 2, 2, 2, 4 ),
 ( 0.000000000000000000, 0.0001954311564186861697, 0.0003908623128373723394, 0.0005862934692560584820, 0.0007817246256747446788 ),
 .UNSPECIFIED. ) ;
#8456=EDGE_LOOP ( 'NONE', ( #33582, #63134 ) ) ;
#8458=CARTESIAN_POINT ( 'NONE',  ( -14.08467946359890988, -9.172514111537584114, 34.72667873470787470 ) ) ;
#8459=CARTESIAN_POINT ( 'NONE',  ( -3.903900635498010807, -2.587454068350147462, 30.68340429815432202 ) ) ;
#8460=CARTESIAN_POINT ( 'NONE',  ( -5.207614543590634248, -11.71456829005830080, 32.44064028649416542 ) ) ;
#8461=CARTESIAN_POINT ( 'NONE',  ( 8.068933515131908152, -6.717445702608402236, 34.94155399931962336 ) ) ;
#8462=DIRECTION ( 'NONE',  ( 0.000000000000000000, -6.938893903907222067E-15, 1.000000000000000000 ) ) ;
#8463=FACE_BOUND ( 'NONE', #4284, .T. ) ;
#8464=CARTESIAN_POINT ( 'NONE',  ( -1.449885385171703289, -6.835583212224499938, 34.95778746994557906 ) ) ;
#8466=CYLINDRICAL_SURFACE ( 'NONE', #33842, 0.2500000000000009437 ) ;
#8468=CARTESIAN_POINT ( 'NONE',  ( -14.30769230769230660, -2.708943851104267164, 35.45975837776705220 ) ) ;
#8471=ORIENTED_EDGE ( 'NONE', *, *, #47507, .T. ) ;
#8472=EDGE_LOOP ( 'NONE', ( #68867, #48581 ) ) ;
#8473=AXIS2_PLACEMENT_3D ( 'NONE', #57213, #23847, #44120 ) ;
#8474=CARTESIAN_POINT ( 'NONE',  ( 5.207714884747862705, -6.413143153341454017, 34.63066358083362672 ) ) ;
#8475=CARTESIAN_POINT ( 'NONE',  ( -12.23875879256039489, -6.717445702608402236, 34.94155399931962336 ) ) ;
#8476=CARTESIAN_POINT ( 'NONE',  ( 16.28463659481310799, -2.845873456487966635, 32.17976146951972538 ) ) ;
#8477=CYLINDRICAL_SURFACE ( 'NONE', #3581, 0.2500000000000009437 ) ;
#8478=CARTESIAN_POINT ( 'NONE',  ( -16.21911659980693088, -12.27809138561121394, 31.22303859784730307 ) ) ;
#8480=B_SPLINE_CURVE_WITH_KNOTS ( 'NONE', 3,
 ( #1008, #77549, #14971, #21718, #23047, #9105, #2757, #63137, #15416, #70802 ),
 .UNSPECIFIED., .F., .F.,
 ( 4, 2, 2, 2, 4 ),
 ( 0.0007817246256747434861, 0.0009771112852218859484, 0.001172497944769028411, 0.001367884604316171090, 0.001563271263863313552 ),
 .UNSPECIFIED. ) ;
#8481=CARTESIAN_POINT ( 'NONE',  ( 0.5923289025054119250, -3.957578996910242619, 33.62503395064540257 ) ) ;
#8482=LINE ( 'NONE', #49463, #40282 ) ;
#8483=AXIS2_PLACEMENT_3D ( 'NONE', #74554, #32670, #53831 ) ;
#8484=CARTESIAN_POINT ( 'NONE',  ( -17.20707028636129721, -5.195881422630167279, 34.18770438780618548 ) ) ;
#8485=CARTESIAN_POINT ( 'NONE',  ( -3.164701897419154530, -11.91647553114624358, 32.58852847137148245 ) ) ;
#8487=CARTESIAN_POINT ( 'NONE',  ( -5.011667937410237528, -6.835583212224609184, 34.95778746994559327 ) ) ;
#8488=EDGE_CURVE ( 'NONE', #36228, #86632, #43341, .T. ) ;
#8489=CARTESIAN_POINT ( 'NONE',  ( 14.30769230769231015, -11.69971097300155272, 32.46337939537588113 ) ) ;
#8490=LINE ( 'NONE', #35961, #70098 ) ;
#8491=ORIENTED_EDGE ( 'NONE', *, *, #40453, .T. ) ;
#8493=CARTESIAN_POINT ( 'NONE',  ( 10.68063975489745232, -5.941354392334607049, 34.76329471203374055 ) ) ;
#8496=CARTESIAN_POINT ( 'NONE',  ( -2.373774687052441656, -4.661471528628506888, 34.16647553114621871 ) ) ;
#8498=ORIENTED_EDGE ( 'NONE', *, *, #86823, .F. ) ;
#8499=CARTESIAN_POINT ( 'NONE',  ( -9.822998295418001291, -5.496505350115501010, 34.60290016733514307 ) ) ;
#8500=CARTESIAN_POINT ( 'NONE',  ( 3.903822916553187028, -5.851115903089112003, 34.47074536777953568 ) ) ;
#8501=EDGE_LOOP ( 'NONE', ( #39216, #29158, #58541, #53017 ) ) ;
#8503=CARTESIAN_POINT ( 'NONE',  ( 17.01084069756293715, -2.486705287966279432, 31.30864560766543647 ) ) ;
#8504=EDGE_LOOP ( 'NONE', ( #88100, #11085, #12876, #83969 ) ) ;
#8505=CYLINDRICAL_SURFACE ( 'NONE', #21831, 0.2499999999999998890 ) ;
#8506=EDGE_CURVE ( 'NONE', #56881, #50988, #8523, .T. ) ;
#8507=CARTESIAN_POINT ( 'NONE',  ( 10.83816428436268176, -10.97394488606064122, 33.68653795673694873 ) ) ;
#8508=ORIENTED_EDGE ( 'NONE', *, *, #21935, .T. ) ;
#8509=DIRECTION ( 'NONE',  ( 0.000000000000000000, 0.9396926207859126468, -0.3420201433256571111 ) ) ;
#8510=CARTESIAN_POINT ( 'NONE',  ( -11.76194646302587010, -12.47654668319379567, 31.42292124445336654 ) ) ;
#8511=CARTESIAN_POINT ( 'NONE',  ( 12.46153846153846168, -11.91647553114624181, 32.58852847137148245 ) ) ;
#8512=ORIENTED_EDGE ( 'NONE', *, *, #14215, .F. ) ;
#8513=ORIENTED_EDGE ( 'NONE', *, *, #63450, .F. ) ;
#8514=CARTESIAN_POINT ( 'NONE',  ( 15.29602480204525605, -10.90142922261932057, 33.41473453929631887 ) ) ;
#8515=VECTOR ( 'NONE', #30273, 1000.000000000000227 ) ;
#8516=ORIENTED_EDGE ( 'NONE', *, *, #84912, .T. ) ;
#8517=EDGE_CURVE ( 'NONE', #32626, #65460, #36154, .T. ) ;
#8518=FACE_OUTER_BOUND ( 'NONE', #75318, .T. ) ;
#8519=CARTESIAN_POINT ( 'NONE',  ( -15.36091720050093024, -2.373036134822904319, 30.88089517874952250 ) ) ;
#8521=DIRECTION ( 'NONE',  ( -0.000000000000000000, -0.9848077530122086864, -0.1736481776669273613 ) ) ;
#8522=CARTESIAN_POINT ( 'NONE',  ( -17.20761454359063691, -6.413092428213692742, 34.63065189839063152 ) ) ;
#8523=B_SPLINE_CURVE_WITH_KNOTS ( 'NONE', 3,
 ( #69923, #37457, #85219, #29830, #30704, #29397, #57292, #50955, #56846, #64473 ),
 .UNSPECIFIED., .F., .F.,
 ( 4, 2, 2, 2, 4 ),
 ( 0.0007817359430256294638, 0.0009771253907249952391, 0.001172514838424361123, 0.001367904286123726790, 0.001563293733823092673 ),
 .UNSPECIFIED. ) ;
#8524=EDGE_LOOP ( 'NONE', ( #36740, #25811 ) ) ;
#8525=EDGE_LOOP ( 'NONE', ( #32011, #9530, #20385, #1505, #19589, #71220 ) ) ;
#8526=CARTESIAN_POINT ( 'NONE',  ( 9.627037246346919375, -4.481592998940162609, 33.73612834413957984 ) ) ;
#8527=EDGE_LOOP ( 'NONE', ( #38016, #40563 ) ) ;
#8528=CARTESIAN_POINT ( 'NONE',  ( 16.40384615384615685, -2.499999999999999556, 29.81604066197449754 ) ) ;
#8529=VERTEX_POINT ( 'NONE', #84342 ) ;
#8530=AXIS2_PLACEMENT_3D ( 'NONE', #3670, #57739, #72580 ) ;
#8531=VECTOR ( 'NONE', #83529, 1000.000000000000000 ) ;
#8532=DIRECTION ( 'NONE',  ( 0.000000000000000000, 0.8660254037844377084, -0.5000000000000015543 ) ) ;
#8533=CARTESIAN_POINT ( 'NONE',  ( 7.976945653978634532, -4.809403383903225304, 33.96459661697924304 ) ) ;
#8534=ORIENTED_EDGE ( 'NONE', *, *, #89064, .T. ) ;
#8535=DIRECTION ( 'NONE',  ( 0.000000000000000000, 1.000000000000000000, 0.000000000000000000 ) ) ;
#8536=B_SPLINE_CURVE_WITH_KNOTS ( 'NONE', 3,
 ( #39794, #67261, #60935, #5558, #88438, #33031, #88009, #26270, #53736, #81223 ),
 .UNSPECIFIED., .F., .F.,
 ( 4, 2, 2, 2, 4 ),
 ( 0.000000000000000000, 0.0001954339857564100222, 0.0003908679715128200445, 0.0005863019572692300396, 0.0007817359430256400890 ),
 .UNSPECIFIED. ) ;
#8538=B_SPLINE_CURVE_WITH_KNOTS ( 'NONE', 3,
 ( #37299, #85500, #78287, #25125, #52589, #11622, #23779, #44049, #39101, #10284 ),
 .UNSPECIFIED., .F., .F.,
 ( 4, 2, 2, 2, 4 ),
 ( 0.0007817359430256322827, 0.0009771253907249989254, 0.001172514838424365676, 0.001367904286123732428, 0.001563293733823098962 ),
 .UNSPECIFIED. ) ;
#8539=ORIENTED_EDGE ( 'NONE', *, *, #78866, .F. ) ;
#8540=DIRECTION ( 'NONE',  ( 1.000000000000000000, 0.000000000000000000, 0.000000000000000000 ) ) ;
#8542=CARTESIAN_POINT ( 'NONE',  ( -0.5276218724943410043, -10.51840700105979387, 33.73612834413961536 ) ) ;
#8544=EDGE_CURVE ( 'NONE', #64424, #47910, #33245, .T. ) ;
#8545=ORIENTED_EDGE ( 'NONE', *, *, #44605, .T. ) ;
#8546=CARTESIAN_POINT ( 'NONE',  ( 15.16468685140909045, -2.292212530054419606, 30.41441678777542634 ) ) ;
#8547=CARTESIAN_POINT ( 'NONE',  ( 6.856994543716788293, -5.471508081941601986, 34.59228464037088457 ) ) ;
#8548=FACE_BOUND ( 'NONE', #77843, .T. ) ;
#8549=CARTESIAN_POINT ( 'NONE',  ( 1.607394925883794068, -12.44528174975671853, 30.48912976160716681 ) ) ;
#8551=ADVANCED_FACE ( 'NONE', ( #51388 ), #9123, .F. ) ;
#8552=CARTESIAN_POINT ( 'NONE',  ( 4.376857505459002873, -12.39991518177334129, 30.74647679643404530 ) ) ;
#8553=CARTESIAN_POINT ( 'NONE',  ( 16.15384615384603251, -4.320704448113951379, 33.92786785259630022 ) ) ;
#8555=DIRECTION ( 'NONE',  ( 0.000000000000000000, 0.8660254037844377084, 0.5000000000000015543 ) ) ;
#8556=ORIENTED_EDGE ( 'NONE', *, *, #33561, .T. ) ;
#8557=EDGE_CURVE ( 'NONE', #61557, #84346, #84786, .T. ) ;
#8558=LINE ( 'NONE', #27493, #67628 ) ;
#8559=ORIENTED_EDGE ( 'NONE', *, *, #41284, .F. ) ;
#8561=CYLINDRICAL_SURFACE ( 'NONE', #54737, 0.2499999999999994726 ) ;
#8562=FACE_OUTER_BOUND ( 'NONE', #3608, .T. ) ;
#8563=CARTESIAN_POINT ( 'NONE',  ( -9.692307692307691624, -2.833524468853757305, 32.15551576947925838 ) ) ;
#8564=CARTESIAN_POINT ( 'NONE',  ( 7.846153846153723244, -3.643525952248796163, 33.31231777344771672 ) ) ;
#8565=CARTESIAN_POINT ( 'NONE',  ( 17.07692307692295586, -10.33852847137269571, 34.16647553114546554 ) ) ;
#8566=CARTESIAN_POINT ( 'NONE',  ( 14.43848274865926129, -11.37503395064541678, 33.29242100308974273 ) ) ;
#8567=ORIENTED_EDGE ( 'NONE', *, *, #84000, .T. ) ;
#8568=CARTESIAN_POINT ( 'NONE',  ( 13.38461538461538680, -4.786620604624113540, 33.94971097300155094 ) ) ;
#8569=CARTESIAN_POINT ( 'NONE',  ( -6.000000000000119904, -6.879047030192662504, 34.71129190930017927 ) ) ;
#8571=CARTESIAN_POINT ( 'NONE',  ( 3.164685819813350509, -3.050289026998445951, 32.03036669348365706 ) ) ;
#8572=CARTESIAN_POINT ( 'NONE',  ( 2.557746727605761716, -5.642605341092957083, 34.66089969410670335 ) ) ;
#8574=B_SPLINE_CURVE_WITH_KNOTS ( 'NONE', 3,
 ( #16512, #7994, #56619, #70578, #43979, #9327, #2111, #22823, #15198, #29596 ),
 .UNSPECIFIED., .F., .F.,
 ( 4, 2, 2, 2, 4 ),
 ( 0.000000000000000000, 0.0001954311564186861426, 0.0003908623128373722852, 0.0005862934692560583735, 0.0007817246256747445703 ),
 .UNSPECIFIED. ) ;
#8575=AXIS2_PLACEMENT_3D ( 'NONE', #78910, #3248, #22634 ) ;
#8576=CARTESIAN_POINT ( 'NONE',  ( 2.980746006547773774, -12.07920672191015221, 32.31858351112116168 ) ) ;
#8577=EDGE_LOOP ( 'NONE', ( #42958, #40337 ) ) ;
#8578=ORIENTED_EDGE ( 'NONE', *, *, #83886, .T. ) ;
#8579=B_SPLINE_CURVE_WITH_KNOTS ( 'NONE', 3,
 ( #51207, #9808, #45361, #64295, #16127, #65188 ),
 .UNSPECIFIED., .F., .F.,
 ( 4, 2, 4 ),
 ( 4.220987180333913997E-17, 0.0001954756301637146886, 0.0003909512603273872016 ),
 .UNSPECIFIED. ) ;
#8581=EDGE_CURVE ( 'NONE', #50385, #67353, #51561, .T. ) ;
#8582=ORIENTED_EDGE ( 'NONE', *, *, #71164, .F. ) ;
#8583=DIRECTION ( 'NONE',  ( -0.000000000000000000, 0.9396926207859093161, -0.3420201433256663259 ) ) ;
#8584=CARTESIAN_POINT ( 'NONE',  ( 3.230769230769231726, -13.63283147151868846, 33.57946703557072254 ) ) ;
#8585=DIRECTION ( 'NONE',  ( -0.000000000000000000, 0.1736481776669307198, -0.9848077530122080203 ) ) ;
#8586=LINE ( 'NONE', #88473, #6861 ) ;
#8587=CARTESIAN_POINT ( 'NONE',  ( -17.07692307692307665, -12.10708131394839349, 31.69288490824020244 ) ) ;
#8588=FACE_OUTER_BOUND ( 'NONE', #45657, .T. ) ;
#8589=ORIENTED_EDGE ( 'NONE', *, *, #83067, .F. ) ;
#8591=CARTESIAN_POINT ( 'NONE',  ( 17.86944008638663206, -2.254533558242299396, 29.97296025877827930 ) ) ;
#8592=ORIENTED_EDGE ( 'NONE', *, *, #80126, .F. ) ;
#8593=CARTESIAN_POINT ( 'NONE',  ( -10.36543909703647159, -3.712312575010499049, 33.01462480002815170 ) ) ;
#8594=CARTESIAN_POINT ( 'NONE',  ( -17.30040800148741198, -12.11044203135681840, 32.26167407432752299 ) ) ;
#8595=CARTESIAN_POINT ( 'NONE',  ( 11.53846153846153832, -4.098570777380720287, 33.41473453929634729 ) ) ;
#8596=EDGE_CURVE ( 'NONE', #59070, #70481, #15068, .T. ) ;
#8597=CARTESIAN_POINT ( 'NONE',  ( 0.5923302693632450655, -2.729792928343270031, 31.24908615093345432 ) ) ;
#8600=ORIENTED_EDGE ( 'NONE', *, *, #89007, .F. ) ;
#8601=EDGE_CURVE ( 'NONE', #37486, #45648, #89096, .T. ) ;
#8602=CARTESIAN_POINT ( 'NONE',  ( -15.29603923132555110, -6.835583212224499938, 34.95778746994557906 ) ) ;
#8603=B_SPLINE_CURVE_WITH_KNOTS ( 'NONE', 3,
 ( #50127, #15919, #43382, #29873, #78048, #59103, #16785, #38396, #31642, #50995 ),
 .UNSPECIFIED., .F., .F.,
 ( 4, 2, 2, 2, 4 ),
 ( 0.0007817246256747463051, 0.0009771112852218896347, 0.001172497944769033181, 0.001367884604316176728, 0.001563271263863320057 ),
 .UNSPECIFIED. ) ;
#8604=CARTESIAN_POINT ( 'NONE',  ( -17.32694630114453105, -4.931416488878823223, 34.32920672191015399 ) ) ;
#8607=VECTOR ( 'NONE', #16720, 1000.000000000000227 ) ;
#8608=DIRECTION ( 'NONE',  ( -0.000000000000000000, -0.8660254037844397068, -0.4999999999999978906 ) ) ;
#8609=FACE_OUTER_BOUND ( 'NONE', #14018, .T. ) ;
#8610=ORIENTED_EDGE ( 'NONE', *, *, #19797, .T. ) ;
#8611=FACE_OUTER_BOUND ( 'NONE', #22313, .T. ) ;
#8612=CARTESIAN_POINT ( 'NONE',  ( -3.230769230769351186, -10.90142922262034020, 33.41473453929536674 ) ) ;
#8615=CIRCLE ( 'NONE', #58922, 0.2500000000000002220 ) ;
#8617=EDGE_CURVE ( 'NONE', #8229, #63457, #68932, .T. ) ;
#8618=CARTESIAN_POINT ( 'NONE',  ( 9.561698037103610659, -7.722926974430166069, 34.99546784045485737 ) ) ;
#8619=EDGE_LOOP ( 'NONE', ( #50496, #73110, #74874, #30023 ) ) ;
#8621=CARTESIAN_POINT ( 'NONE',  ( 2.307692307692309264, -8.564572088678739092, 35.78748833219616898 ) ) ;
#8622=EDGE_CURVE ( 'NONE', #51137, #53485, #81594, .T. ) ;
#8624=FACE_OUTER_BOUND ( 'NONE', #85714, .T. ) ;
#8625=ORIENTED_EDGE ( 'NONE', *, *, #81418, .T. ) ;
#8627=ORIENTED_EDGE ( 'NONE', *, *, #8118, .F. ) ;
#8628=CARTESIAN_POINT ( 'NONE',  ( -17.77698715590659972, -11.98016756924215187, 32.48728574198910479 ) ) ;
#8629=CARTESIAN_POINT ( 'NONE',  ( -10.74553182482283198, -2.882441371585227508, 31.66841991370172238 ) ) ;
#8630=ORIENTED_EDGE ( 'NONE', *, *, #49330, .T. ) ;
#8631=DIRECTION ( 'NONE',  ( 0.000000000000000000, 0.6427876096865373645, -0.7660444431189797898 ) ) ;
#8632=CYLINDRICAL_SURFACE ( 'NONE', #42167, 0.2499999999999994726 ) ;
#8634=CARTESIAN_POINT ( 'NONE',  ( 3.230769230769231726, -8.318370150425687726, 35.83090037661290239 ) ) ;
#8637=CARTESIAN_POINT ( 'NONE',  ( -4.088591014333315066, -4.320704448112861584, 33.92786785259548310 ) ) ;
#8638=ORIENTED_EDGE ( 'NONE', *, *, #63673, .F. ) ;
#8639=EDGE_LOOP ( 'NONE', ( #56017, #6297, #72657, #28269 ) ) ;
#8640=FACE_BOUND ( 'NONE', #8162, .T. ) ;
#8641=VERTEX_POINT ( 'NONE', #3671 ) ;
#8642=CARTESIAN_POINT ( 'NONE',  ( 15.48082354240754555, -2.564540009722896752, 30.55348353981670684 ) ) ;
#8643=CYLINDRICAL_SURFACE ( 'NONE', #78982, 2.000000000000001776 ) ;
#8644=CARTESIAN_POINT ( 'NONE',  ( 9.469381474791543241, -12.15238873228292071, 31.58232369045353849 ) ) ;
#8645=CARTESIAN_POINT ( 'NONE',  ( -2.057637887778853703, -10.06805714834173848, 34.32951233291982618 ) ) ;
#8646=B_SPLINE_CURVE_WITH_KNOTS ( 'NONE', 3,
 ( #45565, #72146, #31616, #64940, #78023, #71700, #10460, #85673, #37928, #4129 ),
 .UNSPECIFIED., .F., .F.,
 ( 4, 2, 2, 2, 4 ),
 ( 0.0007817246256747478229, 0.0009771112852218911526, 0.001172497944769034482, 0.001367884604316177595, 0.001563271263863320925 ),
 .UNSPECIFIED. ) ;
#8647=EDGE_LOOP ( 'NONE', ( #46101, #6106, #1807, #44948, #17020, #65251 ) ) ;
#8648=ORIENTED_EDGE ( 'NONE', *, *, #33223, .F. ) ;
#8650=CARTESIAN_POINT ( 'NONE',  ( -0.2387589202700509394, -3.236590943229497697, 32.36255958852954251 ) ) ;
#8652=FACE_OUTER_BOUND ( 'NONE', #76883, .T. ) ;
#8653=CARTESIAN_POINT ( 'NONE',  ( -12.21153846153846168, -2.249999999999998668, 29.75000000000000355 ) ) ;
#8654=CARTESIAN_POINT ( 'NONE',  ( -18.06608341095587633, -11.16473453929635440, 33.15142922261927083 ) ) ;
#8655=ORIENTED_EDGE ( 'NONE', *, *, #28948, .F. ) ;
#8656=CARTESIAN_POINT ( 'NONE',  ( 13.31934493865461278, -10.90142922261923886, 33.41473453929638993 ) ) ;
#8657=EDGE_CURVE ( 'NONE', #47954, #22613, #37532, .T. ) ;
#8658=VECTOR ( 'NONE', #20222, 1000.000000000000227 ) ;
#8659=AXIS2_PLACEMENT_3D ( 'NONE', #54172, #81667, #19948 ) ;
#8660=FACE_OUTER_BOUND ( 'NONE', #64758, .T. ) ;
#8661=LINE ( 'NONE', #1453, #30804 ) ;
#8662=CARTESIAN_POINT ( 'NONE',  ( 8.835298102580843249, -6.343179335718452272, 34.87096338111212646 ) ) ;
#8663=ORIENTED_EDGE ( 'NONE', *, *, #79002, .T. ) ;
#8664=EDGE_CURVE ( 'NONE', #48302, #1690, #67706, .T. ) ;
#8665=ORIENTED_EDGE ( 'NONE', *, *, #78746, .T. ) ;
#8667=AXIS2_PLACEMENT_3D ( 'NONE', #53950, #5773, #26489 ) ;
#8668=FACE_OUTER_BOUND ( 'NONE', #77864, .T. ) ;
#8669=FACE_OUTER_BOUND ( 'NONE', #86734, .T. ) ;
#8671=EDGE_CURVE ( 'NONE', #23103, #60060, #5328, .T. ) ;
#8673=CARTESIAN_POINT ( 'NONE',  ( -8.899378738962466784, -6.809168938359901446, 34.95455904226513866 ) ) ;
#8674=FACE_BOUND ( 'NONE', #49397, .T. ) ;
#8675=CARTESIAN_POINT ( 'NONE',  ( 8.096208157792160520, -11.28795663066794575, 33.01431243580653785 ) ) ;
#8676=VERTEX_POINT ( 'NONE', #27509 ) ;
#8677=CARTESIAN_POINT ( 'NONE',  ( -3.007757879156381264, -2.554770724473667709, 30.48948780036025852 ) ) ;
#8678=FACE_OUTER_BOUND ( 'NONE', #33432, .T. ) ;
#8679=CARTESIAN_POINT ( 'NONE',  ( 11.31563484598253311, -7.369208160676172348, 34.74850200257122879 ) ) ;
#8680=CARTESIAN_POINT ( 'NONE',  ( 4.153846153846154188, -6.435427911321262684, 35.78748833219616898 ) ) ;
#8681=ORIENTED_EDGE ( 'NONE', *, *, #19206, .T. ) ;
#8682=EDGE_CURVE ( 'NONE', #38328, #45741, #22900, .T. ) ;
#8683=CARTESIAN_POINT ( 'NONE',  ( -18.00000000000000000, -8.120952969808772792, 34.71129190930000163 ) ) ;
#8685=FACE_BOUND ( 'NONE', #31543, .T. ) ;
#8686=CARTESIAN_POINT ( 'NONE',  ( -17.01166750564705055, -4.481592998940251427, 33.73612834413965089 ) ) ;
#8687=ADVANCED_FACE ( 'NONE', ( #61720 ), #41027, .F. ) ;
#8688=FACE_OUTER_BOUND ( 'NONE', #49817, .T. ) ;
#8689=CARTESIAN_POINT ( 'NONE',  ( 12.23861224402230619, -12.15238873228292071, 31.58232369045353849 ) ) ;
#8690=ORIENTED_EDGE ( 'NONE', *, *, #35351, .F. ) ;
#8692=CARTESIAN_POINT ( 'NONE',  ( -14.43838377435986864, -4.118384482072085184, 33.43331474514187107 ) ) ;
#8693=LINE ( 'NONE', #63619, #55274 ) ;
#8694=CARTESIAN_POINT ( 'NONE',  ( -7.053224132515142131, -10.88202310037935661, 33.43294751532457099 ) ) ;
#8695=ORIENTED_EDGE ( 'NONE', *, *, #70896, .F. ) ;
#8696=CARTESIAN_POINT ( 'NONE',  ( -9.822455662039393687, -3.069018819979302926, 32.56621877034667278 ) ) ;
#8697=EDGE_LOOP ( 'NONE', ( #6053, #69356 ) ) ;
#8698=DIRECTION ( 'NONE',  ( 1.000000000000000000, 0.000000000000000000, 0.000000000000000000 ) ) ;
#8699=EDGE_LOOP ( 'NONE', ( #52953, #19507 ) ) ;
#8700=CARTESIAN_POINT ( 'NONE',  ( 11.78851585009985214, -6.567000820036036579, 34.66262288849541306 ) ) ;
#8701=CARTESIAN_POINT ( 'NONE',  ( -10.86536134632696715, -12.41269422305637171, 30.68257228309993323 ) ) ;
#8702=CARTESIAN_POINT ( 'NONE',  ( 7.780071466793709867, -9.905515769479276145, 34.41647553114623292 ) ) ;
#8703=CARTESIAN_POINT ( 'NONE',  ( -3.931066612577741370, -12.44528174975671853, 30.48912976160716681 ) ) ;
#8704=CARTESIAN_POINT ( 'NONE',  ( -3.164701897419155863, -3.937682226553329556, 33.60647404775216529 ) ) ;
#8705=CYLINDRICAL_SURFACE ( 'NONE', #20163, 0.2499999999999986955 ) ;
#8707=VECTOR ( 'NONE', #71940, 1000.000000000000000 ) ;
#8709=VERTEX_POINT ( 'NONE', #13547 ) ;
#8710=ADVANCED_FACE ( 'NONE', ( #74818 ), #20745, .F. ) ;
#8711=FACE_OUTER_BOUND ( 'NONE', #83800, .T. ) ;
#8712=CARTESIAN_POINT ( 'NONE',  ( 13.63461538461544897, -7.434744860731433924, 35.00000000000000711 ) ) ;
#8713=ORIENTED_EDGE ( 'NONE', *, *, #9611, .T. ) ;
#8714=ORIENTED_EDGE ( 'NONE', *, *, #3500, .T. ) ;
#8716=CARTESIAN_POINT ( 'NONE',  ( 10.86543903529806876, -8.346898887586323923, 34.93166121998716278 ) ) ;
#8717=B_SPLINE_CURVE_WITH_KNOTS ( 'NONE', 3,
 ( #77506, #70756, #72073, #30641, #44141, #63977, #2275, #29770, #85595, #57237 ),
 .UNSPECIFIED., .F., .F.,
 ( 4, 2, 2, 2, 4 ),
 ( 0.000000000000000000, 0.0001954339857564075286, 0.0003908679715128150572, 0.0005863019572692225586, 0.0007817359430256301143 ),
 .UNSPECIFIED. ) ;
#8718=B_SPLINE_CURVE_WITH_KNOTS ( 'NONE', 3,
 ( #2637, #58034, #42331, #8097, #30128, #35568, #49522, #76995, #70232, #43202 ),
 .UNSPECIFIED., .F., .F.,
 ( 4, 2, 2, 2, 4 ),
 ( 0.0007817359430256315238, 0.0009771253907249980580, 0.001172514838424364592, 0.001367904286123730910, 0.001563293733823097444 ),
 .UNSPECIFIED. ) ;
#8721=DIRECTION ( 'NONE',  ( 0.000000000000000000, 0.9848077530122072432, 0.1736481776669354937 ) ) ;
#8722=CARTESIAN_POINT ( 'NONE',  ( 8.639083559792547717, -11.47017969459903952, 32.78971311882035167 ) ) ;
#8723=EDGE_CURVE ( 'NONE', #21125, #29522, #6451, .T. ) ;
#8724=CARTESIAN_POINT ( 'NONE',  ( -9.019253993452222673, -2.985938066672154445, 32.43141759479405550 ) ) ;
#8725=FACE_OUTER_BOUND ( 'NONE', #14849, .T. ) ;
#8726=CARTESIAN_POINT ( 'NONE',  ( 3.007843013253084230, -6.503392248772476236, 34.64988816332204635 ) ) ;
#8727=CARTESIAN_POINT ( 'NONE',  ( 14.98079248672064345, -9.234221910056348293, 34.70572697212741531 ) ) ;
#8728=EDGE_CURVE ( 'NONE', #35073, #12236, #66588, .T. ) ;
#8731=CARTESIAN_POINT ( 'NONE',  ( -1.384615384615069056, -2.255955759149395501, 30.00000000000324363 ) ) ;
#8732=CARTESIAN_POINT ( 'NONE',  ( 3.230769230769231726, -6.189225973068211317, 35.74407628777942847 ) ) ;
#8734=ORIENTED_EDGE ( 'NONE', *, *, #59573, .T. ) ;
#8735=CARTESIAN_POINT ( 'NONE',  ( 0.6845498131513112483, -9.086983370893047862, 34.49168942202179267 ) ) ;
#8736=CARTESIAN_POINT ( 'NONE',  ( -15.93047066807373469, -2.251407671071268712, 29.88021292934942963 ) ) ;
#8738=CARTESIAN_POINT ( 'NONE',  ( -2.241523166729649574, -7.250054483168843156, 34.74374881642865631 ) ) ;
#8739=ORIENTED_EDGE ( 'NONE', *, *, #39774, .F. ) ;
#8740=VECTOR ( 'NONE', #33630, 999.9999999999998863 ) ;
#8742=EDGE_CURVE ( 'NONE', #3690, #3961, #20333, .T. ) ;
#8743=CARTESIAN_POINT ( 'NONE',  ( 4.153846153846030731, -3.643525952248796163, 33.31231777344771672 ) ) ;
#8744=CARTESIAN_POINT ( 'NONE',  ( 8.769230769230647482, -4.481592998941358097, 33.73612834414048933 ) ) ;
#8745=EDGE_CURVE ( 'NONE', #15980, #19105, #75256, .T. ) ;
#8748=CARTESIAN_POINT ( 'NONE',  ( 4.153846153846154188, -13.88283147151868846, 33.14645433367849847 ) ) ;
#8749=EDGE_LOOP ( 'NONE', ( #50171, #88542, #74373, #14419 ) ) ;
#8752=LINE ( 'NONE', #64993, #88838 ) ;
#8753=CARTESIAN_POINT ( 'NONE',  ( 12.23805351781451201, -8.496056993536548418, 34.65000542017679663 ) ) ;
#8754=DIRECTION ( 'NONE',  ( -0.000000000000000000, 0.8660254037844397068, -0.4999999999999978906 ) ) ;
#8755=CARTESIAN_POINT ( 'NONE',  ( 18.06606733335007675, -8.164416787775445883, 34.95778746994558617 ) ) ;
#8756=B_SPLINE_CURVE_WITH_KNOTS ( 'NONE', 3,
 ( #73156, #38937, #66394, #59634, #52870, #80369, #18666, #46128, #11907, #39384 ),
 .UNSPECIFIED., .F., .F.,
 ( 4, 2, 2, 2, 4 ),
 ( 0.0007817359430256384627, 0.0009771253907250067317, 0.001172514838424375001, 0.001367904286123743270, 0.001563293733823111539 ),
 .UNSPECIFIED. ) ;
#8757=VERTEX_POINT ( 'NONE', #71140 ) ;
#8758=ORIENTED_EDGE ( 'NONE', *, *, #66269, .T. ) ;
#8759=ORIENTED_EDGE ( 'NONE', *, *, #47438, .T. ) ;
#8760=CARTESIAN_POINT ( 'NONE',  ( -3.480769230769229061, -2.249999999999998668, 29.75000000000000355 ) ) ;
#8761=CARTESIAN_POINT ( 'NONE',  ( -12.52680846209478460, -12.70778746994557551, 30.41441678777548319 ) ) ;
#8762=VECTOR ( 'NONE', #73268, 1000.000000000000000 ) ;
#8763=CARTESIAN_POINT ( 'NONE',  ( -3.230769230769351186, -10.21337939537710326, 33.94971097300076224 ) ) ;
#8764=EDGE_CURVE ( 'NONE', #68166, #63712, #36910, .T. ) ;
#8765=CARTESIAN_POINT ( 'NONE',  ( 0.3308478584281538404, -12.35290016733513951, 31.75349464988449455 ) ) ;
#8766=DIRECTION ( 'NONE',  ( -0.000000000000000000, -0.8660254037844397068, -0.4999999999999978906 ) ) ;
#8769=ORIENTED_EDGE ( 'NONE', *, *, #77727, .F. ) ;
#8771=CARTESIAN_POINT ( 'NONE',  ( -3.165513659493205623, -10.90142922261932057, 33.41473453929631887 ) ) ;
#8772=ORIENTED_EDGE ( 'NONE', *, *, #56400, .T. ) ;
#8773=CARTESIAN_POINT ( 'NONE',  ( 8.769230769230647482, -8.613356846316285953, 34.62446782046622218 ) ) ;
#8774=CARTESIAN_POINT ( 'NONE',  ( 13.63456079399342791, -4.176053281294518804, 33.81426240980091791 ) ) ;
#8776=ORIENTED_EDGE ( 'NONE', *, *, #75153, .F. ) ;
#8777=B_SPLINE_CURVE_WITH_KNOTS ( 'NONE', 3,
 ( #69581, #50634, #63265, #77666, #76337, #41675, #42128, #15979, #21842, #70918 ),
 .UNSPECIFIED., .F., .F.,
 ( 4, 2, 2, 2, 4 ),
 ( 0.0007817246256747473893, 0.0009771112852218902852, 0.001172497944769033181, 0.001367884604316176294, 0.001563271263863319190 ),
 .UNSPECIFIED. ) ;
#8778=VECTOR ( 'NONE', #44002, 1000.000000000000114 ) ;
#8780=DIRECTION ( 'NONE',  ( -0.000000000000000000, -0.8660254037844399289, -0.4999999999999980016 ) ) ;
#8781=ORIENTED_EDGE ( 'NONE', *, *, #40063, .F. ) ;
#8782=FACE_BOUND ( 'NONE', #6865, .T. ) ;
#8783=CARTESIAN_POINT ( 'NONE',  ( -5.869474561766359066, -3.068774925481847937, 32.56582465632704526 ) ) ;
#8786=DIRECTION ( 'NONE',  ( -0.000000000000000000, 0.5000000000000011102, -0.8660254037844380415 ) ) ;
#8788=CARTESIAN_POINT ( 'NONE',  ( -4.284406745588072774, -2.504760397472873823, 29.97295953869789997 ) ) ;
#8789=CARTESIAN_POINT ( 'NONE',  ( 5.010840697562939816, -8.164416787775445883, 34.95778746994557906 ) ) ;
#8790=CARTESIAN_POINT ( 'NONE',  ( 9.692307692307695177, -11.69971097300155272, 32.46337939537588113 ) ) ;
#8792=CARTESIAN_POINT ( 'NONE',  ( -13.13466986626723987, -11.86320923018887541, 32.19269448109604781 ) ) ;
#8794=EDGE_CURVE ( 'NONE', #51157, #84431, #83839, .T. ) ;
#8795=DIRECTION ( 'NONE',  ( -0.000000000000000000, -0.6427876096865404731, -0.7660444431189770143 ) ) ;
#8796=CARTESIAN_POINT ( 'NONE',  ( -7.976844449264150150, -11.93127051446799847, 32.56575433478202797 ) ) ;
#8797=CARTESIAN_POINT ( 'NONE',  ( -5.076923076923075762, -11.16473453929635440, 33.15142922261926373 ) ) ;
#8798=CARTESIAN_POINT ( 'NONE',  ( -0.4615384615385840772, -5.094484230521993062, 34.41647553114689373 ) ) ;
#8799=CARTESIAN_POINT ( 'NONE',  ( -6.923076923076922462, -2.486705287966279876, 31.30864560766543647 ) ) ;
#8800=CARTESIAN_POINT ( 'NONE',  ( 8.835298102580843249, -3.937682226553329556, 33.60647404775216529 ) ) ;
#8801=CARTESIAN_POINT ( 'NONE',  ( 4.946231610255518163, -11.18331474514187995, 33.13161551792790505 ) ) ;
#8802=CARTESIAN_POINT ( 'NONE',  ( 2.307692307692187583, -10.21337939537710326, 33.94971097300076224 ) ) ;
#8803=CARTESIAN_POINT ( 'NONE',  ( 1.515407192440174189, -11.18335022499818621, 33.13157742990016885 ) ) ;
#8804=CARTESIAN_POINT ( 'NONE',  ( 3.903869409797562806, -5.643011162660950042, 34.66104346484419096 ) ) ;
#8805=CARTESIAN_POINT ( 'NONE',  ( 8.769230769230647482, -2.892918686052165622, 31.69288490824153470 ) ) ;
#8806=CARTESIAN_POINT ( 'NONE',  ( -2.373774687052442545, -5.471508081941601986, 34.59228464037088457 ) ) ;
#8808=VERTEX_POINT ( 'NONE', #2233 ) ;
#8810=ORIENTED_EDGE ( 'NONE', *, *, #81121, .T. ) ;
#8812=VERTEX_POINT ( 'NONE', #16204 ) ;
#8814=CARTESIAN_POINT ( 'NONE',  ( 0.4615384615384611755, -4.102666532097928531, 36.13435417666054406 ) ) ;
#8815=CARTESIAN_POINT ( 'NONE',  ( -3.454254174493179619, -3.236172620538810385, 32.36188796281390267 ) ) ;
#8816=VERTEX_POINT ( 'NONE', #71578 ) ;
#8817=DIRECTION ( 'NONE',  ( 0.000000000000000000, 0.3420201433256641055, -0.9396926207859100932 ) ) ;
#8819=CARTESIAN_POINT ( 'NONE',  ( 17.14217864819909920, -8.613356846314930593, 34.62446782046653482 ) ) ;
#8820=CARTESIAN_POINT ( 'NONE',  ( 13.51540582558234149, -2.845873456487966635, 32.17976146951972538 ) ) ;
#8821=B_SPLINE_CURVE_WITH_KNOTS ( 'NONE', 3,
 ( #22612, #64033, #37006, #86103, #29826, #43774, #58610, #58166, #51383, #10441 ),
 .UNSPECIFIED., .F., .F.,
 ( 4, 2, 2, 2, 4 ),
 ( 0.000000000000000000, 0.0001954311564186858715, 0.0003908623128373717431, 0.0005862934692560576146, 0.0007817246256747434861 ),
 .UNSPECIFIED. ) ;
#8822=CARTESIAN_POINT ( 'NONE',  ( -5.300408020647024543, -5.113361153441932316, 34.14387501736621999 ) ) ;
#8823=CARTESIAN_POINT ( 'NONE',  ( -16.28399412357784826, -10.31621877034669588, 34.18098118002070152 ) ) ;
#8824=LINE ( 'NONE', #21886, #25776 ) ;
#8825=LINE ( 'NONE', #36297, #831 ) ;
#8826=B_SPLINE_CURVE_WITH_KNOTS ( 'NONE', 3,
 ( #20052, #61469, #41658, #21377, #6978, #13296, #27250, #34453, #61912, #8763 ),
 .UNSPECIFIED., .F., .F.,
 ( 4, 2, 2, 2, 4 ),
 ( 0.000000000000000000, 0.0001954339857564090465, 0.0003908679715128180929, 0.0005863019572692271123, 0.0007817359430256361858 ),
 .UNSPECIFIED. ) ;
#8827=AXIS2_PLACEMENT_3D ( 'NONE', #10945, #31660, #42193 ) ;
#8829=CARTESIAN_POINT ( 'NONE',  ( 11.53846153846153832, -5.471508081941601098, 34.59228464037088457 ) ) ;
#8830=DIRECTION ( 'NONE',  ( -0.000000000000000000, 0.3420201433256694346, -0.9396926207859080948 ) ) ;
#8832=VECTOR ( 'NONE', #10813, 1000.000000000000227 ) ;
#8836=ORIENTED_EDGE ( 'NONE', *, *, #87240, .T. ) ;
#8837=CARTESIAN_POINT ( 'NONE',  ( 1.607628228708781526, -8.282913670948747864, 34.94150082978203642 ) ) ;
#8838=CARTESIAN_POINT ( 'NONE',  ( 11.76124107972994537, -5.913360116392397892, 34.49180327182771322 ) ) ;
#8839=DIRECTION ( 'NONE',  ( 0.000000000000000000, 0.7660444431189822323, -0.6427876096865344779 ) ) ;
#8841=CARTESIAN_POINT ( 'NONE',  ( -16.40382288478850725, -10.66389620160130036, 33.62221079203477103 ) ) ;
#8842=CARTESIAN_POINT ( 'NONE',  ( 9.562160482869471068, -11.47017969459903952, 32.78971311882035167 ) ) ;
#8843=CARTESIAN_POINT ( 'NONE',  ( 8.639083559792549494, -10.88202310037935661, 33.43294751532457099 ) ) ;
#8845=EDGE_CURVE ( 'NONE', #37947, #18328, #69773, .T. ) ;
#8846=VECTOR ( 'NONE', #54547, 1000.000000000000000 ) ;
#8847=VERTEX_POINT ( 'NONE', #85113 ) ;
#8848=VERTEX_POINT ( 'NONE', #83796 ) ;
#8849=ORIENTED_EDGE ( 'NONE', *, *, #72762, .F. ) ;
#8850=B_SPLINE_CURVE_WITH_KNOTS ( 'NONE', 3,
 ( #25173, #81909, #87795, #67944, #68376, #80580, #5793, #47213, #26511, #40040 ),
 .UNSPECIFIED., .F., .F.,
 ( 4, 2, 2, 2, 4 ),
 ( 0.000000000000000000, 0.0001954339857564098054, 0.0003908679715128196108, 0.0005863019572692293891, 0.0007817359430256392216 ),
 .UNSPECIFIED. ) ;
#8852=CARTESIAN_POINT ( 'NONE',  ( 3.480714749117373330, -5.852078868378310261, 34.47109172314383585 ) ) ;
#8853=CARTESIAN_POINT ( 'NONE',  ( -6.923076923076922462, -4.098570777380720287, 33.41473453929634729 ) ) ;
#8854=CARTESIAN_POINT ( 'NONE',  ( 6.923076923076924238, -2.833524468853757305, 32.15551576947925838 ) ) ;
#8855=CARTESIAN_POINT ( 'NONE',  ( 4.403900465484468008, -3.627508038966689607, 32.91356715214248396 ) ) ;
#8856=LINE ( 'NONE', #76868, #20795 ) ;
#8857=VECTOR ( 'NONE', #77251, 1000.000000000000227 ) ;
#8859=CARTESIAN_POINT ( 'NONE',  ( -1.384615384615383471, -2.486705287966279876, 31.30864560766543647 ) ) ;
#8860=ORIENTED_EDGE ( 'NONE', *, *, #5431, .F. ) ;
#8861=EDGE_LOOP ( 'NONE', ( #71509, #54945, #40186, #29010 ) ) ;
#8864=CARTESIAN_POINT ( 'NONE',  ( 16.40379167219429846, -12.43552623307873972, 30.55307653245132826 ) ) ;
#8866=CARTESIAN_POINT ( 'NONE',  ( 4.153846153846032507, -4.481592998941358097, 33.73612834414048933 ) ) ;
#8867=CYLINDRICAL_SURFACE ( 'NONE', #38197, 0.2499999999999998890 ) ;
#8868=EDGE_LOOP ( 'NONE', ( #23998, #58084 ) ) ;
#8869=B_SPLINE_CURVE_WITH_KNOTS ( 'NONE', 3,
 ( #24546, #58326, #23657, #77716, #29980, #37616, #57438, #65975, #43931, #71395 ),
 .UNSPECIFIED., .F., .F.,
 ( 4, 2, 2, 2, 4 ),
 ( 0.000000000000000000, 0.0001954339857564125972, 0.0003908679715128181471, 0.0005863019572692237513, 0.0007817359430256293554 ),
 .UNSPECIFIED. ) ;
#8870=EDGE_LOOP ( 'NONE', ( #55065, #59083 ) ) ;
#8872=ORIENTED_EDGE ( 'NONE', *, *, #62029, .F. ) ;
#8873=CARTESIAN_POINT ( 'NONE',  ( -6.792286482109968659, -2.845873456487966635, 32.17976146951972538 ) ) ;
#8874=CARTESIAN_POINT ( 'NONE',  ( 8.769230769230768274, -12.29105614889573062, 35.45975837776705220 ) ) ;
#8875=ORIENTED_EDGE ( 'NONE', *, *, #54892, .F. ) ;
#8877=CARTESIAN_POINT ( 'NONE',  ( 4.853438133199125204, -3.754499324213721234, 33.06261337010820256 ) ) ;
#8878=CYLINDRICAL_SURFACE ( 'NONE', #45056, 0.2499999999999986955 ) ;
#8879=ORIENTED_EDGE ( 'NONE', *, *, #74087, .F. ) ;
#8880=VECTOR ( 'NONE', #33968, 1000.000000000000000 ) ;
#8881=FACE_OUTER_BOUND ( 'NONE', #73444, .T. ) ;
#8882=CARTESIAN_POINT ( 'NONE',  ( -9.692307692307691624, -4.098570777380720287, 33.41473453929634729 ) ) ;
#8883=ORIENTED_EDGE ( 'NONE', *, *, #864, .F. ) ;
#8884=FACE_BOUND ( 'NONE', #52182, .T. ) ;
#8885=LINE ( 'NONE', #78213, #15417 ) ;
#8886=CARTESIAN_POINT ( 'NONE',  ( -7.146561866800869467, -2.847400154188068022, 31.58180166144859058 ) ) ;
#8887=DIRECTION ( 'NONE',  ( 1.000000000000000000, 0.000000000000000000, 0.000000000000000000 ) ) ;
#8888=CARTESIAN_POINT ( 'NONE',  ( -6.699649961215353500, -7.630147231320743018, 34.74852402298682819 ) ) ;
#8889=CARTESIAN_POINT ( 'NONE',  ( -5.076923076923075762, -11.11383981884818262, 36.00935417666054406 ) ) ;
#8890=CARTESIAN_POINT ( 'NONE',  ( 8.703147358274886614, -5.557115091759785130, 34.35708131394839171 ) ) ;
#8891=CARTESIAN_POINT ( 'NONE',  ( 12.71153846153989697, -7.500000000000155431, 34.75000000000007105 ) ) ;
#8893=CARTESIAN_POINT ( 'NONE',  ( -11.31568199719312773, -4.387253974876679230, 33.66317474335728832 ) ) ;
#8895=EDGE_CURVE ( 'NONE', #66929, #42644, #29290, .T. ) ;
#8896=ADVANCED_FACE ( 'NONE', ( #22081 ), #22519, .F. ) ;
#8897=CARTESIAN_POINT ( 'NONE',  ( 11.28843831424008215, -12.07920672191015221, 32.31858351112116168 ) ) ;
#8898=CARTESIAN_POINT ( 'NONE',  ( 15.48082354240754555, -4.235687564193448829, 33.53795663066793509 ) ) ;
#8900=CARTESIAN_POINT ( 'NONE',  ( -16.15384615384615330, -10.51840700105979565, 33.73612834413961536 ) ) ;
#8901=CARTESIAN_POINT ( 'NONE',  ( 2.241609928332173762, -5.471508081941601986, 34.59228464037088457 ) ) ;
#8902=CARTESIAN_POINT ( 'NONE',  ( -0.3954701105360228230, -12.37446782046654192, 30.86335684631486842 ) ) ;
#8903=CARTESIAN_POINT ( 'NONE',  ( 4.284637961670942907, -9.804649428959608670, 34.18742332936588468 ) ) ;
#8904=FACE_BOUND ( 'NONE', #57727, .T. ) ;
#8905=CARTESIAN_POINT ( 'NONE',  ( 6.700149964170072359, -4.026226216239095379, 33.68668979543632958 ) ) ;
#8906=CYLINDRICAL_SURFACE ( 'NONE', #48898, 0.2499999999999979738 ) ;
#8907=CARTESIAN_POINT ( 'NONE',  ( -15.36146069743679021, -8.999036380462717588, 34.52022231692819076 ) ) ;
#8908=CARTESIAN_POINT ( 'NONE',  ( -3.230769230769229949, -11.69971097300155272, 32.46337939537588113 ) ) ;
#8909=CARTESIAN_POINT ( 'NONE',  ( 7.145856464345331283, -12.44528174975671853, 30.48912976160716681 ) ) ;
#8910=CARTESIAN_POINT ( 'NONE',  ( 8.769230769230768274, -10.51840700105979565, 33.73612834413961536 ) ) ;
#8911=B_SPLINE_CURVE_WITH_KNOTS ( 'NONE', 3,
 ( #15505, #9619, #85736, #51467, #78968, #42536, #69992, #70892, #8306, #9199 ),
 .UNSPECIFIED., .F., .F.,
 ( 4, 2, 2, 2, 4 ),
 ( 0.0007817359430256388964, 0.0009771253907250075990, 0.001172514838424376085, 0.001367904286123744571, 0.001563293733823113273 ),
 .UNSPECIFIED. ) ;
#8913=ORIENTED_EDGE ( 'NONE', *, *, #22016, .F. ) ;
#8914=AXIS2_PLACEMENT_3D ( 'NONE', #61935, #35357, #70480 ) ;
#8915=ORIENTED_EDGE ( 'NONE', *, *, #23750, .F. ) ;
#8916=EDGE_CURVE ( 'NONE', #40550, #10987, #24616, .T. ) ;
#8917=VECTOR ( 'NONE', #23418, 1000.000000000000114 ) ;
#8918=DIRECTION ( 'NONE',  ( -0.000000000000000000, -0.9396926207859093161, -0.3420201433256663259 ) ) ;
#8919=CARTESIAN_POINT ( 'NONE',  ( -14.37296275365308418, -6.879047030191174805, 34.71129190930000163 ) ) ;
#8920=CARTESIAN_POINT ( 'NONE',  ( -7.715363405186893786, -11.37503395064541678, 33.29242100308974983 ) ) ;
#8921=CARTESIAN_POINT ( 'NONE',  ( 12.46153846153846168, -1.129524287112498415, 32.06866353760679544 ) ) ;
#8922=EDGE_CURVE ( 'NONE', #47411, #41231, #54780, .T. ) ;
#8923=CARTESIAN_POINT ( 'NONE',  ( -13.13456096470192769, -2.544122305571458575, 31.48381861865057729 ) ) ;
#8925=CARTESIAN_POINT ( 'NONE',  ( 6.792386319966616348, -2.295517848115769421, 30.44137282052136939 ) ) ;
#8926=CARTESIAN_POINT ( 'NONE',  ( 3.230769230769231726, -3.513871655860378418, 32.76840700105978499 ) ) ;
#8927=DIRECTION ( 'NONE',  ( -0.000000000000000000, 0.7660444431189791237, -0.6427876096865379196 ) ) ;
#8928=CARTESIAN_POINT ( 'NONE',  ( 10.61538461538449418, -6.835583212225970762, 34.95778746994575670 ) ) ;
#8929=DIRECTION ( 'NONE',  ( 0.000000000000000000, 0.9396926207859126468, 0.3420201433256571111 ) ) ;
#8930=CARTESIAN_POINT ( 'NONE',  ( 13.63461538461680611, -7.500000000000154543, 35.00000000000007105 ) ) ;
#8931=CARTESIAN_POINT ( 'NONE',  ( 14.53070365930516061, -11.76359900205217635, 32.36225158514719880 ) ) ;
#8932=EDGE_CURVE ( 'NONE', #43893, #4302, #73371, .T. ) ;
#8933=DIRECTION ( 'NONE',  ( -0.000000000000000000, -0.5000000000000009992, -0.8660254037844380415 ) ) ;
#8934=VERTEX_POINT ( 'NONE', #39606 ) ;
#8936=CARTESIAN_POINT ( 'NONE',  ( -8.769230769230768274, -12.62096338111211580, 30.90682066428153263 ) ) ;
#8938=CARTESIAN_POINT ( 'NONE',  ( 7.846153846153846700, -1.790695186598648903, 34.54067556320373455 ) ) ;
#8939=CARTESIAN_POINT ( 'NONE',  ( -10.61538461538461320, -13.63283147151868846, 33.57946703557072254 ) ) ;
#8940=EDGE_LOOP ( 'NONE', ( #66011, #64024, #70456, #87506 ) ) ;
#8941=DIRECTION ( 'NONE',  ( 0.000000000000000000, 0.9396926207859126468, -0.3420201433256571111 ) ) ;
#8942=CARTESIAN_POINT ( 'NONE',  ( 7.622668902429898807, -2.599994579823202923, 30.74605699353653776 ) ) ;
#8943=ORIENTED_EDGE ( 'NONE', *, *, #54144, .F. ) ;
#8944=CARTESIAN_POINT ( 'NONE',  ( 9.469442270104055481, -2.501496062324912284, 29.88072118266895671 ) ) ;
#8945=CARTESIAN_POINT ( 'NONE',  ( 12.59206389977210705, -5.915461855592780260, 34.75538340440931506 ) ) ;
#8947=DIRECTION ( 'NONE',  ( 0.000000000000000000, 0.6427876096865368094, 0.7660444431189802339 ) ) ;
#8948=CARTESIAN_POINT ( 'NONE',  ( 15.23076923076923173, -9.905515769479276145, 34.41647553114623292 ) ) ;
#8949=ORIENTED_EDGE ( 'NONE', *, *, #54889, .T. ) ;
#8950=DIRECTION ( 'NONE',  ( 0.000000000000000000, 0.1736481776669267785, -0.9848077530122087975 ) ) ;
#8952=ADVANCED_FACE ( 'NONE', ( #25181 ), #59411, .F. ) ;
#8953=B_SPLINE_CURVE_WITH_KNOTS ( 'NONE', 3,
 ( #63477, #78314, #77876, #71116, #30141, #50828, #71557, #84219, #1779, #49959 ),
 .UNSPECIFIED., .F., .F.,
 ( 4, 2, 2, 2, 4 ),
 ( 0.0007817246256747465219, 0.0009771112852218900684, 0.001172497944769033615, 0.001367884604316177378, 0.001563271263863320925 ),
 .UNSPECIFIED. ) ;
#8954=CARTESIAN_POINT ( 'NONE',  ( -9.468931751609508396, -2.501478030877323455, 29.88021232661721172 ) ) ;
#8955=VERTEX_POINT ( 'NONE', #31494 ) ;
#8956=EDGE_CURVE ( 'NONE', #55506, #1287, #65708, .T. ) ;
#8958=ORIENTED_EDGE ( 'NONE', *, *, #65458, .F. ) ;
#8959=B_SPLINE_CURVE_WITH_KNOTS ( 'NONE', 3,
 ( #17564, #87370, #3588, #86020, #58979, #72944, #46363, #25205, #66177, #24300 ),
 .UNSPECIFIED., .F., .F.,
 ( 4, 2, 2, 2, 4 ),
 ( 0.000000000000000000, 0.0001954311564186871184, 0.0003908623128373742367, 0.0005862934692560614093, 0.0007817246256747484735 ),
 .UNSPECIFIED. ) ;
#8961=ADVANCED_FACE ( 'NONE', ( #58067 ), #86913, .F. ) ;
#8962=DIRECTION ( 'NONE',  ( 0.000000000000000000, 0.6427876096865373645, -0.7660444431189797898 ) ) ;
#8963=CARTESIAN_POINT ( 'NONE',  ( -15.23076923076935252, -2.379036618888197729, 30.90682066428292885 ) ) ;
#8965=CARTESIAN_POINT ( 'NONE',  ( -2.980823821391187067, -8.476813868363244353, 34.90874843262270133 ) ) ;
#8966=CARTESIAN_POINT ( 'NONE',  ( 14.30769230769218581, -4.320704448113951379, 33.92786785259630022 ) ) ;
#8967=ORIENTED_EDGE ( 'NONE', *, *, #73884, .T. ) ;
#8968=ORIENTED_EDGE ( 'NONE', *, *, #71436, .F. ) ;
#8969=CARTESIAN_POINT ( 'NONE',  ( -1.134615384615447420, -7.565270445406050648, 34.75000000000000000 ) ) ;
#8971=CARTESIAN_POINT ( 'NONE',  ( 12.59206389977210705, -11.66157788607254098, 32.95092075102925833 ) ) ;
#8972=ORIENTED_EDGE ( 'NONE', *, *, #63331, .T. ) ;
#8973=AXIS2_PLACEMENT_3D ( 'NONE', #36865, #55811, #28802 ) ;
#8974=CARTESIAN_POINT ( 'NONE',  ( 11.78846153846154010, -2.499999999999998668, 29.75000000000000355 ) ) ;
#8976=ORIENTED_EDGE ( 'NONE', *, *, #84507, .T. ) ;
#8977=VECTOR ( 'NONE', #55579, 1000.000000000000227 ) ;
#8978=B_SPLINE_CURVE_WITH_KNOTS ( 'NONE', 3,
 ( #6882, #76680, #7776, #56406, #69915, #55511, #35240, #49203, #77560, #77119 ),
 .UNSPECIFIED., .F., .F.,
 ( 4, 2, 2, 2, 4 ),
 ( 0.000000000000000000, 0.0001954311564186876334, 0.0003908623128373752667, 0.0005862934692560629272, 0.0007817246256747505334 ),
 .UNSPECIFIED. ) ;
#8979=B_SPLINE_CURVE_WITH_KNOTS ( 'NONE', 3,
 ( #40580, #47765, #75247, #13537, #76120, #46875, #34249, #41017, #7675, #41457 ),
 .UNSPECIFIED., .F., .F.,
 ( 4, 2, 2, 2, 4 ),
 ( 0.000000000000000000, 0.0001954339857564054957, 0.0003908679715128109914, 0.0005863019572692164871, 0.0007817359430256219828 ),
 .UNSPECIFIED. ) ;
#8980=ORIENTED_EDGE ( 'NONE', *, *, #60693, .F. ) ;
#8981=CARTESIAN_POINT ( 'NONE',  ( -12.23875892027004753, -5.114059244376869984, 34.14424750095245287 ) ) ;
#8982=ORIENTED_EDGE ( 'NONE', *, *, #56462, .F. ) ;
#8983=CARTESIAN_POINT ( 'NONE',  ( 4.219101725122176738, -5.219633306516380244, 34.19971097300157936 ) ) ;
#8984=B_SPLINE_CURVE_WITH_KNOTS ( 'NONE', 3,
 ( #53626, #54059, #73908, #34239, #73465, #27045, #88330, #66700, #81114, #27488 ),
 .UNSPECIFIED., .F., .F.,
 ( 4, 2, 2, 2, 4 ),
 ( 0.0007817246336856293861, 0.0009771112958940105907, 0.001172497958102391904, 0.001367884620310773217, 0.001563271282519154530 ),
 .UNSPECIFIED. ) ;
#8985=B_SPLINE_CURVE_WITH_KNOTS ( 'NONE', 3,
 ( #61632, #19331, #5373, #39169, #26535, #6265, #59863, #19772, #74725, #47233 ),
 .UNSPECIFIED., .F., .F.,
 ( 4, 2, 2, 2, 4 ),
 ( 0.0007817359527651099533, 0.0009771254036996487088, 0.001172514854634187573, 0.001367904305568726220, 0.001563293756503265084 ),
 .UNSPECIFIED. ) ;
#8986=EDGE_CURVE ( 'NONE', #39878, #13065, #79240, .T. ) ;
#8987=CARTESIAN_POINT ( 'NONE',  ( 14.17700170458200404, -5.496505350115501010, 34.60290016733514307 ) ) ;
#8988=ORIENTED_EDGE ( 'NONE', *, *, #66143, .F. ) ;
#8989=CARTESIAN_POINT ( 'NONE',  ( 15.10062126103753855, -2.373036134822904319, 30.88089517874952250 ) ) ;
#8990=CARTESIAN_POINT ( 'NONE',  ( -14.17690186672535901, -12.62708834333097663, 30.88030960425257021 ) ) ;
#8991=CARTESIAN_POINT ( 'NONE',  ( 6.923076923076800782, -5.941354392335915335, 34.76329471203413846 ) ) ;
#8992=FACE_BOUND ( 'NONE', #85133, .T. ) ;
#8993=CARTESIAN_POINT ( 'NONE',  ( -8.769230769230892619, -2.379036618888197729, 30.90682066428292885 ) ) ;
#8994=DIRECTION ( 'NONE',  ( 0.000000000000000000, 0.1736481776669275834, 0.9848077530122086864 ) ) ;
#8995=CARTESIAN_POINT ( 'NONE',  ( 8.519207531937803779, -2.587272538249754117, 30.68239716806877837 ) ) ;
#8996=CARTESIAN_POINT ( 'NONE',  ( -5.999999999999998224, -8.164416787775445883, 34.95778746994557906 ) ) ;
#8997=CARTESIAN_POINT ( 'NONE',  ( -15.90390074446811042, -2.986452184633680229, 32.43230066228895225 ) ) ;
#8998=CARTESIAN_POINT ( 'NONE',  ( -4.826868657009622865, -4.074993327901525575, 33.72946981652012255 ) ) ;
#8999=FACE_OUTER_BOUND ( 'NONE', #45170, .T. ) ;
#9000=EDGE_LOOP ( 'NONE', ( #59965, #48043 ) ) ;
#9001=CARTESIAN_POINT ( 'NONE',  ( 10.36540788444226280, -10.66389620160130036, 33.62221079203477103 ) ) ;
#9002=ORIENTED_EDGE ( 'NONE', *, *, #86075, .F. ) ;
#9003=ORIENTED_EDGE ( 'NONE', *, *, #77748, .T. ) ;
#9004=EDGE_CURVE ( 'NONE', #27408, #18603, #66620, .T. ) ;
#9005=CARTESIAN_POINT ( 'NONE',  ( -1.384615384615506484, -5.094484230521993062, 34.41647553114689373 ) ) ;
#9006=CARTESIAN_POINT ( 'NONE',  ( 16.21910172512217585, -12.27809138561124591, 31.22303859784720359 ) ) ;
#9009=CARTESIAN_POINT ( 'NONE',  ( -11.53846153846153655, -13.87047571288749737, 32.06866353760679544 ) ) ;
#9010=DIRECTION ( 'NONE',  ( -0.000000000000000000, -0.000000000000000000, -1.000000000000000000 ) ) ;
#9011=CARTESIAN_POINT ( 'NONE',  ( -2.373774687052441656, -11.35647404775217595, 33.31231777344666511 ) ) ;
#9012=ORIENTED_EDGE ( 'NONE', *, *, #45343, .T. ) ;
#9013=CARTESIAN_POINT ( 'NONE',  ( 14.05769230769230838, -2.249999999999998668, 29.75000000000000355 ) ) ;
#9014=CARTESIAN_POINT ( 'NONE',  ( 14.30769230769231015, -12.62096338111211580, 30.90682066428153263 ) ) ;
#9016=CARTESIAN_POINT ( 'NONE',  ( 15.45378207486262667, -12.38742843783360748, 31.66772728687926985 ) ) ;
#9017=CARTESIAN_POINT ( 'NONE',  ( 13.60762822870878530, -5.582272713120729257, 34.63742843783360570 ) ) ;
#9019=ORIENTED_EDGE ( 'NONE', *, *, #21243, .F. ) ;
#9020=B_SPLINE_CURVE_WITH_KNOTS ( 'NONE', 3,
 ( #60124, #82189, #80867, #54249, #73210, #74537, #11509, #66446, #38989, #33105 ),
 .UNSPECIFIED., .F., .F.,
 ( 4, 2, 2, 2, 4 ),
 ( 0.000000000000000000, 0.0001954311564186867389, 0.0003908623128373734778, 0.0005862934692560602167, 0.0007817246256747469556 ),
 .UNSPECIFIED. ) ;
#9021=EDGE_LOOP ( 'NONE', ( #65119, #19753, #26900, #32776 ) ) ;
#9022=EDGE_CURVE ( 'NONE', #82557, #54935, #41871, .T. ) ;
#9023=CARTESIAN_POINT ( 'NONE',  ( -7.623374177175780808, -12.11081565061823717, 32.26097654155341843 ) ) ;
#9024=ORIENTED_EDGE ( 'NONE', *, *, #1298, .T. ) ;
#9025=CYLINDRICAL_SURFACE ( 'NONE', #11059, 0.2499999999999994726 ) ;
#9026=CARTESIAN_POINT ( 'NONE',  ( 17.77707304109314634, -11.43668979543635089, 33.22377378376089752 ) ) ;
#9028=ADVANCED_FACE ( 'NONE', ( #85551 ), #23825, .F. ) ;
#9029=CARTESIAN_POINT ( 'NONE',  ( -0.5276208408985973985, -11.91647553114624181, 32.58852847137148245 ) ) ;
#9031=CARTESIAN_POINT ( 'NONE',  ( 14.30769230769231015, -2.708943851104267164, 35.45975837776705220 ) ) ;
#9034=CARTESIAN_POINT ( 'NONE',  ( 18.00000000000031264, -2.255955759149395501, 30.00000000000324363 ) ) ;
#9035=ORIENTED_EDGE ( 'NONE', *, *, #16167, .T. ) ;
#9036=CARTESIAN_POINT ( 'NONE',  ( -13.38461538461550582, -11.48612834414049644, 32.76840700105863391 ) ) ;
#9038=CARTESIAN_POINT ( 'NONE',  ( 6.000000000000001776, -9.058645607665452459, 34.76329471203371924 ) ) ;
#9039=CARTESIAN_POINT ( 'NONE',  ( 0.7115927731767757169, -2.779044189368096607, 31.39831045268885035 ) ) ;
#9040=EDGE_CURVE ( 'NONE', #58008, #82311, #38661, .T. ) ;
#9041=CARTESIAN_POINT ( 'NONE',  ( -9.692307692307691624, -1.629998284177014645, 34.34916445242399163 ) ) ;
#9042=CARTESIAN_POINT ( 'NONE',  ( -11.28840711854808632, -2.920487667080175598, 32.31805714834170828 ) ) ;
#9044=ORIENTED_EDGE ( 'NONE', *, *, #36731, .F. ) ;
#9045=CARTESIAN_POINT ( 'NONE',  ( -17.07692307692319744, -10.90142922262034020, 33.41473453929536674 ) ) ;
#9046=CARTESIAN_POINT ( 'NONE',  ( 4.153846153846030731, -11.06231777344772027, 33.60647404775119895 ) ) ;
#9051=CARTESIAN_POINT ( 'NONE',  ( -13.38461538461538325, -12.37446782046654192, 30.86335684631486131 ) ) ;
#9052=DIRECTION ( 'NONE',  ( -0.000000000000000000, 0.9396926207859092051, -0.3420201433256662704 ) ) ;
#9053=VERTEX_POINT ( 'NONE', #47221 ) ;
#9055=CARTESIAN_POINT ( 'NONE',  ( -5.142193522883852452, -6.879047030191174805, 34.71129190930000163 ) ) ;
#9056=EDGE_CURVE ( 'NONE', #83747, #16683, #9624, .T. ) ;
#9057=ORIENTED_EDGE ( 'NONE', *, *, #63446, .F. ) ;
#9058=CARTESIAN_POINT ( 'NONE',  ( -18.24997674404859183, -4.818429247618089661, 34.26397095200675125 ) ) ;
#9060=CARTESIAN_POINT ( 'NONE',  ( 7.173131342990376247, -4.074993327901525575, 33.72946981652012255 ) ) ;
#9061=CARTESIAN_POINT ( 'NONE',  ( -12.46153846153846168, -2.499999999999998668, 29.50000000000001066 ) ) ;
#9063=DIRECTION ( 'NONE',  ( 0.000000000000000000, 0.000000000000000000, 1.000000000000000000 ) ) ;
#9064=DIRECTION ( 'NONE',  ( -0.000000000000000000, -0.3420201433256694346, -0.9396926207859080948 ) ) ;
#9066=CARTESIAN_POINT ( 'NONE',  ( -3.007756386675836335, -2.308499170217967134, 30.53291367094873721 ) ) ;
#9067=EDGE_CURVE ( 'NONE', #10320, #82155, #4200, .T. ) ;
#9068=ORIENTED_EDGE ( 'NONE', *, *, #46916, .T. ) ;
#9069=CARTESIAN_POINT ( 'NONE',  ( 12.46153846153833911, -12.16647553114689728, 32.15551576947799362 ) ) ;
#9070=CARTESIAN_POINT ( 'NONE',  ( 0.5923289025054103707, -9.929761469519744921, 34.40412654351204225 ) ) ;
#9071=ORIENTED_EDGE ( 'NONE', *, *, #20346, .T. ) ;
#9072=EDGE_CURVE ( 'NONE', #56712, #56271, #46788, .T. ) ;
#9073=DIRECTION ( 'NONE',  ( -0.000000000000000000, 0.8660254037844397068, -0.4999999999999978906 ) ) ;
#9075=LINE ( 'NONE', #8634, #10632 ) ;
#9077=VECTOR ( 'NONE', #84540, 1000.000000000000227 ) ;
#9078=DIRECTION ( 'NONE',  ( -0.000000000000000000, 0.9396926207859093161, -0.3420201433256663259 ) ) ;
#9079=CARTESIAN_POINT ( 'NONE',  ( -3.930833309752757909, -4.026326845037961455, 33.68677907613344047 ) ) ;
#9081=ORIENTED_EDGE ( 'NONE', *, *, #61418, .F. ) ;
#9082=FACE_BOUND ( 'NONE', #50798, .T. ) ;
#9083=ORIENTED_EDGE ( 'NONE', *, *, #8932, .F. ) ;
#9085=EDGE_CURVE ( 'NONE', #37091, #14199, #72967, .T. ) ;
#9087=EDGE_CURVE ( 'NONE', #37061, #67514, #79030, .T. ) ;
#9088=CYLINDRICAL_SURFACE ( 'NONE', #1836, 0.2500000000000004996 ) ;
#9090=VERTEX_POINT ( 'NONE', #40049 ) ;
#9091=EDGE_LOOP ( 'NONE', ( #77364, #9625 ) ) ;
#9092=DIRECTION ( 'NONE',  ( -0.000000000000000000, -0.3420201433256694346, -0.9396926207859080948 ) ) ;
#9093=ORIENTED_EDGE ( 'NONE', *, *, #45927, .T. ) ;
#9094=CYLINDRICAL_SURFACE ( 'NONE', #232, 0.2499999999999986955 ) ;
#9095=EDGE_CURVE ( 'NONE', #47058, #75513, #55718, .T. ) ;
#9097=CARTESIAN_POINT ( 'NONE',  ( 14.08420738312798015, -12.11044203135681840, 32.26167407432752299 ) ) ;
#9098=EDGE_CURVE ( 'NONE', #34676, #34885, #45986, .T. ) ;
#9099=CARTESIAN_POINT ( 'NONE',  ( -18.06608237936013239, -6.343179335718451384, 34.87096338111212646 ) ) ;
#9100=EDGE_LOOP ( 'NONE', ( #65822, #78103 ) ) ;
#9101=B_SPLINE_CURVE_WITH_KNOTS ( 'NONE', 3,
 ( #5595, #79920, #5149, #67299, #88921, #60084 ),
 .UNSPECIFIED., .F., .F.,
 ( 4, 2, 4 ),
 ( 0.000000000000000000, 0.0001954784845028915703, 0.0003909569690057831406 ),
 .UNSPECIFIED. ) ;
#9102=FACE_OUTER_BOUND ( 'NONE', #75969, .T. ) ;
#9103=ADVANCED_FACE ( 'NONE', ( #42256 ), #21524, .F. ) ;
#9104=AXIS2_PLACEMENT_3D ( 'NONE', #63794, #35000, #43525 ) ;
#9105=CARTESIAN_POINT ( 'NONE',  ( -14.98071481085577972, -3.435999193479609914, 33.07426656108010832 ) ) ;
#9106=CARTESIAN_POINT ( 'NONE',  ( -17.93129618099654010, -7.749508974024934105, 34.99406763069168846 ) ) ;
#9107=CARTESIAN_POINT ( 'NONE',  ( -9.692307692307691624, -13.37000171582298513, 34.34916445242398453 ) ) ;
#9109=EDGE_LOOP ( 'NONE', ( #65669, #69428 ) ) ;
#9110=VECTOR ( 'NONE', #88413, 999.9999999999998863 ) ;
#9111=EDGE_LOOP ( 'NONE', ( #71627, #58649 ) ) ;
#9112=ADVANCED_FACE ( 'NONE', ( #69274 ), #16869, .F. ) ;
#9113=CARTESIAN_POINT ( 'NONE',  ( -5.999999999999998224, -2.900454961884010974, 35.62045528018868623 ) ) ;
#9114=CARTESIAN_POINT ( 'NONE',  ( 10.86533013373275836, -6.696923467548660192, 34.68552623307873972 ) ) ;
#9115=CARTESIAN_POINT ( 'NONE',  ( 16.15384615384603251, -6.026961402154118908, 34.52809138561165270 ) ) ;
#9116=CARTESIAN_POINT ( 'NONE',  ( -14.30769230769230660, -12.62096338111211580, 30.90682066428153263 ) ) ;
#9117=FACE_BOUND ( 'NONE', #55522, .T. ) ;
#9118=CARTESIAN_POINT ( 'NONE',  ( -2.307692307692305711, -9.780366693483667717, 34.19971097300155094 ) ) ;
#9119=EDGE_LOOP ( 'NONE', ( #51356, #83465, #3967, #15486 ) ) ;
#9120=CARTESIAN_POINT ( 'NONE',  ( 17.29993442853592711, -10.61302985866384141, 33.66295027996417843 ) ) ;
#9121=DIRECTION ( 'NONE',  ( -0.000000000000000000, -0.9396926207859093161, -0.3420201433256663259 ) ) ;
#9122=B_SPLINE_CURVE_WITH_KNOTS ( 'NONE', 3,
 ( #27225, #20903, #54686, #28111, #1083, #6954, #21796, #6520, #48375, #7406 ),
 .UNSPECIFIED., .F., .F.,
 ( 4, 2, 2, 2, 4 ),
 ( 0.0007817246256747448956, 0.0009771112852218876831, 0.001172497944769030579, 0.001367884604316173475, 0.001563271263863316371 ),
 .UNSPECIFIED. ) ;
#9123=CYLINDRICAL_SURFACE ( 'NONE', #63130, 0.2499999999999986955 ) ;
#9124=CARTESIAN_POINT ( 'NONE',  ( 10.36538461538461675, -7.500000000000001776, 34.75000000000000000 ) ) ;
#9125=ORIENTED_EDGE ( 'NONE', *, *, #61260, .F. ) ;
#9126=B_SPLINE_CURVE_WITH_KNOTS ( 'NONE', 3,
 ( #18839, #5770, #81439, #19725, #82323, #74678, #20604, #61140, #5325, #46750 ),
 .UNSPECIFIED., .F., .F.,
 ( 4, 2, 2, 2, 4 ),
 ( 0.0007817359430256216575, 0.0009771253907249856981, 0.001172514838424349630, 0.001367904286123713779, 0.001563293733823077711 ),
 .UNSPECIFIED. ) ;
#9127=DIRECTION ( 'NONE',  ( 0.000000000000000000, 0.9396926207859126468, 0.3420201433256571111 ) ) ;
#9128=EDGE_LOOP ( 'NONE', ( #79849, #16010, #34978, #1077 ) ) ;
#9129=B_SPLINE_CURVE_WITH_KNOTS ( 'NONE', 3,
 ( #58193, #85684, #49239, #8703, #36180, #32960, #87479, #24858, #4596, #25758 ),
 .UNSPECIFIED., .F., .F.,
 ( 4, 2, 2, 2, 4 ),
 ( 0.0007817359430256322827, 0.0009771253907249989254, 0.001172514838424365676, 0.001367904286123732428, 0.001563293733823098962 ),
 .UNSPECIFIED. ) ;
#9130=FACE_BOUND ( 'NONE', #24148, .T. ) ;
#9131=CARTESIAN_POINT ( 'NONE',  ( 17.99999999999987566, -3.835265460704628815, 33.15142922262033665 ) ) ;
#9132=CARTESIAN_POINT ( 'NONE',  ( -18.00000000000000000, -2.292212530054419606, 30.41441678777542990 ) ) ;
#9133=CARTESIAN_POINT ( 'NONE',  ( -11.53846153846153655, -8.973038597847269315, 34.52809138561121927 ) ) ;
#9134=VERTEX_POINT ( 'NONE', #79470 ) ;
#9135=CARTESIAN_POINT ( 'NONE',  ( 11.76147438255493149, -10.77377354290276124, 33.85451476688484718 ) ) ;
#9136=CARTESIAN_POINT ( 'NONE',  ( -14.55771554498526932, -4.335965774309648246, 33.62209801155881905 ) ) ;
#9137=CARTESIAN_POINT ( 'NONE',  ( -9.757578138268467427, -3.300289026998414865, 32.46337939537583139 ) ) ;
#9138=EDGE_CURVE ( 'NONE', #19850, #81242, #82544, .T. ) ;
#9139=LINE ( 'NONE', #23083, #74819 ) ;
#9140=ORIENTED_EDGE ( 'NONE', *, *, #26398, .T. ) ;
#9141=CARTESIAN_POINT ( 'NONE',  ( -9.757577692864012775, -3.083524468853724443, 32.58852847137143272 ) ) ;
#9145=VECTOR ( 'NONE', #87989, 1000.000000000000227 ) ;
#9146=ORIENTED_EDGE ( 'NONE', *, *, #37247, .T. ) ;
#9147=CARTESIAN_POINT ( 'NONE',  ( 13.38461538461538680, -9.819645486525091727, 36.12317359536749706 ) ) ;
#9148=DIRECTION ( 'NONE',  ( -0.000000000000000000, -0.000000000000000000, -1.000000000000000000 ) ) ;
#9149=CARTESIAN_POINT ( 'NONE',  ( 4.853438152358743096, -2.612411019501189813, 31.66733052389439962 ) ) ;
#9150=CARTESIAN_POINT ( 'NONE',  ( -15.45364874750681849, -7.630690623152299956, 34.99857592706774057 ) ) ;
#9152=CARTESIAN_POINT ( 'NONE',  ( 15.23076923076923173, -5.180354513474913603, 36.12317359536750416 ) ) ;
#9153=CARTESIAN_POINT ( 'NONE',  ( 6.130525701763565039, -2.882268652242224505, 31.66798894389554064 ) ) ;
#9155=ORIENTED_EDGE ( 'NONE', *, *, #24435, .F. ) ;
#9156=DIRECTION ( 'NONE',  ( -0.000000000000000000, -0.1736481776669307198, -0.9848077530122080203 ) ) ;
#9157=CARTESIAN_POINT ( 'NONE',  ( 5.777073041093150785, -8.282780595021769443, 34.94152052738834868 ) ) ;
#9158=ORIENTED_EDGE ( 'NONE', *, *, #17243, .T. ) ;
#9159=VERTEX_POINT ( 'NONE', #76477 ) ;
#9160=ORIENTED_EDGE ( 'NONE', *, *, #10972, .T. ) ;
#9161=CARTESIAN_POINT ( 'NONE',  ( 4.023154687178592148, -12.11776431015576172, 31.66791131148498906 ) ) ;
#9162=CARTESIAN_POINT ( 'NONE',  ( -17.07692307692307665, -8.973038597847269315, 34.52809138561121927 ) ) ;
#9163=B_SPLINE_CURVE_WITH_KNOTS ( 'NONE', 3,
 ( #30219, #85160, #36957, #1854, #14936, #42413 ),
 .UNSPECIFIED., .F., .F.,
 ( 4, 2, 4 ),
 ( 3.879202041849147211E-17, 0.0001954756301637101891, 0.0003909512603273816180 ),
 .UNSPECIFIED. ) ;
#9165=CARTESIAN_POINT ( 'NONE',  ( 6.000000000000001776, -2.538708090699994813, 30.37095296980875503 ) ) ;
#9166=CARTESIAN_POINT ( 'NONE',  ( -13.38461538461538325, -6.343179335718451384, 34.87096338111211935 ) ) ;
#9167=DIRECTION ( 'NONE',  ( -0.000000000000000000, -0.7660444431189791237, -0.6427876096865379196 ) ) ;
#9168=CARTESIAN_POINT ( 'NONE',  ( 0.3962885297643758964, -2.255955759149247619, 30.00000000000013856 ) ) ;
#9169=ORIENTED_EDGE ( 'NONE', *, *, #63015, .F. ) ;
#9170=B_SPLINE_CURVE_WITH_KNOTS ( 'NONE', 3,
 ( #80711, #26634, #82032, #46459, #81585, #61286, #6375, #60412, #40601, #67625 ),
 .UNSPECIFIED., .F., .F.,
 ( 4, 2, 2, 2, 4 ),
 ( 0.0007817246256747458714, 0.0009771112852218889842, 0.001172497944769032097, 0.001367884604316175210, 0.001563271263863318323 ),
 .UNSPECIFIED. ) ;
#9172=CARTESIAN_POINT ( 'NONE',  ( -16.82692307692164135, -7.500000000000155431, 34.75000000000007105 ) ) ;
#9175=CARTESIAN_POINT ( 'NONE',  ( -3.230769230769229949, -5.180354513474913603, 36.12317359536750416 ) ) ;
#9176=DIRECTION ( 'NONE',  ( -0.000000000000000000, -0.1736481776669307198, -0.9848077530122080203 ) ) ;
#9178=EDGE_CURVE ( 'NONE', #67715, #56424, #34197, .T. ) ;
#9179=AXIS2_PLACEMENT_3D ( 'NONE', #72001, #44516, #51254 ) ;
#9180=EDGE_LOOP ( 'NONE', ( #7202, #7955, #6085, #32079 ) ) ;
#9181=CARTESIAN_POINT ( 'NONE',  ( -17.29985003582992320, -2.523278758544490685, 31.42238647778638239 ) ) ;
#9183=LINE ( 'NONE', #42522, #42685 ) ;
#9184=CARTESIAN_POINT ( 'NONE',  ( 6.130525438233648927, -12.70449254468099198, 30.44128974285582956 ) ) ;
#9185=ORIENTED_EDGE ( 'NONE', *, *, #10972, .F. ) ;
#9186=EDGE_CURVE ( 'NONE', #85950, #4986, #27811, .T. ) ;
#9187=CARTESIAN_POINT ( 'NONE',  ( -2.372962308248625085, -6.835583212224499938, 34.95778746994557906 ) ) ;
#9188=CARTESIAN_POINT ( 'NONE',  ( -17.14217406708431923, -2.506253911140460477, 30.00000000000013856 ) ) ;
#9189=ADVANCED_FACE ( 'NONE', ( #10112 ), #50645, .F. ) ;
#9190=CARTESIAN_POINT ( 'NONE',  ( 6.923076923076924238, -12.78798330534102767, 29.49999999999997868 ) ) ;
#9191=ORIENTED_EDGE ( 'NONE', *, *, #54470, .T. ) ;
#9192=CARTESIAN_POINT ( 'NONE',  ( -0.5268089074992371446, -8.613356846314824011, 34.62446782046655613 ) ) ;
#9193=ORIENTED_EDGE ( 'NONE', *, *, #4314, .F. ) ;
#9194=EDGE_CURVE ( 'NONE', #48093, #61557, #19199, .T. ) ;
#9195=CARTESIAN_POINT ( 'NONE',  ( 13.38461538461538680, -12.34228464037088635, 31.77849191805839268 ) ) ;
#9197=CARTESIAN_POINT ( 'NONE',  ( 12.21156173059610772, -8.303909089506435137, 34.68538101551103381 ) ) ;
#9198=B_SPLINE_CURVE_WITH_KNOTS ( 'NONE', 3,
 ( #30454, #7208, #29582, #9312, #15622, #84094, #22809, #43089, #70564, #57037 ),
 .UNSPECIFIED., .F., .F.,
 ( 4, 2, 2, 2, 4 ),
 ( 0.0007817246256747470640, 0.0009771112852218896347, 0.001172497944769032314, 0.001367884604316174993, 0.001563271263863317455 ),
 .UNSPECIFIED. ) ;
#9199=CARTESIAN_POINT ( 'NONE',  ( -14.30769230769230660, -11.69971097300155272, 32.46337939537588113 ) ) ;
#9200=CARTESIAN_POINT ( 'NONE',  ( -3.361378885973311359, -7.722926974430166069, 34.99546784045485737 ) ) ;
#9201=EDGE_LOOP ( 'NONE', ( #47443, #43947 ) ) ;
#9203=ORIENTED_EDGE ( 'NONE', *, *, #57163, .T. ) ;
#9204=ORIENTED_EDGE ( 'NONE', *, *, #11183, .T. ) ;
#9205=CARTESIAN_POINT ( 'NONE',  ( -6.065270445960774914, -11.48612834413959582, 32.76840700105983473 ) ) ;
#9206=CARTESIAN_POINT ( 'NONE',  ( -16.85391172531022619, -3.587049720035815348, 32.86302985866382897 ) ) ;
#9207=ADVANCED_FACE ( 'NONE', ( #66840 ), #31727, .F. ) ;
#9208=CARTESIAN_POINT ( 'NONE',  ( 0.7114838709165038910, -6.653508905675592722, 34.93172785388651391 ) ) ;
#9209=CARTESIAN_POINT ( 'NONE',  ( 0.2380535369741280383, -12.47654668319379567, 31.42292124445336654 ) ) ;
#9210=DIRECTION ( 'NONE',  ( -0.000000000000000000, -0.5000000000000009992, -0.8660254037844380415 ) ) ;
#9212=ORIENTED_EDGE ( 'NONE', *, *, #34213, .F. ) ;
#9213=VERTEX_POINT ( 'NONE', #52869 ) ;
#9214=EDGE_LOOP ( 'NONE', ( #47397, #35475, #51473, #6587 ) ) ;
#9215=CARTESIAN_POINT ( 'NONE',  ( 4.376858997939548246, -4.026326845037961455, 33.68677907613344047 ) ) ;
#9216=EDGE_CURVE ( 'NONE', #14730, #21791, #29895, .T. ) ;
#9217=ORIENTED_EDGE ( 'NONE', *, *, #74705, .T. ) ;
#9218=CARTESIAN_POINT ( 'NONE',  ( 9.019176287578908102, -8.433404298154334455, 34.66254593164985920 ) ) ;
#9219=CARTESIAN_POINT ( 'NONE',  ( -5.207613680033385428, -12.62707690430377383, 30.88035979386743435 ) ) ;
#9221=ORIENTED_EDGE ( 'NONE', *, *, #34560, .T. ) ;
#9222=AXIS2_PLACEMENT_3D ( 'NONE', #77108, #49190, #76671 ) ;
#9223=EDGE_CURVE ( 'NONE', #74234, #26718, #19102, .T. ) ;
#9224=B_SPLINE_CURVE_WITH_KNOTS ( 'NONE', 3,
 ( #86449, #25614, #53070, #40035, #17528, #39593, #60278, #87791, #51725, #19304 ),
 .UNSPECIFIED., .F., .F.,
 ( 4, 2, 2, 2, 4 ),
 ( 0.0007817246256747465219, 0.0009771112852218900684, 0.001172497944769033615, 0.001367884604316177378, 0.001563271263863320925 ),
 .UNSPECIFIED. ) ;
#9225=ORIENTED_EDGE ( 'NONE', *, *, #5495, .T. ) ;
#9226=B_SPLINE_CURVE_WITH_KNOTS ( 'NONE', 3,
 ( #74462, #55072, #25838, #39800, #88015, #48309, #47871, #40244, #81671, #40688 ),
 .UNSPECIFIED., .F., .F.,
 ( 4, 2, 2, 2, 4 ),
 ( 0.000000000000000000, 0.0001954311564186863323, 0.0003908623128373726646, 0.0005862934692560590241, 0.0007817246256747453293 ),
 .UNSPECIFIED. ) ;
#9227=CARTESIAN_POINT ( 'NONE',  ( -7.846153846153967493, -12.16647553114689728, 32.15551576947799362 ) ) ;
#9228=AXIS2_PLACEMENT_3D ( 'NONE', #71638, #23453, #50043 ) ;
#9229=ORIENTED_EDGE ( 'NONE', *, *, #62889, .F. ) ;
#9230=FACE_BOUND ( 'NONE', #59012, .T. ) ;
#9231=CARTESIAN_POINT ( 'NONE',  ( 3.361559671736182864, -2.494656445102013453, 31.33466734024120015 ) ) ;
#9232=VECTOR ( 'NONE', #85093, 1000.000000000000227 ) ;
#9233=FACE_OUTER_BOUND ( 'NONE', #83023, .T. ) ;
#9234=VERTEX_POINT ( 'NONE', #79910 ) ;
#9235=CARTESIAN_POINT ( 'NONE',  ( 16.21991450484859598, -11.16473453929635440, 33.15142922261926373 ) ) ;
#9236=CARTESIAN_POINT ( 'NONE',  ( 5.076923076923075762, -8.164416787775445883, 34.95778746994557906 ) ) ;
#9237=CARTESIAN_POINT ( 'NONE',  ( -20.74999999999999645, -4.499999999999999112, 27.25000000000000000 ) ) ;
#9239=CARTESIAN_POINT ( 'NONE',  ( 1.450682717965461999, -2.486705287966280320, 31.30864560766543647 ) ) ;
#9240=ADVANCED_FACE ( 'NONE', ( #74486 ), #88037, .F. ) ;
#9241=CARTESIAN_POINT ( 'NONE',  ( 8.519254025182180001, -11.47974371597207899, 33.17467449705390692 ) ) ;
#9242=CARTESIAN_POINT ( 'NONE',  ( 3.296837581771669523, -4.098570777380720287, 33.41473453929635440 ) ) ;
#9243=CARTESIAN_POINT ( 'NONE',  ( 0.3962680155776844848, -11.94971097300153140, 32.03036669348370680 ) ) ;
#9246=CARTESIAN_POINT ( 'NONE',  ( -18.24997673094235751, -6.567427716900049006, 34.66269422305636283 ) ) ;
#9247=ADVANCED_FACE ( 'NONE', ( #46127 ), #18213, .F. ) ;
#9248=CARTESIAN_POINT ( 'NONE',  ( 8.899756207464413649, -4.299079248970732792, 33.91157788607253565 ) ) ;
#9249=CARTESIAN_POINT ( 'NONE',  ( 4.284637961670940243, -12.11778462344220841, 31.66786338562085135 ) ) ;
#9251=CARTESIAN_POINT ( 'NONE',  ( -0.2385256174450666455, -8.282913670948747864, 34.94150082978203642 ) ) ;
#9252=CARTESIAN_POINT ( 'NONE',  ( -11.40766973063674961, -11.18335022499818621, 33.13157742990016885 ) ) ;
#9254=CARTESIAN_POINT ( 'NONE',  ( 0.4615384615384611200, -12.37446782046654192, 30.86335684631486131 ) ) ;
#9256=EDGE_CURVE ( 'NONE', #10196, #26718, #87993, .T. ) ;
#9257=ORIENTED_EDGE ( 'NONE', *, *, #51248, .T. ) ;
#9259=EDGE_LOOP ( 'NONE', ( #42412, #73949 ) ) ;
#9260=DIRECTION ( 'NONE',  ( -0.000000000000000000, 0.1736481776669307198, -0.9848077530122080203 ) ) ;
#9261=ORIENTED_EDGE ( 'NONE', *, *, #58675, .T. ) ;
#9263=ORIENTED_EDGE ( 'NONE', *, *, #8452, .F. ) ;
#9264=CARTESIAN_POINT ( 'NONE',  ( -16.15384615384615330, -1.367168528481310208, 33.57946703557072254 ) ) ;
#9266=CARTESIAN_POINT ( 'NONE',  ( 7.846153846153723244, -8.656820664282941280, 34.87096338111179961 ) ) ;
#9267=CARTESIAN_POINT ( 'NONE',  ( -3.165514091256390827, -12.51329471203373700, 31.30864560766537963 ) ) ;
#9268=CARTESIAN_POINT ( 'NONE',  ( 17.74997677577853850, -2.341070481393820124, 30.72580821765574299 ) ) ;
#9269=VECTOR ( 'NONE', #55187, 1000.000000000000000 ) ;
#9270=DIRECTION ( 'NONE',  ( -0.000000000000000000, -1.000000000000000000, -8.673617379884033500E-16 ) ) ;
#9271=CARTESIAN_POINT ( 'NONE',  ( 1.161130460051055024, -4.988325925672468131, 34.36044203135681130 ) ) ;
#9272=DIRECTION ( 'NONE',  ( 0.000000000000000000, 0.3420201433256610524, 0.9396926207859113145 ) ) ;
#9274=CARTESIAN_POINT ( 'NONE',  ( 18.06525513951283202, -11.67786785259547777, 32.92929555188713664 ) ) ;
#9276=CARTESIAN_POINT ( 'NONE',  ( 13.60739492588379562, -4.387253974876679230, 33.66317474335728832 ) ) ;
#9278=EDGE_CURVE ( 'NONE', #9598, #57919, #11906, .T. ) ;
#9279=CARTESIAN_POINT ( 'NONE',  ( -14.05763799605399278, -10.66356715214248396, 33.62249196103329751 ) ) ;
#9280=ORIENTED_EDGE ( 'NONE', *, *, #43658, .T. ) ;
#9281=CYLINDRICAL_SURFACE ( 'NONE', #34258, 0.2499999999999995559 ) ;
#9282=CYLINDRICAL_SURFACE ( 'NONE', #44511, 0.2499999999999986955 ) ;
#9283=DIRECTION ( 'NONE',  ( -0.000000000000000000, 0.9848077530122086864, -0.1736481776669273891 ) ) ;
#9284=LINE ( 'NONE', #44819, #15362 ) ;
#9285=CARTESIAN_POINT ( 'NONE',  ( -1.608100328339332474, -10.81261337010820256, 33.49550067578627477 ) ) ;
#9287=EDGE_CURVE ( 'NONE', #52855, #86735, #59633, .T. ) ;
#9288=B_SPLINE_CURVE_WITH_KNOTS ( 'NONE', 3,
 ( #40723, #27635, #55107, #82600, #55991, #6047 ),
 .UNSPECIFIED., .F., .F.,
 ( 4, 2, 4 ),
 ( 4.336808689942017736E-19, 0.0001954784845028939555, 0.0003909569690057874774 ),
 .UNSPECIFIED. ) ;
#9289=DIRECTION ( 'NONE',  ( -0.000000000000000000, -0.1736481776669307198, -0.9848077530122080203 ) ) ;
#9290=B_SPLINE_CURVE_WITH_KNOTS ( 'NONE', 3,
 ( #50712, #51142, #86763, #2974, #11528, #11079, #72767, #4317, #51587, #30453 ),
 .UNSPECIFIED., .F., .F.,
 ( 4, 2, 2, 2, 4 ),
 ( 0.000000000000000000, 0.0001954311564186871184, 0.0003908623128373742367, 0.0005862934692560614093, 0.0007817246256747484735 ),
 .UNSPECIFIED. ) ;
#9293=EDGE_LOOP ( 'NONE', ( #82227, #30318 ) ) ;
#9294=EDGE_CURVE ( 'NONE', #63541, #69885, #63221, .T. ) ;
#9296=ORIENTED_EDGE ( 'NONE', *, *, #65655, .T. ) ;
#9297=LINE ( 'NONE', #38088, #67346 ) ;
#9298=CARTESIAN_POINT ( 'NONE',  ( 16.40384615384759215, -7.500000000000155431, 34.75000000000007105 ) ) ;
#9299=CARTESIAN_POINT ( 'NONE',  ( 1.515407192440173079, -11.71459661697925903, 32.44059661609676937 ) ) ;
#9300=CARTESIAN_POINT ( 'NONE',  ( 17.93391762063986050, -9.058645607665454236, 34.76329471203372634 ) ) ;
#9301=VERTEX_POINT ( 'NONE', #5583 ) ;
#9302=EDGE_CURVE ( 'NONE', #54584, #87771, #71843, .T. ) ;
#9304=VERTEX_POINT ( 'NONE', #155 ) ;
#9305=ORIENTED_EDGE ( 'NONE', *, *, #53256, .F. ) ;
#9306=DIRECTION ( 'NONE',  ( -0.000000000000000000, 0.8660254037844397068, -0.4999999999999978906 ) ) ;
#9307=CARTESIAN_POINT ( 'NONE',  ( 8.638539302563215116, -2.729777683071817229, 31.24903638046269450 ) ) ;
#9308=EDGE_CURVE ( 'NONE', #28968, #20065, #73920, .T. ) ;
#9309=CARTESIAN_POINT ( 'NONE',  ( -14.30769230769230660, -7.500000000000001776, 35.04278698407183867 ) ) ;
#9310=CARTESIAN_POINT ( 'NONE',  ( -3.165513659493205623, -4.481592998940250538, 33.73612834413965089 ) ) ;
#9311=ADVANCED_FACE ( 'NONE', ( #75374 ), #69939, .F. ) ;
#9312=CARTESIAN_POINT ( 'NONE',  ( -15.93106648486808119, -5.827830569534415694, 34.72679350104403539 ) ) ;
#9313=ORIENTED_EDGE ( 'NONE', *, *, #56372, .F. ) ;
#9314=ORIENTED_EDGE ( 'NONE', *, *, #48626, .F. ) ;
#9316=B_SPLINE_CURVE_WITH_KNOTS ( 'NONE', 3,
 ( #44797, #38056, #80390, #3821, #80840, #18687, #32629, #11930, #5161, #25878 ),
 .UNSPECIFIED., .F., .F.,
 ( 4, 2, 2, 2, 4 ),
 ( 0.0007817359430256361858, 0.0009771253907250041296, 0.001172514838424372182, 0.001367904286123740234, 0.001563293733823108286 ),
 .UNSPECIFIED. ) ;
#9317=ORIENTED_EDGE ( 'NONE', *, *, #8794, .F. ) ;
#9318=CARTESIAN_POINT ( 'NONE',  ( 4.284637961670941131, -11.18335022499818621, 33.13157742990016885 ) ) ;
#9319=ORIENTED_EDGE ( 'NONE', *, *, #18067, .F. ) ;
#9320=CARTESIAN_POINT ( 'NONE',  ( -7.146561866800870355, -12.44517049084099725, 30.48991314939691932 ) ) ;
#9321=LINE ( 'NONE', #49845, #66202 ) ;
#9322=CARTESIAN_POINT ( 'NONE',  ( 7.173022441425066731, -11.86320923018887541, 32.19269448109604781 ) ) ;
#9323=EDGE_LOOP ( 'NONE', ( #79209, #45554 ) ) ;
#9326=CARTESIAN_POINT ( 'NONE',  ( 15.23076923076911093, -10.90142922262034020, 33.41473453929536674 ) ) ;
#9327=CARTESIAN_POINT ( 'NONE',  ( 14.98074600654777200, -2.588893531581426988, 31.60682220781847818 ) ) ;
#9329=FACE_BOUND ( 'NONE', #17510, .T. ) ;
#9330=CARTESIAN_POINT ( 'NONE',  ( -11.53846153846166089, -11.67786785259630911, 32.92929555188603530 ) ) ;
#9331=LINE ( 'NONE', #64244, #34289 ) ;
#9334=CARTESIAN_POINT ( 'NONE',  ( -1.384615384615505151, -6.026961402154118908, 34.52809138561165270 ) ) ;
#9335=CARTESIAN_POINT ( 'NONE',  ( 4.853438133199127869, -2.599994579823202923, 30.74605699353653776 ) ) ;
#9336=CARTESIAN_POINT ( 'NONE',  ( -15.90379184220783948, -9.148310452688871663, 34.47095581063188519 ) ) ;
#9337=VERTEX_POINT ( 'NONE', #62286 ) ;
#9338=CARTESIAN_POINT ( 'NONE',  ( -11.28851602011339672, -4.336752205174649433, 33.62275283266504289 ) ) ;
#9339=EDGE_CURVE ( 'NONE', #47459, #60558, #35313, .T. ) ;
#9340=ORIENTED_EDGE ( 'NONE', *, *, #53723, .F. ) ;
#9341=CARTESIAN_POINT ( 'NONE',  ( 6.988332494352946789, -2.892918686051625166, 31.69288490824025928 ) ) ;
#9342=CARTESIAN_POINT ( 'NONE',  ( 17.01165307636676260, -11.06231777344662959, 33.60647404775220082 ) ) ;
#9343=CYLINDRICAL_SURFACE ( 'NONE', #6576, 0.2500000000000002220 ) ;
#9344=CARTESIAN_POINT ( 'NONE',  ( -7.623141002060451754, -10.77377354290276301, 33.85451476688484718 ) ) ;
#9345=CARTESIAN_POINT ( 'NONE',  ( 18.00000000000000000, -1.117168528481311540, 33.14645433367849847 ) ) ;
#9346=EDGE_CURVE ( 'NONE', #5967, #60430, #80464, .T. ) ;
#9348=EDGE_CURVE ( 'NONE', #80176, #84519, #54597, .T. ) ;
#9350=FACE_BOUND ( 'NONE', #23606, .T. ) ;
#9351=CARTESIAN_POINT ( 'NONE',  ( -1.607542343522232464, -6.459968553980839800, 34.89616026154728701 ) ) ;
#9352=CYLINDRICAL_SURFACE ( 'NONE', #74764, 0.2499999999999995559 ) ;
#9353=CARTESIAN_POINT ( 'NONE',  ( -18.24997674404858827, -8.347322224742352859, 34.93158281831414058 ) ) ;
#9354=CARTESIAN_POINT ( 'NONE',  ( -3.230769230769229949, -1.466349020453238561, 30.81389545987213907 ) ) ;
#9356=CARTESIAN_POINT ( 'NONE',  ( -3.230769230769229949, -11.11383981884818262, 36.00935417666054406 ) ) ;
#9358=EDGE_LOOP ( 'NONE', ( #23435, #40477 ) ) ;
#9359=AXIS2_PLACEMENT_3D ( 'NONE', #6373, #12231, #6796 ) ;
#9360=CARTESIAN_POINT ( 'NONE',  ( -4.219116599806927326, -11.94971097300153140, 32.03036669348370680 ) ) ;
#9361=B_SPLINE_CURVE_WITH_KNOTS ( 'NONE', 3,
 ( #75923, #41257, #62828, #56093, #41695, #27292, #42588, #70047, #82694, #21422 ),
 .UNSPECIFIED., .F., .F.,
 ( 4, 2, 2, 2, 4 ),
 ( 0.0007817246256747448956, 0.0009771112852218876831, 0.001172497944769030579, 0.001367884604316173475, 0.001563271263863316371 ),
 .UNSPECIFIED. ) ;
#9362=CYLINDRICAL_SURFACE ( 'NONE', #45516, 0.2500000000000008882 ) ;
#9363=CARTESIAN_POINT ( 'NONE',  ( -9.626239341305254271, -8.973038597847271092, 34.52809138561121216 ) ) ;
#9365=CARTESIAN_POINT ( 'NONE',  ( -4.376773112753001627, -4.762599654559228846, 34.23009711892697737 ) ) ;
#9367=CARTESIAN_POINT ( 'NONE',  ( -2.307692307692305711, -3.322132147404559976, 32.92929555188717927 ) ) ;
#9368=CARTESIAN_POINT ( 'NONE',  ( -8.769230769230768274, -6.386643153685126251, 34.62446782046654192 ) ) ;
#9369=CARTESIAN_POINT ( 'NONE',  ( -16.85414353565466072, -5.913360116392398780, 34.49180327182771322 ) ) ;
#9370=CARTESIAN_POINT ( 'NONE',  ( -11.53846153846153655, -9.584722331328613620, 36.20867863119891439 ) ) ;
#9371=CARTESIAN_POINT ( 'NONE',  ( 2.557692307692308376, -2.249999999999998668, 29.75000000000000355 ) ) ;
#9372=CARTESIAN_POINT ( 'NONE',  ( 4.023698944407932743, -10.88202310037935661, 33.43294751532457099 ) ) ;
#9374=CARTESIAN_POINT ( 'NONE',  ( 8.068933387422251968, -6.760870238392817200, 34.69528174975672385 ) ) ;
#9376=CARTESIAN_POINT ( 'NONE',  ( 7.846153846153846700, -13.04860791097971706, 34.73218667398347037 ) ) ;
#9377=CARTESIAN_POINT ( 'NONE',  ( 7.145856464345331283, -5.114059244376869984, 34.14424750095245287 ) ) ;
#9379=CYLINDRICAL_SURFACE ( 'NONE', #70605, 0.2500000000000012212 ) ;
#9380=DIRECTION ( 'NONE',  ( -0.000000000000000000, 0.3420201433256694346, -0.9396926207859080948 ) ) ;
#9381=ORIENTED_EDGE ( 'NONE', *, *, #7602, .F. ) ;
#9382=CARTESIAN_POINT ( 'NONE',  ( -16.40386937806761125, -4.175268141568689195, 33.81360843649122216 ) ) ;
#9383=CARTESIAN_POINT ( 'NONE',  ( 7.596177115211490083, -2.564618984488975961, 30.55390908950641915 ) ) ;
#9385=DIRECTION ( 'NONE',  ( -0.000000000000000000, 0.8660254037844399289, -0.4999999999999980016 ) ) ;
#9386=CARTESIAN_POINT ( 'NONE',  ( 3.930919936330006248, -8.239355502252617924, 34.69524867566427417 ) ) ;
#9387=FACE_OUTER_BOUND ( 'NONE', #19600, .T. ) ;
#9388=AXIS2_PLACEMENT_3D ( 'NONE', #60419, #19437, #26196 ) ;
#9389=CARTESIAN_POINT ( 'NONE',  ( -15.29601916254331329, -2.255955759149247619, 30.00000000000013856 ) ) ;
#9392=CARTESIAN_POINT ( 'NONE',  ( 5.142116065217731347, -2.255955759149235629, 29.99999999999988631 ) ) ;
#9393=B_SPLINE_CURVE_WITH_KNOTS ( 'NONE', 3,
 ( #80842, #10142, #37606, #79041, #52002, #11932, #44799, #58768, #73640, #73182 ),
 .UNSPECIFIED., .F., .F.,
 ( 4, 2, 2, 2, 4 ),
 ( 0.000000000000000000, 0.0001954311564186879044, 0.0003908623128373758088, 0.0005862934692560636861, 0.0007817246256747516176 ),
 .UNSPECIFIED. ) ;
#9394=CARTESIAN_POINT ( 'NONE',  ( 12.59232890250541281, -11.93129842949671726, 32.56571108434900452 ) ) ;
#9396=ORIENTED_EDGE ( 'NONE', *, *, #65193, .F. ) ;
#9397=B_SPLINE_CURVE_WITH_KNOTS ( 'NONE', 3,
 ( #16254, #43719, #56356, #64419, #22128, #2719, #77074, #15379, #10832, #18037 ),
 .UNSPECIFIED., .F., .F.,
 ( 4, 2, 2, 2, 4 ),
 ( 0.000000000000000000, 0.0001954311564186868744, 0.0003908623128373737488, 0.0005862934692560606504, 0.0007817246256747474977 ),
 .UNSPECIFIED. ) ;
#9398=ORIENTED_EDGE ( 'NONE', *, *, #18684, .T. ) ;
#9399=CARTESIAN_POINT ( 'NONE',  ( -17.07692307692307665, -8.973038597847269315, 34.52809138561121927 ) ) ;
#9401=CARTESIAN_POINT ( 'NONE',  ( -7.715315428141081178, -7.277220443632450575, 34.74524770363008486 ) ) ;
#9402=CARTESIAN_POINT ( 'NONE',  ( 15.48076923076923173, -2.499999999999998668, 29.75000000000000355 ) ) ;
#9403=AXIS2_PLACEMENT_3D ( 'NONE', #3566, #31035, #25182 ) ;
#9405=EDGE_LOOP ( 'NONE', ( #51700, #32936 ) ) ;
#9406=CARTESIAN_POINT ( 'NONE',  ( 12.46153846153846168, -1.117168528481311540, 33.14645433367849847 ) ) ;
#9408=CARTESIAN_POINT ( 'NONE',  ( 17.20744877868664346, -5.195472089885680766, 34.18748526763464923 ) ) ;
#9409=EDGE_CURVE ( 'NONE', #72081, #86292, #54640, .T. ) ;
#9410=CARTESIAN_POINT ( 'NONE',  ( -17.77698864838715309, -3.105924265160264319, 32.13625925475356127 ) ) ;
#9411=CARTESIAN_POINT ( 'NONE',  ( -7.976844449264155479, -9.929715669179220328, 34.40415004197138416 ) ) ;
#9414=ORIENTED_EDGE ( 'NONE', *, *, #57036, .F. ) ;
#9415=CARTESIAN_POINT ( 'NONE',  ( -6.673131404728780858, -11.37275283266503756, 32.91324779482534524 ) ) ;
#9416=ORIENTED_EDGE ( 'NONE', *, *, #20713, .T. ) ;
#9417=CARTESIAN_POINT ( 'NONE',  ( -0.5922299282060183856, -10.54014554554150607, 33.71984207302941883 ) ) ;
#9418=CARTESIAN_POINT ( 'NONE',  ( -5.299849294439224145, -9.886141570436013382, 34.14413921362392301 ) ) ;
#9420=ADVANCED_FACE ( 'NONE', ( #49231 ), #13668, .F. ) ;
#9421=CARTESIAN_POINT ( 'NONE',  ( 15.16549923021291058, -2.379036618887870436, 30.90682066428147934 ) ) ;
#9423=DIRECTION ( 'NONE',  ( -0.000000000000000000, 0.6427876096865404731, -0.7660444431189771253 ) ) ;
#9424=FACE_BOUND ( 'NONE', #21190, .T. ) ;
#9425=CARTESIAN_POINT ( 'NONE',  ( 1.384615384615265343, -12.46129190930018460, 30.37095296980731973 ) ) ;
#9426=CARTESIAN_POINT ( 'NONE',  ( -4.403869391139119571, -12.22074536777954989, 31.39888409691088356 ) ) ;
#9427=CARTESIAN_POINT ( 'NONE',  ( 8.638539302563209787, -2.541943142973491554, 30.39792223712631980 ) ) ;
#9428=CARTESIAN_POINT ( 'NONE',  ( -0.2385256174450665345, -2.889357225399415086, 32.26129605718031712 ) ) ;
#9432=CARTESIAN_POINT ( 'NONE',  ( -16.28453675695646652, -2.494641256782729855, 31.33461815524612959 ) ) ;
#9434=CARTESIAN_POINT ( 'NONE',  ( -16.08777882049607655, -3.322132147404559532, 32.92929555188717927 ) ) ;
#9436=ORIENTED_EDGE ( 'NONE', *, *, #71167, .F. ) ;
#9437=VECTOR ( 'NONE', #74971, 1000.000000000000000 ) ;
#9439=DIRECTION ( 'NONE',  ( -0.000000000000000000, -0.5000000000000009992, -0.8660254037844380415 ) ) ;
#9440=CARTESIAN_POINT ( 'NONE',  ( 13.16113046005105858, -11.60425143139329940, 33.02411095842164457 ) ) ;
#9441=CARTESIAN_POINT ( 'NONE',  ( 20.74999999999999645, -10.50000000000000000, 27.25000000000000000 ) ) ;
#9443=CARTESIAN_POINT ( 'NONE',  ( 14.30769230769218581, -11.67786785259630911, 32.92929555188603530 ) ) ;
#9444=ORIENTED_EDGE ( 'NONE', *, *, #7212, .F. ) ;
#9445=EDGE_CURVE ( 'NONE', #39542, #17339, #67550, .T. ) ;
#9447=CARTESIAN_POINT ( 'NONE',  ( 6.923076923076924238, -3.513871655860378418, 32.76840700105978499 ) ) ;
#9449=CARTESIAN_POINT ( 'NONE',  ( -17.07692307692307665, -10.51840700105979565, 33.73612834413961536 ) ) ;
#9450=CARTESIAN_POINT ( 'NONE',  ( 12.46153846153846168, -12.78798330534102945, 29.74999999999997868 ) ) ;
#9452=ORIENTED_EDGE ( 'NONE', *, *, #85914, .F. ) ;
#9453=EDGE_LOOP ( 'NONE', ( #58901, #45691 ) ) ;
#9455=CARTESIAN_POINT ( 'NONE',  ( 14.08420738312797482, -12.47654668319379567, 31.42292124445336654 ) ) ;
#9457=CARTESIAN_POINT ( 'NONE',  ( -7.173100160369888734, -2.587272538249754117, 30.68239716806877837 ) ) ;
#9458=CARTESIAN_POINT ( 'NONE',  ( 18.00000000000000000, -5.557115091759785130, 34.35708131394839171 ) ) ;
#9460=CARTESIAN_POINT ( 'NONE',  ( -8.638705067467205012, -10.88167719472716399, 33.43325721877153711 ) ) ;
#9462=CARTESIAN_POINT ( 'NONE',  ( 0.7114838709165042241, -9.357781135181031829, 34.66075350412533851 ) ) ;
#9464=CARTESIAN_POINT ( 'NONE',  ( 4.377273115707725815, -7.630147231320743018, 34.74852402298682819 ) ) ;
#9465=CARTESIAN_POINT ( 'NONE',  ( -2.176901866725356349, -12.62708834333097663, 30.88030960425257021 ) ) ;
#9466=ORIENTED_EDGE ( 'NONE', *, *, #20584, .F. ) ;
#9467=DIRECTION ( 'NONE',  ( 0.000000000000000000, 0.000000000000000000, 1.000000000000000000 ) ) ;
#9468=DIRECTION ( 'NONE',  ( 0.000000000000000000, 0.6427876096865368094, 0.7660444431189802339 ) ) ;
#9469=CARTESIAN_POINT ( 'NONE',  ( -3.453695448285377001, -4.887634598454295265, 34.01352882383564946 ) ) ;
#9470=CARTESIAN_POINT ( 'NONE',  ( 11.78840694783958298, -8.476813868363244353, 34.90874843262270133 ) ) ;
#9471=CARTESIAN_POINT ( 'NONE',  ( -3.361244415844949263, -7.276987145209184327, 34.99546412871779211 ) ) ;
#9472=CARTESIAN_POINT ( 'NONE',  ( -7.146561866800870355, -5.113361153441932316, 34.14387501736621999 ) ) ;
#9474=ORIENTED_EDGE ( 'NONE', *, *, #29009, .T. ) ;
#9475=CARTESIAN_POINT ( 'NONE',  ( -12.52686247434276900, -7.749976730030849303, 34.74374725381503737 ) ) ;
#9476=DIRECTION ( 'NONE',  ( -0.000000000000000000, -0.6427876096865404731, -0.7660444431189770143 ) ) ;
#9478=CARTESIAN_POINT ( 'NONE',  ( 0.4615384615383396616, -3.835265460704628371, 33.15142922262033665 ) ) ;
#9479=CARTESIAN_POINT ( 'NONE',  ( 9.692307692307695177, -6.343179335718451384, 34.87096338111211935 ) ) ;
#9480=EDGE_LOOP ( 'NONE', ( #36003, #61646, #82215, #45761 ) ) ;
#9481=DIRECTION ( 'NONE',  ( 0.000000000000000000, 0.6427876096865373645, -0.7660444431189797898 ) ) ;
#9482=CARTESIAN_POINT ( 'NONE',  ( 3.100622021331010725, -9.418419913701741919, 34.36755862841477693 ) ) ;
#9484=ORIENTED_EDGE ( 'NONE', *, *, #40138, .F. ) ;
#9485=CARTESIAN_POINT ( 'NONE',  ( -4.219116154402471786, -8.656820664281497102, 34.87096338111211935 ) ) ;
#9486=VERTEX_POINT ( 'NONE', #51404 ) ;
#9488=CARTESIAN_POINT ( 'NONE',  ( 4.023698944407931855, -3.817052484675422797, 33.13202310037935661 ) ) ;
#9489=CARTESIAN_POINT ( 'NONE',  ( -12.52762084089859407, -9.905515769479276145, 34.41647553114623292 ) ) ;
#9491=VERTEX_POINT ( 'NONE', #44663 ) ;
#9492=CARTESIAN_POINT ( 'NONE',  ( -6.857009589726848375, -6.343179335718452272, 34.87096338111212646 ) ) ;
#9493=ORIENTED_EDGE ( 'NONE', *, *, #84815, .T. ) ;
#9494=CARTESIAN_POINT ( 'NONE',  ( -1.384615384615506484, -11.67786785259630911, 32.92929555188603530 ) ) ;
#9495=CARTESIAN_POINT ( 'NONE',  ( -4.219602956360462009, -7.249945686854186278, 34.74374336980224598 ) ) ;
#9496=EDGE_LOOP ( 'NONE', ( #55832, #16505 ) ) ;
#9497=CARTESIAN_POINT ( 'NONE',  ( -5.869208192175211281, -11.18335022499818621, 33.13157742990016885 ) ) ;
#9498=CARTESIAN_POINT ( 'NONE',  ( 10.61538461538461675, -3.050289026998446396, 32.03036669348365706 ) ) ;
#9499=CARTESIAN_POINT ( 'NONE',  ( -3.903846153846152855, -2.499999999999998668, 29.75000000000000355 ) ) ;
#9500=ADVANCED_FACE ( 'NONE', ( #30286 ), #29846, .F. ) ;
#9501=CARTESIAN_POINT ( 'NONE',  ( -11.31544869436814160, -5.582272713120729257, 34.63742843783360570 ) ) ;
#9502=DIRECTION ( 'NONE',  ( 0.000000000000000000, -6.938893903907222067E-15, 1.000000000000000000 ) ) ;
#9503=ORIENTED_EDGE ( 'NONE', *, *, #88754, .T. ) ;
#9504=ORIENTED_EDGE ( 'NONE', *, *, #23915, .T. ) ;
#9505=FACE_BOUND ( 'NONE', #45109, .T. ) ;
#9507=CARTESIAN_POINT ( 'NONE',  ( -7.846153846153844924, -5.471508081941601098, 34.59228464037088457 ) ) ;
#9508=B_SPLINE_CURVE_WITH_KNOTS ( 'NONE', 3,
 ( #83220, #48085, #6236, #49429, #48525, #21504, #76903, #82782, #6664, #62051 ),
 .UNSPECIFIED., .F., .F.,
 ( 4, 2, 2, 2, 4 ),
 ( 0.000000000000000000, 0.0001954339857564058210, 0.0003908679715128116419, 0.0005863019572692174629, 0.0007817359430256232838 ),
 .UNSPECIFIED. ) ;
#9509=ADVANCED_FACE ( 'NONE', ( #36172 ), #44216, .F. ) ;
#9510=CARTESIAN_POINT ( 'NONE',  ( 13.60739492588379385, -10.81320215134717344, 33.49497208177562868 ) ) ;
#9511=CARTESIAN_POINT ( 'NONE',  ( -14.08491276642389423, -9.332535724633409302, 34.40230450496446934 ) ) ;
#9512=B_SPLINE_CURVE_WITH_KNOTS ( 'NONE', 3,
 ( #6296, #12163, #73419, #39646, #13045, #73866, #32425, #33323, #74306, #60781 ),
 .UNSPECIFIED., .F., .F.,
 ( 4, 2, 2, 2, 4 ),
 ( 0.0007817359430256400890, 0.0009771253907250091169, 0.001172514838424378253, 0.001367904286123747173, 0.001563293733823116309 ),
 .UNSPECIFIED. ) ;
#9514=ORIENTED_EDGE ( 'NONE', *, *, #38418, .F. ) ;
#9515=ORIENTED_EDGE ( 'NONE', *, *, #19062, .T. ) ;
#9516=CARTESIAN_POINT ( 'NONE',  ( 0.2115152373170033073, -8.475808217655753651, 34.90892951860618609 ) ) ;
#9517=ORIENTED_EDGE ( 'NONE', *, *, #38313, .F. ) ;
#9518=CARTESIAN_POINT ( 'NONE',  ( 2.530703659305157949, -4.187068189119697692, 33.49521262558774026 ) ) ;
#9520=ADVANCED_FACE ( 'NONE', ( #63624 ), #50970, .F. ) ;
#9521=CARTESIAN_POINT ( 'NONE',  ( -6.923076923076922462, -1.790695186598648903, 34.54067556320373455 ) ) ;
#9522=CARTESIAN_POINT ( 'NONE',  ( 16.82689985270161870, -3.520140089381496473, 33.17453946501458262 ) ) ;
#9523=FACE_BOUND ( 'NONE', #57756, .T. ) ;
#9524=ORIENTED_EDGE ( 'NONE', *, *, #87657, .T. ) ;
#9525=LINE ( 'NONE', #36991, #77361 ) ;
#9526=ADVANCED_FACE ( 'NONE', ( #64060 ), #43793, .F. ) ;
#9528=CARTESIAN_POINT ( 'NONE',  ( 2.084207383127978375, -8.539481045369598178, 34.89627647299170832 ) ) ;
#9530=ORIENTED_EDGE ( 'NONE', *, *, #10202, .F. ) ;
#9531=VECTOR ( 'NONE', #85157, 1000.000000000000000 ) ;
#9532=PRODUCT_DEFINITION_CONTEXT ( 'detailed design', #39452, 'design' ) ;
#9533=VERTEX_POINT ( 'NONE', #37473 ) ;
#9534=ORIENTED_EDGE ( 'NONE', *, *, #47043, .F. ) ;
#9535=CARTESIAN_POINT ( 'NONE',  ( 12.39626801557768943, -6.879047030191174805, 34.71129190930000163 ) ) ;
#9536=CARTESIAN_POINT ( 'NONE',  ( 5.749976762707036393, -3.202444869320336451, 32.30641848906366675 ) ) ;
#9537=FACE_OUTER_BOUND ( 'NONE', #50183, .T. ) ;
#9538=DIRECTION ( 'NONE',  ( -0.000000000000000000, -0.6427876096865404731, -0.7660444431189771253 ) ) ;
#9539=CARTESIAN_POINT ( 'NONE',  ( 7.622668902429898807, -12.44517049084099725, 30.48991314939691932 ) ) ;
#9540=CARTESIAN_POINT ( 'NONE',  ( -11.53846153846166089, -2.379036618888197729, 30.90682066428292885 ) ) ;
#9541=VERTEX_POINT ( 'NONE', #2353 ) ;
#9542=EDGE_CURVE ( 'NONE', #4699, #73779, #85723, .T. ) ;
#9544=B_SPLINE_CURVE_WITH_KNOTS ( 'NONE', 3,
 ( #46573, #68180, #61402, #80824, #60970, #74057, #33945, #41591, #54205, #68617 ),
 .UNSPECIFIED., .F., .F.,
 ( 4, 2, 2, 2, 4 ),
 ( 0.0007817359430256324996, 0.0009771253907249993591, 0.001172514838424366110, 0.001367904286123732861, 0.001563293733823099829 ),
 .UNSPECIFIED. ) ;
#9545=CARTESIAN_POINT ( 'NONE',  ( 17.86985203026830504, -3.625366637846545448, 33.29286588640298561 ) ) ;
#9547=EDGE_CURVE ( 'NONE', #55800, #68993, #84777, .T. ) ;
#9548=CARTESIAN_POINT ( 'NONE',  ( 3.296836564119307589, -11.35647404775217595, 33.31231777344667222 ) ) ;
#9549=EDGE_LOOP ( 'NONE', ( #86115, #45046 ) ) ;
#9551=VERTEX_POINT ( 'NONE', #77588 ) ;
#9552=FACE_BOUND ( 'NONE', #73019, .T. ) ;
#9553=EDGE_CURVE ( 'NONE', #83933, #73212, #9966, .T. ) ;
#9554=CARTESIAN_POINT ( 'NONE',  ( -17.07692307692307665, -1.242168528481310874, 33.36296068462461051 ) ) ;
#9555=CARTESIAN_POINT ( 'NONE',  ( 14.08420736396836226, -11.89387501736622710, 32.13663884655806413 ) ) ;
#9556=EDGE_CURVE ( 'NONE', #18984, #30445, #38374, .T. ) ;
#9557=ORIENTED_EDGE ( 'NONE', *, *, #22267, .F. ) ;
#9558=CARTESIAN_POINT ( 'NONE',  ( -16.15384615384627409, -11.67786785259630911, 32.92929555188603530 ) ) ;
#9559=CARTESIAN_POINT ( 'NONE',  ( -16.15384615384615330, -12.48256725967547354, 35.29906147534542527 ) ) ;
#9561=DIRECTION ( 'NONE',  ( -0.000000000000000000, 0.9848077530122085754, -0.1736481776669273613 ) ) ;
#9562=ORIENTED_EDGE ( 'NONE', *, *, #69703, .T. ) ;
#9563=VECTOR ( 'NONE', #86806, 1000.000000000000227 ) ;
#9564=CARTESIAN_POINT ( 'NONE',  ( -7.715628144390283438, -10.88167719472716399, 33.43325721877153711 ) ) ;
#9565=VERTEX_POINT ( 'NONE', #66733 ) ;
#9566=CARTESIAN_POINT ( 'NONE',  ( 13.63466969625370595, -12.17597550085003810, 31.52189283813460463 ) ) ;
#9567=EDGE_LOOP ( 'NONE', ( #84097, #52609, #81694, #30604 ) ) ;
#9568=CARTESIAN_POINT ( 'NONE',  ( -18.25000000000000000, -12.75000000000000888, 29.74999999999997868 ) ) ;
#9569=CARTESIAN_POINT ( 'NONE',  ( -12.46153846153858424, -3.083524468854526912, 32.58852847137268327 ) ) ;
#9570=DIRECTION ( 'NONE',  ( -0.000000000000000000, -0.7660444431189791237, -0.6427876096865379196 ) ) ;
#9571=CARTESIAN_POINT ( 'NONE',  ( -15.00734283185444440, -7.630147987733840509, 34.99859428049665411 ) ) ;
#9572=DIRECTION ( 'NONE',  ( -0.000000000000000000, 1.000000000000000000, 3.491481338843133355E-15 ) ) ;
#9574=CARTESIAN_POINT ( 'NONE',  ( 12.23805353697412990, -5.827078755546623690, 34.72654668319379567 ) ) ;
#9576=VERTEX_POINT ( 'NONE', #11798 ) ;
#9577=CARTESIAN_POINT ( 'NONE',  ( 13.44987052412822059, -12.70778746994558439, 30.41441678777536595 ) ) ;
#9578=CARTESIAN_POINT ( 'NONE',  ( 13.45078199120703033, -7.250054591869670162, 34.99404684341514127 ) ) ;
#9579=VERTEX_POINT ( 'NONE', #52319 ) ;
#9580=EDGE_LOOP ( 'NONE', ( #56855, #52321 ) ) ;
#9581=ORIENTED_EDGE ( 'NONE', *, *, #11760, .T. ) ;
#9582=CARTESIAN_POINT ( 'NONE',  ( 13.38461538461526423, -11.06231777344772027, 33.60647404775119895 ) ) ;
#9583=CARTESIAN_POINT ( 'NONE',  ( 11.40831356872984514, -5.070767119584671079, 34.40440758774516183 ) ) ;
#9584=CARTESIAN_POINT ( 'NONE',  ( -17.14219352288385778, -9.442884908240170461, 34.35708131394840592 ) ) ;
#9585=CARTESIAN_POINT ( 'NONE',  ( -3.230769230769229949, -7.500000000000001776, 35.04278698407183867 ) ) ;
#9586=CARTESIAN_POINT ( 'NONE',  ( 8.769230769230768274, -2.292212530054420494, 30.41441678777542634 ) ) ;
#9588=CARTESIAN_POINT ( 'NONE',  ( 5.777120483262417672, -7.630690623152302621, 34.99857592706774057 ) ) ;
#9589=B_SPLINE_CURVE_WITH_KNOTS ( 'NONE', 3,
 ( #27439, #13916, #41398, #68860, #9383, #71958, #8942, #36414, #30093, #23324 ),
 .UNSPECIFIED., .F., .F.,
 ( 4, 2, 2, 2, 4 ),
 ( 0.000000000000000000, 0.0001954339857564100765, 0.0003908679715128201529, 0.0005863019572692302565, 0.0007817359430256403058 ),
 .UNSPECIFIED. ) ;
#9590=ORIENTED_EDGE ( 'NONE', *, *, #48894, .F. ) ;
#9591=EDGE_CURVE ( 'NONE', #68628, #52889, #18084, .T. ) ;
#9592=AXIS2_PLACEMENT_3D ( 'NONE', #37707, #3473, #44447 ) ;
#9593=CARTESIAN_POINT ( 'NONE',  ( -4.153846153846152411, -5.557115091759785130, 34.35708131394839171 ) ) ;
#9594=CARTESIAN_POINT ( 'NONE',  ( -1.384615384615505151, -6.879047030192662504, 34.71129190930017927 ) ) ;
#9596=CARTESIAN_POINT ( 'NONE',  ( 7.912222197156285830, -2.721908614388772740, 31.22303859784725333 ) ) ;
#9597=ADVANCED_FACE ( 'NONE', ( #32498 ), #24849, .F. ) ;
#9598=VERTEX_POINT ( 'NONE', #24401 ) ;
#9599=CARTESIAN_POINT ( 'NONE',  ( 7.622668921589514035, -2.353723527008296124, 30.78948104536958397 ) ) ;
#9600=EDGE_CURVE ( 'NONE', #23257, #20836, #42825, .T. ) ;
#9601=EDGE_LOOP ( 'NONE', ( #4474, #3190, #71046, #5881 ) ) ;
#9602=CARTESIAN_POINT ( 'NONE',  ( -17.75005459062195712, -8.476813868363244353, 34.90874843262270133 ) ) ;
#9603=DIRECTION ( 'NONE',  ( -0.000000000000000000, 0.7660444431189791237, -0.6427876096865379196 ) ) ;
#9604=CARTESIAN_POINT ( 'NONE',  ( 11.53846153846153832, -9.780366693483667717, 34.19971097300155094 ) ) ;
#9605=CARTESIAN_POINT ( 'NONE',  ( 12.46153846153846168, -10.51840700105979565, 33.73612834413961536 ) ) ;
#9606=ORIENTED_EDGE ( 'NONE', *, *, #32741, .T. ) ;
#9607=AXIS2_PLACEMENT_3D ( 'NONE', #72077, #31991, #10384 ) ;
#9608=CARTESIAN_POINT ( 'NONE',  ( 15.23076923076923173, -2.499999999999998668, 29.50000000000001066 ) ) ;
#9609=DIRECTION ( 'NONE',  ( 0.000000000000000000, 0.8660254037844377084, -0.5000000000000015543 ) ) ;
#9610=CARTESIAN_POINT ( 'NONE',  ( -17.32692307692308376, -2.499999999999999556, 29.81609845454691765 ) ) ;
#9611=EDGE_CURVE ( 'NONE', #75299, #63322, #32953, .T. ) ;
#9612=FACE_OUTER_BOUND ( 'NONE', #818, .T. ) ;
#9613=EDGE_LOOP ( 'NONE', ( #23989, #1927, #40536, #47332 ) ) ;
#9614=CARTESIAN_POINT ( 'NONE',  ( 7.622668921589515811, -11.60425143139329940, 33.02411095842164457 ) ) ;
#9616=CARTESIAN_POINT ( 'NONE',  ( 12.46153846153846168, -9.819645486525091727, 36.12317359536749706 ) ) ;
#9617=DIRECTION ( 'NONE',  ( -0.000000000000000000, 0.1736481776669307198, -0.9848077530122080203 ) ) ;
#9618=CARTESIAN_POINT ( 'NONE',  ( -13.38461538461538325, -10.67929555188718282, 33.92786785259544047 ) ) ;
#9619=CARTESIAN_POINT ( 'NONE',  ( -14.24243673641628050, -11.94971097300157403, 32.03036669348361443 ) ) ;
#9620=DIRECTION ( 'NONE',  ( 0.000000000000000000, 0.000000000000000000, 1.000000000000000000 ) ) ;
#9621=ADVANCED_FACE ( 'NONE', ( #25304 ), #67629, .F. ) ;
#9622=AXIS2_PLACEMENT_3D ( 'NONE', #35622, #70287, #76148 ) ;
#9624=B_SPLINE_CURVE_WITH_KNOTS ( 'NONE', 3,
 ( #87802, #13441, #5803, #13002, #54421, #48541, #32830, #7132, #88247, #20638 ),
 .UNSPECIFIED., .F., .F.,
 ( 4, 2, 2, 2, 4 ),
 ( 0.000000000000000000, 0.0001954311564186876063, 0.0003908623128373752125, 0.0005862934692560628188, 0.0007817246256747504250 ),
 .UNSPECIFIED. ) ;
#9625=ORIENTED_EDGE ( 'NONE', *, *, #18792, .F. ) ;
#9626=EDGE_LOOP ( 'NONE', ( #60849, #76752, #77419, #67362 ) ) ;
#9627=VECTOR ( 'NONE', #25212, 1000.000000000000227 ) ;
#9628=CARTESIAN_POINT ( 'NONE',  ( -10.39237326377176451, -8.239487800360276282, 34.69522927552633718 ) ) ;
#9629=CARTESIAN_POINT ( 'NONE',  ( 11.31553457955468645, -9.172386477786396597, 34.72672124145550043 ) ) ;
#9630=DIRECTION ( 'NONE',  ( -0.000000000000000000, 0.6427876096865404731, -0.7660444431189771253 ) ) ;
#9631=CARTESIAN_POINT ( 'NONE',  ( -12.21148404162501144, -12.41089969410671223, 31.60739465890703670 ) ) ;
#9633=CARTESIAN_POINT ( 'NONE',  ( 11.53846153846153832, -1.466349020453238561, 30.81389545987213907 ) ) ;
#9634=CYLINDRICAL_SURFACE ( 'NONE', #22026, 0.2500000000000002220 ) ;
#9635=CARTESIAN_POINT ( 'NONE',  ( 9.469380733400843297, -10.01117774369187252, 34.36070679894347535 ) ) ;
#9636=ORIENTED_EDGE ( 'NONE', *, *, #54217, .F. ) ;
#9637=ORIENTED_EDGE ( 'NONE', *, *, #37123, .F. ) ;
#9639=CARTESIAN_POINT ( 'NONE',  ( 11.66925197942849302, -2.494656445102012565, 31.33466734024120015 ) ) ;
#9642=CARTESIAN_POINT ( 'NONE',  ( -10.48459417441766561, -6.369690395747422684, 34.87708834333098196 ) ) ;
#9644=VECTOR ( 'NONE', #27997, 1000.000000000000227 ) ;
#9645=CARTESIAN_POINT ( 'NONE',  ( -10.68146802634049486, -11.69971097300155272, 32.46337939537587403 ) ) ;
#9646=ORIENTED_EDGE ( 'NONE', *, *, #76130, .T. ) ;
#9648=EDGE_CURVE ( 'NONE', #42418, #70591, #51864, .T. ) ;
#9649=ORIENTED_EDGE ( 'NONE', *, *, #18162, .F. ) ;
#9650=CARTESIAN_POINT ( 'NONE',  ( -11.78843828251013015, -12.01397095200674059, 32.43157075238190146 ) ) ;
#9652=ORIENTED_EDGE ( 'NONE', *, *, #1001, .T. ) ;
#9653=EDGE_CURVE ( 'NONE', #36678, #33529, #87030, .T. ) ;
#9654=FACE_BOUND ( 'NONE', #82022, .T. ) ;
#9655=FACE_OUTER_BOUND ( 'NONE', #58028, .T. ) ;
#9656=CARTESIAN_POINT ( 'NONE',  ( 16.08776274289027342, -6.386643153685125363, 34.62446782046654903 ) ) ;
#9657=ORIENTED_EDGE ( 'NONE', *, *, #80772, .F. ) ;
#9658=CARTESIAN_POINT ( 'NONE',  ( -14.30769230769230660, -8.164416787775445883, 34.95778746994557906 ) ) ;
#9659=FACE_OUTER_BOUND ( 'NONE', #60021, .T. ) ;
#9661=AXIS2_PLACEMENT_3D ( 'NONE', #88828, #27100, #74860 ) ;
#9662=CARTESIAN_POINT ( 'NONE',  ( -23.00000000000000000, -5.499999999999981348, 27.25000000000000000 ) ) ;
#9664=CARTESIAN_POINT ( 'NONE',  ( -11.76138849736838488, -4.762599654559228846, 34.23009711892697737 ) ) ;
#9667=CARTESIAN_POINT ( 'NONE',  ( -1.384615384615383471, -13.53365097954675988, 30.81389545987213552 ) ) ;
#9668=DIRECTION ( 'NONE',  ( 0.000000000000000000, -0.000000000000000000, -1.000000000000000000 ) ) ;
#9669=CARTESIAN_POINT ( 'NONE',  ( 2.242422307135988557, -12.16647553114622049, 32.15551576947930812 ) ) ;
#9670=CYLINDRICAL_SURFACE ( 'NONE', #72881, 0.2499999999999998890 ) ;
#9671=CARTESIAN_POINT ( 'NONE',  ( -0.5916864312701582973, -5.070767119584671967, 34.40440758774516183 ) ) ;
#9672=CARTESIAN_POINT ( 'NONE',  ( -4.153846153846152411, -8.564572088678739092, 35.78748833219616898 ) ) ;
#9673=CARTESIAN_POINT ( 'NONE',  ( -13.13466997523734214, -12.45601412856602686, 31.48342859153981621 ) ) ;
#9674=CARTESIAN_POINT ( 'NONE',  ( -1.608100328339330254, -2.847400154188068022, 31.58180166144859058 ) ) ;
#9675=CARTESIAN_POINT ( 'NONE',  ( 11.78851585009985570, -4.235687564193448829, 33.53795663066793509 ) ) ;
#9676=CARTESIAN_POINT ( 'NONE',  ( -1.319360245102545681, -9.528491918058460186, 34.59228464037085615 ) ) ;
#9677=CARTESIAN_POINT ( 'NONE',  ( -18.00000000000000000, -2.249999999999990674, 29.49999999999998579 ) ) ;
#9678=CARTESIAN_POINT ( 'NONE',  ( -10.61538461538473399, -8.613356846316285953, 34.62446782046622218 ) ) ;
#9680=CARTESIAN_POINT ( 'NONE',  ( -0.4615384615384611200, -13.88283147151868846, 33.14645433367849847 ) ) ;
#9682=ORIENTED_EDGE ( 'NONE', *, *, #60650, .F. ) ;
#9683=CARTESIAN_POINT ( 'NONE',  ( 9.692307692307695177, -5.415277668671390821, 36.20867863119892149 ) ) ;
#9685=CARTESIAN_POINT ( 'NONE',  ( -9.757578138268467427, -6.026961402152685388, 34.52809138561120506 ) ) ;
#9686=EDGE_CURVE ( 'NONE', #25656, #50820, #11343, .T. ) ;
#9688=CARTESIAN_POINT ( 'NONE',  ( 16.08776274289027342, -11.16473453929635440, 33.15142922261925662 ) ) ;
#9689=ORIENTED_EDGE ( 'NONE', *, *, #15832, .F. ) ;
#9690=CARTESIAN_POINT ( 'NONE',  ( -7.976845312821408740, -5.582088688514999397, 34.36776431015576350 ) ) ;
#9692=CARTESIAN_POINT ( 'NONE',  ( 17.07692307692295586, -8.613356846316285953, 34.62446782046622218 ) ) ;
#9693=CARTESIAN_POINT ( 'NONE',  ( 6.792929713638706346, -11.47017969459903952, 32.78971311882034456 ) ) ;
#9695=CYLINDRICAL_SURFACE ( 'NONE', #36021, 0.2499999999999994726 ) ;
#9696=CYLINDRICAL_SURFACE ( 'NONE', #44635, 0.2499999999999993616 ) ;
#9697=CARTESIAN_POINT ( 'NONE',  ( 11.40777007179398339, -2.729777683071817229, 31.24903638046269450 ) ) ;
#9698=CARTESIAN_POINT ( 'NONE',  ( -14.30769230769242917, -5.094484230521993062, 34.41647553114689373 ) ) ;
#9700=ADVANCED_FACE ( 'NONE', ( #20326 ), #495, .F. ) ;
#9701=CARTESIAN_POINT ( 'NONE',  ( -11.31544869436814160, -2.523321265292115534, 31.42251411153756990 ) ) ;
#9702=DIRECTION ( 'NONE',  ( -0.000000000000000000, -0.5000000000000009992, -0.8660254037844380415 ) ) ;
#9703=CARTESIAN_POINT ( 'NONE',  ( 10.61538461538449418, -5.941354392335915335, 34.76329471203413846 ) ) ;
#9705=ADVANCED_FACE ( 'NONE', ( #33400 ), #74835, .F. ) ;
#9706=ORIENTED_EDGE ( 'NONE', *, *, #20494, .F. ) ;
#9707=LINE ( 'NONE', #79513, #50062 ) ;
#9709=CARTESIAN_POINT ( 'NONE',  ( -8.835314180186648159, -11.16473453929635440, 33.15142922261925662 ) ) ;
#9710=CARTESIAN_POINT ( 'NONE',  ( 18.06525557127601900, -10.90142922261932057, 33.41473453929631887 ) ) ;
#9711=CARTESIAN_POINT ( 'NONE',  ( 15.48076923076929212, -7.434744429011176159, 34.75000000000000711 ) ) ;
#9712=CARTESIAN_POINT ( 'NONE',  ( -10.61538461538473577, -11.06231777344772027, 33.60647404775119895 ) ) ;
#9713=EDGE_CURVE ( 'NONE', #57265, #29932, #33084, .T. ) ;
#9714=AXIS2_PLACEMENT_3D ( 'NONE', #16304, #58163, #17183 ) ;
#9715=EDGE_CURVE ( 'NONE', #54361, #1645, #13762, .T. ) ;
#9716=B_SPLINE_CURVE_WITH_KNOTS ( 'NONE', 3,
 ( #77546, #9099, #83431, #49185, #21714, #63133, #36132, #69012, #561, #43320 ),
 .UNSPECIFIED., .F., .F.,
 ( 4, 2, 2, 2, 4 ),
 ( 0.000000000000000000, 0.0001954311564186868473, 0.0003908623128373736946, 0.0005862934692560605419, 0.0007817246256747473893 ),
 .UNSPECIFIED. ) ;
#9717=B_SPLINE_CURVE_WITH_KNOTS ( 'NONE', 3,
 ( #2459, #84903, #23188, #14663, #69600, #49334, #76811, #58749, #46133, #79021 ),
 .UNSPECIFIED., .F., .F.,
 ( 4, 2, 2, 2, 4 ),
 ( 0.000000000000000000, 0.0001954311564186871455, 0.0003908623128373742909, 0.0005862934692560614093, 0.0007817246256747485819 ),
 .UNSPECIFIED. ) ;
#9718=ORIENTED_EDGE ( 'NONE', *, *, #10720, .F. ) ;
#9720=EDGE_LOOP ( 'NONE', ( #35564, #24836 ) ) ;
#9721=VECTOR ( 'NONE', #29167, 1000.000000000000000 ) ;
#9722=B_SPLINE_CURVE_WITH_KNOTS ( 'NONE', 3,
 ( #71380, #57874, #78588, #37157, #77703, #50665, #49784, #16891, #78148, #85359 ),
 .UNSPECIFIED., .F., .F.,
 ( 4, 2, 2, 2, 4 ),
 ( 0.0007817359430256257775, 0.0009771253907249909023, 0.001172514838424356136, 0.001367904286123721369, 0.001563293733823086602 ),
 .UNSPECIFIED. ) ;
#9724=CARTESIAN_POINT ( 'NONE',  ( -24.00000000000000000, -9.499999999999982236, 27.25000000000000000 ) ) ;
#9725=CARTESIAN_POINT ( 'NONE',  ( -6.923076923077045919, -5.941354392335915335, 34.76329471203413846 ) ) ;
#9726=CARTESIAN_POINT ( 'NONE',  ( 6.856994543716787405, -2.833524468853757305, 32.15551576947924417 ) ) ;
#9728=CARTESIAN_POINT ( 'NONE',  ( -8.769230769230768274, -13.04860791097971706, 34.73218667398347037 ) ) ;
#9729=CARTESIAN_POINT ( 'NONE',  ( 17.75002325595141173, -9.234221910056350069, 34.70572697212741531 ) ) ;
#9731=ORIENTED_EDGE ( 'NONE', *, *, #35752, .T. ) ;
#9732=ADVANCED_FACE ( 'NONE', ( #88805 ), #34721, .F. ) ;
#9733=CARTESIAN_POINT ( 'NONE',  ( 15.90384615384615330, -7.500000000000001776, 35.04278698407183867 ) ) ;
#9734=EDGE_LOOP ( 'NONE', ( #55932, #24020 ) ) ;
#9735=ORIENTED_EDGE ( 'NONE', *, *, #43717, .T. ) ;
#9736=CARTESIAN_POINT ( 'NONE',  ( 0.4615384615383396616, -11.94971097300221174, 32.03036669348237098 ) ) ;
#9740=CARTESIAN_POINT ( 'NONE',  ( 11.47237915910140416, -10.67929555188718460, 33.92786785259543336 ) ) ;
#9741=CARTESIAN_POINT ( 'NONE',  ( 8.068933515131908152, -12.69155399931963046, 30.53255429739157734 ) ) ;
#9742=ORIENTED_EDGE ( 'NONE', *, *, #81166, .F. ) ;
#9743=ORIENTED_EDGE ( 'NONE', *, *, #68543, .F. ) ;
#9745=B_SPLINE_CURVE_WITH_KNOTS ( 'NONE', 3,
 ( #68608, #87576, #61393, #67288, #27178, #88909, #12339, #39818, #25855, #53312 ),
 .UNSPECIFIED., .F., .F.,
 ( 4, 2, 2, 2, 4 ),
 ( 0.0007817246256747446788, 0.0009771112852218872494, 0.001172497944769029929, 0.001367884604316172391, 0.001563271263863315070 ),
 .UNSPECIFIED. ) ;
#9746=ORIENTED_EDGE ( 'NONE', *, *, #22256, .T. ) ;
#9747=CARTESIAN_POINT ( 'NONE',  ( 11.60452887181161508, -5.471508081941601098, 34.59228464037088457 ) ) ;
#9748=ORIENTED_EDGE ( 'NONE', *, *, #64096, .T. ) ;
#9749=CARTESIAN_POINT ( 'NONE',  ( 3.230769230769108269, -2.379036618888197285, 30.90682066428292885 ) ) ;
#9750=CARTESIAN_POINT ( 'NONE',  ( 11.53846153846153832, -5.557115091759785130, 34.35708131394839171 ) ) ;
#9751=B_SPLINE_CURVE_WITH_KNOTS ( 'NONE', 3,
 ( #22437, #65185, #44459, #63417, #15689, #17457, #43155, #56666, #49901, #10259 ),
 .UNSPECIFIED., .F., .F.,
 ( 4, 2, 2, 2, 4 ),
 ( 0.000000000000000000, 0.0001954339857564074473, 0.0003908679715128148945, 0.0005863019572692223418, 0.0007817359430256297891 ),
 .UNSPECIFIED. ) ;
#9752=B_SPLINE_CURVE_WITH_KNOTS ( 'NONE', 3,
 ( #18789, #3920, #79602, #46696, #73286, #85910, #39514, #80496, #60205, #10695 ),
 .UNSPECIFIED., .F., .F.,
 ( 4, 2, 2, 2, 4 ),
 ( 0.000000000000000000, 0.0001954339857564075828, 0.0003908679715128151656, 0.0005863019572692227755, 0.0007817359430256303312 ),
 .UNSPECIFIED. ) ;
#9753=CARTESIAN_POINT ( 'NONE',  ( -2.307692307692305711, -1.367168528481310208, 33.57946703557072254 ) ) ;
#9754=ORIENTED_EDGE ( 'NONE', *, *, #1263, .F. ) ;
#9755=VECTOR ( 'NONE', #52255, 1000.000000000000227 ) ;
#9756=CYLINDRICAL_SURFACE ( 'NONE', #33981, 0.2500000000000009437 ) ;
#9757=ORIENTED_EDGE ( 'NONE', *, *, #30561, .T. ) ;
#9758=CARTESIAN_POINT ( 'NONE',  ( -10.83831157429146330, -4.762599654559228846, 34.23009711892697737 ) ) ;
#9759=CARTESIAN_POINT ( 'NONE',  ( -13.38461538461538325, -9.819645486525091727, 36.12317359536749706 ) ) ;
#9760=DIRECTION ( 'NONE',  ( -0.000000000000000000, -0.000000000000000000, -1.000000000000000000 ) ) ;
#9761=CARTESIAN_POINT ( 'NONE',  ( -0.3954711281883854790, -11.35647404775217595, 33.31231777344667222 ) ) ;
#9762=CARTESIAN_POINT ( 'NONE',  ( -14.30769230769230660, -8.973038597847269315, 34.52809138561121927 ) ) ;
#9763=CARTESIAN_POINT ( 'NONE',  ( -1.134560964701930796, -8.346898887586323923, 34.93166121998716278 ) ) ;
#9765=ORIENTED_EDGE ( 'NONE', *, *, #11046, .F. ) ;
#9766=CARTESIAN_POINT ( 'NONE',  ( -18.06527044596078113, -10.90142922261924063, 33.41473453929638993 ) ) ;
#9767=EDGE_CURVE ( 'NONE', #55252, #52031, #62112, .T. ) ;
#9768=CARTESIAN_POINT ( 'NONE',  ( 4.853438152358743984, -4.225889041578354544, 33.85425143139329407 ) ) ;
#9769=ORIENTED_EDGE ( 'NONE', *, *, #61583, .T. ) ;
#9770=EDGE_CURVE ( 'NONE', #16297, #61213, #32127, .T. ) ;
#9771=CARTESIAN_POINT ( 'NONE',  ( -16.37733107841048863, -12.69144148231606017, 30.53333754910549303 ) ) ;
#9772=CARTESIAN_POINT ( 'NONE',  ( -4.826868765284762830, -5.728107161865375829, 34.42597550085002922 ) ) ;
#9774=LINE ( 'NONE', #30488, #20294 ) ;
#9775=CIRCLE ( 'NONE', #21279, 0.2500000000000002220 ) ;
#9776=CARTESIAN_POINT ( 'NONE',  ( -10.54931728203453822, -2.833524468853757305, 32.15551576947925838 ) ) ;
#9777=CARTESIAN_POINT ( 'NONE',  ( -14.30769230769242917, -2.657715359629662544, 31.77849191805970364 ) ) ;
#9778=FACE_BOUND ( 'NONE', #5899, .T. ) ;
#9779=CARTESIAN_POINT ( 'NONE',  ( 12.23861150263161157, -10.01117774369187252, 34.36070679894347535 ) ) ;
#9780=DIRECTION ( 'NONE',  ( 0.000000000000000000, 0.9848077530122072432, -0.1736481776669354937 ) ) ;
#9781=CARTESIAN_POINT ( 'NONE',  ( 15.93036121012220541, -3.236172620538810385, 32.36188796281390267 ) ) ;
#9782=FACE_OUTER_BOUND ( 'NONE', #46587, .T. ) ;
#9783=CARTESIAN_POINT ( 'NONE',  ( 0.6843181305165246808, -3.020022701398813236, 32.48759521482552515 ) ) ;
#9784=EDGE_CURVE ( 'NONE', #45204, #59880, #57797, .T. ) ;
#9785=CARTESIAN_POINT ( 'NONE',  ( -6.000000000000119904, -10.90142922262034020, 33.41473453929536674 ) ) ;
#9786=VECTOR ( 'NONE', #62607, 1000.000000000000000 ) ;
#9788=ORIENTED_EDGE ( 'NONE', *, *, #61810, .F. ) ;
#9789=FACE_OUTER_BOUND ( 'NONE', #21188, .T. ) ;
#9791=CARTESIAN_POINT ( 'NONE',  ( 4.153846153846154188, -13.57706302396349152, 30.56769352161908060 ) ) ;
#9792=CARTESIAN_POINT ( 'NONE',  ( 6.000000000000001776, -5.471508081941601098, 34.59228464037088457 ) ) ;
#9797=CARTESIAN_POINT ( 'NONE',  ( -16.28399412357784826, -5.915902021225892149, 34.75552854090298638 ) ) ;
#9798=CARTESIAN_POINT ( 'NONE',  ( 4.087763774486017354, -11.91647553114624181, 32.58852847137148245 ) ) ;
#9799=EDGE_CURVE ( 'NONE', #22144, #53138, #69701, .T. ) ;
#9800=CARTESIAN_POINT ( 'NONE',  ( -7.846153846153967493, -3.083524468854526912, 32.58852847137268327 ) ) ;
#9801=CARTESIAN_POINT ( 'NONE',  ( 18.00000000000030553, -2.506253911140615021, 30.00000000000323297 ) ) ;
#9802=CARTESIAN_POINT ( 'NONE',  ( -16.85391023282967993, -4.762714258010882773, 34.23016756924214832 ) ) ;
#9803=CARTESIAN_POINT ( 'NONE',  ( 5.326868486301119532, -8.476813868363244353, 34.90874843262270133 ) ) ;
#9804=CARTESIAN_POINT ( 'NONE',  ( -6.249976744048589161, -12.01397095200673881, 32.43157075238190146 ) ) ;
#9805=FACE_OUTER_BOUND ( 'NONE', #52983, .T. ) ;
#9806=EDGE_LOOP ( 'NONE', ( #3117, #82029, #13039, #81646 ) ) ;
#9807=CARTESIAN_POINT ( 'NONE',  ( 17.20771351789002424, -12.62708834333097663, 30.88030960425256310 ) ) ;
#9808=CARTESIAN_POINT ( 'NONE',  ( -1.634615384615400124, -2.249999999999999112, 29.81609741502488120 ) ) ;
#9811=CARTESIAN_POINT ( 'NONE',  ( 7.173131342990376247, -10.82426656108011720, 33.81400080652039009 ) ) ;
#9812=CIRCLE ( 'NONE', #41449, 0.2500000000000002220 ) ;
#9813=CARTESIAN_POINT ( 'NONE',  ( -5.299849294439222369, -2.554751324335733820, 30.48935550225260727 ) ) ;
#9814=ORIENTED_EDGE ( 'NONE', *, *, #81201, .F. ) ;
#9815=CARTESIAN_POINT ( 'NONE',  ( 1.515407192440173745, -4.118422570099827595, 33.43335022499816489 ) ) ;
#9816=CYLINDRICAL_SURFACE ( 'NONE', #81464, 0.2500000000000002220 ) ;
#9817=VERTEX_POINT ( 'NONE', #16221 ) ;
#9818=CARTESIAN_POINT ( 'NONE',  ( -12.68502338610279168, -9.417330523894424488, 34.63758898049880486 ) ) ;
#9820=CARTESIAN_POINT ( 'NONE',  ( 17.32692307692301270, -7.565270000091922853, 34.99999999999999289 ) ) ;
#9822=VECTOR ( 'NONE', #30982, 1000.000000000000000 ) ;
#9823=CARTESIAN_POINT ( 'NONE',  ( -13.51476259405360203, -3.285722584762969856, 32.44110544564090759 ) ) ;
#9824=ORIENTED_EDGE ( 'NONE', *, *, #81387, .F. ) ;
#9825=CARTESIAN_POINT ( 'NONE',  ( 8.992010438208831502, -2.353885683473779800, 30.79025554430704403 ) ) ;
#9827=ADVANCED_FACE ( 'NONE', ( #51294 ), #1376, .F. ) ;
#9829=CARTESIAN_POINT ( 'NONE',  ( 4.153846153846154188, -9.780366693483667717, 34.19971097300155094 ) ) ;
#9830=ORIENTED_EDGE ( 'NONE', *, *, #68117, .T. ) ;
#9831=EDGE_LOOP ( 'NONE', ( #82464, #43035 ) ) ;
#9832=ORIENTED_EDGE ( 'NONE', *, *, #74425, .T. ) ;
#9833=CARTESIAN_POINT ( 'NONE',  ( 18.00000000000000000, -2.833524468853757305, 32.15551576947925838 ) ) ;
#9834=CARTESIAN_POINT ( 'NONE',  ( -7.846153846153844924, -12.62096338111211580, 30.90682066428153263 ) ) ;
#9835=CARTESIAN_POINT ( 'NONE',  ( -8.068980538632848365, -7.369208160676172348, 34.74850200257123589 ) ) ;
#9836=EDGE_CURVE ( 'NONE', #21723, #49031, #43686, .T. ) ;
#9837=CARTESIAN_POINT ( 'NONE',  ( -10.48459280755982981, -3.062576670634119758, 32.05464942895959979 ) ) ;
#9838=ADVANCED_FACE ( 'NONE', ( #43254 ), #64388, .F. ) ;
#9840=ORIENTED_EDGE ( 'NONE', *, *, #26247, .F. ) ;
#9841=ORIENTED_EDGE ( 'NONE', *, *, #31867, .F. ) ;
#9842=CARTESIAN_POINT ( 'NONE',  ( 3.230769230769110045, -11.48612834414049644, 32.76840700105863391 ) ) ;
#9843=ORIENTED_EDGE ( 'NONE', *, *, #82230, .T. ) ;
#9844=B_SPLINE_CURVE_WITH_KNOTS ( 'NONE', 3,
 ( #446, #27915, #55383, #82869, #48620, #76093, #14399, #76547, #29692, #63006 ),
 .UNSPECIFIED., .F., .F.,
 ( 4, 2, 2, 2, 4 ),
 ( 0.0007817359430256372700, 0.0009771253907250052138, 0.001172514838424373266, 0.001367904286123741101, 0.001563293733823109153 ),
 .UNSPECIFIED. ) ;
#9845=AXIS2_PLACEMENT_3D ( 'NONE', #63282, #76356, #61505 ) ;
#9846=EDGE_CURVE ( 'NONE', #27810, #16174, #17101, .T. ) ;
#9847=CARTESIAN_POINT ( 'NONE',  ( -10.61538461538461320, -13.53365097954675988, 30.81389545987213552 ) ) ;
#9848=B_SPLINE_CURVE_WITH_KNOTS ( 'NONE', 3,
 ( #48116, #70169, #63403, #62509, #825, #76488, #14792, #62947, #54885, #20651 ),
 .UNSPECIFIED., .F., .F.,
 ( 4, 2, 2, 2, 4 ),
 ( 0.0007817246256747459798, 0.0009771112852218896347, 0.001172497944769033398, 0.001367884604316177161, 0.001563271263863320708 ),
 .UNSPECIFIED. ) ;
#9849=CARTESIAN_POINT ( 'NONE',  ( 2.307692307692187583, -3.835265460704628371, 33.15142922262033665 ) ) ;
#9850=CARTESIAN_POINT ( 'NONE',  ( 13.60739505359345181, -10.23759521482555357, 34.22997729860117033 ) ) ;
#9851=ORIENTED_EDGE ( 'NONE', *, *, #9715, .F. ) ;
#9852=ORIENTED_EDGE ( 'NONE', *, *, #87956, .T. ) ;
#9853=CYLINDRICAL_SURFACE ( 'NONE', #40189, 0.2499999999999994726 ) ;
#9855=CYLINDRICAL_SURFACE ( 'NONE', #4292, 0.2499999999999986955 ) ;
#9856=CARTESIAN_POINT ( 'NONE',  ( -16.02305434602136458, -3.530189275343204702, 32.79018710029569661 ) ) ;
#9857=ORIENTED_EDGE ( 'NONE', *, *, #655, .F. ) ;
#9858=CARTESIAN_POINT ( 'NONE',  ( -8.899377978668987055, -10.88202310037935661, 33.43294751532457099 ) ) ;
#9859=CARTESIAN_POINT ( 'NONE',  ( -2.437839517130527156, -5.195881422630167279, 34.18770438780618548 ) ) ;
#9860=DIRECTION ( 'NONE',  ( -0.000000000000000000, -0.1736481776669307198, -0.9848077530122080203 ) ) ;
#9861=FACE_BOUND ( 'NONE', #69453, .T. ) ;
#9863=CARTESIAN_POINT ( 'NONE',  ( -4.153846153846273204, -12.27809138561165270, 31.22303859784587132 ) ) ;
#9864=DIRECTION ( 'NONE',  ( -0.000000000000000000, -0.6427876096865404731, -0.7660444431189770143 ) ) ;
#9865=CARTESIAN_POINT ( 'NONE',  ( 3.453548899747298062, -3.563462043263030399, 33.22394488606062879 ) ) ;
#9866=CARTESIAN_POINT ( 'NONE',  ( 6.792929713638702793, -11.93770438780619259, 32.05411857736982029 ) ) ;
#9867=AXIS2_PLACEMENT_3D ( 'NONE', #56556, #84045, #22325 ) ;
#9868=CARTESIAN_POINT ( 'NONE',  ( 18.00000000000000000, -6.343179335718451384, 34.87096338111211935 ) ) ;
#9869=CARTESIAN_POINT ( 'NONE',  ( -16.21911659980693443, -8.613356846314824011, 34.62446782046655613 ) ) ;
#9870=ORIENTED_EDGE ( 'NONE', *, *, #36108, .T. ) ;
#9871=FACE_OUTER_BOUND ( 'NONE', #31619, .T. ) ;
#9872=ORIENTED_EDGE ( 'NONE', *, *, #32996, .F. ) ;
#9874=CARTESIAN_POINT ( 'NONE',  ( 5.934729554039225974, -6.879047030191174805, 34.71129190930000163 ) ) ;
#9875=CARTESIAN_POINT ( 'NONE',  ( 1.161130440891438242, -10.81261337010820256, 33.49550067578627477 ) ) ;
#9878=CARTESIAN_POINT ( 'NONE',  ( -13.38461538461550759, -11.67786785259630911, 32.92929555188603530 ) ) ;
#9879=CARTESIAN_POINT ( 'NONE',  ( 14.43773736361208293, -2.254550872974306230, 29.97347326024527092 ) ) ;
#9881=ORIENTED_EDGE ( 'NONE', *, *, #31408, .F. ) ;
#9882=CARTESIAN_POINT ( 'NONE',  ( -13.63461538461538325, -2.499999999999998668, 29.75000000000000355 ) ) ;
#9883=VECTOR ( 'NONE', #46227, 1000.000000000000000 ) ;
#9884=CARTESIAN_POINT ( 'NONE',  ( -15.00798968950081758, -10.11255958852956027, 34.01340905677048454 ) ) ;
#9885=B_SPLINE_CURVE_WITH_KNOTS ( 'NONE', 3,
 ( #9425, #43212, #76562, #8549, #8105, #42343, #23370, #36459, #77006, #36889 ),
 .UNSPECIFIED., .F., .F.,
 ( 4, 2, 2, 2, 4 ),
 ( 0.0007817359430256330417, 0.0009771253907250000096, 0.001172514838424367194, 0.001367904286123734162, 0.001563293733823101130 ),
 .UNSPECIFIED. ) ;
#9886=CARTESIAN_POINT ( 'NONE',  ( -10.36543909703647337, -10.05730279482229683, 34.04704008940765902 ) ) ;
#9887=CARTESIAN_POINT ( 'NONE',  ( 10.61538461538461675, -3.669653830205710676, 35.88435417666054406 ) ) ;
#9888=CARTESIAN_POINT ( 'NONE',  ( 6.000000000000001776, -13.95598074871891292, 31.83374038241031911 ) ) ;
#9889=B_SPLINE_CURVE_WITH_KNOTS ( 'NONE', 3,
 ( #41237, #68700, #1578, #248, #29064, #27711, #76799, #28154, #41679, #56519 ),
 .UNSPECIFIED., .F., .F.,
 ( 4, 2, 2, 2, 4 ),
 ( 0.000000000000000000, 0.0001954311564186865221, 0.0003908623128373730441, 0.0005862934692560595662, 0.0007817246256747460882 ),
 .UNSPECIFIED. ) ;
#9892=B_SPLINE_CURVE_WITH_KNOTS ( 'NONE', 3,
 ( #32396, #74272, #46350, #88695, #60304, #59861, #53094, #80597, #18882, #67073 ),
 .UNSPECIFIED., .F., .F.,
 ( 4, 2, 2, 2, 4 ),
 ( 0.0007817359430256326080, 0.0009771253907250047801, 0.001172514838424369796, 0.001367904286123735030, 0.001563293733823100046 ),
 .UNSPECIFIED. ) ;
#9893=ORIENTED_EDGE ( 'NONE', *, *, #62074, .F. ) ;
#9894=CARTESIAN_POINT ( 'NONE',  ( -7.976844449264153702, -11.37499894934982692, 33.29245874905763003 ) ) ;
#9895=EDGE_LOOP ( 'NONE', ( #35199, #80636, #31357, #13832 ) ) ;
#9896=CARTESIAN_POINT ( 'NONE',  ( -6.988347369037698265, -2.625532179533445198, 30.86335684631481513 ) ) ;
#9897=CARTESIAN_POINT ( 'NONE',  ( -12.33101275977490197, -10.19071101563364756, 33.96452234770658407 ) ) ;
#9898=CARTESIAN_POINT ( 'NONE',  ( -16.40382288478850725, -2.779195860258148798, 31.39871582349836743 ) ) ;
#9899=DIRECTION ( 'NONE',  ( -0.000000000000000000, -0.1736481776669307198, -0.9848077530122080203 ) ) ;
#9901=DIRECTION ( 'NONE',  ( -0.000000000000000000, -0.000000000000000000, -1.000000000000000000 ) ) ;
#9903=CARTESIAN_POINT ( 'NONE',  ( 3.903846153846154632, -7.500000000000001776, 34.75000000000000000 ) ) ;
#9904=CARTESIAN_POINT ( 'NONE',  ( -1.161835843346973984, -9.332535724633405749, 34.40230450496446224 ) ) ;
#9905=ORIENTED_EDGE ( 'NONE', *, *, #16269, .F. ) ;
#9906=CARTESIAN_POINT ( 'NONE',  ( 4.153846153846154188, -13.04860791097971706, 34.73218667398347037 ) ) ;
#9907=DIRECTION ( 'NONE',  ( -0.000000000000000000, 1.000000000000000000, 3.491481338843133355E-15 ) ) ;
#9908=CARTESIAN_POINT ( 'NONE',  ( -18.00000000000012079, -6.835583212225971650, 34.95778746994575670 ) ) ;
#9909=LINE ( 'NONE', #30191, #11679 ) ;
#9910=CARTESIAN_POINT ( 'NONE',  ( -5.999999999999998224, -9.780366693483667717, 34.19971097300155094 ) ) ;
#9911=CARTESIAN_POINT ( 'NONE',  ( 11.28843830116857383, -6.695914987888146541, 34.68535235679833306 ) ) ;
#9915=CIRCLE ( 'NONE', #54528, 0.2500000000000002220 ) ;
#9917=CARTESIAN_POINT ( 'NONE',  ( 1.384615384615265343, -6.026961402154118908, 34.52809138561165270 ) ) ;
#9918=CARTESIAN_POINT ( 'NONE',  ( -17.29985003582992320, -4.762599654559227957, 34.23009711892697737 ) ) ;
#9920=CARTESIAN_POINT ( 'NONE',  ( -3.453695448285377445, -9.086856451489515152, 34.49173150075333183 ) ) ;
#9921=CARTESIAN_POINT ( 'NONE',  ( -17.07692307692319744, -2.625532179533778709, 30.86335684631627174 ) ) ;
#9925=EDGE_LOOP ( 'NONE', ( #21512, #56941, #37531, #39255 ) ) ;
#9926=CARTESIAN_POINT ( 'NONE',  ( -3.903900744468110862, -2.589246495874657938, 31.60778113518102828 ) ) ;
#9927=EDGE_LOOP ( 'NONE', ( #3857, #18015 ) ) ;
#9928=CARTESIAN_POINT ( 'NONE',  ( 14.30769230769231015, -12.10708131394839349, 31.69288490824020244 ) ) ;
#9929=CYLINDRICAL_SURFACE ( 'NONE', #49470, 0.2499999999999995559 ) ;
#9930=ADVANCED_FACE ( 'NONE', ( #8588 ), #50867, .F. ) ;
#9931=LINE ( 'NONE', #24780, #71382 ) ;
#9932=ORIENTED_EDGE ( 'NONE', *, *, #70896, .T. ) ;
#9933=CARTESIAN_POINT ( 'NONE',  ( -12.23852561744506851, -10.77377354290276124, 33.85451476688484718 ) ) ;
#9934=VERTEX_POINT ( 'NONE', #69837 ) ;
#9935=CARTESIAN_POINT ( 'NONE',  ( -2.531177232256634824, -12.11044203135681840, 32.26167407432752299 ) ) ;
#9936=ORIENTED_EDGE ( 'NONE', *, *, #49343, .T. ) ;
#9937=VECTOR ( 'NONE', #73104, 999.9999999999998863 ) ;
#9938=CARTESIAN_POINT ( 'NONE',  ( 12.33139049180676849, -12.15440758774515473, 32.17923288041532004 ) ) ;
#9939=CARTESIAN_POINT ( 'NONE',  ( -0.4615384615385826339, -4.481592998941358097, 33.73612834414048933 ) ) ;
#9940=ORIENTED_EDGE ( 'NONE', *, *, #24872, .F. ) ;
#9941=CARTESIAN_POINT ( 'NONE',  ( -5.933931648997561759, -11.16473453929635440, 33.15142922261926373 ) ) ;
#9942=CYLINDRICAL_SURFACE ( 'NONE', #66582, 0.2499999999999998890 ) ;
#9943=CARTESIAN_POINT ( 'NONE',  ( -11.76194648218548267, -2.847400154188067578, 31.58180166144859058 ) ) ;
#9946=CARTESIAN_POINT ( 'NONE',  ( 4.153846153846154188, -2.708943851104267164, 35.45975837776705220 ) ) ;
#9947=CARTESIAN_POINT ( 'NONE',  ( -13.31854805126531005, -11.91647553114624358, 32.58852847137148245 ) ) ;
#9948=ADVANCED_FACE ( 'NONE', ( #78352 ), #1817, .F. ) ;
#9949=EDGE_CURVE ( 'NONE', #11048, #19576, #81529, .T. ) ;
#9950=ORIENTED_EDGE ( 'NONE', *, *, #67195, .T. ) ;
#9951=EDGE_LOOP ( 'NONE', ( #59721, #44233, #57671, #86222 ) ) ;
#9952=FACE_BOUND ( 'NONE', #20310, .T. ) ;
#9953=ORIENTED_EDGE ( 'NONE', *, *, #19460, .F. ) ;
#9955=ORIENTED_EDGE ( 'NONE', *, *, #57563, .F. ) ;
#9956=DIRECTION ( 'NONE',  ( -0.000000000000000000, -0.7660444431189791237, -0.6427876096865379196 ) ) ;
#9957=CARTESIAN_POINT ( 'NONE',  ( 7.846153846153725020, -11.94971097300221174, 32.03036669348237098 ) ) ;
#9958=ORIENTED_EDGE ( 'NONE', *, *, #57238, .F. ) ;
#9961=CARTESIAN_POINT ( 'NONE',  ( -1.514762594053605360, -11.93770438780619259, 32.05411857736982029 ) ) ;
#9962=ORIENTED_EDGE ( 'NONE', *, *, #43391, .T. ) ;
#9963=B_SPLINE_CURVE_WITH_KNOTS ( 'NONE', 3,
 ( #54852, #55288, #13859, #41340, #21051, #68808, #76004, #356, #14305, #28712 ),
 .UNSPECIFIED., .F., .F.,
 ( 4, 2, 2, 2, 4 ),
 ( 0.000000000000000000, 0.0001954311564186867389, 0.0003908623128373734778, 0.0005862934692560602167, 0.0007817246256747469556 ),
 .UNSPECIFIED. ) ;
#9964=CARTESIAN_POINT ( 'NONE',  ( 2.307692307692309264, -4.098570777380720287, 33.41473453929634729 ) ) ;
#9965=CARTESIAN_POINT ( 'NONE',  ( 3.930919194939304084, -12.64616026154729411, 30.79003144601913533 ) ) ;
#9966=CIRCLE ( 'NONE', #86254, 0.2500000000000002220 ) ;
#9968=FACE_BOUND ( 'NONE', #15268, .T. ) ;
#9970=CARTESIAN_POINT ( 'NONE',  ( 13.38461538461526601, -9.442884908241554243, 34.35708131394783038 ) ) ;
#9971=CYLINDRICAL_SURFACE ( 'NONE', #69008, 0.2499999999999994726 ) ;
#9972=CARTESIAN_POINT ( 'NONE',  ( 6.000000000000001776, -2.538708090699994813, 30.37095296980875503 ) ) ;
#9973=CARTESIAN_POINT ( 'NONE',  ( 11.60371710973756443, -8.613356846314928816, 34.62446782046653482 ) ) ;
#9974=ORIENTED_EDGE ( 'NONE', *, *, #65701, .F. ) ;
#9976=ORIENTED_EDGE ( 'NONE', *, *, #50449, .F. ) ;
#9977=B_SPLINE_CURVE_WITH_KNOTS ( 'NONE', 3,
 ( #30830, #29513, #77244, #56969, #29954, #58300, #85792, #15553, #57411, #43021 ),
 .UNSPECIFIED., .F., .F.,
 ( 4, 2, 2, 2, 4 ),
 ( 0.0007817359430256365111, 0.0009771253907250043464, 0.001172514838424372399, 0.001367904286123740234, 0.001563293733823108069 ),
 .UNSPECIFIED. ) ;
#9978=ORIENTED_EDGE ( 'NONE', *, *, #47230, .T. ) ;
#9979=CYLINDRICAL_SURFACE ( 'NONE', #11620, 0.2500000000000008882 ) ;
#9980=CARTESIAN_POINT ( 'NONE',  ( 5.933916589044121004, -3.050289026998445951, 32.03036669348365706 ) ) ;
#9981=FACE_OUTER_BOUND ( 'NONE', #43949, .T. ) ;
#9982=FACE_OUTER_BOUND ( 'NONE', #9214, .T. ) ;
#9983=CARTESIAN_POINT ( 'NONE',  ( 16.82692307692307665, -7.433931650972299465, 34.75000000000000711 ) ) ;
#9984=CARTESIAN_POINT ( 'NONE',  ( -2.531177251416254936, -10.11188796281391511, 34.01382737946119050 ) ) ;
#9985=VERTEX_POINT ( 'NONE', #4485 ) ;
#9987=CARTESIAN_POINT ( 'NONE',  ( -0.3310130233048161896, -3.625058011473227815, 33.29252011169590020 ) ) ;
#9988=CARTESIAN_POINT ( 'NONE',  ( 11.78846153846297362, -7.500000000000155431, 34.75000000000007105 ) ) ;
#9989=CARTESIAN_POINT ( 'NONE',  ( -13.45069776397551742, -12.62096338111211580, 30.90682066428152908 ) ) ;
#9990=EDGE_LOOP ( 'NONE', ( #5081, #33228, #44372, #84536, #51679, #5873 ) ) ;
#9991=ORIENTED_EDGE ( 'NONE', *, *, #43239, .F. ) ;
#9992=FACE_BOUND ( 'NONE', #46430, .T. ) ;
#9995=EDGE_LOOP ( 'NONE', ( #58558, #84278, #85540, #81521 ) ) ;
#9996=CARTESIAN_POINT ( 'NONE',  ( -1.384615384615506484, -5.941354392335915335, 34.76329471203413846 ) ) ;
#9997=CARTESIAN_POINT ( 'NONE',  ( -6.988833725591232060, -7.249945686854186278, 34.74374336980224598 ) ) ;
#9998=VERTEX_POINT ( 'NONE', #65726 ) ;
#9999=CARTESIAN_POINT ( 'NONE',  ( -7.623374304885436104, -4.387253974876677454, 33.66317474335728832 ) ) ;
#10000=CARTESIAN_POINT ( 'NONE',  ( 6.857806477116147548, -10.90142922261923886, 33.41473453929638993 ) ) ;
#10001=CARTESIAN_POINT ( 'NONE',  ( 1.384615384615265343, -2.625532179533778709, 30.86335684631627174 ) ) ;
#10002=CARTESIAN_POINT ( 'NONE',  ( 4.153846153846154188, -6.343179335718451384, 34.87096338111211935 ) ) ;
#10004=EDGE_CURVE ( 'NONE', #17825, #69315, #86012, .T. ) ;
#10007=EDGE_LOOP ( 'NONE', ( #26592, #30001 ) ) ;
#10010=ORIENTED_EDGE ( 'NONE', *, *, #56011, .T. ) ;
#10011=DIRECTION ( 'NONE',  ( 0.000000000000000000, 0.000000000000000000, 1.000000000000000000 ) ) ;
#10012=EDGE_CURVE ( 'NONE', #74750, #5929, #4021, .T. ) ;
#10013=CARTESIAN_POINT ( 'NONE',  ( 4.153846153846154188, -6.386643153685126251, 34.62446782046654192 ) ) ;
#10014=CARTESIAN_POINT ( 'NONE',  ( -12.46153846153858424, -10.33852847137269571, 34.16647553114546554 ) ) ;
#10015=DIRECTION ( 'NONE',  ( -0.000000000000000000, -0.7660444431189791237, -0.6427876096865379196 ) ) ;
#10016=DIRECTION ( 'NONE',  ( -0.000000000000000000, 0.3420201433256694346, -0.9396926207859080948 ) ) ;
#10017=CARTESIAN_POINT ( 'NONE',  ( 12.46153846153833911, -5.941354392335915335, 34.76329471203413846 ) ) ;
#10019=VERTEX_POINT ( 'NONE', #37816 ) ;
#10020=CARTESIAN_POINT ( 'NONE',  ( -14.98071491913091791, -3.627508038966690496, 32.91356715214248396 ) ) ;
#10021=CARTESIAN_POINT ( 'NONE',  ( -14.30769230769230660, -1.509761064869970415, 31.06009739812519044 ) ) ;
#10022=ADVANCED_FACE ( 'NONE', ( #18448 ), #53100, .F. ) ;
#10023=ORIENTED_EDGE ( 'NONE', *, *, #29186, .T. ) ;
#10024=ORIENTED_EDGE ( 'NONE', *, *, #56308, .F. ) ;
#10025=CARTESIAN_POINT ( 'NONE',  ( 12.46153846153846168, -12.78798330534102767, 29.49999999999997868 ) ) ;
#10026=CARTESIAN_POINT ( 'NONE',  ( -14.30769230769242917, -2.657715359629662544, 31.77849191805970364 ) ) ;
#10027=EDGE_CURVE ( 'NONE', #41438, #39109, #958, .T. ) ;
#10028=CARTESIAN_POINT ( 'NONE',  ( 3.100622021331010281, -10.19110544564092002, 33.96427741523702792 ) ) ;
#10029=CARTESIAN_POINT ( 'NONE',  ( 0.4615384615383382183, -5.941354392335915335, 34.76329471203413846 ) ) ;
#10030=CARTESIAN_POINT ( 'NONE',  ( 13.25392478150507891, -2.845849958028613624, 32.17971566917920967 ) ) ;
#10031=CARTESIAN_POINT ( 'NONE',  ( 16.15384615384615330, -3.322132147404559976, 32.92929555188717927 ) ) ;
#10032=FACE_OUTER_BOUND ( 'NONE', #51511, .T. ) ;
#10033=ORIENTED_EDGE ( 'NONE', *, *, #30398, .T. ) ;
#10034=CARTESIAN_POINT ( 'NONE',  ( -4.087777802843714170, -5.557115091759786019, 34.35708131394839882 ) ) ;
#10035=CARTESIAN_POINT ( 'NONE',  ( -16.15384615384615330, -2.249999999999998668, 29.75000000000001776 ) ) ;
#10036=ADVANCED_FACE ( 'NONE', ( #73843 ), #72939, .F. ) ;
#10037=CARTESIAN_POINT ( 'NONE',  ( -9.019207513279360100, -11.47974371597208076, 33.17467449705390692 ) ) ;
#10038=CYLINDRICAL_SURFACE ( 'NONE', #47893, 0.2499999999999994726 ) ;
#10039=VECTOR ( 'NONE', #38712, 1000.000000000000114 ) ;
#10040=ORIENTED_EDGE ( 'NONE', *, *, #23491, .T. ) ;
#10042=B_SPLINE_CURVE_WITH_KNOTS ( 'NONE', 3,
 ( #39049, #58851, #86357, #31842, #80020, #11570, #66508, #73723, #12017, #39494 ),
 .UNSPECIFIED., .F., .F.,
 ( 4, 2, 2, 2, 4 ),
 ( 0.000000000000000000, 0.0001954311564186878773, 0.0003908623128373757546, 0.0005862934692560635777, 0.0007817246256747515092 ),
 .UNSPECIFIED. ) ;
#10043=VERTEX_POINT ( 'NONE', #38267 ) ;
#10044=CARTESIAN_POINT ( 'NONE',  ( -17.86920955903304886, -8.191423895709844416, 34.95447573519442130 ) ) ;
#10046=CARTESIAN_POINT ( 'NONE',  ( 12.71148397988660328, -10.76462480002816235, 33.53768742498949962 ) ) ;
#10047=ORIENTED_EDGE ( 'NONE', *, *, #42146, .T. ) ;
#10048=CARTESIAN_POINT ( 'NONE',  ( 12.46153846153846168, -10.67929555188718282, 33.92786785259544047 ) ) ;
#10049=CARTESIAN_POINT ( 'NONE',  ( 10.48523740594639087, -3.817052484675422797, 33.13202310037935661 ) ) ;
#10050=CARTESIAN_POINT ( 'NONE',  ( -17.14300648787895653, -3.513871655860377086, 32.76840700105978499 ) ) ;
#10053=EDGE_LOOP ( 'NONE', ( #13055, #72477 ) ) ;
#10054=AXIS2_PLACEMENT_3D ( 'NONE', #69903, #77107, #76212 ) ;
#10055=CARTESIAN_POINT ( 'NONE',  ( -17.07692307692319744, -2.892918686052165622, 31.69288490824153470 ) ) ;
#10056=EDGE_CURVE ( 'NONE', #1686, #20644, #58974, .T. ) ;
#10057=ORIENTED_EDGE ( 'NONE', *, *, #1837, .F. ) ;
#10058=B_SPLINE_CURVE_WITH_KNOTS ( 'NONE', 3,
 ( #30848, #78594, #62519, #24092, #41833, #1271, #16897, #44349, #24537, #10145 ),
 .UNSPECIFIED., .F., .F.,
 ( 4, 2, 2, 2, 4 ),
 ( 0.0007817359430256253438, 0.0009771253907249898181, 0.001172514838424354401, 0.001367904286123718983, 0.001563293733823083566 ),
 .UNSPECIFIED. ) ;
#10059=DIRECTION ( 'NONE',  ( 0.000000000000000000, 0.1736481776669267785, -0.9848077530122087975 ) ) ;
#10060=CIRCLE ( 'NONE', #76211, 0.2500000000000002220 ) ;
#10063=EDGE_CURVE ( 'NONE', #63601, #20057, #84724, .T. ) ;
#10065=EDGE_CURVE ( 'NONE', #32856, #39715, #51754, .T. ) ;
#10066=DIRECTION ( 'NONE',  ( -0.000000000000000000, -0.9848077530122085754, -0.1736481776669273613 ) ) ;
#10067=CARTESIAN_POINT ( 'NONE',  ( 9.468822748583747284, -8.496056993536548418, 34.65000542017679663 ) ) ;
#10069=AXIS2_PLACEMENT_3D ( 'NONE', #4557, #60385, #26163 ) ;
#10070=VERTEX_POINT ( 'NONE', #79257 ) ;
#10071=EDGE_LOOP ( 'NONE', ( #25690, #61515 ) ) ;
#10072=AXIS2_PLACEMENT_3D ( 'NONE', #57790, #8291, #51008 ) ;
#10073=EDGE_LOOP ( 'NONE', ( #1124, #24464, #29061, #70869 ) ) ;
#10074=ORIENTED_EDGE ( 'NONE', *, *, #43323, .F. ) ;
#10075=DIRECTION ( 'NONE',  ( -0.000000000000000000, -0.6427876096865404731, -0.7660444431189771253 ) ) ;
#10076=DIRECTION ( 'NONE',  ( -0.000000000000000000, 0.5000000000000011102, -0.8660254037844381525 ) ) ;
#10077=CARTESIAN_POINT ( 'NONE',  ( -15.09997742294444301, -8.999086150933475636, 34.52020707165672775 ) ) ;
#10079=CARTESIAN_POINT ( 'NONE',  ( -8.769230769230768274, -3.937682226553329556, 33.60647404775216529 ) ) ;
#10080=CARTESIAN_POINT ( 'NONE',  ( 0.7114839798866023912, -5.057305518903949526, 34.11320923018887896 ) ) ;
#10081=DIRECTION ( 'NONE',  ( -0.000000000000000000, 0.5000000000000011102, -0.8660254037844380415 ) ) ;
#10082=CARTESIAN_POINT ( 'NONE',  ( -18.00000000000000000, -6.386643153685127139, 34.62446782046654192 ) ) ;
#10083=ORIENTED_EDGE ( 'NONE', *, *, #39056, .F. ) ;
#10084=VERTEX_POINT ( 'NONE', #66633 ) ;
#10085=VERTEX_POINT ( 'NONE', #4937 ) ;
#10086=FACE_OUTER_BOUND ( 'NONE', #29914, .T. ) ;
#10087=ORIENTED_EDGE ( 'NONE', *, *, #88235, .F. ) ;
#10088=CARTESIAN_POINT ( 'NONE',  ( 16.15384615384603251, -11.94971097300221174, 32.03036669348237098 ) ) ;
#10089=CARTESIAN_POINT ( 'NONE',  ( -16.37677237136229991, -9.886141570436013382, 34.14413921362392301 ) ) ;
#10090=B_SPLINE_CURVE_WITH_KNOTS ( 'NONE', 3,
 ( #1660, #22368, #84092, #77314, #16497, #84528, #71430, #63351, #29145, #63791 ),
 .UNSPECIFIED., .F., .F.,
 ( 4, 2, 2, 2, 4 ),
 ( 0.000000000000000000, 0.0001954339857564071762, 0.0003908679715128143524, 0.0005863019572692215828, 0.0007817359430256287049 ),
 .UNSPECIFIED. ) ;
#10091=ADVANCED_FACE ( 'NONE', ( #17556 ), #18889, .F. ) ;
#10093=CARTESIAN_POINT ( 'NONE',  ( -16.15384615384615330, -4.098570777380720287, 33.41473453929634729 ) ) ;
#10096=ORIENTED_EDGE ( 'NONE', *, *, #86397, .F. ) ;
#10097=CARTESIAN_POINT ( 'NONE',  ( -6.923076923076922462, -1.951392089020283160, 34.73218667398347748 ) ) ;
#10098=ORIENTED_EDGE ( 'NONE', *, *, #11331, .T. ) ;
#10099=FACE_BOUND ( 'NONE', #86598, .T. ) ;
#10100=CARTESIAN_POINT ( 'NONE',  ( 3.230769230769231726, -2.486705287966279876, 31.30864560766543647 ) ) ;
#10101=CARTESIAN_POINT ( 'NONE',  ( 15.90382291655318880, -6.695914987888146541, 34.68535235679833306 ) ) ;
#10102=EDGE_LOOP ( 'NONE', ( #57749, #17846, #10785, #28814 ) ) ;
#10103=CARTESIAN_POINT ( 'NONE',  ( -1.161602540521988969, -5.582272713120728369, 34.63742843783360570 ) ) ;
#10104=CARTESIAN_POINT ( 'NONE',  ( 16.21991450484859598, -4.098570777380720287, 33.41473453929635440 ) ) ;
#10105=CARTESIAN_POINT ( 'NONE',  ( 5.076923076922954969, -2.625532179533778709, 30.86335684631627174 ) ) ;
#10106=EDGE_LOOP ( 'NONE', ( #15957, #53429, #62234, #11666 ) ) ;
#10107=CYLINDRICAL_SURFACE ( 'NONE', #88884, 0.2500000000000002220 ) ;
#10108=CARTESIAN_POINT ( 'NONE',  ( 1.384615384615264011, -2.657715359629662544, 31.77849191805970364 ) ) ;
#10110=ORIENTED_EDGE ( 'NONE', *, *, #22267, .T. ) ;
#10111=ADVANCED_FACE ( 'NONE', ( #33735 ), #61189, .F. ) ;
#10112=FACE_OUTER_BOUND ( 'NONE', #33230, .T. ) ;
#10113=DIRECTION ( 'NONE',  ( -0.000000000000000000, -0.8660254037844397068, -0.4999999999999978906 ) ) ;
#10115=CYLINDRICAL_SURFACE ( 'NONE', #67444, 0.2500000000000002220 ) ;
#10116=CARTESIAN_POINT ( 'NONE',  ( -2.307692307692305711, -13.57706302396349152, 30.56769352161908060 ) ) ;
#10117=DIRECTION ( 'NONE',  ( -0.000000000000000000, 0.9848077530122085754, -0.1736481776669273613 ) ) ;
#10118=CARTESIAN_POINT ( 'NONE',  ( 7.596153846153847589, -7.433931650972299465, 34.75000000000000000 ) ) ;
#10119=CARTESIAN_POINT ( 'NONE',  ( -18.00000000000012079, -6.879047030192663392, 34.71129190930017927 ) ) ;
#10120=CARTESIAN_POINT ( 'NONE',  ( 17.07692307692295586, -5.094484230521993062, 34.41647553114689373 ) ) ;
#10121=DIRECTION ( 'NONE',  ( 0.000000000000000000, 0.7660444431189807890, 0.6427876096865361433 ) ) ;
#10122=CARTESIAN_POINT ( 'NONE',  ( 2.557746619330623972, -9.943054286541407549, 34.11300777759954883 ) ) ;
#10124=CARTESIAN_POINT ( 'NONE',  ( -15.93106661257773915, -11.89424750095246175, 32.13594075562311758 ) ) ;
#10125=CARTESIAN_POINT ( 'NONE',  ( -12.71153846153846168, -2.249999999999998668, 29.75000000000000355 ) ) ;
#10126=CARTESIAN_POINT ( 'NONE',  ( -10.83886955910856464, -8.496056993536548418, 34.65000542017679663 ) ) ;
#10127=CARTESIAN_POINT ( 'NONE',  ( -5.777220458731586739, -12.44528174975671853, 30.48912976160716681 ) ) ;
#10129=ORIENTED_EDGE ( 'NONE', *, *, #18407, .T. ) ;
#10130=CARTESIAN_POINT ( 'NONE',  ( 18.13079180782478872, -11.71459661697925903, 32.44059661609676937 ) ) ;
#10132=VECTOR ( 'NONE', #10795, 1000.000000000000227 ) ;
#10133=VECTOR ( 'NONE', #50699, 1000.000000000000114 ) ;
#10136=VERTEX_POINT ( 'NONE', #6270 ) ;
#10137=B_SPLINE_CURVE_WITH_KNOTS ( 'NONE', 3,
 ( #65941, #51518, #66844, #38038, #18669, #4250, #25413, #17774, #3801, #52873 ),
 .UNSPECIFIED., .F., .F.,
 ( 4, 2, 2, 2, 4 ),
 ( 0.0007817359430256392216, 0.0009771253907250080327, 0.001172514838424376952, 0.001367904286123745872, 0.001563293733823114791 ),
 .UNSPECIFIED. ) ;
#10138=CARTESIAN_POINT ( 'NONE',  ( 15.93036121012220185, -11.41268669641499756, 32.86336882939238535 ) ) ;
#10139=ORIENTED_EDGE ( 'NONE', *, *, #53594, .F. ) ;
#10140=CARTESIAN_POINT ( 'NONE',  ( -7.911424292114620727, -6.026961402152685388, 34.52809138561120506 ) ) ;
#10142=CARTESIAN_POINT ( 'NONE',  ( 3.164686851409094004, -2.292212530054419606, 30.41441678777542634 ) ) ;
#10143=ADVANCED_FACE ( 'NONE', ( #26539 ), #47687, .F. ) ;
#10144=AXIS2_PLACEMENT_3D ( 'NONE', #24645, #51197, #44021 ) ;
#10145=CARTESIAN_POINT ( 'NONE',  ( 9.692307692307695177, -11.16473453929635440, 33.15142922261926373 ) ) ;
#10146=CARTESIAN_POINT ( 'NONE',  ( 13.63456079399342791, -2.986452184633680673, 32.43230066228895225 ) ) ;
#10148=AXIS2_PLACEMENT_3D ( 'NONE', #25944, #53409, #5673 ) ;
#10149=CARTESIAN_POINT ( 'NONE',  ( 12.46153846153833911, -11.06231777344772027, 33.60647404775119895 ) ) ;
#10150=DIRECTION ( 'NONE',  ( -0.000000000000000000, 0.7660444431189791237, -0.6427876096865379196 ) ) ;
#10151=DIRECTION ( 'NONE',  ( -0.000000000000000000, -0.000000000000000000, -1.000000000000000000 ) ) ;
#10155=DIRECTION ( 'NONE',  ( -0.000000000000000000, -0.1736481776669307198, -0.9848077530122080203 ) ) ;
#10156=EDGE_CURVE ( 'NONE', #83859, #75335, #7332, .T. ) ;
#10157=DIRECTION ( 'NONE',  ( 0.000000000000000000, 0.8660254037844377084, 0.5000000000000015543 ) ) ;
#10159=ORIENTED_EDGE ( 'NONE', *, *, #74577, .F. ) ;
#10161=CARTESIAN_POINT ( 'NONE',  ( 16.08776274289027342, -12.10708131394839349, 31.69288490824020244 ) ) ;
#10162=CYLINDRICAL_SURFACE ( 'NONE', #36827, 0.2500000000000009437 ) ;
#10163=CARTESIAN_POINT ( 'NONE',  ( -3.230769230769229949, -2.249999999999998668, 29.75000000000001776 ) ) ;
#10164=EDGE_CURVE ( 'NONE', #23513, #26351, #44856, .T. ) ;
#10165=CARTESIAN_POINT ( 'NONE',  ( 17.14299041027315695, -12.34228464037088813, 31.77849191805839268 ) ) ;
#10166=CARTESIAN_POINT ( 'NONE',  ( -14.30769230769230660, -3.937682226553329556, 33.60647404775216529 ) ) ;
#10167=EDGE_CURVE ( 'NONE', #10019, #64009, #11639, .T. ) ;
#10168=EDGE_LOOP ( 'NONE', ( #46737, #80657 ) ) ;
#10169=CARTESIAN_POINT ( 'NONE',  ( 7.623226887246995709, -2.889293201056495786, 32.26117774369186009 ) ) ;
#10170=VERTEX_POINT ( 'NONE', #395 ) ;
#10171=VECTOR ( 'NONE', #53782, 1000.000000000000227 ) ;
#10172=EDGE_CURVE ( 'NONE', #13065, #38188, #3001, .T. ) ;
#10173=ORIENTED_EDGE ( 'NONE', *, *, #52088, .F. ) ;
#10174=CARTESIAN_POINT ( 'NONE',  ( -9.442253272394237840, -2.920487667080175598, 32.31805714834170828 ) ) ;
#10175=CARTESIAN_POINT ( 'NONE',  ( -6.923076923076922462, -5.471508081941601098, 34.59228464037088457 ) ) ;
#10176=CARTESIAN_POINT ( 'NONE',  ( -15.48074597481782178, -10.82459398097509329, 33.81372124010185587 ) ) ;
#10177=ADVANCED_FACE ( 'NONE', ( #46802 ), #55325, .F. ) ;
#10178=CARTESIAN_POINT ( 'NONE',  ( 11.53846153846153832, -9.058645607665452459, 34.76329471203371924 ) ) ;
#10179=CARTESIAN_POINT ( 'NONE',  ( 13.16168842570853492, -5.582147617184174848, 34.63737895849758530 ) ) ;
#10180=ORIENTED_EDGE ( 'NONE', *, *, #16276, .T. ) ;
#10181=CARTESIAN_POINT ( 'NONE',  ( -14.05774678934416499, -12.22109172314383052, 31.39792113162168263 ) ) ;
#10182=ORIENTED_EDGE ( 'NONE', *, *, #6214, .T. ) ;
#10183=ORIENTED_EDGE ( 'NONE', *, *, #38518, .T. ) ;
#10185=CARTESIAN_POINT ( 'NONE',  ( 18.25005441991345378, -2.318338780012835443, 30.59689888758630616 ) ) ;
#10186=LINE ( 'NONE', #16496, #37308 ) ;
#10187=ADVANCED_FACE ( 'NONE', ( #76040 ), #830, .F. ) ;
#10188=B_SPLINE_CURVE_WITH_KNOTS ( 'NONE', 3,
 ( #25042, #3872, #87654, #85861, #11088, #39464, #73235, #25930, #10203, #37664 ),
 .UNSPECIFIED., .F., .F.,
 ( 4, 2, 2, 2, 4 ),
 ( 0.0007817359430256323911, 0.0009771253907249991422, 0.001172514838424365893, 0.001367904286123732861, 0.001563293733823099612 ),
 .UNSPECIFIED. ) ;
#10189=CARTESIAN_POINT ( 'NONE',  ( -16.21992956480203318, -4.098570777380720287, 33.41473453929634729 ) ) ;
#10190=VECTOR ( 'NONE', #56637, 1000.000000000000000 ) ;
#10192=ADVANCED_FACE ( 'NONE', ( #15681 ), #57095, .F. ) ;
#10193=CARTESIAN_POINT ( 'NONE',  ( -17.01166750564705410, -3.300289026998475261, 32.46337939537591666 ) ) ;
#10194=CARTESIAN_POINT ( 'NONE',  ( 17.75002326905764605, -8.303909089506435137, 34.68538101551103381 ) ) ;
#10195=ORIENTED_EDGE ( 'NONE', *, *, #82259, .T. ) ;
#10196=VERTEX_POINT ( 'NONE', #36826 ) ;
#10199=ORIENTED_EDGE ( 'NONE', *, *, #54161, .T. ) ;
#10200=CARTESIAN_POINT ( 'NONE',  ( -13.63463860883683942, -5.765609946408404518, 34.70566812827425451 ) ) ;
#10201=VERTEX_POINT ( 'NONE', #49894 ) ;
#10202=EDGE_CURVE ( 'NONE', #64231, #11769, #86291, .T. ) ;
#10203=CARTESIAN_POINT ( 'NONE',  ( 7.912222197156284054, -12.37446782046654192, 30.86335684631486842 ) ) ;
#10204=CARTESIAN_POINT ( 'NONE',  ( 6.223011351612852238, -12.39991518177334129, 30.74647679643404530 ) ) ;
#10205=EDGE_CURVE ( 'NONE', #76909, #21625, #63854, .T. ) ;
#10206=LINE ( 'NONE', #5221, #68146 ) ;
#10207=ORIENTED_EDGE ( 'NONE', *, *, #40990, .F. ) ;
#10208=FACE_OUTER_BOUND ( 'NONE', #83814, .T. ) ;
#10209=ORIENTED_EDGE ( 'NONE', *, *, #50931, .F. ) ;
#10210=EDGE_CURVE ( 'NONE', #62470, #26559, #62952, .T. ) ;
#10213=LINE ( 'NONE', #16081, #45156 ) ;
#10214=LINE ( 'NONE', #44868, #15853 ) ;
#10216=ADVANCED_FACE ( 'NONE', ( #56658 ), #71490, .F. ) ;
#10218=CARTESIAN_POINT ( 'NONE',  ( -3.230769230769229949, -8.164416787775445883, 34.95778746994557906 ) ) ;
#10219=VERTEX_POINT ( 'NONE', #64283 ) ;
#10220=DIRECTION ( 'NONE',  ( -0.000000000000000000, 0.9396926207859093161, -0.3420201433256663259 ) ) ;
#10222=ORIENTED_EDGE ( 'NONE', *, *, #62108, .T. ) ;
#10223=ADVANCED_FACE ( 'NONE', ( #85025 ), #70174, .F. ) ;
#10224=CYLINDRICAL_SURFACE ( 'NONE', #32148, 0.2500000000000004996 ) ;
#10225=VECTOR ( 'NONE', #11385, 1000.000000000000000 ) ;
#10226=CARTESIAN_POINT ( 'NONE',  ( 17.07692307692307665, -10.67929555188718282, 33.92786785259544047 ) ) ;
#10227=CARTESIAN_POINT ( 'NONE',  ( 16.02369818411445834, -6.809168938359901446, 34.95455904226513866 ) ) ;
#10228=CARTESIAN_POINT ( 'NONE',  ( -16.28399412357784826, -12.15440758774515473, 32.17923288041532004 ) ) ;
#10229=CARTESIAN_POINT ( 'NONE',  ( 7.780883400193070898, -8.613356846314824011, 34.62446782046655613 ) ) ;
#10230=B_SPLINE_CURVE_WITH_KNOTS ( 'NONE', 3,
 ( #4896, #46313, #38221, #78760, #73801, #31009, #12102, #58474, #85970, #58931 ),
 .UNSPECIFIED., .F., .F.,
 ( 4, 2, 2, 2, 4 ),
 ( 0.000000000000000000, 0.0001954339857564079623, 0.0003908679715128159245, 0.0005863019572692238597, 0.0007817359430256318490 ),
 .UNSPECIFIED. ) ;
#10231=FACE_BOUND ( 'NONE', #40413, .T. ) ;
#10232=CARTESIAN_POINT ( 'NONE',  ( 17.07692307692307665, -13.78497067705608181, 32.30358669280327177 ) ) ;
#10233=CARTESIAN_POINT ( 'NONE',  ( 17.86930939688969033, -10.70098750199973203, 33.91152734681376302 ) ) ;
#10234=B_SPLINE_CURVE_WITH_KNOTS ( 'NONE', 3,
 ( #83277, #21564, #8059, #35529, #1289, #56242, #83727, #22012, #49488, #76956 ),
 .UNSPECIFIED., .F., .F.,
 ( 4, 2, 2, 2, 4 ),
 ( 0.000000000000000000, 0.0001954311564186864949, 0.0003908623128373729899, 0.0005862934692560594577, 0.0007817246256747459798 ),
 .UNSPECIFIED. ) ;
#10235=CARTESIAN_POINT ( 'NONE',  ( 15.93091993633000492, -3.105860786376062332, 32.13614157043599562 ) ) ;
#10236=CARTESIAN_POINT ( 'NONE',  ( 3.007843013253084230, -4.186968288167446595, 33.49512374952580274 ) ) ;
#10237=CARTESIAN_POINT ( 'NONE',  ( -11.28840711854808632, -10.82426656108012075, 33.81400080652039009 ) ) ;
#10238=DIRECTION ( 'NONE',  ( 0.000000000000000000, 0.9848077530122072432, 0.1736481776669354937 ) ) ;
#10239=VECTOR ( 'NONE', #272, 1000.000000000000227 ) ;
#10240=CARTESIAN_POINT ( 'NONE',  ( 11.53846153846185274, -2.255955759149395501, 30.00000000000324363 ) ) ;
#10242=ORIENTED_EDGE ( 'NONE', *, *, #15057, .F. ) ;
#10243=CARTESIAN_POINT ( 'NONE',  ( -1.384615384615383471, -12.78798330534102945, 29.74999999999997868 ) ) ;
#10244=CARTESIAN_POINT ( 'NONE',  ( -4.946131269098291483, -3.062576670634119758, 32.05464942895959979 ) ) ;
#10245=DIRECTION ( 'NONE',  ( -0.000000000000000000, 1.000000000000000000, 3.491481338843133355E-15 ) ) ;
#10247=CARTESIAN_POINT ( 'NONE',  ( -4.284536756956462078, -4.684245665217972032, 34.18127051446801090 ) ) ;
#10248=CARTESIAN_POINT ( 'NONE',  ( -16.82697766754503377, -8.476813868363244353, 34.90874843262270133 ) ) ;
#10250=EDGE_CURVE ( 'NONE', #45495, #38893, #2585, .T. ) ;
#10251=CARTESIAN_POINT ( 'NONE',  ( -11.28846153846011902, -7.500000000000154543, 35.00000000000007105 ) ) ;
#10254=CARTESIAN_POINT ( 'NONE',  ( 17.86985203026830504, -8.630895178749536711, 34.87696386517710323 ) ) ;
#10255=DIRECTION ( 'NONE',  ( -0.000000000000000000, 0.3420201433256694901, -0.9396926207859082059 ) ) ;
#10256=DIRECTION ( 'NONE',  ( 0.000000000000000000, 0.3420201433256610524, 0.9396926207859113145 ) ) ;
#10257=CARTESIAN_POINT ( 'NONE',  ( -9.692307692307691624, -1.422936976036506707, 30.56769352161908415 ) ) ;
#10258=AXIS2_PLACEMENT_3D ( 'NONE', #42148, #35829, #49770 ) ;
#10259=CARTESIAN_POINT ( 'NONE',  ( 14.30769230769218758, -6.879047030192662504, 34.71129190930017927 ) ) ;
#10260=VERTEX_POINT ( 'NONE', #22862 ) ;
#10261=CARTESIAN_POINT ( 'NONE',  ( -11.53846153846153655, -11.11383981884818262, 36.00935417666054406 ) ) ;
#10262=CARTESIAN_POINT ( 'NONE',  ( -3.230769230769229949, -6.386643153685126251, 34.62446782046654192 ) ) ;
#10264=CARTESIAN_POINT ( 'NONE',  ( 6.249945518348143381, -4.336752205174647656, 33.62275283266504289 ) ) ;
#10265=CARTESIAN_POINT ( 'NONE',  ( 3.361561038594017337, -11.71459661697925903, 32.44059661609676937 ) ) ;
#10266=ORIENTED_EDGE ( 'NONE', *, *, #29790, .T. ) ;
#10267=CARTESIAN_POINT ( 'NONE',  ( -16.37677311275300340, -4.026226216239093603, 33.68668979543632958 ) ) ;
#10269=CARTESIAN_POINT ( 'NONE',  ( 4.023154687178594813, -5.582088688514999397, 34.36776431015576350 ) ) ;
#10270=ORIENTED_EDGE ( 'NONE', *, *, #78671, .T. ) ;
#10271=CARTESIAN_POINT ( 'NONE',  ( 2.307692307692309264, -13.75783147151868846, 33.36296068462461051 ) ) ;
#10272=CARTESIAN_POINT ( 'NONE',  ( -13.25408968285182532, -10.19071101563364756, 33.96452234770658407 ) ) ;
#10273=CYLINDRICAL_SURFACE ( 'NONE', #42101, 0.2499999999999997502 ) ;
#10275=CYLINDRICAL_SURFACE ( 'NONE', #80275, 0.2499999999999994726 ) ;
#10276=EDGE_LOOP ( 'NONE', ( #51440, #38812, #86210, #83993 ) ) ;
#10277=CARTESIAN_POINT ( 'NONE',  ( -12.46153846153846168, -13.57706302396349152, 30.56769352161908060 ) ) ;
#10278=CARTESIAN_POINT ( 'NONE',  ( 15.16549923021291058, -10.33852847137145048, 34.16647553114627556 ) ) ;
#10279=ORIENTED_EDGE ( 'NONE', *, *, #41502, .T. ) ;
#10281=EDGE_CURVE ( 'NONE', #62019, #35285, #8482, .T. ) ;
#10282=ORIENTED_EDGE ( 'NONE', *, *, #41002, .T. ) ;
#10283=CYLINDRICAL_SURFACE ( 'NONE', #32816, 0.2500000000000004996 ) ;
#10284=CARTESIAN_POINT ( 'NONE',  ( -8.769230769230768274, -3.050289026998446396, 32.03036669348365706 ) ) ;
#10285=EDGE_CURVE ( 'NONE', #80414, #16715, #8455, .T. ) ;
#10286=CARTESIAN_POINT ( 'NONE',  ( 0.2115384615384615641, -7.500000000000001776, 35.00000000000000000 ) ) ;
#10287=EDGE_CURVE ( 'NONE', #16973, #64228, #31712, .T. ) ;
#10288=CARTESIAN_POINT ( 'NONE',  ( 15.00784301325307979, -3.586966769969701208, 32.86292498521069660 ) ) ;
#10289=VECTOR ( 'NONE', #83892, 1000.000000000000227 ) ;
#10290=VERTEX_POINT ( 'NONE', #76936 ) ;
#10291=ORIENTED_EDGE ( 'NONE', *, *, #78257, .F. ) ;
#10292=CARTESIAN_POINT ( 'NONE',  ( 15.29602480204525605, -5.219633306516380244, 34.19971097300157936 ) ) ;
#10294=VECTOR ( 'NONE', #24865, 1000.000000000000114 ) ;
#10295=EDGE_CURVE ( 'NONE', #10290, #33013, #41802, .T. ) ;
#10296=CARTESIAN_POINT ( 'NONE',  ( 17.20771488474786892, -4.809403383903225304, 33.96459661697925014 ) ) ;
#10297=CARTESIAN_POINT ( 'NONE',  ( -8.546219417617921366, -12.39991518177334129, 30.74647679643404530 ) ) ;
#10298=CARTESIAN_POINT ( 'NONE',  ( -13.16183584334697443, -12.44528174975671853, 30.48912976160716681 ) ) ;
#10299=VERTEX_POINT ( 'NONE', #8926 ) ;
#10300=ORIENTED_EDGE ( 'NONE', *, *, #33109, .F. ) ;
#10301=ORIENTED_EDGE ( 'NONE', *, *, #42106, .F. ) ;
#10302=CARTESIAN_POINT ( 'NONE',  ( 3.230769230769231726, -1.466349020453238561, 30.81389545987213907 ) ) ;
#10304=CARTESIAN_POINT ( 'NONE',  ( 5.076923076923075762, -5.471508081941601098, 34.59228464037088457 ) ) ;
#10305=DIRECTION ( 'NONE',  ( 0.000000000000000000, 0.000000000000000000, 1.000000000000000000 ) ) ;
#10306=EDGE_LOOP ( 'NONE', ( #75024, #34935 ) ) ;
#10307=CARTESIAN_POINT ( 'NONE',  ( 6.857825932915681655, -2.506253911140460477, 30.00000000000013856 ) ) ;
#10309=FACE_OUTER_BOUND ( 'NONE', #7849, .T. ) ;
#10310=FACE_BOUND ( 'NONE', #12952, .T. ) ;
#10313=CARTESIAN_POINT ( 'NONE',  ( 9.626550889793387356, -7.249945686854186278, 34.74374336980224598 ) ) ;
#10314=AXIS2_PLACEMENT_3D ( 'NONE', #47090, #18754, #12870 ) ;
#10315=CARTESIAN_POINT ( 'NONE',  ( 13.25392478150508069, -12.62707690430377383, 30.88035979386743435 ) ) ;
#10316=CARTESIAN_POINT ( 'NONE',  ( 14.55769230769372946, -7.500000000000154543, 35.00000000000007105 ) ) ;
#10317=CARTESIAN_POINT ( 'NONE',  ( -16.08777882049607655, -2.833524468853757750, 32.15551576947925838 ) ) ;
#10318=CARTESIAN_POINT ( 'NONE',  ( 18.00000000000000000, -13.95598074871891292, 31.83374038241031911 ) ) ;
#10320=VERTEX_POINT ( 'NONE', #9368 ) ;
#10321=CARTESIAN_POINT ( 'NONE',  ( -5.869208192175213945, -11.71459661697925903, 32.44059661609676937 ) ) ;
#10322=ORIENTED_EDGE ( 'NONE', *, *, #80431, .F. ) ;
#10323=ORIENTED_EDGE ( 'NONE', *, *, #86756, .T. ) ;
#10324=VECTOR ( 'NONE', #69753, 1000.000000000000000 ) ;
#10325=CARTESIAN_POINT ( 'NONE',  ( 5.749976762707036393, -6.695914987888143877, 34.68535235679833306 ) ) ;
#10326=CARTESIAN_POINT ( 'NONE',  ( -6.000000000000119904, -12.27809138561165270, 31.22303859784587132 ) ) ;
#10328=CARTESIAN_POINT ( 'NONE',  ( -6.673131404728780858, -6.696923467548660192, 34.68552623307873972 ) ) ;
#10329=CARTESIAN_POINT ( 'NONE',  ( 15.23076923076923173, -8.973038597847269315, 34.52809138561121927 ) ) ;
#10330=CARTESIAN_POINT ( 'NONE',  ( -3.931066484868084299, -3.563462043263029067, 33.22394488606062879 ) ) ;
#10331=EDGE_LOOP ( 'NONE', ( #21817, #83851 ) ) ;
#10332=CARTESIAN_POINT ( 'NONE',  ( 4.153846153846030731, -5.094484230521993062, 34.41647553114689373 ) ) ;
#10333=EDGE_CURVE ( 'NONE', #4609, #68238, #66228, .T. ) ;
#10334=EDGE_CURVE ( 'NONE', #80428, #33744, #4376, .T. ) ;
#10335=CARTESIAN_POINT ( 'NONE',  ( -15.16470087976679082, -9.780366693483667717, 34.19971097300155805 ) ) ;
#10336=DIRECTION ( 'NONE',  ( -0.000000000000000000, 0.1736481776669307198, -0.9848077530122080203 ) ) ;
#10337=CARTESIAN_POINT ( 'NONE',  ( 0.2380535369741302032, -3.562934362175799841, 33.22335522853832401 ) ) ;
#10338=DIRECTION ( 'NONE',  ( -0.000000000000000000, -0.1736481776669307198, -0.9848077530122080203 ) ) ;
#10339=B_SPLINE_CURVE_WITH_KNOTS ( 'NONE', 3,
 ( #60053, #87558, #88885, #53293, #80796, #74027, #28953, #8673, #16305, #55954 ),
 .UNSPECIFIED., .F., .F.,
 ( 4, 2, 2, 2, 4 ),
 ( 0.000000000000000000, 0.0001954311564186868744, 0.0003908623128373737488, 0.0005862934692560606504, 0.0007817246256747474977 ),
 .UNSPECIFIED. ) ;
#10342=ORIENTED_EDGE ( 'NONE', *, *, #38744, .F. ) ;
#10343=CARTESIAN_POINT ( 'NONE',  ( -14.55771553191376277, -4.931416488878822335, 34.32920672191015399 ) ) ;
#10344=ORIENTED_EDGE ( 'NONE', *, *, #30504, .T. ) ;
#10346=CARTESIAN_POINT ( 'NONE',  ( -12.46153846153846168, -9.780366693483667717, 34.19971097300155094 ) ) ;
#10347=DIRECTION ( 'NONE',  ( 0.000000000000000000, 0.3420201433256610524, 0.9396926207859113145 ) ) ;
#10348=DIRECTION ( 'NONE',  ( 0.000000000000000000, 0.7660444431189807890, 0.6427876096865361433 ) ) ;
#10351=CARTESIAN_POINT ( 'NONE',  ( -13.63463862190834952, -8.432397168068783699, 34.66272746175022945 ) ) ;
#10352=ORIENTED_EDGE ( 'NONE', *, *, #86756, .F. ) ;
#10354=DIRECTION ( 'NONE',  ( -0.000000000000000000, 0.9396926207859092051, -0.3420201433256662704 ) ) ;
#10357=FACE_OUTER_BOUND ( 'NONE', #9626, .T. ) ;
#10358=EDGE_CURVE ( 'NONE', #18795, #11372, #72879, .T. ) ;
#10359=EDGE_CURVE ( 'NONE', #24353, #57187, #67471, .T. ) ;
#10360=CARTESIAN_POINT ( 'NONE',  ( -2.980769230769166445, -7.434744429011176159, 34.75000000000000711 ) ) ;
#10361=CARTESIAN_POINT ( 'NONE',  ( 11.60452887181161508, -8.164416787775445883, 34.95778746994558617 ) ) ;
#10362=CARTESIAN_POINT ( 'NONE',  ( -14.30769230769242917, -11.67786785259630911, 32.92929555188603530 ) ) ;
#10364=CARTESIAN_POINT ( 'NONE',  ( -7.173100160369889622, -5.056417327199099532, 34.11270091957320716 ) ) ;
#10365=VECTOR ( 'NONE', #17806, 1000.000000000000000 ) ;
#10367=EDGE_LOOP ( 'NONE', ( #84539, #15281, #67349, #10969 ) ) ;
#10368=EDGE_CURVE ( 'NONE', #23052, #81809, #52553, .T. ) ;
#10369=CARTESIAN_POINT ( 'NONE',  ( -16.08859101433330707, -6.835583212224605631, 34.95778746994559327 ) ) ;
#10370=CARTESIAN_POINT ( 'NONE',  ( -13.16160254052199008, -10.01129605718032600, 34.36064277460058491 ) ) ;
#10371=B_SPLINE_CURVE_WITH_KNOTS ( 'NONE', 3,
 ( #39166, #40497, #60748, #32394, #60302, #67960, #73381, #81925, #53092, #18881 ),
 .UNSPECIFIED., .F., .F.,
 ( 4, 2, 2, 2, 4 ),
 ( 0.000000000000000000, 0.0001954311564186865492, 0.0003908623128373730983, 0.0005862934692560596746, 0.0007817246256747461966 ),
 .UNSPECIFIED. ) ;
#10372=CARTESIAN_POINT ( 'NONE',  ( -4.219928533206288357, -5.471508081941601986, 34.59228464037088457 ) ) ;
#10374=CARTESIAN_POINT ( 'NONE',  ( 0.2115152242454959863, -3.711651800289232916, 33.01384336483936011 ) ) ;
#10375=CARTESIAN_POINT ( 'NONE',  ( 8.519207545009313876, -10.18141759479407327, 34.26406193332782379 ) ) ;
#10378=CARTESIAN_POINT ( 'NONE',  ( 3.100077764101673239, -8.999036380462717588, 34.52022231692819076 ) ) ;
#10379=ORIENTED_EDGE ( 'NONE', *, *, #45373, .F. ) ;
#10380=CARTESIAN_POINT ( 'NONE',  ( -4.153846153846152411, -8.164416787775445883, 34.95778746994557906 ) ) ;
#10381=ORIENTED_EDGE ( 'NONE', *, *, #60976, .T. ) ;
#10382=LINE ( 'NONE', #15818, #27584 ) ;
#10383=CARTESIAN_POINT ( 'NONE',  ( 13.31934493865461278, -10.21337939537584383, 33.94971097300158647 ) ) ;
#10384=DIRECTION ( 'NONE',  ( 0.000000000000000000, 0.4999999999999985567, 0.8660254037844395958 ) ) ;
#10385=ORIENTED_EDGE ( 'NONE', *, *, #26761, .F. ) ;
#10386=DIRECTION ( 'NONE',  ( -0.000000000000000000, -0.7660444431189791237, -0.6427876096865379196 ) ) ;
#10387=ORIENTED_EDGE ( 'NONE', *, *, #49931, .F. ) ;
#10389=EDGE_CURVE ( 'NONE', #18498, #3281, #49178, .T. ) ;
#10390=VECTOR ( 'NONE', #82803, 1000.000000000000227 ) ;
#10391=ORIENTED_EDGE ( 'NONE', *, *, #77994, .F. ) ;
#10392=VECTOR ( 'NONE', #38196, 1000.000000000000000 ) ;
#10393=CARTESIAN_POINT ( 'NONE',  ( 12.23805353697413167, -12.11044203135681840, 32.26167407432752299 ) ) ;
#10394=CARTESIAN_POINT ( 'NONE',  ( -17.07692307692307665, -13.87047571288749737, 32.06866353760679544 ) ) ;
#10395=ORIENTED_EDGE ( 'NONE', *, *, #5878, .F. ) ;
#10396=CARTESIAN_POINT ( 'NONE',  ( -6.000000000000119904, -11.48612834414049644, 32.76840700105863391 ) ) ;
#10397=CARTESIAN_POINT ( 'NONE',  ( -14.53061852520844610, -10.61292498521070549, 33.66303323003028680 ) ) ;
#10398=CARTESIAN_POINT ( 'NONE',  ( -11.66860950819323861, -3.069018819979302926, 32.56621877034667278 ) ) ;
#10400=ADVANCED_FACE ( 'NONE', ( #38158 ), #45801, .F. ) ;
#10401=DIRECTION ( 'NONE',  ( -0.000000000000000000, 0.6427876096865404731, -0.7660444431189770143 ) ) ;
#10402=CARTESIAN_POINT ( 'NONE',  ( 18.00000000000000000, -2.292212530054420494, 30.41441678777542634 ) ) ;
#10403=B_SPLINE_CURVE_WITH_KNOTS ( 'NONE', 3,
 ( #9447, #3564, #44098, #36909, #64814, #64371, #51278, #72024, #72472, #31033 ),
 .UNSPECIFIED., .F., .F.,
 ( 4, 2, 2, 2, 4 ),
 ( 0.000000000000000000, 0.0001954339857564093175, 0.0003908679715128186350, 0.0005863019572692279796, 0.0007817359430256372700 ),
 .UNSPECIFIED. ) ;
#10404=B_SPLINE_CURVE_WITH_KNOTS ( 'NONE', 3,
 ( #10740, #45399, #78747, #38654, #17049, #51698, #10297, #37761, #65227, #85955 ),
 .UNSPECIFIED., .F., .F.,
 ( 4, 2, 2, 2, 4 ),
 ( 0.0007817359430256326080, 0.0009771253907249993591, 0.001172514838424366327, 0.001367904286123733078, 0.001563293733823099829 ),
 .UNSPECIFIED. ) ;
#10405=ORIENTED_EDGE ( 'NONE', *, *, #55576, .T. ) ;
#10407=ORIENTED_EDGE ( 'NONE', *, *, #32430, .T. ) ;
#10408=CARTESIAN_POINT ( 'NONE',  ( 2.980792486720639900, -5.643011162660950042, 34.66104346484419096 ) ) ;
#10409=EDGE_LOOP ( 'NONE', ( #39309, #7281 ) ) ;
#10410=EDGE_CURVE ( 'NONE', #59263, #78986, #4828, .T. ) ;
#10411=CARTESIAN_POINT ( 'NONE',  ( 10.39245839786846837, -4.887634598454295265, 34.01352882383564946 ) ) ;
#10413=ORIENTED_EDGE ( 'NONE', *, *, #10004, .T. ) ;
#10414=VERTEX_POINT ( 'NONE', #31403 ) ;
#10415=ADVANCED_FACE ( 'NONE', ( #86372 ), #66528, .F. ) ;
#10416=VERTEX_POINT ( 'NONE', #57981 ) ;
#10417=CARTESIAN_POINT ( 'NONE',  ( 0.3962684609821412463, -8.656820664281497102, 34.87096338111211935 ) ) ;
#10418=EDGE_LOOP ( 'NONE', ( #44227, #9652 ) ) ;
#10419=AXIS2_PLACEMENT_3D ( 'NONE', #33289, #87811, #39613 ) ;
#10420=CARTESIAN_POINT ( 'NONE',  ( -10.36533030374629760, -9.148310452688876993, 34.47095581063188519 ) ) ;
#10421=CARTESIAN_POINT ( 'NONE',  ( 17.01165307636676260, -12.51329471203370325, 31.30864560766548976 ) ) ;
#10422=CARTESIAN_POINT ( 'NONE',  ( 12.39626801557768943, -2.625532179533445198, 30.86335684631481513 ) ) ;
#10423=FACE_BOUND ( 'NONE', #78723, .T. ) ;
#10425=CARTESIAN_POINT ( 'NONE',  ( 12.46153846153846168, -6.681629849574314051, 35.83090037661290239 ) ) ;
#10426=CARTESIAN_POINT ( 'NONE',  ( 1.384615384615386802, -12.62096338111211580, 30.90682066428153263 ) ) ;
#10427=CARTESIAN_POINT ( 'NONE',  ( 8.835299120233207404, -3.050289026998446840, 32.03036669348366416 ) ) ;
#10428=CARTESIAN_POINT ( 'NONE',  ( 17.14299142792551578, -8.973038597847269315, 34.52809138561122637 ) ) ;
#10430=EDGE_CURVE ( 'NONE', #35664, #22972, #21367, .T. ) ;
#10431=B_SPLINE_CURVE_WITH_KNOTS ( 'NONE', 3,
 ( #10326, #17077, #79675, #24267, #57180, #36901, #44533, #3996, #71570, #58491 ),
 .UNSPECIFIED., .F., .F.,
 ( 4, 2, 2, 2, 4 ),
 ( 0.0007817359430256326080, 0.0009771253907250047801, 0.001172514838424369796, 0.001367904286123735030, 0.001563293733823100046 ),
 .UNSPECIFIED. ) ;
#10432=CARTESIAN_POINT ( 'NONE',  ( 9.562160482869472844, -2.619462340734462380, 30.83744416345203021 ) ) ;
#10433=VERTEX_POINT ( 'NONE', #53442 ) ;
#10434=ADVANCED_FACE ( 'NONE', ( #20984 ), #88600, .F. ) ;
#10435=ORIENTED_EDGE ( 'NONE', *, *, #12690, .T. ) ;
#10436=CARTESIAN_POINT ( 'NONE',  ( -7.846153846153967493, -5.094484230521993062, 34.41647553114689373 ) ) ;
#10437=CARTESIAN_POINT ( 'NONE',  ( -1.634592128663975075, -5.643011162660950042, 34.66104346484419096 ) ) ;
#10438=CARTESIAN_POINT ( 'NONE',  ( -10.83831083290076158, -12.15238873228292071, 31.58232369045353849 ) ) ;
#10439=CARTESIAN_POINT ( 'NONE',  ( -3.903846153844716671, -7.500000000000155431, 34.75000000000007105 ) ) ;
#10440=CARTESIAN_POINT ( 'NONE',  ( 16.85409638444407321, -7.369208160676171460, 34.74850200257122879 ) ) ;
#10441=CARTESIAN_POINT ( 'NONE',  ( -15.23076923076935252, -3.643525952248795718, 33.31231777344771672 ) ) ;
#10442=VERTEX_POINT ( 'NONE', #53895 ) ;
#10443=DIRECTION ( 'NONE',  ( -0.000000000000000000, 0.3420201433256694346, -0.9396926207859080948 ) ) ;
#10444=ADVANCED_FACE ( 'NONE', ( #47126 ), #74617, .F. ) ;
#10445=DIRECTION ( 'NONE',  ( -0.000000000000000000, -0.3420201433256694346, -0.9396926207859080948 ) ) ;
#10446=CARTESIAN_POINT ( 'NONE',  ( 10.48523664565292002, -3.069018819979302926, 32.56621877034667278 ) ) ;
#10447=CARTESIAN_POINT ( 'NONE',  ( -13.51530598772569114, -12.62707690430377383, 30.88035979386743435 ) ) ;
#10448=ORIENTED_EDGE ( 'NONE', *, *, #72403, .F. ) ;
#10449=ORIENTED_EDGE ( 'NONE', *, *, #76096, .T. ) ;
#10450=FACE_BOUND ( 'NONE', #44497, .T. ) ;
#10451=VECTOR ( 'NONE', #52776, 1000.000000000000000 ) ;
#10452=ORIENTED_EDGE ( 'NONE', *, *, #37766, .F. ) ;
#10453=VECTOR ( 'NONE', #41095, 1000.000000000000114 ) ;
#10454=CARTESIAN_POINT ( 'NONE',  ( 18.22301284409339672, -12.64618726649961289, 30.78989965857442712 ) ) ;
#10455=CARTESIAN_POINT ( 'NONE',  ( -13.38461538461550582, -10.90142922262034020, 33.41473453929536674 ) ) ;
#10456=ORIENTED_EDGE ( 'NONE', *, *, #27115, .F. ) ;
#10457=DIRECTION ( 'NONE',  ( 0.000000000000000000, 0.8660254037844377084, 0.5000000000000015543 ) ) ;
#10458=CARTESIAN_POINT ( 'NONE',  ( 6.000000000000001776, -3.937682226553329556, 33.60647404775216529 ) ) ;
#10459=CARTESIAN_POINT ( 'NONE',  ( 0.7114839798866031684, -12.22109172314383052, 31.39792113162168263 ) ) ;
#10460=CARTESIAN_POINT ( 'NONE',  ( -1.161602540521988969, -4.026326845037962343, 33.68677907613344047 ) ) ;
#10461=ORIENTED_EDGE ( 'NONE', *, *, #62958, .F. ) ;
#10462=VECTOR ( 'NONE', #73879, 1000.000000000000227 ) ;
#10463=CARTESIAN_POINT ( 'NONE',  ( -3.931066612577742259, -6.760870238392817200, 34.69528174975672385 ) ) ;
#10464=EDGE_LOOP ( 'NONE', ( #57468, #25844, #77721, #42103 ) ) ;
#10465=CARTESIAN_POINT ( 'NONE',  ( -2.307692307692428724, -9.528491918059723176, 34.59228464037033035 ) ) ;
#10466=ORIENTED_EDGE ( 'NONE', *, *, #5175, .F. ) ;
#10467=CARTESIAN_POINT ( 'NONE',  ( -8.546451227962359454, -10.11255958852956027, 34.01340905677048454 ) ) ;
#10468=DIRECTION ( 'NONE',  ( -0.000000000000000000, -0.9848077530122086864, -0.1736481776669273613 ) ) ;
#10469=CARTESIAN_POINT ( 'NONE',  ( -0.4615384615384611200, -1.117168528481311540, 33.14645433367849847 ) ) ;
#10470=EDGE_CURVE ( 'NONE', #62031, #62397, #26871, .T. ) ;
#10471=CARTESIAN_POINT ( 'NONE',  ( 17.07692307692307665, -10.05456864172156806, 36.03766855953608683 ) ) ;
#10472=CARTESIAN_POINT ( 'NONE',  ( -14.43838291080261449, -8.191372820521381826, 34.95448215188424967 ) ) ;
#10473=LINE ( 'NONE', #85247, #43497 ) ;
#10476=CARTESIAN_POINT ( 'NONE',  ( 14.17700170458200226, -2.295517848115769421, 30.44137282052137294 ) ) ;
#10478=CARTESIAN_POINT ( 'NONE',  ( -0.3310127597748983574, -5.195472089885679878, 34.18748526763464213 ) ) ;
#10479=B_SPLINE_CURVE_WITH_KNOTS ( 'NONE', 3,
 ( #83048, #69964, #42066, #41173, #63199, #62311, #8276, #26768, #48802, #54227 ),
 .UNSPECIFIED., .F., .F.,
 ( 4, 2, 2, 2, 4 ),
 ( 0.000000000000000000, 0.0001954339857564063089, 0.0003908679715128126177, 0.0005863019572692189808, 0.0007817359430256252354 ),
 .UNSPECIFIED. ) ;
#10480=ORIENTED_EDGE ( 'NONE', *, *, #79759, .F. ) ;
#10481=ORIENTED_EDGE ( 'NONE', *, *, #10532, .T. ) ;
#10482=CARTESIAN_POINT ( 'NONE',  ( -1.634615384615389466, -2.499999999999999556, 29.81609845454691765 ) ) ;
#10483=CARTESIAN_POINT ( 'NONE',  ( 11.47319153790521717, -5.094484230520674117, 34.41647553114621161 ) ) ;
#10484=B_SPLINE_CURVE_WITH_KNOTS ( 'NONE', 3,
 ( #85064, #84627, #78286, #45386, #50368, #37747, #16153, #72859, #3066, #23778 ),
 .UNSPECIFIED., .F., .F.,
 ( 4, 2, 2, 2, 4 ),
 ( 0.000000000000000000, 0.0001954339857564096428, 0.0003908679715128192855, 0.0005863019572692289554, 0.0007817359430256385711 ),
 .UNSPECIFIED. ) ;
#10485=CARTESIAN_POINT ( 'NONE',  ( -4.946397638689432164, -12.70449254468099198, 30.44128974285582956 ) ) ;
#10486=DIRECTION ( 'NONE',  ( -0.000000000000000000, -0.9848077530122086864, -0.1736481776669273613 ) ) ;
#10487=LINE ( 'NONE', #37953, #18641 ) ;
#10488=AXIS2_PLACEMENT_3D ( 'NONE', #65977, #80403, #87611 ) ;
#10489=CARTESIAN_POINT ( 'NONE',  ( 16.15384615384603251, -11.94971097300221174, 32.03036669348237098 ) ) ;
#10490=CARTESIAN_POINT ( 'NONE',  ( -5.076923076923075762, -2.249999999999998668, 29.75000000000001776 ) ) ;
#10492=CARTESIAN_POINT ( 'NONE',  ( 3.007284287045283389, -6.760086850603068243, 34.69517049084099369 ) ) ;
#10493=CARTESIAN_POINT ( 'NONE',  ( -16.82692307692314415, -7.565270445406050648, 34.75000000000000000 ) ) ;
#10494=CARTESIAN_POINT ( 'NONE',  ( 6.923076923076800782, -6.835583212225970762, 34.95778746994575670 ) ) ;
#10496=ORIENTED_EDGE ( 'NONE', *, *, #84014, .F. ) ;
#10497=CARTESIAN_POINT ( 'NONE',  ( 10.61538461538461675, -9.058645607665452459, 34.76329471203371924 ) ) ;
#10498=ORIENTED_EDGE ( 'NONE', *, *, #38163, .T. ) ;
#10499=CARTESIAN_POINT ( 'NONE',  ( 15.00784301325308157, -11.24512374952581872, 33.06303171183252942 ) ) ;
#10502=DIRECTION ( 'NONE',  ( -0.000000000000000000, -0.5000000000000009992, -0.8660254037844380415 ) ) ;
#10503=ORIENTED_EDGE ( 'NONE', *, *, #48075, .T. ) ;
#10504=CARTESIAN_POINT ( 'NONE',  ( -2.557669051740897537, -6.524016743844655686, 34.90889640711025521 ) ) ;
#10505=CARTESIAN_POINT ( 'NONE',  ( -3.230769230769229949, -1.466349020453238561, 30.81389545987213907 ) ) ;
#10506=CARTESIAN_POINT ( 'NONE',  ( -3.230769230769229949, -8.810774026931790459, 35.74407628777942847 ) ) ;
#10507=CARTESIAN_POINT ( 'NONE',  ( 3.453782074862629337, -2.889357225399416862, 32.26129605718031002 ) ) ;
#10508=VERTEX_POINT ( 'NONE', #20552 ) ;
#10509=CARTESIAN_POINT ( 'NONE',  ( -0.7115151924808160722, -8.303909089506435137, 34.68538101551103381 ) ) ;
#10510=ORIENTED_EDGE ( 'NONE', *, *, #79259, .T. ) ;
#10511=DIRECTION ( 'NONE',  ( -0.000000000000000000, 0.3420201433256694901, -0.9396926207859082059 ) ) ;
#10512=B_SPLINE_CURVE_WITH_KNOTS ( 'NONE', 3,
 ( #4516, #31993, #65759, #66663, #59900, #11274, #4969, #4055, #52694, #65319 ),
 .UNSPECIFIED., .F., .F.,
 ( 4, 2, 2, 2, 4 ),
 ( 0.0007817359430256326080, 0.0009771253907249993591, 0.001172514838424366327, 0.001367904286123733078, 0.001563293733823099829 ),
 .UNSPECIFIED. ) ;
#10514=CYLINDRICAL_SURFACE ( 'NONE', #75079, 0.2499999999999986955 ) ;
#10515=AXIS2_PLACEMENT_3D ( 'NONE', #86207, #24925, #71776 ) ;
#10516=CARTESIAN_POINT ( 'NONE',  ( -3.296039676730005752, -12.27809138561121394, 31.22303859784730307 ) ) ;
#10517=CARTESIAN_POINT ( 'NONE',  ( -17.07692307692307665, -12.78798330534102767, 29.49999999999997868 ) ) ;
#10518=CARTESIAN_POINT ( 'NONE',  ( 5.076923076923383071, -2.506253911140614576, 30.00000000000323297 ) ) ;
#10519=CARTESIAN_POINT ( 'NONE',  ( 16.08857615328984281, -12.16647553114622049, 32.15551576947930812 ) ) ;
#10521=ORIENTED_EDGE ( 'NONE', *, *, #67361, .T. ) ;
#10523=ORIENTED_EDGE ( 'NONE', *, *, #5117, .T. ) ;
#10525=EDGE_LOOP ( 'NONE', ( #66337, #46151 ) ) ;
#10527=CARTESIAN_POINT ( 'NONE',  ( -1.319359813339359144, -12.46129190930001052, 30.37095296980870174 ) ) ;
#10528=DIRECTION ( 'NONE',  ( -0.000000000000000000, 0.5000000000000011102, -0.8660254037844380415 ) ) ;
#10529=DIRECTION ( 'NONE',  ( -0.000000000000000000, -0.6427876096865404731, -0.7660444431189771253 ) ) ;
#10530=CYLINDRICAL_SURFACE ( 'NONE', #29894, 0.2500000000000002220 ) ;
#10531=CARTESIAN_POINT ( 'NONE',  ( -12.68446542044531000, -12.38737895849757820, 31.66785238281580206 ) ) ;
#10532=EDGE_CURVE ( 'NONE', #87552, #63347, #74019, .T. ) ;
#10533=FACE_OUTER_BOUND ( 'NONE', #61216, .T. ) ;
#10534=CARTESIAN_POINT ( 'NONE',  ( -18.00000000000012079, -6.879047030192663392, 34.71129190930017927 ) ) ;
#10535=CARTESIAN_POINT ( 'NONE',  ( 7.846153846153723244, -2.379036618888197729, 30.90682066428292885 ) ) ;
#10536=EDGE_LOOP ( 'NONE', ( #38546, #69007, #54151, #33815 ) ) ;
#10537=EDGE_LOOP ( 'NONE', ( #81268, #81094 ) ) ;
#10538=EDGE_LOOP ( 'NONE', ( #3855, #29671, #36248, #36547 ) ) ;
#10539=CARTESIAN_POINT ( 'NONE',  ( 0.2386115026316112386, -2.889293201056495786, 32.26117774369186009 ) ) ;
#10540=VERTEX_POINT ( 'NONE', #12907 ) ;
#10542=LINE ( 'NONE', #18638, #40304 ) ;
#10543=CARTESIAN_POINT ( 'NONE',  ( 9.692307692307695177, -12.10708131394839349, 31.69288490824020244 ) ) ;
#10544=AXIS2_PLACEMENT_3D ( 'NONE', #1985, #10066, #23577 ) ;
#10545=DIRECTION ( 'NONE',  ( -0.000000000000000000, 0.6427876096865404731, -0.7660444431189770143 ) ) ;
#10546=CARTESIAN_POINT ( 'NONE',  ( -11.31568186948346977, -9.418065098278013636, 34.63729479722530158 ) ) ;
#10547=ORIENTED_EDGE ( 'NONE', *, *, #11925, .T. ) ;
#10548=ADVANCED_FACE ( 'NONE', ( #12468 ), #40831, .F. ) ;
#10549=ORIENTED_EDGE ( 'NONE', *, *, #36299, .F. ) ;
#10550=CARTESIAN_POINT ( 'NONE',  ( -11.78848476268299628, -12.07920672191015221, 32.31858351112116168 ) ) ;
#10551=VERTEX_POINT ( 'NONE', #40397 ) ;
#10552=FACE_BOUND ( 'NONE', #49761, .T. ) ;
#10554=CARTESIAN_POINT ( 'NONE',  ( -14.55766905174090020, -6.524016743844655686, 34.90889640711025521 ) ) ;
#10555=EDGE_LOOP ( 'NONE', ( #9976, #76996 ) ) ;
#10556=CARTESIAN_POINT ( 'NONE',  ( 17.77651505627605033, -2.847400154188068910, 31.58180166144859768 ) ) ;
#10559=EDGE_LOOP ( 'NONE', ( #51227, #43315 ) ) ;
#10560=FACE_OUTER_BOUND ( 'NONE', #50269, .T. ) ;
#10561=CYLINDRICAL_SURFACE ( 'NONE', #45178, 0.2500000000000002220 ) ;
#10563=CARTESIAN_POINT ( 'NONE',  ( 7.911408985666684046, -11.67786785259547777, 32.92929555188713664 ) ) ;
#10564=CARTESIAN_POINT ( 'NONE',  ( -9.442362282929646966, -9.357781135181031829, 34.66075350412533851 ) ) ;
#10565=ORIENTED_EDGE ( 'NONE', *, *, #45999, .T. ) ;
#10566=FACE_OUTER_BOUND ( 'NONE', #75774, .T. ) ;
#10567=CARTESIAN_POINT ( 'NONE',  ( -10.54931626438217585, -4.786620604624113540, 33.94971097300155805 ) ) ;
#10568=DIRECTION ( 'NONE',  ( -1.000000000000000000, -0.000000000000000000, -0.000000000000000000 ) ) ;
#10569=CARTESIAN_POINT ( 'NONE',  ( -10.39237326377176274, -5.667800583137506010, 34.40243808032445827 ) ) ;
#10570=FACE_OUTER_BOUND ( 'NONE', #8525, .T. ) ;
#10574=CARTESIAN_POINT ( 'NONE',  ( -15.45369544828537656, -12.39988816332205701, 30.74660775122750778 ) ) ;
#10575=CARTESIAN_POINT ( 'NONE',  ( -7.846153846153844924, -13.87047571288749737, 32.06866353760679544 ) ) ;
#10576=CARTESIAN_POINT ( 'NONE',  ( 4.153846153846030731, -5.094484230521993062, 34.41647553114689373 ) ) ;
#10577=CARTESIAN_POINT ( 'NONE',  ( -10.86536134632696715, -8.303909089506435137, 34.68538101551103381 ) ) ;
#10578=EDGE_CURVE ( 'NONE', #71586, #80366, #89034, .T. ) ;
#10580=VERTEX_POINT ( 'NONE', #74171 ) ;
#10584=VERTEX_POINT ( 'NONE', #13792 ) ;
#10587=VERTEX_POINT ( 'NONE', #75492 ) ;
#10588=CARTESIAN_POINT ( 'NONE',  ( -2.176900499867520988, -12.38066358083363738, 30.83685684665853444 ) ) ;
#10589=VERTEX_POINT ( 'NONE', #68739 ) ;
#10590=CARTESIAN_POINT ( 'NONE',  ( -5.869209559033048862, -9.929761469519744921, 34.40412654351204225 ) ) ;
#10592=CYLINDRICAL_SURFACE ( 'NONE', #21379, 0.2500000000000002220 ) ;
#10593=CARTESIAN_POINT ( 'NONE',  ( -9.942330916529147800, -12.68155406624981119, 30.59749803192733708 ) ) ;
#10594=CARTESIAN_POINT ( 'NONE',  ( -0.4615384615385826339, -6.026961402154118908, 34.52809138561165270 ) ) ;
#10595=CARTESIAN_POINT ( 'NONE',  ( -5.999999999999998224, -2.486705287966279876, 31.30864560766543647 ) ) ;
#10597=CARTESIAN_POINT ( 'NONE',  ( -7.596099534515531992, -2.779044189368096163, 31.39831045268886456 ) ) ;
#10598=CARTESIAN_POINT ( 'NONE',  ( 0.5267936010512987988, -2.657715359629131857, 31.77849191805844242 ) ) ;
#10600=DIRECTION ( 'NONE',  ( 0.000000000000000000, -6.938893903907222067E-15, 1.000000000000000000 ) ) ;
#10601=CARTESIAN_POINT ( 'NONE',  ( 5.076923076922954969, -8.613356846316285953, 34.62446782046622218 ) ) ;
#10603=EDGE_LOOP ( 'NONE', ( #41531, #61146, #802, #14183 ) ) ;
#10604=EDGE_LOOP ( 'NONE', ( #59159, #22755, #2203, #69060 ) ) ;
#10605=CARTESIAN_POINT ( 'NONE',  ( 14.55763782604044998, -5.057305518903948638, 34.11320923018887896 ) ) ;
#10606=CARTESIAN_POINT ( 'NONE',  ( -17.32694631421604115, -8.432397168068783699, 34.66272746175022945 ) ) ;
#10608=CARTESIAN_POINT ( 'NONE',  ( 5.142178648199100977, -2.892918686051625166, 31.69288490824025928 ) ) ;
#10609=CARTESIAN_POINT ( 'NONE',  ( 14.98076923076923173, -7.500000000000001776, 34.75000000000000000 ) ) ;
#10610=CARTESIAN_POINT ( 'NONE',  ( -16.28399336328437386, -9.418419913701741919, 34.36755862841477693 ) ) ;
#10611=AXIS2_PLACEMENT_3D ( 'NONE', #73251, #16197, #46224 ) ;
#10613=VERTEX_POINT ( 'NONE', #56558 ) ;
#10614=CARTESIAN_POINT ( 'NONE',  ( 7.596130621932389637, -2.985938066672154445, 32.43141759479405550 ) ) ;
#10615=ORIENTED_EDGE ( 'NONE', *, *, #15278, .T. ) ;
#10616=VERTEX_POINT ( 'NONE', #15135 ) ;
#10617=CARTESIAN_POINT ( 'NONE',  ( -9.626240358957616650, -2.833524468853757305, 32.15551576947925838 ) ) ;
#10618=CARTESIAN_POINT ( 'NONE',  ( -11.47239420511146157, -11.35647404775217595, 33.31231777344666511 ) ) ;
#10619=CARTESIAN_POINT ( 'NONE',  ( -13.38461538461550759, -2.657715359629662544, 31.77849191805970364 ) ) ;
#10620=CARTESIAN_POINT ( 'NONE',  ( 2.242421861731533017, -6.026961402152685388, 34.52809138561120506 ) ) ;
#10621=CARTESIAN_POINT ( 'NONE',  ( -2.307692307692305711, -11.69971097300155272, 32.46337939537588113 ) ) ;
#10622=EDGE_CURVE ( 'NONE', #53698, #71149, #35234, .T. ) ;
#10624=ORIENTED_EDGE ( 'NONE', *, *, #49933, .F. ) ;
#10626=VERTEX_POINT ( 'NONE', #2485 ) ;
#10627=VECTOR ( 'NONE', #66466, 1000.000000000000000 ) ;
#10628=CARTESIAN_POINT ( 'NONE',  ( 12.71153846153846523, -2.499999999999999556, 29.81604066197449754 ) ) ;
#10629=CARTESIAN_POINT ( 'NONE',  ( 9.757562831820528970, -2.379036618887895305, 30.90682066428158592 ) ) ;
#10630=B_SPLINE_CURVE_WITH_KNOTS ( 'NONE', 3,
 ( #75662, #68464, #62152, #54055, #61698, #81552, #7662, #33795, #69362, #27485 ),
 .UNSPECIFIED., .F., .F.,
 ( 4, 2, 2, 2, 4 ),
 ( 0.000000000000000000, 0.0001954339857564073388, 0.0003908679715128146777, 0.0005863019572692220165, 0.0007817359430256293554 ),
 .UNSPECIFIED. ) ;
#10632=VECTOR ( 'NONE', #23018, 1000.000000000000000 ) ;
#10633=VECTOR ( 'NONE', #34133, 1000.000000000000000 ) ;
#10634=CARTESIAN_POINT ( 'NONE',  ( -15.16470087976679437, -3.050289026998446840, 32.03036669348366416 ) ) ;
#10636=CARTESIAN_POINT ( 'NONE',  ( -4.403822884788508141, -8.303909089506435137, 34.68538101551103381 ) ) ;
#10637=DIRECTION ( 'NONE',  ( 0.000000000000000000, 0.9396926207859126468, 0.3420201433256571111 ) ) ;
#10638=VERTEX_POINT ( 'NONE', #1616 ) ;
#10639=EDGE_CURVE ( 'NONE', #22873, #86754, #87927, .T. ) ;
#10640=ORIENTED_EDGE ( 'NONE', *, *, #54380, .F. ) ;
#10642=ORIENTED_EDGE ( 'NONE', *, *, #41663, .F. ) ;
#10643=CARTESIAN_POINT ( 'NONE',  ( -12.46153846153858247, -11.48612834414049644, 32.76840700105863391 ) ) ;
#10644=ORIENTED_EDGE ( 'NONE', *, *, #68694, .F. ) ;
#10645=CARTESIAN_POINT ( 'NONE',  ( 1.134592147322421196, -10.05641848906368452, 34.04755513067966177 ) ) ;
#10646=CARTESIAN_POINT ( 'NONE',  ( -2.242437168179467033, -4.320704448112861584, 33.92786785259548310 ) ) ;
#10648=ORIENTED_EDGE ( 'NONE', *, *, #24978, .F. ) ;
#10649=ADVANCED_FACE ( 'NONE', ( #69622 ), #22327, .F. ) ;
#10650=DIRECTION ( 'NONE',  ( -0.000000000000000000, 1.000000000000000000, 3.491481338843133355E-15 ) ) ;
#10651=ORIENTED_EDGE ( 'NONE', *, *, #12299, .T. ) ;
#10652=CARTESIAN_POINT ( 'NONE',  ( -4.153846153846152411, -13.53365097954675988, 30.81389545987213552 ) ) ;
#10653=CARTESIAN_POINT ( 'NONE',  ( -7.053768389744479173, -2.729777683071817229, 31.24903638046268739 ) ) ;
#10654=FACE_BOUND ( 'NONE', #67921, .T. ) ;
#10655=LINE ( 'NONE', #64246, #57567 ) ;
#10657=ADVANCED_FACE ( 'NONE', ( #29975 ), #63308, .F. ) ;
#10658=CARTESIAN_POINT ( 'NONE',  ( 8.703960323269994248, -6.026961402152685388, 34.52809138561120506 ) ) ;
#10659=CARTESIAN_POINT ( 'NONE',  ( -3.480745974817821331, -8.347322224742351082, 34.93158281831414769 ) ) ;
#10660=EDGE_LOOP ( 'NONE', ( #80879, #42791, #16990, #56690 ) ) ;
#10662=EDGE_CURVE ( 'NONE', #69035, #44275, #39570, .T. ) ;
#10665=VECTOR ( 'NONE', #21643, 1000.000000000000114 ) ;
#10667=CARTESIAN_POINT ( 'NONE',  ( 12.33097786979653776, -2.504760397472875155, 29.97295953869789997 ) ) ;
#10669=DIRECTION ( 'NONE',  ( -1.000000000000000000, 0.000000000000000000, 0.000000000000000000 ) ) ;
#10670=CARTESIAN_POINT ( 'NONE',  ( 20.99999999999999645, -7.500000000000000000, 29.75000000000000355 ) ) ;
#10671=EDGE_CURVE ( 'NONE', #87581, #36938, #30916, .T. ) ;
#10672=FACE_BOUND ( 'NONE', #64893, .T. ) ;
#10673=CARTESIAN_POINT ( 'NONE',  ( 12.21151523731700550, -10.18141759479407327, 34.26406193332782379 ) ) ;
#10674=CARTESIAN_POINT ( 'NONE',  ( -10.36538461538455280, -7.434744860731433924, 35.00000000000000711 ) ) ;
#10676=CARTESIAN_POINT ( 'NONE',  ( -1.161835843346973318, -12.24180327182771855, 31.33663988360758168 ) ) ;
#10677=CYLINDRICAL_SURFACE ( 'NONE', #44893, 0.2499999999999973355 ) ;
#10678=CARTESIAN_POINT ( 'NONE',  ( 6.000000000000001776, -13.78497067705608181, 32.30358669280327177 ) ) ;
#10679=DIRECTION ( 'NONE',  ( 0.000000000000000000, 0.4999999999999960032, -0.8660254037844410391 ) ) ;
#10681=ORIENTED_EDGE ( 'NONE', *, *, #1596, .F. ) ;
#10682=CARTESIAN_POINT ( 'NONE',  ( 16.08857615328984281, -9.528491918058357157, 34.59228464037090589 ) ) ;
#10683=EDGE_CURVE ( 'NONE', #18413, #63168, #42754, .T. ) ;
#10684=EDGE_CURVE ( 'NONE', #67703, #44265, #57881, .T. ) ;
#10685=CARTESIAN_POINT ( 'NONE',  ( -14.30769230769230660, -1.466349020453238561, 30.81389545987213907 ) ) ;
#10686=DIRECTION ( 'NONE',  ( 0.000000000000000000, -6.938893903907222067E-15, 1.000000000000000000 ) ) ;
#10689=CARTESIAN_POINT ( 'NONE',  ( 5.326868486301118644, -12.07971442181322352, 32.31769673815850297 ) ) ;
#10691=CARTESIAN_POINT ( 'NONE',  ( -1.134615384615321076, -7.434744860731434812, 35.00000000000000711 ) ) ;
#10692=CARTESIAN_POINT ( 'NONE',  ( -2.242437168179467033, -6.835583212224609184, 34.95778746994559327 ) ) ;
#10693=CARTESIAN_POINT ( 'NONE',  ( -7.715628407920200438, -10.31582465632705237, 34.18122507451815295 ) ) ;
#10694=CARTESIAN_POINT ( 'NONE',  ( 5.076923076922953193, -12.70778746994576025, 30.41441678777401236 ) ) ;
#10695=CARTESIAN_POINT ( 'NONE',  ( -6.923076923077044142, -4.481592998941358097, 33.73612834414048933 ) ) ;
#10696=LINE ( 'NONE', #16556, #3703 ) ;
#10698=CARTESIAN_POINT ( 'NONE',  ( -18.22292621751615016, -2.758268499246660621, 31.33685645148950272 ) ) ;
#10699=CARTESIAN_POINT ( 'NONE',  ( 8.096208266067295156, -9.233818618650603938, 34.70587769442853698 ) ) ;
#10701=CARTESIAN_POINT ( 'NONE',  ( 3.296024370282069516, -12.51329471203373700, 31.30864560766537963 ) ) ;
#10702=CARTESIAN_POINT ( 'NONE',  ( 0.4615384615383396616, -10.90142922262034020, 33.41473453929536674 ) ) ;
#10705=DIRECTION ( 'NONE',  ( -0.000000000000000000, 0.9848077530122085754, -0.1736481776669273613 ) ) ;
#10708=ADVANCED_FACE ( 'NONE', ( #65968 ), #9695, .F. ) ;
#10709=CARTESIAN_POINT ( 'NONE',  ( -18.22292621751614305, -9.086856451489518705, 34.49173150075333183 ) ) ;
#10710=FACE_OUTER_BOUND ( 'NONE', #26145, .T. ) ;
#10711=CARTESIAN_POINT ( 'NONE',  ( 8.096099255531886030, -2.589246495874658383, 31.60778113518102828 ) ) ;
#10712=ORIENTED_EDGE ( 'NONE', *, *, #16924, .T. ) ;
#10713=CARTESIAN_POINT ( 'NONE',  ( -13.45069776397551564, -9.905515769479276145, 34.41647553114623292 ) ) ;
#10714=CARTESIAN_POINT ( 'NONE',  ( 17.14206785764270080, -7.750023224968865421, 34.99404313364389907 ) ) ;
#10715=CARTESIAN_POINT ( 'NONE',  ( -8.519176457592452678, -2.564540009722895419, 30.55348353981670684 ) ) ;
#10716=CYLINDRICAL_SURFACE ( 'NONE', #5434, 0.2500000000000008882 ) ;
#10717=ORIENTED_EDGE ( 'NONE', *, *, #26671, .F. ) ;
#10718=B_SPLINE_CURVE_WITH_KNOTS ( 'NONE', 3,
 ( #68742, #20987, #75069, #13355, #61531, #89039, #88160, #26435, #61978, #40400 ),
 .UNSPECIFIED., .F., .F.,
 ( 4, 2, 2, 2, 4 ),
 ( 0.0007817246256747484735, 0.0009771112852218928873, 0.001172497944769037084, 0.001367884604316181498, 0.001563271263863325912 ),
 .UNSPECIFIED. ) ;
#10719=CARTESIAN_POINT ( 'NONE',  ( -6.923076923076922462, -5.180354513474913603, 36.12317359536750416 ) ) ;
#10720=EDGE_CURVE ( 'NONE', #40851, #20364, #63142, .T. ) ;
#10722=CARTESIAN_POINT ( 'NONE',  ( -1.254089682851821763, -6.001044277235011215, 34.52024696741798948 ) ) ;
#10723=ORIENTED_EDGE ( 'NONE', *, *, #35617, .F. ) ;
#10724=ORIENTED_EDGE ( 'NONE', *, *, #4479, .F. ) ;
#10725=EDGE_CURVE ( 'NONE', #17506, #3164, #16849, .T. ) ;
#10726=VERTEX_POINT ( 'NONE', #58771 ) ;
#10727=ADVANCED_FACE ( 'NONE', ( #52453 ), #38061, .F. ) ;
#10728=DIRECTION ( 'NONE',  ( -0.000000000000000000, -0.8660254037844397068, -0.4999999999999978906 ) ) ;
#10729=CARTESIAN_POINT ( 'NONE',  ( 15.23076923076910916, -11.67786785259630911, 32.92929555188603530 ) ) ;
#10730=CARTESIAN_POINT ( 'NONE',  ( 2.372947878968333146, -6.026961402152789304, 34.52809138561124769 ) ) ;
#10731=EDGE_CURVE ( 'NONE', #60841, #82469, #59215, .T. ) ;
#10734=EDGE_LOOP ( 'NONE', ( #6754, #32538, #83656, #41931 ) ) ;
#10735=ORIENTED_EDGE ( 'NONE', *, *, #38234, .F. ) ;
#10736=CARTESIAN_POINT ( 'NONE',  ( 11.60452887181161508, -11.35647404775217595, 33.31231777344666511 ) ) ;
#10737=VERTEX_POINT ( 'NONE', #71838 ) ;
#10738=CARTESIAN_POINT ( 'NONE',  ( 6.792517009463559852, -2.254533558242299396, 29.97296025877828285 ) ) ;
#10739=CARTESIAN_POINT ( 'NONE',  ( 15.00784301325307979, -3.105860786376062332, 32.13614157043599562 ) ) ;
#10740=CARTESIAN_POINT ( 'NONE',  ( -8.769230769230890843, -12.46129190930018460, 30.37095296980731973 ) ) ;
#10741=CARTESIAN_POINT ( 'NONE',  ( -7.976301815885543434, -10.31621877034669588, 34.18098118002070152 ) ) ;
#10744=ORIENTED_EDGE ( 'NONE', *, *, #36401, .T. ) ;
#10745=EDGE_CURVE ( 'NONE', #11766, #18984, #8259, .T. ) ;
#10746=ORIENTED_EDGE ( 'NONE', *, *, #42753, .T. ) ;
#10747=CARTESIAN_POINT ( 'NONE',  ( 9.019285080869083870, -2.564540009722896752, 30.55348353981670684 ) ) ;
#10749=CARTESIAN_POINT ( 'NONE',  ( 3.100077764101675015, -11.71456829005830080, 32.44064028649416542 ) ) ;
#10750=CARTESIAN_POINT ( 'NONE',  ( 18.22277966897806678, -5.827830569534415694, 34.72679350104403539 ) ) ;
#10752=CARTESIAN_POINT ( 'NONE',  ( 9.692307692307695177, -1.790695186598648903, 34.54067556320373455 ) ) ;
#10753=DIRECTION ( 'NONE',  ( -0.000000000000000000, -0.5000000000000009992, -0.8660254037844380415 ) ) ;
#10754=CARTESIAN_POINT ( 'NONE',  ( 10.68145296638705410, -3.513871655860379306, 32.76840700105978499 ) ) ;
#10755=FACE_BOUND ( 'NONE', #31138, .T. ) ;
#10757=CARTESIAN_POINT ( 'NONE',  ( 9.942307692309128697, -7.500000000000155431, 34.75000000000007105 ) ) ;
#10758=CARTESIAN_POINT ( 'NONE',  ( 1.384615384615386802, -1.242168528481310874, 33.36296068462461051 ) ) ;
#10759=CARTESIAN_POINT ( 'NONE',  ( 17.07692307692295586, -9.528491918059723176, 34.59228464037033035 ) ) ;
#10761=CARTESIAN_POINT ( 'NONE',  ( 8.769230769230645706, -9.528491918059723176, 34.59228464037033035 ) ) ;
#10763=EDGE_LOOP ( 'NONE', ( #87595, #1507 ) ) ;
#10764=CARTESIAN_POINT ( 'NONE',  ( -6.000000000000119904, -11.94971097300221174, 32.03036669348237098 ) ) ;
#10765=B_SPLINE_CURVE_WITH_KNOTS ( 'NONE', 3,
 ( #63879, #2178, #71968, #76964, #15265, #16144, #36423, #36851, #22455, #17028 ),
 .UNSPECIFIED., .F., .F.,
 ( 4, 2, 2, 2, 4 ),
 ( 0.000000000000000000, 0.0001954311564186876063, 0.0003908623128373752125, 0.0005862934692560628188, 0.0007817246256747504250 ),
 .UNSPECIFIED. ) ;
#10766=LINE ( 'NONE', #59395, #32190 ) ;
#10767=VERTEX_POINT ( 'NONE', #45703 ) ;
#10768=B_SPLINE_CURVE_WITH_KNOTS ( 'NONE', 3,
 ( #19726, #13847, #41327, #62466, #81883, #53499, #6651, #27809, #80996, #46751 ),
 .UNSPECIFIED., .F., .F.,
 ( 4, 2, 2, 2, 4 ),
 ( 0.0007817246256747446788, 0.0009771112852218874663, 0.001172497944769030145, 0.001367884604316172825, 0.001563271263863315720 ),
 .UNSPECIFIED. ) ;
#10769=ORIENTED_EDGE ( 'NONE', *, *, #47227, .F. ) ;
#10770=CARTESIAN_POINT ( 'NONE',  ( 14.30769230769231015, -13.88283147151868846, 33.14645433367849847 ) ) ;
#10771=CARTESIAN_POINT ( 'NONE',  ( 1.319344938654610555, -10.90142922261923886, 33.41473453929638993 ) ) ;
#10772=CARTESIAN_POINT ( 'NONE',  ( 11.40777093535123399, -8.191372820521381826, 34.95448215188423546 ) ) ;
#10773=CARTESIAN_POINT ( 'NONE',  ( 0.4615384615383396616, -10.21337939537710326, 33.94971097300076224 ) ) ;
#10774=CARTESIAN_POINT ( 'NONE',  ( -3.480769230769229061, -2.499999999999998668, 29.75000000000000355 ) ) ;
#10775=VERTEX_POINT ( 'NONE', #24094 ) ;
#10777=EDGE_CURVE ( 'NONE', #27408, #62746, #54501, .T. ) ;
#10778=EDGE_CURVE ( 'NONE', #67178, #49738, #17983, .T. ) ;
#10779=CARTESIAN_POINT ( 'NONE',  ( 18.06525557127602610, -3.835265460703683349, 33.15142922261929925 ) ) ;
#10780=CARTESIAN_POINT ( 'NONE',  ( -9.758391103263571509, -4.098570777380719399, 33.41473453929634729 ) ) ;
#10781=CARTESIAN_POINT ( 'NONE',  ( -1.514763354347079316, -10.31621877034669588, 34.18098118002070152 ) ) ;
#10783=CARTESIAN_POINT ( 'NONE',  ( -16.82697766754503377, -2.589246495874658827, 31.60778113518102828 ) ) ;
#10785=ORIENTED_EDGE ( 'NONE', *, *, #3206, .F. ) ;
#10786=EDGE_CURVE ( 'NONE', #4262, #49317, #27982, .T. ) ;
#10787=ORIENTED_EDGE ( 'NONE', *, *, #59543, .F. ) ;
#10788=CARTESIAN_POINT ( 'NONE',  ( 14.30769230769231015, -10.51840700105979565, 33.73612834413961536 ) ) ;
#10789=ADVANCED_FACE ( 'NONE', ( #39413 ), #48687, .F. ) ;
#10790=CARTESIAN_POINT ( 'NONE',  ( -17.86995239374431677, -7.723484964179501588, 34.74522123443823318 ) ) ;
#10791=CARTESIAN_POINT ( 'NONE',  ( 8.769230769230647482, -12.27809138561165270, 31.22303859784587132 ) ) ;
#10792=CARTESIAN_POINT ( 'NONE',  ( -14.17690049986752321, -6.413143153341454017, 34.63066358083362672 ) ) ;
#10793=CARTESIAN_POINT ( 'NONE',  ( -0.5268084620947817154, -12.16647553114622049, 32.15551576947930812 ) ) ;
#10795=DIRECTION ( 'NONE',  ( -0.000000000000000000, -0.7660444431189791237, -0.6427876096865379196 ) ) ;
#10796=CARTESIAN_POINT ( 'NONE',  ( 14.24242230713598900, -6.835583212224499938, 34.95778746994557906 ) ) ;
#10798=ORIENTED_EDGE ( 'NONE', *, *, #71941, .F. ) ;
#10799=ADVANCED_FACE ( 'NONE', ( #55451 ), #76163, .F. ) ;
#10800=CARTESIAN_POINT ( 'NONE',  ( 17.07692307692295586, -12.27809138561165270, 31.22303859784587132 ) ) ;
#10801=CARTESIAN_POINT ( 'NONE',  ( -18.24999999999999289, -12.50000000000000000, 29.81604066197449043 ) ) ;
#10803=CARTESIAN_POINT ( 'NONE',  ( -15.23076923076922995, -2.538708090699994813, 30.37095296980875503 ) ) ;
#10804=CARTESIAN_POINT ( 'NONE',  ( -3.007806327207746211, -7.369474270740069777, 34.74850911626239736 ) ) ;
#10805=CARTESIAN_POINT ( 'NONE',  ( 6.923076923076924238, -2.292212530054420494, 30.41441678777542634 ) ) ;
#10806=CARTESIAN_POINT ( 'NONE',  ( -0.3307466537136740103, -11.18335022499818621, 33.13157742990016885 ) ) ;
#10807=CARTESIAN_POINT ( 'NONE',  ( -4.283993363284374745, -9.418419913701741919, 34.36755862841477693 ) ) ;
#10808=CARTESIAN_POINT ( 'NONE',  ( 15.45378058238208219, -11.24521262558773493, 33.06293181088029343 ) ) ;
#10809=EDGE_CURVE ( 'NONE', #79867, #5991, #5061, .T. ) ;
#10810=ORIENTED_EDGE ( 'NONE', *, *, #7910, .F. ) ;
#10812=CARTESIAN_POINT ( 'NONE',  ( 9.019285080869083870, -11.79725096376909654, 32.30694842903959341 ) ) ;
#10813=DIRECTION ( 'NONE',  ( -0.000000000000000000, 0.6427876096865404731, -0.7660444431189771253 ) ) ;
#10815=B_SPLINE_CURVE_WITH_KNOTS ( 'NONE', 3,
 ( #20906, #55139, #62333, #1973, #27669, #1533, #48377, #14156, #41632, #28565 ),
 .UNSPECIFIED., .F., .F.,
 ( 4, 2, 2, 2, 4 ),
 ( 0.000000000000000000, 0.0001954339857564073659, 0.0003908679715128147319, 0.0005863019572692221250, 0.0007817359430256294638 ),
 .UNSPECIFIED. ) ;
#10816=CARTESIAN_POINT ( 'NONE',  ( 0.3962684609821413573, -5.941354392334500467, 34.76329471203369792 ) ) ;
#10817=CARTESIAN_POINT ( 'NONE',  ( -17.20761454359064047, -2.541943142973489334, 30.39792223712631980 ) ) ;
#10818=ADVANCED_FACE ( 'NONE', ( #48244 ), #82935, .F. ) ;
#10820=ORIENTED_EDGE ( 'NONE', *, *, #74310, .T. ) ;
#10822=CARTESIAN_POINT ( 'NONE',  ( -15.48079245499068612, -4.175268141568685643, 33.81360843649122216 ) ) ;
#10823=B_SPLINE_CURVE_WITH_KNOTS ( 'NONE', 3,
 ( #77503, #1404, #82507, #15816, #55023, #70754, #48694, #14475, #14028, #61760 ),
 .UNSPECIFIED., .F., .F.,
 ( 4, 2, 2, 2, 4 ),
 ( 0.000000000000000000, 0.0001954311564186865221, 0.0003908623128373730441, 0.0005862934692560595662, 0.0007817246256747460882 ),
 .UNSPECIFIED. ) ;
#10824=ORIENTED_EDGE ( 'NONE', *, *, #6213, .F. ) ;
#10825=CARTESIAN_POINT ( 'NONE',  ( -4.153846153846274980, -2.657715359629662988, 31.77849191805970364 ) ) ;
#10826=ORIENTED_EDGE ( 'NONE', *, *, #70670, .F. ) ;
#10827=CARTESIAN_POINT ( 'NONE',  ( 13.38461538461526601, -12.46129190930018460, 30.37095296980731973 ) ) ;
#10828=ADVANCED_FACE ( 'NONE', ( #88822 ), #13579, .F. ) ;
#10829=CARTESIAN_POINT ( 'NONE',  ( -7.715628144390281662, -11.93748526763465279, 32.05452791011430946 ) ) ;
#10831=ORIENTED_EDGE ( 'NONE', *, *, #76048, .F. ) ;
#10832=CARTESIAN_POINT ( 'NONE',  ( -4.219116154402472674, -11.67786785259541027, 32.92929555188721480 ) ) ;
#10833=ORIENTED_EDGE ( 'NONE', *, *, #57453, .F. ) ;
#10835=EDGE_CURVE ( 'NONE', #22135, #519, #32982, .T. ) ;
#10836=EDGE_LOOP ( 'NONE', ( #62007, #72139 ) ) ;
#10837=CYLINDRICAL_SURFACE ( 'NONE', #21261, 0.2500000000000009437 ) ;
#10838=CARTESIAN_POINT ( 'NONE',  ( 2.438484115517093986, -3.062576670634119758, 32.05464942895959979 ) ) ;
#10839=ORIENTED_EDGE ( 'NONE', *, *, #16040, .T. ) ;
#10841=DIRECTION ( 'NONE',  ( -0.000000000000000000, 0.1736481776669307198, -0.9848077530122080203 ) ) ;
#10842=CARTESIAN_POINT ( 'NONE',  ( 10.74617642320940369, -3.062576670634119758, 32.05464942895959979 ) ) ;
#10843=CARTESIAN_POINT ( 'NONE',  ( -1.134669975237339701, -10.92531984108285670, 33.72920026020278073 ) ) ;
#10845=CARTESIAN_POINT ( 'NONE',  ( -14.30769230769230660, -9.905515769479276145, 34.41647553114623292 ) ) ;
#10846=CARTESIAN_POINT ( 'NONE',  ( -13.25408994638174320, -12.15418822224088835, 32.17964115625579069 ) ) ;
#10847=ORIENTED_EDGE ( 'NONE', *, *, #38090, .T. ) ;
#10848=ORIENTED_EDGE ( 'NONE', *, *, #76712, .F. ) ;
#10849=EDGE_CURVE ( 'NONE', #16242, #10922, #20778, .T. ) ;
#10850=VERTEX_POINT ( 'NONE', #70299 ) ;
#10851=CARTESIAN_POINT ( 'NONE',  ( 3.007842271862382066, -5.582147617184174848, 34.63737895849758530 ) ) ;
#10852=ORIENTED_EDGE ( 'NONE', *, *, #55315, .T. ) ;
#10853=B_SPLINE_CURVE_WITH_KNOTS ( 'NONE', 3,
 ( #13783, #41707, #20975, #62401, #22320, #51094, #23204, #2918, #30843, #16011 ),
 .UNSPECIFIED., .F., .F.,
 ( 4, 2, 2, 2, 4 ),
 ( 0.000000000000000000, 0.0001954339857564084773, 0.0003908679715128169545, 0.0005863019572692254860, 0.0007817359430256339090 ),
 .UNSPECIFIED. ) ;
#10854=CARTESIAN_POINT ( 'NONE',  ( -8.992715712954719720, -10.11188796281391511, 34.01382737946119050 ) ) ;
#10855=CARTESIAN_POINT ( 'NONE',  ( 9.942307692309128697, -7.500000000000155431, 34.75000000000007105 ) ) ;
#10856=ORIENTED_EDGE ( 'NONE', *, *, #2391, .T. ) ;
#10857=EDGE_CURVE ( 'NONE', #83807, #80479, #84505, .T. ) ;
#10859=EDGE_CURVE ( 'NONE', #11372, #18795, #25473, .T. ) ;
#10860=ORIENTED_EDGE ( 'NONE', *, *, #24978, .T. ) ;
#10861=CARTESIAN_POINT ( 'NONE',  ( 0.4615384615383382183, -8.656820664282941280, 34.87096338111179961 ) ) ;
#10862=ORIENTED_EDGE ( 'NONE', *, *, #75572, .T. ) ;
#10863=CARTESIAN_POINT ( 'NONE',  ( 11.60371710973756443, -11.48612834413965977, 32.76840700105972815 ) ) ;
#10864=EDGE_CURVE ( 'NONE', #5477, #55982, #21156, .T. ) ;
#10865=CARTESIAN_POINT ( 'NONE',  ( -7.976301055592061928, -2.619462340734462380, 30.83744416345203021 ) ) ;
#10866=CARTESIAN_POINT ( 'NONE',  ( -9.942307692307691624, -7.500000000000001776, 35.00000000000000000 ) ) ;
#10867=FACE_BOUND ( 'NONE', #78060, .T. ) ;
#10868=EDGE_LOOP ( 'NONE', ( #15970, #33705 ) ) ;
#10869=CYLINDRICAL_SURFACE ( 'NONE', #70112, 0.2499999999999995837 ) ;
#10871=CARTESIAN_POINT ( 'NONE',  ( 4.853996118016225658, -3.395401636524186362, 33.02366814457250399 ) ) ;
#10872=DIRECTION ( 'NONE',  ( -0.000000000000000000, -0.9848077530122085754, -0.1736481776669273613 ) ) ;
#10874=ORIENTED_EDGE ( 'NONE', *, *, #86920, .T. ) ;
#10875=DIRECTION ( 'NONE',  ( 0.000000000000000000, 0.9396926207859126468, -0.3420201433256571111 ) ) ;
#10877=VERTEX_POINT ( 'NONE', #85147 ) ;
#10878=CARTESIAN_POINT ( 'NONE',  ( -15.23076923076935252, -3.643525952248795718, 33.31231777344771672 ) ) ;
#10879=DIRECTION ( 'NONE',  ( 0.000000000000000000, 0.9396926207859126468, -0.3420201433256571111 ) ) ;
#10880=DIRECTION ( 'NONE',  ( -0.000000000000000000, -0.7660444431189791237, -0.6427876096865379196 ) ) ;
#10881=CARTESIAN_POINT ( 'NONE',  ( 2.307692307692309264, -2.499999999999998668, 29.50000000000001066 ) ) ;
#10882=CARTESIAN_POINT ( 'NONE',  ( -4.153846153846152411, -2.292212530054420494, 30.41441678777542634 ) ) ;
#10883=CARTESIAN_POINT ( 'NONE',  ( 14.05771556364371655, -2.920706130388546651, 32.31842814019191223 ) ) ;
#10884=EDGE_LOOP ( 'NONE', ( #36133, #10921 ) ) ;
#10885=VECTOR ( 'NONE', #6136, 1000.000000000000000 ) ;
#10886=CARTESIAN_POINT ( 'NONE',  ( -5.076923076923199218, -6.835583212225970762, 34.95778746994575670 ) ) ;
#10887=CYLINDRICAL_SURFACE ( 'NONE', #50233, 0.2499999999999994726 ) ;
#10888=CARTESIAN_POINT ( 'NONE',  ( -1.607541602131532077, -3.586966769969700763, 32.86292498521069660 ) ) ;
#10889=CARTESIAN_POINT ( 'NONE',  ( 14.43821774592595375, -2.647132371071621471, 31.75357179365171589 ) ) ;
#10891=EDGE_LOOP ( 'NONE', ( #39839, #16856 ) ) ;
#10892=FACE_BOUND ( 'NONE', #25233, .T. ) ;
#10893=VERTEX_POINT ( 'NONE', #22552 ) ;
#10894=CARTESIAN_POINT ( 'NONE',  ( -17.74999999976641973, -2.249999999999989786, 29.74999979494859303 ) ) ;
#10895=CARTESIAN_POINT ( 'NONE',  ( 5.010840697562940704, -2.833524468853757305, 32.15551576947924417 ) ) ;
#10896=EDGE_CURVE ( 'NONE', #80092, #61727, #78108, .T. ) ;
#10897=EDGE_LOOP ( 'NONE', ( #60211, #8273, #85221, #79989 ) ) ;
#10898=AXIS2_PLACEMENT_3D ( 'NONE', #84983, #14753, #50724 ) ;
#10900=CARTESIAN_POINT ( 'NONE',  ( 6.792929713638703682, -10.88202310037935661, 33.43294751532457099 ) ) ;
#10901=CARTESIAN_POINT ( 'NONE',  ( 4.826899839630108602, -2.823816976329319495, 31.52131813110795733 ) ) ;
#10902=DIRECTION ( 'NONE',  ( -0.000000000000000000, 0.1736481776669307198, -0.9848077530122080203 ) ) ;
#10903=CARTESIAN_POINT ( 'NONE',  ( -0.5276218724943415594, -11.16473453929635440, 33.15142922261925662 ) ) ;
#10904=ORIENTED_EDGE ( 'NONE', *, *, #12821, .F. ) ;
#10905=EDGE_CURVE ( 'NONE', #23097, #43624, #50885, .T. ) ;
#10906=CARTESIAN_POINT ( 'NONE',  ( -14.30769230769199929, -2.506253911140614576, 30.00000000000323297 ) ) ;
#10907=ORIENTED_EDGE ( 'NONE', *, *, #77754, .F. ) ;
#10908=CARTESIAN_POINT ( 'NONE',  ( -7.623374304885435215, -9.332535724633405749, 34.40230450496446934 ) ) ;
#10909=DIRECTION ( 'NONE',  ( -0.000000000000000000, -0.6427876096865404731, -0.7660444431189770143 ) ) ;
#10910=CARTESIAN_POINT ( 'NONE',  ( 12.46153846153846168, -13.20930481340135110, 34.54067556320372745 ) ) ;
#10911=CARTESIAN_POINT ( 'NONE',  ( 17.99999999999987566, -8.613356846316285953, 34.62446782046622218 ) ) ;
#10913=CARTESIAN_POINT ( 'NONE',  ( 6.000000000000001776, -2.721908614388771852, 31.22303859784724978 ) ) ;
#10914=EDGE_CURVE ( 'NONE', #45514, #42058, #16240, .T. ) ;
#10916=ORIENTED_EDGE ( 'NONE', *, *, #36409, .F. ) ;
#10917=DIRECTION ( 'NONE',  ( 0.000000000000000000, -0.000000000000000000, -1.000000000000000000 ) ) ;
#10918=CARTESIAN_POINT ( 'NONE',  ( -9.442362173959551797, -8.433404298154334455, 34.66254593164985920 ) ) ;
#10919=FACE_OUTER_BOUND ( 'NONE', #62962, .T. ) ;
#10920=VECTOR ( 'NONE', #19780, 1000.000000000000114 ) ;
#10921=ORIENTED_EDGE ( 'NONE', *, *, #41668, .T. ) ;
#10922=VERTEX_POINT ( 'NONE', #43704 ) ;
#10923=CARTESIAN_POINT ( 'NONE',  ( 9.823098133274648092, -3.338503747796866872, 32.95102852606553512 ) ) ;
#10924=CARTESIAN_POINT ( 'NONE',  ( 12.71159288145191724, -4.074993327901527351, 33.72946981652012255 ) ) ;
#10925=LINE ( 'NONE', #65853, #18818 ) ;
#10926=CARTESIAN_POINT ( 'NONE',  ( 10.39189967166066708, -5.912607949931405926, 34.49155766932282319 ) ) ;
#10927=CARTESIAN_POINT ( 'NONE',  ( 15.90386940979756503, -10.06842814019191401, 34.32929386961144758 ) ) ;
#10928=EDGE_CURVE ( 'NONE', #50664, #60409, #64853, .T. ) ;
#10929=CYLINDRICAL_SURFACE ( 'NONE', #31270, 0.2499999999999995559 ) ;
#10930=DIRECTION ( 'NONE',  ( -0.000000000000000000, 0.7660444431189791237, -0.6427876096865379196 ) ) ;
#10931=ORIENTED_EDGE ( 'NONE', *, *, #84971, .F. ) ;
#10932=CARTESIAN_POINT ( 'NONE',  ( 9.469381474791546793, -10.61292498521070549, 33.66303323003028680 ) ) ;
#10933=CARTESIAN_POINT ( 'NONE',  ( -0.4615384615384611200, -8.120952969808772792, 34.71129190930000163 ) ) ;
#10934=CARTESIAN_POINT ( 'NONE',  ( -6.130610359624526495, -7.722926236386453702, 34.74524107206102030 ) ) ;
#10935=CARTESIAN_POINT ( 'NONE',  ( 17.01165263096229907, -9.442884908240170461, 34.35708131394840592 ) ) ;
#10936=ORIENTED_EDGE ( 'NONE', *, *, #40498, .F. ) ;
#10937=CARTESIAN_POINT ( 'NONE',  ( 12.39545608217832218, -2.486705287966279432, 31.30864560766542937 ) ) ;
#10938=EDGE_CURVE ( 'NONE', #64231, #9817, #58537, .T. ) ;
#10939=ORIENTED_EDGE ( 'NONE', *, *, #16316, .T. ) ;
#10940=CARTESIAN_POINT ( 'NONE',  ( 8.769230769230768274, -5.180354513474913603, 36.12317359536750416 ) ) ;
#10941=CARTESIAN_POINT ( 'NONE',  ( -1.608100328339332252, -9.331801661448606566, 34.40259984581193464 ) ) ;
#10942=CARTESIAN_POINT ( 'NONE',  ( 15.23076923076923173, -7.500000000000001776, 35.04278698407183867 ) ) ;
#10944=EDGE_CURVE ( 'NONE', #11726, #43122, #76999, .T. ) ;
#10945=CARTESIAN_POINT ( 'NONE',  ( -10.61538461538461320, -1.466349020453238561, 30.81389545987213907 ) ) ;
#10946=CARTESIAN_POINT ( 'NONE',  ( 5.933916589044118339, -9.780366693483667717, 34.19971097300155805 ) ) ;
#10947=B_SPLINE_CURVE_WITH_KNOTS ( 'NONE', 3,
 ( #31795, #43960, #79084, #58805, #10628, #30886 ),
 .UNSPECIFIED., .F., .F.,
 ( 4, 2, 4 ),
 ( 0.0003909569690057805385, 0.0005862646681846044039, 0.0007815723673634283235 ),
 .UNSPECIFIED. ) ;
#10948=CARTESIAN_POINT ( 'NONE',  ( 10.61538461538449418, -12.70778746994576025, 30.41441678777401236 ) ) ;
#10949=CARTESIAN_POINT ( 'NONE',  ( -3.230769230769229949, -3.669653830205710676, 35.88435417666054406 ) ) ;
#10950=DIRECTION ( 'NONE',  ( 0.000000000000000000, 0.3420201433256610524, 0.9396926207859113145 ) ) ;
#10952=ORIENTED_EDGE ( 'NONE', *, *, #36402, .F. ) ;
#10953=CARTESIAN_POINT ( 'NONE',  ( 5.076923076923075762, -2.833524468853757305, 32.15551576947925838 ) ) ;
#10955=CARTESIAN_POINT ( 'NONE',  ( -15.23076923076922995, -6.343179335718451384, 34.87096338111211935 ) ) ;
#10956=FACE_OUTER_BOUND ( 'NONE', #36844, .T. ) ;
#10957=CARTESIAN_POINT ( 'NONE',  ( -0.4615384615384611200, -2.486705287966279876, 31.30864560766543647 ) ) ;
#10960=CARTESIAN_POINT ( 'NONE',  ( 4.854057654719437842, -2.501496062324911840, 29.88072118266895671 ) ) ;
#10961=CARTESIAN_POINT ( 'NONE',  ( 15.90382292962469535, -12.07920672191015221, 32.31858351112116168 ) ) ;
#10962=ADVANCED_FACE ( 'NONE', ( #73410 ), #74294, .F. ) ;
#10963=VERTEX_POINT ( 'NONE', #32417 ) ;
#10964=ORIENTED_EDGE ( 'NONE', *, *, #54687, .F. ) ;
#10965=ORIENTED_EDGE ( 'NONE', *, *, #3817, .F. ) ;
#10966=EDGE_CURVE ( 'NONE', #86663, #72654, #41592, .T. ) ;
#10967=EDGE_CURVE ( 'NONE', #70118, #57312, #11430, .T. ) ;
#10969=ORIENTED_EDGE ( 'NONE', *, *, #82126, .F. ) ;
#10970=CARTESIAN_POINT ( 'NONE',  ( -10.39260507411620260, -8.496831190052096971, 34.64984203495476578 ) ) ;
#10971=CARTESIAN_POINT ( 'NONE',  ( -11.78843826940389405, -9.148715823498378086, 34.47080413974185120 ) ) ;
#10972=EDGE_CURVE ( 'NONE', #37880, #48499, #24767, .T. ) ;
#10973=B_SPLINE_CURVE_WITH_KNOTS ( 'NONE', 3,
 ( #45400, #79204, #44954, #17501, #3966, #4885, #17050, #31451, #4421, #66579 ),
 .UNSPECIFIED., .F., .F.,
 ( 4, 2, 2, 2, 4 ),
 ( 0.0007817246256747515092, 0.0009771112852218961399, 0.001172497944769040554, 0.001367884604316184968, 0.001563271263863329598 ),
 .UNSPECIFIED. ) ;
#10974=CARTESIAN_POINT ( 'NONE',  ( -15.36091644020745051, -10.88202310037935661, 33.43294751532457099 ) ) ;
#10975=ADVANCED_FACE ( 'NONE', ( #46377 ), #46816, .F. ) ;
#10976=FACE_OUTER_BOUND ( 'NONE', #69430, .T. ) ;
#10977=DIRECTION ( 'NONE',  ( -0.000000000000000000, -0.8660254037844399289, -0.4999999999999980016 ) ) ;
#10978=CARTESIAN_POINT ( 'NONE',  ( -6.250023224221454399, -2.985938066672154445, 32.43141759479405550 ) ) ;
#10979=LINE ( 'NONE', #44285, #3298 ) ;
#10980=CARTESIAN_POINT ( 'NONE',  ( -4.153846153846273204, -10.90142922262034020, 33.41473453929536674 ) ) ;
#10981=CARTESIAN_POINT ( 'NONE',  ( 7.911408985666684046, -5.094484230520773593, 34.41647553114626845 ) ) ;
#10982=VERTEX_POINT ( 'NONE', #45478 ) ;
#10983=VERTEX_POINT ( 'NONE', #17578 ) ;
#10984=AXIS2_PLACEMENT_3D ( 'NONE', #10394, #11279, #18488 ) ;
#10985=EDGE_LOOP ( 'NONE', ( #80655, #15396, #16377, #88338 ) ) ;
#10986=CARTESIAN_POINT ( 'NONE',  ( 6.223012844093394946, -12.38742843783360748, 31.66772728687926985 ) ) ;
#10987=VERTEX_POINT ( 'NONE', #4500 ) ;
#10989=CARTESIAN_POINT ( 'NONE',  ( -17.86947456176635640, -11.66157788607254098, 32.95092075102925833 ) ) ;
#10990=CARTESIAN_POINT ( 'NONE',  ( 1.515405825582335941, -4.684288915650983043, 34.18129842949671371 ) ) ;
#10991=CARTESIAN_POINT ( 'NONE',  ( -11.53846153846166089, -9.528491918059723176, 34.59228464037033035 ) ) ;
#10992=FACE_BOUND ( 'NONE', #59052, .T. ) ;
#10993=EDGE_LOOP ( 'NONE', ( #73196, #31247 ) ) ;
#10994=VERTEX_POINT ( 'NONE', #25216 ) ;
#10995=CARTESIAN_POINT ( 'NONE',  ( -12.46153846153846168, -12.62096338111211580, 30.90682066428153263 ) ) ;
#10996=B_SPLINE_CURVE_WITH_KNOTS ( 'NONE', 3,
 ( #84155, #22432, #49897, #77374, #15684, #63856, #43150, #70620, #2155, #24646 ),
 .UNSPECIFIED., .F., .F.,
 ( 4, 2, 2, 2, 4 ),
 ( 0.000000000000000000, 0.0001954339857564082604, 0.0003908679715128165208, 0.0005863019572692248355, 0.0007817359430256330417 ),
 .UNSPECIFIED. ) ;
#10997=VERTEX_POINT ( 'NONE', #52678 ) ;
#10998=FACE_BOUND ( 'NONE', #53242, .T. ) ;
#10999=CARTESIAN_POINT ( 'NONE',  ( -17.07692307692307665, -12.78798330534103123, 29.99999999999997868 ) ) ;
#11001=DIRECTION ( 'NONE',  ( -0.000000000000000000, 0.7660444431189791237, -0.6427876096865379196 ) ) ;
#11002=ORIENTED_EDGE ( 'NONE', *, *, #55258, .T. ) ;
#11003=CARTESIAN_POINT ( 'NONE',  ( -1.384615384615506484, -5.941354392335915335, 34.76329471203413846 ) ) ;
#11005=CARTESIAN_POINT ( 'NONE',  ( -18.25002322422145440, -4.175268141568687419, 33.81360843649122216 ) ) ;
#11006=ORIENTED_EDGE ( 'NONE', *, *, #66327, .T. ) ;
#11007=CARTESIAN_POINT ( 'NONE',  ( 12.23805351781451201, -5.113361153441934093, 34.14387501736622710 ) ) ;
#11008=CARTESIAN_POINT ( 'NONE',  ( 7.146089767170319185, -5.582272713120727481, 34.63742843783360570 ) ) ;
#11009=EDGE_LOOP ( 'NONE', ( #44288, #30691, #10129, #28482 ) ) ;
#11010=CARTESIAN_POINT ( 'NONE',  ( -8.769230769230768274, -2.708943851104267164, 35.45975837776705220 ) ) ;
#11011=CARTESIAN_POINT ( 'NONE',  ( 7.173131234715237170, -10.66356715214248396, 33.62249196103329751 ) ) ;
#11012=ORIENTED_EDGE ( 'NONE', *, *, #26914, .T. ) ;
#11013=CARTESIAN_POINT ( 'NONE',  ( -12.59222906464877134, -5.496505350115501010, 34.60290016733514307 ) ) ;
#11014=CARTESIAN_POINT ( 'NONE',  ( 13.16113044089144068, -2.599994579823202923, 30.74605699353653776 ) ) ;
#11015=CARTESIAN_POINT ( 'NONE',  ( -16.15384615384615330, -8.120952969808772792, 34.71129190930000163 ) ) ;
#11016=CARTESIAN_POINT ( 'NONE',  ( -10.36543909703647159, -5.852078868378309373, 34.47109172314383585 ) ) ;
#11017=CARTESIAN_POINT ( 'NONE',  ( 2.307692307692309264, -4.945431358278436385, 36.03766855953609394 ) ) ;
#11018=VECTOR ( 'NONE', #62308, 1000.000000000000000 ) ;
#11019=CYLINDRICAL_SURFACE ( 'NONE', #85475, 0.2499999999999995559 ) ;
#11020=FACE_OUTER_BOUND ( 'NONE', #22202, .T. ) ;
#11021=CARTESIAN_POINT ( 'NONE',  ( 9.757562831820530747, -5.094484230520773593, 34.41647553114626845 ) ) ;
#11022=CARTESIAN_POINT ( 'NONE',  ( 10.61538461538449418, -9.528491918059723176, 34.59228464037033035 ) ) ;
#11023=DIRECTION ( 'NONE',  ( 0.000000000000000000, 0.1736481776669275834, 0.9848077530122086864 ) ) ;
#11024=DIRECTION ( 'NONE',  ( 0.000000000000000000, 0.000000000000000000, 1.000000000000000000 ) ) ;
#11026=ORIENTED_EDGE ( 'NONE', *, *, #86740, .T. ) ;
#11029=EDGE_LOOP ( 'NONE', ( #55903, #5368 ) ) ;
#11030=CARTESIAN_POINT ( 'NONE',  ( -7.715363405186893786, -2.494656445102013453, 31.33466734024120015 ) ) ;
#11031=VECTOR ( 'NONE', #53240, 1000.000000000000227 ) ;
#11032=EDGE_LOOP ( 'NONE', ( #86077, #43231, #74603, #66163 ) ) ;
#11033=CARTESIAN_POINT ( 'NONE',  ( -5.750054590621955342, -10.18230066228895758, 34.26354781536631577 ) ) ;
#11035=CARTESIAN_POINT ( 'NONE',  ( -18.00000000000000000, -5.557115091759784242, 34.35708131394839171 ) ) ;
#11036=CARTESIAN_POINT ( 'NONE',  ( -18.13069060311030611, -11.93127051446800024, 32.56575433478201376 ) ) ;
#11037=DIRECTION ( 'NONE',  ( -0.000000000000000000, -0.8660254037844399289, -0.4999999999999980016 ) ) ;
#11038=CARTESIAN_POINT ( 'NONE',  ( -6.065270000556317598, -2.657715359629089225, 31.77849191805834295 ) ) ;
#11040=CARTESIAN_POINT ( 'NONE',  ( -10.86536134632696715, -4.236021600441997492, 33.53823185664189310 ) ) ;
#11041=CARTESIAN_POINT ( 'NONE',  ( 5.933916589044120116, -4.098570777380720287, 33.41473453929634729 ) ) ;
#11043=CARTESIAN_POINT ( 'NONE',  ( -11.47320639894870276, -2.657715359629131857, 31.77849191805844242 ) ) ;
#11044=CARTESIAN_POINT ( 'NONE',  ( -2.241624974342230292, -11.91647553114624358, 32.58852847137148245 ) ) ;
#11045=CARTESIAN_POINT ( 'NONE',  ( -2.372962753653082846, -4.481592998940161721, 33.73612834413957984 ) ) ;
#11046=EDGE_CURVE ( 'NONE', #81511, #72329, #25988, .T. ) ;
#11048=VERTEX_POINT ( 'NONE', #81064 ) ;
#11049=AXIS2_PLACEMENT_3D ( 'NONE', #2396, #77183, #16803 ) ;
#11050=CARTESIAN_POINT ( 'NONE',  ( -13.45069776397551564, -6.343179335718451384, 34.87096338111212646 ) ) ;
#11051=CARTESIAN_POINT ( 'NONE',  ( -17.29984929443922681, -8.239355502252617924, 34.69524867566427417 ) ) ;
#11052=CARTESIAN_POINT ( 'NONE',  ( -1.384615384615383471, -13.87047571288749737, 32.06866353760679544 ) ) ;
#11053=CARTESIAN_POINT ( 'NONE',  ( -6.250023237292963607, -3.711651800289232916, 33.01384336483936011 ) ) ;
#11054=CYLINDRICAL_SURFACE ( 'NONE', #24793, 0.2499999999999995559 ) ;
#11055=B_SPLINE_CURVE_WITH_KNOTS ( 'NONE', 3,
 ( #43227, #72465, #10772, #71571, #50409, #70702, #3559, #30155, #78777, #57623 ),
 .UNSPECIFIED., .F., .F.,
 ( 4, 2, 2, 2, 4 ),
 ( 0.000000000000000000, 0.0001954311564186870913, 0.0003908623128373741825, 0.0005862934692560613009, 0.0007817246256747483650 ),
 .UNSPECIFIED. ) ;
#11057=CARTESIAN_POINT ( 'NONE',  ( 11.53846153846153832, -1.466349020453238561, 30.81389545987213907 ) ) ;
#11058=EDGE_CURVE ( 'NONE', #54717, #60134, #85613, .T. ) ;
#11059=AXIS2_PLACEMENT_3D ( 'NONE', #44550, #78346, #71150 ) ;
#11060=ORIENTED_EDGE ( 'NONE', *, *, #82172, .T. ) ;
#11061=DIRECTION ( 'NONE',  ( -0.000000000000000000, -0.8660254037844399289, -0.4999999999999980016 ) ) ;
#11063=ORIENTED_EDGE ( 'NONE', *, *, #31793, .F. ) ;
#11064=CARTESIAN_POINT ( 'NONE',  ( -5.934744428723973897, -6.026961402152789304, 34.52809138561124769 ) ) ;
#11066=CARTESIAN_POINT ( 'NONE',  ( -14.24162497434223162, -2.833524468853757305, 32.15551576947925838 ) ) ;
#11067=CARTESIAN_POINT ( 'NONE',  ( 6.222779668978068557, -8.540255544307065350, 34.89611431652622286 ) ) ;
#11068=CARTESIAN_POINT ( 'NONE',  ( -13.16183584334697443, -3.236590943229499029, 32.36255958852954251 ) ) ;
#11069=ORIENTED_EDGE ( 'NONE', *, *, #13412, .T. ) ;
#11070=VERTEX_POINT ( 'NONE', #86493 ) ;
#11071=AXIS2_PLACEMENT_3D ( 'NONE', #6833, #82517, #35196 ) ;
#11072=EDGE_CURVE ( 'NONE', #52884, #30224, #70623, .T. ) ;
#11073=EDGE_CURVE ( 'NONE', #50622, #47174, #26555, .T. ) ;
#11075=CARTESIAN_POINT ( 'NONE',  ( 11.53846153846141576, -9.528491918059723176, 34.59228464037033035 ) ) ;
#11077=FACE_OUTER_BOUND ( 'NONE', #19345, .T. ) ;
#11079=CARTESIAN_POINT ( 'NONE',  ( -11.78848476268299628, -8.475808217655753651, 34.90892951860618609 ) ) ;
#11080=CARTESIAN_POINT ( 'NONE',  ( -15.93106661257774626, -2.847695495035524438, 31.58253572463339154 ) ) ;
#11081=EDGE_LOOP ( 'NONE', ( #23055, #38895 ) ) ;
#11083=ORIENTED_EDGE ( 'NONE', *, *, #71200, .T. ) ;
#11084=CARTESIAN_POINT ( 'NONE',  ( 11.53846153846184563, -2.506253911140615021, 30.00000000000323297 ) ) ;
#11085=ORIENTED_EDGE ( 'NONE', *, *, #16962, .T. ) ;
#11086=CARTESIAN_POINT ( 'NONE',  ( 2.372947878968333590, -12.46129190930001052, 30.37095296980870174 ) ) ;
#11087=EDGE_LOOP ( 'NONE', ( #36165, #21532, #76178, #52157 ) ) ;
#11088=CARTESIAN_POINT ( 'NONE',  ( 8.096099364501988305, -12.43552623307873972, 30.55307653245132826 ) ) ;
#11089=CARTESIAN_POINT ( 'NONE',  ( -2.307692307692305711, -3.937682226553329556, 33.60647404775216529 ) ) ;
#11092=CARTESIAN_POINT ( 'NONE',  ( -13.60754160213153163, -12.15238873228292071, 31.58232369045353849 ) ) ;
#11093=ORIENTED_EDGE ( 'NONE', *, *, #35952, .F. ) ;
#11094=CARTESIAN_POINT ( 'NONE',  ( 5.869852030268307708, -9.504002272028875709, 34.60269587691767867 ) ) ;
#11095=CARTESIAN_POINT ( 'NONE',  ( 0.3308478584281527302, -11.37499894934982159, 33.29245874905763003 ) ) ;
#11096=FACE_BOUND ( 'NONE', #989, .T. ) ;
#11097=CARTESIAN_POINT ( 'NONE',  ( -0.2387587925603965044, -11.60474049983370648, 33.02348890104160262 ) ) ;
#11098=CARTESIAN_POINT ( 'NONE',  ( 23.00000000000000000, -9.499999999999982236, 27.74999999999999645 ) ) ;
#11099=CARTESIAN_POINT ( 'NONE',  ( -1.634592128663976185, -3.436278759898155233, 33.07459398097509506 ) ) ;
#11102=FACE_OUTER_BOUND ( 'NONE', #46034, .T. ) ;
#11103=CARTESIAN_POINT ( 'NONE',  ( 15.10007776410167502, -4.118384482072086072, 33.43331474514187107 ) ) ;
#11104=EDGE_LOOP ( 'NONE', ( #41554, #62892 ) ) ;
#11105=B_SPLINE_CURVE_WITH_KNOTS ( 'NONE', 3,
 ( #30040, #84553, #3441, #77336, #15643, #77775, #30908, #43110, #70583, #57499 ),
 .UNSPECIFIED., .F., .F.,
 ( 4, 2, 2, 2, 4 ),
 ( 0.000000000000000000, 0.0001954311564186882026, 0.0003908623128373764051, 0.0005862934692560646619, 0.0007817246256747528103 ),
 .UNSPECIFIED. ) ;
#11106=CARTESIAN_POINT ( 'NONE',  ( -8.519176349317319819, -3.435999193479609914, 33.07426656108010832 ) ) ;
#11107=CARTESIAN_POINT ( 'NONE',  ( -9.561782254074051579, -5.070358843744210198, 34.40418822224088302 ) ) ;
#11108=CARTESIAN_POINT ( 'NONE',  ( -6.249976730942353953, -10.66389620160130036, 33.62221079203477103 ) ) ;
#11111=FACE_BOUND ( 'NONE', #53189, .T. ) ;
#11112=CARTESIAN_POINT ( 'NONE',  ( 13.38461538461538680, -12.10708131394839349, 31.69288490824020244 ) ) ;
#11114=AXIS2_PLACEMENT_3D ( 'NONE', #88609, #11596, #86834 ) ;
#11115=CARTESIAN_POINT ( 'NONE',  ( -6.673131404728780858, -10.76462480002816235, 33.53768742498949962 ) ) ;
#11116=CARTESIAN_POINT ( 'NONE',  ( 3.165498784808455035, -4.481592998940161721, 33.73612834413957984 ) ) ;
#11118=CARTESIAN_POINT ( 'NONE',  ( 16.08857570788537572, -10.90142922261923886, 33.41473453929638993 ) ) ;
#11119=CARTESIAN_POINT ( 'NONE',  ( 6.000000000000001776, -1.367168528481310208, 33.57946703557072254 ) ) ;
#11122=CYLINDRICAL_SURFACE ( 'NONE', #57918, 0.2500000000000002220 ) ;
#11123=CARTESIAN_POINT ( 'NONE',  ( -15.10072162451355027, -7.723484964179501588, 34.74522123443823318 ) ) ;
#11124=LINE ( 'NONE', #79592, #57454 ) ;
#11125=CARTESIAN_POINT ( 'NONE',  ( 17.07692307692295586, -8.656820664282941280, 34.87096338111179961 ) ) ;
#11126=CARTESIAN_POINT ( 'NONE',  ( -4.403869378067609475, -4.931416488878822335, 34.32920672191015399 ) ) ;
#11127=CARTESIAN_POINT ( 'NONE',  ( 6.065255139512837346, -3.643525952247864463, 33.31231777344670064 ) ) ;
#11129=EDGE_CURVE ( 'NONE', #60966, #43000, #73821, .T. ) ;
#11130=CARTESIAN_POINT ( 'NONE',  ( -16.37733107841048508, -5.827078755546626354, 34.72654668319379567 ) ) ;
#11131=CARTESIAN_POINT ( 'NONE',  ( -7.846153846153844924, -2.708943851104267164, 35.45975837776705220 ) ) ;
#11132=CARTESIAN_POINT ( 'NONE',  ( 3.361294669002876212, -4.299079248970732792, 33.91157788607253565 ) ) ;
#11133=CARTESIAN_POINT ( 'NONE',  ( 9.626225312947559232, -3.937682226553330445, 33.60647404775217240 ) ) ;
#11134=CARTESIAN_POINT ( 'NONE',  ( 8.519254038288414321, -9.943427161483782584, 34.11278801902876978 ) ) ;
#11135=CARTESIAN_POINT ( 'NONE',  ( -8.769230769230768274, -8.973038597847269315, 34.52809138561121927 ) ) ;
#11136=VECTOR ( 'NONE', #54069, 999.9999999999998863 ) ;
#11138=CARTESIAN_POINT ( 'NONE',  ( 2.307692307692187583, -10.21337939537710326, 33.94971097300076224 ) ) ;
#11140=CYLINDRICAL_SURFACE ( 'NONE', #44143, 0.2499999999999994726 ) ;
#11141=LINE ( 'NONE', #37722, #33099 ) ;
#11144=EDGE_CURVE ( 'NONE', #86745, #19674, #41394, .T. ) ;
#11145=LINE ( 'NONE', #80506, #53372 ) ;
#11147=ORIENTED_EDGE ( 'NONE', *, *, #31665, .T. ) ;
#11148=CARTESIAN_POINT ( 'NONE',  ( -18.13069146666756382, -8.999036380462717588, 34.52022231692819076 ) ) ;
#11150=CARTESIAN_POINT ( 'NONE',  ( -7.623374177175780808, -12.47679350104403007, 31.42216943046557276 ) ) ;
#11152=CARTESIAN_POINT ( 'NONE',  ( 16.15384615384615330, -2.249999999999998668, 29.75000000000001776 ) ) ;
#11153=CARTESIAN_POINT ( 'NONE',  ( -2.530571824429892036, -7.630690623152302621, 34.99857592706774057 ) ) ;
#11156=DIRECTION ( 'NONE',  ( -0.000000000000000000, 0.9848077530122085754, -0.1736481776669273613 ) ) ;
#11157=DIRECTION ( 'NONE',  ( -0.000000000000000000, -0.3420201433256694901, -0.9396926207859082059 ) ) ;
#11158=EDGE_LOOP ( 'NONE', ( #10480, #83018 ) ) ;
#11159=CARTESIAN_POINT ( 'NONE',  ( -15.23076923076922995, -2.499999999999998668, 29.50000000000001066 ) ) ;
#11161=DIRECTION ( 'NONE',  ( -0.000000000000000000, 0.8660254037844397068, -0.4999999999999978906 ) ) ;
#11162=EDGE_CURVE ( 'NONE', #55982, #31594, #27875, .T. ) ;
#11163=ORIENTED_EDGE ( 'NONE', *, *, #46620, .F. ) ;
#11164=ORIENTED_EDGE ( 'NONE', *, *, #75215, .F. ) ;
#11166=EDGE_CURVE ( 'NONE', #77760, #56699, #408, .T. ) ;
#11167=VECTOR ( 'NONE', #41356, 1000.000000000000227 ) ;
#11168=CARTESIAN_POINT ( 'NONE',  ( 17.07692307692307665, -6.435427911321262684, 35.78748833219616898 ) ) ;
#11169=CARTESIAN_POINT ( 'NONE',  ( -3.007756386675832783, -2.889357225399416862, 32.26129605718031002 ) ) ;
#11170=CARTESIAN_POINT ( 'NONE',  ( -17.07692307692319744, -12.46129190930018460, 30.37095296980731973 ) ) ;
#11171=VECTOR ( 'NONE', #56824, 1000.000000000000227 ) ;
#11173=EDGE_CURVE ( 'NONE', #66677, #66580, #62003, .T. ) ;
#11174=EDGE_LOOP ( 'NONE', ( #49943, #70857 ) ) ;
#11176=CARTESIAN_POINT ( 'NONE',  ( -1.253823576790597860, -4.809403383903225304, 33.96459661697924304 ) ) ;
#11177=EDGE_CURVE ( 'NONE', #62136, #219, #74946, .T. ) ;
#11179=DIRECTION ( 'NONE',  ( -0.000000000000000000, 0.1736481776669307198, -0.9848077530122080203 ) ) ;
#11180=B_SPLINE_CURVE_WITH_KNOTS ( 'NONE', 3,
 ( #84098, #42223, #1216, #22376, #55715, #778, #77322, #8873, #48966, #34570 ),
 .UNSPECIFIED., .F., .F.,
 ( 4, 2, 2, 2, 4 ),
 ( 0.0007817246256747447872, 0.0009771112852218874663, 0.001172497944769030362, 0.001367884604316173258, 0.001563271263863315937 ),
 .UNSPECIFIED. ) ;
#11181=CYLINDRICAL_SURFACE ( 'NONE', #23472, 0.2500000000000002220 ) ;
#11182=EDGE_CURVE ( 'NONE', #75988, #86865, #37268, .T. ) ;
#11183=EDGE_CURVE ( 'NONE', #456, #17855, #72679, .T. ) ;
#11184=CARTESIAN_POINT ( 'NONE',  ( 6.000000000000001776, -9.584722331328613620, 36.20867863119891439 ) ) ;
#11185=DIRECTION ( 'NONE',  ( 0.000000000000000000, 0.000000000000000000, 1.000000000000000000 ) ) ;
#11186=ORIENTED_EDGE ( 'NONE', *, *, #26029, .F. ) ;
#11187=ORIENTED_EDGE ( 'NONE', *, *, #24631, .F. ) ;
#11188=ORIENTED_EDGE ( 'NONE', *, *, #41617, .T. ) ;
#11189=CYLINDRICAL_SURFACE ( 'NONE', #30076, 0.2500000000000008882 ) ;
#11190=ORIENTED_EDGE ( 'NONE', *, *, #69425, .T. ) ;
#11191=CARTESIAN_POINT ( 'NONE',  ( 16.85399611801622655, -5.582147617184174848, 34.63737895849758530 ) ) ;
#11192=VECTOR ( 'NONE', #20424, 1000.000000000000227 ) ;
#11193=CARTESIAN_POINT ( 'NONE',  ( -13.63459211555773720, -6.567427716900048118, 34.66269422305636283 ) ) ;
#11194=ORIENTED_EDGE ( 'NONE', *, *, #46588, .F. ) ;
#11195=FACE_OUTER_BOUND ( 'NONE', #49177, .T. ) ;
#11196=FACE_OUTER_BOUND ( 'NONE', #36285, .T. ) ;
#11197=CARTESIAN_POINT ( 'NONE',  ( 8.899756470994335089, -6.001044277235009439, 34.52024696741798948 ) ) ;
#11198=AXIS2_PLACEMENT_3D ( 'NONE', #47756, #49960, #13968 ) ;
#11199=FACE_BOUND ( 'NONE', #74650, .T. ) ;
#11200=CARTESIAN_POINT ( 'NONE',  ( 15.10007776410167324, -5.582088688514999397, 34.36776431015576350 ) ) ;
#11201=CARTESIAN_POINT ( 'NONE',  ( 2.373760658694747061, -8.120952969808772792, 34.71129190929999453 ) ) ;
#11202=CARTESIAN_POINT ( 'NONE',  ( -7.846153846153965716, -12.27809138561165270, 31.22303859784587132 ) ) ;
#11203=CARTESIAN_POINT ( 'NONE',  ( 16.15384615384615330, -3.937682226553329556, 33.60647404775216529 ) ) ;
#11204=CARTESIAN_POINT ( 'NONE',  ( 14.30769230769218581, -3.083524468854526912, 32.58852847137268327 ) ) ;
#11206=CARTESIAN_POINT ( 'NONE',  ( -0.4615384615384611200, -8.973038597847269315, 34.52809138561121927 ) ) ;
#11207=EDGE_LOOP ( 'NONE', ( #60888, #19930 ) ) ;
#11209=CARTESIAN_POINT ( 'NONE',  ( -17.30040800148741198, -5.827078755546626354, 34.72654668319379567 ) ) ;
#11210=CARTESIAN_POINT ( 'NONE',  ( 12.59232890250541281, -3.338503747796866872, 32.95102852606553512 ) ) ;
#11211=ORIENTED_EDGE ( 'NONE', *, *, #19148, .F. ) ;
#11212=EDGE_LOOP ( 'NONE', ( #14437, #11818 ) ) ;
#11213=B_SPLINE_CURVE_WITH_KNOTS ( 'NONE', 3,
 ( #193, #27660, #66996, #12491, #62759, #4848, #11607, #7839, #74191, #83057 ),
 .UNSPECIFIED., .F., .F.,
 ( 4, 2, 2, 2, 4 ),
 ( 0.0007817359430256288133, 0.0009771253907249948054, 0.001172514838424360689, 0.001367904286123726573, 0.001563293733823092457 ),
 .UNSPECIFIED. ) ;
#11214=CARTESIAN_POINT ( 'NONE',  ( -11.66860950819323328, -12.70455904226513866, 30.44083106164009322 ) ) ;
#11215=CARTESIAN_POINT ( 'NONE',  ( 1.450682717965462221, -5.471508081941601098, 34.59228464037088457 ) ) ;
#11216=CARTESIAN_POINT ( 'NONE',  ( 16.37662569511456567, -2.600157965045223563, 30.74683119005207033 ) ) ;
#11217=B_SPLINE_CURVE_WITH_KNOTS ( 'NONE', 3,
 ( #2756, #30251, #86088, #45084, #23478, #50935, #78871, #78426, #72113, #24363 ),
 .UNSPECIFIED., .F., .F.,
 ( 4, 2, 2, 2, 4 ),
 ( 0.000000000000000000, 0.0001954311564186862781, 0.0003908623128373725562, 0.0005862934692560588072, 0.0007817246256747451124 ),
 .UNSPECIFIED. ) ;
#11218=DIRECTION ( 'NONE',  ( -0.000000000000000000, -0.7660444431189791237, -0.6427876096865379196 ) ) ;
#11219=CARTESIAN_POINT ( 'NONE',  ( -11.53846153846153655, -9.905515769479276145, 34.41647553114623292 ) ) ;
#11220=B_SPLINE_CURVE_WITH_KNOTS ( 'NONE', 3,
 ( #41581, #53760, #69054, #39817, #26292, #74482, #12778, #60960, #88465, #15002 ),
 .UNSPECIFIED., .F., .F.,
 ( 4, 2, 2, 2, 4 ),
 ( 0.000000000000000000, 0.0001954339857564126514, 0.0003908679715128183098, 0.0005863019572692239681, 0.0007817359430256294638 ),
 .UNSPECIFIED. ) ;
#11221=ORIENTED_EDGE ( 'NONE', *, *, #65948, .T. ) ;
#11222=ADVANCED_FACE ( 'NONE', ( #16130 ), #9379, .F. ) ;
#11224=CARTESIAN_POINT ( 'NONE',  ( 4.403791563224197070, -4.932303261841489039, 34.32971442181322885 ) ) ;
#11225=CARTESIAN_POINT ( 'NONE',  ( 11.66898697669518192, -3.068774925481848825, 32.56582465632704526 ) ) ;
#11227=DIRECTION ( 'NONE',  ( -0.000000000000000000, -0.8660254037844397068, -0.4999999999999978906 ) ) ;
#11228=DIRECTION ( 'NONE',  ( -0.000000000000000000, 1.000000000000000000, -0.000000000000000000 ) ) ;
#11229=FACE_OUTER_BOUND ( 'NONE', #49290, .T. ) ;
#11231=EDGE_LOOP ( 'NONE', ( #53024, #81535 ) ) ;
#11233=VECTOR ( 'NONE', #28165, 1000.000000000000000 ) ;
#11234=LINE ( 'NONE', #58075, #75107 ) ;
#11235=CARTESIAN_POINT ( 'NONE',  ( -17.86947456176635640, -3.625058011473225150, 33.29252011169590020 ) ) ;
#11237=FACE_OUTER_BOUND ( 'NONE', #10367, .T. ) ;
#11238=CARTESIAN_POINT ( 'NONE',  ( 2.530655211253793890, -7.369474270740069777, 34.74850911626239736 ) ) ;
#11240=ADVANCED_FACE ( 'NONE', ( #22442 ), #62969, .F. ) ;
#11241=CARTESIAN_POINT ( 'NONE',  ( 8.769230769230768274, -3.937682226553329556, 33.60647404775216529 ) ) ;
#11242=DIRECTION ( 'NONE',  ( -0.000000000000000000, -0.9848077530122086864, -0.1736481776669273613 ) ) ;
#11243=VECTOR ( 'NONE', #47390, 1000.000000000000000 ) ;
#11244=CARTESIAN_POINT ( 'NONE',  ( -9.019253993452226226, -12.68155406624981119, 30.59749803192733708 ) ) ;
#11245=CARTESIAN_POINT ( 'NONE',  ( 11.53846153846153832, -12.10708131394839349, 31.69288490824020244 ) ) ;
#11246=CARTESIAN_POINT ( 'NONE',  ( -6.130147209438215228, -2.882441371585227063, 31.66841991370171527 ) ) ;
#11247=CARTESIAN_POINT ( 'NONE',  ( 14.17700084102474989, -12.11776431015576172, 31.66791131148498906 ) ) ;
#11248=FACE_OUTER_BOUND ( 'NONE', #40863, .T. ) ;
#11249=CARTESIAN_POINT ( 'NONE',  ( 7.846153846153723244, -8.656820664282941280, 34.87096338111179961 ) ) ;
#11250=CARTESIAN_POINT ( 'NONE',  ( 6.000000000000001776, -3.050289026998446396, 32.03036669348365706 ) ) ;
#11251=CARTESIAN_POINT ( 'NONE',  ( -4.219116599806927326, -9.442884908240170461, 34.35708131394840592 ) ) ;
#11252=DIRECTION ( 'NONE',  ( -0.000000000000000000, -0.6427876096865404731, -0.7660444431189771253 ) ) ;
#11253=ORIENTED_EDGE ( 'NONE', *, *, #23861, .F. ) ;
#11254=DIRECTION ( 'NONE',  ( -0.000000000000000000, -0.000000000000000000, -1.000000000000000000 ) ) ;
#11255=CARTESIAN_POINT ( 'NONE',  ( 8.835299120233207404, -11.69971097300155272, 32.46337939537588113 ) ) ;
#11258=EDGE_CURVE ( 'NONE', #72317, #54354, #42727, .T. ) ;
#11259=CARTESIAN_POINT ( 'NONE',  ( -14.17716660592874689, -5.195472089885680766, 34.18748526763464923 ) ) ;
#11260=CARTESIAN_POINT ( 'NONE',  ( 2.557746727605762160, -12.01375889529407637, 32.43194544308182969 ) ) ;
#11261=DIRECTION ( 'NONE',  ( 0.000000000000000000, 0.8660254037844377084, -0.5000000000000015543 ) ) ;
#11264=CARTESIAN_POINT ( 'NONE',  ( 3.230769230769231726, -8.973038597847269315, 34.52809138561121927 ) ) ;
#11265=EDGE_CURVE ( 'NONE', #86404, #45405, #57695, .T. ) ;
#11266=ORIENTED_EDGE ( 'NONE', *, *, #21243, .T. ) ;
#11267=LINE ( 'NONE', #59894, #44232 ) ;
#11268=ORIENTED_EDGE ( 'NONE', *, *, #35160, .T. ) ;
#11269=CARTESIAN_POINT ( 'NONE',  ( 9.692307692307695177, -1.790695186598648903, 34.54067556320373455 ) ) ;
#11271=CARTESIAN_POINT ( 'NONE',  ( 16.94623247381277054, -6.369640206132551441, 34.87707690430378449 ) ) ;
#11272=EDGE_CURVE ( 'NONE', #8235, #43627, #36179, .T. ) ;
#11273=VERTEX_POINT ( 'NONE', #77824 ) ;
#11274=CARTESIAN_POINT ( 'NONE',  ( -10.36533030374629938, -12.41262288849542017, 30.68299917996395010 ) ) ;
#11275=ORIENTED_EDGE ( 'NONE', *, *, #75105, .T. ) ;
#11276=CARTESIAN_POINT ( 'NONE',  ( 11.28843830116857383, -3.711651800289232028, 33.01384336483936011 ) ) ;
#11277=ORIENTED_EDGE ( 'NONE', *, *, #45726, .T. ) ;
#11278=CARTESIAN_POINT ( 'NONE',  ( 2.057669083470851756, -9.356822207818506598, 34.66110646841856635 ) ) ;
#11279=DIRECTION ( 'NONE',  ( -0.000000000000000000, 0.9396926207859093161, -0.3420201433256663259 ) ) ;
#11280=ORIENTED_EDGE ( 'NONE', *, *, #2831, .T. ) ;
#11281=CARTESIAN_POINT ( 'NONE',  ( 9.468822748583747284, -9.331801661448606566, 34.40259984581193464 ) ) ;
#11282=CYLINDRICAL_SURFACE ( 'NONE', #83835, 0.2499999999999973355 ) ;
#11283=CARTESIAN_POINT ( 'NONE',  ( 12.68454981315131214, -4.887748414852792322, 34.01359900205216746 ) ) ;
#11284=DIRECTION ( 'NONE',  ( -0.000000000000000000, -0.7660444431189791237, -0.6427876096865379196 ) ) ;
#11286=ORIENTED_EDGE ( 'NONE', *, *, #85056, .T. ) ;
#11287=VERTEX_POINT ( 'NONE', #71071 ) ;
#11288=ORIENTED_EDGE ( 'NONE', *, *, #36750, .T. ) ;
#11289=CARTESIAN_POINT ( 'NONE',  ( 3.453548772037640990, -3.755027918224367767, 33.06320215134714857 ) ) ;
#11290=ORIENTED_EDGE ( 'NONE', *, *, #25503, .F. ) ;
#11291=EDGE_CURVE ( 'NONE', #12426, #861, #81318, .T. ) ;
#11293=EDGE_CURVE ( 'NONE', #41920, #32972, #46844, .T. ) ;
#11294=DIRECTION ( 'NONE',  ( -0.000000000000000000, 0.1736481776669307198, -0.9848077530122080203 ) ) ;
#11295=CARTESIAN_POINT ( 'NONE',  ( -10.61538461538461320, -6.681629849574314051, 35.83090037661290239 ) ) ;
#11296=ORIENTED_EDGE ( 'NONE', *, *, #2486, .T. ) ;
#11297=ORIENTED_EDGE ( 'NONE', *, *, #58686, .F. ) ;
#11298=CARTESIAN_POINT ( 'NONE',  ( 17.32686848630112308, -9.357781135181033605, 34.66075350412533851 ) ) ;
#11299=EDGE_LOOP ( 'NONE', ( #36616, #71525 ) ) ;
#11300=DIRECTION ( 'NONE',  ( -0.000000000000000000, 0.3420201433256694901, -0.9396926207859082059 ) ) ;
#11301=AXIS2_PLACEMENT_3D ( 'NONE', #83895, #15429, #62703 ) ;
#11302=CARTESIAN_POINT ( 'NONE',  ( -8.069080063669993308, -2.554751324335734708, 30.48935550225260727 ) ) ;
#11304=CARTESIAN_POINT ( 'NONE',  ( -11.40767109749459074, -11.93129842949671726, 32.56571108434900452 ) ) ;
#11305=FACE_BOUND ( 'NONE', #44375, .T. ) ;
#11306=CARTESIAN_POINT ( 'NONE',  ( 5.076923076923075762, -6.435427911321262684, 35.78748833219616898 ) ) ;
#11307=DIRECTION ( 'NONE',  ( -0.000000000000000000, -0.7660444431189791237, -0.6427876096865379196 ) ) ;
#11309=CARTESIAN_POINT ( 'NONE',  ( -14.30769230769230660, -5.557115091759785130, 34.35708131394839171 ) ) ;
#11310=EDGE_CURVE ( 'NONE', #65891, #45448, #4841, .T. ) ;
#11311=CARTESIAN_POINT ( 'NONE',  ( 9.019176287578909879, -3.202959910592335646, 32.30730279482227019 ) ) ;
#11312=CARTESIAN_POINT ( 'NONE',  ( 7.912222197156284054, -10.51840700105979565, 33.73612834413962247 ) ) ;
#11313=ORIENTED_EDGE ( 'NONE', *, *, #35473, .T. ) ;
#11314=CARTESIAN_POINT ( 'NONE',  ( -11.53846153846166089, -3.643525952248795718, 33.31231777344771672 ) ) ;
#11315=ORIENTED_EDGE ( 'NONE', *, *, #69854, .F. ) ;
#11316=ORIENTED_EDGE ( 'NONE', *, *, #65950, .T. ) ;
#11317=CARTESIAN_POINT ( 'NONE',  ( 10.86533013373275836, -12.43552623307873972, 30.55307653245132826 ) ) ;
#11318=CARTESIAN_POINT ( 'NONE',  ( 10.74617642320940369, -5.582136614379148654, 34.36778462344220486 ) ) ;
#11319=CARTESIAN_POINT ( 'NONE',  ( 16.37685899793955357, -11.43677907613345113, 33.22367315496201456 ) ) ;
#11320=CARTESIAN_POINT ( 'NONE',  ( -13.38461538461550759, -12.16647553114689728, 32.15551576947799362 ) ) ;
#11322=CARTESIAN_POINT ( 'NONE',  ( -15.23076923076922995, -3.513871655860378418, 32.76840700105978499 ) ) ;
#11323=VERTEX_POINT ( 'NONE', #24658 ) ;
#11324=EDGE_CURVE ( 'NONE', #33070, #19283, #85440, .T. ) ;
#11325=CARTESIAN_POINT ( 'NONE',  ( 16.94623161025551639, -5.582088688514999397, 34.36776431015576350 ) ) ;
#11326=CARTESIAN_POINT ( 'NONE',  ( 3.007284306204901281, -9.417330523894424488, 34.63758898049880486 ) ) ;
#11327=CARTESIAN_POINT ( 'NONE',  ( 10.48469314871705649, -3.062553014421049546, 32.05460306192773601 ) ) ;
#11328=CARTESIAN_POINT ( 'NONE',  ( -4.153846153846152411, -3.513871655860378418, 32.76840700105978499 ) ) ;
#11329=ORIENTED_EDGE ( 'NONE', *, *, #61789, .T. ) ;
#11331=EDGE_CURVE ( 'NONE', #28697, #5010, #18935, .T. ) ;
#11332=ORIENTED_EDGE ( 'NONE', *, *, #35351, .T. ) ;
#11335=CARTESIAN_POINT ( 'NONE',  ( 18.25000000000006395, -7.434744429011175271, 34.75000000000000711 ) ) ;
#11336=CARTESIAN_POINT ( 'NONE',  ( -13.25408968285182176, -10.88167719472716399, 33.43325721877153711 ) ) ;
#11337=VERTEX_POINT ( 'NONE', #72838 ) ;
#11338=DIRECTION ( 'NONE',  ( 0.000000000000000000, 0.6427876096865373645, -0.7660444431189797898 ) ) ;
#11339=CYLINDRICAL_SURFACE ( 'NONE', #52913, 0.2499999999999994726 ) ;
#11340=CARTESIAN_POINT ( 'NONE',  ( 4.946775867484856093, -2.882441371585227063, 31.66841991370171527 ) ) ;
#11341=CARTESIAN_POINT ( 'NONE',  ( 14.55769230769374367, -7.500000000000155431, 34.75000000000007105 ) ) ;
#11342=EDGE_CURVE ( 'NONE', #68109, #88418, #65628, .T. ) ;
#11343=LINE ( 'NONE', #31159, #5741 ) ;
#11344=EDGE_LOOP ( 'NONE', ( #27919, #79427, #71422, #16865 ) ) ;
#11345=CYLINDRICAL_SURFACE ( 'NONE', #9388, 0.2500000000000014988 ) ;
#11347=CARTESIAN_POINT ( 'NONE',  ( -8.546219417617919589, -9.886259254753566594, 34.14407573483972413 ) ) ;
#11348=DIRECTION ( 'NONE',  ( -1.000000000000000000, -0.000000000000000000, -0.000000000000000000 ) ) ;
#11349=DIRECTION ( 'NONE',  ( 0.000000000000000000, 0.6427876096865368094, 0.7660444431189802339 ) ) ;
#11350=CARTESIAN_POINT ( 'NONE',  ( -10.68065461594093435, -3.643525952247789412, 33.31231777344662959 ) ) ;
#11351=CARTESIAN_POINT ( 'NONE',  ( 13.38461538461538680, -3.937682226553329556, 33.60647404775216529 ) ) ;
#11352=EDGE_CURVE ( 'NONE', #29059, #62900, #79068, .T. ) ;
#11353=CARTESIAN_POINT ( 'NONE',  ( 18.13052570176356681, -2.619367082507847666, 30.83698974864643461 ) ) ;
#11355=ORIENTED_EDGE ( 'NONE', *, *, #76532, .T. ) ;
#11356=DIRECTION ( 'NONE',  ( 0.000000000000000000, 0.9396926207859126468, 0.3420201433256571111 ) ) ;
#11357=DIRECTION ( 'NONE',  ( -0.000000000000000000, -0.6427876096865404731, -0.7660444431189771253 ) ) ;
#11359=B_SPLINE_CURVE_WITH_KNOTS ( 'NONE', 3,
 ( #11135, #80948, #19235, #72827, #80497, #25094, #67417, #52557, #18790, #80043 ),
 .UNSPECIFIED., .F., .F.,
 ( 4, 2, 2, 2, 4 ),
 ( 0.000000000000000000, 0.0001954339857564073659, 0.0003908679715128147319, 0.0005863019572692221250, 0.0007817359430256294638 ),
 .UNSPECIFIED. ) ;
#11361=ORIENTED_EDGE ( 'NONE', *, *, #22386, .T. ) ;
#11362=VERTEX_POINT ( 'NONE', #80050 ) ;
#11363=CARTESIAN_POINT ( 'NONE',  ( -8.899921372341079717, -5.496505350115501010, 34.60290016733514307 ) ) ;
#11364=CARTESIAN_POINT ( 'NONE',  ( -7.623141002060451754, -5.582272713120728369, 34.63742843783360570 ) ) ;
#11365=EDGE_CURVE ( 'NONE', #69312, #62369, #11145, .T. ) ;
#11366=CARTESIAN_POINT ( 'NONE',  ( 17.29993592101647693, -3.395485233115139501, 33.02377354290276656 ) ) ;
#11367=CARTESIAN_POINT ( 'NONE',  ( -8.835313148590902443, -10.67929555188718460, 33.92786785259543336 ) ) ;
#11368=EDGE_CURVE ( 'NONE', #11539, #73925, #28491, .T. ) ;
#11369=CARTESIAN_POINT ( 'NONE',  ( 16.21910129335899597, -3.643525952247864019, 33.31231777344670064 ) ) ;
#11370=AXIS2_PLACEMENT_3D ( 'NONE', #85909, #51649, #13354 ) ;
#11371=CARTESIAN_POINT ( 'NONE',  ( -15.00775638667583678, -8.282913670948747864, 34.94150082978203642 ) ) ;
#11372=VERTEX_POINT ( 'NONE', #45813 ) ;
#11373=CARTESIAN_POINT ( 'NONE',  ( 5.749976762707037281, -3.711651800289232916, 33.01384336483936011 ) ) ;
#11374=VECTOR ( 'NONE', #80465, 1000.000000000000114 ) ;
#11375=CARTESIAN_POINT ( 'NONE',  ( 16.15384615384615330, -1.242168528481310874, 33.36296068462461051 ) ) ;
#11376=CARTESIAN_POINT ( 'NONE',  ( 16.85343813319912698, -9.331801661448606566, 34.40259984581193464 ) ) ;
#11377=EDGE_LOOP ( 'NONE', ( #87127, #27031, #23662, #63551 ) ) ;
#11378=CARTESIAN_POINT ( 'NONE',  ( 10.39189969082028497, -9.417330523894424488, 34.63758898049880486 ) ) ;
#11379=ORIENTED_EDGE ( 'NONE', *, *, #84483, .T. ) ;
#11382=FACE_OUTER_BOUND ( 'NONE', #15092, .T. ) ;
#11383=CARTESIAN_POINT ( 'NONE',  ( 17.99999999999987566, -10.33852847137269571, 34.16647553114546554 ) ) ;
#11384=ORIENTED_EDGE ( 'NONE', *, *, #11817, .F. ) ;
#11385=DIRECTION ( 'NONE',  ( 1.000000000000000000, 0.000000000000000000, 0.000000000000000000 ) ) ;
#11386=LINE ( 'NONE', #88404, #36367 ) ;
#11387=DIRECTION ( 'NONE',  ( -0.000000000000000000, -0.8660254037844399289, -0.4999999999999980016 ) ) ;
#11388=B_SPLINE_CURVE_WITH_KNOTS ( 'NONE', 3,
 ( #46957, #75336, #75763, #41105, #5547, #559, #26256, #82977, #115, #74445 ),
 .UNSPECIFIED., .F., .F.,
 ( 4, 2, 2, 2, 4 ),
 ( 0.0007817246256747460882, 0.0009771112852218892010, 0.001172497944769032314, 0.001367884604316175210, 0.001563271263863318323 ),
 .UNSPECIFIED. ) ;
#11389=CARTESIAN_POINT ( 'NONE',  ( -6.130147969731695845, -5.915902021225892149, 34.75552854090298638 ) ) ;
#11390=CARTESIAN_POINT ( 'NONE',  ( -3.007757879156381264, -12.39991518177334129, 30.74647679643404530 ) ) ;
#11391=EDGE_LOOP ( 'NONE', ( #42646, #6891, #60136, #64086 ) ) ;
#11392=DIRECTION ( 'NONE',  ( 0.000000000000000000, -6.938893903907222067E-15, 1.000000000000000000 ) ) ;
#11393=EDGE_LOOP ( 'NONE', ( #42293, #4283, #64855, #33209 ) ) ;
#11396=CARTESIAN_POINT ( 'NONE',  ( 4.946775867484852540, -12.27039167877662251, 31.24851455888617835 ) ) ;
#11397=EDGE_CURVE ( 'NONE', #1287, #21191, #86585, .T. ) ;
#11398=FACE_OUTER_BOUND ( 'NONE', #23203, .T. ) ;
#11399=CARTESIAN_POINT ( 'NONE',  ( -8.769230769230768274, -13.57706302396349152, 30.56769352161908060 ) ) ;
#11401=CARTESIAN_POINT ( 'NONE',  ( -6.000000000000119904, -4.481592998941358097, 33.73612834414048933 ) ) ;
#11402=CARTESIAN_POINT ( 'NONE',  ( 9.692307692307572609, -8.613356846316285953, 34.62446782046622218 ) ) ;
#11404=ORIENTED_EDGE ( 'NONE', *, *, #33774, .T. ) ;
#11406=ORIENTED_EDGE ( 'NONE', *, *, #29559, .T. ) ;
#11407=ORIENTED_EDGE ( 'NONE', *, *, #73136, .T. ) ;
#11408=EDGE_LOOP ( 'NONE', ( #59627, #46853, #17136, #1841 ) ) ;
#11409=CARTESIAN_POINT ( 'NONE',  ( -16.21911659980693443, -3.835265460703609186, 33.15142922261924241 ) ) ;
#11410=CARTESIAN_POINT ( 'NONE',  ( -11.76138775597768671, -9.086856451489515152, 34.49173150075333183 ) ) ;
#11411=EDGE_CURVE ( 'NONE', #6875, #38908, #41422, .T. ) ;
#11412=CARTESIAN_POINT ( 'NONE',  ( -4.153846153846273204, -9.442884908241554243, 34.35708131394783038 ) ) ;
#11413=CARTESIAN_POINT ( 'NONE',  ( -7.146561866800870355, -3.236172620538810385, 32.36188796281390267 ) ) ;
#11414=CARTESIAN_POINT ( 'NONE',  ( -13.45069776397551564, -3.322132147404559532, 32.92929555188719348 ) ) ;
#11415=DIRECTION ( 'NONE',  ( -0.000000000000000000, -0.9848077530122085754, -0.1736481776669273613 ) ) ;
#11418=CARTESIAN_POINT ( 'NONE',  ( -5.299849294439221481, -8.239355502252617924, 34.69524867566427417 ) ) ;
#11419=CARTESIAN_POINT ( 'NONE',  ( -7.715628144390278997, -3.285477652293413264, 32.44071101563363158 ) ) ;
#11420=B_SPLINE_CURVE_WITH_KNOTS ( 'NONE', 3,
 ( #80019, #12016, #12886, #5686, #40376, #53876, #66953, #47556, #53422, #39048 ),
 .UNSPECIFIED., .F., .F.,
 ( 4, 2, 2, 2, 4 ),
 ( 0.000000000000000000, 0.0001954311564186865492, 0.0003908623128373730983, 0.0005862934692560596746, 0.0007817246256747461966 ),
 .UNSPECIFIED. ) ;
#11422=ORIENTED_EDGE ( 'NONE', *, *, #80030, .T. ) ;
#11423=ORIENTED_EDGE ( 'NONE', *, *, #66872, .T. ) ;
#11425=ORIENTED_EDGE ( 'NONE', *, *, #10683, .T. ) ;
#11426=FACE_OUTER_BOUND ( 'NONE', #17052, .T. ) ;
#11427=VERTEX_POINT ( 'NONE', #68754 ) ;
#11428=CYLINDRICAL_SURFACE ( 'NONE', #38881, 0.2500000000000008882 ) ;
#11429=FACE_OUTER_BOUND ( 'NONE', #18079, .T. ) ;
#11430=B_SPLINE_CURVE_WITH_KNOTS ( 'NONE', 3,
 ( #72506, #65742, #11259, #87380, #79276, #80624, #11713, #72958, #4039, #18022 ),
 .UNSPECIFIED., .F., .F.,
 ( 4, 2, 2, 2, 4 ),
 ( 0.0007817359430256287049, 0.0009771253907249945886, 0.001172514838424360255, 0.001367904286123725922, 0.001563293733823091806 ),
 .UNSPECIFIED. ) ;
#11431=CARTESIAN_POINT ( 'NONE',  ( -1.634638608836841200, -4.931416488878823223, 34.32920672191015399 ) ) ;
#11432=CARTESIAN_POINT ( 'NONE',  ( 7.053602624840487501, -2.619367082507848554, 30.83698974864644171 ) ) ;
#11433=FACE_BOUND ( 'NONE', #62326, .T. ) ;
#11434=VERTEX_POINT ( 'NONE', #61542 ) ;
#11435=EDGE_LOOP ( 'NONE', ( #46390, #9398, #11904, #10496 ) ) ;
#11437=EDGE_CURVE ( 'NONE', #78559, #27260, #35031, .T. ) ;
#11438=ORIENTED_EDGE ( 'NONE', *, *, #37757, .F. ) ;
#11439=FACE_BOUND ( 'NONE', #56805, .T. ) ;
#11441=CARTESIAN_POINT ( 'NONE',  ( -13.51530685128294351, -10.54014554554150607, 33.71984207302941883 ) ) ;
#11442=ORIENTED_EDGE ( 'NONE', *, *, #36567, .T. ) ;
#11443=CARTESIAN_POINT ( 'NONE',  ( -18.00000000000000000, -11.32085034345903729, 35.86790692298802696 ) ) ;
#11444=CARTESIAN_POINT ( 'NONE',  ( -1.607542343522232686, -8.282780595021769443, 34.94152052738834868 ) ) ;
#11445=CARTESIAN_POINT ( 'NONE',  ( -5.326923076923075762, -7.566082377512563184, 35.00000000000000711 ) ) ;
#11446=ORIENTED_EDGE ( 'NONE', *, *, #12302, .F. ) ;
#11447=DIRECTION ( 'NONE',  ( -0.000000000000000000, 0.8660254037844399289, -0.4999999999999980016 ) ) ;
#11448=CARTESIAN_POINT ( 'NONE',  ( 6.923076923076800782, -5.941354392335915335, 34.76329471203413846 ) ) ;
#11449=CARTESIAN_POINT ( 'NONE',  ( -5.299849294439221481, -11.76352882383564769, 32.36236540154569497 ) ) ;
#11450=ORIENTED_EDGE ( 'NONE', *, *, #35770, .F. ) ;
#11451=EDGE_CURVE ( 'NONE', #71975, #29766, #77798, .T. ) ;
#11452=CARTESIAN_POINT ( 'NONE',  ( -2.307692307692427391, -11.48612834414049644, 32.76840700105863391 ) ) ;
#11453=CARTESIAN_POINT ( 'NONE',  ( 6.989145274079362480, -10.51840700105979565, 33.73612834413962247 ) ) ;
#11454=EDGE_LOOP ( 'NONE', ( #11878, #46848 ) ) ;
#11455=CARTESIAN_POINT ( 'NONE',  ( -17.14300545628321260, -12.62096338111211580, 30.90682066428152908 ) ) ;
#11456=CARTESIAN_POINT ( 'NONE',  ( -5.076923076923075762, -9.905515769479276145, 34.41647553114623292 ) ) ;
#11457=CARTESIAN_POINT ( 'NONE',  ( 15.90386940979756503, -2.920706130388546651, 32.31842814019191223 ) ) ;
#11458=CARTESIAN_POINT ( 'NONE',  ( -11.53846153846165912, -3.300289026999228881, 32.46337939537708905 ) ) ;
#11459=CARTESIAN_POINT ( 'NONE',  ( -16.02305434602136103, -4.118422570099827595, 33.43335022499816489 ) ) ;
#11460=CARTESIAN_POINT ( 'NONE',  ( 17.07692307692295586, -6.026961402154118908, 34.52809138561165270 ) ) ;
#11461=CARTESIAN_POINT ( 'NONE',  ( -1.607541602131531633, -4.887634598454295265, 34.01352882383564946 ) ) ;
#11462=CARTESIAN_POINT ( 'NONE',  ( -15.29685264172511161, -12.37446782046654192, 30.86335684631486487 ) ) ;
#11463=ADVANCED_FACE ( 'NONE', ( #47142 ), #34525, .F. ) ;
#11464=EDGE_CURVE ( 'NONE', #1706, #66304, #296, .T. ) ;
#11466=CARTESIAN_POINT ( 'NONE',  ( -15.00798956179116317, -2.612705202774698421, 31.66806509827799943 ) ) ;
#11467=CARTESIAN_POINT ( 'NONE',  ( 12.23805353697412812, -4.988325925672468131, 34.36044203135681130 ) ) ;
#11468=B_SPLINE_CURVE_WITH_KNOTS ( 'NONE', 3,
 ( #82623, #26772, #20893, #69085, #34849, #62314, #28101, #83945, #76731, #50131 ),
 .UNSPECIFIED., .F., .F.,
 ( 4, 2, 2, 2, 4 ),
 ( 0.000000000000000000, 0.0001954339857564093175, 0.0003908679715128186350, 0.0005863019572692279796, 0.0007817359430256372700 ),
 .UNSPECIFIED. ) ;
#11469=AXIS2_PLACEMENT_3D ( 'NONE', #46341, #11678, #66157 ) ;
#11473=VERTEX_POINT ( 'NONE', #74630 ) ;
#11474=ORIENTED_EDGE ( 'NONE', *, *, #34582, .T. ) ;
#11475=CARTESIAN_POINT ( 'NONE',  ( -2.241623956689867470, -12.37446782046654192, 30.86335684631486842 ) ) ;
#11476=ORIENTED_EDGE ( 'NONE', *, *, #37138, .F. ) ;
#11477=CARTESIAN_POINT ( 'NONE',  ( -14.98071491913091791, -5.728107161865378494, 34.42597550085002922 ) ) ;
#11480=EDGE_CURVE ( 'NONE', #40124, #63956, #54342, .T. ) ;
#11481=CARTESIAN_POINT ( 'NONE',  ( 12.46153846153846168, -2.292212530054420494, 30.41441678777542634 ) ) ;
#11482=CARTESIAN_POINT ( 'NONE',  ( 9.942362112221147186, -9.233818618650603938, 34.70587769442853698 ) ) ;
#11483=CARTESIAN_POINT ( 'NONE',  ( 9.822833130541335223, -3.068774925481848825, 32.56582465632704526 ) ) ;
#11484=CARTESIAN_POINT ( 'NONE',  ( -10.54931728203453822, -3.322132147404559976, 32.92929555188717927 ) ) ;
#11485=FACE_OUTER_BOUND ( 'NONE', #32353, .T. ) ;
#11486=CARTESIAN_POINT ( 'NONE',  ( 0.4615384615383382183, -11.06231777344772027, 33.60647404775119895 ) ) ;
#11488=EDGE_CURVE ( 'NONE', #3191, #81167, #27763, .T. ) ;
#11490=CARTESIAN_POINT ( 'NONE',  ( 17.29993592101647693, -2.308499170217968022, 30.53291367094874076 ) ) ;
#11491=LINE ( 'NONE', #74084, #83706 ) ;
#11493=LINE ( 'NONE', #52017, #52187 ) ;
#11494=EDGE_CURVE ( 'NONE', #4654, #70883, #60709, .T. ) ;
#11495=CIRCLE ( 'NONE', #53199, 1.999999999999998224 ) ;
#11496=AXIS2_PLACEMENT_3D ( 'NONE', #73128, #4675, #46545 ) ;
#11497=EDGE_LOOP ( 'NONE', ( #77654, #61795, #2760, #45957 ) ) ;
#11499=CARTESIAN_POINT ( 'NONE',  ( 6.856993512121041690, -2.538708090699994813, 30.37095296980875148 ) ) ;
#11501=CARTESIAN_POINT ( 'NONE',  ( 16.37685899793954292, -12.38742843783360748, 31.66772728687926985 ) ) ;
#11502=CARTESIAN_POINT ( 'NONE',  ( -7.053767526187231240, -5.496505350115500121, 34.60290016733514307 ) ) ;
#11503=VECTOR ( 'NONE', #69412, 1000.000000000000114 ) ;
#11504=CARTESIAN_POINT ( 'NONE',  ( 8.769230769230647482, -11.94971097300221174, 32.03036669348237098 ) ) ;
#11509=CARTESIAN_POINT ( 'NONE',  ( 3.007284306204901281, -6.716662450894490100, 34.94144148231605840 ) ) ;
#11510=VERTEX_POINT ( 'NONE', #21453 ) ;
#11511=ORIENTED_EDGE ( 'NONE', *, *, #61274, .T. ) ;
#11514=CARTESIAN_POINT ( 'NONE',  ( 5.934243197485690402, -7.249945686854186278, 34.74374336980224598 ) ) ;
#11515=CARTESIAN_POINT ( 'NONE',  ( -9.469528151039281028, -6.760870238392817200, 34.69528174975672385 ) ) ;
#11516=CARTESIAN_POINT ( 'NONE',  ( 6.130525438233648039, -8.630441415882550871, 34.87705825610312615 ) ) ;
#11517=CARTESIAN_POINT ( 'NONE',  ( 17.07692307692307665, -9.780366693483667717, 34.19971097300155094 ) ) ;
#11518=ORIENTED_EDGE ( 'NONE', *, *, #56904, .T. ) ;
#11519=ORIENTED_EDGE ( 'NONE', *, *, #2936, .F. ) ;
#11520=B_SPLINE_CURVE_WITH_KNOTS ( 'NONE', 3,
 ( #28278, #42255, #1699, #6681, #61620, #62066, #48102, #35938, #7131, #8018 ),
 .UNSPECIFIED., .F., .F.,
 ( 4, 2, 2, 2, 4 ),
 ( 0.0007817359430256334753, 0.0009771253907250058643, 0.001172514838424371098, 0.001367904286123736764, 0.001563293733823101998 ),
 .UNSPECIFIED. ) ;
#11521=ORIENTED_EDGE ( 'NONE', *, *, #40172, .T. ) ;
#11523=CARTESIAN_POINT ( 'NONE',  ( 10.36540787133602670, -11.47974371597207899, 33.17467449705390692 ) ) ;
#11524=AXIS2_PLACEMENT_3D ( 'NONE', #31050, #3580, #80148 ) ;
#11526=CARTESIAN_POINT ( 'NONE',  ( -4.153846153846152411, -3.886160181151819604, 36.00935417666054406 ) ) ;
#11528=CARTESIAN_POINT ( 'NONE',  ( -11.78843828251013015, -8.347322224742351082, 34.93158281831414058 ) ) ;
#11529=DIRECTION ( 'NONE',  ( -0.000000000000000000, -0.6427876096865404731, -0.7660444431189770143 ) ) ;
#11530=ORIENTED_EDGE ( 'NONE', *, *, #16207, .F. ) ;
#11531=ORIENTED_EDGE ( 'NONE', *, *, #68224, .F. ) ;
#11532=CARTESIAN_POINT ( 'NONE',  ( -3.230769230769351186, -3.835265460704628371, 33.15142922262033665 ) ) ;
#11534=CARTESIAN_POINT ( 'NONE',  ( 15.36129493253280032, -6.001044277235009439, 34.52024696741798948 ) ) ;
#11535=VERTEX_POINT ( 'NONE', #7941 ) ;
#11536=CARTESIAN_POINT ( 'NONE',  ( -10.48459417441766206, -3.957578996910242619, 33.62503395064540257 ) ) ;
#11537=CARTESIAN_POINT ( 'NONE',  ( -9.692307692307812417, -11.94971097300221174, 32.03036669348237098 ) ) ;
#11539=VERTEX_POINT ( 'NONE', #62860 ) ;
#11540=AXIS2_PLACEMENT_3D ( 'NONE', #47977, #55621, #76797 ) ;
#11541=CARTESIAN_POINT ( 'NONE',  ( 10.68145194873469173, -2.292212530054420494, 30.41441678777542990 ) ) ;
#11542=VERTEX_POINT ( 'NONE', #70972 ) ;
#11543=CARTESIAN_POINT ( 'NONE',  ( 5.869309396889694774, -9.084618155246140248, 34.75535874321725771 ) ) ;
#11545=CARTESIAN_POINT ( 'NONE',  ( -17.07692307692307665, -11.91647553114624181, 32.58852847137148245 ) ) ;
#11546=CARTESIAN_POINT ( 'NONE',  ( -7.146003140593069958, -3.586966769969700763, 32.86292498521069660 ) ) ;
#11547=CARTESIAN_POINT ( 'NONE',  ( -15.00739329007105027, -2.501478030877323455, 29.88021232661721172 ) ) ;
#11548=VECTOR ( 'NONE', #40017, 1000.000000000000000 ) ;
#11549=CARTESIAN_POINT ( 'NONE',  ( 18.25005431163831560, -2.779044189368097051, 31.39831045268885745 ) ) ;
#11550=ORIENTED_EDGE ( 'NONE', *, *, #3160, .F. ) ;
#11551=ADVANCED_FACE ( 'NONE', ( #77720 ), #29114, .F. ) ;
#11552=CARTESIAN_POINT ( 'NONE',  ( 12.46153846153833911, -6.879047030192662504, 34.71129190930017927 ) ) ;
#11553=B_SPLINE_CURVE_WITH_KNOTS ( 'NONE', 3,
 ( #82109, #5561, #13639, #27597, #19949, #47416, #60939, #19512, #39797, #55069 ),
 .UNSPECIFIED., .F., .F.,
 ( 4, 2, 2, 2, 4 ),
 ( 0.000000000000000000, 0.0001954339857564078267, 0.0003908679715128156535, 0.0005863019572692235344, 0.0007817359430256313069 ),
 .UNSPECIFIED. ) ;
#11556=CARTESIAN_POINT ( 'NONE',  ( 5.076923076923075762, -12.29105614889573062, 35.45975837776705220 ) ) ;
#11557=ORIENTED_EDGE ( 'NONE', *, *, #81387, .T. ) ;
#11559=B_SPLINE_CURVE_WITH_KNOTS ( 'NONE', 3,
 ( #58315, #39845, #72277, #81276, #68198, #81717, #47022, #88934, #27205, #75831 ),
 .UNSPECIFIED., .F., .F.,
 ( 4, 2, 2, 2, 4 ),
 ( 0.0007817246256747455461, 0.0009771112852218885505, 0.001172497944769031663, 0.001367884604316174559, 0.001563271263863317672 ),
 .UNSPECIFIED. ) ;
#11562=CARTESIAN_POINT ( 'NONE',  ( -6.222926217516144831, -10.61292498521070549, 33.66303323003028680 ) ) ;
#11563=CARTESIAN_POINT ( 'NONE',  ( 11.40777007179397984, -5.582088688514999397, 34.36776431015576350 ) ) ;
#11564=CARTESIAN_POINT ( 'NONE',  ( 7.846153846153725020, -3.300289026999228881, 32.46337939537708905 ) ) ;
#11565=FACE_BOUND ( 'NONE', #15272, .T. ) ;
#11566=CARTESIAN_POINT ( 'NONE',  ( 12.46153846153833911, -10.33852847137269571, 34.16647553114546554 ) ) ;
#11568=EDGE_CURVE ( 'NONE', #62713, #56593, #48922, .T. ) ;
#11569=DIRECTION ( 'NONE',  ( -0.000000000000000000, 0.5000000000000011102, -0.8660254037844380415 ) ) ;
#11570=CARTESIAN_POINT ( 'NONE',  ( 1.134592160393928628, -12.68155406624981119, 30.59749803192733708 ) ) ;
#11571=DIRECTION ( 'NONE',  ( -0.000000000000000000, -0.6427876096865404731, -0.7660444431189771253 ) ) ;
#11572=CARTESIAN_POINT ( 'NONE',  ( 16.02315468717859304, -10.54014554554151140, 33.71984207302941883 ) ) ;
#11573=CARTESIAN_POINT ( 'NONE',  ( -8.638705067467203236, -3.816742781228458004, 33.13167719472716044 ) ) ;
#11575=CARTESIAN_POINT ( 'NONE',  ( -8.519285250882626670, -5.852078868378309373, 34.47109172314383585 ) ) ;
#11576=EDGE_LOOP ( 'NONE', ( #31568, #31942, #15757, #65307 ) ) ;
#11577=DIRECTION ( 'NONE',  ( -0.000000000000000000, 0.8660254037844399289, -0.4999999999999980016 ) ) ;
#11581=CARTESIAN_POINT ( 'NONE',  ( -10.36533019547116119, -12.01375889529407281, 32.43194544308182969 ) ) ;
#11582=CARTESIAN_POINT ( 'NONE',  ( 1.318533005255250412, -11.91647553114624181, 32.58852847137148245 ) ) ;
#11584=CARTESIAN_POINT ( 'NONE',  ( 2.307692307692309264, -11.69971097300155272, 32.46337939537588113 ) ) ;
#11585=DIRECTION ( 'NONE',  ( -0.000000000000000000, 0.7660444431189791237, -0.6427876096865379196 ) ) ;
#11586=CARTESIAN_POINT ( 'NONE',  ( -5.076923076923199218, -12.16647553114689728, 32.15551576947799362 ) ) ;
#11587=CARTESIAN_POINT ( 'NONE',  ( -0.7115616857599187384, -8.475808217655753651, 34.90892951860618609 ) ) ;
#11588=CARTESIAN_POINT ( 'NONE',  ( 14.37376065869474751, -5.557115091759786019, 34.35708131394839882 ) ) ;
#11589=CARTESIAN_POINT ( 'NONE',  ( 9.627037691751374027, -3.643525952247789412, 33.31231777344662959 ) ) ;
#11590=EDGE_CURVE ( 'NONE', #70275, #12547, #87713, .T. ) ;
#11591=CYLINDRICAL_SURFACE ( 'NONE', #53466, 0.2500000000000008882 ) ;
#11592=CARTESIAN_POINT ( 'NONE',  ( -11.47239318745910275, -10.51840700105979565, 33.73612834413962247 ) ) ;
#11594=B_SPLINE_CURVE_WITH_KNOTS ( 'NONE', 3,
 ( #29348, #49162, #64433, #1422, #36968, #22578, #50908, #83858, #69881, #36544 ),
 .UNSPECIFIED., .F., .F.,
 ( 4, 2, 2, 2, 4 ),
 ( 0.000000000000000000, 0.0001954339857564082062, 0.0003908679715128164124, 0.0005863019572692246186, 0.0007817359430256328248 ),
 .UNSPECIFIED. ) ;
#11595=AXIS2_PLACEMENT_3D ( 'NONE', #83148, #724, #43044 ) ;
#11596=DIRECTION ( 'NONE',  ( -0.000000000000000000, 0.9848077530122086864, -0.1736481776669273891 ) ) ;
#11597=CARTESIAN_POINT ( 'NONE',  ( 15.48071464014727283, -10.92531984108285670, 33.72920026020278073 ) ) ;
#11599=B_SPLINE_CURVE_WITH_KNOTS ( 'NONE', 3,
 ( #38063, #17348, #3828, #33535, #45705, #87605, #39851, #19128, #5168, #88496 ),
 .UNSPECIFIED., .F., .F.,
 ( 4, 2, 2, 2, 4 ),
 ( 0.0007817359430256287049, 0.0009771253907249945886, 0.001172514838424360255, 0.001367904286123725922, 0.001563293733823091806 ),
 .UNSPECIFIED. ) ;
#11600=CARTESIAN_POINT ( 'NONE',  ( -10.68065461594093435, -10.33852847137145048, 34.16647553114627556 ) ) ;
#11601=DIRECTION ( 'NONE',  ( -0.000000000000000000, -0.5000000000000009992, -0.8660254037844380415 ) ) ;
#11603=CARTESIAN_POINT ( 'NONE',  ( 0.4615384615383382183, -3.083524468854526912, 32.58852847137268327 ) ) ;
#11604=DIRECTION ( 'NONE',  ( -0.000000000000000000, -0.000000000000000000, -1.000000000000000000 ) ) ;
#11605=CARTESIAN_POINT ( 'NONE',  ( 4.826899852701617810, -12.45566812827425096, 31.48439005359158926 ) ) ;
#11606=ORIENTED_EDGE ( 'NONE', *, *, #8764, .T. ) ;
#11607=CARTESIAN_POINT ( 'NONE',  ( 11.76147289007438701, -4.887748414852792322, 34.01359900205216746 ) ) ;
#11608=DIRECTION ( 'NONE',  ( -0.000000000000000000, -0.1736481776669307198, -0.9848077530122080203 ) ) ;
#11609=DIRECTION ( 'NONE',  ( -0.000000000000000000, 0.5000000000000011102, -0.8660254037844381525 ) ) ;
#11611=VERTEX_POINT ( 'NONE', #56569 ) ;
#11612=DIRECTION ( 'NONE',  ( -0.000000000000000000, 0.7660444431189791237, -0.6427876096865379196 ) ) ;
#11613=LINE ( 'NONE', #39094, #39401 ) ;
#11615=CARTESIAN_POINT ( 'NONE',  ( -14.30769230769242739, -8.613356846316285953, 34.62446782046622218 ) ) ;
#11616=ORIENTED_EDGE ( 'NONE', *, *, #13906, .T. ) ;
#11617=ORIENTED_EDGE ( 'NONE', *, *, #58091, .F. ) ;
#11618=ORIENTED_EDGE ( 'NONE', *, *, #88423, .T. ) ;
#11619=VECTOR ( 'NONE', #39120, 1000.000000000000227 ) ;
#11620=AXIS2_PLACEMENT_3D ( 'NONE', #3221, #14979, #56404 ) ;
#11621=CARTESIAN_POINT ( 'NONE',  ( -9.942284423250045577, -2.779195860258146578, 31.39871582349836032 ) ) ;
#11622=CARTESIAN_POINT ( 'NONE',  ( -8.519176457592452678, -3.136992222400443175, 32.19305428654138979 ) ) ;
#11623=CARTESIAN_POINT ( 'NONE',  ( 13.13459214732242408, -11.37209801155882793, 32.91403422569033665 ) ) ;
#11624=AXIS2_PLACEMENT_3D ( 'NONE', #44976, #63923, #50836 ) ;
#11626=CARTESIAN_POINT ( 'NONE',  ( 14.98079249982687955, -3.627789207965226748, 32.91389620160131102 ) ) ;
#11627=VERTEX_POINT ( 'NONE', #35861 ) ;
#11628=B_SPLINE_CURVE_WITH_KNOTS ( 'NONE', 3,
 ( #4760, #52922, #25911, #80421, #19156, #73215, #74104, #12398, #3852, #32229 ),
 .UNSPECIFIED., .F., .F.,
 ( 4, 2, 2, 2, 4 ),
 ( 0.000000000000000000, 0.0001954311564186879315, 0.0003908623128373758630, 0.0005862934692560637946, 0.0007817246256747517261 ),
 .UNSPECIFIED. ) ;
#11629=EDGE_LOOP ( 'NONE', ( #49623, #62547, #46773, #80321 ) ) ;
#11630=CARTESIAN_POINT ( 'NONE',  ( 4.403900573759606196, -5.642605341092957083, 34.66089969410670335 ) ) ;
#11631=ORIENTED_EDGE ( 'NONE', *, *, #88013, .F. ) ;
#11632=B_SPLINE_CURVE_WITH_KNOTS ( 'NONE', 3,
 ( #26507, #43120, #29611, #49864, #2124, #57067, #49434, #64254, #16088, #8454 ),
 .UNSPECIFIED., .F., .F.,
 ( 4, 2, 2, 2, 4 ),
 ( 0.0007817246256747481482, 0.0009771112852218909357, 0.001172497944769033832, 0.001367884604316176728, 0.001563271263863319407 ),
 .UNSPECIFIED. ) ;
#11633=CARTESIAN_POINT ( 'NONE',  ( -6.792551484843277976, -4.299079248970732792, 33.91157788607253565 ) ) ;
#11634=B_SPLINE_CURVE_WITH_KNOTS ( 'NONE', 3,
 ( #42616, #56124, #13804, #68750, #7048, #34522, #61987, #49367, #27760, #83614 ),
 .UNSPECIFIED., .F., .F.,
 ( 4, 2, 2, 2, 4 ),
 ( 0.0007817359430256364027, 0.0009771253907250043464, 0.001172514838424372399, 0.001367904286123740234, 0.001563293733823108286 ),
 .UNSPECIFIED. ) ;
#11635=FACE_OUTER_BOUND ( 'NONE', #36575, .T. ) ;
#11636=CARTESIAN_POINT ( 'NONE',  ( 1.449870955891410906, -10.90142922261932057, 33.41473453929631887 ) ) ;
#11637=CARTESIAN_POINT ( 'NONE',  ( -7.846153846153967493, -10.33852847137269571, 34.16647553114546554 ) ) ;
#11638=ORIENTED_EDGE ( 'NONE', *, *, #5379, .T. ) ;
#11639=B_SPLINE_CURVE_WITH_KNOTS ( 'NONE', 3,
 ( #47237, #75172, #67967, #40938, #82372, #68400, #6698, #69295, #34170, #61636 ),
 .UNSPECIFIED., .F., .F.,
 ( 4, 2, 2, 2, 4 ),
 ( 0.000000000000000000, 0.0001954311564186864407, 0.0003908623128373728815, 0.0005862934692560593493, 0.0007817246256747457630 ),
 .UNSPECIFIED. ) ;
#11640=ORIENTED_EDGE ( 'NONE', *, *, #58514, .F. ) ;
#11641=ORIENTED_EDGE ( 'NONE', *, *, #80830, .T. ) ;
#11642=LINE ( 'NONE', #80556, #11619 ) ;
#11643=CARTESIAN_POINT ( 'NONE',  ( 5.076923076922954969, -5.219633306517616589, 34.19971097300220464 ) ) ;
#11644=ORIENTED_EDGE ( 'NONE', *, *, #59706, .T. ) ;
#11645=EDGE_CURVE ( 'NONE', #68166, #78927, #1552, .T. ) ;
#11646=CARTESIAN_POINT ( 'NONE',  ( 18.25005441991345734, -12.01375889529407992, 32.43194544308182969 ) ) ;
#11648=CARTESIAN_POINT ( 'NONE',  ( 12.39626801557768765, -11.48612834413959582, 32.76840700105983473 ) ) ;
#11649=CARTESIAN_POINT ( 'NONE',  ( -13.51530685128294529, -4.118384482072085184, 33.43331474514187107 ) ) ;
#11651=CARTESIAN_POINT ( 'NONE',  ( -13.51517597635730539, -2.504760397472875155, 29.97295953869789997 ) ) ;
#11652=CARTESIAN_POINT ( 'NONE',  ( 8.992242120843620512, -5.667800583137506010, 34.40243808032445827 ) ) ;
#11653=FACE_BOUND ( 'NONE', #12992, .T. ) ;
#11654=CARTESIAN_POINT ( 'NONE',  ( -0.4615384615384611200, -4.098570777380720287, 33.41473453929634729 ) ) ;
#11655=LINE ( 'NONE', #45865, #27027 ) ;
#11656=EDGE_CURVE ( 'NONE', #16922, #72102, #76395, .T. ) ;
#11657=CARTESIAN_POINT ( 'NONE',  ( -8.899377978668990608, -4.460286881179643004, 33.72017969459903242 ) ) ;
#11659=CARTESIAN_POINT ( 'NONE',  ( -5.933931648997560870, -2.721908614388772296, 31.22303859784725333 ) ) ;
#11660=CARTESIAN_POINT ( 'NONE',  ( -3.903846153844733102, -7.500000000000154543, 35.00000000000007105 ) ) ;
#11662=ORIENTED_EDGE ( 'NONE', *, *, #49111, .T. ) ;
#11663=CARTESIAN_POINT ( 'NONE',  ( 11.40777007179397984, -3.062553014421049546, 32.05460306192773601 ) ) ;
#11664=EDGE_CURVE ( 'NONE', #70063, #8324, #1633, .T. ) ;
#11665=CARTESIAN_POINT ( 'NONE',  ( 12.52679360105129547, -3.643525952247864463, 33.31231777344670064 ) ) ;
#11666=ORIENTED_EDGE ( 'NONE', *, *, #60481, .F. ) ;
#11667=ORIENTED_EDGE ( 'NONE', *, *, #52951, .T. ) ;
#11668=CARTESIAN_POINT ( 'NONE',  ( -6.673131404728781746, -8.433404298154334455, 34.66254593164985920 ) ) ;
#11669=CARTESIAN_POINT ( 'NONE',  ( 2.307692307692615685, -2.506253911140615021, 30.00000000000323297 ) ) ;
#11670=CARTESIAN_POINT ( 'NONE',  ( -0.6844038837421002608, -2.501496062324912284, 29.88072118266895671 ) ) ;
#11671=CARTESIAN_POINT ( 'NONE',  ( -13.51476335434707821, -5.070767119584671079, 34.40440758774516183 ) ) ;
#11672=CARTESIAN_POINT ( 'NONE',  ( -15.09993081275646176, -7.277220443632450575, 34.74524770363009196 ) ) ;
#11673=ORIENTED_EDGE ( 'NONE', *, *, #63094, .F. ) ;
#11674=CARTESIAN_POINT ( 'NONE',  ( -13.38461538461550759, -12.51329471203414379, 31.30864560766407578 ) ) ;
#11675=DIRECTION ( 'NONE',  ( -0.000000000000000000, 0.9848077530122086864, -0.1736481776669273891 ) ) ;
#11676=CARTESIAN_POINT ( 'NONE',  ( 11.76147438255493682, -2.889357225399416418, 32.26129605718031002 ) ) ;
#11677=FACE_OUTER_BOUND ( 'NONE', #77589, .T. ) ;
#11678=DIRECTION ( 'NONE',  ( -0.000000000000000000, 0.5000000000000011102, -0.8660254037844381525 ) ) ;
#11679=VECTOR ( 'NONE', #37824, 1000.000000000000114 ) ;
#11680=EDGE_CURVE ( 'NONE', #50951, #13993, #45724, .T. ) ;
#11682=CARTESIAN_POINT ( 'NONE',  ( -15.23076923076935252, -11.06231777344772027, 33.60647404775119895 ) ) ;
#11685=AXIS2_PLACEMENT_3D ( 'NONE', #62592, #77011, #8555 ) ;
#11686=AXIS2_PLACEMENT_3D ( 'NONE', #19099, #12779, #13665 ) ;
#11687=VERTEX_POINT ( 'NONE', #49370 ) ;
#11688=CARTESIAN_POINT ( 'NONE',  ( 5.207448778686639024, -6.852161475712352789, 34.70806712695775786 ) ) ;
#11689=CARTESIAN_POINT ( 'NONE',  ( 12.71153846153852385, -7.434744429011176159, 34.75000000000000711 ) ) ;
#11690=CYLINDRICAL_SURFACE ( 'NONE', #27240, 0.2499999999999993616 ) ;
#11691=CARTESIAN_POINT ( 'NONE',  ( -16.37677237136229991, -4.887634598454295265, 34.01352882383564946 ) ) ;
#11692=CYLINDRICAL_SURFACE ( 'NONE', #34195, 0.2499999999999997502 ) ;
#11695=CARTESIAN_POINT ( 'NONE',  ( 8.769230769230768274, -8.810774026931790459, 35.74407628777942847 ) ) ;
#11696=CARTESIAN_POINT ( 'NONE',  ( -13.38461538461538325, -8.120952969808772792, 34.71129190930000163 ) ) ;
#11697=CARTESIAN_POINT ( 'NONE',  ( -5.999999999999998224, -1.044019251281081972, 31.83374038241031911 ) ) ;
#11699=CARTESIAN_POINT ( 'NONE',  ( 9.692307692307695177, -2.721908614388771852, 31.22303859784724978 ) ) ;
#11700=CARTESIAN_POINT ( 'NONE',  ( 14.98079248672064345, -12.41104346484419452, 31.60698883733904196 ) ) ;
#11701=CARTESIAN_POINT ( 'NONE',  ( 15.23076923076923173, -2.249999999999998668, 29.75000000000001776 ) ) ;
#11704=CARTESIAN_POINT ( 'NONE',  ( -5.933932666649923249, -4.661471528628508665, 34.16647553114624003 ) ) ;
#11705=CARTESIAN_POINT ( 'NONE',  ( -17.01085574357300345, -2.833524468853757750, 32.15551576947925838 ) ) ;
#11706=ADVANCED_FACE ( 'NONE', ( #28499 ), #6017, .F. ) ;
#11707=ORIENTED_EDGE ( 'NONE', *, *, #59609, .T. ) ;
#11708=CARTESIAN_POINT ( 'NONE',  ( 8.992243613324164997, -4.762714258010881885, 34.23016756924214832 ) ) ;
#11709=CARTESIAN_POINT ( 'NONE',  ( -3.361460697436791545, -3.530157926970578508, 32.79014554554150607 ) ) ;
#11710=CARTESIAN_POINT ( 'NONE',  ( 13.38461538461538680, -6.343179335718451384, 34.87096338111211935 ) ) ;
#11712=ADVANCED_FACE ( 'NONE', ( #82574 ), #14095, .F. ) ;
#11713=CARTESIAN_POINT ( 'NONE',  ( -14.08468095607945791, -4.887748414852792322, 34.01359900205216746 ) ) ;
#11714=FACE_OUTER_BOUND ( 'NONE', #41414, .T. ) ;
#11715=EDGE_CURVE ( 'NONE', #10987, #40550, #7125, .T. ) ;
#11716=FACE_OUTER_BOUND ( 'NONE', #64439, .T. ) ;
#11717=ORIENTED_EDGE ( 'NONE', *, *, #75820, .T. ) ;
#11719=CARTESIAN_POINT ( 'NONE',  ( -3.230769230769352962, -12.70778746994576025, 30.41441678777401236 ) ) ;
#11721=CARTESIAN_POINT ( 'NONE',  ( 0.3308469948709040209, -2.729777683071817229, 31.24903638046269450 ) ) ;
#11722=ORIENTED_EDGE ( 'NONE', *, *, #27918, .T. ) ;
#11723=DIRECTION ( 'NONE',  ( -0.000000000000000000, 0.9848077530122086864, -0.1736481776669273891 ) ) ;
#11724=CARTESIAN_POINT ( 'NONE',  ( -15.29603923132555288, -3.083524468853724443, 32.58852847137143272 ) ) ;
#11725=CARTESIAN_POINT ( 'NONE',  ( 15.36156103859401867, -2.729792928343269587, 31.24908615093345077 ) ) ;
#11726=VERTEX_POINT ( 'NONE', #20846 ) ;
#11727=CARTESIAN_POINT ( 'NONE',  ( 0.2115152373170037237, -4.931416488878823223, 34.32920672191015399 ) ) ;
#11729=CARTESIAN_POINT ( 'NONE',  ( -5.999999999999998224, -2.292212530054420494, 30.41441678777542634 ) ) ;
#11730=ORIENTED_EDGE ( 'NONE', *, *, #77999, .T. ) ;
#11731=CARTESIAN_POINT ( 'NONE',  ( 13.63466969625370417, -11.79725096376909654, 32.30694842903959341 ) ) ;
#11732=CARTESIAN_POINT ( 'NONE',  ( 12.71148397988660150, -12.22109172314383052, 31.39792113162168263 ) ) ;
#11733=LINE ( 'NONE', #87404, #39837 ) ;
#11734=B_SPLINE_CURVE_WITH_KNOTS ( 'NONE', 3,
 ( #40787, #7443, #34897, #676, #62363, #53396, #74123, #12420, #20061, #47523 ),
 .UNSPECIFIED., .F., .F.,
 ( 4, 2, 2, 2, 4 ),
 ( 0.000000000000000000, 0.0001954339857564081249, 0.0003908679715128162498, 0.0005863019572692244018, 0.0007817359430256324996 ),
 .UNSPECIFIED. ) ;
#11735=LINE ( 'NONE', #39211, #36145 ) ;
#11736=CARTESIAN_POINT ( 'NONE',  ( -17.07692307692307665, -9.819645486525091727, 36.12317359536749706 ) ) ;
#11737=CARTESIAN_POINT ( 'NONE',  ( -1.318548051265308052, -10.67929555188718282, 33.92786785259544757 ) ) ;
#11738=CARTESIAN_POINT ( 'NONE',  ( 5.076923076922954969, -9.442884908241554243, 34.35708131394783038 ) ) ;
#11740=EDGE_LOOP ( 'NONE', ( #87564, #58835 ) ) ;
#11741=ORIENTED_EDGE ( 'NONE', *, *, #32681, .F. ) ;
#11742=EDGE_LOOP ( 'NONE', ( #50390, #67308, #27814, #11211 ) ) ;
#11743=CARTESIAN_POINT ( 'NONE',  ( 3.480714749117372886, -3.712312575010499938, 33.01462480002815170 ) ) ;
#11745=CARTESIAN_POINT ( 'NONE',  ( -14.08491263871423982, -10.97394488606064122, 33.68653795673694873 ) ) ;
#11746=CARTESIAN_POINT ( 'NONE',  ( -10.68146802634049486, -8.973038597847271092, 34.52809138561120506 ) ) ;
#11747=ORIENTED_EDGE ( 'NONE', *, *, #78758, .T. ) ;
#11748=CARTESIAN_POINT ( 'NONE',  ( -12.33074802057151409, -11.37503395064541678, 33.29242100308974273 ) ) ;
#11749=EDGE_CURVE ( 'NONE', #3675, #40454, #1025, .T. ) ;
#11752=VERTEX_POINT ( 'NONE', #7783 ) ;
#11753=CARTESIAN_POINT ( 'NONE',  ( -9.468932206535269458, -2.251407671071268712, 29.88021292934943318 ) ) ;
#11754=CARTESIAN_POINT ( 'NONE',  ( -2.307692307692305711, -13.87047571288749737, 32.06866353760679544 ) ) ;
#11755=CARTESIAN_POINT ( 'NONE',  ( 3.930979890783055097, -2.251424796025575770, 29.88072029997477586 ) ) ;
#11756=FACE_BOUND ( 'NONE', #19867, .T. ) ;
#11757=B_SPLINE_CURVE_WITH_KNOTS ( 'NONE', 3,
 ( #46841, #4524, #4976, #47281, #59908, #53145, #46400, #67567, #39663, #74772 ),
 .UNSPECIFIED., .F., .F.,
 ( 4, 2, 2, 2, 4 ),
 ( 0.0007817246256747499913, 0.0009771112852218944052, 0.001172497944769038819, 0.001367884604316183016, 0.001563271263863327430 ),
 .UNSPECIFIED. ) ;
#11758=CARTESIAN_POINT ( 'NONE',  ( -7.846153846153844924, -10.05456864172156806, 36.03766855953608683 ) ) ;
#11760=EDGE_CURVE ( 'NONE', #45538, #16403, #138, .T. ) ;
#11761=CARTESIAN_POINT ( 'NONE',  ( 5.749999999999988454, -2.499999999999999556, 29.81609845454692120 ) ) ;
#11762=B_SPLINE_CURVE_WITH_KNOTS ( 'NONE', 3,
 ( #76612, #42397, #69855, #63528, #29319, #56340, #15359, #84716, #48685, #1390 ),
 .UNSPECIFIED., .F., .F.,
 ( 4, 2, 2, 2, 4 ),
 ( 0.0007817359430256258859, 0.0009771253907249909023, 0.001172514838424355919, 0.001367904286123720935, 0.001563293733823085951 ),
 .UNSPECIFIED. ) ;
#11763=CARTESIAN_POINT ( 'NONE',  ( -13.38461538461538325, -5.180354513474913603, 36.12317359536750416 ) ) ;
#11764=LINE ( 'NONE', #59938, #75436 ) ;
#11765=CARTESIAN_POINT ( 'NONE',  ( 17.07692307692307665, -8.973038597847269315, 34.52809138561121927 ) ) ;
#11766=VERTEX_POINT ( 'NONE', #48315 ) ;
#11767=CARTESIAN_POINT ( 'NONE',  ( -10.39260507411620260, -4.387253974876679230, 33.66317474335728832 ) ) ;
#11769=VERTEX_POINT ( 'NONE', #81675 ) ;
#11770=ORIENTED_EDGE ( 'NONE', *, *, #12521, .F. ) ;
#11771=CARTESIAN_POINT ( 'NONE',  ( -0.6844646790546091708, -9.086856451489515152, 34.49173150075333183 ) ) ;
#11772=CARTESIAN_POINT ( 'NONE',  ( -5.076923076923075762, -3.886160181151819604, 36.00935417666054406 ) ) ;
#11773=CARTESIAN_POINT ( 'NONE',  ( 3.230769230769231726, -3.322132147404559976, 32.92929555188717927 ) ) ;
#11774=CARTESIAN_POINT ( 'NONE',  ( -11.53846153846153655, -1.129524287112498415, 32.06866353760679544 ) ) ;
#11775=CARTESIAN_POINT ( 'NONE',  ( 16.82689983963011926, -8.432397168068783699, 34.66272746175022945 ) ) ;
#11776=CARTESIAN_POINT ( 'NONE',  ( -15.36091644020745584, -3.817052484675422797, 33.13202310037935661 ) ) ;
#11779=CARTESIAN_POINT ( 'NONE',  ( -4.946131269098290595, -2.541949514083464479, 30.39797389878540557 ) ) ;
#11780=CARTESIAN_POINT ( 'NONE',  ( 10.61538461538461675, -3.050289026998446396, 32.03036669348365706 ) ) ;
#11781=ADVANCED_FACE ( 'NONE', ( #7346 ), #41127, .F. ) ;
#11782=CARTESIAN_POINT ( 'NONE',  ( 8.769230769230647482, -11.94971097300221174, 32.03036669348237098 ) ) ;
#11783=VECTOR ( 'NONE', #40299, 1000.000000000000000 ) ;
#11784=VERTEX_POINT ( 'NONE', #74918 ) ;
#11785=B_SPLINE_CURVE_WITH_KNOTS ( 'NONE', 3,
 ( #25328, #3711, #24874, #11823, #10927, #87054, #65419, #31185, #51430, #24422 ),
 .UNSPECIFIED., .F., .F.,
 ( 4, 2, 2, 2, 4 ),
 ( 0.000000000000000000, 0.0001954311564186867660, 0.0003908623128373735320, 0.0005862934692560603251, 0.0007817246256747470640 ),
 .UNSPECIFIED. ) ;
#11788=ORIENTED_EDGE ( 'NONE', *, *, #32787, .T. ) ;
#11789=EDGE_CURVE ( 'NONE', #16668, #41132, #38216, .T. ) ;
#11790=CARTESIAN_POINT ( 'NONE',  ( -1.384615384615505151, -2.892918686052166066, 31.69288490824153470 ) ) ;
#11791=CARTESIAN_POINT ( 'NONE',  ( -5.869161669513237811, -7.277220318596959281, 34.99547417642776992 ) ) ;
#11792=ORIENTED_EDGE ( 'NONE', *, *, #72403, .T. ) ;
#11793=ADVANCED_FACE ( 'NONE', ( #76231 ), #14538, .F. ) ;
#11795=CARTESIAN_POINT ( 'NONE',  ( -5.207614543590633360, -2.729777683071817229, 31.24903638046268739 ) ) ;
#11796=CARTESIAN_POINT ( 'NONE',  ( 15.93091993633000847, -8.239355502252617924, 34.69524867566427417 ) ) ;
#11797=CARTESIAN_POINT ( 'NONE',  ( 8.992243613324164997, -3.395485233115139057, 33.02377354290275946 ) ) ;
#11798=CARTESIAN_POINT ( 'NONE',  ( 18.00000000000000000, -2.538708090699994813, 30.37095296980875503 ) ) ;
#11799=ORIENTED_EDGE ( 'NONE', *, *, #62043, .F. ) ;
#11800=CARTESIAN_POINT ( 'NONE',  ( -15.16551409125639260, -2.379036618887895305, 30.90682066428158592 ) ) ;
#11802=CARTESIAN_POINT ( 'NONE',  ( -8.519285250882630223, -10.05730279482229683, 34.04704008940765902 ) ) ;
#11803=CARTESIAN_POINT ( 'NONE',  ( -2.373775718648186484, -8.973038597847271092, 34.52809138561120506 ) ) ;
#11804=CARTESIAN_POINT ( 'NONE',  ( -13.51476259405360203, -5.195881422630166391, 34.18770438780619259 ) ) ;
#11805=CARTESIAN_POINT ( 'NONE',  ( 15.36156103859401867, -12.38066358083363738, 30.83685684665853444 ) ) ;
#11806=CARTESIAN_POINT ( 'NONE',  ( -4.088591014333314178, -5.094484230520773593, 34.41647553114626845 ) ) ;
#11808=FACE_OUTER_BOUND ( 'NONE', #77762, .T. ) ;
#11809=CARTESIAN_POINT ( 'NONE',  ( 9.562160482869472844, -6.852621066184266141, 34.70813303252209181 ) ) ;
#11812=B_SPLINE_CURVE_WITH_KNOTS ( 'NONE', 3,
 ( #3150, #63195, #23857, #66186, #4496, #78368, #16669, #65737, #24763, #58986 ),
 .UNSPECIFIED., .F., .F.,
 ( 4, 2, 2, 2, 4 ),
 ( 0.000000000000000000, 0.0001954311564186870371, 0.0003908623128373740741, 0.0005862934692560610840, 0.0007817246256747481482 ),
 .UNSPECIFIED. ) ;
#11813=DIRECTION ( 'NONE',  ( -0.000000000000000000, 0.9848077530122085754, -0.1736481776669273613 ) ) ;
#11814=CARTESIAN_POINT ( 'NONE',  ( -9.561515884482908234, -8.147973898785416225, 34.70805048591653730 ) ) ;
#11816=EDGE_LOOP ( 'NONE', ( #70466, #9381 ) ) ;
#11817=EDGE_CURVE ( 'NONE', #40406, #11287, #88143, .T. ) ;
#11818=ORIENTED_EDGE ( 'NONE', *, *, #7924, .T. ) ;
#11819=CARTESIAN_POINT ( 'NONE',  ( -11.78848477575450282, -10.76384336483936011, 33.53834819971076087 ) ) ;
#11823=CARTESIAN_POINT ( 'NONE',  ( 15.93091919493929964, -10.01117774369187252, 34.36070679894347535 ) ) ;
#11824=CYLINDRICAL_SURFACE ( 'NONE', #88844, 0.2500000000000009437 ) ;
#11825=CARTESIAN_POINT ( 'NONE',  ( -6.923076923076922462, -11.69971097300155272, 32.46337939537588113 ) ) ;
#11826=ORIENTED_EDGE ( 'NONE', *, *, #63941, .T. ) ;
#11827=DIRECTION ( 'NONE',  ( -0.000000000000000000, -0.1736481776669307198, -0.9848077530122080203 ) ) ;
#11828=CARTESIAN_POINT ( 'NONE',  ( 4.153846153846154188, -13.53365097954675988, 30.81389545987213552 ) ) ;
#11829=EDGE_CURVE ( 'NONE', #28663, #47075, #66126, .T. ) ;
#11830=CARTESIAN_POINT ( 'NONE',  ( 3.930919194939304973, -8.282780595021769443, 34.94152052738834868 ) ) ;
#11831=ORIENTED_EDGE ( 'NONE', *, *, #82010, .F. ) ;
#11832=CARTESIAN_POINT ( 'NONE',  ( 12.46153846153833911, -2.657715359629662544, 31.77849191805970364 ) ) ;
#11834=ORIENTED_EDGE ( 'NONE', *, *, #49289, .T. ) ;
#11838=EDGE_CURVE ( 'NONE', #83826, #76411, #86811, .T. ) ;
#11839=CARTESIAN_POINT ( 'NONE',  ( 15.36129466900287532, -5.070358843744210198, 34.40418822224088302 ) ) ;
#11840=EDGE_LOOP ( 'NONE', ( #46590, #53298 ) ) ;
#11841=CARTESIAN_POINT ( 'NONE',  ( 0.5920641633020244932, -4.459921816937788996, 33.71989282347011851 ) ) ;
#11842=CARTESIAN_POINT ( 'NONE',  ( 15.23076923076923173, -9.819645486525091727, 36.12317359536749706 ) ) ;
#11844=B_SPLINE_CURVE_WITH_KNOTS ( 'NONE', 3,
 ( #65797, #30689, #23482, #45087, #72562, #85643, #9528, #52290, #79778, #64907 ),
 .UNSPECIFIED., .F., .F.,
 ( 4, 2, 2, 2, 4 ),
 ( 0.000000000000000000, 0.0001954311564186873623, 0.0003908623128373747246, 0.0005862934692560620598, 0.0007817246256747494492 ),
 .UNSPECIFIED. ) ;
#11846=CARTESIAN_POINT ( 'NONE',  ( -7.780898706641007578, -5.094484230520773593, 34.41647553114626845 ) ) ;
#11847=CARTESIAN_POINT ( 'NONE',  ( -5.076923076923075762, -10.67929555188718282, 33.92786785259544047 ) ) ;
#11848=B_SPLINE_CURVE_WITH_KNOTS ( 'NONE', 3,
 ( #48458, #27316, #53898, #81385, #20119, #287, #34950, #54778, #67858, #19668 ),
 .UNSPECIFIED., .F., .F.,
 ( 4, 2, 2, 2, 4 ),
 ( 0.0007817359430256302227, 0.0009771253907249963233, 0.001172514838424362424, 0.001367904286123728524, 0.001563293733823094625 ),
 .UNSPECIFIED. ) ;
#11849=ADVANCED_FACE ( 'NONE', ( #25079 ), #40820, .F. ) ;
#11851=FACE_BOUND ( 'NONE', #71276, .T. ) ;
#11852=ORIENTED_EDGE ( 'NONE', *, *, #64696, .F. ) ;
#11853=CARTESIAN_POINT ( 'NONE',  ( 8.703960323269994248, -12.46129190929999986, 30.37095296980880832 ) ) ;
#11854=EDGE_CURVE ( 'NONE', #56424, #67715, #70454, .T. ) ;
#11855=DIRECTION ( 'NONE',  ( 0.000000000000000000, 0.6427876096865373645, -0.7660444431189797898 ) ) ;
#11858=CARTESIAN_POINT ( 'NONE',  ( -3.230769230769229949, -4.098570777380720287, 33.41473453929634729 ) ) ;
#11859=CARTESIAN_POINT ( 'NONE',  ( -14.30769230769242739, -12.27809138561165270, 31.22303859784587132 ) ) ;
#11860=CARTESIAN_POINT ( 'NONE',  ( -9.442362282929648742, -6.653508905675592722, 34.93172785388651391 ) ) ;
#11861=CARTESIAN_POINT ( 'NONE',  ( 9.561616225640134914, -8.147922237126337563, 34.70805685702651999 ) ) ;
#11862=ORIENTED_EDGE ( 'NONE', *, *, #39023, .F. ) ;
#11863=EDGE_CURVE ( 'NONE', #74976, #27257, #13505, .T. ) ;
#11864=VERTEX_POINT ( 'NONE', #19652 ) ;
#11865=ORIENTED_EDGE ( 'NONE', *, *, #33322, .T. ) ;
#11866=ORIENTED_EDGE ( 'NONE', *, *, #46432, .T. ) ;
#11867=ORIENTED_EDGE ( 'NONE', *, *, #37717, .F. ) ;
#11868=CARTESIAN_POINT ( 'NONE',  ( -5.076923076923199218, -4.320704448113951379, 33.92786785259630022 ) ) ;
#11869=CARTESIAN_POINT ( 'NONE',  ( -11.66860874789975888, -9.418419913701741919, 34.36755862841477693 ) ) ;
#11870=CARTESIAN_POINT ( 'NONE',  ( -10.48485917715097138, -5.070358843744210198, 34.40418822224088302 ) ) ;
#11871=CARTESIAN_POINT ( 'NONE',  ( 4.853438152358744873, -11.60425143139329940, 33.02411095842164457 ) ) ;
#11872=CARTESIAN_POINT ( 'NONE',  ( 14.55769230769374367, -7.500000000000155431, 34.75000000000007105 ) ) ;
#11873=FACE_OUTER_BOUND ( 'NONE', #4970, .T. ) ;
#11874=CARTESIAN_POINT ( 'NONE',  ( 17.93391658904411656, -2.538708090699995257, 30.37095296980875148 ) ) ;
#11875=CARTESIAN_POINT ( 'NONE',  ( 0.3954550505825804030, -3.050289026998445951, 32.03036669348365706 ) ) ;
#11876=EDGE_LOOP ( 'NONE', ( #56262, #29776 ) ) ;
#11877=EDGE_CURVE ( 'NONE', #70675, #61992, #82271, .T. ) ;
#11878=ORIENTED_EDGE ( 'NONE', *, *, #11715, .T. ) ;
#11879=AXIS2_PLACEMENT_3D ( 'NONE', #15050, #29019, #56474 ) ;
#11881=CARTESIAN_POINT ( 'NONE',  ( -1.384615384615505151, -11.48612834414049644, 32.76840700105863391 ) ) ;
#11882=ORIENTED_EDGE ( 'NONE', *, *, #32747, .F. ) ;
#11883=CARTESIAN_POINT ( 'NONE',  ( 6.923076923076800782, -11.67786785259630911, 32.92929555188603530 ) ) ;
#11884=CARTESIAN_POINT ( 'NONE',  ( 10.61538461538461675, -8.973038597847269315, 34.52809138561121927 ) ) ;
#11885=B_SPLINE_CURVE_WITH_KNOTS ( 'NONE', 3,
 ( #1144, #62824, #41251, #1592, #29079, #49767, #14664, #83125, #68715, #76812 ),
 .UNSPECIFIED., .F., .F.,
 ( 4, 2, 2, 2, 4 ),
 ( 0.0007817359430256388964, 0.0009771253907250075990, 0.001172514838424376085, 0.001367904286123744571, 0.001563293733823113273 ),
 .UNSPECIFIED. ) ;
#11886=CARTESIAN_POINT ( 'NONE',  ( 15.90384615384615330, -7.500000000000001776, 34.75000000000000000 ) ) ;
#11887=CARTESIAN_POINT ( 'NONE',  ( 4.284637961670941131, -2.541949514083464479, 30.39797389878540557 ) ) ;
#11888=FACE_BOUND ( 'NONE', #13848, .T. ) ;
#11890=ORIENTED_EDGE ( 'NONE', *, *, #76838, .T. ) ;
#11891=CARTESIAN_POINT ( 'NONE',  ( 1.384615384615701439, -2.255955759149395501, 30.00000000000324363 ) ) ;
#11893=FACE_BOUND ( 'NONE', #29847, .T. ) ;
#11894=CARTESIAN_POINT ( 'NONE',  ( 7.846153846153725020, -11.94971097300221174, 32.03036669348237098 ) ) ;
#11895=CARTESIAN_POINT ( 'NONE',  ( -13.44988583057615905, -10.90142922261923886, 33.41473453929638993 ) ) ;
#11896=VERTEX_POINT ( 'NONE', #31848 ) ;
#11897=CARTESIAN_POINT ( 'NONE',  ( -15.23076923076922995, -12.10708131394839349, 31.69288490824020244 ) ) ;
#11899=CARTESIAN_POINT ( 'NONE',  ( 2.177001704582000929, -11.37499894934982514, 33.29245874905763003 ) ) ;
#11900=VERTEX_POINT ( 'NONE', #40383 ) ;
#11901=DIRECTION ( 'NONE',  ( 0.000000000000000000, 0.9848077530122072432, 0.1736481776669354937 ) ) ;
#11902=CARTESIAN_POINT ( 'NONE',  ( -14.37296275365308418, -6.026961402152685388, 34.52809138561120506 ) ) ;
#11903=CARTESIAN_POINT ( 'NONE',  ( -1.384615384615383471, -11.11383981884818262, 36.00935417666054406 ) ) ;
#11904=ORIENTED_EDGE ( 'NONE', *, *, #19419, .F. ) ;
#11905=B_SPLINE_CURVE_WITH_KNOTS ( 'NONE', 3,
 ( #71009, #16506, #83205, #49842, #21489, #77323, #43972, #71440, #57044, #84976 ),
 .UNSPECIFIED., .F., .F.,
 ( 4, 2, 2, 2, 4 ),
 ( 0.0007817246256747504250, 0.0009771112852218954894, 0.001172497944769040554, 0.001367884604316185401, 0.001563271263863330466 ),
 .UNSPECIFIED. ) ;
#11906=LINE ( 'NONE', #6037, #34467 ) ;
#11907=CARTESIAN_POINT ( 'NONE',  ( -17.01085472592063397, -11.69971097300155272, 32.46337939537588113 ) ) ;
#11908=AXIS2_PLACEMENT_3D ( 'NONE', #5042, #9260, #80724 ) ;
#11909=VERTEX_POINT ( 'NONE', #67843 ) ;
#11910=CARTESIAN_POINT ( 'NONE',  ( -12.46153846153846168, -5.471508081941601098, 34.59228464037088457 ) ) ;
#11911=CARTESIAN_POINT ( 'NONE',  ( -5.076923076923075762, -1.790695186598648903, 34.54067556320373455 ) ) ;
#11912=CARTESIAN_POINT ( 'NONE',  ( -14.53061926659915315, -2.523278758544489797, 31.42238647778637528 ) ) ;
#11913=CARTESIAN_POINT ( 'NONE',  ( -8.546219417617917813, -9.086983370893049639, 34.49168942202179267 ) ) ;
#11914=CARTESIAN_POINT ( 'NONE',  ( 1.384615384615386802, -8.810774026931790459, 35.74407628777942847 ) ) ;
#11915=DIRECTION ( 'NONE',  ( -0.000000000000000000, -0.9848077530122086864, -0.1736481776669273613 ) ) ;
#11916=CARTESIAN_POINT ( 'NONE',  ( 6.065255571276024327, -11.94971097300157403, 32.03036669348361443 ) ) ;
#11917=DIRECTION ( 'NONE',  ( 0.000000000000000000, -0.000000000000000000, -1.000000000000000000 ) ) ;
#11918=EDGE_CURVE ( 'NONE', #59335, #13064, #61821, .T. ) ;
#11919=LINE ( 'NONE', #45236, #782 ) ;
#11922=EDGE_LOOP ( 'NONE', ( #1924, #60635 ) ) ;
#11923=CARTESIAN_POINT ( 'NONE',  ( -7.846153846153844924, -2.249999999999998668, 29.75000000000001776 ) ) ;
#11924=VERTEX_POINT ( 'NONE', #63294 ) ;
#11925=EDGE_CURVE ( 'NONE', #57743, #76336, #37089, .T. ) ;
#11926=EDGE_LOOP ( 'NONE', ( #52166, #34725, #25260, #37870 ) ) ;
#11927=CARTESIAN_POINT ( 'NONE',  ( -7.846153846153844924, -3.886160181151819604, 36.00935417666054406 ) ) ;
#11929=ORIENTED_EDGE ( 'NONE', *, *, #88659, .F. ) ;
#11930=CARTESIAN_POINT ( 'NONE',  ( 3.361561038594018225, -9.804649428959608670, 34.18742332936588468 ) ) ;
#11932=CARTESIAN_POINT ( 'NONE',  ( 2.980746006547774218, -2.341070481393819236, 30.72580821765574299 ) ) ;
#11933=CARTESIAN_POINT ( 'NONE',  ( 11.53846153846141576, -11.06231777344772027, 33.60647404775119895 ) ) ;
#11934=CARTESIAN_POINT ( 'NONE',  ( -7.623142494540996239, -5.667800583137508674, 34.40243808032445827 ) ) ;
#11935=CARTESIAN_POINT ( 'NONE',  ( 7.846153846153846700, -2.538708090699994813, 30.37095296980875503 ) ) ;
#11936=CARTESIAN_POINT ( 'NONE',  ( -5.142193077479396024, -3.643525952247789412, 33.31231777344662959 ) ) ;
#11937=CARTESIAN_POINT ( 'NONE',  ( -7.623142494540997127, -2.758310577978208222, 31.33698337089303010 ) ) ;
#11938=CARTESIAN_POINT ( 'NONE',  ( 5.869308533332445066, -4.118384482072085184, 33.43331474514187107 ) ) ;
#11939=EDGE_CURVE ( 'NONE', #18184, #19674, #32800, .T. ) ;
#11941=CARTESIAN_POINT ( 'NONE',  ( -7.173100147298380413, -4.931416488878822335, 34.32920672191015399 ) ) ;
#11942=CARTESIAN_POINT ( 'NONE',  ( -17.93474486048716088, -2.379036618887894416, 30.90682066428159303 ) ) ;
#11943=EDGE_CURVE ( 'NONE', #86110, #40731, #68222, .T. ) ;
#11945=AXIS2_PLACEMENT_3D ( 'NONE', #69700, #82790, #60727 ) ;
#11946=VECTOR ( 'NONE', #83093, 1000.000000000000227 ) ;
#11947=ORIENTED_EDGE ( 'NONE', *, *, #75227, .F. ) ;
#11948=ORIENTED_EDGE ( 'NONE', *, *, #37842, .T. ) ;
#11949=CARTESIAN_POINT ( 'NONE',  ( -9.692307692307812417, -3.835265460704628371, 33.15142922262033665 ) ) ;
#11951=CARTESIAN_POINT ( 'NONE',  ( 12.46153846153846168, -11.35647404775217417, 33.31231777344666511 ) ) ;
#11952=CARTESIAN_POINT ( 'NONE',  ( 9.692307692307695177, -1.466349020453238561, 30.81389545987213907 ) ) ;
#11953=CARTESIAN_POINT ( 'NONE',  ( 14.05766908347085575, -3.520140089381495585, 33.17453946501458262 ) ) ;
#11954=AXIS2_PLACEMENT_3D ( 'NONE', #68443, #41868, #14839 ) ;
#11955=CARTESIAN_POINT ( 'NONE',  ( -4.826868657009622865, -2.920487667080175154, 32.31805714834170828 ) ) ;
#11956=ORIENTED_EDGE ( 'NONE', *, *, #73989, .F. ) ;
#11957=CARTESIAN_POINT ( 'NONE',  ( -6.673131404728783522, -10.05730279482229683, 34.04704008940765902 ) ) ;
#11958=ORIENTED_EDGE ( 'NONE', *, *, #44810, .T. ) ;
#11959=EDGE_CURVE ( 'NONE', #66553, #84339, #62835, .T. ) ;
#11961=CARTESIAN_POINT ( 'NONE',  ( 5.076923076922954969, -8.613356846316285953, 34.62446782046622218 ) ) ;
#11962=CARTESIAN_POINT ( 'NONE',  ( -2.557715531913763218, -9.356822207818506598, 34.66110646841856635 ) ) ;
#11963=EDGE_CURVE ( 'NONE', #5202, #83400, #55208, .T. ) ;
#11964=CARTESIAN_POINT ( 'NONE',  ( 9.942362003946010773, -12.17597550085003810, 31.52189283813460463 ) ) ;
#11965=CARTESIAN_POINT ( 'NONE',  ( 23.00000000000000000, -5.499999999999981348, 27.75000000000000000 ) ) ;
#11966=CARTESIAN_POINT ( 'NONE',  ( -13.16160403300253634, -3.105924265160262543, 32.13625925475356127 ) ) ;
#11967=EDGE_LOOP ( 'NONE', ( #82432, #5179 ) ) ;
#11969=VECTOR ( 'NONE', #61877, 1000.000000000000227 ) ;
#11971=EDGE_LOOP ( 'NONE', ( #37426, #23692 ) ) ;
#11972=ORIENTED_EDGE ( 'NONE', *, *, #40878, .T. ) ;
#11974=CARTESIAN_POINT ( 'NONE',  ( 3.230769230769110045, -12.46129190930018460, 30.37095296980731973 ) ) ;
#11975=CARTESIAN_POINT ( 'NONE',  ( 9.758375025657770152, -2.292212530054420494, 30.41441678777542990 ) ) ;
#11977=FACE_OUTER_BOUND ( 'NONE', #85062, .T. ) ;
#11978=CARTESIAN_POINT ( 'NONE',  ( -15.23076923076922995, -9.058645607665452459, 34.76329471203371924 ) ) ;
#11979=CARTESIAN_POINT ( 'NONE',  ( 3.230769230769108269, -2.657715359629662544, 31.77849191805970364 ) ) ;
#11980=ORIENTED_EDGE ( 'NONE', *, *, #43333, .T. ) ;
#11981=EDGE_CURVE ( 'NONE', #35784, #57265, #51531, .T. ) ;
#11982=VERTEX_POINT ( 'NONE', #23638 ) ;
#11983=CARTESIAN_POINT ( 'NONE',  ( 4.826946332874483936, -10.06842814019191401, 34.32929386961144758 ) ) ;
#11984=CARTESIAN_POINT ( 'NONE',  ( 2.373760658694747505, -12.37446782046654192, 30.86335684631486842 ) ) ;
#11986=FACE_OUTER_BOUND ( 'NONE', #5557, .T. ) ;
#11988=EDGE_CURVE ( 'NONE', #58055, #74098, #29461, .T. ) ;
#11989=EDGE_CURVE ( 'NONE', #34824, #77581, #2472, .T. ) ;
#11991=ORIENTED_EDGE ( 'NONE', *, *, #58006, .F. ) ;
#11992=CARTESIAN_POINT ( 'NONE',  ( -1.384615384615383471, -11.35647404775217417, 33.31231777344666511 ) ) ;
#11993=VERTEX_POINT ( 'NONE', #3367 ) ;
#11994=EDGE_CURVE ( 'NONE', #53679, #14267, #42389, .T. ) ;
#11995=CARTESIAN_POINT ( 'NONE',  ( -8.992157728137618378, -4.762599654559228846, 34.23009711892697737 ) ) ;
#11997=AXIS2_PLACEMENT_3D ( 'NONE', #45874, #66144, #5347 ) ;
#11998=CARTESIAN_POINT ( 'NONE',  ( 7.715463243043537034, -3.957541250942359756, 33.62499894934981626 ) ) ;
#12000=DIRECTION ( 'NONE',  ( 0.000000000000000000, -6.938893903907222067E-15, 1.000000000000000000 ) ) ;
#12003=ORIENTED_EDGE ( 'NONE', *, *, #58507, .F. ) ;
#12004=CARTESIAN_POINT ( 'NONE',  ( 6.923076923076802558, -8.613356846316285953, 34.62446782046622218 ) ) ;
#12005=CARTESIAN_POINT ( 'NONE',  ( 8.992010310499175318, -6.760870238392817200, 34.69528174975672385 ) ) ;
#12006=LINE ( 'NONE', #80462, #65312 ) ;
#12007=EDGE_LOOP ( 'NONE', ( #20243, #33580, #51334, #48177 ) ) ;
#12008=DIRECTION ( 'NONE',  ( -0.000000000000000000, -0.6427876096865404731, -0.7660444431189771253 ) ) ;
#12009=CARTESIAN_POINT ( 'NONE',  ( -15.23076923076922995, -5.471508081941601098, 34.59228464037088457 ) ) ;
#12010=B_SPLINE_CURVE_WITH_KNOTS ( 'NONE', 3,
 ( #29310, #50441, #57210, #56762, #84258, #22537, #36503, #63955, #2250, #29746 ),
 .UNSPECIFIED., .F., .F.,
 ( 4, 2, 2, 2, 4 ),
 ( 0.0007817359430256219828, 0.0009771253907249863487, 0.001172514838424350498, 0.001367904286123714647, 0.001563293733823079013 ),
 .UNSPECIFIED. ) ;
#12011=CARTESIAN_POINT ( 'NONE',  ( -16.40382289789474157, -12.01397095200673881, 32.43157075238190146 ) ) ;
#12012=CARTESIAN_POINT ( 'NONE',  ( 9.692307692307572609, -4.481592998941358097, 33.73612834414048933 ) ) ;
#12013=FACE_BOUND ( 'NONE', #32426, .T. ) ;
#12014=CARTESIAN_POINT ( 'NONE',  ( 13.38461538461526423, -12.51329471203414379, 31.30864560766407578 ) ) ;
#12015=CARTESIAN_POINT ( 'NONE',  ( -2.980769230769230393, -2.499999999999998668, 29.75000000000000355 ) ) ;
#12016=CARTESIAN_POINT ( 'NONE',  ( 2.241609928332172874, -9.905515769479276145, 34.41647553114623292 ) ) ;
#12017=CARTESIAN_POINT ( 'NONE',  ( 1.319345384059067428, -12.70778746994557551, 30.41441678777548319 ) ) ;
#12018=CARTESIAN_POINT ( 'NONE',  ( -2.242437168179467477, -8.656820664281605460, 34.87096338111211224 ) ) ;
#12019=CARTESIAN_POINT ( 'NONE',  ( 1.607395053593450029, -3.020022701398814124, 32.48759521482552515 ) ) ;
#12020=CARTESIAN_POINT ( 'NONE',  ( 6.066067333350078528, -4.661471528628508665, 34.16647553114624003 ) ) ;
#12022=ORIENTED_EDGE ( 'NONE', *, *, #12273, .F. ) ;
#12023=EDGE_CURVE ( 'NONE', #45139, #59816, #83208, .T. ) ;
#12024=CARTESIAN_POINT ( 'NONE',  ( -9.692307692307691624, -4.102666532097928531, 36.13435417666054406 ) ) ;
#12025=ORIENTED_EDGE ( 'NONE', *, *, #4840, .F. ) ;
#12027=CARTESIAN_POINT ( 'NONE',  ( 7.846153846153846700, -8.973038597847269315, 34.52809138561121927 ) ) ;
#12028=DIRECTION ( 'NONE',  ( -0.000000000000000000, -0.000000000000000000, -1.000000000000000000 ) ) ;
#12029=CARTESIAN_POINT ( 'NONE',  ( -4.946132635956126400, -9.084667340241226796, 34.75534355489798344 ) ) ;
#12030=ORIENTED_EDGE ( 'NONE', *, *, #65948, .F. ) ;
#12031=DIRECTION ( 'NONE',  ( -0.000000000000000000, -0.6427876096865404731, -0.7660444431189771253 ) ) ;
#12032=CARTESIAN_POINT ( 'NONE',  ( 6.249945409378045547, -3.520799739797213501, 33.17531984108286025 ) ) ;
#12034=CARTESIAN_POINT ( 'NONE',  ( 15.00728430620490350, -12.11044203135681840, 32.26167407432752299 ) ) ;
#12035=CARTESIAN_POINT ( 'NONE',  ( 8.519207545009310323, -2.588893531581426988, 31.60682220781847818 ) ) ;
#12037=LINE ( 'NONE', #66975, #47543 ) ;
#12038=CARTESIAN_POINT ( 'NONE',  ( -12.46153846153858247, -8.613356846316285953, 34.62446782046622218 ) ) ;
#12039=CARTESIAN_POINT ( 'NONE',  ( 0.2115617305961066397, -11.28823185664190376, 33.01397839955799896 ) ) ;
#12040=CYLINDRICAL_SURFACE ( 'NONE', #26728, 0.2499999999999973355 ) ;
#12041=EDGE_CURVE ( 'NONE', #67890, #28697, #74501, .T. ) ;
#12042=VECTOR ( 'NONE', #1650, 999.9999999999998863 ) ;
#12044=CARTESIAN_POINT ( 'NONE',  ( 14.05766907039934210, -5.851115903089112003, 34.47074536777953568 ) ) ;
#12045=LINE ( 'NONE', #66982, #85931 ) ;
#12046=ORIENTED_EDGE ( 'NONE', *, *, #54849, .F. ) ;
#12048=CARTESIAN_POINT ( 'NONE',  ( 6.857754007584749623, -7.749976743299137993, 34.99404534957040624 ) ) ;
#12051=CARTESIAN_POINT ( 'NONE',  ( -15.00739374499680778, -2.251407671071270489, 29.88021292934942963 ) ) ;
#12052=DIRECTION ( 'NONE',  ( -0.000000000000000000, -0.3420201433256694346, -0.9396926207859080948 ) ) ;
#12053=VERTEX_POINT ( 'NONE', #86710 ) ;
#12055=CARTESIAN_POINT ( 'NONE',  ( -12.21159305216042057, -12.68172785388650681, 30.59649109432439218 ) ) ;
#12056=CARTESIAN_POINT ( 'NONE',  ( 8.069166690247243423, -2.523321265292118198, 31.42251411153756990 ) ) ;
#12057=EDGE_LOOP ( 'NONE', ( #70026, #88451 ) ) ;
#12058=CARTESIAN_POINT ( 'NONE',  ( -9.915792616872023402, -11.60425143139329940, 33.02411095842164457 ) ) ;
#12059=CARTESIAN_POINT ( 'NONE',  ( -2.057692307692368772, -7.565270000091922853, 34.99999999999999289 ) ) ;
#12060=CARTESIAN_POINT ( 'NONE',  ( 15.29683656411930848, -5.471508081941601098, 34.59228464037088457 ) ) ;
#12062=EDGE_CURVE ( 'NONE', #64228, #6730, #37620, .T. ) ;
#12063=EDGE_LOOP ( 'NONE', ( #64275, #79826, #50427, #42765 ) ) ;
#12064=CARTESIAN_POINT ( 'NONE',  ( 6.988269911371578047, -2.255955759149235629, 29.99999999999988631 ) ) ;
#12065=CARTESIAN_POINT ( 'NONE',  ( -15.36145983387954139, -11.37499894934982692, 33.29245874905763003 ) ) ;
#12066=AXIS2_PLACEMENT_3D ( 'NONE', #71879, #59704, #4315 ) ;
#12067=CARTESIAN_POINT ( 'NONE',  ( 1.253924781505076913, -2.845849958028613624, 32.17971566917920967 ) ) ;
#12068=ORIENTED_EDGE ( 'NONE', *, *, #72018, .T. ) ;
#12069=ORIENTED_EDGE ( 'NONE', *, *, #42323, .T. ) ;
#12072=CIRCLE ( 'NONE', #79631, 0.2500000000000002220 ) ;
#12073=CARTESIAN_POINT ( 'NONE',  ( -13.38461538461538325, -12.34228464037088635, 31.77849191805839268 ) ) ;
#12074=DIRECTION ( 'NONE',  ( 0.000000000000000000, 0.9848077530122072432, 0.1736481776669354937 ) ) ;
#12075=EDGE_CURVE ( 'NONE', #83278, #66274, #52085, .T. ) ;
#12076=CARTESIAN_POINT ( 'NONE',  ( -12.52680890749923748, -3.835265460703609186, 33.15142922261924241 ) ) ;
#12077=B_SPLINE_CURVE_WITH_KNOTS ( 'NONE', 3,
 ( #61031, #61466, #87199, #67354, #88975, #46194, #54710, #39450, #47956, #6976 ),
 .UNSPECIFIED., .F., .F.,
 ( 4, 2, 2, 2, 4 ),
 ( 0.0007817246256747470640, 0.0009771112852218898515, 0.001172497944769032747, 0.001367884604316175643, 0.001563271263863318539 ),
 .UNSPECIFIED. ) ;
#12078=CARTESIAN_POINT ( 'NONE',  ( -16.82686876528476105, -4.943051570960395047, 34.04725096376909477 ) ) ;
#12079=EDGE_LOOP ( 'NONE', ( #72673, #84952 ) ) ;
#12081=ADVANCED_FACE ( 'NONE', ( #87149 ), #66860, .F. ) ;
#12082=EDGE_LOOP ( 'NONE', ( #11831, #48186 ) ) ;
#12083=DIRECTION ( 'NONE',  ( -0.000000000000000000, 0.7660444431189792347, -0.6427876096865379196 ) ) ;
#12084=VERTEX_POINT ( 'NONE', #38499 ) ;
#12085=CARTESIAN_POINT ( 'NONE',  ( -5.076923076923075762, -2.486705287966279876, 31.30864560766543647 ) ) ;
#12086=CARTESIAN_POINT ( 'NONE',  ( 15.10062202133100939, -3.285722584762969856, 32.44110544564090759 ) ) ;
#12087=CARTESIAN_POINT ( 'NONE',  ( -1.384615384615383471, -2.249999999999998668, 29.75000000000001776 ) ) ;
#12088=CARTESIAN_POINT ( 'NONE',  ( 14.30769230769231015, -13.63283147151868846, 33.57946703557072254 ) ) ;
#12092=VECTOR ( 'NONE', #49094, 1000.000000000000114 ) ;
#12094=CARTESIAN_POINT ( 'NONE',  ( -10.86540783960607293, -10.92453946501458795, 33.72985991061850086 ) ) ;
#12095=CARTESIAN_POINT ( 'NONE',  ( -13.31942239632073210, -2.255955759149234741, 29.99999999999988631 ) ) ;
#12096=ORIENTED_EDGE ( 'NONE', *, *, #13938, .T. ) ;
#12097=CARTESIAN_POINT ( 'NONE',  ( 5.076923076922954969, -4.481592998941358097, 33.73612834414048933 ) ) ;
#12098=ADVANCED_FACE ( 'NONE', ( #46145 ), #73633, .F. ) ;
#12099=EDGE_CURVE ( 'NONE', #19612, #87599, #78883, .T. ) ;
#12100=CARTESIAN_POINT ( 'NONE',  ( 12.33084699487090319, -11.18331474514187995, 33.13161551792790505 ) ) ;
#12101=CARTESIAN_POINT ( 'NONE',  ( -11.28851612908349544, -4.176053281294518804, 33.81426240980091791 ) ) ;
#12102=CARTESIAN_POINT ( 'NONE',  ( -1.608100328339332696, -8.496056993536548418, 34.65000542017679663 ) ) ;
#12103=CARTESIAN_POINT ( 'NONE',  ( -2.084680956079457470, -11.24521262558773671, 33.06293181088029343 ) ) ;
#12104=FACE_BOUND ( 'NONE', #68075, .T. ) ;
#12105=CARTESIAN_POINT ( 'NONE',  ( -15.23076923076922995, -10.67929555188718282, 33.92786785259544047 ) ) ;
#12106=CARTESIAN_POINT ( 'NONE',  ( -18.00000000000000000, -12.34228464037088635, 31.77849191805839268 ) ) ;
#12107=CARTESIAN_POINT ( 'NONE',  ( 12.46153846153846168, -5.180354513474913603, 36.12317359536750416 ) ) ;
#12108=CARTESIAN_POINT ( 'NONE',  ( 0.4615384615384611200, -1.466349020453238561, 30.81389545987213907 ) ) ;
#12109=CARTESIAN_POINT ( 'NONE',  ( 15.23076923076923173, -9.905515769479276145, 34.41647553114623292 ) ) ;
#12110=CARTESIAN_POINT ( 'NONE',  ( -16.15384615384615330, -6.435427911321262684, 35.78748833219616898 ) ) ;
#12111=CARTESIAN_POINT ( 'NONE',  ( -0.7115616988314261704, -3.711651800289232028, 33.01384336483936011 ) ) ;
#12113=CARTESIAN_POINT ( 'NONE',  ( -15.93088325028466734, -7.369474270740072441, 34.74850911626239736 ) ) ;
#12114=FACE_OUTER_BOUND ( 'NONE', #39569, .T. ) ;
#12115=EDGE_LOOP ( 'NONE', ( #40087, #31030, #65202, #7900 ) ) ;
#12116=ORIENTED_EDGE ( 'NONE', *, *, #43323, .T. ) ;
#12119=CARTESIAN_POINT ( 'NONE',  ( -11.76138849736838488, -10.01117774369187252, 34.36070679894347535 ) ) ;
#12120=EDGE_LOOP ( 'NONE', ( #67307, #45407, #22975, #20992 ) ) ;
#12122=CARTESIAN_POINT ( 'NONE',  ( -4.403869378067609475, -9.356822207818506598, 34.66110646841856635 ) ) ;
#12123=AXIS2_PLACEMENT_3D ( 'NONE', #70905, #669, #83094 ) ;
#12124=CARTESIAN_POINT ( 'NONE',  ( -14.37377468705243722, -3.937682226553330445, 33.60647404775217240 ) ) ;
#12125=CARTESIAN_POINT ( 'NONE',  ( 5.999999999999878320, -6.835583212225970762, 34.95778746994575670 ) ) ;
#12126=CARTESIAN_POINT ( 'NONE',  ( -12.52680890749923570, -5.219633306516282545, 34.19971097300152962 ) ) ;
#12127=CARTESIAN_POINT ( 'NONE',  ( 0.7115928814519140166, -4.818054556918156983, 34.26375889529406749 ) ) ;
#12128=LINE ( 'NONE', #39609, #65008 ) ;
#12130=ORIENTED_EDGE ( 'NONE', *, *, #69022, .F. ) ;
#12131=B_SPLINE_CURVE_WITH_KNOTS ( 'NONE', 3,
 ( #19778, #6271, #35058, #62088, #6699, #67968, #34171, #88702, #54440, #81934 ),
 .UNSPECIFIED., .F., .F.,
 ( 4, 2, 2, 2, 4 ),
 ( 0.000000000000000000, 0.0001954311564186869015, 0.0003908623128373738030, 0.0005862934692560607588, 0.0007817246256747476061 ),
 .UNSPECIFIED. ) ;
#12134=CYLINDRICAL_SURFACE ( 'NONE', #10419, 0.2500000000000009437 ) ;
#12135=CARTESIAN_POINT ( 'NONE',  ( -4.284537620513710010, -12.38065189839062263, 30.83690757178629482 ) ) ;
#12136=FACE_OUTER_BOUND ( 'NONE', #74962, .T. ) ;
#12137=DIRECTION ( 'NONE',  ( -0.000000000000000000, 0.8660254037844399289, -0.4999999999999980016 ) ) ;
#12138=DIRECTION ( 'NONE',  ( -0.000000000000000000, -0.3420201433256694901, -0.9396926207859082059 ) ) ;
#12140=CARTESIAN_POINT ( 'NONE',  ( -8.992157728137618378, -10.01117774369187252, 34.36070679894347535 ) ) ;
#12142=CARTESIAN_POINT ( 'NONE',  ( 16.85399685940691938, -12.15238873228291716, 31.58232369045353849 ) ) ;
#12143=CARTESIAN_POINT ( 'NONE',  ( 5.749976775778544713, -10.18141759479407327, 34.26406193332782379 ) ) ;
#12144=CARTESIAN_POINT ( 'NONE',  ( 18.06525557127602610, -10.21337939537593797, 33.94971097300152252 ) ) ;
#12145=DIRECTION ( 'NONE',  ( 0.000000000000000000, 0.000000000000000000, 1.000000000000000000 ) ) ;
#12146=CARTESIAN_POINT ( 'NONE',  ( -0.2387587925603950056, -4.226511098958374291, 33.85474049983370293 ) ) ;
#12147=FACE_OUTER_BOUND ( 'NONE', #78149, .T. ) ;
#12148=CARTESIAN_POINT ( 'NONE',  ( 13.38461538461538680, -2.292212530054420494, 30.41441678777542634 ) ) ;
#12149=CARTESIAN_POINT ( 'NONE',  ( -3.230769230769229949, -12.34228464037088635, 31.77849191805839268 ) ) ;
#12150=VERTEX_POINT ( 'NONE', #52442 ) ;
#12151=DIRECTION ( 'NONE',  ( -0.000000000000000000, 1.000000000000000000, 3.491481338843133355E-15 ) ) ;
#12152=CYLINDRICAL_SURFACE ( 'NONE', #83440, 0.2500000000000002220 ) ;
#12153=CARTESIAN_POINT ( 'NONE',  ( 0.4615384615383382183, -8.656820664282941280, 34.87096338111179961 ) ) ;
#12155=CARTESIAN_POINT ( 'NONE',  ( 13.63466969625370417, -4.943051570960394159, 34.04725096376909477 ) ) ;
#12156=CARTESIAN_POINT ( 'NONE',  ( -1.134615384613947953, -7.500000000000155431, 34.75000000000007105 ) ) ;
#12163=CARTESIAN_POINT ( 'NONE',  ( -2.242436736416281828, -2.625532179533470512, 30.86335684631491105 ) ) ;
#12164=ORIENTED_EDGE ( 'NONE', *, *, #22696, .T. ) ;
#12165=CARTESIAN_POINT ( 'NONE',  ( -18.13014720943822056, -11.93770438780619259, 32.05411857736982029 ) ) ;
#12166=CARTESIAN_POINT ( 'NONE',  ( -9.692307692307812417, -2.892918686052166066, 31.69288490824153470 ) ) ;
#12167=CARTESIAN_POINT ( 'NONE',  ( 2.177544337960611198, -12.70455904226513866, 30.44083106164009322 ) ) ;
#12169=ORIENTED_EDGE ( 'NONE', *, *, #49174, .T. ) ;
#12170=EDGE_CURVE ( 'NONE', #71930, #54393, #14460, .T. ) ;
#12171=EDGE_LOOP ( 'NONE', ( #63462, #16522, #44316, #74552 ) ) ;
#12172=CARTESIAN_POINT ( 'NONE',  ( -15.90390074446811042, -2.341251567377310217, 30.72681386836322659 ) ) ;
#12173=CARTESIAN_POINT ( 'NONE',  ( 12.39545505058258001, -12.37446782046654192, 30.86335684631486487 ) ) ;
#12174=CYLINDRICAL_SURFACE ( 'NONE', #31197, 0.2500000000000008882 ) ;
#12175=CARTESIAN_POINT ( 'NONE',  ( -17.29984929443921970, -5.667676309546437530, 34.40238873228292249 ) ) ;
#12177=DIRECTION ( 'NONE',  ( -0.000000000000000000, 0.9396926207859092051, -0.3420201433256662704 ) ) ;
#12178=CARTESIAN_POINT ( 'NONE',  ( 11.28848480751918437, -11.79746400365624659, 32.30657167506340954 ) ) ;
#12179=CARTESIAN_POINT ( 'NONE',  ( -12.71156169883143150, -6.695914987888146541, 34.68535235679833306 ) ) ;
#12181=ORIENTED_EDGE ( 'NONE', *, *, #67653, .F. ) ;
#12182=ORIENTED_EDGE ( 'NONE', *, *, #70162, .F. ) ;
#12184=EDGE_LOOP ( 'NONE', ( #16271, #35220, #29818, #51877 ) ) ;
#12185=CARTESIAN_POINT ( 'NONE',  ( 3.453782074862625784, -12.64618726649961289, 30.78989965857442712 ) ) ;
#12186=EDGE_LOOP ( 'NONE', ( #63254, #26285, #73699, #63562 ) ) ;
#12187=AXIS2_PLACEMENT_3D ( 'NONE', #19276, #67466, #5760 ) ;
#12189=CARTESIAN_POINT ( 'NONE',  ( 3.230769230769538147, -2.506253911140615021, 30.00000000000323297 ) ) ;
#12191=ORIENTED_EDGE ( 'NONE', *, *, #39771, .T. ) ;
#12192=CARTESIAN_POINT ( 'NONE',  ( -0.4615384615385840772, -12.70778746994576025, 30.41441678777401236 ) ) ;
#12193=ORIENTED_EDGE ( 'NONE', *, *, #34538, .T. ) ;
#12196=CARTESIAN_POINT ( 'NONE',  ( 9.692307692307572609, -8.613356846316285953, 34.62446782046622218 ) ) ;
#12197=ADVANCED_FACE ( 'NONE', ( #40727 ), #68192, .F. ) ;
#12198=ADVANCED_FACE ( 'NONE', ( #55551 ), #69511, .F. ) ;
#12199=CARTESIAN_POINT ( 'NONE',  ( -8.899377978668987055, -5.195881422630166391, 34.18770438780619259 ) ) ;
#12200=CARTESIAN_POINT ( 'NONE',  ( -11.47320639894870276, -12.16647553114626490, 32.15551576947920864 ) ) ;
#12201=FACE_BOUND ( 'NONE', #26513, .T. ) ;
#12202=CARTESIAN_POINT ( 'NONE',  ( -6.000000000000121680, -8.656820664282941280, 34.87096338111179961 ) ) ;
#12203=CARTESIAN_POINT ( 'NONE',  ( 16.02369818411445834, -3.625366637846545448, 33.29286588640298561 ) ) ;
#12205=ADVANCED_FACE ( 'NONE', ( #618 ), #21322, .F. ) ;
#12206=CARTESIAN_POINT ( 'NONE',  ( -3.230769230769351186, -4.481592998941358097, 33.73612834414048933 ) ) ;
#12207=DIRECTION ( 'NONE',  ( 0.000000000000000000, 0.7660444431189807890, 0.6427876096865361433 ) ) ;
#12209=VERTEX_POINT ( 'NONE', #28990 ) ;
#12210=CARTESIAN_POINT ( 'NONE',  ( 1.607990870387806526, -2.251407671071270489, 29.88021292934942252 ) ) ;
#12211=ORIENTED_EDGE ( 'NONE', *, *, #31318, .T. ) ;
#12212=ORIENTED_EDGE ( 'NONE', *, *, #50083, .F. ) ;
#12213=AXIS2_PLACEMENT_3D ( 'NONE', #40826, #74610, #4823 ) ;
#12214=CARTESIAN_POINT ( 'NONE',  ( -6.988346923633241836, -4.320704448112771878, 33.92786785259540494 ) ) ;
#12215=LINE ( 'NONE', #67159, #87994 ) ;
#12216=CARTESIAN_POINT ( 'NONE',  ( -4.403846153846151523, -7.566082377512563184, 35.00000000000000711 ) ) ;
#12217=CYLINDRICAL_SURFACE ( 'NONE', #49436, 0.2500000000000012212 ) ;
#12218=CARTESIAN_POINT ( 'NONE',  ( 9.019230769232187583, -7.500000000000154543, 35.00000000000007105 ) ) ;
#12219=CARTESIAN_POINT ( 'NONE',  ( -12.33074665371366940, -4.118422570099831148, 33.43335022499816489 ) ) ;
#12220=ORIENTED_EDGE ( 'NONE', *, *, #71941, .T. ) ;
#12221=CARTESIAN_POINT ( 'NONE',  ( -11.66860874789976243, -12.27039167877662251, 31.24851455888617835 ) ) ;
#12222=CARTESIAN_POINT ( 'NONE',  ( 14.08420736396836048, -11.41268669641499756, 32.86336882939238535 ) ) ;
#12223=DIRECTION ( 'NONE',  ( 0.000000000000000000, 1.000000000000000000, 0.000000000000000000 ) ) ;
#12224=CYLINDRICAL_SURFACE ( 'NONE', #88515, 0.2499999999999986955 ) ;
#12225=EDGE_LOOP ( 'NONE', ( #32835, #26253, #70312, #74313 ) ) ;
#12226=ORIENTED_EDGE ( 'NONE', *, *, #32924, .T. ) ;
#12227=ORIENTED_EDGE ( 'NONE', *, *, #75849, .F. ) ;
#12228=CARTESIAN_POINT ( 'NONE',  ( 10.61538461538461675, -3.937682226553329556, 33.60647404775216529 ) ) ;
#12229=DIRECTION ( 'NONE',  ( -0.000000000000000000, 0.3420201433256694901, -0.9396926207859082059 ) ) ;
#12231=DIRECTION ( 'NONE',  ( -0.000000000000000000, 1.000000000000000000, 3.491481338843133355E-15 ) ) ;
#12232=CARTESIAN_POINT ( 'NONE',  ( 14.37294744720514572, -5.941354392334607049, 34.76329471203374055 ) ) ;
#12234=CARTESIAN_POINT ( 'NONE',  ( 1.384615384615386802, -3.050289026998446396, 32.03036669348365706 ) ) ;
#12235=CARTESIAN_POINT ( 'NONE',  ( -0.7115151924808155171, -11.28823185664190376, 33.01397839955799896 ) ) ;
#12236=VERTEX_POINT ( 'NONE', #61416 ) ;
#12237=CARTESIAN_POINT ( 'NONE',  ( 0.2386122440223122920, -9.886141570436013382, 34.14413921362392301 ) ) ;
#12238=ORIENTED_EDGE ( 'NONE', *, *, #25267, .F. ) ;
#12239=CARTESIAN_POINT ( 'NONE',  ( 4.153846153846154188, -13.63283147151868846, 33.57946703557072254 ) ) ;
#12240=CARTESIAN_POINT ( 'NONE',  ( -3.099978789802278811, -2.494656445102013453, 31.33466734024120015 ) ) ;
#12241=DIRECTION ( 'NONE',  ( -0.000000000000000000, 0.6427876096865404731, -0.7660444431189771253 ) ) ;
#12242=CARTESIAN_POINT ( 'NONE',  ( 18.22301135161285046, -8.239487800360276282, 34.69522927552633718 ) ) ;
#12243=CARTESIAN_POINT ( 'NONE',  ( 13.25392478150507891, -3.957541250942358424, 33.62499894934981626 ) ) ;
#12244=VECTOR ( 'NONE', #58500, 999.9999999999998863 ) ;
#12245=CARTESIAN_POINT ( 'NONE',  ( -5.076923076923075762, -10.67929555188718282, 33.92786785259544047 ) ) ;
#12246=CARTESIAN_POINT ( 'NONE',  ( -3.480745961711583902, -6.567427716900047230, 34.66269422305636283 ) ) ;
#12248=ORIENTED_EDGE ( 'NONE', *, *, #255, .T. ) ;
#12250=CARTESIAN_POINT ( 'NONE',  ( 2.530471976670375156, -4.226511098958374291, 33.85474049983370293 ) ) ;
#12252=EDGE_LOOP ( 'NONE', ( #48815, #65931 ) ) ;
#12253=CARTESIAN_POINT ( 'NONE',  ( -5.750054481651856619, -2.587454068350147462, 30.68340429815432202 ) ) ;
#12254=CARTESIAN_POINT ( 'NONE',  ( -3.164700879766791708, -5.557115091759786019, 34.35708131394839882 ) ) ;
#12255=CARTESIAN_POINT ( 'NONE',  ( 13.38461538461526601, -3.835265460704628371, 33.15142922262033665 ) ) ;
#12257=CARTESIAN_POINT ( 'NONE',  ( -9.692307692307691624, -8.810774026931790459, 35.74407628777942847 ) ) ;
#12259=CARTESIAN_POINT ( 'NONE',  ( -7.053768389744480949, -11.71456829005830080, 32.44064028649416542 ) ) ;
#12260=ORIENTED_EDGE ( 'NONE', *, *, #16557, .F. ) ;
#12261=CARTESIAN_POINT ( 'NONE',  ( -2.307692307692305711, -6.435427911321262684, 35.78748833219616898 ) ) ;
#12262=CARTESIAN_POINT ( 'NONE',  ( -5.750000000000061284, -7.565270445406050648, 34.75000000000000000 ) ) ;
#12263=CARTESIAN_POINT ( 'NONE',  ( 17.07692307692295586, -9.442884908241554243, 34.35708131394783038 ) ) ;
#12264=EDGE_LOOP ( 'NONE', ( #72433, #35155 ) ) ;
#12266=B_SPLINE_CURVE_WITH_KNOTS ( 'NONE', 3,
 ( #14672, #34495, #62393, #1152, #27732, #7476, #28632, #83133, #69171, #26854 ),
 .UNSPECIFIED., .F., .F.,
 ( 4, 2, 2, 2, 4 ),
 ( 0.000000000000000000, 0.0001954339857564094801, 0.0003908679715128189603, 0.0005863019572692284133, 0.0007817359430256379206 ),
 .UNSPECIFIED. ) ;
#12267=EDGE_CURVE ( 'NONE', #66483, #40963, #13683, .T. ) ;
#12268=ORIENTED_EDGE ( 'NONE', *, *, #73075, .T. ) ;
#12269=DIRECTION ( 'NONE',  ( -0.000000000000000000, -0.6427876096865404731, -0.7660444431189771253 ) ) ;
#12271=CARTESIAN_POINT ( 'NONE',  ( 5.750000000000002665, -2.499999999999998668, 29.75000000000000355 ) ) ;
#12272=ORIENTED_EDGE ( 'NONE', *, *, #64648, .F. ) ;
#12273=EDGE_CURVE ( 'NONE', #57, #17236, #27199, .T. ) ;
#12274=CARTESIAN_POINT ( 'NONE',  ( -0.4615384615384611200, -1.129524287112498415, 32.06866353760679544 ) ) ;
#12275=CARTESIAN_POINT ( 'NONE',  ( -6.130690603110307890, -2.295517848115769421, 30.44137282052136939 ) ) ;
#12276=FACE_OUTER_BOUND ( 'NONE', #58063, .T. ) ;
#12278=CARTESIAN_POINT ( 'NONE',  ( 8.638620409606241779, -7.722926236386453702, 34.74524107206102030 ) ) ;
#12279=CARTESIAN_POINT ( 'NONE',  ( 3.230769230769231726, -9.819645486525091727, 36.12317359536749706 ) ) ;
#12280=ORIENTED_EDGE ( 'NONE', *, *, #69232, .T. ) ;
#12282=LINE ( 'NONE', #32111, #14145 ) ;
#12283=ORIENTED_EDGE ( 'NONE', *, *, #4064, .T. ) ;
#12285=B_SPLINE_CURVE_WITH_KNOTS ( 'NONE', 3,
 ( #4812, #72365, #46236, #87242, #85893, #4359, #65600, #52537, #52093, #3901 ),
 .UNSPECIFIED., .F., .F.,
 ( 4, 2, 2, 2, 4 ),
 ( 0.0007817359430256252354, 0.0009771253907249902518, 0.001172514838424355051, 0.001367904286123720068, 0.001563293733823085084 ),
 .UNSPECIFIED. ) ;
#12286=CARTESIAN_POINT ( 'NONE',  ( -10.36533019547115941, -10.06805714834173493, 34.32951233291982618 ) ) ;
#12287=EDGE_CURVE ( 'NONE', #40972, #67271, #21943, .T. ) ;
#12288=DIRECTION ( 'NONE',  ( 0.000000000000000000, 0.4999999999999985567, 0.8660254037844395958 ) ) ;
#12289=CARTESIAN_POINT ( 'NONE',  ( 6.249945518348142492, -9.272278438253401589, 34.42582936511637826 ) ) ;
#12290=CARTESIAN_POINT ( 'NONE',  ( -6.700297381808513641, -5.913360116392398780, 34.49180327182771322 ) ) ;
#12291=CARTESIAN_POINT ( 'NONE',  ( -9.442253272394237840, -6.523592122091592671, 34.90882529074906415 ) ) ;
#12292=CARTESIAN_POINT ( 'NONE',  ( -5.207613680033387205, -4.684245665217972032, 34.18127051446801090 ) ) ;
#12293=VERTEX_POINT ( 'NONE', #41603 ) ;
#12294=ORIENTED_EDGE ( 'NONE', *, *, #1423, .F. ) ;
#12295=VERTEX_POINT ( 'NONE', #62303 ) ;
#12296=VERTEX_POINT ( 'NONE', #1058 ) ;
#12297=B_SPLINE_CURVE_WITH_KNOTS ( 'NONE', 3,
 ( #88961, #55583, #47937, #53813, #81742, #83070, #61013, #69544, #69107, #41634 ),
 .UNSPECIFIED., .F., .F.,
 ( 4, 2, 2, 2, 4 ),
 ( 0.000000000000000000, 0.0001954311564186873623, 0.0003908623128373747246, 0.0005862934692560620598, 0.0007817246256747494492 ),
 .UNSPECIFIED. ) ;
#12299=EDGE_CURVE ( 'NONE', #80991, #58896, #74592, .T. ) ;
#12300=CARTESIAN_POINT ( 'NONE',  ( -10.39237326377176451, -11.24521262558773493, 33.06293181088029343 ) ) ;
#12301=CARTESIAN_POINT ( 'NONE',  ( 11.53846153846141576, -9.528491918059723176, 34.59228464037033035 ) ) ;
#12302=EDGE_CURVE ( 'NONE', #20877, #63575, #27375, .T. ) ;
#12303=B_SPLINE_CURVE_WITH_KNOTS ( 'NONE', 3,
 ( #12985, #31473, #58938, #86444, #24717, #52176, #79666, #17968, #73339, #13406 ),
 .UNSPECIFIED., .F., .F.,
 ( 4, 2, 2, 2, 4 ),
 ( 0.0007817246256747447872, 0.0009771112852218876831, 0.001172497944769030579, 0.001367884604316173475, 0.001563271263863316371 ),
 .UNSPECIFIED. ) ;
#12304=CARTESIAN_POINT ( 'NONE',  ( -10.61538461538473577, -5.094484230521993062, 34.41647553114689373 ) ) ;
#12305=CARTESIAN_POINT ( 'NONE',  ( 4.023154687178594813, -3.062553014421049546, 32.05460306192773601 ) ) ;
#12306=B_SPLINE_CURVE_WITH_KNOTS ( 'NONE', 3,
 ( #42932, #70401, #9150, #2361, #30727, #84816, #29855, #9571, #23524, #78467 ),
 .UNSPECIFIED., .F., .F.,
 ( 4, 2, 2, 2, 4 ),
 ( 0.000000000000000000, 0.0001954311584214072923, 0.0003908623168428145846, 0.0005862934752642218498, 0.0007817246336856291692 ),
 .UNSPECIFIED. ) ;
#12307=DIRECTION ( 'NONE',  ( 0.000000000000000000, 0.9848077530122072432, 0.1736481776669354937 ) ) ;
#12308=EDGE_CURVE ( 'NONE', #86632, #1486, #43491, .T. ) ;
#12309=DIRECTION ( 'NONE',  ( -0.000000000000000000, -0.1736481776669307198, -0.9848077530122080203 ) ) ;
#12310=ADVANCED_FACE ( 'NONE', ( #1943 ), #70408, .F. ) ;
#12311=DIRECTION ( 'NONE',  ( -0.000000000000000000, 0.7660444431189791237, -0.6427876096865379196 ) ) ;
#12314=AXIS2_PLACEMENT_3D ( 'NONE', #32564, #53277, #53726 ) ;
#12315=VERTEX_POINT ( 'NONE', #78039 ) ;
#12316=ORIENTED_EDGE ( 'NONE', *, *, #13114, .T. ) ;
#12317=CARTESIAN_POINT ( 'NONE',  ( -1.607541602131530967, -11.24512374952581872, 33.06303171183252942 ) ) ;
#12318=ORIENTED_EDGE ( 'NONE', *, *, #2317, .T. ) ;
#12319=CYLINDRICAL_SURFACE ( 'NONE', #63296, 0.2500000000000008882 ) ;
#12322=CARTESIAN_POINT ( 'NONE',  ( -15.23076923076922995, -6.386643153685126251, 34.62446782046654192 ) ) ;
#12323=FACE_BOUND ( 'NONE', #67648, .T. ) ;
#12324=ORIENTED_EDGE ( 'NONE', *, *, #71663, .F. ) ;
#12325=VERTEX_POINT ( 'NONE', #43372 ) ;
#12326=DIRECTION ( 'NONE',  ( -0.000000000000000000, 1.000000000000000000, 3.491481338843133355E-15 ) ) ;
#12327=VERTEX_POINT ( 'NONE', #64500 ) ;
#12328=FACE_BOUND ( 'NONE', #78904, .T. ) ;
#12330=CYLINDRICAL_SURFACE ( 'NONE', #77879, 0.2500000000000012212 ) ;
#12331=ORIENTED_EDGE ( 'NONE', *, *, #73572, .F. ) ;
#12333=CARTESIAN_POINT ( 'NONE',  ( 10.61538461538461675, -5.415277668671390821, 36.20867863119892149 ) ) ;
#12334=CARTESIAN_POINT ( 'NONE',  ( -7.846153846153844924, -12.37446782046654192, 30.86335684631486131 ) ) ;
#12336=EDGE_LOOP ( 'NONE', ( #26241, #74454 ) ) ;
#12337=CARTESIAN_POINT ( 'NONE',  ( 14.30769230769218581, -11.67786785259630911, 32.92929555188603530 ) ) ;
#12338=CARTESIAN_POINT ( 'NONE',  ( -3.230769230769229949, -1.044019251281081972, 31.83374038241031911 ) ) ;
#12339=CARTESIAN_POINT ( 'NONE',  ( 2.530705151785706430, -2.889357225399416862, 32.26129605718031002 ) ) ;
#12342=DIRECTION ( 'NONE',  ( -0.000000000000000000, 0.7660444431189791237, -0.6427876096865379196 ) ) ;
#12343=CARTESIAN_POINT ( 'NONE',  ( -15.90390074446811042, -10.18230066228895758, 34.26354781536631577 ) ) ;
#12344=ORIENTED_EDGE ( 'NONE', *, *, #46004, .F. ) ;
#12345=CARTESIAN_POINT ( 'NONE',  ( 8.703960768674447124, -11.67786785259540849, 32.92929555188721480 ) ) ;
#12346=CARTESIAN_POINT ( 'NONE',  ( -5.999999999999998224, -12.48256725967547354, 35.29906147534542527 ) ) ;
#12347=CARTESIAN_POINT ( 'NONE',  ( 0.5920638997721030528, -11.04252011169590020, 33.62494198852677130 ) ) ;
#12349=B_SPLINE_CURVE_WITH_KNOTS ( 'NONE', 3,
 ( #75652, #63008, #36013, #63463, #56709, #34680, #61687, #1766, #35111, #48178 ),
 .UNSPECIFIED., .F., .F.,
 ( 4, 2, 2, 2, 4 ),
 ( 0.0007817359430256319575, 0.0009771253907249987086, 0.001172514838424365460, 0.001367904286123732428, 0.001563293733823099179 ),
 .UNSPECIFIED. ) ;
#12350=LINE ( 'NONE', #11914, #14225 ) ;
#12351=B_SPLINE_CURVE_WITH_KNOTS ( 'NONE', 3,
 ( #1038, #22631, #77584, #85231, #28515, #70835, #23511, #84801, #9137, #36599 ),
 .UNSPECIFIED., .F., .F.,
 ( 4, 2, 2, 2, 4 ),
 ( 0.000000000000000000, 0.0001954339857564080707, 0.0003908679715128161414, 0.0005863019572692241849, 0.0007817359430256322827 ),
 .UNSPECIFIED. ) ;
#12352=EDGE_CURVE ( 'NONE', #37303, #72857, #36000, .T. ) ;
#12353=CARTESIAN_POINT ( 'NONE',  ( -0.4615384615381466493, -2.255955759149395501, 30.00000000000324363 ) ) ;
#12355=CARTESIAN_POINT ( 'NONE',  ( 8.769230769230768274, -2.833524468853757305, 32.15551576947925838 ) ) ;
#12356=CARTESIAN_POINT ( 'NONE',  ( 9.019176287578909879, -12.22109172314383052, 31.39792113162168263 ) ) ;
#12357=FACE_OUTER_BOUND ( 'NONE', #79621, .T. ) ;
#12358=ADVANCED_FACE ( 'NONE', ( #8711 ), #85691, .F. ) ;
#12360=ORIENTED_EDGE ( 'NONE', *, *, #1452, .F. ) ;
#12362=ORIENTED_EDGE ( 'NONE', *, *, #53585, .T. ) ;
#12363=ADVANCED_FACE ( 'NONE', ( #17224 ), #56877, .F. ) ;
#12364=EDGE_LOOP ( 'NONE', ( #36639, #57683 ) ) ;
#12365=CARTESIAN_POINT ( 'NONE',  ( -7.715628407920203990, -2.647132371071621471, 31.75357179365171589 ) ) ;
#12366=ORIENTED_EDGE ( 'NONE', *, *, #36409, .T. ) ;
#12367=CARTESIAN_POINT ( 'NONE',  ( 18.22342696186156985, -7.630147231320743018, 34.74852402298682819 ) ) ;
#12370=CARTESIAN_POINT ( 'NONE',  ( -18.24997674404858827, -12.01397095200674769, 32.43157075238189435 ) ) ;
#12371=FACE_OUTER_BOUND ( 'NONE', #48443, .T. ) ;
#12372=EDGE_CURVE ( 'NONE', #1831, #37364, #36188, .T. ) ;
#12373=FACE_OUTER_BOUND ( 'NONE', #16410, .T. ) ;
#12374=CARTESIAN_POINT ( 'NONE',  ( -13.38461538461550582, -2.625532179533778709, 30.86335684631627174 ) ) ;
#12375=CARTESIAN_POINT ( 'NONE',  ( 2.557746619330623528, -11.28795663066794219, 33.01431243580653785 ) ) ;
#12377=VECTOR ( 'NONE', #21855, 1000.000000000000227 ) ;
#12378=CARTESIAN_POINT ( 'NONE',  ( 17.20771351789003489, -2.295524264805589354, 30.44142389570982488 ) ) ;
#12379=CARTESIAN_POINT ( 'NONE',  ( -4.376773112752998962, -11.98009711892699691, 32.48740034544075428 ) ) ;
#12381=ORIENTED_EDGE ( 'NONE', *, *, #17169, .T. ) ;
#12382=EDGE_LOOP ( 'NONE', ( #64328, #29253 ) ) ;
#12383=CARTESIAN_POINT ( 'NONE',  ( 6.923076923076924238, -2.538708090699994813, 30.37095296980875503 ) ) ;
#12385=CARTESIAN_POINT ( 'NONE',  ( 16.21910129335899597, -12.51329471203373345, 31.30864560766537963 ) ) ;
#12386=CYLINDRICAL_SURFACE ( 'NONE', #8213, 0.2500000000000008882 ) ;
#12387=AXIS2_PLACEMENT_3D ( 'NONE', #80450, #51602, #18745 ) ;
#12388=ADVANCED_FACE ( 'NONE', ( #77602 ), #15910, .F. ) ;
#12390=DIRECTION ( 'NONE',  ( 0.000000000000000000, -1.000000000000000000, 0.000000000000000000 ) ) ;
#12391=VERTEX_POINT ( 'NONE', #71716 ) ;
#12392=CARTESIAN_POINT ( 'NONE',  ( -5.010854725920637520, -12.37446782046654192, 30.86335684631486842 ) ) ;
#12393=ORIENTED_EDGE ( 'NONE', *, *, #81414, .F. ) ;
#12394=VERTEX_POINT ( 'NONE', #30733 ) ;
#12395=CARTESIAN_POINT ( 'NONE',  ( 5.299934428535925335, -8.239487800360276282, 34.69522927552633718 ) ) ;
#12396=CARTESIAN_POINT ( 'NONE',  ( -14.08467946359891165, -6.460100341425560444, 34.89618726649961644 ) ) ;
#12398=CARTESIAN_POINT ( 'NONE',  ( -4.283994123577849145, -12.70455904226513866, 30.44083106164009322 ) ) ;
#12399=CARTESIAN_POINT ( 'NONE',  ( 4.153846153846154188, -2.833524468853757305, 32.15551576947925838 ) ) ;
#12402=VERTEX_POINT ( 'NONE', #70854 ) ;
#12404=ORIENTED_EDGE ( 'NONE', *, *, #32652, .F. ) ;
#12406=EDGE_CURVE ( 'NONE', #30720, #17545, #37945, .T. ) ;
#12407=CARTESIAN_POINT ( 'NONE',  ( 5.750023269057646047, -2.564618984488975961, 30.55390908950641915 ) ) ;
#12408=B_SPLINE_CURVE_WITH_KNOTS ( 'NONE', 3,
 ( #76967, #9392, #64313, #22458, #35537, #50791 ),
 .UNSPECIFIED., .F., .F.,
 ( 4, 2, 4 ),
 ( 0.0003909512603273906169, 0.0005862562993132179340, 0.0007815613382990451970 ),
 .UNSPECIFIED. ) ;
#12409=DIRECTION ( 'NONE',  ( -0.000000000000000000, -0.5000000000000009992, -0.8660254037844380415 ) ) ;
#12411=EDGE_CURVE ( 'NONE', #8100, #14985, #25131, .T. ) ;
#12412=CARTESIAN_POINT ( 'NONE',  ( -16.40386937806761125, -2.341070481393820124, 30.72580821765574299 ) ) ;
#12413=CARTESIAN_POINT ( 'NONE',  ( -15.23076923076935252, -9.528491918059723176, 34.59228464037033035 ) ) ;
#12414=EDGE_CURVE ( 'NONE', #73086, #27850, #18124, .T. ) ;
#12415=CARTESIAN_POINT ( 'NONE',  ( -10.55012904410858710, -12.27809138561124591, 31.22303859784720359 ) ) ;
#12416=ORIENTED_EDGE ( 'NONE', *, *, #22159, .F. ) ;
#12417=ORIENTED_EDGE ( 'NONE', *, *, #84563, .T. ) ;
#12418=DIRECTION ( 'NONE',  ( -0.000000000000000000, 0.7660444431189791237, -0.6427876096865379196 ) ) ;
#12419=ORIENTED_EDGE ( 'NONE', *, *, #60821, .T. ) ;
#12420=CARTESIAN_POINT ( 'NONE',  ( 10.48523740594639619, -12.45813303252208648, 30.39737893381572675 ) ) ;
#12421=CARTESIAN_POINT ( 'NONE',  ( -3.230769230769229949, -4.945431358278436385, 36.03766855953609394 ) ) ;
#12423=VERTEX_POINT ( 'NONE', #24414 ) ;
#12424=EDGE_CURVE ( 'NONE', #77096, #38831, #5046, .T. ) ;
#12425=DIRECTION ( 'NONE',  ( 0.000000000000000000, 0.9848077530122072432, -0.1736481776669354937 ) ) ;
#12426=VERTEX_POINT ( 'NONE', #31632 ) ;
#12428=CARTESIAN_POINT ( 'NONE',  ( 0.2380535369741297036, -11.60425143139329762, 33.02411095842163746 ) ) ;
#12429=FACE_BOUND ( 'NONE', #74053, .T. ) ;
#12430=CARTESIAN_POINT ( 'NONE',  ( -6.000000000000121680, -3.083524468854526912, 32.58852847137268327 ) ) ;
#12431=CARTESIAN_POINT ( 'NONE',  ( 8.769230769230768274, -4.786620604624113540, 33.94971097300155094 ) ) ;
#12432=EDGE_LOOP ( 'NONE', ( #71291, #20200 ) ) ;
#12433=EDGE_CURVE ( 'NONE', #37311, #20057, #4144, .T. ) ;
#12434=LINE ( 'NONE', #39478, #109 ) ;
#12435=VECTOR ( 'NONE', #14255, 1000.000000000000227 ) ;
#12437=CARTESIAN_POINT ( 'NONE',  ( -39.05038313613820122, -2.499999999999999556, 29.75000000000000355 ) ) ;
#12438=ORIENTED_EDGE ( 'NONE', *, *, #7213, .F. ) ;
#12439=CARTESIAN_POINT ( 'NONE',  ( -39.05038313613820122, -2.249999999999998668, 29.75000000000000355 ) ) ;
#12442=CARTESIAN_POINT ( 'NONE',  ( -2.307692307692305711, -9.058645607665452459, 34.76329471203371924 ) ) ;
#12443=CARTESIAN_POINT ( 'NONE',  ( -0.5268624743427701151, -7.749976730030849303, 34.74374725381503737 ) ) ;
#12444=EDGE_CURVE ( 'NONE', #33663, #6421, #67108, .T. ) ;
#12445=FACE_BOUND ( 'NONE', #26271, .T. ) ;
#12446=DIRECTION ( 'NONE',  ( 0.000000000000000000, 0.000000000000000000, 1.000000000000000000 ) ) ;
#12448=CARTESIAN_POINT ( 'NONE',  ( -15.16551409125639260, -5.094484230520773593, 34.41647553114626845 ) ) ;
#12449=FACE_OUTER_BOUND ( 'NONE', #70636, .T. ) ;
#12450=CARTESIAN_POINT ( 'NONE',  ( -9.442362173959551797, -10.76462480002816235, 33.53768742498949962 ) ) ;
#12451=DIRECTION ( 'NONE',  ( -0.000000000000000000, -0.3420201433256694346, -0.9396926207859080948 ) ) ;
#12453=ORIENTED_EDGE ( 'NONE', *, *, #29609, .T. ) ;
#12454=EDGE_CURVE ( 'NONE', #57330, #67890, #45544, .T. ) ;
#12455=CARTESIAN_POINT ( 'NONE',  ( -7.173100160369890510, -9.271318131107980420, 34.42618302367067429 ) ) ;
#12456=ORIENTED_EDGE ( 'NONE', *, *, #21815, .T. ) ;
#12457=CARTESIAN_POINT ( 'NONE',  ( 1.254054792873465995, -2.504760397472875155, 29.97295953869789997 ) ) ;
#12458=VECTOR ( 'NONE', #19686, 1000.000000000000000 ) ;
#12459=VERTEX_POINT ( 'NONE', #74397 ) ;
#12460=CARTESIAN_POINT ( 'NONE',  ( 7.846153846153846700, -9.905515769479276145, 34.41647553114623292 ) ) ;
#12461=CARTESIAN_POINT ( 'NONE',  ( -13.63461538461538325, -2.249999999999998668, 29.75000000000000355 ) ) ;
#12462=CARTESIAN_POINT ( 'NONE',  ( 3.230769230769231726, -2.833524468853757305, 32.15551576947925838 ) ) ;
#12464=CARTESIAN_POINT ( 'NONE',  ( -16.94613263595612551, -2.295524264805590686, 30.44142389570982488 ) ) ;
#12465=CARTESIAN_POINT ( 'NONE',  ( 1.254467414883694065, -12.15440758774515473, 32.17923288041532004 ) ) ;
#12467=CARTESIAN_POINT ( 'NONE',  ( 14.98074600654777377, -12.07920672191015221, 32.31858351112116168 ) ) ;
#12468=FACE_OUTER_BOUND ( 'NONE', #17754, .T. ) ;
#12471=CARTESIAN_POINT ( 'NONE',  ( 3.930919936330006248, -11.76352882383564769, 32.36236540154569497 ) ) ;
#12472=CARTESIAN_POINT ( 'NONE',  ( -13.38461538461538325, -6.386643153685126251, 34.62446782046654192 ) ) ;
#12473=CARTESIAN_POINT ( 'NONE',  ( 1.634669804528838810, -10.06805714834173848, 34.32951233291982618 ) ) ;
#12474=B_SPLINE_CURVE_WITH_KNOTS ( 'NONE', 3,
 ( #87589, #11021, #25867, #3808, #53325, #80828, #18225, #19113, #46578, #74061 ),
 .UNSPECIFIED., .F., .F.,
 ( 4, 2, 2, 2, 4 ),
 ( 0.0007817246256747484735, 0.0009771112852218931041, 0.001172497944769037735, 0.001367884604316182365, 0.001563271263863326996 ),
 .UNSPECIFIED. ) ;
#12476=CARTESIAN_POINT ( 'NONE',  ( 9.942307692309128697, -7.500000000000155431, 34.75000000000007105 ) ) ;
#12477=ADVANCED_FACE ( 'NONE', ( #52782 ), #87487, .F. ) ;
#12479=CARTESIAN_POINT ( 'NONE',  ( -1.318548051265307830, -11.91647553114624358, 32.58852847137148245 ) ) ;
#12480=ORIENTED_EDGE ( 'NONE', *, *, #57321, .F. ) ;
#12481=CARTESIAN_POINT ( 'NONE',  ( 7.173076923078343548, -7.500000000000154543, 35.00000000000007105 ) ) ;
#12482=CARTESIAN_POINT ( 'NONE',  ( 15.23076923076923173, -10.67929555188718282, 33.92786785259544047 ) ) ;
#12484=CARTESIAN_POINT ( 'NONE',  ( -15.23076923076922995, -6.189225973068211317, 35.74407628777942847 ) ) ;
#12485=CARTESIAN_POINT ( 'NONE',  ( 14.30769230769231015, -12.10708131394839349, 31.69288490824020244 ) ) ;
#12486=ORIENTED_EDGE ( 'NONE', *, *, #25503, .T. ) ;
#12487=CARTESIAN_POINT ( 'NONE',  ( -11.53846153846153655, -13.75783147151868846, 33.36296068462461051 ) ) ;
#12489=CARTESIAN_POINT ( 'NONE',  ( 9.019285189144223835, -2.544122305571458575, 31.48381861865057729 ) ) ;
#12491=CARTESIAN_POINT ( 'NONE',  ( 11.76124107972994359, -5.114059244376869984, 34.14424750095245287 ) ) ;
#12492=CARTESIAN_POINT ( 'NONE',  ( 8.769230769230768274, -4.102666532097928531, 36.13435417666054406 ) ) ;
#12493=EDGE_CURVE ( 'NONE', #30065, #87319, #60432, .T. ) ;
#12494=CARTESIAN_POINT ( 'NONE',  ( -17.29975117455795441, -7.369209533119136069, 34.99857337881830688 ) ) ;
#12495=CYLINDRICAL_SURFACE ( 'NONE', #88903, 0.2499999999999986955 ) ;
#12496=ADVANCED_FACE ( 'NONE', ( #31174 ), #59541, .F. ) ;
#12497=ORIENTED_EDGE ( 'NONE', *, *, #72458, .T. ) ;
#12498=CARTESIAN_POINT ( 'NONE',  ( -9.692307692307814193, -2.657715359629662544, 31.77849191805970364 ) ) ;
#12501=ORIENTED_EDGE ( 'NONE', *, *, #72612, .F. ) ;
#12502=VERTEX_POINT ( 'NONE', #87045 ) ;
#12503=ORIENTED_EDGE ( 'NONE', *, *, #3736, .F. ) ;
#12505=CARTESIAN_POINT ( 'NONE',  ( 14.08420736396836226, -4.386631170607603991, 33.66268669641500111 ) ) ;
#12506=VECTOR ( 'NONE', #11161, 1000.000000000000227 ) ;
#12507=CARTESIAN_POINT ( 'NONE',  ( -8.096130590202436750, -12.65889640711025521, 30.72598325615533454 ) ) ;
#12508=CYLINDRICAL_SURFACE ( 'NONE', #79760, 0.2499999999999986955 ) ;
#12509=CARTESIAN_POINT ( 'NONE',  ( 16.02369894440793630, -5.195881422630167279, 34.18770438780618548 ) ) ;
#12510=ORIENTED_EDGE ( 'NONE', *, *, #23861, .T. ) ;
#12511=B_SPLINE_CURVE_WITH_KNOTS ( 'NONE', 3,
 ( #40363, #20520, #47985, #692, #48425, #75910, #28160, #55628, #54296, #81792 ),
 .UNSPECIFIED., .F., .F.,
 ( 4, 2, 2, 2, 4 ),
 ( 0.000000000000000000, 0.0001954311564186867931, 0.0003908623128373735862, 0.0005862934692560603251, 0.0007817246256747471724 ),
 .UNSPECIFIED. ) ;
#12512=EDGE_LOOP ( 'NONE', ( #31176, #12169, #57461, #52733 ) ) ;
#12513=ORIENTED_EDGE ( 'NONE', *, *, #5663, .T. ) ;
#12514=CARTESIAN_POINT ( 'NONE',  ( -7.912237257109724808, -4.786620604624113540, 33.94971097300155805 ) ) ;
#12515=ORIENTED_EDGE ( 'NONE', *, *, #81933, .T. ) ;
#12517=CARTESIAN_POINT ( 'NONE',  ( -3.230769230769352962, -5.094484230521993062, 34.41647553114689373 ) ) ;
#12518=EDGE_CURVE ( 'NONE', #62711, #69942, #87538, .T. ) ;
#12519=DIRECTION ( 'NONE',  ( -0.000000000000000000, -0.9396926207859094271, -0.3420201433256663814 ) ) ;
#12521=EDGE_CURVE ( 'NONE', #64358, #50015, #82050, .T. ) ;
#12522=ORIENTED_EDGE ( 'NONE', *, *, #8008, .F. ) ;
#12523=VERTEX_POINT ( 'NONE', #14468 ) ;
#12524=AXIS2_PLACEMENT_3D ( 'NONE', #34826, #41590, #7368 ) ;
#12525=VERTEX_POINT ( 'NONE', #41058 ) ;
#12526=CARTESIAN_POINT ( 'NONE',  ( -4.826923076923139710, -7.565270445406050648, 34.75000000000000000 ) ) ;
#12527=CARTESIAN_POINT ( 'NONE',  ( -15.23076923076922995, -13.04860791097971706, 34.73218667398347037 ) ) ;
#12530=CARTESIAN_POINT ( 'NONE',  ( 2.177544337960608534, -2.647304123082328875, 31.75400227202885262 ) ) ;
#12532=ORIENTED_EDGE ( 'NONE', *, *, #80413, .F. ) ;
#12533=CARTESIAN_POINT ( 'NONE',  ( 16.40390046548447245, -8.303483539816726378, 34.68545999027711702 ) ) ;
#12534=CARTESIAN_POINT ( 'NONE',  ( 8.899756470994333313, -12.45806712695776319, 30.39783852428763922 ) ) ;
#12536=FACE_OUTER_BOUND ( 'NONE', #16400, .T. ) ;
#12537=FACE_BOUND ( 'NONE', #63563, .T. ) ;
#12538=FACE_OUTER_BOUND ( 'NONE', #86129, .T. ) ;
#12539=CARTESIAN_POINT ( 'NONE',  ( -12.52680890749923570, -9.442884908240170461, 34.35708131394840592 ) ) ;
#12540=CARTESIAN_POINT ( 'NONE',  ( -7.911424292114618950, -12.27809138561121394, 31.22303859784730307 ) ) ;
#12541=CARTESIAN_POINT ( 'NONE',  ( 8.769230769230768274, -12.78798330534102767, 29.49999999999997868 ) ) ;
#12542=CARTESIAN_POINT ( 'NONE',  ( 15.45354889974729673, -10.23759521482555357, 34.22997729860117033 ) ) ;
#12543=B_SPLINE_CURVE_WITH_KNOTS ( 'NONE', 3,
 ( #263, #77685, #56536, #69603, #42585, #70045, #48887, #21419, #63728, #22739 ),
 .UNSPECIFIED., .F., .F.,
 ( 4, 2, 2, 2, 4 ),
 ( 0.0007817359430256374869, 0.0009771253907250054306, 0.001172514838424373266, 0.001367904286123741101, 0.001563293733823109153 ),
 .UNSPECIFIED. ) ;
#12544=EDGE_CURVE ( 'NONE', #49278, #57134, #15582, .T. ) ;
#12546=DIRECTION ( 'NONE',  ( -0.000000000000000000, 0.5000000000000011102, -0.8660254037844381525 ) ) ;
#12547=VERTEX_POINT ( 'NONE', #34291 ) ;
#12548=CARTESIAN_POINT ( 'NONE',  ( -16.28432286196261458, -7.276988635370451597, 34.74523720219453793 ) ) ;
#12549=CARTESIAN_POINT ( 'NONE',  ( -7.780898274877818821, -2.625532179533470512, 30.86335684631491105 ) ) ;
#12550=ORIENTED_EDGE ( 'NONE', *, *, #33141, .T. ) ;
#12552=CARTESIAN_POINT ( 'NONE',  ( -6.792551221313360088, -5.195472089885680766, 34.18748526763464923 ) ) ;
#12553=EDGE_CURVE ( 'NONE', #79092, #78459, #4734, .T. ) ;
#12554=CARTESIAN_POINT ( 'NONE',  ( 16.15384615384603251, -3.835265460704628815, 33.15142922262033665 ) ) ;
#12555=LINE ( 'NONE', #72467, #26017 ) ;
#12556=EDGE_LOOP ( 'NONE', ( #28243, #59158 ) ) ;
#12558=CARTESIAN_POINT ( 'NONE',  ( -4.219116154402471786, -9.528491918058357157, 34.59228464037090589 ) ) ;
#12559=FACE_BOUND ( 'NONE', #68328, .T. ) ;
#12560=CARTESIAN_POINT ( 'NONE',  ( -18.06608341095587988, -3.050289026998447284, 32.03036669348365706 ) ) ;
#12562=CARTESIAN_POINT ( 'NONE',  ( 7.911409417429871027, -9.442884908240271713, 34.35708131394835618 ) ) ;
#12563=CYLINDRICAL_SURFACE ( 'NONE', #25229, 0.2499999999999973355 ) ;
#12565=CARTESIAN_POINT ( 'NONE',  ( 0.4615384615384611200, -5.557115091759785130, 34.35708131394839171 ) ) ;
#12568=ADVANCED_FACE ( 'NONE', ( #516 ), #81604, .F. ) ;
#12569=EDGE_LOOP ( 'NONE', ( #43117, #77644 ) ) ;
#12571=EDGE_CURVE ( 'NONE', #14333, #24897, #76843, .T. ) ;
#12572=AXIS2_PLACEMENT_3D ( 'NONE', #5276, #39961, #66535 ) ;
#12573=DIRECTION ( 'NONE',  ( -0.000000000000000000, 0.9848077530122086864, -0.1736481776669273891 ) ) ;
#12574=CARTESIAN_POINT ( 'NONE',  ( -17.75000000000000355, -7.500000000000000000, 35.00000000000000000 ) ) ;
#12575=DIRECTION ( 'NONE',  ( 0.000000000000000000, 0.4999999999999985567, 0.8660254037844395958 ) ) ;
#12576=DIRECTION ( 'NONE',  ( 0.000000000000000000, 0.3420201433256641055, -0.9396926207859100932 ) ) ;
#12578=CARTESIAN_POINT ( 'NONE',  ( 0.6849654234000311925, -7.630147231320743018, 34.74852402298682819 ) ) ;
#12579=CARTESIAN_POINT ( 'NONE',  ( -6.222926958906846551, -8.282780595021769443, 34.94152052738834868 ) ) ;
#12580=CARTESIAN_POINT ( 'NONE',  ( 14.30769230769231015, -13.75783147151868846, 33.36296068462461051 ) ) ;
#12581=DIRECTION ( 'NONE',  ( 0.000000000000000000, 0.3420201433256641055, -0.9396926207859100932 ) ) ;
#12582=CARTESIAN_POINT ( 'NONE',  ( 9.942253210655838558, -2.824170634883621744, 31.52227843825338738 ) ) ;
#12583=DIRECTION ( 'NONE',  ( 0.000000000000000000, 0.000000000000000000, 1.000000000000000000 ) ) ;
#12584=CARTESIAN_POINT ( 'NONE',  ( 7.146089767170320073, -3.395485233115139057, 33.02377354290275946 ) ) ;
#12587=EDGE_CURVE ( 'NONE', #17248, #58442, #84334, .T. ) ;
#12588=CARTESIAN_POINT ( 'NONE',  ( -15.45425417449318317, -8.496056993536548418, 34.65000542017679663 ) ) ;
#12589=B_SPLINE_CURVE_WITH_KNOTS ( 'NONE', 3,
 ( #30311, #2380, #9588, #64518, #70422, #29875, #37055, #43819, #29441, #28550 ),
 .UNSPECIFIED., .F., .F.,
 ( 4, 2, 2, 2, 4 ),
 ( 0.000000000000000000, 0.0001954311584214072923, 0.0003908623168428145846, 0.0005862934752642218498, 0.0007817246336856291692 ),
 .UNSPECIFIED. ) ;
#12590=EDGE_LOOP ( 'NONE', ( #12238, #38535, #82048, #8883 ) ) ;
#12591=CARTESIAN_POINT ( 'NONE',  ( -5.076923076923197442, -11.94971097300221174, 32.03036669348237098 ) ) ;
#12592=DIRECTION ( 'NONE',  ( -1.000000000000000000, 0.000000000000000000, 0.000000000000000000 ) ) ;
#12594=CARTESIAN_POINT ( 'NONE',  ( -18.06525099016123548, -2.506253911140459145, 30.00000000000011369 ) ) ;
#12596=DIRECTION ( 'NONE',  ( 0.000000000000000000, 0.3420201433256610524, 0.9396926207859113145 ) ) ;
#12597=CARTESIAN_POINT ( 'NONE',  ( 10.54930120442873687, -5.557115091759785130, 34.35708131394839171 ) ) ;
#12598=CARTESIAN_POINT ( 'NONE',  ( 5.207448515156721136, -4.299079248970732792, 33.91157788607253565 ) ) ;
#12599=ORIENTED_EDGE ( 'NONE', *, *, #64216, .T. ) ;
#12601=CARTESIAN_POINT ( 'NONE',  ( 17.77707378248384629, -3.586966769969702540, 32.86292498521069660 ) ) ;
#12602=EDGE_CURVE ( 'NONE', #81210, #80449, #73320, .T. ) ;
#12603=EDGE_LOOP ( 'NONE', ( #58369, #9978, #54127, #1739 ) ) ;
#12604=CARTESIAN_POINT ( 'NONE',  ( 8.545745825506822158, -8.496056993536548418, 34.65000542017679663 ) ) ;
#12605=CARTESIAN_POINT ( 'NONE',  ( 0.2380535178145145869, -2.847400154188068022, 31.58180166144859058 ) ) ;
#12606=EDGE_LOOP ( 'NONE', ( #18866, #81302, #1313, #69869 ) ) ;
#12607=DIRECTION ( 'NONE',  ( -0.000000000000000000, 0.9396926207859092051, -0.3420201433256662704 ) ) ;
#12608=ADVANCED_FACE ( 'NONE', ( #3152 ), #16671, .F. ) ;
#12609=ADVANCED_FACE ( 'NONE', ( #84717 ), #22988, .F. ) ;
#12610=CARTESIAN_POINT ( 'NONE',  ( 2.372947447205147942, -8.656820664281605460, 34.87096338111211224 ) ) ;
#12611=AXIS2_PLACEMENT_3D ( 'NONE', #81066, #82389, #48139 ) ;
#12612=CARTESIAN_POINT ( 'NONE',  ( 14.30769230769231015, -2.517432740324522911, 35.29906147534542527 ) ) ;
#12613=ORIENTED_EDGE ( 'NONE', *, *, #30019, .F. ) ;
#12615=ADVANCED_FACE ( 'NONE', ( #85145 ), #83828, .F. ) ;
#12616=ORIENTED_EDGE ( 'NONE', *, *, #1070, .F. ) ;
#12617=FACE_OUTER_BOUND ( 'NONE', #63975, .T. ) ;
#12618=CARTESIAN_POINT ( 'NONE',  ( 12.23805351781451201, -12.44517049084099725, 30.48991314939691932 ) ) ;
#12619=FACE_OUTER_BOUND ( 'NONE', #55973, .T. ) ;
#12621=CARTESIAN_POINT ( 'NONE',  ( -10.68065461594093435, -12.16647553114622049, 32.15551576947930812 ) ) ;
#12622=LINE ( 'NONE', #40546, #65089 ) ;
#12623=CARTESIAN_POINT ( 'NONE',  ( -1.384615384615506484, -11.06231777344772027, 33.60647404775119895 ) ) ;
#12624=B_SPLINE_CURVE_WITH_KNOTS ( 'NONE', 3,
 ( #82358, #7133, #62068, #42696, #70155, #62937, #28739, #27403, #381, #42257 ),
 .UNSPECIFIED., .F., .F.,
 ( 4, 2, 2, 2, 4 ),
 ( 0.0007817246256747515092, 0.0009771112852218961399, 0.001172497944769040554, 0.001367884604316184968, 0.001563271263863329598 ),
 .UNSPECIFIED. ) ;
#12625=CARTESIAN_POINT ( 'NONE',  ( -0.2114840416250085564, -12.41089969410671223, 31.60739465890703670 ) ) ;
#12626=AXIS2_PLACEMENT_3D ( 'NONE', #73149, #11447, #17767 ) ;
#12627=ORIENTED_EDGE ( 'NONE', *, *, #7427, .F. ) ;
#12628=ORIENTED_EDGE ( 'NONE', *, *, #42372, .F. ) ;
#12629=ORIENTED_EDGE ( 'NONE', *, *, #63136, .T. ) ;
#12631=ORIENTED_EDGE ( 'NONE', *, *, #28904, .F. ) ;
#12633=CARTESIAN_POINT ( 'NONE',  ( 14.05769230769230838, -2.499999999999998668, 29.75000000000000355 ) ) ;
#12634=CARTESIAN_POINT ( 'NONE',  ( 9.627037246346917598, -5.219633306516282545, 34.19971097300152962 ) ) ;
#12635=ORIENTED_EDGE ( 'NONE', *, *, #71311, .T. ) ;
#12636=CARTESIAN_POINT ( 'NONE',  ( -12.21148404162501144, -11.47946981652013498, 33.17500667209847620 ) ) ;
#12638=CARTESIAN_POINT ( 'NONE',  ( -9.692307692307691624, -3.937682226553329556, 33.60647404775216529 ) ) ;
#12640=CARTESIAN_POINT ( 'NONE',  ( -12.59214811674254442, -7.722926974430166069, 34.99546784045485737 ) ) ;
#12641=B_SPLINE_CURVE_WITH_KNOTS ( 'NONE', 3,
 ( #40487, #26964, #81916, #5360, #67951, #6254 ),
 .UNSPECIFIED., .F., .F.,
 ( 4, 2, 4 ),
 ( 0.0003909512603273650297, 0.0005862562993131907206, 0.0007815613382990164656 ),
 .UNSPECIFIED. ) ;
#12642=B_SPLINE_CURVE_WITH_KNOTS ( 'NONE', 3,
 ( #71206, #44166, #36118, #9510, #71651, #29360, #64891, #22588, #57705, #3196 ),
 .UNSPECIFIED., .F., .F.,
 ( 4, 2, 2, 2, 4 ),
 ( 0.0007817359430256216575, 0.0009771253907249856981, 0.001172514838424349630, 0.001367904286123713779, 0.001563293733823077711 ),
 .UNSPECIFIED. ) ;
#12643=CARTESIAN_POINT ( 'NONE',  ( -8.769230769230890843, -5.219633306517616589, 34.19971097300220464 ) ) ;
#12644=CARTESIAN_POINT ( 'NONE',  ( 10.68064018666064108, -5.219633306516380244, 34.19971097300157936 ) ) ;
#12645=FACE_BOUND ( 'NONE', #42008, .T. ) ;
#12647=CARTESIAN_POINT ( 'NONE',  ( 18.00000000000000000, -2.249999999999998668, 29.75000000000001776 ) ) ;
#12649=CARTESIAN_POINT ( 'NONE',  ( 4.153846153846154188, -8.120952969808772792, 34.71129190930000163 ) ) ;
#12652=DIRECTION ( 'NONE',  ( -0.000000000000000000, -0.9396926207859093161, -0.3420201433256663259 ) ) ;
#12653=DIRECTION ( 'NONE',  ( -0.000000000000000000, -0.6427876096865404731, -0.7660444431189770143 ) ) ;
#12654=ORIENTED_EDGE ( 'NONE', *, *, #30958, .T. ) ;
#12655=EDGE_LOOP ( 'NONE', ( #66353, #3218 ) ) ;
#12656=CARTESIAN_POINT ( 'NONE',  ( 2.177001704581999597, -2.845849958028613624, 32.17971566917920967 ) ) ;
#12657=DIRECTION ( 'NONE',  ( -0.000000000000000000, -0.5000000000000009992, -0.8660254037844380415 ) ) ;
#12658=EDGE_CURVE ( 'NONE', #45245, #720, #2483, .T. ) ;
#12659=CARTESIAN_POINT ( 'NONE',  ( 15.48082365068268018, -8.346898887586323923, 34.93166121998716278 ) ) ;
#12660=LINE ( 'NONE', #5904, #574 ) ;
#12661=DIRECTION ( 'NONE',  ( -0.000000000000000000, 0.1736481776669307198, -0.9848077530122080203 ) ) ;
#12662=CARTESIAN_POINT ( 'NONE',  ( -1.384615384615383471, -10.89733346790207413, 36.13435417666054406 ) ) ;
#12663=ORIENTED_EDGE ( 'NONE', *, *, #71119, .F. ) ;
#12664=CARTESIAN_POINT ( 'NONE',  ( -5.749945580086545327, -8.346898887586323923, 34.93166121998716278 ) ) ;
#12665=VECTOR ( 'NONE', #12269, 1000.000000000000227 ) ;
#12666=CARTESIAN_POINT ( 'NONE',  ( 15.00728430620490172, -4.225889041578353655, 33.85425143139329407 ) ) ;
#12667=DIRECTION ( 'NONE',  ( -0.000000000000000000, 1.000000000000000000, -0.000000000000000000 ) ) ;
#12668=DIRECTION ( 'NONE',  ( 0.000000000000000000, 0.000000000000000000, 1.000000000000000000 ) ) ;
#12669=ORIENTED_EDGE ( 'NONE', *, *, #47027, .F. ) ;
#12672=VERTEX_POINT ( 'NONE', #69856 ) ;
#12673=CARTESIAN_POINT ( 'NONE',  ( 0.7115384615398965273, -7.500000000000155431, 34.75000000000007105 ) ) ;
#12674=EDGE_CURVE ( 'NONE', #58928, #56507, #64674, .T. ) ;
#12677=CARTESIAN_POINT ( 'NONE',  ( -6.249976744048591826, -9.234221910056348293, 34.70572697212741531 ) ) ;
#12678=CARTESIAN_POINT ( 'NONE',  ( 5.011652630962299959, -6.879047030191174805, 34.71129190930000163 ) ) ;
#12679=CARTESIAN_POINT ( 'NONE',  ( -2.437839517130528044, -8.587444163452046197, 34.63053765926554206 ) ) ;
#12680=B_SPLINE_CURVE_WITH_KNOTS ( 'NONE', 3,
 ( #28704, #13409, #35008, #55719, #19728, #40459, #83207, #67918, #6224, #21491 ),
 .UNSPECIFIED., .F., .F.,
 ( 4, 2, 2, 2, 4 ),
 ( 0.000000000000000000, 0.0001954339857564097241, 0.0003908679715128194482, 0.0005863019572692291723, 0.0007817359430256388964 ),
 .UNSPECIFIED. ) ;
#12681=CARTESIAN_POINT ( 'NONE',  ( -11.28851602011339672, -9.272278438253398036, 34.42582936511637115 ) ) ;
#12682=ORIENTED_EDGE ( 'NONE', *, *, #70891, .T. ) ;
#12683=CARTESIAN_POINT ( 'NONE',  ( -15.36145983387953606, -11.93127051446799847, 32.56575433478202797 ) ) ;
#12685=DIRECTION ( 'NONE',  ( -0.000000000000000000, 0.3420201433256694901, -0.9396926207859082059 ) ) ;
#12687=LINE ( 'NONE', #19001, #78925 ) ;
#12688=CARTESIAN_POINT ( 'NONE',  ( 11.76124120743960333, -10.23759521482555357, 34.22997729860117033 ) ) ;
#12689=CARTESIAN_POINT ( 'NONE',  ( -5.776624514227577833, -2.251407671071270489, 29.88021292934942252 ) ) ;
#12690=EDGE_CURVE ( 'NONE', #43255, #48795, #30628, .T. ) ;
#12691=DIRECTION ( 'NONE',  ( -0.000000000000000000, 0.3420201433256694346, -0.9396926207859080948 ) ) ;
#12692=CARTESIAN_POINT ( 'NONE',  ( -3.453695448285377445, -6.503392248772476236, 34.64988816332204635 ) ) ;
#12695=AXIS2_PLACEMENT_3D ( 'NONE', #28051, #73701, #66931 ) ;
#12696=CARTESIAN_POINT ( 'NONE',  ( 11.60371710973756620, -2.892918686051625166, 31.69288490824026638 ) ) ;
#12697=DIRECTION ( 'NONE',  ( 0.000000000000000000, 0.4999999999999985567, 0.8660254037844395958 ) ) ;
#12698=ORIENTED_EDGE ( 'NONE', *, *, #63673, .T. ) ;
#12700=EDGE_LOOP ( 'NONE', ( #88862, #16958 ) ) ;
#12701=CARTESIAN_POINT ( 'NONE',  ( -4.153846153846152411, -4.786620604624113540, 33.94971097300155094 ) ) ;
#12702=CARTESIAN_POINT ( 'NONE',  ( 11.53846153846153832, -12.62096338111211580, 30.90682066428153263 ) ) ;
#12703=CARTESIAN_POINT ( 'NONE',  ( -10.83831157429146330, -2.308479472611653094, 30.53278059502174457 ) ) ;
#12705=CARTESIAN_POINT ( 'NONE',  ( 0.6843181305165273454, -2.353885683473779800, 30.79025554430704759 ) ) ;
#12707=CYLINDRICAL_SURFACE ( 'NONE', #13192, 0.2500000000000002220 ) ;
#12708=EDGE_CURVE ( 'NONE', #10084, #63192, #37900, .T. ) ;
#12709=EDGE_CURVE ( 'NONE', #59816, #45139, #74437, .T. ) ;
#12710=CARTESIAN_POINT ( 'NONE',  ( -14.30769230769242739, -2.892918686052166066, 31.69288490824153470 ) ) ;
#12711=CARTESIAN_POINT ( 'NONE',  ( -3.480792468062194889, -11.86270091957321249, 32.19358267280087915 ) ) ;
#12713=DIRECTION ( 'NONE',  ( -0.000000000000000000, 0.9848077530122086864, -0.1736481776669273891 ) ) ;
#12715=B_SPLINE_CURVE_WITH_KNOTS ( 'NONE', 3,
 ( #37556, #71342, #84880, #16406, #43875, #78994, #18191, #85319, #79890, #3329 ),
 .UNSPECIFIED., .F., .F.,
 ( 4, 2, 2, 2, 4 ),
 ( 0.0007817359527651101701, 0.0009771254036996489256, 0.001172514854634187790, 0.001367904305568726653, 0.001563293756503265517 ),
 .UNSPECIFIED. ) ;
#12716=CYLINDRICAL_SURFACE ( 'NONE', #18458, 0.2499999999999995559 ) ;
#12717=CARTESIAN_POINT ( 'NONE',  ( 11.31497661389720477, -2.612411019501189369, 31.66733052389439962 ) ) ;
#12718=ORIENTED_EDGE ( 'NONE', *, *, #62653, .F. ) ;
#12719=B_SPLINE_CURVE_WITH_KNOTS ( 'NONE', 3,
 ( #87744, #73775, #81861, #47615, #5744, #88192, #67892, #31892, #59797, #47164 ),
 .UNSPECIFIED., .F., .F.,
 ( 4, 2, 2, 2, 4 ),
 ( 0.0007817359430256326080, 0.0009771253907250047801, 0.001172514838424369796, 0.001367904286123735030, 0.001563293733823100046 ),
 .UNSPECIFIED. ) ;
#12720=DIRECTION ( 'NONE',  ( -0.000000000000000000, -0.9396926207859093161, -0.3420201433256663259 ) ) ;
#12721=CARTESIAN_POINT ( 'NONE',  ( -5.999999999999998224, -2.292212530054420494, 30.41441678777542634 ) ) ;
#12722=CARTESIAN_POINT ( 'NONE',  ( -9.915792636031637741, -2.599994579823203367, 30.74605699353653776 ) ) ;
#12723=VECTOR ( 'NONE', #47839, 1000.000000000000227 ) ;
#12724=VECTOR ( 'NONE', #79923, 999.9999999999998863 ) ;
#12725=CARTESIAN_POINT ( 'NONE',  ( -4.153846153846152411, -13.63283147151868846, 33.57946703557072254 ) ) ;
#12726=CARTESIAN_POINT ( 'NONE',  ( -1.515305987725690917, -10.70098750199973203, 33.91152734681376302 ) ) ;
#12727=AXIS2_PLACEMENT_3D ( 'NONE', #45274, #84950, #50694 ) ;
#12728=VERTEX_POINT ( 'NONE', #37832 ) ;
#12729=FACE_BOUND ( 'NONE', #56879, .T. ) ;
#12730=VERTEX_POINT ( 'NONE', #18464 ) ;
#12731=CARTESIAN_POINT ( 'NONE',  ( -8.769230769230892619, -12.51329471203414379, 31.30864560766407578 ) ) ;
#12732=CARTESIAN_POINT ( 'NONE',  ( -12.21148404162501144, -2.920487667080175598, 32.31805714834170828 ) ) ;
#12733=CARTESIAN_POINT ( 'NONE',  ( 6.065255571276024327, -9.442884908240271713, 34.35708131394835618 ) ) ;
#12735=FACE_OUTER_BOUND ( 'NONE', #62179, .T. ) ;
#12736=ORIENTED_EDGE ( 'NONE', *, *, #18080, .T. ) ;
#12738=ORIENTED_EDGE ( 'NONE', *, *, #24444, .F. ) ;
#12739=ORIENTED_EDGE ( 'NONE', *, *, #30189, .T. ) ;
#12740=CARTESIAN_POINT ( 'NONE',  ( -5.142193077479396024, -4.320704448112771878, 33.92786785259540494 ) ) ;
#12741=CARTESIAN_POINT ( 'NONE',  ( 15.10062126103753499, -3.625366637846545892, 33.29286588640298561 ) ) ;
#12742=CIRCLE ( 'NONE', #48684, 2.000000000000001776 ) ;
#12743=CARTESIAN_POINT ( 'NONE',  ( -2.242546528360342073, -7.750023238201980469, 34.74374492549440419 ) ) ;
#12744=CARTESIAN_POINT ( 'NONE',  ( 6.065255571276026103, -12.27809138561124591, 31.22303859784720359 ) ) ;
#12747=CARTESIAN_POINT ( 'NONE',  ( -5.076923076923075762, -4.098570777380720287, 33.41473453929634729 ) ) ;
#12748=CYLINDRICAL_SURFACE ( 'NONE', #76418, 0.2499999999999986955 ) ;
#12750=ORIENTED_EDGE ( 'NONE', *, *, #76965, .T. ) ;
#12751=ORIENTED_EDGE ( 'NONE', *, *, #79177, .T. ) ;
#12752=LINE ( 'NONE', #39356, #61817 ) ;
#12753=ORIENTED_EDGE ( 'NONE', *, *, #69657, .T. ) ;
#12754=CARTESIAN_POINT ( 'NONE',  ( -1.384615384615383471, -2.486705287966279876, 31.30864560766543647 ) ) ;
#12756=EDGE_CURVE ( 'NONE', #34882, #66105, #72955, .T. ) ;
#12759=DIRECTION ( 'NONE',  ( 0.000000000000000000, 0.7660444431189822323, -0.6427876096865344779 ) ) ;
#12760=FACE_BOUND ( 'NONE', #33115, .T. ) ;
#12761=ORIENTED_EDGE ( 'NONE', *, *, #34356, .T. ) ;
#12762=CARTESIAN_POINT ( 'NONE',  ( -3.480745974817822663, -3.436278759898155233, 33.07459398097509506 ) ) ;
#12763=ORIENTED_EDGE ( 'NONE', *, *, #33980, .T. ) ;
#12764=CARTESIAN_POINT ( 'NONE',  ( 17.07692307692295586, -5.941354392335915335, 34.76329471203413846 ) ) ;
#12765=VERTEX_POINT ( 'NONE', #32415 ) ;
#12766=FACE_BOUND ( 'NONE', #10168, .T. ) ;
#12767=CARTESIAN_POINT ( 'NONE',  ( -1.384615384615506484, -11.06231777344772027, 33.60647404775119895 ) ) ;
#12769=CARTESIAN_POINT ( 'NONE',  ( 15.23076923076910916, -6.835583212225970762, 34.95778746994575670 ) ) ;
#12770=ORIENTED_EDGE ( 'NONE', *, *, #81609, .F. ) ;
#12772=CARTESIAN_POINT ( 'NONE',  ( -12.21153846153846168, -7.500000000000001776, 35.04278698407183867 ) ) ;
#12773=CARTESIAN_POINT ( 'NONE',  ( -0.6844654204453102242, -2.308479472611653094, 30.53278059502174457 ) ) ;
#12774=ORIENTED_EDGE ( 'NONE', *, *, #61801, .T. ) ;
#12776=DIRECTION ( 'NONE',  ( -0.000000000000000000, -0.7660444431189791237, -0.6427876096865379196 ) ) ;
#12777=CARTESIAN_POINT ( 'NONE',  ( 14.05771556364371833, -11.47974371597207899, 33.17467449705390692 ) ) ;
#12778=CARTESIAN_POINT ( 'NONE',  ( -3.454254174493176954, -2.847400154188067578, 31.58180166144859768 ) ) ;
#12779=DIRECTION ( 'NONE',  ( -0.000000000000000000, -0.6427876096865404731, -0.7660444431189770143 ) ) ;
#12780=VERTEX_POINT ( 'NONE', #12153 ) ;
#12781=VECTOR ( 'NONE', #83647, 1000.000000000000227 ) ;
#12782=CARTESIAN_POINT ( 'NONE',  ( -1.384615384615505151, -6.026961402154118908, 34.52809138561165270 ) ) ;
#12783=LINE ( 'NONE', #55095, #15401 ) ;
#12784=AXIS2_PLACEMENT_3D ( 'NONE', #50225, #15579, #7931 ) ;
#12785=VERTEX_POINT ( 'NONE', #79274 ) ;
#12786=CARTESIAN_POINT ( 'NONE',  ( -12.71151520558705172, -5.643011162660950042, 34.66104346484419096 ) ) ;
#12787=CARTESIAN_POINT ( 'NONE',  ( 9.758474298899335153, -7.250054591869670162, 34.99404684341514127 ) ) ;
#12788=CARTESIAN_POINT ( 'NONE',  ( -7.912236225513981758, -12.34228464037088280, 31.77849191805838558 ) ) ;
#12789=DIRECTION ( 'NONE',  ( -0.000000000000000000, 0.8660254037844397068, -0.4999999999999978906 ) ) ;
#12790=CARTESIAN_POINT ( 'NONE',  ( 0.3954560821783256186, -2.486705287966280320, 31.30864560766544002 ) ) ;
#12791=CARTESIAN_POINT ( 'NONE',  ( 17.01165307636676260, -5.094484230520675894, 34.41647553114621161 ) ) ;
#12792=DIRECTION ( 'NONE',  ( 0.000000000000000000, 0.7660444431189807890, 0.6427876096865361433 ) ) ;
#12793=CARTESIAN_POINT ( 'NONE',  ( 16.21991450484859598, -5.557115091759786019, 34.35708131394839882 ) ) ;
#12795=EDGE_CURVE ( 'NONE', #87491, #14948, #81955, .T. ) ;
#12796=CARTESIAN_POINT ( 'NONE',  ( 18.00000000000000000, -1.790695186598648903, 34.54067556320373455 ) ) ;
#12798=ORIENTED_EDGE ( 'NONE', *, *, #62528, .T. ) ;
#12799=CARTESIAN_POINT ( 'NONE',  ( 17.74997676270703550, -4.335965774309648246, 33.62209801155881905 ) ) ;
#12800=ORIENTED_EDGE ( 'NONE', *, *, #83946, .T. ) ;
#12801=EDGE_LOOP ( 'NONE', ( #75487, #7024 ) ) ;
#12802=CARTESIAN_POINT ( 'NONE',  ( -8.769230769230768274, -6.343179335718451384, 34.87096338111211935 ) ) ;
#12803=EDGE_LOOP ( 'NONE', ( #19364, #86743, #38988, #9081 ) ) ;
#12804=CARTESIAN_POINT ( 'NONE',  ( -4.403869378067613027, -2.588893531581426544, 31.60682220781847818 ) ) ;
#12806=CARTESIAN_POINT ( 'NONE',  ( 12.33106327646274103, -7.276987145209184327, 34.99546412871779211 ) ) ;
#12807=CARTESIAN_POINT ( 'NONE',  ( -13.38461538461538325, -11.91647553114624181, 32.58852847137148245 ) ) ;
#12808=CARTESIAN_POINT ( 'NONE',  ( -4.153846153846273204, -3.835265460704628371, 33.15142922262033665 ) ) ;
#12810=CARTESIAN_POINT ( 'NONE',  ( 14.30769230769231015, -11.35647404775217417, 33.31231777344666511 ) ) ;
#12811=CARTESIAN_POINT ( 'NONE',  ( 2.557637826040450868, -11.37275283266503756, 32.91324779482534524 ) ) ;
#12813=CARTESIAN_POINT ( 'NONE',  ( 10.86543903529806876, -12.41089969410671223, 31.60739465890703670 ) ) ;
#12814=CARTESIAN_POINT ( 'NONE',  ( -4.219928533206287469, -11.91647553114624181, 32.58852847137148245 ) ) ;
#12815=ADVANCED_FACE ( 'NONE', ( #24310 ), #65739, .F. ) ;
#12816=EDGE_CURVE ( 'NONE', #42788, #45049, #3599, .T. ) ;
#12817=CARTESIAN_POINT ( 'NONE',  ( 18.25000000000000000, -2.499999999999999556, 29.81604066197449754 ) ) ;
#12818=VECTOR ( 'NONE', #1907, 1000.000000000000114 ) ;
#12820=VERTEX_POINT ( 'NONE', #86491 ) ;
#12821=EDGE_CURVE ( 'NONE', #73573, #17458, #17488, .T. ) ;
#12822=CARTESIAN_POINT ( 'NONE',  ( 6.923076923076802558, -2.625532179533778709, 30.86335684631627174 ) ) ;
#12823=DIRECTION ( 'NONE',  ( -0.000000000000000000, 0.8660254037844399289, -0.4999999999999980016 ) ) ;
#12825=CARTESIAN_POINT ( 'NONE',  ( 6.000000000000317080, -2.255955759149395501, 30.00000000000324363 ) ) ;
#12826=EDGE_CURVE ( 'NONE', #7659, #45196, #46373, .T. ) ;
#12828=CARTESIAN_POINT ( 'NONE',  ( -5.999999999999998224, -8.120952969808772792, 34.71129190930000163 ) ) ;
#12829=FACE_OUTER_BOUND ( 'NONE', #50735, .T. ) ;
#12831=CARTESIAN_POINT ( 'NONE',  ( -5.011667505647053211, -12.46129190930001052, 30.37095296980870174 ) ) ;
#12834=CARTESIAN_POINT ( 'NONE',  ( 17.93391658904412012, -3.050289026998445951, 32.03036669348365706 ) ) ;
#12837=CARTESIAN_POINT ( 'NONE',  ( 14.17754509825408960, -5.195881422630166391, 34.18770438780619259 ) ) ;
#12838=CARTESIAN_POINT ( 'NONE',  ( 5.999999999999878320, -8.656820664282941280, 34.87096338111179961 ) ) ;
#12839=CARTESIAN_POINT ( 'NONE',  ( -13.38461538461550759, -2.657715359629662544, 31.77849191805970364 ) ) ;
#12840=AXIS2_PLACEMENT_3D ( 'NONE', #42772, #37314, #36877 ) ;
#12842=VECTOR ( 'NONE', #26217, 1000.000000000000227 ) ;
#12843=ORIENTED_EDGE ( 'NONE', *, *, #60235, .T. ) ;
#12844=EDGE_CURVE ( 'NONE', #86258, #54572, #89042, .T. ) ;
#12845=EDGE_LOOP ( 'NONE', ( #9955, #50916, #35208, #49349, #12025, #62804 ) ) ;
#12846=EDGE_LOOP ( 'NONE', ( #36419, #48731, #84634, #87750 ) ) ;
#12847=CARTESIAN_POINT ( 'NONE',  ( -17.14300648787895653, -10.51840700105979565, 33.73612834413961536 ) ) ;
#12848=CARTESIAN_POINT ( 'NONE',  ( 5.010839665967196765, -10.51840700105979387, 33.73612834413961536 ) ) ;
#12850=CARTESIAN_POINT ( 'NONE',  ( -16.40382289789473802, -2.318417181685854978, 30.59732222474233865 ) ) ;
#12851=LINE ( 'NONE', #46640, #16292 ) ;
#12852=CYLINDRICAL_SURFACE ( 'NONE', #35117, 0.2499999999999997502 ) ;
#12853=EDGE_LOOP ( 'NONE', ( #55817, #53038, #84820, #32332 ) ) ;
#12854=ORIENTED_EDGE ( 'NONE', *, *, #42597, .T. ) ;
#12855=EDGE_CURVE ( 'NONE', #57187, #53046, #44572, .T. ) ;
#12856=VERTEX_POINT ( 'NONE', #62853 ) ;
#12857=CARTESIAN_POINT ( 'NONE',  ( -0.4615384615384611200, -9.819645486525091727, 36.12317359536749706 ) ) ;
#12858=ORIENTED_EDGE ( 'NONE', *, *, #26788, .T. ) ;
#12859=CARTESIAN_POINT ( 'NONE',  ( 9.692307692307695177, -8.164416787775445883, 34.95778746994557906 ) ) ;
#12860=CARTESIAN_POINT ( 'NONE',  ( 6.857320120562612864, -7.249945686854186278, 34.74374336980224598 ) ) ;
#12862=ORIENTED_EDGE ( 'NONE', *, *, #36567, .F. ) ;
#12863=CYLINDRICAL_SURFACE ( 'NONE', #55505, 0.2499999999999995559 ) ;
#12864=AXIS2_PLACEMENT_3D ( 'NONE', #64942, #50543, #37026 ) ;
#12865=ORIENTED_EDGE ( 'NONE', *, *, #86142, .T. ) ;
#12866=DIRECTION ( 'NONE',  ( -0.000000000000000000, -0.3420201433256694346, -0.9396926207859080948 ) ) ;
#12867=FACE_BOUND ( 'NONE', #30426, .T. ) ;
#12868=CYLINDRICAL_SURFACE ( 'NONE', #74881, 0.2499999999999973355 ) ;
#12870=DIRECTION ( 'NONE',  ( 0.000000000000000000, 0.8660254037844377084, 0.5000000000000015543 ) ) ;
#12872=DIRECTION ( 'NONE',  ( -0.000000000000000000, 0.7660444431189792347, -0.6427876096865379196 ) ) ;
#12873=B_SPLINE_CURVE_WITH_KNOTS ( 'NONE', 3,
 ( #16786, #37954, #79389, #65422, #85704, #17234, #84831, #44690, #43818, #58657 ),
 .UNSPECIFIED., .F., .F.,
 ( 4, 2, 2, 2, 4 ),
 ( 0.0007817246256747489071, 0.0009771112852218920199, 0.001172497944769035133, 0.001367884604316178246, 0.001563271263863321358 ),
 .UNSPECIFIED. ) ;
#12874=ADVANCED_FACE ( 'NONE', ( #56998 ), #35401, .F. ) ;
#12875=CARTESIAN_POINT ( 'NONE',  ( 5.076923076923075762, -1.509761064869970415, 31.06009739812519044 ) ) ;
#12876=ORIENTED_EDGE ( 'NONE', *, *, #66341, .F. ) ;
#12877=CARTESIAN_POINT ( 'NONE',  ( -9.442362282929648742, -4.932303261841489928, 34.32971442181322885 ) ) ;
#12878=CARTESIAN_POINT ( 'NONE',  ( 1.253924781505077579, -3.957541250942359756, 33.62499894934981626 ) ) ;
#12879=CARTESIAN_POINT ( 'NONE',  ( -3.930833309752758797, -2.308499170217967134, 30.53291367094873721 ) ) ;
#12880=DIRECTION ( 'NONE',  ( 0.000000000000000000, 0.8660254037844377084, 0.5000000000000015543 ) ) ;
#12881=DIRECTION ( 'NONE',  ( -0.000000000000000000, 0.8660254037844397068, -0.4999999999999978906 ) ) ;
#12882=FACE_BOUND ( 'NONE', #29180, .T. ) ;
#12883=CARTESIAN_POINT ( 'NONE',  ( 5.750023255951409951, -4.818429247618089661, 34.26397095200675125 ) ) ;
#12884=CARTESIAN_POINT ( 'NONE',  ( -7.846153846153967493, -11.06231777344772027, 33.60647404775119895 ) ) ;
#12885=EDGE_CURVE ( 'NONE', #17603, #28930, #83065, .T. ) ;
#12886=CARTESIAN_POINT ( 'NONE',  ( 2.177001704581999597, -9.929715669179220328, 34.40415004197138416 ) ) ;
#12887=CARTESIAN_POINT ( 'NONE',  ( 3.295915010101195364, -7.750023238201980469, 34.74374492549440419 ) ) ;
#12888=CARTESIAN_POINT ( 'NONE',  ( -9.626239341305252495, -10.51840700105979565, 33.73612834413962247 ) ) ;
#12889=CARTESIAN_POINT ( 'NONE',  ( -8.703975197954742171, -3.835265460703683349, 33.15142922261929925 ) ) ;
#12891=EDGE_LOOP ( 'NONE', ( #55595, #13985, #3249, #84377 ) ) ;
#12893=ORIENTED_EDGE ( 'NONE', *, *, #82910, .F. ) ;
#12894=EDGE_CURVE ( 'NONE', #32391, #79032, #50802, .T. ) ;
#12895=CARTESIAN_POINT ( 'NONE',  ( -18.00000000000012079, -3.643525952248793498, 33.31231777344770961 ) ) ;
#12897=CARTESIAN_POINT ( 'NONE',  ( 7.780070435197966816, -8.973038597847269315, 34.52809138561120506 ) ) ;
#12898=DIRECTION ( 'NONE',  ( -0.000000000000000000, -0.1736481776669307198, -0.9848077530122080203 ) ) ;
#12899=EDGE_CURVE ( 'NONE', #38093, #25274, #21798, .T. ) ;
#12900=CARTESIAN_POINT ( 'NONE',  ( 15.10020863902730959, -2.504760397472875155, 29.97295953869789997 ) ) ;
#12901=EDGE_LOOP ( 'NONE', ( #50495, #69490, #6948, #7314 ) ) ;
#12902=CARTESIAN_POINT ( 'NONE',  ( -11.53846153846153655, -2.249999999999998668, 29.75000000000001776 ) ) ;
#12903=CARTESIAN_POINT ( 'NONE',  ( 18.13083833048675686, -7.277220318596959281, 34.99547417642776992 ) ) ;
#12906=CARTESIAN_POINT ( 'NONE',  ( 4.376625695114562120, -10.81320215134717344, 33.49497208177562868 ) ) ;
#12907=CARTESIAN_POINT ( 'NONE',  ( 10.61538461538449418, -9.528491918059723176, 34.59228464037033035 ) ) ;
#12908=CARTESIAN_POINT ( 'NONE',  ( -4.853910232829680815, -11.98016756924215009, 32.48728574198911190 ) ) ;
#12910=DIRECTION ( 'NONE',  ( 0.000000000000000000, 0.7660444431189807890, 0.6427876096865361433 ) ) ;
#12911=CARTESIAN_POINT ( 'NONE',  ( -11.28851602011339672, -10.05730279482229683, 34.04704008940765902 ) ) ;
#12912=AXIS2_PLACEMENT_3D ( 'NONE', #69965, #50571, #63200 ) ;
#12914=CARTESIAN_POINT ( 'NONE',  ( 3.480769230769293898, -7.434744860731434812, 35.00000000000000711 ) ) ;
#12915=EDGE_CURVE ( 'NONE', #26314, #27369, #27756, .T. ) ;
#12916=B_SPLINE_CURVE_WITH_KNOTS ( 'NONE', 3,
 ( #23627, #73623, #85789, #30389, #3803, #86697, #11913, #32177, #66399, #51078 ),
 .UNSPECIFIED., .F., .F.,
 ( 4, 2, 2, 2, 4 ),
 ( 0.0007817359430256294638, 0.0009771253907249948054, 0.001172514838424360255, 0.001367904286123725489, 0.001563293733823090939 ),
 .UNSPECIFIED. ) ;
#12917=CARTESIAN_POINT ( 'NONE',  ( 6.989145274079363368, -11.16473453929635440, 33.15142922261926373 ) ) ;
#12918=VERTEX_POINT ( 'NONE', #75950 ) ;
#12919=CARTESIAN_POINT ( 'NONE',  ( 8.769230769230645706, -9.528491918059723176, 34.59228464037033035 ) ) ;
#12920=DIRECTION ( 'NONE',  ( -0.000000000000000000, 1.000000000000000000, -0.000000000000000000 ) ) ;
#12922=EDGE_CURVE ( 'NONE', #19281, #39535, #55228, .T. ) ;
#12923=CARTESIAN_POINT ( 'NONE',  ( -17.93474442872397034, -12.46129190930001052, 30.37095296980869819 ) ) ;
#12924=LINE ( 'NONE', #53006, #2398 ) ;
#12925=EDGE_LOOP ( 'NONE', ( #63115, #42892 ) ) ;
#12926=FACE_OUTER_BOUND ( 'NONE', #49168, .T. ) ;
#12928=DIRECTION ( 'NONE',  ( 0.000000000000000000, 0.9396926207859126468, 0.3420201433256571111 ) ) ;
#12930=CARTESIAN_POINT ( 'NONE',  ( 12.71148397988660150, -12.43552623307873972, 30.55307653245132826 ) ) ;
#12932=CARTESIAN_POINT ( 'NONE',  ( 5.326923076923138822, -7.434744860731433924, 35.00000000000000711 ) ) ;
#12933=CARTESIAN_POINT ( 'NONE',  ( -11.53846153846153655, -2.486705287966279876, 31.30864560766543647 ) ) ;
#12935=CARTESIAN_POINT ( 'NONE',  ( -11.53846153846166089, -4.320704448113951379, 33.92786785259630022 ) ) ;
#12938=EDGE_LOOP ( 'NONE', ( #81441, #2082, #37092, #74916 ) ) ;
#12940=EDGE_CURVE ( 'NONE', #79735, #58351, #29543, .T. ) ;
#12941=ORIENTED_EDGE ( 'NONE', *, *, #69620, .T. ) ;
#12942=EDGE_LOOP ( 'NONE', ( #64362, #55957, #60394, #54027 ) ) ;
#12943=CARTESIAN_POINT ( 'NONE',  ( 12.52760579488853665, -9.905515769479276145, 34.41647553114623292 ) ) ;
#12945=EDGE_CURVE ( 'NONE', #27787, #31685, #48584, .T. ) ;
#12946=CARTESIAN_POINT ( 'NONE',  ( 13.38461538461538680, -3.050289026998446396, 32.03036669348365706 ) ) ;
#12947=CARTESIAN_POINT ( 'NONE',  ( -16.85349667800829465, -7.630147987733843173, 34.99859428049665411 ) ) ;
#12948=CARTESIAN_POINT ( 'NONE',  ( 5.326977388561388693, -5.728107161865375829, 34.42597550085002922 ) ) ;
#12950=B_SPLINE_CURVE_WITH_KNOTS ( 'NONE', 3,
 ( #34408, #6063, #61872, #26328, #82622, #14141, #69084, #88498, #25885, #80848 ),
 .UNSPECIFIED., .F., .F.,
 ( 4, 2, 2, 2, 4 ),
 ( 0.000000000000000000, 0.0001954339857564071762, 0.0003908679715128143524, 0.0005863019572692215828, 0.0007817359430256287049 ),
 .UNSPECIFIED. ) ;
#12951=EDGE_CURVE ( 'NONE', #74505, #57294, #36734, .T. ) ;
#12952=EDGE_LOOP ( 'NONE', ( #1361, #5542 ) ) ;
#12953=EDGE_LOOP ( 'NONE', ( #40090, #63762 ) ) ;
#12954=CARTESIAN_POINT ( 'NONE',  ( -7.146003881983771677, -8.282780595021769443, 34.94152052738834868 ) ) ;
#12955=ORIENTED_EDGE ( 'NONE', *, *, #63416, .T. ) ;
#12957=EDGE_CURVE ( 'NONE', #19489, #83181, #55138, .T. ) ;
#12958=CARTESIAN_POINT ( 'NONE',  ( -10.55023883605264956, -7.750023238201979581, 34.74374492549440419 ) ) ;
#12960=VECTOR ( 'NONE', #28041, 999.9999999999998863 ) ;
#12962=CARTESIAN_POINT ( 'NONE',  ( 5.999999999999878320, -4.320704448113951379, 33.92786785259630022 ) ) ;
#12963=CARTESIAN_POINT ( 'NONE',  ( -14.98071491913091791, -9.148310452688876993, 34.47095581063188519 ) ) ;
#12964=ORIENTED_EDGE ( 'NONE', *, *, #67670, .T. ) ;
#12965=VECTOR ( 'NONE', #76504, 1000.000000000000114 ) ;
#12966=ORIENTED_EDGE ( 'NONE', *, *, #70824, .T. ) ;
#12968=ADVANCED_FACE ( 'NONE', ( #43492 ), #30855, .F. ) ;
#12970=CARTESIAN_POINT ( 'NONE',  ( -10.61538461538473577, -11.06231777344772027, 33.60647404775119895 ) ) ;
#12971=DIRECTION ( 'NONE',  ( 0.000000000000000000, 0.9848077530122072432, -0.1736481776669354937 ) ) ;
#12972=ORIENTED_EDGE ( 'NONE', *, *, #71227, .F. ) ;
#12974=CARTESIAN_POINT ( 'NONE',  ( -11.53846153846166089, -12.70778746994576025, 30.41441678777401236 ) ) ;
#12975=CARTESIAN_POINT ( 'NONE',  ( -14.43783951713052716, -2.619462340734462380, 30.83744416345203021 ) ) ;
#12976=ORIENTED_EDGE ( 'NONE', *, *, #81263, .F. ) ;
#12977=CARTESIAN_POINT ( 'NONE',  ( -17.07692307692319744, -9.442884908241554243, 34.35708131394783038 ) ) ;
#12978=CARTESIAN_POINT ( 'NONE',  ( 8.834486340506792601, -12.46129190930001052, 30.37095296980870174 ) ) ;
#12980=FACE_BOUND ( 'NONE', #27114, .T. ) ;
#12981=CARTESIAN_POINT ( 'NONE',  ( -17.07692307692307665, -1.509761064869970415, 31.06009739812519044 ) ) ;
#12982=CARTESIAN_POINT ( 'NONE',  ( -15.23076923076922995, -9.584722331328613620, 36.20867863119891439 ) ) ;
#12983=CARTESIAN_POINT ( 'NONE',  ( -3.230769230769229949, -8.164416787775445883, 34.95778746994557906 ) ) ;
#12984=CARTESIAN_POINT ( 'NONE',  ( -2.307692307692305711, -8.120952969808772792, 34.71129190930000163 ) ) ;
#12985=CARTESIAN_POINT ( 'NONE',  ( -8.769230769230892619, -12.16647553114689728, 32.15551576947799362 ) ) ;
#12986=CARTESIAN_POINT ( 'NONE',  ( -4.854143535654665165, -10.81320215134717344, 33.49497208177562868 ) ) ;
#12987=CARTESIAN_POINT ( 'NONE',  ( 12.68455130563185840, -2.889357225399416418, 32.26129605718031002 ) ) ;
#12988=ORIENTED_EDGE ( 'NONE', *, *, #28431, .F. ) ;
#12989=CARTESIAN_POINT ( 'NONE',  ( -17.29985003582992320, -5.582147617184174848, 34.63737895849758530 ) ) ;
#12991=ADVANCED_FACE ( 'NONE', ( #2491 ), #64631, .F. ) ;
#12992=EDGE_LOOP ( 'NONE', ( #38295, #71646 ) ) ;
#12993=CARTESIAN_POINT ( 'NONE',  ( -6.673022611438607754, -4.943051570960391494, 34.04725096376909477 ) ) ;
#12994=CARTESIAN_POINT ( 'NONE',  ( -14.55771554498526932, -5.056417327199099532, 34.11270091957321426 ) ) ;
#12995=CARTESIAN_POINT ( 'NONE',  ( -7.715628407920204879, -2.372941743896878286, 30.88044141588253666 ) ) ;
#12996=ORIENTED_EDGE ( 'NONE', *, *, #57907, .T. ) ;
#12997=FACE_OUTER_BOUND ( 'NONE', #9895, .T. ) ;
#12998=CARTESIAN_POINT ( 'NONE',  ( 6.792386319966617236, -8.191372820521381826, 34.95448215188423546 ) ) ;
#12999=FACE_BOUND ( 'NONE', #75713, .T. ) ;
#13000=DIRECTION ( 'NONE',  ( -0.000000000000000000, -0.8660254037844397068, -0.4999999999999978906 ) ) ;
#13001=DIRECTION ( 'NONE',  ( 0.000000000000000000, 0.6427876096865368094, 0.7660444431189802339 ) ) ;
#13002=CARTESIAN_POINT ( 'NONE',  ( -13.60754234352223335, -2.308479472611653094, 30.53278059502174457 ) ) ;
#13003=CARTESIAN_POINT ( 'NONE',  ( -16.15384615384615330, -5.180354513474913603, 36.12317359536750416 ) ) ;
#13005=CARTESIAN_POINT ( 'NONE',  ( -10.54931728203453822, -11.35647404775217595, 33.31231777344666511 ) ) ;
#13009=ORIENTED_EDGE ( 'NONE', *, *, #77213, .T. ) ;
#13010=ORIENTED_EDGE ( 'NONE', *, *, #82942, .T. ) ;
#13011=DIRECTION ( 'NONE',  ( -0.000000000000000000, 0.6427876096865404731, -0.7660444431189771253 ) ) ;
#13012=CARTESIAN_POINT ( 'NONE',  ( 12.21153846153846168, -7.500000000000001776, 34.75000000000000000 ) ) ;
#13013=CARTESIAN_POINT ( 'NONE',  ( 16.21910129335899242, -3.083524468853783951, 32.58852847137153930 ) ) ;
#13014=CARTESIAN_POINT ( 'NONE',  ( 10.83816428436267820, -3.020022701398814569, 32.48759521482552515 ) ) ;
#13015=CARTESIAN_POINT ( 'NONE',  ( 5.142990410273151625, -3.322132147404559976, 32.92929555188717927 ) ) ;
#13017=CARTESIAN_POINT ( 'NONE',  ( -1.608100309179715470, -4.225889041578353655, 33.85425143139329407 ) ) ;
#13018=CARTESIAN_POINT ( 'NONE',  ( 5.934729999443682402, -3.083524468853724443, 32.58852847137143272 ) ) ;
#13019=CYLINDRICAL_SURFACE ( 'NONE', #50176, 0.2500000000000002220 ) ;
#13020=CARTESIAN_POINT ( 'NONE',  ( -1.634615384615382805, -7.566082377512563184, 35.00000000000000711 ) ) ;
#13021=CARTESIAN_POINT ( 'NONE',  ( 9.822833394071254887, -2.882268652242222284, 31.66798894389554064 ) ) ;
#13022=CARTESIAN_POINT ( 'NONE',  ( 13.25446817517716447, -4.460286881179643004, 33.72017969459903242 ) ) ;
#13023=CARTESIAN_POINT ( 'NONE',  ( 6.923076923076924238, -11.16473453929635440, 33.15142922261926373 ) ) ;
#13024=CARTESIAN_POINT ( 'NONE',  ( 10.61538461538461675, -2.538708090699994813, 30.37095296980875503 ) ) ;
#13027=CARTESIAN_POINT ( 'NONE',  ( -16.85414340794500987, -3.020022701398814569, 32.48759521482552515 ) ) ;
#13028=ORIENTED_EDGE ( 'NONE', *, *, #69781, .F. ) ;
#13029=CARTESIAN_POINT ( 'NONE',  ( 1.318531973659504697, -2.538708090699994813, 30.37095296980875148 ) ) ;
#13030=FACE_OUTER_BOUND ( 'NONE', #48326, .T. ) ;
#13032=EDGE_CURVE ( 'NONE', #81366, #38816, #8869, .T. ) ;
#13033=CIRCLE ( 'NONE', #31674, 0.2500000000000002220 ) ;
#13035=DIRECTION ( 'NONE',  ( -0.000000000000000000, 0.3420201433256694901, -0.9396926207859082059 ) ) ;
#13036=FACE_OUTER_BOUND ( 'NONE', #56502, .T. ) ;
#13037=CARTESIAN_POINT ( 'NONE',  ( -11.28840711854808632, -4.818054556918156983, 34.26375889529406749 ) ) ;
#13038=DIRECTION ( 'NONE',  ( -0.000000000000000000, -0.5000000000000009992, -0.8660254037844380415 ) ) ;
#13039=ORIENTED_EDGE ( 'NONE', *, *, #28306, .T. ) ;
#13041=CARTESIAN_POINT ( 'NONE',  ( 3.361559671736180643, -8.191423895709840863, 34.95447573519442130 ) ) ;
#13042=EDGE_CURVE ( 'NONE', #77857, #46107, #66940, .T. ) ;
#13043=ORIENTED_EDGE ( 'NONE', *, *, #59532, .T. ) ;
#13045=CARTESIAN_POINT ( 'NONE',  ( -2.057746789344163663, -2.587454068350147907, 30.68340429815432202 ) ) ;
#13046=EDGE_CURVE ( 'NONE', #33447, #28242, #51110, .T. ) ;
#13047=( GEOMETRIC_REPRESENTATION_CONTEXT ( 3 ) GLOBAL_UNCERTAINTY_ASSIGNED_CONTEXT ( ( #36572 ) ) GLOBAL_UNIT_ASSIGNED_CONTEXT ( ( #18432, #17991, #38698 ) ) REPRESENTATION_CONTEXT ( 'NONE', 'WORKASPACE' ) );
#13048=VERTEX_POINT ( 'NONE', #51549 ) ;
#13049=CARTESIAN_POINT ( 'NONE',  ( 10.86538461538461675, -2.249999999999998668, 29.75000000000000355 ) ) ;
#13050=CARTESIAN_POINT ( 'NONE',  ( 8.519207545009313876, -6.652501968072648708, 34.93155406624980941 ) ) ;
#13051=VERTEX_POINT ( 'NONE', #84490 ) ;
#13052=EDGE_LOOP ( 'NONE', ( #72517, #69997 ) ) ;
#13053=EDGE_CURVE ( 'NONE', #3349, #11323, #62620, .T. ) ;
#13054=B_SPLINE_CURVE_WITH_KNOTS ( 'NONE', 3,
 ( #64199, #29121, #27772, #48476, #21006, #76855, #9285, #35415, #7951, #75964 ),
 .UNSPECIFIED., .F., .F.,
 ( 4, 2, 2, 2, 4 ),
 ( 0.000000000000000000, 0.0001954339857564054686, 0.0003908679715128109372, 0.0005863019572692163787, 0.0007817359430256218744 ),
 .UNSPECIFIED. ) ;
#13055=ORIENTED_EDGE ( 'NONE', *, *, #70274, .F. ) ;
#13056=CARTESIAN_POINT ( 'NONE',  ( -15.00775638667583500, -4.026326845037962343, 33.68677907613344047 ) ) ;
#13057=FACE_OUTER_BOUND ( 'NONE', #46542, .T. ) ;
#13058=CARTESIAN_POINT ( 'NONE',  ( -17.75000000000000711, -12.75000000000000178, 29.75000000000000355 ) ) ;
#13059=CARTESIAN_POINT ( 'NONE',  ( -1.515305987725692249, -11.37499894934982514, 33.29245874905763003 ) ) ;
#13061=LINE ( 'NONE', #80649, #10462 ) ;
#13062=DIRECTION ( 'NONE',  ( -0.000000000000000000, 1.000000000000000000, -0.000000000000000000 ) ) ;
#13063=DIRECTION ( 'NONE',  ( -0.000000000000000000, -0.5000000000000009992, -0.8660254037844380415 ) ) ;
#13064=VERTEX_POINT ( 'NONE', #67763 ) ;
#13065=VERTEX_POINT ( 'NONE', #18697 ) ;
#13068=VECTOR ( 'NONE', #82723, 1000.000000000000227 ) ;
#13069=EDGE_CURVE ( 'NONE', #67310, #36896, #46605, .T. ) ;
#13070=B_SPLINE_CURVE_WITH_KNOTS ( 'NONE', 3,
 ( #88159, #40834, #53897, #61530, #75068, #83150, #55224, #20554, #20986, #82713 ),
 .UNSPECIFIED., .F., .F.,
 ( 4, 2, 2, 2, 4 ),
 ( 0.000000000000000000, 0.0001954311564186861426, 0.0003908623128373722852, 0.0005862934692560583735, 0.0007817246256747445703 ),
 .UNSPECIFIED. ) ;
#13071=CARTESIAN_POINT ( 'NONE',  ( -13.31844877802374327, -7.250054591869670162, 34.99404684341514127 ) ) ;
#13072=LINE ( 'NONE', #75650, #45347 ) ;
#13073=ORIENTED_EDGE ( 'NONE', *, *, #22371, .T. ) ;
#13074=CARTESIAN_POINT ( 'NONE',  ( -12.23852561744506495, -11.43677907613344757, 33.22367315496202167 ) ) ;
#13075=EDGE_CURVE ( 'NONE', #11627, #26195, #78738, .T. ) ;
#13076=ORIENTED_EDGE ( 'NONE', *, *, #39541, .F. ) ;
#13077=CARTESIAN_POINT ( 'NONE',  ( 17.07692307692295586, -9.528491918059723176, 34.59228464037033035 ) ) ;
#13078=ORIENTED_EDGE ( 'NONE', *, *, #28818, .T. ) ;
#13079=CARTESIAN_POINT ( 'NONE',  ( 9.942253210655836781, -8.433404298154334455, 34.66254593164985920 ) ) ;
#13080=ORIENTED_EDGE ( 'NONE', *, *, #79676, .F. ) ;
#13081=EDGE_CURVE ( 'NONE', #4198, #77888, #61497, .T. ) ;
#13082=VECTOR ( 'NONE', #65924, 1000.000000000000000 ) ;
#13083=CARTESIAN_POINT ( 'NONE',  ( -8.769230769230768274, -4.786620604624113540, 33.94971097300155094 ) ) ;
#13084=CARTESIAN_POINT ( 'NONE',  ( 10.74617642320940369, -4.809403383903225304, 33.96459661697924304 ) ) ;
#13085=FACE_BOUND ( 'NONE', #80664, .T. ) ;
#13086=B_SPLINE_CURVE_WITH_KNOTS ( 'NONE', 3,
 ( #13998, #1811, #7249, #48221, #29301, #84250, #82477, #54987, #15783, #43248 ),
 .UNSPECIFIED., .F., .F.,
 ( 4, 2, 2, 2, 4 ),
 ( 0.000000000000000000, 0.0001954339857564081520, 0.0003908679715128163040, 0.0005863019572692244018, 0.0007817359430256326080 ),
 .UNSPECIFIED. ) ;
#13087=CARTESIAN_POINT ( 'NONE',  ( -17.75000000000000355, -2.499999999999999556, 29.81604066197449043 ) ) ;
#13088=CARTESIAN_POINT ( 'NONE',  ( 1.134615384615387246, -2.249999999999998668, 29.75000000000000355 ) ) ;
#13089=AXIS2_PLACEMENT_3D ( 'NONE', #53513, #73808, #19299 ) ;
#13090=AXIS2_PLACEMENT_3D ( 'NONE', #62060, #35478, #6247 ) ;
#13091=CARTESIAN_POINT ( 'NONE',  ( -1.514763354347080870, -2.373036134822905208, 30.88089517874951540 ) ) ;
#13092=CARTESIAN_POINT ( 'NONE',  ( 4.219914504848592429, -8.120952969808772792, 34.71129190929999453 ) ) ;
#13093=CARTESIAN_POINT ( 'NONE',  ( 14.30769230769231015, -2.499999999999998668, 29.50000000000001066 ) ) ;
#13095=CARTESIAN_POINT ( 'NONE',  ( -10.61538461538461320, -4.098570777380720287, 33.41473453929634729 ) ) ;
#13096=EDGE_LOOP ( 'NONE', ( #21272, #54152, #38084, #89027 ) ) ;
#13097=EDGE_CURVE ( 'NONE', #76314, #76451, #24984, .T. ) ;
#13098=VERTEX_POINT ( 'NONE', #86729 ) ;
#13099=AXIS2_PLACEMENT_3D ( 'NONE', #35259, #6898, #88901 ) ;
#13101=CARTESIAN_POINT ( 'NONE',  ( -18.06608237936013239, -9.905515769479279697, 34.41647553114623292 ) ) ;
#13102=CARTESIAN_POINT ( 'NONE',  ( 16.21991348719623360, -11.35647404775217595, 33.31231777344667222 ) ) ;
#13103=CARTESIAN_POINT ( 'NONE',  ( -3.903791733932699515, -9.233818618650603938, 34.70587769442853698 ) ) ;
#13104=EDGE_CURVE ( 'NONE', #63264, #45061, #4558, .T. ) ;
#13105=CARTESIAN_POINT ( 'NONE',  ( 5.076923076923075762, -2.249999999999998668, 29.75000000000001776 ) ) ;
#13106=CARTESIAN_POINT ( 'NONE',  ( -13.31935981333936603, -2.892918686051626498, 31.69288490824026638 ) ) ;
#13107=ADVANCED_FACE ( 'NONE', ( #47032 ), #19571, .F. ) ;
#13108=ORIENTED_EDGE ( 'NONE', *, *, #11162, .F. ) ;
#13109=CARTESIAN_POINT ( 'NONE',  ( -5.934744860487159102, -8.656820664281605460, 34.87096338111211224 ) ) ;
#13112=CARTESIAN_POINT ( 'NONE',  ( -3.230769230769352962, -12.70778746994576025, 30.41441678777401236 ) ) ;
#13113=ORIENTED_EDGE ( 'NONE', *, *, #47017, .T. ) ;
#13114=EDGE_CURVE ( 'NONE', #37535, #8529, #73190, .T. ) ;
#13115=ORIENTED_EDGE ( 'NONE', *, *, #76428, .F. ) ;
#13116=ORIENTED_EDGE ( 'NONE', *, *, #9302, .F. ) ;
#13117=DIRECTION ( 'NONE',  ( -0.000000000000000000, -0.9396926207859093161, -0.3420201433256663259 ) ) ;
#13119=CARTESIAN_POINT ( 'NONE',  ( 2.980746006547773330, -12.68155406624981119, 30.59749803192733708 ) ) ;
#13120=CARTESIAN_POINT ( 'NONE',  ( 14.98074599347626368, -9.271318131107980420, 34.42618302367067429 ) ) ;
#13121=CARTESIAN_POINT ( 'NONE',  ( -5.142193522883852452, -4.481592998940161721, 33.73612834413957984 ) ) ;
#13122=CARTESIAN_POINT ( 'NONE',  ( 8.899756207464417201, -3.625058011473228703, 33.29252011169590020 ) ) ;
#13123=B_SPLINE_CURVE_WITH_KNOTS ( 'NONE', 3,
 ( #9118, #44194, #15875, #43337, #71683, #78887, #9984, #70815, #64921, #36582 ),
 .UNSPECIFIED., .F., .F.,
 ( 4, 2, 2, 2, 4 ),
 ( 0.000000000000000000, 0.0001954339857564090465, 0.0003908679715128180929, 0.0005863019572692271123, 0.0007817359430256361858 ),
 .UNSPECIFIED. ) ;
#13124=DIRECTION ( 'NONE',  ( 0.000000000000000000, 0.9396926207859126468, -0.3420201433256571111 ) ) ;
#13125=ORIENTED_EDGE ( 'NONE', *, *, #20823, .F. ) ;
#13126=CARTESIAN_POINT ( 'NONE',  ( 15.23076923076923173, -11.16473453929635440, 33.15142922261926373 ) ) ;
#13127=DIRECTION ( 'NONE',  ( -0.000000000000000000, 0.7660444431189791237, -0.6427876096865379196 ) ) ;
#13128=ORIENTED_EDGE ( 'NONE', *, *, #73089, .T. ) ;
#13130=CARTESIAN_POINT ( 'NONE',  ( -4.153846153846152411, -13.20930481340135110, 34.54067556320372745 ) ) ;
#13131=CARTESIAN_POINT ( 'NONE',  ( 1.514662990871069592, -7.723484964179500700, 34.74522123443823318 ) ) ;
#13133=B_SPLINE_CURVE_WITH_KNOTS ( 'NONE', 3,
 ( #2617, #29233, #57130, #84622, #48594, #76968, #56688, #9394, #84183, #8511 ),
 .UNSPECIFIED., .F., .F.,
 ( 4, 2, 2, 2, 4 ),
 ( 0.0007817246256747448956, 0.0009771112852218876831, 0.001172497944769030579, 0.001367884604316173475, 0.001563271263863316371 ),
 .UNSPECIFIED. ) ;
#13134=CARTESIAN_POINT ( 'NONE',  ( 8.992243613324164997, -11.98016756924215009, 32.48728574198911190 ) ) ;
#13135=DIRECTION ( 'NONE',  ( 0.000000000000000000, 1.000000000000000000, 0.000000000000000000 ) ) ;
#13136=CARTESIAN_POINT ( 'NONE',  ( 18.25005431163831204, -2.564540009722896752, 30.55348353981672105 ) ) ;
#13137=CARTESIAN_POINT ( 'NONE',  ( -9.692307692307812417, -6.026961402154118019, 34.52809138561165270 ) ) ;
#13140=CARTESIAN_POINT ( 'NONE',  ( 11.78851585009985214, -2.779044189368095719, 31.39831045268885745 ) ) ;
#13143=CARTESIAN_POINT ( 'NONE',  ( -6.923076923076922462, -3.322132147404559976, 32.92929555188717927 ) ) ;
#13144=VERTEX_POINT ( 'NONE', #33539 ) ;
#13145=CARTESIAN_POINT ( 'NONE',  ( -5.777220458731590291, -2.600157965045225339, 30.74683119005207743 ) ) ;
#13146=CARTESIAN_POINT ( 'NONE',  ( -12.71156169883143150, -3.202444869320336451, 32.30641848906366675 ) ) ;
#13147=CARTESIAN_POINT ( 'NONE',  ( -7.053768389744482725, -5.582088688514999397, 34.36776431015576350 ) ) ;
#13148=CARTESIAN_POINT ( 'NONE',  ( -4.946877914088298134, -2.504778602574660340, 29.97347330155780298 ) ) ;
#13149=EDGE_CURVE ( 'NONE', #3410, #9565, #16370, .T. ) ;
#13150=CARTESIAN_POINT ( 'NONE',  ( -15.23076923076935252, -8.656820664282941280, 34.87096338111179961 ) ) ;
#13151=EDGE_LOOP ( 'NONE', ( #19153, #17053, #34750, #13184 ) ) ;
#13152=CARTESIAN_POINT ( 'NONE',  ( 16.94677586748485965, -3.285722584762969856, 32.44110544564090759 ) ) ;
#13154=CARTESIAN_POINT ( 'NONE',  ( 9.692307692307572609, -3.835265460704628371, 33.15142922262033665 ) ) ;
#13155=CARTESIAN_POINT ( 'NONE',  ( -14.05769230769088729, -7.500000000000154543, 35.00000000000007105 ) ) ;
#13156=VERTEX_POINT ( 'NONE', #1521 ) ;
#13157=ADVANCED_FACE ( 'NONE', ( #20894 ), #7833, .F. ) ;
#13159=AXIS2_PLACEMENT_3D ( 'NONE', #20298, #12652, #40137 ) ;
#13161=DIRECTION ( 'NONE',  ( 0.000000000000000000, 0.1736481776669275834, 0.9848077530122086864 ) ) ;
#13163=ORIENTED_EDGE ( 'NONE', *, *, #20905, .F. ) ;
#13164=DIRECTION ( 'NONE',  ( 0.000000000000000000, 0.000000000000000000, 1.000000000000000000 ) ) ;
#13165=DIRECTION ( 'NONE',  ( -0.000000000000000000, 0.9396926207859092051, -0.3420201433256662704 ) ) ;
#13166=CARTESIAN_POINT ( 'NONE',  ( -6.792286482109973988, -12.35292014791297710, 31.75344720912887198 ) ) ;
#13168=EDGE_CURVE ( 'NONE', #53882, #83423, #7756, .T. ) ;
#13169=CARTESIAN_POINT ( 'NONE',  ( 9.692307692307572609, -6.026961402154118019, 34.52809138561165270 ) ) ;
#13170=LINE ( 'NONE', #542, #28183 ) ;
#13171=B_SPLINE_CURVE_WITH_KNOTS ( 'NONE', 3,
 ( #87913, #47775, #88788, #33816, #61271, #73927, #40149, #12221, #27062, #54523 ),
 .UNSPECIFIED., .F., .F.,
 ( 4, 2, 2, 2, 4 ),
 ( 0.000000000000000000, 0.0001954339857564083417, 0.0003908679715128166835, 0.0005863019572692250523, 0.0007817359430256333669 ),
 .UNSPECIFIED. ) ;
#13172=VERTEX_POINT ( 'NONE', #14143 ) ;
#13173=DIRECTION ( 'NONE',  ( 0.000000000000000000, 0.000000000000000000, 1.000000000000000000 ) ) ;
#13175=CARTESIAN_POINT ( 'NONE',  ( -8.769230769230890843, -4.481592998941358097, 33.73612834414048933 ) ) ;
#13176=CARTESIAN_POINT ( 'NONE',  ( -12.39547112818838492, -2.833524468853757305, 32.15551576947925838 ) ) ;
#13177=CARTESIAN_POINT ( 'NONE',  ( 4.853438133199127869, -11.89387501736622710, 32.13663884655806413 ) ) ;
#13178=ADVANCED_FACE ( 'NONE', ( #63204 ), #83947, .F. ) ;
#13179=CARTESIAN_POINT ( 'NONE',  ( 6.065255139512838234, -5.941354392334606160, 34.76329471203374055 ) ) ;
#13182=B_SPLINE_CURVE_WITH_KNOTS ( 'NONE', 3,
 ( #80826, #73626, #18673, #19111, #46575, #38491, #86247, #58752, #65506, #32180 ),
 .UNSPECIFIED., .F., .F.,
 ( 4, 2, 2, 2, 4 ),
 ( 0.000000000000000000, 0.0001954339857564073659, 0.0003908679715128147319, 0.0005863019572692221250, 0.0007817359430256294638 ),
 .UNSPECIFIED. ) ;
#13183=VERTEX_POINT ( 'NONE', #69527 ) ;
#13184=ORIENTED_EDGE ( 'NONE', *, *, #48131, .F. ) ;
#13185=ORIENTED_EDGE ( 'NONE', *, *, #57147, .F. ) ;
#13186=VECTOR ( 'NONE', #25835, 1000.000000000000114 ) ;
#13187=EDGE_LOOP ( 'NONE', ( #35600, #68783 ) ) ;
#13188=ADVANCED_FACE ( 'NONE', ( #41179 ), #22230, .F. ) ;
#13189=CARTESIAN_POINT ( 'NONE',  ( 2.057715576749953978, -4.943428324936578910, 34.04746400365624481 ) ) ;
#13190=ADVANCED_FACE ( 'NONE', ( #41619 ), #61434, .F. ) ;
#13191=CARTESIAN_POINT ( 'NONE',  ( 16.15384615384615330, -10.67929555188718282, 33.92786785259544047 ) ) ;
#13192=AXIS2_PLACEMENT_3D ( 'NONE', #25332, #88388, #52345 ) ;
#13194=CARTESIAN_POINT ( 'NONE',  ( -12.46153846153846168, -11.33034616979429110, 35.88435417666054406 ) ) ;
#13195=ORIENTED_EDGE ( 'NONE', *, *, #42470, .T. ) ;
#13196=CARTESIAN_POINT ( 'NONE',  ( 3.480714640147274164, -9.357781135181031829, 34.66075350412533851 ) ) ;
#13197=CARTESIAN_POINT ( 'NONE',  ( -2.307692307692305711, -4.786620604624113540, 33.94971097300155094 ) ) ;
#13198=CARTESIAN_POINT ( 'NONE',  ( 17.99999999999987566, -2.625532179533778709, 30.86335684631627174 ) ) ;
#13199=CARTESIAN_POINT ( 'NONE',  ( 2.307692307692186251, -9.528491918059723176, 34.59228464037033035 ) ) ;
#13200=EDGE_LOOP ( 'NONE', ( #49302, #84788, #47595, #16160 ) ) ;
#13201=ORIENTED_EDGE ( 'NONE', *, *, #58690, .T. ) ;
#13203=DIRECTION ( 'NONE',  ( 0.000000000000000000, 0.8660254037844377084, 0.5000000000000015543 ) ) ;
#13204=CARTESIAN_POINT ( 'NONE',  ( -2.980823821391186623, -10.18230066228895758, 34.26354781536631577 ) ) ;
#13205=CARTESIAN_POINT ( 'NONE',  ( -9.915792616872023402, -4.225889041578353655, 33.85425143139329407 ) ) ;
#13206=LINE ( 'NONE', #74460, #75874 ) ;
#13207=DIRECTION ( 'NONE',  ( 0.000000000000000000, 0.9848077530122072432, -0.1736481776669354937 ) ) ;
#13208=EDGE_CURVE ( 'NONE', #62266, #48201, #59450, .T. ) ;
#13209=FACE_BOUND ( 'NONE', #85961, .T. ) ;
#13212=CARTESIAN_POINT ( 'NONE',  ( -3.099977422944443006, -6.413143153341454017, 34.63066358083362672 ) ) ;
#13213=EDGE_LOOP ( 'NONE', ( #8009, #27095 ) ) ;
#13214=CARTESIAN_POINT ( 'NONE',  ( 17.07692307692307665, -5.471508081941601098, 34.59228464037088457 ) ) ;
#13215=B_SPLINE_CURVE_WITH_KNOTS ( 'NONE', 3,
 ( #20483, #47946, #75429, #41203, #35323, #6968, #68667, #75868, #7420, #34879 ),
 .UNSPECIFIED., .F., .F.,
 ( 4, 2, 2, 2, 4 ),
 ( 0.000000000000000000, 0.0001954339857564080707, 0.0003908679715128161414, 0.0005863019572692241849, 0.0007817359430256322827 ),
 .UNSPECIFIED. ) ;
#13216=EDGE_LOOP ( 'NONE', ( #56546, #47262 ) ) ;
#13217=FACE_BOUND ( 'NONE', #33620, .T. ) ;
#13218=CARTESIAN_POINT ( 'NONE',  ( -15.93047021314797007, -2.501478030877323011, 29.88021232661721172 ) ) ;
#13219=AXIS2_PLACEMENT_3D ( 'NONE', #86229, #57845, #51965 ) ;
#13222=DIRECTION ( 'NONE',  ( 0.000000000000000000, 0.4999999999999985567, 0.8660254037844395958 ) ) ;
#13223=LINE ( 'NONE', #12772, #26021 ) ;
#13225=ORIENTED_EDGE ( 'NONE', *, *, #51944, .F. ) ;
#13226=LINE ( 'NONE', #20423, #13431 ) ;
#13227=CARTESIAN_POINT ( 'NONE',  ( 14.17700170458200581, -11.37499894934982692, 33.29245874905763003 ) ) ;
#13228=CARTESIAN_POINT ( 'NONE',  ( 15.23076923076923173, -11.91647553114624181, 32.58852847137148245 ) ) ;
#13229=CARTESIAN_POINT ( 'NONE',  ( -9.627052121031661969, -2.625532179533470512, 30.86335684631491105 ) ) ;
#13230=ORIENTED_EDGE ( 'NONE', *, *, #8435, .F. ) ;
#13232=CARTESIAN_POINT ( 'NONE',  ( -12.39628289026243380, -3.300289026998473041, 32.46337939537591666 ) ) ;
#13233=CARTESIAN_POINT ( 'NONE',  ( 3.930361229281822855, -10.23692288466677880, 34.23039457007281072 ) ) ;
#13236=CARTESIAN_POINT ( 'NONE',  ( 9.823146022794453813, -7.277220318596961057, 34.99547417642776992 ) ) ;
#13237=CARTESIAN_POINT ( 'NONE',  ( 5.934729554039226862, -9.442884908240170461, 34.35708131394840592 ) ) ;
#13238=CARTESIAN_POINT ( 'NONE',  ( -5.076923076923197442, -8.613356846316285953, 34.62446782046622218 ) ) ;
#13239=CARTESIAN_POINT ( 'NONE',  ( -10.61538461538461320, -2.538708090699994813, 30.37095296980875503 ) ) ;
#13240=DIRECTION ( 'NONE',  ( -0.000000000000000000, 0.6427876096865404731, -0.7660444431189771253 ) ) ;
#13241=CARTESIAN_POINT ( 'NONE',  ( -1.384615384615383471, -4.786620604624113540, 33.94971097300155094 ) ) ;
#13242=CARTESIAN_POINT ( 'NONE',  ( -16.15384615384615330, -8.164416787775445883, 34.95778746994557906 ) ) ;
#13243=CARTESIAN_POINT ( 'NONE',  ( -9.692307692307691624, -6.681629849574314051, 35.83090037661290239 ) ) ;
#13247=ORIENTED_EDGE ( 'NONE', *, *, #65779, .F. ) ;
#13249=DIRECTION ( 'NONE',  ( -0.000000000000000000, 0.9848077530122086864, -0.1736481776669273891 ) ) ;
#13250=ORIENTED_EDGE ( 'NONE', *, *, #81810, .T. ) ;
#13251=CARTESIAN_POINT ( 'NONE',  ( -5.143005456283213483, -11.35647404775217595, 33.31231777344666511 ) ) ;
#13253=CARTESIAN_POINT ( 'NONE',  ( 14.30769230769218758, -11.48612834414049644, 32.76840700105863391 ) ) ;
#13254=CARTESIAN_POINT ( 'NONE',  ( -11.53846153846166089, -10.33852847137269571, 34.16647553114546554 ) ) ;
#13255=CARTESIAN_POINT ( 'NONE',  ( -2.307692307692305711, -6.386643153685126251, 34.62446782046654192 ) ) ;
#13256=DIRECTION ( 'NONE',  ( -0.000000000000000000, -0.8660254037844399289, -0.4999999999999980016 ) ) ;
#13257=CARTESIAN_POINT ( 'NONE',  ( -13.63459211555773720, -2.564618984488975073, 30.55390908950641915 ) ) ;
#13260=CARTESIAN_POINT ( 'NONE',  ( -16.15384615384615330, -8.564572088678739092, 35.78748833219616898 ) ) ;
#13261=CARTESIAN_POINT ( 'NONE',  ( -6.988346923633242724, -5.094484230520674117, 34.41647553114621161 ) ) ;
#13263=B_SPLINE_CURVE_WITH_KNOTS ( 'NONE', 3,
 ( #62383, #43459, #2026, #16431, #698, #28164, #76354, #76810, #9243, #42143 ),
 .UNSPECIFIED., .F., .F.,
 ( 4, 2, 2, 2, 4 ),
 ( 0.000000000000000000, 0.0001954339857564098596, 0.0003908679715128197192, 0.0005863019572692296059, 0.0007817359430256394385 ),
 .UNSPECIFIED. ) ;
#13264=CARTESIAN_POINT ( 'NONE',  ( 5.776515075435670887, -11.60425143139329940, 33.02411095842164457 ) ) ;
#13265=ORIENTED_EDGE ( 'NONE', *, *, #45343, .F. ) ;
#13267=CARTESIAN_POINT ( 'NONE',  ( -11.40793583669797506, -6.001044277235009439, 34.52024696741798948 ) ) ;
#13268=DIRECTION ( 'NONE',  ( -0.000000000000000000, -0.5000000000000009992, -0.8660254037844380415 ) ) ;
#13269=DIRECTION ( 'NONE',  ( -0.000000000000000000, -0.9848077530122086864, -0.1736481776669273613 ) ) ;
#13270=CARTESIAN_POINT ( 'NONE',  ( 5.869308533332442401, -5.582088688514999397, 34.36776431015576350 ) ) ;
#13273=CARTESIAN_POINT ( 'NONE',  ( -39.05038313613820122, -2.499999999999999556, 29.75000000000000355 ) ) ;
#13275=FACE_OUTER_BOUND ( 'NONE', #30377, .T. ) ;
#13276=ORIENTED_EDGE ( 'NONE', *, *, #31567, .F. ) ;
#13277=VERTEX_POINT ( 'NONE', #69969 ) ;
#13279=CARTESIAN_POINT ( 'NONE',  ( 17.77651505627605033, -3.236172620538810385, 32.36188796281390267 ) ) ;
#13280=EDGE_CURVE ( 'NONE', #27014, #54976, #42953, .T. ) ;
#13281=CARTESIAN_POINT ( 'NONE',  ( 3.903846153846155520, -7.433932668274256805, 35.00000000000000711 ) ) ;
#13282=CARTESIAN_POINT ( 'NONE',  ( -4.403869391139117795, -4.335965774309649134, 33.62209801155881905 ) ) ;
#13283=CARTESIAN_POINT ( 'NONE',  ( -1.384615384615505151, -6.879047030192662504, 34.71129190930017927 ) ) ;
#13284=CARTESIAN_POINT ( 'NONE',  ( 5.776515056276056548, -2.847400154188068022, 31.58180166144859058 ) ) ;
#13286=B_SPLINE_CURVE_WITH_KNOTS ( 'NONE', 3,
 ( #59054, #67158, #17640, #17181, #51378, #87445, #66258, #51840, #45984, #4562 ),
 .UNSPECIFIED., .F., .F.,
 ( 4, 2, 2, 2, 4 ),
 ( 0.000000000000000000, 0.0001954311564186861697, 0.0003908623128373723394, 0.0005862934692560584820, 0.0007817246256747446788 ),
 .UNSPECIFIED. ) ;
#13288=B_SPLINE_CURVE_WITH_KNOTS ( 'NONE', 3,
 ( #52375, #72204, #72653, #79426, #17267, #3304, #80318, #51468, #18165, #46077 ),
 .UNSPECIFIED., .F., .F.,
 ( 4, 2, 2, 2, 4 ),
 ( 0.0007817359430256364027, 0.0009771253907250043464, 0.001172514838424372399, 0.001367904286123740234, 0.001563293733823108286 ),
 .UNSPECIFIED. ) ;
#13289=ORIENTED_EDGE ( 'NONE', *, *, #53178, .T. ) ;
#13290=B_SPLINE_CURVE_WITH_KNOTS ( 'NONE', 3,
 ( #53729, #47855, #80784, #6441, #41547, #54602, #5104, #67695, #33899, #13628 ),
 .UNSPECIFIED., .F., .F.,
 ( 4, 2, 2, 2, 4 ),
 ( 0.000000000000000000, 0.0001954339857564097512, 0.0003908679715128195024, 0.0005863019572692292807, 0.0007817359430256390048 ),
 .UNSPECIFIED. ) ;
#13291=ORIENTED_EDGE ( 'NONE', *, *, #51202, .T. ) ;
#13292=ORIENTED_EDGE ( 'NONE', *, *, #81649, .T. ) ;
#13293=EDGE_CURVE ( 'NONE', #70102, #33999, #15482, .T. ) ;
#13294=CARTESIAN_POINT ( 'NONE',  ( 18.06606733335007675, -2.292212530054420050, 30.41441678777542990 ) ) ;
#13295=CARTESIAN_POINT ( 'NONE',  ( 4.946231610255519051, -10.54014554554150607, 33.71984207302941883 ) ) ;
#13296=CARTESIAN_POINT ( 'NONE',  ( -3.480792468062195333, -10.05641848906368097, 34.04755513067966177 ) ) ;
#13297=CARTESIAN_POINT ( 'NONE',  ( 17.99999999999987566, -5.941354392335915335, 34.76329471203413846 ) ) ;
#13298=CARTESIAN_POINT ( 'NONE',  ( -17.07692307692307665, -6.435427911321262684, 35.78748833219616898 ) ) ;
#13299=ORIENTED_EDGE ( 'NONE', *, *, #23539, .F. ) ;
#13300=ORIENTED_EDGE ( 'NONE', *, *, #57086, .T. ) ;
#13301=VERTEX_POINT ( 'NONE', #86156 ) ;
#13302=CARTESIAN_POINT ( 'NONE',  ( -4.153846153846152411, -12.48256725967547354, 35.29906147534542527 ) ) ;
#13303=ORIENTED_EDGE ( 'NONE', *, *, #32323, .T. ) ;
#13304=CARTESIAN_POINT ( 'NONE',  ( 17.20771351789002424, -10.70102852606553157, 33.91149625220312913 ) ) ;
#13305=CARTESIAN_POINT ( 'NONE',  ( 7.173076923078359535, -7.500000000000155431, 34.75000000000007105 ) ) ;
#13306=VECTOR ( 'NONE', #44896, 1000.000000000000227 ) ;
#13308=EDGE_CURVE ( 'NONE', #622, #6303, #18443, .T. ) ;
#13309=ORIENTED_EDGE ( 'NONE', *, *, #53086, .F. ) ;
#13310=CARTESIAN_POINT ( 'NONE',  ( -1.134560964701929464, -2.544122305571458575, 31.48381861865057729 ) ) ;
#13311=ORIENTED_EDGE ( 'NONE', *, *, #83911, .T. ) ;
#13312=LINE ( 'NONE', #19622, #84476 ) ;
#13313=ADVANCED_FACE ( 'NONE', ( #24428 ), #45148, .F. ) ;
#13314=FACE_BOUND ( 'NONE', #79606, .T. ) ;
#13315=DIRECTION ( 'NONE',  ( 0.000000000000000000, 0.7660444431189807890, 0.6427876096865361433 ) ) ;
#13317=CARTESIAN_POINT ( 'NONE',  ( 8.769230769230647482, -5.219633306517616589, 34.19971097300220464 ) ) ;
#13319=LINE ( 'NONE', #61938, #34645 ) ;
#13320=CARTESIAN_POINT ( 'NONE',  ( 6.792386319966616348, -11.93127051446800024, 32.56575433478200665 ) ) ;
#13321=CARTESIAN_POINT ( 'NONE',  ( -13.31946960528342139, -7.750023238201979581, 34.74374492549440419 ) ) ;
#13322=CARTESIAN_POINT ( 'NONE',  ( 0.7115927731767756059, -12.41262288849542017, 30.68299917996395010 ) ) ;
#13323=ORIENTED_EDGE ( 'NONE', *, *, #86586, .T. ) ;
#13324=CARTESIAN_POINT ( 'NONE',  ( -0.2381120626236742921, -7.630147987733843173, 34.99859428049665411 ) ) ;
#13325=DIRECTION ( 'NONE',  ( -0.000000000000000000, 0.5000000000000011102, -0.8660254037844381525 ) ) ;
#13326=CARTESIAN_POINT ( 'NONE',  ( 4.403900573759606196, -11.47946981652013498, 33.17500667209846910 ) ) ;
#13327=CARTESIAN_POINT ( 'NONE',  ( 7.846153846153846700, -13.95598074871891292, 31.83374038241031911 ) ) ;
#13329=FACE_BOUND ( 'NONE', #85216, .T. ) ;
#13330=CARTESIAN_POINT ( 'NONE',  ( -6.989159302437059296, -12.34228464037088280, 31.77849191805838558 ) ) ;
#13331=CARTESIAN_POINT ( 'NONE',  ( -5.999999999999998224, -9.905515769479276145, 34.41647553114623292 ) ) ;
#13332=CARTESIAN_POINT ( 'NONE',  ( -9.442362282929648742, -12.07971442181322175, 32.31769673815850297 ) ) ;
#13333=DIRECTION ( 'NONE',  ( 0.000000000000000000, 0.9848077530122072432, -0.1736481776669354937 ) ) ;
#13334=CARTESIAN_POINT ( 'NONE',  ( -9.627052121031667298, -10.90142922261932057, 33.41473453929631887 ) ) ;
#13335=CARTESIAN_POINT ( 'NONE',  ( -5.076923076923199218, -12.51329471203414379, 31.30864560766407578 ) ) ;
#13337=EDGE_LOOP ( 'NONE', ( #81958, #25707 ) ) ;
#13339=CARTESIAN_POINT ( 'NONE',  ( -12.21153846153704237, -7.500000000000154543, 35.00000000000007105 ) ) ;
#13341=VECTOR ( 'NONE', #2197, 999.9999999999998863 ) ;
#13342=DIRECTION ( 'NONE',  ( -0.000000000000000000, 0.3420201433256694901, -0.9396926207859082059 ) ) ;
#13343=ORIENTED_EDGE ( 'NONE', *, *, #64136, .F. ) ;
#13344=CYLINDRICAL_SURFACE ( 'NONE', #75730, 0.2500000000000009437 ) ;
#13345=DIRECTION ( 'NONE',  ( -0.000000000000000000, -0.7660444431189791237, -0.6427876096865379196 ) ) ;
#13346=DIRECTION ( 'NONE',  ( -0.000000000000000000, 0.1736481776669307198, -0.9848077530122080203 ) ) ;
#13347=ORIENTED_EDGE ( 'NONE', *, *, #64791, .F. ) ;
#13348=CARTESIAN_POINT ( 'NONE',  ( -15.29685264172511161, -4.786620604624113540, 33.94971097300155805 ) ) ;
#13350=AXIS2_PLACEMENT_3D ( 'NONE', #83853, #48268, #75740 ) ;
#13351=CARTESIAN_POINT ( 'NONE',  ( -18.00000000000000000, -2.721908614388771852, 31.22303859784724978 ) ) ;
#13352=CARTESIAN_POINT ( 'NONE',  ( -6.923076923076922462, -12.62096338111211580, 30.90682066428153263 ) ) ;
#13353=CARTESIAN_POINT ( 'NONE',  ( -5.142193522883852452, -12.46129190929999986, 30.37095296980880832 ) ) ;
#13354=DIRECTION ( 'NONE',  ( -1.000000000000000000, 0.000000000000000000, 0.000000000000000000 ) ) ;
#13355=CARTESIAN_POINT ( 'NONE',  ( -12.23875879256039489, -8.540255544307065350, 34.89611431652622286 ) ) ;
#13356=CARTESIAN_POINT ( 'NONE',  ( -5.776988648387150427, -10.61302985866383963, 33.66295027996417843 ) ) ;
#13359=CARTESIAN_POINT ( 'NONE',  ( 5.207448515156718472, -2.647132371071621471, 31.75357179365173010 ) ) ;
#13360=VERTEX_POINT ( 'NONE', #30746 ) ;
#13361=DIRECTION ( 'NONE',  ( -0.000000000000000000, 0.3420201433256694901, -0.9396926207859082059 ) ) ;
#13363=CARTESIAN_POINT ( 'NONE',  ( -5.999999999999998224, -13.37000171582298513, 34.34916445242398453 ) ) ;
#13364=CARTESIAN_POINT ( 'NONE',  ( 5.299935921016470708, -6.460100341425561332, 34.89618726649961644 ) ) ;
#13365=ORIENTED_EDGE ( 'NONE', *, *, #8664, .T. ) ;
#13366=CARTESIAN_POINT ( 'NONE',  ( -0.7115384615384606759, -7.500000000000001776, 34.75000000000000000 ) ) ;
#13368=CARTESIAN_POINT ( 'NONE',  ( -23.00000000000000000, -10.75000000000000000, 29.75000000000000355 ) ) ;
#13369=ORIENTED_EDGE ( 'NONE', *, *, #49974, .F. ) ;
#13370=CARTESIAN_POINT ( 'NONE',  ( -7.716106239898160801, -7.723484964179499812, 34.74522123443822608 ) ) ;
#13371=DIRECTION ( 'NONE',  ( 0.000000000000000000, 0.9848077530122072432, 0.1736481776669354937 ) ) ;
#13372=EDGE_CURVE ( 'NONE', #36979, #25874, #85707, .T. ) ;
#13373=CYLINDRICAL_SURFACE ( 'NONE', #61550, 0.2500000000000004996 ) ;
#13375=CARTESIAN_POINT ( 'NONE',  ( -17.01166750564705410, -2.892918686051626054, 31.69288490824025928 ) ) ;
#13376=LINE ( 'NONE', #81853, #7752 ) ;
#13377=CARTESIAN_POINT ( 'NONE',  ( -13.38461538461538325, -8.164416787775445883, 34.95778746994557906 ) ) ;
#13378=ORIENTED_EDGE ( 'NONE', *, *, #70926, .F. ) ;
#13379=VERTEX_POINT ( 'NONE', #51434 ) ;
#13380=ORIENTED_EDGE ( 'NONE', *, *, #53594, .T. ) ;
#13383=CARTESIAN_POINT ( 'NONE',  ( -9.627052121031665521, -3.300289026998473041, 32.46337939537591666 ) ) ;
#13384=CARTESIAN_POINT ( 'NONE',  ( 14.30769230769231015, -4.098570777380720287, 33.41473453929634729 ) ) ;
#13386=CARTESIAN_POINT ( 'NONE',  ( -13.38461538461550582, -12.27809138561165270, 31.22303859784587132 ) ) ;
#13387=CYLINDRICAL_SURFACE ( 'NONE', #35124, 0.2500000000000009437 ) ;
#13388=CARTESIAN_POINT ( 'NONE',  ( 5.207714884747862705, -5.582136614379148654, 34.36778462344220486 ) ) ;
#13389=EDGE_LOOP ( 'NONE', ( #42349, #73873 ) ) ;
#13390=ORIENTED_EDGE ( 'NONE', *, *, #69998, .F. ) ;
#13391=EDGE_CURVE ( 'NONE', #36002, #67813, #88337, .T. ) ;
#13392=VERTEX_POINT ( 'NONE', #63651 ) ;
#13393=CARTESIAN_POINT ( 'NONE',  ( -7.173100147298381302, -8.475808217655753651, 34.90892951860618609 ) ) ;
#13395=CARTESIAN_POINT ( 'NONE',  ( -1.634592128663975741, -2.920706130388546651, 32.31842814019191223 ) ) ;
#13396=CARTESIAN_POINT ( 'NONE',  ( -10.74599497500914325, -7.722926236386453702, 34.74524107206102030 ) ) ;
#13397=EDGE_CURVE ( 'NONE', #64660, #14886, #58216, .T. ) ;
#13399=CARTESIAN_POINT ( 'NONE',  ( 7.053602361310566948, -5.070358843744210198, 34.40418822224088302 ) ) ;
#13400=LINE ( 'NONE', #41322, #30939 ) ;
#13401=EDGE_CURVE ( 'NONE', #87539, #86167, #78054, .T. ) ;
#13402=ORIENTED_EDGE ( 'NONE', *, *, #29009, .F. ) ;
#13403=AXIS2_PLACEMENT_3D ( 'NONE', #50907, #9078, #63560 ) ;
#13404=ORIENTED_EDGE ( 'NONE', *, *, #68033, .T. ) ;
#13406=CARTESIAN_POINT ( 'NONE',  ( -8.769230769230768274, -11.91647553114624181, 32.58852847137148245 ) ) ;
#13408=ORIENTED_EDGE ( 'NONE', *, *, #7732, .T. ) ;
#13409=CARTESIAN_POINT ( 'NONE',  ( 9.626224281351811740, -11.69971097300155272, 32.46337939537587403 ) ) ;
#13410=B_SPLINE_CURVE_WITH_KNOTS ( 'NONE', 3,
 ( #11584, #54328, #39953, #60201, #53894, #18336, #80943, #39066, #66063, #52991 ),
 .UNSPECIFIED., .F., .F.,
 ( 4, 2, 2, 2, 4 ),
 ( 0.000000000000000000, 0.0001954339857564098054, 0.0003908679715128196108, 0.0005863019572692293891, 0.0007817359430256392216 ),
 .UNSPECIFIED. ) ;
#13412=EDGE_CURVE ( 'NONE', #14506, #85420, #40932, .T. ) ;
#13413=ORIENTED_EDGE ( 'NONE', *, *, #29791, .T. ) ;
#13414=CARTESIAN_POINT ( 'NONE',  ( -4.023320452082589149, -5.195472089885680766, 34.18748526763464923 ) ) ;
#13415=DIRECTION ( 'NONE',  ( 0.000000000000000000, -6.938893903907222067E-15, 1.000000000000000000 ) ) ;
#13416=B_SPLINE_CURVE_WITH_KNOTS ( 'NONE', 3,
 ( #21309, #14559, #1047, #1932, #15900, #7806, #83476, #50548, #64492, #70844 ),
 .UNSPECIFIED., .F., .F.,
 ( 4, 2, 2, 2, 4 ),
 ( 0.000000000000000000, 0.0001954339857564054144, 0.0003908679715128108288, 0.0005863019572692162703, 0.0007817359430256216575 ),
 .UNSPECIFIED. ) ;
#13417=FACE_BOUND ( 'NONE', #37156, .T. ) ;
#13418=CARTESIAN_POINT ( 'NONE',  ( -0.5916856709766825650, -10.19110544564092002, 33.96427741523702792 ) ) ;
#13420=CARTESIAN_POINT ( 'NONE',  ( 12.39626846098214230, -6.835583212224499938, 34.95778746994557906 ) ) ;
#13421=CARTESIAN_POINT ( 'NONE',  ( -17.77440776823446100, -12.74866226681162296, 29.87809195722894628 ) ) ;
#13423=EDGE_CURVE ( 'NONE', #2558, #7803, #64520, .T. ) ;
#13424=CYLINDRICAL_SURFACE ( 'NONE', #71108, 0.2500000000000004996 ) ;
#13425=CARTESIAN_POINT ( 'NONE',  ( -0.4615384615385826339, -3.835265460704628371, 33.15142922262033665 ) ) ;
#13427=EDGE_CURVE ( 'NONE', #64802, #80981, #51748, .T. ) ;
#13428=CARTESIAN_POINT ( 'NONE',  ( -2.437840277424002444, -4.299443229763728169, 33.91186481527756058 ) ) ;
#13431=VECTOR ( 'NONE', #12776, 1000.000000000000227 ) ;
#13432=AXIS2_PLACEMENT_3D ( 'NONE', #40766, #48391, #55592 ) ;
#13433=CARTESIAN_POINT ( 'NONE',  ( -14.55766903863466055, -4.943428324936578910, 34.04746400365624481 ) ) ;
#13434=CARTESIAN_POINT ( 'NONE',  ( -4.153846153846274980, -3.643525952248796163, 33.31231777344771672 ) ) ;
#13435=ORIENTED_EDGE ( 'NONE', *, *, #69105, .F. ) ;
#13436=DIRECTION ( 'NONE',  ( -0.000000000000000000, 0.9848077530122086864, -0.1736481776669273891 ) ) ;
#13437=CARTESIAN_POINT ( 'NONE',  ( -15.09997878980228059, -12.62708834333097663, 30.88030960425257021 ) ) ;
#13438=FACE_BOUND ( 'NONE', #2747, .T. ) ;
#13439=CARTESIAN_POINT ( 'NONE',  ( -15.45369544828538011, -5.667676309546437530, 34.40238873228292249 ) ) ;
#13440=CARTESIAN_POINT ( 'NONE',  ( -16.85414353565466428, -12.44528174975671853, 30.48912976160715615 ) ) ;
#13441=CARTESIAN_POINT ( 'NONE',  ( -13.45069776397551742, -2.292212530054419606, 30.41441678777542634 ) ) ;
#13443=CARTESIAN_POINT ( 'NONE',  ( -8.703975197954742171, -12.27809138561124591, 31.22303859784720359 ) ) ;
#13445=ORIENTED_EDGE ( 'NONE', *, *, #74326, .F. ) ;
#13447=CARTESIAN_POINT ( 'NONE',  ( -5.076923076923075762, -13.04860791097971706, 34.73218667398347037 ) ) ;
#13449=DIRECTION ( 'NONE',  ( -0.000000000000000000, -0.9848077530122085754, -0.1736481776669273613 ) ) ;
#13450=DIRECTION ( 'NONE',  ( 0.000000000000000000, 0.7660444431189807890, 0.6427876096865361433 ) ) ;
#13451=CARTESIAN_POINT ( 'NONE',  ( -7.846153846153530509, -2.255955759149395501, 30.00000000000324363 ) ) ;
#13453=CARTESIAN_POINT ( 'NONE',  ( -7.780898274877820597, -8.613356846314928816, 34.62446782046653482 ) ) ;
#13454=CARTESIAN_POINT ( 'NONE',  ( -6.250023224221455287, -8.475808217655753651, 34.90892951860618609 ) ) ;
#13455=CARTESIAN_POINT ( 'NONE',  ( -4.826868657009623753, -2.318338780012835443, 30.59689888758630261 ) ) ;
#13456=CARTESIAN_POINT ( 'NONE',  ( 10.83816428436267820, -3.563462043263030399, 33.22394488606062879 ) ) ;
#13457=CARTESIAN_POINT ( 'NONE',  ( -4.946397638689432164, -6.808710257144159783, 34.95449254468098843 ) ) ;
#13458=B_SPLINE_CURVE_WITH_KNOTS ( 'NONE', 3,
 ( #45837, #30983, #66103, #31895, #39102, #59800, #87298, #25575, #12076, #39553 ),
 .UNSPECIFIED., .F., .F.,
 ( 4, 2, 2, 2, 4 ),
 ( 0.000000000000000000, 0.0001954339857564092362, 0.0003908679715128184724, 0.0005863019572692276544, 0.0007817359430256369448 ),
 .UNSPECIFIED. ) ;
#13459=DIRECTION ( 'NONE',  ( -0.000000000000000000, 0.9396926207859093161, -0.3420201433256663259 ) ) ;
#13460=B_SPLINE_CURVE_WITH_KNOTS ( 'NONE', 3,
 ( #63250, #1555, #8765, #29042, #56499, #70903, #9209, #36234, #50618, #36672 ),
 .UNSPECIFIED., .F., .F.,
 ( 4, 2, 2, 2, 4 ),
 ( 0.000000000000000000, 0.0001954311564186880670, 0.0003908623128373761341, 0.0005862934692560642282, 0.0007817246256747522682 ),
 .UNSPECIFIED. ) ;
#13461=CARTESIAN_POINT ( 'NONE',  ( 17.32692307692307665, -2.249999999999998668, 29.75000000000000355 ) ) ;
#13462=EDGE_CURVE ( 'NONE', #19422, #27220, #66774, .T. ) ;
#13463=VECTOR ( 'NONE', #75430, 1000.000000000000114 ) ;
#13464=CARTESIAN_POINT ( 'NONE',  ( -3.453695448285377445, -8.239355502252617924, 34.69524867566427417 ) ) ;
#13465=CARTESIAN_POINT ( 'NONE',  ( 6.000000000000001776, -5.557115091759785130, 34.35708131394839171 ) ) ;
#13466=ORIENTED_EDGE ( 'NONE', *, *, #15508, .F. ) ;
#13467=ADVANCED_FACE ( 'NONE', ( #67656 ), #5062, .F. ) ;
#13468=CARTESIAN_POINT ( 'NONE',  ( -5.010854725920637520, -11.69971097300155272, 32.46337939537588113 ) ) ;
#13469=ADVANCED_FACE ( 'NONE', ( #73971 ), #12707, .F. ) ;
#13470=CARTESIAN_POINT ( 'NONE',  ( -3.454254174493179619, -3.754499324213721234, 33.06261337010820256 ) ) ;
#13474=CIRCLE ( 'NONE', #7694, 0.2500000000000002220 ) ;
#13475=CARTESIAN_POINT ( 'NONE',  ( -16.15384615384615330, -13.04860791097971706, 34.73218667398347037 ) ) ;
#13476=CARTESIAN_POINT ( 'NONE',  ( -17.77698864838715309, -10.61302985866384141, 33.66295027996417843 ) ) ;
#13477=CARTESIAN_POINT ( 'NONE',  ( -11.47239420511146513, -4.661471528628508665, 34.16647553114624003 ) ) ;
#13478=CARTESIAN_POINT ( 'NONE',  ( -9.626239341305252495, -4.786620604624113540, 33.94971097300155805 ) ) ;
#13479=ORIENTED_EDGE ( 'NONE', *, *, #75333, .T. ) ;
#13481=DIRECTION ( 'NONE',  ( -0.000000000000000000, 0.1736481776669307198, -0.9848077530122080203 ) ) ;
#13482=ORIENTED_EDGE ( 'NONE', *, *, #59609, .F. ) ;
#13484=ADVANCED_FACE ( 'NONE', ( #79840 ), #5957, .F. ) ;
#13485=CARTESIAN_POINT ( 'NONE',  ( 4.153846153846154188, -6.343179335718451384, 34.87096338111211935 ) ) ;
#13486=ORIENTED_EDGE ( 'NONE', *, *, #15552, .T. ) ;
#13487=CARTESIAN_POINT ( 'NONE',  ( -10.86536135943320502, -4.075325502946081535, 33.72974371597206300 ) ) ;
#13489=CARTESIAN_POINT ( 'NONE',  ( 15.29683758177167086, -2.721908614388771852, 31.22303859784725333 ) ) ;
#13490=ORIENTED_EDGE ( 'NONE', *, *, #64503, .T. ) ;
#13491=ORIENTED_EDGE ( 'NONE', *, *, #34818, .T. ) ;
#13492=CARTESIAN_POINT ( 'NONE',  ( 17.93391762063986405, -9.905515769479276145, 34.41647553114623292 ) ) ;
#13493=ORIENTED_EDGE ( 'NONE', *, *, #9556, .F. ) ;
#13494=B_SPLINE_CURVE_WITH_KNOTS ( 'NONE', 3,
 ( #69765, #31779, #65988, #10169, #4298, #10614, #29998, #37633, #65095, #3400 ),
 .UNSPECIFIED., .F., .F.,
 ( 4, 2, 2, 2, 4 ),
 ( 0.000000000000000000, 0.0001954311564186859800, 0.0003908623128373719599, 0.0005862934692560579399, 0.0007817246256747439198 ),
 .UNSPECIFIED. ) ;
#13495=CARTESIAN_POINT ( 'NONE',  ( -17.86920955903305597, -4.684288915650983043, 34.18129842949671371 ) ) ;
#13496=CARTESIAN_POINT ( 'NONE',  ( -9.442253380669374252, -9.943054286541403997, 34.11300777759954883 ) ) ;
#13497=CARTESIAN_POINT ( 'NONE',  ( -17.30040802064702987, -5.912607949931405038, 34.49155766932282319 ) ) ;
#13498=B_SPLINE_CURVE_WITH_KNOTS ( 'NONE', 3,
 ( #452, #40997, #30021, #9741, #11, #27480, #77317, #20716, #41437, #57481 ),
 .UNSPECIFIED., .F., .F.,
 ( 4, 2, 2, 2, 4 ),
 ( 0.0007817246256747506419, 0.0009771112852218957062, 0.001172497944769040771, 0.001367884604316185835, 0.001563271263863330899 ),
 .UNSPECIFIED. ) ;
#13499=CARTESIAN_POINT ( 'NONE',  ( 3.230769230769231726, -6.435427911321262684, 35.78748833219616898 ) ) ;
#13500=CARTESIAN_POINT ( 'NONE',  ( 15.00784301325308157, -6.503392248772476236, 34.64988816332204635 ) ) ;
#13502=CARTESIAN_POINT ( 'NONE',  ( 13.51514108637895006, -3.285477652293413264, 32.44071101563363158 ) ) ;
#13503=VECTOR ( 'NONE', #36038, 1000.000000000000000 ) ;
#13504=DIRECTION ( 'NONE',  ( -0.000000000000000000, -0.000000000000000000, -1.000000000000000000 ) ) ;
#13505=B_SPLINE_CURVE_WITH_KNOTS ( 'NONE', 3,
 ( #46681, #81368, #39941, #66960, #52982, #80478, #75053, #5693, #60188, #52542 ),
 .UNSPECIFIED., .F., .F.,
 ( 4, 2, 2, 2, 4 ),
 ( 0.000000000000000000, 0.0001954311564186862239, 0.0003908623128373724478, 0.0005862934692560586988, 0.0007817246256747448956 ),
 .UNSPECIFIED. ) ;
#13506=ORIENTED_EDGE ( 'NONE', *, *, #32299, .T. ) ;
#13507=ORIENTED_EDGE ( 'NONE', *, *, #48820, .T. ) ;
#13508=CYLINDRICAL_SURFACE ( 'NONE', #78931, 0.2500000000000002220 ) ;
#13509=VERTEX_POINT ( 'NONE', #53687 ) ;
#13510=CARTESIAN_POINT ( 'NONE',  ( -39.05038313613820122, -2.249999999999998668, 29.75000000000000355 ) ) ;
#13511=CARTESIAN_POINT ( 'NONE',  ( 9.692307692307572609, -5.219633306517616589, 34.19971097300220464 ) ) ;
#13512=EDGE_LOOP ( 'NONE', ( #45247, #49213 ) ) ;
#13513=CARTESIAN_POINT ( 'NONE',  ( 15.45378207486262667, -9.172514111537584114, 34.72667873470787470 ) ) ;
#13514=EDGE_LOOP ( 'NONE', ( #599, #37743, #68344, #84511 ) ) ;
#13516=ORIENTED_EDGE ( 'NONE', *, *, #36717, .F. ) ;
#13517=FACE_OUTER_BOUND ( 'NONE', #80501, .T. ) ;
#13518=VECTOR ( 'NONE', #17839, 1000.000000000000227 ) ;
#13519=EDGE_CURVE ( 'NONE', #74089, #88595, #74274, .T. ) ;
#13520=ORIENTED_EDGE ( 'NONE', *, *, #87265, .T. ) ;
#13521=EDGE_CURVE ( 'NONE', #27705, #67440, #52795, .T. ) ;
#13522=CARTESIAN_POINT ( 'NONE',  ( -4.219928533206287469, -3.937682226553329556, 33.60647404775217240 ) ) ;
#13524=FACE_BOUND ( 'NONE', #366, .T. ) ;
#13525=DIRECTION ( 'NONE',  ( -0.000000000000000000, 0.3420201433256694346, -0.9396926207859080948 ) ) ;
#13526=CARTESIAN_POINT ( 'NONE',  ( -18.25000000000000355, -7.500000000000000000, 35.00000000000000000 ) ) ;
#13529=CARTESIAN_POINT ( 'NONE',  ( 3.230769230769231726, -12.78798330534102945, 29.74999999999997868 ) ) ;
#13530=CARTESIAN_POINT ( 'NONE',  ( 1.318533005255249746, -12.34228464037088280, 31.77849191805838558 ) ) ;
#13531=CARTESIAN_POINT ( 'NONE',  ( -9.692307692307812417, -8.613356846316285953, 34.62446782046622218 ) ) ;
#13533=EDGE_CURVE ( 'NONE', #52054, #57554, #47468, .T. ) ;
#13534=CARTESIAN_POINT ( 'NONE',  ( -14.08468095607945969, -3.587049720035815348, 32.86302985866382897 ) ) ;
#13535=ORIENTED_EDGE ( 'NONE', *, *, #81115, .F. ) ;
#13536=EDGE_LOOP ( 'NONE', ( #29023, #28902, #26791, #68341 ) ) ;
#13537=CARTESIAN_POINT ( 'NONE',  ( 2.084766090176162212, -10.61292498521070549, 33.66303323003028680 ) ) ;
#13539=EDGE_CURVE ( 'NONE', #48169, #54584, #22728, .T. ) ;
#13540=CARTESIAN_POINT ( 'NONE',  ( 7.146088274689773812, -6.503523203565942268, 34.64991518177335195 ) ) ;
#13541=CARTESIAN_POINT ( 'NONE',  ( -3.230769230769229949, -5.557115091759785130, 34.35708131394839171 ) ) ;
#13543=CARTESIAN_POINT ( 'NONE',  ( 9.692307692307695177, -13.49023893513002648, 31.06009739812518688 ) ) ;
#13544=ORIENTED_EDGE ( 'NONE', *, *, #60808, .T. ) ;
#13545=CARTESIAN_POINT ( 'NONE',  ( 17.20771488474786182, -3.062576670634119758, 32.05464942895959979 ) ) ;
#13546=CARTESIAN_POINT ( 'NONE',  ( 15.23076923076923173, -3.937682226553329556, 33.60647404775216529 ) ) ;
#13547=CARTESIAN_POINT ( 'NONE',  ( 5.999999999999880096, -12.27809138561165270, 31.22303859784587132 ) ) ;
#13548=CARTESIAN_POINT ( 'NONE',  ( -2.307692307692305711, -4.102666532097928531, 36.13435417666054406 ) ) ;
#13550=EDGE_CURVE ( 'NONE', #54586, #13301, #41069, .T. ) ;
#13551=ORIENTED_EDGE ( 'NONE', *, *, #33119, .T. ) ;
#13552=ORIENTED_EDGE ( 'NONE', *, *, #74581, .F. ) ;
#13553=CARTESIAN_POINT ( 'NONE',  ( 15.23076923076911093, -6.879047030192662504, 34.71129190930017927 ) ) ;
#13554=EDGE_CURVE ( 'NONE', #39978, #29264, #5525, .T. ) ;
#13555=VERTEX_POINT ( 'NONE', #34746 ) ;
#13556=CARTESIAN_POINT ( 'NONE',  ( 3.007284306204899504, -12.69144148231606017, 30.53333754910549303 ) ) ;
#13557=CARTESIAN_POINT ( 'NONE',  ( -9.692307692307812417, -11.94971097300221174, 32.03036669348237098 ) ) ;
#13558=CARTESIAN_POINT ( 'NONE',  ( -5.326899807865431491, -4.236021600441998380, 33.53823185664189310 ) ) ;
#13559=CARTESIAN_POINT ( 'NONE',  ( -17.07692307692307665, -9.058645607665452459, 34.76329471203371924 ) ) ;
#13560=CARTESIAN_POINT ( 'NONE',  ( 14.37376065869474751, -4.098570777380720287, 33.41473453929635440 ) ) ;
#13561=AXIS2_PLACEMENT_3D ( 'NONE', #47095, #61061, #88564 ) ;
#13562=ORIENTED_EDGE ( 'NONE', *, *, #17908, .T. ) ;
#13564=CARTESIAN_POINT ( 'NONE',  ( -16.28453762051371712, -11.71456829005830080, 32.44064028649416542 ) ) ;
#13565=ORIENTED_EDGE ( 'NONE', *, *, #10172, .F. ) ;
#13566=CARTESIAN_POINT ( 'NONE',  ( 0.4615384615383396616, -6.026961402154118908, 34.52809138561165270 ) ) ;
#13568=CARTESIAN_POINT ( 'NONE',  ( 1.319291371811078362, -7.749976730030849303, 34.74374725381503737 ) ) ;
#13569=CARTESIAN_POINT ( 'NONE',  ( -4.153846153846152411, -1.044019251281081972, 31.83374038241031911 ) ) ;
#13570=EDGE_CURVE ( 'NONE', #57920, #48838, #48256, .T. ) ;
#13571=CARTESIAN_POINT ( 'NONE',  ( -12.52762187249434156, -2.721908614388770964, 31.22303859784723912 ) ) ;
#13572=DIRECTION ( 'NONE',  ( -0.000000000000000000, -0.7660444431189791237, -0.6427876096865379196 ) ) ;
#13573=CARTESIAN_POINT ( 'NONE',  ( 12.46153846153846168, -11.16473453929635440, 33.15142922261926373 ) ) ;
#13576=EDGE_CURVE ( 'NONE', #84581, #68662, #53842, .T. ) ;
#13577=CARTESIAN_POINT ( 'NONE',  ( 14.98074599347626368, -8.432397168068783699, 34.66272746175022945 ) ) ;
#13578=DIRECTION ( 'NONE',  ( 0.000000000000000000, 0.3420201433256641055, -0.9396926207859100932 ) ) ;
#13579=CYLINDRICAL_SURFACE ( 'NONE', #5807, 0.2500000000000009437 ) ;
#13580=CARTESIAN_POINT ( 'NONE',  ( -13.13456107297706588, -8.303483539816728154, 34.68545999027711702 ) ) ;
#13581=VERTEX_POINT ( 'NONE', #7731 ) ;
#13583=CARTESIAN_POINT ( 'NONE',  ( 11.31497661389720832, -12.69144148231606017, 30.53333754910549303 ) ) ;
#13584=CARTESIAN_POINT ( 'NONE',  ( 2.557637717070352590, -10.92531984108285670, 33.72920026020278073 ) ) ;
#13585=EDGE_CURVE ( 'NONE', #28571, #2346, #82945, .T. ) ;
#13587=CARTESIAN_POINT ( 'NONE',  ( 16.15384615384615330, -3.886160181151819604, 36.00935417666054406 ) ) ;
#13588=VERTEX_POINT ( 'NONE', #55460 ) ;
#13589=B_SPLINE_CURVE_WITH_KNOTS ( 'NONE', 3,
 ( #46801, #33297, #60755, #61635, #26538, #52660, #13017, #73842, #87818, #80147 ),
 .UNSPECIFIED., .F., .F.,
 ( 4, 2, 2, 2, 4 ),
 ( 0.000000000000000000, 0.0001954311564186869557, 0.0003908623128373739115, 0.0005862934692560608672, 0.0007817246256747478229 ),
 .UNSPECIFIED. ) ;
#13590=CARTESIAN_POINT ( 'NONE',  ( -16.37733107841048508, -6.716662450894490100, 34.94144148231605840 ) ) ;
#13591=B_SPLINE_CURVE_WITH_KNOTS ( 'NONE', 3,
 ( #42326, #56269, #85076, #35108, #29691, #42766, #9410, #57150, #43631, #62571 ),
 .UNSPECIFIED., .F., .F.,
 ( 4, 2, 2, 2, 4 ),
 ( 0.0007817359430256324996, 0.0009771253907249991422, 0.001172514838424365676, 0.001367904286123732428, 0.001563293733823098962 ),
 .UNSPECIFIED. ) ;
#13592=EDGE_CURVE ( 'NONE', #65829, #2166, #69961, .T. ) ;
#13593=DIRECTION ( 'NONE',  ( -0.000000000000000000, -0.7660444431189791237, -0.6427876096865379196 ) ) ;
#13594=CARTESIAN_POINT ( 'NONE',  ( -14.53052040532718614, -7.369209533119140509, 34.99857337881830688 ) ) ;
#13595=ORIENTED_EDGE ( 'NONE', *, *, #70142, .F. ) ;
#13596=CARTESIAN_POINT ( 'NONE',  ( -5.999999999999998224, -13.04860791097971706, 34.73218667398347037 ) ) ;
#13597=VECTOR ( 'NONE', #8521, 999.9999999999998863 ) ;
#13598=B_SPLINE_CURVE_WITH_KNOTS ( 'NONE', 3,
 ( #40170, #27082, #67189, #47347, #20332, #67635, #73507, #73951, #25309, #19440 ),
 .UNSPECIFIED., .F., .F.,
 ( 4, 2, 2, 2, 4 ),
 ( 0.0007817246256747524850, 0.0009771112852218972241, 0.001172497944769042072, 0.001367884604316186702, 0.001563271263863331550 ),
 .UNSPECIFIED. ) ;
#13600=ORIENTED_EDGE ( 'NONE', *, *, #81007, .T. ) ;
#13604=CARTESIAN_POINT ( 'NONE',  ( 7.596177115211492747, -12.17611988154120972, 31.52148481390971213 ) ) ;
#13605=CARTESIAN_POINT ( 'NONE',  ( -14.37296230824862775, -2.379036618887870436, 30.90682066428147934 ) ) ;
#13606=EDGE_CURVE ( 'NONE', #37663, #71986, #86072, .T. ) ;
#13607=CARTESIAN_POINT ( 'NONE',  ( -10.61538461538461320, -5.557115091759785130, 34.35708131394839171 ) ) ;
#13608=ADVANCED_FACE ( 'NONE', ( #47369 ), #40634, .F. ) ;
#13609=CARTESIAN_POINT ( 'NONE',  ( 6.988332062589760696, -12.51329471203373700, 31.30864560766537963 ) ) ;
#13610=CARTESIAN_POINT ( 'NONE',  ( -0.4615384615384611200, -11.35647404775217417, 33.31231777344666511 ) ) ;
#13611=ORIENTED_EDGE ( 'NONE', *, *, #29112, .F. ) ;
#13612=FACE_BOUND ( 'NONE', #75017, .T. ) ;
#13613=EDGE_LOOP ( 'NONE', ( #62150, #17032, #28522, #14523 ) ) ;
#13614=CARTESIAN_POINT ( 'NONE',  ( 11.53846153846153832, -2.292212530054420494, 30.41441678777542634 ) ) ;
#13616=CARTESIAN_POINT ( 'NONE',  ( 3.165499230212911019, -11.67786785259541027, 32.92929555188721480 ) ) ;
#13619=B_SPLINE_CURVE_WITH_KNOTS ( 'NONE', 3,
 ( #52890, #59210, #65962, #32198, #31753, #85808, #66419, #12367, #87155, #39408 ),
 .UNSPECIFIED., .F., .F.,
 ( 4, 2, 2, 2, 4 ),
 ( 0.000000000000000000, 0.0001954339881912783286, 0.0003908679763825566571, 0.0005863019645738349857, 0.0007817359527651133143 ),
 .UNSPECIFIED. ) ;
#13620=VECTOR ( 'NONE', #53994, 1000.000000000000000 ) ;
#13622=EDGE_LOOP ( 'NONE', ( #26211, #46992, #78375, #45198 ) ) ;
#13623=DIRECTION ( 'NONE',  ( 0.000000000000000000, 0.6427876096865373645, -0.7660444431189797898 ) ) ;
#13624=VERTEX_POINT ( 'NONE', #64862 ) ;
#13625=CARTESIAN_POINT ( 'NONE',  ( -3.230769230769229949, -8.973038597847269315, 34.52809138561121927 ) ) ;
#13626=LINE ( 'NONE', #82097, #71249 ) ;
#13627=CARTESIAN_POINT ( 'NONE',  ( 4.853996118016225658, -11.43668979543635089, 33.22377378376089752 ) ) ;
#13628=CARTESIAN_POINT ( 'NONE',  ( 11.53846153846141753, -2.625532179533778709, 30.86335684631627174 ) ) ;
#13629=FACE_OUTER_BOUND ( 'NONE', #80211, .T. ) ;
#13630=CARTESIAN_POINT ( 'NONE',  ( -3.230769230769229949, -1.509761064869970415, 31.06009739812519044 ) ) ;
#13631=CARTESIAN_POINT ( 'NONE',  ( -7.846153846153844924, -3.050289026998446396, 32.03036669348365706 ) ) ;
#13632=CARTESIAN_POINT ( 'NONE',  ( -5.326899807865431491, -3.627789207965226748, 32.91389620160131102 ) ) ;
#13636=EDGE_LOOP ( 'NONE', ( #16690, #17624, #66023, #1755 ) ) ;
#13637=CARTESIAN_POINT ( 'NONE',  ( -11.66915300512910214, -12.38065189839062263, 30.83690757178629482 ) ) ;
#13639=CARTESIAN_POINT ( 'NONE',  ( -7.976845312821407852, -4.118384482072085184, 33.43331474514187107 ) ) ;
#13640=EDGE_CURVE ( 'NONE', #59182, #26485, #10382, .T. ) ;
#13642=CARTESIAN_POINT ( 'NONE',  ( -9.822999158975251888, -6.413092428213692742, 34.63065189839063152 ) ) ;
#13643=FACE_BOUND ( 'NONE', #85297, .T. ) ;
#13644=DIRECTION ( 'NONE',  ( -0.000000000000000000, -0.6427876096865404731, -0.7660444431189771253 ) ) ;
#13645=ORIENTED_EDGE ( 'NONE', *, *, #13702, .T. ) ;
#13649=CARTESIAN_POINT ( 'NONE',  ( 3.165498784808455923, -10.90142922261923886, 33.41473453929638993 ) ) ;
#13650=VERTEX_POINT ( 'NONE', #17128 ) ;
#13651=EDGE_CURVE ( 'NONE', #25023, #32515, #50464, .T. ) ;
#13652=CARTESIAN_POINT ( 'NONE',  ( 17.29970274590113632, -5.827830569534415694, 34.72679350104403539 ) ) ;
#13653=EDGE_LOOP ( 'NONE', ( #33878, #73585, #81815, #39014 ) ) ;
#13654=FACE_BOUND ( 'NONE', #86055, .T. ) ;
#13655=CARTESIAN_POINT ( 'NONE',  ( -4.153846153846273204, -11.48612834414049644, 32.76840700105863391 ) ) ;
#13656=B_SPLINE_CURVE_WITH_KNOTS ( 'NONE', 3,
 ( #24421, #12597, #26106, #79387, #33315, #47256, #10926, #3710, #40953, #61208 ),
 .UNSPECIFIED., .F., .F.,
 ( 4, 2, 2, 2, 4 ),
 ( 0.000000000000000000, 0.0001954339857564074473, 0.0003908679715128148945, 0.0005863019572692223418, 0.0007817359430256297891 ),
 .UNSPECIFIED. ) ;
#13658=DIRECTION ( 'NONE',  ( 0.000000000000000000, 0.8660254037844377084, 0.5000000000000015543 ) ) ;
#13659=ORIENTED_EDGE ( 'NONE', *, *, #39986, .T. ) ;
#13661=B_SPLINE_CURVE_WITH_KNOTS ( 'NONE', 3,
 ( #38753, #86972, #31549, #37860, #17602, #16694, #25238, #59014, #45943, #65325 ),
 .UNSPECIFIED., .F., .F.,
 ( 4, 2, 2, 2, 4 ),
 ( 0.0007817359430256261028, 0.0009771253907249911191, 0.001172514838424356136, 0.001367904286123721152, 0.001563293733823086168 ),
 .UNSPECIFIED. ) ;
#13664=CARTESIAN_POINT ( 'NONE',  ( -16.21911659980693443, -12.46129190929999986, 30.37095296980880832 ) ) ;
#13665=DIRECTION ( 'NONE',  ( 0.000000000000000000, 0.7660444431189822323, -0.6427876096865344779 ) ) ;
#13666=VERTEX_POINT ( 'NONE', #58550 ) ;
#13668=CYLINDRICAL_SURFACE ( 'NONE', #51680, 0.2499999999999994726 ) ;
#13669=CARTESIAN_POINT ( 'NONE',  ( -15.23076923076935074, -4.481592998941358097, 33.73612834414048933 ) ) ;
#13670=CARTESIAN_POINT ( 'NONE',  ( 16.15384615384615330, -3.513871655860378418, 32.76840700105978499 ) ) ;
#13671=VERTEX_POINT ( 'NONE', #22125 ) ;
#13672=CARTESIAN_POINT ( 'NONE',  ( 16.08857615328984281, -4.320704448112772766, 33.92786785259540494 ) ) ;
#13673=CARTESIAN_POINT ( 'NONE',  ( 5.776515056276054771, -9.331801661448606566, 34.40259984581193464 ) ) ;
#13674=CARTESIAN_POINT ( 'NONE',  ( -11.76138775597768138, -8.239355502252617924, 34.69524867566427417 ) ) ;
#13675=CARTESIAN_POINT ( 'NONE',  ( -10.54931626438217585, -2.538708090699994813, 30.37095296980875503 ) ) ;
#13676=CARTESIAN_POINT ( 'NONE',  ( 16.15384615384645883, -2.506253911140615021, 30.00000000000323297 ) ) ;
#13677=LINE ( 'NONE', #41156, #24650 ) ;
#13678=CARTESIAN_POINT ( 'NONE',  ( -16.40386937806761125, -8.475808217655753651, 34.90892951860618609 ) ) ;
#13679=DIRECTION ( 'NONE',  ( -0.000000000000000000, 0.8660254037844399289, -0.4999999999999980016 ) ) ;
#13681=ORIENTED_EDGE ( 'NONE', *, *, #43828, .T. ) ;
#13682=EDGE_CURVE ( 'NONE', #12459, #31749, #37850, .T. ) ;
#13683=LINE ( 'NONE', #34836, #83613 ) ;
#13684=EDGE_LOOP ( 'NONE', ( #76119, #29988, #14149, #17158 ) ) ;
#13687=CARTESIAN_POINT ( 'NONE',  ( -18.25000000000000000, -12.75000000000000888, 29.74999999999997868 ) ) ;
#13688=ORIENTED_EDGE ( 'NONE', *, *, #41493, .F. ) ;
#13689=CARTESIAN_POINT ( 'NONE',  ( 14.30769230769231015, -8.120952969808772792, 34.71129190930000163 ) ) ;
#13691=CARTESIAN_POINT ( 'NONE',  ( 17.99999999999987566, -5.094484230521993062, 34.41647553114689373 ) ) ;
#13693=CARTESIAN_POINT ( 'NONE',  ( -16.15384615384615330, -5.557115091759785130, 34.35708131394839171 ) ) ;
#13695=DIRECTION ( 'NONE',  ( 0.000000000000000000, 0.6427876096865373645, -0.7660444431189797898 ) ) ;
#13696=CYLINDRICAL_SURFACE ( 'NONE', #22925, 0.2500000000000012212 ) ;
#13697=CARTESIAN_POINT ( 'NONE',  ( 2.177545098254087375, -10.19110544564092002, 33.96427741523702792 ) ) ;
#13699=CARTESIAN_POINT ( 'NONE',  ( 6.700149964170072359, -10.01117774369187252, 34.36070679894347535 ) ) ;
#13700=DIRECTION ( 'NONE',  ( 0.000000000000000000, 0.9396926207859126468, -0.3420201433256571111 ) ) ;
#13701=B_SPLINE_CURVE_WITH_KNOTS ( 'NONE', 3,
 ( #41644, #14168, #27237, #88967, #20038, #13282, #19595, #5638, #75428, #88094 ),
 .UNSPECIFIED., .F., .F.,
 ( 4, 2, 2, 2, 4 ),
 ( 0.000000000000000000, 0.0001954339857564075828, 0.0003908679715128151656, 0.0005863019572692227755, 0.0007817359430256303312 ),
 .UNSPECIFIED. ) ;
#13702=EDGE_CURVE ( 'NONE', #530, #72319, #6631, .T. ) ;
#13703=B_SPLINE_CURVE_WITH_KNOTS ( 'NONE', 3,
 ( #33426, #67211, #68100, #12705, #81174, #60887, #88386, #14029, #20357, #19458 ),
 .UNSPECIFIED., .F., .F.,
 ( 4, 2, 2, 2, 4 ),
 ( 0.0007817246256747514008, 0.0009771112852218961399, 0.001172497944769040771, 0.001367884604316185401, 0.001563271263863330032 ),
 .UNSPECIFIED. ) ;
#13704=CARTESIAN_POINT ( 'NONE',  ( 5.326977496836529546, -10.82426656108011720, 33.81400080652039009 ) ) ;
#13706=VERTEX_POINT ( 'NONE', #44587 ) ;
#13707=CARTESIAN_POINT ( 'NONE',  ( 12.46153846153846168, -2.486705287966279876, 31.30864560766543647 ) ) ;
#13708=CARTESIAN_POINT ( 'NONE',  ( 0.6843181305165253470, -12.11081565061823717, 32.26097654155341843 ) ) ;
#13709=DIRECTION ( 'NONE',  ( 0.000000000000000000, 0.7660444431189807890, 0.6427876096865361433 ) ) ;
#13710=CARTESIAN_POINT ( 'NONE',  ( 5.934729554039225974, -6.026961402152685388, 34.52809138561120506 ) ) ;
#13712=EDGE_CURVE ( 'NONE', #33744, #34857, #8717, .T. ) ;
#13716=EDGE_CURVE ( 'NONE', #62266, #83312, #23005, .T. ) ;
#13717=AXIS2_PLACEMENT_3D ( 'NONE', #77901, #72027, #85114 ) ;
#13718=ORIENTED_EDGE ( 'NONE', *, *, #19717, .F. ) ;
#13719=DIRECTION ( 'NONE',  ( -0.000000000000000000, 0.8660254037844397068, -0.4999999999999978906 ) ) ;
#13720=EDGE_LOOP ( 'NONE', ( #29034, #51704 ) ) ;
#13721=EDGE_CURVE ( 'NONE', #60694, #683, #14135, .T. ) ;
#13722=ADVANCED_FACE ( 'NONE', ( #53580 ), #79287, .F. ) ;
#13723=B_SPLINE_CURVE_WITH_KNOTS ( 'NONE', 3,
 ( #71799, #51505, #17308, #44765, #65491, #31267, #58732, #86231, #24499, #51967 ),
 .UNSPECIFIED., .F., .F.,
 ( 4, 2, 2, 2, 4 ),
 ( 0.000000000000000000, 0.0001954339857564073659, 0.0003908679715128147319, 0.0005863019572692221250, 0.0007817359430256294638 ),
 .UNSPECIFIED. ) ;
#13724=CARTESIAN_POINT ( 'NONE',  ( -14.43816901580877143, -7.276988635370452485, 34.74523720219453793 ) ) ;
#13725=B_SPLINE_CURVE_WITH_KNOTS ( 'NONE', 3,
 ( #43222, #65252, #30149, #50404, #9001, #79228, #3554, #71566, #77887, #58942 ),
 .UNSPECIFIED., .F., .F.,
 ( 4, 2, 2, 2, 4 ),
 ( 0.000000000000000000, 0.0001954339857564054144, 0.0003908679715128108288, 0.0005863019572692162703, 0.0007817359430256216575 ),
 .UNSPECIFIED. ) ;
#13726=CARTESIAN_POINT ( 'NONE',  ( 4.088092725532820992, -7.249945578846651806, 34.99404164642496795 ) ) ;
#13728=FACE_OUTER_BOUND ( 'NONE', #35569, .T. ) ;
#13729=CARTESIAN_POINT ( 'NONE',  ( 17.99999999999987566, -3.083524468854526912, 32.58852847137268327 ) ) ;
#13730=VERTEX_POINT ( 'NONE', #38742 ) ;
#13731=ORIENTED_EDGE ( 'NONE', *, *, #80505, .T. ) ;
#13732=ORIENTED_EDGE ( 'NONE', *, *, #22754, .T. ) ;
#13733=ORIENTED_EDGE ( 'NONE', *, *, #78326, .T. ) ;
#13734=DIRECTION ( 'NONE',  ( 0.000000000000000000, 0.4999999999999960032, -0.8660254037844410391 ) ) ;
#13735=CARTESIAN_POINT ( 'NONE',  ( 7.622668902429896143, -3.754499324213721234, 33.06261337010820256 ) ) ;
#13737=CARTESIAN_POINT ( 'NONE',  ( 16.37662569511456212, -10.11255958852955672, 34.01340905677048454 ) ) ;
#13738=CARTESIAN_POINT ( 'NONE',  ( -17.01085472592063752, -3.050289026998446840, 32.03036669348366416 ) ) ;
#13739=CARTESIAN_POINT ( 'NONE',  ( 12.21156171748986985, -2.920706130388546651, 32.31842814019191223 ) ) ;
#13740=ORIENTED_EDGE ( 'NONE', *, *, #13894, .F. ) ;
#13741=ORIENTED_EDGE ( 'NONE', *, *, #18584, .F. ) ;
#13742=AXIS2_PLACEMENT_3D ( 'NONE', #55661, #61094, #47580 ) ;
#13743=ORIENTED_EDGE ( 'NONE', *, *, #46376, .T. ) ;
#13744=CARTESIAN_POINT ( 'NONE',  ( -3.453696189676078276, -2.523278758544489353, 31.42238647778637528 ) ) ;
#13745=ORIENTED_EDGE ( 'NONE', *, *, #77768, .T. ) ;
#13746=DIRECTION ( 'NONE',  ( -0.000000000000000000, 0.9848077530122086864, -0.1736481776669273891 ) ) ;
#13747=CARTESIAN_POINT ( 'NONE',  ( -4.854143535654667829, -11.41317474335729187, 32.86274602512330034 ) ) ;
#13749=VERTEX_POINT ( 'NONE', #51783 ) ;
#13750=CARTESIAN_POINT ( 'NONE',  ( -14.98076923076922995, -2.249999999999998668, 29.75000000000000355 ) ) ;
#13751=EDGE_LOOP ( 'NONE', ( #67052, #7780 ) ) ;
#13753=FACE_BOUND ( 'NONE', #59476, .T. ) ;
#13754=CARTESIAN_POINT ( 'NONE',  ( 6.923076923076924238, -4.098570777380720287, 33.41473453929634729 ) ) ;
#13756=ORIENTED_EDGE ( 'NONE', *, *, #34973, .F. ) ;
#13757=CARTESIAN_POINT ( 'NONE',  ( -9.758390071667825794, -4.661471528628507777, 34.16647553114621871 ) ) ;
#13758=CARTESIAN_POINT ( 'NONE',  ( 6.673100179028334189, -12.01397095200673881, 32.43157075238190146 ) ) ;
#13760=CARTESIAN_POINT ( 'NONE',  ( 14.08476534878545827, -9.172386477786396597, 34.72672124145550043 ) ) ;
#13761=VERTEX_POINT ( 'NONE', #39648 ) ;
#13762=B_SPLINE_CURVE_WITH_KNOTS ( 'NONE', 3,
 ( #61288, #83361, #14451, #48225, #82917, #68945, #62188, #6378, #76142, #47791 ),
 .UNSPECIFIED., .F., .F.,
 ( 4, 2, 2, 2, 4 ),
 ( 0.0007817359430256297891, 0.0009771253907249958896, 0.001172514838424361990, 0.001367904286123728091, 0.001563293733823094191 ),
 .UNSPECIFIED. ) ;
#13763=CARTESIAN_POINT ( 'NONE',  ( 11.78840705680968171, -3.202959910592335646, 32.30730279482227019 ) ) ;
#13764=CARTESIAN_POINT ( 'NONE',  ( 1.634669696253701732, -8.303483539816728154, 34.68545999027711702 ) ) ;
#13765=CARTESIAN_POINT ( 'NONE',  ( 4.376858997939548246, -11.43677907613344757, 33.22367315496201456 ) ) ;
#13766=CARTESIAN_POINT ( 'NONE',  ( -2.084912638714238931, -9.418065098278011860, 34.63729479722530158 ) ) ;
#13767=CARTESIAN_POINT ( 'NONE',  ( 8.096153846153846700, -2.249999999999998668, 29.75000000000000355 ) ) ;
#13769=FACE_BOUND ( 'NONE', #22628, .T. ) ;
#13770=CARTESIAN_POINT ( 'NONE',  ( 5.749976775778542937, -4.931416488878822335, 34.32920672191015399 ) ) ;
#13771=CYLINDRICAL_SURFACE ( 'NONE', #64693, 0.2499999999999994726 ) ;
#13772=CARTESIAN_POINT ( 'NONE',  ( -14.43784027742400156, -3.625366637846544116, 33.29286588640298561 ) ) ;
#13773=CARTESIAN_POINT ( 'NONE',  ( 3.360816837024914960, -7.723484964179500700, 34.74522123443823318 ) ) ;
#13774=CARTESIAN_POINT ( 'NONE',  ( -2.057637887778852814, -8.346898887586323923, 34.93166121998716278 ) ) ;
#13775=DIRECTION ( 'NONE',  ( 0.000000000000000000, 0.1736481776669275834, 0.9848077530122086864 ) ) ;
#13777=ORIENTED_EDGE ( 'NONE', *, *, #54258, .F. ) ;
#13778=CARTESIAN_POINT ( 'NONE',  ( 12.46153846153833911, -2.625532179533778709, 30.86335684631627174 ) ) ;
#13779=VERTEX_POINT ( 'NONE', #10827 ) ;
#13780=EDGE_CURVE ( 'NONE', #3936, #67310, #59262, .T. ) ;
#13781=CARTESIAN_POINT ( 'NONE',  ( -13.25408994638174320, -9.503571793651731880, 34.60286762892837942 ) ) ;
#13782=ORIENTED_EDGE ( 'NONE', *, *, #52361, .F. ) ;
#13783=CARTESIAN_POINT ( 'NONE',  ( 18.00000000000000000, -12.10708131394839349, 31.69288490824020244 ) ) ;
#13784=CARTESIAN_POINT ( 'NONE',  ( -16.08777882049607655, -11.91647553114624358, 32.58852847137148245 ) ) ;
#13785=B_SPLINE_CURVE_WITH_KNOTS ( 'NONE', 3,
 ( #77018, #21620, #27942, #28838, #15762, #14880, #54970, #56299, #83784, #43226 ),
 .UNSPECIFIED., .F., .F.,
 ( 4, 2, 2, 2, 4 ),
 ( 0.0007817359430256365111, 0.0009771253907250045632, 0.001172514838424372615, 0.001367904286123740668, 0.001563293733823108720 ),
 .UNSPECIFIED. ) ;
#13786=DIRECTION ( 'NONE',  ( -0.000000000000000000, -0.8660254037844397068, -0.4999999999999978906 ) ) ;
#13787=VECTOR ( 'NONE', #72892, 1000.000000000000114 ) ;
#13789=CARTESIAN_POINT ( 'NONE',  ( -15.48079246806219267, -5.056417327199099532, 34.11270091957321426 ) ) ;
#13791=CARTESIAN_POINT ( 'NONE',  ( 3.930919936330004472, -9.086856451489516928, 34.49173150075333183 ) ) ;
#13792=CARTESIAN_POINT ( 'NONE',  ( -14.05769230769230660, -2.499999999999998668, 29.75000000000000355 ) ) ;
#13793=B_SPLINE_CURVE_WITH_KNOTS ( 'NONE', 3,
 ( #84524, #55703, #29142, #56598, #76430, #84088, #22365, #57030, #49830, #15616 ),
 .UNSPECIFIED., .F., .F.,
 ( 4, 2, 2, 2, 4 ),
 ( 0.0007817246256747518345, 0.0009771112852218970073, 0.001172497944769042072, 0.001367884604316187136, 0.001563271263863332200 ),
 .UNSPECIFIED. ) ;
#13794=DIRECTION ( 'NONE',  ( -0.000000000000000000, 0.7660444431189791237, -0.6427876096865379196 ) ) ;
#13795=CARTESIAN_POINT ( 'NONE',  ( 3.930361210122205406, -11.89387501736622710, 32.13663884655806413 ) ) ;
#13796=CARTESIAN_POINT ( 'NONE',  ( 2.557637826040450424, -2.824170634883621744, 31.52227843825338738 ) ) ;
#13797=DIRECTION ( 'NONE',  ( 0.000000000000000000, 0.4999999999999960032, -0.8660254037844410391 ) ) ;
#13798=B_SPLINE_CURVE_WITH_KNOTS ( 'NONE', 3,
 ( #73961, #19011, #47810, #19451, #75290, #13580, #82501, #41501, #7273, #46482 ),
 .UNSPECIFIED., .F., .F.,
 ( 4, 2, 2, 2, 4 ),
 ( 0.0007817359430256315238, 0.0009771253907249980580, 0.001172514838424364592, 0.001367904286123730910, 0.001563293733823097444 ),
 .UNSPECIFIED. ) ;
#13800=CARTESIAN_POINT ( 'NONE',  ( -18.22348492456433178, -11.60425143139329940, 33.02411095842164457 ) ) ;
#13801=CARTESIAN_POINT ( 'NONE',  ( 10.61538461538461675, -11.16473453929635440, 33.15142922261926373 ) ) ;
#13802=ADVANCED_FACE ( 'NONE', ( #38299 ), #24777, .F. ) ;
#13804=CARTESIAN_POINT ( 'NONE',  ( 8.899756470994329760, -10.19071101563364756, 33.96452234770658407 ) ) ;
#13806=CARTESIAN_POINT ( 'NONE',  ( 2.307692307692186251, -5.094484230521993062, 34.41647553114689373 ) ) ;
#13807=CARTESIAN_POINT ( 'NONE',  ( -8.769230769230892619, -11.67786785259630911, 32.92929555188603530 ) ) ;
#13808=ORIENTED_EDGE ( 'NONE', *, *, #64688, .T. ) ;
#13809=VECTOR ( 'NONE', #30184, 1000.000000000000000 ) ;
#13811=CARTESIAN_POINT ( 'NONE',  ( -0.2385271099256117411, -9.886259254753566594, 34.14407573483973124 ) ) ;
#13812=CARTESIAN_POINT ( 'NONE',  ( 3.930919194939303196, -9.172386477786396597, 34.72672124145550043 ) ) ;
#13813=VERTEX_POINT ( 'NONE', #18033 ) ;
#13814=CARTESIAN_POINT ( 'NONE',  ( -7.596153846152408740, -7.500000000000155431, 34.75000000000007105 ) ) ;
#13815=CARTESIAN_POINT ( 'NONE',  ( -16.85395994265639885, -7.369474539155830506, 34.99858011523957657 ) ) ;
#13816=AXIS2_PLACEMENT_3D ( 'NONE', #47147, #20568, #12928 ) ;
#13817=CARTESIAN_POINT ( 'NONE',  ( 0.4615384615384611200, -1.242168528481310874, 33.36296068462461051 ) ) ;
#13818=CARTESIAN_POINT ( 'NONE',  ( 3.100621261037531440, -2.647304123082328875, 31.75400227202885262 ) ) ;
#13819=CARTESIAN_POINT ( 'NONE',  ( 6.856993512121044354, -4.786620604624113540, 33.94971097300155805 ) ) ;
#13821=EDGE_CURVE ( 'NONE', #42909, #64027, #65754, .T. ) ;
#13822=EDGE_LOOP ( 'NONE', ( #64736, #14150 ) ) ;
#13823=EDGE_LOOP ( 'NONE', ( #43885, #45123, #86981, #59265 ) ) ;
#13824=B_SPLINE_CURVE_WITH_KNOTS ( 'NONE', 3,
 ( #23702, #58371, #31363, #11092, #79101, #39024, #4332, #86778, #17408, #25048 ),
 .UNSPECIFIED., .F., .F.,
 ( 4, 2, 2, 2, 4 ),
 ( 0.000000000000000000, 0.0001954339857564083417, 0.0003908679715128166835, 0.0005863019572692250523, 0.0007817359430256333669 ),
 .UNSPECIFIED. ) ;
#13825=ORIENTED_EDGE ( 'NONE', *, *, #80658, .F. ) ;
#13826=ADVANCED_FACE ( 'NONE', ( #66659 ), #45489, .F. ) ;
#13828=CARTESIAN_POINT ( 'NONE',  ( -2.176900499867519212, -5.582136614379148654, 34.36778462344220486 ) ) ;
#13829=DIRECTION ( 'NONE',  ( -0.000000000000000000, 1.000000000000000000, 3.491481338843133355E-15 ) ) ;
#13830=CARTESIAN_POINT ( 'NONE',  ( -8.069080805060693251, -10.77366814457252175, 33.85459836347579454 ) ) ;
#13831=CARTESIAN_POINT ( 'NONE',  ( 16.08857570788537572, -5.219633306516282545, 34.19971097300152252 ) ) ;
#13832=ORIENTED_EDGE ( 'NONE', *, *, #26692, .F. ) ;
#13833=VECTOR ( 'NONE', #51868, 1000.000000000000114 ) ;
#13834=ORIENTED_EDGE ( 'NONE', *, *, #10905, .F. ) ;
#13835=ORIENTED_EDGE ( 'NONE', *, *, #38226, .T. ) ;
#13836=CARTESIAN_POINT ( 'NONE',  ( -21.00000000000000355, -12.75000000000000178, 27.25000000000000000 ) ) ;
#13837=EDGE_LOOP ( 'NONE', ( #35288, #73676 ) ) ;
#13839=B_SPLINE_CURVE_WITH_KNOTS ( 'NONE', 3,
 ( #51117, #16914, #50686, #22342, #77283, #43502, #15591, #15149, #57450, #35865 ),
 .UNSPECIFIED., .F., .F.,
 ( 4, 2, 2, 2, 4 ),
 ( 0.0007817359430256314154, 0.0009771253907249978412, 0.001172514838424364375, 0.001367904286123730693, 0.001563293733823097227 ),
 .UNSPECIFIED. ) ;
#13840=CARTESIAN_POINT ( 'NONE',  ( -3.296851610129365895, -11.91647553114624181, 32.58852847137148245 ) ) ;
#13842=LINE ( 'NONE', #74224, #2149 ) ;
#13844=ORIENTED_EDGE ( 'NONE', *, *, #15956, .F. ) ;
#13845=VERTEX_POINT ( 'NONE', #72970 ) ;
#13846=CARTESIAN_POINT ( 'NONE',  ( -13.38461538461538325, -3.937682226553329556, 33.60647404775216529 ) ) ;
#13847=CARTESIAN_POINT ( 'NONE',  ( -10.55012947587177763, -2.657715359629131857, 31.77849191805844242 ) ) ;
#13848=EDGE_LOOP ( 'NONE', ( #15522, #46621 ) ) ;
#13849=DIRECTION ( 'NONE',  ( -0.000000000000000000, -0.1736481776669307198, -0.9848077530122080203 ) ) ;
#13850=CARTESIAN_POINT ( 'NONE',  ( -2.307692307692305711, -2.517432740324522911, 35.29906147534542527 ) ) ;
#13851=EDGE_LOOP ( 'NONE', ( #47724, #69389 ) ) ;
#13852=B_SPLINE_CURVE_WITH_KNOTS ( 'NONE', 3,
 ( #13238, #67296, #161, #40719, #82595, #67738, #48339, #25863, #53321, #33061 ),
 .UNSPECIFIED., .F., .F.,
 ( 4, 2, 2, 2, 4 ),
 ( 0.0007817359430256319575, 0.0009771253907249984917, 0.001172514838424365026, 0.001367904286123731343, 0.001563293733823097878 ),
 .UNSPECIFIED. ) ;
#13853=B_SPLINE_CURVE_WITH_KNOTS ( 'NONE', 3,
 ( #42590, #48891, #21865, #76819, #8360, #62830, #1151, #15559, #35833, #64165 ),
 .UNSPECIFIED., .F., .F.,
 ( 4, 2, 2, 2, 4 ),
 ( 0.000000000000000000, 0.0001954311564186868473, 0.0003908623128373736946, 0.0005862934692560605419, 0.0007817246256747473893 ),
 .UNSPECIFIED. ) ;
#13854=CARTESIAN_POINT ( 'NONE',  ( 9.019176287578909879, -12.43552623307873972, 30.55307653245132826 ) ) ;
#13856=ORIENTED_EDGE ( 'NONE', *, *, #70714, .T. ) ;
#13857=FACE_BOUND ( 'NONE', #65122, .T. ) ;
#13858=CARTESIAN_POINT ( 'NONE',  ( 10.83839596699746721, -9.886259254753566594, 34.14407573483972413 ) ) ;
#13859=CARTESIAN_POINT ( 'NONE',  ( 16.02315555073584008, -2.494641256782728966, 31.33461815524612959 ) ) ;
#13860=CARTESIAN_POINT ( 'NONE',  ( 3.480714749117372442, -9.272278438253398036, 34.42582936511637826 ) ) ;
#13861=CARTESIAN_POINT ( 'NONE',  ( 18.06525513951284267, -3.083524468853783951, 32.58852847137153930 ) ) ;
#13862=CARTESIAN_POINT ( 'NONE',  ( 18.13079180782478872, -4.118422570099827595, 33.43335022499816489 ) ) ;
#13863=AXIS2_PLACEMENT_3D ( 'NONE', #70196, #42734, #415 ) ;
#13864=CARTESIAN_POINT ( 'NONE',  ( -4.153846153846273204, -2.625532179533778709, 30.86335684631627174 ) ) ;
#13865=CARTESIAN_POINT ( 'NONE',  ( -4.023055712879200385, -11.37503395064541678, 33.29242100308974983 ) ) ;
#13866=ORIENTED_EDGE ( 'NONE', *, *, #72574, .T. ) ;
#13867=CARTESIAN_POINT ( 'NONE',  ( -18.25002323729296450, -10.76384336483936011, 33.53834819971076087 ) ) ;
#13870=ADVANCED_FACE ( 'NONE', ( #67552 ), #4512, .F. ) ;
#13871=AXIS2_PLACEMENT_3D ( 'NONE', #60454, #74418, #60897 ) ;
#13872=FACE_OUTER_BOUND ( 'NONE', #52695, .T. ) ;
#13873=CARTESIAN_POINT ( 'NONE',  ( -4.219116154402471786, -3.643525952247789412, 33.31231777344662959 ) ) ;
#13874=EDGE_LOOP ( 'NONE', ( #30779, #78990 ) ) ;
#13875=CARTESIAN_POINT ( 'NONE',  ( -15.93083480223330817, -11.24521262558773493, 33.06293181088029343 ) ) ;
#13876=CARTESIAN_POINT ( 'NONE',  ( -9.019207500173124004, -5.728515186090277211, 34.42611988154120439 ) ) ;
#13877=FACE_BOUND ( 'NONE', #53500, .T. ) ;
#13878=CARTESIAN_POINT ( 'NONE',  ( -15.36091644020745051, -6.001485441113819874, 34.52039167877662607 ) ) ;
#13879=CARTESIAN_POINT ( 'NONE',  ( -17.07692307692319744, -3.083524468854526912, 32.58852847137268327 ) ) ;
#13880=CARTESIAN_POINT ( 'NONE',  ( 2.307692307692186251, -6.835583212225970762, 34.95778746994575670 ) ) ;
#13881=AXIS2_PLACEMENT_3D ( 'NONE', #88057, #86261, #58764 ) ;
#13882=CARTESIAN_POINT ( 'NONE',  ( -5.076923076922761346, -2.255955759149395501, 30.00000000000324363 ) ) ;
#13884=CARTESIAN_POINT ( 'NONE',  ( -8.546451227962361230, -12.24180327182772388, 31.33663988360758168 ) ) ;
#13885=CARTESIAN_POINT ( 'NONE',  ( -5.999999999999998224, -13.63283147151868846, 33.57946703557072254 ) ) ;
#13887=ORIENTED_EDGE ( 'NONE', *, *, #68228, .T. ) ;
#13888=VERTEX_POINT ( 'NONE', #25672 ) ;
#13889=EDGE_CURVE ( 'NONE', #33135, #40550, #31989, .T. ) ;
#13890=CARTESIAN_POINT ( 'NONE',  ( 5.299702618191483694, -6.760870238392817200, 34.69528174975672385 ) ) ;
#13891=CARTESIAN_POINT ( 'NONE',  ( -0.5916856709766799005, -2.882441371585227952, 31.66841991370172948 ) ) ;
#13892=DIRECTION ( 'NONE',  ( -0.000000000000000000, 0.7660444431189791237, -0.6427876096865379196 ) ) ;
#13893=CARTESIAN_POINT ( 'NONE',  ( -1.384615384615383471, -3.050289026998446396, 32.03036669348365706 ) ) ;
#13894=EDGE_CURVE ( 'NONE', #32821, #69536, #38867, .T. ) ;
#13895=CARTESIAN_POINT ( 'NONE',  ( -16.94639737515951339, -6.852161475712351013, 34.70806712695775786 ) ) ;
#13897=CARTESIAN_POINT ( 'NONE',  ( -24.00000000000000000, -5.499999999999981348, 27.75000000000000000 ) ) ;
#13898=CARTESIAN_POINT ( 'NONE',  ( 2.084826044629209729, -2.251424796025575770, 29.88072029997477586 ) ) ;
#13899=CARTESIAN_POINT ( 'NONE',  ( 9.469380733400843297, -10.77366814457252175, 33.85459836347579454 ) ) ;
#13900=CARTESIAN_POINT ( 'NONE',  ( 7.846153846153723244, -5.941354392335915335, 34.76329471203413846 ) ) ;
#13902=CARTESIAN_POINT ( 'NONE',  ( 16.21991450484859598, -4.786620604624113540, 33.94971097300155805 ) ) ;
#13903=CARTESIAN_POINT ( 'NONE',  ( -0.2114840416250090560, -4.074993327901525575, 33.72946981652012255 ) ) ;
#13904=VECTOR ( 'NONE', #19226, 1000.000000000000114 ) ;
#13905=CARTESIAN_POINT ( 'NONE',  ( -3.230769230769229949, -13.87047571288749737, 32.06866353760679544 ) ) ;
#13906=EDGE_CURVE ( 'NONE', #79258, #77968, #35674, .T. ) ;
#13907=CARTESIAN_POINT ( 'NONE',  ( -2.307692307692305711, -13.95598074871891292, 31.83374038241031911 ) ) ;
#13908=VERTEX_POINT ( 'NONE', #13049 ) ;
#13909=CARTESIAN_POINT ( 'NONE',  ( 12.21156171748987163, -4.075325502946081535, 33.72974371597206300 ) ) ;
#13910=CARTESIAN_POINT ( 'NONE',  ( 0.5920641633020234940, -2.619367082507848998, 30.83698974864644171 ) ) ;
#13912=EDGE_CURVE ( 'NONE', #38831, #45094, #74105, .T. ) ;
#13913=CARTESIAN_POINT ( 'NONE',  ( 18.00000000000000000, -10.05456864172156806, 36.03766855953608683 ) ) ;
#13914=CYLINDRICAL_SURFACE ( 'NONE', #25359, 0.2500000000000012212 ) ;
#13915=FACE_OUTER_BOUND ( 'NONE', #4592, .T. ) ;
#13916=CARTESIAN_POINT ( 'NONE',  ( 7.780070435197965040, -2.538708090699994813, 30.37095296980875148 ) ) ;
#13917=EDGE_LOOP ( 'NONE', ( #66683, #44661 ) ) ;
#13919=CARTESIAN_POINT ( 'NONE',  ( 13.38461538461538680, -12.34228464037088635, 31.77849191805839268 ) ) ;
#13921=ORIENTED_EDGE ( 'NONE', *, *, #80490, .T. ) ;
#13922=CARTESIAN_POINT ( 'NONE',  ( 11.76124120743960333, -9.418065098278013636, 34.63729479722530158 ) ) ;
#13923=CARTESIAN_POINT ( 'NONE',  ( 10.86543903529806876, -10.82426656108012075, 33.81400080652039009 ) ) ;
#13924=EDGE_LOOP ( 'NONE', ( #15978, #71675 ) ) ;
#13925=CARTESIAN_POINT ( 'NONE',  ( 14.30769230769218758, -2.625532179533778709, 30.86335684631627174 ) ) ;
#13926=CARTESIAN_POINT ( 'NONE',  ( 2.438217745925952862, -8.630441415882550871, 34.87705825610312615 ) ) ;
#13928=CYLINDRICAL_SURFACE ( 'NONE', #68631, 0.2499999999999986955 ) ;
#13930=EDGE_CURVE ( 'NONE', #10, #47709, #34199, .T. ) ;
#13931=ORIENTED_EDGE ( 'NONE', *, *, #27924, .F. ) ;
#13932=CARTESIAN_POINT ( 'NONE',  ( 15.45378058238208041, -10.61302985866384141, 33.66295027996417843 ) ) ;
#13933=VERTEX_POINT ( 'NONE', #75620 ) ;
#13934=CARTESIAN_POINT ( 'NONE',  ( -7.911423846710166075, -2.379036618887870436, 30.90682066428147934 ) ) ;
#13935=EDGE_CURVE ( 'NONE', #80357, #2602, #31180, .T. ) ;
#13936=CARTESIAN_POINT ( 'NONE',  ( 15.36129466900287532, -12.70449254468099198, 30.44128974285582956 ) ) ;
#13937=CARTESIAN_POINT ( 'NONE',  ( -17.07692307692307665, -5.557115091759785130, 34.35708131394839171 ) ) ;
#13938=EDGE_CURVE ( 'NONE', #11611, #5488, #87051, .T. ) ;
#13939=FACE_OUTER_BOUND ( 'NONE', #5567, .T. ) ;
#13940=CARTESIAN_POINT ( 'NONE',  ( 12.46153846153846168, -13.57706302396349152, 30.56769352161908060 ) ) ;
#13942=AXIS2_PLACEMENT_3D ( 'NONE', #71160, #3139, #9467 ) ;
#13943=FACE_OUTER_BOUND ( 'NONE', #73554, .T. ) ;
#13944=ORIENTED_EDGE ( 'NONE', *, *, #69513, .F. ) ;
#13945=VERTEX_POINT ( 'NONE', #33761 ) ;
#13948=CARTESIAN_POINT ( 'NONE',  ( -5.076923076923199218, -5.094484230521993062, 34.41647553114689373 ) ) ;
#13949=EDGE_LOOP ( 'NONE', ( #28584, #17270 ) ) ;
#13950=CARTESIAN_POINT ( 'NONE',  ( -8.638705330997128229, -11.04252011169590020, 33.62494198852677130 ) ) ;
#13951=FACE_OUTER_BOUND ( 'NONE', #62045, .T. ) ;
#13952=B_SPLINE_CURVE_WITH_KNOTS ( 'NONE', 3,
 ( #59120, #76857, #70537, #49382, #2505, #36747, #57458, #8843, #86173, #24441 ),
 .UNSPECIFIED., .F., .F.,
 ( 4, 2, 2, 2, 4 ),
 ( 0.000000000000000000, 0.0001954339857564054144, 0.0003908679715128108288, 0.0005863019572692162703, 0.0007817359430256216575 ),
 .UNSPECIFIED. ) ;
#13954=CARTESIAN_POINT ( 'NONE',  ( -12.33074665371367651, -5.582136614379148654, 34.36778462344220486 ) ) ;
#13955=B_SPLINE_CURVE_WITH_KNOTS ( 'NONE', 3,
 ( #4544, #52278, #81548, #12640, #87884, #79769, #40126, #18064, #18950, #5443 ),
 .UNSPECIFIED., .F., .F.,
 ( 4, 2, 2, 2, 4 ),
 ( 0.000000000000000000, 0.0001954311584214072923, 0.0003908623168428145846, 0.0005862934752642218498, 0.0007817246336856291692 ),
 .UNSPECIFIED. ) ;
#13956=EDGE_LOOP ( 'NONE', ( #89150, #50924, #49613, #9057 ) ) ;
#13961=VECTOR ( 'NONE', #24212, 1000.000000000000227 ) ;
#13963=CARTESIAN_POINT ( 'NONE',  ( -13.38461538461550582, -12.46129190930018460, 30.37095296980731973 ) ) ;
#13964=CARTESIAN_POINT ( 'NONE',  ( -4.377331078410484189, -6.716662450894490100, 34.94144148231605840 ) ) ;
#13966=FACE_BOUND ( 'NONE', #77871, .T. ) ;
#13967=DIRECTION ( 'NONE',  ( -1.000000000000000000, 0.000000000000000000, 0.000000000000000000 ) ) ;
#13968=DIRECTION ( 'NONE',  ( 0.000000000000000000, 0.7660444431189822323, -0.6427876096865344779 ) ) ;
#13969=CARTESIAN_POINT ( 'NONE',  ( 9.626225312947561008, -11.35647404775217595, 33.31231777344666511 ) ) ;
#13970=CARTESIAN_POINT ( 'NONE',  ( -3.453695448285377001, -4.186968288167446595, 33.49512374952580274 ) ) ;
#13971=CARTESIAN_POINT ( 'NONE',  ( 5.076923076923391065, -2.255955759149395501, 30.00000000000324363 ) ) ;
#13972=CARTESIAN_POINT ( 'NONE',  ( 16.08776274289027342, -4.098570777380720287, 33.41473453929634729 ) ) ;
#13974=CARTESIAN_POINT ( 'NONE',  ( 10.48469314871706004, -9.804603061927743113, 34.18744698557895845 ) ) ;
#13975=ORIENTED_EDGE ( 'NONE', *, *, #30391, .F. ) ;
#13976=EDGE_CURVE ( 'NONE', #62924, #87005, #59100, .T. ) ;
#13980=CARTESIAN_POINT ( 'NONE',  ( -3.296039231325549324, -5.941354392334500467, 34.76329471203369792 ) ) ;
#13981=CARTESIAN_POINT ( 'NONE',  ( 18.00000000000000000, -12.78798330534102945, 29.74999999999997868 ) ) ;
#13982=DIRECTION ( 'NONE',  ( -0.000000000000000000, 0.9396926207859093161, -0.3420201433256663259 ) ) ;
#13983=DIRECTION ( 'NONE',  ( -1.000000000000000000, 0.000000000000000000, 0.000000000000000000 ) ) ;
#13984=LINE ( 'NONE', #13543, #77823 ) ;
#13985=ORIENTED_EDGE ( 'NONE', *, *, #4164, .T. ) ;
#13986=CARTESIAN_POINT ( 'NONE',  ( -5.869209559033047974, -8.191423895709842640, 34.95447573519442130 ) ) ;
#13987=DIRECTION ( 'NONE',  ( 1.000000000000000000, 0.000000000000000000, 0.000000000000000000 ) ) ;
#13988=DIRECTION ( 'NONE',  ( -0.000000000000000000, 0.6427876096865404731, -0.7660444431189770143 ) ) ;
#13989=CYLINDRICAL_SURFACE ( 'NONE', #59742, 0.2499999999999973355 ) ;
#13990=VERTEX_POINT ( 'NONE', #69757 ) ;
#13991=B_SPLINE_CURVE_WITH_KNOTS ( 'NONE', 3,
 ( #62685, #7322, #21713, #28029, #42440, #49184 ),
 .UNSPECIFIED., .F., .F.,
 ( 4, 2, 4 ),
 ( 0.0003909512603273892074, 0.0005862562993132157656, 0.0007815613382990422697 ),
 .UNSPECIFIED. ) ;
#13992=VERTEX_POINT ( 'NONE', #26566 ) ;
#13993=VERTEX_POINT ( 'NONE', #81515 ) ;
#13994=EDGE_CURVE ( 'NONE', #11726, #80537, #19804, .T. ) ;
#13997=EDGE_LOOP ( 'NONE', ( #16494, #51032 ) ) ;
#13998=CARTESIAN_POINT ( 'NONE',  ( -9.692307692307691624, -12.37446782046654192, 30.86335684631486131 ) ) ;
#13999=DIRECTION ( 'NONE',  ( -0.000000000000000000, 0.8660254037844399289, -0.4999999999999980016 ) ) ;
#14000=CARTESIAN_POINT ( 'NONE',  ( -5.999999999999998224, -1.466349020453238561, 30.81389545987213907 ) ) ;
#14001=EDGE_CURVE ( 'NONE', #18284, #88230, #78395, .T. ) ;
#14004=EDGE_LOOP ( 'NONE', ( #71643, #12068, #46541, #38993 ) ) ;
#14006=CARTESIAN_POINT ( 'NONE',  ( -12.21159294319032007, -11.86320923018887541, 32.19269448109604781 ) ) ;
#14007=EDGE_LOOP ( 'NONE', ( #84562, #18506, #12522, #55415 ) ) ;
#14008=CARTESIAN_POINT ( 'NONE',  ( -5.326946301144534601, -2.341070481393820124, 30.72580821765574299 ) ) ;
#14010=CARTESIAN_POINT ( 'NONE',  ( 18.00000000000000000, -7.500000000000001776, 35.04278698407183867 ) ) ;
#14011=CARTESIAN_POINT ( 'NONE',  ( 9.757563263583717728, -10.90142922261932057, 33.41473453929631887 ) ) ;
#14012=CARTESIAN_POINT ( 'NONE',  ( -17.86947456176635640, -11.04252011169590197, 33.62494198852677840 ) ) ;
#14013=VECTOR ( 'NONE', #70082, 1000.000000000000114 ) ;
#14014=CARTESIAN_POINT ( 'NONE',  ( 16.82692307692308376, -7.566083408709835645, 34.74999999999999289 ) ) ;
#14016=CARTESIAN_POINT ( 'NONE',  ( -2.980769230767811084, -7.500000000000154543, 35.00000000000007105 ) ) ;
#14018=EDGE_LOOP ( 'NONE', ( #82282, #55132, #26037, #46834 ) ) ;
#14019=CARTESIAN_POINT ( 'NONE',  ( -3.099978789802281032, -6.369690395747422684, 34.87708834333098196 ) ) ;
#14020=B_SPLINE_CURVE_WITH_KNOTS ( 'NONE', 3,
 ( #41955, #83389, #42404, #70305, #14027, #65195, #7278, #36087, #7727, #62645 ),
 .UNSPECIFIED., .F., .F.,
 ( 4, 2, 2, 2, 4 ),
 ( 0.0007817359430256307648, 0.0009771253907249971907, 0.001172514838424363508, 0.001367904286123729826, 0.001563293733823096143 ),
 .UNSPECIFIED. ) ;
#14021=CARTESIAN_POINT ( 'NONE',  ( 8.769230769230768274, -10.05456864172156806, 36.03766855953608683 ) ) ;
#14023=EDGE_LOOP ( 'NONE', ( #52709, #14495, #1276, #55645 ) ) ;
#14024=ORIENTED_EDGE ( 'NONE', *, *, #40538, .T. ) ;
#14025=CARTESIAN_POINT ( 'NONE',  ( 2.557692307692372324, -7.434744860731434812, 35.00000000000000711 ) ) ;
#14026=CARTESIAN_POINT ( 'NONE',  ( 16.15384615384615330, -3.050289026998446396, 32.03036669348365706 ) ) ;
#14027=CARTESIAN_POINT ( 'NONE',  ( -1.134669866267241645, -6.696923467548660192, 34.68552623307873972 ) ) ;
#14028=CARTESIAN_POINT ( 'NONE',  ( -0.5268084620947816044, -11.06231777344662781, 33.60647404775220082 ) ) ;
#14029=CARTESIAN_POINT ( 'NONE',  ( 0.5923289025054093715, -2.295524264805589354, 30.44142389570982488 ) ) ;
#14030=VERTEX_POINT ( 'NONE', #22018 ) ;
#14031=AXIS2_PLACEMENT_3D ( 'NONE', #66713, #5013, #87908 ) ;
#14032=CARTESIAN_POINT ( 'NONE',  ( 6.000000000000001776, -5.557115091759785130, 34.35708131394839171 ) ) ;
#14034=B_SPLINE_CURVE_WITH_KNOTS ( 'NONE', 3,
 ( #53596, #39659, #87861, #82415, #19369, #20261, #47727, #48160, #19816, #40976 ),
 .UNSPECIFIED., .F., .F.,
 ( 4, 2, 2, 2, 4 ),
 ( 0.000000000000000000, 0.0001954339857564098054, 0.0003908679715128196108, 0.0005863019572692293891, 0.0007817359430256392216 ),
 .UNSPECIFIED. ) ;
#14035=CARTESIAN_POINT ( 'NONE',  ( 3.361294932532796320, -12.27024696741798770, 31.24895572276497546 ) ) ;
#14036=CARTESIAN_POINT ( 'NONE',  ( 17.99999999999987566, -12.51329471203414379, 31.30864560766407578 ) ) ;
#14037=ORIENTED_EDGE ( 'NONE', *, *, #70283, .F. ) ;
#14038=CARTESIAN_POINT ( 'NONE',  ( -17.07692307692307665, -11.91647553114624181, 32.58852847137148245 ) ) ;
#14039=EDGE_CURVE ( 'NONE', #25666, #76945, #10765, .T. ) ;
#14040=ORIENTED_EDGE ( 'NONE', *, *, #47555, .T. ) ;
#14042=CARTESIAN_POINT ( 'NONE',  ( 10.61538461538449418, -2.379036618888197729, 30.90682066428292885 ) ) ;
#14044=EDGE_CURVE ( 'NONE', #60933, #373, #39815, .T. ) ;
#14046=CARTESIAN_POINT ( 'NONE',  ( 7.780070435197965928, -12.10708131394839349, 31.69288490824020244 ) ) ;
#14047=DIRECTION ( 'NONE',  ( -0.000000000000000000, -0.5000000000000009992, -0.8660254037844380415 ) ) ;
#14048=CARTESIAN_POINT ( 'NONE',  ( -13.38461538461538325, -9.819645486525091727, 36.12317359536749706 ) ) ;
#14049=CARTESIAN_POINT ( 'NONE',  ( -7.911423846710166075, -5.094484230520674117, 34.41647553114621161 ) ) ;
#14050=CARTESIAN_POINT ( 'NONE',  ( 3.296024802045255164, -12.46129190930001052, 30.37095296980870174 ) ) ;
#14052=FACE_BOUND ( 'NONE', #8699, .T. ) ;
#14053=ORIENTED_EDGE ( 'NONE', *, *, #55304, .F. ) ;
#14054=CARTESIAN_POINT ( 'NONE',  ( -9.019253993452224449, -12.45566812827425451, 31.48439005359158926 ) ) ;
#14055=EDGE_CURVE ( 'NONE', #78946, #1158, #70201, .T. ) ;
#14057=CARTESIAN_POINT ( 'NONE',  ( 18.00000000000000000, -12.10708131394839349, 31.69288490824020244 ) ) ;
#14058=ADVANCED_FACE ( 'NONE', ( #84619 ), #35535, .F. ) ;
#14059=DIRECTION ( 'NONE',  ( -0.000000000000000000, 0.3420201433256694346, -0.9396926207859080948 ) ) ;
#14060=CARTESIAN_POINT ( 'NONE',  ( 14.43848274865925774, -8.191423895709840863, 34.95447573519442130 ) ) ;
#14061=ORIENTED_EDGE ( 'NONE', *, *, #36088, .F. ) ;
#14062=VECTOR ( 'NONE', #63512, 1000.000000000000114 ) ;
#14064=EDGE_LOOP ( 'NONE', ( #31521, #13311, #88795, #68143 ) ) ;
#14065=B_SPLINE_CURVE_WITH_KNOTS ( 'NONE', 3,
 ( #4940, #31510, #32404, #19337, #59428, #12143, #52215, #18006, #39624, #72491 ),
 .UNSPECIFIED., .F., .F.,
 ( 4, 2, 2, 2, 4 ),
 ( 0.000000000000000000, 0.0001954311564186865221, 0.0003908623128373730441, 0.0005862934692560595662, 0.0007817246256747460882 ),
 .UNSPECIFIED. ) ;
#14066=CARTESIAN_POINT ( 'NONE',  ( 13.63461538461532285, -7.565270445406050648, 34.75000000000000000 ) ) ;
#14067=ORIENTED_EDGE ( 'NONE', *, *, #64670, .T. ) ;
#14068=ADVANCED_FACE ( 'NONE', ( #30100 ), #71519, .F. ) ;
#14069=FACE_OUTER_BOUND ( 'NONE', #88530, .T. ) ;
#14070=CARTESIAN_POINT ( 'NONE',  ( -9.561469274294926990, -7.277220443632450575, 34.74524770363009196 ) ) ;
#14071=EDGE_CURVE ( 'NONE', #78927, #84142, #37288, .T. ) ;
#14072=CARTESIAN_POINT ( 'NONE',  ( 3.230769230769108269, -8.656820664282941280, 34.87096338111179961 ) ) ;
#14073=CARTESIAN_POINT ( 'NONE',  ( 3.230769230769231726, -9.058645607665452459, 34.76329471203371924 ) ) ;
#14075=CARTESIAN_POINT ( 'NONE',  ( 5.076923076923075762, -9.905515769479276145, 34.41647553114623292 ) ) ;
#14076=CARTESIAN_POINT ( 'NONE',  ( 15.45378058238208219, -9.086983370893049639, 34.49168942202179267 ) ) ;
#14077=DIRECTION ( 'NONE',  ( -0.000000000000000000, 0.8660254037844397068, -0.4999999999999978906 ) ) ;
#14078=CARTESIAN_POINT ( 'NONE',  ( 11.28843830116857383, -10.05641848906368097, 34.04755513067966177 ) ) ;
#14079=EDGE_LOOP ( 'NONE', ( #86488, #40350, #23639, #52871 ) ) ;
#14080=ORIENTED_EDGE ( 'NONE', *, *, #62198, .F. ) ;
#14081=ORIENTED_EDGE ( 'NONE', *, *, #54258, .T. ) ;
#14082=CARTESIAN_POINT ( 'NONE',  ( 4.153846153846154188, -2.538708090699994813, 30.37095296980875503 ) ) ;
#14084=CARTESIAN_POINT ( 'NONE',  ( -3.099978789802281032, -9.929761469519744921, 34.40412654351204225 ) ) ;
#14085=CARTESIAN_POINT ( 'NONE',  ( -5.933931648997561759, -3.513871655860379306, 32.76840700105978499 ) ) ;
#14086=CARTESIAN_POINT ( 'NONE',  ( 1.515140822849027957, -12.50538340440932394, 31.33453814440721885 ) ) ;
#14087=AXIS2_PLACEMENT_3D ( 'NONE', #33931, #88907, #41141 ) ;
#14088=LINE ( 'NONE', #47421, #65233 ) ;
#14089=FACE_BOUND ( 'NONE', #29530, .T. ) ;
#14090=CARTESIAN_POINT ( 'NONE',  ( 9.822833394071260216, -3.816742781228458448, 33.13167719472716044 ) ) ;
#14092=CARTESIAN_POINT ( 'NONE',  ( 14.53070515178570332, -12.38742843783360748, 31.66772728687926985 ) ) ;
#14093=ADVANCED_FACE ( 'NONE', ( #50356 ), #42742, .F. ) ;
#14094=CARTESIAN_POINT ( 'NONE',  ( -0.2115929431903201818, -9.272278438253398036, 34.42582936511637826 ) ) ;
#14095=CYLINDRICAL_SURFACE ( 'NONE', #26049, 0.2499999999999973355 ) ;
#14096=CARTESIAN_POINT ( 'NONE',  ( 6.000000000000001776, -11.11383981884818262, 36.00935417666054406 ) ) ;
#14097=VERTEX_POINT ( 'NONE', #4400 ) ;
#14098=CARTESIAN_POINT ( 'NONE',  ( 2.530703659305157949, -11.76359900205217457, 32.36225158514719880 ) ) ;
#14100=ORIENTED_EDGE ( 'NONE', *, *, #49815, .F. ) ;
#14101=FACE_BOUND ( 'NONE', #29318, .T. ) ;
#14102=CARTESIAN_POINT ( 'NONE',  ( -17.30040800148741198, -4.225889041578354544, 33.85425143139329407 ) ) ;
#14103=CARTESIAN_POINT ( 'NONE',  ( 18.00000000000000000, -8.810774026931790459, 35.74407628777942847 ) ) ;
#14105=VECTOR ( 'NONE', #45825, 1000.000000000000227 ) ;
#14106=EDGE_LOOP ( 'NONE', ( #6995, #85630 ) ) ;
#14107=CARTESIAN_POINT ( 'NONE',  ( -14.55771554498526932, -12.43535235679832596, 30.55408501211184813 ) ) ;
#14108=CARTESIAN_POINT ( 'NONE',  ( -5.869474561766354626, -9.503571793651733657, 34.60286762892837942 ) ) ;
#14109=DIRECTION ( 'NONE',  ( -0.000000000000000000, -0.9396926207859092051, -0.3420201433256662704 ) ) ;
#14111=CARTESIAN_POINT ( 'NONE',  ( 4.153846153846154188, -2.708943851104267164, 35.45975837776705220 ) ) ;
#14112=VERTEX_POINT ( 'NONE', #11159 ) ;
#14113=CARTESIAN_POINT ( 'NONE',  ( 13.25392391794782654, -5.582088688514999397, 34.36776431015576350 ) ) ;
#14114=FACE_OUTER_BOUND ( 'NONE', #15899, .T. ) ;
#14115=CARTESIAN_POINT ( 'NONE',  ( 3.903846153846154632, -2.499999999999998668, 29.75000000000000355 ) ) ;
#14116=ORIENTED_EDGE ( 'NONE', *, *, #71737, .F. ) ;
#14117=CARTESIAN_POINT ( 'NONE',  ( 16.02315555073584008, -3.957541250942358424, 33.62499894934981626 ) ) ;
#14118=DIRECTION ( 'NONE',  ( -1.000000000000000000, 0.000000000000000000, 0.000000000000000000 ) ) ;
#14119=CARTESIAN_POINT ( 'NONE',  ( 16.40390057375961064, -12.01375889529407992, 32.43194544308182969 ) ) ;
#14120=CARTESIAN_POINT ( 'NONE',  ( -13.38461538461550582, -3.835265460704628371, 33.15142922262033665 ) ) ;
#14121=CARTESIAN_POINT ( 'NONE',  ( 11.53846153846141576, -8.656820664282941280, 34.87096338111179961 ) ) ;
#14122=CARTESIAN_POINT ( 'NONE',  ( -6.000000000000121680, -6.835583212225970762, 34.95778746994575670 ) ) ;
#14124=CARTESIAN_POINT ( 'NONE',  ( 14.17754509825408604, -3.817052484675422797, 33.13202310037935661 ) ) ;
#14127=CARTESIAN_POINT ( 'NONE',  ( -17.93393164899756087, -8.973038597847269315, 34.52809138561122637 ) ) ;
#14128=ORIENTED_EDGE ( 'NONE', *, *, #74646, .T. ) ;
#14130=ORIENTED_EDGE ( 'NONE', *, *, #88659, .T. ) ;
#14131=CYLINDRICAL_SURFACE ( 'NONE', #67196, 0.2499999999999979738 ) ;
#14133=CYLINDRICAL_SURFACE ( 'NONE', #916, 0.2499999999999995559 ) ;
#14135=B_SPLINE_CURVE_WITH_KNOTS ( 'NONE', 3,
 ( #58113, #31081, #78382, #2714, #50894, #71623, #3612, #51326, #49593, #9928 ),
 .UNSPECIFIED., .F., .F.,
 ( 4, 2, 2, 2, 4 ),
 ( 0.0007817359430256334753, 0.0009771253907250058643, 0.001172514838424371098, 0.001367904286123736764, 0.001563293733823101998 ),
 .UNSPECIFIED. ) ;
#14136=FACE_OUTER_BOUND ( 'NONE', #51806, .T. ) ;
#14137=CARTESIAN_POINT ( 'NONE',  ( 2.980745993476266786, -8.432397168068783699, 34.66272746175022945 ) ) ;
#14139=CARTESIAN_POINT ( 'NONE',  ( -7.146003881983771677, -9.172386477786396597, 34.72672124145550043 ) ) ;
#14140=CARTESIAN_POINT ( 'NONE',  ( 9.942253101685738059, -12.45601412856602686, 31.48342859153981621 ) ) ;
#14141=CARTESIAN_POINT ( 'NONE',  ( -11.78848477575450282, -5.056417327199099532, 34.11270091957321426 ) ) ;
#14143=CARTESIAN_POINT ( 'NONE',  ( -7.846153846153844924, -11.69971097300155272, 32.46337939537588113 ) ) ;
#14144=CARTESIAN_POINT ( 'NONE',  ( 15.00784227186238162, -9.172386477786396597, 34.72672124145550043 ) ) ;
#14145=VECTOR ( 'NONE', #39767, 1000.000000000000114 ) ;
#14146=FACE_OUTER_BOUND ( 'NONE', #24820, .T. ) ;
#14147=CARTESIAN_POINT ( 'NONE',  ( -13.38461538461550582, -11.48612834414049644, 32.76840700105863391 ) ) ;
#14148=ADVANCED_FACE ( 'NONE', ( #80062 ), #31885, .F. ) ;
#14149=ORIENTED_EDGE ( 'NONE', *, *, #39338, .T. ) ;
#14150=ORIENTED_EDGE ( 'NONE', *, *, #66195, .T. ) ;
#14151=CARTESIAN_POINT ( 'NONE',  ( -39.05038313613820122, -2.249999999999998668, 29.75000000000000355 ) ) ;
#14152=DIRECTION ( 'NONE',  ( -0.000000000000000000, 0.6427876096865404731, -0.7660444431189771253 ) ) ;
#14153=CARTESIAN_POINT ( 'NONE',  ( -16.15384615384615330, -11.33034616979429110, 35.88435417666054406 ) ) ;
#14154=CARTESIAN_POINT ( 'NONE',  ( -11.78846153846154010, -7.433931650972299465, 34.75000000000000711 ) ) ;
#14155=ADVANCED_FACE ( 'NONE', ( #86851 ), #4856, .F. ) ;
#14156=CARTESIAN_POINT ( 'NONE',  ( 12.33139125210024112, -9.418419913701741919, 34.36755862841477693 ) ) ;
#14157=CARTESIAN_POINT ( 'NONE',  ( -9.822455662039388358, -6.809168938359901446, 34.95455904226513866 ) ) ;
#14158=EDGE_CURVE ( 'NONE', #62900, #27787, #79622, .T. ) ;
#14159=CYLINDRICAL_SURFACE ( 'NONE', #50858, 0.2499999999999986955 ) ;
#14160=ORIENTED_EDGE ( 'NONE', *, *, #84483, .F. ) ;
#14161=CARTESIAN_POINT ( 'NONE',  ( 15.93036121012220541, -2.847400154188068910, 31.58180166144859768 ) ) ;
#14163=EDGE_CURVE ( 'NONE', #5477, #15866, #30973, .T. ) ;
#14165=B_SPLINE_CURVE_WITH_KNOTS ( 'NONE', 3,
 ( #59338, #66550, #37285, #65639, #64750, #10715, #32324, #59785, #45372, #73305 ),
 .UNSPECIFIED., .F., .F.,
 ( 4, 2, 2, 2, 4 ),
 ( 0.0007817359430256392216, 0.0009771253907250080327, 0.001172514838424376952, 0.001367904286123745872, 0.001563293733823114791 ),
 .UNSPECIFIED. ) ;
#14166=CARTESIAN_POINT ( 'NONE',  ( 9.822833394071260216, -11.93748526763465279, 32.05452791011430946 ) ) ;
#14167=CARTESIAN_POINT ( 'NONE',  ( 18.00000000000000000, -12.78798330534103123, 29.99999999999997868 ) ) ;
#14168=CARTESIAN_POINT ( 'NONE',  ( -4.219929564802033184, -4.098570777380720287, 33.41473453929634729 ) ) ;
#14169=CARTESIAN_POINT ( 'NONE',  ( 3.930919194939304973, -6.459968553980839800, 34.89616026154728701 ) ) ;
#14171=EDGE_LOOP ( 'NONE', ( #33173, #59631, #23338, #31666 ) ) ;
#14172=ORIENTED_EDGE ( 'NONE', *, *, #35105, .F. ) ;
#14173=ORIENTED_EDGE ( 'NONE', *, *, #41024, .T. ) ;
#14175=DIRECTION ( 'NONE',  ( -0.000000000000000000, 0.9848077530122085754, -0.1736481776669273613 ) ) ;
#14176=CARTESIAN_POINT ( 'NONE',  ( 7.780070435197965928, -3.513871655860377086, 32.76840700105978499 ) ) ;
#14177=ADVANCED_FACE ( 'NONE', ( #44931 ), #18367, .F. ) ;
#14179=CARTESIAN_POINT ( 'NONE',  ( -15.29685264172511161, -11.16473453929635440, 33.15142922261925662 ) ) ;
#14180=AXIS2_PLACEMENT_3D ( 'NONE', #27083, #68509, #6807 ) ;
#14181=CARTESIAN_POINT ( 'NONE',  ( 7.780400417840515281, -7.249945578846652694, 34.99404164642496795 ) ) ;
#14183=ORIENTED_EDGE ( 'NONE', *, *, #8895, .F. ) ;
#14184=ORIENTED_EDGE ( 'NONE', *, *, #58544, .F. ) ;
#14185=ORIENTED_EDGE ( 'NONE', *, *, #58318, .F. ) ;
#14186=LINE ( 'NONE', #41666, #77641 ) ;
#14187=EDGE_CURVE ( 'NONE', #17157, #63787, #73148, .T. ) ;
#14188=EDGE_LOOP ( 'NONE', ( #44401, #48071, #38739, #85769 ) ) ;
#14189=CARTESIAN_POINT ( 'NONE',  ( 9.442330948259101575, -8.347322224742351082, 34.93158281831414769 ) ) ;
#14190=CARTESIAN_POINT ( 'NONE',  ( -12.33074802057151409, -11.93129842949671726, 32.56571108434900452 ) ) ;
#14191=AXIS2_PLACEMENT_3D ( 'NONE', #30496, #49448, #49001 ) ;
#14193=VERTEX_POINT ( 'NONE', #46281 ) ;
#14194=EDGE_CURVE ( 'NONE', #85648, #21721, #66555, .T. ) ;
#14195=AXIS2_PLACEMENT_3D ( 'NONE', #36476, #76577, #36039 ) ;
#14196=ADVANCED_FACE ( 'NONE', ( #72851 ), #32763, .F. ) ;
#14197=B_SPLINE_CURVE_WITH_KNOTS ( 'NONE', 3,
 ( #38446, #4209, #18177, #45642, #73117, #38901, #25371, #59597, #87097, #46092 ),
 .UNSPECIFIED., .F., .F.,
 ( 4, 2, 2, 2, 4 ),
 ( 0.000000000000000000, 0.0001954339857564079623, 0.0003908679715128159245, 0.0005863019572692238597, 0.0007817359430256318490 ),
 .UNSPECIFIED. ) ;
#14198=B_SPLINE_CURVE_WITH_KNOTS ( 'NONE', 3,
 ( #3097, #69797, #35577, #22059, #56283, #30573, #29707, #83772, #1337, #49532 ),
 .UNSPECIFIED., .F., .F.,
 ( 4, 2, 2, 2, 4 ),
 ( 0.000000000000000000, 0.0001954339857564098054, 0.0003908679715128196108, 0.0005863019572692293891, 0.0007817359430256392216 ),
 .UNSPECIFIED. ) ;
#14199=VERTEX_POINT ( 'NONE', #46722 ) ;
#14200=CARTESIAN_POINT ( 'NONE',  ( 13.38461538461538680, -10.67929555188718282, 33.92786785259544047 ) ) ;
#14201=EDGE_LOOP ( 'NONE', ( #9940, #23972 ) ) ;
#14202=FACE_BOUND ( 'NONE', #55167, .T. ) ;
#14203=DIRECTION ( 'NONE',  ( -0.000000000000000000, 0.9396926207859093161, -0.3420201433256663259 ) ) ;
#14204=DIRECTION ( 'NONE',  ( -0.000000000000000000, -0.000000000000000000, -1.000000000000000000 ) ) ;
#14206=DIRECTION ( 'NONE',  ( -0.000000000000000000, 1.000000000000000000, 3.491481338843133355E-15 ) ) ;
#14207=DIRECTION ( 'NONE',  ( -0.000000000000000000, -0.5000000000000011102, -0.8660254037844381525 ) ) ;
#14208=CARTESIAN_POINT ( 'NONE',  ( -13.38461538461550759, -4.320704448113951379, 33.92786785259630022 ) ) ;
#14210=EDGE_LOOP ( 'NONE', ( #82121, #65484, #54720, #28127 ) ) ;
#14211=CARTESIAN_POINT ( 'NONE',  ( -12.39547112818838492, -2.292212530054420494, 30.41441678777542990 ) ) ;
#14212=CARTESIAN_POINT ( 'NONE',  ( -4.023055712879203938, -9.929761469519744921, 34.40412654351204225 ) ) ;
#14213=CARTESIAN_POINT ( 'NONE',  ( 4.284371592079796010, -11.66157788607254275, 32.95092075102925833 ) ) ;
#14214=CARTESIAN_POINT ( 'NONE',  ( -2.057746898314262829, -9.357781135181031829, 34.66075350412533851 ) ) ;
#14215=EDGE_CURVE ( 'NONE', #23399, #9486, #2147, .T. ) ;
#14216=DIRECTION ( 'NONE',  ( -0.000000000000000000, 0.5000000000000011102, -0.8660254037844380415 ) ) ;
#14217=EDGE_CURVE ( 'NONE', #85803, #69402, #53470, .T. ) ;
#14218=FACE_BOUND ( 'NONE', #56292, .T. ) ;
#14219=CARTESIAN_POINT ( 'NONE',  ( -6.700064078983528404, -12.64618726649961289, 30.78989965857442712 ) ) ;
#14220=CARTESIAN_POINT ( 'NONE',  ( -6.065270000556318486, -10.33852847137145048, 34.16647553114627556 ) ) ;
#14221=CARTESIAN_POINT ( 'NONE',  ( -7.146003140593069958, -12.15238873228292071, 31.58232369045353849 ) ) ;
#14222=CARTESIAN_POINT ( 'NONE',  ( -5.777220458731591179, -10.11255958852956027, 34.01340905677048454 ) ) ;
#14223=CARTESIAN_POINT ( 'NONE',  ( 2.438482748659258625, -6.369690395747422684, 34.87708834333098196 ) ) ;
#14224=CARTESIAN_POINT ( 'NONE',  ( -7.911423846710166075, -4.320704448112771878, 33.92786785259540494 ) ) ;
#14225=VECTOR ( 'NONE', #38943, 1000.000000000000000 ) ;
#14227=EDGE_CURVE ( 'NONE', #35007, #32782, #79531, .T. ) ;
#14228=VERTEX_POINT ( 'NONE', #81852 ) ;
#14229=CARTESIAN_POINT ( 'NONE',  ( 1.134592147322421196, -12.22074536777954989, 31.39888409691088356 ) ) ;
#14230=ORIENTED_EDGE ( 'NONE', *, *, #58489, .T. ) ;
#14231=CARTESIAN_POINT ( 'NONE',  ( -13.31854805126531005, -10.67929555188718282, 33.92786785259544757 ) ) ;
#14232=ORIENTED_EDGE ( 'NONE', *, *, #54818, .T. ) ;
#14233=CARTESIAN_POINT ( 'NONE',  ( -11.53846153846166089, -6.835583212225970762, 34.95778746994575670 ) ) ;
#14234=CARTESIAN_POINT ( 'NONE',  ( 14.17754433796061875, -4.299443229763728169, 33.91186481527756058 ) ) ;
#14235=EDGE_LOOP ( 'NONE', ( #41700, #89092, #67946, #46715 ) ) ;
#14236=CARTESIAN_POINT ( 'NONE',  ( 2.307692307692309264, -8.120952969808772792, 34.71129190930000163 ) ) ;
#14238=CARTESIAN_POINT ( 'NONE',  ( 3.930361210122205406, -9.331801661448606566, 34.40259984581193464 ) ) ;
#14239=B_SPLINE_CURVE_WITH_KNOTS ( 'NONE', 3,
 ( #83783, #1791, #50407, #23383, #28377, #55848, #69809, #14879, #43659, #49972 ),
 .UNSPECIFIED., .F., .F.,
 ( 4, 2, 2, 2, 4 ),
 ( 0.000000000000000000, 0.0001954339857564076912, 0.0003908679715128153824, 0.0005863019572692231007, 0.0007817359430256307648 ),
 .UNSPECIFIED. ) ;
#14240=CARTESIAN_POINT ( 'NONE',  ( 5.010839665967195877, -4.786620604624113540, 33.94971097300155805 ) ) ;
#14241=CARTESIAN_POINT ( 'NONE',  ( -3.100724174849458059, -2.254550872974306674, 29.97347326024527447 ) ) ;
#14243=CARTESIAN_POINT ( 'NONE',  ( 2.373760658694747061, -2.721908614388771852, 31.22303859784725333 ) ) ;
#14244=CARTESIAN_POINT ( 'NONE',  ( -5.749945688361683516, -10.66356715214248396, 33.62249196103329751 ) ) ;
#14245=B_SPLINE_CURVE_WITH_KNOTS ( 'NONE', 3,
 ( #27876, #63426, #84167, #63868, #22443, #49909, #7609, #14356, #77387, #43162 ),
 .UNSPECIFIED., .F., .F.,
 ( 4, 2, 2, 2, 4 ),
 ( 0.0007817246256747469556, 0.0009771112852218892010, 0.001172497944769031230, 0.001367884604316173258, 0.001563271263863315504 ),
 .UNSPECIFIED. ) ;
#14247=CARTESIAN_POINT ( 'NONE',  ( -18.13069060311031677, -11.37499894934982514, 33.29245874905763003 ) ) ;
#14248=CARTESIAN_POINT ( 'NONE',  ( 10.61538461538449596, -11.48612834414049644, 32.76840700105863391 ) ) ;
#14249=VERTEX_POINT ( 'NONE', #20137 ) ;
#14250=CARTESIAN_POINT ( 'NONE',  ( 17.07692307692307665, -3.886160181151819604, 36.00935417666054406 ) ) ;
#14252=EDGE_CURVE ( 'NONE', #76909, #41676, #54796, .T. ) ;
#14253=CARTESIAN_POINT ( 'NONE',  ( -15.93106648486808119, -12.47679350104403007, 31.42216943046555855 ) ) ;
#14255=DIRECTION ( 'NONE',  ( -0.000000000000000000, -0.8660254037844397068, -0.4999999999999978906 ) ) ;
#14256=ORIENTED_EDGE ( 'NONE', *, *, #62567, .T. ) ;
#14257=CARTESIAN_POINT ( 'NONE',  ( 14.37376065869474751, -2.538708090699994813, 30.37095296980875503 ) ) ;
#14258=CARTESIAN_POINT ( 'NONE',  ( -14.55771554498527287, -11.37209801155882971, 32.91403422569032955 ) ) ;
#14260=ORIENTED_EDGE ( 'NONE', *, *, #27613, .F. ) ;
#14261=CARTESIAN_POINT ( 'NONE',  ( 14.30769230769231015, -13.53365097954675988, 30.81389545987213552 ) ) ;
#14262=CARTESIAN_POINT ( 'NONE',  ( 13.51514108637895184, -2.619367082507849442, 30.83698974864643461 ) ) ;
#14263=AXIS2_PLACEMENT_3D ( 'NONE', #82665, #61479, #6552 ) ;
#14264=CARTESIAN_POINT ( 'NONE',  ( 16.15384615384615330, -8.973038597847269315, 34.52809138561121927 ) ) ;
#14265=CARTESIAN_POINT ( 'NONE',  ( -17.07692307692307665, -2.721908614388771852, 31.22303859784724978 ) ) ;
#14266=CARTESIAN_POINT ( 'NONE',  ( 6.699591979352975457, -5.113361153441932316, 34.14387501736621999 ) ) ;
#14267=VERTEX_POINT ( 'NONE', #69209 ) ;
#14268=VERTEX_POINT ( 'NONE', #68321 ) ;
#14269=ORIENTED_EDGE ( 'NONE', *, *, #84507, .F. ) ;
#14270=B_SPLINE_CURVE_WITH_KNOTS ( 'NONE', 3,
 ( #7569, #20629, #69266, #76469, #1240, #42248, #42687, #22404, #89118, #21515 ),
 .UNSPECIFIED., .F., .F.,
 ( 4, 2, 2, 2, 4 ),
 ( 0.000000000000000000, 0.0001954339857564080707, 0.0003908679715128161414, 0.0005863019572692241849, 0.0007817359430256322827 ),
 .UNSPECIFIED. ) ;
#14272=LINE ( 'NONE', #35426, #60149 ) ;
#14273=CYLINDRICAL_SURFACE ( 'NONE', #37794, 0.2499999999999994726 ) ;
#14274=CARTESIAN_POINT ( 'NONE',  ( -6.923076923076922462, -3.937682226553329556, 33.60647404775216529 ) ) ;
#14275=ORIENTED_EDGE ( 'NONE', *, *, #29640, .T. ) ;
#14276=EDGE_CURVE ( 'NONE', #23267, #50940, #36626, .T. ) ;
#14277=CARTESIAN_POINT ( 'NONE',  ( 17.14217821643591577, -11.67786785259547777, 32.92929555188713664 ) ) ;
#14278=VERTEX_POINT ( 'NONE', #12935 ) ;
#14279=ORIENTED_EDGE ( 'NONE', *, *, #35933, .F. ) ;
#14281=CARTESIAN_POINT ( 'NONE',  ( -15.36091644020745584, -12.27039167877662251, 31.24851455888617835 ) ) ;
#14282=VERTEX_POINT ( 'NONE', #309 ) ;
#14283=CARTESIAN_POINT ( 'NONE',  ( -0.7115616988314262814, -5.056417327199099532, 34.11270091957321426 ) ) ;
#14285=CARTESIAN_POINT ( 'NONE',  ( 5.869852030268304155, -12.70455904226513866, 30.44083106164009322 ) ) ;
#14286=CARTESIAN_POINT ( 'NONE',  ( -10.61538461538461320, -6.343179335718451384, 34.87096338111211935 ) ) ;
#14287=EDGE_CURVE ( 'NONE', #67890, #57330, #90, .T. ) ;
#14288=CARTESIAN_POINT ( 'NONE',  ( -6.923076923076922462, -8.564572088678739092, 35.78748833219616898 ) ) ;
#14289=ORIENTED_EDGE ( 'NONE', *, *, #49496, .F. ) ;
#14290=EDGE_CURVE ( 'NONE', #2529, #29364, #41301, .T. ) ;
#14291=ORIENTED_EDGE ( 'NONE', *, *, #26863, .F. ) ;
#14293=CARTESIAN_POINT ( 'NONE',  ( -2.307692307692305711, -3.322132147404559976, 32.92929555188717927 ) ) ;
#14295=ORIENTED_EDGE ( 'NONE', *, *, #2645, .T. ) ;
#14296=LINE ( 'NONE', #75126, #15867 ) ;
#14297=CARTESIAN_POINT ( 'NONE',  ( -0.5276208408985970655, -6.343179335718451384, 34.87096338111212646 ) ) ;
#14298=ORIENTED_EDGE ( 'NONE', *, *, #61408, .T. ) ;
#14299=EDGE_CURVE ( 'NONE', #45063, #56304, #35500, .T. ) ;
#14300=CYLINDRICAL_SURFACE ( 'NONE', #23554, 0.2500000000000002220 ) ;
#14303=FACE_BOUND ( 'NONE', #27001, .T. ) ;
#14304=CARTESIAN_POINT ( 'NONE',  ( -0.4615384615385826339, -10.21337939537710326, 33.94971097300076224 ) ) ;
#14305=CARTESIAN_POINT ( 'NONE',  ( 16.08857615328984281, -2.657715359629089669, 31.77849191805833584 ) ) ;
#14306=CARTESIAN_POINT ( 'NONE',  ( 12.21156171748986985, -6.524016743844655686, 34.90889640711025521 ) ) ;
#14307=CARTESIAN_POINT ( 'NONE',  ( 18.13052543823364360, -3.068774925481847937, 32.56582465632704526 ) ) ;
#14308=AXIS2_PLACEMENT_3D ( 'NONE', #87349, #32829, #66619 ) ;
#14309=CARTESIAN_POINT ( 'NONE',  ( -9.692307692307812417, -2.892918686052166066, 31.69288490824153470 ) ) ;
#14310=DIRECTION ( 'NONE',  ( 0.000000000000000000, 0.6427876096865373645, -0.7660444431189797898 ) ) ;
#14311=CARTESIAN_POINT ( 'NONE',  ( -2.307692307692427391, -3.835265460704628371, 33.15142922262033665 ) ) ;
#14312=ORIENTED_EDGE ( 'NONE', *, *, #64096, .F. ) ;
#14313=DIRECTION ( 'NONE',  ( -0.000000000000000000, -0.3420201433256694346, -0.9396926207859080948 ) ) ;
#14314=CARTESIAN_POINT ( 'NONE',  ( 13.60757828817687276, -7.369474270740069777, 34.74850911626239736 ) ) ;
#14315=VERTEX_POINT ( 'NONE', #21464 ) ;
#14316=VECTOR ( 'NONE', #70235, 1000.000000000000114 ) ;
#14320=ORIENTED_EDGE ( 'NONE', *, *, #70443, .F. ) ;
#14321=CARTESIAN_POINT ( 'NONE',  ( 18.00000000000000000, -5.557115091759785130, 34.35708131394839171 ) ) ;
#14322=ADVANCED_FACE ( 'NONE', ( #74198 ), #39979, .F. ) ;
#14323=DIRECTION ( 'NONE',  ( 0.000000000000000000, 0.6427876096865373645, -0.7660444431189797898 ) ) ;
#14324=FACE_BOUND ( 'NONE', #72014, .T. ) ;
#14325=CARTESIAN_POINT ( 'NONE',  ( 6.673053698855467175, -4.175268141568689195, 33.81360843649122216 ) ) ;
#14326=CARTESIAN_POINT ( 'NONE',  ( 4.088576153289833925, -12.51329471203370325, 31.30864560766548976 ) ) ;
#14327=CARTESIAN_POINT ( 'NONE',  ( -9.019254006523732770, -6.695914987888146541, 34.68535235679833306 ) ) ;
#14328=CARTESIAN_POINT ( 'NONE',  ( -15.29685264172511161, -8.973038597847271092, 34.52809138561120506 ) ) ;
#14330=CARTESIAN_POINT ( 'NONE',  ( 0.2115152242454954590, -5.851115903089113779, 34.47074536777953568 ) ) ;
#14331=CARTESIAN_POINT ( 'NONE',  ( -17.86920819217521483, -4.809403383903224416, 33.96459661697924304 ) ) ;
#14333=VERTEX_POINT ( 'NONE', #72636 ) ;
#14334=B_SPLINE_CURVE_WITH_KNOTS ( 'NONE', 3,
 ( #42178, #35402, #63316, #1626, #29109, #36302, #38517, #77717, #51550, #30422 ),
 .UNSPECIFIED., .F., .F.,
 ( 4, 2, 2, 2, 4 ),
 ( 0.0007817359430256216575, 0.0009771253907249856981, 0.001172514838424349630, 0.001367904286123713779, 0.001563293733823077711 ),
 .UNSPECIFIED. ) ;
#14336=CARTESIAN_POINT ( 'NONE',  ( -9.758390071667831123, -2.292212530054419606, 30.41441678777542634 ) ) ;
#14338=CARTESIAN_POINT ( 'NONE',  ( 1.515140822849031732, -9.503571793651733657, 34.60286762892837942 ) ) ;
#14339=CARTESIAN_POINT ( 'NONE',  ( -8.899378738962466784, -8.630895178749533159, 34.87696386517710323 ) ) ;
#14340=CARTESIAN_POINT ( 'NONE',  ( -16.28399336328438096, -12.27039167877662251, 31.24851455888617835 ) ) ;
#14342=CYLINDRICAL_SURFACE ( 'NONE', #18751, 0.2500000000000008882 ) ;
#14343=CARTESIAN_POINT ( 'NONE',  ( 5.750023255951409951, -2.920706130388546651, 32.31842814019191223 ) ) ;
#14344=CARTESIAN_POINT ( 'NONE',  ( 6.065255139512838234, -4.320704448112861584, 33.92786785259548310 ) ) ;
#14345=DIRECTION ( 'NONE',  ( 0.000000000000000000, 0.000000000000000000, 1.000000000000000000 ) ) ;
#14346=CARTESIAN_POINT ( 'NONE',  ( -15.10024352900566846, -11.46989282347013095, 32.79007818306219946 ) ) ;
#14347=CARTESIAN_POINT ( 'NONE',  ( 18.24994551834813805, -10.05730279482229683, 34.04704008940765902 ) ) ;
#14348=CARTESIAN_POINT ( 'NONE',  ( -9.692307692307691624, -12.62096338111211580, 30.90682066428153263 ) ) ;
#14349=FACE_OUTER_BOUND ( 'NONE', #29933, .T. ) ;
#14350=CARTESIAN_POINT ( 'NONE',  ( 2.980745993476267675, -2.587272538249755449, 30.68239716806877837 ) ) ;
#14351=EDGE_LOOP ( 'NONE', ( #71419, #35741, #18136, #34396 ) ) ;
#14352=CARTESIAN_POINT ( 'NONE',  ( 2.084765348785459160, -3.395401636524185474, 33.02366814457250399 ) ) ;
#14353=LINE ( 'NONE', #62526, #21583 ) ;
#14355=CARTESIAN_POINT ( 'NONE',  ( -0.3307480205715112032, -10.70102852606553157, 33.91149625220312913 ) ) ;
#14356=CARTESIAN_POINT ( 'NONE',  ( -16.02305571287920216, -2.494656445102014342, 31.33466734024120015 ) ) ;
#14357=EDGE_LOOP ( 'NONE', ( #11384, #59528, #83362, #32793 ) ) ;
#14358=CARTESIAN_POINT ( 'NONE',  ( 10.39251919318097883, -2.501496062324912284, 29.88072118266895671 ) ) ;
#14359=CARTESIAN_POINT ( 'NONE',  ( -5.934855219280366967, -7.750023224968867197, 34.99404313364389907 ) ) ;
#14360=ORIENTED_EDGE ( 'NONE', *, *, #57133, .F. ) ;
#14362=CARTESIAN_POINT ( 'NONE',  ( -9.626240358957616650, -5.471508081941601098, 34.59228464037088457 ) ) ;
#14363=VERTEX_POINT ( 'NONE', #8396 ) ;
#14364=CARTESIAN_POINT ( 'NONE',  ( -5.143006487878956534, -12.10708131394839349, 31.69288490824020244 ) ) ;
#14365=CARTESIAN_POINT ( 'NONE',  ( 7.976201452409529047, -7.723484964179499812, 34.74522123443822608 ) ) ;
#14366=ORIENTED_EDGE ( 'NONE', *, *, #75165, .T. ) ;
#14367=B_SPLINE_CURVE_WITH_KNOTS ( 'NONE', 3,
 ( #28095, #35292, #14579, #27649, #8275, #14137, #61428, #82619, #55558, #83494 ),
 .UNSPECIFIED., .F., .F.,
 ( 4, 2, 2, 2, 4 ),
 ( 0.000000000000000000, 0.0001954339857564079352, 0.0003908679715128158703, 0.0005863019572692237513, 0.0007817359430256317406 ),
 .UNSPECIFIED. ) ;
#14368=CARTESIAN_POINT ( 'NONE',  ( -10.83886953994894675, -4.225889041578353655, 33.85425143139329407 ) ) ;
#14369=CARTESIAN_POINT ( 'NONE',  ( -16.02379854759047006, -7.723484964179501588, 34.74522123443823318 ) ) ;
#14370=B_SPLINE_CURVE_WITH_KNOTS ( 'NONE', 3,
 ( #49272, #200, #76294, #21353, #40752, #27667, #8293, #26784, #34862, #83064 ),
 .UNSPECIFIED., .F., .F.,
 ( 4, 2, 2, 2, 4 ),
 ( 0.000000000000000000, 0.0001954311564186865763, 0.0003908623128373730441, 0.0005862934692560595662, 0.0007817246256747460882 ),
 .UNSPECIFIED. ) ;
#14371=AXIS2_PLACEMENT_3D ( 'NONE', #11763, #45535, #17174 ) ;
#14372=CARTESIAN_POINT ( 'NONE',  ( 9.692307692307570832, -6.835583212225970762, 34.95778746994575670 ) ) ;
#14374=ORIENTED_EDGE ( 'NONE', *, *, #65155, .T. ) ;
#14375=CARTESIAN_POINT ( 'NONE',  ( -6.923076923076922462, -8.164416787775445883, 34.95778746994557906 ) ) ;
#14376=B_SPLINE_CURVE_WITH_KNOTS ( 'NONE', 3,
 ( #17739, #10981, #86662, #66363, #22815, #51484, #4667, #78985, #34343, #55503 ),
 .UNSPECIFIED., .F., .F.,
 ( 4, 2, 2, 2, 4 ),
 ( 0.0007817246256747494492, 0.0009771112852218941883, 0.001172497944769039036, 0.001367884604316183883, 0.001563271263863328731 ),
 .UNSPECIFIED. ) ;
#14377=B_SPLINE_CURVE_WITH_KNOTS ( 'NONE', 3,
 ( #39179, #10360, #10804, #85575, #38273, #45016, #32407, #51301, #31514, #66638 ),
 .UNSPECIFIED., .F., .F.,
 ( 4, 2, 2, 2, 4 ),
 ( 0.0007817359527651096280, 0.0009771254036996484919, 0.001172514854634187573, 0.001367904305568726653, 0.001563293756503265517 ),
 .UNSPECIFIED. ) ;
#14380=VECTOR ( 'NONE', #80793, 1000.000000000000114 ) ;
#14381=CARTESIAN_POINT ( 'NONE',  ( -17.93393266664992325, -4.661471528628506888, 34.16647553114624003 ) ) ;
#14382=CARTESIAN_POINT ( 'NONE',  ( -6.988346923633241836, -2.379036618887870436, 30.90682066428147934 ) ) ;
#14383=CARTESIAN_POINT ( 'NONE',  ( 3.230769230769231726, -8.564572088678739092, 35.78748833219616898 ) ) ;
#14384=CARTESIAN_POINT ( 'NONE',  ( 12.46153846153846168, -8.318370150425687726, 35.83090037661290239 ) ) ;
#14385=CARTESIAN_POINT ( 'NONE',  ( -0.2115930521604186265, -5.766571408460171355, 34.70601412856602508 ) ) ;
#14386=CARTESIAN_POINT ( 'NONE',  ( 1.161130460051056135, -2.353723527008297012, 30.78948104536958397 ) ) ;
#14387=AXIS2_PLACEMENT_3D ( 'NONE', #30198, #50882, #38727 ) ;
#14388=AXIS2_PLACEMENT_3D ( 'NONE', #1566, #28601, #10875 ) ;
#14390=FACE_OUTER_BOUND ( 'NONE', #83957, .T. ) ;
#14391=ORIENTED_EDGE ( 'NONE', *, *, #40180, .F. ) ;
#14392=EDGE_LOOP ( 'NONE', ( #40033, #5672, #51796, #6921 ) ) ;
#14393=CARTESIAN_POINT ( 'NONE',  ( -0.3962828902624367933, -12.27809138561124591, 31.22303859784720359 ) ) ;
#14396=ADVANCED_FACE ( 'NONE', ( #1185 ), #22782, .F. ) ;
#14398=DIRECTION ( 'NONE',  ( -0.000000000000000000, 1.000000000000000000, 3.491481338843133355E-15 ) ) ;
#14399=CARTESIAN_POINT ( 'NONE',  ( 5.299934428535925335, -3.587049720035815348, 32.86302985866382897 ) ) ;
#14400=EDGE_LOOP ( 'NONE', ( #31361, #42561 ) ) ;
#14401=CARTESIAN_POINT ( 'NONE',  ( -9.942307692307695177, -2.499999999999999556, 29.81609845454691765 ) ) ;
#14403=ORIENTED_EDGE ( 'NONE', *, *, #82442, .T. ) ;
#14404=CARTESIAN_POINT ( 'NONE',  ( -10.48454619737184679, -7.277220443632450575, 34.74524770363009196 ) ) ;
#14405=B_SPLINE_CURVE_WITH_KNOTS ( 'NONE', 3,
 ( #28477, #21266, #55940, #77106, #70354, #49187, #14970, #50067, #8656, #77548 ),
 .UNSPECIFIED., .F., .F.,
 ( 4, 2, 2, 2, 4 ),
 ( 0.000000000000000000, 0.0001954339857564054144, 0.0003908679715128108288, 0.0005863019572692162703, 0.0007817359430256216575 ),
 .UNSPECIFIED. ) ;
#14406=ORIENTED_EDGE ( 'NONE', *, *, #79507, .F. ) ;
#14408=CARTESIAN_POINT ( 'NONE',  ( 17.77707378248384629, -10.61292498521070549, 33.66303323003028680 ) ) ;
#14409=CARTESIAN_POINT ( 'NONE',  ( 17.07692307692307665, -2.721908614388771852, 31.22303859784724978 ) ) ;
#14410=FACE_BOUND ( 'NONE', #13720, .T. ) ;
#14411=DIRECTION ( 'NONE',  ( -0.000000000000000000, 0.9848077530122085754, -0.1736481776669273613 ) ) ;
#14412=FACE_OUTER_BOUND ( 'NONE', #12225, .T. ) ;
#14413=CARTESIAN_POINT ( 'NONE',  ( 4.403900465484468008, -12.41262288849542017, 30.68299917996395010 ) ) ;
#14414=CARTESIAN_POINT ( 'NONE',  ( 3.480823650682683734, -4.818054556918156983, 34.26375889529406749 ) ) ;
#14415=CARTESIAN_POINT ( 'NONE',  ( 5.076923076923075762, -10.51840700105979565, 33.73612834413961536 ) ) ;
#14416=CARTESIAN_POINT ( 'NONE',  ( -9.822867605921057788, -2.254533558242300284, 29.97296025877828285 ) ) ;
#14417=ORIENTED_EDGE ( 'NONE', *, *, #67038, .F. ) ;
#14418=CARTESIAN_POINT ( 'NONE',  ( 14.53070515178570332, -6.460100341425560444, 34.89618726649961644 ) ) ;
#14419=ORIENTED_EDGE ( 'NONE', *, *, #1622, .F. ) ;
#14420=ORIENTED_EDGE ( 'NONE', *, *, #4802, .T. ) ;
#14421=FACE_OUTER_BOUND ( 'NONE', #44277, .T. ) ;
#14422=CYLINDRICAL_SURFACE ( 'NONE', #33325, 0.2500000000000004996 ) ;
#14423=CARTESIAN_POINT ( 'NONE',  ( -9.561517251340744039, -12.35292014791297710, 31.75344720912887198 ) ) ;
#14424=LINE ( 'NONE', #41460, #7773 ) ;
#14425=CARTESIAN_POINT ( 'NONE',  ( 1.607628228708781082, -10.77377354290276301, 33.85451476688484718 ) ) ;
#14426=DIRECTION ( 'NONE',  ( -0.000000000000000000, 0.1736481776669307198, -0.9848077530122080203 ) ) ;
#14427=VERTEX_POINT ( 'NONE', #45162 ) ;
#14429=DIRECTION ( 'NONE',  ( -0.000000000000000000, 0.7660444431189791237, -0.6427876096865379196 ) ) ;
#14430=CARTESIAN_POINT ( 'NONE',  ( -14.55771553191376277, -10.18141759479407327, 34.26406193332782379 ) ) ;
#14431=CARTESIAN_POINT ( 'NONE',  ( -14.30769230769230660, -12.34228464037088635, 31.77849191805839268 ) ) ;
#14433=EDGE_CURVE ( 'NONE', #74452, #21962, #86623, .T. ) ;
#14434=CYLINDRICAL_SURFACE ( 'NONE', #22333, 0.2500000000000002220 ) ;
#14435=CARTESIAN_POINT ( 'NONE',  ( 14.30769230769231015, -8.120952969808772792, 34.71129190930000163 ) ) ;
#14436=ORIENTED_EDGE ( 'NONE', *, *, #70283, .T. ) ;
#14437=ORIENTED_EDGE ( 'NONE', *, *, #86872, .T. ) ;
#14440=ORIENTED_EDGE ( 'NONE', *, *, #51673, .T. ) ;
#14441=ADVANCED_FACE ( 'NONE', ( #84504 ), #1641, .F. ) ;
#14442=DIRECTION ( 'NONE',  ( -0.000000000000000000, 0.5000000000000011102, -0.8660254037844380415 ) ) ;
#14443=ADVANCED_FACE ( 'NONE', ( #29125 ), #70088, .F. ) ;
#14444=B_SPLINE_CURVE_WITH_KNOTS ( 'NONE', 3,
 ( #64946, #86582, #3252, #10908, #65832, #59084, #52324, #66288, #58190, #32066 ),
 .UNSPECIFIED., .F., .F.,
 ( 4, 2, 2, 2, 4 ),
 ( 0.0007817359430256294638, 0.0009771253907249948054, 0.001172514838424360255, 0.001367904286123725706, 0.001563293733823091156 ),
 .UNSPECIFIED. ) ;
#14445=EDGE_LOOP ( 'NONE', ( #87627, #52521 ) ) ;
#14446=DIRECTION ( 'NONE',  ( -0.000000000000000000, 0.5000000000000011102, -0.8660254037844381525 ) ) ;
#14448=CARTESIAN_POINT ( 'NONE',  ( 14.24242230713598900, -10.33852847137145048, 34.16647553114627556 ) ) ;
#14449=CARTESIAN_POINT ( 'NONE',  ( -17.32694630114453105, -9.356822207818511927, 34.66110646841856635 ) ) ;
#14450=CIRCLE ( 'NONE', #63356, 0.2500000000000002220 ) ;
#14451=CARTESIAN_POINT ( 'NONE',  ( -11.40793583669797506, -6.852161475712352789, 34.70806712695775786 ) ) ;
#14452=VERTEX_POINT ( 'NONE', #56581 ) ;
#14453=( GEOMETRIC_REPRESENTATION_CONTEXT ( 3 ) GLOBAL_UNCERTAINTY_ASSIGNED_CONTEXT ( ( #83445 ) ) GLOBAL_UNIT_ASSIGNED_CONTEXT ( ( #81033, #52199, #58960 ) ) REPRESENTATION_CONTEXT ( 'NONE', 'WORKASPACE' ) );
#14454=CARTESIAN_POINT ( 'NONE',  ( -11.28846153846011902, -7.500000000000154543, 35.00000000000007105 ) ) ;
#14455=DIRECTION ( 'NONE',  ( -0.000000000000000000, -0.9396926207859092051, -0.3420201433256662704 ) ) ;
#14456=ORIENTED_EDGE ( 'NONE', *, *, #23340, .F. ) ;
#14457=DIRECTION ( 'NONE',  ( -0.000000000000000000, 0.9848077530122085754, -0.1736481776669273613 ) ) ;
#14459=CARTESIAN_POINT ( 'NONE',  ( 17.29993442853592711, -11.24521262558773493, 33.06293181088029343 ) ) ;
#14460=B_SPLINE_CURVE_WITH_KNOTS ( 'NONE', 3,
 ( #18681, #18231, #19553, #88053, #47015, #12799, #45692, #69073, #76264, #7380 ),
 .UNSPECIFIED., .F., .F.,
 ( 4, 2, 2, 2, 4 ),
 ( 0.000000000000000000, 0.0001954339857564078538, 0.0003908679715128157077, 0.0005863019572692235344, 0.0007817359430256314154 ),
 .UNSPECIFIED. ) ;
#14461=CARTESIAN_POINT ( 'NONE',  ( -16.40384615384615330, -7.500000000000001776, 35.00000000000000000 ) ) ;
#14462=CARTESIAN_POINT ( 'NONE',  ( -18.00000000000012079, -11.06231777344772027, 33.60647404775119895 ) ) ;
#14463=CARTESIAN_POINT ( 'NONE',  ( 9.627037246346917598, -10.21337939537584383, 33.94971097300158647 ) ) ;
#14464=CARTESIAN_POINT ( 'NONE',  ( -12.52762187249434156, -12.37446782046654192, 30.86335684631486487 ) ) ;
#14467=LINE ( 'NONE', #41946, #11503 ) ;
#14468=CARTESIAN_POINT ( 'NONE',  ( -16.15384615384615330, -5.471508081941601098, 34.59228464037088457 ) ) ;
#14469=CARTESIAN_POINT ( 'NONE',  ( 7.912222197156284054, -2.538708090699994813, 30.37095296980875503 ) ) ;
#14471=EDGE_LOOP ( 'NONE', ( #75584, #20703, #21404, #58134 ) ) ;
#14472=CARTESIAN_POINT ( 'NONE',  ( 18.00000000000000000, -3.886160181151819604, 36.00935417666054406 ) ) ;
#14473=CARTESIAN_POINT ( 'NONE',  ( 10.61538461538461675, -1.129524287112498415, 32.06866353760679544 ) ) ;
#14474=CARTESIAN_POINT ( 'NONE',  ( 1.319344938654610777, -9.442884908240170461, 34.35708131394840592 ) ) ;
#14475=CARTESIAN_POINT ( 'NONE',  ( -0.5916864312701604067, -11.04286588640298561, 33.62463336215343901 ) ) ;
#14476=ORIENTED_EDGE ( 'NONE', *, *, #9004, .T. ) ;
#14477=ADVANCED_FACE ( 'NONE', ( #38416 ), #84069, .F. ) ;
#14478=CARTESIAN_POINT ( 'NONE',  ( -12.21159294319032362, -9.272278438253398036, 34.42582936511637115 ) ) ;
#14479=CARTESIAN_POINT ( 'NONE',  ( -14.55766903863466055, -2.779195860258146578, 31.39871582349836032 ) ) ;
#14480=CARTESIAN_POINT ( 'NONE',  ( 7.596177115211492747, -9.943427161483782584, 34.11278801902876978 ) ) ;
#14482=CARTESIAN_POINT ( 'NONE',  ( -2.307692307692305711, -12.29105614889573062, 35.45975837776705220 ) ) ;
#14483=ORIENTED_EDGE ( 'NONE', *, *, #30452, .F. ) ;
#14484=CYLINDRICAL_SURFACE ( 'NONE', #70204, 0.2500000000000009437 ) ;
#14485=CARTESIAN_POINT ( 'NONE',  ( 5.010840697562940704, -5.471508081941601986, 34.59228464037088457 ) ) ;
#14486=ORIENTED_EDGE ( 'NONE', *, *, #19290, .T. ) ;
#14487=CARTESIAN_POINT ( 'NONE',  ( -17.93474486048716088, -10.33852847137154463, 34.16647553114620450 ) ) ;
#14488=CARTESIAN_POINT ( 'NONE',  ( 17.07692307692307665, -10.67929555188718282, 33.92786785259544047 ) ) ;
#14489=CARTESIAN_POINT ( 'NONE',  ( -11.78846153846153832, -7.500000000000001776, 34.75000000000000000 ) ) ;
#14491=CARTESIAN_POINT ( 'NONE',  ( 18.00000000000000000, -12.34228464037088635, 31.77849191805839268 ) ) ;
#14493=EDGE_LOOP ( 'NONE', ( #70951, #75931, #37434, #43302 ) ) ;
#14494=FACE_BOUND ( 'NONE', #41863, .T. ) ;
#14495=ORIENTED_EDGE ( 'NONE', *, *, #14290, .T. ) ;
#14496=CARTESIAN_POINT ( 'NONE',  ( -11.53846153846153655, -13.04860791097971706, 34.73218667398347037 ) ) ;
#14497=VECTOR ( 'NONE', #24927, 1000.000000000000227 ) ;
#14498=VECTOR ( 'NONE', #5469, 1000.000000000000114 ) ;
#14499=EDGE_CURVE ( 'NONE', #86398, #50071, #16039, .T. ) ;
#14500=CARTESIAN_POINT ( 'NONE',  ( 4.153846153846154188, -11.69971097300155272, 32.46337939537588113 ) ) ;
#14502=CARTESIAN_POINT ( 'NONE',  ( 7.173022441425064066, -10.05730279482229683, 34.04704008940765902 ) ) ;
#14503=EDGE_CURVE ( 'NONE', #328, #10043, #13952, .T. ) ;
#14504=VECTOR ( 'NONE', #69280, 1000.000000000000227 ) ;
#14505=VERTEX_POINT ( 'NONE', #51910 ) ;
#14506=VERTEX_POINT ( 'NONE', #79407 ) ;
#14507=CARTESIAN_POINT ( 'NONE',  ( -5.999999999999998224, -13.95598074871891292, 31.83374038241031911 ) ) ;
#14508=ORIENTED_EDGE ( 'NONE', *, *, #62276, .F. ) ;
#14511=ADVANCED_FACE ( 'NONE', ( #76406 ), #15155, .F. ) ;
#14512=CARTESIAN_POINT ( 'NONE',  ( 15.23076923076910916, -3.643525952248795718, 33.31231777344771672 ) ) ;
#14513=CARTESIAN_POINT ( 'NONE',  ( 1.449870955891411795, -3.835265460703683349, 33.15142922261929925 ) ) ;
#14514=CARTESIAN_POINT ( 'NONE',  ( 13.38461538461526423, -11.67786785259630911, 32.92929555188603530 ) ) ;
#14515=B_SPLINE_CURVE_WITH_KNOTS ( 'NONE', 3,
 ( #70290, #51302, #78808, #56767, #30619, #9039, #43694, #8597, #50010, #85576 ),
 .UNSPECIFIED., .F., .F.,
 ( 4, 2, 2, 2, 4 ),
 ( 0.0007817359430256295722, 0.0009771253907249976244, 0.001172514838424365460, 0.001367904286123733729, 0.001563293733823094625 ),
 .UNSPECIFIED. ) ;
#14516=CARTESIAN_POINT ( 'NONE',  ( -1.134615384615320410, -7.434744429011176159, 34.75000000000000711 ) ) ;
#14517=EDGE_CURVE ( 'NONE', #83778, #20800, #69644, .T. ) ;
#14518=DIRECTION ( 'NONE',  ( -0.000000000000000000, -0.6427876096865404731, -0.7660444431189770143 ) ) ;
#14519=CARTESIAN_POINT ( 'NONE',  ( -6.923076923076922462, -12.10708131394839349, 31.69288490824020244 ) ) ;
#14520=CARTESIAN_POINT ( 'NONE',  ( -5.300408020647027207, -3.754499324213721234, 33.06261337010820256 ) ) ;
#14521=ORIENTED_EDGE ( 'NONE', *, *, #30993, .T. ) ;
#14522=EDGE_CURVE ( 'NONE', #9579, #67514, #46503, .T. ) ;
#14523=ORIENTED_EDGE ( 'NONE', *, *, #48667, .F. ) ;
#14524=ORIENTED_EDGE ( 'NONE', *, *, #5651, .T. ) ;
#14525=CARTESIAN_POINT ( 'NONE',  ( -3.903900635498012139, -10.05730279482229506, 34.04704008940765902 ) ) ;
#14526=CARTESIAN_POINT ( 'NONE',  ( 1.450683735617824821, -5.557115091759786019, 34.35708131394839882 ) ) ;
#14527=CARTESIAN_POINT ( 'NONE',  ( 1.515405825582338828, -11.37503395064541678, 33.29242100308974983 ) ) ;
#14528=B_SPLINE_CURVE_WITH_KNOTS ( 'NONE', 3,
 ( #49359, #55220, #68295, #41275, #69621, #7928, #42607, #21438, #48453, #48908 ),
 .UNSPECIFIED., .F., .F.,
 ( 4, 2, 2, 2, 4 ),
 ( 0.0007817246256747507503, 0.0009771112852218957062, 0.001172497944769040771, 0.001367884604316185835, 0.001563271263863330682 ),
 .UNSPECIFIED. ) ;
#14529=AXIS2_PLACEMENT_3D ( 'NONE', #57013, #77730, #56135 ) ;
#14530=CARTESIAN_POINT ( 'NONE',  ( -11.53846153846165912, -2.625532179533778709, 30.86335684631627174 ) ) ;
#14531=CARTESIAN_POINT ( 'NONE',  ( -6.700297381808511865, -3.755027918224367767, 33.06320215134714857 ) ) ;
#14532=FACE_BOUND ( 'NONE', #45594, .T. ) ;
#14533=LINE ( 'NONE', #27602, #48956 ) ;
#14534=ORIENTED_EDGE ( 'NONE', *, *, #83665, .T. ) ;
#14535=EDGE_CURVE ( 'NONE', #4865, #49069, #44085, .T. ) ;
#14536=CARTESIAN_POINT ( 'NONE',  ( 17.14299142792551578, -10.51840700105979565, 33.73612834413962247 ) ) ;
#14537=DIRECTION ( 'NONE',  ( 0.000000000000000000, 0.3420201433256641055, -0.9396926207859100932 ) ) ;
#14538=CYLINDRICAL_SURFACE ( 'NONE', #59090, 0.2500000000000009437 ) ;
#14539=DIRECTION ( 'NONE',  ( -0.000000000000000000, -0.5000000000000009992, -0.8660254037844380415 ) ) ;
#14541=ORIENTED_EDGE ( 'NONE', *, *, #69225, .T. ) ;
#14542=CARTESIAN_POINT ( 'NONE',  ( 6.250054419913455561, -10.82426656108011720, 33.81400080652039009 ) ) ;
#14543=ORIENTED_EDGE ( 'NONE', *, *, #58469, .T. ) ;
#14544=FACE_BOUND ( 'NONE', #44483, .T. ) ;
#14545=CARTESIAN_POINT ( 'NONE',  ( 9.692307692307572609, -6.026961402154118019, 34.52809138561165270 ) ) ;
#14549=VERTEX_POINT ( 'NONE', #46058 ) ;
#14550=CARTESIAN_POINT ( 'NONE',  ( 11.60452887181161508, -10.67929555188718282, 33.92786785259544757 ) ) ;
#14551=CARTESIAN_POINT ( 'NONE',  ( -5.750054590621955342, -9.357781135181031829, 34.66075350412533851 ) ) ;
#14552=CARTESIAN_POINT ( 'NONE',  ( 8.703960768674447124, -2.379036618887870436, 30.90682066428147934 ) ) ;
#14553=CARTESIAN_POINT ( 'NONE',  ( -5.076923076923075762, -5.471508081941601098, 34.59228464037088457 ) ) ;
#14554=EDGE_LOOP ( 'NONE', ( #5949, #58963 ) ) ;
#14555=CARTESIAN_POINT ( 'NONE',  ( 13.13459214732242408, -5.851115903089112003, 34.47074536777953568 ) ) ;
#14556=VERTEX_POINT ( 'NONE', #25344 ) ;
#14557=CARTESIAN_POINT ( 'NONE',  ( 16.22001276043779328, -7.250054591869668386, 34.99404684341514127 ) ) ;
#14558=ORIENTED_EDGE ( 'NONE', *, *, #49505, .T. ) ;
#14559=CARTESIAN_POINT ( 'NONE',  ( 7.780070435197965040, -10.51840700105979387, 33.73612834413961536 ) ) ;
#14560=CARTESIAN_POINT ( 'NONE',  ( -4.403822884788506364, -2.779195860258147022, 31.39871582349836743 ) ) ;
#14561=CARTESIAN_POINT ( 'NONE',  ( 11.53846153846153832, -2.900454961884010974, 35.62045528018868623 ) ) ;
#14562=CARTESIAN_POINT ( 'NONE',  ( 12.46153846153846168, -6.435427911321262684, 35.78748833219616898 ) ) ;
#14563=LINE ( 'NONE', #42049, #40928 ) ;
#14564=CARTESIAN_POINT ( 'NONE',  ( 13.60762673622823726, -5.667800583137506010, 34.40243808032445827 ) ) ;
#14565=CARTESIAN_POINT ( 'NONE',  ( 16.15384615384603251, -6.026961402154118908, 34.52809138561165270 ) ) ;
#14566=DIRECTION ( 'NONE',  ( 0.000000000000000000, 0.9396926207859126468, -0.3420201433256571111 ) ) ;
#14568=ORIENTED_EDGE ( 'NONE', *, *, #53864, .T. ) ;
#14569=DIRECTION ( 'NONE',  ( 0.000000000000000000, 0.4999999999999960032, -0.8660254037844410391 ) ) ;
#14570=EDGE_LOOP ( 'NONE', ( #18554, #1138, #14825, #61797 ) ) ;
#14573=EDGE_LOOP ( 'NONE', ( #48585, #21832, #32728, #52759 ) ) ;
#14574=CARTESIAN_POINT ( 'NONE',  ( -8.546451100252703270, -6.717445702608402236, 34.94155399931962336 ) ) ;
#14575=ORIENTED_EDGE ( 'NONE', *, *, #28153, .F. ) ;
#14576=CARTESIAN_POINT ( 'NONE',  ( -13.38461538461538325, -1.466349020453238561, 30.81389545987213907 ) ) ;
#14578=CARTESIAN_POINT ( 'NONE',  ( -8.069638770718176701, -8.539481045369596401, 34.89627647299170832 ) ) ;
#14579=CARTESIAN_POINT ( 'NONE',  ( 3.100077764101672795, -8.147922237126337563, 34.70805685702651999 ) ) ;
#14580=VECTOR ( 'NONE', #70943, 1000.000000000000227 ) ;
#14581=CYLINDRICAL_SURFACE ( 'NONE', #81650, 0.2500000000000004996 ) ;
#14582=LINE ( 'NONE', #69523, #57457 ) ;
#14583=CARTESIAN_POINT ( 'NONE',  ( 12.33139125210024112, -10.88202310037935661, 33.43294751532457099 ) ) ;
#14584=CARTESIAN_POINT ( 'NONE',  ( -7.846153846153844924, -2.292212530054420494, 30.41441678777542634 ) ) ;
#14586=B_SPLINE_CURVE_WITH_KNOTS ( 'NONE', 3,
 ( #4316, #31800, #59258, #18280, #67357, #54268, #68244, #62354, #20493, #20929 ),
 .UNSPECIFIED., .F., .F.,
 ( 4, 2, 2, 2, 4 ),
 ( 0.000000000000000000, 0.0001954339857564065528, 0.0003908679715128131056, 0.0005863019572692196313, 0.0007817359430256262112 ),
 .UNSPECIFIED. ) ;
#14587=B_SPLINE_CURVE_WITH_KNOTS ( 'NONE', 3,
 ( #20081, #47544, #35364, #88127, #75034, #13322, #26399, #75463, #28616, #77237 ),
 .UNSPECIFIED., .F., .F.,
 ( 4, 2, 2, 2, 4 ),
 ( 0.0007817359430256327164, 0.0009771253907249995759, 0.001172514838424366327, 0.001367904286123733078, 0.001563293733823099829 ),
 .UNSPECIFIED. ) ;
#14588=EDGE_CURVE ( 'NONE', #9053, #68539, #64509, .T. ) ;
#14589=DIRECTION ( 'NONE',  ( 0.000000000000000000, 0.1736481776669267785, -0.9848077530122087975 ) ) ;
#14590=CARTESIAN_POINT ( 'NONE',  ( -17.01166793741023042, -11.06231777344670775, 33.60647404775212266 ) ) ;
#14591=CARTESIAN_POINT ( 'NONE',  ( 24.00000000000000000, 0.000000000000000000, 0.000000000000000000 ) ) ;
#14592=CARTESIAN_POINT ( 'NONE',  ( -13.51476335434707821, -10.31621877034669588, 34.18098118002070152 ) ) ;
#14593=EDGE_CURVE ( 'NONE', #31453, #46051, #28004, .T. ) ;
#14594=EDGE_CURVE ( 'NONE', #28534, #86900, #33438, .T. ) ;
#14595=ORIENTED_EDGE ( 'NONE', *, *, #3553, .F. ) ;
#14596=EDGE_LOOP ( 'NONE', ( #28698, #46000 ) ) ;
#14597=LINE ( 'NONE', #14151, #32779 ) ;
#14598=CARTESIAN_POINT ( 'NONE',  ( 0.5920638997721040520, -12.15418822224088657, 32.17964115625579069 ) ) ;
#14599=DIRECTION ( 'NONE',  ( 0.000000000000000000, 0.9848077530122072432, -0.1736481776669354937 ) ) ;
#14600=CARTESIAN_POINT ( 'NONE',  ( -11.31549863490005237, -7.369474270740069777, 34.74850911626239736 ) ) ;
#14601=ORIENTED_EDGE ( 'NONE', *, *, #42355, .T. ) ;
#14602=CARTESIAN_POINT ( 'NONE',  ( -0.4615384615384611200, -13.57706302396349152, 30.56769352161908060 ) ) ;
#14603=CARTESIAN_POINT ( 'NONE',  ( 10.61538461538461675, -13.75783147151868846, 33.36296068462461051 ) ) ;
#14605=AXIS2_PLACEMENT_3D ( 'NONE', #19178, #60597, #54723 ) ;
#14607=VERTEX_POINT ( 'NONE', #19035 ) ;
#14609=ORIENTED_EDGE ( 'NONE', *, *, #47267, .T. ) ;
#14610=CARTESIAN_POINT ( 'NONE',  ( 9.823099500132483897, -11.71459661697925903, 32.44059661609676937 ) ) ;
#14611=B_SPLINE_CURVE_WITH_KNOTS ( 'NONE', 3,
 ( #33716, #12124, #68382, #20205, #48101, #47219, #60738, #73827, #5359, #75155 ),
 .UNSPECIFIED., .F., .F.,
 ( 4, 2, 2, 2, 4 ),
 ( 0.000000000000000000, 0.0001954311564186866305, 0.0003908623128373732609, 0.0005862934692560598914, 0.0007817246256747465219 ),
 .UNSPECIFIED. ) ;
#14612=CARTESIAN_POINT ( 'NONE',  ( 15.23076923076923173, -3.322132147404559976, 32.92929555188717927 ) ) ;
#14614=B_SPLINE_CURVE_WITH_KNOTS ( 'NONE', 3,
 ( #75046, #12448, #52536, #81803, #74598, #18321, #81361, #60625, #80472, #73722 ),
 .UNSPECIFIED., .F., .F.,
 ( 4, 2, 2, 2, 4 ),
 ( 0.0007817246256747484735, 0.0009771112852218922368, 0.001172497944769036217, 0.001367884604316180197, 0.001563271263863323960 ),
 .UNSPECIFIED. ) ;
#14615=CARTESIAN_POINT ( 'NONE',  ( 3.230769230769108269, -8.656820664282941280, 34.87096338111179961 ) ) ;
#14616=B_SPLINE_CURVE_WITH_KNOTS ( 'NONE', 3,
 ( #62293, #55542, #48784, #76251, #14560, #69502, #7807, #62733, #24856, #57760 ),
 .UNSPECIFIED., .F., .F.,
 ( 4, 2, 2, 2, 4 ),
 ( 0.000000000000000000, 0.0001954339857564126514, 0.0003908679715128183098, 0.0005863019572692239681, 0.0007817359430256294638 ),
 .UNSPECIFIED. ) ;
#14617=CARTESIAN_POINT ( 'NONE',  ( 10.61538461538461675, -5.180354513474913603, 36.12317359536750416 ) ) ;
#14618=ADVANCED_FACE ( 'NONE', ( #74420 ), #68113, .F. ) ;
#14619=VERTEX_POINT ( 'NONE', #60899 ) ;
#14620=ORIENTED_EDGE ( 'NONE', *, *, #1872, .T. ) ;
#14622=ORIENTED_EDGE ( 'NONE', *, *, #87665, .T. ) ;
#14623=CARTESIAN_POINT ( 'NONE',  ( -10.83831157429145975, -12.38737895849757820, 31.66785238281580206 ) ) ;
#14624=CARTESIAN_POINT ( 'NONE',  ( -15.93083330975275658, -9.172514111537580561, 34.72667873470787470 ) ) ;
#14626=VECTOR ( 'NONE', #52961, 1000.000000000000000 ) ;
#14627=CARTESIAN_POINT ( 'NONE',  ( 6.923076923076802558, -2.892918686052165622, 31.69288490824153470 ) ) ;
#14629=CARTESIAN_POINT ( 'NONE',  ( -2.307692307692427391, -12.27809138561165270, 31.22303859784587132 ) ) ;
#14630=VERTEX_POINT ( 'NONE', #88403 ) ;
#14631=EDGE_LOOP ( 'NONE', ( #27880, #7567, #75202, #15760 ) ) ;
#14632=ORIENTED_EDGE ( 'NONE', *, *, #62582, .F. ) ;
#14633=CYLINDRICAL_SURFACE ( 'NONE', #48837, 0.2499999999999997502 ) ;
#14634=ORIENTED_EDGE ( 'NONE', *, *, #7601, .T. ) ;
#14635=CARTESIAN_POINT ( 'NONE',  ( -16.82686876528476105, -9.148310452688871663, 34.47095581063188519 ) ) ;
#14636=CARTESIAN_POINT ( 'NONE',  ( 14.53047197667037516, -4.989023458446560255, 34.36081565061822118 ) ) ;
#14639=EDGE_LOOP ( 'NONE', ( #22944, #891 ) ) ;
#14640=EDGE_CURVE ( 'NONE', #72902, #70346, #62038, .T. ) ;
#14641=B_SPLINE_CURVE_WITH_KNOTS ( 'NONE', 3,
 ( #67553, #41408, #21570, #20687, #68869, #13050, #61218, #20251, #55354, #76069 ),
 .UNSPECIFIED., .F., .F.,
 ( 4, 2, 2, 2, 4 ),
 ( 0.000000000000000000, 0.0001954311564186868473, 0.0003908623128373736946, 0.0005862934692560605419, 0.0007817246256747473893 ),
 .UNSPECIFIED. ) ;
#14643=B_SPLINE_CURVE_WITH_KNOTS ( 'NONE', 3,
 ( #75353, #68151, #60941, #6453, #46548, #6884, #33912, #34352, #19953, #41560 ),
 .UNSPECIFIED., .F., .F.,
 ( 4, 2, 2, 2, 4 ),
 ( 0.000000000000000000, 0.0001954339857564092362, 0.0003908679715128184724, 0.0005863019572692276544, 0.0007817359430256369448 ),
 .UNSPECIFIED. ) ;
#14644=CARTESIAN_POINT ( 'NONE',  ( -6.923076923076922462, -4.661471528628507777, 34.16647553114623292 ) ) ;
#14645=VERTEX_POINT ( 'NONE', #24891 ) ;
#14646=EDGE_CURVE ( 'NONE', #36124, #11535, #52362, .T. ) ;
#14647=FACE_BOUND ( 'NONE', #76795, .T. ) ;
#14648=CARTESIAN_POINT ( 'NONE',  ( 4.946232473812766983, -4.684245665217972032, 34.18127051446801090 ) ) ;
#14649=CARTESIAN_POINT ( 'NONE',  ( 8.069166690247241647, -5.582272713120729257, 34.63742843783360570 ) ) ;
#14651=CARTESIAN_POINT ( 'NONE',  ( 1.384615384615386802, -5.471508081941601098, 34.59228464037088457 ) ) ;
#14652=CARTESIAN_POINT ( 'NONE',  ( 8.703960768674448900, -12.16647553114622049, 32.15551576947930812 ) ) ;
#14654=CARTESIAN_POINT ( 'NONE',  ( 10.36540788444226635, -2.779195860258146578, 31.39871582349836032 ) ) ;
#14655=CARTESIAN_POINT ( 'NONE',  ( 0.7115927731767752729, -6.567000820036038355, 34.66262288849541306 ) ) ;
#14658=ADVANCED_FACE ( 'NONE', ( #1418 ), #21238, .F. ) ;
#14659=VECTOR ( 'NONE', #81243, 1000.000000000000227 ) ;
#14660=CARTESIAN_POINT ( 'NONE',  ( -11.53846153846153655, -12.34228464037088635, 31.77849191805839268 ) ) ;
#14661=CARTESIAN_POINT ( 'NONE',  ( 1.450683735617824599, -8.120952969808772792, 34.71129190929999453 ) ) ;
#14662=CARTESIAN_POINT ( 'NONE',  ( 16.28463796167094557, -8.999086150933472084, 34.52020707165672064 ) ) ;
#14663=CARTESIAN_POINT ( 'NONE',  ( 15.93091919493930675, -10.77366814457252175, 33.85459836347580875 ) ) ;
#14664=CARTESIAN_POINT ( 'NONE',  ( -15.00775787915638126, -11.76359900205217457, 32.36225158514719880 ) ) ;
#14665=FACE_BOUND ( 'NONE', #45855, .T. ) ;
#14666=CARTESIAN_POINT ( 'NONE',  ( -8.992096191434411523, -2.501496062324912284, 29.88072118266895671 ) ) ;
#14667=CARTESIAN_POINT ( 'NONE',  ( 11.28848480751918437, -12.41269422305637171, 30.68257228309993323 ) ) ;
#14668=CARTESIAN_POINT ( 'NONE',  ( 5.207448515156721136, -2.372941743896878286, 30.88044141588254377 ) ) ;
#14669=DIRECTION ( 'NONE',  ( -0.000000000000000000, -0.9848077530122085754, -0.1736481776669273613 ) ) ;
#14670=CARTESIAN_POINT ( 'NONE',  ( 9.692307692307570832, -3.083524468854526912, 32.58852847137268327 ) ) ;
#14671=EDGE_CURVE ( 'NONE', #34671, #68238, #69434, .T. ) ;
#14672=CARTESIAN_POINT ( 'NONE',  ( -18.00000000000000000, -9.780366693483671270, 34.19971097300155094 ) ) ;
#14674=EDGE_LOOP ( 'NONE', ( #12248, #9950 ) ) ;
#14675=CARTESIAN_POINT ( 'NONE',  ( -5.869209559033048862, -10.70102852606553157, 33.91149625220312913 ) ) ;
#14676=ORIENTED_EDGE ( 'NONE', *, *, #76201, .F. ) ;
#14677=CARTESIAN_POINT ( 'NONE',  ( -14.98071491913091613, -4.235687564193445276, 33.53795663066793509 ) ) ;
#14678=EDGE_CURVE ( 'NONE', #21592, #19635, #77081, .T. ) ;
#14679=EDGE_LOOP ( 'NONE', ( #20146, #39263 ) ) ;
#14680=CARTESIAN_POINT ( 'NONE',  ( -11.53846153846165912, -2.892918686052166066, 31.69288490824153470 ) ) ;
#14681=DIRECTION ( 'NONE',  ( -0.000000000000000000, -0.3420201433256694901, -0.9396926207859082059 ) ) ;
#14682=ORIENTED_EDGE ( 'NONE', *, *, #2696, .F. ) ;
#14683=CARTESIAN_POINT ( 'NONE',  ( -9.942307692307691624, -7.500000000000001776, 34.75000000000000000 ) ) ;
#14685=DIRECTION ( 'NONE',  ( -0.000000000000000000, 1.000000000000000000, 3.491481338843133355E-15 ) ) ;
#14686=CARTESIAN_POINT ( 'NONE',  ( -5.142193522883853340, -5.219633306516282545, 34.19971097300152252 ) ) ;
#14687=CARTESIAN_POINT ( 'NONE',  ( -5.207614543590634248, -12.38065189839062263, 30.83690757178629482 ) ) ;
#14688=CARTESIAN_POINT ( 'NONE',  ( 15.45419619263079802, -7.630147231320743018, 34.74852402298682819 ) ) ;
#14690=CARTESIAN_POINT ( 'NONE',  ( -17.07692307692307665, -1.629998284177014645, 34.34916445242399163 ) ) ;
#14692=CARTESIAN_POINT ( 'NONE',  ( -9.822999158975251888, -3.530157926970578952, 32.79014554554150607 ) ) ;
#14693=CARTESIAN_POINT ( 'NONE',  ( 10.74617642320940369, -11.18335022499818621, 33.13157742990016885 ) ) ;
#14694=ORIENTED_EDGE ( 'NONE', *, *, #30761, .T. ) ;
#14697=ADVANCED_FACE ( 'NONE', ( #62661 ), #63106, .F. ) ;
#14698=CARTESIAN_POINT ( 'NONE',  ( -14.24243673641628050, -10.90142922261932057, 33.41473453929631887 ) ) ;
#14699=CARTESIAN_POINT ( 'NONE',  ( 9.692307692307695177, -13.75783147151868846, 33.36296068462461051 ) ) ;
#14700=VECTOR ( 'NONE', #11284, 1000.000000000000227 ) ;
#14701=VERTEX_POINT ( 'NONE', #54578 ) ;
#14702=ADVANCED_FACE ( 'NONE', ( #34757 ), #41080, .F. ) ;
#14703=CARTESIAN_POINT ( 'NONE',  ( 14.55763782604045176, -2.587454068350148351, 30.68340429815432202 ) ) ;
#14704=CARTESIAN_POINT ( 'NONE',  ( 16.40390057375960708, -2.544122305571458575, 31.48381861865057729 ) ) ;
#14705=CARTESIAN_POINT ( 'NONE',  ( 12.46153846153846168, -2.900454961884010974, 35.62045528018868623 ) ) ;
#14707=CARTESIAN_POINT ( 'NONE',  ( 8.703960768674447124, -5.941354392334499579, 34.76329471203369792 ) ) ;
#14709=VECTOR ( 'NONE', #32653, 1000.000000000000227 ) ;
#14710=CYLINDRICAL_SURFACE ( 'NONE', #18415, 0.2500000000000009437 ) ;
#14711=EDGE_CURVE ( 'NONE', #70329, #30760, #88006, .T. ) ;
#14712=DIRECTION ( 'NONE',  ( 0.000000000000000000, 0.9848077530122072432, -0.1736481776669354937 ) ) ;
#14713=CARTESIAN_POINT ( 'NONE',  ( 10.36536139116315880, -12.68155406624981119, 30.59749803192733708 ) ) ;
#14714=B_SPLINE_CURVE_WITH_KNOTS ( 'NONE', 3,
 ( #66113, #11636, #38207, #52603, #30558, #79203, #79646, #59812, #87311, #65667 ),
 .UNSPECIFIED., .F., .F.,
 ( 4, 2, 2, 2, 4 ),
 ( 0.0007817359430256218744, 0.0009771253907249861318, 0.001172514838424350498, 0.001367904286123714864, 0.001563293733823079229 ),
 .UNSPECIFIED. ) ;
#14715=ADVANCED_FACE ( 'NONE', ( #28446 ), #42858, .F. ) ;
#14717=CARTESIAN_POINT ( 'NONE',  ( -0.2385271099256124627, -10.61302985866383963, 33.66295027996417843 ) ) ;
#14718=ORIENTED_EDGE ( 'NONE', *, *, #75899, .T. ) ;
#14720=ORIENTED_EDGE ( 'NONE', *, *, #64191, .F. ) ;
#14721=CARTESIAN_POINT ( 'NONE',  ( -13.63463862190834952, -3.711651800289232028, 33.01384336483936011 ) ) ;
#14722=DIRECTION ( 'NONE',  ( -0.000000000000000000, 0.6427876096865404731, -0.7660444431189771253 ) ) ;
#14725=EDGE_CURVE ( 'NONE', #8176, #47629, #49376, .T. ) ;
#14726=EDGE_LOOP ( 'NONE', ( #27511, #15472, #70161, #82127 ) ) ;
#14728=LINE ( 'NONE', #43078, #42029 ) ;
#14729=AXIS2_PLACEMENT_3D ( 'NONE', #52544, #25081, #5697 ) ;
#14730=VERTEX_POINT ( 'NONE', #82075 ) ;
#14731=EDGE_CURVE ( 'NONE', #54551, #79352, #61161, .T. ) ;
#14732=ORIENTED_EDGE ( 'NONE', *, *, #85858, .T. ) ;
#14733=ORIENTED_EDGE ( 'NONE', *, *, #62181, .T. ) ;
#14734=CARTESIAN_POINT ( 'NONE',  ( -16.15384615384615330, -1.466349020453238561, 30.81389545987213907 ) ) ;
#14735=ORIENTED_EDGE ( 'NONE', *, *, #28365, .T. ) ;
#14736=CARTESIAN_POINT ( 'NONE',  ( -0.4615384615385826339, -5.219633306517616589, 34.19971097300220464 ) ) ;
#14737=CARTESIAN_POINT ( 'NONE',  ( 6.250054419913457338, -2.544122305571457687, 31.48381861865059150 ) ) ;
#14738=CARTESIAN_POINT ( 'NONE',  ( -3.099977422944443450, -4.118422570099827595, 33.43335022499816489 ) ) ;
#14739=CARTESIAN_POINT ( 'NONE',  ( -4.853960173361592467, -7.369474270740069777, 34.74850911626239736 ) ) ;
#14740=B_SPLINE_CURVE_WITH_KNOTS ( 'NONE', 3,
 ( #28378, #77892, #44089, #58058, #44982, #38686, #85989, #2660, #51272, #65256 ),
 .UNSPECIFIED., .F., .F.,
 ( 4, 2, 2, 2, 4 ),
 ( 0.0007817246256747507503, 0.0009771112852218959231, 0.001172497944769040987, 0.001367884604316186052, 0.001563271263863331116 ),
 .UNSPECIFIED. ) ;
#14741=VERTEX_POINT ( 'NONE', #79300 ) ;
#14742=ORIENTED_EDGE ( 'NONE', *, *, #52006, .T. ) ;
#14743=B_SPLINE_CURVE_WITH_KNOTS ( 'NONE', 3,
 ( #61971, #13348, #1162, #68293, #48904, #13789, #721, #54771, #6597, #28185 ),
 .UNSPECIFIED., .F., .F.,
 ( 4, 2, 2, 2, 4 ),
 ( 0.000000000000000000, 0.0001954339857564071762, 0.0003908679715128143524, 0.0005863019572692215828, 0.0007817359430256287049 ),
 .UNSPECIFIED. ) ;
#14745=CARTESIAN_POINT ( 'NONE',  ( -2.176901866725355461, -3.338503747796865984, 32.95102852606552801 ) ) ;
#14746=CARTESIAN_POINT ( 'NONE',  ( -2.531177251416252272, -2.847400154188067578, 31.58180166144859768 ) ) ;
#14747=EDGE_LOOP ( 'NONE', ( #8582, #41860, #80788, #56384 ) ) ;
#14748=CYLINDRICAL_SURFACE ( 'NONE', #85318, 0.2500000000000002220 ) ;
#14749=CARTESIAN_POINT ( 'NONE',  ( 13.31936439445414422, -2.506253911140460922, 30.00000000000013856 ) ) ;
#14750=CARTESIAN_POINT ( 'NONE',  ( 5.999999999999880096, -6.026961402154118908, 34.52809138561165270 ) ) ;
#14751=ORIENTED_EDGE ( 'NONE', *, *, #25311, .F. ) ;
#14752=DIRECTION ( 'NONE',  ( -0.000000000000000000, -0.3420201433256694901, -0.9396926207859082059 ) ) ;
#14753=DIRECTION ( 'NONE',  ( -0.000000000000000000, -0.7660444431189791237, -0.6427876096865379196 ) ) ;
#14754=ORIENTED_EDGE ( 'NONE', *, *, #61565, .T. ) ;
#14755=FACE_BOUND ( 'NONE', #60244, .T. ) ;
#14757=CARTESIAN_POINT ( 'NONE',  ( -9.692307692307691624, -8.120952969808772792, 34.71129190930000163 ) ) ;
#14758=VECTOR ( 'NONE', #16339, 1000.000000000000000 ) ;
#14760=CARTESIAN_POINT ( 'NONE',  ( 18.22277966897806323, -3.020022701398814569, 32.48759521482552515 ) ) ;
#14761=CYLINDRICAL_SURFACE ( 'NONE', #6646, 0.2499999999999973355 ) ;
#14763=CARTESIAN_POINT ( 'NONE',  ( -17.07692307692307665, -12.78798330534102945, 29.74999999999997868 ) ) ;
#14764=CARTESIAN_POINT ( 'NONE',  ( 14.37375964104238513, -2.292212530054420494, 30.41441678777542990 ) ) ;
#14765=ORIENTED_EDGE ( 'NONE', *, *, #62702, .T. ) ;
#14766=CARTESIAN_POINT ( 'NONE',  ( -9.692307692307691624, -12.29105614889573062, 35.45975837776705220 ) ) ;
#14768=VERTEX_POINT ( 'NONE', #58124 ) ;
#14769=AXIS2_PLACEMENT_3D ( 'NONE', #11842, #32540, #74421 ) ;
#14770=EDGE_CURVE ( 'NONE', #43224, #29911, #44599, .T. ) ;
#14771=CARTESIAN_POINT ( 'NONE',  ( -9.692307692307691624, -1.242168528481310874, 33.36296068462461051 ) ) ;
#14773=ORIENTED_EDGE ( 'NONE', *, *, #59345, .F. ) ;
#14774=CARTESIAN_POINT ( 'NONE',  ( 2.307692307692186251, -8.656820664282941280, 34.87096338111179961 ) ) ;
#14775=CARTESIAN_POINT ( 'NONE',  ( 2.438217745925953750, -5.070358843744209310, 34.40418822224088302 ) ) ;
#14776=FACE_BOUND ( 'NONE', #56808, .T. ) ;
#14777=CARTESIAN_POINT ( 'NONE',  ( -2.307692307692427391, -6.879047030192662504, 34.71129190930017927 ) ) ;
#14778=DIRECTION ( 'NONE',  ( 1.000000000000000000, 0.000000000000000000, 0.000000000000000000 ) ) ;
#14779=CARTESIAN_POINT ( 'NONE',  ( -6.673131404728782634, -9.272278438253401589, 34.42582936511637826 ) ) ;
#14780=CARTESIAN_POINT ( 'NONE',  ( -15.48079246806219267, -9.271318131107980420, 34.42618302367067429 ) ) ;
#14781=CARTESIAN_POINT ( 'NONE',  ( -12.46153846153858247, -3.835265460704628371, 33.15142922262033665 ) ) ;
#14783=B_SPLINE_CURVE_WITH_KNOTS ( 'NONE', 3,
 ( #28385, #30594, #85112, #9884, #78336, #58066, #79239, #36481, #10335, #63935 ),
 .UNSPECIFIED., .F., .F.,
 ( 4, 2, 2, 2, 4 ),
 ( 0.0007817359430256360774, 0.0009771253907250041296, 0.001172514838424371965, 0.001367904286123740017, 0.001563293733823108069 ),
 .UNSPECIFIED. ) ;
#14784=EDGE_CURVE ( 'NONE', #54531, #64679, #7419, .T. ) ;
#14785=CARTESIAN_POINT ( 'NONE',  ( -14.30769230769242917, -5.941354392335915335, 34.76329471203413846 ) ) ;
#14787=ORIENTED_EDGE ( 'NONE', *, *, #52743, .F. ) ;
#14788=ORIENTED_EDGE ( 'NONE', *, *, #73192, .T. ) ;
#14789=B_SPLINE_CURVE_WITH_KNOTS ( 'NONE', 3,
 ( #47883, #61384, #34808, #75797, #76693, #27168, #82125, #28507, #28060, #14545 ),
 .UNSPECIFIED., .F., .F.,
 ( 4, 2, 2, 2, 4 ),
 ( 0.000000000000000000, 0.0001954339857564074473, 0.0003908679715128148945, 0.0005863019572692223418, 0.0007817359430256297891 ),
 .UNSPECIFIED. ) ;
#14791=CARTESIAN_POINT ( 'NONE',  ( -10.48459417441766561, -8.191423895709840863, 34.95447573519442130 ) ) ;
#14792=CARTESIAN_POINT ( 'NONE',  ( 14.53070515178570332, -9.172514111537584114, 34.72667873470787470 ) ) ;
#14793=CARTESIAN_POINT ( 'NONE',  ( -1.450698795571264021, -3.050289026998445951, 32.03036669348365706 ) ) ;
#14794=CARTESIAN_POINT ( 'NONE',  ( -3.903900744468109973, -2.986452184633680229, 32.43230066228895225 ) ) ;
#14796=CARTESIAN_POINT ( 'NONE',  ( -12.46153846153858424, -4.320704448113951379, 33.92786785259630022 ) ) ;
#14797=DIRECTION ( 'NONE',  ( 0.000000000000000000, 0.4999999999999960032, -0.8660254037844410391 ) ) ;
#14798=EDGE_CURVE ( 'NONE', #40731, #86110, #40765, .T. ) ;
#14800=CARTESIAN_POINT ( 'NONE',  ( 6.066067333350076751, -3.937682226553329556, 33.60647404775216529 ) ) ;
#14801=CARTESIAN_POINT ( 'NONE',  ( 14.30769230769231015, -2.249999999999998668, 29.75000000000001776 ) ) ;
#14802=CARTESIAN_POINT ( 'NONE',  ( -15.23076923076922995, -11.16473453929635440, 33.15142922261926373 ) ) ;
#14803=LINE ( 'NONE', #20227, #15232 ) ;
#14805=CARTESIAN_POINT ( 'NONE',  ( -5.869474561766359066, -11.66157788607254275, 32.95092075102925833 ) ) ;
#14806=CARTESIAN_POINT ( 'NONE',  ( 12.59232890250541281, -2.295524264805589354, 30.44142389570982488 ) ) ;
#14807=CARTESIAN_POINT ( 'NONE',  ( 12.68454981315130858, -2.758310577978208666, 31.33698337089302299 ) ) ;
#14808=ORIENTED_EDGE ( 'NONE', *, *, #48958, .T. ) ;
#14809=CARTESIAN_POINT ( 'NONE',  ( -14.53117725141625627, -3.754499324213721234, 33.06261337010820256 ) ) ;
#14810=CARTESIAN_POINT ( 'NONE',  ( 5.999999999999878320, -12.16647553114689728, 32.15551576947799362 ) ) ;
#14812=EDGE_CURVE ( 'NONE', #20155, #55155, #26705, .T. ) ;
#14813=CARTESIAN_POINT ( 'NONE',  ( -5.934744860487159102, -12.51329471203373700, 31.30864560766537963 ) ) ;
#14814=CARTESIAN_POINT ( 'NONE',  ( 17.01084069756293715, -11.35647404775217595, 33.31231777344666511 ) ) ;
#14815=VERTEX_POINT ( 'NONE', #23450 ) ;
#14816=CARTESIAN_POINT ( 'NONE',  ( -6.923076923077045919, -3.083524468854526912, 32.58852847137268327 ) ) ;
#14817=CARTESIAN_POINT ( 'NONE',  ( -14.55771554498526932, -12.22074536777954989, 31.39888409691088356 ) ) ;
#14819=CARTESIAN_POINT ( 'NONE',  ( 7.912222197156284054, -3.513871655860379306, 32.76840700105978499 ) ) ;
#14821=DIRECTION ( 'NONE',  ( -0.000000000000000000, -0.9848077530122085754, -0.1736481776669273613 ) ) ;
#14822=ORIENTED_EDGE ( 'NONE', *, *, #56224, .F. ) ;
#14823=LINE ( 'NONE', #21566, #69291 ) ;
#14825=ORIENTED_EDGE ( 'NONE', *, *, #47187, .F. ) ;
#14827=LINE ( 'NONE', #57566, #27873 ) ;
#14829=CARTESIAN_POINT ( 'NONE',  ( 9.823098133274644539, -6.369690395747422684, 34.87708834333098196 ) ) ;
#14830=ORIENTED_EDGE ( 'NONE', *, *, #41284, .T. ) ;
#14831=VERTEX_POINT ( 'NONE', #23016 ) ;
#14832=CARTESIAN_POINT ( 'NONE',  ( -6.673022503163470454, -8.346898887586323923, 34.93166121998716278 ) ) ;
#14833=VECTOR ( 'NONE', #29068, 1000.000000000000114 ) ;
#14835=CARTESIAN_POINT ( 'NONE',  ( -7.912236225513983534, -2.292212530054419606, 30.41441678777542634 ) ) ;
#14836=CARTESIAN_POINT ( 'NONE',  ( -1.384615384615505151, -2.625532179533778709, 30.86335684631627174 ) ) ;
#14837=CARTESIAN_POINT ( 'NONE',  ( -14.43783951713053249, -3.285722584762969856, 32.44110544564090759 ) ) ;
#14838=DIRECTION ( 'NONE',  ( 0.000000000000000000, 0.9396926207859126468, 0.3420201433256571111 ) ) ;
#14839=DIRECTION ( 'NONE',  ( 0.000000000000000000, 0.7660444431189807890, 0.6427876096865361433 ) ) ;
#14840=CARTESIAN_POINT ( 'NONE',  ( 0.3957850332251287018, -7.249945578846653582, 34.99404164642496795 ) ) ;
#14841=EDGE_CURVE ( 'NONE', #14278, #373, #51798, .T. ) ;
#14843=CARTESIAN_POINT ( 'NONE',  ( -17.07692307692307665, -6.386643153685126251, 34.62446782046654192 ) ) ;
#14844=EDGE_CURVE ( 'NONE', #81167, #64959, #39660, .T. ) ;
#14845=EDGE_CURVE ( 'NONE', #37064, #45937, #57251, .T. ) ;
#14846=VERTEX_POINT ( 'NONE', #84740 ) ;
#14847=ORIENTED_EDGE ( 'NONE', *, *, #31312, .T. ) ;
#14848=CARTESIAN_POINT ( 'NONE',  ( -2.307692307692428724, -2.379036618888197285, 30.90682066428292885 ) ) ;
#14849=EDGE_LOOP ( 'NONE', ( #33617, #5704, #67007, #60878 ) ) ;
#14852=ORIENTED_EDGE ( 'NONE', *, *, #72931, .T. ) ;
#14853=B_SPLINE_CURVE_WITH_KNOTS ( 'NONE', 3,
 ( #7565, #20194, #6669, #42681, #21509, #21059, #48091, #48986, #68815, #35025 ),
 .UNSPECIFIED., .F., .F.,
 ( 4, 2, 2, 2, 4 ),
 ( 0.000000000000000000, 0.0001954311564186868744, 0.0003908623128373737488, 0.0005862934692560606504, 0.0007817246256747474977 ),
 .UNSPECIFIED. ) ;
#14854=LINE ( 'NONE', #49517, #13341 ) ;
#14855=CARTESIAN_POINT ( 'NONE',  ( -8.769230769230892619, -12.70778746994576025, 30.41441678777401236 ) ) ;
#14856=ORIENTED_EDGE ( 'NONE', *, *, #29572, .T. ) ;
#14857=CARTESIAN_POINT ( 'NONE',  ( 14.30769230769231015, -13.87047571288749737, 32.06866353760679544 ) ) ;
#14858=AXIS2_PLACEMENT_3D ( 'NONE', #47189, #34124, #40894 ) ;
#14860=B_SPLINE_CURVE_WITH_KNOTS ( 'NONE', 3,
 ( #27388, #796, #20621, #55732, #83221, #21506, #48087, #75562, #48983, #76463 ),
 .UNSPECIFIED., .F., .F.,
 ( 4, 2, 2, 2, 4 ),
 ( 0.0007817246256747442451, 0.0009771112852218870326, 0.001172497944769029929, 0.001367884604316172825, 0.001563271263863315504 ),
 .UNSPECIFIED. ) ;
#14861=CYLINDRICAL_SURFACE ( 'NONE', #12840, 0.2500000000000009437 ) ;
#14863=VECTOR ( 'NONE', #76609, 1000.000000000000227 ) ;
#14865=ORIENTED_EDGE ( 'NONE', *, *, #37749, .F. ) ;
#14866=CARTESIAN_POINT ( 'NONE',  ( 5.326923076924511946, -7.500000000000155431, 34.75000000000007105 ) ) ;
#14867=CARTESIAN_POINT ( 'NONE',  ( -8.899378738962463231, -12.15440758774515473, 32.17923288041532004 ) ) ;
#14868=FACE_BOUND ( 'NONE', #35978, .T. ) ;
#14870=CARTESIAN_POINT ( 'NONE',  ( -17.93393164899756442, -12.10708131394839882, 31.69288490824020954 ) ) ;
#14871=CARTESIAN_POINT ( 'NONE',  ( 9.692307692307695177, -11.35647404775217417, 33.31231777344666511 ) ) ;
#14873=CARTESIAN_POINT ( 'NONE',  ( -17.20707104665477161, -8.630895178749536711, 34.87696386517710323 ) ) ;
#14874=CARTESIAN_POINT ( 'NONE',  ( -16.21992956480203318, -8.120952969808774569, 34.71129190930000163 ) ) ;
#14875=ORIENTED_EDGE ( 'NONE', *, *, #88572, .T. ) ;
#14876=DIRECTION ( 'NONE',  ( -0.000000000000000000, -0.1736481776669307198, -0.9848077530122080203 ) ) ;
#14877=VERTEX_POINT ( 'NONE', #53598 ) ;
#14878=ORIENTED_EDGE ( 'NONE', *, *, #78056, .F. ) ;
#14879=CARTESIAN_POINT ( 'NONE',  ( 7.716006636715624367, -6.852621066184267029, 34.70813303252209181 ) ) ;
#14880=CARTESIAN_POINT ( 'NONE',  ( 8.096208157792160520, -9.943054286541403997, 34.11300777759954883 ) ) ;
#14881=FACE_OUTER_BOUND ( 'NONE', #29484, .T. ) ;
#14882=B_SPLINE_CURVE_WITH_KNOTS ( 'NONE', 3,
 ( #3119, #45441, #50416, #77899, #78784, #65266, #52196, #57189, #22956, #23392 ),
 .UNSPECIFIED., .F., .F.,
 ( 4, 2, 2, 2, 4 ),
 ( 0.000000000000000000, 0.0001954311564186878502, 0.0003908623128373757004, 0.0005862934692560635777, 0.0007817246256747514008 ),
 .UNSPECIFIED. ) ;
#14883=FACE_OUTER_BOUND ( 'NONE', #78494, .T. ) ;
#14884=CARTESIAN_POINT ( 'NONE',  ( -12.39628332202562788, -2.657715359629131857, 31.77849191805844242 ) ) ;
#14886=VERTEX_POINT ( 'NONE', #47280 ) ;
#14887=CARTESIAN_POINT ( 'NONE',  ( 11.40831356872984514, -3.625366637846545892, 33.29286588640298561 ) ) ;
#14888=AXIS2_PLACEMENT_3D ( 'NONE', #87757, #25138, #17945 ) ;
#14889=CARTESIAN_POINT ( 'NONE',  ( -13.38461538461538325, -13.20930481340135110, 34.54067556320372745 ) ) ;
#14891=CARTESIAN_POINT ( 'NONE',  ( -8.519285359852730721, -2.589246495874658383, 31.60778113518102828 ) ) ;
#14892=CARTESIAN_POINT ( 'NONE',  ( 13.51514082284903040, -5.915461855592780260, 34.75538340440931506 ) ) ;
#14893=ORIENTED_EDGE ( 'NONE', *, *, #58929, .F. ) ;
#14894=CARTESIAN_POINT ( 'NONE',  ( 1.161130440891438020, -3.236172620538810385, 32.36188796281390267 ) ) ;
#14895=EDGE_LOOP ( 'NONE', ( #58995, #51491, #45157, #58694 ) ) ;
#14896=VECTOR ( 'NONE', #71728, 1000.000000000000000 ) ;
#14897=ORIENTED_EDGE ( 'NONE', *, *, #88519, .T. ) ;
#14898=CARTESIAN_POINT ( 'NONE',  ( -7.053224132515142131, -8.587444163452046197, 34.63053765926554206 ) ) ;
#14899=ORIENTED_EDGE ( 'NONE', *, *, #24855, .T. ) ;
#14900=CARTESIAN_POINT ( 'NONE',  ( -1.384615384615505151, -8.613356846316285953, 34.62446782046622218 ) ) ;
#14901=CARTESIAN_POINT ( 'NONE',  ( -12.33101275977490019, -6.852161475712352789, 34.70806712695775786 ) ) ;
#14902=CARTESIAN_POINT ( 'NONE',  ( -13.38461538461538325, -13.04860791097971706, 34.73218667398347037 ) ) ;
#14903=CARTESIAN_POINT ( 'NONE',  ( -17.30040800148741553, -12.69144148231606017, 30.53333754910549303 ) ) ;
#14904=CARTESIAN_POINT ( 'NONE',  ( -17.14300545628321260, -9.058645607665454236, 34.76329471203372634 ) ) ;
#14905=CARTESIAN_POINT ( 'NONE',  ( 12.23805351781451201, -10.11188796281391511, 34.01382737946119050 ) ) ;
#14907=DIRECTION ( 'NONE',  ( -0.000000000000000000, -0.7660444431189791237, -0.6427876096865379196 ) ) ;
#14908=DIRECTION ( 'NONE',  ( -1.000000000000000000, 0.000000000000000000, 0.000000000000000000 ) ) ;
#14909=ORIENTED_EDGE ( 'NONE', *, *, #37512, .T. ) ;
#14910=CARTESIAN_POINT ( 'NONE',  ( -3.453634652972869201, -2.501496062324912284, 29.88072118266895671 ) ) ;
#14911=CARTESIAN_POINT ( 'NONE',  ( -8.704085988511138794, -7.750023224968867197, 34.99404313364389907 ) ) ;
#14912=CARTESIAN_POINT ( 'NONE',  ( 17.07692307692307665, -11.16473453929635440, 33.15142922261926373 ) ) ;
#14913=CARTESIAN_POINT ( 'NONE',  ( -18.00000000000012079, -11.94971097300221352, 32.03036669348236387 ) ) ;
#14914=CARTESIAN_POINT ( 'NONE',  ( -2.307692307692428724, -2.379036618888197285, 30.90682066428292885 ) ) ;
#14915=CARTESIAN_POINT ( 'NONE',  ( 9.692307692307572609, -10.21337939537710326, 33.94971097300076224 ) ) ;
#14916=CARTESIAN_POINT ( 'NONE',  ( -3.296522659082562257, -7.249945578846654470, 34.99404164642496795 ) ) ;
#14918=VERTEX_POINT ( 'NONE', #66671 ) ;
#14919=LINE ( 'NONE', #84271, #50298 ) ;
#14920=CARTESIAN_POINT ( 'NONE',  ( 12.52760579488853665, -4.661471528628508665, 34.16647553114624003 ) ) ;
#14921=ADVANCED_FACE ( 'NONE', ( #74771 ), #87405, .F. ) ;
#14922=CARTESIAN_POINT ( 'NONE',  ( 6.923076923076924238, -13.75783147151868846, 33.36296068462461051 ) ) ;
#14923=CARTESIAN_POINT ( 'NONE',  ( -3.007756386675836335, -10.77377354290276301, 33.85451476688484718 ) ) ;
#14925=LINE ( 'NONE', #76617, #44158 ) ;
#14926=CARTESIAN_POINT ( 'NONE',  ( -5.076923076923075762, -8.810774026931790459, 35.74407628777942847 ) ) ;
#14928=B_SPLINE_CURVE_WITH_KNOTS ( 'NONE', 3,
 ( #79310, #38768, #4531, #86980, #86067, #18939, #12185, #24801, #72992, #52270 ),
 .UNSPECIFIED., .F., .F.,
 ( 4, 2, 2, 2, 4 ),
 ( 0.0007817246256747511840, 0.0009771112852218952725, 0.001172497944769039470, 0.001367884604316183667, 0.001563271263863327864 ),
 .UNSPECIFIED. ) ;
#14929=CARTESIAN_POINT ( 'NONE',  ( 14.30769230769218758, -3.300289026999228881, 32.46337939537708905 ) ) ;
#14930=ORIENTED_EDGE ( 'NONE', *, *, #46203, .T. ) ;
#14931=CARTESIAN_POINT ( 'NONE',  ( -15.36146069743678844, -2.729777683071817229, 31.24903638046269450 ) ) ;
#14932=EDGE_CURVE ( 'NONE', #27837, #6801, #23508, .T. ) ;
#14933=CARTESIAN_POINT ( 'NONE',  ( -8.638440328263817136, -5.496552790871120031, 34.60292014791297532 ) ) ;
#14934=CARTESIAN_POINT ( 'NONE',  ( -6.923076923076922462, -6.681629849574314051, 35.83090037661290239 ) ) ;
#14936=CARTESIAN_POINT ( 'NONE',  ( -8.834480701004853387, -2.255955759149247619, 30.00000000000013856 ) ) ;
#14938=CARTESIAN_POINT ( 'NONE',  ( 12.71148387091650278, -12.45601412856602686, 31.48342859153981621 ) ) ;
#14939=CARTESIAN_POINT ( 'NONE',  ( -4.087677012883497163, -7.250054483168843156, 34.74374881642865631 ) ) ;
#14940=ORIENTED_EDGE ( 'NONE', *, *, #42281, .T. ) ;
#14941=CARTESIAN_POINT ( 'NONE',  ( -17.74994558008654622, -10.06805714834173848, 34.32951233291982618 ) ) ;
#14942=CARTESIAN_POINT ( 'NONE',  ( -8.992156986746916658, -2.554751324335734708, 30.48935550225260727 ) ) ;
#14943=CARTESIAN_POINT ( 'NONE',  ( -10.86540785267757947, -5.851115903089112003, 34.47074536777953568 ) ) ;
#14944=CARTESIAN_POINT ( 'NONE',  ( -11.28840711854808632, -5.642605341092957971, 34.66089969410670335 ) ) ;
#14946=EDGE_CURVE ( 'NONE', #36760, #15767, #25240, .T. ) ;
#14947=EDGE_CURVE ( 'NONE', #76455, #47929, #4065, .T. ) ;
#14948=VERTEX_POINT ( 'NONE', #33337 ) ;
#14950=FACE_BOUND ( 'NONE', #70822, .T. ) ;
#14951=ORIENTED_EDGE ( 'NONE', *, *, #11749, .T. ) ;
#14952=CARTESIAN_POINT ( 'NONE',  ( 8.769230769230647482, -3.835265460704628371, 33.15142922262033665 ) ) ;
#14953=B_SPLINE_CURVE_WITH_KNOTS ( 'NONE', 3,
 ( #65294, #4945, #23851, #32409, #86939, #24302, #4029, #25207, #79713, #65733 ),
 .UNSPECIFIED., .F., .F.,
 ( 4, 2, 2, 2, 4 ),
 ( 0.0007817359430256294638, 0.0009771253907249941549, 0.001172514838424358954, 0.001367904286123723754, 0.001563293733823095492 ),
 .UNSPECIFIED. ) ;
#14954=VECTOR ( 'NONE', #4632, 1000.000000000000227 ) ;
#14955=AXIS2_PLACEMENT_3D ( 'NONE', #38872, #87076, #78958 ) ;
#14957=CARTESIAN_POINT ( 'NONE',  ( 4.219101725122177626, -11.94971097300157403, 32.03036669348361443 ) ) ;
#14958=CARTESIAN_POINT ( 'NONE',  ( 17.99999999999987566, -5.941354392335915335, 34.76329471203413846 ) ) ;
#14960=B_SPLINE_CURVE_WITH_KNOTS ( 'NONE', 3,
 ( #60121, #5628, #66443, #17821, #88081, #33102, #31326, #18713, #74095, #38984 ),
 .UNSPECIFIED., .F., .F.,
 ( 4, 2, 2, 2, 4 ),
 ( 0.000000000000000000, 0.0001954339857564077183, 0.0003908679715128154366, 0.0005863019572692231007, 0.0007817359430256308733 ),
 .UNSPECIFIED. ) ;
#14961=ORIENTED_EDGE ( 'NONE', *, *, #68822, .T. ) ;
#14963=ORIENTED_EDGE ( 'NONE', *, *, #14194, .F. ) ;
#14966=CARTESIAN_POINT ( 'NONE',  ( -4.946131269098290595, -4.809403383903225304, 33.96459661697924304 ) ) ;
#14968=CYLINDRICAL_SURFACE ( 'NONE', #58740, 0.2500000000000012212 ) ;
#14970=CARTESIAN_POINT ( 'NONE',  ( 13.16113044089144068, -10.81261337010820256, 33.49550067578627477 ) ) ;
#14971=CARTESIAN_POINT ( 'NONE',  ( -15.10024379253558635, -3.625058011473228703, 33.29252011169590020 ) ) ;
#14972=CARTESIAN_POINT ( 'NONE',  ( 14.43821800945587519, -6.852161475712352789, 34.70806712695775786 ) ) ;
#14974=VERTEX_POINT ( 'NONE', #38757 ) ;
#14975=VERTEX_POINT ( 'NONE', #31551 ) ;
#14976=ORIENTED_EDGE ( 'NONE', *, *, #54694, .T. ) ;
#14977=CARTESIAN_POINT ( 'NONE',  ( 3.930919194939304084, -2.889293201056495786, 32.26117774369186009 ) ) ;
#14979=DIRECTION ( 'NONE',  ( -0.000000000000000000, 0.9396926207859093161, -0.3420201433256663259 ) ) ;
#14980=CARTESIAN_POINT ( 'NONE',  ( 10.39245765647776309, -2.308479472611653094, 30.53278059502174457 ) ) ;
#14981=CARTESIAN_POINT ( 'NONE',  ( 1.634560793993430128, -12.45601412856602686, 31.48342859153981621 ) ) ;
#14982=CARTESIAN_POINT ( 'NONE',  ( -3.454254174493177842, -11.41268669641500466, 32.86336882939237825 ) ) ;
#14983=FACE_BOUND ( 'NONE', #7505, .T. ) ;
#14984=FACE_OUTER_BOUND ( 'NONE', #31157, .T. ) ;
#14985=VERTEX_POINT ( 'NONE', #53144 ) ;
#14986=CARTESIAN_POINT ( 'NONE',  ( -2.980714919130916130, -2.564540009722895419, 30.55348353981670684 ) ) ;
#14987=B_SPLINE_CURVE_WITH_KNOTS ( 'NONE', 3,
 ( #87938, #75279, #60423, #53669, #13568, #74842, #13131, #88812, #60869, #81156 ),
 .UNSPECIFIED., .F., .F.,
 ( 4, 2, 2, 2, 4 ),
 ( 0.000000000000000000, 0.0001954339881912774612, 0.0003908679763825549224, 0.0005863019645738323836, 0.0007817359527651098448 ),
 .UNSPECIFIED. ) ;
#14988=CARTESIAN_POINT ( 'NONE',  ( -0.2387589202700517999, -9.332535724633405749, 34.40230450496446224 ) ) ;
#14989=DIRECTION ( 'NONE',  ( -0.000000000000000000, -0.000000000000000000, -1.000000000000000000 ) ) ;
#14990=CARTESIAN_POINT ( 'NONE',  ( 7.173022332454967120, -9.357781135181031829, 34.66075350412533851 ) ) ;
#14991=B_SPLINE_CURVE_WITH_KNOTS ( 'NONE', 3,
 ( #58642, #23966, #2365, #23526, #86136, #78919, #50555, #29858, #30296, #78035 ),
 .UNSPECIFIED., .F., .F.,
 ( 4, 2, 2, 2, 4 ),
 ( 0.000000000000000000, 0.0001954311564186861968, 0.0003908623128373723936, 0.0005862934692560585904, 0.0007817246256747447872 ),
 .UNSPECIFIED. ) ;
#14992=EDGE_LOOP ( 'NONE', ( #79168, #62362, #7758, #75762 ) ) ;
#14993=CARTESIAN_POINT ( 'NONE',  ( 4.946775107191379028, -12.70455904226513866, 30.44083106164009322 ) ) ;
#14994=ORIENTED_EDGE ( 'NONE', *, *, #87105, .T. ) ;
#14995=FACE_BOUND ( 'NONE', #2207, .T. ) ;
#14997=CARTESIAN_POINT ( 'NONE',  ( 17.01165263096229907, -11.94971097300153140, 32.03036669348370680 ) ) ;
#14998=CARTESIAN_POINT ( 'NONE',  ( 14.08476609017615644, -11.76352882383564769, 32.36236540154569497 ) ) ;
#15000=CARTESIAN_POINT ( 'NONE',  ( 5.326868595271218254, -3.202959910592335202, 32.30730279482227019 ) ) ;
#15001=CARTESIAN_POINT ( 'NONE',  ( -3.296851610129365451, -2.292212530054419606, 30.41441678777542634 ) ) ;
#15002=CARTESIAN_POINT ( 'NONE',  ( -3.230769230769351186, -2.892918686052166066, 31.69288490824153470 ) ) ;
#15003=CARTESIAN_POINT ( 'NONE',  ( -6.989160334032800570, -10.51840700105979387, 33.73612834413961536 ) ) ;
#15004=VERTEX_POINT ( 'NONE', #88307 ) ;
#15005=ADVANCED_FACE ( 'NONE', ( #32887 ), #79747, .F. ) ;
#15006=CARTESIAN_POINT ( 'NONE',  ( 12.68491394731088029, -2.251407671071270489, 29.88021292934942963 ) ) ;
#15007=EDGE_LOOP ( 'NONE', ( #41503, #21897 ) ) ;
#15009=EDGE_LOOP ( 'NONE', ( #2370, #38166, #11519, #34566 ) ) ;
#15010=CARTESIAN_POINT ( 'NONE',  ( 9.562160482869471068, -3.817052484675422797, 33.13202310037935661 ) ) ;
#15011=CARTESIAN_POINT ( 'NONE',  ( -8.769230769230768274, -11.11383981884818262, 36.00935417666054406 ) ) ;
#15012=CARTESIAN_POINT ( 'NONE',  ( -18.00000000000012079, -4.320704448113953156, 33.92786785259630022 ) ) ;
#15013=CARTESIAN_POINT ( 'NONE',  ( -20.74999999999999645, -4.499999999999999112, 29.75000000000000355 ) ) ;
#15014=CARTESIAN_POINT ( 'NONE',  ( -12.71151520558705172, -10.82459398097509329, 33.81372124010185587 ) ) ;
#15015=CARTESIAN_POINT ( 'NONE',  ( -12.46153846153858424, -12.70778746994576025, 30.41441678777401236 ) ) ;
#15016=VECTOR ( 'NONE', #14077, 1000.000000000000227 ) ;
#15017=LINE ( 'NONE', #4484, #10132 ) ;
#15018=CYLINDRICAL_SURFACE ( 'NONE', #32051, 0.2499999999999986955 ) ;
#15020=ORIENTED_EDGE ( 'NONE', *, *, #3404, .T. ) ;
#15021=CARTESIAN_POINT ( 'NONE',  ( -16.37677311275300340, -4.762599654559227957, 34.23009711892697737 ) ) ;
#15022=EDGE_LOOP ( 'NONE', ( #17666, #24776 ) ) ;
#15023=ADVANCED_FACE ( 'NONE', ( #72982 ), #46840, .F. ) ;
#15024=ORIENTED_EDGE ( 'NONE', *, *, #88565, .F. ) ;
#15025=CARTESIAN_POINT ( 'NONE',  ( 11.78851585009985570, -11.79725096376909654, 32.30694842903959341 ) ) ;
#15026=ORIENTED_EDGE ( 'NONE', *, *, #26087, .T. ) ;
#15027=LINE ( 'NONE', #2813, #38330 ) ;
#15029=CARTESIAN_POINT ( 'NONE',  ( 7.623287583090747610, -2.251424796025575770, 29.88072029997477586 ) ) ;
#15030=B_SPLINE_CURVE_WITH_KNOTS ( 'NONE', 3,
 ( #38673, #38228, #31472, #17967, #31015, #50831, #66137, #4441, #58937, #10759 ),
 .UNSPECIFIED., .F., .F.,
 ( 4, 2, 2, 2, 4 ),
 ( 0.000000000000000000, 0.0001954311564186871184, 0.0003908623128373742367, 0.0005862934692560614093, 0.0007817246256747484735 ),
 .UNSPECIFIED. ) ;
#15031=CYLINDRICAL_SURFACE ( 'NONE', #28659, 0.2499999999999973355 ) ;
#15032=FACE_OUTER_BOUND ( 'NONE', #43571, .T. ) ;
#15033=CARTESIAN_POINT ( 'NONE',  ( 8.769230769230647482, -11.48612834414049644, 32.76840700105863391 ) ) ;
#15034=CARTESIAN_POINT ( 'NONE',  ( -16.15384615384627409, -5.219633306517616589, 34.19971097300220464 ) ) ;
#15035=DIRECTION ( 'NONE',  ( 0.000000000000000000, 0.9848077530122072432, -0.1736481776669354937 ) ) ;
#15036=B_SPLINE_CURVE_WITH_KNOTS ( 'NONE', 3,
 ( #83609, #35398, #56561, #77713, #76383, #43489, #57436, #22331, #49796, #77271 ),
 .UNSPECIFIED., .F., .F.,
 ( 4, 2, 2, 2, 4 ),
 ( 0.000000000000000000, 0.0001954339857564079894, 0.0003908679715128159787, 0.0005863019572692239681, 0.0007817359430256319575 ),
 .UNSPECIFIED. ) ;
#15037=CARTESIAN_POINT ( 'NONE',  ( 10.48469314871705826, -2.541943142973491554, 30.39792223712631980 ) ) ;
#15038=CARTESIAN_POINT ( 'NONE',  ( 15.16549923021291058, -9.528491918058357157, 34.59228464037090589 ) ) ;
#15039=EDGE_CURVE ( 'NONE', #74721, #44439, #55736, .T. ) ;
#15040=CARTESIAN_POINT ( 'NONE',  ( 5.749976775778542049, -11.56360843649121861, 33.07473185843129926 ) ) ;
#15041=CARTESIAN_POINT ( 'NONE',  ( 7.716005876422148191, -2.373036134822904319, 30.88089517874951540 ) ) ;
#15042=EDGE_CURVE ( 'NONE', #44439, #82483, #19817, .T. ) ;
#15043=ORIENTED_EDGE ( 'NONE', *, *, #31470, .T. ) ;
#15044=EDGE_LOOP ( 'NONE', ( #69875, #29148, #27198, #55212 ) ) ;
#15045=CARTESIAN_POINT ( 'NONE',  ( 12.71148387091650278, -2.589246495874658383, 31.60778113518102828 ) ) ;
#15046=CARTESIAN_POINT ( 'NONE',  ( 1.384615384615386802, -13.04860791097971706, 34.73218667398347037 ) ) ;
#15047=LINE ( 'NONE', #22676, #68525 ) ;
#15049=ORIENTED_EDGE ( 'NONE', *, *, #78326, .F. ) ;
#15050=CARTESIAN_POINT ( 'NONE',  ( 13.38461538461538680, -13.20930481340135110, 34.54067556320372745 ) ) ;
#15051=CARTESIAN_POINT ( 'NONE',  ( -10.83831157429145975, -12.64616026154729411, 30.79003144601914244 ) ) ;
#15053=CARTESIAN_POINT ( 'NONE',  ( -12.33074665371367651, -10.54018710029568595, 33.71981072465678864 ) ) ;
#15054=ADVANCED_FACE ( 'NONE', ( #86973 ), #67566, .F. ) ;
#15055=ORIENTED_EDGE ( 'NONE', *, *, #40666, .T. ) ;
#15056=DIRECTION ( 'NONE',  ( -0.000000000000000000, -0.000000000000000000, -1.000000000000000000 ) ) ;
#15057=EDGE_CURVE ( 'NONE', #47954, #39557, #11735, .T. ) ;
#15058=EDGE_LOOP ( 'NONE', ( #66437, #50891 ) ) ;
#15059=CARTESIAN_POINT ( 'NONE',  ( 10.61538461538449418, -2.657715359629662544, 31.77849191805970364 ) ) ;
#15061=ADVANCED_FACE ( 'NONE', ( #69336 ), #82416, .F. ) ;
#15062=DIRECTION ( 'NONE',  ( 0.000000000000000000, 0.000000000000000000, 1.000000000000000000 ) ) ;
#15063=ADVANCED_FACE ( 'NONE', ( #13939 ), #61673, .F. ) ;
#15064=CARTESIAN_POINT ( 'NONE',  ( 14.30769230769231015, -8.564572088678739092, 35.78748833219616898 ) ) ;
#15065=CARTESIAN_POINT ( 'NONE',  ( -17.74994558008654622, -12.41089969410671046, 31.60739465890703670 ) ) ;
#15067=EDGE_LOOP ( 'NONE', ( #30794, #47678 ) ) ;
#15068=B_SPLINE_CURVE_WITH_KNOTS ( 'NONE', 3,
 ( #59064, #73032, #72581, #87457, #59956, #25289 ),
 .UNSPECIFIED., .F., .F.,
 ( 4, 2, 4 ),
 ( 0.0003909512603273637287, 0.0005862562993131885522, 0.0007815613382990133215 ),
 .UNSPECIFIED. ) ;
#15069=VERTEX_POINT ( 'NONE', #28335 ) ;
#15070=ORIENTED_EDGE ( 'NONE', *, *, #69016, .F. ) ;
#15071=CARTESIAN_POINT ( 'NONE',  ( 13.25392391794782654, -3.062553014421049546, 32.05460306192773601 ) ) ;
#15072=CARTESIAN_POINT ( 'NONE',  ( 8.096153846153846700, -7.500000000000001776, 35.04278698407183867 ) ) ;
#15073=CYLINDRICAL_SURFACE ( 'NONE', #35062, 0.2499999999999994726 ) ;
#15074=AXIS2_PLACEMENT_3D ( 'NONE', #6091, #6535, #33567 ) ;
#15075=CIRCLE ( 'NONE', #61104, 0.2500000000000002220 ) ;
#15077=CARTESIAN_POINT ( 'NONE',  ( 5.076923076922953193, -12.51329471203414379, 31.30864560766407578 ) ) ;
#15078=CARTESIAN_POINT ( 'NONE',  ( 14.53070365930516061, -9.886259254753566594, 34.14407573483972413 ) ) ;
#15079=ORIENTED_EDGE ( 'NONE', *, *, #33984, .T. ) ;
#15080=VERTEX_POINT ( 'NONE', #6311 ) ;
#15082=CARTESIAN_POINT ( 'NONE',  ( 12.46153846153846168, -8.120952969808772792, 34.71129190930000163 ) ) ;
#15083=EDGE_LOOP ( 'NONE', ( #77363, #12966, #32102, #67008 ) ) ;
#15084=CARTESIAN_POINT ( 'NONE',  ( -16.94613126909829148, -8.999086150933472084, 34.52020707165672064 ) ) ;
#15085=CARTESIAN_POINT ( 'NONE',  ( 14.43821774592595197, -5.070358843744210198, 34.40418822224088302 ) ) ;
#15087=EDGE_CURVE ( 'NONE', #43722, #17581, #20698, .T. ) ;
#15088=CARTESIAN_POINT ( 'NONE',  ( -10.86540785267757947, -11.86270091957321249, 32.19358267280087915 ) ) ;
#15089=ORIENTED_EDGE ( 'NONE', *, *, #21148, .T. ) ;
#15090=ORIENTED_EDGE ( 'NONE', *, *, #51389, .T. ) ;
#15091=DIRECTION ( 'NONE',  ( 0.000000000000000000, 0.4999999999999960032, -0.8660254037844410391 ) ) ;
#15092=EDGE_LOOP ( 'NONE', ( #24598, #73476, #63875, #42129 ) ) ;
#15093=FACE_BOUND ( 'NONE', #33832, .T. ) ;
#15094=CARTESIAN_POINT ( 'NONE',  ( -1.134615384615383915, -2.499999999999998668, 29.75000000000000355 ) ) ;
#15095=EDGE_CURVE ( 'NONE', #39467, #16561, #56856, .T. ) ;
#15096=CARTESIAN_POINT ( 'NONE',  ( -3.230769230769352962, -2.379036618888197285, 30.90682066428292885 ) ) ;
#15097=ORIENTED_EDGE ( 'NONE', *, *, #88574, .T. ) ;
#15099=CARTESIAN_POINT ( 'NONE',  ( 3.296837581771669523, -3.050289026998446840, 32.03036669348366416 ) ) ;
#15100=PLANE ( 'NONE',  #34933 ) ;
#15101=CARTESIAN_POINT ( 'NONE',  ( -15.36091644020745051, -6.852621066184266141, 34.70813303252209181 ) ) ;
#15102=CARTESIAN_POINT ( 'NONE',  ( -7.846153846153844924, -9.905515769479276145, 34.41647553114623292 ) ) ;
#15103=ORIENTED_EDGE ( 'NONE', *, *, #77646, .T. ) ;
#15104=EDGE_CURVE ( 'NONE', #69549, #32791, #30997, .T. ) ;
#15106=CARTESIAN_POINT ( 'NONE',  ( -12.23852561744506851, -2.308499170217967134, 30.53291367094873721 ) ) ;
#15107=CARTESIAN_POINT ( 'NONE',  ( -7.715362038329057981, -6.413143153341454017, 34.63066358083362672 ) ) ;
#15108=CARTESIAN_POINT ( 'NONE',  ( 16.15384615384603251, -9.442884908241554243, 34.35708131394783038 ) ) ;
#15109=CARTESIAN_POINT ( 'NONE',  ( -0.6850233861027930082, -4.988325925672468131, 34.36044203135681130 ) ) ;
#15110=LINE ( 'NONE', #84024, #57361 ) ;
#15111=FACE_BOUND ( 'NONE', #75161, .T. ) ;
#15112=FACE_OUTER_BOUND ( 'NONE', #20416, .T. ) ;
#15114=CARTESIAN_POINT ( 'NONE',  ( 5.142990410273153401, -2.292212530054420494, 30.41441678777542990 ) ) ;
#15115=CARTESIAN_POINT ( 'NONE',  ( -3.361459833879539172, -2.845849958028613624, 32.17971566917920967 ) ) ;
#15117=CARTESIAN_POINT ( 'NONE',  ( -5.142193077479396912, -12.51329471203370325, 31.30864560766548976 ) ) ;
#15118=B_SPLINE_CURVE_WITH_KNOTS ( 'NONE', 3,
 ( #39347, #46533, #25369, #32134, #58702, #52385, #79874, #86202, #74012, #5999 ),
 .UNSPECIFIED., .F., .F.,
 ( 4, 2, 2, 2, 4 ),
 ( 0.000000000000000000, 0.0001954339857564072033, 0.0003908679715128144066, 0.0005863019572692215828, 0.0007817359430256288133 ),
 .UNSPECIFIED. ) ;
#15120=ORIENTED_EDGE ( 'NONE', *, *, #53473, .F. ) ;
#15121=CARTESIAN_POINT ( 'NONE',  ( -3.230769230769229949, -1.951392089020283160, 34.73218667398347748 ) ) ;
#15122=ORIENTED_EDGE ( 'NONE', *, *, #86699, .F. ) ;
#15123=CARTESIAN_POINT ( 'NONE',  ( -18.00000000000012079, -5.094484230521992174, 34.41647553114689373 ) ) ;
#15124=ADVANCED_FACE ( 'NONE', ( #42315 ), #41867, .F. ) ;
#15125=B_SPLINE_CURVE_WITH_KNOTS ( 'NONE', 3,
 ( #17443, #38151, #15676, #43575, #58865, #70612, #22423, #8920, #36387, #39946 ),
 .UNSPECIFIED., .F., .F.,
 ( 4, 2, 2, 2, 4 ),
 ( 0.0007817246256747463051, 0.0009771112852218898515, 0.001172497944769033181, 0.001367884604316176728, 0.001563271263863320274 ),
 .UNSPECIFIED. ) ;
#15126=ORIENTED_EDGE ( 'NONE', *, *, #18055, .F. ) ;
#15127=DIRECTION ( 'NONE',  ( -0.000000000000000000, -0.9396926207859092051, -0.3420201433256662704 ) ) ;
#15128=CARTESIAN_POINT ( 'NONE',  ( -18.00000000000000000, -2.538708090699994813, 30.37095296980875858 ) ) ;
#15129=ORIENTED_EDGE ( 'NONE', *, *, #27888, .F. ) ;
#15132=LINE ( 'NONE', #15575, #76032 ) ;
#15134=CARTESIAN_POINT ( 'NONE',  ( 4.088575707885377497, -9.442884908240170461, 34.35708131394840592 ) ) ;
#15135=CARTESIAN_POINT ( 'NONE',  ( 4.153846153846030731, -4.320704448113951379, 33.92786785259630022 ) ) ;
#15136=CARTESIAN_POINT ( 'NONE',  ( -14.30769230769230660, -12.29105614889573062, 35.45975837776705220 ) ) ;
#15137=FACE_OUTER_BOUND ( 'NONE', #84143, .T. ) ;
#15138=CARTESIAN_POINT ( 'NONE',  ( -9.692307692307691624, -3.050289026998446396, 32.03036669348365706 ) ) ;
#15142=CYLINDRICAL_SURFACE ( 'NONE', #29048, 0.2499999999999986955 ) ;
#15143=DIRECTION ( 'NONE',  ( -0.000000000000000000, -0.8660254037844397068, -0.4999999999999978906 ) ) ;
#15145=B_SPLINE_CURVE_WITH_KNOTS ( 'NONE', 3,
 ( #88497, #26769, #20009, #61871, #14140, #47920, #47472, #88941, #82167, #74970 ),
 .UNSPECIFIED., .F., .F.,
 ( 4, 2, 2, 2, 4 ),
 ( 0.0007817246256747524850, 0.0009771112852218972241, 0.001172497944769042072, 0.001367884604316186702, 0.001563271263863331550 ),
 .UNSPECIFIED. ) ;
#15147=EDGE_LOOP ( 'NONE', ( #32677, #75757 ) ) ;
#15148=LINE ( 'NONE', #82283, #14013 ) ;
#15149=CARTESIAN_POINT ( 'NONE',  ( -11.40766973063675493, -8.147973898785416225, 34.70805048591653730 ) ) ;
#15150=CARTESIAN_POINT ( 'NONE',  ( 9.915087233576103998, -6.760870238392817200, 34.69528174975672385 ) ) ;
#15151=CARTESIAN_POINT ( 'NONE',  ( 8.546303810323914618, -5.582147617184174848, 34.63737895849758530 ) ) ;
#15152=VECTOR ( 'NONE', #86071, 1000.000000000000114 ) ;
#15153=CARTESIAN_POINT ( 'NONE',  ( -3.165513659493206067, -5.219633306516380244, 34.19971097300157936 ) ) ;
#15154=CARTESIAN_POINT ( 'NONE',  ( -18.00000000000000000, -13.72934399251292170, 33.34651343095209342 ) ) ;
#15155=CYLINDRICAL_SURFACE ( 'NONE', #8827, 0.2500000000000008882 ) ;
#15159=B_SPLINE_CURVE_WITH_KNOTS ( 'NONE', 3,
 ( #29730, #56748, #57192, #28388, #29292, #56310 ),
 .UNSPECIFIED., .F., .F.,
 ( 4, 2, 4 ),
 ( 0.000000000000000000, 0.0001954784845028895374, 0.0003909569690057790748 ),
 .UNSPECIFIED. ) ;
#15160=EDGE_CURVE ( 'NONE', #43765, #83533, #81977, .T. ) ;
#15161=ORIENTED_EDGE ( 'NONE', *, *, #3228, .F. ) ;
#15162=CARTESIAN_POINT ( 'NONE',  ( 5.326977388561390470, -11.79725096376909299, 32.30694842903960762 ) ) ;
#15163=CARTESIAN_POINT ( 'NONE',  ( 3.230769230769231726, -8.164416787775445883, 34.95778746994557906 ) ) ;
#15164=CARTESIAN_POINT ( 'NONE',  ( -17.07692307692307665, -13.20930481340135110, 34.54067556320372745 ) ) ;
#15165=EDGE_CURVE ( 'NONE', #82297, #11287, #84798, .T. ) ;
#15166=DIRECTION ( 'NONE',  ( 0.000000000000000000, 0.9848077530122072432, 0.1736481776669354937 ) ) ;
#15167=DIRECTION ( 'NONE',  ( -0.000000000000000000, 0.1736481776669307198, -0.9848077530122080203 ) ) ;
#15168=VECTOR ( 'NONE', #4024, 1000.000000000000227 ) ;
#15171=ORIENTED_EDGE ( 'NONE', *, *, #62116, .T. ) ;
#15172=VERTEX_POINT ( 'NONE', #61482 ) ;
#15174=CARTESIAN_POINT ( 'NONE',  ( 8.703960768674448900, -12.51329471203370325, 31.30864560766548976 ) ) ;
#15175=ORIENTED_EDGE ( 'NONE', *, *, #86295, .T. ) ;
#15176=CARTESIAN_POINT ( 'NONE',  ( 4.284637961670941131, -5.582136614379148654, 34.36778462344220486 ) ) ;
#15177=EDGE_CURVE ( 'NONE', #4656, #48169, #39038, .T. ) ;
#15178=CARTESIAN_POINT ( 'NONE',  ( 10.61538461538461675, -12.78798330534102945, 29.74999999999997868 ) ) ;
#15179=EDGE_CURVE ( 'NONE', #44047, #56065, #48249, .T. ) ;
#15180=DIRECTION ( 'NONE',  ( -0.000000000000000000, 0.7660444431189791237, -0.6427876096865379196 ) ) ;
#15181=CARTESIAN_POINT ( 'NONE',  ( -7.173076923076929567, -2.499999999999999556, 29.81609845454692120 ) ) ;
#15182=EDGE_LOOP ( 'NONE', ( #87064, #6690 ) ) ;
#15183=ORIENTED_EDGE ( 'NONE', *, *, #41889, .T. ) ;
#15184=B_SPLINE_CURVE_WITH_KNOTS ( 'NONE', 3,
 ( #23821, #16199, #37343, #85108, #36905, #15766, #50412, #64368, #85992, #29723 ),
 .UNSPECIFIED., .F., .F.,
 ( 4, 2, 2, 2, 4 ),
 ( 0.000000000000000000, 0.0001954339857564097783, 0.0003908679715128195566, 0.0005863019572692293891, 0.0007817359430256391132 ),
 .UNSPECIFIED. ) ;
#15185=ORIENTED_EDGE ( 'NONE', *, *, #61798, .F. ) ;
#15188=ORIENTED_EDGE ( 'NONE', *, *, #83244, .T. ) ;
#15189=B_SPLINE_CURVE_WITH_KNOTS ( 'NONE', 3,
 ( #58708, #32141, #59600, #31240, #78535, #24033 ),
 .UNSPECIFIED., .F., .F.,
 ( 4, 2, 4 ),
 ( 4.220987180333913997E-17, 0.0001954756301637163962, 0.0003909512603273906169 ),
 .UNSPECIFIED. ) ;
#15191=CARTESIAN_POINT ( 'NONE',  ( -13.38461538461538325, -8.164416787775445883, 34.95778746994557906 ) ) ;
#15192=B_SPLINE_CURVE_WITH_KNOTS ( 'NONE', 3,
 ( #3032, #77375, #16555, #71057, #84596, #2589, #9802, #77812, #23747, #22866 ),
 .UNSPECIFIED., .F., .F.,
 ( 4, 2, 2, 2, 4 ),
 ( 0.0007817246256747514008, 0.0009771112852218952725, 0.001172497944769039253, 0.001367884604316183233, 0.001563271263863327213 ),
 .UNSPECIFIED. ) ;
#15193=ADVANCED_FACE ( 'NONE', ( #67809 ), #53847, .F. ) ;
#15194=VECTOR ( 'NONE', #9092, 1000.000000000000114 ) ;
#15195=CARTESIAN_POINT ( 'NONE',  ( -3.100243529005668019, -10.19071101563364401, 33.96452234770658407 ) ) ;
#15196=ORIENTED_EDGE ( 'NONE', *, *, #31049, .T. ) ;
#15197=CARTESIAN_POINT ( 'NONE',  ( -11.40766973063674961, -4.809403383903225304, 33.96459661697924304 ) ) ;
#15198=CARTESIAN_POINT ( 'NONE',  ( 15.16549923021291235, -2.657715359629088780, 31.77849191805832874 ) ) ;
#15199=VERTEX_POINT ( 'NONE', #75892 ) ;
#15200=FACE_BOUND ( 'NONE', #40681, .T. ) ;
#15201=ADVANCED_FACE ( 'NONE', ( #19615 ), #40343, .F. ) ;
#15202=LINE ( 'NONE', #23268, #29815 ) ;
#15203=LINE ( 'NONE', #63371, #9721 ) ;
#15204=DIRECTION ( 'NONE',  ( 0.000000000000000000, 0.000000000000000000, -1.000000000000000000 ) ) ;
#15205=LINE ( 'NONE', #42239, #46064 ) ;
#15206=DIRECTION ( 'NONE',  ( -0.000000000000000000, -0.3420201433256694346, -0.9396926207859080948 ) ) ;
#15207=CARTESIAN_POINT ( 'NONE',  ( -4.153846153846152411, -2.721908614388771852, 31.22303859784724978 ) ) ;
#15209=ORIENTED_EDGE ( 'NONE', *, *, #5551, .F. ) ;
#15210=LINE ( 'NONE', #62485, #7254 ) ;
#15212=CARTESIAN_POINT ( 'NONE',  ( 4.826899852701619587, -4.175268141568689195, 33.81360843649122216 ) ) ;
#15213=ORIENTED_EDGE ( 'NONE', *, *, #13397, .T. ) ;
#15214=ADVANCED_FACE ( 'NONE', ( #27701 ), #68689, .F. ) ;
#15216=CARTESIAN_POINT ( 'NONE',  ( -3.903791842207838592, -2.564540009722896752, 30.55348353981670684 ) ) ;
#15218=CARTESIAN_POINT ( 'NONE',  ( 17.74997676270703550, -5.851115903089112003, 34.47074536777953568 ) ) ;
#15219=CARTESIAN_POINT ( 'NONE',  ( 4.376857505459002873, -9.886259254753566594, 34.14407573483972413 ) ) ;
#15220=FACE_BOUND ( 'NONE', #56434, .T. ) ;
#15221=ADVANCED_FACE ( 'NONE', ( #82216 ), #69135, .F. ) ;
#15222=CARTESIAN_POINT ( 'NONE',  ( 13.31853300525524908, -2.292212530054419606, 30.41441678777542634 ) ) ;
#15223=CARTESIAN_POINT ( 'NONE',  ( 17.07692307692295586, -9.442884908241554243, 34.35708131394783038 ) ) ;
#15224=CARTESIAN_POINT ( 'NONE',  ( 12.46153846153833911, -12.51329471203414379, 31.30864560766407578 ) ) ;
#15225=CARTESIAN_POINT ( 'NONE',  ( -4.826977667545033768, -10.18230066228895758, 34.26354781536631577 ) ) ;
#15226=CARTESIAN_POINT ( 'NONE',  ( -14.08426590877751927, -7.630147987733840509, 34.99859428049665411 ) ) ;
#15227=CARTESIAN_POINT ( 'NONE',  ( -18.00000000000000000, -4.786620604624112651, 33.94971097300155094 ) ) ;
#15229=ORIENTED_EDGE ( 'NONE', *, *, #69846, .T. ) ;
#15230=ORIENTED_EDGE ( 'NONE', *, *, #39982, .F. ) ;
#15231=CARTESIAN_POINT ( 'NONE',  ( 15.93091919493930320, -9.172386477786394821, 34.72672124145550043 ) ) ;
#15232=VECTOR ( 'NONE', #47690, 1000.000000000000114 ) ;
#15233=CARTESIAN_POINT ( 'NONE',  ( -0.5268089074992367005, -2.892918686051582977, 31.69288490824016691 ) ) ;
#15234=CARTESIAN_POINT ( 'NONE',  ( -9.627052121031665521, -9.442884908240273489, 34.35708131394835618 ) ) ;
#15236=CARTESIAN_POINT ( 'NONE',  ( 3.230769230769110045, -11.48612834414049644, 32.76840700105863391 ) ) ;
#15238=EDGE_CURVE ( 'NONE', #20998, #1316, #22399, .T. ) ;
#15239=CARTESIAN_POINT ( 'NONE',  ( 10.61538461538461675, -9.905515769479276145, 34.41647553114623292 ) ) ;
#15240=DIRECTION ( 'NONE',  ( 0.000000000000000000, 0.000000000000000000, 1.000000000000000000 ) ) ;
#15241=VECTOR ( 'NONE', #20891, 1000.000000000000227 ) ;
#15242=EDGE_CURVE ( 'NONE', #2963, #22454, #11734, .T. ) ;
#15243=CARTESIAN_POINT ( 'NONE',  ( -17.29984929443922681, -4.887634598454295265, 34.01352882383564946 ) ) ;
#15244=CARTESIAN_POINT ( 'NONE',  ( -3.100243792535587684, -12.15418822224088657, 32.17964115625579069 ) ) ;
#15245=CARTESIAN_POINT ( 'NONE',  ( 5.206968239757855166, -2.504778602574660340, 29.97347330155780298 ) ) ;
#15247=CYLINDRICAL_SURFACE ( 'NONE', #80754, 0.2499999999999986955 ) ;
#15250=CARTESIAN_POINT ( 'NONE',  ( 12.23805353697412812, -4.225889041578353655, 33.85425143139329407 ) ) ;
#15251=CYLINDRICAL_SURFACE ( 'NONE', #86345, 0.2499999999999994726 ) ;
#15254=CARTESIAN_POINT ( 'NONE',  ( 1.384615384615386802, -2.900454961884010974, 35.62045528018868623 ) ) ;
#15255=ORIENTED_EDGE ( 'NONE', *, *, #83797, .F. ) ;
#15257=PLANE ( 'NONE',  #3771 ) ;
#15258=ORIENTED_EDGE ( 'NONE', *, *, #8557, .T. ) ;
#15259=CARTESIAN_POINT ( 'NONE',  ( 7.053868730901711182, -3.530189275343204702, 32.79018710029569661 ) ) ;
#15260=CARTESIAN_POINT ( 'NONE',  ( -5.010854725920637520, -9.780366693483667717, 34.19971097300155805 ) ) ;
#15261=ORIENTED_EDGE ( 'NONE', *, *, #241, .F. ) ;
#15262=CARTESIAN_POINT ( 'NONE',  ( -13.13456107297707121, -2.564540009722895419, 30.55348353981670684 ) ) ;
#15263=CARTESIAN_POINT ( 'NONE',  ( 13.25446741488369362, -9.504002272028875709, 34.60269587691767867 ) ) ;
#15264=ORIENTED_EDGE ( 'NONE', *, *, #73825, .F. ) ;
#15265=CARTESIAN_POINT ( 'NONE',  ( -12.71151520558705172, -2.318417181685855422, 30.59732222474233865 ) ) ;
#15266=LINE ( 'NONE', #49921, #39454 ) ;
#15268=EDGE_LOOP ( 'NONE', ( #39437, #61320 ) ) ;
#15269=EDGE_LOOP ( 'NONE', ( #11929, #547, #67051, #45816 ) ) ;
#15270=CARTESIAN_POINT ( 'NONE',  ( 3.007284306204898172, -3.019605429927184836, 32.48692288466676814 ) ) ;
#15272=EDGE_LOOP ( 'NONE', ( #77203, #57840 ) ) ;
#15273=CARTESIAN_POINT ( 'NONE',  ( -13.38461538461538325, -13.20930481340135110, 34.54067556320372745 ) ) ;
#15274=DIRECTION ( 'NONE',  ( -0.000000000000000000, 0.1736481776669307198, -0.9848077530122080203 ) ) ;
#15275=EDGE_CURVE ( 'NONE', #8288, #34216, #63234, .T. ) ;
#15277=CARTESIAN_POINT ( 'NONE',  ( -3.903846153846152855, -2.499999999999998668, 29.75000000000000355 ) ) ;
#15278=EDGE_CURVE ( 'NONE', #58032, #59229, #38528, .T. ) ;
#15279=CARTESIAN_POINT ( 'NONE',  ( -17.14300648787895298, -6.386643153685125363, 34.62446782046654903 ) ) ;
#15280=ORIENTED_EDGE ( 'NONE', *, *, #32219, .T. ) ;
#15281=ORIENTED_EDGE ( 'NONE', *, *, #46868, .T. ) ;
#15282=CARTESIAN_POINT ( 'NONE',  ( -1.161188422753813176, -7.630147231320743018, 34.74852402298682819 ) ) ;
#15283=ORIENTED_EDGE ( 'NONE', *, *, #32794, .T. ) ;
#15284=EDGE_CURVE ( 'NONE', #9541, #37535, #1984, .T. ) ;
#15285=B_SPLINE_CURVE_WITH_KNOTS ( 'NONE', 3,
 ( #51810, #11746, #79314, #45068, #4991, #4536, #53156, #79763, #59030, #17619 ),
 .UNSPECIFIED., .F., .F.,
 ( 4, 2, 2, 2, 4 ),
 ( 0.000000000000000000, 0.0001954339857564073659, 0.0003908679715128147319, 0.0005863019572692221250, 0.0007817359430256294638 ),
 .UNSPECIFIED. ) ;
#15286=B_SPLINE_CURVE_WITH_KNOTS ( 'NONE', 3,
 ( #24429, #51893, #77617, #15925, #3276, #78055, #51435, #86157, #43822, #30747 ),
 .UNSPECIFIED., .F., .F.,
 ( 4, 2, 2, 2, 4 ),
 ( 0.000000000000000000, 0.0001954339857564084502, 0.0003908679715128169003, 0.0005863019572692253776, 0.0007817359430256338006 ),
 .UNSPECIFIED. ) ;
#15287=CARTESIAN_POINT ( 'NONE',  ( 24.00000000000000000, -9.499999999999982236, 27.74999999999999645 ) ) ;
#15289=EDGE_CURVE ( 'NONE', #77161, #37000, #37546, .T. ) ;
#15290=CARTESIAN_POINT ( 'NONE',  ( 7.780883845597525550, -12.16647553114622049, 32.15551576947930812 ) ) ;
#15291=CARTESIAN_POINT ( 'NONE',  ( 6.856994543716788293, -9.058645607665454236, 34.76329471203372634 ) ) ;
#15292=ORIENTED_EDGE ( 'NONE', *, *, #30780, .F. ) ;
#15293=CYLINDRICAL_SURFACE ( 'NONE', #5365, 0.2500000000000012212 ) ;
#15294=AXIS2_PLACEMENT_3D ( 'NONE', #16473, #42624, #8839 ) ;
#15295=EDGE_CURVE ( 'NONE', #33331, #80197, #15973, .T. ) ;
#15296=ORIENTED_EDGE ( 'NONE', *, *, #14593, .F. ) ;
#15297=CARTESIAN_POINT ( 'NONE',  ( 9.758375025657770152, -8.164416787775445883, 34.95778746994558617 ) ) ;
#15299=CARTESIAN_POINT ( 'NONE',  ( -12.46153846153858424, -3.643525952248795718, 33.31231777344771672 ) ) ;
#15300=CARTESIAN_POINT ( 'NONE',  ( 14.30769230769218581, -5.941354392335915335, 34.76329471203413846 ) ) ;
#15302=CARTESIAN_POINT ( 'NONE',  ( 16.15384615384603251, -12.46129190930018460, 30.37095296980731973 ) ) ;
#15303=LINE ( 'NONE', #1335, #81376 ) ;
#15304=FACE_BOUND ( 'NONE', #1758, .T. ) ;
#15305=EDGE_CURVE ( 'NONE', #66929, #27245, #45050, .T. ) ;
#15307=CARTESIAN_POINT ( 'NONE',  ( -6.857821783564084228, -9.528491918058460186, 34.59228464037085615 ) ) ;
#15308=CARTESIAN_POINT ( 'NONE',  ( 9.442284468086237226, -2.341070481393819236, 30.72580821765574299 ) ) ;
#15309=CARTESIAN_POINT ( 'NONE',  ( -0.3307480205715113142, -2.845873456487964859, 32.17976146951973249 ) ) ;
#15310=CARTESIAN_POINT ( 'NONE',  ( -17.07692307692307665, -8.164416787775445883, 34.95778746994557906 ) ) ;
#15311=CYLINDRICAL_SURFACE ( 'NONE', #85040, 0.2499999999999997502 ) ;
#15314=FACE_OUTER_BOUND ( 'NONE', #14210, .T. ) ;
#15315=ORIENTED_EDGE ( 'NONE', *, *, #70455, .F. ) ;
#15316=VERTEX_POINT ( 'NONE', #29928 ) ;
#15317=CARTESIAN_POINT ( 'NONE',  ( 14.37376065869474751, -3.513871655860379306, 32.76840700105978499 ) ) ;
#15318=CARTESIAN_POINT ( 'NONE',  ( -3.230769230769229949, -5.471508081941601098, 34.59228464037088457 ) ) ;
#15319=CARTESIAN_POINT ( 'NONE',  ( 11.53846153846141576, -12.16647553114689728, 32.15551576947799362 ) ) ;
#15320=CARTESIAN_POINT ( 'NONE',  ( 7.911408985666682270, -3.643525952247864463, 33.31231777344670064 ) ) ;
#15321=CARTESIAN_POINT ( 'NONE',  ( -12.33074802057151409, -2.494656445102012565, 31.33466734024120015 ) ) ;
#15322=CARTESIAN_POINT ( 'NONE',  ( 9.823099500132480344, -2.541949514083464479, 30.39797389878540557 ) ) ;
#15323=ORIENTED_EDGE ( 'NONE', *, *, #2980, .T. ) ;
#15325=CARTESIAN_POINT ( 'NONE',  ( 13.16168916709923664, -4.887634598454295265, 34.01352882383564946 ) ) ;
#15327=ADVANCED_FACE ( 'NONE', ( #30799 ), #30364, .F. ) ;
#15328=CARTESIAN_POINT ( 'NONE',  ( 1.515141086378952062, -12.27024696741798770, 31.24895572276497546 ) ) ;
#15330=DIRECTION ( 'NONE',  ( -0.000000000000000000, 1.000000000000000000, 3.491481338843133355E-15 ) ) ;
#15331=CARTESIAN_POINT ( 'NONE',  ( -11.78846153846153832, -2.499999999999998668, 29.75000000000000355 ) ) ;
#15332=B_SPLINE_CURVE_WITH_KNOTS ( 'NONE', 3,
 ( #61360, #75773, #27149, #35231, #54607, #14078, #74451, #62254, #82103, #41113 ),
 .UNSPECIFIED., .F., .F.,
 ( 4, 2, 2, 2, 4 ),
 ( 0.000000000000000000, 0.0001954339857564091007, 0.0003908679715128182013, 0.0005863019572692273291, 0.0007817359430256364027 ),
 .UNSPECIFIED. ) ;
#15333=CARTESIAN_POINT ( 'NONE',  ( 3.100078627658924280, -11.93127051446800024, 32.56575433478200665 ) ) ;
#15334=ORIENTED_EDGE ( 'NONE', *, *, #28251, .T. ) ;
#15335=EDGE_LOOP ( 'NONE', ( #61115, #66119 ) ) ;
#15337=ORIENTED_EDGE ( 'NONE', *, *, #22899, .F. ) ;
#15338=CYLINDRICAL_SURFACE ( 'NONE', #63985, 0.2500000000000008882 ) ;
#15339=CARTESIAN_POINT ( 'NONE',  ( 15.29683656411930848, -3.937682226553329556, 33.60647404775216529 ) ) ;
#15340=CARTESIAN_POINT ( 'NONE',  ( -14.24243673641627872, -6.879047030191282275, 34.71129190930002295 ) ) ;
#15343=EDGE_CURVE ( 'NONE', #43192, #4609, #24458, .T. ) ;
#15345=ORIENTED_EDGE ( 'NONE', *, *, #10662, .T. ) ;
#15346=CARTESIAN_POINT ( 'NONE',  ( 3.930967471417507131, -7.630691491037286056, 34.74850469731152458 ) ) ;
#15347=CARTESIAN_POINT ( 'NONE',  ( -2.177166869458663889, -12.70449254468099198, 30.44128974285582956 ) ) ;
#15348=ORIENTED_EDGE ( 'NONE', *, *, #15509, .F. ) ;
#15349=CARTESIAN_POINT ( 'NONE',  ( 3.165498784808455479, -12.46129190929999986, 30.37095296980880832 ) ) ;
#15350=CARTESIAN_POINT ( 'NONE',  ( -17.20761368003338987, -11.93127051446800380, 32.56575433478200665 ) ) ;
#15351=EDGE_CURVE ( 'NONE', #76215, #87554, #62128, .T. ) ;
#15352=ADVANCED_FACE ( 'NONE', ( #11429 ), #66371, .F. ) ;
#15353=CARTESIAN_POINT ( 'NONE',  ( 15.36129466900287177, -3.068774925481848825, 32.56582465632704526 ) ) ;
#15354=CARTESIAN_POINT ( 'NONE',  ( -9.758390071667831123, -12.34228464037088280, 31.77849191805838558 ) ) ;
#15355=CARTESIAN_POINT ( 'NONE',  ( -12.68502340526241312, -12.44517049084099725, 30.48991314939691932 ) ) ;
#15357=ORIENTED_EDGE ( 'NONE', *, *, #39036, .F. ) ;
#15359=CARTESIAN_POINT ( 'NONE',  ( -1.161604033002534342, -11.24521262558773671, 33.06293181088029343 ) ) ;
#15360=CARTESIAN_POINT ( 'NONE',  ( -13.44988583057615905, -9.442884908240170461, 34.35708131394840592 ) ) ;
#15361=CARTESIAN_POINT ( 'NONE',  ( -3.296852641725108946, -8.973038597847271092, 34.52809138561120506 ) ) ;
#15362=VECTOR ( 'NONE', #17362, 1000.000000000000114 ) ;
#15363=CARTESIAN_POINT ( 'NONE',  ( -3.007989561791164945, -10.97394488606064122, 33.68653795673694873 ) ) ;
#15364=ORIENTED_EDGE ( 'NONE', *, *, #83244, .F. ) ;
#15365=DIRECTION ( 'NONE',  ( -0.000000000000000000, -0.7660444431189791237, -0.6427876096865379196 ) ) ;
#15366=CARTESIAN_POINT ( 'NONE',  ( 11.31497661389720477, -4.225889041578353655, 33.85425143139329407 ) ) ;
#15368=B_SPLINE_CURVE_WITH_KNOTS ( 'NONE', 3,
 ( #37450, #64918, #57731, #65805, #4106, #17642, #44191, #29823, #84778, #2765 ),
 .UNSPECIFIED., .F., .F.,
 ( 4, 2, 2, 2, 4 ),
 ( 0.0007817246256747530271, 0.0009771112852218978746, 0.001172497944769042939, 0.001367884604316188003, 0.001563271263863332851 ),
 .UNSPECIFIED. ) ;
#15370=DIRECTION ( 'NONE',  ( -0.000000000000000000, 0.1736481776669307198, -0.9848077530122080203 ) ) ;
#15371=CYLINDRICAL_SURFACE ( 'NONE', #2577, 0.2500000000000008882 ) ;
#15372=VERTEX_POINT ( 'NONE', #72233 ) ;
#15373=B_SPLINE_CURVE_WITH_KNOTS ( 'NONE', 3,
 ( #37059, #20564, #34961, #16792, #10037, #51002, #78058, #62422, #43824, #13807 ),
 .UNSPECIFIED., .F., .F.,
 ( 4, 2, 2, 2, 4 ),
 ( 0.000000000000000000, 0.0001954311564186865763, 0.0003908623128373731525, 0.0005862934692560596746, 0.0007817246256747463051 ),
 .UNSPECIFIED. ) ;
#15374=B_SPLINE_CURVE_WITH_KNOTS ( 'NONE', 3,
 ( #58470, #79211, #44961, #10750, #65676, #31462, #58927, #24704, #84810, #16763 ),
 .UNSPECIFIED., .F., .F.,
 ( 4, 2, 2, 2, 4 ),
 ( 0.0007817246256747473893, 0.0009771112852218900684, 0.001172497944769032747, 0.001367884604316175643, 0.001563271263863318323 ),
 .UNSPECIFIED. ) ;
#15375=CARTESIAN_POINT ( 'NONE',  ( 0.4615384615384611200, -8.318370150425687726, 35.83090037661290239 ) ) ;
#15376=CARTESIAN_POINT ( 'NONE',  ( -17.30040800148741198, -2.353723527008297012, 30.78948104536958752 ) ) ;
#15378=CARTESIAN_POINT ( 'NONE',  ( 8.096208157792160520, -5.728107161865378494, 34.42597550085002922 ) ) ;
#15379=CARTESIAN_POINT ( 'NONE',  ( -4.283994123577849145, -11.66186481527757479, 32.95055677023626117 ) ) ;
#15381=CARTESIAN_POINT ( 'NONE',  ( -13.38461538461550759, -3.083524468854526912, 32.58852847137268327 ) ) ;
#15382=EDGE_CURVE ( 'NONE', #28930, #17603, #49194, .T. ) ;
#15383=ORIENTED_EDGE ( 'NONE', *, *, #72295, .T. ) ;
#15384=CARTESIAN_POINT ( 'NONE',  ( -6.857882941293567569, -2.506253911140448487, 29.99999999999988631 ) ) ;
#15385=CARTESIAN_POINT ( 'NONE',  ( 0.6845513056318554002, -10.01129605718032778, 34.36064277460058491 ) ) ;
#15386=ORIENTED_EDGE ( 'NONE', *, *, #84475, .F. ) ;
#15387=CARTESIAN_POINT ( 'NONE',  ( -17.86920955903305597, -9.929761469519744921, 34.40412654351204225 ) ) ;
#15388=CARTESIAN_POINT ( 'NONE',  ( 16.15384615384615330, -13.78497067705608181, 32.30358669280327177 ) ) ;
#15389=CARTESIAN_POINT ( 'NONE',  ( -3.930470213147969183, -2.501478030877322567, 29.88021232661720816 ) ) ;
#15390=CYLINDRICAL_SURFACE ( 'NONE', #23298, 0.2499999999999973355 ) ;
#15392=VECTOR ( 'NONE', #28556, 1000.000000000000000 ) ;
#15393=ORIENTED_EDGE ( 'NONE', *, *, #19484, .F. ) ;
#15395=FACE_BOUND ( 'NONE', #49828, .T. ) ;
#15396=ORIENTED_EDGE ( 'NONE', *, *, #73469, .T. ) ;
#15397=CARTESIAN_POINT ( 'NONE',  ( 15.45354877203763877, -2.600157965045224895, 30.74683119005207743 ) ) ;
#15398=CIRCLE ( 'NONE', #65711, 0.2500000000000002220 ) ;
#15399=B_SPLINE_CURVE_WITH_KNOTS ( 'NONE', 3,
 ( #70593, #34144, #21063, #55739, #61612, #48533, #76015, #38134, #30919, #44879 ),
 .UNSPECIFIED., .F., .F.,
 ( 4, 2, 2, 2, 4 ),
 ( 0.000000000000000000, 0.0001954339857564091007, 0.0003908679715128182013, 0.0005863019572692273291, 0.0007817359430256364027 ),
 .UNSPECIFIED. ) ;
#15400=CARTESIAN_POINT ( 'NONE',  ( 13.13461538461538680, -7.500000000000001776, 34.75000000000000000 ) ) ;
#15401=VECTOR ( 'NONE', #19539, 1000.000000000000227 ) ;
#15402=CARTESIAN_POINT ( 'NONE',  ( 17.93391762063986761, -5.471508081941601986, 34.59228464037088457 ) ) ;
#15403=CARTESIAN_POINT ( 'NONE',  ( -14.05774678934416499, -9.272278438253398036, 34.42582936511637115 ) ) ;
#15404=ORIENTED_EDGE ( 'NONE', *, *, #47334, .T. ) ;
#15405=EDGE_CURVE ( 'NONE', #76676, #2738, #23343, .T. ) ;
#15406=ORIENTED_EDGE ( 'NONE', *, *, #32140, .T. ) ;
#15407=VERTEX_POINT ( 'NONE', #51493 ) ;
#15408=B_SPLINE_CURVE_WITH_KNOTS ( 'NONE', 3,
 ( #20187, #68362, #47652, #40468, #75135, #74240, #73349, #31925, #39131, #80105 ),
 .UNSPECIFIED., .F., .F.,
 ( 4, 2, 2, 2, 4 ),
 ( 0.000000000000000000, 0.0001954311564186879857, 0.0003908623128373759715, 0.0005862934692560640114, 0.0007817246256747519429 ),
 .UNSPECIFIED. ) ;
#15409=CARTESIAN_POINT ( 'NONE',  ( -10.83831157429145975, -8.282780595021769443, 34.94152052738834158 ) ) ;
#15410=VERTEX_POINT ( 'NONE', #10543 ) ;
#15411=CARTESIAN_POINT ( 'NONE',  ( 13.25392391794783542, -2.729777683071817229, 31.24903638046269450 ) ) ;
#15412=CARTESIAN_POINT ( 'NONE',  ( -12.23816297576603951, -2.251407671071268712, 29.88021292934943318 ) ) ;
#15413=CARTESIAN_POINT ( 'NONE',  ( -17.32694630114453105, -2.985938066672154445, 32.43141759479405550 ) ) ;
#15414=VERTEX_POINT ( 'NONE', #38010 ) ;
#15415=CARTESIAN_POINT ( 'NONE',  ( 8.900022577055558770, -8.999086150933475636, 34.52020707165672775 ) ) ;
#15416=CARTESIAN_POINT ( 'NONE',  ( -15.16470189741915320, -3.322132147404559976, 32.92929555188717927 ) ) ;
#15417=VECTOR ( 'NONE', #71019, 1000.000000000000000 ) ;
#15418=CARTESIAN_POINT ( 'NONE',  ( 14.55763782604045176, -6.696923467548660192, 34.68552623307873972 ) ) ;
#15420=VERTEX_POINT ( 'NONE', #58717 ) ;
#15421=ADVANCED_FACE ( 'NONE', ( #86218 ), #45200, .F. ) ;
#15422=EDGE_LOOP ( 'NONE', ( #20487, #79612 ) ) ;
#15424=DIRECTION ( 'NONE',  ( 0.000000000000000000, 1.000000000000000000, 0.000000000000000000 ) ) ;
#15426=CARTESIAN_POINT ( 'NONE',  ( -13.60754160213153163, -5.667676309546437530, 34.40238873228292249 ) ) ;
#15427=FACE_OUTER_BOUND ( 'NONE', #59893, .T. ) ;
#15428=CARTESIAN_POINT ( 'NONE',  ( -2.176901866725354573, -2.494656445102013453, 31.33466734024120015 ) ) ;
#15429=DIRECTION ( 'NONE',  ( 1.000000000000000000, 0.000000000000000000, 0.000000000000000000 ) ) ;
#15430=CARTESIAN_POINT ( 'NONE',  ( 7.976945653978634532, -11.18335022499818621, 33.13157742990016885 ) ) ;
#15431=EDGE_LOOP ( 'NONE', ( #76132, #66816 ) ) ;
#15432=CARTESIAN_POINT ( 'NONE',  ( -7.716106410903393886, -7.723484941389745728, 34.99544897038809665 ) ) ;
#15433=EDGE_CURVE ( 'NONE', #87441, #88485, #32150, .T. ) ;
#15435=CYLINDRICAL_SURFACE ( 'NONE', #41641, 0.2500000000000012212 ) ;
#15436=CARTESIAN_POINT ( 'NONE',  ( -17.32689980786543060, -11.79746400365624659, 32.30657167506340954 ) ) ;
#15437=FACE_OUTER_BOUND ( 'NONE', #64332, .T. ) ;
#15439=CARTESIAN_POINT ( 'NONE',  ( 6.000000000000001776, -9.819645486525091727, 36.12317359536749706 ) ) ;
#15440=ORIENTED_EDGE ( 'NONE', *, *, #58698, .T. ) ;
#15441=FACE_BOUND ( 'NONE', #8527, .T. ) ;
#15442=CARTESIAN_POINT ( 'NONE',  ( -17.07692307692319744, -4.481592998941358097, 33.73612834414048933 ) ) ;
#15443=DIRECTION ( 'NONE',  ( -1.000000000000000000, 0.000000000000000000, 0.000000000000000000 ) ) ;
#15444=CARTESIAN_POINT ( 'NONE',  ( -16.15384615384615330, -8.973038597847269315, 34.52809138561121927 ) ) ;
#15445=EDGE_LOOP ( 'NONE', ( #11792, #68946, #5676, #23822 ) ) ;
#15447=CARTESIAN_POINT ( 'NONE',  ( -5.869209559033047974, -9.084667340241226796, 34.75534355489798344 ) ) ;
#15448=CARTESIAN_POINT ( 'NONE',  ( 8.545745844666436497, -8.539481045369596401, 34.89627647299170832 ) ) ;
#15449=CARTESIAN_POINT ( 'NONE',  ( -5.010855743573000787, -5.471508081941601098, 34.59228464037088457 ) ) ;
#15450=VERTEX_POINT ( 'NONE', #41120 ) ;
#15451=CARTESIAN_POINT ( 'NONE',  ( -4.087777802843714170, -6.386643153685127139, 34.62446782046654192 ) ) ;
#15452=ORIENTED_EDGE ( 'NONE', *, *, #12273, .T. ) ;
#15453=CARTESIAN_POINT ( 'NONE',  ( 16.28468448433291016, -7.277220318596959281, 34.99547417642776992 ) ) ;
#15454=ORIENTED_EDGE ( 'NONE', *, *, #71377, .T. ) ;
#15455=CARTESIAN_POINT ( 'NONE',  ( 9.469381474791543241, -3.586966769969701208, 32.86292498521069660 ) ) ;
#15456=CARTESIAN_POINT ( 'NONE',  ( -10.61538461538461320, -12.37446782046654192, 30.86335684631486131 ) ) ;
#15457=CARTESIAN_POINT ( 'NONE',  ( 13.38461538461526601, -9.442884908241554243, 34.35708131394783038 ) ) ;
#15458=AXIS2_PLACEMENT_3D ( 'NONE', #81669, #20405, #25387 ) ;
#15459=EDGE_CURVE ( 'NONE', #49638, #83085, #81227, .T. ) ;
#15461=CARTESIAN_POINT ( 'NONE',  ( 12.52760681254089725, -4.098570777380720287, 33.41473453929635440 ) ) ;
#15462=CARTESIAN_POINT ( 'NONE',  ( -3.007989561791163169, -4.226511098958374291, 33.85474049983370293 ) ) ;
#15463=CARTESIAN_POINT ( 'NONE',  ( -11.76138849736838488, -9.172386477786396597, 34.72672124145550043 ) ) ;
#15464=CARTESIAN_POINT ( 'NONE',  ( 8.069165197766697162, -4.187068189119699468, 33.49521262558774026 ) ) ;
#15466=ORIENTED_EDGE ( 'NONE', *, *, #56002, .T. ) ;
#15468=DIRECTION ( 'NONE',  ( 0.000000000000000000, 0.4999999999999960032, -0.8660254037844410391 ) ) ;
#15469=CARTESIAN_POINT ( 'NONE',  ( -9.692307692307691624, -11.35647404775217417, 33.31231777344666511 ) ) ;
#15470=EDGE_LOOP ( 'NONE', ( #70549, #75362, #14298, #32666 ) ) ;
#15471=B_SPLINE_CURVE_WITH_KNOTS ( 'NONE', 3,
 ( #48567, #21096, #76049, #62520, #837, #28303, #55772, #21549, #71497, #38164 ),
 .UNSPECIFIED., .F., .F.,
 ( 4, 2, 2, 2, 4 ),
 ( 0.0007817359430256322827, 0.0009771253907249989254, 0.001172514838424365676, 0.001367904286123732428, 0.001563293733823098962 ),
 .UNSPECIFIED. ) ;
#15472=ORIENTED_EDGE ( 'NONE', *, *, #71880, .T. ) ;
#15474=VERTEX_POINT ( 'NONE', #88012 ) ;
#15475=CARTESIAN_POINT ( 'NONE',  ( 10.68145194873469173, -8.164416787775445883, 34.95778746994558617 ) ) ;
#15477=CYLINDRICAL_SURFACE ( 'NONE', #70126, 0.2500000000000008882 ) ;
#15478=DIRECTION ( 'NONE',  ( -0.000000000000000000, -0.3420201433256694346, -0.9396926207859080948 ) ) ;
#15479=CARTESIAN_POINT ( 'NONE',  ( -16.21911659980693443, -3.300289026998414865, 32.46337939537583850 ) ) ;
#15480=CARTESIAN_POINT ( 'NONE',  ( -8.769230769230768274, -2.833524468853757305, 32.15551576947925838 ) ) ;
#15481=CARTESIAN_POINT ( 'NONE',  ( 13.51466044053515958, -2.254550872974306674, 29.97347326024527092 ) ) ;
#15482=LINE ( 'NONE', #70423, #8880 ) ;
#15483=CARTESIAN_POINT ( 'NONE',  ( 11.28843830116857383, -10.76384336483936011, 33.53834819971076087 ) ) ;
#15484=CARTESIAN_POINT ( 'NONE',  ( 12.23861224402230974, -11.76352882383564769, 32.36236540154569497 ) ) ;
#15485=CARTESIAN_POINT ( 'NONE',  ( -6.923076923076922462, -2.708943851104267164, 35.45975837776705220 ) ) ;
#15486=ORIENTED_EDGE ( 'NONE', *, *, #82733, .F. ) ;
#15487=VERTEX_POINT ( 'NONE', #53741 ) ;
#15488=VECTOR ( 'NONE', #45208, 1000.000000000000227 ) ;
#15489=CARTESIAN_POINT ( 'NONE',  ( -17.77713457779637807, -12.49850393767509260, 29.88072118266894250 ) ) ;
#15492=CARTESIAN_POINT ( 'NONE',  ( -14.30769230769230660, -9.780366693483667717, 34.19971097300155094 ) ) ;
#15495=CARTESIAN_POINT ( 'NONE',  ( -10.61538461538461320, -12.62096338111211580, 30.90682066428153263 ) ) ;
#15497=VECTOR ( 'NONE', #80961, 1000.000000000000227 ) ;
#15499=B_SPLINE_CURVE_WITH_KNOTS ( 'NONE', 3,
 ( #74145, #34039, #14213, #54302, #68712, #13326, #13765, #75468, #33156, #40808 ),
 .UNSPECIFIED., .F., .F.,
 ( 4, 2, 2, 2, 4 ),
 ( 0.0007817246256747477145, 0.0009771112852218911526, 0.001172497944769034699, 0.001367884604316178246, 0.001563271263863321792 ),
 .UNSPECIFIED. ) ;
#15500=CARTESIAN_POINT ( 'NONE',  ( -13.60754160213153163, -9.886141570436013382, 34.14413921362392301 ) ) ;
#15502=CARTESIAN_POINT ( 'NONE',  ( 13.25446741488368829, -12.50552854090298638, 31.33409797877408920 ) ) ;
#15503=CARTESIAN_POINT ( 'NONE',  ( 6.988332062589762472, -3.083524468853784839, 32.58852847137153930 ) ) ;
#15504=CARTESIAN_POINT ( 'NONE',  ( 6.923076923076802558, -8.613356846316285953, 34.62446782046622218 ) ) ;
#15505=CARTESIAN_POINT ( 'NONE',  ( -14.30769230769242739, -11.94971097300221174, 32.03036669348237098 ) ) ;
#15506=CARTESIAN_POINT ( 'NONE',  ( 18.00000000000000000, -8.164416787775445883, 34.95778746994557906 ) ) ;
#15507=ORIENTED_EDGE ( 'NONE', *, *, #70785, .T. ) ;
#15508=EDGE_CURVE ( 'NONE', #86943, #36959, #77111, .T. ) ;
#15509=EDGE_CURVE ( 'NONE', #26228, #29264, #33910, .T. ) ;
#15510=ORIENTED_EDGE ( 'NONE', *, *, #10167, .T. ) ;
#15512=CARTESIAN_POINT ( 'NONE',  ( -6.222926217516143055, -11.24512374952581872, 33.06303171183252942 ) ) ;
#15513=CARTESIAN_POINT ( 'NONE',  ( 5.076923076923075762, -11.11383981884818262, 36.00935417666054406 ) ) ;
#15514=CARTESIAN_POINT ( 'NONE',  ( 17.20744877868664346, -4.459921816937789885, 33.71989282347011851 ) ) ;
#15515=CARTESIAN_POINT ( 'NONE',  ( 16.85343815235874132, -10.23692288466677880, 34.23039457007281072 ) ) ;
#15516=ADVANCED_FACE ( 'NONE', ( #46546 ), #81668, .F. ) ;
#15517=CARTESIAN_POINT ( 'NONE',  ( -17.93474442872397034, -4.481592998940253203, 33.73612834413965089 ) ) ;
#15520=ORIENTED_EDGE ( 'NONE', *, *, #67891, .F. ) ;
#15521=EDGE_CURVE ( 'NONE', #87868, #59899, #11553, .T. ) ;
#15522=ORIENTED_EDGE ( 'NONE', *, *, #53764, .F. ) ;
#15523=B_SPLINE_CURVE_WITH_KNOTS ( 'NONE', 3,
 ( #73976, #86614, #59560, #39754, #24884, #87065, #25336, #86165, #52800, #18588 ),
 .UNSPECIFIED., .F., .F.,
 ( 4, 2, 2, 2, 4 ),
 ( 0.000000000000000000, 0.0001954311564186880399, 0.0003908623128373760799, 0.0005862934692560641198, 0.0007817246256747521597 ),
 .UNSPECIFIED. ) ;
#15524=B_SPLINE_CURVE_WITH_KNOTS ( 'NONE', 3,
 ( #63146, #64915, #16301, #1461, #84775, #77997, #22177, #50075, #77117, #50516 ),
 .UNSPECIFIED., .F., .F.,
 ( 4, 2, 2, 2, 4 ),
 ( 0.000000000000000000, 0.0001954339857564074473, 0.0003908679715128148945, 0.0005863019572692223418, 0.0007817359430256297891 ),
 .UNSPECIFIED. ) ;
#15525=ORIENTED_EDGE ( 'NONE', *, *, #88323, .F. ) ;
#15526=CARTESIAN_POINT ( 'NONE',  ( 4.023154687178595701, -2.729777683071817229, 31.24903638046268739 ) ) ;
#15527=ORIENTED_EDGE ( 'NONE', *, *, #17696, .F. ) ;
#15528=CARTESIAN_POINT ( 'NONE',  ( 9.019285080869085647, -8.303483539816731707, 34.68545999027711702 ) ) ;
#15529=CARTESIAN_POINT ( 'NONE',  ( 14.30769230769231015, -4.661471528628507777, 34.16647553114623292 ) ) ;
#15532=EDGE_CURVE ( 'NONE', #35909, #79975, #88957, .T. ) ;
#15533=ORIENTED_EDGE ( 'NONE', *, *, #52025, .F. ) ;
#15534=CARTESIAN_POINT ( 'NONE',  ( 13.63461538461538680, -2.499999999999998668, 29.75000000000000355 ) ) ;
#15535=ORIENTED_EDGE ( 'NONE', *, *, #30073, .T. ) ;
#15536=FACE_BOUND ( 'NONE', #31659, .T. ) ;
#15537=CARTESIAN_POINT ( 'NONE',  ( 4.853996118016225658, -4.762599654559228846, 34.23009711892697737 ) ) ;
#15538=AXIS2_PLACEMENT_3D ( 'NONE', #20958, #41689, #54752 ) ;
#15539=CARTESIAN_POINT ( 'NONE',  ( -8.769230769230768274, -1.215029322943914858, 32.30358669280327177 ) ) ;
#15540=ORIENTED_EDGE ( 'NONE', *, *, #43863, .T. ) ;
#15541=CARTESIAN_POINT ( 'NONE',  ( -14.08467946359890988, -8.282913670948747864, 34.94150082978203642 ) ) ;
#15544=CARTESIAN_POINT ( 'NONE',  ( -15.45369544828537656, -6.503392248772476236, 34.64988816332204635 ) ) ;
#15545=DIRECTION ( 'NONE',  ( -0.000000000000000000, -0.9848077530122085754, -0.1736481776669273613 ) ) ;
#15547=CARTESIAN_POINT ( 'NONE',  ( -7.173053654019277303, -11.28823185664190376, 33.01397839955799896 ) ) ;
#15548=DIRECTION ( 'NONE',  ( 1.000000000000000000, 0.000000000000000000, 0.000000000000000000 ) ) ;
#15552=EDGE_CURVE ( 'NONE', #26886, #68329, #21271, .T. ) ;
#15553=CARTESIAN_POINT ( 'NONE',  ( 6.130791807824789608, -9.804649428959608670, 34.18742332936588468 ) ) ;
#15555=CARTESIAN_POINT ( 'NONE',  ( -7.846153846153844924, -12.29105614889573062, 35.45975837776705220 ) ) ;
#15557=CARTESIAN_POINT ( 'NONE',  ( 8.703979779069525691, -2.506253911140460922, 30.00000000000013856 ) ) ;
#15558=CARTESIAN_POINT ( 'NONE',  ( -3.453696189676079609, -2.889293201056495786, 32.26117774369186009 ) ) ;
#15559=CARTESIAN_POINT ( 'NONE',  ( -18.13014796973169851, -3.069018819979306034, 32.56621877034668699 ) ) ;
#15560=EDGE_CURVE ( 'NONE', #45585, #32628, #68584, .T. ) ;
#15561=CARTESIAN_POINT ( 'NONE',  ( -2.307692307692305711, -5.471508081941601098, 34.59228464037088457 ) ) ;
#15563=ORIENTED_EDGE ( 'NONE', *, *, #59556, .T. ) ;
#15565=VERTEX_POINT ( 'NONE', #6881 ) ;
#15566=CARTESIAN_POINT ( 'NONE',  ( 0.5267324433218166790, -2.506253911140448043, 29.99999999999988631 ) ) ;
#15567=EDGE_CURVE ( 'NONE', #74976, #16308, #53290, .T. ) ;
#15569=EDGE_CURVE ( 'NONE', #48285, #87573, #76221, .T. ) ;
#15570=CARTESIAN_POINT ( 'NONE',  ( -13.25382494364843389, -2.295524264805589354, 30.44142389570982488 ) ) ;
#15571=CARTESIAN_POINT ( 'NONE',  ( 17.29993592101647693, -2.889357225399416418, 32.26129605718031002 ) ) ;
#15572=EDGE_LOOP ( 'NONE', ( #21637, #21797, #67792, #46496 ) ) ;
#15573=CARTESIAN_POINT ( 'NONE',  ( -18.06527044596078113, -12.46129190929999986, 30.37095296980880832 ) ) ;
#15575=CARTESIAN_POINT ( 'NONE',  ( 7.846153846153846700, -1.509761064869970415, 31.06009739812519044 ) ) ;
#15576=CARTESIAN_POINT ( 'NONE',  ( -3.230769230769352962, -12.51329471203414379, 31.30864560766407578 ) ) ;
#15577=CARTESIAN_POINT ( 'NONE',  ( 7.173131234715239835, -9.148310452688871663, 34.47095581063188519 ) ) ;
#15578=CARTESIAN_POINT ( 'NONE',  ( 8.769230769230768274, -3.513871655860378418, 32.76840700105978499 ) ) ;
#15579=DIRECTION ( 'NONE',  ( -0.000000000000000000, -0.000000000000000000, -1.000000000000000000 ) ) ;
#15580=CARTESIAN_POINT ( 'NONE',  ( 1.384615384615386802, -2.292212530054420494, 30.41441678777542634 ) ) ;
#15582=B_SPLINE_CURVE_WITH_KNOTS ( 'NONE', 3,
 ( #40621, #41948, #49135, #33416, #20348, #35181, #88820, #68091, #55012, #41498 ),
 .UNSPECIFIED., .F., .F.,
 ( 4, 2, 2, 2, 4 ),
 ( 0.000000000000000000, 0.0001954311564186867931, 0.0003908623128373735862, 0.0005862934692560603251, 0.0007817246256747471724 ),
 .UNSPECIFIED. ) ;
#15583=CARTESIAN_POINT ( 'NONE',  ( 11.47237915910140771, -5.471508081941602875, 34.59228464037088457 ) ) ;
#15584=CYLINDRICAL_SURFACE ( 'NONE', #40561, 0.2499999999999979738 ) ;
#15586=AXIS2_PLACEMENT_3D ( 'NONE', #83794, #1799, #84679 ) ;
#15590=CARTESIAN_POINT ( 'NONE',  ( 14.43848411551709709, -2.541949514083464479, 30.39797389878540557 ) ) ;
#15591=CARTESIAN_POINT ( 'NONE',  ( -11.31545018684868964, -8.239487800360276282, 34.69522927552633718 ) ) ;
#15592=CARTESIAN_POINT ( 'NONE',  ( 1.384615384615265343, -12.46129190930018460, 30.37095296980731973 ) ) ;
#15593=CARTESIAN_POINT ( 'NONE',  ( 16.37727255276093530, -7.630147987733843173, 34.99859428049665411 ) ) ;
#15594=CARTESIAN_POINT ( 'NONE',  ( -2.980823712421089233, -5.057305518903949526, 34.11320923018887896 ) ) ;
#15595=CARTESIAN_POINT ( 'NONE',  ( -8.992715712954719720, -8.496056993536548418, 34.65000542017679663 ) ) ;
#15597=EDGE_CURVE ( 'NONE', #62488, #64833, #36578, .T. ) ;
#15598=ORIENTED_EDGE ( 'NONE', *, *, #51644, .F. ) ;
#15599=B_SPLINE_CURVE_WITH_KNOTS ( 'NONE', 3,
 ( #83283, #75200, #40095, #27452, #5853, #67999, #14369, #88294, #27891, #19805 ),
 .UNSPECIFIED., .F., .F.,
 ( 4, 2, 2, 2, 4 ),
 ( 0.000000000000000000, 0.0001954339881912783015, 0.0003908679763825566029, 0.0005863019645738348773, 0.0007817359527651132059 ),
 .UNSPECIFIED. ) ;
#15600=ORIENTED_EDGE ( 'NONE', *, *, #86325, .F. ) ;
#15602=VECTOR ( 'NONE', #45126, 999.9999999999998863 ) ;
#15603=CARTESIAN_POINT ( 'NONE',  ( 3.296024802045255164, -6.026961402152789304, 34.52809138561124769 ) ) ;
#15604=CARTESIAN_POINT ( 'NONE',  ( 6.699591979352978122, -2.847400154188068022, 31.58180166144859058 ) ) ;
#15605=CYLINDRICAL_SURFACE ( 'NONE', #23046, 0.2500000000000009437 ) ;
#15606=CARTESIAN_POINT ( 'NONE',  ( 1.384615384615265343, -11.94971097300221174, 32.03036669348237098 ) ) ;
#15607=CARTESIAN_POINT ( 'NONE',  ( 17.77651505627605033, -9.331801661448606566, 34.40259984581193464 ) ) ;
#15608=EDGE_CURVE ( 'NONE', #74921, #47774, #82558, .T. ) ;
#15609=VECTOR ( 'NONE', #26684, 1000.000000000000000 ) ;
#15610=ORIENTED_EDGE ( 'NONE', *, *, #36512, .F. ) ;
#15611=CARTESIAN_POINT ( 'NONE',  ( -7.846153846153844924, -2.708943851104267164, 35.45975837776705220 ) ) ;
#15612=AXIS2_PLACEMENT_3D ( 'NONE', #40377, #61511, #13333 ) ;
#15613=ORIENTED_EDGE ( 'NONE', *, *, #26758, .T. ) ;
#15615=AXIS2_PLACEMENT_3D ( 'NONE', #18717, #6526, #68226 ) ;
#15616=CARTESIAN_POINT ( 'NONE',  ( 4.153846153846154188, -12.34228464037088635, 31.77849191805839268 ) ) ;
#15617=ORIENTED_EDGE ( 'NONE', *, *, #12915, .T. ) ;
#15618=CARTESIAN_POINT ( 'NONE',  ( 16.37662569511456212, -12.44528174975671853, 30.48912976160715615 ) ) ;
#15619=CARTESIAN_POINT ( 'NONE',  ( -16.40386939113911779, -4.335965774309648246, 33.62209801155881905 ) ) ;
#15620=EDGE_CURVE ( 'NONE', #80339, #39978, #56837, .T. ) ;
#15622=CARTESIAN_POINT ( 'NONE',  ( -15.90390074446811042, -5.766571408460170467, 34.70601412856602508 ) ) ;
#15623=ORIENTED_EDGE ( 'NONE', *, *, #20312, .T. ) ;
#15625=ORIENTED_EDGE ( 'NONE', *, *, #57544, .F. ) ;
#15626=VERTEX_POINT ( 'NONE', #42013 ) ;
#15627=CARTESIAN_POINT ( 'NONE',  ( -9.469528151039279251, -5.913360116392397892, 34.49180327182771322 ) ) ;
#15628=CARTESIAN_POINT ( 'NONE',  ( 1.318531973659506251, -8.120952969808774569, 34.71129190930000163 ) ) ;
#15629=VERTEX_POINT ( 'NONE', #70811 ) ;
#15631=CARTESIAN_POINT ( 'NONE',  ( 6.130525701763564150, -12.45806712695776319, 30.39783852428763922 ) ) ;
#15632=LINE ( 'NONE', #78655, #83919 ) ;
#15633=ORIENTED_EDGE ( 'NONE', *, *, #23028, .F. ) ;
#15634=EDGE_CURVE ( 'NONE', #86086, #86521, #20168, .T. ) ;
#15635=CARTESIAN_POINT ( 'NONE',  ( -10.61538461538461320, -1.509761064869970415, 31.06009739812519044 ) ) ;
#15639=FACE_BOUND ( 'NONE', #73541, .T. ) ;
#15640=CARTESIAN_POINT ( 'NONE',  ( 11.28848480751918437, -4.943428324936578910, 34.04746400365624481 ) ) ;
#15642=B_SPLINE_CURVE_WITH_KNOTS ( 'NONE', 3,
 ( #59536, #11806, #80264, #66742, #5040, #32961, #25759, #26645, #53220, #19443 ),
 .UNSPECIFIED., .F., .F.,
 ( 4, 2, 2, 2, 4 ),
 ( 0.0007817246256747503166, 0.0009771112852218946220, 0.001172497944769039036, 0.001367884604316183450, 0.001563271263863327864 ),
 .UNSPECIFIED. ) ;
#15643=CARTESIAN_POINT ( 'NONE',  ( 2.057715563643718326, -12.41104346484419452, 31.60698883733904196 ) ) ;
#15644=CARTESIAN_POINT ( 'NONE',  ( 8.096099255531889582, -10.92531984108285670, 33.72920026020278073 ) ) ;
#15645=CARTESIAN_POINT ( 'NONE',  ( -10.86536135943320502, -5.643011162660950042, 34.66104346484419096 ) ) ;
#15647=CARTESIAN_POINT ( 'NONE',  ( 15.90382291655318880, -2.587272538249754117, 30.68239716806877837 ) ) ;
#15648=CARTESIAN_POINT ( 'NONE',  ( -2.438383774359867751, -3.530157926970578508, 32.79014554554150607 ) ) ;
#15650=CYLINDRICAL_SURFACE ( 'NONE', #5847, 0.2500000000000008882 ) ;
#15651=EDGE_CURVE ( 'NONE', #59172, #43517, #25589, .T. ) ;
#15652=CARTESIAN_POINT ( 'NONE',  ( 5.076923076923075762, -3.937682226553329556, 33.60647404775216529 ) ) ;
#15656=DIRECTION ( 'NONE',  ( 0.000000000000000000, -6.938893903907222067E-15, 1.000000000000000000 ) ) ;
#15657=CARTESIAN_POINT ( 'NONE',  ( 6.923076923076924238, -6.343179335718451384, 34.87096338111211935 ) ) ;
#15658=CARTESIAN_POINT ( 'NONE',  ( 7.912221179503920787, -6.343179335718452272, 34.87096338111212646 ) ) ;
#15659=CARTESIAN_POINT ( 'NONE',  ( -4.283994123577848256, -2.373036134822904319, 30.88089517874952250 ) ) ;
#15660=EDGE_CURVE ( 'NONE', #80250, #71551, #29908, .T. ) ;
#15661=FACE_BOUND ( 'NONE', #40342, .T. ) ;
#15662=CARTESIAN_POINT ( 'NONE',  ( 6.699591998512592461, -4.225889041578354544, 33.85425143139329407 ) ) ;
#15663=CARTESIAN_POINT ( 'NONE',  ( 17.77707304109314279, -10.77366814457252175, 33.85459836347580875 ) ) ;
#15664=CARTESIAN_POINT ( 'NONE',  ( -15.23076923076935074, -9.442884908241554243, 34.35708131394783038 ) ) ;
#15665=CARTESIAN_POINT ( 'NONE',  ( -17.75005448165186195, -11.37275283266504111, 32.91324779482534524 ) ) ;
#15666=CARTESIAN_POINT ( 'NONE',  ( -12.71156169883143150, -4.335965774309648246, 33.62209801155881905 ) ) ;
#15669=ORIENTED_EDGE ( 'NONE', *, *, #21776, .F. ) ;
#15670=EDGE_CURVE ( 'NONE', #68060, #12150, #50297, .T. ) ;
#15671=B_SPLINE_CURVE_WITH_KNOTS ( 'NONE', 3,
 ( #73846, #12144, #39625, #62956, #14347, #6701, #54896, #55770, #21994, #83712 ),
 .UNSPECIFIED., .F., .F.,
 ( 4, 2, 2, 2, 4 ),
 ( 0.0007817359430256365111, 0.0009771253907250045632, 0.001172514838424372399, 0.001367904286123740451, 0.001563293733823108503 ),
 .UNSPECIFIED. ) ;
#15672=VERTEX_POINT ( 'NONE', #30264 ) ;
#15673=CARTESIAN_POINT ( 'NONE',  ( -9.442253380669377805, -11.79725096376909299, 32.30694842903960762 ) ) ;
#15675=CARTESIAN_POINT ( 'NONE',  ( -4.854143535654665165, -3.236590943229499029, 32.36255958852954251 ) ) ;
#15676=CARTESIAN_POINT ( 'NONE',  ( -7.715628407920203102, -11.66157788607254098, 32.95092075102925833 ) ) ;
#15677=CARTESIAN_POINT ( 'NONE',  ( -16.94613126909829148, -11.18335022499818621, 33.13157742990016885 ) ) ;
#15678=CARTESIAN_POINT ( 'NONE',  ( -4.087778820496077437, -2.833524468853757750, 32.15551576947925838 ) ) ;
#15681=FACE_OUTER_BOUND ( 'NONE', #18815, .T. ) ;
#15682=AXIS2_PLACEMENT_3D ( 'NONE', #45518, #17153, #18053 ) ;
#15683=CARTESIAN_POINT ( 'NONE',  ( 15.29602480204525605, -11.94971097300157403, 32.03036669348361443 ) ) ;
#15684=CARTESIAN_POINT ( 'NONE',  ( -1.634592115557738090, -12.41269422305637171, 30.68257228309993323 ) ) ;
#15686=CARTESIAN_POINT ( 'NONE',  ( 12.23861150263161157, -12.64616026154729411, 30.79003144601914244 ) ) ;
#15687=CARTESIAN_POINT ( 'NONE',  ( 14.37294787896832915, -11.94971097300157403, 32.03036669348361443 ) ) ;
#15688=VECTOR ( 'NONE', #17318, 1000.000000000000000 ) ;
#15689=CARTESIAN_POINT ( 'NONE',  ( 14.05771557674995442, -6.567427716900048118, 34.66269422305636283 ) ) ;
#15690=EDGE_CURVE ( 'NONE', #17646, #21818, #51841, .T. ) ;
#15691=EDGE_LOOP ( 'NONE', ( #45875, #58275, #3088, #16051 ) ) ;
#15693=CARTESIAN_POINT ( 'NONE',  ( 7.780883845597524662, -5.094484230520674117, 34.41647553114621161 ) ) ;
#15695=CARTESIAN_POINT ( 'NONE',  ( 4.088576153289833037, -5.094484230520674117, 34.41647553114621161 ) ) ;
#15697=ORIENTED_EDGE ( 'NONE', *, *, #34909, .T. ) ;
#15698=EDGE_CURVE ( 'NONE', #57142, #17177, #59891, .T. ) ;
#15699=DIRECTION ( 'NONE',  ( -0.000000000000000000, -0.3420201433256694901, -0.9396926207859082059 ) ) ;
#15700=CARTESIAN_POINT ( 'NONE',  ( 12.46153846153846168, -5.557115091759785130, 34.35708131394839171 ) ) ;
#15701=ORIENTED_EDGE ( 'NONE', *, *, #40386, .T. ) ;
#15703=CARTESIAN_POINT ( 'NONE',  ( 17.01165307636676260, -2.657715359629089669, 31.77849191805833584 ) ) ;
#15704=VERTEX_POINT ( 'NONE', #31133 ) ;
#15705=CYLINDRICAL_SURFACE ( 'NONE', #46332, 0.2499999999999997502 ) ;
#15706=B_SPLINE_CURVE_WITH_KNOTS ( 'NONE', 3,
 ( #1334, #42338, #36885, #49954, #36020, #77872, #16178, #76105, #63474, #15302 ),
 .UNSPECIFIED., .F., .F.,
 ( 4, 2, 2, 2, 4 ),
 ( 0.000000000000000000, 0.0001954339857564080978, 0.0003908679715128161956, 0.0005863019572692242934, 0.0007817359430256323911 ),
 .UNSPECIFIED. ) ;
#15707=DIRECTION ( 'NONE',  ( 0.000000000000000000, 0.1736481776669275834, 0.9848077530122086864 ) ) ;
#15708=ORIENTED_EDGE ( 'NONE', *, *, #75218, .T. ) ;
#15709=DIRECTION ( 'NONE',  ( -0.000000000000000000, -0.9848077530122085754, -0.1736481776669273613 ) ) ;
#15710=B_SPLINE_CURVE_WITH_KNOTS ( 'NONE', 3,
 ( #51924, #4645, #4192, #86187, #80313, #18610, #58688, #80763, #59133, #10957 ),
 .UNSPECIFIED., .F., .F.,
 ( 4, 2, 2, 2, 4 ),
 ( 0.0007817246256747455461, 0.0009771112852218881168, 0.001172497944769030796, 0.001367884604316173475, 0.001563271263863316154 ),
 .UNSPECIFIED. ) ;
#15713=CARTESIAN_POINT ( 'NONE',  ( -9.442307692307691624, -2.499999999999998668, 29.75000000000000355 ) ) ;
#15715=ORIENTED_EDGE ( 'NONE', *, *, #43407, .T. ) ;
#15716=AXIS2_PLACEMENT_3D ( 'NONE', #25864, #73163, #52432 ) ;
#15717=EDGE_CURVE ( 'NONE', #34093, #59880, #86099, .T. ) ;
#15718=ORIENTED_EDGE ( 'NONE', *, *, #79367, .T. ) ;
#15719=ADVANCED_FACE ( 'NONE', ( #85650 ), #16737, .F. ) ;
#15720=CARTESIAN_POINT ( 'NONE',  ( 15.48082365068268018, -12.65882529074907126, 30.72640787790839312 ) ) ;
#15721=CARTESIAN_POINT ( 'NONE',  ( -14.53117725141625627, -3.236172620538810385, 32.36188796281390267 ) ) ;
#15723=EDGE_CURVE ( 'NONE', #75481, #51727, #78882, .T. ) ;
#15724=CYLINDRICAL_SURFACE ( 'NONE', #40623, 0.2499999999999986955 ) ;
#15725=ORIENTED_EDGE ( 'NONE', *, *, #48854, .F. ) ;
#15726=EDGE_LOOP ( 'NONE', ( #11770, #46242, #72549, #5732 ) ) ;
#15727=CARTESIAN_POINT ( 'NONE',  ( -2.373445736005638462, -7.249945578846654470, 34.99404164642496795 ) ) ;
#15728=ORIENTED_EDGE ( 'NONE', *, *, #17567, .T. ) ;
#15729=DIRECTION ( 'NONE',  ( -0.000000000000000000, 0.9848077530122085754, -0.1736481776669273613 ) ) ;
#15730=ORIENTED_EDGE ( 'NONE', *, *, #41973, .F. ) ;
#15731=VECTOR ( 'NONE', #69713, 1000.000000000000114 ) ;
#15732=VECTOR ( 'NONE', #28236, 1000.000000000000000 ) ;
#15734=CARTESIAN_POINT ( 'NONE',  ( 8.096099364501986528, -5.057305518903948638, 34.11320923018887896 ) ) ;
#15735=ORIENTED_EDGE ( 'NONE', *, *, #80063, .F. ) ;
#15736=EDGE_CURVE ( 'NONE', #61262, #16685, #84630, .T. ) ;
#15737=VECTOR ( 'NONE', #13345, 1000.000000000000227 ) ;
#15738=AXIS2_PLACEMENT_3D ( 'NONE', #8874, #1666, #42662 ) ;
#15740=CARTESIAN_POINT ( 'NONE',  ( 9.692307692307695177, -8.164416787775445883, 34.95778746994557906 ) ) ;
#15741=ORIENTED_EDGE ( 'NONE', *, *, #20905, .T. ) ;
#15742=AXIS2_PLACEMENT_3D ( 'NONE', #40190, #74859, #54117 ) ;
#15743=CARTESIAN_POINT ( 'NONE',  ( -0.7115616988314267255, -10.76384336483936011, 33.53834819971076087 ) ) ;
#15744=CARTESIAN_POINT ( 'NONE',  ( -6.923076923077044142, -3.835265460704628371, 33.15142922262033665 ) ) ;
#15745=EDGE_LOOP ( 'NONE', ( #23281, #6368, #23815, #84360 ) ) ;
#15746=CARTESIAN_POINT ( 'NONE',  ( 15.23076923076910916, -2.379036618888197729, 30.90682066428292885 ) ) ;
#15747=CARTESIAN_POINT ( 'NONE',  ( -2.557715544985270206, -5.056417327199099532, 34.11270091957320716 ) ) ;
#15748=CARTESIAN_POINT ( 'NONE',  ( 6.857806922520604864, -5.941354392334500467, 34.76329471203369792 ) ) ;
#15749=FACE_BOUND ( 'NONE', #52914, .T. ) ;
#15750=DIRECTION ( 'NONE',  ( -0.000000000000000000, -0.1736481776669307198, -0.9848077530122080203 ) ) ;
#15751=CARTESIAN_POINT ( 'NONE',  ( -6.923076923076922462, -12.10708131394839349, 31.69288490824020244 ) ) ;
#15752=CARTESIAN_POINT ( 'NONE',  ( -15.23076923076922995, -5.471508081941601098, 34.59228464037088457 ) ) ;
#15753=DIRECTION ( 'NONE',  ( -0.000000000000000000, 0.9848077530122085754, -0.1736481776669273613 ) ) ;
#15754=CARTESIAN_POINT ( 'NONE',  ( 4.403900573759605308, -2.318338780012835443, 30.59689888758630261 ) ) ;
#15755=CARTESIAN_POINT ( 'NONE',  ( -2.980714919130916574, -3.136992222400443175, 32.19305428654138979 ) ) ;
#15756=LINE ( 'NONE', #57614, #46197 ) ;
#15757=ORIENTED_EDGE ( 'NONE', *, *, #24031, .F. ) ;
#15758=DIRECTION ( 'NONE',  ( 0.000000000000000000, 0.8660254037844377084, -0.5000000000000015543 ) ) ;
#15759=ORIENTED_EDGE ( 'NONE', *, *, #70436, .F. ) ;
#15760=ORIENTED_EDGE ( 'NONE', *, *, #24182, .F. ) ;
#15762=CARTESIAN_POINT ( 'NONE',  ( 8.096099364501986528, -10.05730279482229683, 34.04704008940765902 ) ) ;
#15763=CARTESIAN_POINT ( 'NONE',  ( -5.869208192175211281, -6.413143153341454017, 34.63066358083362672 ) ) ;
#15764=FACE_OUTER_BOUND ( 'NONE', #22505, .T. ) ;
#15765=CARTESIAN_POINT ( 'NONE',  ( -10.48485917715096960, -12.50538340440932394, 31.33453814440721885 ) ) ;
#15766=CARTESIAN_POINT ( 'NONE',  ( 1.134592147322421862, -11.86270091957321249, 32.19358267280087915 ) ) ;
#15767=VERTEX_POINT ( 'NONE', #24373 ) ;
#15768=FACE_OUTER_BOUND ( 'NONE', #78452, .T. ) ;
#15769=ADVANCED_FACE ( 'NONE', ( #17641 ), #4563, .F. ) ;
#15770=CARTESIAN_POINT ( 'NONE',  ( -14.55766905174090020, -10.06842814019191401, 34.32929386961144758 ) ) ;
#15772=CARTESIAN_POINT ( 'NONE',  ( -18.00000000000000000, -8.164416787775447659, 34.95778746994557906 ) ) ;
#15773=B_SPLINE_CURVE_WITH_KNOTS ( 'NONE', 3,
 ( #54632, #8132, #60956, #12773, #35601, #1364, #60067, #40259, #56312, #83801 ),
 .UNSPECIFIED., .F., .F.,
 ( 4, 2, 2, 2, 4 ),
 ( 0.000000000000000000, 0.0001954311564186879315, 0.0003908623128373758630, 0.0005862934692560637946, 0.0007817246256747517261 ),
 .UNSPECIFIED. ) ;
#15774=FACE_OUTER_BOUND ( 'NONE', #39099, .T. ) ;
#15775=AXIS2_PLACEMENT_3D ( 'NONE', #84683, #49984, #43235 ) ;
#15777=ORIENTED_EDGE ( 'NONE', *, *, #86886, .F. ) ;
#15778=EDGE_CURVE ( 'NONE', #16542, #37672, #53494, .T. ) ;
#15779=ORIENTED_EDGE ( 'NONE', *, *, #4938, .T. ) ;
#15780=CARTESIAN_POINT ( 'NONE',  ( 3.480769230769230838, -2.499999999999998668, 29.75000000000000355 ) ) ;
#15781=ADVANCED_FACE ( 'NONE', ( #32474 ), #29, .F. ) ;
#15782=ORIENTED_EDGE ( 'NONE', *, *, #18060, .F. ) ;
#15783=CARTESIAN_POINT ( 'NONE',  ( -9.757578138268467427, -12.46129190929999986, 30.37095296980880832 ) ) ;
#15784=CARTESIAN_POINT ( 'NONE',  ( -12.46153846153846168, -6.386643153685126251, 34.62446782046654192 ) ) ;
#15785=CARTESIAN_POINT ( 'NONE',  ( 14.30769230769218581, -10.33852847137269571, 34.16647553114546554 ) ) ;
#15786=LINE ( 'NONE', #76596, #60105 ) ;
#15789=ORIENTED_EDGE ( 'NONE', *, *, #23423, .T. ) ;
#15790=EDGE_CURVE ( 'NONE', #51461, #65658, #2919, .T. ) ;
#15791=CARTESIAN_POINT ( 'NONE',  ( 16.15384615384615330, -12.78798330534103123, 29.99999999999997868 ) ) ;
#15792=CARTESIAN_POINT ( 'NONE',  ( 17.75000000000000000, -2.249999999999998668, 29.75000000000000355 ) ) ;
#15793=VERTEX_POINT ( 'NONE', #53183 ) ;
#15794=CARTESIAN_POINT ( 'NONE',  ( -10.48485891362104816, -3.816742781228458004, 33.13167719472716044 ) ) ;
#15795=CARTESIAN_POINT ( 'NONE',  ( 16.94677586748485965, -3.817052484675422797, 33.13202310037935661 ) ) ;
#15796=CARTESIAN_POINT ( 'NONE',  ( 15.36155967173618642, -2.845873456487966635, 32.17976146951972538 ) ) ;
#15797=CARTESIAN_POINT ( 'NONE',  ( -2.057637887778853703, -2.318338780012835443, 30.59689888758630261 ) ) ;
#15798=AXIS2_PLACEMENT_3D ( 'NONE', #1485, #55091, #41582 ) ;
#15801=EDGE_CURVE ( 'NONE', #5654, #13172, #80688, .T. ) ;
#15803=ORIENTED_EDGE ( 'NONE', *, *, #39418, .F. ) ;
#15804=CARTESIAN_POINT ( 'NONE',  ( -15.36145983387953962, -6.369640206132551441, 34.87707690430378449 ) ) ;
#15805=CARTESIAN_POINT ( 'NONE',  ( -1.514762594053607803, -12.27039167877662251, 31.24851455888617835 ) ) ;
#15807=B_SPLINE_CURVE_WITH_KNOTS ( 'NONE', 3,
 ( #9236, #8789, #64588, #22726, #84893, #23614, #15987, #23179, #51064, #71353 ),
 .UNSPECIFIED., .F., .F.,
 ( 4, 2, 2, 2, 4 ),
 ( 0.000000000000000000, 0.0001954311564186872810, 0.0003908623128373745620, 0.0005862934692560618430, 0.0007817246256747491240 ),
 .UNSPECIFIED. ) ;
#15808=AXIS2_PLACEMENT_3D ( 'NONE', #76207, #34779, #69010 ) ;
#15809=CARTESIAN_POINT ( 'NONE',  ( -13.51530685128294529, -12.38065189839062263, 30.83690757178629482 ) ) ;
#15810=LINE ( 'NONE', #70747, #50421 ) ;
#15811=ORIENTED_EDGE ( 'NONE', *, *, #11368, .T. ) ;
#15813=CARTESIAN_POINT ( 'NONE',  ( 11.53846153846153832, -3.937682226553329556, 33.60647404775216529 ) ) ;
#15814=EDGE_LOOP ( 'NONE', ( #33935, #61292, #28085, #44794 ) ) ;
#15815=AXIS2_PLACEMENT_3D ( 'NONE', #62149, #21601, #56277 ) ;
#15816=CARTESIAN_POINT ( 'NONE',  ( -0.6844654204453101132, -10.77366814457252175, 33.85459836347579454 ) ) ;
#15817=ORIENTED_EDGE ( 'NONE', *, *, #86135, .T. ) ;
#15818=CARTESIAN_POINT ( 'NONE',  ( 0.4615384615384611755, -13.37000171582298513, 34.34916445242398453 ) ) ;
#15819=CARTESIAN_POINT ( 'NONE',  ( 16.82692307692308020, -2.499999999999999556, 29.81609845454690699 ) ) ;
#15820=CARTESIAN_POINT ( 'NONE',  ( 7.846153846153846700, -5.557115091759785130, 34.35708131394839171 ) ) ;
#15823=CARTESIAN_POINT ( 'NONE',  ( -6.923076923077045919, -6.835583212225970762, 34.95778746994575670 ) ) ;
#15826=CARTESIAN_POINT ( 'NONE',  ( -17.86920955903304886, -11.93129842949672437, 32.56571108434900452 ) ) ;
#15827=CARTESIAN_POINT ( 'NONE',  ( 8.769230769230647482, -3.300289026999228881, 32.46337939537708905 ) ) ;
#15829=CARTESIAN_POINT ( 'NONE',  ( 8.546303810323914618, -4.762599654559228846, 34.23009711892697737 ) ) ;
#15830=FACE_OUTER_BOUND ( 'NONE', #53816, .T. ) ;
#15831=CARTESIAN_POINT ( 'NONE',  ( 11.53846153846153832, -1.129524287112498415, 32.06866353760679544 ) ) ;
#15832=EDGE_CURVE ( 'NONE', #55623, #17845, #7248, .T. ) ;
#15833=CARTESIAN_POINT ( 'NONE',  ( 1.161130460051055913, -6.716662450894490100, 34.94144148231605840 ) ) ;
#15834=CARTESIAN_POINT ( 'NONE',  ( -4.023320715612507925, -4.299079248970732792, 33.91157788607253565 ) ) ;
#15835=B_SPLINE_CURVE_WITH_KNOTS ( 'NONE', 3,
 ( #70337, #43744, #16709, #8644, #36553, #1435, #57262, #42431, #69888, #77974 ),
 .UNSPECIFIED., .F., .F.,
 ( 4, 2, 2, 2, 4 ),
 ( 0.000000000000000000, 0.0001954339857564083688, 0.0003908679715128167377, 0.0005863019572692250523, 0.0007817359430256334753 ),
 .UNSPECIFIED. ) ;
#15836=EDGE_LOOP ( 'NONE', ( #75234, #68112, #3425, #52812 ) ) ;
#15837=VERTEX_POINT ( 'NONE', #39699 ) ;
#15838=ADVANCED_FACE ( 'NONE', ( #46436 ), #81125, .F. ) ;
#15839=FACE_BOUND ( 'NONE', #86560, .T. ) ;
#15840=ORIENTED_EDGE ( 'NONE', *, *, #34592, .T. ) ;
#15841=CARTESIAN_POINT ( 'NONE',  ( 8.546304551714618114, -3.586966769969701208, 32.86292498521069660 ) ) ;
#15842=AXIS2_PLACEMENT_3D ( 'NONE', #9031, #22096, #28867 ) ;
#15843=DIRECTION ( 'NONE',  ( -0.000000000000000000, 0.1736481776669307198, -0.9848077530122080203 ) ) ;
#15844=CARTESIAN_POINT ( 'NONE',  ( 6.000000000000001776, -2.833524468853757305, 32.15551576947925838 ) ) ;
#15845=DIRECTION ( 'NONE',  ( -0.000000000000000000, 0.6427876096865404731, -0.7660444431189771253 ) ) ;
#15846=EDGE_CURVE ( 'NONE', #83859, #77663, #12215, .T. ) ;
#15847=EDGE_LOOP ( 'NONE', ( #86532, #74720 ) ) ;
#15848=ORIENTED_EDGE ( 'NONE', *, *, #57127, .T. ) ;
#15850=CARTESIAN_POINT ( 'NONE',  ( 2.557637826040450424, -4.336752205174647656, 33.62275283266504289 ) ) ;
#15851=ADVANCED_FACE ( 'NONE', ( #61712 ), #67603, .F. ) ;
#15852=ADVANCED_FACE ( 'NONE', ( #34250 ), #87905, .F. ) ;
#15853=VECTOR ( 'NONE', #36793, 1000.000000000000227 ) ;
#15854=DIRECTION ( 'NONE',  ( -0.000000000000000000, -0.7660444431189791237, -0.6427876096865379196 ) ) ;
#15855=CARTESIAN_POINT ( 'NONE',  ( 14.17700170458200759, -11.93127051446799847, 32.56575433478202797 ) ) ;
#15856=EDGE_CURVE ( 'NONE', #30760, #70329, #28797, .T. ) ;
#15857=DIRECTION ( 'NONE',  ( 0.000000000000000000, 0.3420201433256641055, -0.9396926207859100932 ) ) ;
#15858=EDGE_LOOP ( 'NONE', ( #752, #3741, #15527, #23603 ) ) ;
#15859=CARTESIAN_POINT ( 'NONE',  ( 8.899756470994333313, -9.417988943895561960, 34.36773134775777550 ) ) ;
#15860=CARTESIAN_POINT ( 'NONE',  ( -6.000000000000121680, -6.835583212225970762, 34.95778746994575670 ) ) ;
#15861=CARTESIAN_POINT ( 'NONE',  ( 4.153846153846154188, -10.51840700105979565, 33.73612834413961536 ) ) ;
#15862=CARTESIAN_POINT ( 'NONE',  ( 11.76147289007438523, -8.239487800360276282, 34.69522927552633718 ) ) ;
#15863=VERTEX_POINT ( 'NONE', #22508 ) ;
#15864=VERTEX_POINT ( 'NONE', #49092 ) ;
#15865=CIRCLE ( 'NONE', #27310, 0.2500000000000002220 ) ;
#15866=VERTEX_POINT ( 'NONE', #42354 ) ;
#15867=VECTOR ( 'NONE', #781, 1000.000000000000227 ) ;
#15868=CARTESIAN_POINT ( 'NONE',  ( 12.21156173059610772, -6.567427716900048118, 34.66269422305636283 ) ) ;
#15869=CARTESIAN_POINT ( 'NONE',  ( -9.561782254074046250, -8.630441415882550871, 34.87705825610312615 ) ) ;
#15871=B_SPLINE_CURVE_WITH_KNOTS ( 'NONE', 3,
 ( #30204, #86949, #10817, #58539, #44134, #59444, #3603, #16676, #71615, #9921 ),
 .UNSPECIFIED., .F., .F.,
 ( 4, 2, 2, 2, 4 ),
 ( 0.000000000000000000, 0.0001954339857564098867, 0.0003908679715128197734, 0.0005863019572692296059, 0.0007817359430256395469 ),
 .UNSPECIFIED. ) ;
#15872=DIRECTION ( 'NONE',  ( 0.000000000000000000, 0.9396926207859126468, -0.3420201433256571111 ) ) ;
#15873=CARTESIAN_POINT ( 'NONE',  ( -10.61538461538473399, -10.90142922262034020, 33.41473453929536674 ) ) ;
#15874=FACE_BOUND ( 'NONE', #30583, .T. ) ;
#15875=CARTESIAN_POINT ( 'NONE',  ( -2.438383774359865086, -9.804603061927743113, 34.18744698557895845 ) ) ;
#15876=VERTEX_POINT ( 'NONE', #35138 ) ;
#15878=CARTESIAN_POINT ( 'NONE',  ( 9.692307692307695177, -11.91647553114624181, 32.58852847137148245 ) ) ;
#15879=CARTESIAN_POINT ( 'NONE',  ( -17.14300648787895653, -11.69971097300155272, 32.46337939537587403 ) ) ;
#15880=CARTESIAN_POINT ( 'NONE',  ( -11.31545018684868964, -3.587049720035815348, 32.86302985866382897 ) ) ;
#15881=ORIENTED_EDGE ( 'NONE', *, *, #8313, .F. ) ;
#15882=DIRECTION ( 'NONE',  ( -0.000000000000000000, 0.3420201433256694346, -0.9396926207859080948 ) ) ;
#15883=ORIENTED_EDGE ( 'NONE', *, *, #47708, .F. ) ;
#15884=FACE_BOUND ( 'NONE', #20880, .T. ) ;
#15886=CARTESIAN_POINT ( 'NONE',  ( -16.82686876528476105, -4.235687564193445276, 33.53795663066793509 ) ) ;
#15887=CARTESIAN_POINT ( 'NONE',  ( 12.46153846153833911, -3.083524468854526912, 32.58852847137268327 ) ) ;
#15888=CARTESIAN_POINT ( 'NONE',  ( 12.23805351781451378, -12.24155766932282496, 31.33739205006857986 ) ) ;
#15889=ORIENTED_EDGE ( 'NONE', *, *, #54236, .T. ) ;
#15890=CARTESIAN_POINT ( 'NONE',  ( -12.68502340526241312, -10.11188796281391511, 34.01382737946119050 ) ) ;
#15891=CARTESIAN_POINT ( 'NONE',  ( 5.011166274408766164, -7.249945686854186278, 34.74374336980224598 ) ) ;
#15892=CARTESIAN_POINT ( 'NONE',  ( 8.546303810323914618, -2.308479472611653094, 30.53278059502174457 ) ) ;
#15893=DIRECTION ( 'NONE',  ( -0.000000000000000000, -0.5000000000000009992, -0.8660254037844380415 ) ) ;
#15894=ORIENTED_EDGE ( 'NONE', *, *, #71839, .F. ) ;
#15895=DIRECTION ( 'NONE',  ( -0.000000000000000000, 0.5000000000000011102, -0.8660254037844381525 ) ) ;
#15897=ADVANCED_FACE ( 'NONE', ( #8562 ), #1792, .F. ) ;
#15899=EDGE_LOOP ( 'NONE', ( #67247, #65547, #2470, #54107 ) ) ;
#15900=CARTESIAN_POINT ( 'NONE',  ( 7.596177115211490971, -10.66389620160130036, 33.62221079203477103 ) ) ;
#15901=CARTESIAN_POINT ( 'NONE',  ( -1.634592128663974853, -12.41104346484419452, 31.60698883733904196 ) ) ;
#15903=CARTESIAN_POINT ( 'NONE',  ( -12.39628289026243912, -2.892918686051626498, 31.69288490824026638 ) ) ;
#15904=CARTESIAN_POINT ( 'NONE',  ( 13.45068373561782593, -5.557115091759786019, 34.35708131394839882 ) ) ;
#15905=CARTESIAN_POINT ( 'NONE',  ( -11.78848476268299628, -9.356822207818506598, 34.66110646841856635 ) ) ;
#15906=CARTESIAN_POINT ( 'NONE',  ( -0.4615384615384611200, -1.509761064869970415, 31.06009739812519044 ) ) ;
#15909=ORIENTED_EDGE ( 'NONE', *, *, #61449, .F. ) ;
#15910=CYLINDRICAL_SURFACE ( 'NONE', #49131, 0.2499999999999994726 ) ;
#15911=CARTESIAN_POINT ( 'NONE',  ( 15.23076923076923173, -12.78798330534102767, 29.49999999999997868 ) ) ;
#15912=ORIENTED_EDGE ( 'NONE', *, *, #4038, .F. ) ;
#15913=ORIENTED_EDGE ( 'NONE', *, *, #69996, .T. ) ;
#15914=ORIENTED_EDGE ( 'NONE', *, *, #28018, .T. ) ;
#15915=CARTESIAN_POINT ( 'NONE',  ( 17.07692307692295586, -5.219633306517616589, 34.19971097300220464 ) ) ;
#15916=B_SPLINE_CURVE_WITH_KNOTS ( 'NONE', 3,
 ( #41633, #33554, #26786, #54245, #81741, #20025, #16808, #69981, #42526, #2401 ),
 .UNSPECIFIED., .F., .F.,
 ( 4, 2, 2, 2, 4 ),
 ( 0.000000000000000000, 0.0001954311564186863323, 0.0003908623128373726646, 0.0005862934692560590241, 0.0007817246256747453293 ),
 .UNSPECIFIED. ) ;
#15917=CARTESIAN_POINT ( 'NONE',  ( 6.223011351612852238, -11.24521262558773671, 33.06293181088029343 ) ) ;
#15918=CYLINDRICAL_SURFACE ( 'NONE', #24101, 0.2499999999999993616 ) ;
#15919=CARTESIAN_POINT ( 'NONE',  ( 8.834485908743605620, -11.67786785259547777, 32.92929555188713664 ) ) ;
#15920=CARTESIAN_POINT ( 'NONE',  ( -13.16183571563731647, -6.717445702608402236, 34.94155399931962336 ) ) ;
#15921=EDGE_CURVE ( 'NONE', #38438, #22548, #80315, .T. ) ;
#15922=CARTESIAN_POINT ( 'NONE',  ( 18.00000000000000000, -1.951392089020283160, 34.73218667398347748 ) ) ;
#15923=CARTESIAN_POINT ( 'NONE',  ( -20.74999999999999645, -7.500000000000000000, 29.75000000000000355 ) ) ;
#15924=CARTESIAN_POINT ( 'NONE',  ( -3.903900635498010807, -5.852078868378310261, 34.47109172314383585 ) ) ;
#15925=CARTESIAN_POINT ( 'NONE',  ( -17.29984929443921970, -12.15238873228291716, 31.58232369045353849 ) ) ;
#15926=CIRCLE ( 'NONE', #49022, 0.2500000000000002220 ) ;
#15927=CARTESIAN_POINT ( 'NONE',  ( 2.057715576749953978, -3.627789207965226748, 32.91389620160131102 ) ) ;
#15928=CARTESIAN_POINT ( 'NONE',  ( 15.23076923076923173, -12.10708131394839349, 31.69288490824020244 ) ) ;
#15929=EDGE_CURVE ( 'NONE', #56147, #50666, #13785, .T. ) ;
#15930=ORIENTED_EDGE ( 'NONE', *, *, #85067, .F. ) ;
#15931=CARTESIAN_POINT ( 'NONE',  ( 15.00728428704528561, -11.41268669641499756, 32.86336882939238535 ) ) ;
#15933=CARTESIAN_POINT ( 'NONE',  ( 12.46153846153846168, -2.833524468853757305, 32.15551576947925838 ) ) ;
#15934=ORIENTED_EDGE ( 'NONE', *, *, #68888, .F. ) ;
#15935=EDGE_CURVE ( 'NONE', #20644, #80080, #8370, .T. ) ;
#15936=CARTESIAN_POINT ( 'NONE',  ( -2.307692307692428724, -6.835583212225970762, 34.95778746994575670 ) ) ;
#15937=AXIS2_PLACEMENT_3D ( 'NONE', #77674, #56956, #30379 ) ;
#15938=CARTESIAN_POINT ( 'NONE',  ( 9.442284468086239002, -2.985938066672154445, 32.43141759479405550 ) ) ;
#15939=PRODUCT_DEFINITION_FORMATION_WITH_SPECIFIED_SOURCE ( 'ANY', '', #963, .NOT_KNOWN. ) ;
#15940=CARTESIAN_POINT ( 'NONE',  ( -8.834500769787091201, -9.528491918058357157, 34.59228464037090589 ) ) ;
#15941=B_SPLINE_CURVE_WITH_KNOTS ( 'NONE', 3,
 ( #88492, #68200, #61865, #60546, #88061, #54664, #40734, #81719, #6499, #13691 ),
 .UNSPECIFIED., .F., .F.,
 ( 4, 2, 2, 2, 4 ),
 ( 0.000000000000000000, 0.0001954311564186878502, 0.0003908623128373757004, 0.0005862934692560635777, 0.0007817246256747514008 ),
 .UNSPECIFIED. ) ;
#15942=EDGE_CURVE ( 'NONE', #54183, #88905, #83515, .T. ) ;
#15944=CARTESIAN_POINT ( 'NONE',  ( -1.384615384615383471, -3.513871655860378418, 32.76840700105978499 ) ) ;
#15945=ADVANCED_FACE ( 'NONE', ( #76121 ), #14422, .F. ) ;
#15947=CARTESIAN_POINT ( 'NONE',  ( -3.453695448285377445, -12.15238873228292071, 31.58232369045353849 ) ) ;
#15948=CARTESIAN_POINT ( 'NONE',  ( 12.23861224402231151, -8.239355502252617924, 34.69524867566427417 ) ) ;
#15949=CARTESIAN_POINT ( 'NONE',  ( 1.319345384059067428, -8.656820664281497102, 34.87096338111211935 ) ) ;
#15950=CYLINDRICAL_SURFACE ( 'NONE', #30873, 0.2499999999999986955 ) ;
#15951=EDGE_CURVE ( 'NONE', #55459, #25295, #14740, .T. ) ;
#15952=ORIENTED_EDGE ( 'NONE', *, *, #21224, .T. ) ;
#15954=EDGE_CURVE ( 'NONE', #67048, #56388, #63057, .T. ) ;
#15956=EDGE_CURVE ( 'NONE', #27257, #74976, #30932, .T. ) ;
#15957=ORIENTED_EDGE ( 'NONE', *, *, #49266, .F. ) ;
#15958=CARTESIAN_POINT ( 'NONE',  ( -6.249976730942353065, -11.28823185664190376, 33.01397839955799896 ) ) ;
#15959=CARTESIAN_POINT ( 'NONE',  ( -13.38461538461538325, -1.790695186598648903, 34.54067556320373455 ) ) ;
#15960=VECTOR ( 'NONE', #77279, 1000.000000000000000 ) ;
#15961=CARTESIAN_POINT ( 'NONE',  ( -4.153846153846274980, -12.51329471203414379, 31.30864560766407578 ) ) ;
#15962=CARTESIAN_POINT ( 'NONE',  ( 15.23076923076923173, -10.89733346790207413, 36.13435417666054406 ) ) ;
#15963=CARTESIAN_POINT ( 'NONE',  ( -17.77698864838715309, -4.187068189119697692, 33.49521262558774026 ) ) ;
#15964=LINE ( 'NONE', #56935, #29424 ) ;
#15965=EDGE_LOOP ( 'NONE', ( #11741, #80183 ) ) ;
#15966=ORIENTED_EDGE ( 'NONE', *, *, #58338, .F. ) ;
#15967=B_SPLINE_CURVE_WITH_KNOTS ( 'NONE', 3,
 ( #76007, #13861, #14307, #14760, #21053, #76461, #21957, #1232, #7109, #21502 ),
 .UNSPECIFIED., .F., .F.,
 ( 4, 2, 2, 2, 4 ),
 ( 0.0007817246256747550871, 0.0009771112852218989588, 0.001172497944769042939, 0.001367884604316186702, 0.001563271263863330682 ),
 .UNSPECIFIED. ) ;
#15969=CARTESIAN_POINT ( 'NONE',  ( -2.980823712421088345, -10.76462480002816235, 33.53768742498949962 ) ) ;
#15970=ORIENTED_EDGE ( 'NONE', *, *, #76926, .F. ) ;
#15971=B_SPLINE_CURVE_WITH_KNOTS ( 'NONE', 3,
 ( #2553, #43115, #23709, #30911, #37678, #9763, #49860, #16968, #43548, #22832 ),
 .UNSPECIFIED., .F., .F.,
 ( 4, 2, 2, 2, 4 ),
 ( 0.0007817246256747497745, 0.0009771112852218937547, 0.001172497944769037518, 0.001367884604316181498, 0.001563271263863325478 ),
 .UNSPECIFIED. ) ;
#15972=DIRECTION ( 'NONE',  ( -0.000000000000000000, 0.5000000000000011102, -0.8660254037844380415 ) ) ;
#15973=LINE ( 'NONE', #84879, #27580 ) ;
#15974=CARTESIAN_POINT ( 'NONE',  ( 13.38461538461526601, -8.613356846316285953, 34.62446782046622218 ) ) ;
#15975=ORIENTED_EDGE ( 'NONE', *, *, #50866, .F. ) ;
#15977=VECTOR ( 'NONE', #55452, 1000.000000000000000 ) ;
#15978=ORIENTED_EDGE ( 'NONE', *, *, #45472, .F. ) ;
#15979=CARTESIAN_POINT ( 'NONE',  ( -17.86920955903304886, -2.845873456487967079, 32.17976146951973959 ) ) ;
#15980=VERTEX_POINT ( 'NONE', #66148 ) ;
#15981=FACE_BOUND ( 'NONE', #67365, .T. ) ;
#15982=CARTESIAN_POINT ( 'NONE',  ( 8.769230769230768274, -3.669653830205710676, 35.88435417666054406 ) ) ;
#15984=CARTESIAN_POINT ( 'NONE',  ( 15.93091993633000847, -6.503392248772476236, 34.64988816332204635 ) ) ;
#15986=CARTESIAN_POINT ( 'NONE',  ( 16.40379167219429846, -11.37275283266504111, 32.91324779482534524 ) ) ;
#15987=CARTESIAN_POINT ( 'NONE',  ( 4.853438152358744873, -8.539481045369598178, 34.89627647299170832 ) ) ;
#15988=CARTESIAN_POINT ( 'NONE',  ( 2.307692307692309264, -4.098570777380720287, 33.41473453929634729 ) ) ;
#15990=CARTESIAN_POINT ( 'NONE',  ( 1.515140822849028179, -2.647132371071621471, 31.75357179365173010 ) ) ;
#15992=CARTESIAN_POINT ( 'NONE',  ( 8.769230769230768274, -11.35647404775217417, 33.31231777344666511 ) ) ;
#15994=CARTESIAN_POINT ( 'NONE',  ( -7.846153846153844924, -13.20930481340135110, 34.54067556320372745 ) ) ;
#15995=LINE ( 'NONE', #35826, #2600 ) ;
#15996=CARTESIAN_POINT ( 'NONE',  ( -18.13069146666755671, -6.413092428213692742, 34.63065189839063152 ) ) ;
#15997=FACE_BOUND ( 'NONE', #50868, .T. ) ;
#15998=B_SPLINE_CURVE_WITH_KNOTS ( 'NONE', 3,
 ( #40981, #40549, #5867, #62132, #53602, #437, #27465, #54036, #33778, #82420 ),
 .UNSPECIFIED., .F., .F.,
 ( 4, 2, 2, 2, 4 ),
 ( 0.000000000000000000, 0.0001954311564186879857, 0.0003908623128373759715, 0.0005862934692560640114, 0.0007817246256747519429 ),
 .UNSPECIFIED. ) ;
#16000=CARTESIAN_POINT ( 'NONE',  ( -15.23076923076922995, -4.098570777380720287, 33.41473453929634729 ) ) ;
#16001=DIRECTION ( 'NONE',  ( 0.000000000000000000, 0.9396926207859126468, 0.3420201433256571111 ) ) ;
#16002=CARTESIAN_POINT ( 'NONE',  ( -6.923076923076922462, -1.466349020453238561, 30.81389545987213907 ) ) ;
#16004=CARTESIAN_POINT ( 'NONE',  ( 8.769230769230647482, -11.48612834414049644, 32.76840700105863391 ) ) ;
#16008=VERTEX_POINT ( 'NONE', #29719 ) ;
#16009=CYLINDRICAL_SURFACE ( 'NONE', #20505, 0.2499999999999994726 ) ;
#16010=ORIENTED_EDGE ( 'NONE', *, *, #62187, .T. ) ;
#16011=CARTESIAN_POINT ( 'NONE',  ( 17.99999999999987566, -12.27809138561165270, 31.22303859784587132 ) ) ;
#16012=ORIENTED_EDGE ( 'NONE', *, *, #20299, .F. ) ;
#16013=DIRECTION ( 'NONE',  ( -0.000000000000000000, -0.9396926207859093161, -0.3420201433256663259 ) ) ;
#16015=CARTESIAN_POINT ( 'NONE',  ( 17.20744877868664346, -8.586989748646450593, 34.63063291749215011 ) ) ;
#16016=CARTESIAN_POINT ( 'NONE',  ( 6.988332062589762472, -10.33852847137154107, 34.16647553114620450 ) ) ;
#16018=CARTESIAN_POINT ( 'NONE',  ( -3.903846153846152855, -7.500000000000001776, 35.04278698407183867 ) ) ;
#16020=CARTESIAN_POINT ( 'NONE',  ( 6.923076923076924238, -13.87047571288749737, 32.06866353760679544 ) ) ;
#16021=AXIS2_PLACEMENT_3D ( 'NONE', #13499, #870, #41418 ) ;
#16023=CARTESIAN_POINT ( 'NONE',  ( -10.54931626438217407, -2.721908614388772296, 31.22303859784725333 ) ) ;
#16024=CARTESIAN_POINT ( 'NONE',  ( -2.307692307692305711, -11.91647553114624181, 32.58852847137148245 ) ) ;
#16025=VECTOR ( 'NONE', #67645, 1000.000000000000114 ) ;
#16026=CARTESIAN_POINT ( 'NONE',  ( -2.438383774359863310, -4.118384482072085184, 33.43331474514187107 ) ) ;
#16028=EDGE_CURVE ( 'NONE', #49403, #70118, #43660, .T. ) ;
#16030=ORIENTED_EDGE ( 'NONE', *, *, #9542, .T. ) ;
#16031=CARTESIAN_POINT ( 'NONE',  ( -13.63459212866397685, -6.524016743844655686, 34.90889640711025521 ) ) ;
#16032=CARTESIAN_POINT ( 'NONE',  ( 12.23861150263161335, -8.282780595021769443, 34.94152052738834868 ) ) ;
#16033=CARTESIAN_POINT ( 'NONE',  ( 9.692307692307572609, -6.879047030192662504, 34.71129190930017927 ) ) ;
#16034=CARTESIAN_POINT ( 'NONE',  ( 14.98076923076922995, -7.566082377512564960, 35.00000000000000711 ) ) ;
#16035=B_SPLINE_CURVE_WITH_KNOTS ( 'NONE', 3,
 ( #40238, #47414, #13637, #46543, #19946, #6009, #128, #46100, #67702, #6879 ),
 .UNSPECIFIED., .F., .F.,
 ( 4, 2, 2, 2, 4 ),
 ( 0.000000000000000000, 0.0001954339857564081520, 0.0003908679715128163040, 0.0005863019572692244018, 0.0007817359430256326080 ),
 .UNSPECIFIED. ) ;
#16036=CARTESIAN_POINT ( 'NONE',  ( -3.230769230769229949, -2.499999999999998668, 29.75000000000001421 ) ) ;
#16037=CARTESIAN_POINT ( 'NONE',  ( -14.05763788777885281, -4.074993327901527351, 33.72946981652012255 ) ) ;
#16038=B_SPLINE_CURVE_WITH_KNOTS ( 'NONE', 3,
 ( #57701, #84752, #50489, #85182, #23462, #49618 ),
 .UNSPECIFIED., .F., .F.,
 ( 4, 2, 4 ),
 ( 0.0003909512603273906169, 0.0005862562993132179340, 0.0007815613382990451970 ),
 .UNSPECIFIED. ) ;
#16039=LINE ( 'NONE', #21907, #72072 ) ;
#16040=EDGE_CURVE ( 'NONE', #29682, #81991, #10431, .T. ) ;
#16041=ORIENTED_EDGE ( 'NONE', *, *, #22123, .T. ) ;
#16042=ORIENTED_EDGE ( 'NONE', *, *, #771, .T. ) ;
#16043=ORIENTED_EDGE ( 'NONE', *, *, #41663, .T. ) ;
#16044=CARTESIAN_POINT ( 'NONE',  ( 3.453780582382080855, -5.667800583137508674, 34.40243808032445827 ) ) ;
#16045=FACE_OUTER_BOUND ( 'NONE', #10603, .T. ) ;
#16046=CARTESIAN_POINT ( 'NONE',  ( -13.31854703361294767, -8.973038597847271092, 34.52809138561121216 ) ) ;
#16047=CARTESIAN_POINT ( 'NONE',  ( 10.74591005361826213, -10.31582465632705237, 34.18122507451815295 ) ) ;
#16048=VECTOR ( 'NONE', #17006, 1000.000000000000227 ) ;
#16049=EDGE_LOOP ( 'NONE', ( #30560, #79792, #19359, #35726 ) ) ;
#16050=FACE_OUTER_BOUND ( 'NONE', #46467, .T. ) ;
#16051=ORIENTED_EDGE ( 'NONE', *, *, #50996, .F. ) ;
#16052=EDGE_CURVE ( 'NONE', #85070, #40219, #22241, .T. ) ;
#16053=ORIENTED_EDGE ( 'NONE', *, *, #42392, .F. ) ;
#16054=CARTESIAN_POINT ( 'NONE',  ( -7.846153846153965716, -5.219633306517616589, 34.19971097300220464 ) ) ;
#16055=CARTESIAN_POINT ( 'NONE',  ( -11.53846153846153655, -11.16473453929635440, 33.15142922261926373 ) ) ;
#16056=EDGE_CURVE ( 'NONE', #48397, #30065, #78166, .T. ) ;
#16057=B_SPLINE_CURVE_WITH_KNOTS ( 'NONE', 3,
 ( #86747, #45732, #30875, #73213, #85838, #44830, #79074, #80418, #17373, #24117 ),
 .UNSPECIFIED., .F., .F.,
 ( 4, 2, 2, 2, 4 ),
 ( 0.0007817246256747522682, 0.0009771112852218972241, 0.001172497944769042288, 0.001367884604316187353, 0.001563271263863332417 ),
 .UNSPECIFIED. ) ;
#16058=DIRECTION ( 'NONE',  ( -1.000000000000000000, 0.000000000000000000, 0.000000000000000000 ) ) ;
#16059=ADVANCED_FACE ( 'NONE', ( #32822 ), #45879, .F. ) ;
#16060=B_SPLINE_CURVE_WITH_KNOTS ( 'NONE', 3,
 ( #17905, #38168, #72835, #32745, #39076, #59773, #88168, #87719, #39523, #45810 ),
 .UNSPECIFIED., .F., .F.,
 ( 4, 2, 2, 2, 4 ),
 ( 0.0007817359430256253438, 0.0009771253907249898181, 0.001172514838424354401, 0.001367904286123718983, 0.001563293733823083566 ),
 .UNSPECIFIED. ) ;
#16064=ORIENTED_EDGE ( 'NONE', *, *, #10027, .F. ) ;
#16066=ORIENTED_EDGE ( 'NONE', *, *, #34838, .F. ) ;
#16067=CARTESIAN_POINT ( 'NONE',  ( -11.53846153846166089, -12.70778746994576025, 30.41441678777401236 ) ) ;
#16068=EDGE_LOOP ( 'NONE', ( #5327, #48167 ) ) ;
#16069=CARTESIAN_POINT ( 'NONE',  ( 18.00000000000000000, -6.435427911321262684, 35.78748833219616898 ) ) ;
#16070=DIRECTION ( 'NONE',  ( -0.000000000000000000, -0.000000000000000000, -1.000000000000000000 ) ) ;
#16071=CARTESIAN_POINT ( 'NONE',  ( 6.988332494352947677, -11.94971097300157403, 32.03036669348361443 ) ) ;
#16074=LINE ( 'NONE', #43537, #72415 ) ;
#16076=ORIENTED_EDGE ( 'NONE', *, *, #17879, .F. ) ;
#16077=FACE_BOUND ( 'NONE', #64318, .T. ) ;
#16078=B_SPLINE_CURVE_WITH_KNOTS ( 'NONE', 3,
 ( #89052, #41295, #20567, #7056, #48031, #14258, #40415, #83166, #81400, #34964 ),
 .UNSPECIFIED., .F., .F.,
 ( 4, 2, 2, 2, 4 ),
 ( 0.000000000000000000, 0.0001954339857564063089, 0.0003908679715128126177, 0.0005863019572692189808, 0.0007817359430256252354 ),
 .UNSPECIFIED. ) ;
#16079=CARTESIAN_POINT ( 'NONE',  ( 11.31553532094539172, -4.887634598454295265, 34.01352882383564946 ) ) ;
#16080=CARTESIAN_POINT ( 'NONE',  ( -17.07692307692307665, -12.48256725967547354, 35.29906147534542527 ) ) ;
#16081=CARTESIAN_POINT ( 'NONE',  ( -39.05038313613820122, -12.50000000000000000, 27.25000000000000000 ) ) ;
#16082=LINE ( 'NONE', #17413, #60465 ) ;
#16083=CARTESIAN_POINT ( 'NONE',  ( 5.011652630962299959, -3.300289026998414865, 32.46337939537583139 ) ) ;
#16084=CARTESIAN_POINT ( 'NONE',  ( 4.946231610255516387, -2.541943142973490666, 30.39792223712631980 ) ) ;
#16085=CARTESIAN_POINT ( 'NONE',  ( 14.30769230769218581, -2.379036618888197729, 30.90682066428292885 ) ) ;
#16086=EDGE_LOOP ( 'NONE', ( #33866, #10498 ) ) ;
#16087=CARTESIAN_POINT ( 'NONE',  ( -10.86540785267757947, -10.05641848906368097, 34.04755513067966177 ) ) ;
#16088=CARTESIAN_POINT ( 'NONE',  ( -17.01085574357299990, -6.343179335718451384, 34.87096338111212646 ) ) ;
#16089=ORIENTED_EDGE ( 'NONE', *, *, #34225, .F. ) ;
#16091=CARTESIAN_POINT ( 'NONE',  ( 16.94623247381277054, -10.70098750199973203, 33.91152734681376302 ) ) ;
#16092=DIRECTION ( 'NONE',  ( 0.000000000000000000, 0.000000000000000000, 1.000000000000000000 ) ) ;
#16093=CARTESIAN_POINT ( 'NONE',  ( 2.084207383127978819, -5.827078755546623690, 34.72654668319379567 ) ) ;
#16094=CARTESIAN_POINT ( 'NONE',  ( -0.4615384615385826339, -12.46129190930018460, 30.37095296980731973 ) ) ;
#16095=CARTESIAN_POINT ( 'NONE',  ( 12.46153846153846168, -4.098570777380720287, 33.41473453929634729 ) ) ;
#16096=FACE_BOUND ( 'NONE', #16068, .T. ) ;
#16097=DIRECTION ( 'NONE',  ( 0.000000000000000000, 0.9848077530122072432, 0.1736481776669354937 ) ) ;
#16098=CARTESIAN_POINT ( 'NONE',  ( 1.634669696253701288, -2.564540009722895419, 30.55348353981670684 ) ) ;
#16099=B_SPLINE_CURVE_WITH_KNOTS ( 'NONE', 3,
 ( #16094, #37237, #64709, #8014, #84130, #29185, #1695, #49442, #8902, #50746 ),
 .UNSPECIFIED., .F., .F.,
 ( 4, 2, 2, 2, 4 ),
 ( 0.0007817359430256330417, 0.0009771253907250000096, 0.001172514838424367194, 0.001367904286123734162, 0.001563293733823101130 ),
 .UNSPECIFIED. ) ;
#16101=CARTESIAN_POINT ( 'NONE',  ( -7.846153846153844924, -12.62096338111211580, 30.90682066428153263 ) ) ;
#16103=B_SPLINE_CURVE_WITH_KNOTS ( 'NONE', 3,
 ( #1599, #2034, #29086, #56540, #69169, #84030, #77250, #14223, #36277, #7474 ),
 .UNSPECIFIED., .F., .F.,
 ( 4, 2, 2, 2, 4 ),
 ( 0.0007817246256747469556, 0.0009771112852218902852, 0.001172497944769033615, 0.001367884604316176728, 0.001563271263863320057 ),
 .UNSPECIFIED. ) ;
#16104=LINE ( 'NONE', #3464, #46159 ) ;
#16106=VECTOR ( 'NONE', #37349, 1000.000000000000114 ) ;
#16107=ORIENTED_EDGE ( 'NONE', *, *, #47261, .T. ) ;
#16108=VECTOR ( 'NONE', #32997, 1000.000000000000227 ) ;
#16109=DIRECTION ( 'NONE',  ( 0.000000000000000000, -6.938893903907222067E-15, 1.000000000000000000 ) ) ;
#16110=FACE_OUTER_BOUND ( 'NONE', #82328, .T. ) ;
#16111=CARTESIAN_POINT ( 'NONE',  ( -9.469296340694841163, -9.086983370893049639, 34.49168942202179267 ) ) ;
#16112=CARTESIAN_POINT ( 'NONE',  ( 3.230769230769231726, -13.37000171582298513, 34.34916445242398453 ) ) ;
#16113=CARTESIAN_POINT ( 'NONE',  ( -4.219928533206289245, -4.661471528628507777, 34.16647553114621871 ) ) ;
#16117=FACE_OUTER_BOUND ( 'NONE', #85547, .T. ) ;
#16118=CARTESIAN_POINT ( 'NONE',  ( 3.903822929624694904, -12.07920672191015221, 32.31858351112116168 ) ) ;
#16119=CARTESIAN_POINT ( 'NONE',  ( 3.361559671736181976, -3.957578996910244395, 33.62503395064540257 ) ) ;
#16120=CARTESIAN_POINT ( 'NONE',  ( 10.55011461482829738, -6.835583212224499938, 34.95778746994557906 ) ) ;
#16121=CARTESIAN_POINT ( 'NONE',  ( 2.557692307692323475, -2.249999999999999112, 29.81603969181031033 ) ) ;
#16122=CARTESIAN_POINT ( 'NONE',  ( 12.46153846153846168, -12.62096338111211580, 30.90682066428153263 ) ) ;
#16123=CARTESIAN_POINT ( 'NONE',  ( 14.55774661933062575, -11.79725096376909654, 32.30694842903959341 ) ) ;
#16124=CARTESIAN_POINT ( 'NONE',  ( -14.30769230769230660, -12.78798330534102945, 29.74999999999997868 ) ) ;
#16125=ORIENTED_EDGE ( 'NONE', *, *, #49514, .F. ) ;
#16127=CARTESIAN_POINT ( 'NONE',  ( -1.449865316389469028, -2.255955759149247619, 30.00000000000013856 ) ) ;
#16129=ADVANCED_FACE ( 'NONE', ( #40038 ), #60730, .F. ) ;
#16130=FACE_OUTER_BOUND ( 'NONE', #5052, .T. ) ;
#16131=CARTESIAN_POINT ( 'NONE',  ( -4.153846153846152411, -13.37000171582298513, 34.34916445242398453 ) ) ;
#16132=VERTEX_POINT ( 'NONE', #11669 ) ;
#16133=CARTESIAN_POINT ( 'NONE',  ( -14.30769230769242917, -9.528491918059723176, 34.59228464037033035 ) ) ;
#16134=CARTESIAN_POINT ( 'NONE',  ( -7.780898706641007578, -12.51329471203373700, 31.30864560766537963 ) ) ;
#16135=EDGE_LOOP ( 'NONE', ( #9305, #74564, #79348, #72255 ) ) ;
#16136=CARTESIAN_POINT ( 'NONE',  ( -15.23076923076922995, -12.09954503811598769, 35.62045528018868623 ) ) ;
#16137=CARTESIAN_POINT ( 'NONE',  ( 4.023154687178594813, -8.147922237126337563, 34.70805685702651999 ) ) ;
#16139=B_SPLINE_CURVE_WITH_KNOTS ( 'NONE', 3,
 ( #82587, #75805, #50099, #7800, #69055, #84356, #56428, #83470, #76700, #83916 ),
 .UNSPECIFIED., .F., .F.,
 ( 4, 2, 2, 2, 4 ),
 ( 0.0007817359430256372700, 0.0009771253907250052138, 0.001172514838424373266, 0.001367904286123741101, 0.001563293733823109153 ),
 .UNSPECIFIED. ) ;
#16140=DIRECTION ( 'NONE',  ( -0.000000000000000000, -0.3420201433256694346, -0.9396926207859080948 ) ) ;
#16141=CARTESIAN_POINT ( 'NONE',  ( 8.769230769230768274, -4.786620604624113540, 33.94971097300155094 ) ) ;
#16142=VERTEX_POINT ( 'NONE', #26065 ) ;
#16143=B_SPLINE_CURVE_WITH_KNOTS ( 'NONE', 3,
 ( #62313, #67319, #40739, #41616, #5614, #88942, #75403, #13697, #27213, #68640 ),
 .UNSPECIFIED., .F., .F.,
 ( 4, 2, 2, 2, 4 ),
 ( 0.000000000000000000, 0.0001954339857564090465, 0.0003908679715128180929, 0.0005863019572692271123, 0.0007817359430256361858 ),
 .UNSPECIFIED. ) ;
#16144=CARTESIAN_POINT ( 'NONE',  ( -12.71156168575991785, -2.341070481393819236, 30.72580821765574299 ) ) ;
#16145=CARTESIAN_POINT ( 'NONE',  ( -15.90379184220783948, -3.136992222400443175, 32.19305428654138979 ) ) ;
#16147=EDGE_CURVE ( 'NONE', #12780, #12459, #6124, .T. ) ;
#16148=VERTEX_POINT ( 'NONE', #4912 ) ;
#16149=AXIS2_PLACEMENT_3D ( 'NONE', #4050, #26117, #59896 ) ;
#16152=EDGE_CURVE ( 'NONE', #62016, #45177, #86810, .T. ) ;
#16153=CARTESIAN_POINT ( 'NONE',  ( -18.22348494372394612, -3.754499324213722122, 33.06261337010820256 ) ) ;
#16154=DIRECTION ( 'NONE',  ( 0.000000000000000000, 0.9848077530122072432, 0.1736481776669354937 ) ) ;
#16157=FACE_OUTER_BOUND ( 'NONE', #3716, .T. ) ;
#16159=EDGE_LOOP ( 'NONE', ( #77472, #74219, #42494, #22963 ) ) ;
#16160=ORIENTED_EDGE ( 'NONE', *, *, #29541, .F. ) ;
#16161=CARTESIAN_POINT ( 'NONE',  ( -1.319469605283419389, -7.750023238201980469, 34.74374492549440419 ) ) ;
#16162=ORIENTED_EDGE ( 'NONE', *, *, #54939, .F. ) ;
#16164=CARTESIAN_POINT ( 'NONE',  ( 16.28463659481310799, -8.191423895709842640, 34.95447573519442130 ) ) ;
#16166=VECTOR ( 'NONE', #23782, 1000.000000000000227 ) ;
#16167=EDGE_CURVE ( 'NONE', #27137, #62928, #21217, .T. ) ;
#16168=EDGE_CURVE ( 'NONE', #88199, #44873, #17932, .T. ) ;
#16169=LINE ( 'NONE', #36010, #32054 ) ;
#16171=ORIENTED_EDGE ( 'NONE', *, *, #57988, .F. ) ;
#16173=LINE ( 'NONE', #43636, #27241 ) ;
#16174=VERTEX_POINT ( 'NONE', #22725 ) ;
#16175=DIRECTION ( 'NONE',  ( -0.000000000000000000, -0.8660254037844399289, -0.4999999999999980016 ) ) ;
#16176=CARTESIAN_POINT ( 'NONE',  ( -15.90379184220783948, -3.627508038966690496, 32.91356715214248396 ) ) ;
#16177=ORIENTED_EDGE ( 'NONE', *, *, #14770, .T. ) ;
#16178=CARTESIAN_POINT ( 'NONE',  ( 15.93036121012220541, -12.44517049084099725, 30.48991314939691932 ) ) ;
#16179=CARTESIAN_POINT ( 'NONE',  ( -2.372962753653081958, -5.219633306516282545, 34.19971097300152252 ) ) ;
#16180=CARTESIAN_POINT ( 'NONE',  ( 10.61538461538449596, -3.835265460704628371, 33.15142922262033665 ) ) ;
#16181=FACE_BOUND ( 'NONE', #37295, .T. ) ;
#16182=CARTESIAN_POINT ( 'NONE',  ( 14.30769230769231015, -5.557115091759785130, 34.35708131394839171 ) ) ;
#16183=CARTESIAN_POINT ( 'NONE',  ( 11.31553532094539172, -8.239355502252617924, 34.69524867566427417 ) ) ;
#16184=CARTESIAN_POINT ( 'NONE',  ( -15.16551365949320740, -10.90142922261932057, 33.41473453929631887 ) ) ;
#16185=CARTESIAN_POINT ( 'NONE',  ( -16.85391023282967993, -12.38742843783360748, 31.66772728687926985 ) ) ;
#16186=CARTESIAN_POINT ( 'NONE',  ( 6.673053685783957967, -11.86270091957321249, 32.19358267280087915 ) ) ;
#16187=DIRECTION ( 'NONE',  ( 0.000000000000000000, 0.000000000000000000, 1.000000000000000000 ) ) ;
#16188=CARTESIAN_POINT ( 'NONE',  ( -9.915173955370791603, -2.251424796025575326, 29.88072029997477586 ) ) ;
#16189=EDGE_LOOP ( 'NONE', ( #29685, #66395 ) ) ;
#16190=DIRECTION ( 'NONE',  ( -0.000000000000000000, -0.000000000000000000, -1.000000000000000000 ) ) ;
#16191=VERTEX_POINT ( 'NONE', #78556 ) ;
#16192=B_SPLINE_CURVE_WITH_KNOTS ( 'NONE', 3,
 ( #22048, #77429, #49948, #57594, #50386, #22923, #85081, #71546, #15297, #15740 ),
 .UNSPECIFIED., .F., .F.,
 ( 4, 2, 2, 2, 4 ),
 ( 0.0007817246256747483650, 0.0009771112852218926705, 0.001172497944769037084, 0.001367884604316181498, 0.001563271263863325695 ),
 .UNSPECIFIED. ) ;
#16193=ORIENTED_EDGE ( 'NONE', *, *, #70436, .T. ) ;
#16195=CARTESIAN_POINT ( 'NONE',  ( 1.318531973659507139, -10.51840700105979387, 33.73612834413961536 ) ) ;
#16196=CARTESIAN_POINT ( 'NONE',  ( 2.438218009455871638, -2.619367082507848998, 30.83698974864644171 ) ) ;
#16197=DIRECTION ( 'NONE',  ( 0.000000000000000000, 0.000000000000000000, 1.000000000000000000 ) ) ;
#16198=CARTESIAN_POINT ( 'NONE',  ( 2.307692307692186251, -2.379036618888197285, 30.90682066428292885 ) ) ;
#16199=CARTESIAN_POINT ( 'NONE',  ( 1.318531973659505363, -11.69971097300155272, 32.46337939537587403 ) ) ;
#16200=ORIENTED_EDGE ( 'NONE', *, *, #65887, .T. ) ;
#16201=EDGE_CURVE ( 'NONE', #49352, #23024, #58858, .T. ) ;
#16203=CARTESIAN_POINT ( 'NONE',  ( 15.10007862765892739, -10.70098750199973203, 33.91152734681376302 ) ) ;
#16204=CARTESIAN_POINT ( 'NONE',  ( -18.25000000000000711, -2.249999999999998668, 29.75000000000000355 ) ) ;
#16205=CARTESIAN_POINT ( 'NONE',  ( -6.923076923076922462, -2.249999999999998668, 29.75000000000001776 ) ) ;
#16206=CARTESIAN_POINT ( 'NONE',  ( 15.23076923076923173, -1.129524287112498415, 32.06866353760679544 ) ) ;
#16207=EDGE_CURVE ( 'NONE', #20943, #35516, #74990, .T. ) ;
#16208=EDGE_CURVE ( 'NONE', #88347, #57345, #70482, .T. ) ;
#16210=ORIENTED_EDGE ( 'NONE', *, *, #15567, .F. ) ;
#16211=VERTEX_POINT ( 'NONE', #36695 ) ;
#16212=EDGE_CURVE ( 'NONE', #69974, #46007, #38344, .T. ) ;
#16213=CARTESIAN_POINT ( 'NONE',  ( -15.23076923076922995, -8.564572088678739092, 35.78748833219616898 ) ) ;
#16214=ORIENTED_EDGE ( 'NONE', *, *, #53478, .F. ) ;
#16215=CARTESIAN_POINT ( 'NONE',  ( 17.20744851515672025, -4.299079248970731015, 33.91157788607253565 ) ) ;
#16216=CARTESIAN_POINT ( 'NONE',  ( -1.384615384615383471, -5.180354513474913603, 36.12317359536750416 ) ) ;
#16217=FACE_OUTER_BOUND ( 'NONE', #87561, .T. ) ;
#16218=CARTESIAN_POINT ( 'NONE',  ( -8.703162418228330921, -10.51840700105979565, 33.73612834413962247 ) ) ;
#16221=CARTESIAN_POINT ( 'NONE',  ( -8.096153846153844924, -2.499999999999998668, 29.75000000000000355 ) ) ;
#16222=ORIENTED_EDGE ( 'NONE', *, *, #62521, .F. ) ;
#16223=DIRECTION ( 'NONE',  ( -0.000000000000000000, 0.7660444431189791237, -0.6427876096865379196 ) ) ;
#16224=CARTESIAN_POINT ( 'NONE',  ( -10.61538461538461320, -10.67929555188718282, 33.92786785259544047 ) ) ;
#16225=EDGE_LOOP ( 'NONE', ( #25828, #32559 ) ) ;
#16226=CARTESIAN_POINT ( 'NONE',  ( -12.46153846153846168, -5.471508081941601098, 34.59228464037088457 ) ) ;
#16227=CARTESIAN_POINT ( 'NONE',  ( -9.822999158975251888, -12.11776431015576172, 31.66791131148498906 ) ) ;
#16228=CYLINDRICAL_SURFACE ( 'NONE', #78316, 0.2499999999999997502 ) ;
#16229=CARTESIAN_POINT ( 'NONE',  ( 11.76124120743959978, -8.540255544307065350, 34.89611431652622286 ) ) ;
#16230=CYLINDRICAL_SURFACE ( 'NONE', #7657, 0.2499999999999986955 ) ;
#16231=CARTESIAN_POINT ( 'NONE',  ( 3.230769230769110045, -2.625532179533779154, 30.86335684631627174 ) ) ;
#16233=ORIENTED_EDGE ( 'NONE', *, *, #49145, .T. ) ;
#16234=B_SPLINE_CURVE_WITH_KNOTS ( 'NONE', 3,
 ( #37539, #75987, #2859, #3314, #35445, #82760, #37997, #64556, #30786, #65465 ),
 .UNSPECIFIED., .F., .F.,
 ( 4, 2, 2, 2, 4 ),
 ( 0.0007817246256747484735, 0.0009771112852218920199, 0.001172497944769035566, 0.001367884604316179113, 0.001563271263863322659 ),
 .UNSPECIFIED. ) ;
#16235=CARTESIAN_POINT ( 'NONE',  ( -5.142676505236408069, -7.249945578846651806, 34.99404164642496795 ) ) ;
#16236=CARTESIAN_POINT ( 'NONE',  ( 0.4615384615384611200, -12.78798330534102945, 29.74999999999997868 ) ) ;
#16238=VECTOR ( 'NONE', #37126, 1000.000000000000114 ) ;
#16239=AXIS2_PLACEMENT_3D ( 'NONE', #61239, #14398, #5875 ) ;
#16240=LINE ( 'NONE', #43272, #86381 ) ;
#16241=CARTESIAN_POINT ( 'NONE',  ( 2.530471976670373380, -12.11081565061823717, 32.26097654155341843 ) ) ;
#16242=VERTEX_POINT ( 'NONE', #57399 ) ;
#16243=CYLINDRICAL_SURFACE ( 'NONE', #26898, 0.2499999999999998890 ) ;
#16244=CARTESIAN_POINT ( 'NONE',  ( -15.45425415533356350, -4.225889041578353655, 33.85425143139329407 ) ) ;
#16245=B_SPLINE_CURVE_WITH_KNOTS ( 'NONE', 3,
 ( #61198, #41836, #48129, #68409, #75180, #21097, #14807, #81942, #68852, #82824 ),
 .UNSPECIFIED., .F., .F.,
 ( 4, 2, 2, 2, 4 ),
 ( 0.0007817359430256294638, 0.0009771253907249941549, 0.001172514838424358954, 0.001367904286123723754, 0.001563293733823095492 ),
 .UNSPECIFIED. ) ;
#16247=AXIS2_PLACEMENT_3D ( 'NONE', #20264, #20699, #69337 ) ;
#16248=ORIENTED_EDGE ( 'NONE', *, *, #35443, .F. ) ;
#16249=CARTESIAN_POINT ( 'NONE',  ( 6.792928953345228393, -6.809168938359898782, 34.95455904226513866 ) ) ;
#16251=DIRECTION ( 'NONE',  ( -0.000000000000000000, 0.1736481776669307198, -0.9848077530122080203 ) ) ;
#16252=CARTESIAN_POINT ( 'NONE',  ( 3.007842271862381622, -4.026226216239095379, 33.68668979543632958 ) ) ;
#16253=CARTESIAN_POINT ( 'NONE',  ( -12.46153846153858424, -10.33852847137269571, 34.16647553114546554 ) ) ;
#16254=CARTESIAN_POINT ( 'NONE',  ( -4.153846153846152411, -11.35647404775217417, 33.31231777344666511 ) ) ;
#16255=EDGE_LOOP ( 'NONE', ( #61322, #80747 ) ) ;
#16256=CARTESIAN_POINT ( 'NONE',  ( -2.437840277423998891, -12.15440758774515473, 32.17923288041532004 ) ) ;
#16257=B_SPLINE_CURVE_WITH_KNOTS ( 'NONE', 3,
 ( #84050, #56560, #9697, #57883, #35852, #62849, #1168, #85368, #63753, #29537 ),
 .UNSPECIFIED., .F., .F.,
 ( 4, 2, 2, 2, 4 ),
 ( 0.000000000000000000, 0.0001954339857564073659, 0.0003908679715128147319, 0.0005863019572692221250, 0.0007817359430256294638 ),
 .UNSPECIFIED. ) ;
#16258=ORIENTED_EDGE ( 'NONE', *, *, #81015, .F. ) ;
#16259=CARTESIAN_POINT ( 'NONE',  ( -6.699700982378739234, -2.501478030877322567, 29.88021232661720816 ) ) ;
#16260=CYLINDRICAL_SURFACE ( 'NONE', #5269, 0.2499999999999994726 ) ;
#16262=CARTESIAN_POINT ( 'NONE',  ( 8.769230769230645706, -5.094484230521993062, 34.41647553114689373 ) ) ;
#16263=CARTESIAN_POINT ( 'NONE',  ( -12.59168567097668401, -6.001485441113819874, 34.52039167877662607 ) ) ;
#16264=DIRECTION ( 'NONE',  ( 0.000000000000000000, 0.3420201433256641055, -0.9396926207859100932 ) ) ;
#16265=AXIS2_PLACEMENT_3D ( 'NONE', #5217, #87212, #79097 ) ;
#16266=CARTESIAN_POINT ( 'NONE',  ( 1.318533005255250856, -6.343179335718451384, 34.87096338111212646 ) ) ;
#16267=FACE_OUTER_BOUND ( 'NONE', #44988, .T. ) ;
#16268=EDGE_CURVE ( 'NONE', #88393, #70106, #6232, .T. ) ;
#16269=EDGE_CURVE ( 'NONE', #37364, #7653, #22338, .T. ) ;
#16271=ORIENTED_EDGE ( 'NONE', *, *, #43978, .T. ) ;
#16272=FACE_BOUND ( 'NONE', #73041, .T. ) ;
#16273=EDGE_LOOP ( 'NONE', ( #23432, #74376 ) ) ;
#16274=DIRECTION ( 'NONE',  ( -0.000000000000000000, -0.1736481776669307198, -0.9848077530122080203 ) ) ;
#16275=EDGE_CURVE ( 'NONE', #72596, #27372, #1912, .T. ) ;
#16276=EDGE_CURVE ( 'NONE', #16685, #61262, #54460, .T. ) ;
#16277=DIRECTION ( 'NONE',  ( 0.000000000000000000, 0.4999999999999960032, -0.8660254037844410391 ) ) ;
#16279=ORIENTED_EDGE ( 'NONE', *, *, #41385, .F. ) ;
#16280=ORIENTED_EDGE ( 'NONE', *, *, #82877, .F. ) ;
#16281=EDGE_CURVE ( 'NONE', #66547, #37408, #70667, .T. ) ;
#16282=CARTESIAN_POINT ( 'NONE',  ( 0.2386115026316120158, -8.282780595021769443, 34.94152052738834868 ) ) ;
#16283=ORIENTED_EDGE ( 'NONE', *, *, #61363, .T. ) ;
#16284=CARTESIAN_POINT ( 'NONE',  ( 2.057692307692309708, -7.500000000000001776, 35.00000000000000000 ) ) ;
#16285=DIRECTION ( 'NONE',  ( 0.000000000000000000, 0.6427876096865373645, -0.7660444431189797898 ) ) ;
#16286=EDGE_CURVE ( 'NONE', #70329, #485, #4237, .T. ) ;
#16287=CARTESIAN_POINT ( 'NONE',  ( -12.39634547324380520, -2.255955759149235629, 29.99999999999988987 ) ) ;
#16288=FACE_BOUND ( 'NONE', #22417, .T. ) ;
#16290=VECTOR ( 'NONE', #47094, 1000.000000000000227 ) ;
#16291=CARTESIAN_POINT ( 'NONE',  ( -8.519176349317316266, -4.074993327901527351, 33.72946981652012255 ) ) ;
#16292=VECTOR ( 'NONE', #67358, 999.9999999999998863 ) ;
#16295=CARTESIAN_POINT ( 'NONE',  ( -14.53117725141625627, -9.331801661448606566, 34.40259984581193464 ) ) ;
#16297=VERTEX_POINT ( 'NONE', #4691 ) ;
#16299=B_SPLINE_CURVE_WITH_KNOTS ( 'NONE', 3,
 ( #63170, #20860, #14108, #28970, #14551, #1037, #7798, #15447, #83914, #28514 ),
 .UNSPECIFIED., .F., .F.,
 ( 4, 2, 2, 2, 4 ),
 ( 0.0007817246256747472808, 0.0009771112852218907189, 0.001172497944769034265, 0.001367884604316177595, 0.001563271263863321141 ),
 .UNSPECIFIED. ) ;
#16300=ORIENTED_EDGE ( 'NONE', *, *, #66974, .F. ) ;
#16301=CARTESIAN_POINT ( 'NONE',  ( -7.976845312821407852, -6.413092428213692742, 34.63065189839063152 ) ) ;
#16302=CARTESIAN_POINT ( 'NONE',  ( 10.68145296638705410, -5.557115091759786019, 34.35708131394839882 ) ) ;
#16303=B_SPLINE_CURVE_WITH_KNOTS ( 'NONE', 3,
 ( #45932, #31082, #4051, #46388, #65316, #58551, #73869, #24778, #59458, #52246 ),
 .UNSPECIFIED., .F., .F.,
 ( 4, 2, 2, 2, 4 ),
 ( 0.000000000000000000, 0.0001954311564186863865, 0.0003908623128373727731, 0.0005862934692560591325, 0.0007817246256747455461 ),
 .UNSPECIFIED. ) ;
#16304=CARTESIAN_POINT ( 'NONE',  ( -5.076923076923075762, -5.180354513474913603, 36.12317359536750416 ) ) ;
#16305=CARTESIAN_POINT ( 'NONE',  ( -8.834500769787091201, -6.835583212224499938, 34.95778746994557906 ) ) ;
#16306=FACE_BOUND ( 'NONE', #12655, .T. ) ;
#16307=CARTESIAN_POINT ( 'NONE',  ( -11.78843828251013015, -2.318417181685855422, 30.59732222474233865 ) ) ;
#16308=VERTEX_POINT ( 'NONE', #5130 ) ;
#16309=ADVANCED_FACE ( 'NONE', ( #80358 ), #44309, .F. ) ;
#16310=FACE_OUTER_BOUND ( 'NONE', #42104, .T. ) ;
#16311=CARTESIAN_POINT ( 'NONE',  ( 9.692307692307570832, -11.06231777344772027, 33.60647404775119895 ) ) ;
#16312=CARTESIAN_POINT ( 'NONE',  ( -17.30040802064702632, -11.89387501736623420, 32.13663884655804992 ) ) ;
#16313=DIRECTION ( 'NONE',  ( -0.000000000000000000, -0.6427876096865404731, -0.7660444431189770143 ) ) ;
#16315=DIRECTION ( 'NONE',  ( -0.000000000000000000, 0.1736481776669307198, -0.9848077530122080203 ) ) ;
#16316=EDGE_CURVE ( 'NONE', #19193, #13671, #13723, .T. ) ;
#16317=VERTEX_POINT ( 'NONE', #17762 ) ;
#16318=FACE_BOUND ( 'NONE', #32688, .T. ) ;
#16319=CARTESIAN_POINT ( 'NONE',  ( 4.284636594813102661, -2.494656445102013453, 31.33466734024120015 ) ) ;
#16320=CARTESIAN_POINT ( 'NONE',  ( 12.33139125210024112, -12.27039167877662251, 31.24851455888617835 ) ) ;
#16321=EDGE_LOOP ( 'NONE', ( #56359, #34421 ) ) ;
#16322=CARTESIAN_POINT ( 'NONE',  ( 4.153846153846154188, -11.35647404775217417, 33.31231777344666511 ) ) ;
#16323=CARTESIAN_POINT ( 'NONE',  ( -2.242436736416281384, -4.481592998940250538, 33.73612834413965089 ) ) ;
#16325=LINE ( 'NONE', #37024, #28785 ) ;
#16326=EDGE_LOOP ( 'NONE', ( #11730, #54376 ) ) ;
#16329=VERTEX_POINT ( 'NONE', #6466 ) ;
#16330=CYLINDRICAL_SURFACE ( 'NONE', #69808, 2.000000000000001776 ) ;
#16333=CARTESIAN_POINT ( 'NONE',  ( -8.834554782035079157, -7.749976730030849303, 34.74374725381503737 ) ) ;
#16334=CARTESIAN_POINT ( 'NONE',  ( 15.10007776410167857, -2.729777683071817229, 31.24903638046269450 ) ) ;
#16335=CARTESIAN_POINT ( 'NONE',  ( -15.23076923076935252, -11.06231777344772027, 33.60647404775119895 ) ) ;
#16336=FACE_OUTER_BOUND ( 'NONE', #37901, .T. ) ;
#16338=EDGE_CURVE ( 'NONE', #12423, #28595, #74475, .T. ) ;
#16339=DIRECTION ( 'NONE',  ( -0.000000000000000000, 0.1736481776669307198, -0.9848077530122080203 ) ) ;
#16341=VERTEX_POINT ( 'NONE', #54630 ) ;
#16342=CARTESIAN_POINT ( 'NONE',  ( -14.98082371242109012, -3.712312575010499049, 33.01462480002815170 ) ) ;
#16343=CARTESIAN_POINT ( 'NONE',  ( 5.076923076923075762, -9.584722331328613620, 36.20867863119891439 ) ) ;
#16344=EDGE_LOOP ( 'NONE', ( #693, #59782 ) ) ;
#16345=EDGE_LOOP ( 'NONE', ( #49884, #75544, #54084, #55053 ) ) ;
#16346=EDGE_LOOP ( 'NONE', ( #88747, #13043, #68580, #14632 ) ) ;
#16347=CARTESIAN_POINT ( 'NONE',  ( -10.68065506134539078, -11.48612834413959582, 32.76840700105983473 ) ) ;
#16348=CARTESIAN_POINT ( 'NONE',  ( 6.000000000000001776, -12.29105614889573062, 35.45975837776705220 ) ) ;
#16349=EDGE_CURVE ( 'NONE', #65895, #19974, #53754, .T. ) ;
#16350=CARTESIAN_POINT ( 'NONE',  ( 6.222779541268408821, -11.41317474335729187, 32.86274602512330034 ) ) ;
#16352=CARTESIAN_POINT ( 'NONE',  ( 5.999999999999880096, -2.625532179533778709, 30.86335684631627174 ) ) ;
#16354=CARTESIAN_POINT ( 'NONE',  ( 16.37685899793955357, -3.395485233115139501, 33.02377354290276656 ) ) ;
#16355=CARTESIAN_POINT ( 'NONE',  ( 13.63461538461538680, -2.249999999999998668, 29.75000000000000355 ) ) ;
#16356=ORIENTED_EDGE ( 'NONE', *, *, #65444, .T. ) ;
#16357=CARTESIAN_POINT ( 'NONE',  ( -3.903791842207838148, -5.728107161865378494, 34.42597550085002922 ) ) ;
#16358=CARTESIAN_POINT ( 'NONE',  ( -1.634638621908349077, -6.695914987888143877, 34.68535235679833306 ) ) ;
#16359=CARTESIAN_POINT ( 'NONE',  ( -9.469528151039282804, -11.41317474335729543, 32.86274602512330034 ) ) ;
#16360=CARTESIAN_POINT ( 'NONE',  ( 12.23805351781451201, -11.89387501736622710, 32.13663884655806413 ) ) ;
#16361=ORIENTED_EDGE ( 'NONE', *, *, #38894, .F. ) ;
#16363=VECTOR ( 'NONE', #39747, 1000.000000000000114 ) ;
#16364=AXIS2_PLACEMENT_3D ( 'NONE', #28114, #62770, #26346 ) ;
#16366=CARTESIAN_POINT ( 'NONE',  ( -17.32694630114453460, -2.588893531581426544, 31.60682220781847818 ) ) ;
#16368=CARTESIAN_POINT ( 'NONE',  ( 9.692307692307695177, -2.499999999999998668, 29.50000000000001066 ) ) ;
#16370=B_SPLINE_CURVE_WITH_KNOTS ( 'NONE', 3,
 ( #80853, #61000, #59223, #83053, #56012, #34850, #47925, #42072, #20463, #35300 ),
 .UNSPECIFIED., .F., .F.,
 ( 4, 2, 2, 2, 4 ),
 ( 0.000000000000000000, 0.0001954339857564100493, 0.0003908679715128200987, 0.0005863019572692301480, 0.0007817359430256401974 ),
 .UNSPECIFIED. ) ;
#16372=FACE_OUTER_BOUND ( 'NONE', #86552, .T. ) ;
#16373=CARTESIAN_POINT ( 'NONE',  ( 9.468822767743361624, -3.019605429927184392, 32.48692288466676814 ) ) ;
#16374=CARTESIAN_POINT ( 'NONE',  ( -9.019253993452224449, -9.356822207818506598, 34.66110646841856635 ) ) ;
#16375=ORIENTED_EDGE ( 'NONE', *, *, #41533, .F. ) ;
#16376=CARTESIAN_POINT ( 'NONE',  ( -0.4615384615385826339, -8.613356846316285953, 34.62446782046622218 ) ) ;
#16377=ORIENTED_EDGE ( 'NONE', *, *, #88796, .F. ) ;
#16378=CARTESIAN_POINT ( 'NONE',  ( -8.769230769230768274, -1.466349020453238561, 30.81389545987213907 ) ) ;
#16379=CARTESIAN_POINT ( 'NONE',  ( -16.15384615384615330, -8.810774026931790459, 35.74407628777942847 ) ) ;
#16380=CARTESIAN_POINT ( 'NONE',  ( 12.33084699487090319, -8.147922237126337563, 34.70805685702651999 ) ) ;
#16381=EDGE_CURVE ( 'NONE', #52756, #16542, #34367, .T. ) ;
#16382=CARTESIAN_POINT ( 'NONE',  ( 15.23076923076911093, -10.90142922262034020, 33.41473453929536674 ) ) ;
#16383=CYLINDRICAL_SURFACE ( 'NONE', #3542, 0.2500000000000008882 ) ;
#16384=ORIENTED_EDGE ( 'NONE', *, *, #71516, .T. ) ;
#16385=AXIS2_PLACEMENT_3D ( 'NONE', #54175, #68586, #13207 ) ;
#16386=EDGE_CURVE ( 'NONE', #20537, #10414, #39811, .T. ) ;
#16387=ORIENTED_EDGE ( 'NONE', *, *, #3589, .F. ) ;
#16388=ORIENTED_EDGE ( 'NONE', *, *, #84313, .F. ) ;
#16392=B_SPLINE_CURVE_WITH_KNOTS ( 'NONE', 3,
 ( #37986, #45175, #86189, #108, #14502, #60916, #41988, #6430, #34771, #69451 ),
 .UNSPECIFIED., .F., .F.,
 ( 4, 2, 2, 2, 4 ),
 ( 0.0007817359430256365111, 0.0009771253907250043464, 0.001172514838424372399, 0.001367904286123740234, 0.001563293733823108069 ),
 .UNSPECIFIED. ) ;
#16393=CARTESIAN_POINT ( 'NONE',  ( 17.07692307692307665, -4.098570777380720287, 33.41473453929634729 ) ) ;
#16394=CARTESIAN_POINT ( 'NONE',  ( -16.15384615384627409, -2.625532179533778709, 30.86335684631627174 ) ) ;
#16395=CARTESIAN_POINT ( 'NONE',  ( 11.28848480751918437, -12.17611988154120972, 31.52148481390971213 ) ) ;
#16396=FACE_OUTER_BOUND ( 'NONE', #893, .T. ) ;
#16397=LINE ( 'NONE', #34891, #42336 ) ;
#16398=EDGE_LOOP ( 'NONE', ( #43805, #41552 ) ) ;
#16400=EDGE_LOOP ( 'NONE', ( #23675, #75701, #69456, #78793, #71797, #53091 ) ) ;
#16401=EDGE_CURVE ( 'NONE', #6730, #36558, #47051, .T. ) ;
#16402=CARTESIAN_POINT ( 'NONE',  ( 11.78851595837499566, -2.544122305571458575, 31.48381861865057729 ) ) ;
#16403=VERTEX_POINT ( 'NONE', #60514 ) ;
#16404=LINE ( 'NONE', #29053, #27361 ) ;
#16405=CARTESIAN_POINT ( 'NONE',  ( -8.638705067467208565, -11.46989282347013095, 32.79007818306219946 ) ) ;
#16406=CARTESIAN_POINT ( 'NONE',  ( 8.900069187243529356, -7.277220443632450575, 34.74524770363009196 ) ) ;
#16408=ORIENTED_EDGE ( 'NONE', *, *, #65534, .T. ) ;
#16409=VECTOR ( 'NONE', #80786, 1000.000000000000114 ) ;
#16410=EDGE_LOOP ( 'NONE', ( #18360, #58582, #56743, #19452 ) ) ;
#16412=CARTESIAN_POINT ( 'NONE',  ( -11.60454391782167605, -11.91647553114624181, 32.58852847137148245 ) ) ;
#16413=EDGE_CURVE ( 'NONE', #25620, #67642, #63161, .T. ) ;
#16414=B_SPLINE_CURVE_WITH_KNOTS ( 'NONE', 3,
 ( #14454, #82484, #20763, #8145, #56325, #41482, #6381, #40607, #74837, #41932 ),
 .UNSPECIFIED., .F., .F.,
 ( 4, 2, 2, 2, 4 ),
 ( 0.0007817246336856291692, 0.0009771112958940105907, 0.001172497958102391904, 0.001367884620310773434, 0.001563271282519154747 ),
 .UNSPECIFIED. ) ;
#16415=EDGE_LOOP ( 'NONE', ( #48474, #84559, #55470, #30025 ) ) ;
#16416=FACE_BOUND ( 'NONE', #73107, .T. ) ;
#16417=CARTESIAN_POINT ( 'NONE',  ( -6.222926217516146608, -9.086856451489516928, 34.49173150075333183 ) ) ;
#16419=CARTESIAN_POINT ( 'NONE',  ( 9.692307692307695177, -4.786620604624113540, 33.94971097300155094 ) ) ;
#16420=ORIENTED_EDGE ( 'NONE', *, *, #74834, .F. ) ;
#16421=CARTESIAN_POINT ( 'NONE',  ( -15.00798968950081758, -5.114059244376869984, 34.14424750095245287 ) ) ;
#16422=EDGE_CURVE ( 'NONE', #10508, #63945, #7355, .T. ) ;
#16423=CARTESIAN_POINT ( 'NONE',  ( 16.40379167219429490, -4.336752205174650321, 33.62275283266504289 ) ) ;
#16426=CARTESIAN_POINT ( 'NONE',  ( 1.384615384615386802, -2.486705287966279876, 31.30864560766543647 ) ) ;
#16428=CARTESIAN_POINT ( 'NONE',  ( 10.61538461538449596, -8.613356846316285953, 34.62446782046622218 ) ) ;
#16429=FACE_OUTER_BOUND ( 'NONE', #77318, .T. ) ;
#16430=CARTESIAN_POINT ( 'NONE',  ( 2.084207383127980595, -12.11044203135681840, 32.26167407432752299 ) ) ;
#16431=CARTESIAN_POINT ( 'NONE',  ( 0.2386122440223129304, -11.76352882383564769, 32.36236540154569497 ) ) ;
#16433=CARTESIAN_POINT ( 'NONE',  ( -18.00000000000000000, -8.563426751879235965, 35.78099280442780383 ) ) ;
#16434=CARTESIAN_POINT ( 'NONE',  ( -13.13456096470193302, -12.41089969410671223, 31.60739465890703670 ) ) ;
#16436=CARTESIAN_POINT ( 'NONE',  ( 2.438484115517095763, -9.804649428959608670, 34.18742332936588468 ) ) ;
#16439=CYLINDRICAL_SURFACE ( 'NONE', #27120, 0.2500000000000008882 ) ;
#16440=LINE ( 'NONE', #23634, #36356 ) ;
#16441=CARTESIAN_POINT ( 'NONE',  ( 13.31929246912321396, -7.749976743299138882, 34.99404534957040624 ) ) ;
#16442=B_SPLINE_CURVE_WITH_KNOTS ( 'NONE', 3,
 ( #2218, #76114, #16188, #14416, #28831, #76567 ),
 .UNSPECIFIED., .F., .F.,
 ( 4, 2, 4 ),
 ( 3.508529156471553821E-17, 0.0001954756301637064486, 0.0003909512603273778233 ),
 .UNSPECIFIED. ) ;
#16444=ORIENTED_EDGE ( 'NONE', *, *, #41996, .F. ) ;
#16446=ORIENTED_EDGE ( 'NONE', *, *, #27668, .F. ) ;
#16447=CARTESIAN_POINT ( 'NONE',  ( -2.307692307692305711, -2.833524468853757305, 32.15551576947925838 ) ) ;
#16448=EDGE_LOOP ( 'NONE', ( #35587, #24721 ) ) ;
#16449=CARTESIAN_POINT ( 'NONE',  ( -15.23076923076922995, -3.513871655860378418, 32.76840700105978499 ) ) ;
#16451=CARTESIAN_POINT ( 'NONE',  ( -6.249976730942353953, -11.79746400365624659, 32.30657167506340954 ) ) ;
#16453=CARTESIAN_POINT ( 'NONE',  ( 7.596177102105253987, -8.347322224742351082, 34.93158281831414769 ) ) ;
#16454=ADVANCED_FACE ( 'NONE', ( #74929 ), #60954, .F. ) ;
#16455=CARTESIAN_POINT ( 'NONE',  ( 6.700150705560775855, -11.24512374952581872, 33.06303171183252942 ) ) ;
#16456=CARTESIAN_POINT ( 'NONE',  ( -2.980823821391187511, -12.45601412856602686, 31.48342859153981621 ) ) ;
#16457=CARTESIAN_POINT ( 'NONE',  ( 15.93036122928182330, -8.539481045369598178, 34.89627647299170832 ) ) ;
#16458=AXIS2_PLACEMENT_3D ( 'NONE', #31615, #87469, #51401 ) ;
#16459=CARTESIAN_POINT ( 'NONE',  ( -17.87219494718144119, -2.249999999999999556, 29.52383875849255546 ) ) ;
#16460=CARTESIAN_POINT ( 'NONE',  ( 1.384615384615264011, -5.094484230521993062, 34.41647553114689373 ) ) ;
#16461=CARTESIAN_POINT ( 'NONE',  ( -14.08491263871423982, -4.989023458446560255, 34.36081565061822118 ) ) ;
#16463=EDGE_CURVE ( 'NONE', #87599, #19612, #791, .T. ) ;
#16464=EDGE_CURVE ( 'NONE', #56650, #33104, #51230, .T. ) ;
#16466=CARTESIAN_POINT ( 'NONE',  ( 17.07692307692307665, -2.486705287966279876, 31.30864560766543647 ) ) ;
#16469=ADVANCED_FACE ( 'NONE', ( #21745 ), #36163, .F. ) ;
#16470=ORIENTED_EDGE ( 'NONE', *, *, #4354, .T. ) ;
#16471=CARTESIAN_POINT ( 'NONE',  ( 17.14217864819909920, -12.27809138561124591, 31.22303859784720359 ) ) ;
#16472=CARTESIAN_POINT ( 'NONE',  ( 11.78840705680968171, -5.852078868378309373, 34.47109172314383585 ) ) ;
#16473=CARTESIAN_POINT ( 'NONE',  ( 6.923076923076924238, -2.708943851104267164, 35.45975837776705220 ) ) ;
#16474=CARTESIAN_POINT ( 'NONE',  ( 15.45419562968402261, -7.630147987733840509, 34.99859428049665411 ) ) ;
#16475=CARTESIAN_POINT ( 'NONE',  ( 3.930361229281823743, -3.562934362175799841, 33.22335522853832401 ) ) ;
#16476=B_SPLINE_CURVE_WITH_KNOTS ( 'NONE', 3,
 ( #40582, #12216, #54518, #80232, #81568, #47318, #53185, #66260, #68051, #33811 ),
 .UNSPECIFIED., .F., .F.,
 ( 4, 2, 2, 2, 4 ),
 ( 0.000000000000000000, 0.0001954311584214072652, 0.0003908623168428145304, 0.0005862934752642217414, 0.0007817246336856290608 ),
 .UNSPECIFIED. ) ;
#16478=B_SPLINE_CURVE_WITH_KNOTS ( 'NONE', 3,
 ( #29708, #21608, #1338, #49080, #82447, #48192, #75665, #27930, #14870, #8106 ),
 .UNSPECIFIED., .F., .F.,
 ( 4, 2, 2, 2, 4 ),
 ( 0.0007817359430256341259, 0.0009771253907250067317, 0.001172514838424372399, 0.001367904286123738065, 0.001563293733823103732 ),
 .UNSPECIFIED. ) ;
#16482=EDGE_LOOP ( 'NONE', ( #58013, #40567 ) ) ;
#16483=AXIS2_PLACEMENT_3D ( 'NONE', #58452, #17489, #73321 ) ;
#16485=CARTESIAN_POINT ( 'NONE',  ( -0.2385256174450663957, -5.582272713120728369, 34.63742843783360570 ) ) ;
#16486=VECTOR ( 'NONE', #81157, 1000.000000000000114 ) ;
#16489=CARTESIAN_POINT ( 'NONE',  ( -6.250023237292964495, -3.202444869320336451, 32.30641848906366675 ) ) ;
#16490=CARTESIAN_POINT ( 'NONE',  ( -3.903846153844733102, -7.500000000000154543, 35.00000000000007105 ) ) ;
#16491=ORIENTED_EDGE ( 'NONE', *, *, #69732, .T. ) ;
#16492=FACE_OUTER_BOUND ( 'NONE', #72236, .T. ) ;
#16493=ORIENTED_EDGE ( 'NONE', *, *, #58312, .F. ) ;
#16494=ORIENTED_EDGE ( 'NONE', *, *, #12411, .F. ) ;
#16495=CARTESIAN_POINT ( 'NONE',  ( 1.384615384615386802, -11.16473453929635440, 33.15142922261926373 ) ) ;
#16496=CARTESIAN_POINT ( 'NONE',  ( 0.4615384615384611200, -1.117168528481311540, 33.14645433367849847 ) ) ;
#16497=CARTESIAN_POINT ( 'NONE',  ( -10.86536134632696715, -4.943428324936578910, 34.04746400365624481 ) ) ;
#16498=B_SPLINE_CURVE_WITH_KNOTS ( 'NONE', 3,
 ( #87011, #25283, #80234, #66715, #54520, #11775, #74363, #54071, #46879, #87910 ),
 .UNSPECIFIED., .F., .F.,
 ( 4, 2, 2, 2, 4 ),
 ( 0.000000000000000000, 0.0001954339857564080165, 0.0003908679715128160329, 0.0005863019572692240765, 0.0007817359430256320659 ),
 .UNSPECIFIED. ) ;
#16499=CARTESIAN_POINT ( 'NONE',  ( -17.07692307692319744, -3.300289026999228437, 32.46337939537709616 ) ) ;
#16501=EDGE_LOOP ( 'NONE', ( #66558, #67766, #80578, #83136 ) ) ;
#16502=EDGE_LOOP ( 'NONE', ( #86771, #49639, #9484, #5022 ) ) ;
#16504=VECTOR ( 'NONE', #50118, 999.9999999999998863 ) ;
#16505=ORIENTED_EDGE ( 'NONE', *, *, #22369, .T. ) ;
#16506=CARTESIAN_POINT ( 'NONE',  ( -14.24243716817946925, -2.379036618887895305, 30.90682066428158592 ) ) ;
#16507=ORIENTED_EDGE ( 'NONE', *, *, #31530, .T. ) ;
#16508=FACE_OUTER_BOUND ( 'NONE', #14895, .T. ) ;
#16510=LINE ( 'NONE', #28705, #42247 ) ;
#16511=VERTEX_POINT ( 'NONE', #9132 ) ;
#16512=CARTESIAN_POINT ( 'NONE',  ( 15.23076923076923173, -2.486705287966279876, 31.30864560766543647 ) ) ;
#16513=EDGE_LOOP ( 'NONE', ( #46297, #55250 ) ) ;
#16514=CARTESIAN_POINT ( 'NONE',  ( 15.36155967173617931, -11.37503395064541678, 33.29242100308974273 ) ) ;
#16515=CARTESIAN_POINT ( 'NONE',  ( 10.74617642320940725, -8.999086150933475636, 34.52020707165672775 ) ) ;
#16516=EDGE_CURVE ( 'NONE', #81813, #33011, #18983, .T. ) ;
#16517=CARTESIAN_POINT ( 'NONE',  ( -17.77698715590659972, -2.523321265292116866, 31.42251411153756990 ) ) ;
#16518=CARTESIAN_POINT ( 'NONE',  ( 10.36538461538461675, -7.500000000000001776, 34.75000000000000000 ) ) ;
#16519=CARTESIAN_POINT ( 'NONE',  ( -10.83886953994894498, -5.827078755546623690, 34.72654668319379567 ) ) ;
#16520=CARTESIAN_POINT ( 'NONE',  ( 4.853996859406926490, -2.554751324335733820, 30.48935550225260727 ) ) ;
#16521=CARTESIAN_POINT ( 'NONE',  ( -0.2114840416250090838, -12.65882529074907126, 30.72640787790839312 ) ) ;
#16522=ORIENTED_EDGE ( 'NONE', *, *, #11989, .T. ) ;
#16523=CARTESIAN_POINT ( 'NONE',  ( -11.47239318745910275, -4.098570777380720287, 33.41473453929635440 ) ) ;
#16524=CARTESIAN_POINT ( 'NONE',  ( -6.222926958906846551, -11.43668979543635089, 33.22377378376089752 ) ) ;
#16526=CARTESIAN_POINT ( 'NONE',  ( -16.40386937806761836, -12.68155406624981119, 30.59749803192733708 ) ) ;
#16527=CARTESIAN_POINT ( 'NONE',  ( -4.853911725310227077, -5.667800583137508674, 34.40243808032445827 ) ) ;
#16529=CARTESIAN_POINT ( 'NONE',  ( -5.207070286361298095, -11.93770438780619259, 32.05411857736982029 ) ) ;
#16530=CARTESIAN_POINT ( 'NONE',  ( -10.61538461538461320, -2.833524468853757305, 32.15551576947925838 ) ) ;
#16531=CARTESIAN_POINT ( 'NONE',  ( 2.307692307692187583, -8.613356846316285953, 34.62446782046622218 ) ) ;
#16532=CIRCLE ( 'NONE', #730, 0.2500000000000002220 ) ;
#16533=FACE_BOUND ( 'NONE', #14596, .T. ) ;
#16534=CARTESIAN_POINT ( 'NONE',  ( 12.33139049180676672, -10.31621877034669588, 34.18098118002070152 ) ) ;
#16535=CARTESIAN_POINT ( 'NONE',  ( -10.74585980046033562, -7.276987145209185215, 34.99546412871779211 ) ) ;
#16536=ADVANCED_FACE ( 'NONE', ( #64479 ), #22193, .F. ) ;
#16537=CARTESIAN_POINT ( 'NONE',  ( -12.21153846153846168, -2.249999999999998668, 29.75000000000000355 ) ) ;
#16538=CARTESIAN_POINT ( 'NONE',  ( -4.946132635956127288, -9.929761469519744921, 34.40412654351204225 ) ) ;
#16539=CARTESIAN_POINT ( 'NONE',  ( 9.692307692307572609, -4.481592998941358097, 33.73612834414048933 ) ) ;
#16542=VERTEX_POINT ( 'NONE', #29405 ) ;
#16543=AXIS2_PLACEMENT_3D ( 'NONE', #68040, #45975, #45534 ) ;
#16544=LINE ( 'NONE', #44010, #67972 ) ;
#16545=CARTESIAN_POINT ( 'NONE',  ( -4.826868765284762830, -3.136992222400443175, 32.19305428654138979 ) ) ;
#16546=CARTESIAN_POINT ( 'NONE',  ( -0.5922290646487706756, -3.338472653186242756, 32.95098750199972670 ) ) ;
#16547=CARTESIAN_POINT ( 'NONE',  ( 14.30769230769231015, -11.33034616979429110, 35.88435417666054406 ) ) ;
#16548=CARTESIAN_POINT ( 'NONE',  ( 6.792386319966616348, -12.62707690430377383, 30.88035979386743435 ) ) ;
#16549=CARTESIAN_POINT ( 'NONE',  ( -9.561515884482904681, -4.118422570099831148, 33.43335022499816489 ) ) ;
#16551=CARTESIAN_POINT ( 'NONE',  ( -16.37677311275299985, -5.582147617184174848, 34.63737895849758530 ) ) ;
#16552=CARTESIAN_POINT ( 'NONE',  ( -39.05038313613820122, -2.499999999999999556, 29.75000000000000355 ) ) ;
#16553=CARTESIAN_POINT ( 'NONE',  ( -17.07692307692307665, -5.557115091759785130, 34.35708131394839171 ) ) ;
#16554=DIRECTION ( 'NONE',  ( -0.000000000000000000, 0.3420201433256694901, -0.9396926207859082059 ) ) ;
#16555=CARTESIAN_POINT ( 'NONE',  ( -16.94639763868943660, -5.070358843744209310, 34.40418822224088302 ) ) ;
#16556=CARTESIAN_POINT ( 'NONE',  ( 4.153846153846154188, -4.945431358278436385, 36.03766855953609394 ) ) ;
#16557=EDGE_CURVE ( 'NONE', #32412, #19193, #83011, .T. ) ;
#16558=EDGE_CURVE ( 'NONE', #74563, #47506, #55498, .T. ) ;
#16559=DIRECTION ( 'NONE',  ( 0.000000000000000000, 0.7660444431189807890, 0.6427876096865361433 ) ) ;
#16560=CARTESIAN_POINT ( 'NONE',  ( 17.32686848630112308, -2.589246495874658827, 31.60778113518102828 ) ) ;
#16561=VERTEX_POINT ( 'NONE', #84350 ) ;
#16562=CARTESIAN_POINT ( 'NONE',  ( 15.10007862765892739, -11.37499894934982692, 33.29245874905763003 ) ) ;
#16563=CARTESIAN_POINT ( 'NONE',  ( -17.20707028636129365, -2.882441371585227508, 31.66841991370172238 ) ) ;
#16565=B_SPLINE_CURVE_WITH_KNOTS ( 'NONE', 3,
 ( #33741, #5388, #47246, #88708, #81054, #20663, #68851, #54004, #40512, #34625 ),
 .UNSPECIFIED., .F., .F.,
 ( 4, 2, 2, 2, 4 ),
 ( 0.0007817246256747463051, 0.0009771112852218896347, 0.001172497944769032747, 0.001367884604316176077, 0.001563271263863319407 ),
 .UNSPECIFIED. ) ;
#16566=ADVANCED_FACE ( 'NONE', ( #49659 ), #77135, .F. ) ;
#16567=CARTESIAN_POINT ( 'NONE',  ( 7.053602361310566948, -11.04252011169590020, 33.62494198852677130 ) ) ;
#16568=CARTESIAN_POINT ( 'NONE',  ( 3.296024802045256941, -11.94971097300157403, 32.03036669348361443 ) ) ;
#16569=ORIENTED_EDGE ( 'NONE', *, *, #67934, .F. ) ;
#16570=CARTESIAN_POINT ( 'NONE',  ( -16.15384615384615330, -3.937682226553329556, 33.60647404775216529 ) ) ;
#16571=CARTESIAN_POINT ( 'NONE',  ( 17.07692307692307665, -11.35647404775217417, 33.31231777344666511 ) ) ;
#16572=ORIENTED_EDGE ( 'NONE', *, *, #54053, .F. ) ;
#16573=CARTESIAN_POINT ( 'NONE',  ( 6.673053685783957967, -3.202444869320336451, 32.30641848906366675 ) ) ;
#16574=DIRECTION ( 'NONE',  ( -0.000000000000000000, -0.8660254037844397068, -0.4999999999999978906 ) ) ;
#16577=ORIENTED_EDGE ( 'NONE', *, *, #36764, .T. ) ;
#16579=CARTESIAN_POINT ( 'NONE',  ( -14.30769230769230660, -12.34228464037088635, 31.77849191805839268 ) ) ;
#16581=EDGE_LOOP ( 'NONE', ( #3677, #30869 ) ) ;
#16582=VERTEX_POINT ( 'NONE', #15887 ) ;
#16583=ORIENTED_EDGE ( 'NONE', *, *, #36300, .T. ) ;
#16584=DIRECTION ( 'NONE',  ( 0.000000000000000000, 0.4999999999999960032, -0.8660254037844410391 ) ) ;
#16585=CARTESIAN_POINT ( 'NONE',  ( 5.999999999999878320, -2.379036618888197729, 30.90682066428292885 ) ) ;
#16586=CARTESIAN_POINT ( 'NONE',  ( -8.096153846153848477, -7.433931650972301242, 34.75000000000000711 ) ) ;
#16587=CARTESIAN_POINT ( 'NONE',  ( 15.10062202133101295, -3.817052484675422797, 33.13202310037935661 ) ) ;
#16588=B_SPLINE_CURVE_WITH_KNOTS ( 'NONE', 3,
 ( #28591, #15517, #82660, #42112, #70007, #22704, #15963, #56053, #20931, #84429 ),
 .UNSPECIFIED., .F., .F.,
 ( 4, 2, 2, 2, 4 ),
 ( 0.0007817359430256328248, 0.0009771253907249995759, 0.001172514838424366327, 0.001367904286123732861, 0.001563293733823099612 ),
 .UNSPECIFIED. ) ;
#16589=AXIS2_PLACEMENT_3D ( 'NONE', #6755, #55389, #68898 ) ;
#16590=ORIENTED_EDGE ( 'NONE', *, *, #80160, .T. ) ;
#16591=B_SPLINE_CURVE_WITH_KNOTS ( 'NONE', 3,
 ( #27770, #55240, #75514, #41298, #61997, #48929, #82730, #76853, #8392, #55678 ),
 .UNSPECIFIED., .F., .F.,
 ( 4, 2, 2, 2, 4 ),
 ( 0.000000000000000000, 0.0001954339857564070678, 0.0003908679715128141356, 0.0005863019572692211492, 0.0007817359430256282712 ),
 .UNSPECIFIED. ) ;
#16592=ORIENTED_EDGE ( 'NONE', *, *, #9799, .F. ) ;
#16593=CARTESIAN_POINT ( 'NONE',  ( 9.442330961365339448, -4.236021600441997492, 33.53823185664189310 ) ) ;
#16595=B_SPLINE_CURVE_WITH_KNOTS ( 'NONE', 3,
 ( #40721, #74494, #28527, #7373, #68182, #83480, #69065, #27192, #12791, #34830 ),
 .UNSPECIFIED., .F., .F.,
 ( 4, 2, 2, 2, 4 ),
 ( 0.000000000000000000, 0.0001954311564186878502, 0.0003908623128373757004, 0.0005862934692560635777, 0.0007817246256747514008 ),
 .UNSPECIFIED. ) ;
#16596=CARTESIAN_POINT ( 'NONE',  ( 9.823099500132483897, -12.38066358083363738, 30.83685684665853444 ) ) ;
#16597=CARTESIAN_POINT ( 'NONE',  ( 15.48076923076924949, -2.249999999999997780, 29.81603969181029257 ) ) ;
#16598=CARTESIAN_POINT ( 'NONE',  ( -7.912236225513983534, -9.905515769479276145, 34.41647553114623292 ) ) ;
#16599=VECTOR ( 'NONE', #76896, 1000.000000000000227 ) ;
#16600=ORIENTED_EDGE ( 'NONE', *, *, #30986, .T. ) ;
#16602=ORIENTED_EDGE ( 'NONE', *, *, #53839, .T. ) ;
#16603=CARTESIAN_POINT ( 'NONE',  ( -10.61538461538461320, -11.16473453929635440, 33.15142922261926373 ) ) ;
#16604=ORIENTED_EDGE ( 'NONE', *, *, #60883, .F. ) ;
#16605=ADVANCED_FACE ( 'NONE', ( #8688 ), #70830, .F. ) ;
#16606=CARTESIAN_POINT ( 'NONE',  ( 12.46153846153846168, -1.466349020453238561, 30.81389545987213907 ) ) ;
#16607=CARTESIAN_POINT ( 'NONE',  ( -16.15384615384627409, -3.835265460704628815, 33.15142922262033665 ) ) ;
#16609=CARTESIAN_POINT ( 'NONE',  ( 12.71148387091650278, -6.653508905675592722, 34.93172785388651391 ) ) ;
#16610=CARTESIAN_POINT ( 'NONE',  ( 15.23076923076923173, -8.973038597847269315, 34.52809138561121927 ) ) ;
#16611=CARTESIAN_POINT ( 'NONE',  ( 10.83839596699746544, -3.587049720035815348, 32.86302985866382897 ) ) ;
#16612=FACE_BOUND ( 'NONE', #66658, .T. ) ;
#16613=CARTESIAN_POINT ( 'NONE',  ( 8.096099255531889582, -12.45601412856602863, 31.48342859153981621 ) ) ;
#16614=CARTESIAN_POINT ( 'NONE',  ( -6.673131513698878692, -9.357781135181031829, 34.66075350412533851 ) ) ;
#16616=CARTESIAN_POINT ( 'NONE',  ( -14.98071491913091791, -10.66356715214248396, 33.62249196103329751 ) ) ;
#16617=CARTESIAN_POINT ( 'NONE',  ( 17.20696823975784895, -2.504778602574659896, 29.97347330155780654 ) ) ;
#16619=CARTESIAN_POINT ( 'NONE',  ( 11.47319109250076430, -11.48612834413959582, 32.76840700105983473 ) ) ;
#16620=CARTESIAN_POINT ( 'NONE',  ( -16.28399336328437386, -8.587444163452046197, 34.63053765926554206 ) ) ;
#16621=ORIENTED_EDGE ( 'NONE', *, *, #13539, .F. ) ;
#16622=CARTESIAN_POINT ( 'NONE',  ( 9.942307692307695177, -2.249999999999998668, 29.75000000000000355 ) ) ;
#16623=EDGE_CURVE ( 'NONE', #69664, #79083, #33971, .T. ) ;
#16625=ORIENTED_EDGE ( 'NONE', *, *, #24338, .F. ) ;
#16626=B_SPLINE_CURVE_WITH_KNOTS ( 'NONE', 3,
 ( #29702, #43643, #64346, #14408, #28820, #69361, #7661, #69793, #56279, #83768 ),
 .UNSPECIFIED., .F., .F.,
 ( 4, 2, 2, 2, 4 ),
 ( 0.000000000000000000, 0.0001954339857564055499, 0.0003908679715128110998, 0.0005863019572692165955, 0.0007817359430256221996 ),
 .UNSPECIFIED. ) ;
#16627=AXIS2_PLACEMENT_3D ( 'NONE', #7394, #61431, #74080 ) ;
#16628=DIRECTION ( 'NONE',  ( -0.000000000000000000, -0.5000000000000009992, -0.8660254037844380415 ) ) ;
#16629=CARTESIAN_POINT ( 'NONE',  ( 1.634669804528840142, -5.642605341092957083, 34.66089969410670335 ) ) ;
#16630=B_SPLINE_CURVE_WITH_KNOTS ( 'NONE', 3,
 ( #46627, #54705, #75870, #62343, #82195, #80877, #53824, #5640, #47948, #12839 ),
 .UNSPECIFIED., .F., .F.,
 ( 4, 2, 2, 2, 4 ),
 ( 0.000000000000000000, 0.0001954311564186861697, 0.0003908623128373723394, 0.0005862934692560584820, 0.0007817246256747446788 ),
 .UNSPECIFIED. ) ;
#16631=CARTESIAN_POINT ( 'NONE',  ( 13.38461538461526423, -11.67786785259630911, 32.92929555188603530 ) ) ;
#16632=CARTESIAN_POINT ( 'NONE',  ( 14.43848274865926129, -3.957578996910242619, 33.62503395064540257 ) ) ;
#16633=CARTESIAN_POINT ( 'NONE',  ( 1.161689167099239084, -6.503392248772476236, 34.64988816332204635 ) ) ;
#16634=CARTESIAN_POINT ( 'NONE',  ( -10.61538461538461320, -8.120952969808772792, 34.71129190930000163 ) ) ;
#16635=ORIENTED_EDGE ( 'NONE', *, *, #37876, .F. ) ;
#16636=CARTESIAN_POINT ( 'NONE',  ( 18.06606733335007320, -3.937682226553329556, 33.60647404775216529 ) ) ;
#16637=CARTESIAN_POINT ( 'NONE',  ( -0.4615384615385840772, -10.33852847137269571, 34.16647553114546554 ) ) ;
#16638=CARTESIAN_POINT ( 'NONE',  ( 17.32686859527121470, -6.696923467548659303, 34.68552623307873972 ) ) ;
#16639=ADVANCED_FACE ( 'NONE', ( #51395 ), #78901, .F. ) ;
#16640=CARTESIAN_POINT ( 'NONE',  ( 0.4615384615384611200, -10.89733346790207413, 36.13435417666054406 ) ) ;
#16643=EDGE_LOOP ( 'NONE', ( #58592, #44065, #15533, #50218 ) ) ;
#16646=ORIENTED_EDGE ( 'NONE', *, *, #30477, .F. ) ;
#16648=CARTESIAN_POINT ( 'NONE',  ( 17.75002325595141173, -11.47974371597207899, 33.17467449705390692 ) ) ;
#16649=CARTESIAN_POINT ( 'NONE',  ( -16.28399336328437386, -2.882441371585227508, 31.66841991370172238 ) ) ;
#16650=DIRECTION ( 'NONE',  ( -0.000000000000000000, 0.6427876096865404731, -0.7660444431189770143 ) ) ;
#16652=DIRECTION ( 'NONE',  ( 0.000000000000000000, 0.7660444431189807890, 0.6427876096865361433 ) ) ;
#16653=ORIENTED_EDGE ( 'NONE', *, *, #19415, .T. ) ;
#16654=CARTESIAN_POINT ( 'NONE',  ( 13.38461538461538680, -2.486705287966279876, 31.30864560766543647 ) ) ;
#16655=CARTESIAN_POINT ( 'NONE',  ( -16.21911659980693443, -11.94971097300153140, 32.03036669348370680 ) ) ;
#16656=VERTEX_POINT ( 'NONE', #17198 ) ;
#16657=CARTESIAN_POINT ( 'NONE',  ( -13.51530685128294351, -11.18331474514187995, 33.13161551792790505 ) ) ;
#16658=CARTESIAN_POINT ( 'NONE',  ( 14.24160889673642849, -12.10708131394839349, 31.69288490824020244 ) ) ;
#16659=CARTESIAN_POINT ( 'NONE',  ( 15.45354889974729318, -3.020022701398814569, 32.48759521482552515 ) ) ;
#16660=CARTESIAN_POINT ( 'NONE',  ( 11.60371667797437567, -8.656820664281605460, 34.87096338111211224 ) ) ;
#16661=AXIS2_PLACEMENT_3D ( 'NONE', #60526, #80822, #68615 ) ;
#16662=EDGE_CURVE ( 'NONE', #77586, #57769, #42594, .T. ) ;
#16663=CARTESIAN_POINT ( 'NONE',  ( -0.3962828902624371263, -11.48612834413965977, 32.76840700105972815 ) ) ;
#16664=CARTESIAN_POINT ( 'NONE',  ( 11.40777007179398161, -6.413092428213692742, 34.63065189839063152 ) ) ;
#16665=CARTESIAN_POINT ( 'NONE',  ( -7.912237257109724808, -12.37446782046654192, 30.86335684631486487 ) ) ;
#16666=EDGE_CURVE ( 'NONE', #42722, #76991, #65224, .T. ) ;
#16668=VERTEX_POINT ( 'NONE', #11790 ) ;
#16669=CARTESIAN_POINT ( 'NONE',  ( -16.37733107841048508, -9.417330523894424488, 34.63758898049880486 ) ) ;
#16670=CARTESIAN_POINT ( 'NONE',  ( 8.992242120843618736, -11.76359900205217635, 32.36225158514719880 ) ) ;
#16671=CYLINDRICAL_SURFACE ( 'NONE', #5940, 0.2499999999999979738 ) ;
#16673=B_SPLINE_CURVE_WITH_KNOTS ( 'NONE', 3,
 ( #68540, #21234, #47378, #61771, #14938, #83401, #35653, #40641, #21683, #55032 ),
 .UNSPECIFIED., .F., .F.,
 ( 4, 2, 2, 2, 4 ),
 ( 0.0007817246256747524850, 0.0009771112852218972241, 0.001172497944769042072, 0.001367884604316186702, 0.001563271263863331550 ),
 .UNSPECIFIED. ) ;
#16674=ADVANCED_FACE ( 'NONE', ( #52312 ), #79803, .F. ) ;
#16675=DIRECTION ( 'NONE',  ( -0.000000000000000000, 0.1736481776669307198, -0.9848077530122080203 ) ) ;
#16676=CARTESIAN_POINT ( 'NONE',  ( -17.20707028636129721, -2.619462340734462380, 30.83744416345203021 ) ) ;
#16677=EDGE_CURVE ( 'NONE', #26012, #17825, #71610, .T. ) ;
#16678=B_SPLINE_CURVE_WITH_KNOTS ( 'NONE', 3,
 ( #43526, #22372, #34682, #84532, #62147, #47747 ),
 .UNSPECIFIED., .F., .F.,
 ( 4, 2, 4 ),
 ( 0.0003909569690057804843, 0.0005862646681846042955, 0.0007815723673634281067 ),
 .UNSPECIFIED. ) ;
#16679=ORIENTED_EDGE ( 'NONE', *, *, #70850, .T. ) ;
#16681=CARTESIAN_POINT ( 'NONE',  ( -15.29685161012936412, -3.937682226553330445, 33.60647404775217240 ) ) ;
#16683=VERTEX_POINT ( 'NONE', #51856 ) ;
#16684=DIRECTION ( 'NONE',  ( 0.000000000000000000, 0.1736481776669275834, 0.9848077530122086864 ) ) ;
#16685=VERTEX_POINT ( 'NONE', #9996 ) ;
#16686=CARTESIAN_POINT ( 'NONE',  ( 7.145856592054988354, -4.226511098958374291, 33.85474049983370293 ) ) ;
#16687=CARTESIAN_POINT ( 'NONE',  ( 3.165499230212911908, -4.320704448112771878, 33.92786785259540494 ) ) ;
#16688=CARTESIAN_POINT ( 'NONE',  ( -12.71151520558705528, -10.06842814019191401, 34.32929386961144758 ) ) ;
#16689=DIRECTION ( 'NONE',  ( -0.000000000000000000, 0.7660444431189791237, -0.6427876096865379196 ) ) ;
#16690=ORIENTED_EDGE ( 'NONE', *, *, #3112, .F. ) ;
#16691=DIRECTION ( 'NONE',  ( 0.000000000000000000, 0.3420201433256641055, -0.9396926207859100932 ) ) ;
#16693=CARTESIAN_POINT ( 'NONE',  ( -17.86947456176635640, -12.15418822224088835, 32.17964115625579069 ) ) ;
#16694=CARTESIAN_POINT ( 'NONE',  ( 0.7115927731767747177, -11.28795663066794219, 33.01431243580653785 ) ) ;
#16697=CARTESIAN_POINT ( 'NONE',  ( 11.60371667797437567, -12.70778746994558439, 30.41441678777536595 ) ) ;
#16698=CARTESIAN_POINT ( 'NONE',  ( -14.43783951713053249, -10.88202310037935661, 33.43294751532457099 ) ) ;
#16699=CARTESIAN_POINT ( 'NONE',  ( -11.76138775597768316, -2.758268499246657068, 31.33685645148948140 ) ) ;
#16700=AXIS2_PLACEMENT_3D ( 'NONE', #11052, #17816, #46613 ) ;
#16701=DIRECTION ( 'NONE',  ( 0.000000000000000000, 0.7660444431189822323, -0.6427876096865344779 ) ) ;
#16702=CARTESIAN_POINT ( 'NONE',  ( -16.37677311275300340, -2.889293201056495786, 32.26117774369186009 ) ) ;
#16703=EDGE_CURVE ( 'NONE', #20844, #87573, #22163, .T. ) ;
#16704=ORIENTED_EDGE ( 'NONE', *, *, #5651, .F. ) ;
#16705=ORIENTED_EDGE ( 'NONE', *, *, #63030, .F. ) ;
#16706=FACE_BOUND ( 'NONE', #88777, .T. ) ;
#16707=VERTEX_POINT ( 'NONE', #52757 ) ;
#16708=CARTESIAN_POINT ( 'NONE',  ( -8.096177070375304652, -5.765609946408404518, 34.70566812827425451 ) ) ;
#16709=CARTESIAN_POINT ( 'NONE',  ( 9.561616225640133138, -12.11776431015576172, 31.66791131148498906 ) ) ;
#16710=CARTESIAN_POINT ( 'NONE',  ( 0.5923289025054110368, -12.62708834333097663, 30.88030960425257021 ) ) ;
#16711=ORIENTED_EDGE ( 'NONE', *, *, #55538, .T. ) ;
#16713=VERTEX_POINT ( 'NONE', #18546 ) ;
#16714=EDGE_CURVE ( 'NONE', #37962, #42538, #81367, .T. ) ;
#16715=VERTEX_POINT ( 'NONE', #39713 ) ;
#16716=CARTESIAN_POINT ( 'NONE',  ( -1.450698795571264688, -11.69971097300155272, 32.46337939537587403 ) ) ;
#16717=ORIENTED_EDGE ( 'NONE', *, *, #63505, .F. ) ;
#16718=CYLINDRICAL_SURFACE ( 'NONE', #43380, 0.2500000000000008882 ) ;
#16719=VECTOR ( 'NONE', #14457, 1000.000000000000114 ) ;
#16720=DIRECTION ( 'NONE',  ( -0.000000000000000000, 0.8660254037844397068, -0.4999999999999978906 ) ) ;
#16721=CARTESIAN_POINT ( 'NONE',  ( -2.438382910802612713, -12.35290016733513951, 31.75349464988449455 ) ) ;
#16722=FACE_BOUND ( 'NONE', #31884, .T. ) ;
#16723=ORIENTED_EDGE ( 'NONE', *, *, #17473, .T. ) ;
#16724=CARTESIAN_POINT ( 'NONE',  ( -1.515092092731847861, -7.276988635370452485, 34.74523720219453793 ) ) ;
#16726=DIRECTION ( 'NONE',  ( 0.000000000000000000, 0.9848077530122072432, -0.1736481776669354937 ) ) ;
#16727=CARTESIAN_POINT ( 'NONE',  ( 14.30769230769231015, -6.681629849574314051, 35.83090037661290239 ) ) ;
#16728=CARTESIAN_POINT ( 'NONE',  ( -11.53846153846153655, -3.050289026998446396, 32.03036669348365706 ) ) ;
#16729=VERTEX_POINT ( 'NONE', #61280 ) ;
#16730=VECTOR ( 'NONE', #34080, 1000.000000000000000 ) ;
#16733=ADVANCED_FACE ( 'NONE', ( #5479 ), #20752, .F. ) ;
#16734=EDGE_LOOP ( 'NONE', ( #72780, #65253 ) ) ;
#16735=ORIENTED_EDGE ( 'NONE', *, *, #35123, .F. ) ;
#16736=CARTESIAN_POINT ( 'NONE',  ( -18.22559223176554966, -2.251337733188375267, 29.87809195722895339 ) ) ;
#16737=CYLINDRICAL_SURFACE ( 'NONE', #26116, 0.2500000000000002220 ) ;
#16738=CARTESIAN_POINT ( 'NONE',  ( 16.08776274289027342, -5.557115091759785130, 34.35708131394839171 ) ) ;
#16739=CARTESIAN_POINT ( 'NONE',  ( -4.023054346021365468, -4.118422570099827595, 33.43335022499816489 ) ) ;
#16740=CARTESIAN_POINT ( 'NONE',  ( 13.38461538461538680, -1.509761064869970415, 31.06009739812519044 ) ) ;
#16741=DIRECTION ( 'NONE',  ( 0.000000000000000000, 0.7660444431189807890, 0.6427876096865361433 ) ) ;
#16742=ORIENTED_EDGE ( 'NONE', *, *, #7047, .T. ) ;
#16743=CYLINDRICAL_SURFACE ( 'NONE', #86051, 0.2499999999999986955 ) ;
#16744=CARTESIAN_POINT ( 'NONE',  ( 10.61538461538461675, -4.945431358278436385, 36.03766855953609394 ) ) ;
#16746=EDGE_CURVE ( 'NONE', #42102, #56815, #24386, .T. ) ;
#16747=CARTESIAN_POINT ( 'NONE',  ( 15.48076923077066702, -7.500000000000155431, 34.75000000000007105 ) ) ;
#16748=ORIENTED_EDGE ( 'NONE', *, *, #29442, .T. ) ;
#16749=ORIENTED_EDGE ( 'NONE', *, *, #83334, .F. ) ;
#16750=FACE_BOUND ( 'NONE', #2002, .T. ) ;
#16751=VECTOR ( 'NONE', #13481, 1000.000000000000000 ) ;
#16752=CARTESIAN_POINT ( 'NONE',  ( 11.60452887181161508, -12.34228464037088813, 31.77849191805839268 ) ) ;
#16753=CARTESIAN_POINT ( 'NONE',  ( -6.700114019515439168, -7.369474270740069777, 34.74850911626239736 ) ) ;
#16754=ORIENTED_EDGE ( 'NONE', *, *, #13423, .F. ) ;
#16755=CARTESIAN_POINT ( 'NONE',  ( 3.930919194939304084, -11.43668979543635089, 33.22377378376089752 ) ) ;
#16756=CARTESIAN_POINT ( 'NONE',  ( 6.700150705560777631, -10.61292498521070549, 33.66303323003028680 ) ) ;
#16757=CARTESIAN_POINT ( 'NONE',  ( 15.93036121012220541, -8.496056993536548418, 34.65000542017679663 ) ) ;
#16759=ORIENTED_EDGE ( 'NONE', *, *, #22544, .T. ) ;
#16761=CARTESIAN_POINT ( 'NONE',  ( -7.623142494540996239, -10.61302985866384141, 33.66295027996417843 ) ) ;
#16762=EDGE_LOOP ( 'NONE', ( #50973, #8967 ) ) ;
#16763=CARTESIAN_POINT ( 'NONE',  ( 18.00000000000000000, -5.471508081941601098, 34.59228464037088457 ) ) ;
#16764=ORIENTED_EDGE ( 'NONE', *, *, #64435, .F. ) ;
#16767=CYLINDRICAL_SURFACE ( 'NONE', #73081, 0.2500000000000009437 ) ;
#16768=B_SPLINE_CURVE_WITH_KNOTS ( 'NONE', 3,
 ( #8802, #2464, #64604, #30832, #44328, #10122, #58302, #16436, #72263, #43464 ),
 .UNSPECIFIED., .F., .F.,
 ( 4, 2, 2, 2, 4 ),
 ( 0.0007817359430256361858, 0.0009771253907250041296, 0.001172514838424372182, 0.001367904286123740234, 0.001563293733823108286 ),
 .UNSPECIFIED. ) ;
#16769=CARTESIAN_POINT ( 'NONE',  ( -12.52762084089859584, -10.67929555188718460, 33.92786785259543336 ) ) ;
#16770=CARTESIAN_POINT ( 'NONE',  ( -14.55771553191376277, -8.475808217655753651, 34.90892951860618609 ) ) ;
#16771=EDGE_CURVE ( 'NONE', #35211, #14267, #47784, .T. ) ;
#16772=CARTESIAN_POINT ( 'NONE',  ( 6.222779541268410597, -2.847695495035524882, 31.58253572463339509 ) ) ;
#16774=ORIENTED_EDGE ( 'NONE', *, *, #14499, .T. ) ;
#16775=DIRECTION ( 'NONE',  ( 0.000000000000000000, 0.8660254037844377084, -0.5000000000000015543 ) ) ;
#16776=CARTESIAN_POINT ( 'NONE',  ( 13.60757851888206105, -7.369474539155828730, 34.99858011523957657 ) ) ;
#16777=EDGE_CURVE ( 'NONE', #52397, #85757, #70502, .T. ) ;
#16778=ORIENTED_EDGE ( 'NONE', *, *, #74903, .F. ) ;
#16780=ORIENTED_EDGE ( 'NONE', *, *, #36781, .F. ) ;
#16781=CARTESIAN_POINT ( 'NONE',  ( -10.61538461538461320, -11.16473453929635440, 33.15142922261926373 ) ) ;
#16784=CARTESIAN_POINT ( 'NONE',  ( -5.076923076923075762, -2.499999999999998668, 29.50000000000001066 ) ) ;
#16785=CARTESIAN_POINT ( 'NONE',  ( 8.992243613324164997, -11.43677907613344757, 33.22367315496202167 ) ) ;
#16786=CARTESIAN_POINT ( 'NONE',  ( -17.07692307692319744, -11.67786785259630911, 32.92929555188603530 ) ) ;
#16787=DIRECTION ( 'NONE',  ( -0.000000000000000000, -0.9848077530122086864, -0.1736481776669273613 ) ) ;
#16788=ORIENTED_EDGE ( 'NONE', *, *, #41453, .T. ) ;
#16789=AXIS2_PLACEMENT_3D ( 'NONE', #414, #55346, #1736 ) ;
#16791=LINE ( 'NONE', #41403, #49159 ) ;
#16792=CARTESIAN_POINT ( 'NONE',  ( -8.992157728137614825, -11.43668979543635089, 33.22377378376089752 ) ) ;
#16793=EDGE_CURVE ( 'NONE', #87653, #42680, #86635, .T. ) ;
#16795=ORIENTED_EDGE ( 'NONE', *, *, #53839, .F. ) ;
#16797=VECTOR ( 'NONE', #6088, 1000.000000000000227 ) ;
#16798=VERTEX_POINT ( 'NONE', #44 ) ;
#16799=CARTESIAN_POINT ( 'NONE',  ( -18.00000000000012079, -8.656820664282943056, 34.87096338111179961 ) ) ;
#16801=CARTESIAN_POINT ( 'NONE',  ( 10.54930223602447903, -3.322132147404559532, 32.92929555188719348 ) ) ;
#16802=ADVANCED_FACE ( 'NONE', ( #26629 ), #54086, .F. ) ;
#16803=DIRECTION ( 'NONE',  ( 0.000000000000000000, 0.8660254037844377084, 0.5000000000000015543 ) ) ;
#16804=ORIENTED_EDGE ( 'NONE', *, *, #62280, .F. ) ;
#16806=CARTESIAN_POINT ( 'NONE',  ( -1.514763354347081092, -12.70455904226513866, 30.44083106164009322 ) ) ;
#16807=CARTESIAN_POINT ( 'NONE',  ( 10.48469314871705826, -3.530157926970578952, 32.79014554554150607 ) ) ;
#16808=CARTESIAN_POINT ( 'NONE',  ( -13.60810030917971680, -10.97335522853832579, 33.68706563782419749 ) ) ;
#16809=CARTESIAN_POINT ( 'NONE',  ( -9.692307692307691624, -3.322132147404559976, 32.92929555188717927 ) ) ;
#16810=B_SPLINE_CURVE_WITH_KNOTS ( 'NONE', 3,
 ( #4565, #59506, #87010, #30698, #37004, #45988, #78439, #16739, #44192, #71681 ),
 .UNSPECIFIED., .F., .F.,
 ( 4, 2, 2, 2, 4 ),
 ( 0.0007817359430256303312, 0.0009771253907249965402, 0.001172514838424362641, 0.001367904286123728958, 0.001563293733823095059 ),
 .UNSPECIFIED. ) ;
#16811=ADVANCED_FACE ( 'NONE', ( #6793 ), #74827, .F. ) ;
#16813=CARTESIAN_POINT ( 'NONE',  ( 7.715463243043538810, -11.37499894934982514, 33.29245874905763003 ) ) ;
#16816=CARTESIAN_POINT ( 'NONE',  ( -9.627052121031661969, -12.27809138561124591, 31.22303859784720359 ) ) ;
#16817=EDGE_CURVE ( 'NONE', #72129, #68389, #74822, .T. ) ;
#16818=CARTESIAN_POINT ( 'NONE',  ( -16.21992956480203318, -11.16473453929635440, 33.15142922261925662 ) ) ;
#16819=AXIS2_PLACEMENT_3D ( 'NONE', #54473, #54924, #75627 ) ;
#16820=CARTESIAN_POINT ( 'NONE',  ( 7.596130621932389637, -12.45566812827425096, 31.48439005359158926 ) ) ;
#16821=DIRECTION ( 'NONE',  ( -0.000000000000000000, -0.7660444431189791237, -0.6427876096865379196 ) ) ;
#16822=CARTESIAN_POINT ( 'NONE',  ( 9.626224281351815293, -8.120952969808774569, 34.71129190930000163 ) ) ;
#16824=ORIENTED_EDGE ( 'NONE', *, *, #18960, .F. ) ;
#16825=EDGE_CURVE ( 'NONE', #58630, #58791, #87756, .T. ) ;
#16826=ORIENTED_EDGE ( 'NONE', *, *, #1445, .F. ) ;
#16827=ORIENTED_EDGE ( 'NONE', *, *, #37390, .T. ) ;
#16828=ORIENTED_EDGE ( 'NONE', *, *, #30781, .F. ) ;
#16829=VECTOR ( 'NONE', #30955, 1000.000000000000114 ) ;
#16830=CARTESIAN_POINT ( 'NONE',  ( -1.384615384615505151, -3.300289026999228881, 32.46337939537708905 ) ) ;
#16831=CARTESIAN_POINT ( 'NONE',  ( 11.47237915910140771, -9.058645607665454236, 34.76329471203372634 ) ) ;
#16832=CYLINDRICAL_SURFACE ( 'NONE', #68371, 0.2499999999999995559 ) ;
#16833=CARTESIAN_POINT ( 'NONE',  ( 17.14299142792551578, -4.098570777380720287, 33.41473453929635440 ) ) ;
#16834=CARTESIAN_POINT ( 'NONE',  ( -13.25408968285182176, -6.001044277235009439, 34.52024696741798948 ) ) ;
#16835=CARTESIAN_POINT ( 'NONE',  ( 2.980745993476265898, -5.851115903089112003, 34.47074536777953568 ) ) ;
#16836=B_SPLINE_CURVE_WITH_KNOTS ( 'NONE', 3,
 ( #8290, #68214, #88953, #1080, #27222, #35764, #34859, #7403, #28561, #82630 ),
 .UNSPECIFIED., .F., .F.,
 ( 4, 2, 2, 2, 4 ),
 ( 0.0007817359430256314154, 0.0009771253907249978412, 0.001172514838424364375, 0.001367904286123730693, 0.001563293733823097227 ),
 .UNSPECIFIED. ) ;
#16837=CARTESIAN_POINT ( 'NONE',  ( -18.00000000000012079, -10.21337939537710504, 33.94971097300076224 ) ) ;
#16838=CARTESIAN_POINT ( 'NONE',  ( 17.01167314514899331, -2.255955759149247619, 30.00000000000014566 ) ) ;
#16839=B_SPLINE_CURVE_WITH_KNOTS ( 'NONE', 3,
 ( #72266, #51084, #56972, #36275, #15557, #64605 ),
 .UNSPECIFIED., .F., .F.,
 ( 4, 2, 4 ),
 ( 0.000000000000000000, 0.0001954784845028888327, 0.0003909569690057776653 ),
 .UNSPECIFIED. ) ;
#16840=ORIENTED_EDGE ( 'NONE', *, *, #20438, .F. ) ;
#16841=B_SPLINE_CURVE_WITH_KNOTS ( 'NONE', 3,
 ( #37514, #79404, #45159, #64979, #72633, #38863, #10941, #3283, #31656, #32100 ),
 .UNSPECIFIED., .F., .F.,
 ( 4, 2, 2, 2, 4 ),
 ( 0.000000000000000000, 0.0001954339857564073388, 0.0003908679715128146777, 0.0005863019572692220165, 0.0007817359430256293554 ),
 .UNSPECIFIED. ) ;
#16842=EDGE_CURVE ( 'NONE', #29464, #54551, #7695, .T. ) ;
#16843=ORIENTED_EDGE ( 'NONE', *, *, #18400, .T. ) ;
#16844=ORIENTED_EDGE ( 'NONE', *, *, #49109, .T. ) ;
#16846=ORIENTED_EDGE ( 'NONE', *, *, #35105, .T. ) ;
#16847=CARTESIAN_POINT ( 'NONE',  ( -9.942330929600657896, -9.271318131107980420, 34.42618302367067429 ) ) ;
#16848=CARTESIAN_POINT ( 'NONE',  ( -17.86920955903304886, -11.37503395064541678, 33.29242100308974983 ) ) ;
#16849=B_SPLINE_CURVE_WITH_KNOTS ( 'NONE', 3,
 ( #59661, #65525, #4729, #85814, #87160, #30416, #51102, #32204, #51543, #38966 ),
 .UNSPECIFIED., .F., .F.,
 ( 4, 2, 2, 2, 4 ),
 ( 0.000000000000000000, 0.0001954311564186863323, 0.0003908623128373726646, 0.0005862934692560590241, 0.0007817246256747453293 ),
 .UNSPECIFIED. ) ;
#16850=CARTESIAN_POINT ( 'NONE',  ( -0.4615384615385840772, -3.643525952248795718, 33.31231777344771672 ) ) ;
#16852=CARTESIAN_POINT ( 'NONE',  ( 4.403900465484467119, -2.564540009722896752, 30.55348353981670684 ) ) ;
#16853=ORIENTED_EDGE ( 'NONE', *, *, #47781, .T. ) ;
#16854=ORIENTED_EDGE ( 'NONE', *, *, #68012, .T. ) ;
#16855=CARTESIAN_POINT ( 'NONE',  ( -13.38461538461538325, -2.833524468853757305, 32.15551576947925838 ) ) ;
#16856=ORIENTED_EDGE ( 'NONE', *, *, #78621, .T. ) ;
#16857=FACE_BOUND ( 'NONE', #7115, .T. ) ;
#16858=CARTESIAN_POINT ( 'NONE',  ( 8.769230769230768274, -12.34228464037088635, 31.77849191805839268 ) ) ;
#16859=CARTESIAN_POINT ( 'NONE',  ( -4.087777802843713282, -11.69971097300155272, 32.46337939537588113 ) ) ;
#16861=CARTESIAN_POINT ( 'NONE',  ( -4.153846153845845102, -2.506253911140614576, 30.00000000000323297 ) ) ;
#16862=CARTESIAN_POINT ( 'NONE',  ( 11.40777093535123043, -6.369640206132551441, 34.87707690430378449 ) ) ;
#16863=AXIS2_PLACEMENT_3D ( 'NONE', #46811, #39630, #32411 ) ;
#16864=CARTESIAN_POINT ( 'NONE',  ( -5.076923076923075762, -12.78798330534102945, 29.74999999999997868 ) ) ;
#16865=ORIENTED_EDGE ( 'NONE', *, *, #78573, .F. ) ;
#16866=CARTESIAN_POINT ( 'NONE',  ( -18.00000000000000000, -9.580279128651994824, 36.19647103217484130 ) ) ;
#16867=CARTESIAN_POINT ( 'NONE',  ( -13.25382357679059986, -11.71459661697925903, 32.44059661609676937 ) ) ;
#16868=EDGE_LOOP ( 'NONE', ( #10964, #2510, #78224, #14360 ) ) ;
#16869=CYLINDRICAL_SURFACE ( 'NONE', #27267, 0.2499999999999997502 ) ;
#16871=CARTESIAN_POINT ( 'NONE',  ( 8.703148389870634105, -11.35647404775217595, 33.31231777344666511 ) ) ;
#16872=CARTESIAN_POINT ( 'NONE',  ( 13.38461538461526601, -2.625532179533778709, 30.86335684631627174 ) ) ;
#16873=CARTESIAN_POINT ( 'NONE',  ( 13.38461538461538680, -1.790695186598648903, 34.54067556320373455 ) ) ;
#16874=CARTESIAN_POINT ( 'NONE',  ( 7.912322987116502837, -7.250054483168843156, 34.74374881642865631 ) ) ;
#16875=CARTESIAN_POINT ( 'NONE',  ( -10.61538461538461320, -2.708943851104267164, 35.45975837776705220 ) ) ;
#16876=LINE ( 'NONE', #44326, #79761 ) ;
#16877=DIRECTION ( 'NONE',  ( -0.000000000000000000, 0.6427876096865404731, -0.7660444431189770143 ) ) ;
#16878=DIRECTION ( 'NONE',  ( -0.000000000000000000, 0.1736481776669307198, -0.9848077530122080203 ) ) ;
#16879=CARTESIAN_POINT ( 'NONE',  ( 1.450683735617824821, -11.16473453929635440, 33.15142922261926373 ) ) ;
#16880=CARTESIAN_POINT ( 'NONE',  ( 3.480769230769234834, -2.499999999999999556, 29.81604066197450109 ) ) ;
#16881=CARTESIAN_POINT ( 'NONE',  ( -0.4615384615384611200, -4.786620604624113540, 33.94971097300155094 ) ) ;
#16882=DIRECTION ( 'NONE',  ( 0.000000000000000000, 0.4999999999999985567, 0.8660254037844395958 ) ) ;
#16884=ORIENTED_EDGE ( 'NONE', *, *, #12690, .F. ) ;
#16886=EDGE_LOOP ( 'NONE', ( #83392, #38682 ) ) ;
#16887=EDGE_CURVE ( 'NONE', #22384, #53843, #76136, .T. ) ;
#16888=CARTESIAN_POINT ( 'NONE',  ( -9.692307692307691624, -5.557115091759785130, 34.35708131394839171 ) ) ;
#16890=VERTEX_POINT ( 'NONE', #83806 ) ;
#16891=CARTESIAN_POINT ( 'NONE',  ( -4.023054346021365468, -11.18335022499818621, 33.13157742990016885 ) ) ;
#16892=EDGE_CURVE ( 'NONE', #17395, #84497, #3963, .T. ) ;
#16893=ORIENTED_EDGE ( 'NONE', *, *, #27145, .T. ) ;
#16894=CYLINDRICAL_SURFACE ( 'NONE', #64221, 0.2500000000000012212 ) ;
#16896=CARTESIAN_POINT ( 'NONE',  ( 17.07692307692307665, -9.058645607665452459, 34.76329471203371924 ) ) ;
#16897=CARTESIAN_POINT ( 'NONE',  ( 9.915319043920545639, -11.24521262558773493, 33.06293181088029343 ) ) ;
#16898=CARTESIAN_POINT ( 'NONE',  ( -3.100243792535588128, -12.50538340440932217, 31.33453814440721885 ) ) ;
#16899=CARTESIAN_POINT ( 'NONE',  ( -6.222926958906846551, -2.523278758544489797, 31.42238647778637528 ) ) ;
#16901=CARTESIAN_POINT ( 'NONE',  ( -7.596208327805705096, -2.824170634883622633, 31.52227843825338738 ) ) ;
#16902=CARTESIAN_POINT ( 'NONE',  ( -7.846153846153965716, -12.27809138561165270, 31.22303859784587132 ) ) ;
#16903=ADVANCED_FACE ( 'NONE', ( #28857 ), #35606, .F. ) ;
#16905=CARTESIAN_POINT ( 'NONE',  ( 1.634669696253700621, -3.136992222400443175, 32.19305428654138979 ) ) ;
#16907=VECTOR ( 'NONE', #72172, 1000.000000000000114 ) ;
#16909=DIRECTION ( 'NONE',  ( 0.000000000000000000, 0.4999999999999985567, 0.8660254037844395958 ) ) ;
#16911=B_SPLINE_CURVE_WITH_KNOTS ( 'NONE', 3,
 ( #79463, #39375, #17763, #11444, #53307, #38927, #66385, #4692, #66833, #32164 ),
 .UNSPECIFIED., .F., .F.,
 ( 4, 2, 2, 2, 4 ),
 ( 0.000000000000000000, 0.0001954311564186874436, 0.0003908623128373748873, 0.0005862934692560622767, 0.0007817246256747497745 ),
 .UNSPECIFIED. ) ;
#16914=CARTESIAN_POINT ( 'NONE',  ( -11.47320596718551045, -8.613356846314928816, 34.62446782046653482 ) ) ;
#16915=CARTESIAN_POINT ( 'NONE',  ( 1.161130460051056579, -5.827078755546626354, 34.72654668319379567 ) ) ;
#16917=CARTESIAN_POINT ( 'NONE',  ( 14.24160992833217065, -3.322132147404559532, 32.92929555188719348 ) ) ;
#16918=CARTESIAN_POINT ( 'NONE',  ( 2.177545098254085154, -12.27039167877662251, 31.24851455888617835 ) ) ;
#16920=ORIENTED_EDGE ( 'NONE', *, *, #85141, .F. ) ;
#16921=CARTESIAN_POINT ( 'NONE',  ( -10.48533718013415950, -7.723484941389743952, 34.99544897038808955 ) ) ;
#16922=VERTEX_POINT ( 'NONE', #15780 ) ;
#16923=AXIS2_PLACEMENT_3D ( 'NONE', #69798, #83326, #7221 ) ;
#16924=EDGE_CURVE ( 'NONE', #76326, #5654, #38284, .T. ) ;
#16926=CARTESIAN_POINT ( 'NONE',  ( -15.23076923076922995, -12.37446782046654192, 30.86335684631486131 ) ) ;
#16927=CARTESIAN_POINT ( 'NONE',  ( 5.076923076923075762, -11.69971097300155272, 32.46337939537588113 ) ) ;
#16928=CARTESIAN_POINT ( 'NONE',  ( 6.700149964170072359, -2.889293201056495786, 32.26117774369186009 ) ) ;
#16930=CARTESIAN_POINT ( 'NONE',  ( -13.31935981333936425, -9.442884908240273489, 34.35708131394835618 ) ) ;
#16932=VERTEX_POINT ( 'NONE', #17548 ) ;
#16934=CARTESIAN_POINT ( 'NONE',  ( 8.769230769230647482, -3.835265460704628371, 33.15142922262033665 ) ) ;
#16935=VERTEX_POINT ( 'NONE', #23832 ) ;
#16938=EDGE_CURVE ( 'NONE', #73980, #35887, #67327, .T. ) ;
#16939=CARTESIAN_POINT ( 'NONE',  ( 18.22277966897806678, -2.353885683473779800, 30.79025554430704759 ) ) ;
#16940=CARTESIAN_POINT ( 'NONE',  ( 16.28437185560971656, -12.45806712695776319, 30.39783852428763566 ) ) ;
#16941=DIRECTION ( 'NONE',  ( -0.000000000000000000, -0.000000000000000000, -1.000000000000000000 ) ) ;
#16942=CARTESIAN_POINT ( 'NONE',  ( 10.48469401227430708, -4.684245665217972032, 34.18127051446801090 ) ) ;
#16943=CARTESIAN_POINT ( 'NONE',  ( -4.376724836274800801, -7.630691491037286056, 34.74850469731152458 ) ) ;
#16944=CARTESIAN_POINT ( 'NONE',  ( 16.15384615384615330, -1.044019251281081972, 31.83374038241031911 ) ) ;
#16945=ORIENTED_EDGE ( 'NONE', *, *, #51918, .T. ) ;
#16946=EDGE_CURVE ( 'NONE', #34142, #84846, #83430, .T. ) ;
#16947=ORIENTED_EDGE ( 'NONE', *, *, #19034, .F. ) ;
#16949=ORIENTED_EDGE ( 'NONE', *, *, #15238, .F. ) ;
#16950=CIRCLE ( 'NONE', #50001, 0.2500000000000002220 ) ;
#16951=CARTESIAN_POINT ( 'NONE',  ( 15.45354877203763877, -5.913360116392397892, 34.49180327182771322 ) ) ;
#16952=ORIENTED_EDGE ( 'NONE', *, *, #56076, .F. ) ;
#16953=CARTESIAN_POINT ( 'NONE',  ( -9.942330916529147800, -10.18141759479407327, 34.26406193332782379 ) ) ;
#16954=CARTESIAN_POINT ( 'NONE',  ( 5.999999999999880096, -12.46129190930018460, 30.37095296980731973 ) ) ;
#16955=EDGE_CURVE ( 'NONE', #72548, #35799, #11234, .T. ) ;
#16956=EDGE_CURVE ( 'NONE', #65236, #34858, #4013, .T. ) ;
#16957=CARTESIAN_POINT ( 'NONE',  ( -0.3310130233048164672, -9.503571793651733657, 34.60286762892837942 ) ) ;
#16958=ORIENTED_EDGE ( 'NONE', *, *, #48163, .T. ) ;
#16959=AXIS2_PLACEMENT_3D ( 'NONE', #33435, #19469, #87068 ) ;
#16960=CYLINDRICAL_SURFACE ( 'NONE', #62692, 0.2500000000000008882 ) ;
#16961=ORIENTED_EDGE ( 'NONE', *, *, #1623, .T. ) ;
#16962=EDGE_CURVE ( 'NONE', #12394, #67447, #38704, .T. ) ;
#16963=CARTESIAN_POINT ( 'NONE',  ( 2.307692307692187583, -9.442884908241554243, 34.35708131394783038 ) ) ;
#16965=CARTESIAN_POINT ( 'NONE',  ( -17.86920955903304886, -2.494656445102014342, 31.33466734024120015 ) ) ;
#16966=CARTESIAN_POINT ( 'NONE',  ( 5.869309396889695662, -12.35290016733513951, 31.75349464988449455 ) ) ;
#16967=CARTESIAN_POINT ( 'NONE',  ( 1.384615384615264011, -8.656820664282941280, 34.87096338111179961 ) ) ;
#16968=CARTESIAN_POINT ( 'NONE',  ( -1.253824943648433887, -8.191423895709840863, 34.95447573519442130 ) ) ;
#16969=FACE_OUTER_BOUND ( 'NONE', #42880, .T. ) ;
#16970=ORIENTED_EDGE ( 'NONE', *, *, #10864, .F. ) ;
#16971=CARTESIAN_POINT ( 'NONE',  ( -11.40793583669797151, -12.27024696741798948, 31.24895572276497546 ) ) ;
#16972=CARTESIAN_POINT ( 'NONE',  ( 6.923076923076924238, -8.318370150425687726, 35.83090037661290239 ) ) ;
#16973=VERTEX_POINT ( 'NONE', #44999 ) ;
#16974=CARTESIAN_POINT ( 'NONE',  ( 6.923076923076924238, -2.721908614388771852, 31.22303859784724978 ) ) ;
#16975=CARTESIAN_POINT ( 'NONE',  ( 10.61538461538449596, -6.879047030192662504, 34.71129190930017927 ) ) ;
#16976=CARTESIAN_POINT ( 'NONE',  ( 15.93091919493930320, -6.459968553980840689, 34.89616026154728701 ) ) ;
#16977=AXIS2_PLACEMENT_3D ( 'NONE', #931, #70723, #62184 ) ;
#16978=CARTESIAN_POINT ( 'NONE',  ( -16.37733107841048508, -12.11044203135681840, 32.26167407432752299 ) ) ;
#16979=CARTESIAN_POINT ( 'NONE',  ( -7.779987239562206724, -7.250054591869668386, 34.99404684341514127 ) ) ;
#16980=FACE_BOUND ( 'NONE', #6094, .T. ) ;
#16981=LINE ( 'NONE', #10232, #8778 ) ;
#16982=CARTESIAN_POINT ( 'NONE',  ( -15.23076923076922995, -5.180354513474913603, 36.12317359536750416 ) ) ;
#16984=CARTESIAN_POINT ( 'NONE',  ( -1.161604033002533898, -12.15243808032445827, 31.58219941686247978 ) ) ;
#16985=CYLINDRICAL_SURFACE ( 'NONE', #3176, 0.2499999999999986955 ) ;
#16986=CARTESIAN_POINT ( 'NONE',  ( -10.61538461538461320, -8.564572088678739092, 35.78748833219616898 ) ) ;
#16987=DIRECTION ( 'NONE',  ( -0.000000000000000000, -0.8660254037844399289, -0.4999999999999980016 ) ) ;
#16989=EDGE_CURVE ( 'NONE', #33332, #49403, #80243, .T. ) ;
#16990=ORIENTED_EDGE ( 'NONE', *, *, #671, .T. ) ;
#16991=CARTESIAN_POINT ( 'NONE',  ( 16.15384615384603251, -9.528491918059723176, 34.59228464037033035 ) ) ;
#16992=AXIS2_PLACEMENT_3D ( 'NONE', #55253, #1647, #40867 ) ;
#16993=CARTESIAN_POINT ( 'NONE',  ( -4.284537620513712675, -3.062553014421049546, 32.05460306192773601 ) ) ;
#16994=CARTESIAN_POINT ( 'NONE',  ( 5.749976775778542937, -5.765609946408404518, 34.70566812827425451 ) ) ;
#16995=LINE ( 'NONE', #58406, #58235 ) ;
#16996=CARTESIAN_POINT ( 'NONE',  ( 7.715462379486287325, -4.809359713505815925, 33.96456829005828837 ) ) ;
#16997=CARTESIAN_POINT ( 'NONE',  ( -5.207483668664997012, -2.504760397472873823, 29.97295953869789997 ) ) ;
#16999=CARTESIAN_POINT ( 'NONE',  ( -1.634615384615383027, -7.500000000000001776, 35.00000000000000000 ) ) ;
#17000=CARTESIAN_POINT ( 'NONE',  ( 0.6843180028068712728, -3.755027918224367767, 33.06320215134714857 ) ) ;
#17001=CARTESIAN_POINT ( 'NONE',  ( -7.846153846153967493, -10.33852847137269571, 34.16647553114546554 ) ) ;
#17002=LINE ( 'NONE', #9370, #34380 ) ;
#17003=LINE ( 'NONE', #71944, #42553 ) ;
#17004=DIRECTION ( 'NONE',  ( -0.000000000000000000, 0.9396926207859093161, -0.3420201433256663259 ) ) ;
#17005=EDGE_CURVE ( 'NONE', #52632, #43220, #43456, .T. ) ;
#17006=DIRECTION ( 'NONE',  ( -0.000000000000000000, 0.7660444431189791237, -0.6427876096865379196 ) ) ;
#17007=CARTESIAN_POINT ( 'NONE',  ( -17.07692307692307665, -5.557115091759785130, 34.35708131394839171 ) ) ;
#17009=B_SPLINE_CURVE_WITH_KNOTS ( 'NONE', 3,
 ( #86177, #32108, #87077, #79412, #65877, #52811, #10507, #25796, #24446, #51456 ),
 .UNSPECIFIED., .F., .F.,
 ( 4, 2, 2, 2, 4 ),
 ( 0.0007817246256747446788, 0.0009771112852218872494, 0.001172497944769029929, 0.001367884604316172391, 0.001563271263863315070 ),
 .UNSPECIFIED. ) ;
#17010=FACE_OUTER_BOUND ( 'NONE', #72206, .T. ) ;
#17011=CYLINDRICAL_SURFACE ( 'NONE', #74833, 0.2500000000000008882 ) ;
#17013=CARTESIAN_POINT ( 'NONE',  ( 6.673100179028331524, -4.818429247618089661, 34.26397095200675125 ) ) ;
#17014=VECTOR ( 'NONE', #12789, 1000.000000000000227 ) ;
#17015=CARTESIAN_POINT ( 'NONE',  ( 5.999999999999880096, -10.90142922262034020, 33.41473453929536674 ) ) ;
#17016=EDGE_LOOP ( 'NONE', ( #56794, #27153 ) ) ;
#17017=CARTESIAN_POINT ( 'NONE',  ( -18.25002323729296450, -9.271318131107980420, 34.42618302367067429 ) ) ;
#17018=CARTESIAN_POINT ( 'NONE',  ( -6.923076923076922462, -2.499999999999998668, 29.75000000000001421 ) ) ;
#17019=CARTESIAN_POINT ( 'NONE',  ( -15.23076923076922995, -4.102666532097928531, 36.13435417666054406 ) ) ;
#17020=ORIENTED_EDGE ( 'NONE', *, *, #29687, .F. ) ;
#17021=CARTESIAN_POINT ( 'NONE',  ( -12.71156168575991785, -9.356822207818506598, 34.66110646841856635 ) ) ;
#17022=FACE_OUTER_BOUND ( 'NONE', #81463, .T. ) ;
#17023=CARTESIAN_POINT ( 'NONE',  ( 4.153846153846154188, -13.49023893513002648, 31.06009739812518688 ) ) ;
#17024=AXIS2_PLACEMENT_3D ( 'NONE', #27017, #27461, #76351 ) ;
#17025=CARTESIAN_POINT ( 'NONE',  ( 1.384615384615386802, -13.87047571288749737, 32.06866353760679544 ) ) ;
#17026=ADVANCED_FACE ( 'NONE', ( #58508 ), #24284, .T. ) ;
#17027=ORIENTED_EDGE ( 'NONE', *, *, #61851, .T. ) ;
#17028=CARTESIAN_POINT ( 'NONE',  ( -12.46153846153858424, -2.379036618888197729, 30.90682066428292885 ) ) ;
#17029=VECTOR ( 'NONE', #20029, 1000.000000000000114 ) ;
#17030=CARTESIAN_POINT ( 'NONE',  ( -1.384615384615383471, -5.557115091759785130, 34.35708131394839171 ) ) ;
#17031=VERTEX_POINT ( 'NONE', #72481 ) ;
#17032=ORIENTED_EDGE ( 'NONE', *, *, #36849, .T. ) ;
#17034=VERTEX_POINT ( 'NONE', #10788 ) ;
#17036=DIRECTION ( 'NONE',  ( -0.000000000000000000, -0.8660254037844399289, -0.4999999999999980016 ) ) ;
#17038=EDGE_CURVE ( 'NONE', #70094, #42102, #4930, .T. ) ;
#17039=CARTESIAN_POINT ( 'NONE',  ( -5.999999999999998224, -7.500000000000001776, 35.04278698407183867 ) ) ;
#17040=CARTESIAN_POINT ( 'NONE',  ( -10.61538461538473399, -3.300289026999228881, 32.46337939537708905 ) ) ;
#17042=B_SPLINE_CURVE_WITH_KNOTS ( 'NONE', 3,
 ( #36506, #63958, #15350, #76605, #8150, #42826, #8594, #70288, #62630, #35623 ),
 .UNSPECIFIED., .F., .F.,
 ( 4, 2, 2, 2, 4 ),
 ( 0.000000000000000000, 0.0001954311564186867660, 0.0003908623128373735320, 0.0005862934692560603251, 0.0007817246256747470640 ),
 .UNSPECIFIED. ) ;
#17043=EDGE_CURVE ( 'NONE', #78354, #56712, #10371, .T. ) ;
#17044=ORIENTED_EDGE ( 'NONE', *, *, #56551, .F. ) ;
#17045=CARTESIAN_POINT ( 'NONE',  ( 10.86538461538463274, -2.249999999999999112, 29.81603969181029967 ) ) ;
#17046=EDGE_LOOP ( 'NONE', ( #68780, #7916, #76599, #68817 ) ) ;
#17047=B_SPLINE_CURVE_WITH_KNOTS ( 'NONE', 3,
 ( #86344, #71911, #52079, #12005, #60168, #65147, #38580, #5235, #53410, #66035 ),
 .UNSPECIFIED., .F., .F.,
 ( 4, 2, 2, 2, 4 ),
 ( 0.0007817359430256297891, 0.0009771253907249958896, 0.001172514838424361990, 0.001367904286123728091, 0.001563293733823094191 ),
 .UNSPECIFIED. ) ;
#17048=CARTESIAN_POINT ( 'NONE',  ( 9.692307692307572609, -12.27809138561165270, 31.22303859784587132 ) ) ;
#17049=CARTESIAN_POINT ( 'NONE',  ( -8.519285250882628446, -12.43552623307873972, 30.55307653245132826 ) ) ;
#17050=CARTESIAN_POINT ( 'NONE',  ( -1.161602540521988525, -12.64618726649961289, 30.78989965857442712 ) ) ;
#17052=EDGE_LOOP ( 'NONE', ( #36620, #11379, #48144, #22619 ) ) ;
#17053=ORIENTED_EDGE ( 'NONE', *, *, #73902, .T. ) ;
#17054=CARTESIAN_POINT ( 'NONE',  ( 8.900022577055555217, -2.541949514083464479, 30.39797389878540557 ) ) ;
#17056=CARTESIAN_POINT ( 'NONE',  ( 15.23076923076923173, -13.57706302396349152, 30.56769352161908060 ) ) ;
#17058=CARTESIAN_POINT ( 'NONE',  ( -10.83831157429146330, -9.172386477786396597, 34.72672124145550043 ) ) ;
#17059=ORIENTED_EDGE ( 'NONE', *, *, #48961, .F. ) ;
#17060=CARTESIAN_POINT ( 'NONE',  ( -13.45069879557126669, -4.098570777380719399, 33.41473453929634729 ) ) ;
#17062=LINE ( 'NONE', #18848, #20918 ) ;
#17063=FACE_BOUND ( 'NONE', #2621, .T. ) ;
#17064=CARTESIAN_POINT ( 'NONE',  ( 15.00728428704528561, -5.912607949931405926, 34.49155766932282319 ) ) ;
#17065=CARTESIAN_POINT ( 'NONE',  ( 9.915270595869179360, -7.369474270740069777, 34.74850911626239736 ) ) ;
#17066=CARTESIAN_POINT ( 'NONE',  ( 13.31853300525524908, -12.62096338111211580, 30.90682066428152908 ) ) ;
#17067=B_SPLINE_CURVE_WITH_KNOTS ( 'NONE', 3,
 ( #79991, #25043, #80447, #45305, #5660, #5218, #38111, #72336, #79554, #19179 ),
 .UNSPECIFIED., .F., .F.,
 ( 4, 2, 2, 2, 4 ),
 ( 0.0007817246256747483650, 0.0009771112852218926705, 0.001172497944769037084, 0.001367884604316181498, 0.001563271263863325695 ),
 .UNSPECIFIED. ) ;
#17068=CARTESIAN_POINT ( 'NONE',  ( 3.453782074862626228, -3.395485233115138168, 33.02377354290276656 ) ) ;
#17070=CARTESIAN_POINT ( 'NONE',  ( 17.93391762063986761, -6.343179335718451384, 34.87096338111212646 ) ) ;
#17071=CARTESIAN_POINT ( 'NONE',  ( 5.299934428535924447, -2.554770724473668153, 30.48948780036025852 ) ) ;
#17073=CYLINDRICAL_SURFACE ( 'NONE', #11624, 0.2500000000000012212 ) ;
#17074=ORIENTED_EDGE ( 'NONE', *, *, #58271, .F. ) ;
#17075=ORIENTED_EDGE ( 'NONE', *, *, #56121, .F. ) ;
#17076=CARTESIAN_POINT ( 'NONE',  ( -6.792285115252135519, -8.147973898785416225, 34.70805048591653730 ) ) ;
#17077=CARTESIAN_POINT ( 'NONE',  ( -5.934744428723974785, -12.27809138561124591, 31.22303859784720359 ) ) ;
#17078=B_SPLINE_CURVE_WITH_KNOTS ( 'NONE', 3,
 ( #78218, #77339, #57949, #57505, #71906, #15647, #79112, #71457, #43986, #50733 ),
 .UNSPECIFIED., .F., .F.,
 ( 4, 2, 2, 2, 4 ),
 ( 0.000000000000000000, 0.0001954339857564098054, 0.0003908679715128196108, 0.0005863019572692293891, 0.0007817359430256392216 ),
 .UNSPECIFIED. ) ;
#17079=AXIS2_PLACEMENT_3D ( 'NONE', #39180, #31968, #73849 ) ;
#17080=B_SPLINE_CURVE_WITH_KNOTS ( 'NONE', 3,
 ( #62533, #28315, #61653, #849, #6289, #48140, #33752, #26997, #34189, #89159 ),
 .UNSPECIFIED., .F., .F.,
 ( 4, 2, 2, 2, 4 ),
 ( 0.0007817359430256302227, 0.0009771253907249963233, 0.001172514838424362424, 0.001367904286123728524, 0.001563293733823094625 ),
 .UNSPECIFIED. ) ;
#17082=CARTESIAN_POINT ( 'NONE',  ( 15.23076923076910916, -5.094484230521993062, 34.41647553114689373 ) ) ;
#17083=CARTESIAN_POINT ( 'NONE',  ( 14.55763771707034948, -11.56426240980093745, 33.07394671870546432 ) ) ;
#17084=ORIENTED_EDGE ( 'NONE', *, *, #78565, .F. ) ;
#17085=CARTESIAN_POINT ( 'NONE',  ( 18.22277966897806678, -2.612705202774696200, 31.66806509827799943 ) ) ;
#17087=LINE ( 'NONE', #58498, #40229 ) ;
#17088=CARTESIAN_POINT ( 'NONE',  ( -1.608100309179714582, -10.23692288466677880, 34.23039457007281072 ) ) ;
#17089=CARTESIAN_POINT ( 'NONE',  ( 10.61538461538449596, -8.613356846316285953, 34.62446782046622218 ) ) ;
#17090=CARTESIAN_POINT ( 'NONE',  ( -15.23076923076922995, -10.67929555188718282, 33.92786785259544047 ) ) ;
#17092=EDGE_LOOP ( 'NONE', ( #35816, #67688 ) ) ;
#17094=DIRECTION ( 'NONE',  ( -0.000000000000000000, -0.7660444431189791237, -0.6427876096865379196 ) ) ;
#17095=ORIENTED_EDGE ( 'NONE', *, *, #4045, .F. ) ;
#17096=CARTESIAN_POINT ( 'NONE',  ( 17.20771351789003489, -3.957578996910245284, 33.62503395064540257 ) ) ;
#17097=CARTESIAN_POINT ( 'NONE',  ( -12.46153846153858247, -10.21337939537710326, 33.94971097300076224 ) ) ;
#17098=CARTESIAN_POINT ( 'NONE',  ( -16.40382288478850725, -4.943428324936578910, 34.04746400365624481 ) ) ;
#17099=CARTESIAN_POINT ( 'NONE',  ( -15.00798968950081935, -2.847695495035523550, 31.58253572463339154 ) ) ;
#17101=LINE ( 'NONE', #22534, #56066 ) ;
#17103=CARTESIAN_POINT ( 'NONE',  ( 4.023235794221623252, -7.722926236386453702, 34.74524107206102030 ) ) ;
#17104=FACE_OUTER_BOUND ( 'NONE', #77996, .T. ) ;
#17106=CARTESIAN_POINT ( 'NONE',  ( 3.007284306204899060, -12.47654668319379567, 31.42292124445336654 ) ) ;
#17107=CARTESIAN_POINT ( 'NONE',  ( 3.453548772037639658, -2.847695495035523550, 31.58253572463339154 ) ) ;
#17108=DIRECTION ( 'NONE',  ( 0.000000000000000000, 0.4999999999999960032, -0.8660254037844410391 ) ) ;
#17109=CARTESIAN_POINT ( 'NONE',  ( 6.792928953345230170, -3.625366637846544560, 33.29286588640298561 ) ) ;
#17110=CARTESIAN_POINT ( 'NONE',  ( 17.07692307692307665, -4.102666532097928531, 36.13435417666054406 ) ) ;
#17112=CARTESIAN_POINT ( 'NONE',  ( 15.36156103859402222, -11.18335022499818621, 33.13157742990016885 ) ) ;
#17114=VERTEX_POINT ( 'NONE', #6691 ) ;
#17116=CARTESIAN_POINT ( 'NONE',  ( -4.219929564802033184, -4.786620604624113540, 33.94971097300155805 ) ) ;
#17117=CARTESIAN_POINT ( 'NONE',  ( 8.769230769230768274, -11.69971097300155272, 32.46337939537588113 ) ) ;
#17118=CARTESIAN_POINT ( 'NONE',  ( 4.219101293358991533, -11.06231777344671130, 33.60647404775212266 ) ) ;
#17120=CARTESIAN_POINT ( 'NONE',  ( 0.2380535178145108122, -3.754499324213721234, 33.06261337010820256 ) ) ;
#17121=CARTESIAN_POINT ( 'NONE',  ( 8.703148389870632329, -9.905515769479276145, 34.41647553114623292 ) ) ;
#17122=ORIENTED_EDGE ( 'NONE', *, *, #1961, .F. ) ;
#17124=CARTESIAN_POINT ( 'NONE',  ( -1.134560964701931240, -12.41089969410671223, 31.60739465890703670 ) ) ;
#17126=FACE_OUTER_BOUND ( 'NONE', #12853, .T. ) ;
#17127=VERTEX_POINT ( 'NONE', #46349 ) ;
#17128=CARTESIAN_POINT ( 'NONE',  ( 6.250000000001437961, -7.500000000000155431, 34.75000000000007105 ) ) ;
#17129=CARTESIAN_POINT ( 'NONE',  ( -5.776624059301814107, -2.501478030877322567, 29.88021232661720816 ) ) ;
#17130=CARTESIAN_POINT ( 'NONE',  ( -0.3310130233048171333, -6.808710257144159783, 34.95449254468098843 ) ) ;
#17133=ORIENTED_EDGE ( 'NONE', *, *, #36151, .F. ) ;
#17134=CARTESIAN_POINT ( 'NONE',  ( -0.4615384615384611200, -3.669653830205710676, 35.88435417666054406 ) ) ;
#17135=EDGE_CURVE ( 'NONE', #14030, #75330, #75164, .T. ) ;
#17136=ORIENTED_EDGE ( 'NONE', *, *, #53932, .F. ) ;
#17138=CARTESIAN_POINT ( 'NONE',  ( -15.23076923076922995, -9.819645486525091727, 36.12317359536749706 ) ) ;
#17139=CARTESIAN_POINT ( 'NONE',  ( 12.68431800280686872, -12.24180327182771855, 31.33663988360758879 ) ) ;
#17140=ORIENTED_EDGE ( 'NONE', *, *, #47661, .F. ) ;
#17141=ADVANCED_FACE ( 'NONE', ( #26974 ), #12134, .F. ) ;
#17142=CARTESIAN_POINT ( 'NONE',  ( -6.250023224221457951, -10.92453946501458439, 33.72985991061850086 ) ) ;
#17143=FACE_OUTER_BOUND ( 'NONE', #57586, .T. ) ;
#17144=LINE ( 'NONE', #43729, #59561 ) ;
#17145=AXIS2_PLACEMENT_3D ( 'NONE', #55277, #344, #82765 ) ;
#17146=B_SPLINE_CURVE_WITH_KNOTS ( 'NONE', 3,
 ( #83184, #2078, #77297, #43072, #318, #42200, #15604, #70545, #7962, #27783 ),
 .UNSPECIFIED., .F., .F.,
 ( 4, 2, 2, 2, 4 ),
 ( 0.000000000000000000, 0.0001954339857564126514, 0.0003908679715128183098, 0.0005863019572692239681, 0.0007817359430256294638 ),
 .UNSPECIFIED. ) ;
#17147=CARTESIAN_POINT ( 'NONE',  ( -14.08467946359890988, -10.01129605718032600, 34.36064277460058491 ) ) ;
#17148=CARTESIAN_POINT ( 'NONE',  ( -16.15384615384627409, -3.083524468854526912, 32.58852847137268327 ) ) ;
#17151=EDGE_CURVE ( 'NONE', #41676, #76909, #79104, .T. ) ;
#17152=EDGE_LOOP ( 'NONE', ( #26026, #31393 ) ) ;
#17153=DIRECTION ( 'NONE',  ( -0.000000000000000000, 0.5000000000000011102, -0.8660254037844381525 ) ) ;
#17154=ORIENTED_EDGE ( 'NONE', *, *, #5663, .F. ) ;
#17155=CARTESIAN_POINT ( 'NONE',  ( 10.61538461538461675, -4.786620604624113540, 33.94971097300155094 ) ) ;
#17156=CARTESIAN_POINT ( 'NONE',  ( 5.999999999999878320, -10.33852847137269571, 34.16647553114546554 ) ) ;
#17157=VERTEX_POINT ( 'NONE', #46795 ) ;
#17158=ORIENTED_EDGE ( 'NONE', *, *, #34466, .F. ) ;
#17160=CARTESIAN_POINT ( 'NONE',  ( -1.607541602131531189, -11.76352882383564769, 32.36236540154569497 ) ) ;
#17161=ORIENTED_EDGE ( 'NONE', *, *, #64682, .T. ) ;
#17162=CARTESIAN_POINT ( 'NONE',  ( 16.08857570788537572, -10.21337939537584383, 33.94971097300158647 ) ) ;
#17163=EDGE_CURVE ( 'NONE', #36033, #72869, #75929, .T. ) ;
#17164=CARTESIAN_POINT ( 'NONE',  ( 16.82694633287449193, -12.41104346484419452, 31.60698883733904196 ) ) ;
#17166=AXIS2_PLACEMENT_3D ( 'NONE', #78785, #10336, #65267 ) ;
#17167=CARTESIAN_POINT ( 'NONE',  ( 12.21156173059610772, -2.564618984488975517, 30.55390908950641915 ) ) ;
#17168=FACE_BOUND ( 'NONE', #33765, .T. ) ;
#17169=EDGE_CURVE ( 'NONE', #41455, #27570, #54883, .T. ) ;
#17171=B_SPLINE_CURVE_WITH_KNOTS ( 'NONE', 3,
 ( #3626, #23017, #50477, #77962, #84298, #64877, #3183, #16263, #57690, #17605 ),
 .UNSPECIFIED., .F., .F.,
 ( 4, 2, 2, 2, 4 ),
 ( 0.000000000000000000, 0.0001954339857564074473, 0.0003908679715128148945, 0.0005863019572692223418, 0.0007817359430256297891 ),
 .UNSPECIFIED. ) ;
#17172=CARTESIAN_POINT ( 'NONE',  ( -1.634615384615383027, -7.433931650972300353, 34.75000000000000711 ) ) ;
#17173=EDGE_CURVE ( 'NONE', #42667, #82873, #48001, .T. ) ;
#17174=DIRECTION ( 'NONE',  ( 0.000000000000000000, 0.9396926207859126468, -0.3420201433256571111 ) ) ;
#17175=FACE_OUTER_BOUND ( 'NONE', #38109, .T. ) ;
#17176=CARTESIAN_POINT ( 'NONE',  ( -1.608100328339331586, -2.599994579823203367, 30.74605699353653776 ) ) ;
#17177=VERTEX_POINT ( 'NONE', #35496 ) ;
#17178=CARTESIAN_POINT ( 'NONE',  ( -5.076923076923199218, -2.379036618888197729, 30.90682066428292885 ) ) ;
#17179=ORIENTED_EDGE ( 'NONE', *, *, #57485, .T. ) ;
#17180=ORIENTED_EDGE ( 'NONE', *, *, #43740, .T. ) ;
#17181=CARTESIAN_POINT ( 'NONE',  ( 5.777073041093152561, -11.98009711892699691, 32.48740034544075428 ) ) ;
#17182=CARTESIAN_POINT ( 'NONE',  ( -1.450697763975519416, -5.471508081941601986, 34.59228464037088457 ) ) ;
#17183=DIRECTION ( 'NONE',  ( 0.000000000000000000, 0.9396926207859126468, -0.3420201433256571111 ) ) ;
#17184=CARTESIAN_POINT ( 'NONE',  ( -13.44988538517170795, -3.083524468853724443, 32.58852847137143272 ) ) ;
#17185=CARTESIAN_POINT ( 'NONE',  ( 7.596177115211490971, -12.41269422305637171, 30.68257228309993323 ) ) ;
#17186=CARTESIAN_POINT ( 'NONE',  ( -12.23875892027004753, -4.387253974876679230, 33.66317474335728832 ) ) ;
#17187=ORIENTED_EDGE ( 'NONE', *, *, #26214, .F. ) ;
#17188=CYLINDRICAL_SURFACE ( 'NONE', #40021, 0.2499999999999998890 ) ;
#17189=CARTESIAN_POINT ( 'NONE',  ( 0.4615384615383382183, -9.528491918059723176, 34.59228464037033035 ) ) ;
#17190=CARTESIAN_POINT ( 'NONE',  ( -1.515306851282945511, -3.530157926970578508, 32.79014554554150607 ) ) ;
#17191=CARTESIAN_POINT ( 'NONE',  ( 13.31934493865461278, -12.46129190929999986, 30.37095296980880832 ) ) ;
#17192=ORIENTED_EDGE ( 'NONE', *, *, #51259, .F. ) ;
#17193=B_SPLINE_CURVE_WITH_KNOTS ( 'NONE', 3,
 ( #5057, #60438, #6824, #59996, #75724, #41065, #87495, #87955, #67651, #40630 ),
 .UNSPECIFIED., .F., .F.,
 ( 4, 2, 2, 2, 4 ),
 ( 0.0007817246256747484735, 0.0009771112852218931041, 0.001172497944769037735, 0.001367884604316182365, 0.001563271263863326996 ),
 .UNSPECIFIED. ) ;
#17195=FACE_BOUND ( 'NONE', #77332, .T. ) ;
#17196=AXIS2_PLACEMENT_3D ( 'NONE', #66156, #4462, #31946 ) ;
#17197=ORIENTED_EDGE ( 'NONE', *, *, #12041, .T. ) ;
#17198=CARTESIAN_POINT ( 'NONE',  ( -6.000000000000121680, -5.094484230521993062, 34.41647553114689373 ) ) ;
#17199=CARTESIAN_POINT ( 'NONE',  ( -1.253824943648435442, -2.295524264805589354, 30.44142389570982488 ) ) ;
#17200=VERTEX_POINT ( 'NONE', #41371 ) ;
#17201=CARTESIAN_POINT ( 'NONE',  ( -3.480792468062195333, -12.43535235679832596, 30.55408501211184813 ) ) ;
#17202=CARTESIAN_POINT ( 'NONE',  ( -10.61538461538473399, -6.879047030192662504, 34.71129190930017927 ) ) ;
#17203=CARTESIAN_POINT ( 'NONE',  ( 14.30769230769231015, -11.69971097300155272, 32.46337939537588113 ) ) ;
#17204=CYLINDRICAL_SURFACE ( 'NONE', #53193, 0.2499999999999995559 ) ;
#17205=EDGE_LOOP ( 'NONE', ( #21140, #33171 ) ) ;
#17206=VECTOR ( 'NONE', #59928, 1000.000000000000000 ) ;
#17207=CARTESIAN_POINT ( 'NONE',  ( -7.846153846153844924, -10.51840700105979565, 33.73612834413961536 ) ) ;
#17209=VECTOR ( 'NONE', #41615, 1000.000000000000000 ) ;
#17210=CARTESIAN_POINT ( 'NONE',  ( 13.38461538461526423, -8.656820664282941280, 34.87096338111179961 ) ) ;
#17211=ORIENTED_EDGE ( 'NONE', *, *, #56345, .T. ) ;
#17212=DIRECTION ( 'NONE',  ( -0.000000000000000000, -0.1736481776669307198, -0.9848077530122080203 ) ) ;
#17213=FACE_OUTER_BOUND ( 'NONE', #75434, .T. ) ;
#17214=LINE ( 'NONE', #10469, #63102 ) ;
#17215=ADVANCED_FACE ( 'NONE', ( #35946 ), #22420, .F. ) ;
#17216=CARTESIAN_POINT ( 'NONE',  ( 15.45378058238208396, -12.39991518177334129, 30.74647679643404530 ) ) ;
#17217=CARTESIAN_POINT ( 'NONE',  ( -14.55766905174089842, -8.347322224742351082, 34.93158281831414058 ) ) ;
#17218=CARTESIAN_POINT ( 'NONE',  ( 5.076923076923075762, -12.37446782046654192, 30.86335684631486131 ) ) ;
#17219=B_SPLINE_CURVE_WITH_KNOTS ( 'NONE', 3,
 ( #31843, #24177, #17434, #9783, #51629, #65601, #72366, #3902, #31388, #85448 ),
 .UNSPECIFIED., .F., .F.,
 ( 4, 2, 2, 2, 4 ),
 ( 0.0007817246256747453293, 0.0009771112852218881168, 0.001172497944769030796, 0.001367884604316173475, 0.001563271263863316154 ),
 .UNSPECIFIED. ) ;
#17221=EDGE_LOOP ( 'NONE', ( #64897, #3236, #77100, #67826 ) ) ;
#17222=B_SPLINE_CURVE_WITH_KNOTS ( 'NONE', 3,
 ( #35964, #63420, #55335, #14352, #70628, #62965, #48132, #1727, #29216, #22439 ),
 .UNSPECIFIED., .F., .F.,
 ( 4, 2, 2, 2, 4 ),
 ( 0.000000000000000000, 0.0001954311564186860613, 0.0003908623128373721225, 0.0005862934692560581567, 0.0007817246256747442451 ),
 .UNSPECIFIED. ) ;
#17224=FACE_OUTER_BOUND ( 'NONE', #62307, .T. ) ;
#17226=VERTEX_POINT ( 'NONE', #68835 ) ;
#17227=ORIENTED_EDGE ( 'NONE', *, *, #105, .T. ) ;
#17228=DIRECTION ( 'NONE',  ( 0.000000000000000000, 0.1736481776669275834, 0.9848077530122086864 ) ) ;
#17230=CARTESIAN_POINT ( 'NONE',  ( 2.980745993476265898, -10.05641848906368097, 34.04755513067966177 ) ) ;
#17231=EDGE_CURVE ( 'NONE', #68982, #36238, #63401, .T. ) ;
#17232=CARTESIAN_POINT ( 'NONE',  ( 9.692307692307572609, -12.46129190930018460, 30.37095296980731973 ) ) ;
#17233=CARTESIAN_POINT ( 'NONE',  ( 10.36536137809165403, -4.335965774309649134, 33.62209801155881905 ) ) ;
#17234=CARTESIAN_POINT ( 'NONE',  ( -16.82686865700962642, -11.47946981652013498, 33.17500667209846910 ) ) ;
#17235=DIRECTION ( 'NONE',  ( -0.000000000000000000, 0.5000000000000011102, -0.8660254037844381525 ) ) ;
#17236=VERTEX_POINT ( 'NONE', #55757 ) ;
#17237=CARTESIAN_POINT ( 'NONE',  ( 3.100077764101673683, -6.413092428213692742, 34.63065189839063152 ) ) ;
#17238=CARTESIAN_POINT ( 'NONE',  ( -16.85349611506149969, -7.630147231320743018, 34.74852402298682819 ) ) ;
#17239=CARTESIAN_POINT ( 'NONE',  ( 4.403846153846090239, -7.565270000091922853, 34.99999999999999289 ) ) ;
#17240=CARTESIAN_POINT ( 'NONE',  ( 7.846153846153846700, -3.886160181151819604, 36.00935417666054406 ) ) ;
#17241=ORIENTED_EDGE ( 'NONE', *, *, #57086, .F. ) ;
#17242=CARTESIAN_POINT ( 'NONE',  ( -7.715628144390278997, -3.816742781228458448, 33.13167719472716044 ) ) ;
#17243=EDGE_CURVE ( 'NONE', #40454, #74101, #44623, .T. ) ;
#17244=ORIENTED_EDGE ( 'NONE', *, *, #22877, .T. ) ;
#17245=CARTESIAN_POINT ( 'NONE',  ( -0.4615384615385826339, -2.892918686052166066, 31.69288490824153470 ) ) ;
#17246=DIRECTION ( 'NONE',  ( -1.000000000000000000, 0.000000000000000000, 0.000000000000000000 ) ) ;
#17247=CARTESIAN_POINT ( 'NONE',  ( -2.176853889679542853, -7.277220443632450575, 34.74524770363009196 ) ) ;
#17248=VERTEX_POINT ( 'NONE', #21534 ) ;
#17249=EDGE_CURVE ( 'NONE', #69237, #1870, #88713, .T. ) ;
#17250=CYLINDRICAL_SURFACE ( 'NONE', #6092, 0.2500000000000009437 ) ;
#17251=LINE ( 'NONE', #51912, #58073 ) ;
#17252=CYLINDRICAL_SURFACE ( 'NONE', #14955, 0.2500000000000004996 ) ;
#17253=CARTESIAN_POINT ( 'NONE',  ( 7.846153846153846700, -9.058645607665452459, 34.76329471203371924 ) ) ;
#17256=ADVANCED_FACE ( 'NONE', ( #21081 ), #77365, .F. ) ;
#17257=CARTESIAN_POINT ( 'NONE',  ( -1.134669866267241423, -3.712312575010499938, 33.01462480002815170 ) ) ;
#17259=LINE ( 'NONE', #35879, #77398 ) ;
#17260=CARTESIAN_POINT ( 'NONE',  ( 5.076923076922954969, -12.27809138561165270, 31.22303859784587132 ) ) ;
#17261=AXIS2_PLACEMENT_3D ( 'NONE', #49183, #53166, #64901 ) ;
#17262=EDGE_CURVE ( 'NONE', #60982, #47138, #36385, .T. ) ;
#17263=CARTESIAN_POINT ( 'NONE',  ( -16.37733109757011007, -11.41268669641499756, 32.86336882939238535 ) ) ;
#17264=CARTESIAN_POINT ( 'NONE',  ( 8.769230769230647482, -2.892918686052165622, 31.69288490824153470 ) ) ;
#17266=DIRECTION ( 'NONE',  ( 0.000000000000000000, 0.000000000000000000, 1.000000000000000000 ) ) ;
#17267=CARTESIAN_POINT ( 'NONE',  ( 12.71148397988660150, -10.05730279482229683, 34.04704008940765902 ) ) ;
#17268=AXIS2_PLACEMENT_3D ( 'NONE', #30522, #78714, #79159 ) ;
#17269=AXIS2_PLACEMENT_3D ( 'NONE', #26381, #75893, #67810 ) ;
#17270=ORIENTED_EDGE ( 'NONE', *, *, #61896, .T. ) ;
#17271=ORIENTED_EDGE ( 'NONE', *, *, #71855, .T. ) ;
#17273=ORIENTED_EDGE ( 'NONE', *, *, #49450, .F. ) ;
#17274=ORIENTED_EDGE ( 'NONE', *, *, #15856, .T. ) ;
#17275=ORIENTED_EDGE ( 'NONE', *, *, #39736, .T. ) ;
#17277=CARTESIAN_POINT ( 'NONE',  ( -12.71153846153846168, -2.249999999999998668, 29.75000000000000355 ) ) ;
#17278=CARTESIAN_POINT ( 'NONE',  ( -11.76194648218548622, -9.331801661448606566, 34.40259984581193464 ) ) ;
#17279=CARTESIAN_POINT ( 'NONE',  ( -5.326923076923075762, -7.433931650972300353, 34.75000000000000711 ) ) ;
#17280=CARTESIAN_POINT ( 'NONE',  ( -0.4615384615385826339, -6.879047030192662504, 34.71129190930017927 ) ) ;
#17281=CARTESIAN_POINT ( 'NONE',  ( -16.40382288478850725, -2.564618984488975517, 30.55390908950641915 ) ) ;
#17282=CARTESIAN_POINT ( 'NONE',  ( 3.230769230769110045, -6.026961402154118908, 34.52809138561165270 ) ) ;
#17283=EDGE_CURVE ( 'NONE', #69537, #32856, #36050, .T. ) ;
#17284=CARTESIAN_POINT ( 'NONE',  ( 5.934729554039226862, -11.94971097300153140, 32.03036669348370680 ) ) ;
#17285=EDGE_CURVE ( 'NONE', #6434, #58891, #64276, .T. ) ;
#17286=CARTESIAN_POINT ( 'NONE',  ( 6.923076923076924238, -11.69971097300155272, 32.46337939537588113 ) ) ;
#17287=DIRECTION ( 'NONE',  ( 0.000000000000000000, 0.7660444431189822323, -0.6427876096865344779 ) ) ;
#17288=ORIENTED_EDGE ( 'NONE', *, *, #79170, .F. ) ;
#17289=ORIENTED_EDGE ( 'NONE', *, *, #68792, .F. ) ;
#17290=ORIENTED_EDGE ( 'NONE', *, *, #45402, .T. ) ;
#17291=DIRECTION ( 'NONE',  ( 0.000000000000000000, 0.4999999999999960032, -0.8660254037844410391 ) ) ;
#17292=ORIENTED_EDGE ( 'NONE', *, *, #84190, .T. ) ;
#17293=FACE_OUTER_BOUND ( 'NONE', #80068, .T. ) ;
#17295=B_SPLINE_CURVE_WITH_KNOTS ( 'NONE', 3,
 ( #19110, #26305, #65944, #86698, #6044, #24965, #74058, #11459, #81259, #80825 ),
 .UNSPECIFIED., .F., .F.,
 ( 4, 2, 2, 2, 4 ),
 ( 0.0007817359430256315238, 0.0009771253907249980580, 0.001172514838424364592, 0.001367904286123731127, 0.001563293733823097661 ),
 .UNSPECIFIED. ) ;
#17296=CARTESIAN_POINT ( 'NONE',  ( -1.319422396320729440, -2.255955759149235629, 29.99999999999988631 ) ) ;
#17297=CARTESIAN_POINT ( 'NONE',  ( 6.923076923076924238, -2.538708090699994813, 30.37095296980875503 ) ) ;
#17298=ORIENTED_EDGE ( 'NONE', *, *, #85975, .T. ) ;
#17299=VECTOR ( 'NONE', #36080, 1000.000000000000000 ) ;
#17300=ORIENTED_EDGE ( 'NONE', *, *, #37296, .T. ) ;
#17301=CARTESIAN_POINT ( 'NONE',  ( -11.66915214157184089, -11.93127051446799847, 32.56575433478202797 ) ) ;
#17302=ORIENTED_EDGE ( 'NONE', *, *, #27895, .F. ) ;
#17303=FACE_BOUND ( 'NONE', #70231, .T. ) ;
#17304=CARTESIAN_POINT ( 'NONE',  ( 3.361294669002873547, -2.647132371071621471, 31.75357179365173010 ) ) ;
#17305=CARTESIAN_POINT ( 'NONE',  ( 11.53846153846153832, -9.584722331328613620, 36.20867863119891439 ) ) ;
#17306=VERTEX_POINT ( 'NONE', #17887 ) ;
#17307=ADVANCED_FACE ( 'NONE', ( #71931 ), #2575, .F. ) ;
#17308=CARTESIAN_POINT ( 'NONE',  ( 14.17700084102475699, -2.729777683071817229, 31.24903638046269450 ) ) ;
#17309=CARTESIAN_POINT ( 'NONE',  ( 8.703477340917435967, -7.249945578846651806, 34.99404164642496795 ) ) ;
#17310=CARTESIAN_POINT ( 'NONE',  ( -5.076923076923197442, -3.835265460704628371, 33.15142922262033665 ) ) ;
#17311=ORIENTED_EDGE ( 'NONE', *, *, #33265, .F. ) ;
#17312=DIRECTION ( 'NONE',  ( -1.000000000000000000, 0.000000000000000000, 0.000000000000000000 ) ) ;
#17313=CARTESIAN_POINT ( 'NONE',  ( -14.55771554498526932, -5.851115903089112003, 34.47074536777953568 ) ) ;
#17314=ORIENTED_EDGE ( 'NONE', *, *, #57195, .F. ) ;
#17315=CARTESIAN_POINT ( 'NONE',  ( 5.869524814924282907, -7.276987145209185215, 34.99546412871779211 ) ) ;
#17316=CARTESIAN_POINT ( 'NONE',  ( 3.230769230769231726, -13.78497067705608181, 32.30358669280327177 ) ) ;
#17317=VERTEX_POINT ( 'NONE', #37702 ) ;
#17318=DIRECTION ( 'NONE',  ( -0.000000000000000000, 0.1736481776669307198, -0.9848077530122080203 ) ) ;
#17319=CARTESIAN_POINT ( 'NONE',  ( 14.43848411551709177, -8.147973898785416225, 34.70805048591653730 ) ) ;
#17320=FACE_OUTER_BOUND ( 'NONE', #37785, .T. ) ;
#17321=DIRECTION ( 'NONE',  ( -0.000000000000000000, 0.5000000000000011102, -0.8660254037844380415 ) ) ;
#17322=DIRECTION ( 'NONE',  ( 0.000000000000000000, 0.7660444431189822323, -0.6427876096865344779 ) ) ;
#17323=ADVANCED_FACE ( 'NONE', ( #65166 ), #78242, .F. ) ;
#17324=DIRECTION ( 'NONE',  ( 0.000000000000000000, 0.000000000000000000, -1.000000000000000000 ) ) ;
#17325=CARTESIAN_POINT ( 'NONE',  ( -9.692307692307691624, -5.471508081941601098, 34.59228464037088457 ) ) ;
#17326=CARTESIAN_POINT ( 'NONE',  ( 7.053868730901709405, -3.062576670634119758, 32.05464942895959979 ) ) ;
#17328=CARTESIAN_POINT ( 'NONE',  ( -1.384615384615383471, -9.058645607665452459, 34.76329471203371924 ) ) ;
#17329=CARTESIAN_POINT ( 'NONE',  ( 12.52668324225809293, -7.750023224968867197, 34.99404313364389907 ) ) ;
#17330=CARTESIAN_POINT ( 'NONE',  ( -8.519230769230754063, -2.249999999999998224, 29.81603969181031033 ) ) ;
#17332=ORIENTED_EDGE ( 'NONE', *, *, #12023, .T. ) ;
#17334=CARTESIAN_POINT ( 'NONE',  ( 0.2380535178145127273, -12.44517049084099725, 30.48991314939691932 ) ) ;
#17335=ORIENTED_EDGE ( 'NONE', *, *, #58338, .T. ) ;
#17336=EDGE_CURVE ( 'NONE', #23503, #31091, #16544, .T. ) ;
#17338=CARTESIAN_POINT ( 'NONE',  ( 16.02315468717859659, -11.18331474514187995, 33.13161551792790505 ) ) ;
#17339=VERTEX_POINT ( 'NONE', #3467 ) ;
#17340=CARTESIAN_POINT ( 'NONE',  ( -15.16470087976679437, -5.557115091759786019, 34.35708131394839882 ) ) ;
#17342=CARTESIAN_POINT ( 'NONE',  ( -18.00000000000012079, -6.026961402154117131, 34.52809138561165270 ) ) ;
#17343=CARTESIAN_POINT ( 'NONE',  ( -4.946397375159514276, -2.882268652242224505, 31.66798894389554064 ) ) ;
#17345=CARTESIAN_POINT ( 'NONE',  ( -6.130147969731699398, -2.647304123082328875, 31.75400227202885262 ) ) ;
#17346=VECTOR ( 'NONE', #50295, 1000.000000000000114 ) ;
#17347=EDGE_CURVE ( 'NONE', #34740, #15372, #67145, .T. ) ;
#17348=CARTESIAN_POINT ( 'NONE',  ( -8.703975197954745724, -5.219633306516380244, 34.19971097300157936 ) ) ;
#17349=DIRECTION ( 'NONE',  ( -0.000000000000000000, 0.6427876096865404731, -0.7660444431189770143 ) ) ;
#17350=CARTESIAN_POINT ( 'NONE',  ( -7.596099534515532881, -12.17597550085003633, 31.52189283813461884 ) ) ;
#17353=CARTESIAN_POINT ( 'NONE',  ( 18.22277966897806678, -11.60474049983370648, 33.02348890104160262 ) ) ;
#17354=CARTESIAN_POINT ( 'NONE',  ( -2.057746898314263717, -12.07971442181321997, 32.31769673815850297 ) ) ;
#17355=CARTESIAN_POINT ( 'NONE',  ( 11.53846153846153832, -12.62096338111211580, 30.90682066428153263 ) ) ;
#17356=B_SPLINE_CURVE_WITH_KNOTS ( 'NONE', 3,
 ( #26690, #41096, #54148, #55048, #48728, #81644, #28020, #19929, #34327, #68129 ),
 .UNSPECIFIED., .F., .F.,
 ( 4, 2, 2, 2, 4 ),
 ( 0.000000000000000000, 0.0001954339857564098054, 0.0003908679715128196108, 0.0005863019572692293891, 0.0007817359430256392216 ),
 .UNSPECIFIED. ) ;
#17361=CARTESIAN_POINT ( 'NONE',  ( -2.557715531913763218, -2.341070481393819236, 30.72580821765574299 ) ) ;
#17362=DIRECTION ( 'NONE',  ( -0.000000000000000000, -0.9396926207859092051, -0.3420201433256662704 ) ) ;
#17363=ADVANCED_FACE ( 'NONE', ( #9789 ), #85899, .F. ) ;
#17364=CARTESIAN_POINT ( 'NONE',  ( 10.61538461538449418, -12.70778746994576025, 30.41441678777401236 ) ) ;
#17365=CARTESIAN_POINT ( 'NONE',  ( -3.007756386675835003, -5.582272713120728369, 34.63742843783360570 ) ) ;
#17366=EDGE_CURVE ( 'NONE', #32906, #74101, #24184, .T. ) ;
#17367=ORIENTED_EDGE ( 'NONE', *, *, #36758, .T. ) ;
#17368=DIRECTION ( 'NONE',  ( 0.000000000000000000, 0.4999999999999960032, -0.8660254037844410391 ) ) ;
#17370=AXIS2_PLACEMENT_3D ( 'NONE', #63321, #42181, #22339 ) ;
#17371=B_SPLINE_CURVE_WITH_KNOTS ( 'NONE', 3,
 ( #42067, #22662, #21782, #629, #35295, #64082, #7829, #42948, #49256, #63646 ),
 .UNSPECIFIED., .F., .F.,
 ( 4, 2, 2, 2, 4 ),
 ( 0.0007817246256747473893, 0.0009771112852218909357, 0.001172497944769034482, 0.001367884604316178246, 0.001563271263863321792 ),
 .UNSPECIFIED. ) ;
#17372=ORIENTED_EDGE ( 'NONE', *, *, #85591, .F. ) ;
#17373=CARTESIAN_POINT ( 'NONE',  ( 0.5276057948885374271, -12.34228464037088813, 31.77849191805839268 ) ) ;
#17374=CARTESIAN_POINT ( 'NONE',  ( -11.53846153846166089, -11.67786785259630911, 32.92929555188603530 ) ) ;
#17375=CARTESIAN_POINT ( 'NONE',  ( 14.30769230769218758, -10.90142922262034020, 33.41473453929536674 ) ) ;
#17376=CARTESIAN_POINT ( 'NONE',  ( 2.084207363968360927, -5.912607949931405038, 34.49155766932282319 ) ) ;
#17377=CARTESIAN_POINT ( 'NONE',  ( -13.31935981333936070, -3.300289026998473041, 32.46337939537591666 ) ) ;
#17378=ORIENTED_EDGE ( 'NONE', *, *, #58312, .T. ) ;
#17379=ORIENTED_EDGE ( 'NONE', *, *, #75404, .T. ) ;
#17380=ORIENTED_EDGE ( 'NONE', *, *, #30220, .F. ) ;
#17381=ADVANCED_FACE ( 'NONE', ( #85017 ), #72371, .F. ) ;
#17382=ADVANCED_FACE ( 'NONE', ( #23299 ), #11122, .F. ) ;
#17384=CARTESIAN_POINT ( 'NONE',  ( 13.13463864056679498, -4.818429247618089661, 34.26397095200675125 ) ) ;
#17385=DIRECTION ( 'NONE',  ( -0.000000000000000000, -0.5000000000000009992, -0.8660254037844380415 ) ) ;
#17386=DIRECTION ( 'NONE',  ( -0.000000000000000000, -0.6427876096865404731, -0.7660444431189770143 ) ) ;
#17387=EDGE_CURVE ( 'NONE', #2854, #19448, #21030, .T. ) ;
#17390=CARTESIAN_POINT ( 'NONE',  ( 1.161689167099237974, -3.586966769969700763, 32.86292498521069660 ) ) ;
#17391=CARTESIAN_POINT ( 'NONE',  ( -2.307692307692305711, -3.886160181151819604, 36.00935417666054406 ) ) ;
#17392=ADVANCED_FACE ( 'NONE', ( #74161 ), #80027, .F. ) ;
#17393=CARTESIAN_POINT ( 'NONE',  ( 17.07692307692307665, -2.708943851104267164, 35.45975837776705220 ) ) ;
#17394=ORIENTED_EDGE ( 'NONE', *, *, #22436, .T. ) ;
#17395=VERTEX_POINT ( 'NONE', #32290 ) ;
#17398=EDGE_LOOP ( 'NONE', ( #18099, #35253, #55555, #82309 ) ) ;
#17399=CARTESIAN_POINT ( 'NONE',  ( -13.51530598772569469, -5.496505350115501010, 34.60290016733514307 ) ) ;
#17402=AXIS2_PLACEMENT_3D ( 'NONE', #53805, #55135, #33548 ) ;
#17403=CARTESIAN_POINT ( 'NONE',  ( -9.692307692307691624, -9.905515769479276145, 34.41647553114623292 ) ) ;
#17404=CARTESIAN_POINT ( 'NONE',  ( -9.915792636031639518, -11.89387501736622710, 32.13663884655806413 ) ) ;
#17406=ORIENTED_EDGE ( 'NONE', *, *, #85504, .F. ) ;
#17407=EDGE_CURVE ( 'NONE', #24055, #72513, #4702, .T. ) ;
#17408=CARTESIAN_POINT ( 'NONE',  ( -13.44988583057615728, -12.27809138561121394, 31.22303859784730307 ) ) ;
#17409=VERTEX_POINT ( 'NONE', #25529 ) ;
#17411=CARTESIAN_POINT ( 'NONE',  ( 4.153846153846154188, -9.058645607665452459, 34.76329471203371924 ) ) ;
#17412=CARTESIAN_POINT ( 'NONE',  ( -15.09997878980228059, -2.845873456487965747, 32.17976146951972538 ) ) ;
#17413=CARTESIAN_POINT ( 'NONE',  ( 11.53846153846153832, -11.33034616979429110, 35.88435417666054406 ) ) ;
#17414=CARTESIAN_POINT ( 'NONE',  ( 4.946775867484856093, -3.285722584762969856, 32.44110544564090759 ) ) ;
#17415=CARTESIAN_POINT ( 'NONE',  ( 5.011652630962300847, -2.625532179533445198, 30.86335684631481513 ) ) ;
#17418=EDGE_CURVE ( 'NONE', #58891, #27959, #60768, .T. ) ;
#17419=CARTESIAN_POINT ( 'NONE',  ( -11.53846153846153655, -12.10708131394839349, 31.69288490824020244 ) ) ;
#17420=CARTESIAN_POINT ( 'NONE',  ( -8.769230769230892619, -4.320704448113951379, 33.92786785259630022 ) ) ;
#17421=EDGE_LOOP ( 'NONE', ( #51948, #51742 ) ) ;
#17422=CARTESIAN_POINT ( 'NONE',  ( -12.23875879256039489, -3.563462043263030399, 33.22394488606062879 ) ) ;
#17424=CARTESIAN_POINT ( 'NONE',  ( 10.61538461538461675, -6.386643153685126251, 34.62446782046654192 ) ) ;
#17425=CARTESIAN_POINT ( 'NONE',  ( -6.130691466667555822, -10.54014554554150607, 33.71984207302941883 ) ) ;
#17426=B_SPLINE_CURVE_WITH_KNOTS ( 'NONE', 3,
 ( #24852, #59974, #52322, #53214, #39723, #66286, #19878, #79814, #67186, #73048 ),
 .UNSPECIFIED., .F., .F.,
 ( 4, 2, 2, 2, 4 ),
 ( 0.0007817359430256360774, 0.0009771253907250039127, 0.001172514838424371965, 0.001367904286123739800, 0.001563293733823107635 ),
 .UNSPECIFIED. ) ;
#17428=CARTESIAN_POINT ( 'NONE',  ( 12.46153846153833911, -4.481592998941358097, 33.73612834414048933 ) ) ;
#17429=FACE_BOUND ( 'NONE', #21292, .T. ) ;
#17430=CARTESIAN_POINT ( 'NONE',  ( 13.16168842570853492, -2.308479472611653094, 30.53278059502174457 ) ) ;
#17431=CARTESIAN_POINT ( 'NONE',  ( -10.86538461538461320, -7.500000000000001776, 35.00000000000000000 ) ) ;
#17432=CARTESIAN_POINT ( 'NONE',  ( 0.4615384615383382183, -12.70778746994576025, 30.41441678777401236 ) ) ;
#17433=CARTESIAN_POINT ( 'NONE',  ( -11.47331575912957469, -7.750023238201979581, 34.74374492549440419 ) ) ;
#17434=CARTESIAN_POINT ( 'NONE',  ( 0.5920638997721023866, -3.068774925481847937, 32.56582465632704526 ) ) ;
#17435=CARTESIAN_POINT ( 'NONE',  ( -17.07692307692307665, -1.951392089020283160, 34.73218667398347748 ) ) ;
#17439=EDGE_CURVE ( 'NONE', #23926, #64222, #55337, .T. ) ;
#17440=ORIENTED_EDGE ( 'NONE', *, *, #75629, .F. ) ;
#17441=DIRECTION ( 'NONE',  ( 0.000000000000000000, 0.7660444431189822323, -0.6427876096865344779 ) ) ;
#17442=CARTESIAN_POINT ( 'NONE',  ( 7.846153846153723244, -10.33852847137269571, 34.16647553114546554 ) ) ;
#17443=CARTESIAN_POINT ( 'NONE',  ( -7.846153846153967493, -11.67786785259630911, 32.92929555188603530 ) ) ;
#17444=LINE ( 'NONE', #64279, #85568 ) ;
#17446=CARTESIAN_POINT ( 'NONE',  ( -16.85391023282967637, -8.282913670948747864, 34.94150082978203642 ) ) ;
#17448=DIRECTION ( 'NONE',  ( 0.000000000000000000, 0.9396926207859126468, 0.3420201433256571111 ) ) ;
#17449=CARTESIAN_POINT ( 'NONE',  ( -2.307692307692305711, -6.343179335718451384, 34.87096338111211935 ) ) ;
#17450=ADVANCED_FACE ( 'NONE', ( #20103 ), #73734, .F. ) ;
#17451=CARTESIAN_POINT ( 'NONE',  ( -8.096130590202436750, -2.920706130388546651, 32.31842814019191223 ) ) ;
#17452=CARTESIAN_POINT ( 'NONE',  ( 9.627037691751372250, -4.320704448112771878, 33.92786785259540494 ) ) ;
#17453=CARTESIAN_POINT ( 'NONE',  ( 7.146088274689773812, -4.187068189119697692, 33.49521262558774026 ) ) ;
#17454=CARTESIAN_POINT ( 'NONE',  ( 5.299935921016470708, -8.282913670948747864, 34.94150082978203642 ) ) ;
#17457=CARTESIAN_POINT ( 'NONE',  ( 14.05766907039934210, -6.695914987888146541, 34.68535235679833306 ) ) ;
#17458=VERTEX_POINT ( 'NONE', #75055 ) ;
#17459=CARTESIAN_POINT ( 'NONE',  ( -5.076923076923075762, -2.900454961884010974, 35.62045528018868623 ) ) ;
#17460=CARTESIAN_POINT ( 'NONE',  ( -5.933932666649924137, -2.486705287966279876, 31.30864560766543647 ) ) ;
#17462=B_SPLINE_CURVE_WITH_KNOTS ( 'NONE', 3,
 ( #10226, #72357, #16091, #64259, #24619, #64706, #37686, #30486, #9342, #31378 ),
 .UNSPECIFIED., .F., .F.,
 ( 4, 2, 2, 2, 4 ),
 ( 0.000000000000000000, 0.0001954311564186871455, 0.0003908623128373742909, 0.0005862934692560614093, 0.0007817246256747485819 ),
 .UNSPECIFIED. ) ;
#17463=VECTOR ( 'NONE', #76672, 1000.000000000000227 ) ;
#17464=CARTESIAN_POINT ( 'NONE',  ( -10.61538461538473577, -10.33852847137269571, 34.16647553114546554 ) ) ;
#17465=DIRECTION ( 'NONE',  ( 0.000000000000000000, 0.3420201433256610524, 0.9396926207859113145 ) ) ;
#17466=ORIENTED_EDGE ( 'NONE', *, *, #30653, .F. ) ;
#17467=CARTESIAN_POINT ( 'NONE',  ( 1.515141086378950508, -4.459921816937788996, 33.71989282347011851 ) ) ;
#17468=DIRECTION ( 'NONE',  ( 0.000000000000000000, 0.3420201433256641055, -0.9396926207859100932 ) ) ;
#17469=CARTESIAN_POINT ( 'NONE',  ( 8.769230769230645706, -2.657715359629662544, 31.77849191805970364 ) ) ;
#17470=ORIENTED_EDGE ( 'NONE', *, *, #26580, .F. ) ;
#17471=CARTESIAN_POINT ( 'NONE',  ( -11.31508559776335510, -2.501478030877323455, 29.88021232661721172 ) ) ;
#17472=CARTESIAN_POINT ( 'NONE',  ( 16.82692307692308020, -7.566082377512564960, 35.00000000000000711 ) ) ;
#17473=EDGE_CURVE ( 'NONE', #28852, #24412, #81814, .T. ) ;
#17474=LINE ( 'NONE', #305, #70838 ) ;
#17477=EDGE_CURVE ( 'NONE', #83475, #41702, #66962, .T. ) ;
#17478=EDGE_LOOP ( 'NONE', ( #32249, #21158 ) ) ;
#17479=CARTESIAN_POINT ( 'NONE',  ( 2.438484115517096207, -12.11778462344221019, 31.66786338562085135 ) ) ;
#17482=DIRECTION ( 'NONE',  ( -0.000000000000000000, -0.000000000000000000, -1.000000000000000000 ) ) ;
#17483=ORIENTED_EDGE ( 'NONE', *, *, #80515, .T. ) ;
#17484=VERTEX_POINT ( 'NONE', #25967 ) ;
#17485=ORIENTED_EDGE ( 'NONE', *, *, #68792, .T. ) ;
#17486=CARTESIAN_POINT ( 'NONE',  ( -9.692307692307812417, -10.21337939537710326, 33.94971097300076224 ) ) ;
#17487=CYLINDRICAL_SURFACE ( 'NONE', #25645, 0.2500000000000004996 ) ;
#17488=B_SPLINE_CURVE_WITH_KNOTS ( 'NONE', 3,
 ( #67093, #24765, #80619, #79720, #5394, #25660, #61535, #53115, #18019, #18903 ),
 .UNSPECIFIED., .F., .F.,
 ( 4, 2, 2, 2, 4 ),
 ( 0.000000000000000000, 0.0001954311564186864407, 0.0003908623128373728815, 0.0005862934692560593493, 0.0007817246256747457630 ),
 .UNSPECIFIED. ) ;
#17489=DIRECTION ( 'NONE',  ( -0.000000000000000000, 1.000000000000000000, 3.491481338843133355E-15 ) ) ;
#17490=B_SPLINE_CURVE_WITH_KNOTS ( 'NONE', 3,
 ( #39473, #67375, #79999, #73702, #33142, #18300, #81344, #39028, #46658, #44867 ),
 .UNSPECIFIED., .F., .F.,
 ( 4, 2, 2, 2, 4 ),
 ( 0.0007817359430256326080, 0.0009771253907249993591, 0.001172514838424366327, 0.001367904286123733078, 0.001563293733823099829 ),
 .UNSPECIFIED. ) ;
#17491=LINE ( 'NONE', #3070, #36309 ) ;
#17492=AXIS2_PLACEMENT_3D ( 'NONE', #19853, #6777, #60389 ) ;
#17494=EDGE_LOOP ( 'NONE', ( #71547, #40140 ) ) ;
#17495=CARTESIAN_POINT ( 'NONE',  ( 10.36538461538461675, -7.500000000000001776, 35.04278698407183867 ) ) ;
#17496=EDGE_LOOP ( 'NONE', ( #12344, #12893 ) ) ;
#17497=FACE_OUTER_BOUND ( 'NONE', #58545, .T. ) ;
#17498=VECTOR ( 'NONE', #7936, 1000.000000000000227 ) ;
#17501=CARTESIAN_POINT ( 'NONE',  ( -1.161835715637316913, -12.69155399931963046, 30.53255429739158444 ) ) ;
#17502=ORIENTED_EDGE ( 'NONE', *, *, #86250, .F. ) ;
#17503=ORIENTED_EDGE ( 'NONE', *, *, #65348, .T. ) ;
#17504=VERTEX_POINT ( 'NONE', #26419 ) ;
#17505=CARTESIAN_POINT ( 'NONE',  ( -13.38461538461506883, -2.255955759149395501, 30.00000000000324363 ) ) ;
#17506=VERTEX_POINT ( 'NONE', #80934 ) ;
#17507=EDGE_CURVE ( 'NONE', #10416, #36685, #77984, .T. ) ;
#17508=DIRECTION ( 'NONE',  ( -0.000000000000000000, -0.1736481776669307198, -0.9848077530122080203 ) ) ;
#17509=CARTESIAN_POINT ( 'NONE',  ( -7.846153846153844924, -3.050289026998446396, 32.03036669348365706 ) ) ;
#17510=EDGE_LOOP ( 'NONE', ( #36321, #6639 ) ) ;
#17512=DIRECTION ( 'NONE',  ( 0.000000000000000000, 0.9848077530122072432, -0.1736481776669354937 ) ) ;
#17514=DIRECTION ( 'NONE',  ( 0.000000000000000000, -6.938893903907222067E-15, 1.000000000000000000 ) ) ;
#17515=B_SPLINE_CURVE_WITH_KNOTS ( 'NONE', 3,
 ( #32663, #6090, #33566, #14169, #27680, #76308, #69555, #61902, #56038, #28122 ),
 .UNSPECIFIED., .F., .F.,
 ( 4, 2, 2, 2, 4 ),
 ( 0.000000000000000000, 0.0001954311564186871184, 0.0003908623128373742367, 0.0005862934692560614093, 0.0007817246256747484735 ),
 .UNSPECIFIED. ) ;
#17516=FACE_BOUND ( 'NONE', #82836, .T. ) ;
#17517=DIRECTION ( 'NONE',  ( 0.000000000000000000, 1.000000000000000000, 0.000000000000000000 ) ) ;
#17518=CARTESIAN_POINT ( 'NONE',  ( 11.28843830116857383, -8.432397168068783699, 34.66272746175022945 ) ) ;
#17520=CARTESIAN_POINT ( 'NONE',  ( -15.00775787915638304, -10.61302985866383963, 33.66295027996417843 ) ) ;
#17522=CARTESIAN_POINT ( 'NONE',  ( 9.692307692307695177, -3.050289026998446396, 32.03036669348365706 ) ) ;
#17523=AXIS2_PLACEMENT_3D ( 'NONE', #24011, #44721, #23134 ) ;
#17525=CARTESIAN_POINT ( 'NONE',  ( 1.634669804528839254, -2.318338780012835443, 30.59689888758630261 ) ) ;
#17526=VERTEX_POINT ( 'NONE', #69613 ) ;
#17527=CYLINDRICAL_SURFACE ( 'NONE', #37446, 0.2499999999999994726 ) ;
#17528=CARTESIAN_POINT ( 'NONE',  ( -13.13466997523734392, -4.176053281294518804, 33.81426240980091791 ) ) ;
#17531=CARTESIAN_POINT ( 'NONE',  ( -13.38461538461538325, -12.78798330534102945, 29.74999999999997868 ) ) ;
#17532=CARTESIAN_POINT ( 'NONE',  ( 1.384615384615386802, -10.51840700105979565, 33.73612834413961536 ) ) ;
#17533=ADVANCED_FACE ( 'NONE', ( #48445 ), #7483, .F. ) ;
#17534=CARTESIAN_POINT ( 'NONE',  ( -5.777220458731586739, -6.760870238392817200, 34.69528174975672385 ) ) ;
#17535=CARTESIAN_POINT ( 'NONE',  ( 1.319344938654611221, -6.879047030191174805, 34.71129190930000163 ) ) ;
#17536=CARTESIAN_POINT ( 'NONE',  ( -0.4615384615385826339, -11.94971097300221174, 32.03036669348237098 ) ) ;
#17537=ORIENTED_EDGE ( 'NONE', *, *, #25203, .T. ) ;
#17538=LINE ( 'NONE', #78335, #8439 ) ;
#17539=CARTESIAN_POINT ( 'NONE',  ( 11.60452887181161685, -2.833524468853757750, 32.15551576947925838 ) ) ;
#17540=CARTESIAN_POINT ( 'NONE',  ( 15.23076923076910916, -11.06231777344772027, 33.60647404775119895 ) ) ;
#17541=CARTESIAN_POINT ( 'NONE',  ( 7.780070435197966816, -5.557115091759785130, 34.35708131394839171 ) ) ;
#17543=CARTESIAN_POINT ( 'NONE',  ( -7.846153846153967493, -9.528491918059723176, 34.59228464037033035 ) ) ;
#17545=VERTEX_POINT ( 'NONE', #7920 ) ;
#17546=EDGE_CURVE ( 'NONE', #54081, #8200, #37150, .T. ) ;
#17547=EDGE_LOOP ( 'NONE', ( #22784, #4071, #2238, #48260 ) ) ;
#17548=CARTESIAN_POINT ( 'NONE',  ( -15.23076923076935252, -4.320704448113951379, 33.92786785259630022 ) ) ;
#17549=EDGE_CURVE ( 'NONE', #71998, #86919, #48953, .T. ) ;
#17550=DIRECTION ( 'NONE',  ( -0.000000000000000000, -0.9396926207859093161, -0.3420201433256663259 ) ) ;
#17551=CYLINDRICAL_SURFACE ( 'NONE', #4290, 0.2499999999999986955 ) ;
#17553=CARTESIAN_POINT ( 'NONE',  ( 16.85409497928819533, -7.369209533119136069, 34.99857337881830688 ) ) ;
#17555=CARTESIAN_POINT ( 'NONE',  ( -12.46153846153846168, -3.513871655860378418, 32.76840700105978499 ) ) ;
#17556=FACE_OUTER_BOUND ( 'NONE', #78037, .T. ) ;
#17557=EDGE_LOOP ( 'NONE', ( #34766, #49684 ) ) ;
#17558=CARTESIAN_POINT ( 'NONE',  ( -8.835313148590902443, -12.62096338111211580, 30.90682066428152908 ) ) ;
#17559=CARTESIAN_POINT ( 'NONE',  ( 1.384615384615386802, -1.629998284177014645, 34.34916445242399163 ) ) ;
#17560=ORIENTED_EDGE ( 'NONE', *, *, #61348, .T. ) ;
#17561=CARTESIAN_POINT ( 'NONE',  ( -9.915187209045276617, -7.630690623152299956, 34.99857592706774057 ) ) ;
#17562=CARTESIAN_POINT ( 'NONE',  ( -9.757578138268465651, -12.27809138561121394, 31.22303859784730307 ) ) ;
#17563=AXIS2_PLACEMENT_3D ( 'NONE', #54532, #54985, #88798 ) ;
#17564=CARTESIAN_POINT ( 'NONE',  ( -12.46153846153846168, -8.164416787775445883, 34.95778746994557906 ) ) ;
#17566=CARTESIAN_POINT ( 'NONE',  ( 11.53846153846153832, -1.044019251281081972, 31.83374038241031911 ) ) ;
#17567=EDGE_CURVE ( 'NONE', #84690, #47265, #55648, .T. ) ;
#17568=CARTESIAN_POINT ( 'NONE',  ( 7.623226887246995709, -3.395401636524185474, 33.02366814457250399 ) ) ;
#17569=CARTESIAN_POINT ( 'NONE',  ( -8.069080063669991532, -12.39988816332205701, 30.74660775122750778 ) ) ;
#17574=CARTESIAN_POINT ( 'NONE',  ( 8.769230769230647482, -11.94971097300221174, 32.03036669348237098 ) ) ;
#17575=CARTESIAN_POINT ( 'NONE',  ( 13.25446741488368829, -6.809168938359901446, 34.95455904226513866 ) ) ;
#17577=B_SPLINE_CURVE_WITH_KNOTS ( 'NONE', 3,
 ( #63480, #82448, #1782, #56288, #82886, #62589, #83774, #49082, #35128, #29272 ),
 .UNSPECIFIED., .F., .F.,
 ( 4, 2, 2, 2, 4 ),
 ( 0.0007817246256747445703, 0.0009771112852218872494, 0.001172497944769030145, 0.001367884604316172825, 0.001563271263863315504 ),
 .UNSPECIFIED. ) ;
#17578=CARTESIAN_POINT ( 'NONE',  ( 3.230769230769231726, -3.937682226553329556, 33.60647404775216529 ) ) ;
#17579=CYLINDRICAL_SURFACE ( 'NONE', #34184, 0.2500000000000009437 ) ;
#17580=CARTESIAN_POINT ( 'NONE',  ( -9.019253993452226226, -2.588893531581426988, 31.60682220781847818 ) ) ;
#17581=VERTEX_POINT ( 'NONE', #34502 ) ;
#17584=EDGE_CURVE ( 'NONE', #64675, #78946, #27433, .T. ) ;
#17585=ORIENTED_EDGE ( 'NONE', *, *, #86026, .F. ) ;
#17588=CARTESIAN_POINT ( 'NONE',  ( -7.846153846153967493, -6.835583212225970762, 34.95778746994575670 ) ) ;
#17589=EDGE_CURVE ( 'NONE', #43442, #3517, #77257, .T. ) ;
#17590=EDGE_CURVE ( 'NONE', #9159, #67813, #62837, .T. ) ;
#17592=CARTESIAN_POINT ( 'NONE',  ( 16.85399611801622655, -6.459968553980840689, 34.89616026154728701 ) ) ;
#17593=ORIENTED_EDGE ( 'NONE', *, *, #14844, .T. ) ;
#17596=CARTESIAN_POINT ( 'NONE',  ( 13.13461538461537437, -2.249999999999998668, 29.81609741502487410 ) ) ;
#17597=EDGE_CURVE ( 'NONE', #78524, #23088, #39235, .T. ) ;
#17599=VERTEX_POINT ( 'NONE', #1157 ) ;
#17600=AXIS2_PLACEMENT_3D ( 'NONE', #51687, #58023, #31896 ) ;
#17601=CARTESIAN_POINT ( 'NONE',  ( -15.93106648486808119, -2.353885683473779356, 30.79025554430704759 ) ) ;
#17602=CARTESIAN_POINT ( 'NONE',  ( 0.7114839798866035014, -11.37275283266503756, 32.91324779482534524 ) ) ;
#17603=VERTEX_POINT ( 'NONE', #28638 ) ;
#17604=CARTESIAN_POINT ( 'NONE',  ( -6.065270000556320262, -11.06231777344662781, 33.60647404775220082 ) ) ;
#17605=CARTESIAN_POINT ( 'NONE',  ( -12.46153846153858247, -6.026961402154118019, 34.52809138561165270 ) ) ;
#17606=CARTESIAN_POINT ( 'NONE',  ( 12.71159277317677549, -4.943051570960394159, 34.04725096376909477 ) ) ;
#17608=B_SPLINE_CURVE_WITH_KNOTS ( 'NONE', 3,
 ( #24374, #44641, #78000, #10438, #43771, #37906, #72572, #3662, #71232, #79338 ),
 .UNSPECIFIED., .F., .F.,
 ( 4, 2, 2, 2, 4 ),
 ( 0.000000000000000000, 0.0001954339857564083417, 0.0003908679715128166835, 0.0005863019572692250523, 0.0007817359430256333669 ),
 .UNSPECIFIED. ) ;
#17609=B_SPLINE_CURVE_WITH_KNOTS ( 'NONE', 3,
 ( #35324, #62780, #28580, #56039, #83531, #21813, #79864, #18614, #59138, #24016 ),
 .UNSPECIFIED., .F., .F.,
 ( 4, 2, 2, 2, 4 ),
 ( 0.0007817246256747457630, 0.0009771112852218887673, 0.001172497944769031880, 0.001367884604316174993, 0.001563271263863318106 ),
 .UNSPECIFIED. ) ;
#17611=DIRECTION ( 'NONE',  ( -0.000000000000000000, 0.5000000000000011102, -0.8660254037844380415 ) ) ;
#17612=ORIENTED_EDGE ( 'NONE', *, *, #63108, .F. ) ;
#17613=VERTEX_POINT ( 'NONE', #76827 ) ;
#17615=CARTESIAN_POINT ( 'NONE',  ( -39.05038313613820122, -2.499999999999999556, 29.75000000000000355 ) ) ;
#17618=CARTESIAN_POINT ( 'NONE',  ( 4.153846153846154188, -10.05456864172156806, 36.03766855953608683 ) ) ;
#17619=CARTESIAN_POINT ( 'NONE',  ( -10.61538461538473399, -9.442884908241554243, 34.35708131394783038 ) ) ;
#17620=EDGE_LOOP ( 'NONE', ( #14634, #40286 ) ) ;
#17621=ORIENTED_EDGE ( 'NONE', *, *, #62398, .T. ) ;
#17623=CARTESIAN_POINT ( 'NONE',  ( -1.634638621908348410, -11.86270091957321249, 32.19358267280087915 ) ) ;
#17624=ORIENTED_EDGE ( 'NONE', *, *, #30742, .T. ) ;
#17625=VECTOR ( 'NONE', #28179, 1000.000000000000000 ) ;
#17626=CARTESIAN_POINT ( 'NONE',  ( -10.48485891362105171, -9.417988943895561960, 34.36773134775777550 ) ) ;
#17627=CARTESIAN_POINT ( 'NONE',  ( 16.85399611801622655, -12.38737895849757820, 31.66785238281580206 ) ) ;
#17629=FACE_BOUND ( 'NONE', #5481, .T. ) ;
#17630=ORIENTED_EDGE ( 'NONE', *, *, #46184, .F. ) ;
#17631=CARTESIAN_POINT ( 'NONE',  ( -7.846153846153967493, -5.941354392335915335, 34.76329471203413846 ) ) ;
#17632=CARTESIAN_POINT ( 'NONE',  ( 12.68431800280687050, -5.913360116392397892, 34.49180327182771322 ) ) ;
#17633=DIRECTION ( 'NONE',  ( 0.000000000000000000, 0.1736481776669275834, 0.9848077530122086864 ) ) ;
#17634=CARTESIAN_POINT ( 'NONE',  ( -14.55771554498526932, -9.271318131107980420, 34.42618302367067429 ) ) ;
#17635=CARTESIAN_POINT ( 'NONE',  ( 7.976679547917413515, -10.88167719472716399, 33.43325721877153711 ) ) ;
#17636=ORIENTED_EDGE ( 'NONE', *, *, #56477, .T. ) ;
#17637=CARTESIAN_POINT ( 'NONE',  ( -9.692307692307691624, -12.29105614889573062, 35.45975837776705220 ) ) ;
#17638=EDGE_LOOP ( 'NONE', ( #35913, #88483 ) ) ;
#17639=VERTEX_POINT ( 'NONE', #84037 ) ;
#17640=CARTESIAN_POINT ( 'NONE',  ( 5.869309396889695662, -11.93127051446800024, 32.56575433478200665 ) ) ;
#17641=FACE_OUTER_BOUND ( 'NONE', #43321, .T. ) ;
#17642=CARTESIAN_POINT ( 'NONE',  ( -8.519176349317316266, -12.41089969410671223, 31.60739465890703670 ) ) ;
#17644=CARTESIAN_POINT ( 'NONE',  ( 1.634560902963527962, -10.05730279482229683, 34.04704008940765902 ) ) ;
#17645=CARTESIAN_POINT ( 'NONE',  ( -11.78848476268299628, -2.341070481393819236, 30.72580821765574299 ) ) ;
#17646=VERTEX_POINT ( 'NONE', #15123 ) ;
#17648=CARTESIAN_POINT ( 'NONE',  ( 11.53846153846153832, -2.721908614388771852, 31.22303859784724978 ) ) ;
#17649=CARTESIAN_POINT ( 'NONE',  ( 10.48469401227430708, -2.845849958028613624, 32.17971566917920967 ) ) ;
#17650=CARTESIAN_POINT ( 'NONE',  ( 10.74591031714818357, -11.93748526763465279, 32.05452791011430946 ) ) ;
#17651=EDGE_LOOP ( 'NONE', ( #24260, #89023, #3307, #10301 ) ) ;
#17652=VERTEX_POINT ( 'NONE', #8366 ) ;
#17653=FACE_BOUND ( 'NONE', #85329, .T. ) ;
#17655=EDGE_CURVE ( 'NONE', #44478, #19274, #22318, .T. ) ;
#17658=CARTESIAN_POINT ( 'NONE',  ( 18.25000000000143530, -7.500000000000155431, 34.75000000000007105 ) ) ;
#17659=CARTESIAN_POINT ( 'NONE',  ( -13.31854703361294767, -10.51840700105979565, 33.73612834413962247 ) ) ;
#17660=ORIENTED_EDGE ( 'NONE', *, *, #86872, .F. ) ;
#17661=FACE_OUTER_BOUND ( 'NONE', #15814, .T. ) ;
#17663=CARTESIAN_POINT ( 'NONE',  ( 4.946231610255517275, -2.729777683071817229, 31.24903638046268739 ) ) ;
#17664=DIRECTION ( 'NONE',  ( -0.000000000000000000, -0.1736481776669307198, -0.9848077530122080203 ) ) ;
#17666=ORIENTED_EDGE ( 'NONE', *, *, #17813, .T. ) ;
#17667=CARTESIAN_POINT ( 'NONE',  ( 13.51540582558233794, -8.191423895709840863, 34.95447573519442130 ) ) ;
#17669=CARTESIAN_POINT ( 'NONE',  ( -14.30769230769230660, -5.180354513474913603, 36.12317359536750416 ) ) ;
#17670=CYLINDRICAL_SURFACE ( 'NONE', #5129, 0.2499999999999979738 ) ;
#17671=DIRECTION ( 'NONE',  ( -0.000000000000000000, 0.9848077530122086864, -0.1736481776669273891 ) ) ;
#17673=CARTESIAN_POINT ( 'NONE',  ( 12.46153846153833911, -12.27809138561165270, 31.22303859784587132 ) ) ;
#17675=CARTESIAN_POINT ( 'NONE',  ( 12.21156171748987163, -5.643011162660950042, 34.66104346484419096 ) ) ;
#17677=ORIENTED_EDGE ( 'NONE', *, *, #46727, .F. ) ;
#17678=CARTESIAN_POINT ( 'NONE',  ( -3.453695448285378333, -3.105860786376062332, 32.13614157043598851 ) ) ;
#17679=CARTESIAN_POINT ( 'NONE',  ( 7.976201281404299515, -7.723484941389745728, 34.99544897038809665 ) ) ;
#17682=ORIENTED_EDGE ( 'NONE', *, *, #65991, .F. ) ;
#17683=CARTESIAN_POINT ( 'NONE',  ( -8.992157728137616601, -5.582147617184174848, 34.63737895849758530 ) ) ;
#17684=CARTESIAN_POINT ( 'NONE',  ( -14.17690186672535901, -2.494656445102012565, 31.33466734024120015 ) ) ;
#17686=CARTESIAN_POINT ( 'NONE',  ( -4.153846153846152411, -9.058645607665452459, 34.76329471203371924 ) ) ;
#17687=DIRECTION ( 'NONE',  ( -0.000000000000000000, -0.3420201433256694346, -0.9396926207859080948 ) ) ;
#17688=VECTOR ( 'NONE', #34854, 999.9999999999998863 ) ;
#17689=CARTESIAN_POINT ( 'NONE',  ( -8.835314180186648159, -11.69971097300155272, 32.46337939537587403 ) ) ;
#17690=VECTOR ( 'NONE', #63076, 1000.000000000000000 ) ;
#17692=VERTEX_POINT ( 'NONE', #18563 ) ;
#17693=CARTESIAN_POINT ( 'NONE',  ( 6.065255571276024327, -10.90142922261932057, 33.41473453929631887 ) ) ;
#17695=CARTESIAN_POINT ( 'NONE',  ( -17.32692307692307310, -7.566083408709835645, 34.74999999999999289 ) ) ;
#17696=EDGE_CURVE ( 'NONE', #31113, #70330, #43523, .T. ) ;
#17697=DIRECTION ( 'NONE',  ( -0.000000000000000000, -0.8660254037844399289, -0.4999999999999980016 ) ) ;
#17698=CARTESIAN_POINT ( 'NONE',  ( 16.82694634598072270, -9.148715823498378086, 34.47080413974185120 ) ) ;
#17699=EDGE_LOOP ( 'NONE', ( #70208, #12003 ) ) ;
#17700=CARTESIAN_POINT ( 'NONE',  ( 10.54930223602447903, -9.058645607665454236, 34.76329471203372634 ) ) ;
#17701=B_SPLINE_CURVE_WITH_KNOTS ( 'NONE', 3,
 ( #48733, #35221, #35680, #6864, #55052, #70343, #28025, #41102, #21259, #55491 ),
 .UNSPECIFIED., .F., .F.,
 ( 4, 2, 2, 2, 4 ),
 ( 0.0007817246256747478229, 0.0009771112852218913694, 0.001172497944769034916, 0.001367884604316178679, 0.001563271263863322226 ),
 .UNSPECIFIED. ) ;
#17702=EDGE_LOOP ( 'NONE', ( #81995, #63846, #72656, #26267 ) ) ;
#17703=DIRECTION ( 'NONE',  ( 0.000000000000000000, 0.4999999999999960032, -0.8660254037844410391 ) ) ;
#17705=CARTESIAN_POINT ( 'NONE',  ( -13.51522503981946599, -7.722926974430166069, 34.99546784045485737 ) ) ;
#17706=CARTESIAN_POINT ( 'NONE',  ( 6.249945409378044658, -12.07971442181322352, 32.31769673815850297 ) ) ;
#17710=CARTESIAN_POINT ( 'NONE',  ( -1.384615384615506484, -12.70778746994576025, 30.41441678777401236 ) ) ;
#17711=CARTESIAN_POINT ( 'NONE',  ( -10.55012904410859242, -10.90142922261932057, 33.41473453929631887 ) ) ;
#17712=CARTESIAN_POINT ( 'NONE',  ( -7.715363405186896451, -4.684288915650983043, 34.18129842949671371 ) ) ;
#17713=CYLINDRICAL_SURFACE ( 'NONE', #3749, 0.2500000000000008882 ) ;
#17714=ORIENTED_EDGE ( 'NONE', *, *, #65335, .T. ) ;
#17715=CARTESIAN_POINT ( 'NONE',  ( -10.83825003758825467, -2.501496062324912284, 29.88072118266895671 ) ) ;
#17716=ORIENTED_EDGE ( 'NONE', *, *, #77748, .F. ) ;
#17717=CARTESIAN_POINT ( 'NONE',  ( -17.07692307692319744, -5.219633306517616589, 34.19971097300220464 ) ) ;
#17718=VECTOR ( 'NONE', #86233, 1000.000000000000114 ) ;
#17719=CARTESIAN_POINT ( 'NONE',  ( -9.561515884482904681, -12.11778462344220841, 31.66786338562085135 ) ) ;
#17720=VECTOR ( 'NONE', #4212, 1000.000000000000000 ) ;
#17721=CARTESIAN_POINT ( 'NONE',  ( -13.63459211555773720, -2.779195860258146578, 31.39871582349836032 ) ) ;
#17723=CARTESIAN_POINT ( 'NONE',  ( 15.23076923076923173, -1.629998284177014645, 34.34916445242399163 ) ) ;
#17724=CARTESIAN_POINT ( 'NONE',  ( 16.02369818411445834, -12.15440758774515473, 32.17923288041532004 ) ) ;
#17725=AXIS2_PLACEMENT_3D ( 'NONE', #85288, #23574, #51020 ) ;
#17726=ORIENTED_EDGE ( 'NONE', *, *, #82926, .F. ) ;
#17728=ORIENTED_EDGE ( 'NONE', *, *, #29449, .T. ) ;
#17729=ORIENTED_EDGE ( 'NONE', *, *, #67033, .F. ) ;
#17731=CARTESIAN_POINT ( 'NONE',  ( -10.48485891362105171, -8.586989748646452369, 34.63063291749215011 ) ) ;
#17732=CARTESIAN_POINT ( 'NONE',  ( -21.00000000000000000, -2.249999999999998668, 29.75000000000000355 ) ) ;
#17733=DIRECTION ( 'NONE',  ( -0.000000000000000000, 0.7660444431189791237, -0.6427876096865379196 ) ) ;
#17734=DIRECTION ( 'NONE',  ( -0.000000000000000000, -0.9848077530122085754, -0.1736481776669273613 ) ) ;
#17735=CARTESIAN_POINT ( 'NONE',  ( -13.51530598772569469, -3.338472653186243644, 32.95098750199972670 ) ) ;
#17736=CARTESIAN_POINT ( 'NONE',  ( 0.4615384615384611200, -4.786620604624113540, 33.94971097300155094 ) ) ;
#17737=CARTESIAN_POINT ( 'NONE',  ( -0.4615384615384611200, -11.69971097300155272, 32.46337939537588113 ) ) ;
#17738=CARTESIAN_POINT ( 'NONE',  ( 4.153846153846030731, -3.083524468854526912, 32.58852847137268327 ) ) ;
#17739=CARTESIAN_POINT ( 'NONE',  ( 7.846153846153723244, -5.094484230521993062, 34.41647553114689373 ) ) ;
#17742=EDGE_CURVE ( 'NONE', #33011, #78633, #73512, .T. ) ;
#17743=ORIENTED_EDGE ( 'NONE', *, *, #31077, .F. ) ;
#17744=CARTESIAN_POINT ( 'NONE',  ( 0.4615384615384611200, -11.91647553114624181, 32.58852847137148245 ) ) ;
#17745=EDGE_LOOP ( 'NONE', ( #61627, #29844, #43434, #48166 ) ) ;
#17746=AXIS2_PLACEMENT_3D ( 'NONE', #69868, #29335, #43287 ) ;
#17747=LINE ( 'NONE', #65479, #14380 ) ;
#17748=CARTESIAN_POINT ( 'NONE',  ( -18.00000000000000000, -11.35647404775217240, 33.31231777344666511 ) ) ;
#17749=VECTOR ( 'NONE', #52374, 1000.000000000000227 ) ;
#17750=CARTESIAN_POINT ( 'NONE',  ( -1.449885385171703511, -5.094484230520674117, 34.41647553114621161 ) ) ;
#17751=CARTESIAN_POINT ( 'NONE',  ( -13.38461538461538325, -1.215029322943914858, 32.30358669280327177 ) ) ;
#17752=FACE_BOUND ( 'NONE', #56490, .T. ) ;
#17753=ORIENTED_EDGE ( 'NONE', *, *, #62487, .F. ) ;
#17754=EDGE_LOOP ( 'NONE', ( #17314, #12854, #40284, #7866 ) ) ;
#17755=CARTESIAN_POINT ( 'NONE',  ( 17.99999999999987566, -3.835265460704628815, 33.15142922262033665 ) ) ;
#17756=VERTEX_POINT ( 'NONE', #77701 ) ;
#17757=FACE_BOUND ( 'NONE', #47181, .T. ) ;
#17758=CARTESIAN_POINT ( 'NONE',  ( -16.15384615384615330, -3.669653830205710676, 35.88435417666054406 ) ) ;
#17759=EDGE_CURVE ( 'NONE', #51881, #84238, #29672, .T. ) ;
#17760=CARTESIAN_POINT ( 'NONE',  ( -14.30769230769230660, -13.20930481340135110, 34.54067556320372745 ) ) ;
#17761=ORIENTED_EDGE ( 'NONE', *, *, #54725, .F. ) ;
#17762=CARTESIAN_POINT ( 'NONE',  ( 12.21153846153846168, -7.500000000000001776, 35.00000000000000000 ) ) ;
#17763=CARTESIAN_POINT ( 'NONE',  ( -1.515305987725691139, -8.191372820521381826, 34.95448215188423546 ) ) ;
#17764=CARTESIAN_POINT ( 'NONE',  ( 1.161130460051056357, -3.562934362175799841, 33.22335522853832401 ) ) ;
#17765=EDGE_LOOP ( 'NONE', ( #71763, #38131 ) ) ;
#17766=ADVANCED_FACE ( 'NONE', ( #25761 ), #16009, .F. ) ;
#17767=DIRECTION ( 'NONE',  ( 0.000000000000000000, 0.4999999999999985567, 0.8660254037844395958 ) ) ;
#17768=CARTESIAN_POINT ( 'NONE',  ( -18.22292621751613950, -4.887634598454294377, 34.01352882383564946 ) ) ;
#17769=ORIENTED_EDGE ( 'NONE', *, *, #65265, .F. ) ;
#17770=DIRECTION ( 'NONE',  ( -0.000000000000000000, -0.1736481776669307198, -0.9848077530122080203 ) ) ;
#17771=CARTESIAN_POINT ( 'NONE',  ( -9.692307692307691624, -2.721908614388771852, 31.22303859784724978 ) ) ;
#17772=ORIENTED_EDGE ( 'NONE', *, *, #32652, .T. ) ;
#17773=CARTESIAN_POINT ( 'NONE',  ( 18.22277954126840172, -6.760870238392814535, 34.69528174975672385 ) ) ;
#17774=CARTESIAN_POINT ( 'NONE',  ( -12.33074665371367828, -2.541949514083464479, 30.39797389878540557 ) ) ;
#17775=CARTESIAN_POINT ( 'NONE',  ( 16.15384615384603251, -3.083524468854526912, 32.58852847137268327 ) ) ;
#17776=CARTESIAN_POINT ( 'NONE',  ( 15.00784227186237985, -12.64616026154729411, 30.79003144601914244 ) ) ;
#17777=DIRECTION ( 'NONE',  ( -0.000000000000000000, 0.9848077530122085754, -0.1736481776669273613 ) ) ;
#17778=B_SPLINE_CURVE_WITH_KNOTS ( 'NONE', 3,
 ( #46010, #64939, #24398, #18551, #32060, #86123, #45117, #38372, #5030, #52317 ),
 .UNSPECIFIED., .F., .F.,
 ( 4, 2, 2, 2, 4 ),
 ( 0.000000000000000000, 0.0001954339857564097241, 0.0003908679715128194482, 0.0005863019572692291723, 0.0007817359430256388964 ),
 .UNSPECIFIED. ) ;
#17780=CARTESIAN_POINT ( 'NONE',  ( 5.076923076923075762, -12.37446782046654192, 30.86335684631486131 ) ) ;
#17782=CARTESIAN_POINT ( 'NONE',  ( -17.07692307692319744, -8.613356846316285953, 34.62446782046622218 ) ) ;
#17784=CARTESIAN_POINT ( 'NONE',  ( -3.296039676730006640, -2.625532179533444754, 30.86335684631481513 ) ) ;
#17785=CARTESIAN_POINT ( 'NONE',  ( 12.39621554604628706, -7.749976743299138882, 34.99404534957040624 ) ) ;
#17786=FACE_OUTER_BOUND ( 'NONE', #33355, .T. ) ;
#17789=AXIS2_PLACEMENT_3D ( 'NONE', #38850, #17235, #66312 ) ;
#17790=CARTESIAN_POINT ( 'NONE',  ( -12.52762187249433978, -8.120952969808774569, 34.71129190930000163 ) ) ;
#17792=ADVANCED_FACE ( 'NONE', ( #52777 ), #70950, .F. ) ;
#17793=ORIENTED_EDGE ( 'NONE', *, *, #11664, .F. ) ;
#17794=CARTESIAN_POINT ( 'NONE',  ( -16.82686865700962642, -4.074993327901529128, 33.72946981652012255 ) ) ;
#17796=CARTESIAN_POINT ( 'NONE',  ( -5.869474561766354626, -10.31582465632705237, 34.18122507451815295 ) ) ;
#17799=CARTESIAN_POINT ( 'NONE',  ( -15.36091720050092846, -12.50552854090298993, 31.33409797877408920 ) ) ;
#17800=LINE ( 'NONE', #45252, #87892 ) ;
#17801=CARTESIAN_POINT ( 'NONE',  ( -12.21148404162501144, -4.074993327901527351, 33.72946981652012255 ) ) ;
#17802=CARTESIAN_POINT ( 'NONE',  ( -5.076923076923075762, -2.486705287966279876, 31.30864560766543647 ) ) ;
#17803=CARTESIAN_POINT ( 'NONE',  ( -10.86540785267757947, -4.335965774309648246, 33.62209801155881905 ) ) ;
#17804=CARTESIAN_POINT ( 'NONE',  ( 6.000000000000001776, -4.098570777380720287, 33.41473453929634729 ) ) ;
#17806=DIRECTION ( 'NONE',  ( -0.000000000000000000, -0.5000000000000009992, -0.8660254037844380415 ) ) ;
#17807=CARTESIAN_POINT ( 'NONE',  ( -15.09997742294444478, -2.541949514083464479, 30.39797389878540557 ) ) ;
#17808=EDGE_CURVE ( 'NONE', #43520, #75897, #2475, .T. ) ;
#17809=EDGE_CURVE ( 'NONE', #75253, #43597, #53221, .T. ) ;
#17810=DIRECTION ( 'NONE',  ( -0.000000000000000000, 0.7660444431189791237, -0.6427876096865379196 ) ) ;
#17811=VERTEX_POINT ( 'NONE', #78586 ) ;
#17812=ORIENTED_EDGE ( 'NONE', *, *, #84199, .F. ) ;
#17813=EDGE_CURVE ( 'NONE', #45, #52162, #65059, .T. ) ;
#17814=CARTESIAN_POINT ( 'NONE',  ( 14.55774661933062575, -4.943051570960394159, 34.04725096376909477 ) ) ;
#17815=CARTESIAN_POINT ( 'NONE',  ( -17.30040802064702987, -8.496056993536548418, 34.65000542017679663 ) ) ;
#17816=DIRECTION ( 'NONE',  ( -0.000000000000000000, 0.9396926207859093161, -0.3420201433256663259 ) ) ;
#17818=EDGE_CURVE ( 'NONE', #15876, #27342, #28557, .T. ) ;
#17819=B_SPLINE_CURVE_WITH_KNOTS ( 'NONE', 3,
 ( #67737, #87584, #88917, #81700, #68179, #19983, #6482, #33944, #27188, #63182 ),
 .UNSPECIFIED., .F., .F.,
 ( 4, 2, 2, 2, 4 ),
 ( 0.0007817359430256287049, 0.0009771253907249945886, 0.001172514838424360255, 0.001367904286123725922, 0.001563293733823091806 ),
 .UNSPECIFIED. ) ;
#17820=CARTESIAN_POINT ( 'NONE',  ( 3.903869409797561030, -3.436278759898155677, 33.07459398097509506 ) ) ;
#17821=CARTESIAN_POINT ( 'NONE',  ( -0.6844646790546087267, -6.503392248772476236, 34.64988816332204635 ) ) ;
#17822=ORIENTED_EDGE ( 'NONE', *, *, #58663, .T. ) ;
#17823=CARTESIAN_POINT ( 'NONE',  ( -1.254089682851822873, -10.19071101563364756, 33.96452234770658407 ) ) ;
#17824=EDGE_LOOP ( 'NONE', ( #13808, #75219 ) ) ;
#17825=VERTEX_POINT ( 'NONE', #34285 ) ;
#17826=CARTESIAN_POINT ( 'NONE',  ( 7.846153846153846700, -10.67929555188718282, 33.92786785259544047 ) ) ;
#17828=CARTESIAN_POINT ( 'NONE',  ( -0.5920136466141803222, -7.276987145209185215, 34.99546412871779921 ) ) ;
#17829=CARTESIAN_POINT ( 'NONE',  ( 1.319345384059066317, -11.67786785259541027, 32.92929555188721480 ) ) ;
#17830=CARTESIAN_POINT ( 'NONE',  ( 0.4615384615383396616, -8.613356846316285953, 34.62446782046622218 ) ) ;
#17831=ORIENTED_EDGE ( 'NONE', *, *, #35325, .F. ) ;
#17833=ADVANCED_FACE ( 'NONE', ( #54105 ), #21213, .F. ) ;
#17834=EDGE_LOOP ( 'NONE', ( #23905, #34991 ) ) ;
#17835=AXIS2_PLACEMENT_3D ( 'NONE', #35645, #56354, #64863 ) ;
#17836=CARTESIAN_POINT ( 'NONE',  ( -7.173053667125512511, -12.01397095200673881, 32.43157075238190146 ) ) ;
#17837=CARTESIAN_POINT ( 'NONE',  ( 17.07692307692307665, -3.669653830205710676, 35.88435417666054406 ) ) ;
#17838=B_SPLINE_CURVE_WITH_KNOTS ( 'NONE', 3,
 ( #72682, #79891, #78546, #45655, #38915, #16852, #73593, #11887, #5119, #32584 ),
 .UNSPECIFIED., .F., .F.,
 ( 4, 2, 2, 2, 4 ),
 ( 0.0007817359430256399806, 0.0009771253907250089001, 0.001172514838424378036, 0.001367904286123746956, 0.001563293733823115875 ),
 .UNSPECIFIED. ) ;
#17839=DIRECTION ( 'NONE',  ( -0.000000000000000000, -0.6427876096865404731, -0.7660444431189771253 ) ) ;
#17842=CARTESIAN_POINT ( 'NONE',  ( -8.519176349317316266, -10.06805714834173493, 34.32951233291982618 ) ) ;
#17843=CARTESIAN_POINT ( 'NONE',  ( 11.31553457955469000, -10.77366814457252175, 33.85459836347579454 ) ) ;
#17844=FACE_OUTER_BOUND ( 'NONE', #67573, .T. ) ;
#17845=VERTEX_POINT ( 'NONE', #53673 ) ;
#17846=ORIENTED_EDGE ( 'NONE', *, *, #79994, .T. ) ;
#17848=EDGE_CURVE ( 'NONE', #46179, #64437, #2673, .T. ) ;
#17850=CARTESIAN_POINT ( 'NONE',  ( 2.438484115517093986, -12.38066358083363738, 30.83685684665853444 ) ) ;
#17851=EDGE_LOOP ( 'NONE', ( #89160, #47155 ) ) ;
#17852=DIRECTION ( 'NONE',  ( -0.000000000000000000, 0.7660444431189791237, -0.6427876096865379196 ) ) ;
#17855=VERTEX_POINT ( 'NONE', #41054 ) ;
#17856=LINE ( 'NONE', #37221, #62644 ) ;
#17857=ORIENTED_EDGE ( 'NONE', *, *, #47817, .T. ) ;
#17858=CARTESIAN_POINT ( 'NONE',  ( 2.372947878968333146, -9.442884908240271713, 34.35708131394835618 ) ) ;
#17859=DIRECTION ( 'NONE',  ( 0.000000000000000000, 0.1736481776669275834, 0.9848077530122086864 ) ) ;
#17860=FACE_BOUND ( 'NONE', #27644, .T. ) ;
#17861=CARTESIAN_POINT ( 'NONE',  ( 10.48490790726815547, -7.276988635370452485, 34.74523720219453793 ) ) ;
#17862=CARTESIAN_POINT ( 'NONE',  ( -14.98076923076922995, -2.499999999999998668, 29.75000000000000355 ) ) ;
#17863=EDGE_CURVE ( 'NONE', #70222, #78622, #19886, .T. ) ;
#17864=CYLINDRICAL_SURFACE ( 'NONE', #43802, 0.2499999999999994726 ) ;
#17865=CARTESIAN_POINT ( 'NONE',  ( -0.4615384615384611200, -12.62096338111211580, 30.90682066428153263 ) ) ;
#17866=ORIENTED_EDGE ( 'NONE', *, *, #41453, .F. ) ;
#17867=CARTESIAN_POINT ( 'NONE',  ( -11.31544869436814338, -8.282913670948747864, 34.94150082978203642 ) ) ;
#17870=EDGE_LOOP ( 'NONE', ( #36258, #27106 ) ) ;
#17872=CARTESIAN_POINT ( 'NONE',  ( 12.21153846153845812, -2.499999999999999556, 29.81609845454691765 ) ) ;
#17873=CARTESIAN_POINT ( 'NONE',  ( -15.09997878980228059, -5.496552790871120031, 34.60292014791297532 ) ) ;
#17874=CARTESIAN_POINT ( 'NONE',  ( 11.53846153846141753, -6.026961402154118019, 34.52809138561165270 ) ) ;
#17875=DIRECTION ( 'NONE',  ( 0.000000000000000000, 0.4999999999999985567, 0.8660254037844395958 ) ) ;
#17876=FACE_BOUND ( 'NONE', #34263, .T. ) ;
#17877=CARTESIAN_POINT ( 'NONE',  ( 13.13459216039392885, -2.341070481393819236, 30.72580821765574299 ) ) ;
#17879=EDGE_CURVE ( 'NONE', #39364, #87441, #19923, .T. ) ;
#17880=FACE_OUTER_BOUND ( 'NONE', #75447, .T. ) ;
#17881=CARTESIAN_POINT ( 'NONE',  ( -11.28846153846010303, -7.500000000000155431, 34.75000000000007105 ) ) ;
#17882=CARTESIAN_POINT ( 'NONE',  ( 14.24242230713598723, -11.06231777344662781, 33.60647404775220082 ) ) ;
#17883=CARTESIAN_POINT ( 'NONE',  ( 12.46153846153846168, -1.242168528481310874, 33.36296068462461051 ) ) ;
#17884=CARTESIAN_POINT ( 'NONE',  ( -1.634615384615383027, -7.500000000000001776, 35.00000000000000000 ) ) ;
#17886=ORIENTED_EDGE ( 'NONE', *, *, #23348, .T. ) ;
#17887=CARTESIAN_POINT ( 'NONE',  ( -3.230769230769352962, -9.528491918059723176, 34.59228464037033035 ) ) ;
#17888=CARTESIAN_POINT ( 'NONE',  ( 16.21991348719623360, -12.62096338111211757, 30.90682066428152908 ) ) ;
#17890=CARTESIAN_POINT ( 'NONE',  ( 17.01165307636676260, -8.656820664281497102, 34.87096338111211935 ) ) ;
#17891=CARTESIAN_POINT ( 'NONE',  ( 3.230769230769110045, -6.879047030192662504, 34.71129190930017927 ) ) ;
#17892=FACE_OUTER_BOUND ( 'NONE', #71526, .T. ) ;
#17894=CARTESIAN_POINT ( 'NONE',  ( -15.29603923132555110, -12.70778746994557551, 30.41441678777548319 ) ) ;
#17895=CARTESIAN_POINT ( 'NONE',  ( 18.00000000000000000, -6.189225973068211317, 35.74407628777942847 ) ) ;
#17896=CARTESIAN_POINT ( 'NONE',  ( -7.976844449264155479, -2.845849958028613624, 32.17971566917920967 ) ) ;
#17898=CARTESIAN_POINT ( 'NONE',  ( 14.37294787896832915, -6.026961402152789304, 34.52809138561124769 ) ) ;
#17899=CARTESIAN_POINT ( 'NONE',  ( 1.607395053593452694, -10.23759521482555357, 34.22997729860117033 ) ) ;
#17900=CARTESIAN_POINT ( 'NONE',  ( -18.24997673094235751, -2.779195860258149686, 31.39871582349837453 ) ) ;
#17901=EDGE_CURVE ( 'NONE', #42078, #50903, #36975, .T. ) ;
#17902=DIRECTION ( 'NONE',  ( -0.000000000000000000, -0.9848077530122086864, -0.1736481776669273613 ) ) ;
#17903=ORIENTED_EDGE ( 'NONE', *, *, #34316, .F. ) ;
#17904=CARTESIAN_POINT ( 'NONE',  ( 17.29970274590113632, -12.69155399931963046, 30.53255429739158444 ) ) ;
#17905=CARTESIAN_POINT ( 'NONE',  ( 8.769230769230647482, -11.48612834414049644, 32.76840700105863391 ) ) ;
#17907=AXIS2_PLACEMENT_3D ( 'NONE', #76976, #50370, #58022 ) ;
#17908=EDGE_CURVE ( 'NONE', #58446, #77667, #25185, .T. ) ;
#17909=CARTESIAN_POINT ( 'NONE',  ( -10.61538461538473577, -2.657715359629662544, 31.77849191805970364 ) ) ;
#17910=DIRECTION ( 'NONE',  ( 0.000000000000000000, 0.1736481776669267785, -0.9848077530122087975 ) ) ;
#17911=EDGE_LOOP ( 'NONE', ( #4199, #61139, #59113, #25461 ) ) ;
#17912=CARTESIAN_POINT ( 'NONE',  ( -17.86920955903305597, -6.369690395747425349, 34.87708834333098196 ) ) ;
#17913=CARTESIAN_POINT ( 'NONE',  ( 9.626225312947559232, -12.62096338111211580, 30.90682066428152908 ) ) ;
#17915=ORIENTED_EDGE ( 'NONE', *, *, #15832, .T. ) ;
#17916=CARTESIAN_POINT ( 'NONE',  ( -12.71151520558705172, -9.234221910056348293, 34.70572697212741531 ) ) ;
#17917=CARTESIAN_POINT ( 'NONE',  ( -0.4615384615384611200, -13.75783147151868846, 33.36296068462461051 ) ) ;
#17918=ADVANCED_FACE ( 'NONE', ( #77055 ), #84266, .F. ) ;
#17919=CYLINDRICAL_SURFACE ( 'NONE', #40629, 0.2499999999999994726 ) ;
#17920=CARTESIAN_POINT ( 'NONE',  ( 12.46153846153846168, -2.249999999999998668, 29.75000000000001776 ) ) ;
#17921=ORIENTED_EDGE ( 'NONE', *, *, #39881, .T. ) ;
#17922=CARTESIAN_POINT ( 'NONE',  ( 2.438218009455874302, -12.27024696741798770, 31.24895572276497546 ) ) ;
#17923=CARTESIAN_POINT ( 'NONE',  ( -12.52762084089859584, -2.486705287966279432, 31.30864560766542937 ) ) ;
#17924=CARTESIAN_POINT ( 'NONE',  ( 4.087762742890270751, -9.780366693483667717, 34.19971097300155805 ) ) ;
#17926=ORIENTED_EDGE ( 'NONE', *, *, #65348, .F. ) ;
#17927=ADVANCED_FACE ( 'NONE', ( #946 ), #36074, .F. ) ;
#17928=ORIENTED_EDGE ( 'NONE', *, *, #54075, .T. ) ;
#17929=CARTESIAN_POINT ( 'NONE',  ( -16.15384615384615330, -1.117168528481311540, 33.14645433367849847 ) ) ;
#17930=DIRECTION ( 'NONE',  ( 0.000000000000000000, 1.000000000000000000, 0.000000000000000000 ) ) ;
#17931=ADVANCED_FACE ( 'NONE', ( #85138 ), #22545, .F. ) ;
#17932=B_SPLINE_CURVE_WITH_KNOTS ( 'NONE', 3,
 ( #57847, #77673, #78119, #16421, #49756, #21848, #64587, #29501, #23178, #50640 ),
 .UNSPECIFIED., .F., .F.,
 ( 4, 2, 2, 2, 4 ),
 ( 0.0007817359430256287049, 0.0009771253907249945886, 0.001172514838424360255, 0.001367904286123725922, 0.001563293733823091806 ),
 .UNSPECIFIED. ) ;
#17933=CARTESIAN_POINT ( 'NONE',  ( -9.692307692307814193, -12.70778746994576025, 30.41441678777401236 ) ) ;
#17934=B_SPLINE_CURVE_WITH_KNOTS ( 'NONE', 3,
 ( #41657, #81760, #47511, #69563, #1107, #82202, #28586, #88534, #54711, #40777 ),
 .UNSPECIFIED., .F., .F.,
 ( 4, 2, 2, 2, 4 ),
 ( 0.000000000000000000, 0.0001954311564186865492, 0.0003908623128373730983, 0.0005862934692560596746, 0.0007817246256747461966 ),
 .UNSPECIFIED. ) ;
#17935=AXIS2_PLACEMENT_3D ( 'NONE', #18781, #6594, #80033 ) ;
#17936=LINE ( 'NONE', #85503, #16166 ) ;
#17937=B_SPLINE_CURVE_WITH_KNOTS ( 'NONE', 3,
 ( #78517, #16818, #37082, #85732, #51465, #78965, #17263, #44722, #25355, #46520 ),
 .UNSPECIFIED., .F., .F.,
 ( 4, 2, 2, 2, 4 ),
 ( 0.000000000000000000, 0.0001954339857564062817, 0.0003908679715128125635, 0.0005863019572692188723, 0.0007817359430256251270 ),
 .UNSPECIFIED. ) ;
#17938=EDGE_CURVE ( 'NONE', #29227, #43656, #35629, .T. ) ;
#17939=ORIENTED_EDGE ( 'NONE', *, *, #75008, .T. ) ;
#17940=ORIENTED_EDGE ( 'NONE', *, *, #52253, .F. ) ;
#17941=DIRECTION ( 'NONE',  ( -0.000000000000000000, -0.000000000000000000, -1.000000000000000000 ) ) ;
#17942=ORIENTED_EDGE ( 'NONE', *, *, #38343, .T. ) ;
#17943=DIRECTION ( 'NONE',  ( -0.000000000000000000, 0.9848077530122085754, -0.1736481776669273613 ) ) ;
#17944=EDGE_CURVE ( 'NONE', #86388, #38093, #56335, .T. ) ;
#17945=DIRECTION ( 'NONE',  ( 0.000000000000000000, 0.8660254037844377084, 0.5000000000000015543 ) ) ;
#17946=CARTESIAN_POINT ( 'NONE',  ( -14.30769230769230660, -2.538708090699994813, 30.37095296980875503 ) ) ;
#17947=FACE_OUTER_BOUND ( 'NONE', #81139, .T. ) ;
#17949=ORIENTED_EDGE ( 'NONE', *, *, #50505, .F. ) ;
#17950=ADVANCED_FACE ( 'NONE', ( #50012 ), #28417, .F. ) ;
#17951=EDGE_LOOP ( 'NONE', ( #78749, #10860, #39904, #17311 ) ) ;
#17952=CARTESIAN_POINT ( 'NONE',  ( 8.834486340506796154, -2.625532179533470512, 30.86335684631491105 ) ) ;
#17954=CARTESIAN_POINT ( 'NONE',  ( 18.00000000000000000, -11.91647553114624181, 32.58852847137148245 ) ) ;
#17956=CYLINDRICAL_SURFACE ( 'NONE', #78413, 0.2499999999999997502 ) ;
#17959=DIRECTION ( 'NONE',  ( 0.000000000000000000, 0.000000000000000000, 1.000000000000000000 ) ) ;
#17960=CYLINDRICAL_SURFACE ( 'NONE', #20671, 0.2499999999999993616 ) ;
#17961=CARTESIAN_POINT ( 'NONE',  ( 10.61538461538461675, -3.513871655860378418, 32.76840700105978499 ) ) ;
#17962=FACE_BOUND ( 'NONE', #60979, .T. ) ;
#17964=DIRECTION ( 'NONE',  ( 0.000000000000000000, 0.3420201433256641055, -0.9396926207859100932 ) ) ;
#17966=DIRECTION ( 'NONE',  ( -0.000000000000000000, -0.6427876096865404731, -0.7660444431189770143 ) ) ;
#17967=CARTESIAN_POINT ( 'NONE',  ( 16.85399611801622655, -9.172386477786394821, 34.72672124145550043 ) ) ;
#17968=CARTESIAN_POINT ( 'NONE',  ( -8.638440328263820689, -11.93129842949671726, 32.56571108434900452 ) ) ;
#17969=CARTESIAN_POINT ( 'NONE',  ( -7.846153846153965716, -3.300289026999228881, 32.46337939537708905 ) ) ;
#17970=CARTESIAN_POINT ( 'NONE',  ( 5.207714884747862705, -2.541949514083464479, 30.39797389878540557 ) ) ;
#17971=ORIENTED_EDGE ( 'NONE', *, *, #70707, .T. ) ;
#17973=DIRECTION ( 'NONE',  ( -0.000000000000000000, -0.9396926207859092051, -0.3420201433256662704 ) ) ;
#17977=CYLINDRICAL_SURFACE ( 'NONE', #38957, 0.2499999999999979738 ) ;
#17978=CARTESIAN_POINT ( 'NONE',  ( 1.384615384615264011, -5.941354392335915335, 34.76329471203413846 ) ) ;
#17979=ADVANCED_FACE ( 'NONE', ( #77926 ), #16230, .F. ) ;
#17980=CARTESIAN_POINT ( 'NONE',  ( 16.37685899793954292, -6.460100341425561332, 34.89618726649961644 ) ) ;
#17981=CARTESIAN_POINT ( 'NONE',  ( 14.30769230769262279, -2.255955759149395501, 30.00000000000324363 ) ) ;
#17983=B_SPLINE_CURVE_WITH_KNOTS ( 'NONE', 3,
 ( #42399, #49137, #69857, #7272, #952, #28425, #56343, #63083, #14469, #11935 ),
 .UNSPECIFIED., .F., .F.,
 ( 4, 2, 2, 2, 4 ),
 ( 0.0007817359430256403058, 0.0009771253907250093337, 0.001172514838424378470, 0.001367904286123747606, 0.001563293733823116743 ),
 .UNSPECIFIED. ) ;
#17984=ORIENTED_EDGE ( 'NONE', *, *, #28924, .F. ) ;
#17985=CARTESIAN_POINT ( 'NONE',  ( 8.519207545009312099, -12.68155406624981119, 30.59749803192733708 ) ) ;
#17986=DIRECTION ( 'NONE',  ( -0.000000000000000000, -0.7660444431189791237, -0.6427876096865379196 ) ) ;
#17987=DIRECTION ( 'NONE',  ( 0.000000000000000000, 0.1736481776669267785, -0.9848077530122087975 ) ) ;
#17988=CARTESIAN_POINT ( 'NONE',  ( 14.05771556364371833, -12.65889640711025521, 30.72598325615533454 ) ) ;
#17989=CARTESIAN_POINT ( 'NONE',  ( 7.716006636715626144, -6.001485441113818986, 34.52039167877662607 ) ) ;
#17990=CARTESIAN_POINT ( 'NONE',  ( 0.2386115026316113497, -3.395401636524185474, 33.02366814457250399 ) ) ;
#17991=( NAMED_UNIT ( * ) PLANE_ANGLE_UNIT ( ) SI_UNIT ( $, .RADIAN. ) );
#17992=CARTESIAN_POINT ( 'NONE',  ( -15.09997878980228059, -10.70102852606553157, 33.91149625220312913 ) ) ;
#17994=ORIENTED_EDGE ( 'NONE', *, *, #30633, .T. ) ;
#17995=VERTEX_POINT ( 'NONE', #2257 ) ;
#17996=CARTESIAN_POINT ( 'NONE',  ( -7.976301815885543434, -11.66186481527757302, 32.95055677023626117 ) ) ;
#17997=CARTESIAN_POINT ( 'NONE',  ( 17.32697749683652688, -4.074993327901525575, 33.72946981652012255 ) ) ;
#17998=CARTESIAN_POINT ( 'NONE',  ( 10.68064018666064285, -2.625532179533470512, 30.86335684631491105 ) ) ;
#17999=DIRECTION ( 'NONE',  ( -0.000000000000000000, 0.9396926207859093161, -0.3420201433256663259 ) ) ;
#18000=DIRECTION ( 'NONE',  ( -0.000000000000000000, 0.9396926207859093161, -0.3420201433256663259 ) ) ;
#18002=DIRECTION ( 'NONE',  ( 0.000000000000000000, 0.9396926207859126468, -0.3420201433256571111 ) ) ;
#18003=CARTESIAN_POINT ( 'NONE',  ( -13.51530685128294351, -8.147922237126337563, 34.70805685702651999 ) ) ;
#18004=AXIS2_PLACEMENT_3D ( 'NONE', #28405, #82920, #68949 ) ;
#18005=CARTESIAN_POINT ( 'NONE',  ( -8.899921372341076165, -12.62707690430377383, 30.88035979386743435 ) ) ;
#18006=CARTESIAN_POINT ( 'NONE',  ( 5.869852030268307708, -10.31621877034669588, 34.18098118002070152 ) ) ;
#18007=CARTESIAN_POINT ( 'NONE',  ( -13.38461538461538325, -11.16473453929635440, 33.15142922261926373 ) ) ;
#18008=CARTESIAN_POINT ( 'NONE',  ( -9.822454901745915734, -12.27039167877662251, 31.24851455888617835 ) ) ;
#18009=CARTESIAN_POINT ( 'NONE',  ( 2.177000841024749445, -3.062553014421049991, 32.05460306192774311 ) ) ;
#18010=FACE_OUTER_BOUND ( 'NONE', #13653, .T. ) ;
#18011=B_SPLINE_CURVE_WITH_KNOTS ( 'NONE', 3,
 ( #25202, #45909, #87823, #59872, #80610, #53556, #88705, #25649, #53104, #46807 ),
 .UNSPECIFIED., .F., .F.,
 ( 4, 2, 2, 2, 4 ),
 ( 0.0007817246256747445703, 0.0009771112852218872494, 0.001172497944769030145, 0.001367884604316172825, 0.001563271263863315504 ),
 .UNSPECIFIED. ) ;
#18012=CARTESIAN_POINT ( 'NONE',  ( -5.749945580086545327, -4.818054556918156095, 34.26375889529406749 ) ) ;
#18013=CARTESIAN_POINT ( 'NONE',  ( 11.31553532094539172, -6.503392248772476236, 34.64988816332204635 ) ) ;
#18014=CARTESIAN_POINT ( 'NONE',  ( -1.384615384615383471, -9.780366693483667717, 34.19971097300155094 ) ) ;
#18015=ORIENTED_EDGE ( 'NONE', *, *, #38708, .T. ) ;
#18016=B_SPLINE_CURVE_WITH_KNOTS ( 'NONE', 3,
 ( #65591, #35720, #70833, #48771, #48327, #35262, #15890, #62720, #28969, #49663 ),
 .UNSPECIFIED., .F., .F.,
 ( 4, 2, 2, 2, 4 ),
 ( 0.000000000000000000, 0.0001954339857564090194, 0.0003908679715128180387, 0.0005863019572692270039, 0.0007817359430256360774 ),
 .UNSPECIFIED. ) ;
#18017=CARTESIAN_POINT ( 'NONE',  ( 11.66898724022510159, -11.93748526763465279, 32.05452791011430946 ) ) ;
#18019=CARTESIAN_POINT ( 'NONE',  ( 5.934729999443683290, -2.657715359629089225, 31.77849191805834295 ) ) ;
#18021=EDGE_CURVE ( 'NONE', #38647, #69402, #22002, .T. ) ;
#18022=CARTESIAN_POINT ( 'NONE',  ( -14.30769230769230660, -4.786620604624113540, 33.94971097300155094 ) ) ;
#18023=CARTESIAN_POINT ( 'NONE',  ( 8.769230769230768274, -9.905515769479276145, 34.41647553114623292 ) ) ;
#18024=CARTESIAN_POINT ( 'NONE',  ( 17.07692307692307665, -13.20930481340135110, 34.54067556320372745 ) ) ;
#18025=VERTEX_POINT ( 'NONE', #7717 ) ;
#18027=CARTESIAN_POINT ( 'NONE',  ( 2.557692307692308376, -7.500000000000001776, 35.04278698407183867 ) ) ;
#18028=EDGE_CURVE ( 'NONE', #31229, #10290, #62634, .T. ) ;
#18029=ORIENTED_EDGE ( 'NONE', *, *, #13280, .T. ) ;
#18030=CARTESIAN_POINT ( 'NONE',  ( 17.07692307692307665, -13.37000171582298513, 34.34916445242398453 ) ) ;
#18032=ORIENTED_EDGE ( 'NONE', *, *, #45920, .T. ) ;
#18033=CARTESIAN_POINT ( 'NONE',  ( 1.384615384615264011, -3.083524468854526912, 32.58852847137268327 ) ) ;
#18034=DIRECTION ( 'NONE',  ( -0.000000000000000000, -0.6427876096865404731, -0.7660444431189771253 ) ) ;
#18035=CARTESIAN_POINT ( 'NONE',  ( -0.4615384615384611200, -6.343179335718451384, 34.87096338111211935 ) ) ;
#18037=CARTESIAN_POINT ( 'NONE',  ( -4.153846153846274980, -11.67786785259630911, 32.92929555188603530 ) ) ;
#18038=EDGE_LOOP ( 'NONE', ( #21725, #8776 ) ) ;
#18039=ADVANCED_FACE ( 'NONE', ( #1828 ), #29316, .F. ) ;
#18040=CARTESIAN_POINT ( 'NONE',  ( 11.53846153846153832, -3.513871655860378418, 32.76840700105978499 ) ) ;
#18041=EDGE_LOOP ( 'NONE', ( #62256, #20792, #21039, #38391 ) ) ;
#18042=CARTESIAN_POINT ( 'NONE',  ( 2.057715563643717438, -9.234221910056348293, 34.70572697212741531 ) ) ;
#18043=CYLINDRICAL_SURFACE ( 'NONE', #61365, 0.2500000000000009437 ) ;
#18044=ORIENTED_EDGE ( 'NONE', *, *, #86630, .T. ) ;
#18047=CARTESIAN_POINT ( 'NONE',  ( -1.161835715637319133, -10.97394488606064122, 33.68653795673694873 ) ) ;
#18048=CARTESIAN_POINT ( 'NONE',  ( -14.24243716817946925, -10.33852847137154107, 34.16647553114620450 ) ) ;
#18050=VERTEX_POINT ( 'NONE', #72498 ) ;
#18053=DIRECTION ( 'NONE',  ( 0.000000000000000000, 0.8660254037844377084, 0.5000000000000015543 ) ) ;
#18054=ORIENTED_EDGE ( 'NONE', *, *, #87422, .F. ) ;
#18055=EDGE_CURVE ( 'NONE', #48795, #24566, #459, .T. ) ;
#18056=CARTESIAN_POINT ( 'NONE',  ( 10.61538461538449596, -5.219633306517616589, 34.19971097300220464 ) ) ;
#18057=CARTESIAN_POINT ( 'NONE',  ( 6.000000000000001776, -3.513871655860378418, 32.76840700105978499 ) ) ;
#18059=VECTOR ( 'NONE', #412, 1000.000000000000000 ) ;
#18060=EDGE_CURVE ( 'NONE', #75689, #89174, #74653, .T. ) ;
#18061=VERTEX_POINT ( 'NONE', #78811 ) ;
#18062=LINE ( 'NONE', #2306, #55442 ) ;
#18063=ORIENTED_EDGE ( 'NONE', *, *, #70043, .F. ) ;
#18064=CARTESIAN_POINT ( 'NONE',  ( -12.23811206262367435, -7.630147987733840509, 34.99859428049665411 ) ) ;
#18065=B_SPLINE_CURVE_WITH_KNOTS ( 'NONE', 3,
 ( #43777, #52304, #79795, #45104, #71238, #79344, #11326, #85659, #30703, #58169 ),
 .UNSPECIFIED., .F., .F.,
 ( 4, 2, 2, 2, 4 ),
 ( 0.000000000000000000, 0.0001954311564186867931, 0.0003908623128373735862, 0.0005862934692560603251, 0.0007817246256747471724 ),
 .UNSPECIFIED. ) ;
#18067=EDGE_CURVE ( 'NONE', #51804, #87399, #62806, .T. ) ;
#18068=DIRECTION ( 'NONE',  ( 0.000000000000000000, 0.6427876096865373645, -0.7660444431189797898 ) ) ;
#18069=CARTESIAN_POINT ( 'NONE',  ( 0.3313912521002405076, -5.195881422630166391, 34.18770438780619259 ) ) ;
#18070=FACE_BOUND ( 'NONE', #24678, .T. ) ;
#18071=CARTESIAN_POINT ( 'NONE',  ( -17.99999999999969447, -2.506253911140613244, 30.00000000000320455 ) ) ;
#18072=CARTESIAN_POINT ( 'NONE',  ( -14.30769230769230660, -12.10708131394839349, 31.69288490824020244 ) ) ;
#18074=DIRECTION ( 'NONE',  ( -0.000000000000000000, -0.1736481776669307198, -0.9848077530122080203 ) ) ;
#18075=CARTESIAN_POINT ( 'NONE',  ( 8.992010310499175318, -3.236590943229499029, 32.36255958852954251 ) ) ;
#18076=CARTESIAN_POINT ( 'NONE',  ( -1.449885830576159940, -2.625532179533444754, 30.86335684631481513 ) ) ;
#18078=CARTESIAN_POINT ( 'NONE',  ( -17.14219352288385778, -12.46129190929999986, 30.37095296980880832 ) ) ;
#18079=EDGE_LOOP ( 'NONE', ( #12736, #27067, #82989, #36945 ) ) ;
#18080=EDGE_CURVE ( 'NONE', #39225, #61500, #53087, .T. ) ;
#18081=ORIENTED_EDGE ( 'NONE', *, *, #60861, .F. ) ;
#18082=CARTESIAN_POINT ( 'NONE',  ( -6.923076923077044142, -11.94971097300221174, 32.03036669348237098 ) ) ;
#18083=CARTESIAN_POINT ( 'NONE',  ( 10.86533013373275836, -5.852078868378309373, 34.47109172314383585 ) ) ;
#18084=B_SPLINE_CURVE_WITH_KNOTS ( 'NONE', 3,
 ( #5032, #59080, #66284, #18553, #12681, #86126, #60415, #79812, #73945, #80714 ),
 .UNSPECIFIED., .F., .F.,
 ( 4, 2, 2, 2, 4 ),
 ( 0.0007817359430256294638, 0.0009771253907249948054, 0.001172514838424360255, 0.001367904286123725489, 0.001563293733823090939 ),
 .UNSPECIFIED. ) ;
#18085=CARTESIAN_POINT ( 'NONE',  ( 2.980746006547774218, -3.520140089381496473, 33.17453946501458262 ) ) ;
#18086=CARTESIAN_POINT ( 'NONE',  ( -13.63463860883683942, -2.985938066672154445, 32.43141759479405550 ) ) ;
#18087=EDGE_CURVE ( 'NONE', #19800, #5458, #73536, .T. ) ;
#18088=CARTESIAN_POINT ( 'NONE',  ( -18.00000000000012079, -5.941354392335914447, 34.76329471203413846 ) ) ;
#18089=DIRECTION ( 'NONE',  ( -0.000000000000000000, 0.3420201433256694901, -0.9396926207859082059 ) ) ;
#18090=EDGE_CURVE ( 'NONE', #87089, #81733, #7987, .T. ) ;
#18091=ORIENTED_EDGE ( 'NONE', *, *, #55576, .F. ) ;
#18092=AXIS2_PLACEMENT_3D ( 'NONE', #10575, #86251, #44332 ) ;
#18093=CARTESIAN_POINT ( 'NONE',  ( -5.300408001487407539, -6.716662450894490100, 34.94144148231605840 ) ) ;
#18095=CARTESIAN_POINT ( 'NONE',  ( 10.61538461538461675, -2.833524468853757305, 32.15551576947925838 ) ) ;
#18096=CARTESIAN_POINT ( 'NONE',  ( -13.51476335434707821, -12.70455904226513866, 30.44083106164009322 ) ) ;
#18099=ORIENTED_EDGE ( 'NONE', *, *, #19426, .T. ) ;
#18101=ORIENTED_EDGE ( 'NONE', *, *, #29503, .T. ) ;
#18102=CARTESIAN_POINT ( 'NONE',  ( 11.53846153846153832, -12.34228464037088635, 31.77849191805839268 ) ) ;
#18103=CARTESIAN_POINT ( 'NONE',  ( -6.065753428313330531, -7.249945578846651806, 34.99404164642496795 ) ) ;
#18104=ORIENTED_EDGE ( 'NONE', *, *, #84084, .T. ) ;
#18106=CARTESIAN_POINT ( 'NONE',  ( -7.846153846153844924, -4.098570777380720287, 33.41473453929634729 ) ) ;
#18107=DIRECTION ( 'NONE',  ( 0.000000000000000000, 0.1736481776669267785, -0.9848077530122087975 ) ) ;
#18108=CARTESIAN_POINT ( 'NONE',  ( -8.519285250882628446, -6.696923467548660192, 34.68552623307873972 ) ) ;
#18110=B_SPLINE_CURVE_WITH_KNOTS ( 'NONE', 3,
 ( #37770, #8542, #9417, #65237, #84211, #15743, #22488, #3532, #31005, #29698 ),
 .UNSPECIFIED., .F., .F.,
 ( 4, 2, 2, 2, 4 ),
 ( 0.000000000000000000, 0.0001954339857564054686, 0.0003908679715128109372, 0.0005863019572692163787, 0.0007817359430256218744 ),
 .UNSPECIFIED. ) ;
#18111=DIRECTION ( 'NONE',  ( 0.000000000000000000, 0.000000000000000000, 1.000000000000000000 ) ) ;
#18112=VERTEX_POINT ( 'NONE', #30028 ) ;
#18113=CARTESIAN_POINT ( 'NONE',  ( -14.98071481085577972, -2.318338780012835443, 30.59689888758630261 ) ) ;
#18114=ORIENTED_EDGE ( 'NONE', *, *, #20016, .F. ) ;
#18116=CARTESIAN_POINT ( 'NONE',  ( -12.59168643127016374, -3.069018819979302926, 32.56621877034667278 ) ) ;
#18117=DIRECTION ( 'NONE',  ( 0.000000000000000000, 0.6427876096865373645, -0.7660444431189797898 ) ) ;
#18118=CARTESIAN_POINT ( 'NONE',  ( 15.36129493253279499, -12.45806712695776319, 30.39783852428763922 ) ) ;
#18119=DIRECTION ( 'NONE',  ( 1.000000000000000000, 0.000000000000000000, 0.000000000000000000 ) ) ;
#18123=CARTESIAN_POINT ( 'NONE',  ( -20.74999999999999645, -2.499999999999999556, 27.25000000000000000 ) ) ;
#18124=LINE ( 'NONE', #73960, #10294 ) ;
#18125=DIRECTION ( 'NONE',  ( 0.000000000000000000, 0.9396926207859126468, 0.3420201433256571111 ) ) ;
#18126=ADVANCED_FACE ( 'NONE', ( #70573 ), #14748, .F. ) ;
#18128=ORIENTED_EDGE ( 'NONE', *, *, #28490, .F. ) ;
#18130=DIRECTION ( 'NONE',  ( -0.000000000000000000, 1.000000000000000000, 3.491481338843133355E-15 ) ) ;
#18131=CARTESIAN_POINT ( 'NONE',  ( 11.53846153846153832, -4.661471528628507777, 34.16647553114623292 ) ) ;
#18132=CARTESIAN_POINT ( 'NONE',  ( -0.7115616857599190714, -9.356822207818506598, 34.66110646841856635 ) ) ;
#18133=DIRECTION ( 'NONE',  ( -0.000000000000000000, -0.7660444431189791237, -0.6427876096865379196 ) ) ;
#18134=CARTESIAN_POINT ( 'NONE',  ( -8.992715712954719720, -11.89387501736622710, 32.13663884655806413 ) ) ;
#18135=CYLINDRICAL_SURFACE ( 'NONE', #19188, 0.2499999999999995559 ) ;
#18136=ORIENTED_EDGE ( 'NONE', *, *, #68323, .F. ) ;
#18137=CARTESIAN_POINT ( 'NONE',  ( 9.562160482869472844, -10.88202310037935661, 33.43294751532457099 ) ) ;
#18138=CARTESIAN_POINT ( 'NONE',  ( -2.242436736416282272, -10.21337939537593797, 33.94971097300152252 ) ) ;
#18139=CARTESIAN_POINT ( 'NONE',  ( 9.442330948259105128, -2.544273027872575366, 31.48422191005632342 ) ) ;
#18140=ORIENTED_EDGE ( 'NONE', *, *, #38331, .F. ) ;
#18141=CARTESIAN_POINT ( 'NONE',  ( -7.623142494540996239, -3.587049720035815348, 32.86302985866382897 ) ) ;
#18142=ORIENTED_EDGE ( 'NONE', *, *, #25008, .F. ) ;
#18143=CARTESIAN_POINT ( 'NONE',  ( 13.51514108637895184, -3.816742781228458448, 33.13167719472716044 ) ) ;
#18144=CARTESIAN_POINT ( 'NONE',  ( -13.13461538461396394, -7.500000000000154543, 35.00000000000007105 ) ) ;
#18145=LINE ( 'NONE', #87070, #48446 ) ;
#18147=CARTESIAN_POINT ( 'NONE',  ( 12.23861224402230619, -3.586966769969701208, 32.86292498521069660 ) ) ;
#18148=CARTESIAN_POINT ( 'NONE',  ( 9.692307692307570832, -9.528491918059723176, 34.59228464037033035 ) ) ;
#18150=EDGE_CURVE ( 'NONE', #36240, #46929, #56170, .T. ) ;
#18151=CARTESIAN_POINT ( 'NONE',  ( -5.999999999999998224, -1.129524287112498415, 32.06866353760679544 ) ) ;
#18152=CARTESIAN_POINT ( 'NONE',  ( -5.010855743573000787, -10.67929555188718282, 33.92786785259544757 ) ) ;
#18153=AXIS2_PLACEMENT_3D ( 'NONE', #4135, #30724, #10011 ) ;
#18156=ORIENTED_EDGE ( 'NONE', *, *, #54191, .T. ) ;
#18157=CARTESIAN_POINT ( 'NONE',  ( -15.23076923076935252, -6.835583212225970762, 34.95778746994575670 ) ) ;
#18158=B_SPLINE_CURVE_WITH_KNOTS ( 'NONE', 3,
 ( #79514, #46612, #32216, #11051, #58332, #10606, #17815, #72738, #65982, #4286 ),
 .UNSPECIFIED., .F., .F.,
 ( 4, 2, 2, 2, 4 ),
 ( 0.000000000000000000, 0.0001954339857564079080, 0.0003908679715128158161, 0.0005863019572692237513, 0.0007817359430256316322 ),
 .UNSPECIFIED. ) ;
#18159=DIRECTION ( 'NONE',  ( -0.000000000000000000, -0.8660254037844397068, -0.4999999999999978906 ) ) ;
#18160=DIRECTION ( 'NONE',  ( -0.000000000000000000, -0.8660254037844399289, -0.4999999999999980016 ) ) ;
#18162=EDGE_CURVE ( 'NONE', #60114, #41758, #84217, .T. ) ;
#18164=CARTESIAN_POINT ( 'NONE',  ( -6.249976730942353953, -4.236021600441998380, 33.53823185664189310 ) ) ;
#18165=CARTESIAN_POINT ( 'NONE',  ( 12.52760681254089903, -9.780366693483667717, 34.19971097300155805 ) ) ;
#18167=EDGE_LOOP ( 'NONE', ( #45296, #84808, #754, #43166 ) ) ;
#18168=VERTEX_POINT ( 'NONE', #49417 ) ;
#18169=ORIENTED_EDGE ( 'NONE', *, *, #8622, .T. ) ;
#18171=EDGE_CURVE ( 'NONE', #62161, #54250, #1219, .T. ) ;
#18172=CARTESIAN_POINT ( 'NONE',  ( 17.07692307692307665, -1.629998284177014645, 34.34916445242399163 ) ) ;
#18173=CARTESIAN_POINT ( 'NONE',  ( 6.000000000000001776, -6.435427911321262684, 35.78748833219616898 ) ) ;
#18174=B_SPLINE_CURVE_WITH_KNOTS ( 'NONE', 3,
 ( #8805, #63732, #34928, #62392, #65054, #51528, #71821, #24080, #79028, #71371 ),
 .UNSPECIFIED., .F., .F.,
 ( 4, 2, 2, 2, 4 ),
 ( 0.0007817359430256294638, 0.0009771253907249941549, 0.001172514838424358954, 0.001367904286123723754, 0.001563293733823095492 ),
 .UNSPECIFIED. ) ;
#18176=CARTESIAN_POINT ( 'NONE',  ( -5.750054481651857508, -5.057305518903949526, 34.11320923018887896 ) ) ;
#18177=CARTESIAN_POINT ( 'NONE',  ( 13.25392391794782654, -8.147922237126337563, 34.70805685702651999 ) ) ;
#18178=CARTESIAN_POINT ( 'NONE',  ( 8.703147358274888390, -8.973038597847271092, 34.52809138561120506 ) ) ;
#18179=VECTOR ( 'NONE', #54795, 1000.000000000000114 ) ;
#18180=CARTESIAN_POINT ( 'NONE',  ( -17.86920819217521483, -9.804649428959613999, 34.18742332936588468 ) ) ;
#18181=CARTESIAN_POINT ( 'NONE',  ( 9.627037691751374027, -10.33852847137145048, 34.16647553114627556 ) ) ;
#18182=CARTESIAN_POINT ( 'NONE',  ( 6.923076923076924238, -5.415277668671390821, 36.20867863119892149 ) ) ;
#18183=VERTEX_POINT ( 'NONE', #36778 ) ;
#18184=VERTEX_POINT ( 'NONE', #21941 ) ;
#18187=DIRECTION ( 'NONE',  ( -0.000000000000000000, -0.9396926207859093161, -0.3420201433256663259 ) ) ;
#18188=VERTEX_POINT ( 'NONE', #9749 ) ;
#18189=CARTESIAN_POINT ( 'NONE',  ( -15.93083480223330817, -6.503523203565941380, 34.64991518177335195 ) ) ;
#18190=CARTESIAN_POINT ( 'NONE',  ( 1.384615384615386802, -5.180354513474913603, 36.12317359536750416 ) ) ;
#18191=CARTESIAN_POINT ( 'NONE',  ( 8.638754061114305216, -7.276988635370452485, 34.74523720219453793 ) ) ;
#18194=FACE_BOUND ( 'NONE', #87871, .T. ) ;
#18197=VERTEX_POINT ( 'NONE', #57933 ) ;
#18198=CARTESIAN_POINT ( 'NONE',  ( -16.15384615384615330, -1.629998284177014645, 34.34916445242399163 ) ) ;
#18199=ORIENTED_EDGE ( 'NONE', *, *, #33134, .F. ) ;
#18200=FACE_BOUND ( 'NONE', #11231, .T. ) ;
#18201=FACE_OUTER_BOUND ( 'NONE', #25510, .T. ) ;
#18203=ORIENTED_EDGE ( 'NONE', *, *, #60428, .T. ) ;
#18204=CARTESIAN_POINT ( 'NONE',  ( -1.319360245102545015, -5.941354392334606160, 34.76329471203374055 ) ) ;
#18205=CARTESIAN_POINT ( 'NONE',  ( -6.923076923077045919, -2.379036618888197729, 30.90682066428292885 ) ) ;
#18206=CARTESIAN_POINT ( 'NONE',  ( 14.30769230769218581, -10.33852847137269571, 34.16647553114546554 ) ) ;
#18207=ORIENTED_EDGE ( 'NONE', *, *, #67920, .T. ) ;
#18208=LINE ( 'NONE', #71803, #45725 ) ;
#18209=CARTESIAN_POINT ( 'NONE',  ( 3.230769230769110045, -12.27809138561165270, 31.22303859784587132 ) ) ;
#18210=DIRECTION ( 'NONE',  ( 0.000000000000000000, 0.9396926207859126468, 0.3420201433256571111 ) ) ;
#18211=ORIENTED_EDGE ( 'NONE', *, *, #64092, .T. ) ;
#18212=B_SPLINE_CURVE_WITH_KNOTS ( 'NONE', 3,
 ( #13559, #14904, #75270, #21644, #70280, #14449, #27520, #6799, #76597, #34273 ),
 .UNSPECIFIED., .F., .F.,
 ( 4, 2, 2, 2, 4 ),
 ( 0.000000000000000000, 0.0001954311564186870371, 0.0003908623128373740741, 0.0005862934692560610840, 0.0007817246256747481482 ),
 .UNSPECIFIED. ) ;
#18213=CYLINDRICAL_SURFACE ( 'NONE', #1362, 0.2500000000000012212 ) ;
#18214=CARTESIAN_POINT ( 'NONE',  ( -10.61538461538461320, -12.29105614889573062, 35.45975837776705220 ) ) ;
#18215=B_SPLINE_CURVE_WITH_KNOTS ( 'NONE', 3,
 ( #11660, #87786, #46324, #81901, #31930, #86894, #67491, #20191, #18411, #67046 ),
 .UNSPECIFIED., .F., .F.,
 ( 4, 2, 2, 2, 4 ),
 ( 0.0007817246336856290608, 0.0009771112958940101571, 0.001172497958102391253, 0.001367884620310772350, 0.001563271282519153446 ),
 .UNSPECIFIED. ) ;
#18216=EDGE_LOOP ( 'NONE', ( #66859, #9203, #974, #39477 ) ) ;
#18217=CARTESIAN_POINT ( 'NONE',  ( 18.00000000000000000, -6.386643153685126251, 34.62446782046654192 ) ) ;
#18218=CARTESIAN_POINT ( 'NONE',  ( -10.39260507411620260, -5.114059244376869984, 34.14424750095245287 ) ) ;
#18219=CARTESIAN_POINT ( 'NONE',  ( -10.61538461538461320, -2.708943851104267164, 35.45975837776705220 ) ) ;
#18220=CARTESIAN_POINT ( 'NONE',  ( 15.00728430620490172, -12.69144148231606017, 30.53333754910549303 ) ) ;
#18221=CARTESIAN_POINT ( 'NONE',  ( -7.053552108152643108, -7.276987145209185215, 34.99546412871779211 ) ) ;
#18222=AXIS2_PLACEMENT_3D ( 'NONE', #34279, #81592, #47346 ) ;
#18223=DIRECTION ( 'NONE',  ( 1.000000000000000000, 0.000000000000000000, 0.000000000000000000 ) ) ;
#18224=CARTESIAN_POINT ( 'NONE',  ( -1.634638621908348410, -5.056417327199099532, 34.11270091957321426 ) ) ;
#18225=CARTESIAN_POINT ( 'NONE',  ( 9.915320536401090123, -4.762714258010881885, 34.23016756924214832 ) ) ;
#18226=CARTESIAN_POINT ( 'NONE',  ( 10.83839745947800992, -9.172514111537584114, 34.72667873470787470 ) ) ;
#18227=CARTESIAN_POINT ( 'NONE',  ( -15.23076923076935252, -2.657715359629662544, 31.77849191805970364 ) ) ;
#18228=CARTESIAN_POINT ( 'NONE',  ( 12.33084785842815378, -4.684245665217972032, 34.18127051446801090 ) ) ;
#18230=ORIENTED_EDGE ( 'NONE', *, *, #88361, .F. ) ;
#18231=CARTESIAN_POINT ( 'NONE',  ( 17.93391658904412012, -4.098570777380720287, 33.41473453929634729 ) ) ;
#18232=ORIENTED_EDGE ( 'NONE', *, *, #78435, .T. ) ;
#18233=EDGE_LOOP ( 'NONE', ( #31160, #71104, #85666, #72042 ) ) ;
#18234=DIRECTION ( 'NONE',  ( 0.000000000000000000, 0.1736481776669267785, -0.9848077530122087975 ) ) ;
#18235=AXIS2_PLACEMENT_3D ( 'NONE', #14699, #34526, #64524 ) ;
#18237=CARTESIAN_POINT ( 'NONE',  ( -5.777220331021931443, -10.23759521482555357, 34.22997729860117033 ) ) ;
#18239=DIRECTION ( 'NONE',  ( 0.000000000000000000, 0.4999999999999985567, 0.8660254037844395958 ) ) ;
#18240=CARTESIAN_POINT ( 'NONE',  ( 6.000000000000001776, -11.16473453929635440, 33.15142922261926373 ) ) ;
#18241=CARTESIAN_POINT ( 'NONE',  ( -15.23076923076922995, -1.242168528481310874, 33.36296068462461051 ) ) ;
#18243=DIRECTION ( 'NONE',  ( -0.000000000000000000, 0.1736481776669307198, -0.9848077530122080203 ) ) ;
#18244=CARTESIAN_POINT ( 'NONE',  ( 7.846153846153846700, -2.486705287966279876, 31.30864560766543647 ) ) ;
#18245=CARTESIAN_POINT ( 'NONE',  ( -7.623142494540995351, -12.15243808032446005, 31.58219941686247978 ) ) ;
#18247=CARTESIAN_POINT ( 'NONE',  ( 5.076923076923075762, -2.833524468853757305, 32.15551576947925838 ) ) ;
#18248=CARTESIAN_POINT ( 'NONE',  ( 12.46153846153833911, -5.219633306517616589, 34.19971097300220464 ) ) ;
#18249=CARTESIAN_POINT ( 'NONE',  ( 5.777073041093149897, -3.395401636524186362, 33.02366814457250399 ) ) ;
#18251=ORIENTED_EDGE ( 'NONE', *, *, #77562, .T. ) ;
#18252=VECTOR ( 'NONE', #42580, 1000.000000000000227 ) ;
#18253=CARTESIAN_POINT ( 'NONE',  ( 7.846153846153846700, -13.20930481340135110, 34.54067556320372745 ) ) ;
#18254=CARTESIAN_POINT ( 'NONE',  ( 7.846153846153846700, -11.16473453929635440, 33.15142922261926373 ) ) ;
#18255=CARTESIAN_POINT ( 'NONE',  ( 1.318533005255250412, -10.67929555188718460, 33.92786785259543336 ) ) ;
#18256=CARTESIAN_POINT ( 'NONE',  ( -10.61538461538461320, -11.91647553114624181, 32.58852847137148245 ) ) ;
#18257=CARTESIAN_POINT ( 'NONE',  ( -17.07692307692319744, -9.442884908241554243, 34.35708131394783038 ) ) ;
#18258=CARTESIAN_POINT ( 'NONE',  ( -9.758390071667825794, -6.343179335718451384, 34.87096338111212646 ) ) ;
#18259=ADVANCED_FACE ( 'NONE', ( #16508 ), #43974, .F. ) ;
#18261=AXIS2_PLACEMENT_3D ( 'NONE', #5278, #53452, #75074 ) ;
#18262=ORIENTED_EDGE ( 'NONE', *, *, #78997, .T. ) ;
#18263=CARTESIAN_POINT ( 'NONE',  ( -10.86538461538461497, -7.566082377512564960, 35.00000000000000711 ) ) ;
#18264=VERTEX_POINT ( 'NONE', #28703 ) ;
#18265=ORIENTED_EDGE ( 'NONE', *, *, #48482, .F. ) ;
#18266=CARTESIAN_POINT ( 'NONE',  ( -9.561517251340744039, -2.845873456487965747, 32.17976146951972538 ) ) ;
#18267=EDGE_CURVE ( 'NONE', #572, #78341, #4771, .T. ) ;
#18269=CARTESIAN_POINT ( 'NONE',  ( 11.66898724022510514, -10.88167719472716399, 33.43325721877153711 ) ) ;
#18271=FACE_OUTER_BOUND ( 'NONE', #7613, .T. ) ;
#18272=CARTESIAN_POINT ( 'NONE',  ( 13.25392478150507891, -5.496505350115501010, 34.60290016733514307 ) ) ;
#18273=VERTEX_POINT ( 'NONE', #22818 ) ;
#18274=ORIENTED_EDGE ( 'NONE', *, *, #42232, .T. ) ;
#18275=EDGE_LOOP ( 'NONE', ( #45008, #72644, #62771, #34774, #58454, #9637 ) ) ;
#18277=CARTESIAN_POINT ( 'NONE',  ( -5.999999999999998224, -8.973038597847269315, 34.52809138561121927 ) ) ;
#18278=CARTESIAN_POINT ( 'NONE',  ( -14.30769230769230660, -2.499999999999998668, 29.75000000000001421 ) ) ;
#18279=CARTESIAN_POINT ( 'NONE',  ( 16.21910129335899597, -5.941354392334603496, 34.76329471203374055 ) ) ;
#18280=CARTESIAN_POINT ( 'NONE',  ( 2.084766090176162212, -11.24512374952581872, 33.06303171183252942 ) ) ;
#18281=CARTESIAN_POINT ( 'NONE',  ( -4.284456513470680683, -7.722926236386453702, 34.74524107206102030 ) ) ;
#18282=CARTESIAN_POINT ( 'NONE',  ( 5.776515056276055660, -12.44517049084099725, 30.48991314939691932 ) ) ;
#18283=VECTOR ( 'NONE', #11252, 1000.000000000000227 ) ;
#18284=VERTEX_POINT ( 'NONE', #66017 ) ;
#18288=ORIENTED_EDGE ( 'NONE', *, *, #16771, .T. ) ;
#18289=FACE_OUTER_BOUND ( 'NONE', #37199, .T. ) ;
#18290=CARTESIAN_POINT ( 'NONE',  ( -9.757578138268469203, -11.94971097300153140, 32.03036669348370680 ) ) ;
#18292=ADVANCED_FACE ( 'NONE', ( #11986 ), #71892, .F. ) ;
#18293=ORIENTED_EDGE ( 'NONE', *, *, #27286, .T. ) ;
#18294=EDGE_CURVE ( 'NONE', #273, #19105, #10188, .T. ) ;
#18295=LINE ( 'NONE', #44862, #67026 ) ;
#18296=B_SPLINE_CURVE_WITH_KNOTS ( 'NONE', 3,
 ( #2313, #23914, #51364, #78868, #17167, #35686, #38333, #65790, #10422, #87430 ),
 .UNSPECIFIED., .F., .F.,
 ( 4, 2, 2, 2, 4 ),
 ( 0.000000000000000000, 0.0001954339857564097512, 0.0003908679715128195024, 0.0005863019572692292807, 0.0007817359430256390048 ),
 .UNSPECIFIED. ) ;
#18298=CARTESIAN_POINT ( 'NONE',  ( 2.438218009455872970, -9.417988943895561960, 34.36773134775778260 ) ) ;
#18299=FACE_OUTER_BOUND ( 'NONE', #64209, .T. ) ;
#18300=CARTESIAN_POINT ( 'NONE',  ( -12.21148414990014963, -12.41262288849542017, 30.68299917996395010 ) ) ;
#18301=DIRECTION ( 'NONE',  ( -0.000000000000000000, -0.6427876096865404731, -0.7660444431189770143 ) ) ;
#18303=EDGE_CURVE ( 'NONE', #87005, #62924, #5887, .T. ) ;
#18304=B_SPLINE_CURVE_WITH_KNOTS ( 'NONE', 3,
 ( #74853, #12696, #5045, #19889, #32511, #13140, #75287, #34290, #59988, #67202 ),
 .UNSPECIFIED., .F., .F.,
 ( 4, 2, 2, 2, 4 ),
 ( 0.0007817359430256294638, 0.0009771253907249941549, 0.001172514838424358954, 0.001367904286123723754, 0.001563293733823095492 ),
 .UNSPECIFIED. ) ;
#18305=AXIS2_PLACEMENT_3D ( 'NONE', #31012, #17517, #72447 ) ;
#18307=ORIENTED_EDGE ( 'NONE', *, *, #24435, .T. ) ;
#18308=EDGE_CURVE ( 'NONE', #79391, #59502, #42429, .T. ) ;
#18309=DIRECTION ( 'NONE',  ( -0.000000000000000000, 0.7660444431189791237, -0.6427876096865379196 ) ) ;
#18310=CARTESIAN_POINT ( 'NONE',  ( 4.153846153846154188, -8.120952969808772792, 34.71129190930000163 ) ) ;
#18311=CARTESIAN_POINT ( 'NONE',  ( -11.53846153846153655, -13.53365097954675988, 30.81389545987213552 ) ) ;
#18316=CARTESIAN_POINT ( 'NONE',  ( 10.36540788444226280, -11.79746400365624659, 32.30657167506340954 ) ) ;
#18317=FACE_BOUND ( 'NONE', #42741, .T. ) ;
#18318=CARTESIAN_POINT ( 'NONE',  ( 12.23805351781451201, -3.236172620538810385, 32.36188796281390267 ) ) ;
#18319=DIRECTION ( 'NONE',  ( -0.000000000000000000, -0.7660444431189792347, -0.6427876096865379196 ) ) ;
#18321=CARTESIAN_POINT ( 'NONE',  ( -14.98071481085577972, -4.818054556918156983, 34.26375889529406749 ) ) ;
#18322=CARTESIAN_POINT ( 'NONE',  ( 3.164685819813350065, -4.098570777380720287, 33.41473453929634729 ) ) ;
#18323=CARTESIAN_POINT ( 'NONE',  ( 14.08476534878546360, -10.77366814457252175, 33.85459836347579454 ) ) ;
#18324=CARTESIAN_POINT ( 'NONE',  ( 16.08776274289027342, -10.51840700105979565, 33.73612834413961536 ) ) ;
#18325=CARTESIAN_POINT ( 'NONE',  ( 13.13463864056679853, -2.544273027872575366, 31.48422191005632342 ) ) ;
#18328=VERTEX_POINT ( 'NONE', #52944 ) ;
#18329=CARTESIAN_POINT ( 'NONE',  ( 0.3313912521002404521, -6.852621066184267029, 34.70813303252209181 ) ) ;
#18330=CARTESIAN_POINT ( 'NONE',  ( 16.28463659481310444, -12.62708834333097663, 30.88030960425256310 ) ) ;
#18331=CARTESIAN_POINT ( 'NONE',  ( -1.134669866267242089, -10.76462480002816235, 33.53768742498949962 ) ) ;
#18332=CARTESIAN_POINT ( 'NONE',  ( -2.531177251416254936, -11.89387501736622710, 32.13663884655806413 ) ) ;
#18333=CARTESIAN_POINT ( 'NONE',  ( -10.36543920600657209, -12.07971442181322175, 32.31769673815850297 ) ) ;
#18334=CARTESIAN_POINT ( 'NONE',  ( 1.134592160393927740, -12.07920672191015221, 32.31858351112116168 ) ) ;
#18336=CARTESIAN_POINT ( 'NONE',  ( 2.057669070399343880, -11.86270091957321249, 32.19358267280087915 ) ) ;
#18337=CARTESIAN_POINT ( 'NONE',  ( -2.241624974342230736, -6.343179335718452272, 34.87096338111212646 ) ) ;
#18338=CARTESIAN_POINT ( 'NONE',  ( -12.46153846153858424, -9.528491918059723176, 34.59228464037033035 ) ) ;
#18339=CARTESIAN_POINT ( 'NONE',  ( 9.442330948259105128, -4.075325502946081535, 33.72974371597206300 ) ) ;
#18340=CARTESIAN_POINT ( 'NONE',  ( 0.2115152242454953757, -11.37209801155882971, 32.91403422569032955 ) ) ;
#18341=CARTESIAN_POINT ( 'NONE',  ( -5.076923076923075762, -9.819645486525091727, 36.12317359536749706 ) ) ;
#18342=ADVANCED_FACE ( 'NONE', ( #18289 ), #66478, .F. ) ;
#18343=AXIS2_PLACEMENT_3D ( 'NONE', #48308, #50077, #15872 ) ;
#18344=CARTESIAN_POINT ( 'NONE',  ( -2.084316821919886209, -2.251407671071270489, 29.88021292934942252 ) ) ;
#18345=B_SPLINE_CURVE_WITH_KNOTS ( 'NONE', 3,
 ( #20525, #39929, #40809, #48430, #47990, #260, #61947, #40370, #34485, #27722 ),
 .UNSPECIFIED., .F., .F.,
 ( 4, 2, 2, 2, 4 ),
 ( 0.000000000000000000, 0.0001954339857564054957, 0.0003908679715128109914, 0.0005863019572692164871, 0.0007817359430256219828 ),
 .UNSPECIFIED. ) ;
#18347=EDGE_LOOP ( 'NONE', ( #63660, #73135, #26880, #83535 ) ) ;
#18348=B_SPLINE_CURVE_WITH_KNOTS ( 'NONE', 3,
 ( #16539, #85894, #4360, #52094, #57968, #37244, #3462, #44006, #38143, #23728 ),
 .UNSPECIFIED., .F., .F.,
 ( 4, 2, 2, 2, 4 ),
 ( 0.0007817359430256315238, 0.0009771253907249976244, 0.001172514838424363508, 0.001367904286123729392, 0.001563293733823095492 ),
 .UNSPECIFIED. ) ;
#18349=CARTESIAN_POINT ( 'NONE',  ( 17.32697738856139580, -2.779044189368097051, 31.39831045268885745 ) ) ;
#18350=LINE ( 'NONE', #80503, #54688 ) ;
#18353=B_SPLINE_CURVE_WITH_KNOTS ( 'NONE', 3,
 ( #17442, #44897, #72372, #38150, #65608, #31396, #25082, #53434, #60636, #12460 ),
 .UNSPECIFIED., .F., .F.,
 ( 4, 2, 2, 2, 4 ),
 ( 0.0007817246256747452209, 0.0009771112852218889842, 0.001172497944769032747, 0.001367884604316176294, 0.001563271263863320057 ),
 .UNSPECIFIED. ) ;
#18354=CARTESIAN_POINT ( 'NONE',  ( -10.68065461594093435, -2.657715359629089225, 31.77849191805832874 ) ) ;
#18355=CARTESIAN_POINT ( 'NONE',  ( -16.21992853320628925, -10.67929555188718460, 33.92786785259543336 ) ) ;
#18356=ORIENTED_EDGE ( 'NONE', *, *, #72984, .F. ) ;
#18357=LINE ( 'NONE', #45817, #15497 ) ;
#18360=ORIENTED_EDGE ( 'NONE', *, *, #67448, .F. ) ;
#18362=CARTESIAN_POINT ( 'NONE',  ( -4.153846153846152411, -11.11383981884818262, 36.00935417666054406 ) ) ;
#18363=FACE_OUTER_BOUND ( 'NONE', #39711, .T. ) ;
#18364=ADVANCED_FACE ( 'NONE', ( #25491 ), #39019, .F. ) ;
#18365=CARTESIAN_POINT ( 'NONE',  ( -11.78848476268299628, -2.588893531581426988, 31.60682220781847818 ) ) ;
#18366=ORIENTED_EDGE ( 'NONE', *, *, #65892, .T. ) ;
#18367=CYLINDRICAL_SURFACE ( 'NONE', #73509, 0.2499999999999997502 ) ;
#18368=CARTESIAN_POINT ( 'NONE',  ( 10.68063975489745232, -4.320704448112861584, 33.92786785259548310 ) ) ;
#18369=CARTESIAN_POINT ( 'NONE',  ( 9.692307692307695177, -13.63283147151868846, 33.57946703557072254 ) ) ;
#18371=ORIENTED_EDGE ( 'NONE', *, *, #22379, .F. ) ;
#18372=ORIENTED_EDGE ( 'NONE', *, *, #73270, .F. ) ;
#18373=EDGE_CURVE ( 'NONE', #1790, #31437, #45758, .T. ) ;
#18374=AXIS2_PLACEMENT_3D ( 'NONE', #78011, #16315, #43781 ) ;
#18375=CYLINDRICAL_SURFACE ( 'NONE', #51283, 0.2499999999999995559 ) ;
#18376=CARTESIAN_POINT ( 'NONE',  ( -3.230769230769352962, -3.083524468854526912, 32.58852847137268327 ) ) ;
#18377=EDGE_CURVE ( 'NONE', #73835, #32057, #56281, .T. ) ;
#18378=CARTESIAN_POINT ( 'NONE',  ( -18.00000000000000000, -9.905515769479279697, 34.41647553114623292 ) ) ;
#18379=VECTOR ( 'NONE', #76933, 1000.000000000000000 ) ;
#18381=ORIENTED_EDGE ( 'NONE', *, *, #31288, .F. ) ;
#18382=EDGE_CURVE ( 'NONE', #10219, #51322, #64889, .T. ) ;
#18383=EDGE_LOOP ( 'NONE', ( #11438, #75957, #72623, #27246 ) ) ;
#18384=CARTESIAN_POINT ( 'NONE',  ( -1.384615384615383471, -4.786620604624113540, 33.94971097300155094 ) ) ;
#18385=ORIENTED_EDGE ( 'NONE', *, *, #43998, .T. ) ;
#18386=CARTESIAN_POINT ( 'NONE',  ( -5.143005456283209931, -2.486705287966279432, 31.30864560766542937 ) ) ;
#18387=CARTESIAN_POINT ( 'NONE',  ( -3.230769230769229949, -4.661471528628507777, 34.16647553114623292 ) ) ;
#18388=EDGE_CURVE ( 'NONE', #81411, #25475, #28360, .T. ) ;
#18389=CARTESIAN_POINT ( 'NONE',  ( 7.846153846153846700, -2.708943851104267164, 35.45975837776705220 ) ) ;
#18390=CARTESIAN_POINT ( 'NONE',  ( 13.60762822870878352, -10.01129605718032600, 34.36064277460058491 ) ) ;
#18391=EDGE_CURVE ( 'NONE', #66561, #62271, #66004, .T. ) ;
#18392=ORIENTED_EDGE ( 'NONE', *, *, #14932, .T. ) ;
#18393=EDGE_LOOP ( 'NONE', ( #65656, #87690 ) ) ;
#18395=CARTESIAN_POINT ( 'NONE',  ( 8.835299120233207404, -2.538708090699994813, 30.37095296980875503 ) ) ;
#18397=CYLINDRICAL_SURFACE ( 'NONE', #8667, 0.2499999999999986955 ) ;
#18399=CARTESIAN_POINT ( 'NONE',  ( 12.21156173059610772, -11.28823185664190376, 33.01397839955799896 ) ) ;
#18400=EDGE_CURVE ( 'NONE', #26040, #72902, #65107, .T. ) ;
#18402=DIRECTION ( 'NONE',  ( 0.000000000000000000, -1.000000000000000000, -0.000000000000000000 ) ) ;
#18403=CYLINDRICAL_SURFACE ( 'NONE', #55456, 0.2499999999999979738 ) ;
#18404=FACE_BOUND ( 'NONE', #27345, .T. ) ;
#18405=CARTESIAN_POINT ( 'NONE',  ( -0.5916856709766815658, -4.460286881179644780, 33.72017969459903242 ) ) ;
#18406=CARTESIAN_POINT ( 'NONE',  ( -1.134669866267240979, -11.86320923018887719, 32.19269448109604781 ) ) ;
#18407=EDGE_CURVE ( 'NONE', #63342, #84095, #64881, .T. ) ;
#18408=CARTESIAN_POINT ( 'NONE',  ( -8.992715712954719720, -4.386631170607603991, 33.66268669641500111 ) ) ;
#18409=CARTESIAN_POINT ( 'NONE',  ( 16.37685899793955002, -4.026326845037969449, 33.68677907613345468 ) ) ;
#18410=CARTESIAN_POINT ( 'NONE',  ( 15.29602437028207085, -10.33852847137154107, 34.16647553114620450 ) ) ;
#18411=CARTESIAN_POINT ( 'NONE',  ( -4.403846153846151523, -7.433932668274256805, 35.00000000000000711 ) ) ;
#18413=VERTEX_POINT ( 'NONE', #10402 ) ;
#18415=AXIS2_PLACEMENT_3D ( 'NONE', #15154, #28213, #55681 ) ;
#18416=CARTESIAN_POINT ( 'NONE',  ( 11.47237812750566022, -3.050289026998445951, 32.03036669348365706 ) ) ;
#18417=CYLINDRICAL_SURFACE ( 'NONE', #486, 0.2499999999999994726 ) ;
#18418=VERTEX_POINT ( 'NONE', #4069 ) ;
#18419=ORIENTED_EDGE ( 'NONE', *, *, #81201, .T. ) ;
#18420=CARTESIAN_POINT ( 'NONE',  ( 23.00000000000000000, -9.499999999999982236, 27.74999999999999645 ) ) ;
#18422=CARTESIAN_POINT ( 'NONE',  ( 18.00000000000000000, -1.466349020453238561, 30.81389545987213907 ) ) ;
#18423=CARTESIAN_POINT ( 'NONE',  ( 16.02369894440793630, -3.817052484675422797, 33.13202310037935661 ) ) ;
#18424=CARTESIAN_POINT ( 'NONE',  ( -11.66915214157184622, -9.929715669179220328, 34.40415004197138416 ) ) ;
#18425=ORIENTED_EDGE ( 'NONE', *, *, #56684, .T. ) ;
#18427=CARTESIAN_POINT ( 'NONE',  ( 4.284636594813102661, -4.684288915650984819, 34.18129842949671371 ) ) ;
#18429=CARTESIAN_POINT ( 'NONE',  ( 16.15384615384615330, -13.87047571288749737, 32.06866353760679544 ) ) ;
#18430=CARTESIAN_POINT ( 'NONE',  ( -17.07692307692307665, -9.584722331328613620, 36.20867863119891439 ) ) ;
#18431=CARTESIAN_POINT ( 'NONE',  ( -5.207070286361298095, -9.418419913701741919, 34.36755862841477693 ) ) ;
#18432=( LENGTH_UNIT ( ) NAMED_UNIT ( * ) SI_UNIT ( .MILLI., .METRE. ) );
#18433=CARTESIAN_POINT ( 'NONE',  ( -15.00798956179116317, -10.97394488606064122, 33.68653795673694873 ) ) ;
#18436=VERTEX_POINT ( 'NONE', #12946 ) ;
#18437=EDGE_LOOP ( 'NONE', ( #87484, #68449, #37320, #81369 ) ) ;
#18438=AXIS2_PLACEMENT_3D ( 'NONE', #85885, #51622, #79126 ) ;
#18439=DIRECTION ( 'NONE',  ( 0.000000000000000000, 0.000000000000000000, 1.000000000000000000 ) ) ;
#18441=CARTESIAN_POINT ( 'NONE',  ( -2.307692307692305711, -6.681629849574314051, 35.83090037661290239 ) ) ;
#18442=CARTESIAN_POINT ( 'NONE',  ( 4.377222094544336528, -2.501478030877322567, 29.88021232661720816 ) ) ;
#18443=B_SPLINE_CURVE_WITH_KNOTS ( 'NONE', 3,
 ( #23983, #17693, #64971, #70870, #30313, #44243, #31191, #78939, #3719, #78489 ),
 .UNSPECIFIED., .F., .F.,
 ( 4, 2, 2, 2, 4 ),
 ( 0.0007817359430256215491, 0.0009771253907249856981, 0.001172514838424349847, 0.001367904286123713779, 0.001563293733823077928 ),
 .UNSPECIFIED. ) ;
#18444=CARTESIAN_POINT ( 'NONE',  ( -16.40386939113912135, -2.823816976329320827, 31.52131813110797154 ) ) ;
#18445=CARTESIAN_POINT ( 'NONE',  ( -0.6850233861027902327, -12.11044203135681840, 32.26167407432752299 ) ) ;
#18447=CARTESIAN_POINT ( 'NONE',  ( 22.75000000000000000, -4.499999999999999112, 27.25000000000000000 ) ) ;
#18448=FACE_OUTER_BOUND ( 'NONE', #2403, .T. ) ;
#18449=AXIS2_PLACEMENT_3D ( 'NONE', #1192, #42637, #1648 ) ;
#18450=DIRECTION ( 'NONE',  ( -0.000000000000000000, -0.5000000000000009992, -0.8660254037844380415 ) ) ;
#18451=CARTESIAN_POINT ( 'NONE',  ( 12.23861150263161157, -11.43668979543634734, 33.22377378376089752 ) ) ;
#18452=CARTESIAN_POINT ( 'NONE',  ( -9.758391103263569732, -11.16473453929635440, 33.15142922261925662 ) ) ;
#18453=CARTESIAN_POINT ( 'NONE',  ( 13.38461538461538680, -4.098570777380720287, 33.41473453929634729 ) ) ;
#18455=EDGE_CURVE ( 'NONE', #47638, #46856, #7958, .T. ) ;
#18456=DIRECTION ( 'NONE',  ( -0.000000000000000000, 0.9396926207859092051, -0.3420201433256662704 ) ) ;
#18457=CARTESIAN_POINT ( 'NONE',  ( -6.222926217516146608, -9.886141570436013382, 34.14413921362392301 ) ) ;
#18458=AXIS2_PLACEMENT_3D ( 'NONE', #52357, #53696, #81184 ) ;
#18459=CARTESIAN_POINT ( 'NONE',  ( -15.29603967673000575, -8.613356846314824011, 34.62446782046655613 ) ) ;
#18460=ORIENTED_EDGE ( 'NONE', *, *, #84199, .T. ) ;
#18461=CARTESIAN_POINT ( 'NONE',  ( 8.834485908743605620, -5.094484230520773593, 34.41647553114626845 ) ) ;
#18462=ADVANCED_FACE ( 'NONE', ( #19705 ), #51802, .F. ) ;
#18463=DIRECTION ( 'NONE',  ( 0.000000000000000000, 0.000000000000000000, -1.000000000000000000 ) ) ;
#18464=CARTESIAN_POINT ( 'NONE',  ( 5.076923076923075762, -2.721908614388771852, 31.22303859784724978 ) ) ;
#18467=CARTESIAN_POINT ( 'NONE',  ( 0.3313904918067658856, -5.915902021225892149, 34.75552854090298638 ) ) ;
#18468=CARTESIAN_POINT ( 'NONE',  ( 14.24160992833217065, -4.661471528628507777, 34.16647553114621871 ) ) ;
#18469=CARTESIAN_POINT ( 'NONE',  ( -17.99999999841483955, -2.249999999999995115, 29.50000000010503953 ) ) ;
#18472=CARTESIAN_POINT ( 'NONE',  ( 17.93472955403921887, -3.835265460703609186, 33.15142922261924241 ) ) ;
#18473=ORIENTED_EDGE ( 'NONE', *, *, #7328, .T. ) ;
#18474=EDGE_CURVE ( 'NONE', #83657, #9985, #24049, .T. ) ;
#18475=CARTESIAN_POINT ( 'NONE',  ( -6.000000000000121680, -11.67786785259630911, 32.92929555188603530 ) ) ;
#18476=ORIENTED_EDGE ( 'NONE', *, *, #12287, .F. ) ;
#18477=CARTESIAN_POINT ( 'NONE',  ( 3.230769230769231726, -4.661471528628507777, 34.16647553114623292 ) ) ;
#18478=CARTESIAN_POINT ( 'NONE',  ( -15.48079245499068435, -2.985938066672154445, 32.43141759479405550 ) ) ;
#18479=DIRECTION ( 'NONE',  ( -0.000000000000000000, 1.000000000000000000, 3.491481338843133355E-15 ) ) ;
#18480=ORIENTED_EDGE ( 'NONE', *, *, #19694, .T. ) ;
#18481=CYLINDRICAL_SURFACE ( 'NONE', #19161, 0.2500000000000009437 ) ;
#18482=EDGE_LOOP ( 'NONE', ( #52711, #64929 ) ) ;
#18483=CARTESIAN_POINT ( 'NONE',  ( 13.16174912155229038, -2.251424796025574881, 29.88072029997477586 ) ) ;
#18484=B_SPLINE_CURVE_WITH_KNOTS ( 'NONE', 3,
 ( #49173, #37423, #55928, #76653, #83867, #22153, #2303, #57263, #30669, #44614 ),
 .UNSPECIFIED., .F., .F.,
 ( 4, 2, 2, 2, 4 ),
 ( 0.0007817359430256303312, 0.0009771253907249965402, 0.001172514838424362641, 0.001367904286123728958, 0.001563293733823095059 ),
 .UNSPECIFIED. ) ;
#18487=CARTESIAN_POINT ( 'NONE',  ( -0.5268089074992375886, -3.300289026998414865, 32.46337939537583139 ) ) ;
#18488=DIRECTION ( 'NONE',  ( 0.000000000000000000, 0.3420201433256610524, 0.9396926207859113145 ) ) ;
#18489=B_SPLINE_CURVE_WITH_KNOTS ( 'NONE', 3,
 ( #24744, #85562, #79251, #77911, #79697, #23835, #43681, #51290, #58512, #44110 ),
 .UNSPECIFIED., .F., .F.,
 ( 4, 2, 2, 2, 4 ),
 ( 0.0007817359430256364027, 0.0009771253907250043464, 0.001172514838424372399, 0.001367904286123740234, 0.001563293733823108286 ),
 .UNSPECIFIED. ) ;
#18490=CARTESIAN_POINT ( 'NONE',  ( -10.36543909703647159, -6.696923467548660192, 34.68552623307873972 ) ) ;
#18491=DIRECTION ( 'NONE',  ( -0.000000000000000000, 1.000000000000000000, 3.491481338843133355E-15 ) ) ;
#18492=CARTESIAN_POINT ( 'NONE',  ( 15.16468581981335184, -6.386643153685125363, 34.62446782046654903 ) ) ;
#18493=ADVANCED_FACE ( 'NONE', ( #76867 ), #41756, .F. ) ;
#18494=CARTESIAN_POINT ( 'NONE',  ( 12.52760681254089903, -4.786620604624113540, 33.94971097300155805 ) ) ;
#18495=CARTESIAN_POINT ( 'NONE',  ( 5.011652630962299959, -9.442884908240170461, 34.35708131394840592 ) ) ;
#18496=ORIENTED_EDGE ( 'NONE', *, *, #75516, .F. ) ;
#18497=VERTEX_POINT ( 'NONE', #56145 ) ;
#18498=VERTEX_POINT ( 'NONE', #757 ) ;
#18499=CARTESIAN_POINT ( 'NONE',  ( -14.30769230769230660, -8.120952969808772792, 34.71129190930000163 ) ) ;
#18500=VERTEX_POINT ( 'NONE', #42201 ) ;
#18502=FACE_OUTER_BOUND ( 'NONE', #13684, .T. ) ;
#18503=CARTESIAN_POINT ( 'NONE',  ( 1.607626736228234599, -2.758310577978207334, 31.33698337089302299 ) ) ;
#18505=CARTESIAN_POINT ( 'NONE',  ( -14.05763799605399278, -4.235687564193447052, 33.53795663066793509 ) ) ;
#18506=ORIENTED_EDGE ( 'NONE', *, *, #32487, .T. ) ;
#18507=CARTESIAN_POINT ( 'NONE',  ( 16.82694634598072270, -9.943427161483782584, 34.11278801902876978 ) ) ;
#18508=ORIENTED_EDGE ( 'NONE', *, *, #69513, .T. ) ;
#18509=VECTOR ( 'NONE', #51527, 1000.000000000000227 ) ;
#18511=ADVANCED_FACE ( 'NONE', ( #27785 ), #14273, .F. ) ;
#18512=FACE_OUTER_BOUND ( 'NONE', #75826, .T. ) ;
#18513=CARTESIAN_POINT ( 'NONE',  ( 0.2380535178145123110, -5.113361153441934093, 34.14387501736622710 ) ) ;
#18514=FACE_BOUND ( 'NONE', #86907, .T. ) ;
#18515=B_SPLINE_CURVE_WITH_KNOTS ( 'NONE', 3,
 ( #39717, #59522, #33396, #5028, #20321, #13119, #13556, #32494, #80251, #25299 ),
 .UNSPECIFIED., .F., .F.,
 ( 4, 2, 2, 2, 4 ),
 ( 0.000000000000000000, 0.0001954311564186877960, 0.0003908623128373755920, 0.0005862934692560633609, 0.0007817246256747511840 ),
 .UNSPECIFIED. ) ;
#18516=FACE_OUTER_BOUND ( 'NONE', #48200, .T. ) ;
#18517=FACE_OUTER_BOUND ( 'NONE', #34226, .T. ) ;
#18518=EDGE_CURVE ( 'NONE', #88116, #36558, #28224, .T. ) ;
#18520=CARTESIAN_POINT ( 'NONE',  ( -10.61538461538461320, -6.435427911321262684, 35.78748833219616898 ) ) ;
#18522=CARTESIAN_POINT ( 'NONE',  ( 17.07692307692295586, -9.442884908241554243, 34.35708131394783038 ) ) ;
#18523=ORIENTED_EDGE ( 'NONE', *, *, #44810, .F. ) ;
#18524=ADVANCED_FACE ( 'NONE', ( #42640 ), #69218, .F. ) ;
#18525=CARTESIAN_POINT ( 'NONE',  ( -11.76194646302586655, -3.562934362175800285, 33.22335522853832401 ) ) ;
#18526=ORIENTED_EDGE ( 'NONE', *, *, #82740, .T. ) ;
#18527=EDGE_LOOP ( 'NONE', ( #10385, #72015, #18366, #30599 ) ) ;
#18528=DIRECTION ( 'NONE',  ( 0.000000000000000000, 0.8660254037844377084, -0.5000000000000015543 ) ) ;
#18529=CARTESIAN_POINT ( 'NONE',  ( -14.08468095607945969, -12.39991518177334129, 30.74647679643404530 ) ) ;
#18531=DIRECTION ( 'NONE',  ( 0.000000000000000000, 0.4999999999999985567, 0.8660254037844395958 ) ) ;
#18532=LINE ( 'NONE', #57732, #63829 ) ;
#18533=CARTESIAN_POINT ( 'NONE',  ( 7.623227628637698317, -12.39988816332205701, 30.74660775122750778 ) ) ;
#18534=DIRECTION ( 'NONE',  ( -0.000000000000000000, 0.5000000000000011102, -0.8660254037844380415 ) ) ;
#18535=ORIENTED_EDGE ( 'NONE', *, *, #3573, .F. ) ;
#18537=CARTESIAN_POINT ( 'NONE',  ( -4.826868765284761942, -2.564540009722896752, 30.55348353981670684 ) ) ;
#18538=CARTESIAN_POINT ( 'NONE',  ( -14.37377571864818293, -8.120952969808774569, 34.71129190930000163 ) ) ;
#18539=CARTESIAN_POINT ( 'NONE',  ( 13.38461538461538680, -12.37446782046654192, 30.86335684631486131 ) ) ;
#18540=ORIENTED_EDGE ( 'NONE', *, *, #7308, .T. ) ;
#18541=EDGE_CURVE ( 'NONE', #18197, #64611, #68773, .T. ) ;
#18542=CIRCLE ( 'NONE', #38652, 0.2500000000000002220 ) ;
#18543=EDGE_LOOP ( 'NONE', ( #70576, #74032, #30881, #71271 ) ) ;
#18546=CARTESIAN_POINT ( 'NONE',  ( 16.15384615384603251, -6.026961402154118908, 34.52809138561165270 ) ) ;
#18547=CARTESIAN_POINT ( 'NONE',  ( -1.384615384615506484, -2.379036618888197285, 30.90682066428292885 ) ) ;
#18548=ORIENTED_EDGE ( 'NONE', *, *, #40990, .T. ) ;
#18549=CARTESIAN_POINT ( 'NONE',  ( -16.08777780284371772, -4.786620604624113540, 33.94971097300155805 ) ) ;
#18550=CARTESIAN_POINT ( 'NONE',  ( -6.065270000556318486, -9.528491918058357157, 34.59228464037090589 ) ) ;
#18551=CARTESIAN_POINT ( 'NONE',  ( -8.069080063669991532, -11.76352882383564769, 32.36236540154569497 ) ) ;
#18552=CARTESIAN_POINT ( 'NONE',  ( 14.43853072570506946, -7.277220443632450575, 34.74524770363009196 ) ) ;
#18553=CARTESIAN_POINT ( 'NONE',  ( -11.31568199719312773, -9.332535724633409302, 34.40230450496446934 ) ) ;
#18554=ORIENTED_EDGE ( 'NONE', *, *, #31098, .T. ) ;
#18555=CARTESIAN_POINT ( 'NONE',  ( -15.29685161012936945, -11.91647553114624181, 32.58852847137148245 ) ) ;
#18556=EDGE_LOOP ( 'NONE', ( #17726, #80518, #48651, #20684 ) ) ;
#18557=CARTESIAN_POINT ( 'NONE',  ( 15.48071474911737333, -8.433404298154334455, 34.66254593164985920 ) ) ;
#18558=CARTESIAN_POINT ( 'NONE',  ( -3.007756386675835003, -2.523321265292116422, 31.42251411153756990 ) ) ;
#18559=CARTESIAN_POINT ( 'NONE',  ( -13.63459211555773720, -4.943428324936578910, 34.04746400365624481 ) ) ;
#18561=CARTESIAN_POINT ( 'NONE',  ( -8.546451100252699717, -8.540255544307065350, 34.89611431652622286 ) ) ;
#18563=CARTESIAN_POINT ( 'NONE',  ( 2.307692307692186251, -2.657715359629662544, 31.77849191805970364 ) ) ;
#18565=EDGE_LOOP ( 'NONE', ( #44308, #55909 ) ) ;
#18566=EDGE_CURVE ( 'NONE', #43445, #68660, #21472, .T. ) ;
#18567=CARTESIAN_POINT ( 'NONE',  ( 5.076923076922953193, -12.16647553114689728, 32.15551576947799362 ) ) ;
#18568=CARTESIAN_POINT ( 'NONE',  ( -9.627052121031665521, -8.613356846314928816, 34.62446782046653482 ) ) ;
#18569=DIRECTION ( 'NONE',  ( -0.000000000000000000, 1.000000000000000000, 3.491481338843133355E-15 ) ) ;
#18571=ORIENTED_EDGE ( 'NONE', *, *, #79521, .T. ) ;
#18572=ORIENTED_EDGE ( 'NONE', *, *, #25655, .F. ) ;
#18573=CARTESIAN_POINT ( 'NONE',  ( -8.899378738962466784, -5.915902021225889484, 34.75552854090298638 ) ) ;
#18574=CARTESIAN_POINT ( 'NONE',  ( -7.780086512803769949, -5.471508081941601098, 34.59228464037088457 ) ) ;
#18575=CARTESIAN_POINT ( 'NONE',  ( -0.5268084620947812713, -9.528491918058357157, 34.59228464037090589 ) ) ;
#18576=VECTOR ( 'NONE', #88214, 1000.000000000000000 ) ;
#18577=CARTESIAN_POINT ( 'NONE',  ( -20.99999999999999289, -7.500000000000000000, 29.75000000000000355 ) ) ;
#18579=CARTESIAN_POINT ( 'NONE',  ( -15.48076923076922995, -7.500000000000001776, 35.00000000000000000 ) ) ;
#18580=AXIS2_PLACEMENT_3D ( 'NONE', #78252, #57984, #29642 ) ;
#18581=LINE ( 'NONE', #72622, #16363 ) ;
#18584=EDGE_CURVE ( 'NONE', #52830, #26637, #61540, .T. ) ;
#18585=CARTESIAN_POINT ( 'NONE',  ( -6.249999999999996447, -7.566083408709834757, 34.74999999999999289 ) ) ;
#18586=DIRECTION ( 'NONE',  ( 0.000000000000000000, 0.3420201433256641055, -0.9396926207859100932 ) ) ;
#18588=CARTESIAN_POINT ( 'NONE',  ( 16.15384615384603251, -12.51329471203414379, 31.30864560766407578 ) ) ;
#18589=VERTEX_POINT ( 'NONE', #68334 ) ;
#18590=CARTESIAN_POINT ( 'NONE',  ( -0.2115929431903180169, -2.824170634883619524, 31.52227843825337317 ) ) ;
#18592=CARTESIAN_POINT ( 'NONE',  ( 10.55011461482829738, -3.643525952247789412, 33.31231777344662959 ) ) ;
#18593=DIRECTION ( 'NONE',  ( -1.000000000000000000, 0.000000000000000000, 0.000000000000000000 ) ) ;
#18594=ORIENTED_EDGE ( 'NONE', *, *, #80536, .T. ) ;
#18595=CARTESIAN_POINT ( 'NONE',  ( 0.7115927731767753839, -4.235687564193446164, 33.53795663066793509 ) ) ;
#18596=CARTESIAN_POINT ( 'NONE',  ( 13.45068271796546178, -9.058645607665452459, 34.76329471203371924 ) ) ;
#18598=CARTESIAN_POINT ( 'NONE',  ( -9.915233909823841785, -2.554751324335734708, 30.48935550225260727 ) ) ;
#18599=CARTESIAN_POINT ( 'NONE',  ( 24.00000000000000000, -9.499999999999982236, 27.74999999999999645 ) ) ;
#18600=DIRECTION ( 'NONE',  ( 0.000000000000000000, 0.3420201433256610524, 0.9396926207859113145 ) ) ;
#18601=EDGE_CURVE ( 'NONE', #3366, #21486, #26139, .T. ) ;
#18602=EDGE_CURVE ( 'NONE', #54354, #67169, #63776, .T. ) ;
#18603=VERTEX_POINT ( 'NONE', #44834 ) ;
#18604=CYLINDRICAL_SURFACE ( 'NONE', #51525, 0.2500000000000002220 ) ;
#18605=ORIENTED_EDGE ( 'NONE', *, *, #18862, .F. ) ;
#18606=CARTESIAN_POINT ( 'NONE',  ( -15.00775638667583678, -6.460100341425560444, 34.89618726649961644 ) ) ;
#18608=EDGE_CURVE ( 'NONE', #54359, #5224, #83089, .T. ) ;
#18609=CARTESIAN_POINT ( 'NONE',  ( -12.23852561744506851, -2.889357225399414197, 32.26129605718031002 ) ) ;
#18610=CARTESIAN_POINT ( 'NONE',  ( -0.2114840416250075017, -2.544122305571458575, 31.48381861865057729 ) ) ;
#18612=CARTESIAN_POINT ( 'NONE',  ( -6.700065571464073777, -5.667800583137508674, 34.40243808032445827 ) ) ;
#18613=CARTESIAN_POINT ( 'NONE',  ( -6.065270445960775803, -4.481592998940161721, 33.73612834413957984 ) ) ;
#18614=CARTESIAN_POINT ( 'NONE',  ( -6.792286482109971324, -2.494656445102013453, 31.33466734024120015 ) ) ;
#18615=ORIENTED_EDGE ( 'NONE', *, *, #17407, .F. ) ;
#18617=VERTEX_POINT ( 'NONE', #10178 ) ;
#18618=ORIENTED_EDGE ( 'NONE', *, *, #33220, .T. ) ;
#18620=CARTESIAN_POINT ( 'NONE',  ( -5.300408001487407539, -4.225889041578354544, 33.85425143139329407 ) ) ;
#18621=LINE ( 'NONE', #24470, #51697 ) ;
#18622=CARTESIAN_POINT ( 'NONE',  ( -3.903791842207837259, -9.148310452688871663, 34.47095581063188519 ) ) ;
#18625=EDGE_CURVE ( 'NONE', #34790, #34216, #84080, .T. ) ;
#18626=CARTESIAN_POINT ( 'NONE',  ( -12.46153846153858424, -12.51329471203414379, 31.30864560766407578 ) ) ;
#18627=AXIS2_PLACEMENT_3D ( 'NONE', #20411, #80457, #12000 ) ;
#18628=CARTESIAN_POINT ( 'NONE',  ( -5.207070286361298095, -8.587444163452046197, 34.63053765926554206 ) ) ;
#18629=CARTESIAN_POINT ( 'NONE',  ( -4.023320452082588261, -10.88167719472716399, 33.43325721877153711 ) ) ;
#18631=ORIENTED_EDGE ( 'NONE', *, *, #3053, .T. ) ;
#18632=VERTEX_POINT ( 'NONE', #49824 ) ;
#18634=VERTEX_POINT ( 'NONE', #77300 ) ;
#18635=AXIS2_PLACEMENT_3D ( 'NONE', #59605, #78989, #17291 ) ;
#18636=CARTESIAN_POINT ( 'NONE',  ( -1.449885830576158607, -11.48612834413959582, 32.76840700105983473 ) ) ;
#18637=ORIENTED_EDGE ( 'NONE', *, *, #35053, .T. ) ;
#18638=CARTESIAN_POINT ( 'NONE',  ( 14.30769230769231015, -1.422936976036506707, 30.56769352161908415 ) ) ;
#18639=DIRECTION ( 'NONE',  ( -0.000000000000000000, -0.5000000000000009992, -0.8660254037844380415 ) ) ;
#18640=EDGE_CURVE ( 'NONE', #40157, #70140, #18649, .T. ) ;
#18641=VECTOR ( 'NONE', #17687, 1000.000000000000114 ) ;
#18643=CARTESIAN_POINT ( 'NONE',  ( -11.28840711854808632, -9.233818618650603938, 34.70587769442853698 ) ) ;
#18644=FACE_BOUND ( 'NONE', #36870, .T. ) ;
#18645=EDGE_LOOP ( 'NONE', ( #38326, #38369 ) ) ;
#18647=EDGE_CURVE ( 'NONE', #56507, #58928, #71268, .T. ) ;
#18648=CARTESIAN_POINT ( 'NONE',  ( -4.946131269098287930, -6.413143153341454017, 34.63066358083362672 ) ) ;
#18649=B_SPLINE_CURVE_WITH_KNOTS ( 'NONE', 3,
 ( #78186, #71868, #84517, #24121, #43075, #8855, #43953, #22790, #37193, #36326 ),
 .UNSPECIFIED., .F., .F.,
 ( 4, 2, 2, 2, 4 ),
 ( 0.0007817359430256370532, 0.0009771253907250049969, 0.001172514838424372832, 0.001367904286123740668, 0.001563293733823108503 ),
 .UNSPECIFIED. ) ;
#18650=ORIENTED_EDGE ( 'NONE', *, *, #29186, .F. ) ;
#18651=FACE_BOUND ( 'NONE', #20933, .T. ) ;
#18652=B_SPLINE_CURVE_WITH_KNOTS ( 'NONE', 3,
 ( #46606, #12814, #52902, #12379, #18698, #39856, #73650, #39420, #67322, #40300 ),
 .UNSPECIFIED., .F., .F.,
 ( 4, 2, 2, 2, 4 ),
 ( 0.000000000000000000, 0.0001954311564186861697, 0.0003908623128373723394, 0.0005862934692560584820, 0.0007817246256747446788 ),
 .UNSPECIFIED. ) ;
#18655=VERTEX_POINT ( 'NONE', #43515 ) ;
#18656=CARTESIAN_POINT ( 'NONE',  ( 17.74997676270703550, -2.823816976329320827, 31.52131813110797154 ) ) ;
#18658=CARTESIAN_POINT ( 'NONE',  ( 1.384615384615264011, -3.643525952248795718, 33.31231777344771672 ) ) ;
#18659=EDGE_LOOP ( 'NONE', ( #36150, #38320, #85864, #19305 ) ) ;
#18660=DIRECTION ( 'NONE',  ( -0.000000000000000000, -0.9848077530122085754, -0.1736481776669273613 ) ) ;
#18661=CARTESIAN_POINT ( 'NONE',  ( -18.13069146666755671, -4.809359713505812373, 33.96456829005828837 ) ) ;
#18662=FACE_OUTER_BOUND ( 'NONE', #27264, .T. ) ;
#18663=ORIENTED_EDGE ( 'NONE', *, *, #47639, .T. ) ;
#18664=ADVANCED_FACE ( 'NONE', ( #70990 ), #2514, .F. ) ;
#18665=CARTESIAN_POINT ( 'NONE',  ( -1.634592115557737646, -5.728515186090277211, 34.42611988154120439 ) ) ;
#18666=CARTESIAN_POINT ( 'NONE',  ( -16.85391172531022974, -11.76359900205217457, 32.36225158514719880 ) ) ;
#18667=ORIENTED_EDGE ( 'NONE', *, *, #64760, .F. ) ;
#18668=CARTESIAN_POINT ( 'NONE',  ( -12.46153846153858424, -5.941354392335915335, 34.76329471203413846 ) ) ;
#18669=CARTESIAN_POINT ( 'NONE',  ( -12.21159294319032185, -2.587454068350147018, 30.68340429815432202 ) ) ;
#18671=CARTESIAN_POINT ( 'NONE',  ( 15.10007862765892739, -12.62707690430377383, 30.88035979386743435 ) ) ;
#18672=CARTESIAN_POINT ( 'NONE',  ( -7.173076923076922462, -7.433932668274256805, 35.00000000000000711 ) ) ;
#18673=CARTESIAN_POINT ( 'NONE',  ( 6.792385456409367528, -8.999036380462719364, 34.52022231692819076 ) ) ;
#18675=DIRECTION ( 'NONE',  ( -0.000000000000000000, -0.000000000000000000, -1.000000000000000000 ) ) ;
#18676=CARTESIAN_POINT ( 'NONE',  ( -3.361460697436789768, -2.541943142973489778, 30.39792223712631980 ) ) ;
#18679=ORIENTED_EDGE ( 'NONE', *, *, #43900, .F. ) ;
#18681=CARTESIAN_POINT ( 'NONE',  ( 18.00000000000000000, -4.098570777380720287, 33.41473453929634729 ) ) ;
#18683=VERTEX_POINT ( 'NONE', #31787 ) ;
#18684=EDGE_CURVE ( 'NONE', #88590, #19138, #66455, .T. ) ;
#18685=CARTESIAN_POINT ( 'NONE',  ( -16.94613263595612551, -3.957578996910245284, 33.62503395064540257 ) ) ;
#18686=ORIENTED_EDGE ( 'NONE', *, *, #86622, .F. ) ;
#18687=CARTESIAN_POINT ( 'NONE',  ( 3.480823542407546434, -9.943054286541407549, 34.11300777759954883 ) ) ;
#18689=CARTESIAN_POINT ( 'NONE',  ( -13.38461538461538325, -5.471508081941601098, 34.59228464037088457 ) ) ;
#18690=CARTESIAN_POINT ( 'NONE',  ( -18.13014796973169851, -12.15440758774515650, 32.17923288041532004 ) ) ;
#18691=CARTESIAN_POINT ( 'NONE',  ( -7.715628144390279886, -6.001044277235009439, 34.52024696741798948 ) ) ;
#18692=CARTESIAN_POINT ( 'NONE',  ( 9.915087361285756629, -3.020022701398814569, 32.48759521482552515 ) ) ;
#18693=CARTESIAN_POINT ( 'NONE',  ( -4.854143407945009869, -2.612705202774697533, 31.66806509827799943 ) ) ;
#18694=CARTESIAN_POINT ( 'NONE',  ( 0.6843181305165266792, -5.827830569534416583, 34.72679350104403539 ) ) ;
#18695=CARTESIAN_POINT ( 'NONE',  ( 0.6843181305165249029, -2.612705202774697533, 31.66806509827799943 ) ) ;
#18697=CARTESIAN_POINT ( 'NONE',  ( 2.057692307692309708, -2.249999999999998668, 29.75000000000000355 ) ) ;
#18698=CARTESIAN_POINT ( 'NONE',  ( -4.403822897894742461, -12.01397095200673881, 32.43157075238190146 ) ) ;
#18700=B_SPLINE_CURVE_WITH_KNOTS ( 'NONE', 3,
 ( #70878, #57353, #9184, #36643, #84845, #85277, #64533, #2834, #23560, #78500 ),
 .UNSPECIFIED., .F., .F.,
 ( 4, 2, 2, 2, 4 ),
 ( 0.0007817246256747517261, 0.0009771112852218961399, 0.001172497944769040771, 0.001367884604316185401, 0.001563271263863329815 ),
 .UNSPECIFIED. ) ;
#18701=DIRECTION ( 'NONE',  ( -0.000000000000000000, -0.6427876096865404731, -0.7660444431189771253 ) ) ;
#18702=AXIS2_PLACEMENT_3D ( 'NONE', #59643, #4256, #79921 ) ;
#18703=ORIENTED_EDGE ( 'NONE', *, *, #70642, .F. ) ;
#18704=ORIENTED_EDGE ( 'NONE', *, *, #37296, .F. ) ;
#18705=CARTESIAN_POINT ( 'NONE',  ( -8.769230769230890843, -12.46129190930018460, 30.37095296980731973 ) ) ;
#18706=DIRECTION ( 'NONE',  ( -0.000000000000000000, -0.8660254037844397068, -0.4999999999999978906 ) ) ;
#18707=CARTESIAN_POINT ( 'NONE',  ( 1.134592160393928406, -10.92453946501458439, 33.72985991061850086 ) ) ;
#18708=CARTESIAN_POINT ( 'NONE',  ( -6.249976730942354841, -3.627789207965226748, 32.91389620160131102 ) ) ;
#18709=AXIS2_PLACEMENT_3D ( 'NONE', #63965, #56773, #22549 ) ;
#18710=FACE_OUTER_BOUND ( 'NONE', #1671, .T. ) ;
#18711=EDGE_CURVE ( 'NONE', #39142, #3390, #25019, .T. ) ;
#18712=AXIS2_PLACEMENT_3D ( 'NONE', #82217, #81775, #20940 ) ;
#18713=CARTESIAN_POINT ( 'NONE',  ( -0.5916856709766818989, -6.852621066184267029, 34.70813303252209181 ) ) ;
#18714=EDGE_CURVE ( 'NONE', #39878, #84116, #60886, .T. ) ;
#18716=ORIENTED_EDGE ( 'NONE', *, *, #75834, .T. ) ;
#18717=CARTESIAN_POINT ( 'NONE',  ( -12.46153846153846168, -3.886160181151819604, 36.00935417666054406 ) ) ;
#18718=ORIENTED_EDGE ( 'NONE', *, *, #36252, .F. ) ;
#18720=CARTESIAN_POINT ( 'NONE',  ( 17.75002326905764960, -3.137211980971220893, 32.19342716148376837 ) ) ;
#18721=CARTESIAN_POINT ( 'NONE',  ( -14.05774689831426372, -6.653508905675592722, 34.93172785388651391 ) ) ;
#18722=DIRECTION ( 'NONE',  ( -0.000000000000000000, -0.000000000000000000, -1.000000000000000000 ) ) ;
#18723=CARTESIAN_POINT ( 'NONE',  ( 1.384615384615264011, -11.67786785259630911, 32.92929555188603530 ) ) ;
#18724=CARTESIAN_POINT ( 'NONE',  ( 5.933916589044122780, -2.721908614388772740, 31.22303859784724622 ) ) ;
#18725=VERTEX_POINT ( 'NONE', #24571 ) ;
#18726=VERTEX_POINT ( 'NONE', #60131 ) ;
#18727=B_SPLINE_CURVE_WITH_KNOTS ( 'NONE', 3,
 ( #22060, #15307, #42783, #30142, #16614, #79663, #44520, #85091, #3098, #38225 ),
 .UNSPECIFIED., .F., .F.,
 ( 4, 2, 2, 2, 4 ),
 ( 0.0007817246256747472808, 0.0009771112852218907189, 0.001172497944769034265, 0.001367884604316177595, 0.001563271263863321141 ),
 .UNSPECIFIED. ) ;
#18728=EDGE_LOOP ( 'NONE', ( #30677, #47952 ) ) ;
#18729=CARTESIAN_POINT ( 'NONE',  ( -6.130690603110308778, -4.684245665217972032, 34.18127051446801090 ) ) ;
#18731=AXIS2_PLACEMENT_3D ( 'NONE', #4589, #39721, #59526 ) ;
#18732=CARTESIAN_POINT ( 'NONE',  ( 9.019285189144223835, -5.642605341092957971, 34.66089969410670335 ) ) ;
#18733=CARTESIAN_POINT ( 'NONE',  ( -8.769230769230768274, -2.292212530054420494, 30.41441678777542634 ) ) ;
#18734=FACE_OUTER_BOUND ( 'NONE', #68411, .T. ) ;
#18735=ORIENTED_EDGE ( 'NONE', *, *, #86420, .F. ) ;
#18736=ORIENTED_EDGE ( 'NONE', *, *, #28502, .F. ) ;
#18737=CARTESIAN_POINT ( 'NONE',  ( 5.010840697562940704, -9.905515769479276145, 34.41647553114623292 ) ) ;
#18738=CARTESIAN_POINT ( 'NONE',  ( 2.557637826040450868, -12.43552623307873972, 30.55307653245132826 ) ) ;
#18739=VERTEX_POINT ( 'NONE', #12399 ) ;
#18740=CARTESIAN_POINT ( 'NONE',  ( 1.253923917947826983, -9.804603061927743113, 34.18744698557895845 ) ) ;
#18741=CARTESIAN_POINT ( 'NONE',  ( 5.076923076923075762, -8.973038597847269315, 34.52809138561121927 ) ) ;
#18744=AXIS2_PLACEMENT_3D ( 'NONE', #85094, #73351, #52175 ) ;
#18745=DIRECTION ( 'NONE',  ( 0.000000000000000000, -6.938893903907222067E-15, 1.000000000000000000 ) ) ;
#18746=EDGE_LOOP ( 'NONE', ( #78750, #22535 ) ) ;
#18747=CARTESIAN_POINT ( 'NONE',  ( -13.60754234352223158, -11.43668979543635089, 33.22377378376089752 ) ) ;
#18748=CARTESIAN_POINT ( 'NONE',  ( 3.230769230769231726, -2.708943851104267164, 35.45975837776705220 ) ) ;
#18749=CARTESIAN_POINT ( 'NONE',  ( 7.780071466793709867, -3.937682226553329556, 33.60647404775217240 ) ) ;
#18751=AXIS2_PLACEMENT_3D ( 'NONE', #20655, #41826, #29204 ) ;
#18752=FACE_OUTER_BOUND ( 'NONE', #81860, .T. ) ;
#18753=VECTOR ( 'NONE', #60834, 1000.000000000000227 ) ;
#18754=DIRECTION ( 'NONE',  ( -0.000000000000000000, 0.5000000000000011102, -0.8660254037844381525 ) ) ;
#18757=CARTESIAN_POINT ( 'NONE',  ( 15.16468581981334829, -4.098570777380720287, 33.41473453929634729 ) ) ;
#18759=FACE_OUTER_BOUND ( 'NONE', #79866, .T. ) ;
#18760=ORIENTED_EDGE ( 'NONE', *, *, #16623, .T. ) ;
#18761=CARTESIAN_POINT ( 'NONE',  ( -18.00000000000000000, -10.88783764156682032, 36.11790692298802696 ) ) ;
#18762=CARTESIAN_POINT ( 'NONE',  ( 10.61538461538461675, -8.164416787775445883, 34.95778746994557906 ) ) ;
#18763=FACE_OUTER_BOUND ( 'NONE', #31023, .T. ) ;
#18765=FACE_BOUND ( 'NONE', #3411, .T. ) ;
#18766=CARTESIAN_POINT ( 'NONE',  ( 6.000000000000001776, -4.661471528628507777, 34.16647553114623292 ) ) ;
#18767=DIRECTION ( 'NONE',  ( 0.000000000000000000, 0.7660444431189822323, -0.6427876096865344779 ) ) ;
#18768=CARTESIAN_POINT ( 'NONE',  ( -9.627052552794854279, -12.16647553114626490, 32.15551576947920864 ) ) ;
#18769=CARTESIAN_POINT ( 'NONE',  ( -1.318547033612946118, -12.10708131394839704, 31.69288490824020954 ) ) ;
#18770=CARTESIAN_POINT ( 'NONE',  ( 17.75002326905764605, -11.28823185664190376, 33.01397839955799896 ) ) ;
#18771=CARTESIAN_POINT ( 'NONE',  ( -4.088591014333314178, -11.06231777344671130, 33.60647404775212976 ) ) ;
#18772=CARTESIAN_POINT ( 'NONE',  ( 15.23076923076923173, -5.557115091759785130, 34.35708131394839171 ) ) ;
#18774=EDGE_LOOP ( 'NONE', ( #12030, #44343 ) ) ;
#18775=CARTESIAN_POINT ( 'NONE',  ( -6.923076923077044142, -9.442884908241554243, 34.35708131394783038 ) ) ;
#18776=ORIENTED_EDGE ( 'NONE', *, *, #34004, .F. ) ;
#18777=ADVANCED_FACE ( 'NONE', ( #18271 ), #73216, .F. ) ;
#18778=CARTESIAN_POINT ( 'NONE',  ( 1.134615384615387246, -2.499999999999998668, 29.75000000000000355 ) ) ;
#18779=CARTESIAN_POINT ( 'NONE',  ( -14.98076923076779465, -7.500000000000155431, 34.75000000000007105 ) ) ;
#18781=CARTESIAN_POINT ( 'NONE',  ( -5.999999999999998224, -3.886160181151819604, 36.00935417666054406 ) ) ;
#18782=CARTESIAN_POINT ( 'NONE',  ( -10.48459417441766561, -11.93129842949671726, 32.56571108434900452 ) ) ;
#18783=CARTESIAN_POINT ( 'NONE',  ( -11.76138849736838488, -4.026226216239094491, 33.68668979543634379 ) ) ;
#18785=CYLINDRICAL_SURFACE ( 'NONE', #69094, 0.2499999999999995559 ) ;
#18786=CARTESIAN_POINT ( 'NONE',  ( 8.519254025182180001, -2.544273027872575366, 31.48422191005632342 ) ) ;
#18787=CARTESIAN_POINT ( 'NONE',  ( -8.769230769230768274, -4.786620604624113540, 33.94971097300155094 ) ) ;
#18788=CARTESIAN_POINT ( 'NONE',  ( 17.75000000000000000, -7.500000000000001776, 34.75000000000000000 ) ) ;
#18789=CARTESIAN_POINT ( 'NONE',  ( -6.923076923076922462, -4.098570777380720287, 33.41473453929634729 ) ) ;
#18790=CARTESIAN_POINT ( 'NONE',  ( -8.834501215191545853, -9.442884908240170461, 34.35708131394840592 ) ) ;
#18791=CARTESIAN_POINT ( 'NONE',  ( -16.40384615384615330, -2.499999999999998668, 29.75000000000000355 ) ) ;
#18792=EDGE_CURVE ( 'NONE', #79735, #48079, #1413, .T. ) ;
#18793=CARTESIAN_POINT ( 'NONE',  ( 7.846153846153846700, -9.058645607665452459, 34.76329471203371924 ) ) ;
#18794=B_SPLINE_CURVE_WITH_KNOTS ( 'NONE', 3,
 ( #25794, #52808, #60016, #18598, #5971, #60901, #12722, #87976, #46060, #19037 ),
 .UNSPECIFIED., .F., .F.,
 ( 4, 2, 2, 2, 4 ),
 ( 0.000000000000000000, 0.0001954339857564098054, 0.0003908679715128196108, 0.0005863019572692293891, 0.0007817359430256392216 ),
 .UNSPECIFIED. ) ;
#18795=VERTEX_POINT ( 'NONE', #58798 ) ;
#18796=CARTESIAN_POINT ( 'NONE',  ( 16.21910129335899597, -5.094484230520771817, 34.41647553114626845 ) ) ;
#18797=DIRECTION ( 'NONE',  ( -0.000000000000000000, 0.1736481776669307198, -0.9848077530122080203 ) ) ;
#18799=CARTESIAN_POINT ( 'NONE',  ( 6.130525701763565927, -4.459921816937789885, 33.71989282347011851 ) ) ;
#18800=CARTESIAN_POINT ( 'NONE',  ( 17.32697738856138869, -11.79725096376909299, 32.30694842903960762 ) ) ;
#18801=VERTEX_POINT ( 'NONE', #46626 ) ;
#18802=CARTESIAN_POINT ( 'NONE',  ( 7.173022441425065843, -8.433404298154334455, 34.66254593164985920 ) ) ;
#18803=CARTESIAN_POINT ( 'NONE',  ( 9.442330948259103351, -12.65889640711025521, 30.72598325615533454 ) ) ;
#18804=CARTESIAN_POINT ( 'NONE',  ( 11.31497661389720477, -3.019605429927184392, 32.48692288466676814 ) ) ;
#18805=ORIENTED_EDGE ( 'NONE', *, *, #20534, .F. ) ;
#18806=CARTESIAN_POINT ( 'NONE',  ( -9.942284436356285227, -3.436278759898153901, 33.07459398097509506 ) ) ;
#18807=CARTESIAN_POINT ( 'NONE',  ( 12.46153846153833911, -12.46129190930018460, 30.37095296980731973 ) ) ;
#18808=CARTESIAN_POINT ( 'NONE',  ( 15.23076923076923173, -5.471508081941601098, 34.59228464037088457 ) ) ;
#18809=CARTESIAN_POINT ( 'NONE',  ( -3.230769230769229949, -2.900454961884010974, 35.62045528018868623 ) ) ;
#18810=ORIENTED_EDGE ( 'NONE', *, *, #31700, .F. ) ;
#18812=CARTESIAN_POINT ( 'NONE',  ( 10.68145194873469173, -3.937682226553329556, 33.60647404775216529 ) ) ;
#18813=EDGE_CURVE ( 'NONE', #53579, #70248, #74468, .T. ) ;
#18814=CARTESIAN_POINT ( 'NONE',  ( 8.703960768674448900, -3.643525952247789412, 33.31231777344662959 ) ) ;
#18815=EDGE_LOOP ( 'NONE', ( #11866, #40592, #10024, #67725 ) ) ;
#18817=ORIENTED_EDGE ( 'NONE', *, *, #85768, .F. ) ;
#18818=VECTOR ( 'NONE', #50832, 999.9999999999998863 ) ;
#18820=EDGE_CURVE ( 'NONE', #47774, #74921, #37943, .T. ) ;
#18821=CARTESIAN_POINT ( 'NONE',  ( 0.4615384615384611200, -8.120952969808772792, 34.71129190930000163 ) ) ;
#18822=CARTESIAN_POINT ( 'NONE',  ( 9.692307692307570832, -12.51329471203414379, 31.30864560766407578 ) ) ;
#18823=CARTESIAN_POINT ( 'NONE',  ( 13.16113044089143891, -11.41268669641499756, 32.86336882939238535 ) ) ;
#18825=CARTESIAN_POINT ( 'NONE',  ( 7.846153846153846700, -5.557115091759785130, 34.35708131394839171 ) ) ;
#18827=VERTEX_POINT ( 'NONE', #72756 ) ;
#18828=ORIENTED_EDGE ( 'NONE', *, *, #79161, .F. ) ;
#18829=CARTESIAN_POINT ( 'NONE',  ( 15.29683758177167086, -4.786620604624113540, 33.94971097300155805 ) ) ;
#18830=ORIENTED_EDGE ( 'NONE', *, *, #42850, .T. ) ;
#18831=CARTESIAN_POINT ( 'NONE',  ( -16.40386937806761836, -12.45566812827425096, 31.48439005359158926 ) ) ;
#18832=FACE_OUTER_BOUND ( 'NONE', #69467, .T. ) ;
#18833=B_SPLINE_CURVE_WITH_KNOTS ( 'NONE', 3,
 ( #43366, #3695, #10472, #23964, #17217, #16770, #37939, #44224, #71711, #64496 ),
 .UNSPECIFIED., .F., .F.,
 ( 4, 2, 2, 2, 4 ),
 ( 0.000000000000000000, 0.0001954311564186871184, 0.0003908623128373742367, 0.0005862934692560614093, 0.0007817246256747484735 ),
 .UNSPECIFIED. ) ;
#18834=DIRECTION ( 'NONE',  ( 0.000000000000000000, 0.000000000000000000, 1.000000000000000000 ) ) ;
#18835=CARTESIAN_POINT ( 'NONE',  ( -5.776988648387149539, -4.187068189119697692, 33.49521262558774026 ) ) ;
#18836=ORIENTED_EDGE ( 'NONE', *, *, #31917, .T. ) ;
#18837=EDGE_LOOP ( 'NONE', ( #87842, #52718, #19069, #86457 ) ) ;
#18838=ORIENTED_EDGE ( 'NONE', *, *, #54231, .F. ) ;
#18839=CARTESIAN_POINT ( 'NONE',  ( 10.61538461538449596, -10.90142922262034020, 33.41473453929536674 ) ) ;
#18840=CARTESIAN_POINT ( 'NONE',  ( 5.076923076923075762, -2.499999999999998668, 29.50000000000001066 ) ) ;
#18841=VERTEX_POINT ( 'NONE', #46188 ) ;
#18842=CARTESIAN_POINT ( 'NONE',  ( 3.230769230769110045, -11.94971097300221174, 32.03036669348237098 ) ) ;
#18845=CARTESIAN_POINT ( 'NONE',  ( -5.076923076923075762, -4.102666532097928531, 36.13435417666054406 ) ) ;
#18848=CARTESIAN_POINT ( 'NONE',  ( -39.05038313613820122, -2.249999999999998668, 29.75000000000000355 ) ) ;
#18849=FACE_BOUND ( 'NONE', #40421, .T. ) ;
#18852=CARTESIAN_POINT ( 'NONE',  ( -7.846153846153844924, -12.10708131394839349, 31.69288490824020244 ) ) ;
#18853=CARTESIAN_POINT ( 'NONE',  ( -17.93129618099663958, -12.74404781541490372, 29.99992509483736214 ) ) ;
#18854=CARTESIAN_POINT ( 'NONE',  ( 6.700149964170072359, -10.77366814457252175, 33.85459836347579454 ) ) ;
#18856=CARTESIAN_POINT ( 'NONE',  ( -4.087778820496075660, -11.35647404775217595, 33.31231777344667222 ) ) ;
#18857=ORIENTED_EDGE ( 'NONE', *, *, #23019, .F. ) ;
#18858=CARTESIAN_POINT ( 'NONE',  ( 11.40831432902331954, -3.285722584762969856, 32.44110544564090759 ) ) ;
#18859=CARTESIAN_POINT ( 'NONE',  ( 12.71148387091650278, -3.520799739797214389, 33.17531984108286025 ) ) ;
#18860=ORIENTED_EDGE ( 'NONE', *, *, #14844, .F. ) ;
#18861=ORIENTED_EDGE ( 'NONE', *, *, #15433, .T. ) ;
#18862=EDGE_CURVE ( 'NONE', #2073, #68833, #73672, .T. ) ;
#18864=CARTESIAN_POINT ( 'NONE',  ( -5.999999999999998224, -10.89733346790207413, 36.13435417666054406 ) ) ;
#18865=CARTESIAN_POINT ( 'NONE',  ( 12.33139049180676139, -11.04286588640298561, 33.62463336215343901 ) ) ;
#18866=ORIENTED_EDGE ( 'NONE', *, *, #66948, .F. ) ;
#18867=DIRECTION ( 'NONE',  ( -0.000000000000000000, 0.6427876096865404731, -0.7660444431189771253 ) ) ;
#18868=CARTESIAN_POINT ( 'NONE',  ( -7.173100160369890510, -10.05641848906368097, 34.04755513067966177 ) ) ;
#18869=DIRECTION ( 'NONE',  ( 0.000000000000000000, 0.000000000000000000, 1.000000000000000000 ) ) ;
#18870=CARTESIAN_POINT ( 'NONE',  ( 2.307692307692309264, -12.62096338111211580, 30.90682066428153263 ) ) ;
#18871=DIRECTION ( 'NONE',  ( -0.000000000000000000, 0.3420201433256694901, -0.9396926207859082059 ) ) ;
#18872=VECTOR ( 'NONE', #22643, 1000.000000000000000 ) ;
#18873=CARTESIAN_POINT ( 'NONE',  ( 0.6843181305165257911, -4.989023458446561143, 34.36081565061822118 ) ) ;
#18876=ORIENTED_EDGE ( 'NONE', *, *, #88857, .T. ) ;
#18878=CIRCLE ( 'NONE', #35984, 0.2500000000000002220 ) ;
#18879=ORIENTED_EDGE ( 'NONE', *, *, #21446, .T. ) ;
#18880=EDGE_CURVE ( 'NONE', #3322, #7083, #17515, .T. ) ;
#18881=CARTESIAN_POINT ( 'NONE',  ( 5.076923076922953193, -11.06231777344772027, 33.60647404775119895 ) ) ;
#18882=CARTESIAN_POINT ( 'NONE',  ( 6.989145274079364256, -12.10708131394839882, 31.69288490824020954 ) ) ;
#18884=CARTESIAN_POINT ( 'NONE',  ( 13.38461538461538680, -2.900454961884010974, 35.62045528018868623 ) ) ;
#18885=ADVANCED_FACE ( 'NONE', ( #13728 ), #41645, .F. ) ;
#18886=CARTESIAN_POINT ( 'NONE',  ( -7.780960857859191115, -2.255955759149236073, 29.99999999999988631 ) ) ;
#18888=CARTESIAN_POINT ( 'NONE',  ( -7.596099534515528440, -8.303483539816728154, 34.68545999027711702 ) ) ;
#18889=CYLINDRICAL_SURFACE ( 'NONE', #54653, 0.2500000000000009437 ) ;
#18890=CARTESIAN_POINT ( 'NONE',  ( -17.07692307692307665, -2.538708090699994813, 30.37095296980875503 ) ) ;
#18891=CARTESIAN_POINT ( 'NONE',  ( 13.38461538461526423, -10.33852847137269571, 34.16647553114546554 ) ) ;
#18892=CARTESIAN_POINT ( 'NONE',  ( -6.223484943723945229, -2.847400154188068022, 31.58180166144859058 ) ) ;
#18893=FACE_OUTER_BOUND ( 'NONE', #33671, .T. ) ;
#18894=B_SPLINE_CURVE_WITH_KNOTS ( 'NONE', 3,
 ( #213, #27678, #82644, #44269, #29466, #30337, #70889, #1542, #42974, #50150 ),
 .UNSPECIFIED., .F., .F.,
 ( 4, 2, 2, 2, 4 ),
 ( 0.0007817246256747459798, 0.0009771112852218896347, 0.001172497944769033398, 0.001367884604316177161, 0.001563271263863320708 ),
 .UNSPECIFIED. ) ;
#18895=DIRECTION ( 'NONE',  ( 0.000000000000000000, 0.000000000000000000, 1.000000000000000000 ) ) ;
#18896=CARTESIAN_POINT ( 'NONE',  ( 4.088575707885377497, -12.46129190929999986, 30.37095296980880832 ) ) ;
#18898=ADVANCED_FACE ( 'NONE', ( #26799 ), #82194, .F. ) ;
#18899=CARTESIAN_POINT ( 'NONE',  ( -11.53846153846166089, -3.083524468854526912, 32.58852847137268327 ) ) ;
#18900=ORIENTED_EDGE ( 'NONE', *, *, #9346, .T. ) ;
#18901=CARTESIAN_POINT ( 'NONE',  ( -4.219116599806927326, -5.219633306516282545, 34.19971097300152252 ) ) ;
#18902=CARTESIAN_POINT ( 'NONE',  ( -15.23076923076935252, -12.70778746994576025, 30.41441678777401236 ) ) ;
#18903=CARTESIAN_POINT ( 'NONE',  ( 5.999999999999878320, -2.657715359629662988, 31.77849191805970364 ) ) ;
#18906=CARTESIAN_POINT ( 'NONE',  ( -5.999999999999998224, -9.819645486525091727, 36.12317359536749706 ) ) ;
#18907=( NAMED_UNIT ( * ) SI_UNIT ( $, .STERADIAN. ) SOLID_ANGLE_UNIT ( ) );
#18908=CARTESIAN_POINT ( 'NONE',  ( -18.25000000000000711, -2.250000000000000000, 29.68055622560741114 ) ) ;
#18911=DIRECTION ( 'NONE',  ( -0.000000000000000000, -0.1736481776669307198, -0.9848077530122080203 ) ) ;
#18912=ORIENTED_EDGE ( 'NONE', *, *, #56308, .T. ) ;
#18913=CARTESIAN_POINT ( 'NONE',  ( 0.2115617305961081662, -2.779195860258146578, 31.39871582349836032 ) ) ;
#18914=ORIENTED_EDGE ( 'NONE', *, *, #54639, .F. ) ;
#18915=AXIS2_PLACEMENT_3D ( 'NONE', #73919, #88342, #68478 ) ;
#18916=DIRECTION ( 'NONE',  ( 0.000000000000000000, -6.938893903907222067E-15, 1.000000000000000000 ) ) ;
#18917=CARTESIAN_POINT ( 'NONE',  ( -7.623142494540994463, -11.76359900205217635, 32.36225158514719169 ) ) ;
#18920=EDGE_LOOP ( 'NONE', ( #49541, #54216 ) ) ;
#18921=EDGE_CURVE ( 'NONE', #67903, #45764, #21366, .T. ) ;
#18922=FACE_OUTER_BOUND ( 'NONE', #5600, .T. ) ;
#18923=ORIENTED_EDGE ( 'NONE', *, *, #11272, .T. ) ;
#18924=VERTEX_POINT ( 'NONE', #13283 ) ;
#18925=CARTESIAN_POINT ( 'NONE',  ( -0.5276218724943418925, -3.050289026998445951, 32.03036669348365706 ) ) ;
#18926=CARTESIAN_POINT ( 'NONE',  ( 7.846153846153846700, -12.09954503811598769, 35.62045528018868623 ) ) ;
#18927=ADVANCED_FACE ( 'NONE', ( #21812 ), #20041, .F. ) ;
#18928=FACE_OUTER_BOUND ( 'NONE', #25579, .T. ) ;
#18929=CARTESIAN_POINT ( 'NONE',  ( 9.692307692307570832, -9.528491918059723176, 34.59228464037033035 ) ) ;
#18930=EDGE_CURVE ( 'NONE', #47846, #47342, #6834, .T. ) ;
#18931=DIRECTION ( 'NONE',  ( 0.000000000000000000, 0.6427876096865373645, -0.7660444431189797898 ) ) ;
#18932=DIRECTION ( 'NONE',  ( -0.000000000000000000, 0.3420201433256694346, -0.9396926207859080948 ) ) ;
#18933=CARTESIAN_POINT ( 'NONE',  ( 0.2115152373170033351, -2.341070481393820124, 30.72580821765574299 ) ) ;
#18934=CARTESIAN_POINT ( 'NONE',  ( -0.3307480205715124799, -12.35292014791297710, 31.75344720912887198 ) ) ;
#18935=B_SPLINE_CURVE_WITH_KNOTS ( 'NONE', 3,
 ( #87721, #52122, #25993, #3490, #85922, #53456, #79610, #5281, #80958, #24204 ),
 .UNSPECIFIED., .F., .F.,
 ( 4, 2, 2, 2, 4 ),
 ( 0.000000000000000000, 0.0001954339857564076099, 0.0003908679715128152198, 0.0005863019572692228839, 0.0007817359430256304396 ),
 .UNSPECIFIED. ) ;
#18936=VERTEX_POINT ( 'NONE', #7860 ) ;
#18937=VERTEX_POINT ( 'NONE', #20919 ) ;
#18938=ORIENTED_EDGE ( 'NONE', *, *, #11854, .F. ) ;
#18939=CARTESIAN_POINT ( 'NONE',  ( 3.480823650682683734, -12.65882529074907126, 30.72640787790839312 ) ) ;
#18940=EDGE_LOOP ( 'NONE', ( #77451, #12774, #8534, #51812 ) ) ;
#18941=AXIS2_PLACEMENT_3D ( 'NONE', #26835, #82226, #88559 ) ;
#18942=CARTESIAN_POINT ( 'NONE',  ( -14.17716686945866655, -11.04252011169590020, 33.62494198852677130 ) ) ;
#18943=CARTESIAN_POINT ( 'NONE',  ( 9.626225312947559232, -5.471508081941602875, 34.59228464037088457 ) ) ;
#18945=DIRECTION ( 'NONE',  ( -0.000000000000000000, -0.000000000000000000, -1.000000000000000000 ) ) ;
#18947=ORIENTED_EDGE ( 'NONE', *, *, #23837, .T. ) ;
#18948=CARTESIAN_POINT ( 'NONE',  ( 17.07692307692295586, -10.21337939537710326, 33.94971097300076224 ) ) ;
#18949=EDGE_LOOP ( 'NONE', ( #53486, #40201, #81068, #62648 ) ) ;
#18950=CARTESIAN_POINT ( 'NONE',  ( -12.21153846153852385, -7.565270000091922853, 34.99999999999999289 ) ) ;
#18951=EDGE_CURVE ( 'NONE', #31652, #5133, #13215, .T. ) ;
#18952=B_SPLINE_CURVE_WITH_KNOTS ( 'NONE', 3,
 ( #21811, #2849, #57806, #42098, #69553, #63233, #7859, #35321, #84414, #83974 ),
 .UNSPECIFIED., .F., .F.,
 ( 4, 2, 2, 2, 4 ),
 ( 0.000000000000000000, 0.0001954311564186867931, 0.0003908623128373735862, 0.0005862934692560603251, 0.0007817246256747471724 ),
 .UNSPECIFIED. ) ;
#18956=B_SPLINE_CURVE_WITH_KNOTS ( 'NONE', 3,
 ( #37557, #86221, #3779, #66374, #59165, #31708, #4679, #32153, #24044, #71789 ),
 .UNSPECIFIED., .F., .F.,
 ( 4, 2, 2, 2, 4 ),
 ( 0.000000000000000000, 0.0001954339857564090194, 0.0003908679715128180387, 0.0005863019572692270039, 0.0007817359430256360774 ),
 .UNSPECIFIED. ) ;
#18957=FACE_BOUND ( 'NONE', #60681, .T. ) ;
#18958=CARTESIAN_POINT ( 'NONE',  ( 17.32697749683652688, -6.523592122091590895, 34.90882529074906415 ) ) ;
#18960=EDGE_CURVE ( 'NONE', #33835, #74655, #28579, .T. ) ;
#18961=DIRECTION ( 'NONE',  ( -0.000000000000000000, -0.8660254037844399289, -0.4999999999999980016 ) ) ;
#18962=CARTESIAN_POINT ( 'NONE',  ( -3.360916440207450062, -4.460286881179643004, 33.72017969459903242 ) ) ;
#18964=CARTESIAN_POINT ( 'NONE',  ( 17.20744877868664346, -9.417988943895561960, 34.36773134775778260 ) ) ;
#18967=EDGE_LOOP ( 'NONE', ( #35135, #6756 ) ) ;
#18968=EDGE_LOOP ( 'NONE', ( #6863, #8734, #27594, #80406 ) ) ;
#18969=EDGE_CURVE ( 'NONE', #23968, #25274, #37085, .T. ) ;
#18970=LINE ( 'NONE', #87007, #46071 ) ;
#18971=CARTESIAN_POINT ( 'NONE',  ( -14.30769230769230660, -12.37446782046654192, 30.86335684631486131 ) ) ;
#18972=CARTESIAN_POINT ( 'NONE',  ( 3.007284306204900837, -3.562934362175799841, 33.22335522853832401 ) ) ;
#18973=DIRECTION ( 'NONE',  ( -0.000000000000000000, 0.8660254037844397068, -0.4999999999999978906 ) ) ;
#18974=CARTESIAN_POINT ( 'NONE',  ( 8.519230769230768274, -7.500000000000001776, 35.00000000000000000 ) ) ;
#18975=CARTESIAN_POINT ( 'NONE',  ( -15.23076923076935074, -3.835265460704628371, 33.15142922262033665 ) ) ;
#18976=VERTEX_POINT ( 'NONE', #30339 ) ;
#18977=CARTESIAN_POINT ( 'NONE',  ( 17.14217864819909920, -3.300289026998473929, 32.46337939537591666 ) ) ;
#18978=CARTESIAN_POINT ( 'NONE',  ( 11.76188850032310995, -7.630147231320743018, 34.74852402298682819 ) ) ;
#18979=CARTESIAN_POINT ( 'NONE',  ( -14.55771554498526932, -8.432397168068783699, 34.66272746175022945 ) ) ;
#18980=CARTESIAN_POINT ( 'NONE',  ( -16.15384615384627409, -4.320704448113951379, 33.92786785259630022 ) ) ;
#18982=VERTEX_POINT ( 'NONE', #24015 ) ;
#18983=B_SPLINE_CURVE_WITH_KNOTS ( 'NONE', 3,
 ( #64048, #8243, #84795, #76694, #28509, #42917, #1917, #16319, #62717, #43784 ),
 .UNSPECIFIED., .F., .F.,
 ( 4, 2, 2, 2, 4 ),
 ( 0.0007817246256747457630, 0.0009771112852218887673, 0.001172497944769031880, 0.001367884604316174993, 0.001563271263863318106 ),
 .UNSPECIFIED. ) ;
#18984=VERTEX_POINT ( 'NONE', #63678 ) ;
#18986=ORIENTED_EDGE ( 'NONE', *, *, #19777, .T. ) ;
#18987=CARTESIAN_POINT ( 'NONE',  ( 10.39189969082028675, -4.225889041578353655, 33.85425143139329407 ) ) ;
#18988=CARTESIAN_POINT ( 'NONE',  ( -13.31935981333936070, -10.90142922261932057, 33.41473453929631887 ) ) ;
#18989=ORIENTED_EDGE ( 'NONE', *, *, #4651, .T. ) ;
#18990=DIRECTION ( 'NONE',  ( -0.000000000000000000, -0.7660444431189791237, -0.6427876096865379196 ) ) ;
#18991=CARTESIAN_POINT ( 'NONE',  ( 14.30769230769218581, -5.941354392335915335, 34.76329471203413846 ) ) ;
#18992=CARTESIAN_POINT ( 'NONE',  ( 5.010839665967195877, -6.386643153685125363, 34.62446782046654903 ) ) ;
#18993=ADVANCED_FACE ( 'NONE', ( #64113 ), #49725, .F. ) ;
#18994=CARTESIAN_POINT ( 'NONE',  ( -17.01166750564705055, -12.27809138561124591, 31.22303859784720359 ) ) ;
#18995=DIRECTION ( 'NONE',  ( -0.000000000000000000, -0.9848077530122086864, -0.1736481776669273613 ) ) ;
#18996=ORIENTED_EDGE ( 'NONE', *, *, #50810, .T. ) ;
#18997=CARTESIAN_POINT ( 'NONE',  ( -15.48074597481782178, -12.01397095200674059, 32.43157075238190146 ) ) ;
#18998=VERTEX_POINT ( 'NONE', #29468 ) ;
#18999=CARTESIAN_POINT ( 'NONE',  ( 18.25000000000000000, -7.500000000000001776, 35.04278698407183867 ) ) ;
#19000=DIRECTION ( 'NONE',  ( -0.000000000000000000, 0.6427876096865404731, -0.7660444431189770143 ) ) ;
#19001=CARTESIAN_POINT ( 'NONE',  ( 15.23076923076923173, -1.422936976036506707, 30.56769352161908415 ) ) ;
#19002=CARTESIAN_POINT ( 'NONE',  ( -10.68146699474474914, -3.322132147404559532, 32.92929555188719348 ) ) ;
#19003=CARTESIAN_POINT ( 'NONE',  ( -8.769230769230768274, -8.164416787775445883, 34.95778746994557906 ) ) ;
#19004=CYLINDRICAL_SURFACE ( 'NONE', #26260, 0.2499999999999986955 ) ;
#19005=CARTESIAN_POINT ( 'NONE',  ( -6.923076923076922462, -6.189225973068211317, 35.74407628777942847 ) ) ;
#19007=ORIENTED_EDGE ( 'NONE', *, *, #56503, .F. ) ;
#19009=CARTESIAN_POINT ( 'NONE',  ( 7.911298626873478845, -7.750023224968868085, 34.99404313364389907 ) ) ;
#19010=VECTOR ( 'NONE', #20586, 1000.000000000000114 ) ;
#19011=CARTESIAN_POINT ( 'NONE',  ( -13.31935981333936425, -8.613356846314928816, 34.62446782046653482 ) ) ;
#19013=LINE ( 'NONE', #10025, #84386 ) ;
#19014=CYLINDRICAL_SURFACE ( 'NONE', #8089, 0.2499999999999998890 ) ;
#19015=CARTESIAN_POINT ( 'NONE',  ( 13.13459214732242408, -3.711651800289232028, 33.01384336483936011 ) ) ;
#19016=CIRCLE ( 'NONE', #20428, 0.2500000000000002220 ) ;
#19017=CARTESIAN_POINT ( 'NONE',  ( -10.68146699474474914, -2.292212530054419606, 30.41441678777542634 ) ) ;
#19021=B_SPLINE_CURVE_WITH_KNOTS ( 'NONE', 3,
 ( #9014, #30163, #2232, #37346, #17988, #57629, #29727, #37800, #84682, #65706 ),
 .UNSPECIFIED., .F., .F.,
 ( 4, 2, 2, 2, 4 ),
 ( 0.000000000000000000, 0.0001954311564186876876, 0.0003908623128373753751, 0.0005862934692560630356, 0.0007817246256747507503 ),
 .UNSPECIFIED. ) ;
#19022=CARTESIAN_POINT ( 'NONE',  ( 5.777073782483851616, -3.586966769969700763, 32.86292498521069660 ) ) ;
#19023=EDGE_CURVE ( 'NONE', #33753, #74977, #22933, .T. ) ;
#19024=EDGE_CURVE ( 'NONE', #12150, #68060, #29338, .T. ) ;
#19025=DIRECTION ( 'NONE',  ( 0.000000000000000000, 0.1736481776669275834, 0.9848077530122086864 ) ) ;
#19026=CARTESIAN_POINT ( 'NONE',  ( -3.296852641725111166, -11.69971097300155272, 32.46337939537587403 ) ) ;
#19027=ORIENTED_EDGE ( 'NONE', *, *, #52524, .F. ) ;
#19028=CARTESIAN_POINT ( 'NONE',  ( 10.55011461482829738, -9.528491918058357157, 34.59228464037090589 ) ) ;
#19030=VERTEX_POINT ( 'NONE', #16382 ) ;
#19031=CARTESIAN_POINT ( 'NONE',  ( 13.38461538461538680, -3.513871655860378418, 32.76840700105978499 ) ) ;
#19032=CARTESIAN_POINT ( 'NONE',  ( 11.66925197942848769, -6.369690395747422684, 34.87708834333098196 ) ) ;
#19033=EDGE_LOOP ( 'NONE', ( #12628, #52204 ) ) ;
#19034=EDGE_CURVE ( 'NONE', #44514, #21774, #66986, .T. ) ;
#19035=CARTESIAN_POINT ( 'NONE',  ( -7.846153846153844924, -3.322132147404559976, 32.92929555188717927 ) ) ;
#19036=CARTESIAN_POINT ( 'NONE',  ( -14.53055857075540658, -2.251424796025575326, 29.88072029997477586 ) ) ;
#19037=CARTESIAN_POINT ( 'NONE',  ( -9.692307692307812417, -2.625532179533778709, 30.86335684631627174 ) ) ;
#19038=CARTESIAN_POINT ( 'NONE',  ( 8.519230769230768274, -7.566083408709835645, 34.74999999999999289 ) ) ;
#19039=CARTESIAN_POINT ( 'NONE',  ( -4.826977667545033768, -8.476813868363244353, 34.90874843262270133 ) ) ;
#19040=ORIENTED_EDGE ( 'NONE', *, *, #61465, .T. ) ;
#19041=CARTESIAN_POINT ( 'NONE',  ( -4.088591014333315066, -12.51329471203373700, 31.30864560766537963 ) ) ;
#19042=ORIENTED_EDGE ( 'NONE', *, *, #22386, .F. ) ;
#19043=AXIS2_PLACEMENT_3D ( 'NONE', #53129, #11723, #45038 ) ;
#19044=CARTESIAN_POINT ( 'NONE',  ( -15.09997878980228059, -6.369690395747422684, 34.87708834333098196 ) ) ;
#19045=EDGE_CURVE ( 'NONE', #20445, #65338, #8911, .T. ) ;
#19046=CARTESIAN_POINT ( 'NONE',  ( -12.46153846153846168, -2.833524468853757305, 32.15551576947925838 ) ) ;
#19047=CARTESIAN_POINT ( 'NONE',  ( -3.100721624513547159, -7.723484964179500700, 34.74522123443823318 ) ) ;
#19048=DIRECTION ( 'NONE',  ( -0.000000000000000000, -0.9396926207859093161, -0.3420201433256663259 ) ) ;
#19049=EDGE_CURVE ( 'NONE', #63003, #48826, #21822, .T. ) ;
#19050=CARTESIAN_POINT ( 'NONE',  ( -4.153846153846274980, -10.33852847137269571, 34.16647553114546554 ) ) ;
#19053=ORIENTED_EDGE ( 'NONE', *, *, #66481, .T. ) ;
#19054=B_SPLINE_CURVE_WITH_KNOTS ( 'NONE', 3,
 ( #85458, #79145, #23741, #71937, #10248, #30941, #17446, #68951, #7261, #34726 ),
 .UNSPECIFIED., .F., .F.,
 ( 4, 2, 2, 2, 4 ),
 ( 0.0007817246256747477145, 0.0009771112852218907189, 0.001172497944769033615, 0.001367884604316176511, 0.001563271263863319407 ),
 .UNSPECIFIED. ) ;
#19055=ORIENTED_EDGE ( 'NONE', *, *, #11365, .T. ) ;
#19059=CARTESIAN_POINT ( 'NONE',  ( -10.36533030374629938, -11.28795663066794575, 33.01431243580653785 ) ) ;
#19060=CARTESIAN_POINT ( 'NONE',  ( -2.084912766423894670, -3.236590943229497253, 32.36255958852954251 ) ) ;
#19061=CARTESIAN_POINT ( 'NONE',  ( -15.29685264172511161, -10.51840700105979387, 33.73612834413961536 ) ) ;
#19062=EDGE_CURVE ( 'NONE', #71506, #28072, #4649, .T. ) ;
#19064=VECTOR ( 'NONE', #3696, 999.9999999999998863 ) ;
#19065=DIRECTION ( 'NONE',  ( -0.000000000000000000, 0.1736481776669307198, -0.9848077530122080203 ) ) ;
#19066=DIRECTION ( 'NONE',  ( -0.000000000000000000, -0.8660254037844397068, -0.4999999999999978906 ) ) ;
#19067=CARTESIAN_POINT ( 'NONE',  ( -4.853911725310227077, -4.187068189119697692, 33.49521262558774026 ) ) ;
#19069=ORIENTED_EDGE ( 'NONE', *, *, #29492, .F. ) ;
#19070=EDGE_LOOP ( 'NONE', ( #66329, #88051 ) ) ;
#19073=CARTESIAN_POINT ( 'NONE',  ( -13.45069776397551742, -12.34228464037088280, 31.77849191805838558 ) ) ;
#19074=EDGE_CURVE ( 'NONE', #23084, #67515, #24459, .T. ) ;
#19075=ORIENTED_EDGE ( 'NONE', *, *, #10202, .T. ) ;
#19076=CARTESIAN_POINT ( 'NONE',  ( 7.622668902429897919, -3.236172620538810385, 32.36188796281390267 ) ) ;
#19077=CARTESIAN_POINT ( 'NONE',  ( -5.999999999999998224, -3.513871655860378418, 32.76840700105978499 ) ) ;
#19078=CARTESIAN_POINT ( 'NONE',  ( 16.02323579422162680, -7.722926236386454590, 34.74524107206102030 ) ) ;
#19079=CYLINDRICAL_SURFACE ( 'NONE', #86876, 0.2499999999999973355 ) ;
#19080=FACE_BOUND ( 'NONE', #26655, .T. ) ;
#19081=ORIENTED_EDGE ( 'NONE', *, *, #18308, .F. ) ;
#19082=EDGE_CURVE ( 'NONE', #57294, #80708, #45414, .T. ) ;
#19083=VERTEX_POINT ( 'NONE', #87086 ) ;
#19084=CARTESIAN_POINT ( 'NONE',  ( 17.32686848630112308, -5.766571408460170467, 34.70601412856602508 ) ) ;
#19085=EDGE_LOOP ( 'NONE', ( #20370, #1239 ) ) ;
#19086=FACE_BOUND ( 'NONE', #35534, .T. ) ;
#19087=DIRECTION ( 'NONE',  ( -0.000000000000000000, -0.7660444431189791237, -0.6427876096865379196 ) ) ;
#19088=B_SPLINE_CURVE_WITH_KNOTS ( 'NONE', 3,
 ( #65631, #23759, #71956, #37728, #38173, #52125, #31875, #37279, #64745, #30092 ),
 .UNSPECIFIED., .F., .F.,
 ( 4, 2, 2, 2, 4 ),
 ( 0.0007817246256747460882, 0.0009771112852218892010, 0.001172497944769032314, 0.001367884604316175210, 0.001563271263863318323 ),
 .UNSPECIFIED. ) ;
#19089=CARTESIAN_POINT ( 'NONE',  ( 7.976198902073619479, -2.254550872974306674, 29.97347326024527092 ) ) ;
#19090=EDGE_LOOP ( 'NONE', ( #32436, #51061 ) ) ;
#19091=CARTESIAN_POINT ( 'NONE',  ( -7.053767526187233905, -9.929715669179216775, 34.40415004197138416 ) ) ;
#19095=B_SPLINE_CURVE_WITH_KNOTS ( 'NONE', 3,
 ( #12828, #88512, #644, #69104, #34865, #62334, #47494, #48379, #40313, #61011 ),
 .UNSPECIFIED., .F., .F.,
 ( 4, 2, 2, 2, 4 ),
 ( 0.000000000000000000, 0.0001954339857564079894, 0.0003908679715128159787, 0.0005863019572692239681, 0.0007817359430256319575 ),
 .UNSPECIFIED. ) ;
#19096=CARTESIAN_POINT ( 'NONE',  ( -7.780898706641007578, -8.656820664281605460, 34.87096338111211224 ) ) ;
#19097=CARTESIAN_POINT ( 'NONE',  ( -18.00000000000012079, -5.219633306517615701, 34.19971097300220464 ) ) ;
#19099=CARTESIAN_POINT ( 'NONE',  ( -3.230769230769229949, -2.708943851104267164, 35.45975837776705220 ) ) ;
#19100=ORIENTED_EDGE ( 'NONE', *, *, #65978, .T. ) ;
#19101=EDGE_CURVE ( 'NONE', #78927, #7315, #20628, .T. ) ;
#19102=LINE ( 'NONE', #40268, #67533 ) ;
#19103=VECTOR ( 'NONE', #15143, 1000.000000000000227 ) ;
#19104=CARTESIAN_POINT ( 'NONE',  ( -15.45425417449318317, -4.386631170607604879, 33.66268669641500111 ) ) ;
#19105=VERTEX_POINT ( 'NONE', #74002 ) ;
#19106=CYLINDRICAL_SURFACE ( 'NONE', #75912, 0.2500000000000008882 ) ;
#19107=LINE ( 'NONE', #12346, #33967 ) ;
#19108=CARTESIAN_POINT ( 'NONE',  ( 0.5923289025054110368, -10.70102852606553157, 33.91149625220312913 ) ) ;
#19110=CARTESIAN_POINT ( 'NONE',  ( -16.15384615384627409, -4.481592998941358097, 33.73612834414048933 ) ) ;
#19111=CARTESIAN_POINT ( 'NONE',  ( 6.700150705560775855, -9.086856451489516928, 34.49173150075333183 ) ) ;
#19112=CARTESIAN_POINT ( 'NONE',  ( 6.250054311638313820, -11.79725096376909299, 32.30694842903960762 ) ) ;
#19113=CARTESIAN_POINT ( 'NONE',  ( 9.823098133274644539, -4.684288915650983043, 34.18129842949671371 ) ) ;
#19115=CARTESIAN_POINT ( 'NONE',  ( -6.700297381808512753, -2.847695495035524882, 31.58253572463339509 ) ) ;
#19118=CARTESIAN_POINT ( 'NONE',  ( -4.087778820496076548, -5.471508081941601098, 34.59228464037088457 ) ) ;
#19119=EDGE_LOOP ( 'NONE', ( #51920, #56415, #17380, #55887 ) ) ;
#19120=ORIENTED_EDGE ( 'NONE', *, *, #4631, .F. ) ;
#19121=LINE ( 'NONE', #47019, #58472 ) ;
#19123=CARTESIAN_POINT ( 'NONE',  ( -0.4615384615384611200, -13.04860791097971706, 34.73218667398347037 ) ) ;
#19126=CARTESIAN_POINT ( 'NONE',  ( 10.74617505635156789, -2.494656445102012565, 31.33466734024120015 ) ) ;
#19127=CARTESIAN_POINT ( 'NONE',  ( 9.822833130541338775, -9.503571793651731880, 34.60286762892837942 ) ) ;
#19128=CARTESIAN_POINT ( 'NONE',  ( -8.638438961405983108, -4.809403383903225304, 33.96459661697924304 ) ) ;
#19129=CARTESIAN_POINT ( 'NONE',  ( -15.48074597481782178, -4.818429247618089661, 34.26397095200675125 ) ) ;
#19130=FACE_OUTER_BOUND ( 'NONE', #56912, .T. ) ;
#19132=CARTESIAN_POINT ( 'NONE',  ( 14.30769230769231015, -3.669653830205710676, 35.88435417666054406 ) ) ;
#19134=CARTESIAN_POINT ( 'NONE',  ( 5.750023255951409951, -3.436278759898155677, 33.07459398097509506 ) ) ;
#19136=EDGE_CURVE ( 'NONE', #44956, #9090, #59585, .T. ) ;
#19138=VERTEX_POINT ( 'NONE', #5541 ) ;
#19140=CARTESIAN_POINT ( 'NONE',  ( -11.28851602011339672, -5.852078868378309373, 34.47109172314383585 ) ) ;
#19142=DIRECTION ( 'NONE',  ( -0.000000000000000000, 0.5000000000000011102, -0.8660254037844380415 ) ) ;
#19143=CARTESIAN_POINT ( 'NONE',  ( -6.130691466667561151, -3.530157926970578508, 32.79014554554150607 ) ) ;
#19145=CARTESIAN_POINT ( 'NONE',  ( 8.703960323269994248, -4.481592998940162609, 33.73612834413957984 ) ) ;
#19147=CARTESIAN_POINT ( 'NONE',  ( -16.40382288478850725, -9.148715823498378086, 34.47080413974185120 ) ) ;
#19148=EDGE_CURVE ( 'NONE', #87474, #23981, #60028, .T. ) ;
#19149=ORIENTED_EDGE ( 'NONE', *, *, #3036, .T. ) ;
#19150=CARTESIAN_POINT ( 'NONE',  ( -18.00000000000000000, -1.546599033411489632, 31.05360187035683239 ) ) ;
#19151=ORIENTED_EDGE ( 'NONE', *, *, #85914, .T. ) ;
#19152=EDGE_CURVE ( 'NONE', #29922, #78448, #4601, .T. ) ;
#19153=ORIENTED_EDGE ( 'NONE', *, *, #31105, .T. ) ;
#19154=CARTESIAN_POINT ( 'NONE',  ( -8.519285359852727169, -4.932303261841489928, 34.32971442181322885 ) ) ;
#19155=CARTESIAN_POINT ( 'NONE',  ( -14.08491263871423982, -6.717445702608402236, 34.94155399931962336 ) ) ;
#19156=CARTESIAN_POINT ( 'NONE',  ( -4.403822897894743349, -12.65889640711025521, 30.72598325615533454 ) ) ;
#19158=FACE_OUTER_BOUND ( 'NONE', #67542, .T. ) ;
#19159=ORIENTED_EDGE ( 'NONE', *, *, #449, .T. ) ;
#19161=AXIS2_PLACEMENT_3D ( 'NONE', #45936, #73428, #87398 ) ;
#19162=B_SPLINE_CURVE_WITH_KNOTS ( 'NONE', 3,
 ( #18539, #51390, #30705, #30274, #86564, #45997, #58171, #24834, #17191, #44649 ),
 .UNSPECIFIED., .F., .F.,
 ( 4, 2, 2, 2, 4 ),
 ( 0.000000000000000000, 0.0001954339857564081249, 0.0003908679715128162498, 0.0005863019572692244018, 0.0007817359430256324996 ),
 .UNSPECIFIED. ) ;
#19163=VECTOR ( 'NONE', #71442, 1000.000000000000227 ) ;
#19164=ORIENTED_EDGE ( 'NONE', *, *, #39305, .F. ) ;
#19165=EDGE_LOOP ( 'NONE', ( #19081, #29717 ) ) ;
#19166=CARTESIAN_POINT ( 'NONE',  ( 5.869308533332442401, -2.541943142973490666, 30.39792223712631980 ) ) ;
#19167=CARTESIAN_POINT ( 'NONE',  ( -0.3962833220256234412, -10.33852847137154107, 34.16647553114620450 ) ) ;
#19168=ADVANCED_FACE ( 'NONE', ( #67244 ), #66346, .F. ) ;
#19169=LINE ( 'NONE', #44844, #4861 ) ;
#19170=CARTESIAN_POINT ( 'NONE',  ( 4.153846153846154188, -13.20930481340135110, 34.54067556320372745 ) ) ;
#19171=CARTESIAN_POINT ( 'NONE',  ( 17.93391762063986050, -2.833524468853757305, 32.15551576947924417 ) ) ;
#19172=EDGE_CURVE ( 'NONE', #4579, #83312, #16392, .T. ) ;
#19173=DIRECTION ( 'NONE',  ( 0.000000000000000000, 0.9848077530122072432, -0.1736481776669354937 ) ) ;
#19174=VERTEX_POINT ( 'NONE', #27576 ) ;
#19176=CARTESIAN_POINT ( 'NONE',  ( 17.29970261819148192, -12.44528174975671853, 30.48912976160715615 ) ) ;
#19178=CARTESIAN_POINT ( 'NONE',  ( -5.999999999999998224, -1.466349020453238561, 30.81389545987213907 ) ) ;
#19179=CARTESIAN_POINT ( 'NONE',  ( 12.46153846153846168, -8.164416787775445883, 34.95778746994557906 ) ) ;
#19181=ORIENTED_EDGE ( 'NONE', *, *, #81536, .T. ) ;
#19183=EDGE_CURVE ( 'NONE', #81991, #29682, #48614, .T. ) ;
#19184=CARTESIAN_POINT ( 'NONE',  ( -1.161835715637318689, -11.60474049983370648, 33.02348890104160262 ) ) ;
#19185=EDGE_LOOP ( 'NONE', ( #44579, #60243, #81332, #19164 ) ) ;
#19186=CARTESIAN_POINT ( 'NONE',  ( 13.51514082284902862, -11.04252011169590020, 33.62494198852677130 ) ) ;
#19187=CARTESIAN_POINT ( 'NONE',  ( 0.2115617174898700992, -11.47974371597208076, 33.17467449705390692 ) ) ;
#19188=AXIS2_PLACEMENT_3D ( 'NONE', #78936, #53236, #80738 ) ;
#19189=FACE_BOUND ( 'NONE', #88005, .T. ) ;
#19190=CARTESIAN_POINT ( 'NONE',  ( -4.946131269098289707, -12.11778462344220841, 31.66786338562085135 ) ) ;
#19192=CARTESIAN_POINT ( 'NONE',  ( -14.05769230769230660, -2.499999999999998668, 29.75000000000000355 ) ) ;
#19193=VERTEX_POINT ( 'NONE', #68560 ) ;
#19194=CARTESIAN_POINT ( 'NONE',  ( 11.53846153846153832, -11.35647404775217417, 33.31231777344666511 ) ) ;
#19196=FACE_OUTER_BOUND ( 'NONE', #41609, .T. ) ;
#19198=ORIENTED_EDGE ( 'NONE', *, *, #2543, .T. ) ;
#19199=B_SPLINE_CURVE_WITH_KNOTS ( 'NONE', 3,
 ( #3350, #30822, #58292, #24066, #51514, #79015, #17315, #72253, #51975, #41812 ),
 .UNSPECIFIED., .F., .F.,
 ( 4, 2, 2, 2, 4 ),
 ( 0.0007817246336856291692, 0.0009771112958940103739, 0.001172497958102391470, 0.001367884620310772566, 0.001563271282519153879 ),
 .UNSPECIFIED. ) ;
#19201=CARTESIAN_POINT ( 'NONE',  ( -15.00798956179115962, -5.827830569534417471, 34.72679350104403539 ) ) ;
#19202=CARTESIAN_POINT ( 'NONE',  ( -12.71156169883142795, -12.22074536777954989, 31.39888409691088356 ) ) ;
#19203=CARTESIAN_POINT ( 'NONE',  ( -8.769230769230768274, -8.318370150425687726, 35.83090037661290239 ) ) ;
#19204=EDGE_CURVE ( 'NONE', #75911, #6016, #17356, .T. ) ;
#19205=LINE ( 'NONE', #80014, #78896 ) ;
#19206=EDGE_CURVE ( 'NONE', #8429, #65065, #78604, .T. ) ;
#19207=FACE_BOUND ( 'NONE', #45401, .T. ) ;
#19208=LINE ( 'NONE', #73720, #69140 ) ;
#19209=CARTESIAN_POINT ( 'NONE',  ( 4.219101293358990645, -12.70778746994558439, 30.41441678777537305 ) ) ;
#19210=CARTESIAN_POINT ( 'NONE',  ( -15.23076923076922995, -1.242168528481310874, 33.36296068462461051 ) ) ;
#19211=DIRECTION ( 'NONE',  ( -0.000000000000000000, 0.1736481776669307198, -0.9848077530122080203 ) ) ;
#19212=FACE_OUTER_BOUND ( 'NONE', #54201, .T. ) ;
#19213=CARTESIAN_POINT ( 'NONE',  ( 8.834485908743603844, -12.70778746994558439, 30.41441678777536595 ) ) ;
#19217=CARTESIAN_POINT ( 'NONE',  ( -12.52729188985179221, -7.249945578846652694, 34.99404164642496795 ) ) ;
#19219=CARTESIAN_POINT ( 'NONE',  ( -18.00000000000000000, -3.322132147404558200, 32.92929555188717217 ) ) ;
#19221=CARTESIAN_POINT ( 'NONE',  ( 2.307692307692309264, -2.292212530054420494, 30.41441678777542634 ) ) ;
#19223=CARTESIAN_POINT ( 'NONE',  ( -4.826868657009622865, -9.233818618650603938, 34.70587769442853698 ) ) ;
#19224=EDGE_LOOP ( 'NONE', ( #69815, #10270, #3989, #81479 ) ) ;
#19225=CARTESIAN_POINT ( 'NONE',  ( -16.82697766754503377, -2.341251567377310217, 30.72681386836322659 ) ) ;
#19226=DIRECTION ( 'NONE',  ( -0.000000000000000000, 0.9396926207859092051, -0.3420201433256662704 ) ) ;
#19228=B_SPLINE_CURVE_WITH_KNOTS ( 'NONE', 3,
 ( #83319, #28817, #20718, #14404, #40999, #35116, #61248, #33791, #62580, #49524 ),
 .UNSPECIFIED., .F., .F.,
 ( 4, 2, 2, 2, 4 ),
 ( 0.0007817359527651104954, 0.0009771254036996493593, 0.001172514854634188223, 0.001367904305568727087, 0.001563293756503265951 ),
 .UNSPECIFIED. ) ;
#19229=CARTESIAN_POINT ( 'NONE',  ( 4.376857505459002873, -10.61302985866383963, 33.66295027996417843 ) ) ;
#19230=CARTESIAN_POINT ( 'NONE',  ( -7.173053667125515176, -12.65889640711025521, 30.72598325615533454 ) ) ;
#19231=VECTOR ( 'NONE', #27994, 1000.000000000000227 ) ;
#19232=CARTESIAN_POINT ( 'NONE',  ( -4.854143407945010757, -12.11081565061823717, 32.26097654155341843 ) ) ;
#19233=CARTESIAN_POINT ( 'NONE',  ( -0.6844654204453100022, -8.282780595021769443, 34.94152052738834868 ) ) ;
#19234=CARTESIAN_POINT ( 'NONE',  ( 0.2386122440223135410, -11.24512374952581872, 33.06303171183252942 ) ) ;
#19235=CARTESIAN_POINT ( 'NONE',  ( -8.899922235898328537, -8.999036380462717588, 34.52022231692819076 ) ) ;
#19237=CARTESIAN_POINT ( 'NONE',  ( 5.326868486301116867, -2.589246495874657938, 31.60778113518102828 ) ) ;
#19238=CARTESIAN_POINT ( 'NONE',  ( 8.096099255531889582, -9.357781135181031829, 34.66075350412533851 ) ) ;
#19240=CARTESIAN_POINT ( 'NONE',  ( 16.40390057375961064, -4.818054556918155207, 34.26375889529406749 ) ) ;
#19241=CARTESIAN_POINT ( 'NONE',  ( -15.23076923076922995, -11.11383981884818262, 36.00935417666054406 ) ) ;
#19243=CARTESIAN_POINT ( 'NONE',  ( -10.83886953994894853, -2.612411019501189369, 31.66733052389439962 ) ) ;
#19244=CARTESIAN_POINT ( 'NONE',  ( 5.076923076923075762, -6.343179335718451384, 34.87096338111211935 ) ) ;
#19245=EDGE_LOOP ( 'NONE', ( #37499, #47780, #64998, #32145 ) ) ;
#19248=CARTESIAN_POINT ( 'NONE',  ( 8.992010438208827949, -2.612705202774698421, 31.66806509827799943 ) ) ;
#19249=ORIENTED_EDGE ( 'NONE', *, *, #44932, .T. ) ;
#19250=CARTESIAN_POINT ( 'NONE',  ( -13.44988538517170440, -10.33852847137145048, 34.16647553114627556 ) ) ;
#19251=CARTESIAN_POINT ( 'NONE',  ( -2.373015223184481215, -7.749976743299137993, 34.99404534957040624 ) ) ;
#19252=CARTESIAN_POINT ( 'NONE',  ( 2.241608896736428047, -12.37446782046654192, 30.86335684631486487 ) ) ;
#19253=CARTESIAN_POINT ( 'NONE',  ( 11.76124107972994359, -9.332535724633409302, 34.40230450496446934 ) ) ;
#19255=CARTESIAN_POINT ( 'NONE',  ( 6.923076923076924238, -9.819645486525091727, 36.12317359536749706 ) ) ;
#19258=CARTESIAN_POINT ( 'NONE',  ( -13.38461538461550759, -8.656820664282941280, 34.87096338111179961 ) ) ;
#19259=ORIENTED_EDGE ( 'NONE', *, *, #79178, .T. ) ;
#19260=VERTEX_POINT ( 'NONE', #20815 ) ;
#19261=B_SPLINE_CURVE_WITH_KNOTS ( 'NONE', 3,
 ( #9195, #76758, #69111, #70887, #77193, #34873, #56483, #15502, #7416, #21809 ),
 .UNSPECIFIED., .F., .F.,
 ( 4, 2, 2, 2, 4 ),
 ( 0.000000000000000000, 0.0001954311564186881213, 0.0003908623128373762425, 0.0005862934692560643367, 0.0007817246256747524850 ),
 .UNSPECIFIED. ) ;
#19262=AXIS2_PLACEMENT_3D ( 'NONE', #10505, #65440, #3733 ) ;
#19263=ORIENTED_EDGE ( 'NONE', *, *, #49174, .F. ) ;
#19264=VECTOR ( 'NONE', #45165, 1000.000000000000227 ) ;
#19265=CARTESIAN_POINT ( 'NONE',  ( -9.942330929600657896, -2.823816976329319051, 31.52131813110795733 ) ) ;
#19267=DIRECTION ( 'NONE',  ( -0.000000000000000000, -0.3420201433256694901, -0.9396926207859082059 ) ) ;
#19268=ADVANCED_FACE ( 'NONE', ( #12735 ), #48284, .F. ) ;
#19269=CARTESIAN_POINT ( 'NONE',  ( -7.846153846153844924, -10.67929555188718282, 33.92786785259544047 ) ) ;
#19270=VERTEX_POINT ( 'NONE', #67682 ) ;
#19272=ORIENTED_EDGE ( 'NONE', *, *, #29559, .F. ) ;
#19273=DIRECTION ( 'NONE',  ( -0.000000000000000000, -0.9848077530122085754, -0.1736481776669273613 ) ) ;
#19274=VERTEX_POINT ( 'NONE', #40659 ) ;
#19275=CARTESIAN_POINT ( 'NONE',  ( 3.230769230769546141, -2.255955759149395501, 30.00000000000324363 ) ) ;
#19276=CARTESIAN_POINT ( 'NONE',  ( -0.4615384615384611200, -12.29105614889573062, 35.45975837776705220 ) ) ;
#19277=FACE_OUTER_BOUND ( 'NONE', #1663, .T. ) ;
#19278=EDGE_CURVE ( 'NONE', #39220, #48663, #71097, .T. ) ;
#19280=ORIENTED_EDGE ( 'NONE', *, *, #62108, .F. ) ;
#19281=VERTEX_POINT ( 'NONE', #84754 ) ;
#19282=AXIS2_PLACEMENT_3D ( 'NONE', #27944, #22512, #22074 ) ;
#19283=VERTEX_POINT ( 'NONE', #57706 ) ;
#19284=CARTESIAN_POINT ( 'NONE',  ( 14.43848274865925774, -10.70102852606553157, 33.91149625220312913 ) ) ;
#19285=CARTESIAN_POINT ( 'NONE',  ( -8.769230769230892619, -11.67786785259630911, 32.92929555188603530 ) ) ;
#19286=VERTEX_POINT ( 'NONE', #56812 ) ;
#19287=CARTESIAN_POINT ( 'NONE',  ( 17.07692307692295586, -5.941354392335915335, 34.76329471203413846 ) ) ;
#19289=VERTEX_POINT ( 'NONE', #77537 ) ;
#19290=EDGE_CURVE ( 'NONE', #35211, #37367, #29163, .T. ) ;
#19291=CARTESIAN_POINT ( 'NONE',  ( 16.21991450484859598, -8.120952969808772792, 34.71129190929999453 ) ) ;
#19292=CARTESIAN_POINT ( 'NONE',  ( -3.903791842207837259, -4.943051570960391494, 34.04725096376909477 ) ) ;
#19294=FACE_BOUND ( 'NONE', #57557, .T. ) ;
#19295=CARTESIAN_POINT ( 'NONE',  ( -0.5276218724943426697, -9.780366693483667717, 34.19971097300155805 ) ) ;
#19296=LINE ( 'NONE', #12982, #81679 ) ;
#19297=CARTESIAN_POINT ( 'NONE',  ( 15.90384615384615330, -7.500000000000001776, 35.00000000000000000 ) ) ;
#19298=DIRECTION ( 'NONE',  ( 1.000000000000000000, 0.000000000000000000, 0.000000000000000000 ) ) ;
#19299=DIRECTION ( 'NONE',  ( 0.000000000000000000, 0.4999999999999960032, -0.8660254037844410391 ) ) ;
#19300=CARTESIAN_POINT ( 'NONE',  ( 16.15384615384603251, -6.835583212225970762, 34.95778746994575670 ) ) ;
#19301=CARTESIAN_POINT ( 'NONE',  ( 13.38461538461538680, -2.517432740324522911, 35.29906147534542527 ) ) ;
#19302=VERTEX_POINT ( 'NONE', #63122 ) ;
#19303=CARTESIAN_POINT ( 'NONE',  ( -17.07692307692307665, -5.471508081941601098, 34.59228464037088457 ) ) ;
#19304=CARTESIAN_POINT ( 'NONE',  ( -13.38461538461538325, -3.937682226553329556, 33.60647404775216529 ) ) ;
#19305=ORIENTED_EDGE ( 'NONE', *, *, #33220, .F. ) ;
#19306=ORIENTED_EDGE ( 'NONE', *, *, #23798, .F. ) ;
#19308=CARTESIAN_POINT ( 'NONE',  ( 15.93091993633000136, -3.586966769969702540, 32.86292498521069660 ) ) ;
#19309=CARTESIAN_POINT ( 'NONE',  ( -15.29652603328353955, -7.249945686854186278, 34.74374336980224598 ) ) ;
#19310=EDGE_LOOP ( 'NONE', ( #28637, #73773, #20944, #49197 ) ) ;
#19311=CARTESIAN_POINT ( 'NONE',  ( 14.53070365930516061, -9.086983370893049639, 34.49168942202179267 ) ) ;
#19312=EDGE_CURVE ( 'NONE', #69245, #77080, #49621, .T. ) ;
#19314=CARTESIAN_POINT ( 'NONE',  ( -13.38461538461550759, -10.33852847137269571, 34.16647553114546554 ) ) ;
#19316=FACE_BOUND ( 'NONE', #6549, .T. ) ;
#19317=CARTESIAN_POINT ( 'NONE',  ( -39.05038313613820122, -2.249999999999998668, 29.75000000000000355 ) ) ;
#19319=CARTESIAN_POINT ( 'NONE',  ( 2.307692307692309264, -6.343179335718451384, 34.87096338111211935 ) ) ;
#19320=CARTESIAN_POINT ( 'NONE',  ( -8.769230769230768274, -9.819645486525091727, 36.12317359536749706 ) ) ;
#19321=CARTESIAN_POINT ( 'NONE',  ( -8.703162418228332697, -12.10708131394839882, 31.69288490824020954 ) ) ;
#19322=APPLICATION_CONTEXT ( 'automotive_design' ) ;
#19324=EDGE_LOOP ( 'NONE', ( #13265, #78729, #20761, #67941 ) ) ;
#19326=ORIENTED_EDGE ( 'NONE', *, *, #74241, .F. ) ;
#19327=AXIS2_PLACEMENT_3D ( 'NONE', #4027, #52219, #73848 ) ;
#19329=CARTESIAN_POINT ( 'NONE',  ( 16.28463796167094557, -6.413143153341454017, 34.63066358083362672 ) ) ;
#19330=FACE_OUTER_BOUND ( 'NONE', #15044, .T. ) ;
#19331=CARTESIAN_POINT ( 'NONE',  ( -0.2115384615383979761, -7.434744429011175271, 34.75000000000000711 ) ) ;
#19332=CARTESIAN_POINT ( 'NONE',  ( -15.16470087976679082, -2.721908614388772296, 31.22303859784725333 ) ) ;
#19334=CARTESIAN_POINT ( 'NONE',  ( -7.715362038329059757, -8.147973898785416225, 34.70805048591653730 ) ) ;
#19335=DIRECTION ( 'NONE',  ( 0.000000000000000000, 0.7660444431189807890, 0.6427876096865361433 ) ) ;
#19337=CARTESIAN_POINT ( 'NONE',  ( 5.777073041093149897, -10.01117774369187252, 34.36070679894347535 ) ) ;
#19338=CARTESIAN_POINT ( 'NONE',  ( -9.942330929600657896, -11.37209801155882971, 32.91403422569032955 ) ) ;
#19339=CARTESIAN_POINT ( 'NONE',  ( 13.25392391794783187, -4.118384482072086072, 33.43331474514187107 ) ) ;
#19340=B_SPLINE_CURVE_WITH_KNOTS ( 'NONE', 3,
 ( #28548, #83050, #62752, #38290, #56007, #3604, #76729, #8722, #50128, #15033 ),
 .UNSPECIFIED., .F., .F.,
 ( 4, 2, 2, 2, 4 ),
 ( 0.000000000000000000, 0.0001954339857564063360, 0.0003908679715128126719, 0.0005863019572692189808, 0.0007817359430256253438 ),
 .UNSPECIFIED. ) ;
#19342=CARTESIAN_POINT ( 'NONE',  ( 4.153846153846154188, -12.37446782046654192, 30.86335684631486131 ) ) ;
#19343=CARTESIAN_POINT ( 'NONE',  ( -3.296852641725108946, -8.120952969808774569, 34.71129190930000163 ) ) ;
#19344=CARTESIAN_POINT ( 'NONE',  ( -15.36091644020745051, -10.19110544564092002, 33.96427741523702792 ) ) ;
#19345=EDGE_LOOP ( 'NONE', ( #6192, #22689, #44127, #64651 ) ) ;
#19346=CARTESIAN_POINT ( 'NONE',  ( 9.019285189144222059, -4.818054556918156983, 34.26375889529406749 ) ) ;
#19347=DIRECTION ( 'NONE',  ( -0.000000000000000000, -0.1736481776669307198, -0.9848077530122080203 ) ) ;
#19349=DIRECTION ( 'NONE',  ( -0.000000000000000000, 0.3420201433256694346, -0.9396926207859080948 ) ) ;
#19350=CARTESIAN_POINT ( 'NONE',  ( -11.40767109749459074, -4.684288915650983043, 34.18129842949671371 ) ) ;
#19351=CARTESIAN_POINT ( 'NONE',  ( 10.48490943030889788, -7.276987145209184327, 34.99546412871779211 ) ) ;
#19354=CARTESIAN_POINT ( 'NONE',  ( 17.07692307692307665, -2.486705287966279876, 31.30864560766543647 ) ) ;
#19355=ORIENTED_EDGE ( 'NONE', *, *, #86846, .T. ) ;
#19356=CARTESIAN_POINT ( 'NONE',  ( -11.31508605268911793, -2.251407671071268712, 29.88021292934943318 ) ) ;
#19358=CARTESIAN_POINT ( 'NONE',  ( -17.86920819217521483, -3.530189275343200705, 32.79018710029568240 ) ) ;
#19359=ORIENTED_EDGE ( 'NONE', *, *, #73893, .F. ) ;
#19361=CARTESIAN_POINT ( 'NONE',  ( -15.36091720050093024, -3.069018819979302926, 32.56621877034667278 ) ) ;
#19362=DIRECTION ( 'NONE',  ( -0.000000000000000000, -0.6427876096865404731, -0.7660444431189771253 ) ) ;
#19364=ORIENTED_EDGE ( 'NONE', *, *, #74843, .F. ) ;
#19365=ORIENTED_EDGE ( 'NONE', *, *, #60821, .F. ) ;
#19366=CARTESIAN_POINT ( 'NONE',  ( -16.02332071561251325, -2.372941743896878286, 30.88044141588253311 ) ) ;
#19367=LINE ( 'NONE', #18926, #57011 ) ;
#19368=FACE_OUTER_BOUND ( 'NONE', #49953, .T. ) ;
#19369=CARTESIAN_POINT ( 'NONE',  ( -10.86536134632696715, -2.564618984488975073, 30.55390908950641915 ) ) ;
#19370=CARTESIAN_POINT ( 'NONE',  ( -5.999999999999998224, -1.242168528481310874, 33.36296068462461051 ) ) ;
#19371=CARTESIAN_POINT ( 'NONE',  ( 15.23076923076923173, -12.29105614889573062, 35.45975837776705220 ) ) ;
#19372=CARTESIAN_POINT ( 'NONE',  ( 11.47237812750565666, -11.69971097300155272, 32.46337939537587403 ) ) ;
#19373=EDGE_CURVE ( 'NONE', #68660, #21721, #49580, .T. ) ;
#19374=DIRECTION ( 'NONE',  ( 0.000000000000000000, 0.8660254037844377084, -0.5000000000000015543 ) ) ;
#19375=EDGE_CURVE ( 'NONE', #79832, #57707, #66803, .T. ) ;
#19376=B_SPLINE_CURVE_WITH_KNOTS ( 'NONE', 3,
 ( #5879, #39226, #19389, #47293, #74337, #12636, #13074, #11748, #54048, #88756 ),
 .UNSPECIFIED., .F., .F.,
 ( 4, 2, 2, 2, 4 ),
 ( 0.0007817246256747463051, 0.0009771112852218896347, 0.001172497944769032747, 0.001367884604316176077, 0.001563271263863319407 ),
 .UNSPECIFIED. ) ;
#19377=VECTOR ( 'NONE', #69259, 1000.000000000000000 ) ;
#19378=ORIENTED_EDGE ( 'NONE', *, *, #41998, .T. ) ;
#19379=ORIENTED_EDGE ( 'NONE', *, *, #86886, .T. ) ;
#19380=ORIENTED_EDGE ( 'NONE', *, *, #33487, .F. ) ;
#19381=CARTESIAN_POINT ( 'NONE',  ( 18.25005441991345734, -9.233818618650598609, 34.70587769442853698 ) ) ;
#19382=ORIENTED_EDGE ( 'NONE', *, *, #10662, .F. ) ;
#19383=VECTOR ( 'NONE', #22913, 1000.000000000000114 ) ;
#19384=VECTOR ( 'NONE', #54666, 1000.000000000000000 ) ;
#19385=ADVANCED_FACE ( 'NONE', ( #85184 ), #50923, .F. ) ;
#19386=CARTESIAN_POINT ( 'NONE',  ( 11.66898697669518725, -3.625058011473228703, 33.29252011169590020 ) ) ;
#19387=FACE_OUTER_BOUND ( 'NONE', #61654, .T. ) ;
#19388=VERTEX_POINT ( 'NONE', #71652 ) ;
#19389=CARTESIAN_POINT ( 'NONE',  ( -12.33101302330481808, -11.66157788607254098, 32.95092075102925833 ) ) ;
#19390=ORIENTED_EDGE ( 'NONE', *, *, #82314, .F. ) ;
#19392=VERTEX_POINT ( 'NONE', #56381 ) ;
#19395=CARTESIAN_POINT ( 'NONE',  ( -4.153846153846152411, -3.937682226553329556, 33.60647404775216529 ) ) ;
#19396=CARTESIAN_POINT ( 'NONE',  ( -9.469344558041020932, -7.369474539155828730, 34.99858011523957657 ) ) ;
#19397=FACE_BOUND ( 'NONE', #66494, .T. ) ;
#19398=CARTESIAN_POINT ( 'NONE',  ( -6.000000000000119904, -6.026961402154118908, 34.52809138561165270 ) ) ;
#19399=CARTESIAN_POINT ( 'NONE',  ( 15.93036122928181975, -3.562934362175799841, 33.22335522853832401 ) ) ;
#19403=CARTESIAN_POINT ( 'NONE',  ( 10.61538461538461675, -10.67929555188718282, 33.92786785259544047 ) ) ;
#19404=CARTESIAN_POINT ( 'NONE',  ( -13.16123944391720180, -2.501478030877323455, 29.88021232661721172 ) ) ;
#19405=VERTEX_POINT ( 'NONE', #9957 ) ;
#19406=ORIENTED_EDGE ( 'NONE', *, *, #45927, .F. ) ;
#19408=LINE ( 'NONE', #67602, #31748 ) ;
#19409=CARTESIAN_POINT ( 'NONE',  ( 2.438484115517093986, -10.54018710029568595, 33.71981072465678864 ) ) ;
#19410=DIRECTION ( 'NONE',  ( -0.000000000000000000, 0.8660254037844399289, -0.4999999999999980016 ) ) ;
#19411=CARTESIAN_POINT ( 'NONE',  ( -14.37296230824862953, -12.16647553114622049, 32.15551576947930812 ) ) ;
#19412=CARTESIAN_POINT ( 'NONE',  ( -17.32694630114453460, -12.45566812827425096, 31.48439005359158926 ) ) ;
#19415=EDGE_CURVE ( 'NONE', #50940, #23267, #18484, .T. ) ;
#19416=CARTESIAN_POINT ( 'NONE',  ( 2.241608896736428491, -8.973038597847271092, 34.52809138561120506 ) ) ;
#19417=CARTESIAN_POINT ( 'NONE',  ( 14.30769230769231015, -11.16473453929635440, 33.15142922261926373 ) ) ;
#19418=DIRECTION ( 'NONE',  ( 0.000000000000000000, 0.7660444431189807890, 0.6427876096865361433 ) ) ;
#19419=EDGE_CURVE ( 'NONE', #65478, #19138, #15285, .T. ) ;
#19420=CARTESIAN_POINT ( 'NONE',  ( -6.988346923633241836, -6.835583212224499938, 34.95778746994557906 ) ) ;
#19421=ORIENTED_EDGE ( 'NONE', *, *, #6437, .F. ) ;
#19422=VERTEX_POINT ( 'NONE', #18057 ) ;
#19423=B_SPLINE_CURVE_WITH_KNOTS ( 'NONE', 3,
 ( #56133, #69206, #28669, #1183, #8841, #1639, #63327, #36315, #63767, #55680 ),
 .UNSPECIFIED., .F., .F.,
 ( 4, 2, 2, 2, 4 ),
 ( 0.000000000000000000, 0.0001954339857564055499, 0.0003908679715128110998, 0.0005863019572692165955, 0.0007817359430256221996 ),
 .UNSPECIFIED. ) ;
#19426=EDGE_CURVE ( 'NONE', #42127, #35784, #1225, .T. ) ;
#19427=CARTESIAN_POINT ( 'NONE',  ( 10.36536139116316058, -4.175268141568685643, 33.81360843649122216 ) ) ;
#19428=ADVANCED_FACE ( 'NONE', ( #45521 ), #65344, .F. ) ;
#19431=CARTESIAN_POINT ( 'NONE',  ( -5.999999999999998224, -9.058645607665452459, 34.76329471203371924 ) ) ;
#19432=CYLINDRICAL_SURFACE ( 'NONE', #35163, 0.2500000000000008882 ) ;
#19433=B_SPLINE_CURVE_WITH_KNOTS ( 'NONE', 3,
 ( #15480, #88607, #1955, #83498, #33637, #8724, #70866, #47137, #77613, #77169 ),
 .UNSPECIFIED., .F., .F.,
 ( 4, 2, 2, 2, 4 ),
 ( 0.000000000000000000, 0.0001954311564186860613, 0.0003908623128373721225, 0.0005862934692560581567, 0.0007817246256747442451 ),
 .UNSPECIFIED. ) ;
#19434=CARTESIAN_POINT ( 'NONE',  ( 14.24193550517800055, -7.249945686854186278, 34.74374336980224598 ) ) ;
#19435=CARTESIAN_POINT ( 'NONE',  ( -12.46153846153846168, -2.517432740324522911, 35.29906147534542527 ) ) ;
#19436=ORIENTED_EDGE ( 'NONE', *, *, #85018, .F. ) ;
#19437=DIRECTION ( 'NONE',  ( -0.000000000000000000, 0.9396926207859094271, -0.3420201433256663259 ) ) ;
#19438=VERTEX_POINT ( 'NONE', #10855 ) ;
#19440=CARTESIAN_POINT ( 'NONE',  ( 8.769230769230768274, -12.34228464037088635, 31.77849191805839268 ) ) ;
#19441=LINE ( 'NONE', #88371, #73141 ) ;
#19442=CARTESIAN_POINT ( 'NONE',  ( -3.230769230769351186, -9.442884908241554243, 34.35708131394783038 ) ) ;
#19443=CARTESIAN_POINT ( 'NONE',  ( -4.153846153846152411, -4.661471528628507777, 34.16647553114623292 ) ) ;
#19444=VECTOR ( 'NONE', #43670, 1000.000000000000000 ) ;
#19448=VERTEX_POINT ( 'NONE', #46412 ) ;
#19449=CARTESIAN_POINT ( 'NONE',  ( 13.38461538461538680, -6.386643153685126251, 34.62446782046654192 ) ) ;
#19450=CARTESIAN_POINT ( 'NONE',  ( 7.846153846153846700, -2.517432740324522911, 35.29906147534542527 ) ) ;
#19451=CARTESIAN_POINT ( 'NONE',  ( -13.16183584334697265, -8.496831190052096971, 34.64984203495476578 ) ) ;
#19452=ORIENTED_EDGE ( 'NONE', *, *, #19415, .F. ) ;
#19453=CARTESIAN_POINT ( 'NONE',  ( 10.61538461538461675, -3.937682226553329556, 33.60647404775216529 ) ) ;
#19455=VECTOR ( 'NONE', #36873, 1000.000000000000114 ) ;
#19456=CARTESIAN_POINT ( 'NONE',  ( -6.988347369037697376, -6.026961402152685388, 34.52809138561120506 ) ) ;
#19457=CARTESIAN_POINT ( 'NONE',  ( 7.053868730901711182, -5.582136614379148654, 34.36778462344220486 ) ) ;
#19458=CARTESIAN_POINT ( 'NONE',  ( 0.4615384615384611200, -2.292212530054420494, 30.41441678777542634 ) ) ;
#19459=ORIENTED_EDGE ( 'NONE', *, *, #15179, .F. ) ;
#19460=EDGE_CURVE ( 'NONE', #38816, #81366, #72214, .T. ) ;
#19461=CARTESIAN_POINT ( 'NONE',  ( -3.164701897419154530, -12.62096338111211757, 30.90682066428152908 ) ) ;
#19462=B_SPLINE_CURVE_WITH_KNOTS ( 'NONE', 3,
 ( #8032, #827, #68839, #48557, #35502, #8923, #1261, #62511, #63405, #49012 ),
 .UNSPECIFIED., .F., .F.,
 ( 4, 2, 2, 2, 4 ),
 ( 0.0007817246256747446788, 0.0009771112852218874663, 0.001172497944769030145, 0.001367884604316172825, 0.001563271263863315720 ),
 .UNSPECIFIED. ) ;
#19463=CARTESIAN_POINT ( 'NONE',  ( 17.20744877868664346, -6.001044277235009439, 34.52024696741798948 ) ) ;
#19464=CARTESIAN_POINT ( 'NONE',  ( -2.084679463598910765, -5.582272713120728369, 34.63742843783360570 ) ) ;
#19465=B_SPLINE_CURVE_WITH_KNOTS ( 'NONE', 3,
 ( #15331, #77029, #64374, #83349, #76585, #22959 ),
 .UNSPECIFIED., .F., .F.,
 ( 4, 2, 4 ),
 ( 0.000000000000000000, 0.0001954784845028908655, 0.0003909569690057817311 ),
 .UNSPECIFIED. ) ;
#19466=ORIENTED_EDGE ( 'NONE', *, *, #81414, .T. ) ;
#19468=ORIENTED_EDGE ( 'NONE', *, *, #23312, .T. ) ;
#19469=DIRECTION ( 'NONE',  ( -0.000000000000000000, 0.6427876096865404731, -0.7660444431189770143 ) ) ;
#19471=ORIENTED_EDGE ( 'NONE', *, *, #22493, .T. ) ;
#19472=DIRECTION ( 'NONE',  ( -0.000000000000000000, 0.3420201433256694901, -0.9396926207859082059 ) ) ;
#19473=CARTESIAN_POINT ( 'NONE',  ( -11.31545018684868964, -12.39991518177334129, 30.74647679643404530 ) ) ;
#19475=EDGE_CURVE ( 'NONE', #58032, #40441, #72997, .T. ) ;
#19476=AXIS2_PLACEMENT_3D ( 'NONE', #78307, #77869, #23799 ) ;
#19477=CARTESIAN_POINT ( 'NONE',  ( -7.912236225513983534, -4.661471528628507777, 34.16647553114621871 ) ) ;
#19478=CARTESIAN_POINT ( 'NONE',  ( -0.4615384615385840772, -11.67786785259630911, 32.92929555188603530 ) ) ;
#19479=ORIENTED_EDGE ( 'NONE', *, *, #22242, .F. ) ;
#19481=ORIENTED_EDGE ( 'NONE', *, *, #67814, .T. ) ;
#19482=CARTESIAN_POINT ( 'NONE',  ( -5.076923076923199218, -6.835583212225970762, 34.95778746994575670 ) ) ;
#19483=CARTESIAN_POINT ( 'NONE',  ( -12.21159305216042057, -2.986452184633680229, 32.43230066228895225 ) ) ;
#19484=EDGE_CURVE ( 'NONE', #66313, #32743, #66686, .T. ) ;
#19485=CARTESIAN_POINT ( 'NONE',  ( 4.826946345980720920, -11.79746400365624659, 32.30657167506340954 ) ) ;
#19486=CARTESIAN_POINT ( 'NONE',  ( 3.230769230769231726, -11.35647404775217417, 33.31231777344666511 ) ) ;
#19489=VERTEX_POINT ( 'NONE', #25697 ) ;
#19490=VERTEX_POINT ( 'NONE', #39675 ) ;
#19491=EDGE_LOOP ( 'NONE', ( #83193, #43775 ) ) ;
#19492=B_SPLINE_CURVE_WITH_KNOTS ( 'NONE', 3,
 ( #43718, #71186, #36954, #65317, #45933, #3615, #71625, #51329, #25675, #4967 ),
 .UNSPECIFIED., .F., .F.,
 ( 4, 2, 2, 2, 4 ),
 ( 0.000000000000000000, 0.0001954339857564075557, 0.0003908679715128151114, 0.0005863019572692226671, 0.0007817359430256302227 ),
 .UNSPECIFIED. ) ;
#19493=ORIENTED_EDGE ( 'NONE', *, *, #81941, .T. ) ;
#19494=VECTOR ( 'NONE', #55639, 1000.000000000000227 ) ;
#19495=CARTESIAN_POINT ( 'NONE',  ( -5.326899820971668476, -4.075325502946086864, 33.72974371597207721 ) ) ;
#19496=EDGE_CURVE ( 'NONE', #30224, #28230, #67135, .T. ) ;
#19497=CARTESIAN_POINT ( 'NONE',  ( 16.28437159207980045, -11.04252011169589842, 33.62494198852677840 ) ) ;
#19498=CARTESIAN_POINT ( 'NONE',  ( -10.36543920600657209, -4.932303261841489928, 34.32971442181322885 ) ) ;
#19499=CARTESIAN_POINT ( 'NONE',  ( 5.999999999999880096, -12.27809138561165270, 31.22303859784587132 ) ) ;
#19500=CARTESIAN_POINT ( 'NONE',  ( -5.299849294439221481, -10.61292498521070549, 33.66303323003028680 ) ) ;
#19501=CARTESIAN_POINT ( 'NONE',  ( -5.076923076923197442, -8.613356846316285953, 34.62446782046622218 ) ) ;
#19502=FACE_OUTER_BOUND ( 'NONE', #32125, .T. ) ;
#19504=EDGE_LOOP ( 'NONE', ( #42197, #924, #80542, #85617 ) ) ;
#19506=AXIS2_PLACEMENT_3D ( 'NONE', #88426, #6868, #81654 ) ;
#19507=ORIENTED_EDGE ( 'NONE', *, *, #64324, .F. ) ;
#19508=ORIENTED_EDGE ( 'NONE', *, *, #78903, .F. ) ;
#19509=CARTESIAN_POINT ( 'NONE',  ( -10.61538461538430589, -2.506253911140614576, 30.00000000000323297 ) ) ;
#19510=ORIENTED_EDGE ( 'NONE', *, *, #9085, .T. ) ;
#19511=DIRECTION ( 'NONE',  ( 0.000000000000000000, 0.3420201433256610524, 0.9396926207859113145 ) ) ;
#19512=CARTESIAN_POINT ( 'NONE',  ( -7.976301055592065481, -4.460286881179644780, 33.72017969459903242 ) ) ;
#19514=CYLINDRICAL_SURFACE ( 'NONE', #53739, 0.2499999999999979738 ) ;
#19515=FACE_BOUND ( 'NONE', #27990, .T. ) ;
#19517=EDGE_CURVE ( 'NONE', #12327, #76524, #55009, .T. ) ;
#19518=CARTESIAN_POINT ( 'NONE',  ( -2.980714919130916130, -6.567000820036038355, 34.66262288849541306 ) ) ;
#19519=ORIENTED_EDGE ( 'NONE', *, *, #5953, .F. ) ;
#19520=CYLINDRICAL_SURFACE ( 'NONE', #60095, 0.2499999999999986955 ) ;
#19521=ORIENTED_EDGE ( 'NONE', *, *, #50008, .F. ) ;
#19522=EDGE_CURVE ( 'NONE', #12053, #7293, #79739, .T. ) ;
#19523=FACE_BOUND ( 'NONE', #27479, .T. ) ;
#19524=CARTESIAN_POINT ( 'NONE',  ( 9.942253101685738059, -5.766571408460171355, 34.70601412856602508 ) ) ;
#19525=CYLINDRICAL_SURFACE ( 'NONE', #226, 0.2499999999999995837 ) ;
#19526=VERTEX_POINT ( 'NONE', #47740 ) ;
#19527=VECTOR ( 'NONE', #1721, 999.9999999999998863 ) ;
#19529=CARTESIAN_POINT ( 'NONE',  ( 17.01084069756293715, -11.91647553114624181, 32.58852847137148245 ) ) ;
#19530=EDGE_CURVE ( 'NONE', #46303, #52843, #13072, .T. ) ;
#19531=LINE ( 'NONE', #42809, #36428 ) ;
#19532=ORIENTED_EDGE ( 'NONE', *, *, #41772, .T. ) ;
#19533=CARTESIAN_POINT ( 'NONE',  ( 6.792929713638702793, -10.19110544564092002, 33.96427741523702792 ) ) ;
#19534=CARTESIAN_POINT ( 'NONE',  ( 14.24160992833217421, -11.35647404775217595, 33.31231777344666511 ) ) ;
#19535=CARTESIAN_POINT ( 'NONE',  ( 6.673053685783957967, -12.43535235679832596, 30.55408501211184813 ) ) ;
#19536=CARTESIAN_POINT ( 'NONE',  ( -9.626239341305252495, -2.538708090699994813, 30.37095296980875503 ) ) ;
#19537=VERTEX_POINT ( 'NONE', #67578 ) ;
#19538=CARTESIAN_POINT ( 'NONE',  ( 12.46153846153877609, -2.255955759149395501, 30.00000000000324363 ) ) ;
#19539=DIRECTION ( 'NONE',  ( -0.000000000000000000, -0.8660254037844397068, -0.4999999999999978906 ) ) ;
#19540=ORIENTED_EDGE ( 'NONE', *, *, #13550, .T. ) ;
#19541=CARTESIAN_POINT ( 'NONE',  ( -5.999999999999998224, -13.87047571288749737, 32.06866353760679544 ) ) ;
#19543=CARTESIAN_POINT ( 'NONE',  ( 0.7115928814519127954, -10.82426656108011720, 33.81400080652039009 ) ) ;
#19544=CARTESIAN_POINT ( 'NONE',  ( 16.28463659481310444, -11.93129842949672437, 32.56571108434900452 ) ) ;
#19545=DIRECTION ( 'NONE',  ( -0.000000000000000000, -0.1736481776669307198, -0.9848077530122080203 ) ) ;
#19546=FACE_OUTER_BOUND ( 'NONE', #5098, .T. ) ;
#19547=CARTESIAN_POINT ( 'NONE',  ( 0.6845513056318561773, -11.43677907613345113, 33.22367315496201456 ) ) ;
#19548=CARTESIAN_POINT ( 'NONE',  ( 8.519207545009310323, -2.985938066672154445, 32.43141759479405550 ) ) ;
#19549=DIRECTION ( 'NONE',  ( -0.000000000000000000, 0.8660254037844399289, -0.4999999999999980016 ) ) ;
#19550=ADVANCED_FACE ( 'NONE', ( #82431, #19387 ), #26144, .F. ) ;
#19552=EDGE_LOOP ( 'NONE', ( #74470, #24138, #46729, #21283 ) ) ;
#19553=CARTESIAN_POINT ( 'NONE',  ( 17.86930853333243618, -4.118384482072086072, 33.43331474514187107 ) ) ;
#19554=EDGE_LOOP ( 'NONE', ( #24128, #36190, #33057, #80903 ) ) ;
#19555=EDGE_CURVE ( 'NONE', #26637, #52830, #69986, .T. ) ;
#19557=FACE_OUTER_BOUND ( 'NONE', #67647, .T. ) ;
#19559=CYLINDRICAL_SURFACE ( 'NONE', #55565, 0.2500000000000002220 ) ;
#19561=CARTESIAN_POINT ( 'NONE',  ( 14.37294787896833270, -11.48612834413965977, 32.76840700105972815 ) ) ;
#19562=CARTESIAN_POINT ( 'NONE',  ( -8.834501215191545853, -3.300289026998414865, 32.46337939537583139 ) ) ;
#19563=B_SPLINE_CURVE_WITH_KNOTS ( 'NONE', 3,
 ( #26367, #12847, #35790, #56048, #22264, #42107, #76770, #20926, #83536, #50158 ),
 .UNSPECIFIED., .F., .F.,
 ( 4, 2, 2, 2, 4 ),
 ( 0.000000000000000000, 0.0001954339857564055499, 0.0003908679715128110998, 0.0005863019572692165955, 0.0007817359430256221996 ),
 .UNSPECIFIED. ) ;
#19565=CARTESIAN_POINT ( 'NONE',  ( -5.076923076923199218, -3.643525952248796163, 33.31231777344771672 ) ) ;
#19567=CARTESIAN_POINT ( 'NONE',  ( 2.372947878968333146, -11.48612834413965977, 32.76840700105972815 ) ) ;
#19568=CARTESIAN_POINT ( 'NONE',  ( 6.673100179028333301, -12.41104346484419452, 31.60698883733904196 ) ) ;
#19569=EDGE_CURVE ( 'NONE', #83335, #69315, #31391, .T. ) ;
#19570=VECTOR ( 'NONE', #26198, 1000.000000000000000 ) ;
#19571=CYLINDRICAL_SURFACE ( 'NONE', #50601, 0.2499999999999995559 ) ;
#19572=CARTESIAN_POINT ( 'NONE',  ( -18.00000000000012079, -2.379036618888197285, 30.90682066428292885 ) ) ;
#19574=ADVANCED_FACE ( 'NONE', ( #13951 ), #33785, .F. ) ;
#19575=ADVANCED_FACE ( 'NONE', ( #27030 ), #81988, .F. ) ;
#19576=VERTEX_POINT ( 'NONE', #62142 ) ;
#19577=EDGE_LOOP ( 'NONE', ( #79374, #57904, #22484, #77969 ) ) ;
#19578=CYLINDRICAL_SURFACE ( 'NONE', #67324, 0.2499999999999997502 ) ;
#19579=LINE ( 'NONE', #69100, #37394 ) ;
#19580=CARTESIAN_POINT ( 'NONE',  ( 2.307692307692309264, -6.435427911321262684, 35.78748833219616898 ) ) ;
#19581=CARTESIAN_POINT ( 'NONE',  ( -16.08777780284371417, -12.37446782046654192, 30.86335684631486842 ) ) ;
#19583=FACE_OUTER_BOUND ( 'NONE', #63292, .T. ) ;
#19584=DIRECTION ( 'NONE',  ( -0.000000000000000000, 0.3420201433256694346, -0.9396926207859080948 ) ) ;
#19585=EDGE_CURVE ( 'NONE', #48512, #5871, #9844, .T. ) ;
#19586=CARTESIAN_POINT ( 'NONE',  ( -3.230769230769351186, -5.219633306517616589, 34.19971097300220464 ) ) ;
#19587=ORIENTED_EDGE ( 'NONE', *, *, #33552, .F. ) ;
#19588=CARTESIAN_POINT ( 'NONE',  ( -6.857821351800898135, -10.21337939537593620, 33.94971097300152252 ) ) ;
#19589=ORIENTED_EDGE ( 'NONE', *, *, #27515, .T. ) ;
#19591=CARTESIAN_POINT ( 'NONE',  ( 10.61538461538461675, -12.29105614889573062, 35.45975837776705220 ) ) ;
#19592=CARTESIAN_POINT ( 'NONE',  ( -14.24162497434223162, -6.343179335718452272, 34.87096338111212646 ) ) ;
#19593=B_SPLINE_CURVE_WITH_KNOTS ( 'NONE', 3,
 ( #19431, #54535, #66730, #46894, #12677, #68497, #74378, #73942, #18550, #59967 ),
 .UNSPECIFIED., .F., .F.,
 ( 4, 2, 2, 2, 4 ),
 ( 0.000000000000000000, 0.0001954311564186868202, 0.0003908623128373736404, 0.0005862934692560604335, 0.0007817246256747472808 ),
 .UNSPECIFIED. ) ;
#19594=VECTOR ( 'NONE', #7615, 1000.000000000000114 ) ;
#19595=CARTESIAN_POINT ( 'NONE',  ( -4.377331097570101193, -4.386631170607603991, 33.66268669641500111 ) ) ;
#19596=CARTESIAN_POINT ( 'NONE',  ( 11.53846153846141576, -2.379036618888197729, 30.90682066428292885 ) ) ;
#19597=CARTESIAN_POINT ( 'NONE',  ( 7.846153846153725020, -3.300289026999228881, 32.46337939537708905 ) ) ;
#19598=EDGE_CURVE ( 'NONE', #28403, #2875, #84057, .T. ) ;
#19599=VECTOR ( 'NONE', #13269, 999.9999999999998863 ) ;
#19600=EDGE_LOOP ( 'NONE', ( #67579, #19681, #1910, #85163 ) ) ;
#19602=ORIENTED_EDGE ( 'NONE', *, *, #63165, .T. ) ;
#19603=ORIENTED_EDGE ( 'NONE', *, *, #4753, .F. ) ;
#19605=CARTESIAN_POINT ( 'NONE',  ( 5.076923076923075762, -10.51840700105979565, 33.73612834413961536 ) ) ;
#19608=CARTESIAN_POINT ( 'NONE',  ( 17.74997676270703550, -5.056417327199097755, 34.11270091957320716 ) ) ;
#19609=CARTESIAN_POINT ( 'NONE',  ( 12.46153846153846168, -2.833524468853757305, 32.15551576947925838 ) ) ;
#19610=VERTEX_POINT ( 'NONE', #28348 ) ;
#19611=VERTEX_POINT ( 'NONE', #35563 ) ;
#19612=VERTEX_POINT ( 'NONE', #21594 ) ;
#19613=CARTESIAN_POINT ( 'NONE',  ( -4.153846153846273204, -3.300289026999228881, 32.46337939537708905 ) ) ;
#19615=FACE_OUTER_BOUND ( 'NONE', #32316, .T. ) ;
#19616=FACE_OUTER_BOUND ( 'NONE', #24553, .T. ) ;
#19618=ORIENTED_EDGE ( 'NONE', *, *, #216, .T. ) ;
#19619=B_SPLINE_CURVE_WITH_KNOTS ( 'NONE', 3,
 ( #84109, #22390, #36354, #2115, #790, #29599, #48978, #1229, #77773, #9330 ),
 .UNSPECIFIED., .F., .F.,
 ( 4, 2, 2, 2, 4 ),
 ( 0.000000000000000000, 0.0001954311564186865763, 0.0003908623128373731525, 0.0005862934692560596746, 0.0007817246256747463051 ),
 .UNSPECIFIED. ) ;
#19620=CARTESIAN_POINT ( 'NONE',  ( 3.480769230769245937, -2.249999999999999112, 29.81603969181031033 ) ) ;
#19621=EDGE_LOOP ( 'NONE', ( #30882, #77409, #6725, #85048 ) ) ;
#19622=CARTESIAN_POINT ( 'NONE',  ( 3.230769230769231726, -4.945431358278436385, 36.03766855953609394 ) ) ;
#19623=CARTESIAN_POINT ( 'NONE',  ( 14.37294744720514927, -12.51329471203373345, 31.30864560766537963 ) ) ;
#19624=B_SPLINE_CURVE_WITH_KNOTS ( 'NONE', 3,
 ( #1258, #70168, #48115, #68836, #84146, #7141, #83701, #35048, #34612, #62078 ),
 .UNSPECIFIED., .F., .F.,
 ( 4, 2, 2, 2, 4 ),
 ( 0.000000000000000000, 0.0001954311564186862781, 0.0003908623128373725562, 0.0005862934692560588072, 0.0007817246256747451124 ),
 .UNSPECIFIED. ) ;
#19626=FACE_BOUND ( 'NONE', #84086, .T. ) ;
#19627=DIRECTION ( 'NONE',  ( -0.000000000000000000, -0.000000000000000000, -1.000000000000000000 ) ) ;
#19628=CARTESIAN_POINT ( 'NONE',  ( 8.639083559792549494, -5.195881422630166391, 34.18770438780619259 ) ) ;
#19630=CARTESIAN_POINT ( 'NONE',  ( 6.792385456409365752, -8.147922237126337563, 34.70805685702651999 ) ) ;
#19631=EDGE_CURVE ( 'NONE', #42943, #41914, #40020, .T. ) ;
#19632=VECTOR ( 'NONE', #26224, 1000.000000000000000 ) ;
#19633=LINE ( 'NONE', #81790, #16290 ) ;
#19634=CARTESIAN_POINT ( 'NONE',  ( 15.45378207486262667, -6.460100341425560444, 34.89618726649961644 ) ) ;
#19635=VERTEX_POINT ( 'NONE', #42327 ) ;
#19636=EDGE_CURVE ( 'NONE', #5555, #13671, #70227, .T. ) ;
#19637=CARTESIAN_POINT ( 'NONE',  ( -9.469294848214296678, -4.762714258010881885, 34.23016756924214832 ) ) ;
#19638=CARTESIAN_POINT ( 'NONE',  ( -7.846153846153844924, -11.16473453929635440, 33.15142922261926373 ) ) ;
#19639=CARTESIAN_POINT ( 'NONE',  ( -3.230769230769229949, -13.63283147151868846, 33.57946703557072254 ) ) ;
#19640=FACE_OUTER_BOUND ( 'NONE', #62773, .T. ) ;
#19641=CARTESIAN_POINT ( 'NONE',  ( 8.769230769230768274, -9.905515769479276145, 34.41647553114623292 ) ) ;
#19642=FACE_BOUND ( 'NONE', #69264, .T. ) ;
#19644=FACE_OUTER_BOUND ( 'NONE', #54386, .T. ) ;
#19645=CARTESIAN_POINT ( 'NONE',  ( 17.75000000000000000, -2.249999999999998668, 29.75000000000000355 ) ) ;
#19646=CARTESIAN_POINT ( 'NONE',  ( -18.06608237936013595, -2.292212530054419606, 30.41441678777542634 ) ) ;
#19647=CARTESIAN_POINT ( 'NONE',  ( -9.442253380669377805, -10.66356715214248396, 33.62249196103329751 ) ) ;
#19648=EDGE_CURVE ( 'NONE', #46336, #43624, #80869, .T. ) ;
#19649=CARTESIAN_POINT ( 'NONE',  ( -8.638438961405983108, -3.530189275343204702, 32.79018710029569661 ) ) ;
#19651=ORIENTED_EDGE ( 'NONE', *, *, #87825, .T. ) ;
#19652=CARTESIAN_POINT ( 'NONE',  ( -13.13461538461538325, -2.249999999999998668, 29.75000000000000355 ) ) ;
#19653=ORIENTED_EDGE ( 'NONE', *, *, #73060, .F. ) ;
#19654=CARTESIAN_POINT ( 'NONE',  ( -18.24997674404859183, -3.436278759898155233, 33.07459398097509506 ) ) ;
#19655=VECTOR ( 'NONE', #7848, 1000.000000000000227 ) ;
#19656=EDGE_LOOP ( 'NONE', ( #52512, #63672 ) ) ;
#19657=CARTESIAN_POINT ( 'NONE',  ( 2.307692307692186251, -2.379036618888197285, 30.90682066428292885 ) ) ;
#19658=CARTESIAN_POINT ( 'NONE',  ( 7.846153846153846700, -2.833524468853757305, 32.15551576947925838 ) ) ;
#19659=CARTESIAN_POINT ( 'NONE',  ( -10.74553258511631171, -11.66186481527757302, 32.95055677023626117 ) ) ;
#19660=ORIENTED_EDGE ( 'NONE', *, *, #47569, .T. ) ;
#19661=DIRECTION ( 'NONE',  ( 0.000000000000000000, 0.000000000000000000, 1.000000000000000000 ) ) ;
#19662=CARTESIAN_POINT ( 'NONE',  ( -9.562260086052006613, -7.723484964179501588, 34.74522123443823318 ) ) ;
#19665=DIRECTION ( 'NONE',  ( 0.000000000000000000, 0.9396926207859126468, -0.3420201433256571111 ) ) ;
#19667=CARTESIAN_POINT ( 'NONE',  ( 1.384615384615386802, -4.661471528628507777, 34.16647553114623292 ) ) ;
#19668=CARTESIAN_POINT ( 'NONE',  ( -0.4615384615384611200, -4.098570777380720287, 33.41473453929634729 ) ) ;
#19669=CARTESIAN_POINT ( 'NONE',  ( 9.468822767743363400, -3.562934362175799841, 33.22335522853832401 ) ) ;
#19671=CARTESIAN_POINT ( 'NONE',  ( 5.207713517890026012, -2.494656445102013453, 31.33466734024120015 ) ) ;
#19672=AXIS2_PLACEMENT_3D ( 'NONE', #3910, #71483, #24186 ) ;
#19673=CARTESIAN_POINT ( 'NONE',  ( 6.923076923076802558, -11.48612834414049644, 32.76840700105863391 ) ) ;
#19674=VERTEX_POINT ( 'NONE', #50816 ) ;
#19675=CARTESIAN_POINT ( 'NONE',  ( 6.792467267872841497, -7.722926974430166069, 34.99546784045485737 ) ) ;
#19676=CARTESIAN_POINT ( 'NONE',  ( 17.07692307692307665, -2.499999999999998668, 29.50000000000001066 ) ) ;
#19679=CARTESIAN_POINT ( 'NONE',  ( -16.08859101433330707, -12.51329471203373700, 31.30864560766537963 ) ) ;
#19680=CARTESIAN_POINT ( 'NONE',  ( -11.53846153846153655, -2.499999999999998668, 29.75000000000001421 ) ) ;
#19681=ORIENTED_EDGE ( 'NONE', *, *, #12756, .T. ) ;
#19682=CARTESIAN_POINT ( 'NONE',  ( 4.153846153846154188, -3.937682226553329556, 33.60647404775216529 ) ) ;
#19683=CARTESIAN_POINT ( 'NONE',  ( 3.100077764101670574, -3.530157926970578508, 32.79014554554150607 ) ) ;
#19684=CARTESIAN_POINT ( 'NONE',  ( 4.087763774486018242, -9.058645607665454236, 34.76329471203372634 ) ) ;
#19685=ORIENTED_EDGE ( 'NONE', *, *, #9770, .F. ) ;
#19686=DIRECTION ( 'NONE',  ( -0.000000000000000000, -0.5000000000000009992, -0.8660254037844380415 ) ) ;
#19687=CARTESIAN_POINT ( 'NONE',  ( 2.307692307692187583, -12.46129190930018460, 30.37095296980731973 ) ) ;
#19688=CARTESIAN_POINT ( 'NONE',  ( -12.71151520558705528, -4.818429247618089661, 34.26397095200675125 ) ) ;
#19689=EDGE_CURVE ( 'NONE', #73212, #71584, #48176, .T. ) ;
#19690=VERTEX_POINT ( 'NONE', #63461 ) ;
#19691=CARTESIAN_POINT ( 'NONE',  ( -9.442362282929652295, -2.589246495874658383, 31.60778113518102828 ) ) ;
#19692=CARTESIAN_POINT ( 'NONE',  ( -18.22348494372395322, -12.24155766932282496, 31.33739205006857986 ) ) ;
#19693=VECTOR ( 'NONE', #69750, 1000.000000000000227 ) ;
#19694=EDGE_CURVE ( 'NONE', #67157, #9337, #62473, .T. ) ;
#19695=ADVANCED_FACE ( 'NONE', ( #17947 ), #65668, .F. ) ;
#19696=CARTESIAN_POINT ( 'NONE',  ( 7.173076923078359535, -7.500000000000155431, 34.75000000000007105 ) ) ;
#19697=ORIENTED_EDGE ( 'NONE', *, *, #42274, .F. ) ;
#19698=ORIENTED_EDGE ( 'NONE', *, *, #71480, .T. ) ;
#19699=ORIENTED_EDGE ( 'NONE', *, *, #88636, .F. ) ;
#19700=AXIS2_PLACEMENT_3D ( 'NONE', #6079, #21800, #74533 ) ;
#19701=ORIENTED_EDGE ( 'NONE', *, *, #1547, .T. ) ;
#19702=FACE_OUTER_BOUND ( 'NONE', #71212, .T. ) ;
#19704=VECTOR ( 'NONE', #53922, 999.9999999999998863 ) ;
#19705=FACE_OUTER_BOUND ( 'NONE', #60817, .T. ) ;
#19706=CARTESIAN_POINT ( 'NONE',  ( -16.15384615384627409, -3.643525952248796163, 33.31231777344771672 ) ) ;
#19707=EDGE_CURVE ( 'NONE', #52584, #82252, #66899, .T. ) ;
#19708=DIRECTION ( 'NONE',  ( -0.000000000000000000, 0.6427876096865404731, -0.7660444431189771253 ) ) ;
#19709=ORIENTED_EDGE ( 'NONE', *, *, #6370, .T. ) ;
#19710=EDGE_CURVE ( 'NONE', #18801, #17226, #38655, .T. ) ;
#19712=ORIENTED_EDGE ( 'NONE', *, *, #87956, .F. ) ;
#19713=ORIENTED_EDGE ( 'NONE', *, *, #47736, .F. ) ;
#19714=CARTESIAN_POINT ( 'NONE',  ( -7.146561847641257792, -2.612411019501189813, 31.66733052389439962 ) ) ;
#19715=VERTEX_POINT ( 'NONE', #86871 ) ;
#19716=CARTESIAN_POINT ( 'NONE',  ( -6.700064078983528404, -4.026326845037961455, 33.68677907613344047 ) ) ;
#19717=EDGE_CURVE ( 'NONE', #83441, #13051, #10973, .T. ) ;
#19718=CARTESIAN_POINT ( 'NONE',  ( 6.000000000000001776, -2.486705287966279876, 31.30864560766543647 ) ) ;
#19721=CARTESIAN_POINT ( 'NONE',  ( -15.10024352900566846, -9.417988943895561960, 34.36773134775777550 ) ) ;
#19722=EDGE_LOOP ( 'NONE', ( #84891, #9140, #23023, #23685 ) ) ;
#19723=VERTEX_POINT ( 'NONE', #87312 ) ;
#19724=ORIENTED_EDGE ( 'NONE', *, *, #31584, .F. ) ;
#19725=CARTESIAN_POINT ( 'NONE',  ( 10.83816415665302202, -10.81320215134717344, 33.49497208177562868 ) ) ;
#19726=CARTESIAN_POINT ( 'NONE',  ( -10.61538461538473577, -2.657715359629662544, 31.77849191805970364 ) ) ;
#19728=CARTESIAN_POINT ( 'NONE',  ( 9.442330961365341224, -11.79746400365624659, 32.30657167506340954 ) ) ;
#19729=CARTESIAN_POINT ( 'NONE',  ( -14.37377571864818293, -2.538708090699994813, 30.37095296980875148 ) ) ;
#19730=VERTEX_POINT ( 'NONE', #44504 ) ;
#19731=VECTOR ( 'NONE', #12151, 1000.000000000000000 ) ;
#19732=CARTESIAN_POINT ( 'NONE',  ( 17.07692307692307665, -8.564572088678739092, 35.78748833219616898 ) ) ;
#19733=DIRECTION ( 'NONE',  ( -0.000000000000000000, 1.000000000000000000, 3.491481338843133355E-15 ) ) ;
#19734=CYLINDRICAL_SURFACE ( 'NONE', #59758, 0.2500000000000002220 ) ;
#19735=FACE_BOUND ( 'NONE', #54659, .T. ) ;
#19736=CARTESIAN_POINT ( 'NONE',  ( -0.5268089074992373666, -10.21337939537584383, 33.94971097300158647 ) ) ;
#19738=EDGE_CURVE ( 'NONE', #80479, #83807, #23880, .T. ) ;
#19739=FACE_OUTER_BOUND ( 'NONE', #2326, .T. ) ;
#19740=CARTESIAN_POINT ( 'NONE',  ( 0.2115617174898692943, -6.524016743844655686, 34.90889640711025521 ) ) ;
#19741=DIRECTION ( 'NONE',  ( -0.000000000000000000, 1.000000000000000000, 3.491481338843133355E-15 ) ) ;
#19742=DIRECTION ( 'NONE',  ( 1.000000000000000000, 0.000000000000000000, 0.000000000000000000 ) ) ;
#19743=CARTESIAN_POINT ( 'NONE',  ( 11.53846153846153832, -9.780366693483667717, 34.19971097300155094 ) ) ;
#19744=ORIENTED_EDGE ( 'NONE', *, *, #21658, .F. ) ;
#19745=CARTESIAN_POINT ( 'NONE',  ( -17.14219307747939425, -5.941354392334501355, 34.76329471203369792 ) ) ;
#19747=EDGE_LOOP ( 'NONE', ( #85755, #66963, #57016, #37753 ) ) ;
#19748=ORIENTED_EDGE ( 'NONE', *, *, #71535, .F. ) ;
#19749=CARTESIAN_POINT ( 'NONE',  ( -6.673131404728781746, -5.057305518903949526, 34.11320923018887896 ) ) ;
#19750=ADVANCED_FACE ( 'NONE', ( #3525 ), #31908, .F. ) ;
#19751=CARTESIAN_POINT ( 'NONE',  ( 8.769230769230645706, -12.51329471203414379, 31.30864560766407578 ) ) ;
#19752=CARTESIAN_POINT ( 'NONE',  ( -7.846153846153967493, -2.379036618888197729, 30.90682066428292885 ) ) ;
#19753=ORIENTED_EDGE ( 'NONE', *, *, #25287, .T. ) ;
#19754=CARTESIAN_POINT ( 'NONE',  ( -9.692307692307691624, -9.058645607665452459, 34.76329471203371924 ) ) ;
#19755=CARTESIAN_POINT ( 'NONE',  ( -4.403822897894744237, -9.234221910056348293, 34.70572697212741531 ) ) ;
#19756=FACE_BOUND ( 'NONE', #50047, .T. ) ;
#19760=CARTESIAN_POINT ( 'NONE',  ( -5.076923076923197442, -9.442884908241554243, 34.35708131394783038 ) ) ;
#19762=CARTESIAN_POINT ( 'NONE',  ( -8.519285250882626670, -12.22109172314383052, 31.39792113162168263 ) ) ;
#19763=EDGE_CURVE ( 'NONE', #5737, #40194, #40993, .T. ) ;
#19764=VECTOR ( 'NONE', #58706, 1000.000000000000000 ) ;
#19766=ORIENTED_EDGE ( 'NONE', *, *, #9556, .T. ) ;
#19767=VERTEX_POINT ( 'NONE', #80087 ) ;
#19768=CARTESIAN_POINT ( 'NONE',  ( -9.915234651214539952, -2.523278758544489797, 31.42238647778637528 ) ) ;
#19770=CARTESIAN_POINT ( 'NONE',  ( 12.52770760250111870, -7.250054483168843156, 34.74374881642865631 ) ) ;
#19771=DIRECTION ( 'NONE',  ( -1.000000000000000000, 0.000000000000000000, 0.000000000000000000 ) ) ;
#19772=CARTESIAN_POINT ( 'NONE',  ( -0.6843651540174652270, -7.369208160676172348, 34.74850200257122879 ) ) ;
#19773=CARTESIAN_POINT ( 'NONE',  ( -3.296852641725110722, -5.557115091759785130, 34.35708131394839171 ) ) ;
#19775=CARTESIAN_POINT ( 'NONE',  ( -8.992715693795100051, -10.23692288466677880, 34.23039457007281072 ) ) ;
#19776=CARTESIAN_POINT ( 'NONE',  ( 5.776515075435669111, -3.019605429927184836, 32.48692288466676814 ) ) ;
#19777=EDGE_CURVE ( 'NONE', #47021, #86793, #88378, .T. ) ;
#19778=CARTESIAN_POINT ( 'NONE',  ( 18.00000000000000000, -3.937682226553329556, 33.60647404775216529 ) ) ;
#19780=DIRECTION ( 'NONE',  ( -0.000000000000000000, -0.3420201433256694346, -0.9396926207859080948 ) ) ;
#19781=CARTESIAN_POINT ( 'NONE',  ( 15.10007862765892739, -12.35290016733513951, 31.75349464988449455 ) ) ;
#19782=CARTESIAN_POINT ( 'NONE',  ( -3.230769230769352962, -10.33852847137269571, 34.16647553114546554 ) ) ;
#19783=CARTESIAN_POINT ( 'NONE',  ( -6.792551484843277976, -3.625058011473227815, 33.29252011169590020 ) ) ;
#19784=CARTESIAN_POINT ( 'NONE',  ( -17.07692307692319744, -3.083524468854526912, 32.58852847137268327 ) ) ;
#19786=CARTESIAN_POINT ( 'NONE',  ( -4.826977558574933269, -11.86320923018887541, 32.19269448109604781 ) ) ;
#19787=DIRECTION ( 'NONE',  ( -0.000000000000000000, -0.1736481776669307198, -0.9848077530122080203 ) ) ;
#19789=B_SPLINE_CURVE_WITH_KNOTS ( 'NONE', 3,
 ( #11249, #80612, #60316, #38718, #87371, #66178, #4491, #25651, #53107, #87826 ),
 .UNSPECIFIED., .F., .F.,
 ( 4, 2, 2, 2, 4 ),
 ( 0.0007817246256747482566, 0.0009771112852218926705, 0.001172497944769037084, 0.001367884604316181281, 0.001563271263863325695 ),
 .UNSPECIFIED. ) ;
#19790=CARTESIAN_POINT ( 'NONE',  ( 4.023155550735844521, -4.684245665217972032, 34.18127051446801090 ) ) ;
#19792=DIRECTION ( 'NONE',  ( -0.000000000000000000, -0.1736481776669307198, -0.9848077530122080203 ) ) ;
#19794=CARTESIAN_POINT ( 'NONE',  ( -0.2387589202700528268, -2.600157965045225783, 30.74683119005207743 ) ) ;
#19797=EDGE_CURVE ( 'NONE', #19260, #80757, #51790, .T. ) ;
#19798=CARTESIAN_POINT ( 'NONE',  ( 3.453548899747296730, -8.540255544307065350, 34.89611431652622286 ) ) ;
#19799=EDGE_CURVE ( 'NONE', #11510, #58008, #32790, .T. ) ;
#19800=VERTEX_POINT ( 'NONE', #81875 ) ;
#19801=CARTESIAN_POINT ( 'NONE',  ( 8.769230769230647482, -8.613356846316285953, 34.62446782046622218 ) ) ;
#19802=CARTESIAN_POINT ( 'NONE',  ( 18.00000000000000000, -8.973038597847269315, 34.52809138561121927 ) ) ;
#19803=ORIENTED_EDGE ( 'NONE', *, *, #37081, .T. ) ;
#19804=LINE ( 'NONE', #47266, #77786 ) ;
#19805=CARTESIAN_POINT ( 'NONE',  ( -15.90384615384471800, -7.500000000000155431, 34.75000000000007105 ) ) ;
#19806=EDGE_CURVE ( 'NONE', #84840, #24050, #13400, .T. ) ;
#19807=VECTOR ( 'NONE', #33199, 1000.000000000000114 ) ;
#19808=B_SPLINE_CURVE_WITH_KNOTS ( 'NONE', 3,
 ( #42963, #3284, #30759, #17247, #8738, #1530, #37068, #70433, #36212, #22677 ),
 .UNSPECIFIED., .F., .F.,
 ( 4, 2, 2, 2, 4 ),
 ( 0.0007817359527651096280, 0.0009771254036996484919, 0.001172514854634187573, 0.001367904305568726653, 0.001563293756503265517 ),
 .UNSPECIFIED. ) ;
#19809=CARTESIAN_POINT ( 'NONE',  ( -7.846153846153844924, -3.513871655860378418, 32.76840700105978499 ) ) ;
#19810=ORIENTED_EDGE ( 'NONE', *, *, #30140, .T. ) ;
#19811=EDGE_LOOP ( 'NONE', ( #62538, #26931, #22655, #35586 ) ) ;
#19813=CARTESIAN_POINT ( 'NONE',  ( -15.16551409125639260, -4.320704448112861584, 33.92786785259548310 ) ) ;
#19815=CARTESIAN_POINT ( 'NONE',  ( 18.06525513951284267, -10.33852847137154107, 34.16647553114620450 ) ) ;
#19816=CARTESIAN_POINT ( 'NONE',  ( -10.68065506134538722, -2.625532179533444754, 30.86335684631481513 ) ) ;
#19817=LINE ( 'NONE', #59016, #60567 ) ;
#19818=FACE_OUTER_BOUND ( 'NONE', #49568, .T. ) ;
#19819=DIRECTION ( 'NONE',  ( -0.000000000000000000, -0.5000000000000009992, -0.8660254037844380415 ) ) ;
#19820=CARTESIAN_POINT ( 'NONE',  ( 10.61538461538461675, -12.10708131394839349, 31.69288490824020244 ) ) ;
#19822=EDGE_CURVE ( 'NONE', #4054, #67556, #68790, .T. ) ;
#19823=ORIENTED_EDGE ( 'NONE', *, *, #19648, .F. ) ;
#19824=ORIENTED_EDGE ( 'NONE', *, *, #81922, .F. ) ;
#19825=CARTESIAN_POINT ( 'NONE',  ( 17.99999999999987566, -9.528491918059723176, 34.59228464037033035 ) ) ;
#19826=VERTEX_POINT ( 'NONE', #55270 ) ;
#19827=AXIS2_PLACEMENT_3D ( 'NONE', #26945, #47199, #32809 ) ;
#19829=CARTESIAN_POINT ( 'NONE',  ( 11.76124107972994537, -12.24180327182771855, 31.33663988360758879 ) ) ;
#19830=ORIENTED_EDGE ( 'NONE', *, *, #29370, .F. ) ;
#19831=CARTESIAN_POINT ( 'NONE',  ( 14.43848274865925774, -11.93129842949671726, 32.56571108434900452 ) ) ;
#19832=ORIENTED_EDGE ( 'NONE', *, *, #36064, .T. ) ;
#19833=CARTESIAN_POINT ( 'NONE',  ( 11.78851585009985570, -2.564540009722896752, 30.55348353981670684 ) ) ;
#19834=ORIENTED_EDGE ( 'NONE', *, *, #51576, .T. ) ;
#19835=CARTESIAN_POINT ( 'NONE',  ( 9.822833394071260216, -8.586989748646452369, 34.63063291749215011 ) ) ;
#19836=B_SPLINE_CURVE_WITH_KNOTS ( 'NONE', 3,
 ( #54536, #18992, #20323, #75269, #34272, #26191, #61732, #48, #12678, #54989 ),
 .UNSPECIFIED., .F., .F.,
 ( 4, 2, 2, 2, 4 ),
 ( 0.000000000000000000, 0.0001954339857564077183, 0.0003908679715128154366, 0.0005863019572692231007, 0.0007817359430256308733 ),
 .UNSPECIFIED. ) ;
#19837=EDGE_LOOP ( 'NONE', ( #75794, #59793 ) ) ;
#19838=CARTESIAN_POINT ( 'NONE',  ( -16.15384615384627409, -6.879047030192662504, 34.71129190930017927 ) ) ;
#19839=CARTESIAN_POINT ( 'NONE',  ( 16.82694634598072625, -2.779195860258148798, 31.39871582349836743 ) ) ;
#19840=FACE_BOUND ( 'NONE', #64460, .T. ) ;
#19841=CYLINDRICAL_SURFACE ( 'NONE', #31296, 0.2500000000000009437 ) ;
#19842=CARTESIAN_POINT ( 'NONE',  ( -4.153846153846274980, -11.67786785259630911, 32.92929555188603530 ) ) ;
#19844=CARTESIAN_POINT ( 'NONE',  ( 1.319345384059066983, -12.51329471203370325, 31.30864560766548976 ) ) ;
#19846=FACE_OUTER_BOUND ( 'NONE', #73774, .T. ) ;
#19847=CARTESIAN_POINT ( 'NONE',  ( 15.90382291655318880, -4.335965774309648246, 33.62209801155881905 ) ) ;
#19848=CARTESIAN_POINT ( 'NONE',  ( 1.449808372910040388, -2.255955759149235629, 29.99999999999988631 ) ) ;
#19849=VERTEX_POINT ( 'NONE', #80990 ) ;
#19850=VERTEX_POINT ( 'NONE', #5320 ) ;
#19851=AXIS2_PLACEMENT_3D ( 'NONE', #3913, #85022, #72375 ) ;
#19852=CARTESIAN_POINT ( 'NONE',  ( -5.207613680033384540, -11.93127051446800024, 32.56575433478200665 ) ) ;
#19853=CARTESIAN_POINT ( 'NONE',  ( 1.384615384615386802, -1.466349020453238561, 30.81389545987213907 ) ) ;
#19854=CARTESIAN_POINT ( 'NONE',  ( 3.100621261037536769, -3.625366637846545448, 33.29286588640298561 ) ) ;
#19856=CARTESIAN_POINT ( 'NONE',  ( 8.519230769230766498, -7.566082377512564960, 35.00000000000000711 ) ) ;
#19857=CARTESIAN_POINT ( 'NONE',  ( -13.31854703361294412, -2.721908614388772296, 31.22303859784725333 ) ) ;
#19858=ORIENTED_EDGE ( 'NONE', *, *, #36984, .T. ) ;
#19859=CYLINDRICAL_SURFACE ( 'NONE', #80270, 0.2499999999999994726 ) ;
#19861=CARTESIAN_POINT ( 'NONE',  ( 15.00784227186238162, -4.026226216239094491, 33.68668979543634379 ) ) ;
#19863=CARTESIAN_POINT ( 'NONE',  ( 12.46153846153833911, -6.835583212225970762, 34.95778746994575670 ) ) ;
#19864=ORIENTED_EDGE ( 'NONE', *, *, #69441, .F. ) ;
#19866=B_SPLINE_CURVE_WITH_KNOTS ( 'NONE', 3,
 ( #79297, #66214, #79743, #45047, #86971, #11731, #65763, #32439, #86053, #67562 ),
 .UNSPECIFIED., .F., .F.,
 ( 4, 2, 2, 2, 4 ),
 ( 0.0007817359430256388964, 0.0009771253907250073822, 0.001172514838424375868, 0.001367904286123744571, 0.001563293733823113056 ),
 .UNSPECIFIED. ) ;
#19867=EDGE_LOOP ( 'NONE', ( #21109, #51852 ) ) ;
#19869=B_SPLINE_CURVE_WITH_KNOTS ( 'NONE', 3,
 ( #48880, #54750, #12878, #89009, #27282, #20523, #75038, #54301, #55191, #47988 ),
 .UNSPECIFIED., .F., .F.,
 ( 4, 2, 2, 2, 4 ),
 ( 0.000000000000000000, 0.0001954311564186869557, 0.0003908623128373739115, 0.0005862934692560608672, 0.0007817246256747478229 ),
 .UNSPECIFIED. ) ;
#19870=VERTEX_POINT ( 'NONE', #26924 ) ;
#19871=CARTESIAN_POINT ( 'NONE',  ( 12.46153846153846168, -1.951392089020283160, 34.73218667398347748 ) ) ;
#19872=CARTESIAN_POINT ( 'NONE',  ( 14.43848274865926129, -5.496552790871120031, 34.60292014791297532 ) ) ;
#19873=CARTESIAN_POINT ( 'NONE',  ( 9.692307692307570832, -2.379036618888197729, 30.90682066428292885 ) ) ;
#19874=CARTESIAN_POINT ( 'NONE',  ( -4.153846153846273204, -10.21337939537710326, 33.94971097300076224 ) ) ;
#19875=DIRECTION ( 'NONE',  ( -0.000000000000000000, 0.1736481776669307198, -0.9848077530122080203 ) ) ;
#19876=EDGE_LOOP ( 'NONE', ( #61121, #47462, #26080, #17133 ) ) ;
#19877=CARTESIAN_POINT ( 'NONE',  ( 2.980769230769210409, -2.249999999999999112, 29.81609741502488120 ) ) ;
#19878=CARTESIAN_POINT ( 'NONE',  ( -7.623142494540996239, -9.886259254753566594, 34.14407573483972413 ) ) ;
#19879=ORIENTED_EDGE ( 'NONE', *, *, #16558, .F. ) ;
#19880=DIRECTION ( 'NONE',  ( -0.000000000000000000, 0.8660254037844397068, -0.4999999999999978906 ) ) ;
#19881=LINE ( 'NONE', #88370, #55658 ) ;
#19882=CYLINDRICAL_SURFACE ( 'NONE', #65925, 0.2499999999999986955 ) ;
#19883=CARTESIAN_POINT ( 'NONE',  ( -2.438382910802614045, -12.62707690430377383, 30.88035979386743435 ) ) ;
#19884=CARTESIAN_POINT ( 'NONE',  ( -23.00000000000000000, -10.75000000000000000, 27.25000000000000000 ) ) ;
#19885=CARTESIAN_POINT ( 'NONE',  ( 18.24994551834813805, -2.587454068350149239, 30.68340429815432557 ) ) ;
#19886=LINE ( 'NONE', #68086, #36399 ) ;
#19888=ORIENTED_EDGE ( 'NONE', *, *, #81653, .T. ) ;
#19889=CARTESIAN_POINT ( 'NONE',  ( 11.76124107972994892, -2.847695495035523550, 31.58253572463339154 ) ) ;
#19890=CARTESIAN_POINT ( 'NONE',  ( 12.68431813051652846, -4.989023458446560255, 34.36081565061822118 ) ) ;
#19891=ADVANCED_FACE ( 'NONE', ( #40885 ), #27363, .F. ) ;
#19895=CARTESIAN_POINT ( 'NONE',  ( -7.146003140593070846, -5.667676309546437530, 34.40238873228292249 ) ) ;
#19896=CARTESIAN_POINT ( 'NONE',  ( -4.826923076923076650, -2.499999999999998668, 29.75000000000000355 ) ) ;
#19897=DIRECTION ( 'NONE',  ( -0.000000000000000000, -0.5000000000000009992, -0.8660254037844380415 ) ) ;
#19898=VERTEX_POINT ( 'NONE', #60253 ) ;
#19899=CARTESIAN_POINT ( 'NONE',  ( -16.28453675695646652, -6.369640206132551441, 34.87707690430378449 ) ) ;
#19900=EDGE_CURVE ( 'NONE', #10019, #73835, #13842, .T. ) ;
#19901=LINE ( 'NONE', #47372, #19632 ) ;
#19902=CARTESIAN_POINT ( 'NONE',  ( 5.076923076922953193, -12.51329471203414379, 31.30864560766407578 ) ) ;
#19903=EDGE_LOOP ( 'NONE', ( #20388, #64780 ) ) ;
#19904=CARTESIAN_POINT ( 'NONE',  ( -9.019230769230768274, -7.500000000000001776, 35.00000000000000000 ) ) ;
#19905=EDGE_LOOP ( 'NONE', ( #77698, #25737, #64977, #69074 ) ) ;
#19906=CARTESIAN_POINT ( 'NONE',  ( -2.437839517130529821, -12.27039167877662251, 31.24851455888617835 ) ) ;
#19907=CYLINDRICAL_SURFACE ( 'NONE', #78614, 0.2499999999999998890 ) ;
#19908=ORIENTED_EDGE ( 'NONE', *, *, #9542, .F. ) ;
#19909=CARTESIAN_POINT ( 'NONE',  ( 12.39626801557768943, -3.835265460703609186, 33.15142922261924241 ) ) ;
#19910=DIRECTION ( 'NONE',  ( 0.000000000000000000, 0.9396926207859126468, 0.3420201433256571111 ) ) ;
#19914=CYLINDRICAL_SURFACE ( 'NONE', #66452, 0.2500000000000004996 ) ;
#19915=CARTESIAN_POINT ( 'NONE',  ( -1.607542343522232242, -10.77366814457252175, 33.85459836347579454 ) ) ;
#19921=ORIENTED_EDGE ( 'NONE', *, *, #37247, .F. ) ;
#19922=CARTESIAN_POINT ( 'NONE',  ( 1.384615384615386802, -12.78798330534103123, 29.99999999999997868 ) ) ;
#19923=B_SPLINE_CURVE_WITH_KNOTS ( 'NONE', 3,
 ( #67640, #40616, #73956, #88816, #67199, #41492, #7267, #61746, #46907, #62200 ),
 .UNSPECIFIED., .F., .F.,
 ( 4, 2, 2, 2, 4 ),
 ( 0.000000000000000000, 0.0001954311564186863865, 0.0003908623128373727731, 0.0005862934692560591325, 0.0007817246256747455461 ),
 .UNSPECIFIED. ) ;
#19924=ADVANCED_FACE ( 'NONE', ( #47636 ), #61581, .F. ) ;
#19925=DIRECTION ( 'NONE',  ( -0.000000000000000000, -0.5000000000000009992, -0.8660254037844380415 ) ) ;
#19927=CARTESIAN_POINT ( 'NONE',  ( 18.13052570176356326, -12.27024696741798770, 31.24895572276497546 ) ) ;
#19928=CARTESIAN_POINT ( 'NONE',  ( -1.384615384615383471, -3.322132147404559976, 32.92929555188717927 ) ) ;
#19929=CARTESIAN_POINT ( 'NONE',  ( 16.94677586748485965, -2.619462340734461048, 30.83744416345203021 ) ) ;
#19930=ORIENTED_EDGE ( 'NONE', *, *, #50291, .F. ) ;
#19932=ORIENTED_EDGE ( 'NONE', *, *, #49703, .F. ) ;
#19933=ORIENTED_EDGE ( 'NONE', *, *, #68223, .F. ) ;
#19934=CARTESIAN_POINT ( 'NONE',  ( -4.219116599806928214, -6.026961402152685388, 34.52809138561120506 ) ) ;
#19935=CARTESIAN_POINT ( 'NONE',  ( 16.21991348719623360, -10.67929555188718282, 33.92786785259544757 ) ) ;
#19936=VECTOR ( 'NONE', #47217, 1000.000000000000114 ) ;
#19937=CARTESIAN_POINT ( 'NONE',  ( 2.307692307692186251, -3.643525952248796163, 33.31231777344771672 ) ) ;
#19938=CARTESIAN_POINT ( 'NONE',  ( -11.53846153846153655, -13.87047571288749737, 32.06866353760679544 ) ) ;
#19939=CARTESIAN_POINT ( 'NONE',  ( 3.453548899747297618, -9.418065098278011860, 34.63729479722530158 ) ) ;
#19941=CARTESIAN_POINT ( 'NONE',  ( -1.384615384615383471, -6.343179335718451384, 34.87096338111211935 ) ) ;
#19942=CARTESIAN_POINT ( 'NONE',  ( -4.853910232829680815, -11.43677907613344757, 33.22367315496201456 ) ) ;
#19943=ORIENTED_EDGE ( 'NONE', *, *, #79510, .T. ) ;
#19945=EDGE_LOOP ( 'NONE', ( #78042, #61335 ) ) ;
#19946=CARTESIAN_POINT ( 'NONE',  ( -11.78843826940389583, -12.41269422305637171, 30.68257228309993323 ) ) ;
#19947=EDGE_LOOP ( 'NONE', ( #76390, #10648 ) ) ;
#19948=DIRECTION ( 'NONE',  ( 0.000000000000000000, 0.8660254037844377084, -0.5000000000000015543 ) ) ;
#19949=CARTESIAN_POINT ( 'NONE',  ( -8.096130577096200653, -4.236021600441997492, 33.53823185664189310 ) ) ;
#19950=B_SPLINE_CURVE_WITH_KNOTS ( 'NONE', 3,
 ( #63729, #29956, #84908, #49771, #77246, #9675, #43023, #2031, #50654, #56971 ),
 .UNSPECIFIED., .F., .F.,
 ( 4, 2, 2, 2, 4 ),
 ( 0.0007817359430256315238, 0.0009771253907249976244, 0.001172514838424363508, 0.001367904286123729392, 0.001563293733823095492 ),
 .UNSPECIFIED. ) ;
#19951=EDGE_CURVE ( 'NONE', #78448, #29922, #51603, .T. ) ;
#19952=CARTESIAN_POINT ( 'NONE',  ( -0.3307480205715128685, -2.295524264805589354, 30.44142389570982488 ) ) ;
#19953=CARTESIAN_POINT ( 'NONE',  ( -10.68065506134538722, -3.835265460703609186, 33.15142922261924241 ) ) ;
#19954=FACE_BOUND ( 'NONE', #52568, .T. ) ;
#19955=ORIENTED_EDGE ( 'NONE', *, *, #32140, .F. ) ;
#19956=B_SPLINE_CURVE_WITH_KNOTS ( 'NONE', 3,
 ( #20782, #6398, #33853, #61311, #88826, #54561, #84280, #63087, #9055, #76168 ),
 .UNSPECIFIED., .F., .F.,
 ( 4, 2, 2, 2, 4 ),
 ( 0.000000000000000000, 0.0001954339857564077183, 0.0003908679715128154366, 0.0005863019572692231007, 0.0007817359430256308733 ),
 .UNSPECIFIED. ) ;
#19957=DIRECTION ( 'NONE',  ( -1.000000000000000000, 0.000000000000000000, 0.000000000000000000 ) ) ;
#19959=ORIENTED_EDGE ( 'NONE', *, *, #53627, .F. ) ;
#19960=CARTESIAN_POINT ( 'NONE',  ( 5.076923076922953193, -2.379036618888197729, 30.90682066428292885 ) ) ;
#19961=ORIENTED_EDGE ( 'NONE', *, *, #56981, .T. ) ;
#19962=FACE_BOUND ( 'NONE', #69023, .T. ) ;
#19963=CARTESIAN_POINT ( 'NONE',  ( -10.74607521849492464, -2.845849958028613624, 32.17971566917920967 ) ) ;
#19964=DIRECTION ( 'NONE',  ( 1.000000000000000000, 0.000000000000000000, 0.000000000000000000 ) ) ;
#19965=EDGE_LOOP ( 'NONE', ( #25098, #79934, #11644, #17074 ) ) ;
#19966=CARTESIAN_POINT ( 'NONE',  ( -12.21148414990014786, -8.303483539816728154, 34.68545999027711702 ) ) ;
#19967=CARTESIAN_POINT ( 'NONE',  ( -1.384615384615383471, -2.249999999999998668, 29.75000000000001776 ) ) ;
#19968=CYLINDRICAL_SURFACE ( 'NONE', #86782, 0.2499999999999973355 ) ;
#19969=EDGE_LOOP ( 'NONE', ( #8592, #57595 ) ) ;
#19970=CARTESIAN_POINT ( 'NONE',  ( 6.673053685783957967, -5.851115903089112003, 34.47074536777953568 ) ) ;
#19971=CARTESIAN_POINT ( 'NONE',  ( 14.08420738312797837, -11.60425143139329940, 33.02411095842164457 ) ) ;
#19972=CARTESIAN_POINT ( 'NONE',  ( 6.857806477116147548, -12.46129190929999986, 30.37095296980880832 ) ) ;
#19973=CARTESIAN_POINT ( 'NONE',  ( -17.75005459062195712, -12.68172785388650681, 30.59649109432439573 ) ) ;
#19974=VERTEX_POINT ( 'NONE', #82318 ) ;
#19976=AXIS2_PLACEMENT_3D ( 'NONE', #54377, #19273, #75111 ) ;
#19977=CARTESIAN_POINT ( 'NONE',  ( 9.692307692307695177, -2.708943851104267164, 35.45975837776705220 ) ) ;
#19978=CARTESIAN_POINT ( 'NONE',  ( 4.153846153846030731, -10.33852847137269571, 34.16647553114546554 ) ) ;
#19980=EDGE_LOOP ( 'NONE', ( #57853, #54740, #87183, #22319 ) ) ;
#19981=CARTESIAN_POINT ( 'NONE',  ( -8.519285250882630223, -10.76462480002816235, 33.53768742498949962 ) ) ;
#19982=CARTESIAN_POINT ( 'NONE',  ( -8.519230769230768274, -7.500000000000001776, 35.04278698407183867 ) ) ;
#19983=CARTESIAN_POINT ( 'NONE',  ( -13.13456107297706588, -4.943051570960394159, 34.04725096376909477 ) ) ;
#19984=CARTESIAN_POINT ( 'NONE',  ( -11.53846153846153655, -8.120952969808772792, 34.71129190930000163 ) ) ;
#19985=DIRECTION ( 'NONE',  ( 0.000000000000000000, 0.000000000000000000, 1.000000000000000000 ) ) ;
#19987=CARTESIAN_POINT ( 'NONE',  ( 9.822833394071260216, -9.417988943895561960, 34.36773134775777550 ) ) ;
#19989=CARTESIAN_POINT ( 'NONE',  ( -16.21992853320628925, -8.164416787775445883, 34.95778746994557906 ) ) ;
#19991=CYLINDRICAL_SURFACE ( 'NONE', #7557, 0.2500000000000009437 ) ;
#19994=CARTESIAN_POINT ( 'NONE',  ( -16.15384615384627409, -5.094484230521993062, 34.41647553114689373 ) ) ;
#19997=EDGE_CURVE ( 'NONE', #48855, #23593, #6513, .T. ) ;
#19998=ORIENTED_EDGE ( 'NONE', *, *, #57726, .T. ) ;
#19999=CARTESIAN_POINT ( 'NONE',  ( -11.47239420511146513, -2.292212530054420494, 30.41441678777542990 ) ) ;
#20001=DIRECTION ( 'NONE',  ( -0.000000000000000000, -0.000000000000000000, -1.000000000000000000 ) ) ;
#20004=ADVANCED_FACE ( 'NONE', ( #773 ), #16832, .F. ) ;
#20005=CARTESIAN_POINT ( 'NONE',  ( -11.40767109749459074, -9.929761469519743144, 34.40412654351204225 ) ) ;
#20006=CARTESIAN_POINT ( 'NONE',  ( -2.176900499867519212, -6.413143153341454017, 34.63066358083362672 ) ) ;
#20007=B_SPLINE_CURVE_WITH_KNOTS ( 'NONE', 3,
 ( #13689, #21329, #33958, #41167, #54662, #33530, #82160, #68633, #20452, #48798 ),
 .UNSPECIFIED., .F., .F.,
 ( 4, 2, 2, 2, 4 ),
 ( 0.000000000000000000, 0.0001954339857564079623, 0.0003908679715128159245, 0.0005863019572692238597, 0.0007817359430256318490 ),
 .UNSPECIFIED. ) ;
#20008=CARTESIAN_POINT ( 'NONE',  ( 1.253924781505080688, -2.494641256782728966, 31.33461815524612959 ) ) ;
#20009=CARTESIAN_POINT ( 'NONE',  ( 9.822833130541336999, -12.50538340440932394, 31.33453814440721885 ) ) ;
#20010=DIRECTION ( 'NONE',  ( -0.000000000000000000, 1.000000000000000000, 3.491481338843133355E-15 ) ) ;
#20011=CARTESIAN_POINT ( 'NONE',  ( -0.4615384615384611200, -12.48256725967547354, 35.29906147534542527 ) ) ;
#20012=CARTESIAN_POINT ( 'NONE',  ( 10.83816428436267820, -12.47679350104403007, 31.42216943046555855 ) ) ;
#20013=CARTESIAN_POINT ( 'NONE',  ( -13.38461538461550582, -6.879047030192662504, 34.71129190930017927 ) ) ;
#20014=EDGE_CURVE ( 'NONE', #67514, #64117, #47328, .T. ) ;
#20015=DIRECTION ( 'NONE',  ( -0.000000000000000000, 0.9396926207859093161, -0.3420201433256663259 ) ) ;
#20016=EDGE_CURVE ( 'NONE', #21487, #37386, #4417, .T. ) ;
#20017=ORIENTED_EDGE ( 'NONE', *, *, #52186, .T. ) ;
#20018=ORIENTED_EDGE ( 'NONE', *, *, #85698, .F. ) ;
#20019=FACE_OUTER_BOUND ( 'NONE', #7970, .T. ) ;
#20020=CARTESIAN_POINT ( 'NONE',  ( 5.299702618191484582, -9.332535724633407526, 34.40230450496446224 ) ) ;
#20021=DIRECTION ( 'NONE',  ( 1.000000000000000000, 0.000000000000000000, 0.000000000000000000 ) ) ;
#20022=LINE ( 'NONE', #47489, #67174 ) ;
#20023=EDGE_CURVE ( 'NONE', #41920, #31746, #83653, .T. ) ;
#20024=CARTESIAN_POINT ( 'NONE',  ( 6.249945518348142492, -5.057305518903949526, 34.11320923018887896 ) ) ;
#20025=CARTESIAN_POINT ( 'NONE',  ( -13.63463860883684475, -10.92453946501458795, 33.72985991061850086 ) ) ;
#20026=CARTESIAN_POINT ( 'NONE',  ( -1.384615384615505151, -8.613356846316285953, 34.62446782046622218 ) ) ;
#20027=EDGE_CURVE ( 'NONE', #20780, #13277, #71769, .T. ) ;
#20028=EDGE_LOOP ( 'NONE', ( #83556, #71691 ) ) ;
#20029=DIRECTION ( 'NONE',  ( -0.000000000000000000, -0.3420201433256694346, -0.9396926207859080948 ) ) ;
#20030=ORIENTED_EDGE ( 'NONE', *, *, #30527, .T. ) ;
#20031=ORIENTED_EDGE ( 'NONE', *, *, #28322, .F. ) ;
#20032=CARTESIAN_POINT ( 'NONE',  ( -14.05769230769224087, -7.434744429011176159, 34.75000000000000711 ) ) ;
#20033=AXIS2_PLACEMENT_3D ( 'NONE', #14889, #35146, #84240 ) ;
#20034=B_SPLINE_CURVE_WITH_KNOTS ( 'NONE', 3,
 ( #47669, #75576, #67507, #13439, #32828, #39604, #46786, #13878, #60291, #34599 ),
 .UNSPECIFIED., .F., .F.,
 ( 4, 2, 2, 2, 4 ),
 ( 0.000000000000000000, 0.0001954339857564074473, 0.0003908679715128148945, 0.0005863019572692223418, 0.0007817359430256297891 ),
 .UNSPECIFIED. ) ;
#20038=CARTESIAN_POINT ( 'NONE',  ( -4.403822884788508141, -4.236021600441998380, 33.53823185664189310 ) ) ;
#20039=EDGE_CURVE ( 'NONE', #42366, #37921, #16234, .T. ) ;
#20040=B_SPLINE_CURVE_WITH_KNOTS ( 'NONE', 3,
 ( #80831, #74062, #25422, #79483, #12356, #79922, #52437, #72711, #39833, #52881 ),
 .UNSPECIFIED., .F., .F.,
 ( 4, 2, 2, 2, 4 ),
 ( 0.0007817359430256334753, 0.0009771253907250058643, 0.001172514838424371098, 0.001367904286123736764, 0.001563293733823101998 ),
 .UNSPECIFIED. ) ;
#20041=CYLINDRICAL_SURFACE ( 'NONE', #13432, 0.2500000000000012212 ) ;
#20042=B_SPLINE_CURVE_WITH_KNOTS ( 'NONE', 3,
 ( #83022, #48781, #21755, #15453, #14557, #82140, #69499, #35269, #76705, #20431 ),
 .UNSPECIFIED., .F., .F.,
 ( 4, 2, 2, 2, 4 ),
 ( 0.0007817246336856289524, 0.0009771112958940099402, 0.001172497958102391036, 0.001367884620310772133, 0.001563271282519153229 ),
 .UNSPECIFIED. ) ;
#20044=AXIS2_PLACEMENT_3D ( 'NONE', #66354, #60484, #32131 ) ;
#20045=EDGE_LOOP ( 'NONE', ( #20614, #39280 ) ) ;
#20046=CIRCLE ( 'NONE', #64647, 0.2500000000000002220 ) ;
#20047=EDGE_LOOP ( 'NONE', ( #80798, #24731, #21576, #71517 ) ) ;
#20048=EDGE_LOOP ( 'NONE', ( #63504, #33597 ) ) ;
#20049=ORIENTED_EDGE ( 'NONE', *, *, #10430, .F. ) ;
#20050=CARTESIAN_POINT ( 'NONE',  ( -6.222926958906846551, -4.762599654559228846, 34.23009711892697737 ) ) ;
#20051=LINE ( 'NONE', #75004, #89178 ) ;
#20052=CARTESIAN_POINT ( 'NONE',  ( -3.230769230769229949, -9.780366693483667717, 34.19971097300155094 ) ) ;
#20053=CARTESIAN_POINT ( 'NONE',  ( -16.21911615440247090, -2.379036618887870880, 30.90682066428148644 ) ) ;
#20054=CARTESIAN_POINT ( 'NONE',  ( 18.00000000000000000, -4.786620604624113540, 33.94971097300155094 ) ) ;
#20056=ORIENTED_EDGE ( 'NONE', *, *, #80127, .F. ) ;
#20057=VERTEX_POINT ( 'NONE', #69236 ) ;
#20058=VERTEX_POINT ( 'NONE', #7538 ) ;
#20059=DIRECTION ( 'NONE',  ( -0.000000000000000000, -0.9396926207859092051, -0.3420201433256662704 ) ) ;
#20060=ORIENTED_EDGE ( 'NONE', *, *, #80695, .T. ) ;
#20061=CARTESIAN_POINT ( 'NONE',  ( 10.55011416942384095, -12.46129190929999986, 30.37095296980880832 ) ) ;
#20063=ADVANCED_FACE ( 'NONE', ( #85746 ), #21035, .F. ) ;
#20065=VERTEX_POINT ( 'NONE', #85304 ) ;
#20066=B_SPLINE_CURVE_WITH_KNOTS ( 'NONE', 3,
 ( #61021, #88524, #20917, #62341, #26798, #54255, #81750, #652, #47502, #28121 ),
 .UNSPECIFIED., .F., .F.,
 ( 4, 2, 2, 2, 4 ),
 ( 0.0007817359430256308733, 0.0009771253907249974075, 0.001172514838424363725, 0.001367904286123730259, 0.001563293733823096577 ),
 .UNSPECIFIED. ) ;
#20067=CARTESIAN_POINT ( 'NONE',  ( 7.846153846153846700, -3.937682226553329556, 33.60647404775216529 ) ) ;
#20068=EDGE_CURVE ( 'NONE', #83912, #41035, #66643, .T. ) ;
#20069=VECTOR ( 'NONE', #87932, 1000.000000000000227 ) ;
#20070=EDGE_LOOP ( 'NONE', ( #80384, #58763, #78879, #36969 ) ) ;
#20071=B_SPLINE_CURVE_WITH_KNOTS ( 'NONE', 3,
 ( #36166, #41579, #8247, #595, #83014, #69933, #21299, #1482, #77582, #76241 ),
 .UNSPECIFIED., .F., .F.,
 ( 4, 2, 2, 2, 4 ),
 ( 0.000000000000000000, 0.0001954339857564054415, 0.0003908679715128108830, 0.0005863019572692163787, 0.0007817359430256217660 ),
 .UNSPECIFIED. ) ;
#20074=FACE_BOUND ( 'NONE', #67686, .T. ) ;
#20075=CARTESIAN_POINT ( 'NONE',  ( -4.854143535654666053, -12.24180327182771855, 31.33663988360758168 ) ) ;
#20076=EDGE_CURVE ( 'NONE', #75373, #62016, #4660, .T. ) ;
#20077=DIRECTION ( 'NONE',  ( -0.000000000000000000, -0.9396926207859092051, -0.3420201433256662704 ) ) ;
#20078=ORIENTED_EDGE ( 'NONE', *, *, #42106, .T. ) ;
#20079=CARTESIAN_POINT ( 'NONE',  ( 4.826923076923076650, -2.249999999999998668, 29.75000000000000355 ) ) ;
#20080=CARTESIAN_POINT ( 'NONE',  ( -13.25456777835970179, -7.723484964179501588, 34.74522123443823318 ) ) ;
#20081=CARTESIAN_POINT ( 'NONE',  ( 0.4615384615383396616, -12.46129190930018460, 30.37095296980731973 ) ) ;
#20082=EDGE_LOOP ( 'NONE', ( #61014, #84984 ) ) ;
#20083=EDGE_CURVE ( 'NONE', #75897, #31900, #15118, .T. ) ;
#20084=CARTESIAN_POINT ( 'NONE',  ( -3.230769230769229949, -13.87047571288749737, 32.06866353760679544 ) ) ;
#20085=CARTESIAN_POINT ( 'NONE',  ( 1.607394925883795622, -8.496831190052093419, 34.64984203495476578 ) ) ;
#20086=LINE ( 'NONE', #54751, #36943 ) ;
#20087=CARTESIAN_POINT ( 'NONE',  ( -10.61538461538461320, -13.49023893513002648, 31.06009739812518688 ) ) ;
#20088=CARTESIAN_POINT ( 'NONE',  ( 8.992010438208833278, -10.23759521482555357, 34.22997729860117033 ) ) ;
#20089=FACE_BOUND ( 'NONE', #11104, .T. ) ;
#20090=CARTESIAN_POINT ( 'NONE',  ( 5.933917620639865831, -4.661471528628507777, 34.16647553114621871 ) ) ;
#20091=DIRECTION ( 'NONE',  ( -0.000000000000000000, -0.5000000000000009992, -0.8660254037844380415 ) ) ;
#20092=LINE ( 'NONE', #52975, #66949 ) ;
#20093=CARTESIAN_POINT ( 'NONE',  ( -18.13069060311030967, -2.295517848115768977, 30.44137282052137650 ) ) ;
#20094=CARTESIAN_POINT ( 'NONE',  ( 17.74997676270703550, -11.37209801155882793, 32.91403422569033665 ) ) ;
#20095=CARTESIAN_POINT ( 'NONE',  ( -3.230769230769229949, -13.49023893513002648, 31.06009739812518688 ) ) ;
#20097=VERTEX_POINT ( 'NONE', #40225 ) ;
#20098=CARTESIAN_POINT ( 'NONE',  ( -8.769230769230890843, -6.026961402154118019, 34.52809138561165270 ) ) ;
#20099=VERTEX_POINT ( 'NONE', #45185 ) ;
#20100=B_SPLINE_CURVE_WITH_KNOTS ( 'NONE', 3,
 ( #85331, #78557, #16862, #85777, #49324, #42572, #8342, #63272, #56522, #49757 ),
 .UNSPECIFIED., .F., .F.,
 ( 4, 2, 2, 2, 4 ),
 ( 0.000000000000000000, 0.0001954311564186868473, 0.0003908623128373736946, 0.0005862934692560605419, 0.0007817246256747473893 ),
 .UNSPECIFIED. ) ;
#20101=AXIS2_PLACEMENT_3D ( 'NONE', #39492, #79582, #66952 ) ;
#20102=CIRCLE ( 'NONE', #73272, 0.2500000000000002220 ) ;
#20103=FACE_OUTER_BOUND ( 'NONE', #86447, .T. ) ;
#20104=ORIENTED_EDGE ( 'NONE', *, *, #76024, .F. ) ;
#20105=CARTESIAN_POINT ( 'NONE',  ( -4.153846153846152411, -12.10708131394839349, 31.69288490824020244 ) ) ;
#20106=CARTESIAN_POINT ( 'NONE',  ( 14.17700170458200404, -3.957541250942358424, 33.62499894934981626 ) ) ;
#20107=LINE ( 'NONE', #75061, #52454 ) ;
#20108=ORIENTED_EDGE ( 'NONE', *, *, #461, .F. ) ;
#20109=CARTESIAN_POINT ( 'NONE',  ( -13.38461538461538325, -1.466349020453238561, 30.81389545987213907 ) ) ;
#20112=VECTOR ( 'NONE', #67405, 1000.000000000000114 ) ;
#20113=DIRECTION ( 'NONE',  ( 0.000000000000000000, 0.4999999999999960032, -0.8660254037844410391 ) ) ;
#20114=CARTESIAN_POINT ( 'NONE',  ( 9.692307692307695177, -2.517432740324522911, 35.29906147534542527 ) ) ;
#20116=EDGE_CURVE ( 'NONE', #11864, #84142, #52485, .T. ) ;
#20117=DIRECTION ( 'NONE',  ( -0.000000000000000000, 1.000000000000000000, 3.491481338843133355E-15 ) ) ;
#20118=LINE ( 'NONE', #81384, #30081 ) ;
#20119=CARTESIAN_POINT ( 'NONE',  ( -0.2115929431903197377, -4.336752205174647656, 33.62275283266504289 ) ) ;
#20120=CARTESIAN_POINT ( 'NONE',  ( 11.66925334628632527, -3.530189275343204702, 32.79018710029569661 ) ) ;
#20121=VECTOR ( 'NONE', #9603, 1000.000000000000227 ) ;
#20123=CARTESIAN_POINT ( 'NONE',  ( 14.24160889673642849, -5.557115091759785130, 34.35708131394839171 ) ) ;
#20125=CARTESIAN_POINT ( 'NONE',  ( 17.14217864819910275, -2.892918686051626498, 31.69288490824026638 ) ) ;
#20127=CARTESIAN_POINT ( 'NONE',  ( -14.98076923076922107, -2.249999999999999112, 29.81603969181033165 ) ) ;
#20128=CARTESIAN_POINT ( 'NONE',  ( 5.207448515156721136, -6.808710257144159783, 34.95449254468098843 ) ) ;
#20130=LINE ( 'NONE', #6614, #5410 ) ;
#20131=CARTESIAN_POINT ( 'NONE',  ( -0.4615384615384611200, -9.780366693483667717, 34.19971097300155094 ) ) ;
#20133=EDGE_LOOP ( 'NONE', ( #40340, #86363 ) ) ;
#20134=CARTESIAN_POINT ( 'NONE',  ( -2.084265908777518828, -7.630147987733843173, 34.99859428049665411 ) ) ;
#20135=CARTESIAN_POINT ( 'NONE',  ( 2.084766090176161324, -12.39988816332205701, 30.74660775122750778 ) ) ;
#20136=FACE_OUTER_BOUND ( 'NONE', #68489, .T. ) ;
#20137=CARTESIAN_POINT ( 'NONE',  ( -4.153846153846152411, -2.538708090699994813, 30.37095296980875503 ) ) ;
#20139=EDGE_CURVE ( 'NONE', #45673, #85149, #57054, .T. ) ;
#20140=EDGE_CURVE ( 'NONE', #38794, #67806, #62321, .T. ) ;
#20141=CARTESIAN_POINT ( 'NONE',  ( 8.769230769230768274, -1.509761064869970415, 31.06009739812519044 ) ) ;
#20142=ORIENTED_EDGE ( 'NONE', *, *, #41184, .F. ) ;
#20144=ORIENTED_EDGE ( 'NONE', *, *, #15521, .F. ) ;
#20145=EDGE_CURVE ( 'NONE', #88347, #30358, #61162, .T. ) ;
#20146=ORIENTED_EDGE ( 'NONE', *, *, #85558, .T. ) ;
#20147=DIRECTION ( 'NONE',  ( -0.000000000000000000, 1.000000000000000000, -0.000000000000000000 ) ) ;
#20148=CARTESIAN_POINT ( 'NONE',  ( 0.2115617305961061678, -2.564618984488975961, 30.55390908950641915 ) ) ;
#20149=EDGE_CURVE ( 'NONE', #24566, #48795, #55937, .T. ) ;
#20150=CARTESIAN_POINT ( 'NONE',  ( 9.822833394071260216, -5.195472089885680766, 34.18748526763464923 ) ) ;
#20151=CARTESIAN_POINT ( 'NONE',  ( -8.096177070375302876, -10.92453946501458795, 33.72985991061850086 ) ) ;
#20152=EDGE_CURVE ( 'NONE', #62404, #275, #38724, .T. ) ;
#20154=ORIENTED_EDGE ( 'NONE', *, *, #61409, .F. ) ;
#20155=VERTEX_POINT ( 'NONE', #47402 ) ;
#20156=VECTOR ( 'NONE', #70135, 1000.000000000000000 ) ;
#20157=VERTEX_POINT ( 'NONE', #48738 ) ;
#20158=DIRECTION ( 'NONE',  ( -0.000000000000000000, -0.1736481776669307198, -0.9848077530122080203 ) ) ;
#20159=EDGE_LOOP ( 'NONE', ( #70286, #75062 ) ) ;
#20160=CARTESIAN_POINT ( 'NONE',  ( 10.61538461538461675, -13.49023893513002648, 31.06009739812518688 ) ) ;
#20162=CARTESIAN_POINT ( 'NONE',  ( -10.83826329781326159, -7.630691491037285168, 34.74850469731152458 ) ) ;
#20163=AXIS2_PLACEMENT_3D ( 'NONE', #9152, #79256, #18002 ) ;
#20164=AXIS2_PLACEMENT_3D ( 'NONE', #82564, #55509, #21276 ) ;
#20165=EDGE_CURVE ( 'NONE', #24900, #60879, #78420, .T. ) ;
#20166=CARTESIAN_POINT ( 'NONE',  ( -12.21148414990014963, -12.17597550085003633, 31.52189283813461884 ) ) ;
#20167=CARTESIAN_POINT ( 'NONE',  ( -9.692307692307691624, -13.53365097954675988, 30.81389545987213552 ) ) ;
#20168=B_SPLINE_CURVE_WITH_KNOTS ( 'NONE', 3,
 ( #21277, #77118, #42451, #15426, #83447, #23058, #7775, #62699, #7337, #22608 ),
 .UNSPECIFIED., .F., .F.,
 ( 4, 2, 2, 2, 4 ),
 ( 0.000000000000000000, 0.0001954339857564074473, 0.0003908679715128148945, 0.0005863019572692223418, 0.0007817359430256297891 ),
 .UNSPECIFIED. ) ;
#20169=VERTEX_POINT ( 'NONE', #54600 ) ;
#20170=B_SPLINE_CURVE_WITH_KNOTS ( 'NONE', 3,
 ( #45759, #10646, #86774, #46649, #85862, #59716, #59269, #66923, #39020, #11089 ),
 .UNSPECIFIED., .F., .F.,
 ( 4, 2, 2, 2, 4 ),
 ( 0.0007817246256747472808, 0.0009771112852218905021, 0.001172497944769033832, 0.001367884604316177161, 0.001563271263863320274 ),
 .UNSPECIFIED. ) ;
#20171=ORIENTED_EDGE ( 'NONE', *, *, #17163, .T. ) ;
#20172=AXIS2_PLACEMENT_3D ( 'NONE', #63363, #16070, #85418 ) ;
#20173=ORIENTED_EDGE ( 'NONE', *, *, #40958, .F. ) ;
#20175=CARTESIAN_POINT ( 'NONE',  ( 10.61538461538461675, -1.466349020453238561, 30.81389545987213907 ) ) ;
#20176=ORIENTED_EDGE ( 'NONE', *, *, #9278, .F. ) ;
#20177=CARTESIAN_POINT ( 'NONE',  ( 6.699591979352975457, -6.760086850603068243, 34.69517049084099369 ) ) ;
#20178=B_SPLINE_CURVE_WITH_KNOTS ( 'NONE', 3,
 ( #51317, #18468, #31072, #50886, #72507, #39190, #65744, #38733, #58993, #45922 ),
 .UNSPECIFIED., .F., .F.,
 ( 4, 2, 2, 2, 4 ),
 ( 0.000000000000000000, 0.0001954311564186871184, 0.0003908623128373742367, 0.0005862934692560614093, 0.0007817246256747484735 ),
 .UNSPECIFIED. ) ;
#20179=EDGE_CURVE ( 'NONE', #5216, #88472, #80701, .T. ) ;
#20180=CARTESIAN_POINT ( 'NONE',  ( -14.30769230769230660, -2.538708090699994813, 30.37095296980875503 ) ) ;
#20181=ORIENTED_EDGE ( 'NONE', *, *, #73173, .T. ) ;
#20182=CARTESIAN_POINT ( 'NONE',  ( 16.28463796167094202, -3.530189275343204702, 32.79018710029569661 ) ) ;
#20183=CARTESIAN_POINT ( 'NONE',  ( 0.3954560821783251190, -9.058645607665454236, 34.76329471203372634 ) ) ;
#20184=FACE_BOUND ( 'NONE', #6026, .T. ) ;
#20185=EDGE_CURVE ( 'NONE', #43220, #6788, #13626, .T. ) ;
#20186=DIRECTION ( 'NONE',  ( -0.000000000000000000, -0.6427876096865404731, -0.7660444431189770143 ) ) ;
#20187=CARTESIAN_POINT ( 'NONE',  ( -5.999999999999998224, -12.34228464037088635, 31.77849191805839268 ) ) ;
#20188=CARTESIAN_POINT ( 'NONE',  ( -5.999999999999690914, -2.506253911140614576, 30.00000000000323297 ) ) ;
#20191=CARTESIAN_POINT ( 'NONE',  ( -4.376674251481031064, -7.369209533119140509, 34.99857337881830688 ) ) ;
#20192=CYLINDRICAL_SURFACE ( 'NONE', #67800, 0.2499999999999994726 ) ;
#20193=EDGE_LOOP ( 'NONE', ( #52938, #6035 ) ) ;
#20194=CARTESIAN_POINT ( 'NONE',  ( -7.912236225513979981, -6.343179335718451384, 34.87096338111212646 ) ) ;
#20195=CARTESIAN_POINT ( 'NONE',  ( 0.3962684609821406356, -11.06231777344662781, 33.60647404775220082 ) ) ;
#20197=EDGE_CURVE ( 'NONE', #44046, #75329, #13991, .T. ) ;
#20198=CARTESIAN_POINT ( 'NONE',  ( -14.53061852520844965, -4.887634598454295265, 34.01352882383564946 ) ) ;
#20200=ORIENTED_EDGE ( 'NONE', *, *, #74581, .T. ) ;
#20201=CARTESIAN_POINT ( 'NONE',  ( 11.47237915910140771, -9.905515769479276145, 34.41647553114623292 ) ) ;
#20202=LINE ( 'NONE', #67061, #19936 ) ;
#20203=FACE_BOUND ( 'NONE', #6383, .T. ) ;
#20204=EDGE_CURVE ( 'NONE', #51377, #62161, #31213, .T. ) ;
#20205=CARTESIAN_POINT ( 'NONE',  ( -14.53061926659915315, -4.026226216239094491, 33.68668979543634379 ) ) ;
#20206=CYLINDRICAL_SURFACE ( 'NONE', #17196, 0.2499999999999979738 ) ;
#20208=DIRECTION ( 'NONE',  ( -0.000000000000000000, -0.6427876096865404731, -0.7660444431189771253 ) ) ;
#20209=CARTESIAN_POINT ( 'NONE',  ( -10.61538461538473577, -11.67786785259630911, 32.92929555188603530 ) ) ;
#20210=B_SPLINE_CURVE_WITH_KNOTS ( 'NONE', 3,
 ( #26830, #60601, #53853, #88117, #47085, #20509, #46653, #74575, #39468, #20067 ),
 .UNSPECIFIED., .F., .F.,
 ( 4, 2, 2, 2, 4 ),
 ( 0.0007817246256747465219, 0.0009771112852218900684, 0.001172497944769033615, 0.001367884604316176944, 0.001563271263863320491 ),
 .UNSPECIFIED. ) ;
#20211=VECTOR ( 'NONE', #13035, 999.9999999999998863 ) ;
#20213=ORIENTED_EDGE ( 'NONE', *, *, #79416, .T. ) ;
#20214=VERTEX_POINT ( 'NONE', #62247 ) ;
#20215=CARTESIAN_POINT ( 'NONE',  ( -12.23875879256039312, -5.827830569534417471, 34.72679350104403539 ) ) ;
#20216=CARTESIAN_POINT ( 'NONE',  ( -18.00000000000012079, -3.643525952248793498, 33.31231777344770961 ) ) ;
#20218=LINE ( 'NONE', #89137, #45254 ) ;
#20219=CYLINDRICAL_SURFACE ( 'NONE', #87444, 0.2500000000000008882 ) ;
#20221=EDGE_CURVE ( 'NONE', #17526, #18050, #77491, .T. ) ;
#20222=DIRECTION ( 'NONE',  ( -0.000000000000000000, -0.8660254037844397068, -0.4999999999999978906 ) ) ;
#20223=CARTESIAN_POINT ( 'NONE',  ( 5.749976775778544713, -2.985938066672154445, 32.43141759479405550 ) ) ;
#20224=ADVANCED_FACE ( 'NONE', ( #28475 ), #68569, .F. ) ;
#20227=CARTESIAN_POINT ( 'NONE',  ( 3.230769230769231726, -1.215029322943914858, 32.30358669280327177 ) ) ;
#20228=CARTESIAN_POINT ( 'NONE',  ( 8.638539302563209787, -12.11776431015576172, 31.66791131148498906 ) ) ;
#20229=FACE_OUTER_BOUND ( 'NONE', #31456, .T. ) ;
#20230=CARTESIAN_POINT ( 'NONE',  ( -6.700064078983527516, -3.395485233115139057, 33.02377354290275946 ) ) ;
#20232=CARTESIAN_POINT ( 'NONE',  ( 10.61538461538461675, -1.117168528481311540, 33.14645433367849847 ) ) ;
#20235=FACE_OUTER_BOUND ( 'NONE', #34647, .T. ) ;
#20237=VECTOR ( 'NONE', #33686, 1000.000000000000114 ) ;
#20239=CARTESIAN_POINT ( 'NONE',  ( 5.076923076923075762, -9.905515769479276145, 34.41647553114623292 ) ) ;
#20240=CARTESIAN_POINT ( 'NONE',  ( -17.74994568836168440, -10.66356715214248752, 33.62249196103329751 ) ) ;
#20241=DIRECTION ( 'NONE',  ( -0.000000000000000000, -0.5000000000000009992, -0.8660254037844380415 ) ) ;
#20242=CARTESIAN_POINT ( 'NONE',  ( -39.05038313613820122, -2.499999999999999556, 29.75000000000000355 ) ) ;
#20243=ORIENTED_EDGE ( 'NONE', *, *, #36663, .F. ) ;
#20245=CARTESIAN_POINT ( 'NONE',  ( -14.55766905174089665, -5.643011162660950042, 34.66104346484419096 ) ) ;
#20246=ORIENTED_EDGE ( 'NONE', *, *, #60883, .T. ) ;
#20247=CARTESIAN_POINT ( 'NONE',  ( 11.78851595837499211, -9.233818618650603938, 34.70587769442853698 ) ) ;
#20248=CARTESIAN_POINT ( 'NONE',  ( -17.77698864838715664, -3.587049720035813127, 32.86302985866382897 ) ) ;
#20249=EDGE_LOOP ( 'NONE', ( #8879, #85572, #59035, #32547 ) ) ;
#20250=CARTESIAN_POINT ( 'NONE',  ( 14.30769230769231015, -2.538708090699994813, 30.37095296980875503 ) ) ;
#20251=CARTESIAN_POINT ( 'NONE',  ( 8.639082799499073317, -6.809168938359901446, 34.95455904226513866 ) ) ;
#20252=B_SPLINE_CURVE_WITH_KNOTS ( 'NONE', 3,
 ( #81937, #54002, #19781, #75176, #11700, #31965, #39177, #52665, #66637, #80154 ),
 .UNSPECIFIED., .F., .F.,
 ( 4, 2, 2, 2, 4 ),
 ( 0.000000000000000000, 0.0001954311564186881213, 0.0003908623128373762425, 0.0005862934692560643367, 0.0007817246256747524850 ),
 .UNSPECIFIED. ) ;
#20253=LINE ( 'NONE', #61663, #75829 ) ;
#20255=B_SPLINE_CURVE_WITH_KNOTS ( 'NONE', 3,
 ( #47540, #27276, #13320, #47983, #13758, #7004, #68703, #34477, #61939, #251 ),
 .UNSPECIFIED., .F., .F.,
 ( 4, 2, 2, 2, 4 ),
 ( 0.000000000000000000, 0.0001954311564186861697, 0.0003908623128373723394, 0.0005862934692560584820, 0.0007817246256747446788 ),
 .UNSPECIFIED. ) ;
#20256=VERTEX_POINT ( 'NONE', #19937 ) ;
#20257=CARTESIAN_POINT ( 'NONE',  ( 15.45354889974729495, -4.989023458446560255, 34.36081565061822118 ) ) ;
#20258=VERTEX_POINT ( 'NONE', #34336 ) ;
#20259=CARTESIAN_POINT ( 'NONE',  ( -8.069080805060693251, -2.308479472611653094, 30.53278059502174457 ) ) ;
#20260=CARTESIAN_POINT ( 'NONE',  ( -13.38461538461538325, -2.538708090699994813, 30.37095296980875503 ) ) ;
#20261=CARTESIAN_POINT ( 'NONE',  ( -10.86540785267757592, -2.587272538249755893, 30.68239716806877837 ) ) ;
#20262=ADVANCED_FACE ( 'NONE', ( #61802 ), #27585, .F. ) ;
#20263=CARTESIAN_POINT ( 'NONE',  ( -4.153846153846152411, -1.215029322943914858, 32.30358669280327177 ) ) ;
#20264=CARTESIAN_POINT ( 'NONE',  ( 17.07692307692307665, -12.29105614889573062, 35.45975837776705220 ) ) ;
#20265=CARTESIAN_POINT ( 'NONE',  ( -2.557692307692305267, -2.249999999999998668, 29.75000000000000355 ) ) ;
#20266=EDGE_CURVE ( 'NONE', #30501, #60387, #43028, .T. ) ;
#20267=CARTESIAN_POINT ( 'NONE',  ( 10.36536137809165403, -12.22074536777954989, 31.39888409691088356 ) ) ;
#20268=VERTEX_POINT ( 'NONE', #30248 ) ;
#20269=ORIENTED_EDGE ( 'NONE', *, *, #36522, .T. ) ;
#20270=CARTESIAN_POINT ( 'NONE',  ( -17.14219352288385778, -10.21337939537584383, 33.94971097300158647 ) ) ;
#20271=ORIENTED_EDGE ( 'NONE', *, *, #37201, .F. ) ;
#20274=B_SPLINE_CURVE_WITH_KNOTS ( 'NONE', 3,
 ( #19303, #5346, #5788, #12989, #72904, #73812, #11209, #80575, #19745, #38679 ),
 .UNSPECIFIED., .F., .F.,
 ( 4, 2, 2, 2, 4 ),
 ( 0.000000000000000000, 0.0001954311564186867660, 0.0003908623128373735320, 0.0005862934692560603251, 0.0007817246256747470640 ),
 .UNSPECIFIED. ) ;
#20275=CARTESIAN_POINT ( 'NONE',  ( -8.769230769230768274, -10.67929555188718282, 33.92786785259544047 ) ) ;
#20276=CARTESIAN_POINT ( 'NONE',  ( 9.626224281351815293, -4.786620604624113540, 33.94971097300155805 ) ) ;
#20277=VERTEX_POINT ( 'NONE', #70349 ) ;
#20278=CARTESIAN_POINT ( 'NONE',  ( 14.53047197667037516, -12.11081565061823717, 32.26097654155341843 ) ) ;
#20279=B_SPLINE_CURVE_WITH_KNOTS ( 'NONE', 3,
 ( #82781, #78216, #58377, #51611, #79108, #38122, #17861, #31824, #59278, #16518 ),
 .UNSPECIFIED., .F., .F.,
 ( 4, 2, 2, 2, 4 ),
 ( 0.0007817359527651101701, 0.0009771254036996489256, 0.001172514854634187790, 0.001367904305568726653, 0.001563293756503265517 ),
 .UNSPECIFIED. ) ;
#20280=EDGE_CURVE ( 'NONE', #70987, #62668, #88203, .T. ) ;
#20281=ORIENTED_EDGE ( 'NONE', *, *, #20291, .T. ) ;
#20282=CARTESIAN_POINT ( 'NONE',  ( -15.23076923076922995, -2.249999999999998668, 29.75000000000001776 ) ) ;
#20283=B_SPLINE_CURVE_WITH_KNOTS ( 'NONE', 3,
 ( #73931, #5021, #33819, #39261, #46446, #26623, #81135, #74369, #25736, #13112 ),
 .UNSPECIFIED., .F., .F.,
 ( 4, 2, 2, 2, 4 ),
 ( 0.000000000000000000, 0.0001954311564186877960, 0.0003908623128373755920, 0.0005862934692560633609, 0.0007817246256747511840 ),
 .UNSPECIFIED. ) ;
#20284=ORIENTED_EDGE ( 'NONE', *, *, #71311, .F. ) ;
#20288=CARTESIAN_POINT ( 'NONE',  ( -8.899922235898330314, -4.809359713505814149, 33.96456829005828837 ) ) ;
#20289=DIRECTION ( 'NONE',  ( -0.000000000000000000, -0.9396926207859092051, -0.3420201433256662704 ) ) ;
#20290=FACE_BOUND ( 'NONE', #60932, .T. ) ;
#20291=EDGE_CURVE ( 'NONE', #45665, #50666, #44622, .T. ) ;
#20292=CARTESIAN_POINT ( 'NONE',  ( 14.30769230769231015, -13.95598074871891292, 31.83374038241031911 ) ) ;
#20293=CYLINDRICAL_SURFACE ( 'NONE', #11198, 0.2499999999999979738 ) ;
#20294=VECTOR ( 'NONE', #35932, 1000.000000000000000 ) ;
#20295=CARTESIAN_POINT ( 'NONE',  ( -15.93083330975275658, -4.762714258010882773, 34.23016756924214832 ) ) ;
#20297=CYLINDRICAL_SURFACE ( 'NONE', #84132, 0.2499999999999995559 ) ;
#20298=CARTESIAN_POINT ( 'NONE',  ( -1.384615384615383471, -1.129524287112498415, 32.06866353760679544 ) ) ;
#20299=EDGE_CURVE ( 'NONE', #4054, #64954, #116, .T. ) ;
#20300=CARTESIAN_POINT ( 'NONE',  ( 9.692307692307695177, -2.292212530054420494, 30.41441678777542634 ) ) ;
#20301=EDGE_LOOP ( 'NONE', ( #22603, #48660, #43357, #10833 ) ) ;
#20302=ORIENTED_EDGE ( 'NONE', *, *, #39056, .T. ) ;
#20303=VECTOR ( 'NONE', #72589, 1000.000000000000114 ) ;
#20304=CARTESIAN_POINT ( 'NONE',  ( -16.82697755857493149, -10.05730279482229683, 34.04704008940765902 ) ) ;
#20305=CARTESIAN_POINT ( 'NONE',  ( -18.06527000055631405, -10.33852847137145403, 34.16647553114627556 ) ) ;
#20306=DIRECTION ( 'NONE',  ( 0.000000000000000000, -6.938893903907222067E-15, 1.000000000000000000 ) ) ;
#20307=CARTESIAN_POINT ( 'NONE',  ( 3.230769230769231726, -10.51840700105979565, 33.73612834413961536 ) ) ;
#20308=CARTESIAN_POINT ( 'NONE',  ( 8.638621114026685532, -7.722926974430166069, 34.99546784045485737 ) ) ;
#20310=EDGE_LOOP ( 'NONE', ( #52579, #62113 ) ) ;
#20311=CARTESIAN_POINT ( 'NONE',  ( 17.20744877868664346, -3.285477652293413264, 32.44071101563363158 ) ) ;
#20312=EDGE_CURVE ( 'NONE', #72884, #35268, #60249, .T. ) ;
#20313=CARTESIAN_POINT ( 'NONE',  ( 0.5920641633020228278, -10.19071101563364401, 33.96452234770658407 ) ) ;
#20314=CARTESIAN_POINT ( 'NONE',  ( -3.296039231325550656, -11.67786785259541027, 32.92929555188721480 ) ) ;
#20315=CARTESIAN_POINT ( 'NONE',  ( -6.923076923076922462, -6.343179335718451384, 34.87096338111211935 ) ) ;
#20316=ORIENTED_EDGE ( 'NONE', *, *, #8416, .F. ) ;
#20317=EDGE_LOOP ( 'NONE', ( #40654, #14951, #63924, #26609 ) ) ;
#20318=ORIENTED_EDGE ( 'NONE', *, *, #4330, .T. ) ;
#20319=CARTESIAN_POINT ( 'NONE',  ( 0.5923302693632472860, -10.54018710029568595, 33.71981072465678864 ) ) ;
#20320=EDGE_LOOP ( 'NONE', ( #82382, #10096 ) ) ;
#20321=CARTESIAN_POINT ( 'NONE',  ( 2.980792486720640788, -12.65889640711025521, 30.72598325615533454 ) ) ;
#20323=CARTESIAN_POINT ( 'NONE',  ( 4.946231610255518163, -6.413092428213692742, 34.63065189839063152 ) ) ;
#20324=CARTESIAN_POINT ( 'NONE',  ( -2.307692307692305711, -8.120952969808772792, 34.71129190930000163 ) ) ;
#20325=ADVANCED_FACE ( 'NONE', ( #85197 ), #85636, .F. ) ;
#20326=FACE_OUTER_BOUND ( 'NONE', #76611, .T. ) ;
#20327=VERTEX_POINT ( 'NONE', #8209 ) ;
#20328=LINE ( 'NONE', #61736, #42951 ) ;
#20330=ORIENTED_EDGE ( 'NONE', *, *, #72873, .T. ) ;
#20332=CARTESIAN_POINT ( 'NONE',  ( 9.019176178608812933, -12.45601412856602686, 31.48342859153981621 ) ) ;
#20333=B_SPLINE_CURVE_WITH_KNOTS ( 'NONE', 3,
 ( #7686, #6785, #62609, #68058, #6364, #33818, #88790, #27065, #20314, #47777 ),
 .UNSPECIFIED., .F., .F.,
 ( 4, 2, 2, 2, 4 ),
 ( 0.000000000000000000, 0.0001954311564186869557, 0.0003908623128373739115, 0.0005862934692560608672, 0.0007817246256747478229 ),
 .UNSPECIFIED. ) ;
#20334=DIRECTION ( 'NONE',  ( -0.000000000000000000, -0.3420201433256694901, -0.9396926207859082059 ) ) ;
#20335=VECTOR ( 'NONE', #36103, 1000.000000000000000 ) ;
#20337=EDGE_CURVE ( 'NONE', #76336, #57743, #18296, .T. ) ;
#20338=CARTESIAN_POINT ( 'NONE',  ( 11.76147438255493149, -10.01129605718032600, 34.36064277460058491 ) ) ;
#20339=CARTESIAN_POINT ( 'NONE',  ( 9.692307692307695177, -13.88283147151868846, 33.14645433367849847 ) ) ;
#20340=CARTESIAN_POINT ( 'NONE',  ( 17.01159906411876932, -7.749976730030849303, 34.74374725381503737 ) ) ;
#20342=AXIS2_PLACEMENT_3D ( 'NONE', #5601, #46586, #26756 ) ;
#20345=EDGE_LOOP ( 'NONE', ( #13303, #62890 ) ) ;
#20346=EDGE_CURVE ( 'NONE', #67440, #32572, #34414, .T. ) ;
#20347=CARTESIAN_POINT ( 'NONE',  ( 13.38461538461538680, -5.471508081941601098, 34.59228464037088457 ) ) ;
#20348=CARTESIAN_POINT ( 'NONE',  ( 1.134638640566795420, -9.234221910056348293, 34.70572697212741531 ) ) ;
#20349=CARTESIAN_POINT ( 'NONE',  ( 9.942362112221147186, -10.82426656108012075, 33.81400080652039009 ) ) ;
#20351=ORIENTED_EDGE ( 'NONE', *, *, #60462, .F. ) ;
#20352=CARTESIAN_POINT ( 'NONE',  ( -5.749945688361683516, -2.564540009722896752, 30.55348353981670684 ) ) ;
#20353=CARTESIAN_POINT ( 'NONE',  ( -16.15384615384615330, -1.790695186598648903, 34.54067556320373455 ) ) ;
#20354=CARTESIAN_POINT ( 'NONE',  ( 2.372947447205147942, -11.06231777344671130, 33.60647404775212976 ) ) ;
#20355=B_SPLINE_CURVE_WITH_KNOTS ( 'NONE', 3,
 ( #18157, #39328, #73100, #79859, #53261, #46067, #18606, #19044, #46514, #10955 ),
 .UNSPECIFIED., .F., .F.,
 ( 4, 2, 2, 2, 4 ),
 ( 0.0007817246256747474977, 0.0009771112852218911526, 0.001172497944769034699, 0.001367884604316178462, 0.001563271263863322009 ),
 .UNSPECIFIED. ) ;
#20357=CARTESIAN_POINT ( 'NONE',  ( 0.5276057948885373161, -2.292212530054420494, 30.41441678777542990 ) ) ;
#20360=CARTESIAN_POINT ( 'NONE',  ( 12.21153846153846168, -2.249999999999998668, 29.75000000000000355 ) ) ;
#20361=VECTOR ( 'NONE', #29514, 1000.000000000000227 ) ;
#20362=DIRECTION ( 'NONE',  ( -0.000000000000000000, -0.5000000000000009992, -0.8660254037844380415 ) ) ;
#20363=CARTESIAN_POINT ( 'NONE',  ( 5.142990410273153401, -12.34228464037088813, 31.77849191805839268 ) ) ;
#20364=VERTEX_POINT ( 'NONE', #39234 ) ;
#20365=CARTESIAN_POINT ( 'NONE',  ( -16.94639763868943660, -12.15418822224088657, 32.17964115625579069 ) ) ;
#20366=ORIENTED_EDGE ( 'NONE', *, *, #78889, .F. ) ;
#20367=CARTESIAN_POINT ( 'NONE',  ( -2.557669038634660552, -12.17611988154120972, 31.52148481390971213 ) ) ;
#20369=CARTESIAN_POINT ( 'NONE',  ( -5.934744860487160878, -12.16647553114626490, 32.15551576947920864 ) ) ;
#20370=ORIENTED_EDGE ( 'NONE', *, *, #12899, .T. ) ;
#20371=CARTESIAN_POINT ( 'NONE',  ( 18.00000000000000000, -12.78798330534102767, 29.49999999999997868 ) ) ;
#20372=CARTESIAN_POINT ( 'NONE',  ( 4.219101293358989757, -9.528491918058460186, 34.59228464037085615 ) ) ;
#20373=CARTESIAN_POINT ( 'NONE',  ( 13.25392391794782654, -6.413092428213692742, 34.63065189839063152 ) ) ;
#20375=CARTESIAN_POINT ( 'NONE',  ( 3.230769230769110045, -12.46129190930018460, 30.37095296980731973 ) ) ;
#20376=ORIENTED_EDGE ( 'NONE', *, *, #60235, .F. ) ;
#20377=FACE_BOUND ( 'NONE', #49312, .T. ) ;
#20378=EDGE_LOOP ( 'NONE', ( #22388, #14403, #5255, #87717 ) ) ;
#20379=CARTESIAN_POINT ( 'NONE',  ( -8.835313148590904220, -12.34228464037088280, 31.77849191805838558 ) ) ;
#20380=DIRECTION ( 'NONE',  ( 0.000000000000000000, 0.7660444431189822323, -0.6427876096865344779 ) ) ;
#20381=DIRECTION ( 'NONE',  ( -0.000000000000000000, 0.9848077530122085754, -0.1736481776669273613 ) ) ;
#20382=CARTESIAN_POINT ( 'NONE',  ( -6.066083410955878108, -12.10708131394839349, 31.69288490824020244 ) ) ;
#20383=EDGE_LOOP ( 'NONE', ( #2762, #7414 ) ) ;
#20384=ORIENTED_EDGE ( 'NONE', *, *, #83805, .F. ) ;
#20385=ORIENTED_EDGE ( 'NONE', *, *, #76620, .F. ) ;
#20387=CARTESIAN_POINT ( 'NONE',  ( -0.3962828902624365157, -3.300289026998475705, 32.46337939537591666 ) ) ;
#20388=ORIENTED_EDGE ( 'NONE', *, *, #35123, .T. ) ;
#20389=CARTESIAN_POINT ( 'NONE',  ( -17.32689982097166492, -10.06842814019191401, 34.32929386961144758 ) ) ;
#20390=VECTOR ( 'NONE', #82063, 1000.000000000000000 ) ;
#20391=CARTESIAN_POINT ( 'NONE',  ( 1.607626736228235931, -3.587049720035815348, 32.86302985866382897 ) ) ;
#20392=CYLINDRICAL_SURFACE ( 'NONE', #87640, 0.2500000000000002220 ) ;
#20394=EDGE_CURVE ( 'NONE', #47301, #82157, #3295, .T. ) ;
#20396=CARTESIAN_POINT ( 'NONE',  ( -4.376712416909251502, -2.251424796025575770, 29.88072029997477586 ) ) ;
#20397=CARTESIAN_POINT ( 'NONE',  ( 18.00000000000000000, -2.538708090699994813, 30.37095296980875503 ) ) ;
#20398=FACE_OUTER_BOUND ( 'NONE', #57869, .T. ) ;
#20402=FACE_OUTER_BOUND ( 'NONE', #87185, .T. ) ;
#20403=CARTESIAN_POINT ( 'NONE',  ( -3.007756386675836779, -10.01129605718032778, 34.36064277460058491 ) ) ;
#20404=CARTESIAN_POINT ( 'NONE',  ( -5.869474298236433185, -3.816742781228458448, 33.13167719472716044 ) ) ;
#20405=DIRECTION ( 'NONE',  ( -0.000000000000000000, -0.9848077530122085754, -0.1736481776669273613 ) ) ;
#20406=CARTESIAN_POINT ( 'NONE',  ( 3.230769230769108269, -10.33852847137269571, 34.16647553114546554 ) ) ;
#20407=FACE_BOUND ( 'NONE', #16273, .T. ) ;
#20408=CARTESIAN_POINT ( 'NONE',  ( 16.40379167219429490, -3.202959910592336090, 32.30730279482227019 ) ) ;
#20409=ORIENTED_EDGE ( 'NONE', *, *, #54134, .F. ) ;
#20410=EDGE_CURVE ( 'NONE', #71524, #47112, #72057, .T. ) ;
#20411=CARTESIAN_POINT ( 'NONE',  ( 15.23076923076923173, -12.78798330534102945, 29.74999999999997868 ) ) ;
#20412=CARTESIAN_POINT ( 'NONE',  ( 16.94677586748485965, -6.852621066184266141, 34.70813303252209181 ) ) ;
#20414=EDGE_LOOP ( 'NONE', ( #65148, #50364, #89112, #85109 ) ) ;
#20415=CARTESIAN_POINT ( 'NONE',  ( 4.853996118016226546, -2.308479472611653094, 30.53278059502174457 ) ) ;
#20416=EDGE_LOOP ( 'NONE', ( #28107, #1845, #75651, #86899 ) ) ;
#20417=FACE_BOUND ( 'NONE', #31726, .T. ) ;
#20418=CARTESIAN_POINT ( 'NONE',  ( -18.00000000000000000, -1.652287802724643262, 34.33046132563154629 ) ) ;
#20419=VECTOR ( 'NONE', #35319, 1000.000000000000000 ) ;
#20420=DIRECTION ( 'NONE',  ( -0.000000000000000000, -0.3420201433256694346, -0.9396926207859080948 ) ) ;
#20421=DIRECTION ( 'NONE',  ( 0.000000000000000000, 0.8660254037844377084, -0.5000000000000015543 ) ) ;
#20422=VERTEX_POINT ( 'NONE', #86084 ) ;
#20423=CARTESIAN_POINT ( 'NONE',  ( 4.153846153846154188, -1.951392089020283160, 34.73218667398347748 ) ) ;
#20424=DIRECTION ( 'NONE',  ( -0.000000000000000000, -0.8660254037844397068, -0.4999999999999978906 ) ) ;
#20425=CARTESIAN_POINT ( 'NONE',  ( 16.15384615384615330, -1.509761064869970415, 31.06009739812519044 ) ) ;
#20426=CARTESIAN_POINT ( 'NONE',  ( -8.069638789877792817, -2.847400154188067578, 31.58180166144859058 ) ) ;
#20427=ORIENTED_EDGE ( 'NONE', *, *, #31459, .F. ) ;
#20428=AXIS2_PLACEMENT_3D ( 'NONE', #10035, #22667, #31192 ) ;
#20429=DIRECTION ( 'NONE',  ( -0.000000000000000000, 0.5000000000000011102, -0.8660254037844380415 ) ) ;
#20430=CARTESIAN_POINT ( 'NONE',  ( -15.45369544828537656, -4.186968288167451036, 33.49512374952580274 ) ) ;
#20431=CARTESIAN_POINT ( 'NONE',  ( 15.90384615384615330, -7.500000000000001776, 35.00000000000000000 ) ) ;
#20432=ORIENTED_EDGE ( 'NONE', *, *, #49208, .F. ) ;
#20433=DIRECTION ( 'NONE',  ( -0.000000000000000000, -0.7660444431189791237, -0.6427876096865379196 ) ) ;
#20435=CARTESIAN_POINT ( 'NONE',  ( 15.48076923076923173, -7.500000000000001776, 35.04278698407183867 ) ) ;
#20438=EDGE_CURVE ( 'NONE', #36014, #42886, #50503, .T. ) ;
#20439=ADVANCED_FACE ( 'NONE', ( #25265 ), #52725, .F. ) ;
#20440=CARTESIAN_POINT ( 'NONE',  ( 9.915087233576098669, -9.332535724633409302, 34.40230450496446934 ) ) ;
#20443=CARTESIAN_POINT ( 'NONE',  ( 14.24160889673642494, -3.513871655860377086, 32.76840700105978499 ) ) ;
#20445=VERTEX_POINT ( 'NONE', #45971 ) ;
#20446=CARTESIAN_POINT ( 'NONE',  ( -10.61538461538461320, -13.20930481340135110, 34.54067556320372745 ) ) ;
#20447=ORIENTED_EDGE ( 'NONE', *, *, #29128, .T. ) ;
#20448=EDGE_CURVE ( 'NONE', #19635, #8641, #80525, .T. ) ;
#20449=VERTEX_POINT ( 'NONE', #5445 ) ;
#20451=VERTEX_POINT ( 'NONE', #88326 ) ;
#20452=CARTESIAN_POINT ( 'NONE',  ( 14.24242186173153435, -8.613356846314824011, 34.62446782046655613 ) ) ;
#20455=CARTESIAN_POINT ( 'NONE',  ( 12.21153846153846345, -7.433932668274256805, 35.00000000000000711 ) ) ;
#20456=CARTESIAN_POINT ( 'NONE',  ( 3.230769230769231726, -1.129524287112498415, 32.06866353760679544 ) ) ;
#20457=CARTESIAN_POINT ( 'NONE',  ( -2.084912766423896446, -6.760870238392817200, 34.69528174975672385 ) ) ;
#20458=CARTESIAN_POINT ( 'NONE',  ( 17.07692307692307665, -8.120952969808772792, 34.71129190930000163 ) ) ;
#20459=CARTESIAN_POINT ( 'NONE',  ( -17.07692307692307665, -13.78497067705608181, 32.30358669280327177 ) ) ;
#20462=LINE ( 'NONE', #55564, #59491 ) ;
#20463=CARTESIAN_POINT ( 'NONE',  ( -0.5268089074992378107, -2.625532179533444754, 30.86335684631481513 ) ) ;
#20464=CARTESIAN_POINT ( 'NONE',  ( 17.74997676270703550, -11.86270091957321071, 32.19358267280088626 ) ) ;
#20465=VECTOR ( 'NONE', #12607, 1000.000000000000114 ) ;
#20466=PLANE ( 'NONE',  #27774 ) ;
#20467=VERTEX_POINT ( 'NONE', #34687 ) ;
#20469=CARTESIAN_POINT ( 'NONE',  ( -18.22292695890684655, -2.523278758544489353, 31.42238647778637528 ) ) ;
#20470=CARTESIAN_POINT ( 'NONE',  ( 12.46153846153846168, -3.886160181151819604, 36.00935417666054406 ) ) ;
#20471=DIRECTION ( 'NONE',  ( -0.000000000000000000, 0.6427876096865404731, -0.7660444431189770143 ) ) ;
#20472=CARTESIAN_POINT ( 'NONE',  ( 5.750023269057647823, -5.728515186090277211, 34.42611988154120439 ) ) ;
#20473=CARTESIAN_POINT ( 'NONE',  ( -14.30769230769242739, -12.46129190930018460, 30.37095296980731973 ) ) ;
#20474=CARTESIAN_POINT ( 'NONE',  ( 11.66898697669518548, -4.299079248970732792, 33.91157788607253565 ) ) ;
#20475=CARTESIAN_POINT ( 'NONE',  ( 8.769230769230647482, -10.21337939537710326, 33.94971097300076224 ) ) ;
#20477=CARTESIAN_POINT ( 'NONE',  ( 18.13079044096695469, -3.338503747796866872, 32.95102852606552801 ) ) ;
#20478=ORIENTED_EDGE ( 'NONE', *, *, #7950, .F. ) ;
#20479=AXIS2_PLACEMENT_3D ( 'NONE', #29959, #86705, #57417 ) ;
#20480=CARTESIAN_POINT ( 'NONE',  ( -8.519176349317314489, -4.818054556918156983, 34.26375889529406749 ) ) ;
#20481=CARTESIAN_POINT ( 'NONE',  ( 15.48071464014727283, -3.520799739797214389, 33.17531984108286025 ) ) ;
#20482=CARTESIAN_POINT ( 'NONE',  ( -20.74999999999999289, -7.500000000000000000, 29.75000000000000355 ) ) ;
#20483=CARTESIAN_POINT ( 'NONE',  ( -15.23076923076922995, -3.050289026998446396, 32.03036669348365706 ) ) ;
#20484=FACE_OUTER_BOUND ( 'NONE', #11032, .T. ) ;
#20485=EDGE_CURVE ( 'NONE', #26693, #23594, #68907, .T. ) ;
#20487=ORIENTED_EDGE ( 'NONE', *, *, #44870, .T. ) ;
#20488=VERTEX_POINT ( 'NONE', #20722 ) ;
#20489=ORIENTED_EDGE ( 'NONE', *, *, #82946, .F. ) ;
#20491=CARTESIAN_POINT ( 'NONE',  ( 5.999999999999878320, -2.379036618888197729, 30.90682066428292885 ) ) ;
#20493=CARTESIAN_POINT ( 'NONE',  ( 2.242421861731534349, -11.48612834413959582, 32.76840700105983473 ) ) ;
#20494=EDGE_CURVE ( 'NONE', #62209, #80426, #71878, .T. ) ;
#20495=CARTESIAN_POINT ( 'NONE',  ( 17.77707304109313924, -2.889293201056495786, 32.26117774369186009 ) ) ;
#20496=CARTESIAN_POINT ( 'NONE',  ( 12.39626846098214052, -3.083524468853724443, 32.58852847137143272 ) ) ;
#20498=EDGE_CURVE ( 'NONE', #28583, #66822, #10630, .T. ) ;
#20500=ORIENTED_EDGE ( 'NONE', *, *, #78873, .T. ) ;
#20501=CARTESIAN_POINT ( 'NONE',  ( -10.48485891362104816, -11.93748526763465279, 32.05452791011430946 ) ) ;
#20502=EDGE_LOOP ( 'NONE', ( #7289, #22695, #82197, #44290 ) ) ;
#20503=CARTESIAN_POINT ( 'NONE',  ( 12.46153846153846168, -13.53365097954675988, 30.81389545987213552 ) ) ;
#20504=DIRECTION ( 'NONE',  ( 0.000000000000000000, 0.8660254037844377084, 0.5000000000000015543 ) ) ;
#20505=AXIS2_PLACEMENT_3D ( 'NONE', #3370, #66744, #43475 ) ;
#20507=ORIENTED_EDGE ( 'NONE', *, *, #59355, .T. ) ;
#20508=EDGE_CURVE ( 'NONE', #37921, #42366, #24677, .T. ) ;
#20509=CARTESIAN_POINT ( 'NONE',  ( 8.096208266067295156, -4.074993327901524687, 33.72946981652012255 ) ) ;
#20510=EDGE_LOOP ( 'NONE', ( #73505, #71159, #70792, #63789 ) ) ;
#20511=CARTESIAN_POINT ( 'NONE',  ( 8.068933387422253745, -12.24180327182772210, 31.33663988360758168 ) ) ;
#20512=FACE_BOUND ( 'NONE', #40690, .T. ) ;
#20513=CYLINDRICAL_SURFACE ( 'NONE', #11540, 0.2499999999999995559 ) ;
#20514=EDGE_CURVE ( 'NONE', #62121, #75871, #64375, .T. ) ;
#20515=CARTESIAN_POINT ( 'NONE',  ( -14.05769230769230482, -2.499999999999999556, 29.81604066197449754 ) ) ;
#20516=EDGE_LOOP ( 'NONE', ( #36213, #55092 ) ) ;
#20518=CARTESIAN_POINT ( 'NONE',  ( 8.769230769230768274, -8.164416787775445883, 34.95778746994557906 ) ) ;
#20519=CARTESIAN_POINT ( 'NONE',  ( -16.85414340794500276, -12.69155399931963046, 30.53255429739158444 ) ) ;
#20520=CARTESIAN_POINT ( 'NONE',  ( -3.296851610129365451, -9.058645607665454236, 34.76329471203372634 ) ) ;
#20521=EDGE_LOOP ( 'NONE', ( #2638, #51726, #34122, #11290 ) ) ;
#20522=CARTESIAN_POINT ( 'NONE',  ( 15.90384615384615685, -7.433931650972299465, 34.75000000000000711 ) ) ;
#20523=CARTESIAN_POINT ( 'NONE',  ( 1.134592160393929960, -4.175268141568689195, 33.81360843649122216 ) ) ;
#20524=CARTESIAN_POINT ( 'NONE',  ( -12.52762187249433978, -12.10708131394839349, 31.69288490824020244 ) ) ;
#20525=CARTESIAN_POINT ( 'NONE',  ( -2.307692307692305711, -10.51840700105979565, 33.73612834413961536 ) ) ;
#20528=FACE_BOUND ( 'NONE', #4796, .T. ) ;
#20529=CARTESIAN_POINT ( 'NONE',  ( -6.923076923077045919, -12.51329471203414379, 31.30864560766407578 ) ) ;
#20530=CARTESIAN_POINT ( 'NONE',  ( 11.47237812750565666, -12.37446782046654192, 30.86335684631486487 ) ) ;
#20531=CARTESIAN_POINT ( 'NONE',  ( 5.076923076923075762, -9.058645607665452459, 34.76329471203371924 ) ) ;
#20532=CARTESIAN_POINT ( 'NONE',  ( -5.869474298236438514, -10.19071101563364756, 33.96452234770658407 ) ) ;
#20533=CARTESIAN_POINT ( 'NONE',  ( -2.241624974342229404, -12.34228464037088813, 31.77849191805839268 ) ) ;
#20534=EDGE_CURVE ( 'NONE', #28242, #89067, #85940, .T. ) ;
#20535=CARTESIAN_POINT ( 'NONE',  ( -7.846153846153967493, -4.320704448113951379, 33.92786785259630022 ) ) ;
#20537=VERTEX_POINT ( 'NONE', #6761 ) ;
#20538=CARTESIAN_POINT ( 'NONE',  ( -6.000000000000121680, -11.06231777344772027, 33.60647404775119895 ) ) ;
#20539=EDGE_LOOP ( 'NONE', ( #57546, #2516, #70000, #41509, #46447, #15912 ) ) ;
#20540=CARTESIAN_POINT ( 'NONE',  ( 13.38461538461538680, -7.500000000000001776, 35.04278698407183867 ) ) ;
#20541=EDGE_CURVE ( 'NONE', #16932, #78524, #15303, .T. ) ;
#20542=B_SPLINE_CURVE_WITH_KNOTS ( 'NONE', 3,
 ( #88150, #38602, #66058, #4370, #18331, #4822, #32292, #59756, #20546, #75060 ),
 .UNSPECIFIED., .F., .F.,
 ( 4, 2, 2, 2, 4 ),
 ( 0.0007817359430256218744, 0.0009771253907249861318, 0.001172514838424350498, 0.001367904286123714864, 0.001563293733823079229 ),
 .UNSPECIFIED. ) ;
#20543=ORIENTED_EDGE ( 'NONE', *, *, #8601, .F. ) ;
#20544=ADVANCED_FACE ( 'NONE', ( #21605 ), #57164, .F. ) ;
#20545=FACE_OUTER_BOUND ( 'NONE', #49969, .T. ) ;
#20546=CARTESIAN_POINT ( 'NONE',  ( -1.318547033612946340, -10.51840700105979565, 33.73612834413962247 ) ) ;
#20547=CARTESIAN_POINT ( 'NONE',  ( -5.076923076923075762, -1.117168528481311540, 33.14645433367849847 ) ) ;
#20548=EDGE_LOOP ( 'NONE', ( #38439, #11297 ) ) ;
#20549=CARTESIAN_POINT ( 'NONE',  ( -14.30769230769230660, -13.88283147151868846, 33.14645433367849847 ) ) ;
#20551=CARTESIAN_POINT ( 'NONE',  ( -13.38461538461538325, -2.708943851104267164, 35.45975837776705220 ) ) ;
#20552=CARTESIAN_POINT ( 'NONE',  ( -4.153846153846152411, -11.35647404775217417, 33.31231777344666511 ) ) ;
#20553=DIRECTION ( 'NONE',  ( -0.000000000000000000, 0.6427876096865404731, -0.7660444431189770143 ) ) ;
#20554=CARTESIAN_POINT ( 'NONE',  ( 10.48523664565291469, -2.647304123082328875, 31.75400227202885972 ) ) ;
#20555=DIRECTION ( 'NONE',  ( -0.000000000000000000, -0.3420201433256694346, -0.9396926207859080948 ) ) ;
#20556=CARTESIAN_POINT ( 'NONE',  ( 6.000000000000001776, -2.486705287966279876, 31.30864560766543647 ) ) ;
#20558=CARTESIAN_POINT ( 'NONE',  ( 11.47319153790521717, -5.941354392334499579, 34.76329471203369792 ) ) ;
#20559=CARTESIAN_POINT ( 'NONE',  ( -4.219116154402471786, -3.083524468853724443, 32.58852847137143272 ) ) ;
#20560=VERTEX_POINT ( 'NONE', #36887 ) ;
#20561=CARTESIAN_POINT ( 'NONE',  ( 10.61538461538449418, -6.835583212225970762, 34.95778746994575670 ) ) ;
#20563=CARTESIAN_POINT ( 'NONE',  ( -17.77698864838715309, -12.39991518177334129, 30.74647679643404530 ) ) ;
#20564=CARTESIAN_POINT ( 'NONE',  ( -8.835313148590902443, -11.35647404775217595, 33.31231777344666511 ) ) ;
#20565=ORIENTED_EDGE ( 'NONE', *, *, #61059, .T. ) ;
#20567=CARTESIAN_POINT ( 'NONE',  ( -14.43838377435986864, -11.18331474514187995, 33.13161551792790505 ) ) ;
#20568=DIRECTION ( 'NONE',  ( -0.000000000000000000, 0.3420201433256694346, -0.9396926207859080948 ) ) ;
#20569=ORIENTED_EDGE ( 'NONE', *, *, #61678, .T. ) ;
#20570=DIRECTION ( 'NONE',  ( 0.000000000000000000, 0.3420201433256641055, -0.9396926207859100932 ) ) ;
#20571=CARTESIAN_POINT ( 'NONE',  ( -15.23076923076935252, -12.16647553114689728, 32.15551576947799362 ) ) ;
#20572=LINE ( 'NONE', #82291, #52923 ) ;
#20573=VECTOR ( 'NONE', #48681, 1000.000000000000227 ) ;
#20574=CARTESIAN_POINT ( 'NONE',  ( 2.057669083470853089, -4.175268141568689195, 33.81360843649122216 ) ) ;
#20575=EDGE_CURVE ( 'NONE', #11048, #42810, #64789, .T. ) ;
#20578=EDGE_LOOP ( 'NONE', ( #29286, #74540 ) ) ;
#20579=ORIENTED_EDGE ( 'NONE', *, *, #31751, .T. ) ;
#20580=CARTESIAN_POINT ( 'NONE',  ( 2.307692307692309264, -2.499999999999998668, 29.75000000000001421 ) ) ;
#20581=CARTESIAN_POINT ( 'NONE',  ( 0.2115152242454959586, -2.587272538249754117, 30.68239716806877837 ) ) ;
#20582=CARTESIAN_POINT ( 'NONE',  ( -13.16183584334697088, -12.24180327182772388, 31.33663988360758168 ) ) ;
#20583=FACE_OUTER_BOUND ( 'NONE', #79381, .T. ) ;
#20584=EDGE_CURVE ( 'NONE', #79867, #10043, #63019, .T. ) ;
#20586=DIRECTION ( 'NONE',  ( -0.000000000000000000, -0.9396926207859092051, -0.3420201433256662704 ) ) ;
#20588=ORIENTED_EDGE ( 'NONE', *, *, #16771, .F. ) ;
#20589=ORIENTED_EDGE ( 'NONE', *, *, #60157, .T. ) ;
#20590=CARTESIAN_POINT ( 'NONE',  ( 11.53846153846153832, -13.95598074871891292, 31.83374038241031911 ) ) ;
#20591=ORIENTED_EDGE ( 'NONE', *, *, #1005, .T. ) ;
#20592=CARTESIAN_POINT ( 'NONE',  ( 15.23076923076923173, -8.810774026931790459, 35.74407628777942847 ) ) ;
#20593=DIRECTION ( 'NONE',  ( -0.000000000000000000, -0.1736481776669307198, -0.9848077530122080203 ) ) ;
#20595=CIRCLE ( 'NONE', #83881, 0.2500000000000002220 ) ;
#20596=EDGE_CURVE ( 'NONE', #5035, #33753, #44074, .T. ) ;
#20597=CARTESIAN_POINT ( 'NONE',  ( -12.46153846153858247, -12.27809138561165270, 31.22303859784587132 ) ) ;
#20599=ORIENTED_EDGE ( 'NONE', *, *, #63770, .F. ) ;
#20600=EDGE_CURVE ( 'NONE', #43223, #26530, #45078, .T. ) ;
#20601=VECTOR ( 'NONE', #54135, 999.9999999999998863 ) ;
#20602=EDGE_LOOP ( 'NONE', ( #13292, #51155 ) ) ;
#20603=EDGE_LOOP ( 'NONE', ( #82306, #64041, #11862, #16493 ) ) ;
#20604=CARTESIAN_POINT ( 'NONE',  ( 10.83839596699746544, -10.61302985866384141, 33.66295027996417843 ) ) ;
#20605=DIRECTION ( 'NONE',  ( -0.000000000000000000, -0.1736481776669307198, -0.9848077530122080203 ) ) ;
#20606=ORIENTED_EDGE ( 'NONE', *, *, #84883, .F. ) ;
#20607=B_SPLINE_CURVE_WITH_KNOTS ( 'NONE', 3,
 ( #80886, #18279, #73226, #5206, #80436, #60139, #46637, #74115, #47067, #54713 ),
 .UNSPECIFIED., .F., .F.,
 ( 4, 2, 2, 2, 4 ),
 ( 0.0007817246256747473893, 0.0009771112852218900684, 0.001172497944769032747, 0.001367884604316175643, 0.001563271263863318323 ),
 .UNSPECIFIED. ) ;
#20608=CARTESIAN_POINT ( 'NONE',  ( 13.25405479287346466, -2.504760397472875155, 29.97295953869789997 ) ) ;
#20609=CARTESIAN_POINT ( 'NONE',  ( 15.23076923076923173, -12.62096338111211580, 30.90682066428153263 ) ) ;
#20610=EDGE_LOOP ( 'NONE', ( #39655, #80348 ) ) ;
#20611=EDGE_CURVE ( 'NONE', #57426, #82401, #52586, .T. ) ;
#20612=CARTESIAN_POINT ( 'NONE',  ( -4.088590582570128973, -5.219633306516380244, 34.19971097300157936 ) ) ;
#20613=CARTESIAN_POINT ( 'NONE',  ( -9.692307692307812417, -10.21337939537710326, 33.94971097300076224 ) ) ;
#20614=ORIENTED_EDGE ( 'NONE', *, *, #16275, .T. ) ;
#20615=FACE_BOUND ( 'NONE', #63773, .T. ) ;
#20616=CARTESIAN_POINT ( 'NONE',  ( -13.38461538461538325, -11.35647404775217417, 33.31231777344666511 ) ) ;
#20618=CARTESIAN_POINT ( 'NONE',  ( 12.46153846153846168, -6.343179335718451384, 34.87096338111211935 ) ) ;
#20619=LINE ( 'NONE', #46769, #64755 ) ;
#20620=CYLINDRICAL_SURFACE ( 'NONE', #88649, 0.2500000000000002220 ) ;
#20621=CARTESIAN_POINT ( 'NONE',  ( -3.100243792535585463, -3.625058011473228259, 33.29252011169590020 ) ) ;
#20622=CARTESIAN_POINT ( 'NONE',  ( 6.988270904860278243, -2.506253911140448487, 29.99999999999988631 ) ) ;
#20623=ORIENTED_EDGE ( 'NONE', *, *, #12885, .T. ) ;
#20624=CARTESIAN_POINT ( 'NONE',  ( -14.30769230769242739, -4.481592998941358097, 33.73612834414048933 ) ) ;
#20626=ORIENTED_EDGE ( 'NONE', *, *, #87460, .F. ) ;
#20628=CIRCLE ( 'NONE', #33570, 0.2500000000000002220 ) ;
#20629=CARTESIAN_POINT ( 'NONE',  ( 8.703147358274886614, -3.050289026998445951, 32.03036669348365706 ) ) ;
#20632=CARTESIAN_POINT ( 'NONE',  ( -9.758390071667825794, -9.058645607665454236, 34.76329471203372634 ) ) ;
#20633=CARTESIAN_POINT ( 'NONE',  ( -15.16470189741915675, -12.62096338111211757, 30.90682066428152908 ) ) ;
#20634=EDGE_CURVE ( 'NONE', #6564, #3308, #63263, .T. ) ;
#20635=FACE_BOUND ( 'NONE', #25918, .T. ) ;
#20636=DIRECTION ( 'NONE',  ( -0.000000000000000000, 1.000000000000000000, -0.000000000000000000 ) ) ;
#20637=CARTESIAN_POINT ( 'NONE',  ( -39.05038313613820122, -2.249999999999998668, 29.75000000000000355 ) ) ;
#20638=CARTESIAN_POINT ( 'NONE',  ( -13.38461538461550759, -2.379036618888197729, 30.90682066428292885 ) ) ;
#20639=DIRECTION ( 'NONE',  ( -0.000000000000000000, 0.9848077530122086864, -0.1736481776669273891 ) ) ;
#20641=CARTESIAN_POINT ( 'NONE',  ( -14.17764487244185290, -7.723484941389743952, 34.99544897038808955 ) ) ;
#20642=CARTESIAN_POINT ( 'NONE',  ( -39.05038313613820122, -2.249999999999998668, 29.75000000000000355 ) ) ;
#20644=VERTEX_POINT ( 'NONE', #36457 ) ;
#20645=ADVANCED_FACE ( 'NONE', ( #84653 ), #71554, .F. ) ;
#20646=B_SPLINE_CURVE_WITH_KNOTS ( 'NONE', 3,
 ( #20740, #35141, #83790, #62603, #48207, #62169, #27946, #41912, #76124, #22513 ),
 .UNSPECIFIED., .F., .F.,
 ( 4, 2, 2, 2, 4 ),
 ( 0.0007817359430256372700, 0.0009771253907250054306, 0.001172514838424373483, 0.001367904286123741535, 0.001563293733823109804 ),
 .UNSPECIFIED. ) ;
#20647=ORIENTED_EDGE ( 'NONE', *, *, #6975, .F. ) ;
#20648=DIRECTION ( 'NONE',  ( 0.000000000000000000, 0.1736481776669267785, -0.9848077530122087975 ) ) ;
#20649=EDGE_CURVE ( 'NONE', #29364, #61122, #6337, .T. ) ;
#20650=CARTESIAN_POINT ( 'NONE',  ( -17.07692307692319744, -5.094484230521993062, 34.41647553114689373 ) ) ;
#20651=CARTESIAN_POINT ( 'NONE',  ( 14.30769230769231015, -9.058645607665452459, 34.76329471203371924 ) ) ;
#20652=CARTESIAN_POINT ( 'NONE',  ( 17.30029856269549526, -2.251407671071269601, 29.88021292934942252 ) ) ;
#20653=CARTESIAN_POINT ( 'NONE',  ( -7.596153846153831601, -2.249999999999998224, 29.81603969181031033 ) ) ;
#20655=CARTESIAN_POINT ( 'NONE',  ( -16.15384615384615330, -1.466349020453238561, 30.81389545987213907 ) ) ;
#20656=CARTESIAN_POINT ( 'NONE',  ( 2.057692307692309708, -2.249999999999998668, 29.75000000000000355 ) ) ;
#20657=CARTESIAN_POINT ( 'NONE',  ( 15.23076923076923173, -11.69971097300155272, 32.46337939537588113 ) ) ;
#20659=CARTESIAN_POINT ( 'NONE',  ( -1.161188985700596366, -7.630147987733843173, 34.99859428049665411 ) ) ;
#20660=DIRECTION ( 'NONE',  ( -0.000000000000000000, 0.5000000000000011102, -0.8660254037844380415 ) ) ;
#20661=CARTESIAN_POINT ( 'NONE',  ( 7.173131342990377135, -3.435999193479609914, 33.07426656108010832 ) ) ;
#20662=VECTOR ( 'NONE', #78979, 1000.000000000000000 ) ;
#20663=CARTESIAN_POINT ( 'NONE',  ( -8.519176349317316266, -11.47946981652013498, 33.17500667209847620 ) ) ;
#20664=CARTESIAN_POINT ( 'NONE',  ( 3.164685819813349177, -2.538708090699994813, 30.37095296980875148 ) ) ;
#20665=EDGE_CURVE ( 'NONE', #26718, #10196, #48279, .T. ) ;
#20666=ORIENTED_EDGE ( 'NONE', *, *, #28746, .F. ) ;
#20667=CARTESIAN_POINT ( 'NONE',  ( 3.903869422903798458, -4.943428324936578910, 34.04746400365624481 ) ) ;
#20668=CARTESIAN_POINT ( 'NONE',  ( 17.07692307692307665, -4.661471528628507777, 34.16647553114623292 ) ) ;
#20671=AXIS2_PLACEMENT_3D ( 'NONE', #45412, #350, #5777 ) ;
#20672=CARTESIAN_POINT ( 'NONE',  ( -0.3310130233048192983, -11.04252011169590020, 33.62494198852677130 ) ) ;
#20673=SURFACE_SIDE_STYLE ('',( #88281 ) ) ;
#20674=EDGE_CURVE ( 'NONE', #80960, #10201, #67039, .T. ) ;
#20675=FACE_OUTER_BOUND ( 'NONE', #58693, .T. ) ;
#20676=CARTESIAN_POINT ( 'NONE',  ( -5.776573601085211784, -7.630147987733840509, 34.99859428049665411 ) ) ;
#20679=CARTESIAN_POINT ( 'NONE',  ( -9.692307692307814193, -5.941354392335915335, 34.76329471203413846 ) ) ;
#20680=B_SPLINE_CURVE_WITH_KNOTS ( 'NONE', 3,
 ( #70690, #57169, #9427, #58479, #51718, #8995, #30143, #85976, #78317, #84222 ),
 .UNSPECIFIED., .F., .F.,
 ( 4, 2, 2, 2, 4 ),
 ( 0.000000000000000000, 0.0001954339857564097512, 0.0003908679715128195024, 0.0005863019572692292807, 0.0007817359430256390048 ),
 .UNSPECIFIED. ) ;
#20681=ORIENTED_EDGE ( 'NONE', *, *, #42602, .T. ) ;
#20682=CARTESIAN_POINT ( 'NONE',  ( -15.93083480223330817, -9.886259254753566594, 34.14407573483972413 ) ) ;
#20684=ORIENTED_EDGE ( 'NONE', *, *, #53035, .F. ) ;
#20685=CARTESIAN_POINT ( 'NONE',  ( 14.08476609017615644, -2.554751324335735152, 30.48935550225260727 ) ) ;
#20686=ADVANCED_FACE ( 'NONE', ( #85971 ), #73346, .F. ) ;
#20687=CARTESIAN_POINT ( 'NONE',  ( 8.546303810323914618, -6.459968553980841577, 34.89616026154728701 ) ) ;
#20688=CARTESIAN_POINT ( 'NONE',  ( -15.00798968950081758, -12.44528174975671853, 30.48912976160716681 ) ) ;
#20689=EDGE_LOOP ( 'NONE', ( #9319, #56701 ) ) ;
#20690=EDGE_LOOP ( 'NONE', ( #74413, #78202 ) ) ;
#20691=DIRECTION ( 'NONE',  ( -0.000000000000000000, -0.5000000000000009992, -0.8660254037844380415 ) ) ;
#20692=EDGE_CURVE ( 'NONE', #17599, #2983, #39684, .T. ) ;
#20693=VERTEX_POINT ( 'NONE', #39128 ) ;
#20694=EDGE_CURVE ( 'NONE', #80088, #8812, #17062, .T. ) ;
#20695=CARTESIAN_POINT ( 'NONE',  ( -8.069638770718176701, -2.353723527008296568, 30.78948104536958752 ) ) ;
#20696=CARTESIAN_POINT ( 'NONE',  ( -6.923076923077045919, -2.379036618888197729, 30.90682066428292885 ) ) ;
#20697=CARTESIAN_POINT ( 'NONE',  ( -17.07692307692319744, -6.026961402154118908, 34.52809138561165270 ) ) ;
#20698=LINE ( 'NONE', #14384, #21730 ) ;
#20699=DIRECTION ( 'NONE',  ( -0.000000000000000000, 0.6427876096865404731, -0.7660444431189770143 ) ) ;
#20700=CARTESIAN_POINT ( 'NONE',  ( 13.63456090296352841, -3.202959910592335646, 32.30730279482227019 ) ) ;
#20701=EDGE_CURVE ( 'NONE', #82664, #34676, #86887, .T. ) ;
#20702=FACE_OUTER_BOUND ( 'NONE', #2774, .T. ) ;
#20703=ORIENTED_EDGE ( 'NONE', *, *, #37397, .T. ) ;
#20704=ADVANCED_FACE ( 'NONE', ( #10309 ), #18403, .F. ) ;
#20705=ORIENTED_EDGE ( 'NONE', *, *, #76368, .T. ) ;
#20706=CARTESIAN_POINT ( 'NONE',  ( -0.2115929431903189328, -12.22109172314383052, 31.39792113162168263 ) ) ;
#20707=ORIENTED_EDGE ( 'NONE', *, *, #63760, .T. ) ;
#20708=B_SPLINE_CURVE_WITH_KNOTS ( 'NONE', 3,
 ( #49917, #2173, #62978, #29662, #57123, #1292, #36847, #57561, #77834, #43603 ),
 .UNSPECIFIED., .F., .F.,
 ( 4, 2, 2, 2, 4 ),
 ( 0.000000000000000000, 0.0001954339857564064444, 0.0003908679715128128888, 0.0005863019572692193060, 0.0007817359430256257775 ),
 .UNSPECIFIED. ) ;
#20709=DIRECTION ( 'NONE',  ( -0.000000000000000000, -0.9396926207859093161, -0.3420201433256663259 ) ) ;
#20710=CARTESIAN_POINT ( 'NONE',  ( 10.55013468361053164, -2.255955759149247619, 30.00000000000013856 ) ) ;
#20711=CARTESIAN_POINT ( 'NONE',  ( 12.71159277317677549, -3.136992222400443175, 32.19305428654138979 ) ) ;
#20713=EDGE_CURVE ( 'NONE', #37130, #38219, #23550, .T. ) ;
#20715=ORIENTED_EDGE ( 'NONE', *, *, #39986, .F. ) ;
#20716=CARTESIAN_POINT ( 'NONE',  ( 7.976944287120795174, -12.62708834333097663, 30.88030960425257021 ) ) ;
#20717=EDGE_LOOP ( 'NONE', ( #36748, #81756, #16759, #73793 ) ) ;
#20718=CARTESIAN_POINT ( 'NONE',  ( -10.39242171182312724, -7.369474270740069777, 34.74850911626239736 ) ) ;
#20719=AXIS2_PLACEMENT_3D ( 'NONE', #60382, #54511, #12207 ) ;
#20720=EDGE_LOOP ( 'NONE', ( #88962, #55741, #6098, #4297 ) ) ;
#20721=LINE ( 'NONE', #5444, #71905 ) ;
#20722=CARTESIAN_POINT ( 'NONE',  ( 13.38461538461526423, -12.16647553114689728, 32.15551576947799362 ) ) ;
#20723=FACE_BOUND ( 'NONE', #25580, .T. ) ;
#20724=B_SPLINE_CURVE_WITH_KNOTS ( 'NONE', 3,
 ( #9903, #49569, #15346, #17103, #71157, #58519, #43256, #9464, #36927, #42821 ),
 .UNSPECIFIED., .F., .F.,
 ( 4, 2, 2, 2, 4 ),
 ( 0.000000000000000000, 0.0001954339881912772715, 0.0003908679763825545429, 0.0005863019645738318415, 0.0007817359527651090859 ),
 .UNSPECIFIED. ) ;
#20725=AXIS2_PLACEMENT_3D ( 'NONE', #15831, #64878, #16264 ) ;
#20726=DIRECTION ( 'NONE',  ( -0.000000000000000000, -0.6427876096865404731, -0.7660444431189770143 ) ) ;
#20727=CARTESIAN_POINT ( 'NONE',  ( -11.66860950819323328, -6.809168938359901446, 34.95455904226513866 ) ) ;
#20728=VECTOR ( 'NONE', #21501, 999.9999999999998863 ) ;
#20729=CARTESIAN_POINT ( 'NONE',  ( 4.219101725122176738, -12.46129190930001052, 30.37095296980870174 ) ) ;
#20731=CARTESIAN_POINT ( 'NONE',  ( -3.165513659493203846, -3.300289026998474817, 32.46337939537591666 ) ) ;
#20732=CARTESIAN_POINT ( 'NONE',  ( -4.284537620513710010, -11.18331474514187995, 33.13161551792790505 ) ) ;
#20733=CARTESIAN_POINT ( 'NONE',  ( -14.17690049986752143, -3.530189275343204702, 32.79018710029569661 ) ) ;
#20734=ORIENTED_EDGE ( 'NONE', *, *, #41502, .F. ) ;
#20736=CARTESIAN_POINT ( 'NONE',  ( -20.74999999999999289, -7.500000000000000000, 34.75000000000000000 ) ) ;
#20737=CARTESIAN_POINT ( 'NONE',  ( -3.361459833879539172, -5.496505350115500121, 34.60290016733514307 ) ) ;
#20738=CARTESIAN_POINT ( 'NONE',  ( -9.627052552794854279, -12.51329471203373700, 31.30864560766537963 ) ) ;
#20739=CARTESIAN_POINT ( 'NONE',  ( -4.153846153846152411, -9.058645607665452459, 34.76329471203371924 ) ) ;
#20740=CARTESIAN_POINT ( 'NONE',  ( 15.23076923076911093, -3.835265460704628371, 33.15142922262033665 ) ) ;
#20741=DIRECTION ( 'NONE',  ( -0.000000000000000000, 0.5000000000000011102, -0.8660254037844380415 ) ) ;
#20742=ORIENTED_EDGE ( 'NONE', *, *, #49835, .T. ) ;
#20743=CARTESIAN_POINT ( 'NONE',  ( 2.084207363968360482, -9.331801661448606566, 34.40259984581193464 ) ) ;
#20744=CARTESIAN_POINT ( 'NONE',  ( 3.480823542407545546, -11.28795663066794219, 33.01431243580653785 ) ) ;
#20745=CYLINDRICAL_SURFACE ( 'NONE', #58826, 0.2500000000000008882 ) ;
#20746=CARTESIAN_POINT ( 'NONE',  ( -6.923076923077045919, -6.835583212225970762, 34.95778746994575670 ) ) ;
#20747=EDGE_LOOP ( 'NONE', ( #86283, #39640 ) ) ;
#20748=B_SPLINE_CURVE_WITH_KNOTS ( 'NONE', 3,
 ( #51372, #44631, #17635, #58599, #59939, #59498, #72116, #73015, #11312, #87438 ),
 .UNSPECIFIED., .F., .F.,
 ( 4, 2, 2, 2, 4 ),
 ( 0.0007817359430256216575, 0.0009771253907249856981, 0.001172514838424349847, 0.001367904286123713779, 0.001563293733823077928 ),
 .UNSPECIFIED. ) ;
#20749=VERTEX_POINT ( 'NONE', #52170 ) ;
#20750=EDGE_CURVE ( 'NONE', #63009, #61570, #79659, .T. ) ;
#20751=EDGE_LOOP ( 'NONE', ( #2619, #3126 ) ) ;
#20752=CYLINDRICAL_SURFACE ( 'NONE', #17563, 0.2499999999999997502 ) ;
#20753=EDGE_CURVE ( 'NONE', #35413, #78633, #3123, .T. ) ;
#20754=ORIENTED_EDGE ( 'NONE', *, *, #61784, .T. ) ;
#20755=CARTESIAN_POINT ( 'NONE',  ( -1.161604033002534120, -8.239487800360276282, 34.69522927552633718 ) ) ;
#20756=CARTESIAN_POINT ( 'NONE',  ( -12.39628289026243380, -6.879047030191282275, 34.71129190930002295 ) ) ;
#20757=CARTESIAN_POINT ( 'NONE',  ( -5.207614543590632472, -4.118384482072085184, 33.43331474514187107 ) ) ;
#20759=CARTESIAN_POINT ( 'NONE',  ( 9.942362003946008997, -5.728107161865378494, 34.42597550085002922 ) ) ;
#20760=AXIS2_PLACEMENT_3D ( 'NONE', #78123, #15545, #44315 ) ;
#20761=ORIENTED_EDGE ( 'NONE', *, *, #50937, .T. ) ;
#20762=ADVANCED_FACE ( 'NONE', ( #5778 ), #33254, .F. ) ;
#20763=CARTESIAN_POINT ( 'NONE',  ( -11.31549840419486586, -7.369474539155828730, 34.99858011523957657 ) ) ;
#20764=CARTESIAN_POINT ( 'NONE',  ( -0.5922290646487697874, -5.496505350115500121, 34.60290016733514307 ) ) ;
#20765=ORIENTED_EDGE ( 'NONE', *, *, #50501, .F. ) ;
#20767=CARTESIAN_POINT ( 'NONE',  ( 13.38461538461538680, -12.62096338111211580, 30.90682066428153263 ) ) ;
#20768=CARTESIAN_POINT ( 'NONE',  ( 17.14299142792551578, -11.16473453929635440, 33.15142922261926373 ) ) ;
#20769=CARTESIAN_POINT ( 'NONE',  ( -15.90384615384622258, -7.565270000091922853, 34.99999999999999289 ) ) ;
#20770=CARTESIAN_POINT ( 'NONE',  ( -18.00000000000000000, -10.67929555188718282, 33.92786785259543336 ) ) ;
#20772=CARTESIAN_POINT ( 'NONE',  ( -3.296039676730006196, -6.879047030191174805, 34.71129190930000163 ) ) ;
#20773=EDGE_CURVE ( 'NONE', #53138, #22144, #26753, .T. ) ;
#20775=ORIENTED_EDGE ( 'NONE', *, *, #64087, .T. ) ;
#20776=CARTESIAN_POINT ( 'NONE',  ( 8.769230769230768274, -13.95598074871891292, 31.83374038241031911 ) ) ;
#20778=LINE ( 'NONE', #41500, #24490 ) ;
#20780=VERTEX_POINT ( 'NONE', #34129 ) ;
#20781=DIRECTION ( 'NONE',  ( -0.000000000000000000, -0.5000000000000009992, -0.8660254037844380415 ) ) ;
#20782=CARTESIAN_POINT ( 'NONE',  ( -5.076923076923075762, -6.386643153685126251, 34.62446782046654192 ) ) ;
#20783=B_SPLINE_CURVE_WITH_KNOTS ( 'NONE', 3,
 ( #15823, #56358, #50035, #71628, #35649, #969, #63099, #77512, #9492, #1412 ),
 .UNSPECIFIED., .F., .F.,
 ( 4, 2, 2, 2, 4 ),
 ( 0.0007817246256747484735, 0.0009771112852218920199, 0.001172497944769035783, 0.001367884604316179330, 0.001563271263863322876 ),
 .UNSPECIFIED. ) ;
#20784=CARTESIAN_POINT ( 'NONE',  ( -8.899921372341079717, -10.70098750199973203, 33.91152734681376302 ) ) ;
#20785=FACE_OUTER_BOUND ( 'NONE', #15691, .T. ) ;
#20786=CARTESIAN_POINT ( 'NONE',  ( -2.307692307692305711, -10.51840700105979565, 33.73612834413961536 ) ) ;
#20787=ORIENTED_EDGE ( 'NONE', *, *, #44725, .T. ) ;
#20788=CARTESIAN_POINT ( 'NONE',  ( -15.36091644020745051, -2.882441371585227508, 31.66841991370172238 ) ) ;
#20790=CYLINDRICAL_SURFACE ( 'NONE', #46947, 0.2499999999999994726 ) ;
#20791=CARTESIAN_POINT ( 'NONE',  ( 7.622668902429897919, -10.11188796281391511, 34.01382737946119050 ) ) ;
#20792=ORIENTED_EDGE ( 'NONE', *, *, #39114, .T. ) ;
#20793=CARTESIAN_POINT ( 'NONE',  ( -8.899705954306490696, -7.276987145209185215, 34.99546412871779211 ) ) ;
#20795=VECTOR ( 'NONE', #49825, 1000.000000000000000 ) ;
#20796=AXIS2_PLACEMENT_3D ( 'NONE', #84366, #30294, #23092 ) ;
#20797=EDGE_LOOP ( 'NONE', ( #81982, #11187 ) ) ;
#20800=VERTEX_POINT ( 'NONE', #41335 ) ;
#20801=CARTESIAN_POINT ( 'NONE',  ( 7.716006636715621703, -12.27039167877662251, 31.24851455888617835 ) ) ;
#20802=CYLINDRICAL_SURFACE ( 'NONE', #13350, 0.2500000000000002220 ) ;
#20803=CARTESIAN_POINT ( 'NONE',  ( -8.769230769230890843, -9.442884908241554243, 34.35708131394783038 ) ) ;
#20805=CARTESIAN_POINT ( 'NONE',  ( 6.923076923076800782, -12.51329471203414379, 31.30864560766407578 ) ) ;
#20806=CYLINDRICAL_SURFACE ( 'NONE', #23868, 0.2499999999999995559 ) ;
#20807=EDGE_CURVE ( 'NONE', #58206, #41132, #46762, .T. ) ;
#20808=ORIENTED_EDGE ( 'NONE', *, *, #88186, .T. ) ;
#20810=FACE_BOUND ( 'NONE', #9201, .T. ) ;
#20811=EDGE_LOOP ( 'NONE', ( #3632, #62338, #36762, #45133 ) ) ;
#20812=CARTESIAN_POINT ( 'NONE',  ( 6.250000000001421085, -7.500000000000154543, 35.00000000000007105 ) ) ;
#20813=CARTESIAN_POINT ( 'NONE',  ( 18.13079044096694759, -6.369690395747422684, 34.87708834333098196 ) ) ;
#20814=CARTESIAN_POINT ( 'NONE',  ( 6.249945409378045547, -5.766571408460171355, 34.70601412856602508 ) ) ;
#20815=CARTESIAN_POINT ( 'NONE',  ( 16.15384615384615330, -11.35647404775217417, 33.31231777344666511 ) ) ;
#20817=ORIENTED_EDGE ( 'NONE', *, *, #27451, .F. ) ;
#20818=VECTOR ( 'NONE', #13786, 1000.000000000000227 ) ;
#20819=ORIENTED_EDGE ( 'NONE', *, *, #8064, .T. ) ;
#20820=VERTEX_POINT ( 'NONE', #20613 ) ;
#20821=DIRECTION ( 'NONE',  ( -0.000000000000000000, 0.1736481776669307198, -0.9848077530122080203 ) ) ;
#20822=ADVANCED_FACE ( 'NONE', ( #12536 ), #19734, .F. ) ;
#20823=EDGE_CURVE ( 'NONE', #5830, #21769, #51439, .T. ) ;
#20824=ORIENTED_EDGE ( 'NONE', *, *, #83040, .T. ) ;
#20825=CARTESIAN_POINT ( 'NONE',  ( -17.29985003582992320, -10.01117774369187252, 34.36070679894347535 ) ) ;
#20829=CARTESIAN_POINT ( 'NONE',  ( 4.153846153846460609, -2.506253911140614576, 30.00000000000323297 ) ) ;
#20831=CARTESIAN_POINT ( 'NONE',  ( 15.48071474911737333, -9.272278438253398036, 34.42582936511637115 ) ) ;
#20832=CARTESIAN_POINT ( 'NONE',  ( 17.07692307692307665, -11.91647553114624181, 32.58852847137148245 ) ) ;
#20833=CARTESIAN_POINT ( 'NONE',  ( -8.546451100252703270, -3.020022701398813236, 32.48759521482552515 ) ) ;
#20834=ORIENTED_EDGE ( 'NONE', *, *, #14731, .F. ) ;
#20836=VERTEX_POINT ( 'NONE', #67483 ) ;
#20837=CARTESIAN_POINT ( 'NONE',  ( 3.903869409797562806, -2.920706130388546651, 32.31842814019191223 ) ) ;
#20838=CARTESIAN_POINT ( 'NONE',  ( 1.449870955891410462, -6.026961402152789304, 34.52809138561124769 ) ) ;
#20839=CARTESIAN_POINT ( 'NONE',  ( -9.822455662039388358, -4.299443229763728169, 33.91186481527756058 ) ) ;
#20840=DIRECTION ( 'NONE',  ( 1.000000000000000000, 0.000000000000000000, 0.000000000000000000 ) ) ;
#20841=DIRECTION ( 'NONE',  ( -0.000000000000000000, 0.6427876096865404731, -0.7660444431189770143 ) ) ;
#20842=FACE_BOUND ( 'NONE', #55962, .T. ) ;
#20843=CARTESIAN_POINT ( 'NONE',  ( 16.40390046548446890, -3.136992222400443175, 32.19305428654138979 ) ) ;
#20844=VERTEX_POINT ( 'NONE', #26494 ) ;
#20845=CARTESIAN_POINT ( 'NONE',  ( -0.3962828902624371263, -9.442884908240271713, 34.35708131394835618 ) ) ;
#20846=CARTESIAN_POINT ( 'NONE',  ( 0.4615384615384611200, -5.471508081941601098, 34.59228464037088457 ) ) ;
#20847=CARTESIAN_POINT ( 'NONE',  ( -3.480792454990687013, -3.520140089381496473, 33.17453946501458262 ) ) ;
#20848=ORIENTED_EDGE ( 'NONE', *, *, #82111, .T. ) ;
#20850=VERTEX_POINT ( 'NONE', #61149 ) ;
#20851=FACE_BOUND ( 'NONE', #14679, .T. ) ;
#20852=EDGE_CURVE ( 'NONE', #41806, #26379, #88662, .T. ) ;
#20853=LINE ( 'NONE', #20418, #1569 ) ;
#20854=AXIS2_PLACEMENT_3D ( 'NONE', #81557, #18961, #81116 ) ;
#20855=CARTESIAN_POINT ( 'NONE',  ( -12.46153846153858247, -8.613356846316285953, 34.62446782046622218 ) ) ;
#20856=CARTESIAN_POINT ( 'NONE',  ( -15.23076923076922995, -9.780366693483667717, 34.19971097300155094 ) ) ;
#20857=VERTEX_POINT ( 'NONE', #8882 ) ;
#20858=AXIS2_PLACEMENT_3D ( 'NONE', #994, #75756, #40218 ) ;
#20859=CARTESIAN_POINT ( 'NONE',  ( -14.30769230769242739, -12.46129190930018460, 30.37095296980731973 ) ) ;
#20860=CARTESIAN_POINT ( 'NONE',  ( -5.934744860487159102, -9.528491918058460186, 34.59228464037085615 ) ) ;
#20861=CARTESIAN_POINT ( 'NONE',  ( -16.21992956480203318, -12.37446782046654192, 30.86335684631486487 ) ) ;
#20862=DIRECTION ( 'NONE',  ( -0.000000000000000000, -0.7660444431189791237, -0.6427876096865379196 ) ) ;
#20863=ORIENTED_EDGE ( 'NONE', *, *, #6537, .F. ) ;
#20866=FACE_OUTER_BOUND ( 'NONE', #74122, .T. ) ;
#20868=CARTESIAN_POINT ( 'NONE',  ( 16.15384615384615330, -3.937682226553329556, 33.60647404775216529 ) ) ;
#20869=CARTESIAN_POINT ( 'NONE',  ( 16.15384615384603251, -2.625532179533778709, 30.86335684631627174 ) ) ;
#20870=CARTESIAN_POINT ( 'NONE',  ( -11.60454494941741999, -8.120952969808774569, 34.71129190930000163 ) ) ;
#20871=CARTESIAN_POINT ( 'NONE',  ( 14.30769230769231015, -8.973038597847269315, 34.52809138561121927 ) ) ;
#20872=CARTESIAN_POINT ( 'NONE',  ( 9.692307692307695177, -8.973038597847269315, 34.52809138561121927 ) ) ;
#20874=CYLINDRICAL_SURFACE ( 'NONE', #63352, 0.2500000000000009437 ) ;
#20875=CARTESIAN_POINT ( 'NONE',  ( 12.21153846153846168, -7.500000000000001776, 34.75000000000000000 ) ) ;
#20877=VERTEX_POINT ( 'NONE', #57494 ) ;
#20880=EDGE_LOOP ( 'NONE', ( #52652, #17921 ) ) ;
#20881=CARTESIAN_POINT ( 'NONE',  ( 2.980745993476266342, -5.056417327199099532, 34.11270091957320716 ) ) ;
#20883=CARTESIAN_POINT ( 'NONE',  ( -4.377331078410485965, -2.612411019501189813, 31.66733052389439962 ) ) ;
#20885=CARTESIAN_POINT ( 'NONE',  ( 13.51514108637894473, -2.882268652242222284, 31.66798894389554064 ) ) ;
#20887=CARTESIAN_POINT ( 'NONE',  ( 7.596153846153846700, -2.249999999999998668, 29.75000000000000355 ) ) ;
#20889=CARTESIAN_POINT ( 'NONE',  ( 1.384615384615386802, -2.486705287966279876, 31.30864560766543647 ) ) ;
#20890=CARTESIAN_POINT ( 'NONE',  ( -15.23076923076922995, -4.661471528628507777, 34.16647553114623292 ) ) ;
#20891=DIRECTION ( 'NONE',  ( -0.000000000000000000, -0.6427876096865404731, -0.7660444431189771253 ) ) ;
#20893=CARTESIAN_POINT ( 'NONE',  ( -4.284537620513712675, -3.530157926970578508, 32.79014554554150607 ) ) ;
#20894=FACE_OUTER_BOUND ( 'NONE', #66760, .T. ) ;
#20895=DIRECTION ( 'NONE',  ( -0.000000000000000000, 0.9848077530122085754, -0.1736481776669273613 ) ) ;
#20896=CARTESIAN_POINT ( 'NONE',  ( 5.076923076922953193, -11.06231777344772027, 33.60647404775119895 ) ) ;
#20897=CARTESIAN_POINT ( 'NONE',  ( -9.822998295418001291, -3.338472653186243644, 32.95098750199972670 ) ) ;
#20898=ORIENTED_EDGE ( 'NONE', *, *, #69220, .F. ) ;
#20899=ORIENTED_EDGE ( 'NONE', *, *, #76983, .F. ) ;
#20900=CARTESIAN_POINT ( 'NONE',  ( 3.007842271862382066, -10.77366814457252175, 33.85459836347579454 ) ) ;
#20901=DIRECTION ( 'NONE',  ( 0.000000000000000000, 0.4999999999999985567, 0.8660254037844395958 ) ) ;
#20902=CARTESIAN_POINT ( 'NONE',  ( -6.673022503163469565, -12.01375889529407281, 32.43194544308182969 ) ) ;
#20903=CARTESIAN_POINT ( 'NONE',  ( 9.757562831820528970, -12.16647553114626490, 32.15551576947920864 ) ) ;
#20904=ADVANCED_FACE ( 'NONE', ( #22387 ), #43105, .F. ) ;
#20905=EDGE_CURVE ( 'NONE', #13730, #72856, #8574, .T. ) ;
#20906=CARTESIAN_POINT ( 'NONE',  ( 12.46153846153846168, -8.973038597847269315, 34.52809138561121927 ) ) ;
#20907=CARTESIAN_POINT ( 'NONE',  ( 11.60452887181161508, -3.937682226553329556, 33.60647404775216529 ) ) ;
#20908=B_SPLINE_CURVE_WITH_KNOTS ( 'NONE', 3,
 ( #66527, #59763, #74170, #46252, #73742, #12467, #12034, #39510, #66972, #35849 ),
 .UNSPECIFIED., .F., .F.,
 ( 4, 2, 2, 2, 4 ),
 ( 0.000000000000000000, 0.0001954311564186862239, 0.0003908623128373724478, 0.0005862934692560586988, 0.0007817246256747448956 ),
 .UNSPECIFIED. ) ;
#20910=VECTOR ( 'NONE', #50851, 1000.000000000000114 ) ;
#20911=EDGE_CURVE ( 'NONE', #27559, #11993, #31037, .T. ) ;
#20913=CARTESIAN_POINT ( 'NONE',  ( -14.43838291080261271, -12.62707690430377383, 30.88035979386743435 ) ) ;
#20915=CARTESIAN_POINT ( 'NONE',  ( 10.74591031714818357, -8.586989748646452369, 34.63063291749215011 ) ) ;
#20917=CARTESIAN_POINT ( 'NONE',  ( -0.3310127597748980244, -6.852161475712351901, 34.70806712695776497 ) ) ;
#20918=VECTOR ( 'NONE', #3979, 1000.000000000000000 ) ;
#20919=CARTESIAN_POINT ( 'NONE',  ( 10.61538461538461675, -10.51840700105979565, 33.73612834413961536 ) ) ;
#20921=ORIENTED_EDGE ( 'NONE', *, *, #10928, .F. ) ;
#20922=VERTEX_POINT ( 'NONE', #42669 ) ;
#20923=EDGE_CURVE ( 'NONE', #87771, #63694, #83667, .T. ) ;
#20925=EDGE_LOOP ( 'NONE', ( #58644, #20104 ) ) ;
#20926=CARTESIAN_POINT ( 'NONE',  ( -17.20707028636129721, -10.88202310037936194, 33.43294751532457099 ) ) ;
#20927=CARTESIAN_POINT ( 'NONE',  ( 13.38461538461538680, -1.466349020453238561, 30.81389545987213907 ) ) ;
#20929=CARTESIAN_POINT ( 'NONE',  ( 2.307692307692187583, -11.48612834414049644, 32.76840700105863391 ) ) ;
#20931=CARTESIAN_POINT ( 'NONE',  ( -17.93393164899755732, -4.098570777380720287, 33.41473453929635440 ) ) ;
#20932=CARTESIAN_POINT ( 'NONE',  ( 14.24242186173153435, -12.46129190929999986, 30.37095296980880832 ) ) ;
#20933=EDGE_LOOP ( 'NONE', ( #68853, #3932 ) ) ;
#20934=EDGE_LOOP ( 'NONE', ( #32158, #5982, #48395, #74502 ) ) ;
#20935=VECTOR ( 'NONE', #70621, 1000.000000000000227 ) ;
#20936=EDGE_LOOP ( 'NONE', ( #19508, #56553 ) ) ;
#20937=CYLINDRICAL_SURFACE ( 'NONE', #14263, 0.2499999999999973355 ) ;
#20938=ORIENTED_EDGE ( 'NONE', *, *, #17938, .F. ) ;
#20939=CARTESIAN_POINT ( 'NONE',  ( -9.942330929600657896, -5.056417327199099532, 34.11270091957321426 ) ) ;
#20940=DIRECTION ( 'NONE',  ( 0.000000000000000000, 0.6427876096865368094, 0.7660444431189802339 ) ) ;
#20941=B_SPLINE_CURVE_WITH_KNOTS ( 'NONE', 3,
 ( #72313, #17377, #59697, #11068, #65552, #73673, #11966, #39443, #58799, #65102 ),
 .UNSPECIFIED., .F., .F.,
 ( 4, 2, 2, 2, 4 ),
 ( 0.0007817359430256322827, 0.0009771253907249989254, 0.001172514838424365676, 0.001367904286123732428, 0.001563293733823098962 ),
 .UNSPECIFIED. ) ;
#20943=VERTEX_POINT ( 'NONE', #50281 ) ;
#20944=ORIENTED_EDGE ( 'NONE', *, *, #45127, .T. ) ;
#20945=CARTESIAN_POINT ( 'NONE',  ( 6.923076923076924238, -3.886160181151819604, 36.00935417666054406 ) ) ;
#20946=FACE_BOUND ( 'NONE', #25449, .T. ) ;
#20947=CARTESIAN_POINT ( 'NONE',  ( -15.23076923076922995, -13.87047571288749737, 32.06866353760679544 ) ) ;
#20948=DIRECTION ( 'NONE',  ( -0.000000000000000000, -0.9396926207859092051, -0.3420201433256662704 ) ) ;
#20949=ORIENTED_EDGE ( 'NONE', *, *, #27663, .F. ) ;
#20951=CARTESIAN_POINT ( 'NONE',  ( -1.384615384615383471, -6.189225973068211317, 35.74407628777942847 ) ) ;
#20952=CARTESIAN_POINT ( 'NONE',  ( -16.85391023282967993, -12.64618726649961289, 30.78989965857442712 ) ) ;
#20953=CARTESIAN_POINT ( 'NONE',  ( 15.45354889974729495, -6.717445702608402236, 34.94155399931962336 ) ) ;
#20954=VERTEX_POINT ( 'NONE', #77770 ) ;
#20955=CARTESIAN_POINT ( 'NONE',  ( -11.47239420511146513, -12.34228464037088813, 31.77849191805839268 ) ) ;
#20956=CARTESIAN_POINT ( 'NONE',  ( -7.596208327805703320, -11.37275283266504111, 32.91324779482534524 ) ) ;
#20957=CARTESIAN_POINT ( 'NONE',  ( -4.088591014333315066, -2.379036618887895305, 30.90682066428159303 ) ) ;
#20958=CARTESIAN_POINT ( 'NONE',  ( -1.384615384615383471, -1.242168528481310874, 33.36296068462461051 ) ) ;
#20959=CARTESIAN_POINT ( 'NONE',  ( -15.23076923076922995, -7.500000000000001776, 35.04278698407183867 ) ) ;
#20960=AXIS2_PLACEMENT_3D ( 'NONE', #30926, #58394, #85892 ) ;
#20961=FACE_BOUND ( 'NONE', #61463, .T. ) ;
#20962=CARTESIAN_POINT ( 'NONE',  ( 4.853996859406927378, -11.24512374952581872, 33.06303171183252942 ) ) ;
#20963=CARTESIAN_POINT ( 'NONE',  ( -6.066082379360133281, -9.905515769479276145, 34.41647553114623292 ) ) ;
#20964=CARTESIAN_POINT ( 'NONE',  ( 5.299702745901139878, -2.353885683473779800, 30.79025554430704759 ) ) ;
#20965=CARTESIAN_POINT ( 'NONE',  ( -18.22348492456433178, -2.353723527008296568, 30.78948104536958752 ) ) ;
#20966=CARTESIAN_POINT ( 'NONE',  ( -9.692307692307384315, -2.506253911140614576, 30.00000000000323297 ) ) ;
#20971=ORIENTED_EDGE ( 'NONE', *, *, #5748, .F. ) ;
#20972=B_SPLINE_CURVE_WITH_KNOTS ( 'NONE', 3,
 ( #84395, #51445, #78063, #37513, #71295, #57789, #8735, #50137, #23557, #51007 ),
 .UNSPECIFIED., .F., .F.,
 ( 4, 2, 2, 2, 4 ),
 ( 0.0007817359430256295722, 0.0009771253907249954559, 0.001172514838424361123, 0.001367904286123726790, 0.001563293733823092673 ),
 .UNSPECIFIED. ) ;
#20973=CARTESIAN_POINT ( 'NONE',  ( 0.4615384615387678746, -2.506253911140615021, 30.00000000000323297 ) ) ;
#20974=ORIENTED_EDGE ( 'NONE', *, *, #43963, .F. ) ;
#20975=CARTESIAN_POINT ( 'NONE',  ( 17.86930853333243618, -12.11776431015576172, 31.66791131148498906 ) ) ;
#20976=CARTESIAN_POINT ( 'NONE',  ( -7.976845312821407852, -9.804603061927743113, 34.18744698557895845 ) ) ;
#20977=CARTESIAN_POINT ( 'NONE',  ( 13.51545371510214189, -7.277220318596961057, 34.99547417642776992 ) ) ;
#20979=ORIENTED_EDGE ( 'NONE', *, *, #40498, .T. ) ;
#20980=CARTESIAN_POINT ( 'NONE',  ( 17.93424657168666059, -7.249945578846654470, 34.99404164642496795 ) ) ;
#20982=B_SPLINE_CURVE_WITH_KNOTS ( 'NONE', 3,
 ( #10013, #72600, #45573, #37478, #23522, #57316, #85682, #24406, #51409, #73051 ),
 .UNSPECIFIED., .F., .F.,
 ( 4, 2, 2, 2, 4 ),
 ( 0.000000000000000000, 0.0001954339857564077183, 0.0003908679715128154366, 0.0005863019572692231007, 0.0007817359430256308733 ),
 .UNSPECIFIED. ) ;
#20983=CARTESIAN_POINT ( 'NONE',  ( -11.53846153846153655, -12.78798330534103123, 29.99999999999997868 ) ) ;
#20984=FACE_OUTER_BOUND ( 'NONE', #12603, .T. ) ;
#20986=CARTESIAN_POINT ( 'NONE',  ( 10.55011461482829560, -2.657715359629088780, 31.77849191805832874 ) ) ;
#20987=CARTESIAN_POINT ( 'NONE',  ( -12.39628332202562433, -8.656820664281605460, 34.87096338111211224 ) ) ;
#20990=CARTESIAN_POINT ( 'NONE',  ( -10.36543909703647515, -2.824170634883621744, 31.52227843825338738 ) ) ;
#20991=CARTESIAN_POINT ( 'NONE',  ( -1.384615384615383471, -2.900454961884010974, 35.62045528018868623 ) ) ;
#20992=ORIENTED_EDGE ( 'NONE', *, *, #61560, .F. ) ;
#20995=ADVANCED_FACE ( 'NONE', ( #55724 ), #8438, .F. ) ;
#20997=DIRECTION ( 'NONE',  ( -0.000000000000000000, 1.000000000000000000, -0.000000000000000000 ) ) ;
#20998=VERTEX_POINT ( 'NONE', #48975 ) ;
#20999=VECTOR ( 'NONE', #68300, 1000.000000000000000 ) ;
#21001=CARTESIAN_POINT ( 'NONE',  ( -16.82686865700962286, -9.233818618650598609, 34.70587769442853698 ) ) ;
#21002=DIRECTION ( 'NONE',  ( -0.000000000000000000, -0.5000000000000009992, -0.8660254037844380415 ) ) ;
#21003=ORIENTED_EDGE ( 'NONE', *, *, #14163, .T. ) ;
#21004=CARTESIAN_POINT ( 'NONE',  ( -7.622726884292275074, -7.630147231320743018, 34.74852402298682819 ) ) ;
#21006=CARTESIAN_POINT ( 'NONE',  ( -1.634592115557738090, -10.66389620160130036, 33.62221079203477103 ) ) ;
#21007=VECTOR ( 'NONE', #69639, 1000.000000000000000 ) ;
#21008=CARTESIAN_POINT ( 'NONE',  ( -10.61538461538461320, -9.058645607665452459, 34.76329471203371924 ) ) ;
#21009=CARTESIAN_POINT ( 'NONE',  ( 2.980746006547771554, -2.588893531581426544, 31.60682220781847818 ) ) ;
#21010=CARTESIAN_POINT ( 'NONE',  ( -11.53846153846153655, -13.78497067705608181, 32.30358669280327177 ) ) ;
#21011=EDGE_CURVE ( 'NONE', #8206, #14619, #42233, .T. ) ;
#21012=ORIENTED_EDGE ( 'NONE', *, *, #66591, .T. ) ;
#21013=ORIENTED_EDGE ( 'NONE', *, *, #75153, .T. ) ;
#21014=ORIENTED_EDGE ( 'NONE', *, *, #39422, .F. ) ;
#21015=CARTESIAN_POINT ( 'NONE',  ( -13.51530685128294884, -3.530157926970578952, 32.79014554554150607 ) ) ;
#21016=CARTESIAN_POINT ( 'NONE',  ( -3.903791842207836815, -3.136992222400443175, 32.19305428654139689 ) ) ;
#21018=CARTESIAN_POINT ( 'NONE',  ( -7.911423846710166075, -11.06231777344662781, 33.60647404775220082 ) ) ;
#21019=ORIENTED_EDGE ( 'NONE', *, *, #89064, .F. ) ;
#21020=CARTESIAN_POINT ( 'NONE',  ( -17.30040802064702987, -4.386631170607603991, 33.66268669641500111 ) ) ;
#21022=VECTOR ( 'NONE', #19880, 1000.000000000000227 ) ;
#21023=EDGE_CURVE ( 'NONE', #63925, #19030, #64240, .T. ) ;
#21025=VERTEX_POINT ( 'NONE', #1674 ) ;
#21026=LINE ( 'NONE', #20590, #65997 ) ;
#21029=CARTESIAN_POINT ( 'NONE',  ( 4.219101725122176738, -6.026961402152789304, 34.52809138561124769 ) ) ;
#21030=B_SPLINE_CURVE_WITH_KNOTS ( 'NONE', 3,
 ( #66056, #4368, #77802, #57972, #43573, #71047, #51188, #78696, #9360, #4820 ),
 .UNSPECIFIED., .F., .F.,
 ( 4, 2, 2, 2, 4 ),
 ( 0.000000000000000000, 0.0001954339857564097512, 0.0003908679715128195024, 0.0005863019572692292807, 0.0007817359430256390048 ),
 .UNSPECIFIED. ) ;
#21032=EDGE_CURVE ( 'NONE', #52380, #33767, #89151, .T. ) ;
#21033=EDGE_CURVE ( 'NONE', #1104, #28433, #17856, .T. ) ;
#21035=CYLINDRICAL_SURFACE ( 'NONE', #65474, 0.2499999999999997502 ) ;
#21036=VECTOR ( 'NONE', #64300, 1000.000000000000000 ) ;
#21037=ORIENTED_EDGE ( 'NONE', *, *, #36130, .T. ) ;
#21039=ORIENTED_EDGE ( 'NONE', *, *, #85642, .F. ) ;
#21040=CARTESIAN_POINT ( 'NONE',  ( -11.53846153846153655, -8.318370150425687726, 35.83090037661290239 ) ) ;
#21041=CARTESIAN_POINT ( 'NONE',  ( 13.38461538461538680, -13.75783147151868846, 33.36296068462461051 ) ) ;
#21042=ORIENTED_EDGE ( 'NONE', *, *, #17418, .F. ) ;
#21043=CARTESIAN_POINT ( 'NONE',  ( 6.673053685783957967, -6.695914987888143877, 34.68535235679833306 ) ) ;
#21044=CARTESIAN_POINT ( 'NONE',  ( -0.5268084620947809382, -6.835583212224499938, 34.95778746994557906 ) ) ;
#21045=ORIENTED_EDGE ( 'NONE', *, *, #24394, .T. ) ;
#21046=CARTESIAN_POINT ( 'NONE',  ( -17.86947429823643674, -2.619367082507847222, 30.83698974864643461 ) ) ;
#21047=CARTESIAN_POINT ( 'NONE',  ( 0.2380535369741303697, -9.417330523894424488, 34.63758898049880486 ) ) ;
#21048=ORIENTED_EDGE ( 'NONE', *, *, #35681, .F. ) ;
#21049=FACE_BOUND ( 'NONE', #28218, .T. ) ;
#21050=CARTESIAN_POINT ( 'NONE',  ( -15.29603923132555110, -8.656820664281498878, 34.87096338111211935 ) ) ;
#21051=CARTESIAN_POINT ( 'NONE',  ( 15.90386940979756858, -2.544273027872574477, 31.48422191005632698 ) ) ;
#21052=FACE_OUTER_BOUND ( 'NONE', #21843, .T. ) ;
#21053=CARTESIAN_POINT ( 'NONE',  ( 18.24994540937804288, -2.986452184633680229, 32.43230066228895225 ) ) ;
#21054=DIRECTION ( 'NONE',  ( -0.000000000000000000, 0.6427876096865404731, -0.7660444431189770143 ) ) ;
#21055=VECTOR ( 'NONE', #57230, 1000.000000000000000 ) ;
#21056=DIRECTION ( 'NONE',  ( -0.000000000000000000, -0.7660444431189791237, -0.6427876096865379196 ) ) ;
#21057=CARTESIAN_POINT ( 'NONE',  ( -2.557715544985270206, -3.711651800289232916, 33.01384336483936011 ) ) ;
#21058=ORIENTED_EDGE ( 'NONE', *, *, #56870, .F. ) ;
#21059=CARTESIAN_POINT ( 'NONE',  ( -8.096177070375304652, -6.652501968072648708, 34.93155406624980941 ) ) ;
#21062=B_SPLINE_CURVE_WITH_KNOTS ( 'NONE', 3,
 ( #38946, #11462, #31737, #10574, #24969, #67300, #45235, #5150, #5596, #38044 ),
 .UNSPECIFIED., .F., .F.,
 ( 4, 2, 2, 2, 4 ),
 ( 0.000000000000000000, 0.0001954339857564081520, 0.0003908679715128163040, 0.0005863019572692244018, 0.0007817359430256326080 ),
 .UNSPECIFIED. ) ;
#21063=CARTESIAN_POINT ( 'NONE',  ( 14.17700084102475344, -9.804603061927743113, 34.18744698557895845 ) ) ;
#21064=LINE ( 'NONE', #56195, #82156 ) ;
#21065=ORIENTED_EDGE ( 'NONE', *, *, #55333, .F. ) ;
#21066=EDGE_CURVE ( 'NONE', #29522, #21125, #36486, .T. ) ;
#21067=CYLINDRICAL_SURFACE ( 'NONE', #1130, 0.2499999999999973355 ) ;
#21068=CARTESIAN_POINT ( 'NONE',  ( 4.219101725122177626, -10.21337939537593797, 33.94971097300152252 ) ) ;
#21069=B_SPLINE_CURVE_WITH_KNOTS ( 'NONE', 3,
 ( #35338, #76775, #77651, #42548, #1112, #35795, #42986, #6981, #55605, #1556 ),
 .UNSPECIFIED., .F., .F.,
 ( 4, 2, 2, 2, 4 ),
 ( 0.0007817246256747465219, 0.0009771112852218902852, 0.001172497944769034049, 0.001367884604316177595, 0.001563271263863321358 ),
 .UNSPECIFIED. ) ;
#21070=FACE_BOUND ( 'NONE', #13851, .T. ) ;
#21071=CARTESIAN_POINT ( 'NONE',  ( 6.923076923076800782, -4.320704448113951379, 33.92786785259630022 ) ) ;
#21072=CARTESIAN_POINT ( 'NONE',  ( 0.4615384615384611200, -10.67929555188718282, 33.92786785259544047 ) ) ;
#21073=CARTESIAN_POINT ( 'NONE',  ( -8.834501215191544077, -6.879047030191174805, 34.71129190930000163 ) ) ;
#21074=CARTESIAN_POINT ( 'NONE',  ( -15.23076923076922995, -8.973038597847269315, 34.52809138561121927 ) ) ;
#21079=EDGE_LOOP ( 'NONE', ( #64408, #33490, #24578, #79511 ) ) ;
#21080=ORIENTED_EDGE ( 'NONE', *, *, #18960, .T. ) ;
#21081=FACE_OUTER_BOUND ( 'NONE', #67571, .T. ) ;
#21083=CARTESIAN_POINT ( 'NONE',  ( -5.999999999999998224, -2.486705287966279876, 31.30864560766543647 ) ) ;
#21084=CARTESIAN_POINT ( 'NONE',  ( -8.992715693795101828, -8.539481045369596401, 34.89627647299170832 ) ) ;
#21085=LINE ( 'NONE', #27855, #52896 ) ;
#21088=CARTESIAN_POINT ( 'NONE',  ( -12.71156168575991963, -4.175268141568685643, 33.81360843649122216 ) ) ;
#21089=DIRECTION ( 'NONE',  ( -0.000000000000000000, -0.1736481776669307198, -0.9848077530122080203 ) ) ;
#21090=CARTESIAN_POINT ( 'NONE',  ( 6.130790440966953803, -3.957578996910242619, 33.62503395064540257 ) ) ;
#21091=CARTESIAN_POINT ( 'NONE',  ( -5.076923076923075762, -12.78798330534102945, 29.74999999999997868 ) ) ;
#21092=CARTESIAN_POINT ( 'NONE',  ( -14.98071491913091613, -11.28795663066794575, 33.01431243580653785 ) ) ;
#21094=CARTESIAN_POINT ( 'NONE',  ( -0.3954711281883867002, -3.937682226553329556, 33.60647404775216529 ) ) ;
#21096=CARTESIAN_POINT ( 'NONE',  ( -14.24243673641628050, -3.300289026998473041, 32.46337939537591666 ) ) ;
#21097=CARTESIAN_POINT ( 'NONE',  ( 12.71159277317678082, -2.779044189368095719, 31.39831045268885745 ) ) ;
#21098=ORIENTED_EDGE ( 'NONE', *, *, #54483, .F. ) ;
#21099=CARTESIAN_POINT ( 'NONE',  ( -0.3307466537136750095, -3.530189275343204702, 32.79018710029569661 ) ) ;
#21100=CARTESIAN_POINT ( 'NONE',  ( -2.307692307692427391, -12.46129190930018460, 30.37095296980731973 ) ) ;
#21101=AXIS2_PLACEMENT_3D ( 'NONE', #49275, #22681, #29893 ) ;
#21103=EDGE_CURVE ( 'NONE', #27440, #18632, #66021, .T. ) ;
#21104=CARTESIAN_POINT ( 'NONE',  ( -0.3962833220256226641, -11.06231777344671130, 33.60647404775212976 ) ) ;
#21105=CARTESIAN_POINT ( 'NONE',  ( -2.307692307692305711, -4.661471528628507777, 34.16647553114623292 ) ) ;
#21106=ORIENTED_EDGE ( 'NONE', *, *, #71200, .F. ) ;
#21107=DIRECTION ( 'NONE',  ( -0.000000000000000000, 0.9848077530122086864, -0.1736481776669273891 ) ) ;
#21108=CARTESIAN_POINT ( 'NONE',  ( -9.561515884482904681, -4.809403383903225304, 33.96459661697924304 ) ) ;
#21109=ORIENTED_EDGE ( 'NONE', *, *, #69265, .F. ) ;
#21110=CARTESIAN_POINT ( 'NONE',  ( 8.069165197766695385, -3.587049720035815348, 32.86302985866382897 ) ) ;
#21111=CARTESIAN_POINT ( 'NONE',  ( 12.59232890250541281, -5.496552790871120031, 34.60292014791297532 ) ) ;
#21113=ADVANCED_FACE ( 'NONE', ( #24600 ), #73239, .F. ) ;
#21114=EDGE_LOOP ( 'NONE', ( #27877, #76289, #51780, #74611 ) ) ;
#21116=B_SPLINE_CURVE_WITH_KNOTS ( 'NONE', 3,
 ( #84480, #37604, #9690, #2921, #70064, #63303, #36723, #1611, #10140, #22323 ),
 .UNSPECIFIED., .F., .F.,
 ( 4, 2, 2, 2, 4 ),
 ( 0.000000000000000000, 0.0001954339857564074473, 0.0003908679715128148945, 0.0005863019572692223418, 0.0007817359430256297891 ),
 .UNSPECIFIED. ) ;
#21117=B_SPLINE_CURVE_WITH_KNOTS ( 'NONE', 3,
 ( #7429, #6977, #34887, #34450, #662, #7869, #35333, #63247, #8761, #84425 ),
 .UNSPECIFIED., .F., .F.,
 ( 4, 2, 2, 2, 4 ),
 ( 0.000000000000000000, 0.0001954311564186876876, 0.0003908623128373753751, 0.0005862934692560630356, 0.0007817246256747507503 ),
 .UNSPECIFIED. ) ;
#21119=EDGE_LOOP ( 'NONE', ( #51930, #1035, #10381, #72432 ) ) ;
#21120=CARTESIAN_POINT ( 'NONE',  ( -10.74607521849492464, -3.957541250942358424, 33.62499894934981626 ) ) ;
#21121=B_SPLINE_CURVE_WITH_KNOTS ( 'NONE', 3,
 ( #65933, #79013, #59184, #86688, #87575, #17313, #24954, #66837, #11902, #66389 ),
 .UNSPECIFIED., .F., .F.,
 ( 4, 2, 2, 2, 4 ),
 ( 0.000000000000000000, 0.0001954339857564074473, 0.0003908679715128148945, 0.0005863019572692223418, 0.0007817359430256297891 ),
 .UNSPECIFIED. ) ;
#21124=ADVANCED_FACE ( 'NONE', ( #37671 ), #9756, .F. ) ;
#21125=VERTEX_POINT ( 'NONE', #57940 ) ;
#21126=ORIENTED_EDGE ( 'NONE', *, *, #30433, .F. ) ;
#21127=CARTESIAN_POINT ( 'NONE',  ( 6.222779541268409709, -6.760870238392817200, 34.69528174975672385 ) ) ;
#21128=VERTEX_POINT ( 'NONE', #86330 ) ;
#21129=ADVANCED_FACE ( 'NONE', ( #10208 ), #16960, .F. ) ;
#21130=FACE_OUTER_BOUND ( 'NONE', #79317, .T. ) ;
#21131=CARTESIAN_POINT ( 'NONE',  ( -5.299850035829926753, -9.172386477786396597, 34.72672124145550043 ) ) ;
#21132=CARTESIAN_POINT ( 'NONE',  ( -5.777220331021931443, -5.827830569534416583, 34.72679350104403539 ) ) ;
#21133=EDGE_CURVE ( 'NONE', #71551, #80250, #38550, .T. ) ;
#21134=CARTESIAN_POINT ( 'NONE',  ( -2.557669038634660108, -5.728515186090277211, 34.42611988154120439 ) ) ;
#21135=CARTESIAN_POINT ( 'NONE',  ( -0.3307480205715112032, -5.496552790871119143, 34.60292014791297532 ) ) ;
#21137=AXIS2_PLACEMENT_3D ( 'NONE', #22639, #9148, #14118 ) ;
#21138=CARTESIAN_POINT ( 'NONE',  ( 15.29596321255258928, -2.506253911140448043, 29.99999999999988631 ) ) ;
#21139=EDGE_CURVE ( 'NONE', #9985, #83657, #13824, .T. ) ;
#21140=ORIENTED_EDGE ( 'NONE', *, *, #49791, .T. ) ;
#21142=EDGE_LOOP ( 'NONE', ( #24999, #60234, #19653, #60467 ) ) ;
#21143=CARTESIAN_POINT ( 'NONE',  ( -17.07692307692307665, -9.780366693483667717, 34.19971097300155094 ) ) ;
#21145=CARTESIAN_POINT ( 'NONE',  ( 16.82689985270161870, -2.341070481393820124, 30.72580821765574299 ) ) ;
#21147=B_SPLINE_CURVE_WITH_KNOTS ( 'NONE', 3,
 ( #55967, #35255, #48766, #49658, #76237, #35715, #14102, #41572, #145, #591 ),
 .UNSPECIFIED., .F., .F.,
 ( 4, 2, 2, 2, 4 ),
 ( 0.000000000000000000, 0.0001954311564186870099, 0.0003908623128373740199, 0.0005862934692560609756, 0.0007817246256747480398 ),
 .UNSPECIFIED. ) ;
#21148=EDGE_CURVE ( 'NONE', #70481, #86621, #18295, .T. ) ;
#21149=FACE_OUTER_BOUND ( 'NONE', #33413, .T. ) ;
#21150=CARTESIAN_POINT ( 'NONE',  ( 9.442284455014730682, -5.056417327199099532, 34.11270091957321426 ) ) ;
#21151=EDGE_LOOP ( 'NONE', ( #41117, #88489 ) ) ;
#21152=DIRECTION ( 'NONE',  ( -0.000000000000000000, -0.9396926207859093161, -0.3420201433256663259 ) ) ;
#21153=ORIENTED_EDGE ( 'NONE', *, *, #48661, .F. ) ;
#21154=ORIENTED_EDGE ( 'NONE', *, *, #12372, .F. ) ;
#21156=B_SPLINE_CURVE_WITH_KNOTS ( 'NONE', 3,
 ( #77060, #57665, #36942, #65304, #64406, #77495, #2264, #57226, #22991, #84276 ),
 .UNSPECIFIED., .F., .F.,
 ( 4, 2, 2, 2, 4 ),
 ( 0.0007817246256747489071, 0.0009771112852218920199, 0.001172497944769035133, 0.001367884604316178246, 0.001563271263863321358 ),
 .UNSPECIFIED. ) ;
#21157=AXIS2_PLACEMENT_3D ( 'NONE', #10271, #9385, #58892 ) ;
#21158=ORIENTED_EDGE ( 'NONE', *, *, #64593, .T. ) ;
#21159=CARTESIAN_POINT ( 'NONE',  ( -6.700064078983529292, -4.762714258010880997, 34.23016756924214832 ) ) ;
#21160=EDGE_CURVE ( 'NONE', #37680, #58206, #46046, .T. ) ;
#21161=CARTESIAN_POINT ( 'NONE',  ( 12.39626846098214230, -2.379036618887870436, 30.90682066428147934 ) ) ;
#21163=FACE_BOUND ( 'NONE', #56620, .T. ) ;
#21165=CARTESIAN_POINT ( 'NONE',  ( -11.60454391782167249, -6.343179335718451384, 34.87096338111212646 ) ) ;
#21166=CARTESIAN_POINT ( 'NONE',  ( -16.02332071561251325, -5.070358843744209310, 34.40418822224088302 ) ) ;
#21167=CARTESIAN_POINT ( 'NONE',  ( 1.384615384615386802, -1.129524287112498415, 32.06866353760679544 ) ) ;
#21168=EDGE_CURVE ( 'NONE', #44468, #57842, #39521, .T. ) ;
#21169=CARTESIAN_POINT ( 'NONE',  ( -17.07692307692319744, -8.656820664282941280, 34.87096338111179961 ) ) ;
#21170=DIRECTION ( 'NONE',  ( 0.000000000000000000, 0.6427876096865368094, 0.7660444431189802339 ) ) ;
#21172=DIRECTION ( 'NONE',  ( -0.000000000000000000, 0.7660444431189791237, -0.6427876096865379196 ) ) ;
#21173=VERTEX_POINT ( 'NONE', #75454 ) ;
#21174=ORIENTED_EDGE ( 'NONE', *, *, #21160, .F. ) ;
#21175=CARTESIAN_POINT ( 'NONE',  ( -17.01166750564705055, -10.21337939537593797, 33.94971097300152252 ) ) ;
#21177=CARTESIAN_POINT ( 'NONE',  ( -5.076923076923075762, -1.367168528481310208, 33.57946703557072254 ) ) ;
#21178=DIRECTION ( 'NONE',  ( 0.000000000000000000, 0.8660254037844377084, 0.5000000000000015543 ) ) ;
#21179=CARTESIAN_POINT ( 'NONE',  ( -10.36533019547115941, -12.41089969410671223, 31.60739465890703670 ) ) ;
#21180=CARTESIAN_POINT ( 'NONE',  ( 9.942253210655836781, -2.587454068350148351, 30.68340429815432202 ) ) ;
#21183=CARTESIAN_POINT ( 'NONE',  ( 13.13463865367303285, -4.943428324936578910, 34.04746400365624481 ) ) ;
#21184=B_SPLINE_CURVE_WITH_KNOTS ( 'NONE', 3,
 ( #77921, #31056, #16227, #85135, #51760, #24299, #24754, #18008, #17562, #23414 ),
 .UNSPECIFIED., .F., .F.,
 ( 4, 2, 2, 2, 4 ),
 ( 0.000000000000000000, 0.0001954339857564083417, 0.0003908679715128166835, 0.0005863019572692250523, 0.0007817359430256333669 ),
 .UNSPECIFIED. ) ;
#21185=FACE_OUTER_BOUND ( 'NONE', #58123, .T. ) ;
#21186=CARTESIAN_POINT ( 'NONE',  ( -14.05774689831426372, -12.45601412856602686, 31.48342859153981621 ) ) ;
#21187=CARTESIAN_POINT ( 'NONE',  ( -7.846153846153844924, -11.16473453929635440, 33.15142922261926373 ) ) ;
#21188=EDGE_LOOP ( 'NONE', ( #56520, #4600, #65234, #32143 ) ) ;
#21189=EDGE_CURVE ( 'NONE', #39874, #77096, #20210, .T. ) ;
#21190=EDGE_LOOP ( 'NONE', ( #47966, #74429 ) ) ;
#21191=VERTEX_POINT ( 'NONE', #13750 ) ;
#21192=EDGE_CURVE ( 'NONE', #79428, #21592, #72833, .T. ) ;
#21193=VECTOR ( 'NONE', #44865, 1000.000000000000227 ) ;
#21194=CARTESIAN_POINT ( 'NONE',  ( -7.173100160369890510, -8.432397168068783699, 34.66272746175022945 ) ) ;
#21195=EDGE_LOOP ( 'NONE', ( #5111, #57766 ) ) ;
#21196=FACE_OUTER_BOUND ( 'NONE', #71129, .T. ) ;
#21197=DIRECTION ( 'NONE',  ( 0.000000000000000000, 0.000000000000000000, -1.000000000000000000 ) ) ;
#21198=CARTESIAN_POINT ( 'NONE',  ( 13.38461538461526423, -3.083524468854526912, 32.58852847137268327 ) ) ;
#21200=ADVANCED_FACE ( 'NONE', ( #40792 ), #12863, .F. ) ;
#21201=CARTESIAN_POINT ( 'NONE',  ( 12.39545505058258001, -9.780366693483667717, 34.19971097300155805 ) ) ;
#21202=VERTEX_POINT ( 'NONE', #6558 ) ;
#21203=DIRECTION ( 'NONE',  ( -0.000000000000000000, -0.9396926207859092051, -0.3420201433256662704 ) ) ;
#21204=CYLINDRICAL_SURFACE ( 'NONE', #59712, 0.2500000000000002220 ) ;
#21205=ORIENTED_EDGE ( 'NONE', *, *, #78966, .T. ) ;
#21206=CARTESIAN_POINT ( 'NONE',  ( -17.07692307692307665, -1.422936976036506707, 30.56769352161908415 ) ) ;
#21207=CARTESIAN_POINT ( 'NONE',  ( -6.000000000000121680, -12.16647553114689728, 32.15551576947799362 ) ) ;
#21208=CARTESIAN_POINT ( 'NONE',  ( -0.5916864312701578532, -4.299443229763728169, 33.91186481527756058 ) ) ;
#21209=CARTESIAN_POINT ( 'NONE',  ( -16.21916906933833147, -7.749976743299138882, 34.99404534957040624 ) ) ;
#21210=CARTESIAN_POINT ( 'NONE',  ( -12.71151519248081563, -2.779195860258146578, 31.39871582349836032 ) ) ;
#21211=VECTOR ( 'NONE', #42730, 1000.000000000000114 ) ;
#21212=CARTESIAN_POINT ( 'NONE',  ( 9.692307692307695177, -9.780366693483667717, 34.19971097300155094 ) ) ;
#21213=CYLINDRICAL_SURFACE ( 'NONE', #29211, 0.2500000000000008882 ) ;
#21215=ORIENTED_EDGE ( 'NONE', *, *, #45850, .F. ) ;
#21216=CYLINDRICAL_SURFACE ( 'NONE', #18709, 0.2500000000000008882 ) ;
#21217=B_SPLINE_CURVE_WITH_KNOTS ( 'NONE', 3,
 ( #67054, #46779, #12552, #688, #19749, #12993, #40478, #6243, #33708, #55624 ),
 .UNSPECIFIED., .F., .F.,
 ( 4, 2, 2, 2, 4 ),
 ( 0.0007817359430256282712, 0.0009771253907249945886, 0.001172514838424360689, 0.001367904286123726790, 0.001563293733823093107 ),
 .UNSPECIFIED. ) ;
#21219=CARTESIAN_POINT ( 'NONE',  ( 9.692307692307695177, -2.833524468853757305, 32.15551576947925838 ) ) ;
#21220=CARTESIAN_POINT ( 'NONE',  ( -7.846153846153967493, -3.083524468854526912, 32.58852847137268327 ) ) ;
#21221=ORIENTED_EDGE ( 'NONE', *, *, #86306, .T. ) ;
#21223=CARTESIAN_POINT ( 'NONE',  ( -3.480792468062196221, -10.76384336483936011, 33.53834819971076087 ) ) ;
#21224=EDGE_CURVE ( 'NONE', #74312, #15069, #34022, .T. ) ;
#21225=CARTESIAN_POINT ( 'NONE',  ( -0.7115616857599196265, -12.68155406624981119, 30.59749803192733708 ) ) ;
#21226=CARTESIAN_POINT ( 'NONE',  ( 9.915734091222482505, -7.630147987733840509, 34.99859428049665411 ) ) ;
#21227=EDGE_LOOP ( 'NONE', ( #34198, #83201 ) ) ;
#21228=CARTESIAN_POINT ( 'NONE',  ( 16.85399685940691938, -3.105860786376062332, 32.13614157043599562 ) ) ;
#21229=CARTESIAN_POINT ( 'NONE',  ( 17.07692307692307665, -5.557115091759785130, 34.35708131394839171 ) ) ;
#21230=DIRECTION ( 'NONE',  ( 0.000000000000000000, 0.8660254037844377084, -0.5000000000000015543 ) ) ;
#21232=FACE_OUTER_BOUND ( 'NONE', #82663, .T. ) ;
#21233=VERTEX_POINT ( 'NONE', #40349 ) ;
#21234=CARTESIAN_POINT ( 'NONE',  ( 12.52679360105129902, -12.51329471203373345, 31.30864560766537963 ) ) ;
#21235=CARTESIAN_POINT ( 'NONE',  ( 0.7115928814519132395, -10.06805714834173848, 34.32951233291982618 ) ) ;
#21238=CYLINDRICAL_SURFACE ( 'NONE', #76386, 0.2499999999999998890 ) ;
#21239=CARTESIAN_POINT ( 'NONE',  ( 7.846153846153725020, -10.21337939537710326, 33.94971097300076224 ) ) ;
#21240=CARTESIAN_POINT ( 'NONE',  ( 1.384615384615386802, -4.098570777380720287, 33.41473453929634729 ) ) ;
#21241=CARTESIAN_POINT ( 'NONE',  ( -12.46153846153846168, -10.05456864172156806, 36.03766855953608683 ) ) ;
#21242=CARTESIAN_POINT ( 'NONE',  ( 7.846153846153846700, -1.629998284177014645, 34.34916445242399163 ) ) ;
#21243=EDGE_CURVE ( 'NONE', #41980, #71008, #44914, .T. ) ;
#21244=EDGE_LOOP ( 'NONE', ( #48814, #31911 ) ) ;
#21245=FACE_BOUND ( 'NONE', #75952, .T. ) ;
#21246=VERTEX_POINT ( 'NONE', #17253 ) ;
#21247=LINE ( 'NONE', #60908, #1196 ) ;
#21248=EDGE_CURVE ( 'NONE', #4672, #50472, #80349, .T. ) ;
#21249=VECTOR ( 'NONE', #40251, 1000.000000000000227 ) ;
#21250=CARTESIAN_POINT ( 'NONE',  ( -14.30769230769242917, -11.67786785259630911, 32.92929555188603530 ) ) ;
#21251=EDGE_CURVE ( 'NONE', #76288, #67886, #28821, .T. ) ;
#21252=CARTESIAN_POINT ( 'NONE',  ( 3.100078627658922947, -11.37499894934982514, 33.29245874905763003 ) ) ;
#21253=CARTESIAN_POINT ( 'NONE',  ( -11.53846153846153655, -2.538708090699994813, 30.37095296980875503 ) ) ;
#21254=ORIENTED_EDGE ( 'NONE', *, *, #29759, .T. ) ;
#21255=AXIS2_PLACEMENT_3D ( 'NONE', #88260, #12138, #26536 ) ;
#21256=ORIENTED_EDGE ( 'NONE', *, *, #52473, .T. ) ;
#21257=EDGE_CURVE ( 'NONE', #27164, #68374, #17009, .T. ) ;
#21258=ORIENTED_EDGE ( 'NONE', *, *, #6336, .T. ) ;
#21259=CARTESIAN_POINT ( 'NONE',  ( -3.164701897419154530, -11.35647404775217595, 33.31231777344667222 ) ) ;
#21260=ORIENTED_EDGE ( 'NONE', *, *, #73728, .T. ) ;
#21261=AXIS2_PLACEMENT_3D ( 'NONE', #86513, #5859, #26572 ) ;
#21262=CARTESIAN_POINT ( 'NONE',  ( -5.999999999999998224, -12.37446782046654192, 30.86335684631486131 ) ) ;
#21263=ADVANCED_FACE ( 'NONE', ( #80305 ), #17713, .F. ) ;
#21264=CARTESIAN_POINT ( 'NONE',  ( -9.758064494821999446, -7.249945686854186278, 34.74374336980224598 ) ) ;
#21265=DIRECTION ( 'NONE',  ( -0.000000000000000000, -0.9396926207859093161, -0.3420201433256663259 ) ) ;
#21266=CARTESIAN_POINT ( 'NONE',  ( 13.31853197365950514, -10.51840700105979387, 33.73612834413961536 ) ) ;
#21268=CARTESIAN_POINT ( 'NONE',  ( 14.53070365930516239, -6.503523203565941380, 34.64991518177335195 ) ) ;
#21271=B_SPLINE_CURVE_WITH_KNOTS ( 'NONE', 3,
 ( #34350, #68148, #6450, #74025, #33034, #67264, #61370, #54615, #75351, #60500 ),
 .UNSPECIFIED., .F., .F.,
 ( 4, 2, 2, 2, 4 ),
 ( 0.0007817246256747460882, 0.0009771112852218900684, 0.001172497944769034049, 0.001367884604316177812, 0.001563271263863321792 ),
 .UNSPECIFIED. ) ;
#21272=ORIENTED_EDGE ( 'NONE', *, *, #47833, .F. ) ;
#21273=B_SPLINE_CURVE_WITH_KNOTS ( 'NONE', 3,
 ( #76445, #68355, #34123, #20608, #14749, #2105 ),
 .UNSPECIFIED., .F., .F.,
 ( 4, 2, 4 ),
 ( 0.000000000000000000, 0.0001954784845028888327, 0.0003909569690057776653 ),
 .UNSPECIFIED. ) ;
#21274=EDGE_LOOP ( 'NONE', ( #71575, #45446, #12613, #48734 ) ) ;
#21275=CARTESIAN_POINT ( 'NONE',  ( 3.480769230769168665, -7.565270000091922853, 34.99999999999999289 ) ) ;
#21276=DIRECTION ( 'NONE',  ( 0.000000000000000000, 0.000000000000000000, 1.000000000000000000 ) ) ;
#21277=CARTESIAN_POINT ( 'NONE',  ( -13.38461538461538325, -5.557115091759785130, 34.35708131394839171 ) ) ;
#21278=DIRECTION ( 'NONE',  ( 0.000000000000000000, 0.3420201433256641055, -0.9396926207859100932 ) ) ;
#21279=AXIS2_PLACEMENT_3D ( 'NONE', #47337, #39274, #5029 ) ;
#21281=CYLINDRICAL_SURFACE ( 'NONE', #11301, 5.250000000000000888 ) ;
#21282=CARTESIAN_POINT ( 'NONE',  ( 16.37685750545900021, -3.105924265160262099, 32.13625925475356127 ) ) ;
#21283=ORIENTED_EDGE ( 'NONE', *, *, #54470, .F. ) ;
#21285=CARTESIAN_POINT ( 'NONE',  ( 9.469380733400843297, -11.98009711892699514, 32.48740034544076138 ) ) ;
#21286=CARTESIAN_POINT ( 'NONE',  ( -1.161835843346974650, -2.847695495035523106, 31.58253572463339154 ) ) ;
#21287=CARTESIAN_POINT ( 'NONE',  ( 3.230769230769108269, -11.67786785259630911, 32.92929555188603530 ) ) ;
#21288=EDGE_LOOP ( 'NONE', ( #61942, #16583, #76401, #44036 ) ) ;
#21289=CARTESIAN_POINT ( 'NONE',  ( 18.13079180782478872, -12.38066358083363738, 30.83685684665853444 ) ) ;
#21290=VECTOR ( 'NONE', #2770, 1000.000000000000000 ) ;
#21292=EDGE_LOOP ( 'NONE', ( #60583, #1481 ) ) ;
#21293=FACE_BOUND ( 'NONE', #75122, .T. ) ;
#21295=ADVANCED_FACE ( 'NONE', ( #87521 ), #46507, .F. ) ;
#21297=FACE_OUTER_BOUND ( 'NONE', #55489, .T. ) ;
#21299=CARTESIAN_POINT ( 'NONE',  ( 0.2380535178145125053, -10.81261337010820256, 33.49550067578627477 ) ) ;
#21300=CARTESIAN_POINT ( 'NONE',  ( 4.854096384444071433, -7.369208160676172348, 34.74850200257122879 ) ) ;
#21301=CARTESIAN_POINT ( 'NONE',  ( -16.28399336328437386, -12.45813303252208648, 30.39737893381572675 ) ) ;
#21302=CARTESIAN_POINT ( 'NONE',  ( -4.853910232829682592, -5.582272713120727481, 34.63742843783360570 ) ) ;
#21303=ORIENTED_EDGE ( 'NONE', *, *, #80623, .F. ) ;
#21304=ADVANCED_FACE ( 'NONE', ( #72643 ), #59126, .F. ) ;
#21305=CARTESIAN_POINT ( 'NONE',  ( -4.826868657009623753, -4.818054556918156095, 34.26375889529406749 ) ) ;
#21306=ORIENTED_EDGE ( 'NONE', *, *, #17696, .T. ) ;
#21307=CARTESIAN_POINT ( 'NONE',  ( -9.692307692307812417, -12.46129190930018460, 30.37095296980731973 ) ) ;
#21309=CARTESIAN_POINT ( 'NONE',  ( 7.846153846153846700, -10.51840700105979565, 33.73612834413961536 ) ) ;
#21310=CARTESIAN_POINT ( 'NONE',  ( 12.46153846153846168, -2.499999999999998668, 29.50000000000001066 ) ) ;
#21311=CARTESIAN_POINT ( 'NONE',  ( 7.596130621932389637, -10.18141759479407327, 34.26406193332782379 ) ) ;
#21312=DIRECTION ( 'NONE',  ( -0.000000000000000000, -0.1736481776669307198, -0.9848077530122080203 ) ) ;
#21313=CARTESIAN_POINT ( 'NONE',  ( -13.38461538461538325, -3.322132147404559976, 32.92929555188717927 ) ) ;
#21314=CARTESIAN_POINT ( 'NONE',  ( 13.60739492588379385, -5.913360116392397892, 34.49180327182771322 ) ) ;
#21315=CARTESIAN_POINT ( 'NONE',  ( -17.01085472592063752, -8.120952969808772792, 34.71129190929999453 ) ) ;
#21317=CARTESIAN_POINT ( 'NONE',  ( 8.096099364501986528, -4.336752205174647656, 33.62275283266504289 ) ) ;
#21318=B_SPLINE_CURVE_WITH_KNOTS ( 'NONE', 3,
 ( #13610, #76188, #88850, #68119, #88407, #39763, #47835, #60461, #67233, #19478 ),
 .UNSPECIFIED., .F., .F.,
 ( 4, 2, 2, 2, 4 ),
 ( 0.000000000000000000, 0.0001954311564186869286, 0.0003908623128373738573, 0.0005862934692560607588, 0.0007817246256747477145 ),
 .UNSPECIFIED. ) ;
#21321=B_SPLINE_CURVE_WITH_KNOTS ( 'NONE', 3,
 ( #80312, #40656, #40215, #46069, #19483, #12732, #18609, #39772, #13176, #19046 ),
 .UNSPECIFIED., .F., .F.,
 ( 4, 2, 2, 2, 4 ),
 ( 0.0007817246256747442451, 0.0009771112852218865989, 0.001172497944769029061, 0.001367884604316171523, 0.001563271263863313986 ),
 .UNSPECIFIED. ) ;
#21322=CYLINDRICAL_SURFACE ( 'NONE', #87998, 0.2500000000000004996 ) ;
#21324=B_SPLINE_CURVE_WITH_KNOTS ( 'NONE', 3,
 ( #77373, #15683, #28296, #76938, #1718, #29207, #56659, #41380, #82817, #20657 ),
 .UNSPECIFIED., .F., .F.,
 ( 4, 2, 2, 2, 4 ),
 ( 0.0007817359430256388964, 0.0009771253907250073822, 0.001172514838424375868, 0.001367904286123744571, 0.001563293733823113056 ),
 .UNSPECIFIED. ) ;
#21325=VECTOR ( 'NONE', #75916, 1000.000000000000000 ) ;
#21326=ORIENTED_EDGE ( 'NONE', *, *, #80030, .F. ) ;
#21327=CARTESIAN_POINT ( 'NONE',  ( 3.100077764101672795, -4.809359713505814149, 33.96456829005828837 ) ) ;
#21328=ORIENTED_EDGE ( 'NONE', *, *, #21670, .T. ) ;
#21329=CARTESIAN_POINT ( 'NONE',  ( 14.24160889673642849, -8.120952969808774569, 34.71129190930000163 ) ) ;
#21330=B_SPLINE_CURVE_WITH_KNOTS ( 'NONE', 3,
 ( #70214, #41416, #36431, #27899, #48159, #8075, #27460, #62991, #56256, #82414 ),
 .UNSPECIFIED., .F., .F.,
 ( 4, 2, 2, 2, 4 ),
 ( 0.0007817246256747503166, 0.0009771112852218946220, 0.001172497944769039036, 0.001367884604316183233, 0.001563271263863327647 ),
 .UNSPECIFIED. ) ;
#21331=EDGE_CURVE ( 'NONE', #14831, #3309, #52405, .T. ) ;
#21332=CARTESIAN_POINT ( 'NONE',  ( -8.096177070375304652, -8.475808217655753651, 34.90892951860618609 ) ) ;
#21333=CARTESIAN_POINT ( 'NONE',  ( -14.30769230769230660, -11.35647404775217417, 33.31231777344666511 ) ) ;
#21334=CARTESIAN_POINT ( 'NONE',  ( 1.134592160393927296, -2.588893531581426544, 31.60682220781847818 ) ) ;
#21335=CARTESIAN_POINT ( 'NONE',  ( 6.066068351002442682, -2.538708090699994813, 30.37095296980875503 ) ) ;
#21336=CARTESIAN_POINT ( 'NONE',  ( -16.28453762051371712, -3.062553014421049991, 32.05460306192773601 ) ) ;
#21337=EDGE_CURVE ( 'NONE', #23467, #47762, #13170, .T. ) ;
#21338=CARTESIAN_POINT ( 'NONE',  ( 10.61538461538449418, -3.643525952248795718, 33.31231777344771672 ) ) ;
#21342=CARTESIAN_POINT ( 'NONE',  ( -9.692307692307691624, -1.466349020453238561, 30.81389545987213907 ) ) ;
#21343=CARTESIAN_POINT ( 'NONE',  ( 11.47319109250076430, -10.90142922261923886, 33.41473453929638993 ) ) ;
#21344=AXIS2_PLACEMENT_3D ( 'NONE', #13105, #40584, #68053 ) ;
#21345=LINE ( 'NONE', #34413, #11969 ) ;
#21346=CARTESIAN_POINT ( 'NONE',  ( -9.692307692307691624, -11.35647404775217417, 33.31231777344666511 ) ) ;
#21347=EDGE_CURVE ( 'NONE', #51804, #44547, #47386, .T. ) ;
#21349=ORIENTED_EDGE ( 'NONE', *, *, #2096, .F. ) ;
#21350=CARTESIAN_POINT ( 'NONE',  ( -17.75000000000001066, -12.50000000000000000, 29.81609845454690699 ) ) ;
#21351=CARTESIAN_POINT ( 'NONE',  ( 1.515405825582337718, -3.338503747796865984, 32.95102852606552801 ) ) ;
#21352=DIRECTION ( 'NONE',  ( 0.000000000000000000, -6.938893903907222067E-15, 1.000000000000000000 ) ) ;
#21353=CARTESIAN_POINT ( 'NONE',  ( 0.2386115026316106003, -10.01117774369187252, 34.36070679894347535 ) ) ;
#21354=CARTESIAN_POINT ( 'NONE',  ( -13.38461538461538325, -8.318370150425687726, 35.83090037661290239 ) ) ;
#21355=CARTESIAN_POINT ( 'NONE',  ( 11.60371667797437567, -4.320704448112861584, 33.92786785259548310 ) ) ;
#21357=B_SPLINE_CURVE_WITH_KNOTS ( 'NONE', 3,
 ( #4595, #52772, #31165, #72154, #79818, #58638, #25310, #43799, #80262, #64494 ),
 .UNSPECIFIED., .F., .F.,
 ( 4, 2, 2, 2, 4 ),
 ( 0.0007817246256747434861, 0.0009771112852218861652, 0.001172497944769028844, 0.001367884604316171523, 0.001563271263863314203 ),
 .UNSPECIFIED. ) ;
#21359=CARTESIAN_POINT ( 'NONE',  ( -13.63463862190834952, -10.05641848906368097, 34.04755513067966177 ) ) ;
#21360=EDGE_LOOP ( 'NONE', ( #38657, #67689, #32720, #88982 ) ) ;
#21361=B_SPLINE_CURVE_WITH_KNOTS ( 'NONE', 3,
 ( #61512, #53424, #54759, #89018, #7018, #80927, #28173, #43026, #48437, #63289 ),
 .UNSPECIFIED., .F., .F.,
 ( 4, 2, 2, 2, 4 ),
 ( 0.0007817359430256364027, 0.0009771253907250043464, 0.001172514838424372399, 0.001367904286123740234, 0.001563293733823108286 ),
 .UNSPECIFIED. ) ;
#21362=AXIS2_PLACEMENT_3D ( 'NONE', #25622, #81026, #6678 ) ;
#21364=CARTESIAN_POINT ( 'NONE',  ( -18.00000000000000000, -8.120952969808772792, 34.71129190930000163 ) ) ;
#21365=CARTESIAN_POINT ( 'NONE',  ( -6.923076923076922462, -12.34228464037088635, 31.77849191805839268 ) ) ;
#21366=LINE ( 'NONE', #74995, #29261 ) ;
#21367=B_SPLINE_CURVE_WITH_KNOTS ( 'NONE', 3,
 ( #24644, #66064, #52992, #80492, #18786, #12035, #39511, #5709, #67855, #81382 ),
 .UNSPECIFIED., .F., .F.,
 ( 4, 2, 2, 2, 4 ),
 ( 0.000000000000000000, 0.0001954311564186861426, 0.0003908623128373722852, 0.0005862934692560583735, 0.0007817246256747445703 ),
 .UNSPECIFIED. ) ;
#21368=CARTESIAN_POINT ( 'NONE',  ( -14.30769230769230660, -13.87047571288749737, 32.06866353760679544 ) ) ;
#21369=EDGE_LOOP ( 'NONE', ( #83897, #73567 ) ) ;
#21370=EDGE_CURVE ( 'NONE', #60953, #27674, #21318, .T. ) ;
#21373=VERTEX_POINT ( 'NONE', #5531 ) ;
#21374=DIRECTION ( 'NONE',  ( 0.000000000000000000, 0.7660444431189822323, -0.6427876096865344779 ) ) ;
#21375=CARTESIAN_POINT ( 'NONE',  ( 4.826946345980720920, -10.66389620160130036, 33.62221079203477103 ) ) ;
#21376=ADVANCED_FACE ( 'NONE', ( #87980 ), #81633, .F. ) ;
#21377=CARTESIAN_POINT ( 'NONE',  ( -3.453695448285378333, -9.886141570436013382, 34.14413921362392301 ) ) ;
#21379=AXIS2_PLACEMENT_3D ( 'NONE', #24535, #38508, #87602 ) ;
#21380=CARTESIAN_POINT ( 'NONE',  ( 8.069116980420522722, -7.369474539155828730, 34.99858011523957657 ) ) ;
#21381=FACE_OUTER_BOUND ( 'NONE', #42989, .T. ) ;
#21382=ORIENTED_EDGE ( 'NONE', *, *, #51533, .T. ) ;
#21383=EDGE_LOOP ( 'NONE', ( #73327, #85358 ) ) ;
#21384=B_SPLINE_CURVE_WITH_KNOTS ( 'NONE', 3,
 ( #28368, #22062, #77009, #22938, #50399, #77881, #16185, #42785, #70244, #465 ),
 .UNSPECIFIED., .F., .F.,
 ( 4, 2, 2, 2, 4 ),
 ( 0.0007817246256747525934, 0.0009771112852218970073, 0.001172497944769041204, 0.001367884604316185401, 0.001563271263863329815 ),
 .UNSPECIFIED. ) ;
#21387=EDGE_CURVE ( 'NONE', #28560, #84690, #53537, .T. ) ;
#21388=CARTESIAN_POINT ( 'NONE',  ( -2.980714919130914797, -10.66356715214248396, 33.62249196103329751 ) ) ;
#21389=ORIENTED_EDGE ( 'NONE', *, *, #49109, .F. ) ;
#21390=B_SPLINE_CURVE_WITH_KNOTS ( 'NONE', 3,
 ( #65584, #84557, #68594, #47425, #12762, #20847, #48316, #75790, #6018, #7347 ),
 .UNSPECIFIED., .F., .F.,
 ( 4, 2, 2, 2, 4 ),
 ( 0.000000000000000000, 0.0001954311564186860613, 0.0003908623128373721225, 0.0005862934692560581567, 0.0007817246256747442451 ),
 .UNSPECIFIED. ) ;
#21391=LINE ( 'NONE', #18845, #11548 ) ;
#21392=CARTESIAN_POINT ( 'NONE',  ( -10.36543920600657209, -6.653508905675592722, 34.93172785388651391 ) ) ;
#21393=CARTESIAN_POINT ( 'NONE',  ( 6.673076923076925127, -7.433931650972300353, 34.75000000000000711 ) ) ;
#21395=ORIENTED_EDGE ( 'NONE', *, *, #3536, .T. ) ;
#21396=AXIS2_PLACEMENT_3D ( 'NONE', #58949, #79678, #67057 ) ;
#21397=ORIENTED_EDGE ( 'NONE', *, *, #40247, .T. ) ;
#21398=CARTESIAN_POINT ( 'NONE',  ( -2.530618525208453207, -12.39988816332205701, 30.74660775122750778 ) ) ;
#21399=ADVANCED_FACE ( 'NONE', ( #55041 ), #20806, .F. ) ;
#21401=FACE_BOUND ( 'NONE', #37106, .T. ) ;
#21402=CARTESIAN_POINT ( 'NONE',  ( -1.161239443917200242, -2.501478030877322567, 29.88021232661720816 ) ) ;
#21403=CARTESIAN_POINT ( 'NONE',  ( 7.911408985666682270, -5.941354392334607049, 34.76329471203374055 ) ) ;
#21404=ORIENTED_EDGE ( 'NONE', *, *, #50367, .F. ) ;
#21407=CARTESIAN_POINT ( 'NONE',  ( -15.93083330975275658, -12.64618726649961289, 30.78989965857442712 ) ) ;
#21409=CARTESIAN_POINT ( 'NONE',  ( 3.903869422903799347, -11.28823185664190376, 33.01397839955799896 ) ) ;
#21410=CARTESIAN_POINT ( 'NONE',  ( 15.23076923076923173, -1.367168528481310208, 33.57946703557072254 ) ) ;
#21411=ORIENTED_EDGE ( 'NONE', *, *, #56441, .T. ) ;
#21412=CARTESIAN_POINT ( 'NONE',  ( 6.130791807824788719, -8.147973898785416225, 34.70805048591653730 ) ) ;
#21413=PLANE ( 'NONE',  #26773 ) ;
#21414=CARTESIAN_POINT ( 'NONE',  ( 16.37685750545900376, -9.086983370893049639, 34.49168942202179267 ) ) ;
#21415=CARTESIAN_POINT ( 'NONE',  ( -0.6844654204453110014, -4.762599654559228846, 34.23009711892697737 ) ) ;
#21416=CARTESIAN_POINT ( 'NONE',  ( -0.2381114996768911307, -7.630147231320743018, 34.74852402298682819 ) ) ;
#21417=FACE_BOUND ( 'NONE', #6729, .T. ) ;
#21418=B_SPLINE_CURVE_WITH_KNOTS ( 'NONE', 3,
 ( #37080, #16816, #73102, #4644, #65449, #30771, #86636, #17719, #31672, #84855 ),
 .UNSPECIFIED., .F., .F.,
 ( 4, 2, 2, 2, 4 ),
 ( 0.0007817359430256333669, 0.0009771253907250056474, 0.001172514838424370881, 0.001367904286123736331, 0.001563293733823101564 ),
 .UNSPECIFIED. ) ;
#21419=CARTESIAN_POINT ( 'NONE',  ( 17.20771488474786537, -3.530189275343204702, 32.79018710029569661 ) ) ;
#21420=LINE ( 'NONE', #48888, #57502 ) ;
#21421=EDGE_CURVE ( 'NONE', #49108, #85857, #84651, .T. ) ;
#21422=CARTESIAN_POINT ( 'NONE',  ( 11.53846153846153832, -11.91647553114624181, 32.58852847137148245 ) ) ;
#21424=CARTESIAN_POINT ( 'NONE',  ( -6.249976730942354841, -4.943428324936578910, 34.04746400365624481 ) ) ;
#21425=CARTESIAN_POINT ( 'NONE',  ( -5.299850035829924089, -12.38737895849757820, 31.66785238281580206 ) ) ;
#21427=ORIENTED_EDGE ( 'NONE', *, *, #77554, .F. ) ;
#21428=CARTESIAN_POINT ( 'NONE',  ( -5.749945580086545327, -10.82426656108011720, 33.81400080652039009 ) ) ;
#21429=ORIENTED_EDGE ( 'NONE', *, *, #27051, .T. ) ;
#21430=CARTESIAN_POINT ( 'NONE',  ( -13.38461538461550759, -11.06231777344772027, 33.60647404775119895 ) ) ;
#21432=DIRECTION ( 'NONE',  ( -0.000000000000000000, 0.1736481776669307198, -0.9848077530122080203 ) ) ;
#21433=CARTESIAN_POINT ( 'NONE',  ( 14.08420738312797837, -4.225889041578353655, 33.85425143139329407 ) ) ;
#21435=DIRECTION ( 'NONE',  ( 0.000000000000000000, 0.8660254037844377084, 0.5000000000000015543 ) ) ;
#21438=CARTESIAN_POINT ( 'NONE',  ( -10.48459417441766561, -12.62708834333097663, 30.88030960425257021 ) ) ;
#21439=CARTESIAN_POINT ( 'NONE',  ( -5.076923076923075762, -4.786620604624113540, 33.94971097300155094 ) ) ;
#21440=CARTESIAN_POINT ( 'NONE',  ( -5.076923076923075762, -12.37446782046654192, 30.86335684631486131 ) ) ;
#21441=CARTESIAN_POINT ( 'NONE',  ( 4.153846153846154188, -11.69971097300155272, 32.46337939537588113 ) ) ;
#21442=CARTESIAN_POINT ( 'NONE',  ( -16.15384615384615330, -12.29105614889573062, 35.45975837776705220 ) ) ;
#21445=EDGE_CURVE ( 'NONE', #39535, #56699, #11594, .T. ) ;
#21446=EDGE_CURVE ( 'NONE', #27135, #71888, #76644, .T. ) ;
#21447=CARTESIAN_POINT ( 'NONE',  ( -10.48459280755982981, -2.729792928343269587, 31.24908615093345077 ) ) ;
#21449=EDGE_LOOP ( 'NONE', ( #66608, #9003, #88284, #27893 ) ) ;
#21450=DIRECTION ( 'NONE',  ( -0.000000000000000000, 0.6427876096865404731, -0.7660444431189771253 ) ) ;
#21452=AXIS2_PLACEMENT_3D ( 'NONE', #59216, #18243, #76274 ) ;
#21453=CARTESIAN_POINT ( 'NONE',  ( 7.846153846153846700, -5.471508081941601098, 34.59228464037088457 ) ) ;
#21454=CARTESIAN_POINT ( 'NONE',  ( -9.442253380669377805, -11.28795663066794575, 33.01431243580653785 ) ) ;
#21455=ORIENTED_EDGE ( 'NONE', *, *, #56918, .F. ) ;
#21456=CARTESIAN_POINT ( 'NONE',  ( 1.515140822849031066, -8.630441415882550871, 34.87705825610312615 ) ) ;
#21457=CARTESIAN_POINT ( 'NONE',  ( 2.980792499826876440, -3.627789207965226748, 32.91389620160131102 ) ) ;
#21458=CARTESIAN_POINT ( 'NONE',  ( 4.153846153846030731, -9.528491918059723176, 34.59228464037033035 ) ) ;
#21460=CARTESIAN_POINT ( 'NONE',  ( -7.781008066821878622, -7.750023238201979581, 34.74374492549440419 ) ) ;
#21461=CARTESIAN_POINT ( 'NONE',  ( -3.007989689500821573, -5.114059244376869984, 34.14424750095245287 ) ) ;
#21462=DIRECTION ( 'NONE',  ( -0.000000000000000000, 1.000000000000000000, 3.491481338843133355E-15 ) ) ;
#21463=VECTOR ( 'NONE', #5169, 1000.000000000000227 ) ;
#21464=CARTESIAN_POINT ( 'NONE',  ( -8.769230769230768274, -9.058645607665452459, 34.76329471203371924 ) ) ;
#21465=CARTESIAN_POINT ( 'NONE',  ( -10.36533030374629760, -10.66356715214248396, 33.62249196103329751 ) ) ;
#21466=VERTEX_POINT ( 'NONE', #28915 ) ;
#21467=DIRECTION ( 'NONE',  ( 0.000000000000000000, 0.8660254037844377084, 0.5000000000000015543 ) ) ;
#21468=ORIENTED_EDGE ( 'NONE', *, *, #15351, .F. ) ;
#21469=ORIENTED_EDGE ( 'NONE', *, *, #69339, .T. ) ;
#21470=CARTESIAN_POINT ( 'NONE',  ( -9.692307692307691624, -3.050289026998446396, 32.03036669348365706 ) ) ;
#21472=LINE ( 'NONE', #76422, #12042 ) ;
#21474=ORIENTED_EDGE ( 'NONE', *, *, #10578, .F. ) ;
#21476=ORIENTED_EDGE ( 'NONE', *, *, #21906, .F. ) ;
#21477=ORIENTED_EDGE ( 'NONE', *, *, #13889, .F. ) ;
#21479=CARTESIAN_POINT ( 'NONE',  ( -15.36146069743679199, -12.11776431015576172, 31.66791131148498906 ) ) ;
#21480=ORIENTED_EDGE ( 'NONE', *, *, #12951, .T. ) ;
#21481=CARTESIAN_POINT ( 'NONE',  ( 4.376625695114562120, -5.913360116392398780, 34.49180327182771322 ) ) ;
#21482=CARTESIAN_POINT ( 'NONE',  ( 6.222779668978065004, -2.612705202774697533, 31.66806509827799943 ) ) ;
#21483=CARTESIAN_POINT ( 'NONE',  ( -2.980714919130915685, -4.235687564193446164, 33.53795663066793509 ) ) ;
#21484=DIRECTION ( 'NONE',  ( 0.000000000000000000, 0.9848077530122072432, 0.1736481776669354937 ) ) ;
#21485=EDGE_LOOP ( 'NONE', ( #70010, #42937, #14037, #69722 ) ) ;
#21486=VERTEX_POINT ( 'NONE', #21690 ) ;
#21487=VERTEX_POINT ( 'NONE', #63996 ) ;
#21488=CARTESIAN_POINT ( 'NONE',  ( -14.05769230769087130, -7.500000000000155431, 34.75000000000007105 ) ) ;
#21489=CARTESIAN_POINT ( 'NONE',  ( -14.05774689831426372, -2.341251567377310217, 30.72681386836322659 ) ) ;
#21490=ORIENTED_EDGE ( 'NONE', *, *, #13554, .F. ) ;
#21491=CARTESIAN_POINT ( 'NONE',  ( 9.692307692307572609, -11.94971097300221174, 32.03036669348237098 ) ) ;
#21492=CARTESIAN_POINT ( 'NONE',  ( -0.5922290646487691212, -6.369640206132550553, 34.87707690430378449 ) ) ;
#21493=VERTEX_POINT ( 'NONE', #77967 ) ;
#21494=CARTESIAN_POINT ( 'NONE',  ( 15.16468581981335007, -10.51840700105979387, 33.73612834413961536 ) ) ;
#21495=DIRECTION ( 'NONE',  ( 0.000000000000000000, 0.7660444431189822323, -0.6427876096865344779 ) ) ;
#21496=EDGE_LOOP ( 'NONE', ( #6021, #17292, #1458, #28541 ) ) ;
#21497=FACE_BOUND ( 'NONE', #23784, .T. ) ;
#21498=CARTESIAN_POINT ( 'NONE',  ( 15.23076923076923173, -11.35647404775217417, 33.31231777344666511 ) ) ;
#21499=CARTESIAN_POINT ( 'NONE',  ( 13.60739505359345181, -6.717445702608402236, 34.94155399931962336 ) ) ;
#21501=DIRECTION ( 'NONE',  ( -0.000000000000000000, 0.3420201433256694901, -0.9396926207859082059 ) ) ;
#21502=CARTESIAN_POINT ( 'NONE',  ( 18.00000000000000000, -2.833524468853757305, 32.15551576947925838 ) ) ;
#21504=CARTESIAN_POINT ( 'NONE',  ( -0.7115616988314271696, -12.22074536777954989, 31.39888409691088356 ) ) ;
#21505=AXIS2_PLACEMENT_3D ( 'NONE', #57476, #22367, #65111 ) ;
#21506=CARTESIAN_POINT ( 'NONE',  ( -2.980714810855777497, -3.435999193479609470, 33.07426656108011542 ) ) ;
#21507=CARTESIAN_POINT ( 'NONE',  ( 14.43821774592595197, -2.372941743896879174, 30.88044141588253666 ) ) ;
#21508=ORIENTED_EDGE ( 'NONE', *, *, #49160, .F. ) ;
#21509=CARTESIAN_POINT ( 'NONE',  ( -8.096130590202436750, -6.524016743844655686, 34.90889640711025521 ) ) ;
#21510=CARTESIAN_POINT ( 'NONE',  ( -8.069019268357486396, -2.501496062324912284, 29.88072118266895671 ) ) ;
#21511=AXIS2_PLACEMENT_3D ( 'NONE', #1371, #13999, #70277 ) ;
#21512=ORIENTED_EDGE ( 'NONE', *, *, #11959, .F. ) ;
#21513=VECTOR ( 'NONE', #1332, 1000.000000000000000 ) ;
#21515=CARTESIAN_POINT ( 'NONE',  ( 8.769230769230647482, -3.300289026999228881, 32.46337939537708905 ) ) ;
#21516=LINE ( 'NONE', #62930, #39008 ) ;
#21517=ORIENTED_EDGE ( 'NONE', *, *, #55578, .F. ) ;
#21518=CARTESIAN_POINT ( 'NONE',  ( -9.822455662039388358, -9.504002272028875709, 34.60269587691767867 ) ) ;
#21519=CARTESIAN_POINT ( 'NONE',  ( 12.46153846153846168, -1.790695186598648903, 34.54067556320373455 ) ) ;
#21520=FACE_BOUND ( 'NONE', #41665, .T. ) ;
#21521=DIRECTION ( 'NONE',  ( 0.000000000000000000, 0.7660444431189822323, -0.6427876096865344779 ) ) ;
#21522=CARTESIAN_POINT ( 'NONE',  ( -16.94613126909828793, -12.38066358083363738, 30.83685684665853444 ) ) ;
#21523=B_SPLINE_CURVE_WITH_KNOTS ( 'NONE', 3,
 ( #14321, #27838, #76018, #41807, #7572, #15218, #23720, #70149, #43997, #49872 ),
 .UNSPECIFIED., .F., .F.,
 ( 4, 2, 2, 2, 4 ),
 ( 0.000000000000000000, 0.0001954339857564074202, 0.0003908679715128148403, 0.0005863019572692222334, 0.0007817359430256296806 ),
 .UNSPECIFIED. ) ;
#21524=CYLINDRICAL_SURFACE ( 'NONE', #38781, 0.2500000000000009437 ) ;
#21525=ADVANCED_FACE ( 'NONE', ( #55915 ), #30229, .F. ) ;
#21527=CARTESIAN_POINT ( 'NONE',  ( -4.854143407945009869, -10.23759521482555357, 34.22997729860117033 ) ) ;
#21528=CARTESIAN_POINT ( 'NONE',  ( 6.923076923076802558, -12.46129190930018460, 30.37095296980731973 ) ) ;
#21529=B_SPLINE_CURVE_WITH_KNOTS ( 'NONE', 3,
 ( #2137, #30062, #85012, #70157, #8022, #29193 ),
 .UNSPECIFIED., .F., .F.,
 ( 4, 2, 4 ),
 ( 0.000000000000000000, 0.0001954784845028912450, 0.0003909569690057824900 ),
 .UNSPECIFIED. ) ;
#21530=LINE ( 'NONE', #20642, #77835 ) ;
#21532=ORIENTED_EDGE ( 'NONE', *, *, #65614, .T. ) ;
#21534=CARTESIAN_POINT ( 'NONE',  ( -1.384615384615506484, -3.643525952248795718, 33.31231777344771672 ) ) ;
#21535=CARTESIAN_POINT ( 'NONE',  ( 14.43848274865925774, -12.62708834333097663, 30.88030960425257021 ) ) ;
#21536=CYLINDRICAL_SURFACE ( 'NONE', #7119, 0.2500000000000008882 ) ;
#21537=CARTESIAN_POINT ( 'NONE',  ( -1.607541602131531855, -3.105860786376062332, 32.13614157043599562 ) ) ;
#21538=CARTESIAN_POINT ( 'NONE',  ( -16.85414353565466072, -6.760870238392814535, 34.69528174975672385 ) ) ;
#21540=CARTESIAN_POINT ( 'NONE',  ( 4.376809057407638370, -7.369474270740069777, 34.74850911626239736 ) ) ;
#21541=CARTESIAN_POINT ( 'NONE',  ( 18.22301135161284336, -3.105924265160262099, 32.13625925475356127 ) ) ;
#21542=CARTESIAN_POINT ( 'NONE',  ( 5.999999999999878320, -4.320704448113951379, 33.92786785259630022 ) ) ;
#21543=FACE_OUTER_BOUND ( 'NONE', #38839, .T. ) ;
#21545=CARTESIAN_POINT ( 'NONE',  ( 16.37662569511456567, -5.114059244376869096, 34.14424750095245287 ) ) ;
#21546=DIRECTION ( 'NONE',  ( -0.000000000000000000, -0.5000000000000009992, -0.8660254037844380415 ) ) ;
#21547=ADVANCED_FACE ( 'NONE', ( #8188 ), #49610, .F. ) ;
#21549=CARTESIAN_POINT ( 'NONE',  ( -14.17690049986752143, -3.062576670634119758, 32.05464942895959979 ) ) ;
#21550=DIRECTION ( 'NONE',  ( -0.000000000000000000, 0.9848077530122085754, -0.1736481776669273613 ) ) ;
#21551=ORIENTED_EDGE ( 'NONE', *, *, #34369, .F. ) ;
#21554=CARTESIAN_POINT ( 'NONE',  ( 7.596177102105254875, -4.818429247618089661, 34.26397095200675125 ) ) ;
#21557=CARTESIAN_POINT ( 'NONE',  ( -5.933932666649922361, -12.34228464037088813, 31.77849191805839268 ) ) ;
#21558=LINE ( 'NONE', #16131, #47634 ) ;
#21559=ORIENTED_EDGE ( 'NONE', *, *, #19172, .T. ) ;
#21560=CARTESIAN_POINT ( 'NONE',  ( -7.146003881983771677, -2.889293201056495786, 32.26117774369186009 ) ) ;
#21561=CARTESIAN_POINT ( 'NONE',  ( -18.00000000000000000, -13.60434399251292170, 33.56301978189820545 ) ) ;
#21563=FACE_OUTER_BOUND ( 'NONE', #25115, .T. ) ;
#21564=CARTESIAN_POINT ( 'NONE',  ( -2.373774687052440768, -10.67929555188718460, 33.92786785259543336 ) ) ;
#21565=ORIENTED_EDGE ( 'NONE', *, *, #13539, .T. ) ;
#21566=CARTESIAN_POINT ( 'NONE',  ( -12.46153846153846168, -4.945431358278436385, 36.03766855953609394 ) ) ;
#21567=CARTESIAN_POINT ( 'NONE',  ( 13.16168842570853492, -9.172386477786396597, 34.72672124145550043 ) ) ;
#21568=ORIENTED_EDGE ( 'NONE', *, *, #77856, .T. ) ;
#21569=CARTESIAN_POINT ( 'NONE',  ( -10.74553258511630993, -4.299443229763728169, 33.91186481527756058 ) ) ;
#21570=CARTESIAN_POINT ( 'NONE',  ( 8.638540166120458608, -6.369640206132551441, 34.87707690430378449 ) ) ;
#21571=VECTOR ( 'NONE', #5923, 1000.000000000000227 ) ;
#21572=CARTESIAN_POINT ( 'NONE',  ( 9.942362112221147186, -6.523592122091592671, 34.90882529074906415 ) ) ;
#21573=EDGE_LOOP ( 'NONE', ( #37545, #82611 ) ) ;
#21574=ORIENTED_EDGE ( 'NONE', *, *, #44436, .F. ) ;
#21575=CARTESIAN_POINT ( 'NONE',  ( 1.384615384615265343, -8.613356846316285953, 34.62446782046622218 ) ) ;
#21576=ORIENTED_EDGE ( 'NONE', *, *, #64688, .F. ) ;
#21577=CARTESIAN_POINT ( 'NONE',  ( 3.453782074862625340, -11.98016756924214832, 32.48728574198911190 ) ) ;
#21578=CARTESIAN_POINT ( 'NONE',  ( 12.46153846153833911, -9.442884908241554243, 34.35708131394783038 ) ) ;
#21579=CARTESIAN_POINT ( 'NONE',  ( -5.999999999999998224, -5.471508081941601098, 34.59228464037088457 ) ) ;
#21580=CARTESIAN_POINT ( 'NONE',  ( -6.923076923076922462, -11.35647404775217417, 33.31231777344666511 ) ) ;
#21581=CARTESIAN_POINT ( 'NONE',  ( -13.38461538461550582, -9.442884908241554243, 34.35708131394783038 ) ) ;
#21582=CARTESIAN_POINT ( 'NONE',  ( 0.3310632764627420288, -7.276987145209185215, 34.99546412871779921 ) ) ;
#21583=VECTOR ( 'NONE', #57993, 1000.000000000000000 ) ;
#21584=VECTOR ( 'NONE', #65573, 1000.000000000000114 ) ;
#21586=DIRECTION ( 'NONE',  ( -0.000000000000000000, 0.9848077530122086864, -0.1736481776669273891 ) ) ;
#21587=ORIENTED_EDGE ( 'NONE', *, *, #5456, .T. ) ;
#21588=ORIENTED_EDGE ( 'NONE', *, *, #44164, .T. ) ;
#21589=CARTESIAN_POINT ( 'NONE',  ( 5.076923076923075762, -11.35647404775217417, 33.31231777344666511 ) ) ;
#21592=VERTEX_POINT ( 'NONE', #70327 ) ;
#21593=DIRECTION ( 'NONE',  ( -0.000000000000000000, 0.6427876096865404731, -0.7660444431189771253 ) ) ;
#21594=CARTESIAN_POINT ( 'NONE',  ( -12.46153846153846168, -8.120952969808772792, 34.71129190930000163 ) ) ;
#21595=EDGE_LOOP ( 'NONE', ( #45629, #70501, #9068, #36082 ) ) ;
#21596=CARTESIAN_POINT ( 'NONE',  ( -12.39547011053602432, -5.557115091759786019, 34.35708131394839882 ) ) ;
#21597=EDGE_CURVE ( 'NONE', #65096, #38767, #27689, .T. ) ;
#21598=ORIENTED_EDGE ( 'NONE', *, *, #30958, .F. ) ;
#21599=CARTESIAN_POINT ( 'NONE',  ( 2.242421861731533017, -5.219633306516282545, 34.19971097300152252 ) ) ;
#21601=DIRECTION ( 'NONE',  ( -0.000000000000000000, -0.1736481776669307198, -0.9848077530122080203 ) ) ;
#21602=VERTEX_POINT ( 'NONE', #69440 ) ;
#21603=CARTESIAN_POINT ( 'NONE',  ( -6.792286482109974877, -4.684288915650984819, 34.18129842949671371 ) ) ;
#21604=AXIS2_PLACEMENT_3D ( 'NONE', #35395, #56113, #35850 ) ;
#21605=FACE_OUTER_BOUND ( 'NONE', #84525, .T. ) ;
#21606=FACE_BOUND ( 'NONE', #66861, .T. ) ;
#21607=CARTESIAN_POINT ( 'NONE',  ( -17.86995483716523125, -2.504778602574659008, 29.97347330155778167 ) ) ;
#21608=CARTESIAN_POINT ( 'NONE',  ( -17.93474442872397390, -12.27809138561124591, 31.22303859784719648 ) ) ;
#21609=ADVANCED_FACE ( 'NONE', ( #16267 ), #35207, .F. ) ;
#21610=CARTESIAN_POINT ( 'NONE',  ( 4.284371855609715674, -12.45806712695776319, 30.39783852428763922 ) ) ;
#21611=CYLINDRICAL_SURFACE ( 'NONE', #54674, 0.2500000000000012212 ) ;
#21612=CARTESIAN_POINT ( 'NONE',  ( -17.32694630114453105, -8.475808217655753651, 34.90892951860618609 ) ) ;
#21613=LINE ( 'NONE', #63921, #43308 ) ;
#21614=ORIENTED_EDGE ( 'NONE', *, *, #84475, .T. ) ;
#21615=DIRECTION ( 'NONE',  ( -0.000000000000000000, -0.9396926207859092051, -0.3420201433256662704 ) ) ;
#21617=ORIENTED_EDGE ( 'NONE', *, *, #80281, .F. ) ;
#21618=ORIENTED_EDGE ( 'NONE', *, *, #62647, .T. ) ;
#21619=CARTESIAN_POINT ( 'NONE',  ( 9.627057760533610065, -2.255955759149247619, 30.00000000000013856 ) ) ;
#21620=CARTESIAN_POINT ( 'NONE',  ( 7.911409417429869251, -10.21337939537593620, 33.94971097300152252 ) ) ;
#21621=CYLINDRICAL_SURFACE ( 'NONE', #32739, 0.2500000000000002220 ) ;
#21622=LINE ( 'NONE', #63493, #6315 ) ;
#21623=CARTESIAN_POINT ( 'NONE',  ( 1.515140822849028845, -11.04252011169590020, 33.62494198852677130 ) ) ;
#21624=DIRECTION ( 'NONE',  ( 0.000000000000000000, 0.6427876096865368094, 0.7660444431189802339 ) ) ;
#21625=VERTEX_POINT ( 'NONE', #14309 ) ;
#21626=CARTESIAN_POINT ( 'NONE',  ( 4.153846153846154188, -6.681629849574314051, 35.83090037661290239 ) ) ;
#21628=CARTESIAN_POINT ( 'NONE',  ( -10.48485891362105349, -10.19071101563364756, 33.96452234770658407 ) ) ;
#21629=AXIS2_PLACEMENT_3D ( 'NONE', #29171, #794, #68810 ) ;
#21630=EDGE_CURVE ( 'NONE', #28230, #41653, #49243, .T. ) ;
#21631=CARTESIAN_POINT ( 'NONE',  ( 3.007843013253082010, -3.105860786376062332, 32.13614157043598851 ) ) ;
#21632=DIRECTION ( 'NONE',  ( -0.000000000000000000, -0.9396926207859093161, -0.3420201433256663259 ) ) ;
#21633=ORIENTED_EDGE ( 'NONE', *, *, #87891, .T. ) ;
#21634=CARTESIAN_POINT ( 'NONE',  ( 3.164686851409094004, -11.91647553114624181, 32.58852847137148245 ) ) ;
#21635=ORIENTED_EDGE ( 'NONE', *, *, #17005, .F. ) ;
#21637=ORIENTED_EDGE ( 'NONE', *, *, #22169, .T. ) ;
#21638=ADVANCED_FACE ( 'NONE', ( #41796 ), #20620, .F. ) ;
#21639=CARTESIAN_POINT ( 'NONE',  ( -6.250023224221455287, -4.175268141568689195, 33.81360843649122216 ) ) ;
#21640=EDGE_LOOP ( 'NONE', ( #82862, #15466, #14173, #10395 ) ) ;
#21641=DIRECTION ( 'NONE',  ( -0.000000000000000000, 0.8660254037844397068, -0.4999999999999978906 ) ) ;
#21642=CARTESIAN_POINT ( 'NONE',  ( -12.33074665371367651, -6.413143153341454017, 34.63066358083362672 ) ) ;
#21643=DIRECTION ( 'NONE',  ( -0.000000000000000000, -0.9396926207859092051, -0.3420201433256662704 ) ) ;
#21644=CARTESIAN_POINT ( 'NONE',  ( -17.29985003582992320, -9.172386477786394821, 34.72672124145550043 ) ) ;
#21645=VECTOR ( 'NONE', #35507, 1000.000000000000000 ) ;
#21646=VECTOR ( 'NONE', #2887, 1000.000000000000000 ) ;
#21647=CARTESIAN_POINT ( 'NONE',  ( 12.33139125210024112, -10.19110544564092002, 33.96427741523702792 ) ) ;
#21648=ORIENTED_EDGE ( 'NONE', *, *, #42159, .F. ) ;
#21650=FACE_OUTER_BOUND ( 'NONE', #66667, .T. ) ;
#21651=CARTESIAN_POINT ( 'NONE',  ( -12.46153846153846168, -7.500000000000001776, 35.04278698407183867 ) ) ;
#21652=EDGE_LOOP ( 'NONE', ( #77607, #79082 ) ) ;
#21654=CARTESIAN_POINT ( 'NONE',  ( -8.834553684722942890, -7.749976743299138882, 34.99404534957040624 ) ) ;
#21655=CARTESIAN_POINT ( 'NONE',  ( 17.29970261819148192, -11.41317474335729543, 32.86274602512330034 ) ) ;
#21656=CARTESIAN_POINT ( 'NONE',  ( 5.999999999999878320, -9.528491918059723176, 34.59228464037033035 ) ) ;
#21657=CARTESIAN_POINT ( 'NONE',  ( -17.86920955903305597, -10.70102852606553157, 33.91149625220312913 ) ) ;
#21658=EDGE_CURVE ( 'NONE', #28072, #14886, #9508, .T. ) ;
#21659=CARTESIAN_POINT ( 'NONE',  ( -3.296039231325550656, -11.06231777344662781, 33.60647404775220082 ) ) ;
#21660=DIRECTION ( 'NONE',  ( -0.000000000000000000, 0.8660254037844399289, -0.4999999999999980016 ) ) ;
#21661=ADVANCED_FACE ( 'NONE', ( #55731 ), #14761, .F. ) ;
#21663=ORIENTED_EDGE ( 'NONE', *, *, #44813, .T. ) ;
#21664=CARTESIAN_POINT ( 'NONE',  ( -15.45425415533356350, -6.716662450894489211, 34.94144148231605840 ) ) ;
#21665=CARTESIAN_POINT ( 'NONE',  ( -14.30769230769230660, -3.322132147404559976, 32.92929555188717927 ) ) ;
#21666=B_SPLINE_CURVE_WITH_KNOTS ( 'NONE', 3,
 ( #2947, #9711, #30431, #51559, #59234, #57455, #57897, #79064, #84946, #10609 ),
 .UNSPECIFIED., .F., .F.,
 ( 4, 2, 2, 2, 4 ),
 ( 0.0007817359527651101701, 0.0009771254036996489256, 0.001172514854634187790, 0.001367904305568726653, 0.001563293756503265517 ),
 .UNSPECIFIED. ) ;
#21668=DIRECTION ( 'NONE',  ( 0.000000000000000000, 0.6427876096865373645, -0.7660444431189797898 ) ) ;
#21669=CYLINDRICAL_SURFACE ( 'NONE', #63418, 0.2499999999999995559 ) ;
#21670=EDGE_CURVE ( 'NONE', #54393, #71930, #75096, .T. ) ;
#21671=ORIENTED_EDGE ( 'NONE', *, *, #79676, .T. ) ;
#21673=DIRECTION ( 'NONE',  ( 0.000000000000000000, 0.3420201433256641055, -0.9396926207859100932 ) ) ;
#21674=CARTESIAN_POINT ( 'NONE',  ( -0.5922290646487693433, -12.62707690430377383, 30.88035979386743435 ) ) ;
#21675=CARTESIAN_POINT ( 'NONE',  ( -4.283993363284373856, -10.88202310037935661, 33.43294751532457099 ) ) ;
#21676=ORIENTED_EDGE ( 'NONE', *, *, #86411, .T. ) ;
#21677=CARTESIAN_POINT ( 'NONE',  ( 6.222779541268408821, -5.913360116392398780, 34.49180327182771322 ) ) ;
#21678=CARTESIAN_POINT ( 'NONE',  ( -8.546217925137373328, -5.582272713120729257, 34.63742843783360570 ) ) ;
#21679=CARTESIAN_POINT ( 'NONE',  ( 7.846153846153846700, -9.780366693483667717, 34.19971097300155094 ) ) ;
#21680=ORIENTED_EDGE ( 'NONE', *, *, #63055, .F. ) ;
#21681=CARTESIAN_POINT ( 'NONE',  ( 9.692307692307695177, -1.129524287112498415, 32.06866353760679544 ) ) ;
#21682=ORIENTED_EDGE ( 'NONE', *, *, #15620, .F. ) ;
#21683=CARTESIAN_POINT ( 'NONE',  ( 12.52760579488853665, -12.34228464037088813, 31.77849191805839268 ) ) ;
#21684=DIRECTION ( 'NONE',  ( -0.000000000000000000, 0.1736481776669307198, -0.9848077530122080203 ) ) ;
#21685=ORIENTED_EDGE ( 'NONE', *, *, #9278, .T. ) ;
#21686=CARTESIAN_POINT ( 'NONE',  ( 10.83816428436268176, -11.60474049983371003, 33.02348890104160262 ) ) ;
#21687=DIRECTION ( 'NONE',  ( -0.000000000000000000, -0.3420201433256694901, -0.9396926207859082059 ) ) ;
#21688=CARTESIAN_POINT ( 'NONE',  ( -6.700064078983529292, -12.38742843783360748, 31.66772728687926985 ) ) ;
#21689=FACE_OUTER_BOUND ( 'NONE', #87118, .T. ) ;
#21690=CARTESIAN_POINT ( 'NONE',  ( 2.307692307692187583, -6.026961402154118908, 34.52809138561165270 ) ) ;
#21693=VERTEX_POINT ( 'NONE', #359 ) ;
#21695=FACE_BOUND ( 'NONE', #22322, .T. ) ;
#21696=ORIENTED_EDGE ( 'NONE', *, *, #76754, .F. ) ;
#21697=CARTESIAN_POINT ( 'NONE',  ( 15.29602480204525783, -2.625532179533470512, 30.86335684631491105 ) ) ;
#21698=EDGE_CURVE ( 'NONE', #41427, #5967, #62920, .T. ) ;
#21700=AXIS2_PLACEMENT_3D ( 'NONE', #52867, #73612, #26293 ) ;
#21703=CARTESIAN_POINT ( 'NONE',  ( 18.00000000000000000, -5.471508081941601098, 34.59228464037088457 ) ) ;
#21704=CARTESIAN_POINT ( 'NONE',  ( -2.177166869458661225, -10.31582465632705237, 34.18122507451815295 ) ) ;
#21709=ORIENTED_EDGE ( 'NONE', *, *, #25703, .F. ) ;
#21710=CARTESIAN_POINT ( 'NONE',  ( -0.3954701105360233782, -3.050289026998446840, 32.03036669348366416 ) ) ;
#21711=EDGE_LOOP ( 'NONE', ( #73109, #39823, #84399, #14963 ) ) ;
#21712=CARTESIAN_POINT ( 'NONE',  ( -5.010854725920637520, -4.786620604624113540, 33.94971097300155805 ) ) ;
#21713=CARTESIAN_POINT ( 'NONE',  ( -6.793031867157151460, -2.254550872974306674, 29.97347326024527447 ) ) ;
#21714=CARTESIAN_POINT ( 'NONE',  ( -18.24997674404858827, -6.524016743844656574, 34.90889640711025521 ) ) ;
#21716=CARTESIAN_POINT ( 'NONE',  ( 8.769230769230768274, -8.973038597847269315, 34.52809138561121927 ) ) ;
#21717=EDGE_CURVE ( 'NONE', #56939, #65067, #70781, .T. ) ;
#21718=CARTESIAN_POINT ( 'NONE',  ( -15.00798956179115962, -3.563462043263030399, 33.22394488606062879 ) ) ;
#21720=CARTESIAN_POINT ( 'NONE',  ( -11.78843826940389050, -3.137211980971221781, 32.19342716148376837 ) ) ;
#21721=VERTEX_POINT ( 'NONE', #9762 ) ;
#21722=EDGE_CURVE ( 'NONE', #40455, #78447, #86917, .T. ) ;
#21723=VERTEX_POINT ( 'NONE', #50731 ) ;
#21724=B_SPLINE_CURVE_WITH_KNOTS ( 'NONE', 3,
 ( #31593, #59951, #46880, #59059, #60840, #88346, #52301, #45548, #87451, #32042 ),
 .UNSPECIFIED., .F., .F.,
 ( 4, 2, 2, 2, 4 ),
 ( 0.0007817246256747478229, 0.0009771112852218911526, 0.001172497944769034482, 0.001367884604316177595, 0.001563271263863320925 ),
 .UNSPECIFIED. ) ;
#21725=ORIENTED_EDGE ( 'NONE', *, *, #48735, .F. ) ;
#21726=CARTESIAN_POINT ( 'NONE',  ( 2.980769230769232614, -7.566082377512563184, 35.00000000000000711 ) ) ;
#21727=CARTESIAN_POINT ( 'NONE',  ( 12.21151522424549896, -6.695914987888146541, 34.68535235679833306 ) ) ;
#21729=B_SPLINE_CURVE_WITH_KNOTS ( 'NONE', 3,
 ( #77949, #15819, #29771, #43284, #30643, #58114 ),
 .UNSPECIFIED., .F., .F.,
 ( 4, 2, 4 ),
 ( 0.000000000000000000, 0.0001954784845028886158, 0.0003909569690057772317 ),
 .UNSPECIFIED. ) ;
#21730=VECTOR ( 'NONE', #34209, 1000.000000000000000 ) ;
#21731=CARTESIAN_POINT ( 'NONE',  ( -0.4615384615384611200, -1.790695186598648903, 34.54067556320373455 ) ) ;
#21732=DIRECTION ( 'NONE',  ( -0.000000000000000000, -0.5000000000000009992, -0.8660254037844380415 ) ) ;
#21733=CARTESIAN_POINT ( 'NONE',  ( 24.00000000000000000, -9.499999999999982236, 27.74999999999999645 ) ) ;
#21734=CARTESIAN_POINT ( 'NONE',  ( -6.923076923076922462, -3.322132147404559976, 32.92929555188717927 ) ) ;
#21736=CARTESIAN_POINT ( 'NONE',  ( -7.622727447239059373, -7.630147987733840509, 34.99859428049666121 ) ) ;
#21738=DIRECTION ( 'NONE',  ( 0.000000000000000000, 0.4999999999999985567, 0.8660254037844395958 ) ) ;
#21740=ORIENTED_EDGE ( 'NONE', *, *, #33504, .F. ) ;
#21741=CARTESIAN_POINT ( 'NONE',  ( 5.010840697562939816, -12.62096338111211580, 30.90682066428152197 ) ) ;
#21742=ORIENTED_EDGE ( 'NONE', *, *, #88254, .F. ) ;
#21743=FACE_BOUND ( 'NONE', #50507, .T. ) ;
#21744=CARTESIAN_POINT ( 'NONE',  ( -16.02380099101138455, -2.504778602574659896, 29.97347330155780654 ) ) ;
#21745=FACE_OUTER_BOUND ( 'NONE', #63486, .T. ) ;
#21746=CARTESIAN_POINT ( 'NONE',  ( -3.230769230769351186, -8.613356846316285953, 34.62446782046622218 ) ) ;
#21747=ORIENTED_EDGE ( 'NONE', *, *, #65167, .T. ) ;
#21748=CARTESIAN_POINT ( 'NONE',  ( 5.207448778686640800, -3.285477652293412820, 32.44071101563363158 ) ) ;
#21749=CARTESIAN_POINT ( 'NONE',  ( -17.74994558008654622, -4.074993327901529128, 33.72946981652012255 ) ) ;
#21752=ORIENTED_EDGE ( 'NONE', *, *, #52245, .T. ) ;
#21753=CARTESIAN_POINT ( 'NONE',  ( -4.826977667545033768, -4.932303261841489039, 34.32971442181322885 ) ) ;
#21754=ORIENTED_EDGE ( 'NONE', *, *, #71723, .T. ) ;
#21755=CARTESIAN_POINT ( 'NONE',  ( 16.37680928811283110, -7.369474539155830506, 34.99858011523957657 ) ) ;
#21756=EDGE_LOOP ( 'NONE', ( #73690, #49923, #2940, #72065 ) ) ;
#21757=CARTESIAN_POINT ( 'NONE',  ( 3.361561038594017337, -2.541949514083463590, 30.39797389878540557 ) ) ;
#21758=CARTESIAN_POINT ( 'NONE',  ( -1.514763354347082425, -12.50552854090298993, 31.33409797877408920 ) ) ;
#21759=CYLINDRICAL_SURFACE ( 'NONE', #87509, 0.2500000000000012212 ) ;
#21760=CARTESIAN_POINT ( 'NONE',  ( 14.24160889673643027, -8.973038597847271092, 34.52809138561120506 ) ) ;
#21761=CARTESIAN_POINT ( 'NONE',  ( -13.25408994638174143, -3.625058011473228703, 33.29252011169590020 ) ) ;
#21762=CARTESIAN_POINT ( 'NONE',  ( -7.912237257109724808, -10.51840700105979387, 33.73612834413961536 ) ) ;
#21764=EDGE_CURVE ( 'NONE', #13993, #50951, #82602, .T. ) ;
#21765=ADVANCED_FACE ( 'NONE', ( #77777 ), #85427, .F. ) ;
#21767=LINE ( 'NONE', #76716, #57890 ) ;
#21769=VERTEX_POINT ( 'NONE', #30042 ) ;
#21770=CARTESIAN_POINT ( 'NONE',  ( -16.28453675695646652, -4.684245665217972032, 34.18127051446801090 ) ) ;
#21771=ORIENTED_EDGE ( 'NONE', *, *, #25515, .F. ) ;
#21772=EDGE_CURVE ( 'NONE', #12525, #58918, #63374, .T. ) ;
#21773=AXIS2_PLACEMENT_3D ( 'NONE', #38232, #52628, #24259 ) ;
#21774=VERTEX_POINT ( 'NONE', #16967 ) ;
#21776=EDGE_CURVE ( 'NONE', #61500, #52830, #23273, .T. ) ;
#21778=CARTESIAN_POINT ( 'NONE',  ( -10.61538461538473399, -11.48612834414049644, 32.76840700105863391 ) ) ;
#21779=CARTESIAN_POINT ( 'NONE',  ( -2.242436736416282272, -6.879047030191282275, 34.71129190930002295 ) ) ;
#21780=AXIS2_PLACEMENT_3D ( 'NONE', #28174, #69608, #7914 ) ;
#21781=CARTESIAN_POINT ( 'NONE',  ( -9.692307692307814193, -11.06231777344772027, 33.60647404775119895 ) ) ;
#21782=CARTESIAN_POINT ( 'NONE',  ( 10.74591005361826035, -6.808710257144161559, 34.95449254468098843 ) ) ;
#21783=CARTESIAN_POINT ( 'NONE',  ( -16.21992956480203318, -3.050289026998445951, 32.03036669348365706 ) ) ;
#21784=CARTESIAN_POINT ( 'NONE',  ( 16.08857570788537572, -11.94971097300153140, 32.03036669348370680 ) ) ;
#21785=CARTESIAN_POINT ( 'NONE',  ( -0.4615384615384611200, -8.164416787775445883, 34.95778746994557906 ) ) ;
#21787=CYLINDRICAL_SURFACE ( 'NONE', #79386, 0.2499999999999986955 ) ;
#21789=DIRECTION ( 'NONE',  ( 0.000000000000000000, 0.9396926207859126468, -0.3420201433256571111 ) ) ;
#21790=CARTESIAN_POINT ( 'NONE',  ( -9.692307692307814193, -3.643525952248795718, 33.31231777344771672 ) ) ;
#21791=VERTEX_POINT ( 'NONE', #9334 ) ;
#21792=ORIENTED_EDGE ( 'NONE', *, *, #81451, .F. ) ;
#21793=CARTESIAN_POINT ( 'NONE',  ( -18.13014796973169851, -2.647304123082328875, 31.75400227202885262 ) ) ;
#21795=EDGE_CURVE ( 'NONE', #73491, #69353, #3443, .T. ) ;
#21796=CARTESIAN_POINT ( 'NONE',  ( 9.915320536401090123, -11.98016756924215009, 32.48728574198911190 ) ) ;
#21797=ORIENTED_EDGE ( 'NONE', *, *, #78069, .T. ) ;
#21798=B_SPLINE_CURVE_WITH_KNOTS ( 'NONE', 3,
 ( #69190, #55664, #14692, #63756, #34954, #2059, #29108, #731, #21890, #56564 ),
 .UNSPECIFIED., .F., .F.,
 ( 4, 2, 2, 2, 4 ),
 ( 0.000000000000000000, 0.0001954339857564092362, 0.0003908679715128184724, 0.0005863019572692276544, 0.0007817359430256369448 ),
 .UNSPECIFIED. ) ;
#21799=FACE_OUTER_BOUND ( 'NONE', #36722, .T. ) ;
#21800=DIRECTION ( 'NONE',  ( -0.000000000000000000, 1.000000000000000000, 0.000000000000000000 ) ) ;
#21801=AXIS2_PLACEMENT_3D ( 'NONE', #39905, #47079, #6111 ) ;
#21802=CARTESIAN_POINT ( 'NONE',  ( -9.627052552794856055, -3.643525952247864463, 33.31231777344670064 ) ) ;
#21804=ORIENTED_EDGE ( 'NONE', *, *, #11789, .T. ) ;
#21805=CARTESIAN_POINT ( 'NONE',  ( -9.692307692307814193, -12.70778746994576025, 30.41441678777401236 ) ) ;
#21807=VECTOR ( 'NONE', #79828, 1000.000000000000000 ) ;
#21808=ADVANCED_FACE ( 'NONE', ( #64247 ), #57503, .F. ) ;
#21809=CARTESIAN_POINT ( 'NONE',  ( 13.38461538461526423, -12.51329471203414379, 31.30864560766407578 ) ) ;
#21811=CARTESIAN_POINT ( 'NONE',  ( -1.384615384615383471, -9.058645607665452459, 34.76329471203371924 ) ) ;
#21812=FACE_OUTER_BOUND ( 'NONE', #48640, .T. ) ;
#21813=CARTESIAN_POINT ( 'NONE',  ( -6.673022503163468677, -2.544122305571457687, 31.48381861865059150 ) ) ;
#21814=ORIENTED_EDGE ( 'NONE', *, *, #63567, .F. ) ;
#21815=EDGE_CURVE ( 'NONE', #53903, #57115, #82528, .T. ) ;
#21816=ORIENTED_EDGE ( 'NONE', *, *, #22364, .F. ) ;
#21817=ORIENTED_EDGE ( 'NONE', *, *, #47113, .T. ) ;
#21818=VERTEX_POINT ( 'NONE', #55077 ) ;
#21820=FACE_OUTER_BOUND ( 'NONE', #21847, .T. ) ;
#21822=B_SPLINE_CURVE_WITH_KNOTS ( 'NONE', 3,
 ( #35782, #83975, #42976, #36659, #11860, #12291, #80767, #25360, #72652, #45625 ),
 .UNSPECIFIED., .F., .F.,
 ( 4, 2, 2, 2, 4 ),
 ( 0.0007817246256747474977, 0.0009771112852218911526, 0.001172497944769034699, 0.001367884604316178462, 0.001563271263863322009 ),
 .UNSPECIFIED. ) ;
#21823=CARTESIAN_POINT ( 'NONE',  ( 11.53846153846153832, -5.471508081941601098, 34.59228464037088457 ) ) ;
#21825=CARTESIAN_POINT ( 'NONE',  ( 11.53846153846141753, -12.27809138561165270, 31.22303859784587132 ) ) ;
#21826=CARTESIAN_POINT ( 'NONE',  ( -9.692307692307814193, -10.33852847137269571, 34.16647553114546554 ) ) ;
#21828=ORIENTED_EDGE ( 'NONE', *, *, #87785, .F. ) ;
#21829=EDGE_CURVE ( 'NONE', #25168, #24368, #30872, .T. ) ;
#21831=AXIS2_PLACEMENT_3D ( 'NONE', #49038, #35979, #1740 ) ;
#21832=ORIENTED_EDGE ( 'NONE', *, *, #78548, .T. ) ;
#21833=CARTESIAN_POINT ( 'NONE',  ( 12.71148397988660150, -8.433404298154334455, 34.66254593164985920 ) ) ;
#21834=ORIENTED_EDGE ( 'NONE', *, *, #73315, .F. ) ;
#21835=EDGE_CURVE ( 'NONE', #55506, #56098, #22362, .T. ) ;
#21836=CARTESIAN_POINT ( 'NONE',  ( -11.31544869436814160, -4.026326845037962343, 33.68677907613344047 ) ) ;
#21838=CARTESIAN_POINT ( 'NONE',  ( -2.241623956689868358, -8.973038597847269315, 34.52809138561122637 ) ) ;
#21841=VERTEX_POINT ( 'NONE', #52959 ) ;
#21842=CARTESIAN_POINT ( 'NONE',  ( -17.93393266664992680, -2.833524468853757305, 32.15551576947926549 ) ) ;
#21843=EDGE_LOOP ( 'NONE', ( #8589, #33456, #45894, #57040 ) ) ;
#21844=FACE_BOUND ( 'NONE', #80535, .T. ) ;
#21845=CARTESIAN_POINT ( 'NONE',  ( -2.242437168179467033, -5.094484230520773593, 34.41647553114626845 ) ) ;
#21846=CARTESIAN_POINT ( 'NONE',  ( 8.096099255531887806, -5.766571408460171355, 34.70601412856602508 ) ) ;
#21847=EDGE_LOOP ( 'NONE', ( #13347, #19159, #56945, #66798 ) ) ;
#21848=CARTESIAN_POINT ( 'NONE',  ( -14.98071491913091791, -4.943051570960394159, 34.04725096376909477 ) ) ;
#21849=CARTESIAN_POINT ( 'NONE',  ( -9.692307692307814193, -5.094484230521993062, 34.41647553114689373 ) ) ;
#21851=CARTESIAN_POINT ( 'NONE',  ( -4.153846153846152411, -4.098570777380720287, 33.41473453929634729 ) ) ;
#21852=CARTESIAN_POINT ( 'NONE',  ( 16.15384615384603251, -8.613356846316285953, 34.62446782046622218 ) ) ;
#21853=ORIENTED_EDGE ( 'NONE', *, *, #75849, .T. ) ;
#21854=CARTESIAN_POINT ( 'NONE',  ( 16.02336944572969202, -7.276988635370451597, 34.74523720219453793 ) ) ;
#21855=DIRECTION ( 'NONE',  ( -0.000000000000000000, -0.6427876096865404731, -0.7660444431189771253 ) ) ;
#21856=CARTESIAN_POINT ( 'NONE',  ( -13.38461538461507594, -2.506253911140614576, 30.00000000000323297 ) ) ;
#21858=DIRECTION ( 'NONE',  ( -1.000000000000000000, 0.000000000000000000, 0.000000000000000000 ) ) ;
#21859=FACE_BOUND ( 'NONE', #79318, .T. ) ;
#21860=CARTESIAN_POINT ( 'NONE',  ( 13.16168916709923487, -11.76352882383564769, 32.36236540154569497 ) ) ;
#21861=CARTESIAN_POINT ( 'NONE',  ( -6.249976744048591826, -10.06842814019191401, 34.32929386961144758 ) ) ;
#21862=B_SPLINE_CURVE_WITH_KNOTS ( 'NONE', 3,
 ( #82851, #35088, #42748, #21127, #41862, #49500, #69762, #35541, #56254, #83289 ),
 .UNSPECIFIED., .F., .F.,
 ( 4, 2, 2, 2, 4 ),
 ( 0.0007817359430256308733, 0.0009771253907249971907, 0.001172514838424363725, 0.001367904286123730259, 0.001563293733823096577 ),
 .UNSPECIFIED. ) ;
#21863=DIRECTION ( 'NONE',  ( -0.000000000000000000, -0.8660254037844399289, -0.4999999999999980016 ) ) ;
#21865=CARTESIAN_POINT ( 'NONE',  ( -18.13069060311030611, -2.845849958028614957, 32.17971566917920256 ) ) ;
#21867=DIRECTION ( 'NONE',  ( 1.000000000000000000, 0.000000000000000000, 0.000000000000000000 ) ) ;
#21868=B_SPLINE_CURVE_WITH_KNOTS ( 'NONE', 3,
 ( #67698, #54165, #6444, #6005, #60931, #47409, #19942, #82984, #48299, #88432 ),
 .UNSPECIFIED., .F., .F.,
 ( 4, 2, 2, 2, 4 ),
 ( 0.0007817246256747474977, 0.0009771112852218909357, 0.001172497944769034482, 0.001367884604316178029, 0.001563271263863321575 ),
 .UNSPECIFIED. ) ;
#21870=VERTEX_POINT ( 'NONE', #31825 ) ;
#21871=CARTESIAN_POINT ( 'NONE',  ( 1.318531973659506251, -12.10708131394839349, 31.69288490824020244 ) ) ;
#21872=ORIENTED_EDGE ( 'NONE', *, *, #58162, .F. ) ;
#21873=ADVANCED_FACE ( 'NONE', ( #18752 ), #45769, .F. ) ;
#21874=CARTESIAN_POINT ( 'NONE',  ( -15.23076923076935074, -4.481592998941358097, 33.73612834414048933 ) ) ;
#21876=CARTESIAN_POINT ( 'NONE',  ( -11.40767109749459074, -6.369690395747422684, 34.87708834333098196 ) ) ;
#21878=CYLINDRICAL_SURFACE ( 'NONE', #76169, 0.2499999999999986955 ) ;
#21879=VERTEX_POINT ( 'NONE', #11098 ) ;
#21880=CARTESIAN_POINT ( 'NONE',  ( -6.066083410955879884, -11.69971097300155272, 32.46337939537587403 ) ) ;
#21882=CARTESIAN_POINT ( 'NONE',  ( 6.000000000000001776, -6.343179335718451384, 34.87096338111211935 ) ) ;
#21883=CARTESIAN_POINT ( 'NONE',  ( 4.023154687178596589, -8.999036380462719364, 34.52022231692819076 ) ) ;
#21884=CARTESIAN_POINT ( 'NONE',  ( -5.326946314216041145, -5.056417327199099532, 34.11270091957320716 ) ) ;
#21885=CARTESIAN_POINT ( 'NONE',  ( 12.33084699487090674, -2.729777683071817229, 31.24903638046269450 ) ) ;
#21886=CARTESIAN_POINT ( 'NONE',  ( 23.00000000000000000, -5.499999999999981348, 27.75000000000000000 ) ) ;
#21887=DIRECTION ( 'NONE',  ( -0.000000000000000000, -0.8660254037844397068, -0.4999999999999978906 ) ) ;
#21888=EDGE_CURVE ( 'NONE', #39225, #26637, #137, .T. ) ;
#21890=CARTESIAN_POINT ( 'NONE',  ( -9.757578138268465651, -3.835265460703609186, 33.15142922261924241 ) ) ;
#21891=FACE_OUTER_BOUND ( 'NONE', #21711, .T. ) ;
#21892=ADVANCED_FACE ( 'NONE', ( #24607 ), #66492, .F. ) ;
#21893=CARTESIAN_POINT ( 'NONE',  ( -11.53846153846153655, -1.117168528481311540, 33.14645433367849847 ) ) ;
#21895=CARTESIAN_POINT ( 'NONE',  ( -10.54931728203453822, -5.471508081941601098, 34.59228464037088457 ) ) ;
#21896=VECTOR ( 'NONE', #19708, 1000.000000000000227 ) ;
#21897=ORIENTED_EDGE ( 'NONE', *, *, #69200, .F. ) ;
#21898=EDGE_CURVE ( 'NONE', #5201, #17409, #31369, .T. ) ;
#21899=CARTESIAN_POINT ( 'NONE',  ( -17.86947429823643674, -2.882268652242223173, 31.66798894389554064 ) ) ;
#21901=CARTESIAN_POINT ( 'NONE',  ( 1.319344938654610999, -12.46129190929999986, 30.37095296980880832 ) ) ;
#21902=CARTESIAN_POINT ( 'NONE',  ( 17.07692307692307665, -11.69971097300155272, 32.46337939537588113 ) ) ;
#21904=VECTOR ( 'NONE', #42086, 1000.000000000000114 ) ;
#21905=CARTESIAN_POINT ( 'NONE',  ( -10.48459417441766561, -9.084667340241226796, 34.75534355489798344 ) ) ;
#21906=EDGE_CURVE ( 'NONE', #75988, #78555, #82573, .T. ) ;
#21907=CARTESIAN_POINT ( 'NONE',  ( -39.05038313613820122, -2.499999999999999556, 29.75000000000000355 ) ) ;
#21908=B_SPLINE_CURVE_WITH_KNOTS ( 'NONE', 3,
 ( #74448, #82552, #120, #19939, #13196, #74014, #34338, #60489, #48295, #14073 ),
 .UNSPECIFIED., .F., .F.,
 ( 4, 2, 2, 2, 4 ),
 ( 0.0007817246256747471724, 0.0009771112852218905021, 0.001172497944769033615, 0.001367884604316176944, 0.001563271263863320274 ),
 .UNSPECIFIED. ) ;
#21909=DIRECTION ( 'NONE',  ( 0.000000000000000000, 0.6427876096865368094, 0.7660444431189802339 ) ) ;
#21910=VERTEX_POINT ( 'NONE', #61376 ) ;
#21911=EDGE_LOOP ( 'NONE', ( #13402, #74439 ) ) ;
#21914=CARTESIAN_POINT ( 'NONE',  ( 5.207448778686640800, -11.93748526763465279, 32.05452791011430946 ) ) ;
#21916=CARTESIAN_POINT ( 'NONE',  ( 12.46153846153846168, -1.215029322943914858, 32.30358669280327177 ) ) ;
#21918=DIRECTION ( 'NONE',  ( 0.000000000000000000, 0.9396926207859126468, 0.3420201433256571111 ) ) ;
#21919=CARTESIAN_POINT ( 'NONE',  ( -5.999999999999998224, -11.33034616979429110, 35.88435417666054406 ) ) ;
#21920=EDGE_LOOP ( 'NONE', ( #39184, #77222, #62977, #87933 ) ) ;
#21921=DIRECTION ( 'NONE',  ( 0.000000000000000000, 0.7660444431189822323, -0.6427876096865344779 ) ) ;
#21925=ADVANCED_FACE ( 'NONE', ( #54621 ), #87223, .F. ) ;
#21926=ADVANCED_FACE ( 'NONE', ( #66934 ), #15435, .F. ) ;
#21927=EDGE_LOOP ( 'NONE', ( #26060, #28141 ) ) ;
#21928=CARTESIAN_POINT ( 'NONE',  ( 8.546303810323914618, -12.38737895849757820, 31.66785238281580206 ) ) ;
#21929=ORIENTED_EDGE ( 'NONE', *, *, #5994, .F. ) ;
#21930=DIRECTION ( 'NONE',  ( -0.000000000000000000, 0.1736481776669307198, -0.9848077530122080203 ) ) ;
#21931=CARTESIAN_POINT ( 'NONE',  ( -16.37733109757010652, -4.386631170607603991, 33.66268669641500111 ) ) ;
#21932=CARTESIAN_POINT ( 'NONE',  ( -15.90384615384615330, -2.499999999999998668, 29.75000000000000355 ) ) ;
#21933=CARTESIAN_POINT ( 'NONE',  ( 14.17721712261659128, -7.276987145209184327, 34.99546412871779211 ) ) ;
#21934=EDGE_LOOP ( 'NONE', ( #25497, #78587, #20144, #33216 ) ) ;
#21935=EDGE_CURVE ( 'NONE', #42554, #59805, #7782, .T. ) ;
#21936=ORIENTED_EDGE ( 'NONE', *, *, #86397, .T. ) ;
#21937=EDGE_LOOP ( 'NONE', ( #32162, #17939 ) ) ;
#21938=CARTESIAN_POINT ( 'NONE',  ( -2.177166869458660781, -3.625058011473228259, 33.29252011169590020 ) ) ;
#21939=CARTESIAN_POINT ( 'NONE',  ( -2.437839517130524047, -2.882441371585227508, 31.66841991370171527 ) ) ;
#21940=ORIENTED_EDGE ( 'NONE', *, *, #72031, .F. ) ;
#21941=CARTESIAN_POINT ( 'NONE',  ( -8.519230769229334754, -7.500000000000155431, 34.75000000000007105 ) ) ;
#21943=B_SPLINE_CURVE_WITH_KNOTS ( 'NONE', 3,
 ( #82154, #69955, #171, #48348, #35284, #75825, #55111, #62742, #14127, #47460 ),
 .UNSPECIFIED., .F., .F.,
 ( 4, 2, 2, 2, 4 ),
 ( 0.0007817359430256289217, 0.0009771253907249945886, 0.001172514838424360255, 0.001367904286123725922, 0.001563293733823091589 ),
 .UNSPECIFIED. ) ;
#21944=EDGE_CURVE ( 'NONE', #5455, #38257, #84341, .T. ) ;
#21945=ADVANCED_FACE ( 'NONE', ( #8678 ), #1906, .F. ) ;
#21946=CARTESIAN_POINT ( 'NONE',  ( 6.989145274079363368, -11.69971097300155272, 32.46337939537588113 ) ) ;
#21948=LINE ( 'NONE', #62911, #60912 ) ;
#21949=CARTESIAN_POINT ( 'NONE',  ( 15.23076923076923173, -12.48256725967547354, 35.29906147534542527 ) ) ;
#21951=FACE_BOUND ( 'NONE', #57377, .T. ) ;
#21953=CARTESIAN_POINT ( 'NONE',  ( -10.61538461538473577, -5.094484230521993062, 34.41647553114689373 ) ) ;
#21954=LINE ( 'NONE', #49426, #64349 ) ;
#21955=VECTOR ( 'NONE', #76259, 1000.000000000000114 ) ;
#21956=DIRECTION ( 'NONE',  ( -0.000000000000000000, -0.9848077530122086864, -0.1736481776669273613 ) ) ;
#21957=CARTESIAN_POINT ( 'NONE',  ( 18.22301284409340028, -2.889357225399416418, 32.26129605718031002 ) ) ;
#21959=VECTOR ( 'NONE', #33784, 1000.000000000000227 ) ;
#21960=CARTESIAN_POINT ( 'NONE',  ( -3.930834802233305059, -2.758310577978207778, 31.33698337089303010 ) ) ;
#21961=CARTESIAN_POINT ( 'NONE',  ( 14.30769230769231015, -2.292212530054420494, 30.41441678777542634 ) ) ;
#21962=VERTEX_POINT ( 'NONE', #34800 ) ;
#21963=CARTESIAN_POINT ( 'NONE',  ( -2.438382910802615378, -3.957541250942359756, 33.62499894934981626 ) ) ;
#21965=ORIENTED_EDGE ( 'NONE', *, *, #31041, .F. ) ;
#21966=VECTOR ( 'NONE', #61328, 1000.000000000000227 ) ;
#21967=DIRECTION ( 'NONE',  ( -0.000000000000000000, 0.5000000000000011102, -0.8660254037844381525 ) ) ;
#21968=CARTESIAN_POINT ( 'NONE',  ( 15.90386940979756858, -6.524016743844656574, 34.90889640711025521 ) ) ;
#21969=LINE ( 'NONE', #4698, #23174 ) ;
#21970=ORIENTED_EDGE ( 'NONE', *, *, #29881, .F. ) ;
#21971=CARTESIAN_POINT ( 'NONE',  ( -13.13456096470193124, -11.47946981652013498, 33.17500667209847620 ) ) ;
#21973=FACE_BOUND ( 'NONE', #24798, .T. ) ;
#21974=CARTESIAN_POINT ( 'NONE',  ( -16.15384615384615330, -1.790695186598648903, 34.54067556320373455 ) ) ;
#21975=CARTESIAN_POINT ( 'NONE',  ( 3.903822929624694904, -12.45566812827425096, 31.48439005359158926 ) ) ;
#21976=CARTESIAN_POINT ( 'NONE',  ( -15.90379184220783948, -2.564540009722896752, 30.55348353981672105 ) ) ;
#21977=CARTESIAN_POINT ( 'NONE',  ( -4.853910232829682592, -10.01129605718032778, 34.36064277460058491 ) ) ;
#21978=FACE_OUTER_BOUND ( 'NONE', #14726, .T. ) ;
#21979=CARTESIAN_POINT ( 'NONE',  ( -17.93474442872397034, -5.219633306516379356, 34.19971097300157936 ) ) ;
#21981=EDGE_LOOP ( 'NONE', ( #15889, #28216 ) ) ;
#21982=ORIENTED_EDGE ( 'NONE', *, *, #88519, .F. ) ;
#21983=CARTESIAN_POINT ( 'NONE',  ( 5.076923076923075762, -6.386643153685126251, 34.62446782046654192 ) ) ;
#21984=CARTESIAN_POINT ( 'NONE',  ( 14.37375964104238513, -12.62096338111211757, 30.90682066428152908 ) ) ;
#21985=CYLINDRICAL_SURFACE ( 'NONE', #28723, 0.2500000000000008882 ) ;
#21986=CARTESIAN_POINT ( 'NONE',  ( -17.07692307692307665, -11.16473453929635440, 33.15142922261926373 ) ) ;
#21987=CARTESIAN_POINT ( 'NONE',  ( -16.28453762051371712, -12.11776431015576172, 31.66791131148498906 ) ) ;
#21989=CARTESIAN_POINT ( 'NONE',  ( 6.673053698855467175, -2.341070481393820124, 30.72580821765574299 ) ) ;
#21990=CARTESIAN_POINT ( 'NONE',  ( 4.153846153846030731, -12.16647553114689728, 32.15551576947799362 ) ) ;
#21991=CARTESIAN_POINT ( 'NONE',  ( -4.153846153846274980, -6.835583212225970762, 34.95778746994575670 ) ) ;
#21992=CARTESIAN_POINT ( 'NONE',  ( 17.77713457779636386, -2.501496062324911840, 29.88072118266895671 ) ) ;
#21993=DIRECTION ( 'NONE',  ( -0.000000000000000000, 0.3420201433256694346, -0.9396926207859080948 ) ) ;
#21994=CARTESIAN_POINT ( 'NONE',  ( 18.06606835100244268, -9.780366693483667717, 34.19971097300155805 ) ) ;
#21996=CARTESIAN_POINT ( 'NONE',  ( -5.010854725920639297, -2.721908614388772296, 31.22303859784725333 ) ) ;
#21997=CARTESIAN_POINT ( 'NONE',  ( 10.55006169989244214, -7.749976743299138882, 34.99404534957040624 ) ) ;
#21998=CARTESIAN_POINT ( 'NONE',  ( 3.100622021331011169, -2.619462340734462380, 30.83744416345203021 ) ) ;
#21999=ORIENTED_EDGE ( 'NONE', *, *, #70860, .F. ) ;
#22000=CARTESIAN_POINT ( 'NONE',  ( 12.21151523731700372, -4.175268141568685643, 33.81360843649122216 ) ) ;
#22001=CARTESIAN_POINT ( 'NONE',  ( 14.30769230769231015, -12.62096338111211580, 30.90682066428153263 ) ) ;
#22002=B_SPLINE_CURVE_WITH_KNOTS ( 'NONE', 3,
 ( #71165, #14464, #41942, #36935, #43696, #64398, #15355, #69409, #42829, #2697 ),
 .UNSPECIFIED., .F., .F.,
 ( 4, 2, 2, 2, 4 ),
 ( 0.000000000000000000, 0.0001954339857564081520, 0.0003908679715128163040, 0.0005863019572692244018, 0.0007817359430256326080 ),
 .UNSPECIFIED. ) ;
#22004=B_SPLINE_CURVE_WITH_KNOTS ( 'NONE', 3,
 ( #33166, #88140, #26413, #81364, #18325, #45787, #73266, #39054, #66511, #4815 ),
 .UNSPECIFIED., .F., .F.,
 ( 4, 2, 2, 2, 4 ),
 ( 0.000000000000000000, 0.0001954311564186861426, 0.0003908623128373722852, 0.0005862934692560583735, 0.0007817246256747445703 ),
 .UNSPECIFIED. ) ;
#22005=CARTESIAN_POINT ( 'NONE',  ( 6.856994543716787405, -4.661471528628507777, 34.16647553114621871 ) ) ;
#22008=DIRECTION ( 'NONE',  ( -0.000000000000000000, -0.1736481776669307198, -0.9848077530122080203 ) ) ;
#22009=CARTESIAN_POINT ( 'NONE',  ( -6.222879516737585881, -7.630690623152302621, 34.99857592706774057 ) ) ;
#22010=ORIENTED_EDGE ( 'NONE', *, *, #69854, .T. ) ;
#22011=CARTESIAN_POINT ( 'NONE',  ( 4.153846153846154188, -11.33034616979429110, 35.88435417666054406 ) ) ;
#22012=CARTESIAN_POINT ( 'NONE',  ( -2.437840277424004665, -11.04286588640298561, 33.62463336215343901 ) ) ;
#22013=ORIENTED_EDGE ( 'NONE', *, *, #41630, .F. ) ;
#22014=CARTESIAN_POINT ( 'NONE',  ( -13.16160403300253634, -2.554770724473667265, 30.48948780036025852 ) ) ;
#22015=CARTESIAN_POINT ( 'NONE',  ( 7.623275163725200088, -7.630691491037286056, 34.74850469731151748 ) ) ;
#22016=EDGE_CURVE ( 'NONE', #62711, #42060, #28052, .T. ) ;
#22017=ORIENTED_EDGE ( 'NONE', *, *, #62198, .T. ) ;
#22018=CARTESIAN_POINT ( 'NONE',  ( -5.076923076923075762, -11.35647404775217417, 33.31231777344666511 ) ) ;
#22020=CARTESIAN_POINT ( 'NONE',  ( 15.23076923076923173, -11.35647404775217417, 33.31231777344666511 ) ) ;
#22021=ORIENTED_EDGE ( 'NONE', *, *, #15651, .T. ) ;
#22022=VERTEX_POINT ( 'NONE', #29396 ) ;
#22023=CARTESIAN_POINT ( 'NONE',  ( 2.980792486720639900, -2.920706130388546651, 32.31842814019191223 ) ) ;
#22024=VECTOR ( 'NONE', #30817, 1000.000000000000114 ) ;
#22025=VERTEX_POINT ( 'NONE', #35248 ) ;
#22026=AXIS2_PLACEMENT_3D ( 'NONE', #50619, #64562, #36673 ) ;
#22027=CARTESIAN_POINT ( 'NONE',  ( 10.61538461538449418, -12.51329471203414379, 31.30864560766407578 ) ) ;
#22028=CARTESIAN_POINT ( 'NONE',  ( 2.557746727605762160, -11.47946981652013498, 33.17500667209846910 ) ) ;
#22030=FACE_OUTER_BOUND ( 'NONE', #83532, .T. ) ;
#22031=CARTESIAN_POINT ( 'NONE',  ( -3.007756386675835891, -8.282913670948747864, 34.94150082978203642 ) ) ;
#22032=CARTESIAN_POINT ( 'NONE',  ( 12.46153846153833911, -2.625532179533778709, 30.86335684631627174 ) ) ;
#22033=B_SPLINE_CURVE_WITH_KNOTS ( 'NONE', 3,
 ( #69248, #20612, #13414, #47192, #46761, #19292, #68802, #26938, #40896, #7550 ),
 .UNSPECIFIED., .F., .F.,
 ( 4, 2, 2, 2, 4 ),
 ( 0.0007817359430256282712, 0.0009771253907249943717, 0.001172514838424360689, 0.001367904286123726790, 0.001563293733823092890 ),
 .UNSPECIFIED. ) ;
#22034=EDGE_LOOP ( 'NONE', ( #24440, #28316 ) ) ;
#22035=EDGE_CURVE ( 'NONE', #48826, #8133, #55517, .T. ) ;
#22036=B_SPLINE_CURVE_WITH_KNOTS ( 'NONE', 3,
 ( #82181, #75414, #14600, #69102, #41191, #75855, #74981, #42083, #14154, #69540 ),
 .UNSPECIFIED., .F., .F.,
 ( 4, 2, 2, 2, 4 ),
 ( 0.0007817359527651104954, 0.0009771254036996493593, 0.001172514854634188440, 0.001367904305568727304, 0.001563293756503266168 ),
 .UNSPECIFIED. ) ;
#22037=ORIENTED_EDGE ( 'NONE', *, *, #88552, .F. ) ;
#22038=LINE ( 'NONE', #9406, #86150 ) ;
#22039=ORIENTED_EDGE ( 'NONE', *, *, #3907, .F. ) ;
#22041=VERTEX_POINT ( 'NONE', #77125 ) ;
#22042=CARTESIAN_POINT ( 'NONE',  ( 7.715463243043539698, -11.93127051446800024, 32.56575433478200665 ) ) ;
#22044=ORIENTED_EDGE ( 'NONE', *, *, #7511, .F. ) ;
#22046=AXIS2_PLACEMENT_3D ( 'NONE', #27175, #81247, #67726 ) ;
#22047=VERTEX_POINT ( 'NONE', #63155 ) ;
#22048=CARTESIAN_POINT ( 'NONE',  ( 9.692307692307570832, -8.656820664282941280, 34.87096338111179961 ) ) ;
#22049=VERTEX_POINT ( 'NONE', #83455 ) ;
#22050=VECTOR ( 'NONE', #5197, 1000.000000000000000 ) ;
#22051=CYLINDRICAL_SURFACE ( 'NONE', #34443, 0.2500000000000002220 ) ;
#22052=EDGE_CURVE ( 'NONE', #39944, #55341, #42798, .T. ) ;
#22056=CARTESIAN_POINT ( 'NONE',  ( -6.857009589726848375, -4.661471528628508665, 34.16647553114624003 ) ) ;
#22057=CARTESIAN_POINT ( 'NONE',  ( 17.86930939688969033, -12.35290016733513951, 31.75349464988449455 ) ) ;
#22058=FACE_BOUND ( 'NONE', #13751, .T. ) ;
#22059=CARTESIAN_POINT ( 'NONE',  ( -11.76138775597768138, -2.554751324335734708, 30.48935550225260727 ) ) ;
#22060=CARTESIAN_POINT ( 'NONE',  ( -6.923076923077045919, -9.528491918059723176, 34.59228464037033035 ) ) ;
#22061=CARTESIAN_POINT ( 'NONE',  ( 9.442330948259103351, -2.318417181685855422, 30.59732222474233865 ) ) ;
#22062=CARTESIAN_POINT ( 'NONE',  ( -17.01166793741023042, -12.51329471203373700, 31.30864560766537963 ) ) ;
#22064=CARTESIAN_POINT ( 'NONE',  ( -6.923076923077044142, -6.879047030192662504, 34.71129190930017927 ) ) ;
#22066=CARTESIAN_POINT ( 'NONE',  ( 1.384615384615386802, -12.78798330534102945, 29.74999999999997868 ) ) ;
#22068=ORIENTED_EDGE ( 'NONE', *, *, #62218, .F. ) ;
#22069=B_SPLINE_CURVE_WITH_KNOTS ( 'NONE', 3,
 ( #22448, #82837, #2170, #29658, #28776, #35077, #21110, #43167, #14819, #56241 ),
 .UNSPECIFIED., .F., .F.,
 ( 4, 2, 2, 2, 4 ),
 ( 0.0007817359430256372700, 0.0009771253907250054306, 0.001172514838424373700, 0.001367904286123741969, 0.001563293733823110238 ),
 .UNSPECIFIED. ) ;
#22070=CARTESIAN_POINT ( 'NONE',  ( -5.142193077479397800, -12.16647553114622049, 32.15551576947930812 ) ) ;
#22071=CARTESIAN_POINT ( 'NONE',  ( 16.28437185560971656, -12.27024696741798770, 31.24895572276497546 ) ) ;
#22072=B_SPLINE_CURVE_WITH_KNOTS ( 'NONE', 3,
 ( #5865, #67125, #38759, #45505, #87865, #17606, #11283, #53600, #18494, #80650 ),
 .UNSPECIFIED., .F., .F.,
 ( 4, 2, 2, 2, 4 ),
 ( 0.0007817359430256288133, 0.0009771253907249948054, 0.001172514838424360689, 0.001367904286123726573, 0.001563293733823092457 ),
 .UNSPECIFIED. ) ;
#22073=CARTESIAN_POINT ( 'NONE',  ( 6.988332494352946789, -6.879047030191282275, 34.71129190930002295 ) ) ;
#22074=DIRECTION ( 'NONE',  ( 0.000000000000000000, 0.6427876096865368094, 0.7660444431189802339 ) ) ;
#22075=B_SPLINE_CURVE_WITH_KNOTS ( 'NONE', 3,
 ( #7206, #14401, #27917, #55387, #82871, #69354 ),
 .UNSPECIFIED., .F., .F.,
 ( 4, 2, 4 ),
 ( 0.000000000000000000, 0.0001954784845028902421, 0.0003909569690057804843 ),
 .UNSPECIFIED. ) ;
#22076=CARTESIAN_POINT ( 'NONE',  ( -12.21159305216042235, -2.589246495874658383, 31.60778113518102828 ) ) ;
#22077=CARTESIAN_POINT ( 'NONE',  ( 13.51514108637895184, -11.46989282347013095, 32.79007818306219946 ) ) ;
#22078=VERTEX_POINT ( 'NONE', #56412 ) ;
#22079=DIRECTION ( 'NONE',  ( -0.000000000000000000, 0.3420201433256694901, -0.9396926207859082059 ) ) ;
#22080=CARTESIAN_POINT ( 'NONE',  ( 1.384615384615265343, -12.27809138561165270, 31.22303859784587132 ) ) ;
#22081=FACE_OUTER_BOUND ( 'NONE', #1013, .T. ) ;
#22082=CARTESIAN_POINT ( 'NONE',  ( -0.4615384615385840772, -9.528491918059723176, 34.59228464037033035 ) ) ;
#22085=ORIENTED_EDGE ( 'NONE', *, *, #56918, .T. ) ;
#22086=VECTOR ( 'NONE', #32980, 1000.000000000000227 ) ;
#22087=ORIENTED_EDGE ( 'NONE', *, *, #42683, .F. ) ;
#22088=AXIS2_PLACEMENT_3D ( 'NONE', #77330, #14752, #57051 ) ;
#22089=CARTESIAN_POINT ( 'NONE',  ( -6.223484924564330001, -4.225889041578354544, 33.85425143139329407 ) ) ;
#22090=ORIENTED_EDGE ( 'NONE', *, *, #68149, .F. ) ;
#22093=CARTESIAN_POINT ( 'NONE',  ( -18.00000000000000000, -13.75143057439168182, 32.29137909377919868 ) ) ;
#22094=CARTESIAN_POINT ( 'NONE',  ( -8.769230769230768274, -10.51840700105979565, 33.73612834413961536 ) ) ;
#22095=CARTESIAN_POINT ( 'NONE',  ( -17.01085472592064107, -12.10708131394839882, 31.69288490824020954 ) ) ;
#22096=DIRECTION ( 'NONE',  ( -0.000000000000000000, -0.6427876096865404731, -0.7660444431189770143 ) ) ;
#22097=ORIENTED_EDGE ( 'NONE', *, *, #36491, .T. ) ;
#22098=CARTESIAN_POINT ( 'NONE',  ( 4.153846153846154188, -4.098570777380720287, 33.41473453929634729 ) ) ;
#22099=CARTESIAN_POINT ( 'NONE',  ( -13.16160403300253279, -4.187068189119699468, 33.49521262558774026 ) ) ;
#22102=CARTESIAN_POINT ( 'NONE',  ( 2.980745993476265010, -12.43535235679832596, 30.55408501211184813 ) ) ;
#22103=CARTESIAN_POINT ( 'NONE',  ( -0.4615384615384611200, -3.937682226553329556, 33.60647404775216529 ) ) ;
#22104=CARTESIAN_POINT ( 'NONE',  ( 6.223012844093396723, -9.172514111537584114, 34.72667873470787470 ) ) ;
#22105=CYLINDRICAL_SURFACE ( 'NONE', #43304, 0.2499999999999986955 ) ;
#22106=CARTESIAN_POINT ( 'NONE',  ( 16.85404439449444070, -7.630691491037286056, 34.74850469731152458 ) ) ;
#22109=VERTEX_POINT ( 'NONE', #62268 ) ;
#22110=CARTESIAN_POINT ( 'NONE',  ( 1.384615384615265343, -6.026961402154118908, 34.52809138561165270 ) ) ;
#22111=CARTESIAN_POINT ( 'NONE',  ( 4.284371592079796898, -11.04252011169590020, 33.62494198852677840 ) ) ;
#22112=B_SPLINE_CURVE_WITH_KNOTS ( 'NONE', 3,
 ( #44596, #36537, #30222, #77958, #56795, #71192 ),
 .UNSPECIFIED., .F., .F.,
 ( 4, 2, 4 ),
 ( 0.0003909569690057848211, 0.0005862646681846116680, 0.0007815723673634385150 ),
 .UNSPECIFIED. ) ;
#22113=CARTESIAN_POINT ( 'NONE',  ( 0.3308478584281526191, -5.496505350115500121, 34.60290016733514307 ) ) ;
#22114=CARTESIAN_POINT ( 'NONE',  ( 9.627037691751372250, -6.835583212224499938, 34.95778746994557906 ) ) ;
#22117=CARTESIAN_POINT ( 'NONE',  ( 11.28843831424008215, -4.175268141568685643, 33.81360843649122216 ) ) ;
#22118=VERTEX_POINT ( 'NONE', #83900 ) ;
#22119=CARTESIAN_POINT ( 'NONE',  ( -0.4615384615384611200, -12.62096338111211580, 30.90682066428153263 ) ) ;
#22120=VECTOR ( 'NONE', #18973, 1000.000000000000227 ) ;
#22121=CARTESIAN_POINT ( 'NONE',  ( 14.05771557674995265, -3.137211980971221781, 32.19342716148376837 ) ) ;
#22123=EDGE_CURVE ( 'NONE', #77581, #25833, #63097, .T. ) ;
#22124=VERTEX_POINT ( 'NONE', #78006 ) ;
#22125=CARTESIAN_POINT ( 'NONE',  ( 14.30769230769218758, -2.892918686052165622, 31.69288490824153470 ) ) ;
#22126=CARTESIAN_POINT ( 'NONE',  ( -5.934806018216642443, -2.506253911140448487, 29.99999999999988631 ) ) ;
#22127=CARTESIAN_POINT ( 'NONE',  ( -8.519176349317316266, -5.642605341092957971, 34.66089969410670335 ) ) ;
#22128=CARTESIAN_POINT ( 'NONE',  ( -4.403822897894743349, -11.47974371597207899, 33.17467449705390692 ) ) ;
#22129=ORIENTED_EDGE ( 'NONE', *, *, #51942, .T. ) ;
#22130=CARTESIAN_POINT ( 'NONE',  ( -2.307692307692305711, -11.91647553114624181, 32.58852847137148245 ) ) ;
#22134=CARTESIAN_POINT ( 'NONE',  ( -3.903846153844716671, -7.500000000000155431, 34.75000000000007105 ) ) ;
#22135=VERTEX_POINT ( 'NONE', #16311 ) ;
#22136=EDGE_CURVE ( 'NONE', #42284, #42418, #87872, .T. ) ;
#22137=CARTESIAN_POINT ( 'NONE',  ( 10.86543903529806698, -11.47946981652013498, 33.17500667209847620 ) ) ;
#22138=CARTESIAN_POINT ( 'NONE',  ( -14.30769230769242917, -2.379036618888197729, 30.90682066428292885 ) ) ;
#22139=CARTESIAN_POINT ( 'NONE',  ( 1.134638653673032183, -4.236021600441998380, 33.53823185664189310 ) ) ;
#22140=CARTESIAN_POINT ( 'NONE',  ( -16.15384615384627409, -4.481592998941358097, 33.73612834414048933 ) ) ;
#22142=VECTOR ( 'NONE', #79090, 1000.000000000000227 ) ;
#22144=VERTEX_POINT ( 'NONE', #17189 ) ;
#22145=EDGE_CURVE ( 'NONE', #22188, #35493, #30121, .T. ) ;
#22146=FACE_BOUND ( 'NONE', #48797, .T. ) ;
#22148=CARTESIAN_POINT ( 'NONE',  ( -7.846153846153967493, -5.941354392335915335, 34.76329471203413846 ) ) ;
#22149=VECTOR ( 'NONE', #59790, 1000.000000000000000 ) ;
#22150=VECTOR ( 'NONE', #40314, 1000.000000000000114 ) ;
#22151=CARTESIAN_POINT ( 'NONE',  ( 4.376625695114563008, -11.89424750095246175, 32.13594075562311758 ) ) ;
#22152=CARTESIAN_POINT ( 'NONE',  ( 0.4615384615384611200, -1.242168528481310874, 33.36296068462461051 ) ) ;
#22153=CARTESIAN_POINT ( 'NONE',  ( 5.326977388561388693, -4.235687564193446164, 33.53795663066793509 ) ) ;
#22154=EDGE_LOOP ( 'NONE', ( #84362, #28961 ) ) ;
#22155=VERTEX_POINT ( 'NONE', #58614 ) ;
#22156=VERTEX_POINT ( 'NONE', #2771 ) ;
#22157=CARTESIAN_POINT ( 'NONE',  ( 6.000000000000001776, -8.973038597847269315, 34.52809138561121927 ) ) ;
#22158=ORIENTED_EDGE ( 'NONE', *, *, #11994, .T. ) ;
#22159=EDGE_CURVE ( 'NONE', #4801, #40289, #3058, .T. ) ;
#22160=CYLINDRICAL_SURFACE ( 'NONE', #24389, 0.2500000000000008882 ) ;
#22161=EDGE_CURVE ( 'NONE', #60044, #37672, #50524, .T. ) ;
#22162=CARTESIAN_POINT ( 'NONE',  ( 17.07692307692307665, -3.322132147404559976, 32.92929555188717927 ) ) ;
#22163=B_SPLINE_CURVE_WITH_KNOTS ( 'NONE', 3,
 ( #17658, #11335, #37465, #72588, #38817, #4581, #85226, #32055, #87023, #25296 ),
 .UNSPECIFIED., .F., .F.,
 ( 4, 2, 2, 2, 4 ),
 ( 0.0007817359527651133143, 0.0009771254036996530456, 0.001172514854634192777, 0.001367904305568732291, 0.001563293756503272023 ),
 .UNSPECIFIED. ) ;
#22164=CARTESIAN_POINT ( 'NONE',  ( 13.45068271796546533, -11.35647404775217595, 33.31231777344666511 ) ) ;
#22165=ORIENTED_EDGE ( 'NONE', *, *, #17549, .F. ) ;
#22166=DIRECTION ( 'NONE',  ( -0.000000000000000000, -0.8660254037844399289, -0.4999999999999980016 ) ) ;
#22167=EDGE_CURVE ( 'NONE', #35719, #70760, #71713, .T. ) ;
#22168=FACE_OUTER_BOUND ( 'NONE', #44826, .T. ) ;
#22169=EDGE_CURVE ( 'NONE', #26348, #18634, #18065, .T. ) ;
#22170=CARTESIAN_POINT ( 'NONE',  ( 4.023155550735848074, -2.494641256782728966, 31.33461815524612959 ) ) ;
#22171=CARTESIAN_POINT ( 'NONE',  ( -1.384615384615383471, -2.833524468853757305, 32.15551576947925838 ) ) ;
#22172=ORIENTED_EDGE ( 'NONE', *, *, #81922, .T. ) ;
#22173=VERTEX_POINT ( 'NONE', #17648 ) ;
#22174=EDGE_LOOP ( 'NONE', ( #81183, #49059, #74549, #63466 ) ) ;
#22175=CARTESIAN_POINT ( 'NONE',  ( 0.4615384615384611200, -11.16473453929635440, 33.15142922261926373 ) ) ;
#22176=VECTOR ( 'NONE', #8585, 1000.000000000000000 ) ;
#22177=CARTESIAN_POINT ( 'NONE',  ( -8.069638789877792817, -6.760086850603066466, 34.69517049084099369 ) ) ;
#22178=DIRECTION ( 'NONE',  ( -0.000000000000000000, -0.000000000000000000, -1.000000000000000000 ) ) ;
#22179=CARTESIAN_POINT ( 'NONE',  ( -17.86947456176635640, -5.915461855592775819, 34.75538340440931506 ) ) ;
#22180=CARTESIAN_POINT ( 'NONE',  ( -2.177166869458664777, -2.647132371071621471, 31.75357179365173010 ) ) ;
#22181=DIRECTION ( 'NONE',  ( -0.000000000000000000, -0.5000000000000009992, -0.8660254037844380415 ) ) ;
#22182=CARTESIAN_POINT ( 'NONE',  ( -6.989159302437057519, -3.322132147404559976, 32.92929555188719348 ) ) ;
#22183=EDGE_LOOP ( 'NONE', ( #77526, #11521, #60092, #853 ) ) ;
#22184=CARTESIAN_POINT ( 'NONE',  ( 17.20771351789002424, -11.93129842949672437, 32.56571108434900452 ) ) ;
#22185=CARTESIAN_POINT ( 'NONE',  ( -0.2114841499001460789, -9.148310452688873440, 34.47095581063188519 ) ) ;
#22188=VERTEX_POINT ( 'NONE', #45551 ) ;
#22189=CARTESIAN_POINT ( 'NONE',  ( -18.22348494372394967, -8.496056993536548418, 34.65000542017679663 ) ) ;
#22190=ORIENTED_EDGE ( 'NONE', *, *, #27955, .F. ) ;
#22191=FACE_BOUND ( 'NONE', #32289, .T. ) ;
#22193=CYLINDRICAL_SURFACE ( 'NONE', #83732, 0.2499999999999995559 ) ;
#22194=CARTESIAN_POINT ( 'NONE',  ( 9.692307692307695177, -13.95598074871891292, 31.83374038241031911 ) ) ;
#22196=CARTESIAN_POINT ( 'NONE',  ( 11.53846153846153832, -10.67929555188718282, 33.92786785259544047 ) ) ;
#22197=CARTESIAN_POINT ( 'NONE',  ( 15.45378207486262667, -2.308499170217967134, 30.53291367094873721 ) ) ;
#22198=CARTESIAN_POINT ( 'NONE',  ( 8.769230769230645706, -2.379036618888197729, 30.90682066428292885 ) ) ;
#22199=CARTESIAN_POINT ( 'NONE',  ( -17.93393266664992325, -12.62096338111211757, 30.90682066428152908 ) ) ;
#22200=ORIENTED_EDGE ( 'NONE', *, *, #85493, .T. ) ;
#22201=DIRECTION ( 'NONE',  ( -0.000000000000000000, -0.1736481776669307198, -0.9848077530122080203 ) ) ;
#22202=EDGE_LOOP ( 'NONE', ( #45301, #45243, #25848, #5142 ) ) ;
#22204=ORIENTED_EDGE ( 'NONE', *, *, #13906, .F. ) ;
#22205=CARTESIAN_POINT ( 'NONE',  ( -9.019230769230768274, -7.566083408709835645, 34.74999999999999289 ) ) ;
#22207=CARTESIAN_POINT ( 'NONE',  ( 7.622668921589517588, -10.23692288466677880, 34.23039457007281072 ) ) ;
#22208=ADVANCED_FACE ( 'NONE', ( #86562 ), #10887, .F. ) ;
#22209=CARTESIAN_POINT ( 'NONE',  ( -12.52680846209478460, -11.06231777344662781, 33.60647404775220082 ) ) ;
#22210=DIRECTION ( 'NONE',  ( -0.000000000000000000, -0.6427876096865404731, -0.7660444431189771253 ) ) ;
#22211=CARTESIAN_POINT ( 'NONE',  ( -11.66860950819323328, -9.504002272028875709, 34.60269587691767867 ) ) ;
#22212=CARTESIAN_POINT ( 'NONE',  ( 12.33092810191393518, -7.722926236386453702, 34.74524107206102030 ) ) ;
#22216=CIRCLE ( 'NONE', #85474, 0.2500000000000002220 ) ;
#22217=CARTESIAN_POINT ( 'NONE',  ( -0.7115151924808155171, -5.728515186090277211, 34.42611988154120439 ) ) ;
#22220=CARTESIAN_POINT ( 'NONE',  ( 11.53846153846153832, -11.69971097300155272, 32.46337939537588113 ) ) ;
#22221=EDGE_LOOP ( 'NONE', ( #24917, #50963, #73975, #87218 ) ) ;
#22222=DIRECTION ( 'NONE',  ( -1.000000000000000000, 0.000000000000000000, 0.000000000000000000 ) ) ;
#22223=CARTESIAN_POINT ( 'NONE',  ( -12.46153846153846168, -12.09954503811598769, 35.62045528018868623 ) ) ;
#22225=CARTESIAN_POINT ( 'NONE',  ( -7.846153846153844924, -1.509761064869970415, 31.06009739812519044 ) ) ;
#22226=LINE ( 'NONE', #36629, #61761 ) ;
#22227=CARTESIAN_POINT ( 'NONE',  ( 6.000000000000001776, -8.164416787775445883, 34.95778746994557906 ) ) ;
#22228=CARTESIAN_POINT ( 'NONE',  ( 7.173131234715237170, -11.28795663066794219, 33.01431243580653785 ) ) ;
#22229=CARTESIAN_POINT ( 'NONE',  ( 13.38461538461570122, -2.255955759149395501, 30.00000000000324363 ) ) ;
#22230=CYLINDRICAL_SURFACE ( 'NONE', #29026, 0.2499999999999995559 ) ;
#22231=CARTESIAN_POINT ( 'NONE',  ( 17.86985279056177944, -11.93770438780619259, 32.05411857736982029 ) ) ;
#22232=CARTESIAN_POINT ( 'NONE',  ( 8.068933387422255521, -2.847695495035523994, 31.58253572463339509 ) ) ;
#22234=ORIENTED_EDGE ( 'NONE', *, *, #71855, .F. ) ;
#22235=EDGE_CURVE ( 'NONE', #47910, #64424, #55698, .T. ) ;
#22236=VERTEX_POINT ( 'NONE', #33817 ) ;
#22237=CARTESIAN_POINT ( 'NONE',  ( 3.007284306204898172, -10.97335522853832579, 33.68706563782419749 ) ) ;
#22238=CARTESIAN_POINT ( 'NONE',  ( -3.099977422944445671, -2.729792928343269587, 31.24908615093345077 ) ) ;
#22239=CARTESIAN_POINT ( 'NONE',  ( 12.68431800280686694, -10.81320215134717344, 33.49497208177562868 ) ) ;
#22241=B_SPLINE_CURVE_WITH_KNOTS ( 'NONE', 3,
 ( #51729, #64804, #85103, #30153, #58947, #31484, #85542, #23384, #78328, #37791 ),
 .UNSPECIFIED., .F., .F.,
 ( 4, 2, 2, 2, 4 ),
 ( 0.000000000000000000, 0.0001954311564186860071, 0.0003908623128373720141, 0.0005862934692560580483, 0.0007817246256747440282 ),
 .UNSPECIFIED. ) ;
#22242=EDGE_CURVE ( 'NONE', #45697, #22109, #66400, .T. ) ;
#22243=DIRECTION ( 'NONE',  ( -0.000000000000000000, -0.8660254037844397068, -0.4999999999999978906 ) ) ;
#22244=CARTESIAN_POINT ( 'NONE',  ( -17.07692307692277112, -2.506253911140615021, 30.00000000000323297 ) ) ;
#22245=B_SPLINE_CURVE_WITH_KNOTS ( 'NONE', 3,
 ( #65068, #42604, #8372, #35845, #29099, #84043, #49788, #77264, #15573, #79494 ),
 .UNSPECIFIED., .F., .F.,
 ( 4, 2, 2, 2, 4 ),
 ( 0.000000000000000000, 0.0001954339857564081520, 0.0003908679715128163040, 0.0005863019572692244018, 0.0007817359430256326080 ),
 .UNSPECIFIED. ) ;
#22246=VECTOR ( 'NONE', #46352, 1000.000000000000227 ) ;
#22248=EDGE_LOOP ( 'NONE', ( #58696, #86216, #22909, #17075 ) ) ;
#22250=CARTESIAN_POINT ( 'NONE',  ( 0.4615384615384611200, -5.557115091759785130, 34.35708131394839171 ) ) ;
#22251=ORIENTED_EDGE ( 'NONE', *, *, #64648, .T. ) ;
#22253=EDGE_CURVE ( 'NONE', #72117, #29336, #34175, .T. ) ;
#22254=CARTESIAN_POINT ( 'NONE',  ( -17.07692307692319744, -3.643525952248796163, 33.31231777344771672 ) ) ;
#22255=CARTESIAN_POINT ( 'NONE',  ( -13.38461538461538325, -2.499999999999998668, 29.50000000000001066 ) ) ;
#22256=EDGE_CURVE ( 'NONE', #53989, #79559, #29877, .T. ) ;
#22257=CARTESIAN_POINT ( 'NONE',  ( 1.134638640566794976, -8.347322224742351082, 34.93158281831414769 ) ) ;
#22258=CARTESIAN_POINT ( 'NONE',  ( 18.06525513951284267, -8.656820664281605460, 34.87096338111211224 ) ) ;
#22259=ORIENTED_EDGE ( 'NONE', *, *, #85512, .T. ) ;
#22260=EDGE_LOOP ( 'NONE', ( #24263, #11826, #58781, #51664 ) ) ;
#22261=EDGE_LOOP ( 'NONE', ( #42222, #38678, #18372, #21411, #55351, #88422 ) ) ;
#22264=CARTESIAN_POINT ( 'NONE',  ( -17.32689980786543060, -10.66389620160130036, 33.62221079203477103 ) ) ;
#22265=CARTESIAN_POINT ( 'NONE',  ( 16.08776377448601735, -5.471508081941601986, 34.59228464037088457 ) ) ;
#22266=FACE_OUTER_BOUND ( 'NONE', #82543, .T. ) ;
#22267=EDGE_CURVE ( 'NONE', #4867, #7553, #78191, .T. ) ;
#22268=CARTESIAN_POINT ( 'NONE',  ( 17.01165307636676260, -10.33852847137145048, 34.16647553114627556 ) ) ;
#22269=B_SPLINE_CURVE_WITH_KNOTS ( 'NONE', 3,
 ( #49255, #75838, #47919, #14139, #69522, #54668, #1067, #56005, #6936, #83495 ),
 .UNSPECIFIED., .F., .F.,
 ( 4, 2, 2, 2, 4 ),
 ( 0.000000000000000000, 0.0001954311564186868202, 0.0003908623128373736404, 0.0005862934692560604335, 0.0007817246256747472808 ),
 .UNSPECIFIED. ) ;
#22270=CARTESIAN_POINT ( 'NONE',  ( 17.74997677577853850, -2.985938066672154889, 32.43141759479405550 ) ) ;
#22271=ADVANCED_FACE ( 'NONE', ( #21185 ), #83346, .F. ) ;
#22272=CARTESIAN_POINT ( 'NONE',  ( 4.153846153846154188, -2.486705287966279876, 31.30864560766543647 ) ) ;
#22274=B_SPLINE_CURVE_WITH_KNOTS ( 'NONE', 3,
 ( #26468, #66562, #53927, #86860, #25124, #75100, #74656, #81416, #12943, #26018 ),
 .UNSPECIFIED., .F., .F.,
 ( 4, 2, 2, 2, 4 ),
 ( 0.0007817246256747452209, 0.0009771112852218887673, 0.001172497944769032531, 0.001367884604316176294, 0.001563271263863319840 ),
 .UNSPECIFIED. ) ;
#22275=VERTEX_POINT ( 'NONE', #28845 ) ;
#22276=ORIENTED_EDGE ( 'NONE', *, *, #73716, .F. ) ;
#22277=CARTESIAN_POINT ( 'NONE',  ( 3.903869422903798903, -2.779195860258149686, 31.39871582349837453 ) ) ;
#22278=ORIENTED_EDGE ( 'NONE', *, *, #8956, .T. ) ;
#22279=CARTESIAN_POINT ( 'NONE',  ( -9.692307692307812417, -9.442884908241554243, 34.35708131394783038 ) ) ;
#22282=EDGE_LOOP ( 'NONE', ( #15669, #66769, #77324, #13741 ) ) ;
#22284=ORIENTED_EDGE ( 'NONE', *, *, #10156, .T. ) ;
#22285=CARTESIAN_POINT ( 'NONE',  ( 14.30769230769231015, -1.242168528481310874, 33.36296068462461051 ) ) ;
#22286=VERTEX_POINT ( 'NONE', #34259 ) ;
#22287=FACE_BOUND ( 'NONE', #47845, .T. ) ;
#22288=CARTESIAN_POINT ( 'NONE',  ( 5.011653076366756387, -5.094484230520674117, 34.41647553114621161 ) ) ;
#22290=ORIENTED_EDGE ( 'NONE', *, *, #55272, .F. ) ;
#22291=EDGE_CURVE ( 'NONE', #66107, #2951, #35299, .T. ) ;
#22292=CARTESIAN_POINT ( 'NONE',  ( 16.37685750545900376, -11.24521262558773493, 33.06293181088029343 ) ) ;
#22293=CARTESIAN_POINT ( 'NONE',  ( 16.15384615384615330, -8.318370150425687726, 35.83090037661290239 ) ) ;
#22294=DIRECTION ( 'NONE',  ( -0.000000000000000000, 0.000000000000000000, 1.000000000000000000 ) ) ;
#22296=CARTESIAN_POINT ( 'NONE',  ( 4.403791672194295792, -3.202959910592335202, 32.30730279482227019 ) ) ;
#22297=ORIENTED_EDGE ( 'NONE', *, *, #6437, .T. ) ;
#22299=CARTESIAN_POINT ( 'NONE',  ( -7.173100160369889622, -11.37209801155882971, 32.91403422569032955 ) ) ;
#22300=CARTESIAN_POINT ( 'NONE',  ( 2.084765348785460937, -11.98009711892699691, 32.48740034544075428 ) ) ;
#22301=CARTESIAN_POINT ( 'NONE',  ( -17.07692307692307665, -2.517432740324522911, 35.29906147534542527 ) ) ;
#22302=CARTESIAN_POINT ( 'NONE',  ( 1.384615384615386802, -13.75783147151868846, 33.36296068462461051 ) ) ;
#22303=DIRECTION ( 'NONE',  ( 0.000000000000000000, 0.3420201433256641055, -0.9396926207859100932 ) ) ;
#22304=EDGE_CURVE ( 'NONE', #82752, #34884, #481, .T. ) ;
#22305=CARTESIAN_POINT ( 'NONE',  ( -13.25408994638174498, -12.50538340440932394, 31.33453814440721885 ) ) ;
#22306=CARTESIAN_POINT ( 'NONE',  ( 13.16113044089144068, -11.89387501736622710, 32.13663884655806413 ) ) ;
#22307=DIRECTION ( 'NONE',  ( 0.000000000000000000, 0.7660444431189807890, 0.6427876096865361433 ) ) ;
#22308=CARTESIAN_POINT ( 'NONE',  ( 5.299935921016470708, -9.172514111537584114, 34.72667873470787470 ) ) ;
#22309=CARTESIAN_POINT ( 'NONE',  ( 8.769230769230768274, -9.780366693483667717, 34.19971097300155094 ) ) ;
#22310=CARTESIAN_POINT ( 'NONE',  ( -6.130147209438219669, -5.195881422630167279, 34.18770438780618548 ) ) ;
#22311=CARTESIAN_POINT ( 'NONE',  ( -5.776988648387149539, -12.39991518177334129, 30.74647679643404530 ) ) ;
#22313=EDGE_LOOP ( 'NONE', ( #38502, #12865, #1425, #764 ) ) ;
#22314=EDGE_CURVE ( 'NONE', #9486, #67330, #55417, .T. ) ;
#22316=VERTEX_POINT ( 'NONE', #63498 ) ;
#22317=EDGE_CURVE ( 'NONE', #55756, #5035, #35194, .T. ) ;
#22318=LINE ( 'NONE', #49781, #42123 ) ;
#22319=ORIENTED_EDGE ( 'NONE', *, *, #69620, .F. ) ;
#22320=CARTESIAN_POINT ( 'NONE',  ( 17.75002326905764960, -12.17611988154120795, 31.52148481390971213 ) ) ;
#22321=CARTESIAN_POINT ( 'NONE',  ( 17.32697749683652688, -2.920487667080175154, 32.31805714834170828 ) ) ;
#22322=EDGE_LOOP ( 'NONE', ( #45493, #67329 ) ) ;
#22323=CARTESIAN_POINT ( 'NONE',  ( -7.846153846153965716, -6.026961402154118019, 34.52809138561165270 ) ) ;
#22325=DIRECTION ( 'NONE',  ( 0.000000000000000000, 0.9848077530122072432, -0.1736481776669354937 ) ) ;
#22327=CYLINDRICAL_SURFACE ( 'NONE', #21604, 0.2499999999999993616 ) ;
#22328=EDGE_CURVE ( 'NONE', #13064, #59335, #2952, .T. ) ;
#22329=CARTESIAN_POINT ( 'NONE',  ( -5.300408020647024543, -12.44517049084099725, 30.48991314939691932 ) ) ;
#22330=CARTESIAN_POINT ( 'NONE',  ( 15.48076923077066702, -7.500000000000155431, 34.75000000000007105 ) ) ;
#22331=CARTESIAN_POINT ( 'NONE',  ( 4.946775867484856093, -8.587444163452046197, 34.63053765926554206 ) ) ;
#22333=AXIS2_PLACEMENT_3D ( 'NONE', #57191, #15330, #22520 ) ;
#22334=CARTESIAN_POINT ( 'NONE',  ( 11.40777093535123043, -5.496505350115501010, 34.60290016733514307 ) ) ;
#22335=CARTESIAN_POINT ( 'NONE',  ( -6.223484924564328225, -3.562934362175799841, 33.22335522853832401 ) ) ;
#22336=CARTESIAN_POINT ( 'NONE',  ( -7.846153846153844924, -1.117168528481311540, 33.14645433367849847 ) ) ;
#22338=B_SPLINE_CURVE_WITH_KNOTS ( 'NONE', 3,
 ( #84012, #77231, #2019, #58283, #52416, #39374, #72693, #80808, #86683, #65928 ),
 .UNSPECIFIED., .F., .F.,
 ( 4, 2, 2, 2, 4 ),
 ( 0.000000000000000000, 0.0001954339857564079352, 0.0003908679715128158703, 0.0005863019572692237513, 0.0007817359430256317406 ),
 .UNSPECIFIED. ) ;
#22339=DIRECTION ( 'NONE',  ( 0.000000000000000000, 0.7660444431189822323, -0.6427876096865344779 ) ) ;
#22340=EDGE_LOOP ( 'NONE', ( #16952, #46080 ) ) ;
#22341=DIRECTION ( 'NONE',  ( -0.000000000000000000, -0.1736481776669307198, -0.9848077530122080203 ) ) ;
#22342=CARTESIAN_POINT ( 'NONE',  ( -11.31568199719312773, -8.496831190052096971, 34.64984203495476578 ) ) ;
#22343=CARTESIAN_POINT ( 'NONE',  ( 23.00000000000000000, -4.249999999999998224, 27.25000000000000000 ) ) ;
#22344=CARTESIAN_POINT ( 'NONE',  ( -14.30769230769242739, -11.94971097300221174, 32.03036669348237098 ) ) ;
#22345=EDGE_CURVE ( 'NONE', #31805, #59859, #69383, .T. ) ;
#22347=DIRECTION ( 'NONE',  ( -0.000000000000000000, 0.9396926207859092051, -0.3420201433256662704 ) ) ;
#22348=B_SPLINE_CURVE_WITH_KNOTS ( 'NONE', 3,
 ( #20315, #67168, #82021, #60846, #53647, #34262, #61721, #38, #19420, #20746 ),
 .UNSPECIFIED., .F., .F.,
 ( 4, 2, 2, 2, 4 ),
 ( 0.000000000000000000, 0.0001954311564186871184, 0.0003908623128373742367, 0.0005862934692560614093, 0.0007817246256747484735 ),
 .UNSPECIFIED. ) ;
#22350=EDGE_LOOP ( 'NONE', ( #61326, #16653 ) ) ;
#22351=VERTEX_POINT ( 'NONE', #82466 ) ;
#22352=ORIENTED_EDGE ( 'NONE', *, *, #11365, .F. ) ;
#22353=CARTESIAN_POINT ( 'NONE',  ( -9.626239341305252495, -3.050289026998446840, 32.03036669348366416 ) ) ;
#22354=CARTESIAN_POINT ( 'NONE',  ( -3.903900635498011695, -3.202959910592335202, 32.30730279482228440 ) ) ;
#22355=CARTESIAN_POINT ( 'NONE',  ( 6.923076923076800782, -3.083524468854526912, 32.58852847137268327 ) ) ;
#22356=CARTESIAN_POINT ( 'NONE',  ( 1.449870955891410462, -11.94971097300157403, 32.03036669348361443 ) ) ;
#22357=CARTESIAN_POINT ( 'NONE',  ( -5.076923076923197442, -6.879047030192662504, 34.71129190930017927 ) ) ;
#22358=VECTOR ( 'NONE', #59218, 1000.000000000000000 ) ;
#22359=ORIENTED_EDGE ( 'NONE', *, *, #57218, .T. ) ;
#22360=DIRECTION ( 'NONE',  ( 0.000000000000000000, 0.4999999999999960032, -0.8660254037844410391 ) ) ;
#22361=ORIENTED_EDGE ( 'NONE', *, *, #55475, .F. ) ;
#22362=B_SPLINE_CURVE_WITH_KNOTS ( 'NONE', 3,
 ( #27604, #45315, #39030, #11547, #88889, #17862 ),
 .UNSPECIFIED., .F., .F.,
 ( 4, 2, 4 ),
 ( 0.0003909569690057790748, 0.0005862646681846022355, 0.0007815723673634252877 ),
 .UNSPECIFIED. ) ;
#22363=EDGE_LOOP ( 'NONE', ( #12663, #76235 ) ) ;
#22364=EDGE_CURVE ( 'NONE', #48597, #67515, #47081, .T. ) ;
#22365=CARTESIAN_POINT ( 'NONE',  ( 4.376858997939547358, -12.38742843783360748, 31.66772728687926985 ) ) ;
#22366=ORIENTED_EDGE ( 'NONE', *, *, #68440, .T. ) ;
#22367=DIRECTION ( 'NONE',  ( -0.000000000000000000, 0.5000000000000011102, -0.8660254037844381525 ) ) ;
#22368=CARTESIAN_POINT ( 'NONE',  ( -10.68146802634049308, -4.786620604624113540, 33.94971097300155805 ) ) ;
#22369=EDGE_CURVE ( 'NONE', #41563, #52736, #14783, .T. ) ;
#22371=EDGE_CURVE ( 'NONE', #37367, #35211, #14882, .T. ) ;
#22372=CARTESIAN_POINT ( 'NONE',  ( -12.39634447975510412, -2.506253911140448487, 29.99999999999988631 ) ) ;
#22373=ORIENTED_EDGE ( 'NONE', *, *, #31738, .T. ) ;
#22375=ORIENTED_EDGE ( 'NONE', *, *, #73003, .T. ) ;
#22376=CARTESIAN_POINT ( 'NONE',  ( -6.700297254098856570, -3.020022701398814569, 32.48759521482552515 ) ) ;
#22377=CARTESIAN_POINT ( 'NONE',  ( 11.78840694783958298, -5.766571408460171355, 34.70601412856602508 ) ) ;
#22378=ORIENTED_EDGE ( 'NONE', *, *, #49714, .T. ) ;
#22379=EDGE_CURVE ( 'NONE', #72548, #63925, #77087, .T. ) ;
#22380=CARTESIAN_POINT ( 'NONE',  ( 1.384615384615386802, -8.973038597847269315, 34.52809138561121927 ) ) ;
#22382=VECTOR ( 'NONE', #37687, 1000.000000000000227 ) ;
#22383=CARTESIAN_POINT ( 'NONE',  ( 2.530705151785704654, -9.172514111537584114, 34.72667873470787470 ) ) ;
#22384=VERTEX_POINT ( 'NONE', #16637 ) ;
#22385=CARTESIAN_POINT ( 'NONE',  ( -8.769230769230892619, -5.941354392335915335, 34.76329471203413846 ) ) ;
#22386=EDGE_CURVE ( 'NONE', #41905, #72231, #19021, .T. ) ;
#22387=FACE_OUTER_BOUND ( 'NONE', #87508, .T. ) ;
#22388=ORIENTED_EDGE ( 'NONE', *, *, #20221, .T. ) ;
#22389=FACE_BOUND ( 'NONE', #7673, .T. ) ;
#22390=CARTESIAN_POINT ( 'NONE',  ( -11.60454391782167249, -11.35647404775217595, 33.31231777344666511 ) ) ;
#22391=CARTESIAN_POINT ( 'NONE',  ( 2.307692307692309264, -11.35647404775217417, 33.31231777344666511 ) ) ;
#22392=CARTESIAN_POINT ( 'NONE',  ( 9.692307692307695177, -2.721908614388771852, 31.22303859784724978 ) ) ;
#22394=CARTESIAN_POINT ( 'NONE',  ( 15.16551929899514484, -2.255955759149247619, 30.00000000000013856 ) ) ;
#22395=FACE_OUTER_BOUND ( 'NONE', #83525, .T. ) ;
#22396=CARTESIAN_POINT ( 'NONE',  ( -16.02305434602136103, -8.999086150933472084, 34.52020707165672064 ) ) ;
#22397=ORIENTED_EDGE ( 'NONE', *, *, #35675, .F. ) ;
#22398=CYLINDRICAL_SURFACE ( 'NONE', #86415, 0.2499999999999995559 ) ;
#22399=B_SPLINE_CURVE_WITH_KNOTS ( 'NONE', 3,
 ( #12859, #47967, #61045, #75450, #14189, #88547, #55170, #26824, #82668, #75018 ),
 .UNSPECIFIED., .F., .F.,
 ( 4, 2, 2, 2, 4 ),
 ( 0.000000000000000000, 0.0001954311564186870913, 0.0003908623128373741825, 0.0005862934692560613009, 0.0007817246256747483650 ),
 .UNSPECIFIED. ) ;
#22403=CARTESIAN_POINT ( 'NONE',  ( 7.053602624840485724, -2.882268652242224505, 31.66798894389554064 ) ) ;
#22404=CARTESIAN_POINT ( 'NONE',  ( 8.639083559792549494, -3.285722584762969856, 32.44110544564090759 ) ) ;
#22405=LINE ( 'NONE', #83683, #52595 ) ;
#22406=CARTESIAN_POINT ( 'NONE',  ( -7.596208436775802930, -10.92531984108285670, 33.72920026020278073 ) ) ;
#22407=FACE_OUTER_BOUND ( 'NONE', #46193, .T. ) ;
#22408=CARTESIAN_POINT ( 'NONE',  ( 4.284371855609715674, -10.19071101563364401, 33.96452234770658407 ) ) ;
#22409=FACE_BOUND ( 'NONE', #64098, .T. ) ;
#22410=CARTESIAN_POINT ( 'NONE',  ( -2.530618525208451874, -6.503392248772476236, 34.64988816332204635 ) ) ;
#22413=CYLINDRICAL_SURFACE ( 'NONE', #50130, 0.2500000000000008882 ) ;
#22414=DIRECTION ( 'NONE',  ( -0.000000000000000000, 0.7660444431189791237, -0.6427876096865379196 ) ) ;
#22415=CARTESIAN_POINT ( 'NONE',  ( -3.230769230769229949, -13.37000171582298513, 34.34916445242398453 ) ) ;
#22417=EDGE_LOOP ( 'NONE', ( #69569, #83697 ) ) ;
#22418=ADVANCED_FACE ( 'NONE', ( #51735 ), #4004, .F. ) ;
#22419=ORIENTED_EDGE ( 'NONE', *, *, #78418, .T. ) ;
#22420=CYLINDRICAL_SURFACE ( 'NONE', #88114, 0.2500000000000012212 ) ;
#22421=VECTOR ( 'NONE', #6273, 1000.000000000000114 ) ;
#22422=CARTESIAN_POINT ( 'NONE',  ( -12.39547112818838670, -6.343179335718452272, 34.87096338111212646 ) ) ;
#22423=CARTESIAN_POINT ( 'NONE',  ( -7.623141002060450866, -11.43677907613345113, 33.22367315496201456 ) ) ;
#22424=DIRECTION ( 'NONE',  ( 0.000000000000000000, 0.3420201433256641055, -0.9396926207859100932 ) ) ;
#22425=CARTESIAN_POINT ( 'NONE',  ( -17.07692307692319744, -6.879047030192662504, 34.71129190930017927 ) ) ;
#22427=CARTESIAN_POINT ( 'NONE',  ( 11.53846153846153832, -2.486705287966279876, 31.30864560766543647 ) ) ;
#22428=CARTESIAN_POINT ( 'NONE',  ( 18.06525557127601900, -3.300289026998473929, 32.46337939537591666 ) ) ;
#22429=VECTOR ( 'NONE', #42731, 1000.000000000000227 ) ;
#22430=EDGE_CURVE ( 'NONE', #83085, #47709, #10403, .T. ) ;
#22431=CARTESIAN_POINT ( 'NONE',  ( 6.250054419913453785, -4.074993327901525575, 33.72946981652012255 ) ) ;
#22432=CARTESIAN_POINT ( 'NONE',  ( -1.450698795571264021, -12.37446782046654192, 30.86335684631486487 ) ) ;
#22434=CARTESIAN_POINT ( 'NONE',  ( 3.903822916553187028, -10.76384336483936011, 33.53834819971076087 ) ) ;
#22435=DIRECTION ( 'NONE',  ( -0.000000000000000000, -0.3420201433256694346, -0.9396926207859080948 ) ) ;
#22436=EDGE_CURVE ( 'NONE', #22716, #59465, #17087, .T. ) ;
#22437=CARTESIAN_POINT ( 'NONE',  ( 14.30769230769231015, -6.386643153685126251, 34.62446782046654192 ) ) ;
#22439=CARTESIAN_POINT ( 'NONE',  ( 2.307692307692186251, -3.643525952248796163, 33.31231777344771672 ) ) ;
#22440=CARTESIAN_POINT ( 'NONE',  ( 7.716005876422150855, -5.070767119584671079, 34.40440758774516183 ) ) ;
#22442=FACE_OUTER_BOUND ( 'NONE', #28458, .T. ) ;
#22443=CARTESIAN_POINT ( 'NONE',  ( -15.90390074446811042, -2.589246495874658827, 31.60778113518102828 ) ) ;
#22444=ORIENTED_EDGE ( 'NONE', *, *, #14227, .T. ) ;
#22445=CARTESIAN_POINT ( 'NONE',  ( -9.942330916529147800, -5.765609946408404518, 34.70566812827425451 ) ) ;
#22446=CARTESIAN_POINT ( 'NONE',  ( 12.33139125210024112, -6.001485441113819874, 34.52039167877662607 ) ) ;
#22447=ORIENTED_EDGE ( 'NONE', *, *, #20649, .F. ) ;
#22448=CARTESIAN_POINT ( 'NONE',  ( 7.846153846153725020, -3.835265460704628371, 33.15142922262033665 ) ) ;
#22449=CARTESIAN_POINT ( 'NONE',  ( -9.469528023329626620, -5.827830569534417471, 34.72679350104403539 ) ) ;
#22450=EDGE_CURVE ( 'NONE', #20857, #55599, #43732, .T. ) ;
#22451=EDGE_LOOP ( 'NONE', ( #36589, #43977, #80326, #72907 ) ) ;
#22452=CARTESIAN_POINT ( 'NONE',  ( -13.38461538461538325, -2.538708090699994813, 30.37095296980875503 ) ) ;
#22453=CARTESIAN_POINT ( 'NONE',  ( -13.60754160213153163, -3.105860786376062332, 32.13614157043599562 ) ) ;
#22454=VERTEX_POINT ( 'NONE', #73828 ) ;
#22455=CARTESIAN_POINT ( 'NONE',  ( -12.52680846209478460, -2.379036618887870436, 30.90682066428147934 ) ) ;
#22456=EDGE_CURVE ( 'NONE', #32510, #5283, #63013, .T. ) ;
#22458=CARTESIAN_POINT ( 'NONE',  ( 5.300298562695495264, -2.251407671071270489, 29.88021292934942252 ) ) ;
#22459=AXIS2_PLACEMENT_3D ( 'NONE', #11911, #31280, #32609 ) ;
#22460=CARTESIAN_POINT ( 'NONE',  ( -1.384615384615505151, -12.46129190930018460, 30.37095296980731973 ) ) ;
#22462=ORIENTED_EDGE ( 'NONE', *, *, #27265, .T. ) ;
#22464=ORIENTED_EDGE ( 'NONE', *, *, #77994, .T. ) ;
#22465=CARTESIAN_POINT ( 'NONE',  ( -1.384615384615383471, -2.538708090699994813, 30.37095296980875503 ) ) ;
#22466=CARTESIAN_POINT ( 'NONE',  ( -14.30769230769230660, -3.050289026998446396, 32.03036669348365706 ) ) ;
#22467=AXIS2_PLACEMENT_3D ( 'NONE', #7745, #77525, #77086 ) ;
#22468=CARTESIAN_POINT ( 'NONE',  ( -4.023055712879202162, -12.62708834333097663, 30.88030960425257021 ) ) ;
#22469=CARTESIAN_POINT ( 'NONE',  ( 3.100621261037536769, -10.31621877034669588, 34.18098118002070152 ) ) ;
#22470=EDGE_LOOP ( 'NONE', ( #51425, #18029, #84315, #42993 ) ) ;
#22471=EDGE_LOOP ( 'NONE', ( #55650, #60746, #81219, #46721 ) ) ;
#22472=CARTESIAN_POINT ( 'NONE',  ( -2.557692307692305267, -7.500000000000001776, 35.00000000000000000 ) ) ;
#22473=ORIENTED_EDGE ( 'NONE', *, *, #759, .T. ) ;
#22474=B_SPLINE_CURVE_WITH_KNOTS ( 'NONE', 3,
 ( #46677, #74154, #88139, #6584, #67838, #33612, #87685, #26853, #20533, #68723 ),
 .UNSPECIFIED., .F., .F.,
 ( 4, 2, 2, 2, 4 ),
 ( 0.0007817246256747528103, 0.0009771112852218980915, 0.001172497944769043156, 0.001367884604316188437, 0.001563271263863333718 ),
 .UNSPECIFIED. ) ;
#22475=B_SPLINE_CURVE_WITH_KNOTS ( 'NONE', 3,
 ( #1277, #34629, #28767, #54901, #20667, #55775, #83717, #36406, #62097, #89153 ),
 .UNSPECIFIED., .F., .F.,
 ( 4, 2, 2, 2, 4 ),
 ( 0.000000000000000000, 0.0001954339857564070136, 0.0003908679715128140272, 0.0005863019572692210407, 0.0007817359430256280543 ),
 .UNSPECIFIED. ) ;
#22479=AXIS2_PLACEMENT_3D ( 'NONE', #72067, #4044, #31534 ) ;
#22480=CARTESIAN_POINT ( 'NONE',  ( 0.4615384615384611200, -6.386643153685126251, 34.62446782046654192 ) ) ;
#22481=CARTESIAN_POINT ( 'NONE',  ( 6.792386319966616348, -9.084618155246140248, 34.75535874321725771 ) ) ;
#22482=VERTEX_POINT ( 'NONE', #26520 ) ;
#22483=AXIS2_PLACEMENT_3D ( 'NONE', #31090, #78838, #58560 ) ;
#22484=ORIENTED_EDGE ( 'NONE', *, *, #41256, .F. ) ;
#22485=CARTESIAN_POINT ( 'NONE',  ( -12.33101275977490197, -5.195472089885680766, 34.18748526763464923 ) ) ;
#22486=VERTEX_POINT ( 'NONE', #25626 ) ;
#22487=ADVANCED_FACE ( 'NONE', ( #54420 ), #81473, .F. ) ;
#22488=CARTESIAN_POINT ( 'NONE',  ( -0.6850234052624101233, -10.81261337010820256, 33.49550067578627477 ) ) ;
#22489=CARTESIAN_POINT ( 'NONE',  ( -5.076923076923197442, -10.21337939537710326, 33.94971097300076224 ) ) ;
#22490=EDGE_LOOP ( 'NONE', ( #46201, #35875 ) ) ;
#22491=CARTESIAN_POINT ( 'NONE',  ( 15.29602480204525605, -3.300289026998473041, 32.46337939537591666 ) ) ;
#22492=CARTESIAN_POINT ( 'NONE',  ( 5.299702618191482806, -11.41317474335729187, 32.86274602512330034 ) ) ;
#22493=EDGE_CURVE ( 'NONE', #27221, #9934, #12641, .T. ) ;
#22494=CARTESIAN_POINT ( 'NONE',  ( 6.699591998512595126, -5.827078755546623690, 34.72654668319379567 ) ) ;
#22495=FACE_BOUND ( 'NONE', #20159, .T. ) ;
#22496=CARTESIAN_POINT ( 'NONE',  ( 8.068933515131915257, -12.47679350104403007, 31.42216943046555855 ) ) ;
#22497=DIRECTION ( 'NONE',  ( -0.000000000000000000, 0.9848077530122086864, -0.1736481776669273891 ) ) ;
#22499=CARTESIAN_POINT ( 'NONE',  ( 12.33084785842815378, -3.338472653186243644, 32.95098750199972670 ) ) ;
#22500=CARTESIAN_POINT ( 'NONE',  ( -5.749945688361684404, -2.779044189368096163, 31.39831045268886456 ) ) ;
#22501=CARTESIAN_POINT ( 'NONE',  ( -11.28851602011339672, -3.202959910592335646, 32.30730279482227019 ) ) ;
#22502=CYLINDRICAL_SURFACE ( 'NONE', #87967, 0.2499999999999995559 ) ;
#22503=EDGE_LOOP ( 'NONE', ( #8972, #56902 ) ) ;
#22504=CARTESIAN_POINT ( 'NONE',  ( 17.07692307692307665, -7.500000000000001776, 35.04278698407183867 ) ) ;
#22505=EDGE_LOOP ( 'NONE', ( #69906, #76969, #67721, #26861 ) ) ;
#22506=VERTEX_POINT ( 'NONE', #53081 ) ;
#22507=LINE ( 'NONE', #63926, #63353 ) ;
#22508=CARTESIAN_POINT ( 'NONE',  ( -6.923076923076922462, -11.91647553114624181, 32.58852847137148245 ) ) ;
#22510=B_SPLINE_CURVE_WITH_KNOTS ( 'NONE', 3,
 ( #47759, #41011, #6769, #34243, #87000, #8998, #56731, #28369, #70693, #34694 ),
 .UNSPECIFIED., .F., .F.,
 ( 4, 2, 2, 2, 4 ),
 ( 0.0007817246256747473893, 0.0009771112852218905021, 0.001172497944769033615, 0.001367884604316176944, 0.001563271263863320057 ),
 .UNSPECIFIED. ) ;
#22511=CARTESIAN_POINT ( 'NONE',  ( -6.923076923077044142, -6.879047030192662504, 34.71129190930017927 ) ) ;
#22512=DIRECTION ( 'NONE',  ( -0.000000000000000000, 0.7660444431189792347, -0.6427876096865379196 ) ) ;
#22513=CARTESIAN_POINT ( 'NONE',  ( 15.23076923076923173, -3.513871655860378418, 32.76840700105978499 ) ) ;
#22514=CARTESIAN_POINT ( 'NONE',  ( -3.903791733932699515, -3.435999193479609914, 33.07426656108010832 ) ) ;
#22516=VECTOR ( 'NONE', #5706, 1000.000000000000114 ) ;
#22517=CARTESIAN_POINT ( 'NONE',  ( 11.40777093535123043, -3.338472653186243644, 32.95098750199972670 ) ) ;
#22518=CARTESIAN_POINT ( 'NONE',  ( 1.607626736228236597, -12.15243808032445827, 31.58219941686247978 ) ) ;
#22519=CYLINDRICAL_SURFACE ( 'NONE', #15775, 0.2499999999999986955 ) ;
#22520=DIRECTION ( 'NONE',  ( 0.000000000000000000, -6.938893903907222067E-15, 1.000000000000000000 ) ) ;
#22523=ORIENTED_EDGE ( 'NONE', *, *, #88970, .F. ) ;
#22524=ORIENTED_EDGE ( 'NONE', *, *, #9216, .F. ) ;
#22525=CARTESIAN_POINT ( 'NONE',  ( -7.146003140593069958, -8.239355502252617924, 34.69524867566427417 ) ) ;
#22526=ADVANCED_FACE ( 'NONE', ( #33717 ), #61173, .F. ) ;
#22527=ORIENTED_EDGE ( 'NONE', *, *, #53597, .F. ) ;
#22528=CIRCLE ( 'NONE', #67103, 0.2500000000000002220 ) ;
#22529=CARTESIAN_POINT ( 'NONE',  ( -1.319359813339359588, -8.613356846314930593, 34.62446782046653482 ) ) ;
#22530=CARTESIAN_POINT ( 'NONE',  ( -1.161602540521989191, -10.01129605718032778, 34.36064277460058491 ) ) ;
#22531=DIRECTION ( 'NONE',  ( -0.000000000000000000, 1.000000000000000000, 3.491481338843133355E-15 ) ) ;
#22532=CARTESIAN_POINT ( 'NONE',  ( -4.946397638689431275, -3.625058011473227815, 33.29252011169590020 ) ) ;
#22534=CARTESIAN_POINT ( 'NONE',  ( 6.000000000000001776, -3.669653830205710676, 35.88435417666054406 ) ) ;
#22535=ORIENTED_EDGE ( 'NONE', *, *, #86640, .T. ) ;
#22536=CARTESIAN_POINT ( 'NONE',  ( 1.384615384615386802, -13.37000171582298513, 34.34916445242398453 ) ) ;
#22537=CARTESIAN_POINT ( 'NONE',  ( -2.057637996053991447, -10.66356715214248396, 33.62249196103329751 ) ) ;
#22539=CARTESIAN_POINT ( 'NONE',  ( -18.00000000000000000, -12.75000000000000888, 29.74999999999997868 ) ) ;
#22540=FACE_OUTER_BOUND ( 'NONE', #69956, .T. ) ;
#22541=CARTESIAN_POINT ( 'NONE',  ( 11.31553532094539172, -4.186968288167450147, 33.49512374952580274 ) ) ;
#22542=CARTESIAN_POINT ( 'NONE',  ( 9.692307692307695177, -8.564572088678739092, 35.78748833219616898 ) ) ;
#22543=ADVANCED_FACE ( 'NONE', ( #60292 ), #87801, .F. ) ;
#22544=EDGE_CURVE ( 'NONE', #5084, #30133, #52645, .T. ) ;
#22545=CYLINDRICAL_SURFACE ( 'NONE', #79536, 0.2500000000000008882 ) ;
#22546=CARTESIAN_POINT ( 'NONE',  ( -7.976301055592065481, -12.45813303252208648, 30.39737893381572675 ) ) ;
#22548=VERTEX_POINT ( 'NONE', #45889 ) ;
#22549=DIRECTION ( 'NONE',  ( 0.000000000000000000, 0.3420201433256610524, 0.9396926207859113145 ) ) ;
#22550=DIRECTION ( 'NONE',  ( 0.000000000000000000, -6.938893903907222067E-15, 1.000000000000000000 ) ) ;
#22552=CARTESIAN_POINT ( 'NONE',  ( 13.38461538461526601, -6.879047030192662504, 34.71129190930017927 ) ) ;
#22554=LINE ( 'NONE', #2705, #15977 ) ;
#22555=ORIENTED_EDGE ( 'NONE', *, *, #3732, .T. ) ;
#22557=FACE_OUTER_BOUND ( 'NONE', #9128, .T. ) ;
#22558=ORIENTED_EDGE ( 'NONE', *, *, #10639, .T. ) ;
#22559=AXIS2_PLACEMENT_3D ( 'NONE', #4706, #10568, #80374 ) ;
#22560=CARTESIAN_POINT ( 'NONE',  ( 14.08420736396836226, -3.236172620538810385, 32.36188796281390267 ) ) ;
#22561=EDGE_LOOP ( 'NONE', ( #75368, #10279 ) ) ;
#22562=CARTESIAN_POINT ( 'NONE',  ( 7.146089767170319185, -4.026326845037961455, 33.68677907613344047 ) ) ;
#22563=ADVANCED_FACE ( 'NONE', ( #11677 ), #20206, .F. ) ;
#22564=CARTESIAN_POINT ( 'NONE',  ( -17.07692307692307665, -2.292212530054420494, 30.41441678777542634 ) ) ;
#22565=CARTESIAN_POINT ( 'NONE',  ( -12.68502338610279168, -10.23692288466677880, 34.23039457007281072 ) ) ;
#22566=CARTESIAN_POINT ( 'NONE',  ( -13.16183571563731647, -12.69155399931963046, 30.53255429739157734 ) ) ;
#22567=VERTEX_POINT ( 'NONE', #80587 ) ;
#22568=CARTESIAN_POINT ( 'NONE',  ( -2.373774687052441212, -11.91647553114624181, 32.58852847137148245 ) ) ;
#22569=ORIENTED_EDGE ( 'NONE', *, *, #87668, .T. ) ;
#22570=CARTESIAN_POINT ( 'NONE',  ( 12.23861150263161335, -11.98009711892699514, 32.48740034544076138 ) ) ;
#22571=CARTESIAN_POINT ( 'NONE',  ( -4.376672846325156740, -7.369208160676172348, 34.74850200257122879 ) ) ;
#22572=ORIENTED_EDGE ( 'NONE', *, *, #12433, .F. ) ;
#22573=CARTESIAN_POINT ( 'NONE',  ( 8.545745844666436497, -4.988325925672468131, 34.36044203135681130 ) ) ;
#22574=CARTESIAN_POINT ( 'NONE',  ( -14.43838377435986686, -10.54014554554150607, 33.71984207302941883 ) ) ;
#22575=B_SPLINE_CURVE_WITH_KNOTS ( 'NONE', 3,
 ( #17505, #12095, #24701, #66586, #65235, #32797 ),
 .UNSPECIFIED., .F., .F.,
 ( 4, 2, 4 ),
 ( 0.0003909512603273676860, 0.0005862562993131928890, 0.0007815613382990180920 ),
 .UNSPECIFIED. ) ;
#22576=CARTESIAN_POINT ( 'NONE',  ( -11.78843828251013015, -2.920706130388546651, 32.31842814019191223 ) ) ;
#22577=CARTESIAN_POINT ( 'NONE',  ( 13.44987052412822059, -12.16647553114626490, 32.15551576947920864 ) ) ;
#22578=CARTESIAN_POINT ( 'NONE',  ( -18.25002323729296450, -4.335965774309649134, 33.62209801155881905 ) ) ;
#22581=EDGE_LOOP ( 'NONE', ( #73209, #82308, #44962, #34975 ) ) ;
#22582=FACE_BOUND ( 'NONE', #68791, .T. ) ;
#22583=ORIENTED_EDGE ( 'NONE', *, *, #56395, .T. ) ;
#22584=CARTESIAN_POINT ( 'NONE',  ( 14.98074599347626368, -12.43535235679832596, 30.55408501211184813 ) ) ;
#22585=AXIS2_PLACEMENT_3D ( 'NONE', #14603, #1088, #28567 ) ;
#22586=DIRECTION ( 'NONE',  ( -1.000000000000000000, 0.000000000000000000, 0.000000000000000000 ) ) ;
#22587=VECTOR ( 'NONE', #89065, 999.9999999999998863 ) ;
#22588=CARTESIAN_POINT ( 'NONE',  ( 13.51540719244017374, -10.54018710029568595, 33.71981072465678864 ) ) ;
#22589=CARTESIAN_POINT ( 'NONE',  ( 13.38461538461538680, -11.11383981884818262, 36.00935417666054406 ) ) ;
#22590=EDGE_LOOP ( 'NONE', ( #26650, #48300, #52477, #84269 ) ) ;
#22591=ORIENTED_EDGE ( 'NONE', *, *, #87751, .F. ) ;
#22592=ORIENTED_EDGE ( 'NONE', *, *, #74131, .T. ) ;
#22594=DIRECTION ( 'NONE',  ( 0.000000000000000000, 0.3420201433256610524, 0.9396926207859113145 ) ) ;
#22597=ORIENTED_EDGE ( 'NONE', *, *, #41255, .F. ) ;
#22598=CARTESIAN_POINT ( 'NONE',  ( 16.21910129335899597, -2.379036618887895305, 30.90682066428158592 ) ) ;
#22599=CARTESIAN_POINT ( 'NONE',  ( -6.065270000556318486, -6.835583212224499938, 34.95778746994557906 ) ) ;
#22601=CARTESIAN_POINT ( 'NONE',  ( -18.12796115882773407, -7.725261176542461250, 34.99539040900690168 ) ) ;
#22602=CARTESIAN_POINT ( 'NONE',  ( -1.161602540521988747, -2.889357225399415086, 32.26129605718031002 ) ) ;
#22603=ORIENTED_EDGE ( 'NONE', *, *, #32392, .T. ) ;
#22604=B_SPLINE_CURVE_WITH_KNOTS ( 'NONE', 3,
 ( #31643, #23109, #59104, #66311, #86605, #24875, #45592, #64967, #73071, #38849 ),
 .UNSPECIFIED., .F., .F.,
 ( 4, 2, 2, 2, 4 ),
 ( 0.000000000000000000, 0.0001954311564186867389, 0.0003908623128373734778, 0.0005862934692560602167, 0.0007817246256747469556 ),
 .UNSPECIFIED. ) ;
#22605=ORIENTED_EDGE ( 'NONE', *, *, #57181, .F. ) ;
#22606=VERTEX_POINT ( 'NONE', #32386 ) ;
#22607=CARTESIAN_POINT ( 'NONE',  ( 12.23861224402231151, -6.503392248772476236, 34.64988816332204635 ) ) ;
#22608=CARTESIAN_POINT ( 'NONE',  ( -13.38461538461550582, -6.026961402154118019, 34.52809138561165270 ) ) ;
#22609=CYLINDRICAL_SURFACE ( 'NONE', #18343, 0.2499999999999986955 ) ;
#22610=DIRECTION ( 'NONE',  ( -0.000000000000000000, -0.1736481776669307198, -0.9848077530122080203 ) ) ;
#22611=FACE_BOUND ( 'NONE', #73477, .T. ) ;
#22612=CARTESIAN_POINT ( 'NONE',  ( -15.23076923076922995, -3.322132147404559976, 32.92929555188717927 ) ) ;
#22613=VERTEX_POINT ( 'NONE', #18870 ) ;
#22614=CARTESIAN_POINT ( 'NONE',  ( 17.29970261819148902, -10.81320215134717166, 33.49497208177562868 ) ) ;
#22616=CARTESIAN_POINT ( 'NONE',  ( 9.626225312947559232, -11.91647553114624181, 32.58852847137148245 ) ) ;
#22617=CARTESIAN_POINT ( 'NONE',  ( 11.28846153846153832, -7.500000000000001776, 34.75000000000000000 ) ) ;
#22618=CARTESIAN_POINT ( 'NONE',  ( -11.28851602011339494, -3.712312575010499049, 33.01462480002815170 ) ) ;
#22619=ORIENTED_EDGE ( 'NONE', *, *, #49941, .F. ) ;
#22620=CARTESIAN_POINT ( 'NONE',  ( -18.22292621751613950, -8.239355502252617924, 34.69524867566427417 ) ) ;
#22621=B_SPLINE_CURVE_WITH_KNOTS ( 'NONE', 3,
 ( #8166, #27986, #35187, #35640, #83837, #55457 ),
 .UNSPECIFIED., .F., .F.,
 ( 4, 2, 4 ),
 ( 4.934251614402251635E-17, 0.0001954756301637220611, 0.0003909512603273947911 ),
 .UNSPECIFIED. ) ;
#22622=ORIENTED_EDGE ( 'NONE', *, *, #38351, .T. ) ;
#22623=FACE_BOUND ( 'NONE', #83301, .T. ) ;
#22624=CARTESIAN_POINT ( 'NONE',  ( -16.82697755857493505, -4.336752205174650321, 33.62275283266504289 ) ) ;
#22625=EDGE_CURVE ( 'NONE', #24594, #28775, #71641, .T. ) ;
#22626=CARTESIAN_POINT ( 'NONE',  ( -14.30769230769230660, -7.500000000000001776, 35.04278698407183867 ) ) ;
#22627=DIRECTION ( 'NONE',  ( -0.000000000000000000, 0.9396926207859092051, -0.3420201433256662704 ) ) ;
#22628=EDGE_LOOP ( 'NONE', ( #27889, #64943 ) ) ;
#22629=CARTESIAN_POINT ( 'NONE',  ( 11.78840694783958476, -10.92531984108285670, 33.72920026020278073 ) ) ;
#22630=CARTESIAN_POINT ( 'NONE',  ( -14.43783951713053249, -4.460286881179643004, 33.72017969459903242 ) ) ;
#22631=CARTESIAN_POINT ( 'NONE',  ( -9.758391103263569732, -3.050289026998445951, 32.03036669348365706 ) ) ;
#22632=CARTESIAN_POINT ( 'NONE',  ( -18.00000000000000000, -12.62096338111211580, 30.90682066428153263 ) ) ;
#22633=ORIENTED_EDGE ( 'NONE', *, *, #76005, .F. ) ;
#22634=DIRECTION ( 'NONE',  ( 0.000000000000000000, 0.7660444431189807890, 0.6427876096865361433 ) ) ;
#22636=CARTESIAN_POINT ( 'NONE',  ( 6.923076923076924238, -13.88283147151868846, 33.14645433367849847 ) ) ;
#22637=ORIENTED_EDGE ( 'NONE', *, *, #9553, .T. ) ;
#22638=CARTESIAN_POINT ( 'NONE',  ( 9.442284455014732458, -3.711651800289232028, 33.01384336483936011 ) ) ;
#22639=CARTESIAN_POINT ( 'NONE',  ( 2.307692307692309264, -7.500000000000001776, 35.04278698407183867 ) ) ;
#22641=AXIS2_PLACEMENT_3D ( 'NONE', #58557, #44594, #72082 ) ;
#22642=CARTESIAN_POINT ( 'NONE',  ( 8.769230769230768274, -2.499999999999998668, 29.75000000000001421 ) ) ;
#22643=DIRECTION ( 'NONE',  ( -0.000000000000000000, 0.1736481776669307198, -0.9848077530122080203 ) ) ;
#22645=B_SPLINE_CURVE_WITH_KNOTS ( 'NONE', 3,
 ( #86908, #25176, #46783, #4917, #73367, #81025, #19311, #2339, #39152, #66616 ),
 .UNSPECIFIED., .F., .F.,
 ( 4, 2, 2, 2, 4 ),
 ( 0.0007817359430256294638, 0.0009771253907249950223, 0.001172514838424360472, 0.001367904286123725922, 0.001563293733823091372 ),
 .UNSPECIFIED. ) ;
#22647=CARTESIAN_POINT ( 'NONE',  ( 7.976679547917409963, -4.459921816937791661, 33.71989282347011851 ) ) ;
#22648=B_SPLINE_CURVE_WITH_KNOTS ( 'NONE', 3,
 ( #68829, #13443, #48106, #13884, #19762, #41365, #6258, #88250, #19321, #75159 ),
 .UNSPECIFIED., .F., .F.,
 ( 4, 2, 2, 2, 4 ),
 ( 0.0007817359430256333669, 0.0009771253907250056474, 0.001172514838424370881, 0.001367904286123736331, 0.001563293733823101564 ),
 .UNSPECIFIED. ) ;
#22650=VERTEX_POINT ( 'NONE', #13879 ) ;
#22651=VECTOR ( 'NONE', #75426, 1000.000000000000000 ) ;
#22652=B_SPLINE_CURVE_WITH_KNOTS ( 'NONE', 3,
 ( #29968, #9688, #17338, #56984, #29096, #57427, #10138, #84478, #43918, #51535 ),
 .UNSPECIFIED., .F., .F.,
 ( 4, 2, 2, 2, 4 ),
 ( 0.000000000000000000, 0.0001954339857564063089, 0.0003908679715128126177, 0.0005863019572692189808, 0.0007817359430256252354 ),
 .UNSPECIFIED. ) ;
#22653=CARTESIAN_POINT ( 'NONE',  ( 13.51514082284903040, -12.70449254468099198, 30.44128974285582956 ) ) ;
#22654=CARTESIAN_POINT ( 'NONE',  ( 13.63461538461680611, -7.500000000000154543, 35.00000000000007105 ) ) ;
#22655=ORIENTED_EDGE ( 'NONE', *, *, #11715, .F. ) ;
#22656=ORIENTED_EDGE ( 'NONE', *, *, #24357, .T. ) ;
#22658=ORIENTED_EDGE ( 'NONE', *, *, #78889, .T. ) ;
#22659=CARTESIAN_POINT ( 'NONE',  ( -10.86536134632696715, -11.28823185664190376, 33.01397839955799896 ) ) ;
#22660=CARTESIAN_POINT ( 'NONE',  ( -14.30769230769242917, -5.941354392335915335, 34.76329471203413846 ) ) ;
#22661=CARTESIAN_POINT ( 'NONE',  ( -1.384615384615383471, -1.466349020453238561, 30.81389545987213907 ) ) ;
#22662=CARTESIAN_POINT ( 'NONE',  ( 10.68063975489745232, -6.835583212224610072, 34.95778746994559327 ) ) ;
#22663=CARTESIAN_POINT ( 'NONE',  ( -16.28399336328437386, -3.285722584762970744, 32.44110544564090048 ) ) ;
#22664=CARTESIAN_POINT ( 'NONE',  ( 10.61538461538461675, -11.11383981884818262, 36.00935417666054406 ) ) ;
#22665=DIRECTION ( 'NONE',  ( 0.000000000000000000, 0.000000000000000000, 1.000000000000000000 ) ) ;
#22666=CARTESIAN_POINT ( 'NONE',  ( -4.153846153846273204, -6.026961402154118908, 34.52809138561165270 ) ) ;
#22667=DIRECTION ( 'NONE',  ( -0.000000000000000000, 1.000000000000000000, -0.000000000000000000 ) ) ;
#22668=EDGE_CURVE ( 'NONE', #11864, #86922, #41360, .T. ) ;
#22671=EDGE_CURVE ( 'NONE', #22548, #38438, #11520, .T. ) ;
#22672=VERTEX_POINT ( 'NONE', #15223 ) ;
#22673=EDGE_CURVE ( 'NONE', #4203, #40013, #27842, .T. ) ;
#22674=AXIS2_PLACEMENT_3D ( 'NONE', #77352, #43129, #56638 ) ;
#22675=CARTESIAN_POINT ( 'NONE',  ( 15.23076923076923173, -11.16473453929635440, 33.15142922261926373 ) ) ;
#22676=CARTESIAN_POINT ( 'NONE',  ( 12.46153846153846168, -11.33034616979429110, 35.88435417666054406 ) ) ;
#22677=CARTESIAN_POINT ( 'NONE',  ( -2.557692307692305267, -7.500000000000001776, 34.75000000000000000 ) ) ;
#22679=CARTESIAN_POINT ( 'NONE',  ( 6.223011351612851350, -4.887748414852792322, 34.01359900205216746 ) ) ;
#22680=B_SPLINE_CURVE_WITH_KNOTS ( 'NONE', 3,
 ( #88362, #53661, #25749, #60413, #59525, #26635, #26192, #68072, #52764, #61287 ),
 .UNSPECIFIED., .F., .F.,
 ( 4, 2, 2, 2, 4 ),
 ( 0.0007817246256747471724, 0.0009771112852218905021, 0.001172497944769033615, 0.001367884604316176944, 0.001563271263863320274 ),
 .UNSPECIFIED. ) ;
#22681=DIRECTION ( 'NONE',  ( -0.000000000000000000, 0.7660444431189791237, -0.6427876096865379196 ) ) ;
#22683=B_SPLINE_CURVE_WITH_KNOTS ( 'NONE', 3,
 ( #10534, #38002, #24926, #57826, #37544, #52390, #45191, #65471, #44286, #10082 ),
 .UNSPECIFIED., .F., .F.,
 ( 4, 2, 2, 2, 4 ),
 ( 0.0007817359430256300059, 0.0009771253907249963233, 0.001172514838424362424, 0.001367904286123728741, 0.001563293733823095059 ),
 .UNSPECIFIED. ) ;
#22685=B_SPLINE_CURVE_WITH_KNOTS ( 'NONE', 3,
 ( #87709, #72826, #25542, #65619, #11134, #73746, #51650, #38611, #86827, #32302 ),
 .UNSPECIFIED., .F., .F.,
 ( 4, 2, 2, 2, 4 ),
 ( 0.000000000000000000, 0.0001954339857564091007, 0.0003908679715128182013, 0.0005863019572692273291, 0.0007817359430256364027 ),
 .UNSPECIFIED. ) ;
#22687=VERTEX_POINT ( 'NONE', #21072 ) ;
#22688=CARTESIAN_POINT ( 'NONE',  ( 7.846153846153725020, -4.481592998941358097, 33.73612834414048933 ) ) ;
#22689=ORIENTED_EDGE ( 'NONE', *, *, #72386, .T. ) ;
#22690=CARTESIAN_POINT ( 'NONE',  ( 10.86543892702293412, -8.303483539816731707, 34.68545999027711702 ) ) ;
#22691=CARTESIAN_POINT ( 'NONE',  ( -3.296852641725109834, -12.10708131394839349, 31.69288490824020244 ) ) ;
#22692=CARTESIAN_POINT ( 'NONE',  ( -7.846153846153844924, -2.486705287966279876, 31.30864560766543647 ) ) ;
#22693=CARTESIAN_POINT ( 'NONE',  ( -14.30769230769242739, -10.21337939537710326, 33.94971097300076224 ) ) ;
#22695=ORIENTED_EDGE ( 'NONE', *, *, #27251, .T. ) ;
#22696=EDGE_CURVE ( 'NONE', #63890, #87106, #36246, .T. ) ;
#22698=ORIENTED_EDGE ( 'NONE', *, *, #80702, .F. ) ;
#22699=ORIENTED_EDGE ( 'NONE', *, *, #67325, .F. ) ;
#22700=DIRECTION ( 'NONE',  ( -0.000000000000000000, -0.9396926207859093161, -0.3420201433256663259 ) ) ;
#22701=CARTESIAN_POINT ( 'NONE',  ( -18.00000000000012079, -12.70778746994576025, 30.41441678777401236 ) ) ;
#22702=CARTESIAN_POINT ( 'NONE',  ( 5.999999999999880096, -8.613356846316285953, 34.62446782046622218 ) ) ;
#22703=CARTESIAN_POINT ( 'NONE',  ( -2.307692307692305711, -11.35647404775217417, 33.31231777344666511 ) ) ;
#22704=CARTESIAN_POINT ( 'NONE',  ( -17.74994568836168440, -4.235687564193448829, 33.53795663066793509 ) ) ;
#22705=CARTESIAN_POINT ( 'NONE',  ( 5.076923076922954969, -10.21337939537710326, 33.94971097300076224 ) ) ;
#22706=EDGE_LOOP ( 'NONE', ( #27609, #38999 ) ) ;
#22707=ORIENTED_EDGE ( 'NONE', *, *, #32527, .T. ) ;
#22709=ORIENTED_EDGE ( 'NONE', *, *, #41762, .F. ) ;
#22710=CARTESIAN_POINT ( 'NONE',  ( 3.930361210122207183, -2.847400154188068466, 31.58180166144859768 ) ) ;
#22711=EDGE_LOOP ( 'NONE', ( #56278, #11083, #76367, #50484 ) ) ;
#22712=CARTESIAN_POINT ( 'NONE',  ( 9.692307692307572609, -10.90142922262034020, 33.41473453929536674 ) ) ;
#22713=CARTESIAN_POINT ( 'NONE',  ( -10.55012947587177941, -6.835583212224610072, 34.95778746994559327 ) ) ;
#22715=EDGE_LOOP ( 'NONE', ( #81588, #36066, #51702, #37198, #34716, #79465 ) ) ;
#22716=VERTEX_POINT ( 'NONE', #56642 ) ;
#22717=CARTESIAN_POINT ( 'NONE',  ( -2.438383774359864642, -12.38065189839062263, 30.83690757178629482 ) ) ;
#22718=ORIENTED_EDGE ( 'NONE', *, *, #71377, .F. ) ;
#22719=FACE_BOUND ( 'NONE', #52295, .T. ) ;
#22720=CARTESIAN_POINT ( 'NONE',  ( 15.16468581981334829, -9.780366693483667717, 34.19971097300155805 ) ) ;
#22721=EDGE_CURVE ( 'NONE', #75758, #74098, #7576, .T. ) ;
#22722=AXIS2_PLACEMENT_3D ( 'NONE', #27189, #27631, #54647 ) ;
#22725=CARTESIAN_POINT ( 'NONE',  ( 6.000000000000001776, -4.786620604624113540, 33.94971097300155094 ) ) ;
#22726=CARTESIAN_POINT ( 'NONE',  ( 4.853996118016224770, -8.282780595021769443, 34.94152052738834868 ) ) ;
#22727=CARTESIAN_POINT ( 'NONE',  ( -4.153846153846274980, -3.083524468854526912, 32.58852847137268327 ) ) ;
#22728=B_SPLINE_CURVE_WITH_KNOTS ( 'NONE', 3,
 ( #20360, #76175, #68977, #34302, #33859, #61317 ),
 .UNSPECIFIED., .F., .F.,
 ( 4, 2, 4 ),
 ( 4.563551064100006665E-17, 0.0001954756301637168570, 0.0003909512603273880690 ),
 .UNSPECIFIED. ) ;
#22730=CARTESIAN_POINT ( 'NONE',  ( 3.930919936330005360, -11.24512374952581872, 33.06303171183252942 ) ) ;
#22731=CARTESIAN_POINT ( 'NONE',  ( -7.846153846153965716, -8.613356846316285953, 34.62446782046622218 ) ) ;
#22733=CARTESIAN_POINT ( 'NONE',  ( 7.173131342990377135, -2.544122305571457687, 31.48381861865059150 ) ) ;
#22734=CARTESIAN_POINT ( 'NONE',  ( -7.911423846710166075, -12.16647553114622049, 32.15551576947930812 ) ) ;
#22735=CYLINDRICAL_SURFACE ( 'NONE', #39863, 0.2499999999999998890 ) ;
#22736=CARTESIAN_POINT ( 'NONE',  ( 5.869308533332443290, -4.809359713505814149, 33.96456829005828837 ) ) ;
#22737=CARTESIAN_POINT ( 'NONE',  ( -14.30769230769230660, -13.87047571288749737, 32.06866353760679544 ) ) ;
#22738=CARTESIAN_POINT ( 'NONE',  ( 7.846153846153723244, -3.083524468854526912, 32.58852847137268327 ) ) ;
#22739=CARTESIAN_POINT ( 'NONE',  ( 17.07692307692307665, -3.513871655860378418, 32.76840700105978499 ) ) ;
#22740=CARTESIAN_POINT ( 'NONE',  ( 11.66929986894829696, -7.277220318596961057, 34.99547417642776992 ) ) ;
#22741=EDGE_CURVE ( 'NONE', #30710, #51792, #56663, .T. ) ;
#22742=CARTESIAN_POINT ( 'NONE',  ( -16.08859058257012720, -11.94971097300157403, 32.03036669348361443 ) ) ;
#22743=CARTESIAN_POINT ( 'NONE',  ( -3.480792454990687013, -2.985938066672154445, 32.43141759479405550 ) ) ;
#22747=ORIENTED_EDGE ( 'NONE', *, *, #75939, .T. ) ;
#22748=CARTESIAN_POINT ( 'NONE',  ( 0.2386122440223129304, -12.39988816332205701, 30.74660775122750778 ) ) ;
#22749=ORIENTED_EDGE ( 'NONE', *, *, #33446, .T. ) ;
#22753=CARTESIAN_POINT ( 'NONE',  ( -22.75000000000000000, -10.49999999999999822, 27.25000000000000000 ) ) ;
#22754=EDGE_CURVE ( 'NONE', #59461, #77977, #53469, .T. ) ;
#22755=ORIENTED_EDGE ( 'NONE', *, *, #68888, .T. ) ;
#22756=CARTESIAN_POINT ( 'NONE',  ( -5.999999999999998224, -11.69971097300155272, 32.46337939537588113 ) ) ;
#22758=CARTESIAN_POINT ( 'NONE',  ( 17.29993442853592711, -8.239487800360276282, 34.69522927552633718 ) ) ;
#22759=CARTESIAN_POINT ( 'NONE',  ( 6.923076923076924238, -12.37446782046654192, 30.86335684631486131 ) ) ;
#22760=CARTESIAN_POINT ( 'NONE',  ( 7.145856464345332171, -9.332535724633407526, 34.40230450496446224 ) ) ;
#22761=CARTESIAN_POINT ( 'NONE',  ( -39.05038313613820122, -2.249999999999998668, 29.75000000000000355 ) ) ;
#22762=CARTESIAN_POINT ( 'NONE',  ( -13.45069776397551742, -8.164416787775445883, 34.95778746994557906 ) ) ;
#22763=CARTESIAN_POINT ( 'NONE',  ( -13.60810030917971503, -12.11044203135681840, 32.26167407432752299 ) ) ;
#22765=CARTESIAN_POINT ( 'NONE',  ( -11.28840711854808632, -2.544122305571458575, 31.48381861865057729 ) ) ;
#22766=DIRECTION ( 'NONE',  ( -0.000000000000000000, 0.6427876096865404731, -0.7660444431189770143 ) ) ;
#22767=ADVANCED_FACE ( 'NONE', ( #44003 ), #9352, .F. ) ;
#22768=CARTESIAN_POINT ( 'NONE',  ( -2.307692307692305711, -4.098570777380720287, 33.41473453929634729 ) ) ;
#22771=B_SPLINE_CURVE_WITH_KNOTS ( 'NONE', 3,
 ( #30534, #58005, #51218, #30969, #72847, #86395, #24667, #52576, #79172, #58894 ),
 .UNSPECIFIED., .F., .F.,
 ( 4, 2, 2, 2, 4 ),
 ( 0.0007817359430256294638, 0.0009771253907249952391, 0.001172514838424361123, 0.001367904286123726790, 0.001563293733823092673 ),
 .UNSPECIFIED. ) ;
#22772=CARTESIAN_POINT ( 'NONE',  ( -10.39260494640654642, -5.827830569534417471, 34.72679350104403539 ) ) ;
#22773=EDGE_LOOP ( 'NONE', ( #2755, #20271 ) ) ;
#22774=EDGE_CURVE ( 'NONE', #7402, #67715, #64267, .T. ) ;
#22775=CARTESIAN_POINT ( 'NONE',  ( 14.30769230769218758, -5.219633306517616589, 34.19971097300220464 ) ) ;
#22776=DIRECTION ( 'NONE',  ( -0.000000000000000000, 0.3420201433256694346, -0.9396926207859080948 ) ) ;
#22778=CARTESIAN_POINT ( 'NONE',  ( 16.40384615384608935, -7.565270000091922853, 34.99999999999999289 ) ) ;
#22779=ADVANCED_FACE ( 'NONE', ( #71472 ), #2567, .F. ) ;
#22781=CARTESIAN_POINT ( 'NONE',  ( 9.442330961365339448, -11.28823185664190376, 33.01397839955799896 ) ) ;
#22782=CYLINDRICAL_SURFACE ( 'NONE', #29087, 0.2499999999999997502 ) ;
#22783=AXIS2_PLACEMENT_3D ( 'NONE', #39475, #72788, #61827 ) ;
#22784=ORIENTED_EDGE ( 'NONE', *, *, #59459, .T. ) ;
#22786=ORIENTED_EDGE ( 'NONE', *, *, #58126, .F. ) ;
#22787=CARTESIAN_POINT ( 'NONE',  ( -6.857009589726848375, -5.471508081941601098, 34.59228464037088457 ) ) ;
#22789=CARTESIAN_POINT ( 'NONE',  ( 16.28437185560971301, -2.882268652242222728, 31.66798894389554064 ) ) ;
#22790=CARTESIAN_POINT ( 'NONE',  ( 4.284637961670941131, -3.530189275343204702, 32.79018710029569661 ) ) ;
#22791=CARTESIAN_POINT ( 'NONE',  ( 10.61538461538449418, -10.33852847137269571, 34.16647553114546554 ) ) ;
#22792=EDGE_LOOP ( 'NONE', ( #71729, #55862 ) ) ;
#22793=CARTESIAN_POINT ( 'NONE',  ( 17.20771351789003489, -11.37503395064541678, 33.29242100308974983 ) ) ;
#22794=AXIS2_PLACEMENT_3D ( 'NONE', #28404, #76144, #34276 ) ;
#22796=EDGE_CURVE ( 'NONE', #67575, #15414, #80285, .T. ) ;
#22797=ORIENTED_EDGE ( 'NONE', *, *, #84672, .F. ) ;
#22799=B_SPLINE_CURVE_WITH_KNOTS ( 'NONE', 3,
 ( #70931, #57856, #2024, #84458, #15547, #22299, #49763, #85338, #50193, #36266 ),
 .UNSPECIFIED., .F., .F.,
 ( 4, 2, 2, 2, 4 ),
 ( 0.000000000000000000, 0.0001954339857564064444, 0.0003908679715128128888, 0.0005863019572692193060, 0.0007817359430256257775 ),
 .UNSPECIFIED. ) ;
#22800=B_SPLINE_CURVE_WITH_KNOTS ( 'NONE', 3,
 ( #42782, #29270, #50396, #22496, #16613, #37326, #57167, #64792, #77439, #64351 ),
 .UNSPECIFIED., .F., .F.,
 ( 4, 2, 2, 2, 4 ),
 ( 0.0007817246256747528103, 0.0009771112852218978746, 0.001172497944769042722, 0.001367884604316187570, 0.001563271263863332634 ),
 .UNSPECIFIED. ) ;
#22801=LINE ( 'NONE', #50261, #61637 ) ;
#22803=EDGE_CURVE ( 'NONE', #19870, #48154, #7211, .T. ) ;
#22804=B_SPLINE_CURVE_WITH_KNOTS ( 'NONE', 3,
 ( #39809, #87122, #19089, #81683, #32594, #33045 ),
 .UNSPECIFIED., .F., .F.,
 ( 4, 2, 4 ),
 ( 0.0003909512603273869848, 0.0005862562993132133804, 0.0007815613382990397760 ),
 .UNSPECIFIED. ) ;
#22805=ADVANCED_FACE ( 'NONE', ( #29622 ), #24174, .F. ) ;
#22806=CARTESIAN_POINT ( 'NONE',  ( -12.46153846153846168, -1.422936976036506707, 30.56769352161908415 ) ) ;
#22807=EDGE_CURVE ( 'NONE', #55920, #43958, #10060, .T. ) ;
#22809=CARTESIAN_POINT ( 'NONE',  ( -15.93083330975275658, -5.582272713120730145, 34.63742843783360570 ) ) ;
#22810=ORIENTED_EDGE ( 'NONE', *, *, #23029, .T. ) ;
#22813=ADVANCED_FACE ( 'NONE', ( #78234 ), #64713, .F. ) ;
#22814=ORIENTED_EDGE ( 'NONE', *, *, #30868, .F. ) ;
#22815=CARTESIAN_POINT ( 'NONE',  ( 8.096099255531887806, -4.932303261841489039, 34.32971442181322885 ) ) ;
#22816=CARTESIAN_POINT ( 'NONE',  ( 4.376625695114562120, -11.41317474335729187, 32.86274602512330034 ) ) ;
#22817=ORIENTED_EDGE ( 'NONE', *, *, #11166, .T. ) ;
#22818=CARTESIAN_POINT ( 'NONE',  ( 20.99999999999998224, -12.75000000000000178, 27.25000000000000000 ) ) ;
#22819=CARTESIAN_POINT ( 'NONE',  ( 5.076923076922954969, -3.835265460704628371, 33.15142922262033665 ) ) ;
#22820=CARTESIAN_POINT ( 'NONE',  ( 1.384615384615386802, -1.044019251281081972, 31.83374038241031911 ) ) ;
#22821=ORIENTED_EDGE ( 'NONE', *, *, #40388, .T. ) ;
#22822=CARTESIAN_POINT ( 'NONE',  ( 15.00784301325308157, -10.61292498521070549, 33.66303323003028680 ) ) ;
#22823=CARTESIAN_POINT ( 'NONE',  ( 15.10062126103753322, -2.647304123082328875, 31.75400227202885972 ) ) ;
#22824=VECTOR ( 'NONE', #6132, 1000.000000000000000 ) ;
#22825=ORIENTED_EDGE ( 'NONE', *, *, #11656, .F. ) ;
#22826=FACE_BOUND ( 'NONE', #28313, .T. ) ;
#22827=CARTESIAN_POINT ( 'NONE',  ( -10.61538461538461320, -4.661471528628507777, 34.16647553114623292 ) ) ;
#22829=CYLINDRICAL_SURFACE ( 'NONE', #25031, 0.2500000000000008882 ) ;
#22830=CYLINDRICAL_SURFACE ( 'NONE', #21629, 0.2499999999999973355 ) ;
#22831=CARTESIAN_POINT ( 'NONE',  ( -6.857008572074483332, -2.538708090699994813, 30.37095296980875503 ) ) ;
#22832=CARTESIAN_POINT ( 'NONE',  ( -1.384615384615383471, -8.164416787775445883, 34.95778746994557906 ) ) ;
#22833=CARTESIAN_POINT ( 'NONE',  ( -4.403822897894743349, -10.82459398097509684, 33.81372124010185587 ) ) ;
#22834=ORIENTED_EDGE ( 'NONE', *, *, #4980, .F. ) ;
#22835=CARTESIAN_POINT ( 'NONE',  ( -0.4615384615384611200, -13.49023893513002648, 31.06009739812518688 ) ) ;
#22836=CARTESIAN_POINT ( 'NONE',  ( -6.130690603110307890, -11.37499894934982514, 33.29245874905763003 ) ) ;
#22838=ORIENTED_EDGE ( 'NONE', *, *, #74155, .F. ) ;
#22839=CARTESIAN_POINT ( 'NONE',  ( -16.40382289789473802, -12.65889640711025521, 30.72598325615533454 ) ) ;
#22840=CARTESIAN_POINT ( 'NONE',  ( 10.48523740594639442, -6.852621066184266141, 34.70813303252209181 ) ) ;
#22841=CARTESIAN_POINT ( 'NONE',  ( -16.15384615384627409, -10.90142922262034020, 33.41473453929536674 ) ) ;
#22842=DIRECTION ( 'NONE',  ( -0.000000000000000000, -0.6427876096865404731, -0.7660444431189771253 ) ) ;
#22843=LINE ( 'NONE', #9345, #51444 ) ;
#22844=CARTESIAN_POINT ( 'NONE',  ( -7.911907274467175455, -7.249945578846651806, 34.99404164642496795 ) ) ;
#22845=FACE_BOUND ( 'NONE', #49152, .T. ) ;
#22847=CARTESIAN_POINT ( 'NONE',  ( -10.36538461538319389, -7.500000000000154543, 35.00000000000007105 ) ) ;
#22848=CARTESIAN_POINT ( 'NONE',  ( 16.08857570788537572, -3.300289026998414865, 32.46337939537583139 ) ) ;
#22849=CARTESIAN_POINT ( 'NONE',  ( -6.700297254098858346, -10.97394488606064122, 33.68653795673694873 ) ) ;
#22851=DIRECTION ( 'NONE',  ( -0.000000000000000000, -0.9848077530122086864, -0.1736481776669273613 ) ) ;
#22853=ORIENTED_EDGE ( 'NONE', *, *, #59801, .F. ) ;
#22854=ORIENTED_EDGE ( 'NONE', *, *, #20023, .T. ) ;
#22855=CARTESIAN_POINT ( 'NONE',  ( 16.02369818411445834, -9.504002272028873932, 34.60269587691767867 ) ) ;
#22856=CARTESIAN_POINT ( 'NONE',  ( -5.011667505647051435, -3.300289026998475705, 32.46337939537591666 ) ) ;
#22858=CARTESIAN_POINT ( 'NONE',  ( -1.384615384615505151, -3.300289026999228881, 32.46337939537708905 ) ) ;
#22859=CARTESIAN_POINT ( 'NONE',  ( 3.165498784808456811, -11.48612834413959582, 32.76840700105983473 ) ) ;
#22861=CARTESIAN_POINT ( 'NONE',  ( -16.15384615384627409, -5.941354392335915335, 34.76329471203413846 ) ) ;
#22862=CARTESIAN_POINT ( 'NONE',  ( -18.00000000000012079, -11.48612834414049644, 32.76840700105863391 ) ) ;
#22864=CARTESIAN_POINT ( 'NONE',  ( 3.480714640147274608, -4.176053281294514363, 33.81426240980091791 ) ) ;
#22865=CARTESIAN_POINT ( 'NONE',  ( 10.48523664565292002, -6.809168938359901446, 34.95455904226513866 ) ) ;
#22866=CARTESIAN_POINT ( 'NONE',  ( -17.07692307692307665, -4.661471528628507777, 34.16647553114623292 ) ) ;
#22867=CARTESIAN_POINT ( 'NONE',  ( 10.68057859716797431, -2.506253911140448043, 29.99999999999988631 ) ) ;
#22868=VECTOR ( 'NONE', #43584, 1000.000000000000227 ) ;
#22869=LINE ( 'NONE', #62092, #75014 ) ;
#22870=ADVANCED_FACE ( 'NONE', ( #77356 ), #8906, .F. ) ;
#22872=CARTESIAN_POINT ( 'NONE',  ( 7.976945653978634532, -6.413143153341454017, 34.63066358083362672 ) ) ;
#22873=VERTEX_POINT ( 'NONE', #46233 ) ;
#22875=DIRECTION ( 'NONE',  ( -0.000000000000000000, -0.1736481776669307198, -0.9848077530122080203 ) ) ;
#22877=EDGE_CURVE ( 'NONE', #33903, #31532, #67835, .T. ) ;
#22878=B_SPLINE_CURVE_WITH_KNOTS ( 'NONE', 3,
 ( #88239, #81466, #59845, #20198, #13433, #12994, #33709, #61166, #88676, #26955 ),
 .UNSPECIFIED., .F., .F.,
 ( 4, 2, 2, 2, 4 ),
 ( 0.000000000000000000, 0.0001954339857564071762, 0.0003908679715128143524, 0.0005863019572692215828, 0.0007817359430256287049 ),
 .UNSPECIFIED. ) ;
#22879=CARTESIAN_POINT ( 'NONE',  ( -2.307692307692305711, -4.661471528628507777, 34.16647553114623292 ) ) ;
#22880=CARTESIAN_POINT ( 'NONE',  ( 17.07692307692295586, -11.67786785259630911, 32.92929555188603530 ) ) ;
#22881=ORIENTED_EDGE ( 'NONE', *, *, #53620, .F. ) ;
#22882=CARTESIAN_POINT ( 'NONE',  ( 10.48482402364269639, -2.504760397472875155, 29.97295953869789997 ) ) ;
#22884=VERTEX_POINT ( 'NONE', #12015 ) ;
#22885=CARTESIAN_POINT ( 'NONE',  ( 9.442307692307691624, -2.499999999999999556, 29.81609845454691765 ) ) ;
#22886=CARTESIAN_POINT ( 'NONE',  ( 6.923076923076800782, -12.70778746994576025, 30.41441678777401236 ) ) ;
#22888=VERTEX_POINT ( 'NONE', #73261 ) ;
#22889=CARTESIAN_POINT ( 'NONE',  ( -10.36538461538461320, -7.500000000000001776, 35.04278698407183867 ) ) ;
#22890=CARTESIAN_POINT ( 'NONE',  ( 2.307692307692309264, -5.557115091759785130, 34.35708131394839171 ) ) ;
#22891=ADVANCED_FACE ( 'NONE', ( #19644 ), #25518, .F. ) ;
#22892=VERTEX_POINT ( 'NONE', #45782 ) ;
#22893=B_SPLINE_CURVE_WITH_KNOTS ( 'NONE', 3,
 ( #7998, #69692, #84110, #21499, #6660, #7107, #62477, #62916, #27384, #34581 ),
 .UNSPECIFIED., .F., .F.,
 ( 4, 2, 2, 2, 4 ),
 ( 0.0007817246256747473893, 0.0009771112852218909357, 0.001172497944769034482, 0.001367884604316178246, 0.001563271263863321792 ),
 .UNSPECIFIED. ) ;
#22895=LINE ( 'NONE', #85057, #27799 ) ;
#22896=CARTESIAN_POINT ( 'NONE',  ( 15.23076923076923173, -9.905515769479276145, 34.41647553114623292 ) ) ;
#22897=VERTEX_POINT ( 'NONE', #12884 ) ;
#22898=ORIENTED_EDGE ( 'NONE', *, *, #59874, .T. ) ;
#22899=EDGE_CURVE ( 'NONE', #70106, #84245, #26408, .T. ) ;
#22900=CIRCLE ( 'NONE', #80451, 0.2500000000000002220 ) ;
#22902=CARTESIAN_POINT ( 'NONE',  ( 6.923076923076924238, -1.242168528481310874, 33.36296068462461051 ) ) ;
#22903=CARTESIAN_POINT ( 'NONE',  ( -5.750054590621955342, -5.766571408460171355, 34.70601412856602508 ) ) ;
#22904=EDGE_CURVE ( 'NONE', #18589, #51403, #6095, .T. ) ;
#22905=CARTESIAN_POINT ( 'NONE',  ( -4.153846153846274980, -12.70778746994576025, 30.41441678777401236 ) ) ;
#22906=DIRECTION ( 'NONE',  ( 0.000000000000000000, 0.9396926207859126468, -0.3420201433256571111 ) ) ;
#22907=EDGE_CURVE ( 'NONE', #59376, #64075, #66505, .T. ) ;
#22908=ORIENTED_EDGE ( 'NONE', *, *, #72543, .T. ) ;
#22909=ORIENTED_EDGE ( 'NONE', *, *, #88902, .F. ) ;
#22910=CARTESIAN_POINT ( 'NONE',  ( 4.403791563224197070, -8.476813868363244353, 34.90874843262270133 ) ) ;
#22911=VERTEX_POINT ( 'NONE', #52974 ) ;
#22913=DIRECTION ( 'NONE',  ( -0.000000000000000000, -0.9396926207859092051, -0.3420201433256662704 ) ) ;
#22916=CARTESIAN_POINT ( 'NONE',  ( 7.716005876422152632, -12.15440758774515473, 32.17923288041532004 ) ) ;
#22917=CARTESIAN_POINT ( 'NONE',  ( -8.546451100252703270, -12.69155399931963046, 30.53255429739157734 ) ) ;
#22918=ORIENTED_EDGE ( 'NONE', *, *, #1208, .F. ) ;
#22919=AXIS2_PLACEMENT_3D ( 'NONE', #27743, #70062, #34060 ) ;
#22920=AXIS2_PLACEMENT_3D ( 'NONE', #28597, #79446, #57831 ) ;
#22923=CARTESIAN_POINT ( 'NONE',  ( 9.942362112221147186, -8.346898887586323923, 34.93166121998716278 ) ) ;
#22924=EDGE_LOOP ( 'NONE', ( #43139, #51251, #512, #6474 ) ) ;
#22925=AXIS2_PLACEMENT_3D ( 'NONE', #34847, #33082, #67318 ) ;
#22926=CARTESIAN_POINT ( 'NONE',  ( 4.219914504848592429, -4.786620604624113540, 33.94971097300155805 ) ) ;
#22927=CARTESIAN_POINT ( 'NONE',  ( -10.83886953994894498, -9.417330523894424488, 34.63758898049880486 ) ) ;
#22928=ORIENTED_EDGE ( 'NONE', *, *, #59581, .T. ) ;
#22929=ADVANCED_FACE ( 'NONE', ( #73721 ), #86355, .F. ) ;
#22930=DIRECTION ( 'NONE',  ( -0.000000000000000000, 0.8660254037844399289, -0.4999999999999980016 ) ) ;
#22932=DIRECTION ( 'NONE',  ( -0.000000000000000000, 0.9848077530122086864, -0.1736481776669273891 ) ) ;
#22933=B_SPLINE_CURVE_WITH_KNOTS ( 'NONE', 3,
 ( #22693, #2413, #51025, #84858, #57807, #78084, #64549, #37528, #44271, #50605 ),
 .UNSPECIFIED., .F., .F.,
 ( 4, 2, 2, 2, 4 ),
 ( 0.0007817359430256360774, 0.0009771253907250041296, 0.001172514838424371965, 0.001367904286123740017, 0.001563293733823108069 ),
 .UNSPECIFIED. ) ;
#22934=FACE_BOUND ( 'NONE', #3242, .T. ) ;
#22935=CARTESIAN_POINT ( 'NONE',  ( -8.519285359852727169, -2.341251567377310217, 30.72681386836322659 ) ) ;
#22936=CARTESIAN_POINT ( 'NONE',  ( 2.557637826040450424, -8.433404298154334455, 34.66254593164985920 ) ) ;
#22937=CARTESIAN_POINT ( 'NONE',  ( 13.13463864056679675, -12.65889640711025521, 30.72598325615533454 ) ) ;
#22938=CARTESIAN_POINT ( 'NONE',  ( -16.85414340794500276, -12.47679350104403007, 31.42216943046555855 ) ) ;
#22939=CARTESIAN_POINT ( 'NONE',  ( 4.403791563224197070, -2.341251567377310217, 30.72681386836322659 ) ) ;
#22940=CARTESIAN_POINT ( 'NONE',  ( 17.77707304109314634, -6.459968553980840689, 34.89616026154728701 ) ) ;
#22941=CARTESIAN_POINT ( 'NONE',  ( -7.846153846153967493, -2.657715359629662544, 31.77849191805970364 ) ) ;
#22942=ORIENTED_EDGE ( 'NONE', *, *, #51259, .T. ) ;
#22943=FACE_OUTER_BOUND ( 'NONE', #81967, .T. ) ;
#22944=ORIENTED_EDGE ( 'NONE', *, *, #82877, .T. ) ;
#22945=EDGE_CURVE ( 'NONE', #40194, #40709, #11495, .T. ) ;
#22946=ORIENTED_EDGE ( 'NONE', *, *, #4881, .F. ) ;
#22948=CARTESIAN_POINT ( 'NONE',  ( 10.74591005361826035, -12.15418822224088657, 32.17964115625579069 ) ) ;
#22950=CARTESIAN_POINT ( 'NONE',  ( -5.776988648387149539, -6.503523203565942268, 34.64991518177335195 ) ) ;
#22951=CARTESIAN_POINT ( 'NONE',  ( -0.4615384615384611200, -12.78798330534102945, 29.74999999999997868 ) ) ;
#22952=CARTESIAN_POINT ( 'NONE',  ( 14.55769230769231015, -2.249999999999998668, 29.75000000000000355 ) ) ;
#22953=DIRECTION ( 'NONE',  ( -0.000000000000000000, 0.1736481776669307198, -0.9848077530122080203 ) ) ;
#22954=ORIENTED_EDGE ( 'NONE', *, *, #89117, .T. ) ;
#22955=CARTESIAN_POINT ( 'NONE',  ( -12.46153846153846168, -1.790695186598648903, 34.54067556320373455 ) ) ;
#22956=CARTESIAN_POINT ( 'NONE',  ( 0.3962684609821418014, -12.70778746994557551, 30.41441678777548319 ) ) ;
#22957=CARTESIAN_POINT ( 'NONE',  ( 17.20744877868664346, -6.852161475712351013, 34.70806712695775786 ) ) ;
#22958=FACE_OUTER_BOUND ( 'NONE', #25298, .T. ) ;
#22959=CARTESIAN_POINT ( 'NONE',  ( -11.53846153846123102, -2.506253911140614576, 30.00000000000323297 ) ) ;
#22962=ORIENTED_EDGE ( 'NONE', *, *, #89173, .T. ) ;
#22963=ORIENTED_EDGE ( 'NONE', *, *, #66799, .F. ) ;
#22964=CARTESIAN_POINT ( 'NONE',  ( -7.780086512803768173, -11.91647553114624358, 32.58852847137148245 ) ) ;
#22965=ORIENTED_EDGE ( 'NONE', *, *, #36252, .T. ) ;
#22966=CARTESIAN_POINT ( 'NONE',  ( 17.07692307692307665, -3.937682226553329556, 33.60647404775216529 ) ) ;
#22967=CARTESIAN_POINT ( 'NONE',  ( 18.06606835100243913, -5.557115091759786019, 34.35708131394839882 ) ) ;
#22968=CARTESIAN_POINT ( 'NONE',  ( -5.076923076923075762, -8.164416787775445883, 34.95778746994557906 ) ) ;
#22969=CARTESIAN_POINT ( 'NONE',  ( -8.703975197954745724, -10.90142922261932057, 33.41473453929631887 ) ) ;
#22971=CARTESIAN_POINT ( 'NONE',  ( 17.07692307692307665, -7.500000000000001776, 35.04278698407183867 ) ) ;
#22972=VERTEX_POINT ( 'NONE', #53421 ) ;
#22973=DIRECTION ( 'NONE',  ( -0.000000000000000000, 0.6427876096865404731, -0.7660444431189771253 ) ) ;
#22974=CARTESIAN_POINT ( 'NONE',  ( -9.692307692307691624, -2.292212530054420494, 30.41441678777542634 ) ) ;
#22975=ORIENTED_EDGE ( 'NONE', *, *, #45850, .T. ) ;
#22976=CARTESIAN_POINT ( 'NONE',  ( -9.692307692307691624, -11.11383981884818262, 36.00935417666054406 ) ) ;
#22977=CARTESIAN_POINT ( 'NONE',  ( -12.33101275977489841, -3.816742781228458004, 33.13167719472716044 ) ) ;
#22978=B_SPLINE_CURVE_WITH_KNOTS ( 'NONE', 3,
 ( #75836, #68202, #48801, #34845, #76273, #55121, #41613, #75400, #42064, #13693 ),
 .UNSPECIFIED., .F., .F.,
 ( 4, 2, 2, 2, 4 ),
 ( 0.0007817359430256300059, 0.0009771253907249963233, 0.001172514838424362858, 0.001367904286123729392, 0.001563293733823095709 ),
 .UNSPECIFIED. ) ;
#22979=CARTESIAN_POINT ( 'NONE',  ( 11.53846153846141753, -4.481592998941358097, 33.73612834414048933 ) ) ;
#22980=CARTESIAN_POINT ( 'NONE',  ( 6.792386319966615460, -3.338472653186242756, 32.95098750199972670 ) ) ;
#22981=B_SPLINE_CURVE_WITH_KNOTS ( 'NONE', 3,
 ( #84460, #77681, #64156, #2458, #84901, #23187, #48881, #73008, #52286, #19398 ),
 .UNSPECIFIED., .F., .F.,
 ( 4, 2, 2, 2, 4 ),
 ( 0.000000000000000000, 0.0001954339857564070678, 0.0003908679715128141356, 0.0005863019572692211492, 0.0007817359430256282712 ),
 .UNSPECIFIED. ) ;
#22982=VECTOR ( 'NONE', #82449, 1000.000000000000114 ) ;
#22984=CARTESIAN_POINT ( 'NONE',  ( -7.846153846153844924, -12.37446782046654192, 30.86335684631486131 ) ) ;
#22986=ORIENTED_EDGE ( 'NONE', *, *, #25820, .T. ) ;
#22987=CARTESIAN_POINT ( 'NONE',  ( -2.980823821391186623, -6.653508905675590945, 34.93172785388651391 ) ) ;
#22988=CYLINDRICAL_SURFACE ( 'NONE', #59149, 0.2500000000000002220 ) ;
#22990=AXIS2_PLACEMENT_3D ( 'NONE', #74151, #81360, #47105 ) ;
#22991=CARTESIAN_POINT ( 'NONE',  ( -16.08777882049607655, -11.35647404775217595, 33.31231777344667222 ) ) ;
#22992=DIRECTION ( 'NONE',  ( -0.000000000000000000, -0.000000000000000000, -1.000000000000000000 ) ) ;
#22993=ORIENTED_EDGE ( 'NONE', *, *, #17473, .F. ) ;
#22994=CYLINDRICAL_SURFACE ( 'NONE', #83028, 0.2499999999999994726 ) ;
#22995=CARTESIAN_POINT ( 'NONE',  ( 3.164685819813350509, -8.973038597847271092, 34.52809138561120506 ) ) ;
#22996=ADVANCED_FACE ( 'NONE', ( #38589 ), #80923, .F. ) ;
#22997=AXIS2_PLACEMENT_3D ( 'NONE', #4386, #73294, #5720 ) ;
#22998=ORIENTED_EDGE ( 'NONE', *, *, #61421, .F. ) ;
#23000=CYLINDRICAL_SURFACE ( 'NONE', #42857, 0.2500000000000009437 ) ;
#23004=ORIENTED_EDGE ( 'NONE', *, *, #47817, .F. ) ;
#23005=LINE ( 'NONE', #43715, #40591 ) ;
#23006=DIRECTION ( 'NONE',  ( 0.000000000000000000, 0.9848077530122072432, 0.1736481776669354937 ) ) ;
#23007=CARTESIAN_POINT ( 'NONE',  ( -12.59168643127015841, -10.31621877034669588, 34.18098118002070152 ) ) ;
#23008=CARTESIAN_POINT ( 'NONE',  ( -12.46153846153846168, -10.67929555188718282, 33.92786785259544047 ) ) ;
#23009=VERTEX_POINT ( 'NONE', #8356 ) ;
#23010=EDGE_CURVE ( 'NONE', #41430, #47075, #88578, .T. ) ;
#23011=CARTESIAN_POINT ( 'NONE',  ( 13.13461538461538680, -2.249999999999998668, 29.75000000000000355 ) ) ;
#23012=VERTEX_POINT ( 'NONE', #40813 ) ;
#23013=DIRECTION ( 'NONE',  ( -0.000000000000000000, 0.6427876096865404731, -0.7660444431189771253 ) ) ;
#23014=CARTESIAN_POINT ( 'NONE',  ( -10.86536134632696715, -2.779195860258146578, 31.39871582349836032 ) ) ;
#23015=ORIENTED_EDGE ( 'NONE', *, *, #16381, .F. ) ;
#23016=CARTESIAN_POINT ( 'NONE',  ( -2.307692307692428724, -11.06231777344772027, 33.60647404775119895 ) ) ;
#23017=CARTESIAN_POINT ( 'NONE',  ( -12.52762187249433978, -5.557115091759785130, 34.35708131394839171 ) ) ;
#23018=DIRECTION ( 'NONE',  ( -0.000000000000000000, 0.1736481776669307198, -0.9848077530122080203 ) ) ;
#23019=EDGE_CURVE ( 'NONE', #80339, #26228, #49163, .T. ) ;
#23020=FACE_OUTER_BOUND ( 'NONE', #69469, .T. ) ;
#23022=B_SPLINE_CURVE_WITH_KNOTS ( 'NONE', 3,
 ( #76210, #14516, #69461, #7765, #38786, #30686, #16724, #71668, #17172, #86544 ),
 .UNSPECIFIED., .F., .F.,
 ( 4, 2, 2, 2, 4 ),
 ( 0.0007817359527651098448, 0.0009771254036996487088, 0.001172514854634187573, 0.001367904305568726220, 0.001563293756503265084 ),
 .UNSPECIFIED. ) ;
#23023=ORIENTED_EDGE ( 'NONE', *, *, #58587, .F. ) ;
#23024=VERTEX_POINT ( 'NONE', #62388 ) ;
#23025=FACE_BOUND ( 'NONE', #88720, .T. ) ;
#23028=EDGE_CURVE ( 'NONE', #82752, #20850, #28760, .T. ) ;
#23029=EDGE_CURVE ( 'NONE', #26488, #59736, #44839, .T. ) ;
#23030=CARTESIAN_POINT ( 'NONE',  ( 17.77707304109314634, -5.582147617184174848, 34.63737895849758530 ) ) ;
#23031=CARTESIAN_POINT ( 'NONE',  ( 0.4615384615383382183, -12.70778746994576025, 30.41441678777401236 ) ) ;
#23033=ORIENTED_EDGE ( 'NONE', *, *, #55059, .F. ) ;
#23034=DIRECTION ( 'NONE',  ( -0.000000000000000000, -0.6427876096865404731, -0.7660444431189771253 ) ) ;
#23035=ORIENTED_EDGE ( 'NONE', *, *, #32205, .F. ) ;
#23036=CARTESIAN_POINT ( 'NONE',  ( -10.55012904410859065, -9.442884908240273489, 34.35708131394835618 ) ) ;
#23037=ADVANCED_FACE ( 'NONE', ( #42149 ), #13771, .F. ) ;
#23039=CARTESIAN_POINT ( 'NONE',  ( 13.31853197365950336, -2.721908614388770964, 31.22303859784723912 ) ) ;
#23041=FACE_BOUND ( 'NONE', #81868, .T. ) ;
#23042=ORIENTED_EDGE ( 'NONE', *, *, #74672, .T. ) ;
#23043=CARTESIAN_POINT ( 'NONE',  ( 8.834486340506792601, -9.442884908240273489, 34.35708131394835618 ) ) ;
#23044=B_SPLINE_CURVE_WITH_KNOTS ( 'NONE', 3,
 ( #29888, #3282, #43830, #42960, #86168, #65433, #50584, #70430, #85275, #29451 ),
 .UNSPECIFIED., .F., .F.,
 ( 4, 2, 2, 2, 4 ),
 ( 0.0007817246256747440282, 0.0009771112852218863821, 0.001172497944769028844, 0.001367884604316171307, 0.001563271263863313769 ),
 .UNSPECIFIED. ) ;
#23045=VECTOR ( 'NONE', #74279, 1000.000000000000227 ) ;
#23046=AXIS2_PLACEMENT_3D ( 'NONE', #63780, #78185, #78625 ) ;
#23047=CARTESIAN_POINT ( 'NONE',  ( -14.98082382139119062, -3.520799739797214389, 33.17531984108286025 ) ) ;
#23048=DIRECTION ( 'NONE',  ( 0.000000000000000000, 0.1736481776669267785, -0.9848077530122087975 ) ) ;
#23050=ORIENTED_EDGE ( 'NONE', *, *, #60191, .F. ) ;
#23052=VERTEX_POINT ( 'NONE', #704 ) ;
#23053=VECTOR ( 'NONE', #13794, 1000.000000000000227 ) ;
#23054=ADVANCED_FACE ( 'NONE', ( #34925 ), #82693, .F. ) ;
#23055=ORIENTED_EDGE ( 'NONE', *, *, #41178, .T. ) ;
#23056=VECTOR ( 'NONE', #37899, 1000.000000000000000 ) ;
#23057=DIRECTION ( 'NONE',  ( 0.000000000000000000, 0.7660444431189822323, -0.6427876096865344779 ) ) ;
#23058=CARTESIAN_POINT ( 'NONE',  ( -13.63463862190834952, -5.851115903089112003, 34.47074536777953568 ) ) ;
#23059=FACE_OUTER_BOUND ( 'NONE', #44159, .T. ) ;
#23060=CARTESIAN_POINT ( 'NONE',  ( -6.923076923077044142, -3.835265460704628371, 33.15142922262033665 ) ) ;
#23061=EDGE_CURVE ( 'NONE', #60707, #14975, #24426, .T. ) ;
#23062=CYLINDRICAL_SURFACE ( 'NONE', #83192, 0.2499999999999994726 ) ;
#23063=CARTESIAN_POINT ( 'NONE',  ( 14.17700170458200404, -2.845849958028613624, 32.17971566917920967 ) ) ;
#23064=EDGE_CURVE ( 'NONE', #21870, #49519, #21420, .T. ) ;
#23066=CARTESIAN_POINT ( 'NONE',  ( -15.90384615384615330, -2.249999999999998668, 29.75000000000000355 ) ) ;
#23068=CARTESIAN_POINT ( 'NONE',  ( 5.750000000000002665, -7.500000000000001776, 35.04278698407183867 ) ) ;
#23069=CARTESIAN_POINT ( 'NONE',  ( 6.988332062589762472, -9.528491918058460186, 34.59228464037085615 ) ) ;
#23072=CARTESIAN_POINT ( 'NONE',  ( -2.307692307692305711, -1.790695186598648903, 34.54067556320373455 ) ) ;
#23073=EDGE_CURVE ( 'NONE', #2893, #55087, #68301, .T. ) ;
#23074=EDGE_LOOP ( 'NONE', ( #2642, #6997, #80684, #48968 ) ) ;
#23075=FACE_BOUND ( 'NONE', #79868, .T. ) ;
#23077=CARTESIAN_POINT ( 'NONE',  ( 18.06525513951284267, -12.70778746994558439, 30.41441678777537305 ) ) ;
#23078=CARTESIAN_POINT ( 'NONE',  ( 12.21156173059610772, -12.17611988154120972, 31.52148481390971213 ) ) ;
#23080=CARTESIAN_POINT ( 'NONE',  ( -16.28453675695646652, -11.37499894934982514, 33.29245874905763003 ) ) ;
#23081=CARTESIAN_POINT ( 'NONE',  ( 6.923076923076802558, -10.90142922262034020, 33.41473453929536674 ) ) ;
#23082=CARTESIAN_POINT ( 'NONE',  ( 0.4615384615384611200, -4.786620604624113540, 33.94971097300155094 ) ) ;
#23083=CARTESIAN_POINT ( 'NONE',  ( 1.384615384615386802, -13.57706302396349152, 30.56769352161908060 ) ) ;
#23084=VERTEX_POINT ( 'NONE', #36273 ) ;
#23085=CARTESIAN_POINT ( 'NONE',  ( -9.915234651214539952, -2.889293201056495786, 32.26117774369186009 ) ) ;
#23086=ORIENTED_EDGE ( 'NONE', *, *, #64949, .T. ) ;
#23088=VERTEX_POINT ( 'NONE', #16000 ) ;
#23089=CARTESIAN_POINT ( 'NONE',  ( -5.999999999999998224, -1.215029322943914858, 32.30358669280327177 ) ) ;
#23090=CARTESIAN_POINT ( 'NONE',  ( 15.16549923021291058, -5.094484230520674117, 34.41647553114621161 ) ) ;
#23091=CARTESIAN_POINT ( 'NONE',  ( 5.076923076923075762, -2.486705287966279876, 31.30864560766543647 ) ) ;
#23092=DIRECTION ( 'NONE',  ( 0.000000000000000000, 0.6427876096865368094, 0.7660444431189802339 ) ) ;
#23093=CARTESIAN_POINT ( 'NONE',  ( -7.911424292114620727, -9.442884908240170461, 34.35708131394840592 ) ) ;
#23097=VERTEX_POINT ( 'NONE', #57863 ) ;
#23098=CARTESIAN_POINT ( 'NONE',  ( -0.6844646790546095039, -5.667676309546437530, 34.40238873228292249 ) ) ;
#23100=ORIENTED_EDGE ( 'NONE', *, *, #67661, .F. ) ;
#23102=EDGE_LOOP ( 'NONE', ( #22158, #52142 ) ) ;
#23103=VERTEX_POINT ( 'NONE', #78576 ) ;
#23104=CARTESIAN_POINT ( 'NONE',  ( 16.82689983963011926, -5.056417327199097755, 34.11270091957320716 ) ) ;
#23106=CARTESIAN_POINT ( 'NONE',  ( 3.230769230769110045, -10.21337939537710326, 33.94971097300076224 ) ) ;
#23107=CARTESIAN_POINT ( 'NONE',  ( 9.692307692307695177, -12.37446782046654192, 30.86335684631486131 ) ) ;
#23108=CARTESIAN_POINT ( 'NONE',  ( 6.222779541268408821, -2.600157965045225339, 30.74683119005207743 ) ) ;
#23109=CARTESIAN_POINT ( 'NONE',  ( 17.93391762063986050, -11.91647553114624181, 32.58852847137148245 ) ) ;
#23110=FACE_OUTER_BOUND ( 'NONE', #33455, .T. ) ;
#23111=EDGE_LOOP ( 'NONE', ( #40234, #30434 ) ) ;
#23112=CARTESIAN_POINT ( 'NONE',  ( 3.165498784808455923, -6.879047030191174805, 34.71129190930000163 ) ) ;
#23115=CARTESIAN_POINT ( 'NONE',  ( -9.627052121031667298, -11.48612834413965977, 32.76840700105972815 ) ) ;
#23117=ORIENTED_EDGE ( 'NONE', *, *, #59459, .F. ) ;
#23118=CARTESIAN_POINT ( 'NONE',  ( 7.780071466793708979, -2.292212530054419606, 30.41441678777542634 ) ) ;
#23120=ORIENTED_EDGE ( 'NONE', *, *, #74834, .T. ) ;
#23121=CARTESIAN_POINT ( 'NONE',  ( 12.23861150263161335, -9.172386477786396597, 34.72672124145550043 ) ) ;
#23122=CYLINDRICAL_SURFACE ( 'NONE', #47418, 0.2500000000000009437 ) ;
#23123=LINE ( 'NONE', #28562, #87193 ) ;
#23124=CARTESIAN_POINT ( 'NONE',  ( 12.71159277317677549, -10.66356715214248752, 33.62249196103329751 ) ) ;
#23125=ORIENTED_EDGE ( 'NONE', *, *, #34917, .T. ) ;
#23126=CARTESIAN_POINT ( 'NONE',  ( 12.71159288145191013, -10.82426656108012075, 33.81400080652039009 ) ) ;
#23128=CARTESIAN_POINT ( 'NONE',  ( 9.442330948259101575, -2.920706130388546651, 32.31842814019191223 ) ) ;
#23129=CARTESIAN_POINT ( 'NONE',  ( 8.835299120233205628, -4.098570777380720287, 33.41473453929635440 ) ) ;
#23130=ORIENTED_EDGE ( 'NONE', *, *, #43878, .F. ) ;
#23131=CARTESIAN_POINT ( 'NONE',  ( -1.253823576790597638, -3.530189275343204702, 32.79018710029569661 ) ) ;
#23132=ORIENTED_EDGE ( 'NONE', *, *, #39125, .F. ) ;
#23133=B_SPLINE_CURVE_WITH_KNOTS ( 'NONE', 3,
 ( #28080, #55546, #83030, #21314, #48788, #76255, #14564, #85685, #15904, #57763 ),
 .UNSPECIFIED., .F., .F.,
 ( 4, 2, 2, 2, 4 ),
 ( 0.0007817359430256297891, 0.0009771253907249958896, 0.001172514838424362207, 0.001367904286123728524, 0.001563293733823094625 ),
 .UNSPECIFIED. ) ;
#23134=DIRECTION ( 'NONE',  ( 0.000000000000000000, 0.3420201433256610524, 0.9396926207859113145 ) ) ;
#23136=CARTESIAN_POINT ( 'NONE',  ( 17.07692307692307665, -8.164416787775445883, 34.95778746994557906 ) ) ;
#23137=CARTESIAN_POINT ( 'NONE',  ( -7.912236225513978205, -2.486705287966279432, 31.30864560766542937 ) ) ;
#23139=DIRECTION ( 'NONE',  ( 0.000000000000000000, 0.3420201433256610524, 0.9396926207859113145 ) ) ;
#23140=ORIENTED_EDGE ( 'NONE', *, *, #48187, .T. ) ;
#23141=VECTOR ( 'NONE', #67003, 1000.000000000000114 ) ;
#23142=ORIENTED_EDGE ( 'NONE', *, *, #15569, .F. ) ;
#23143=B_SPLINE_CURVE_WITH_KNOTS ( 'NONE', 3,
 ( #17737, #45190, #60490, #27146, #53281, #38903, #74015, #80785, #52838, #45644 ),
 .UNSPECIFIED., .F., .F.,
 ( 4, 2, 2, 2, 4 ),
 ( 0.000000000000000000, 0.0001954339857564098325, 0.0003908679715128196650, 0.0005863019572692294975, 0.0007817359430256393300 ),
 .UNSPECIFIED. ) ;
#23145=EDGE_CURVE ( 'NONE', #89080, #39107, #40402, .T. ) ;
#23146=CARTESIAN_POINT ( 'NONE',  ( -7.173076923076921574, -7.500000000000001776, 34.75000000000000000 ) ) ;
#23147=CARTESIAN_POINT ( 'NONE',  ( -9.692307692307814193, -4.320704448113951379, 33.92786785259630022 ) ) ;
#23149=B_SPLINE_CURVE_WITH_KNOTS ( 'NONE', 3,
 ( #63720, #56084, #29950, #57407, #50194, #43458, #78569, #15107, #56962, #77680 ),
 .UNSPECIFIED., .F., .F.,
 ( 4, 2, 2, 2, 4 ),
 ( 0.0007817359430256297891, 0.0009771253907249958896, 0.001172514838424361990, 0.001367904286123727874, 0.001563293733823093975 ),
 .UNSPECIFIED. ) ;
#23150=CARTESIAN_POINT ( 'NONE',  ( -12.23852561744506851, -12.38742843783360748, 31.66772728687926985 ) ) ;
#23151=B_SPLINE_CURVE_WITH_KNOTS ( 'NONE', 3,
 ( #78045, #81828, #26875, #28192, #27317, #55662, #83152, #20120, #288, #82269 ),
 .UNSPECIFIED., .F., .F.,
 ( 4, 2, 2, 2, 4 ),
 ( 0.0007817359430256372700, 0.0009771253907250054306, 0.001172514838424373483, 0.001367904286123741535, 0.001563293733823109804 ),
 .UNSPECIFIED. ) ;
#23152=CARTESIAN_POINT ( 'NONE',  ( -8.769230769230892619, -6.835583212225970762, 34.95778746994575670 ) ) ;
#23153=CARTESIAN_POINT ( 'NONE',  ( -6.923076923076922462, -3.513871655860378418, 32.76840700105978499 ) ) ;
#23154=CARTESIAN_POINT ( 'NONE',  ( 5.142991427925515779, -9.780366693483667717, 34.19971097300155805 ) ) ;
#23155=ORIENTED_EDGE ( 'NONE', *, *, #51424, .T. ) ;
#23156=ORIENTED_EDGE ( 'NONE', *, *, #54675, .T. ) ;
#23157=EDGE_LOOP ( 'NONE', ( #69740, #15255 ) ) ;
#23158=CARTESIAN_POINT ( 'NONE',  ( -3.164700879766792596, -10.51840700105979565, 33.73612834413962247 ) ) ;
#23160=CARTESIAN_POINT ( 'NONE',  ( 0.6843180028068700516, -8.496831190052093419, 34.64984203495476578 ) ) ;
#23162=CARTESIAN_POINT ( 'NONE',  ( 1.449870524128225258, -5.094484230520773593, 34.41647553114626845 ) ) ;
#23163=EDGE_CURVE ( 'NONE', #44514, #65922, #37588, .T. ) ;
#23165=EDGE_CURVE ( 'NONE', #2439, #13277, #16768, .T. ) ;
#23166=ORIENTED_EDGE ( 'NONE', *, *, #75120, .T. ) ;
#23168=EDGE_LOOP ( 'NONE', ( #53484, #50403 ) ) ;
#23169=CYLINDRICAL_SURFACE ( 'NONE', #37065, 0.2500000000000002220 ) ;
#23170=ORIENTED_EDGE ( 'NONE', *, *, #35681, .T. ) ;
#23171=FACE_BOUND ( 'NONE', #40640, .T. ) ;
#23172=CARTESIAN_POINT ( 'NONE',  ( -6.130147209438219669, -9.418419913701741919, 34.36755862841477693 ) ) ;
#23173=AXIS2_PLACEMENT_3D ( 'NONE', #67152, #74803, #21170 ) ;
#23174=VECTOR ( 'NONE', #22842, 1000.000000000000227 ) ;
#23175=EDGE_CURVE ( 'NONE', #78911, #57769, #70938, .T. ) ;
#23176=DIRECTION ( 'NONE',  ( -0.000000000000000000, 0.3420201433256694346, -0.9396926207859080948 ) ) ;
#23177=EDGE_LOOP ( 'NONE', ( #8347, #889 ) ) ;
#23178=CARTESIAN_POINT ( 'NONE',  ( -15.16470087976679615, -4.786620604624113540, 33.94971097300155805 ) ) ;
#23179=CARTESIAN_POINT ( 'NONE',  ( 4.946775107191381693, -8.630895178749536711, 34.87696386517710323 ) ) ;
#23180=CARTESIAN_POINT ( 'NONE',  ( 1.134638640566794310, -3.436278759898155233, 33.07459398097509506 ) ) ;
#23182=CARTESIAN_POINT ( 'NONE',  ( 1.607628228708781970, -2.523321265292116422, 31.42251411153756990 ) ) ;
#23183=B_SPLINE_CURVE_WITH_KNOTS ( 'NONE', 3,
 ( #58588, #44176, #45968, #11302, #45077, #66695, #71662, #10865, #65788, #66239 ),
 .UNSPECIFIED., .F., .F.,
 ( 4, 2, 2, 2, 4 ),
 ( 0.000000000000000000, 0.0001954339857564098054, 0.0003908679715128196108, 0.0005863019572692293891, 0.0007817359430256392216 ),
 .UNSPECIFIED. ) ;
#23184=CARTESIAN_POINT ( 'NONE',  ( 8.069166690247241647, -11.43677907613344757, 33.22367315496202167 ) ) ;
#23185=CARTESIAN_POINT ( 'NONE',  ( -14.05769230769087130, -7.500000000000155431, 34.75000000000007105 ) ) ;
#23186=CARTESIAN_POINT ( 'NONE',  ( 2.307692307692309264, -11.91647553114624181, 32.58852847137148245 ) ) ;
#23187=CARTESIAN_POINT ( 'NONE',  ( -6.250023237292964495, -5.851115903089112003, 34.47074536777953568 ) ) ;
#23188=CARTESIAN_POINT ( 'NONE',  ( 16.02315555073584363, -10.70098750199973203, 33.91152734681376302 ) ) ;
#23189=DIRECTION ( 'NONE',  ( 0.000000000000000000, 0.9848077530122072432, 0.1736481776669354937 ) ) ;
#23190=B_SPLINE_CURVE_WITH_KNOTS ( 'NONE', 3,
 ( #11448, #45221, #39380, #60070, #73150, #32602, #11008, #80364, #51510, #87130 ),
 .UNSPECIFIED., .F., .F.,
 ( 4, 2, 2, 2, 4 ),
 ( 0.0007817246256747459798, 0.0009771112852218896347, 0.001172497944769033181, 0.001367884604316176728, 0.001563271263863320491 ),
 .UNSPECIFIED. ) ;
#23191=CARTESIAN_POINT ( 'NONE',  ( -39.05038313613820122, -7.500000000000000000, 29.75000000000000355 ) ) ;
#23192=CARTESIAN_POINT ( 'NONE',  ( -13.44988538517170440, -4.320704448112771878, 33.92786785259540494 ) ) ;
#23194=CARTESIAN_POINT ( 'NONE',  ( -1.161835715637316913, -9.418065098278011860, 34.63729479722530158 ) ) ;
#23195=CARTESIAN_POINT ( 'NONE',  ( 16.15384615384603251, -8.656820664282941280, 34.87096338111179961 ) ) ;
#23196=CARTESIAN_POINT ( 'NONE',  ( 12.23861150263161157, -4.762599654559228846, 34.23009711892697737 ) ) ;
#23197=CARTESIAN_POINT ( 'NONE',  ( -5.934744428723973897, -12.46129190930001052, 30.37095296980870174 ) ) ;
#23199=ORIENTED_EDGE ( 'NONE', *, *, #18820, .F. ) ;
#23201=ORIENTED_EDGE ( 'NONE', *, *, #15935, .F. ) ;
#23202=CARTESIAN_POINT ( 'NONE',  ( -9.942330929600657896, -5.851115903089112003, 34.47074536777953568 ) ) ;
#23203=EDGE_LOOP ( 'NONE', ( #34193, #87536, #86989, #42875 ) ) ;
#23204=CARTESIAN_POINT ( 'NONE',  ( 17.77651505627604678, -12.24155766932282496, 31.33739205006857986 ) ) ;
#23205=ORIENTED_EDGE ( 'NONE', *, *, #35133, .F. ) ;
#23206=CARTESIAN_POINT ( 'NONE',  ( 10.61538461538461675, -2.833524468853757305, 32.15551576947925838 ) ) ;
#23208=CARTESIAN_POINT ( 'NONE',  ( -17.75005459062195712, -9.357781135181033605, 34.66075350412533851 ) ) ;
#23211=CARTESIAN_POINT ( 'NONE',  ( -17.99999999841483955, -2.249999999999995115, 29.50000000010503953 ) ) ;
#23212=CARTESIAN_POINT ( 'NONE',  ( -13.63463860883683942, -8.475808217655753651, 34.90892951860618609 ) ) ;
#23213=CARTESIAN_POINT ( 'NONE',  ( 16.15384615384603251, -11.48612834414049644, 32.76840700105863391 ) ) ;
#23215=CARTESIAN_POINT ( 'NONE',  ( -11.53846153846153655, -2.486705287966279876, 31.30864560766543647 ) ) ;
#23216=CARTESIAN_POINT ( 'NONE',  ( 9.692307692307695177, -13.53365097954675988, 30.81389545987213552 ) ) ;
#23217=AXIS2_PLACEMENT_3D ( 'NONE', #81165, #32076, #12697 ) ;
#23218=CARTESIAN_POINT ( 'NONE',  ( 10.39245765647776309, -5.582147617184174848, 34.63737895849758530 ) ) ;
#23220=B_SPLINE_CURVE_WITH_KNOTS ( 'NONE', 3,
 ( #639, #1528, #76743, #27664, #15045, #42520, #47931, #75411, #63213, #13707 ),
 .UNSPECIFIED., .F., .F.,
 ( 4, 2, 2, 2, 4 ),
 ( 0.0007817246256747445703, 0.0009771112852218872494, 0.001172497944769030145, 0.001367884604316172825, 0.001563271263863315504 ),
 .UNSPECIFIED. ) ;
#23221=CARTESIAN_POINT ( 'NONE',  ( -14.30769230769242739, -10.90142922262034020, 33.41473453929536674 ) ) ;
#23222=ORIENTED_EDGE ( 'NONE', *, *, #81657, .T. ) ;
#23223=CARTESIAN_POINT ( 'NONE',  ( -13.63463860883683942, -6.652501968072648708, 34.93155406624980941 ) ) ;
#23224=CARTESIAN_POINT ( 'NONE',  ( 11.53846153846141753, -6.026961402154118019, 34.52809138561165270 ) ) ;
#23226=CARTESIAN_POINT ( 'NONE',  ( 5.142991427925514891, -2.721908614388772296, 31.22303859784725333 ) ) ;
#23227=B_SPLINE_CURVE_WITH_KNOTS ( 'NONE', 3,
 ( #71707, #84813, #44670, #51869, #30725, #38833, #78465, #78031, #23090, #4136 ),
 .UNSPECIFIED., .F., .F.,
 ( 4, 2, 2, 2, 4 ),
 ( 0.000000000000000000, 0.0001954311564186871184, 0.0003908623128373742367, 0.0005862934692560614093, 0.0007817246256747484735 ),
 .UNSPECIFIED. ) ;
#23230=CARTESIAN_POINT ( 'NONE',  ( -8.769230769230890843, -8.613356846316285953, 34.62446782046622218 ) ) ;
#23232=CARTESIAN_POINT ( 'NONE',  ( -10.86538461538461320, -7.500000000000001776, 35.00000000000000000 ) ) ;
#23233=ORIENTED_EDGE ( 'NONE', *, *, #62958, .T. ) ;
#23234=ORIENTED_EDGE ( 'NONE', *, *, #39240, .T. ) ;
#23235=ADVANCED_FACE ( 'NONE', ( #29083 ), #56537, .F. ) ;
#23236=CARTESIAN_POINT ( 'NONE',  ( -11.28840711854808632, -11.47946981652013498, 33.17500667209847620 ) ) ;
#23237=CARTESIAN_POINT ( 'NONE',  ( -15.45369618967607828, -10.77366814457252175, 33.85459836347579454 ) ) ;
#23238=EDGE_CURVE ( 'NONE', #56029, #31297, #19950, .T. ) ;
#23239=CARTESIAN_POINT ( 'NONE',  ( 1.607394925883796510, -11.89424750095246175, 32.13594075562311758 ) ) ;
#23240=CARTESIAN_POINT ( 'NONE',  ( 7.846153846153723244, -8.656820664282941280, 34.87096338111179961 ) ) ;
#23241=ORIENTED_EDGE ( 'NONE', *, *, #55873, .T. ) ;
#23242=CYLINDRICAL_SURFACE ( 'NONE', #66577, 0.2500000000000008882 ) ;
#23243=ORIENTED_EDGE ( 'NONE', *, *, #12267, .T. ) ;
#23244=ORIENTED_EDGE ( 'NONE', *, *, #19689, .F. ) ;
#23245=ADVANCED_FACE ( 'NONE', ( #78134 ), #37141, .F. ) ;
#23246=CARTESIAN_POINT ( 'NONE',  ( -12.71153846153846168, -7.500000000000001776, 35.04278698407183867 ) ) ;
#23247=CARTESIAN_POINT ( 'NONE',  ( 16.15384615384615330, -12.37446782046654192, 30.86335684631486131 ) ) ;
#23248=CARTESIAN_POINT ( 'NONE',  ( -16.28399336328437386, -4.460286881179643004, 33.72017969459903242 ) ) ;
#23249=EDGE_CURVE ( 'NONE', #56593, #74112, #21062, .T. ) ;
#23251=LINE ( 'NONE', #50266, #88575 ) ;
#23252=VERTEX_POINT ( 'NONE', #45686 ) ;
#23253=ORIENTED_EDGE ( 'NONE', *, *, #30612, .F. ) ;
#23256=CARTESIAN_POINT ( 'NONE',  ( 11.76124120743959978, -5.827830569534417471, 34.72679350104403539 ) ) ;
#23257=VERTEX_POINT ( 'NONE', #72710 ) ;
#23259=CARTESIAN_POINT ( 'NONE',  ( 5.076923076923075762, -3.513871655860378418, 32.76840700105978499 ) ) ;
#23260=AXIS2_PLACEMENT_3D ( 'NONE', #38913, #51953, #72678 ) ;
#23261=CARTESIAN_POINT ( 'NONE',  ( -0.3954711281883859786, -9.058645607665452459, 34.76329471203371924 ) ) ;
#23262=EDGE_CURVE ( 'NONE', #68032, #33581, #80379, .T. ) ;
#23264=ADVANCED_FACE ( 'NONE', ( #66851 ), #52435, .F. ) ;
#23267=VERTEX_POINT ( 'NONE', #33066 ) ;
#23268=CARTESIAN_POINT ( 'NONE',  ( 12.46153846153846168, -1.509761064869970415, 31.06009739812519044 ) ) ;
#23269=CARTESIAN_POINT ( 'NONE',  ( -7.053224132515140354, -2.882441371585227063, 31.66841991370171527 ) ) ;
#23271=B_SPLINE_CURVE_WITH_KNOTS ( 'NONE', 3,
 ( #147, #6028, #61387, #33496, #53755, #55528, #41576, #47885, #88460, #69489 ),
 .UNSPECIFIED., .F., .F.,
 ( 4, 2, 2, 2, 4 ),
 ( 0.000000000000000000, 0.0001954311564186861968, 0.0003908623128373723936, 0.0005862934692560585904, 0.0007817246256747447872 ),
 .UNSPECIFIED. ) ;
#23272=CARTESIAN_POINT ( 'NONE',  ( 5.999999999999878320, -12.51329471203414379, 31.30864560766407578 ) ) ;
#23273=LINE ( 'NONE', #71024, #45485 ) ;
#23275=CARTESIAN_POINT ( 'NONE',  ( 4.946775867484856093, -2.619462340734462380, 30.83744416345203021 ) ) ;
#23276=CARTESIAN_POINT ( 'NONE',  ( -10.68065506134539078, -10.90142922261923886, 33.41473453929638993 ) ) ;
#23277=ORIENTED_EDGE ( 'NONE', *, *, #27358, .T. ) ;
#23279=CARTESIAN_POINT ( 'NONE',  ( -10.61538461538461320, -9.780366693483667717, 34.19971097300155094 ) ) ;
#23280=FACE_OUTER_BOUND ( 'NONE', #589, .T. ) ;
#23281=ORIENTED_EDGE ( 'NONE', *, *, #6508, .F. ) ;
#23283=CARTESIAN_POINT ( 'NONE',  ( -18.22292695890684655, -12.64616026154729411, 30.79003144601914244 ) ) ;
#23284=CARTESIAN_POINT ( 'NONE',  ( -3.230769230769229949, -3.322132147404559976, 32.92929555188717927 ) ) ;
#23285=CARTESIAN_POINT ( 'NONE',  ( -5.076923076923075762, -11.69971097300155272, 32.46337939537588113 ) ) ;
#23286=CARTESIAN_POINT ( 'NONE',  ( 7.976944287120794286, -6.369690395747422684, 34.87708834333098196 ) ) ;
#23287=CARTESIAN_POINT ( 'NONE',  ( 12.23861224402231151, -4.186968288167450147, 33.49512374952580274 ) ) ;
#23288=FACE_BOUND ( 'NONE', #28376, .T. ) ;
#23289=FACE_OUTER_BOUND ( 'NONE', #7617, .T. ) ;
#23290=CARTESIAN_POINT ( 'NONE',  ( 17.77651507543566822, -10.97335522853832934, 33.68706563782419749 ) ) ;
#23291=CYLINDRICAL_SURFACE ( 'NONE', #69849, 0.2500000000000009437 ) ;
#23292=CARTESIAN_POINT ( 'NONE',  ( -5.076923076923199218, -10.33852847137269571, 34.16647553114546554 ) ) ;
#23293=CARTESIAN_POINT ( 'NONE',  ( -15.23076923076922995, -6.386643153685126251, 34.62446782046654192 ) ) ;
#23296=AXIS2_PLACEMENT_3D ( 'NONE', #84911, #24521, #11024 ) ;
#23297=ORIENTED_EDGE ( 'NONE', *, *, #45308, .T. ) ;
#23298=AXIS2_PLACEMENT_3D ( 'NONE', #71198, #70326, #1864 ) ;
#23299=FACE_OUTER_BOUND ( 'NONE', #81843, .T. ) ;
#23300=CARTESIAN_POINT ( 'NONE',  ( -12.46153846153846168, -6.343179335718451384, 34.87096338111211935 ) ) ;
#23301=CARTESIAN_POINT ( 'NONE',  ( 5.776515075435673552, -5.827078755546623690, 34.72654668319379567 ) ) ;
#23302=CARTESIAN_POINT ( 'NONE',  ( -10.61538461538461320, -11.35647404775217417, 33.31231777344666511 ) ) ;
#23303=CARTESIAN_POINT ( 'NONE',  ( 7.780883400193070898, -5.219633306516282545, 34.19971097300152252 ) ) ;
#23305=AXIS2_PLACEMENT_3D ( 'NONE', #62539, #8062, #56682 ) ;
#23306=CARTESIAN_POINT ( 'NONE',  ( -8.519176457592452678, -2.779044189368095275, 31.39831045268885745 ) ) ;
#23307=CARTESIAN_POINT ( 'NONE',  ( 4.023155550735847186, -11.93127051446800024, 32.56575433478200665 ) ) ;
#23308=CARTESIAN_POINT ( 'NONE',  ( 11.60360631918116958, -7.750023224968867197, 34.99404313364389907 ) ) ;
#23309=CARTESIAN_POINT ( 'NONE',  ( 17.74999999999999289, -2.499999999999999556, 29.81609845454691765 ) ) ;
#23311=CARTESIAN_POINT ( 'NONE',  ( 5.076923076923075762, -8.164416787775445883, 34.95778746994557906 ) ) ;
#23312=EDGE_CURVE ( 'NONE', #48689, #86112, #69014, .T. ) ;
#23313=B_SPLINE_CURVE_WITH_KNOTS ( 'NONE', 3,
 ( #5435, #33349, #26143, #54943, #20710, #88315 ),
 .UNSPECIFIED., .F., .F.,
 ( 4, 2, 4 ),
 ( 4.563551064100006665E-17, 0.0001954756301637168570, 0.0003909512603273880690 ),
 .UNSPECIFIED. ) ;
#23314=DIRECTION ( 'NONE',  ( -0.000000000000000000, 0.3420201433256694901, -0.9396926207859082059 ) ) ;
#23315=CARTESIAN_POINT ( 'NONE',  ( 17.20771351789003489, -2.494656445102014342, 31.33466734024120015 ) ) ;
#23316=ORIENTED_EDGE ( 'NONE', *, *, #48958, .F. ) ;
#23317=CARTESIAN_POINT ( 'NONE',  ( 17.32686848630112308, -12.68172785388650681, 30.59649109432439573 ) ) ;
#23318=CARTESIAN_POINT ( 'NONE',  ( -5.934744860487160878, -2.657715359629131857, 31.77849191805844242 ) ) ;
#23320=CARTESIAN_POINT ( 'NONE',  ( 6.923076923076800782, -11.06231777344772027, 33.60647404775119895 ) ) ;
#23321=CARTESIAN_POINT ( 'NONE',  ( -16.85414340794500276, -5.827830569534415694, 34.72679350104403539 ) ) ;
#23322=ORIENTED_EDGE ( 'NONE', *, *, #71208, .T. ) ;
#23324=CARTESIAN_POINT ( 'NONE',  ( 7.846153846153725020, -2.625532179533779154, 30.86335684631627174 ) ) ;
#23325=ORIENTED_EDGE ( 'NONE', *, *, #81007, .F. ) ;
#23326=CARTESIAN_POINT ( 'NONE',  ( 6.700150705560774966, -3.105860786376062332, 32.13614157043599562 ) ) ;
#23327=CARTESIAN_POINT ( 'NONE',  ( -13.31935981333936070, -10.21337939537593620, 33.94971097300152252 ) ) ;
#23329=CARTESIAN_POINT ( 'NONE',  ( -5.326946314216044698, -12.22074536777954989, 31.39888409691088356 ) ) ;
#23330=EDGE_CURVE ( 'NONE', #61500, #39225, #12474, .T. ) ;
#23331=CARTESIAN_POINT ( 'NONE',  ( -13.51530685128294529, -3.062553014421049546, 32.05460306192773601 ) ) ;
#23332=ORIENTED_EDGE ( 'NONE', *, *, #16842, .F. ) ;
#23334=CARTESIAN_POINT ( 'NONE',  ( 8.992243613324164997, -2.308499170217967134, 30.53291367094873721 ) ) ;
#23336=CARTESIAN_POINT ( 'NONE',  ( -1.319359813339359144, -6.026961402152789304, 34.52809138561124769 ) ) ;
#23337=ORIENTED_EDGE ( 'NONE', *, *, #60697, .T. ) ;
#23338=ORIENTED_EDGE ( 'NONE', *, *, #59227, .F. ) ;
#23339=VERTEX_POINT ( 'NONE', #51986 ) ;
#23340=EDGE_CURVE ( 'NONE', #10136, #2618, #85520, .T. ) ;
#23341=CARTESIAN_POINT ( 'NONE',  ( 3.230769230769231726, -2.292212530054420494, 30.41441678777542634 ) ) ;
#23342=DIRECTION ( 'NONE',  ( -0.000000000000000000, 0.8660254037844399289, -0.4999999999999980016 ) ) ;
#23343=B_SPLINE_CURVE_WITH_KNOTS ( 'NONE', 3,
 ( #11884, #44752, #39360, #3328, #24041, #44294, #2872, #3776, #38459, #71786 ),
 .UNSPECIFIED., .F., .F.,
 ( 4, 2, 2, 2, 4 ),
 ( 0.000000000000000000, 0.0001954339857564073659, 0.0003908679715128147319, 0.0005863019572692221250, 0.0007817359430256294638 ),
 .UNSPECIFIED. ) ;
#23345=CARTESIAN_POINT ( 'NONE',  ( -3.903900744468108641, -12.68172785388650681, 30.59649109432439573 ) ) ;
#23347=ORIENTED_EDGE ( 'NONE', *, *, #52468, .F. ) ;
#23348=EDGE_CURVE ( 'NONE', #58923, #72792, #36091, .T. ) ;
#23349=ORIENTED_EDGE ( 'NONE', *, *, #81845, .F. ) ;
#23350=CARTESIAN_POINT ( 'NONE',  ( -2.241525701100665735, -7.250054591869667497, 34.99404684341514127 ) ) ;
#23351=ORIENTED_EDGE ( 'NONE', *, *, #71766, .F. ) ;
#23352=FACE_OUTER_BOUND ( 'NONE', #7878, .T. ) ;
#23355=CARTESIAN_POINT ( 'NONE',  ( -6.923076923077044142, -8.613356846316285953, 34.62446782046622218 ) ) ;
#23356=CARTESIAN_POINT ( 'NONE',  ( 8.069165197766697162, -4.887748414852792322, 34.01359900205216746 ) ) ;
#23357=ORIENTED_EDGE ( 'NONE', *, *, #43401, .F. ) ;
#23358=VECTOR ( 'NONE', #75856, 1000.000000000000000 ) ;
#23360=FACE_OUTER_BOUND ( 'NONE', #39902, .T. ) ;
#23361=VERTEX_POINT ( 'NONE', #27194 ) ;
#23362=CYLINDRICAL_SURFACE ( 'NONE', #2793, 0.2500000000000008882 ) ;
#23363=CARTESIAN_POINT ( 'NONE',  ( -10.61538461538461320, -9.058645607665452459, 34.76329471203371924 ) ) ;
#23365=ORIENTED_EDGE ( 'NONE', *, *, #5866, .T. ) ;
#23366=CARTESIAN_POINT ( 'NONE',  ( 12.68455130563185662, -6.460100341425560444, 34.89618726649961644 ) ) ;
#23367=CARTESIAN_POINT ( 'NONE',  ( 15.45354877203763522, -9.332535724633409302, 34.40230450496446934 ) ) ;
#23368=CARTESIAN_POINT ( 'NONE',  ( 10.83816415665302735, -3.755027918224367767, 33.06320215134714857 ) ) ;
#23369=FACE_BOUND ( 'NONE', #70475, .T. ) ;
#23370=CARTESIAN_POINT ( 'NONE',  ( 1.607626736228235709, -12.39991518177334129, 30.74647679643404530 ) ) ;
#23371=CARTESIAN_POINT ( 'NONE',  ( 3.930919194939304973, -2.308479472611653094, 30.53278059502174457 ) ) ;
#23372=ADVANCED_FACE ( 'NONE', ( #62298 ), #20874, .F. ) ;
#23373=LINE ( 'NONE', #65685, #9232 ) ;
#23374=CARTESIAN_POINT ( 'NONE',  ( 3.230769230769108269, -3.643525952248796163, 33.31231777344771672 ) ) ;
#23375=CARTESIAN_POINT ( 'NONE',  ( 4.284371592079798674, -2.372941743896878286, 30.88044141588254377 ) ) ;
#23376=CARTESIAN_POINT ( 'NONE',  ( -8.096177083446811196, -3.202444869320336451, 32.30641848906366675 ) ) ;
#23377=CARTESIAN_POINT ( 'NONE',  ( 10.39245765647776842, -10.77366814457252175, 33.85459836347579454 ) ) ;
#23378=ORIENTED_EDGE ( 'NONE', *, *, #33376, .T. ) ;
#23379=EDGE_CURVE ( 'NONE', #83302, #49902, #50108, .T. ) ;
#23380=CYLINDRICAL_SURFACE ( 'NONE', #50436, 0.2499999999999979738 ) ;
#23381=EDGE_LOOP ( 'NONE', ( #37069, #7529 ) ) ;
#23383=CARTESIAN_POINT ( 'NONE',  ( 7.623227628637697428, -6.503392248772476236, 34.64988816332204635 ) ) ;
#23384=CARTESIAN_POINT ( 'NONE',  ( 15.10062126103753855, -3.069018819979302926, 32.56621877034667278 ) ) ;
#23386=DIRECTION ( 'NONE',  ( 0.000000000000000000, 0.9848077530122072432, -0.1736481776669354937 ) ) ;
#23387=CARTESIAN_POINT ( 'NONE',  ( -14.17690049986752321, -2.729792928343269587, 31.24908615093345077 ) ) ;
#23388=CARTESIAN_POINT ( 'NONE',  ( 1.384615384615265343, -6.879047030192662504, 34.71129190930017927 ) ) ;
#23389=CARTESIAN_POINT ( 'NONE',  ( -2.437840277424003332, -11.66186481527757479, 32.95055677023626117 ) ) ;
#23391=CARTESIAN_POINT ( 'NONE',  ( 18.22301284409340028, -4.026326845037969449, 33.68677907613345468 ) ) ;
#23392=CARTESIAN_POINT ( 'NONE',  ( 0.4615384615383382183, -12.70778746994576025, 30.41441678777401236 ) ) ;
#23394=CARTESIAN_POINT ( 'NONE',  ( 0.3313904918067667182, -3.625366637846545448, 33.29286588640298561 ) ) ;
#23395=CYLINDRICAL_SURFACE ( 'NONE', #86655, 0.2499999999999979738 ) ;
#23396=ADVANCED_FACE ( 'NONE', ( #54651 ), #83031, .F. ) ;
#23398=ORIENTED_EDGE ( 'NONE', *, *, #80331, .F. ) ;
#23399=VERTEX_POINT ( 'NONE', #26749 ) ;
#23402=ORIENTED_EDGE ( 'NONE', *, *, #39221, .T. ) ;
#23403=CARTESIAN_POINT ( 'NONE',  ( -7.053224132515141243, -2.619462340734462380, 30.83744416345203021 ) ) ;
#23404=CARTESIAN_POINT ( 'NONE',  ( -12.23875892027004753, -10.11255958852956027, 34.01340905677048454 ) ) ;
#23405=CARTESIAN_POINT ( 'NONE',  ( -14.24162395668986747, -6.386643153685127139, 34.62446782046654192 ) ) ;
#23406=CARTESIAN_POINT ( 'NONE',  ( -15.23076923076935074, -2.892918686052166066, 31.69288490824153470 ) ) ;
#23408=CARTESIAN_POINT ( 'NONE',  ( 0.5276057948885365390, -9.058645607665452459, 34.76329471203371924 ) ) ;
#23409=ORIENTED_EDGE ( 'NONE', *, *, #12674, .F. ) ;
#23410=CARTESIAN_POINT ( 'NONE',  ( -12.46153846153858247, -10.90142922262034020, 33.41473453929536674 ) ) ;
#23411=CARTESIAN_POINT ( 'NONE',  ( -16.28399336328437386, -11.93770438780619259, 32.05411857736982029 ) ) ;
#23412=VERTEX_POINT ( 'NONE', #165 ) ;
#23414=CARTESIAN_POINT ( 'NONE',  ( -9.692307692307812417, -12.27809138561165270, 31.22303859784587132 ) ) ;
#23415=CARTESIAN_POINT ( 'NONE',  ( -2.437840277424004221, -12.70455904226513866, 30.44083106164009322 ) ) ;
#23416=EDGE_CURVE ( 'NONE', #85301, #47862, #9288, .T. ) ;
#23418=DIRECTION ( 'NONE',  ( -0.000000000000000000, -0.9396926207859092051, -0.3420201433256662704 ) ) ;
#23419=CARTESIAN_POINT ( 'NONE',  ( 9.626225312947559232, -4.661471528628507777, 34.16647553114621871 ) ) ;
#23422=EDGE_LOOP ( 'NONE', ( #54111, #66231, #82080, #33389, #68688, #8217, #22473 ) ) ;
#23423=EDGE_CURVE ( 'NONE', #48528, #313, #48789, .T. ) ;
#23424=CARTESIAN_POINT ( 'NONE',  ( 1.384615384615386802, -5.557115091759785130, 34.35708131394839171 ) ) ;
#23425=CARTESIAN_POINT ( 'NONE',  ( -1.607541602131528968, -12.15238873228291538, 31.58232369045354915 ) ) ;
#23430=CARTESIAN_POINT ( 'NONE',  ( -3.360916440207450950, -9.418419913701741919, 34.36755862841477693 ) ) ;
#23431=CARTESIAN_POINT ( 'NONE',  ( 16.08776377448601735, -4.661471528628507777, 34.16647553114621871 ) ) ;
#23432=ORIENTED_EDGE ( 'NONE', *, *, #31245, .F. ) ;
#23434=CARTESIAN_POINT ( 'NONE',  ( -1.607541602131532077, -9.886141570436013382, 34.14413921362392301 ) ) ;
#23435=ORIENTED_EDGE ( 'NONE', *, *, #70926, .T. ) ;
#23436=EDGE_CURVE ( 'NONE', #16713, #80197, #88744, .T. ) ;
#23437=CARTESIAN_POINT ( 'NONE',  ( -18.22292695890684655, -4.762599654559228846, 34.23009711892697737 ) ) ;
#23438=EDGE_LOOP ( 'NONE', ( #54762, #36441 ) ) ;
#23439=CARTESIAN_POINT ( 'NONE',  ( 6.988332062589762472, -4.320704448112861584, 33.92786785259548310 ) ) ;
#23440=CARTESIAN_POINT ( 'NONE',  ( 2.980792486720639456, -4.075325502946086864, 33.72974371597207721 ) ) ;
#23441=EDGE_CURVE ( 'NONE', #61249, #1771, #31960, .T. ) ;
#23443=CARTESIAN_POINT ( 'NONE',  ( -12.39628332202562255, -11.06231777344671130, 33.60647404775212976 ) ) ;
#23444=ORIENTED_EDGE ( 'NONE', *, *, #48187, .F. ) ;
#23445=CARTESIAN_POINT ( 'NONE',  ( -2.307692307692428724, -12.16647553114689728, 32.15551576947799362 ) ) ;
#23446=EDGE_LOOP ( 'NONE', ( #7334, #4723 ) ) ;
#23447=DIRECTION ( 'NONE',  ( -0.000000000000000000, 0.3420201433256694346, -0.9396926207859080948 ) ) ;
#23448=CARTESIAN_POINT ( 'NONE',  ( 9.692307692307570832, -4.320704448113951379, 33.92786785259630022 ) ) ;
#23449=ORIENTED_EDGE ( 'NONE', *, *, #15295, .T. ) ;
#23450=CARTESIAN_POINT ( 'NONE',  ( 8.769230769230768274, -11.16473453929635440, 33.15142922261926373 ) ) ;
#23451=DIRECTION ( 'NONE',  ( -0.000000000000000000, 0.1736481776669307198, -0.9848077530122080203 ) ) ;
#23453=DIRECTION ( 'NONE',  ( -0.000000000000000000, -0.5000000000000009992, -0.8660254037844380415 ) ) ;
#23454=AXIS2_PLACEMENT_3D ( 'NONE', #55128, #6945, #21789 ) ;
#23455=VECTOR ( 'NONE', #32255, 1000.000000000000000 ) ;
#23456=CARTESIAN_POINT ( 'NONE',  ( 20.99999999999998934, -12.75000000000000178, 29.75000000000000355 ) ) ;
#23457=CARTESIAN_POINT ( 'NONE',  ( -4.153846153846274980, -4.320704448113951379, 33.92786785259630022 ) ) ;
#23458=ORIENTED_EDGE ( 'NONE', *, *, #39622, .F. ) ;
#23459=VERTEX_POINT ( 'NONE', #43367 ) ;
#23460=FACE_BOUND ( 'NONE', #63153, .T. ) ;
#23461=ORIENTED_EDGE ( 'NONE', *, *, #24908, .F. ) ;
#23462=CARTESIAN_POINT ( 'NONE',  ( -4.826923076923062439, -2.249999999999999112, 29.81603969181031033 ) ) ;
#23463=CARTESIAN_POINT ( 'NONE',  ( 4.153846153846154188, -1.790695186598648903, 34.54067556320373455 ) ) ;
#23464=CARTESIAN_POINT ( 'NONE',  ( -2.241624974342230736, -9.905515769479277921, 34.41647553114623292 ) ) ;
#23466=EDGE_LOOP ( 'NONE', ( #74035, #52269 ) ) ;
#23467=VERTEX_POINT ( 'NONE', #52212 ) ;
#23468=CARTESIAN_POINT ( 'NONE',  ( 17.01165263096229907, -4.481592998940161721, 33.73612834413957984 ) ) ;
#23469=EDGE_LOOP ( 'NONE', ( #43969, #80975, #13611, #42541 ) ) ;
#23470=CARTESIAN_POINT ( 'NONE',  ( 15.93036121012220541, -10.11188796281391511, 34.01382737946119050 ) ) ;
#23471=B_SPLINE_CURVE_WITH_KNOTS ( 'NONE', 3,
 ( #66566, #81421, #39996, #75106, #60687, #12078, #27350, #54819, #53031, #25578 ),
 .UNSPECIFIED., .F., .F.,
 ( 4, 2, 2, 2, 4 ),
 ( 0.0007817359430256285964, 0.0009771253907249945886, 0.001172514838424360472, 0.001367904286123726356, 0.001563293733823092457 ),
 .UNSPECIFIED. ) ;
#23472=AXIS2_PLACEMENT_3D ( 'NONE', #72872, #26032, #66575 ) ;
#23473=CARTESIAN_POINT ( 'NONE',  ( 13.38461538461526601, -2.892918686052165622, 31.69288490824153470 ) ) ;
#23475=FACE_BOUND ( 'NONE', #48638, .T. ) ;
#23476=EDGE_LOOP ( 'NONE', ( #39445, #18274, #45586, #33805 ) ) ;
#23477=VECTOR ( 'NONE', #25166, 999.9999999999998863 ) ;
#23478=CARTESIAN_POINT ( 'NONE',  ( 13.13463864056679853, -10.82459398097509329, 33.81372124010185587 ) ) ;
#23481=DIRECTION ( 'NONE',  ( -0.000000000000000000, -0.1736481776669307198, -0.9848077530122080203 ) ) ;
#23482=CARTESIAN_POINT ( 'NONE',  ( 2.177001704582002262, -8.191372820521381826, 34.95448215188423546 ) ) ;
#23483=CARTESIAN_POINT ( 'NONE',  ( 11.60452988946397745, -8.120952969808772792, 34.71129190929999453 ) ) ;
#23484=ORIENTED_EDGE ( 'NONE', *, *, #37339, .T. ) ;
#23485=EDGE_CURVE ( 'NONE', #31340, #37534, #47869, .T. ) ;
#23486=CARTESIAN_POINT ( 'NONE',  ( 9.626224281351809964, -2.538708090699994813, 30.37095296980875148 ) ) ;
#23487=EDGE_LOOP ( 'NONE', ( #48656, #34798, #26915, #53745 ) ) ;
#23488=VERTEX_POINT ( 'NONE', #64069 ) ;
#23491=EDGE_CURVE ( 'NONE', #58342, #8131, #8170, .T. ) ;
#23493=CARTESIAN_POINT ( 'NONE',  ( -2.307692307692427391, -12.27809138561165270, 31.22303859784587132 ) ) ;
#23494=LINE ( 'NONE', #16740, #80380 ) ;
#23495=CARTESIAN_POINT ( 'NONE',  ( -5.999999999999998224, -12.10708131394839349, 31.69288490824020244 ) ) ;
#23498=CARTESIAN_POINT ( 'NONE',  ( 17.74997677577854560, -3.520140089381496473, 33.17453946501458262 ) ) ;
#23499=LINE ( 'NONE', #50525, #35835 ) ;
#23500=CARTESIAN_POINT ( 'NONE',  ( 5.206970683178758108, -7.723484964179500700, 34.74522123443823318 ) ) ;
#23501=ORIENTED_EDGE ( 'NONE', *, *, #50205, .T. ) ;
#23502=ADVANCED_FACE ( 'NONE', ( #51753 ), #8705, .F. ) ;
#23503=VERTEX_POINT ( 'NONE', #63633 ) ;
#23504=FACE_BOUND ( 'NONE', #1732, .T. ) ;
#23505=CARTESIAN_POINT ( 'NONE',  ( 18.22277966897806678, -12.69155399931963046, 30.53255429739158444 ) ) ;
#23506=CARTESIAN_POINT ( 'NONE',  ( -11.40793583669797329, -11.93748526763465279, 32.05452791011430946 ) ) ;
#23507=ORIENTED_EDGE ( 'NONE', *, *, #80603, .F. ) ;
#23508=B_SPLINE_CURVE_WITH_KNOTS ( 'NONE', 3,
 ( #86516, #52701, #4975, #81087, #38311, #5420, #11281, #59907, #73878, #60797 ),
 .UNSPECIFIED., .F., .F.,
 ( 4, 2, 2, 2, 4 ),
 ( 0.000000000000000000, 0.0001954339857564073659, 0.0003908679715128147319, 0.0005863019572692221250, 0.0007817359430256294638 ),
 .UNSPECIFIED. ) ;
#23509=CARTESIAN_POINT ( 'NONE',  ( -16.28399412357785181, -11.66186481527757479, 32.95055677023626117 ) ) ;
#23510=CARTESIAN_POINT ( 'NONE',  ( -10.83886955910856464, -6.760086850603066466, 34.69517049084099369 ) ) ;
#23511=CARTESIAN_POINT ( 'NONE',  ( -9.915792636031639518, -3.236172620538810385, 32.36188796281390267 ) ) ;
#23512=CARTESIAN_POINT ( 'NONE',  ( -6.700065571464075553, -3.105924265160262543, 32.13625925475356127 ) ) ;
#23513=VERTEX_POINT ( 'NONE', #24292 ) ;
#23514=B_SPLINE_CURVE_WITH_KNOTS ( 'NONE', 3,
 ( #86535, #73899, #24810, #11753, #66692, #25710 ),
 .UNSPECIFIED., .F., .F.,
 ( 4, 2, 4 ),
 ( 0.0003909512603273778233, 0.0005862562993132030805, 0.0007815613382990282835 ),
 .UNSPECIFIED. ) ;
#23515=B_SPLINE_CURVE_WITH_KNOTS ( 'NONE', 3,
 ( #84513, #62442, #57019, #69656, #22354, #21016, #77738, #83636, #69217, #62879 ),
 .UNSPECIFIED., .F., .F.,
 ( 4, 2, 2, 2, 4 ),
 ( 0.0007817359430256320659, 0.0009771253907249987086, 0.001172514838424365460, 0.001367904286123731994, 0.001563293733823098745 ),
 .UNSPECIFIED. ) ;
#23516=DIRECTION ( 'NONE',  ( -0.000000000000000000, -0.7660444431189791237, -0.6427876096865379196 ) ) ;
#23518=ORIENTED_EDGE ( 'NONE', *, *, #58018, .T. ) ;
#23519=CARTESIAN_POINT ( 'NONE',  ( 13.60739505359345181, -8.540255544307065350, 34.89611431652622286 ) ) ;
#23521=FACE_OUTER_BOUND ( 'NONE', #25080, .T. ) ;
#23522=CARTESIAN_POINT ( 'NONE',  ( 3.903869422903799347, -6.567427716900047230, 34.66269422305636283 ) ) ;
#23523=CARTESIAN_POINT ( 'NONE',  ( 23.00000000000000000, -7.500000000000000000, 29.75000000000000355 ) ) ;
#23524=CARTESIAN_POINT ( 'NONE',  ( -14.98076923076929390, -7.565270000091922853, 34.99999999999999289 ) ) ;
#23526=CARTESIAN_POINT ( 'NONE',  ( -9.915234651214536399, -11.98009711892699514, 32.48740034544076138 ) ) ;
#23528=VERTEX_POINT ( 'NONE', #17555 ) ;
#23530=CARTESIAN_POINT ( 'NONE',  ( 10.61538461538461675, -1.242168528481310874, 33.36296068462461051 ) ) ;
#23531=CARTESIAN_POINT ( 'NONE',  ( 7.846153846153846700, -1.367168528481310208, 33.57946703557072254 ) ) ;
#23532=ORIENTED_EDGE ( 'NONE', *, *, #69211, .F. ) ;
#23534=CARTESIAN_POINT ( 'NONE',  ( 17.07692307692307665, -4.786620604624113540, 33.94971097300155094 ) ) ;
#23535=CARTESIAN_POINT ( 'NONE',  ( 11.40777093535123043, -4.684245665217972032, 34.18127051446801090 ) ) ;
#23536=CARTESIAN_POINT ( 'NONE',  ( -17.20761454359064047, -8.999036380462719364, 34.52022231692819076 ) ) ;
#23537=CARTESIAN_POINT ( 'NONE',  ( 0.3962155460462854495, -7.749976743299137993, 34.99404534957040624 ) ) ;
#23539=EDGE_CURVE ( 'NONE', #65380, #35523, #15017, .T. ) ;
#23540=CARTESIAN_POINT ( 'NONE',  ( 16.37662582282421653, -3.563462043263029955, 33.22394488606062879 ) ) ;
#23541=CARTESIAN_POINT ( 'NONE',  ( -7.846153846153844924, -3.886160181151819604, 36.00935417666054406 ) ) ;
#23543=CARTESIAN_POINT ( 'NONE',  ( 3.230769230769110045, -6.879047030192662504, 34.71129190930017927 ) ) ;
#23544=CARTESIAN_POINT ( 'NONE',  ( -0.4615384615385826339, -8.613356846316285953, 34.62446782046622218 ) ) ;
#23545=AXIS2_PLACEMENT_3D ( 'NONE', #25028, #73681, #79979 ) ;
#23546=ADVANCED_FACE ( 'NONE', ( #45457 ), #42490, .F. ) ;
#23547=EDGE_CURVE ( 'NONE', #77538, #31266, #31507, .T. ) ;
#23548=CARTESIAN_POINT ( 'NONE',  ( -9.692307692307691624, -11.16473453929635440, 33.15142922261926373 ) ) ;
#23549=DIRECTION ( 'NONE',  ( 0.000000000000000000, 0.000000000000000000, 1.000000000000000000 ) ) ;
#23550=B_SPLINE_CURVE_WITH_KNOTS ( 'NONE', 3,
 ( #65242, #51714, #79216, #87326, #3540, #25152, #24709, #31466, #25601, #58932 ),
 .UNSPECIFIED., .F., .F.,
 ( 4, 2, 2, 2, 4 ),
 ( 0.0007817246256747444619, 0.0009771112852218868158, 0.001172497944769029061, 0.001367884604316171523, 0.001563271263863313769 ),
 .UNSPECIFIED. ) ;
#23551=EDGE_LOOP ( 'NONE', ( #37212, #3508, #72425, #28254 ) ) ;
#23552=CARTESIAN_POINT ( 'NONE',  ( -17.29978933998617663, -2.251424796025575770, 29.88072029997477586 ) ) ;
#23553=B_SPLINE_CURVE_WITH_KNOTS ( 'NONE', 3,
 ( #433, #76534, #54480, #68880, #14385, #83743, #16485, #21135, #75213, #34660 ),
 .UNSPECIFIED., .F., .F.,
 ( 4, 2, 2, 2, 4 ),
 ( 0.0007817246256747460882, 0.0009771112852218892010, 0.001172497944769032314, 0.001367884604316175427, 0.001563271263863318539 ),
 .UNSPECIFIED. ) ;
#23554=AXIS2_PLACEMENT_3D ( 'NONE', #53957, #19733, #74686 ) ;
#23555=ORIENTED_EDGE ( 'NONE', *, *, #57239, .T. ) ;
#23556=B_SPLINE_CURVE_WITH_KNOTS ( 'NONE', 3,
 ( #72824, #3477, #44907, #65617, #85026, #23308, #85908, #50767, #31404, #85463 ),
 .UNSPECIFIED., .F., .F.,
 ( 4, 2, 2, 2, 4 ),
 ( 0.000000000000000000, 0.0001954311584214072381, 0.0003908623168428144762, 0.0005862934752642217414, 0.0007817246336856289524 ),
 .UNSPECIFIED. ) ;
#23557=CARTESIAN_POINT ( 'NONE',  ( 0.5276068125408986953, -8.973038597847269315, 34.52809138561122637 ) ) ;
#23558=CARTESIAN_POINT ( 'NONE',  ( 1.450682717965460666, -3.322132147404559976, 32.92929555188717927 ) ) ;
#23559=DIRECTION ( 'NONE',  ( -0.000000000000000000, -0.000000000000000000, -1.000000000000000000 ) ) ;
#23560=CARTESIAN_POINT ( 'NONE',  ( 6.066067333350077639, -12.62096338111211757, 30.90682066428152908 ) ) ;
#23561=EDGE_LOOP ( 'NONE', ( #36422, #58633 ) ) ;
#23562=B_SPLINE_CURVE_WITH_KNOTS ( 'NONE', 3,
 ( #64201, #2948, #84947, #63768, #85833, #2071, #15595, #29994, #43063, #23230 ),
 .UNSPECIFIED., .F., .F.,
 ( 4, 2, 2, 2, 4 ),
 ( 0.000000000000000000, 0.0001954339857564078809, 0.0003908679715128157619, 0.0005863019572692236428, 0.0007817359430256315238 ),
 .UNSPECIFIED. ) ;
#23563=CARTESIAN_POINT ( 'NONE',  ( -1.634592128663974409, -12.65889640711025521, 30.72598325615533454 ) ) ;
#23564=EDGE_CURVE ( 'NONE', #25175, #10551, #38711, .T. ) ;
#23565=CARTESIAN_POINT ( 'NONE',  ( 10.54930223602447903, -12.62096338111211580, 30.90682066428152908 ) ) ;
#23566=CARTESIAN_POINT ( 'NONE',  ( -17.29978849912671635, -2.501496062324912284, 29.88072118266895671 ) ) ;
#23567=CARTESIAN_POINT ( 'NONE',  ( -9.692307692307814193, -3.643525952248795718, 33.31231777344771672 ) ) ;
#23568=EDGE_CURVE ( 'NONE', #85757, #52397, #80096, .T. ) ;
#23569=EDGE_CURVE ( 'NONE', #67226, #9533, #7041, .T. ) ;
#23570=ORIENTED_EDGE ( 'NONE', *, *, #16281, .F. ) ;
#23571=CARTESIAN_POINT ( 'NONE',  ( -1.161604033002534342, -3.587049720035815348, 32.86302985866382897 ) ) ;
#23573=EDGE_CURVE ( 'NONE', #69827, #63622, #13589, .T. ) ;
#23574=DIRECTION ( 'NONE',  ( -0.000000000000000000, 1.000000000000000000, -0.000000000000000000 ) ) ;
#23575=CARTESIAN_POINT ( 'NONE',  ( 6.923076923076800782, -3.083524468854526912, 32.58852847137268327 ) ) ;
#23576=CARTESIAN_POINT ( 'NONE',  ( -6.130147209438218781, -2.619462340734462380, 30.83744416345203021 ) ) ;
#23577=DIRECTION ( 'NONE',  ( 0.000000000000000000, 0.1736481776669267785, -0.9848077530122087975 ) ) ;
#23578=LINE ( 'NONE', #59586, #39324 ) ;
#23579=ORIENTED_EDGE ( 'NONE', *, *, #62389, .F. ) ;
#23580=VECTOR ( 'NONE', #475, 1000.000000000000114 ) ;
#23581=EDGE_LOOP ( 'NONE', ( #30242, #11026 ) ) ;
#23582=ORIENTED_EDGE ( 'NONE', *, *, #11988, .F. ) ;
#23583=ORIENTED_EDGE ( 'NONE', *, *, #79497, .F. ) ;
#23585=CARTESIAN_POINT ( 'NONE',  ( 16.08857615328984281, -5.941354392334501355, 34.76329471203369792 ) ) ;
#23587=CARTESIAN_POINT ( 'NONE',  ( 17.29993442853592711, -4.187068189119696804, 33.49521262558774026 ) ) ;
#23589=EDGE_CURVE ( 'NONE', #41513, #5871, #53997, .T. ) ;
#23590=CARTESIAN_POINT ( 'NONE',  ( -12.59222906464876957, -12.35290016733513951, 31.75349464988449455 ) ) ;
#23591=CARTESIAN_POINT ( 'NONE',  ( 13.38461538461538680, -10.89733346790207413, 36.13435417666054406 ) ) ;
#23592=CARTESIAN_POINT ( 'NONE',  ( 9.468822767743363400, -10.23692288466677880, 34.23039457007281072 ) ) ;
#23593=VERTEX_POINT ( 'NONE', #40064 ) ;
#23594=VERTEX_POINT ( 'NONE', #60309 ) ;
#23595=VERTEX_POINT ( 'NONE', #18447 ) ;
#23597=ORIENTED_EDGE ( 'NONE', *, *, #62647, .F. ) ;
#23598=LINE ( 'NONE', #84878, #33091 ) ;
#23599=CARTESIAN_POINT ( 'NONE',  ( -16.21911659980693443, -10.21337939537584383, 33.94971097300158647 ) ) ;
#23600=EDGE_CURVE ( 'NONE', #19490, #12209, #55370, .T. ) ;
#23601=CARTESIAN_POINT ( 'NONE',  ( -1.608100309179715470, -4.988325925672468131, 34.36044203135681130 ) ) ;
#23602=CARTESIAN_POINT ( 'NONE',  ( -11.47239420511146513, -9.058645607665452459, 34.76329471203371924 ) ) ;
#23603=ORIENTED_EDGE ( 'NONE', *, *, #1005, .F. ) ;
#23604=ORIENTED_EDGE ( 'NONE', *, *, #4207, .T. ) ;
#23606=EDGE_LOOP ( 'NONE', ( #79447, #67059 ) ) ;
#23607=FACE_BOUND ( 'NONE', #81231, .T. ) ;
#23611=CARTESIAN_POINT ( 'NONE',  ( 15.90386942290380290, -6.567427716900048118, 34.66269422305636283 ) ) ;
#23613=CARTESIAN_POINT ( 'NONE',  ( -14.08491263871424160, -8.540255544307065350, 34.89611431652622286 ) ) ;
#23614=CARTESIAN_POINT ( 'NONE',  ( 4.826899852701619587, -8.475808217655753651, 34.90892951860618609 ) ) ;
#23615=CARTESIAN_POINT ( 'NONE',  ( -9.692307692307812417, -3.300289026999228881, 32.46337939537708905 ) ) ;
#23616=ORIENTED_EDGE ( 'NONE', *, *, #18601, .T. ) ;
#23617=FACE_OUTER_BOUND ( 'NONE', #27603, .T. ) ;
#23620=B_SPLINE_CURVE_WITH_KNOTS ( 'NONE', 3,
 ( #73911, #13530, #27490, #75241, #88771, #87435, #27047, #48195, #19844, #47309 ),
 .UNSPECIFIED., .F., .F.,
 ( 4, 2, 2, 2, 4 ),
 ( 0.000000000000000000, 0.0001954311564186882026, 0.0003908623128373764051, 0.0005862934692560646619, 0.0007817246256747528103 ),
 .UNSPECIFIED. ) ;
#23621=ADVANCED_FACE ( 'NONE', ( #25643 ), #53099, .F. ) ;
#23622=CARTESIAN_POINT ( 'NONE',  ( 3.361561038594017337, -8.147973898785416225, 34.70805048591653730 ) ) ;
#23623=B_SPLINE_CURVE_WITH_KNOTS ( 'NONE', 3,
 ( #9868, #17070, #37783, #22940, #36894, #38231, #65249, #64356, #31018, #51721 ),
 .UNSPECIFIED., .F., .F.,
 ( 4, 2, 2, 2, 4 ),
 ( 0.000000000000000000, 0.0001954311564186871726, 0.0003908623128373743452, 0.0005862934692560615177, 0.0007817246256747486903 ),
 .UNSPECIFIED. ) ;
#23624=DIRECTION ( 'NONE',  ( 0.000000000000000000, -6.938893903907222067E-15, 1.000000000000000000 ) ) ;
#23625=CARTESIAN_POINT ( 'NONE',  ( 3.453548772037639214, -4.387253974876676565, 33.66317474335728832 ) ) ;
#23626=CARTESIAN_POINT ( 'NONE',  ( -2.373775718648187816, -2.538708090699994813, 30.37095296980875148 ) ) ;
#23627=CARTESIAN_POINT ( 'NONE',  ( -8.769230769230890843, -9.442884908241554243, 34.35708131394783038 ) ) ;
#23628=FACE_OUTER_BOUND ( 'NONE', #29795, .T. ) ;
#23629=CARTESIAN_POINT ( 'NONE',  ( 7.976944287120800503, -2.845873456487966635, 32.17976146951972538 ) ) ;
#23630=CARTESIAN_POINT ( 'NONE',  ( 4.946231610255517275, -12.38065189839062263, 30.83690757178629482 ) ) ;
#23631=CARTESIAN_POINT ( 'NONE',  ( 11.28846153846154010, -7.433932668274256805, 35.00000000000000711 ) ) ;
#23632=CARTESIAN_POINT ( 'NONE',  ( 1.607394925883794068, -11.41317474335729187, 32.86274602512330034 ) ) ;
#23633=DIRECTION ( 'NONE',  ( -0.000000000000000000, -1.000000000000000000, 3.491481338843133355E-15 ) ) ;
#23634=CARTESIAN_POINT ( 'NONE',  ( 0.4615384615384611755, -12.78798330534102767, 29.49999999999997868 ) ) ;
#23635=CARTESIAN_POINT ( 'NONE',  ( -6.923076923076922462, -13.75783147151868846, 33.36296068462461051 ) ) ;
#23637=ORIENTED_EDGE ( 'NONE', *, *, #41649, .F. ) ;
#23638=CARTESIAN_POINT ( 'NONE',  ( 14.30769230769218758, -5.219633306517616589, 34.19971097300220464 ) ) ;
#23639=ORIENTED_EDGE ( 'NONE', *, *, #11162, .T. ) ;
#23640=CARTESIAN_POINT ( 'NONE',  ( -2.530619266599154926, -2.889293201056495786, 32.26117774369186009 ) ) ;
#23641=EDGE_LOOP ( 'NONE', ( #27885, #42942 ) ) ;
#23643=CARTESIAN_POINT ( 'NONE',  ( -13.25408994638174320, -2.372941743896879174, 30.88044141588253666 ) ) ;
#23644=ORIENTED_EDGE ( 'NONE', *, *, #63207, .F. ) ;
#23647=CARTESIAN_POINT ( 'NONE',  ( 17.07692307692307665, -8.120952969808772792, 34.71129190930000163 ) ) ;
#23649=CYLINDRICAL_SURFACE ( 'NONE', #84144, 0.2499999999999994726 ) ;
#23650=CARTESIAN_POINT ( 'NONE',  ( 13.63466980452883703, -2.920487667080175598, 32.31805714834170828 ) ) ;
#23651=CARTESIAN_POINT ( 'NONE',  ( -6.250023224221458840, -2.588893531581426544, 31.60682220781847818 ) ) ;
#23654=CARTESIAN_POINT ( 'NONE',  ( 1.254467414883689624, -5.070767119584671967, 34.40440758774516183 ) ) ;
#23657=CARTESIAN_POINT ( 'NONE',  ( 1.253923917947829869, -2.729777683071817229, 31.24903638046269094 ) ) ;
#23658=CARTESIAN_POINT ( 'NONE',  ( -15.00775787915638304, -2.554770724473667265, 30.48948780036025852 ) ) ;
#23659=EDGE_CURVE ( 'NONE', #26583, #73759, #39619, .T. ) ;
#23660=CARTESIAN_POINT ( 'NONE',  ( 15.23076923076923173, -13.75783147151868846, 33.36296068462461051 ) ) ;
#23662=ORIENTED_EDGE ( 'NONE', *, *, #37339, .F. ) ;
#23664=CARTESIAN_POINT ( 'NONE',  ( -2.307692307692305711, -1.466349020453238561, 30.81389545987213907 ) ) ;
#23665=FACE_OUTER_BOUND ( 'NONE', #54923, .T. ) ;
#23666=CARTESIAN_POINT ( 'NONE',  ( 15.90384615384615330, -7.500000000000001776, 35.00000000000000000 ) ) ;
#23667=CARTESIAN_POINT ( 'NONE',  ( 4.023698184114459231, -3.625366637846544560, 33.29286588640298561 ) ) ;
#23668=CARTESIAN_POINT ( 'NONE',  ( 9.692307692307572609, -11.48612834414049644, 32.76840700105863391 ) ) ;
#23669=EDGE_CURVE ( 'NONE', #39542, #69896, #81931, .T. ) ;
#23670=VECTOR ( 'NONE', #46771, 999.9999999999998863 ) ;
#23671=ORIENTED_EDGE ( 'NONE', *, *, #50931, .T. ) ;
#23672=CYLINDRICAL_SURFACE ( 'NONE', #31435, 0.2499999999999998890 ) ;
#23673=ORIENTED_EDGE ( 'NONE', *, *, #39597, .F. ) ;
#23674=CIRCLE ( 'NONE', #40858, 0.2500000000000002220 ) ;
#23675=ORIENTED_EDGE ( 'NONE', *, *, #43087, .F. ) ;
#23677=AXIS2_PLACEMENT_3D ( 'NONE', #22642, #56871, #44223 ) ;
#23678=CARTESIAN_POINT ( 'NONE',  ( -6.673131513698878692, -5.766571408460171355, 34.70601412856602508 ) ) ;
#23679=CARTESIAN_POINT ( 'NONE',  ( 6.792386319966615460, -2.845849958028613624, 32.17971566917920967 ) ) ;
#23680=CARTESIAN_POINT ( 'NONE',  ( -13.16183584334697265, -9.332535724633409302, 34.40230450496446934 ) ) ;
#23681=CARTESIAN_POINT ( 'NONE',  ( 10.86533002476265963, -10.18230066228895758, 34.26354781536631577 ) ) ;
#23682=ORIENTED_EDGE ( 'NONE', *, *, #31899, .T. ) ;
#23684=ORIENTED_EDGE ( 'NONE', *, *, #33807, .F. ) ;
#23685=ORIENTED_EDGE ( 'NONE', *, *, #66802, .F. ) ;
#23686=CARTESIAN_POINT ( 'NONE',  ( -4.023055712879203938, -11.93129842949671726, 32.56571108434900452 ) ) ;
#23687=CARTESIAN_POINT ( 'NONE',  ( 3.230769230769231726, -8.810774026931790459, 35.74407628777942847 ) ) ;
#23688=CARTESIAN_POINT ( 'NONE',  ( -16.15384615384627409, -4.481592998941358097, 33.73612834414048933 ) ) ;
#23690=CARTESIAN_POINT ( 'NONE',  ( -4.219116599806928214, -8.613356846314824011, 34.62446782046655613 ) ) ;
#23691=CARTESIAN_POINT ( 'NONE',  ( -16.15384615384615330, -2.721908614388771852, 31.22303859784724978 ) ) ;
#23692=ORIENTED_EDGE ( 'NONE', *, *, #71060, .F. ) ;
#23693=ORIENTED_EDGE ( 'NONE', *, *, #81873, .F. ) ;
#23695=EDGE_LOOP ( 'NONE', ( #46066, #67480, #5390, #31376, #48255, #32943, #76519, #30634, #51723, #50102, #25768, #75509, #30461, #82905, #47258, #66350, #9493, #72104, #59483, #32147, #44495, #26277, #53719, #15535, #62679, #48289, #11606, #74479, #44768, #60847, #15613, #76579, #29876, #71568, #53358, #84314, #46983, #68454, #68968, #22259, #28892, #39463, #15334, #18548, #33675, #4124, #25022, #35002, #5412, #56466, #59032, #43872, #52587, #46270, #54020, #64034, #42749, #87764, #79845, #77123, #33806, #2340, #84120, #36529, #8976, #87857, #88234, #1548, #32342, #33169, #68351, #40906, #1417, #56705, #424, #30384, #78780, #63942, #21260, #38792, #65097, #64771, #15055, #21480, #74928, #42891, #39611, #6832, #46098, #2142, #5293, #62839, #32499, #36426, #74583, #38107, #39791, #48850, #49229, #51288, #79843, #16042, #11980, #84096, #78583, #63777, #41885, #15229, #68225, #56526, #46583, #84508, #52257, #44160, #54273, #53151, #4847, #73176, #19998, #18879, #78834, #60733, #18203, #60679, #60851, #16774, #37516, #2247 ) ) ;
#23696=CARTESIAN_POINT ( 'NONE',  ( -5.776988648387152203, -3.105924265160262543, 32.13625925475356127 ) ) ;
#23697=ORIENTED_EDGE ( 'NONE', *, *, #87144, .T. ) ;
#23699=DIRECTION ( 'NONE',  ( -0.000000000000000000, 0.9396926207859092051, -0.3420201433256662704 ) ) ;
#23700=CARTESIAN_POINT ( 'NONE',  ( -4.153846153846273204, -10.90142922262034020, 33.41473453929536674 ) ) ;
#23701=EDGE_LOOP ( 'NONE', ( #61050, #37903 ) ) ;
#23702=CARTESIAN_POINT ( 'NONE',  ( -13.38461538461538325, -12.10708131394839349, 31.69288490824020244 ) ) ;
#23704=CARTESIAN_POINT ( 'NONE',  ( 2.530703659305159725, -9.086983370893047862, 34.49168942202179267 ) ) ;
#23705=CARTESIAN_POINT ( 'NONE',  ( 10.86533013373275658, -9.272278438253398036, 34.42582936511637115 ) ) ;
#23706=CARTESIAN_POINT ( 'NONE',  ( -15.16470189741915675, -2.833524468853757305, 32.15551576947925838 ) ) ;
#23707=CARTESIAN_POINT ( 'NONE',  ( -6.792551221313360088, -12.45806712695776319, 30.39783852428763922 ) ) ;
#23709=CARTESIAN_POINT ( 'NONE',  ( -1.254089946381740095, -8.630441415882550871, 34.87705825610312615 ) ) ;
#23710=CARTESIAN_POINT ( 'NONE',  ( -10.61538461538461320, -10.51840700105979565, 33.73612834413961536 ) ) ;
#23712=FACE_OUTER_BOUND ( 'NONE', #8861, .T. ) ;
#23713=CARTESIAN_POINT ( 'NONE',  ( -4.153846153846152411, -12.37446782046654192, 30.86335684631486131 ) ) ;
#23714=B_SPLINE_CURVE_WITH_KNOTS ( 'NONE', 3,
 ( #1518, #62753, #55563, #83051, #29002, #1071, #28549, #56009, #21784, #10489 ),
 .UNSPECIFIED., .F., .F.,
 ( 4, 2, 2, 2, 4 ),
 ( 0.000000000000000000, 0.0001954339857564096699, 0.0003908679715128193398, 0.0005863019572692289554, 0.0007817359430256386795 ),
 .UNSPECIFIED. ) ;
#23715=ORIENTED_EDGE ( 'NONE', *, *, #18813, .F. ) ;
#23716=DIRECTION ( 'NONE',  ( -0.000000000000000000, -0.5000000000000009992, -0.8660254037844380415 ) ) ;
#23717=CARTESIAN_POINT ( 'NONE',  ( 15.36156103859402222, -4.118422570099828484, 33.43335022499816489 ) ) ;
#23718=CARTESIAN_POINT ( 'NONE',  ( 15.93036122928182330, -6.716662450894490988, 34.94144148231605840 ) ) ;
#23719=DIRECTION ( 'NONE',  ( -0.000000000000000000, 0.3420201433256694346, -0.9396926207859080948 ) ) ;
#23720=CARTESIAN_POINT ( 'NONE',  ( 17.77651505627605033, -5.912607949931405038, 34.49155766932282319 ) ) ;
#23721=CARTESIAN_POINT ( 'NONE',  ( -7.715315515667081847, -7.277220318596959281, 34.99547417642776992 ) ) ;
#23722=AXIS2_PLACEMENT_3D ( 'NONE', #54874, #49879, #28281 ) ;
#23723=FACE_BOUND ( 'NONE', #31987, .T. ) ;
#23725=CARTESIAN_POINT ( 'NONE',  ( 17.86985203026830504, -11.04286588640298916, 33.62463336215343901 ) ) ;
#23726=CARTESIAN_POINT ( 'NONE',  ( -6.700065571464074665, -10.61302985866383963, 33.66295027996417843 ) ) ;
#23727=CARTESIAN_POINT ( 'NONE',  ( 3.100077764101675015, -4.118384482072085184, 33.43331474514187107 ) ) ;
#23728=CARTESIAN_POINT ( 'NONE',  ( 9.692307692307695177, -4.098570777380720287, 33.41473453929634729 ) ) ;
#23729=DIRECTION ( 'NONE',  ( 0.000000000000000000, 0.6427876096865368094, 0.7660444431189802339 ) ) ;
#23730=DIRECTION ( 'NONE',  ( -0.000000000000000000, -0.7660444431189791237, -0.6427876096865379196 ) ) ;
#23734=EDGE_CURVE ( 'NONE', #18984, #11766, #2713, .T. ) ;
#23736=CARTESIAN_POINT ( 'NONE',  ( -4.153846153846152411, -3.050289026998446396, 32.03036669348365706 ) ) ;
#23737=DIRECTION ( 'NONE',  ( -0.000000000000000000, -0.5000000000000009992, -0.8660254037844380415 ) ) ;
#23738=CARTESIAN_POINT ( 'NONE',  ( -9.942284423250047354, -10.66389620160130036, 33.62221079203477103 ) ) ;
#23739=ADVANCED_FACE ( 'NONE', ( #36392 ), #69293, .F. ) ;
#23740=CARTESIAN_POINT ( 'NONE',  ( 7.716006636715625255, -5.195881422630167279, 34.18770438780618548 ) ) ;
#23741=CARTESIAN_POINT ( 'NONE',  ( -16.94639763868943660, -8.630441415882549094, 34.87705825610312615 ) ) ;
#23743=FACE_OUTER_BOUND ( 'NONE', #73036, .T. ) ;
#23744=CARTESIAN_POINT ( 'NONE',  ( 0.6845498131513103601, -3.587049720035815348, 32.86302985866382897 ) ) ;
#23745=LINE ( 'NONE', #58414, #48962 ) ;
#23746=CARTESIAN_POINT ( 'NONE',  ( -6.923076923076922462, -2.517432740324522911, 35.29906147534542527 ) ) ;
#23747=CARTESIAN_POINT ( 'NONE',  ( -17.01085574357299990, -4.661471528628508665, 34.16647553114624003 ) ) ;
#23748=CARTESIAN_POINT ( 'NONE',  ( 10.86538461538461853, -2.499999999999999556, 29.81604066197449754 ) ) ;
#23750=EDGE_CURVE ( 'NONE', #2835, #4529, #25386, .T. ) ;
#23752=ORIENTED_EDGE ( 'NONE', *, *, #66981, .F. ) ;
#23753=CARTESIAN_POINT ( 'NONE',  ( 3.296836564119307589, -12.34228464037088813, 31.77849191805839268 ) ) ;
#23754=CARTESIAN_POINT ( 'NONE',  ( -5.869474561766359066, -2.647132371071621471, 31.75357179365173010 ) ) ;
#23756=CARTESIAN_POINT ( 'NONE',  ( -2.557715531913763218, -4.931416488878823223, 34.32920672191015399 ) ) ;
#23757=FACE_OUTER_BOUND ( 'NONE', #56804, .T. ) ;
#23758=EDGE_LOOP ( 'NONE', ( #36916, #32956 ) ) ;
#23759=CARTESIAN_POINT ( 'NONE',  ( -6.857821783564084228, -10.33852847137154107, 34.16647553114620450 ) ) ;
#23760=CARTESIAN_POINT ( 'NONE',  ( -11.53846153846153655, -11.69971097300155272, 32.46337939537588113 ) ) ;
#23762=VERTEX_POINT ( 'NONE', #54890 ) ;
#23763=CARTESIAN_POINT ( 'NONE',  ( 6.792929713638703682, -3.285722584762969856, 32.44110544564090759 ) ) ;
#23764=LINE ( 'NONE', #36846, #29690 ) ;
#23765=CARTESIAN_POINT ( 'NONE',  ( 17.07692307692307665, -6.189225973068211317, 35.74407628777942847 ) ) ;
#23766=CIRCLE ( 'NONE', #65441, 0.2500000000000002220 ) ;
#23767=CYLINDRICAL_SURFACE ( 'NONE', #25612, 0.2500000000000009437 ) ;
#23768=VERTEX_POINT ( 'NONE', #22427 ) ;
#23769=CARTESIAN_POINT ( 'NONE',  ( -11.66915300512910214, -4.118384482072085184, 33.43331474514187107 ) ) ;
#23770=ADVANCED_FACE ( 'NONE', ( #76493 ), #7592, .T. ) ;
#23771=DIRECTION ( 'NONE',  ( -0.000000000000000000, 0.9396926207859093161, -0.3420201433256663259 ) ) ;
#23772=ORIENTED_EDGE ( 'NONE', *, *, #26671, .T. ) ;
#23774=EDGE_LOOP ( 'NONE', ( #38578, #62793, #29612, #65634 ) ) ;
#23775=ADVANCED_FACE ( 'NONE', ( #82371 ), #14342, .F. ) ;
#23776=VERTEX_POINT ( 'NONE', #48120 ) ;
#23777=EDGE_CURVE ( 'NONE', #11427, #57709, #4979, .T. ) ;
#23778=CARTESIAN_POINT ( 'NONE',  ( -18.00000000000012079, -3.835265460704626150, 33.15142922262032954 ) ) ;
#23779=CARTESIAN_POINT ( 'NONE',  ( -8.546219417617921366, -3.105924265160262543, 32.13625925475356127 ) ) ;
#23780=CARTESIAN_POINT ( 'NONE',  ( -18.00000000000012079, -3.300289026999231545, 32.46337939537709616 ) ) ;
#23781=B_SPLINE_CURVE_WITH_KNOTS ( 'NONE', 3,
 ( #51588, #39458, #72768, #11080, #3863, #32247, #44395, #71884, #37655, #23691 ),
 .UNSPECIFIED., .F., .F.,
 ( 4, 2, 2, 2, 4 ),
 ( 0.0007817359430256347764, 0.0009771253907250036959, 0.001172514838424372832, 0.001367904286123741969, 0.001563293733823103949 ),
 .UNSPECIFIED. ) ;
#23782=DIRECTION ( 'NONE',  ( -0.000000000000000000, 0.6427876096865404731, -0.7660444431189771253 ) ) ;
#23783=CIRCLE ( 'NONE', #30985, 0.2500000000000002220 ) ;
#23784=EDGE_LOOP ( 'NONE', ( #64007, #29276 ) ) ;
#23785=ORIENTED_EDGE ( 'NONE', *, *, #62600, .T. ) ;
#23786=LINE ( 'NONE', #17495, #40120 ) ;
#23787=ORIENTED_EDGE ( 'NONE', *, *, #58690, .F. ) ;
#23788=CARTESIAN_POINT ( 'NONE',  ( -15.23076923076922995, -8.810774026931790459, 35.74407628777942847 ) ) ;
#23789=DIRECTION ( 'NONE',  ( 0.000000000000000000, 0.000000000000000000, 1.000000000000000000 ) ) ;
#23790=DIRECTION ( 'NONE',  ( -0.000000000000000000, 0.5000000000000011102, -0.8660254037844381525 ) ) ;
#23791=VECTOR ( 'NONE', #37776, 1000.000000000000114 ) ;
#23792=VERTEX_POINT ( 'NONE', #15239 ) ;
#23793=ORIENTED_EDGE ( 'NONE', *, *, #4537, .F. ) ;
#23794=ORIENTED_EDGE ( 'NONE', *, *, #14217, .F. ) ;
#23796=ORIENTED_EDGE ( 'NONE', *, *, #9302, .T. ) ;
#23797=CARTESIAN_POINT ( 'NONE',  ( -5.869208192175211281, -8.147973898785416225, 34.70805048591653730 ) ) ;
#23798=EDGE_CURVE ( 'NONE', #87392, #74998, #503, .T. ) ;
#23799=DIRECTION ( 'NONE',  ( 0.000000000000000000, 0.9396926207859126468, 0.3420201433256571111 ) ) ;
#23801=DIRECTION ( 'NONE',  ( 0.000000000000000000, 0.1736481776669275834, 0.9848077530122086864 ) ) ;
#23802=CARTESIAN_POINT ( 'NONE',  ( 16.15384615384603251, -4.320704448113951379, 33.92786785259630022 ) ) ;
#23803=CARTESIAN_POINT ( 'NONE',  ( -2.084912766423897779, -11.41317474335729187, 32.86274602512330034 ) ) ;
#23804=FACE_BOUND ( 'NONE', #58509, .T. ) ;
#23806=CARTESIAN_POINT ( 'NONE',  ( 4.023698184114458343, -2.373036134822904319, 30.88089517874952250 ) ) ;
#23807=CARTESIAN_POINT ( 'NONE',  ( 13.16113046005105325, -12.69144148231606017, 30.53333754910549303 ) ) ;
#23809=CARTESIAN_POINT ( 'NONE',  ( -15.93106648486808652, -3.020022701398814569, 32.48759521482552515 ) ) ;
#23810=CARTESIAN_POINT ( 'NONE',  ( -8.069080063669989755, -3.105860786376062332, 32.13614157043599562 ) ) ;
#23811=CARTESIAN_POINT ( 'NONE',  ( 5.207448778686637247, -2.619367082507848554, 30.83698974864644171 ) ) ;
#23813=CARTESIAN_POINT ( 'NONE',  ( -15.90390074446811042, -3.520799739797214389, 33.17531984108286025 ) ) ;
#23814=VERTEX_POINT ( 'NONE', #82815 ) ;
#23815=ORIENTED_EDGE ( 'NONE', *, *, #78285, .T. ) ;
#23817=CARTESIAN_POINT ( 'NONE',  ( 5.869308533332445066, -6.413092428213692742, 34.63065189839063152 ) ) ;
#23818=CARTESIAN_POINT ( 'NONE',  ( 1.607628228708781748, -5.582272713120728369, 34.63742843783360570 ) ) ;
#23819=FACE_OUTER_BOUND ( 'NONE', #49300, .T. ) ;
#23820=CARTESIAN_POINT ( 'NONE',  ( 14.55769230769232614, -2.249999999999997780, 29.81603969181030322 ) ) ;
#23821=CARTESIAN_POINT ( 'NONE',  ( 1.384615384615386802, -11.69971097300155272, 32.46337939537588113 ) ) ;
#23822=ORIENTED_EDGE ( 'NONE', *, *, #37270, .F. ) ;
#23823=CARTESIAN_POINT ( 'NONE',  ( 18.22277966897806678, -4.226511098958373402, 33.85474049983370293 ) ) ;
#23824=CARTESIAN_POINT ( 'NONE',  ( 15.00784227186238162, -10.77366814457252175, 33.85459836347579454 ) ) ;
#23825=CYLINDRICAL_SURFACE ( 'NONE', #17166, 0.2499999999999995559 ) ;
#23826=CARTESIAN_POINT ( 'NONE',  ( 10.61538461538449596, -4.481592998941358097, 33.73612834414048933 ) ) ;
#23827=CYLINDRICAL_SURFACE ( 'NONE', #39132, 0.2499999999999979738 ) ;
#23829=EDGE_LOOP ( 'NONE', ( #44069, #40168 ) ) ;
#23831=EDGE_CURVE ( 'NONE', #5084, #1104, #7989, .T. ) ;
#23832=CARTESIAN_POINT ( 'NONE',  ( 3.230769230769231726, -8.973038597847269315, 34.52809138561121927 ) ) ;
#23833=EDGE_LOOP ( 'NONE', ( #31611, #62886 ) ) ;
#23835=CARTESIAN_POINT ( 'NONE',  ( 9.942362003946010773, -9.943054286541403997, 34.11300777759954883 ) ) ;
#23836=CARTESIAN_POINT ( 'NONE',  ( 14.55763782604045353, -2.824170634883621744, 31.52227843825338738 ) ) ;
#23837=EDGE_CURVE ( 'NONE', #88055, #69004, #49935, .T. ) ;
#23838=CARTESIAN_POINT ( 'NONE',  ( 5.750000000000002665, -2.249999999999998668, 29.75000000000000355 ) ) ;
#23840=B_SPLINE_CURVE_WITH_KNOTS ( 'NONE', 3,
 ( #86307, #86758, #4312, #51138, #85847, #24581, #52046, #23686, #79539, #57922 ),
 .UNSPECIFIED., .F., .F.,
 ( 4, 2, 2, 2, 4 ),
 ( 0.0007817246256747446788, 0.0009771112852218879000, 0.001172497944769031013, 0.001367884604316174126, 0.001563271263863317238 ),
 .UNSPECIFIED. ) ;
#23841=CARTESIAN_POINT ( 'NONE',  ( 14.08476534878545827, -6.459968553980841577, 34.89616026154728701 ) ) ;
#23842=ORIENTED_EDGE ( 'NONE', *, *, #35053, .F. ) ;
#23843=CARTESIAN_POINT ( 'NONE',  ( -4.153846153845837108, -2.255955759149395501, 30.00000000000324363 ) ) ;
#23844=CARTESIAN_POINT ( 'NONE',  ( -2.084912638714240707, -12.69155399931963046, 30.53255429739157734 ) ) ;
#23845=EDGE_LOOP ( 'NONE', ( #26990, #8491, #56703, #39948 ) ) ;
#23846=CARTESIAN_POINT ( 'NONE',  ( -13.63459211555773720, -11.28823185664190376, 33.01397839955799896 ) ) ;
#23847=DIRECTION ( 'NONE',  ( -0.000000000000000000, 0.1736481776669307198, -0.9848077530122080203 ) ) ;
#23848=CARTESIAN_POINT ( 'NONE',  ( -8.769230769230768274, -1.129524287112498415, 32.06866353760679544 ) ) ;
#23849=CARTESIAN_POINT ( 'NONE',  ( 6.857806922520603976, -3.643525952247789412, 33.31231777344662959 ) ) ;
#23850=AXIS2_PLACEMENT_3D ( 'NONE', #68507, #5930, #33405 ) ;
#23851=CARTESIAN_POINT ( 'NONE',  ( 10.74591031714817824, -2.882268652242222284, 31.66798894389554064 ) ) ;
#23852=ADVANCED_FACE ( 'NONE', ( #23743 ), #51645, .F. ) ;
#23853=CARTESIAN_POINT ( 'NONE',  ( 7.622668921589515811, -3.562934362175799841, 33.22335522853832401 ) ) ;
#23854=CARTESIAN_POINT ( 'NONE',  ( -7.976845312821407852, -12.38065189839062263, 30.83690757178629482 ) ) ;
#23856=VERTEX_POINT ( 'NONE', #2583 ) ;
#23857=CARTESIAN_POINT ( 'NONE',  ( -16.28453675695646652, -9.084618155246140248, 34.75535874321725771 ) ) ;
#23858=CARTESIAN_POINT ( 'NONE',  ( 1.319344938654611221, -6.026961402152685388, 34.52809138561120506 ) ) ;
#23859=CARTESIAN_POINT ( 'NONE',  ( -17.20707104665477516, -5.070767119584671079, 34.40440758774516183 ) ) ;
#23861=EDGE_CURVE ( 'NONE', #66822, #28583, #33839, .T. ) ;
#23862=CARTESIAN_POINT ( 'NONE',  ( -13.45069879557126669, -12.37446782046654192, 30.86335684631486487 ) ) ;
#23863=CARTESIAN_POINT ( 'NONE',  ( -6.923076923076922462, -1.129524287112498415, 32.06866353760679544 ) ) ;
#23864=EDGE_LOOP ( 'NONE', ( #86431, #26150 ) ) ;
#23866=CARTESIAN_POINT ( 'NONE',  ( -1.608100328339333585, -10.11188796281391333, 34.01382737946119050 ) ) ;
#23867=EDGE_CURVE ( 'NONE', #12523, #23814, #38133, .T. ) ;
#23868=AXIS2_PLACEMENT_3D ( 'NONE', #61332, #60903, #54582 ) ;
#23869=ORIENTED_EDGE ( 'NONE', *, *, #82942, .F. ) ;
#23870=CARTESIAN_POINT ( 'NONE',  ( -4.153846153846152411, -2.486705287966279876, 31.30864560766543647 ) ) ;
#23871=ORIENTED_EDGE ( 'NONE', *, *, #42973, .F. ) ;
#23872=DIRECTION ( 'NONE',  ( -0.000000000000000000, 0.7660444431189791237, -0.6427876096865379196 ) ) ;
#23873=DIRECTION ( 'NONE',  ( 0.000000000000000000, 0.9848077530122072432, -0.1736481776669354937 ) ) ;
#23874=EDGE_CURVE ( 'NONE', #67070, #53330, #51030, .T. ) ;
#23875=CARTESIAN_POINT ( 'NONE',  ( 16.82689985270161870, -6.652501968072647820, 34.93155406624980941 ) ) ;
#23876=ORIENTED_EDGE ( 'NONE', *, *, #69545, .T. ) ;
#23877=DIRECTION ( 'NONE',  ( 0.000000000000000000, 0.6427876096865368094, 0.7660444431189802339 ) ) ;
#23880=B_SPLINE_CURVE_WITH_KNOTS ( 'NONE', 3,
 ( #25140, #71989, #86426, #10298, #32346, #30996, #59813, #24697, #80551, #72431 ),
 .UNSPECIFIED., .F., .F.,
 ( 4, 2, 2, 2, 4 ),
 ( 0.0007817359430256326080, 0.0009771253907249993591, 0.001172514838424366327, 0.001367904286123733078, 0.001563293733823099829 ),
 .UNSPECIFIED. ) ;
#23881=ORIENTED_EDGE ( 'NONE', *, *, #35660, .F. ) ;
#23883=CARTESIAN_POINT ( 'NONE',  ( 5.011653076366756387, -5.941354392334500467, 34.76329471203369792 ) ) ;
#23884=EDGE_CURVE ( 'NONE', #62713, #41734, #67191, .T. ) ;
#23885=B_SPLINE_CURVE_WITH_KNOTS ( 'NONE', 3,
 ( #41477, #28399, #76594, #43249, #55870, #48665, #47, #7250, #15339, #27518 ),
 .UNSPECIFIED., .F., .F.,
 ( 4, 2, 2, 2, 4 ),
 ( 0.0007817246256747464135, 0.0009771112852218900684, 0.001172497944769033615, 0.001367884604316177161, 0.001563271263863320925 ),
 .UNSPECIFIED. ) ;
#23886=AXIS2_PLACEMENT_3D ( 'NONE', #62851, #47581, #13797 ) ;
#23887=ORIENTED_EDGE ( 'NONE', *, *, #56400, .F. ) ;
#23888=ADVANCED_FACE ( 'NONE', ( #16117 ), #32297, .F. ) ;
#23889=CARTESIAN_POINT ( 'NONE',  ( 8.639082799499073317, -5.070767119584671079, 34.40440758774516183 ) ) ;
#23890=CARTESIAN_POINT ( 'NONE',  ( -14.55771554498526932, -10.76384336483936011, 33.53834819971076087 ) ) ;
#23891=CARTESIAN_POINT ( 'NONE',  ( -11.53846153846165912, -2.892918686052166066, 31.69288490824153470 ) ) ;
#23892=VECTOR ( 'NONE', #53806, 1000.000000000000000 ) ;
#23895=ORIENTED_EDGE ( 'NONE', *, *, #34041, .T. ) ;
#23898=CARTESIAN_POINT ( 'NONE',  ( 3.230769230769231726, -5.471508081941601098, 34.59228464037088457 ) ) ;
#23899=ORIENTED_EDGE ( 'NONE', *, *, #3589, .T. ) ;
#23901=ADVANCED_FACE ( 'NONE', ( #47125 ), #81822, .F. ) ;
#23902=CARTESIAN_POINT ( 'NONE',  ( 10.55011416942384095, -5.219633306516282545, 34.19971097300152962 ) ) ;
#23903=CARTESIAN_POINT ( 'NONE',  ( 5.076923076923075762, -10.89733346790207413, 36.13435417666054406 ) ) ;
#23904=ORIENTED_EDGE ( 'NONE', *, *, #35714, .F. ) ;
#23905=ORIENTED_EDGE ( 'NONE', *, *, #26553, .T. ) ;
#23906=VERTEX_POINT ( 'NONE', #67412 ) ;
#23907=CARTESIAN_POINT ( 'NONE',  ( 0.3954560821783248969, -8.164416787775445883, 34.95778746994557906 ) ) ;
#23908=EDGE_LOOP ( 'NONE', ( #27712, #34, #69612, #57039 ) ) ;
#23909=CARTESIAN_POINT ( 'NONE',  ( -10.39260507411620260, -9.332535724633409302, 34.40230450496446934 ) ) ;
#23911=VECTOR ( 'NONE', #56452, 999.9999999999998863 ) ;
#23912=B_SPLINE_CURVE_WITH_KNOTS ( 'NONE', 3,
 ( #45864, #87780, #11200, #65244, #85973, #78764, #17064, #44519, #3543, #31468 ),
 .UNSPECIFIED., .F., .F.,
 ( 4, 2, 2, 2, 4 ),
 ( 0.000000000000000000, 0.0001954339857564074473, 0.0003908679715128148945, 0.0005863019572692223418, 0.0007817359430256297891 ),
 .UNSPECIFIED. ) ;
#23913=CARTESIAN_POINT ( 'NONE',  ( 3.903822929624696236, -12.68155406624981119, 30.59749803192733708 ) ) ;
#23914=CARTESIAN_POINT ( 'NONE',  ( 12.39545505058257824, -2.538708090699994813, 30.37095296980875148 ) ) ;
#23915=EDGE_CURVE ( 'NONE', #35763, #33353, #5933, .T. ) ;
#23916=FACE_BOUND ( 'NONE', #85719, .T. ) ;
#23917=ORIENTED_EDGE ( 'NONE', *, *, #33446, .F. ) ;
#23918=CARTESIAN_POINT ( 'NONE',  ( 13.63466969625370240, -9.148310452688876993, 34.47095581063188519 ) ) ;
#23919=EDGE_CURVE ( 'NONE', #17034, #78771, #60614, .T. ) ;
#23920=CARTESIAN_POINT ( 'NONE',  ( 4.853438152358745761, -3.562934362175799841, 33.22335522853832401 ) ) ;
#23921=CARTESIAN_POINT ( 'NONE',  ( 8.834486340506794377, -3.300289026998473041, 32.46337939537591666 ) ) ;
#23922=CARTESIAN_POINT ( 'NONE',  ( 17.14217864819909920, -9.442884908240273489, 34.35708131394835618 ) ) ;
#23925=CARTESIAN_POINT ( 'NONE',  ( -17.32689980786543060, -12.41269422305637171, 30.68257228309993323 ) ) ;
#23926=VERTEX_POINT ( 'NONE', #26870 ) ;
#23927=ORIENTED_EDGE ( 'NONE', *, *, #13032, .T. ) ;
#23928=EDGE_CURVE ( 'NONE', #13509, #83846, #13410, .T. ) ;
#23929=CARTESIAN_POINT ( 'NONE',  ( -16.15384615384615330, -3.886160181151819604, 36.00935417666054406 ) ) ;
#23930=CARTESIAN_POINT ( 'NONE',  ( 5.869852790561781219, -3.285722584762969856, 32.44110544564090759 ) ) ;
#23932=CARTESIAN_POINT ( 'NONE',  ( -13.45069776397551564, -2.833524468853757305, 32.15551576947924417 ) ) ;
#23933=CARTESIAN_POINT ( 'NONE',  ( -18.22348492456433178, -5.827078755546625466, 34.72654668319379567 ) ) ;
#23934=CARTESIAN_POINT ( 'NONE',  ( 6.923076923076924238, -2.517432740324522911, 35.29906147534542527 ) ) ;
#23935=ORIENTED_EDGE ( 'NONE', *, *, #75572, .F. ) ;
#23936=CARTESIAN_POINT ( 'NONE',  ( 6.856994543716787405, -2.486705287966279432, 31.30864560766542937 ) ) ;
#23939=CARTESIAN_POINT ( 'NONE',  ( -13.60754234352223335, -12.64616026154729411, 30.79003144601914244 ) ) ;
#23940=EDGE_LOOP ( 'NONE', ( #63774, #14130, #2000, #68872 ) ) ;
#23941=ORIENTED_EDGE ( 'NONE', *, *, #50007, .T. ) ;
#23942=FACE_BOUND ( 'NONE', #21937, .T. ) ;
#23943=ORIENTED_EDGE ( 'NONE', *, *, #42540, .T. ) ;
#23944=CARTESIAN_POINT ( 'NONE',  ( 14.30769230769231015, -5.180354513474913603, 36.12317359536750416 ) ) ;
#23945=CARTESIAN_POINT ( 'NONE',  ( -7.623374304885435215, -5.114059244376869984, 34.14424750095245287 ) ) ;
#23947=CARTESIAN_POINT ( 'NONE',  ( 16.40384615384615330, -2.249999999999998668, 29.75000000000000355 ) ) ;
#23948=CARTESIAN_POINT ( 'NONE',  ( 17.99999999999987566, -3.643525952248796163, 33.31231777344771672 ) ) ;
#23949=CARTESIAN_POINT ( 'NONE',  ( 4.853996859406929154, -2.758268499246657957, 31.33685645148948140 ) ) ;
#23950=EDGE_CURVE ( 'NONE', #73783, #60358, #87704, .T. ) ;
#23951=CARTESIAN_POINT ( 'NONE',  ( -17.07692307692307665, -3.322132147404559976, 32.92929555188717927 ) ) ;
#23953=VECTOR ( 'NONE', #23559, 1000.000000000000000 ) ;
#23954=ADVANCED_FACE ( 'NONE', ( #81381 ), #18785, .F. ) ;
#23955=CARTESIAN_POINT ( 'NONE',  ( -4.023320452082589149, -6.852161475712352789, 34.70806712695775786 ) ) ;
#23956=VERTEX_POINT ( 'NONE', #46692 ) ;
#23957=B_SPLINE_CURVE_WITH_KNOTS ( 'NONE', 3,
 ( #53041, #74222, #31905, #10739, #73787, #53940, #80545, #12086, #45398, #4418 ),
 .UNSPECIFIED., .F., .F.,
 ( 4, 2, 2, 2, 4 ),
 ( 0.000000000000000000, 0.0001954339857564080707, 0.0003908679715128161414, 0.0005863019572692241849, 0.0007817359430256322827 ),
 .UNSPECIFIED. ) ;
#23958=CARTESIAN_POINT ( 'NONE',  ( 13.44987095589141468, -12.27809138561124591, 31.22303859784720359 ) ) ;
#23959=ORIENTED_EDGE ( 'NONE', *, *, #71750, .T. ) ;
#23960=CARTESIAN_POINT ( 'NONE',  ( 15.36129493253279499, -8.586989748646452369, 34.63063291749215011 ) ) ;
#23961=LINE ( 'NONE', #31164, #28133 ) ;
#23962=DIRECTION ( 'NONE',  ( -0.000000000000000000, -0.9396926207859092051, -0.3420201433256662704 ) ) ;
#23963=CARTESIAN_POINT ( 'NONE',  ( 15.23076923076923173, -12.37446782046654192, 30.86335684631486131 ) ) ;
#23964=CARTESIAN_POINT ( 'NONE',  ( -14.53061926659915315, -8.282780595021769443, 34.94152052738834158 ) ) ;
#23965=AXIS2_PLACEMENT_3D ( 'NONE', #77260, #36720, #43479 ) ;
#23966=CARTESIAN_POINT ( 'NONE',  ( -9.758390071667825794, -11.91647553114624181, 32.58852847137148245 ) ) ;
#23968=VERTEX_POINT ( 'NONE', #45800 ) ;
#23969=DIRECTION ( 'NONE',  ( -0.000000000000000000, -0.1736481776669307198, -0.9848077530122080203 ) ) ;
#23971=DIRECTION ( 'NONE',  ( 0.000000000000000000, 0.9396926207859126468, 0.3420201433256571111 ) ) ;
#23972=ORIENTED_EDGE ( 'NONE', *, *, #60809, .F. ) ;
#23973=ORIENTED_EDGE ( 'NONE', *, *, #66703, .F. ) ;
#23974=CYLINDRICAL_SURFACE ( 'NONE', #29725, 0.2500000000000009437 ) ;
#23975=CARTESIAN_POINT ( 'NONE',  ( 12.68431813051652313, -4.226511098958373402, 33.85474049983370293 ) ) ;
#23976=DIRECTION ( 'NONE',  ( -0.000000000000000000, 0.6427876096865404731, -0.7660444431189771253 ) ) ;
#23977=CARTESIAN_POINT ( 'NONE',  ( 9.627037246346917598, -12.46129190929999986, 30.37095296980880832 ) ) ;
#23978=CARTESIAN_POINT ( 'NONE',  ( 13.13463864056679498, -2.920706130388546651, 32.31842814019191223 ) ) ;
#23979=CARTESIAN_POINT ( 'NONE',  ( -8.769230769230768274, -11.69971097300155272, 32.46337939537588113 ) ) ;
#23980=CARTESIAN_POINT ( 'NONE',  ( -7.053224132515143907, -11.93770438780619259, 32.05411857736982029 ) ) ;
#23981=VERTEX_POINT ( 'NONE', #87257 ) ;
#23982=AXIS2_PLACEMENT_3D ( 'NONE', #21681, #78388, #16691 ) ;
#23983=CARTESIAN_POINT ( 'NONE',  ( 5.999999999999880096, -10.90142922262034020, 33.41473453929536674 ) ) ;
#23984=CARTESIAN_POINT ( 'NONE',  ( -17.14224708972738753, -7.749976730030849303, 34.74374725381503737 ) ) ;
#23985=EDGE_CURVE ( 'NONE', #67360, #30707, #20908, .T. ) ;
#23986=EDGE_CURVE ( 'NONE', #34679, #10626, #40830, .T. ) ;
#23987=DIRECTION ( 'NONE',  ( -0.000000000000000000, 0.8660254037844397068, -0.4999999999999978906 ) ) ;
#23988=CARTESIAN_POINT ( 'NONE',  ( -4.153846153846274980, -4.320704448113951379, 33.92786785259630022 ) ) ;
#23989=ORIENTED_EDGE ( 'NONE', *, *, #85408, .T. ) ;
#23991=VECTOR ( 'NONE', #5303, 1000.000000000000227 ) ;
#23992=EDGE_CURVE ( 'NONE', #19611, #15474, #14528, .T. ) ;
#23993=ORIENTED_EDGE ( 'NONE', *, *, #58698, .F. ) ;
#23994=CARTESIAN_POINT ( 'NONE',  ( 15.16549878480845592, -11.48612834413959582, 32.76840700105983473 ) ) ;
#23997=FACE_OUTER_BOUND ( 'NONE', #55774, .T. ) ;
#23998=ORIENTED_EDGE ( 'NONE', *, *, #194, .F. ) ;
#24000=AXIS2_PLACEMENT_3D ( 'NONE', #33328, #55355, #40535 ) ;
#24001=CARTESIAN_POINT ( 'NONE',  ( 12.52760579488853665, -10.67929555188718282, 33.92786785259544757 ) ) ;
#24003=CARTESIAN_POINT ( 'NONE',  ( -10.61538461538473399, -6.879047030192662504, 34.71129190930017927 ) ) ;
#24004=ADVANCED_FACE ( 'NONE', ( #41715 ), #49792, .F. ) ;
#24005=CARTESIAN_POINT ( 'NONE',  ( 8.992657731092338125, -7.630147231320743018, 34.74852402298682819 ) ) ;
#24006=CARTESIAN_POINT ( 'NONE',  ( -4.826977667545032880, -10.92531984108285670, 33.72920026020278073 ) ) ;
#24008=CARTESIAN_POINT ( 'NONE',  ( 16.28463659481310444, -9.929761469519743144, 34.40412654351204225 ) ) ;
#24009=ORIENTED_EDGE ( 'NONE', *, *, #52535, .T. ) ;
#24010=EDGE_CURVE ( 'NONE', #50376, #82473, #35906, .T. ) ;
#24011=CARTESIAN_POINT ( 'NONE',  ( -17.07692307692307665, -13.87047571288749737, 32.06866353760679544 ) ) ;
#24014=ADVANCED_FACE ( 'NONE', ( #28647 ), #56112, .F. ) ;
#24015=CARTESIAN_POINT ( 'NONE',  ( -12.46153846153846168, -12.34228464037088635, 31.77849191805839268 ) ) ;
#24016=CARTESIAN_POINT ( 'NONE',  ( -6.923076923076922462, -2.486705287966279876, 31.30864560766543647 ) ) ;
#24017=VECTOR ( 'NONE', #66739, 1000.000000000000000 ) ;
#24018=ORIENTED_EDGE ( 'NONE', *, *, #18373, .F. ) ;
#24019=VERTEX_POINT ( 'NONE', #75490 ) ;
#24020=ORIENTED_EDGE ( 'NONE', *, *, #79781, .F. ) ;
#24021=ORIENTED_EDGE ( 'NONE', *, *, #28518, .F. ) ;
#24022=ORIENTED_EDGE ( 'NONE', *, *, #6096, .F. ) ;
#24023=CIRCLE ( 'NONE', #52775, 2.999999999999999112 ) ;
#24024=DIRECTION ( 'NONE',  ( -0.000000000000000000, -0.7660444431189791237, -0.6427876096865379196 ) ) ;
#24025=CARTESIAN_POINT ( 'NONE',  ( -1.134561072977069651, -12.41262288849542017, 30.68299917996395010 ) ) ;
#24026=CARTESIAN_POINT ( 'NONE',  ( -7.173076923076921574, -2.499999999999998668, 29.75000000000000355 ) ) ;
#24027=EDGE_CURVE ( 'NONE', #18998, #52344, #13033, .T. ) ;
#24029=CARTESIAN_POINT ( 'NONE',  ( -16.40386939113911779, -2.587272538249754117, 30.68239716806877837 ) ) ;
#24031=EDGE_CURVE ( 'NONE', #50988, #56881, #87621, .T. ) ;
#24033=CARTESIAN_POINT ( 'NONE',  ( -5.076923076922761346, -2.255955759149395501, 30.00000000000324363 ) ) ;
#24034=ORIENTED_EDGE ( 'NONE', *, *, #46945, .T. ) ;
#24035=VERTEX_POINT ( 'NONE', #70068 ) ;
#24036=ORIENTED_EDGE ( 'NONE', *, *, #37918, .F. ) ;
#24037=CARTESIAN_POINT ( 'NONE',  ( 6.250054419913455561, -12.41089969410671223, 31.60739465890703670 ) ) ;
#24040=LINE ( 'NONE', #36682, #50290 ) ;
#24041=CARTESIAN_POINT ( 'NONE',  ( 10.36540788444226280, -9.148715823498378086, 34.47080413974185120 ) ) ;
#24042=CARTESIAN_POINT ( 'NONE',  ( 1.384615384615386802, -12.29105614889573062, 35.45975837776705220 ) ) ;
#24043=VECTOR ( 'NONE', #55850, 1000.000000000000114 ) ;
#24044=CARTESIAN_POINT ( 'NONE',  ( -14.37296275365308418, -10.21337939537584383, 33.94971097300158647 ) ) ;
#24045=ORIENTED_EDGE ( 'NONE', *, *, #25623, .T. ) ;
#24046=EDGE_CURVE ( 'NONE', #87173, #38328, #34952, .T. ) ;
#24047=EDGE_LOOP ( 'NONE', ( #44716, #85606, #35451, #64072 ) ) ;
#24049=B_SPLINE_CURVE_WITH_KNOTS ( 'NONE', 3,
 ( #13386, #82302, #28682, #20582, #7522, #1194, #34545, #75527, #35881, #54367 ),
 .UNSPECIFIED., .F., .F.,
 ( 4, 2, 2, 2, 4 ),
 ( 0.0007817359430256333669, 0.0009771253907250056474, 0.001172514838424370881, 0.001367904286123736331, 0.001563293733823101564 ),
 .UNSPECIFIED. ) ;
#24050=VERTEX_POINT ( 'NONE', #13351 ) ;
#24051=FACE_BOUND ( 'NONE', #63355, .T. ) ;
#24052=B_SPLINE_CURVE_WITH_KNOTS ( 'NONE', 3,
 ( #19572, #11942, #66879, #5617, #61435, #38974, #87610, #60556, #24994, #79947 ),
 .UNSPECIFIED., .F., .F.,
 ( 4, 2, 2, 2, 4 ),
 ( 0.0007817246256747490156, 0.0009771112852218922368, 0.001172497944769035350, 0.001367884604316178462, 0.001563271263863321575 ),
 .UNSPECIFIED. ) ;
#24053=CARTESIAN_POINT ( 'NONE',  ( 13.51540582558233794, -12.35292014791297710, 31.75344720912887198 ) ) ;
#24054=CARTESIAN_POINT ( 'NONE',  ( 7.846153846153725020, -3.835265460704628371, 33.15142922262033665 ) ) ;
#24055=VERTEX_POINT ( 'NONE', #61527 ) ;
#24056=CARTESIAN_POINT ( 'NONE',  ( -1.384615384615383471, -5.471508081941601098, 34.59228464037088457 ) ) ;
#24057=CARTESIAN_POINT ( 'NONE',  ( 8.900069099717528687, -7.277220318596961057, 34.99547417642776992 ) ) ;
#24059=CYLINDRICAL_SURFACE ( 'NONE', #56544, 0.2499999999999979738 ) ;
#24060=VERTEX_POINT ( 'NONE', #89035 ) ;
#24061=CARTESIAN_POINT ( 'NONE',  ( 12.39626801557768587, -5.219633306516282545, 34.19971097300152962 ) ) ;
#24062=CARTESIAN_POINT ( 'NONE',  ( 2.980745993476265010, -12.22074536777954989, 31.39888409691088356 ) ) ;
#24063=EDGE_CURVE ( 'NONE', #81272, #48918, #45631, .T. ) ;
#24064=ORIENTED_EDGE ( 'NONE', *, *, #50890, .T. ) ;
#24065=EDGE_CURVE ( 'NONE', #36243, #79961, #66190, .T. ) ;
#24066=CARTESIAN_POINT ( 'NONE',  ( 6.130838330486762189, -7.277220318596959281, 34.99547417642776992 ) ) ;
#24067=CARTESIAN_POINT ( 'NONE',  ( -9.561517251340744039, -9.084667340241226796, 34.75534355489798344 ) ) ;
#24068=ORIENTED_EDGE ( 'NONE', *, *, #26034, .F. ) ;
#24069=CARTESIAN_POINT ( 'NONE',  ( 2.307692307692186251, -3.083524468854526912, 32.58852847137268327 ) ) ;
#24070=CARTESIAN_POINT ( 'NONE',  ( 14.30769230769218758, -8.613356846316285953, 34.62446782046622218 ) ) ;
#24071=FACE_OUTER_BOUND ( 'NONE', #470, .T. ) ;
#24072=CARTESIAN_POINT ( 'NONE',  ( -10.61538461538473399, -6.026961402154118019, 34.52809138561165270 ) ) ;
#24073=CARTESIAN_POINT ( 'NONE',  ( -14.30769230769230660, -5.415277668671390821, 36.20867863119892149 ) ) ;
#24075=FACE_BOUND ( 'NONE', #34595, .T. ) ;
#24076=CARTESIAN_POINT ( 'NONE',  ( -1.607541602131530967, -2.758268499246656624, 31.33685645148948140 ) ) ;
#24077=DIRECTION ( 'NONE',  ( -0.000000000000000000, -0.9396926207859092051, -0.3420201433256662704 ) ) ;
#24078=CARTESIAN_POINT ( 'NONE',  ( -1.254089946381738985, -9.503571793651733657, 34.60286762892837942 ) ) ;
#24079=LINE ( 'NONE', #52438, #18509 ) ;
#24080=CARTESIAN_POINT ( 'NONE',  ( 8.900022577055551665, -2.729792928343269587, 31.24908615093345077 ) ) ;
#24082=VERTEX_POINT ( 'NONE', #22759 ) ;
#24083=CARTESIAN_POINT ( 'NONE',  ( 18.00000000000000000, -11.69971097300155272, 32.46337939537588113 ) ) ;
#24084=ORIENTED_EDGE ( 'NONE', *, *, #51580, .F. ) ;
#24088=EDGE_LOOP ( 'NONE', ( #79534, #62236, #84433, #46405 ) ) ;
#24089=CARTESIAN_POINT ( 'NONE',  ( -9.692307692307691624, -8.973038597847269315, 34.52809138561121927 ) ) ;
#24091=DIRECTION ( 'NONE',  ( -0.000000000000000000, -0.8660254037844399289, -0.4999999999999980016 ) ) ;
#24092=CARTESIAN_POINT ( 'NONE',  ( 9.915087233576100445, -11.41317474335729543, 32.86274602512330034 ) ) ;
#24093=CARTESIAN_POINT ( 'NONE',  ( -12.46153846153858424, -2.657715359629662544, 31.77849191805970364 ) ) ;
#24094=CARTESIAN_POINT ( 'NONE',  ( 4.153846153846154188, -8.164416787775445883, 34.95778746994557906 ) ) ;
#24095=CARTESIAN_POINT ( 'NONE',  ( -17.74984401280907775, -2.249999999999999556, 29.68153322838372787 ) ) ;
#24096=DIRECTION ( 'NONE',  ( -0.000000000000000000, 0.3420201433256694346, -0.9396926207859080948 ) ) ;
#24097=CARTESIAN_POINT ( 'NONE',  ( -4.403846153846151523, -7.500000000000001776, 35.04278698407183867 ) ) ;
#24099=CARTESIAN_POINT ( 'NONE',  ( 10.61538461538461675, -4.102666532097928531, 36.13435417666054406 ) ) ;
#24100=CARTESIAN_POINT ( 'NONE',  ( 13.13463864056679498, -3.436278759898153901, 33.07459398097509506 ) ) ;
#24101=AXIS2_PLACEMENT_3D ( 'NONE', #9585, #43381, #3268 ) ;
#24102=CARTESIAN_POINT ( 'NONE',  ( 13.60762673622823726, -4.187068189119697692, 33.49521262558774026 ) ) ;
#24103=B_SPLINE_CURVE_WITH_KNOTS ( 'NONE', 3,
 ( #30577, #57171, #50400, #77882, #51262, #16186, #85534, #9866, #37330, #37782 ),
 .UNSPECIFIED., .F., .F.,
 ( 4, 2, 2, 2, 4 ),
 ( 0.000000000000000000, 0.0001954339857564097512, 0.0003908679715128195024, 0.0005863019572692292807, 0.0007817359430256390048 ),
 .UNSPECIFIED. ) ;
#24104=VERTEX_POINT ( 'NONE', #64625 ) ;
#24105=CARTESIAN_POINT ( 'NONE',  ( -13.51476335434707821, -6.809168938359901446, 34.95455904226513866 ) ) ;
#24106=LINE ( 'NONE', #5181, #87772 ) ;
#24107=CARTESIAN_POINT ( 'NONE',  ( 1.384615384615264011, -11.06231777344772027, 33.60647404775119895 ) ) ;
#24108=CARTESIAN_POINT ( 'NONE',  ( 1.607991325313570252, -2.501478030877322567, 29.88021232661720816 ) ) ;
#24109=CARTESIAN_POINT ( 'NONE',  ( -0.4615384615384611200, -6.435427911321262684, 35.78748833219616898 ) ) ;
#24110=CARTESIAN_POINT ( 'NONE',  ( -2.980823821391187955, -5.766571408460171355, 34.70601412856602508 ) ) ;
#24111=EDGE_CURVE ( 'NONE', #67703, #53125, #4803, .T. ) ;
#24112=ORIENTED_EDGE ( 'NONE', *, *, #27955, .T. ) ;
#24113=FACE_OUTER_BOUND ( 'NONE', #26759, .T. ) ;
#24114=VERTEX_POINT ( 'NONE', #24093 ) ;
#24115=EDGE_CURVE ( 'NONE', #48201, #62266, #25225, .T. ) ;
#24116=EDGE_LOOP ( 'NONE', ( #27136, #75054, #77113, #31889 ) ) ;
#24117=CARTESIAN_POINT ( 'NONE',  ( 0.4615384615384611200, -12.34228464037088635, 31.77849191805839268 ) ) ;
#24118=CARTESIAN_POINT ( 'NONE',  ( 3.480823542407545101, -5.728107161865378494, 34.42597550085002922 ) ) ;
#24119=CARTESIAN_POINT ( 'NONE',  ( 9.692307692307572609, -12.27809138561165270, 31.22303859784587132 ) ) ;
#24120=VECTOR ( 'NONE', #39977, 1000.000000000000000 ) ;
#24121=CARTESIAN_POINT ( 'NONE',  ( 4.376625695114563896, -3.755027918224367767, 33.06320215134714857 ) ) ;
#24122=CARTESIAN_POINT ( 'NONE',  ( -5.142193077479396024, -8.656820664281497102, 34.87096338111211935 ) ) ;
#24123=EDGE_LOOP ( 'NONE', ( #43820, #16030 ) ) ;
#24124=EDGE_CURVE ( 'NONE', #68446, #42909, #28410, .T. ) ;
#24125=B_SPLINE_CURVE_WITH_KNOTS ( 'NONE', 3,
 ( #43420, #70893, #28123, #9200, #55593, #36660, #83082, #48835, #69556, #7861 ),
 .UNSPECIFIED., .F., .F.,
 ( 4, 2, 2, 2, 4 ),
 ( 0.000000000000000000, 0.0001954311584214071026, 0.0003908623168428142051, 0.0005862934752642213077, 0.0007817246336856284103 ),
 .UNSPECIFIED. ) ;
#24126=VERTEX_POINT ( 'NONE', #70516 ) ;
#24127=B_SPLINE_CURVE_WITH_KNOTS ( 'NONE', 3,
 ( #54714, #75007, #34889, #47959, #75882, #666, #81763, #74557, #6545, #88978 ),
 .UNSPECIFIED., .F., .F.,
 ( 4, 2, 2, 2, 4 ),
 ( 0.000000000000000000, 0.0001954311584214072381, 0.0003908623168428144762, 0.0005862934752642217414, 0.0007817246336856289524 ),
 .UNSPECIFIED. ) ;
#24128=ORIENTED_EDGE ( 'NONE', *, *, #78502, .T. ) ;
#24129=CARTESIAN_POINT ( 'NONE',  ( 1.161689167099239084, -11.24512374952581872, 33.06303171183252942 ) ) ;
#24130=CARTESIAN_POINT ( 'NONE',  ( 8.703960323269994248, -2.892918686051582533, 31.69288490824015980 ) ) ;
#24132=CARTESIAN_POINT ( 'NONE',  ( 8.992010438208831502, -5.827830569534417471, 34.72679350104403539 ) ) ;
#24135=CARTESIAN_POINT ( 'NONE',  ( 11.47319153790521717, -11.06231777344662781, 33.60647404775220082 ) ) ;
#24137=CYLINDRICAL_SURFACE ( 'NONE', #36546, 0.2499999999999979738 ) ;
#24138=ORIENTED_EDGE ( 'NONE', *, *, #69009, .T. ) ;
#24139=ORIENTED_EDGE ( 'NONE', *, *, #1840, .F. ) ;
#24141=VERTEX_POINT ( 'NONE', #44350 ) ;
#24143=DIRECTION ( 'NONE',  ( 0.000000000000000000, 0.8660254037844377084, 0.5000000000000015543 ) ) ;
#24144=ORIENTED_EDGE ( 'NONE', *, *, #10896, .T. ) ;
#24145=CARTESIAN_POINT ( 'NONE',  ( -9.758390071667825794, -9.905515769479276145, 34.41647553114623292 ) ) ;
#24146=CARTESIAN_POINT ( 'NONE',  ( -9.822454901745912181, -11.93770438780619259, 32.05411857736982029 ) ) ;
#24148=EDGE_LOOP ( 'NONE', ( #8625, #16041 ) ) ;
#24150=CIRCLE ( 'NONE', #6943, 0.2500000000000002220 ) ;
#24151=CARTESIAN_POINT ( 'NONE',  ( -14.43784027742400866, -12.50552854090298993, 31.33409797877408920 ) ) ;
#24152=ORIENTED_EDGE ( 'NONE', *, *, #64333, .T. ) ;
#24153=CARTESIAN_POINT ( 'NONE',  ( -13.51530598772569292, -11.37499894934982692, 33.29245874905763003 ) ) ;
#24154=CARTESIAN_POINT ( 'NONE',  ( 10.61538461538449596, -9.442884908241554243, 34.35708131394783038 ) ) ;
#24155=CARTESIAN_POINT ( 'NONE',  ( -14.98082382139119062, -2.986452184633680229, 32.43230066228895225 ) ) ;
#24156=CARTESIAN_POINT ( 'NONE',  ( 5.777073041093150785, -12.38737895849757820, 31.66785238281580206 ) ) ;
#24157=DIRECTION ( 'NONE',  ( -0.000000000000000000, 0.5000000000000011102, -0.8660254037844381525 ) ) ;
#24158=CARTESIAN_POINT ( 'NONE',  ( -0.6844654204453104462, -12.38737895849757820, 31.66785238281580206 ) ) ;
#24159=CARTESIAN_POINT ( 'NONE',  ( -3.296851610129365451, -8.164416787775445883, 34.95778746994557906 ) ) ;
#24160=EDGE_LOOP ( 'NONE', ( #5645, #61221 ) ) ;
#24161=CARTESIAN_POINT ( 'NONE',  ( -11.31568199719312773, -12.24180327182772388, 31.33663988360758168 ) ) ;
#24162=CARTESIAN_POINT ( 'NONE',  ( 11.47321160668745677, -2.255955759149247619, 30.00000000000013856 ) ) ;
#24163=EDGE_CURVE ( 'NONE', #1486, #86632, #42452, .T. ) ;
#24164=ORIENTED_EDGE ( 'NONE', *, *, #79750, .T. ) ;
#24165=CARTESIAN_POINT ( 'NONE',  ( 11.28848479441295005, -12.01397095200674059, 32.43157075238190146 ) ) ;
#24166=CARTESIAN_POINT ( 'NONE',  ( -5.076923076923075762, -5.557115091759785130, 34.35708131394839171 ) ) ;
#24168=CARTESIAN_POINT ( 'NONE',  ( -16.15384615384615330, -11.91647553114624181, 32.58852847137148245 ) ) ;
#24169=ADVANCED_FACE ( 'NONE', ( #12371 ), #38965, .F. ) ;
#24170=CARTESIAN_POINT ( 'NONE',  ( 7.846153846153846700, -8.120952969808772792, 34.71129190930000163 ) ) ;
#24171=ADVANCED_FACE ( 'NONE', ( #31757 ), #40294, .F. ) ;
#24172=FACE_BOUND ( 'NONE', #19085, .T. ) ;
#24173=CARTESIAN_POINT ( 'NONE',  ( 5.142178216435913107, -5.941354392334606160, 34.76329471203374055 ) ) ;
#24174=CYLINDRICAL_SURFACE ( 'NONE', #35919, 0.2500000000000002220 ) ;
#24175=CARTESIAN_POINT ( 'NONE',  ( 0.4615384615384611200, -13.53365097954675988, 30.81389545987213552 ) ) ;
#24176=CARTESIAN_POINT ( 'NONE',  ( -18.00000000000000000, -11.16473453929635440, 33.15142922261927083 ) ) ;
#24177=CARTESIAN_POINT ( 'NONE',  ( 0.5267936010512991318, -3.083524468853784839, 32.58852847137153930 ) ) ;
#24178=CARTESIAN_POINT ( 'NONE',  ( 1.634560793993429906, -2.986452184633681117, 32.43230066228895225 ) ) ;
#24182=EDGE_CURVE ( 'NONE', #61727, #80092, #81075, .T. ) ;
#24183=VERTEX_POINT ( 'NONE', #46598 ) ;
#24184=LINE ( 'NONE', #57530, #13306 ) ;
#24185=AXIS2_PLACEMENT_3D ( 'NONE', #11168, #65215, #3512 ) ;
#24186=DIRECTION ( 'NONE',  ( 0.000000000000000000, 0.6427876096865368094, 0.7660444431189802339 ) ) ;
#24187=CARTESIAN_POINT ( 'NONE',  ( -0.4615384615384611200, -3.322132147404559976, 32.92929555188717927 ) ) ;
#24188=DIRECTION ( 'NONE',  ( -0.000000000000000000, -0.000000000000000000, 1.000000000000000000 ) ) ;
#24189=CARTESIAN_POINT ( 'NONE',  ( 10.86543892702293235, -12.17597550085003810, 31.52189283813460463 ) ) ;
#24192=CARTESIAN_POINT ( 'NONE',  ( -8.769230769230890843, -2.892918686052166066, 31.69288490824153470 ) ) ;
#24193=CARTESIAN_POINT ( 'NONE',  ( 0.7114839798866033904, -3.712312575010499938, 33.01462480002815170 ) ) ;
#24194=CARTESIAN_POINT ( 'NONE',  ( -7.780898706641007578, -10.33852847137154107, 34.16647553114620450 ) ) ;
#24195=CARTESIAN_POINT ( 'NONE',  ( -0.7115152055870529457, -8.347322224742351082, 34.93158281831414769 ) ) ;
#24196=CARTESIAN_POINT ( 'NONE',  ( -10.61538461538461320, -12.10708131394839349, 31.69288490824020244 ) ) ;
#24198=CARTESIAN_POINT ( 'NONE',  ( -18.13014720943821700, -2.882441371585227508, 31.66841991370171527 ) ) ;
#24199=CARTESIAN_POINT ( 'NONE',  ( 13.38461538461538680, -13.57706302396349152, 30.56769352161908060 ) ) ;
#24200=ORIENTED_EDGE ( 'NONE', *, *, #10745, .F. ) ;
#24201=DIRECTION ( 'NONE',  ( -0.000000000000000000, -0.6427876096865404731, -0.7660444431189771253 ) ) ;
#24204=CARTESIAN_POINT ( 'NONE',  ( 2.307692307692187583, -4.481592998941358097, 33.73612834414048933 ) ) ;
#24205=VECTOR ( 'NONE', #9570, 1000.000000000000227 ) ;
#24206=CARTESIAN_POINT ( 'NONE',  ( 3.480714749117374218, -11.86320923018887719, 32.19269448109604781 ) ) ;
#24207=ORIENTED_EDGE ( 'NONE', *, *, #51909, .F. ) ;
#24208=CARTESIAN_POINT ( 'NONE',  ( 12.46153846153846168, -6.343179335718451384, 34.87096338111211935 ) ) ;
#24209=CARTESIAN_POINT ( 'NONE',  ( 1.161130440891438464, -9.331801661448606566, 34.40259984581193464 ) ) ;
#24211=ORIENTED_EDGE ( 'NONE', *, *, #54862, .F. ) ;
#24212=DIRECTION ( 'NONE',  ( -0.000000000000000000, -0.6427876096865404731, -0.7660444431189771253 ) ) ;
#24213=FACE_OUTER_BOUND ( 'NONE', #65475, .T. ) ;
#24214=CARTESIAN_POINT ( 'NONE',  ( 6.000000000000001776, -12.78798330534102945, 29.74999999999997868 ) ) ;
#24215=CARTESIAN_POINT ( 'NONE',  ( 8.769230769230647482, -5.219633306517616589, 34.19971097300220464 ) ) ;
#24216=ORIENTED_EDGE ( 'NONE', *, *, #78684, .T. ) ;
#24218=DIRECTION ( 'NONE',  ( 0.000000000000000000, 0.9848077530122072432, 0.1736481776669354937 ) ) ;
#24220=VECTOR ( 'NONE', #29825, 1000.000000000000000 ) ;
#24221=CARTESIAN_POINT ( 'NONE',  ( 3.930361210122205406, -10.11188796281391511, 34.01382737946119050 ) ) ;
#24222=EDGE_LOOP ( 'NONE', ( #30470, #63427, #24862, #57055 ) ) ;
#24224=ORIENTED_EDGE ( 'NONE', *, *, #70292, .F. ) ;
#24225=CARTESIAN_POINT ( 'NONE',  ( -9.942330929600657896, -10.05641848906368097, 34.04755513067966177 ) ) ;
#24226=CARTESIAN_POINT ( 'NONE',  ( -2.980823821391187511, -2.986452184633681117, 32.43230066228895225 ) ) ;
#24227=CARTESIAN_POINT ( 'NONE',  ( -9.561782254074051579, -12.70449254468099198, 30.44128974285582956 ) ) ;
#24228=CYLINDRICAL_SURFACE ( 'NONE', #17600, 0.2499999999999986955 ) ;
#24229=ORIENTED_EDGE ( 'NONE', *, *, #58218, .T. ) ;
#24230=EDGE_LOOP ( 'NONE', ( #21598, #21065 ) ) ;
#24231=CARTESIAN_POINT ( 'NONE',  ( 15.23076923076923173, -6.189225973068211317, 35.74407628777942847 ) ) ;
#24234=CARTESIAN_POINT ( 'NONE',  ( 16.15384615384603251, -8.656820664282941280, 34.87096338111179961 ) ) ;
#24235=EDGE_CURVE ( 'NONE', #51727, #87990, #58548, .T. ) ;
#24236=CARTESIAN_POINT ( 'NONE',  ( 5.869309396889692110, -3.957541250942359756, 33.62499894934981626 ) ) ;
#24237=DIRECTION ( 'NONE',  ( 0.000000000000000000, 0.8660254037844377084, 0.5000000000000015543 ) ) ;
#24238=ORIENTED_EDGE ( 'NONE', *, *, #12922, .T. ) ;
#24240=ORIENTED_EDGE ( 'NONE', *, *, #71896, .F. ) ;
#24241=CARTESIAN_POINT ( 'NONE',  ( 15.00728428704528561, -2.599994579823202923, 30.74605699353653776 ) ) ;
#24242=ORIENTED_EDGE ( 'NONE', *, *, #76813, .F. ) ;
#24243=DIRECTION ( 'NONE',  ( -0.000000000000000000, -0.3420201433256694901, -0.9396926207859082059 ) ) ;
#24244=DIRECTION ( 'NONE',  ( -0.000000000000000000, 0.7660444431189791237, -0.6427876096865379196 ) ) ;
#24245=EDGE_LOOP ( 'NONE', ( #66485, #84961 ) ) ;
#24246=EDGE_CURVE ( 'NONE', #47112, #60879, #66870, .T. ) ;
#24247=CARTESIAN_POINT ( 'NONE',  ( -13.38461538461550582, -4.481592998941358097, 33.73612834414048933 ) ) ;
#24248=CYLINDRICAL_SURFACE ( 'NONE', #9179, 0.2500000000000012212 ) ;
#24249=CARTESIAN_POINT ( 'NONE',  ( -2.307692307692305711, -11.16473453929635440, 33.15142922261926373 ) ) ;
#24250=FACE_BOUND ( 'NONE', #71481, .T. ) ;
#24252=CARTESIAN_POINT ( 'NONE',  ( -4.219929564802032296, -12.10708131394839349, 31.69288490824020244 ) ) ;
#24253=B_SPLINE_CURVE_WITH_KNOTS ( 'NONE', 3,
 ( #65183, #22867, #3033, #85466, #23748, #71945 ),
 .UNSPECIFIED., .F., .F.,
 ( 4, 2, 4 ),
 ( 0.0003909569690057805385, 0.0005862646681846044039, 0.0007815723673634283235 ),
 .UNSPECIFIED. ) ;
#24254=CARTESIAN_POINT ( 'NONE',  ( 14.30769230769231015, -7.500000000000001776, 35.04278698407183867 ) ) ;
#24255=CARTESIAN_POINT ( 'NONE',  ( -7.846153846153965716, -3.300289026999228881, 32.46337939537708905 ) ) ;
#24256=CARTESIAN_POINT ( 'NONE',  ( 4.284636594813102661, -2.295524264805589354, 30.44142389570982488 ) ) ;
#24257=AXIS2_PLACEMENT_3D ( 'NONE', #55439, #9907, #37369 ) ;
#24258=CARTESIAN_POINT ( 'NONE',  ( 8.703148389870632329, -9.058645607665454236, 34.76329471203372634 ) ) ;
#24259=DIRECTION ( 'NONE',  ( 0.000000000000000000, 0.000000000000000000, 1.000000000000000000 ) ) ;
#24260=ORIENTED_EDGE ( 'NONE', *, *, #88539, .F. ) ;
#24261=CARTESIAN_POINT ( 'NONE',  ( 14.08481362526366354, -7.630691491037285168, 34.74850469731152458 ) ) ;
#24262=FACE_OUTER_BOUND ( 'NONE', #85397, .T. ) ;
#24263=ORIENTED_EDGE ( 'NONE', *, *, #60300, .F. ) ;
#24264=ORIENTED_EDGE ( 'NONE', *, *, #5866, .F. ) ;
#24265=VECTOR ( 'NONE', #14175, 1000.000000000000114 ) ;
#24266=CARTESIAN_POINT ( 'NONE',  ( -6.792551221313360088, -8.586989748646452369, 34.63063291749215011 ) ) ;
#24267=CARTESIAN_POINT ( 'NONE',  ( -5.777220458731588515, -12.24180327182771855, 31.33663988360758168 ) ) ;
#24269=CARTESIAN_POINT ( 'NONE',  ( -6.923076923076922462, -6.386643153685126251, 34.62446782046654192 ) ) ;
#24270=CARTESIAN_POINT ( 'NONE',  ( 2.557746727605760384, -2.318338780012835443, 30.59689888758630261 ) ) ;
#24271=DIRECTION ( 'NONE',  ( -0.000000000000000000, 0.9396926207859092051, -0.3420201433256662704 ) ) ;
#24273=EDGE_CURVE ( 'NONE', #56000, #17031, #77852, .T. ) ;
#24275=CYLINDRICAL_SURFACE ( 'NONE', #54474, 0.2500000000000002220 ) ;
#24276=CARTESIAN_POINT ( 'NONE',  ( 15.16468685140909578, -10.67929555188718460, 33.92786785259543336 ) ) ;
#24277=CARTESIAN_POINT ( 'NONE',  ( 7.715462379486287325, -5.582088688514999397, 34.36776431015576350 ) ) ;
#24278=DIRECTION ( 'NONE',  ( -0.000000000000000000, 0.5000000000000011102, -0.8660254037844380415 ) ) ;
#24279=SURFACE_SIDE_STYLE ('',( #59413 ) ) ;
#24282=VERTEX_POINT ( 'NONE', #12808 ) ;
#24284=PLANE ( 'NONE',  #54971 ) ;
#24286=CARTESIAN_POINT ( 'NONE',  ( -18.25000000000000000, -7.500000000000001776, 34.75000000000000000 ) ) ;
#24287=CARTESIAN_POINT ( 'NONE',  ( 18.13079180782478872, -5.582136614379148654, 34.36778462344220486 ) ) ;
#24289=CARTESIAN_POINT ( 'NONE',  ( -16.37677237136229991, -2.758268499246657068, 31.33685645148948851 ) ) ;
#24290=DIRECTION ( 'NONE',  ( -0.000000000000000000, -0.000000000000000000, -1.000000000000000000 ) ) ;
#24292=CARTESIAN_POINT ( 'NONE',  ( 6.000000000000001776, -2.833524468853757305, 32.15551576947925838 ) ) ;
#24293=CARTESIAN_POINT ( 'NONE',  ( 11.53846153846153832, -13.78497067705608181, 32.30358669280327177 ) ) ;
#24296=DIRECTION ( 'NONE',  ( -0.000000000000000000, 0.8660254037844397068, -0.4999999999999978906 ) ) ;
#24298=CARTESIAN_POINT ( 'NONE',  ( 3.230769230769108269, -12.51329471203414379, 31.30864560766407578 ) ) ;
#24299=CARTESIAN_POINT ( 'NONE',  ( -9.942330929600657896, -12.22074536777954989, 31.39888409691088356 ) ) ;
#24300=CARTESIAN_POINT ( 'NONE',  ( -12.46153846153858424, -8.656820664282941280, 34.87096338111179961 ) ) ;
#24301=CARTESIAN_POINT ( 'NONE',  ( 11.78851595837499211, -8.346898887586323923, 34.93166121998716278 ) ) ;
#24302=CARTESIAN_POINT ( 'NONE',  ( 10.86543892702293412, -2.779044189368095719, 31.39831045268885745 ) ) ;
#24303=CARTESIAN_POINT ( 'NONE',  ( 7.846153846153723244, -3.643525952248796163, 33.31231777344771672 ) ) ;
#24304=CARTESIAN_POINT ( 'NONE',  ( -2.980769230769293898, -7.565270445406050648, 34.75000000000000000 ) ) ;
#24306=ORIENTED_EDGE ( 'NONE', *, *, #66481, .F. ) ;
#24307=AXIS2_PLACEMENT_3D ( 'NONE', #15013, #28526, #42047 ) ;
#24308=CARTESIAN_POINT ( 'NONE',  ( -4.153846153846152411, -11.16473453929635440, 33.15142922261926373 ) ) ;
#24309=CARTESIAN_POINT ( 'NONE',  ( -12.21153846153852562, -7.565270445406050648, 34.75000000000000000 ) ) ;
#24310=FACE_OUTER_BOUND ( 'NONE', #68785, .T. ) ;
#24312=DIRECTION ( 'NONE',  ( -0.000000000000000000, 0.3420201433256694901, -0.9396926207859082059 ) ) ;
#24313=CARTESIAN_POINT ( 'NONE',  ( -15.23076923076935074, -10.90142922262034020, 33.41473453929536674 ) ) ;
#24314=CARTESIAN_POINT ( 'NONE',  ( -13.31854805126531005, -6.343179335718452272, 34.87096338111212646 ) ) ;
#24315=EDGE_LOOP ( 'NONE', ( #56161, #3795, #76349, #55854 ) ) ;
#24317=CARTESIAN_POINT ( 'NONE',  ( -1.384615384615383471, -12.34228464037088635, 31.77849191805839268 ) ) ;
#24318=ORIENTED_EDGE ( 'NONE', *, *, #48823, .T. ) ;
#24319=CARTESIAN_POINT ( 'NONE',  ( -4.023320715612509701, -2.647132371071621471, 31.75357179365173010 ) ) ;
#24320=EDGE_LOOP ( 'NONE', ( #64579, #23241, #66903, #69500 ) ) ;
#24321=CARTESIAN_POINT ( 'NONE',  ( -18.22292621751614305, -11.76352882383565301, 32.36236540154568075 ) ) ;
#24322=CARTESIAN_POINT ( 'NONE',  ( 13.31853197365950514, -9.780366693483667717, 34.19971097300155805 ) ) ;
#24323=CARTESIAN_POINT ( 'NONE',  ( 17.07692307692307665, -6.343179335718451384, 34.87096338111211935 ) ) ;
#24324=ORIENTED_EDGE ( 'NONE', *, *, #86961, .T. ) ;
#24325=CARTESIAN_POINT ( 'NONE',  ( -0.5920983751518260618, -2.254533558242299396, 29.97296025877828285 ) ) ;
#24328=EDGE_LOOP ( 'NONE', ( #23973, #1563 ) ) ;
#24329=B_SPLINE_CURVE_WITH_KNOTS ( 'NONE', 3,
 ( #81294, #52469, #33547, #31772, #5180, #60560, #60116, #53360, #74527, #67332 ),
 .UNSPECIFIED., .F., .F.,
 ( 4, 2, 2, 2, 4 ),
 ( 0.000000000000000000, 0.0001954311564186870913, 0.0003908623128373741825, 0.0005862934692560613009, 0.0007817246256747483650 ),
 .UNSPECIFIED. ) ;
#24330=AXIS2_PLACEMENT_3D ( 'NONE', #18429, #88686, #59852 ) ;
#24331=VECTOR ( 'NONE', #79862, 1000.000000000000114 ) ;
#24332=CARTESIAN_POINT ( 'NONE',  ( 2.177001704582000929, -9.084618155246140248, 34.75535874321725771 ) ) ;
#24333=CARTESIAN_POINT ( 'NONE',  ( 12.52760681254090258, -12.10708131394839704, 31.69288490824020954 ) ) ;
#24334=ORIENTED_EDGE ( 'NONE', *, *, #19707, .F. ) ;
#24335=CARTESIAN_POINT ( 'NONE',  ( -5.777220458731590291, -11.41317474335729187, 32.86274602512330034 ) ) ;
#24336=CARTESIAN_POINT ( 'NONE',  ( 10.61538461538461675, -8.564572088678739092, 35.78748833219616898 ) ) ;
#24337=CARTESIAN_POINT ( 'NONE',  ( -11.53846153846166089, -3.083524468854526912, 32.58852847137268327 ) ) ;
#24338=EDGE_CURVE ( 'NONE', #88630, #64217, #17800, .T. ) ;
#24340=CARTESIAN_POINT ( 'NONE',  ( -4.153846153846152411, -8.318370150425687726, 35.83090037661290239 ) ) ;
#24341=CARTESIAN_POINT ( 'NONE',  ( -7.976301815885541657, -12.70455904226513866, 30.44083106164009322 ) ) ;
#24342=EDGE_LOOP ( 'NONE', ( #33217, #23155 ) ) ;
#24344=EDGE_LOOP ( 'NONE', ( #24929, #22898, #21048, #38189 ) ) ;
#24345=CARTESIAN_POINT ( 'NONE',  ( -4.088591014333315066, -8.656820664281605460, 34.87096338111211224 ) ) ;
#24347=EDGE_CURVE ( 'NONE', #17177, #57142, #88567, .T. ) ;
#24348=CARTESIAN_POINT ( 'NONE',  ( 9.692307692307695177, -1.422936976036506707, 30.56769352161908415 ) ) ;
#24349=CARTESIAN_POINT ( 'NONE',  ( 6.249945409378045547, -10.18230066228895758, 34.26354781536631577 ) ) ;
#24350=EDGE_CURVE ( 'NONE', #81242, #19850, #14367, .T. ) ;
#24351=ORIENTED_EDGE ( 'NONE', *, *, #43589, .T. ) ;
#24352=EDGE_LOOP ( 'NONE', ( #86525, #44840 ) ) ;
#24353=VERTEX_POINT ( 'NONE', #21333 ) ;
#24354=LINE ( 'NONE', #65785, #15194 ) ;
#24355=ORIENTED_EDGE ( 'NONE', *, *, #12844, .F. ) ;
#24356=CARTESIAN_POINT ( 'NONE',  ( 2.307692307692187583, -4.481592998941358097, 33.73612834414048933 ) ) ;
#24357=EDGE_CURVE ( 'NONE', #67330, #76071, #55189, .T. ) ;
#24358=CARTESIAN_POINT ( 'NONE',  ( 16.94623247381277054, -12.35290016733513951, 31.75349464988449455 ) ) ;
#24359=CARTESIAN_POINT ( 'NONE',  ( 0.4615384615384611200, -4.786620604624113540, 33.94971097300155094 ) ) ;
#24360=FACE_BOUND ( 'NONE', #80512, .T. ) ;
#24361=ORIENTED_EDGE ( 'NONE', *, *, #81649, .F. ) ;
#24362=CARTESIAN_POINT ( 'NONE',  ( -8.769230769230768274, -8.973038597847269315, 34.52809138561121927 ) ) ;
#24363=CARTESIAN_POINT ( 'NONE',  ( 13.38461538461526423, -11.06231777344772027, 33.60647404775119895 ) ) ;
#24364=EDGE_CURVE ( 'NONE', #50087, #20467, #22978, .T. ) ;
#24365=DIRECTION ( 'NONE',  ( -0.000000000000000000, 0.9848077530122086864, -0.1736481776669273891 ) ) ;
#24366=LINE ( 'NONE', #86091, #40916 ) ;
#24367=DIRECTION ( 'NONE',  ( 0.000000000000000000, 0.4999999999999960032, -0.8660254037844410391 ) ) ;
#24368=VERTEX_POINT ( 'NONE', #69081 ) ;
#24369=CARTESIAN_POINT ( 'NONE',  ( 9.561616225640133138, -2.541943142973491554, 30.39792223712631980 ) ) ;
#24370=ORIENTED_EDGE ( 'NONE', *, *, #17808, .F. ) ;
#24372=DIRECTION ( 'NONE',  ( -0.000000000000000000, 0.5000000000000011102, -0.8660254037844380415 ) ) ;
#24373=CARTESIAN_POINT ( 'NONE',  ( 17.32692307692451195, -7.500000000000155431, 34.75000000000007105 ) ) ;
#24374=CARTESIAN_POINT ( 'NONE',  ( -10.61538461538461320, -12.10708131394839349, 31.69288490824020244 ) ) ;
#24375=FACE_OUTER_BOUND ( 'NONE', #85854, .T. ) ;
#24376=CARTESIAN_POINT ( 'NONE',  ( 1.449870955891409352, -10.21337939537593620, 33.94971097300152252 ) ) ;
#24377=CARTESIAN_POINT ( 'NONE',  ( 14.08476534878545827, -2.889293201056495786, 32.26117774369186009 ) ) ;
#24378=ORIENTED_EDGE ( 'NONE', *, *, #46579, .T. ) ;
#24379=ADVANCED_FACE ( 'NONE', ( #68637 ), #183, .F. ) ;
#24380=CARTESIAN_POINT ( 'NONE',  ( -5.326946301144534601, -6.652501968072646932, 34.93155406624980941 ) ) ;
#24381=CARTESIAN_POINT ( 'NONE',  ( -11.53846153846165912, -10.21337939537710326, 33.94971097300076224 ) ) ;
#24382=CARTESIAN_POINT ( 'NONE',  ( 10.61538461538449596, -3.300289026999228881, 32.46337939537708905 ) ) ;
#24383=ADVANCED_FACE ( 'NONE', ( #627 ), #26767, .F. ) ;
#24384=CARTESIAN_POINT ( 'NONE',  ( -13.60810030917971858, -12.69144148231606017, 30.53333754910549303 ) ) ;
#24385=ORIENTED_EDGE ( 'NONE', *, *, #61521, .T. ) ;
#24386=B_SPLINE_CURVE_WITH_KNOTS ( 'NONE', 3,
 ( #25742, #60406, #40158, #53203, #82027, #87464, #82475, #20319, #32946, #27070 ),
 .UNSPECIFIED., .F., .F.,
 ( 4, 2, 2, 2, 4 ),
 ( 0.0007817359430256217660, 0.0009771253907249859150, 0.001172514838424349847, 0.001367904286123713779, 0.001563293733823077928 ),
 .UNSPECIFIED. ) ;
#24387=EDGE_LOOP ( 'NONE', ( #61574, #49910 ) ) ;
#24388=FACE_BOUND ( 'NONE', #83990, .T. ) ;
#24389=AXIS2_PLACEMENT_3D ( 'NONE', #56821, #84320, #22594 ) ;
#24391=ADVANCED_FACE ( 'NONE', ( #42501 ), #7827, .F. ) ;
#24392=CARTESIAN_POINT ( 'NONE',  ( 11.66925197942848769, -12.35292014791297710, 31.75344720912887198 ) ) ;
#24394=EDGE_CURVE ( 'NONE', #56760, #19723, #75619, .T. ) ;
#24395=ORIENTED_EDGE ( 'NONE', *, *, #51909, .T. ) ;
#24396=CARTESIAN_POINT ( 'NONE',  ( -6.673076923075503153, -7.500000000000154543, 35.00000000000007105 ) ) ;
#24397=DIRECTION ( 'NONE',  ( -0.000000000000000000, -0.9396926207859093161, -0.3420201433256663259 ) ) ;
#24398=CARTESIAN_POINT ( 'NONE',  ( -7.976845312821404299, -11.71456829005830080, 32.44064028649416542 ) ) ;
#24399=CARTESIAN_POINT ( 'NONE',  ( -6.857008572074484221, -3.050289026998446840, 32.03036669348366416 ) ) ;
#24401=CARTESIAN_POINT ( 'NONE',  ( 4.826923076923076650, -7.500000000000001776, 35.00000000000000000 ) ) ;
#24402=VERTEX_POINT ( 'NONE', #40736 ) ;
#24404=ORIENTED_EDGE ( 'NONE', *, *, #1210, .F. ) ;
#24405=DIRECTION ( 'NONE',  ( -0.000000000000000000, 0.9848077530122086864, -0.1736481776669273891 ) ) ;
#24406=CARTESIAN_POINT ( 'NONE',  ( 4.023698944407932743, -6.852621066184267029, 34.70813303252209181 ) ) ;
#24407=DIRECTION ( 'NONE',  ( -0.000000000000000000, -0.7660444431189791237, -0.6427876096865379196 ) ) ;
#24408=CARTESIAN_POINT ( 'NONE',  ( -10.86536135943320502, -3.436278759898153901, 33.07459398097509506 ) ) ;
#24409=CARTESIAN_POINT ( 'NONE',  ( -8.096177083446809419, -9.271318131107980420, 34.42618302367067429 ) ) ;
#24410=CARTESIAN_POINT ( 'NONE',  ( 12.46153846153846168, -5.471508081941601098, 34.59228464037088457 ) ) ;
#24412=VERTEX_POINT ( 'NONE', #2815 ) ;
#24413=CARTESIAN_POINT ( 'NONE',  ( 14.08420738312797837, -2.353723527008296568, 30.78948104536958752 ) ) ;
#24414=CARTESIAN_POINT ( 'NONE',  ( 17.99999999999987566, -8.656820664282941280, 34.87096338111179961 ) ) ;
#24415=CYLINDRICAL_SURFACE ( 'NONE', #28022, 0.2499999999999986955 ) ;
#24416=ORIENTED_EDGE ( 'NONE', *, *, #12826, .T. ) ;
#24418=CARTESIAN_POINT ( 'NONE',  ( 9.758375025657770152, -3.322132147404559976, 32.92929555188717927 ) ) ;
#24420=CARTESIAN_POINT ( 'NONE',  ( 17.07692307692307665, -3.322132147404559976, 32.92929555188717927 ) ) ;
#24421=CARTESIAN_POINT ( 'NONE',  ( 10.61538461538461675, -5.557115091759785130, 34.35708131394839171 ) ) ;
#24422=CARTESIAN_POINT ( 'NONE',  ( 16.15384615384603251, -10.33852847137269571, 34.16647553114546554 ) ) ;
#24423=FACE_OUTER_BOUND ( 'NONE', #47398, .T. ) ;
#24424=CARTESIAN_POINT ( 'NONE',  ( -22.75000000000000000, -4.499999999999999112, 27.25000000000000000 ) ) ;
#24425=EDGE_LOOP ( 'NONE', ( #63584, #89044, #44340, #14676 ) ) ;
#24426=B_SPLINE_CURVE_WITH_KNOTS ( 'NONE', 3,
 ( #13331, #20963, #83585, #76359, #21861, #41254, #34489, #75920, #14220, #83128 ),
 .UNSPECIFIED., .F., .F.,
 ( 4, 2, 2, 2, 4 ),
 ( 0.000000000000000000, 0.0001954311564186865221, 0.0003908623128373730441, 0.0005862934692560595662, 0.0007817246256747460882 ),
 .UNSPECIFIED. ) ;
#24428=FACE_OUTER_BOUND ( 'NONE', #53382, .T. ) ;
#24429=CARTESIAN_POINT ( 'NONE',  ( -17.07692307692307665, -12.10708131394839349, 31.69288490824020244 ) ) ;
#24430=CARTESIAN_POINT ( 'NONE',  ( -13.38461538461538325, -5.180354513474913603, 36.12317359536750416 ) ) ;
#24431=CARTESIAN_POINT ( 'NONE',  ( 9.692307692307695177, -2.486705287966279876, 31.30864560766543647 ) ) ;
#24432=AXIS2_PLACEMENT_3D ( 'NONE', #62085, #7593, #41379 ) ;
#24433=ORIENTED_EDGE ( 'NONE', *, *, #56043, .F. ) ;
#24434=CARTESIAN_POINT ( 'NONE',  ( 12.71159277317677549, -3.627508038966690496, 32.91356715214248396 ) ) ;
#24435=EDGE_CURVE ( 'NONE', #73490, #32743, #46603, .T. ) ;
#24436=VERTEX_POINT ( 'NONE', #50568 ) ;
#24437=CARTESIAN_POINT ( 'NONE',  ( 12.39626846098214230, -9.528491918058357157, 34.59228464037090589 ) ) ;
#24438=CARTESIAN_POINT ( 'NONE',  ( -13.25456794936493310, -7.723484941389743952, 34.99544897038808955 ) ) ;
#24439=CARTESIAN_POINT ( 'NONE',  ( 17.75002325595140817, -10.06842814019191401, 34.32929386961144758 ) ) ;
#24440=ORIENTED_EDGE ( 'NONE', *, *, #40150, .F. ) ;
#24441=CARTESIAN_POINT ( 'NONE',  ( 8.769230769230647482, -10.90142922262034020, 33.41473453929536674 ) ) ;
#24442=DIRECTION ( 'NONE',  ( 1.000000000000000000, 0.000000000000000000, 0.000000000000000000 ) ) ;
#24443=CARTESIAN_POINT ( 'NONE',  ( 10.61538461538461675, -12.62096338111211580, 30.90682066428153263 ) ) ;
#24444=EDGE_CURVE ( 'NONE', #4302, #55479, #34775, .T. ) ;
#24445=CARTESIAN_POINT ( 'NONE',  ( -7.623374177175779920, -4.989023458446560255, 34.36081565061822118 ) ) ;
#24446=CARTESIAN_POINT ( 'NONE',  ( 3.296836564119307145, -2.833524468853757750, 32.15551576947925838 ) ) ;
#24447=ORIENTED_EDGE ( 'NONE', *, *, #39597, .T. ) ;
#24448=AXIS2_PLACEMENT_3D ( 'NONE', #18520, #23481, #16726 ) ;
#24449=CARTESIAN_POINT ( 'NONE',  ( 7.846153846153846700, -11.35647404775217417, 33.31231777344666511 ) ) ;
#24450=EDGE_LOOP ( 'NONE', ( #31689, #66460 ) ) ;
#24451=CARTESIAN_POINT ( 'NONE',  ( 5.076923076923075762, -11.35647404775217417, 33.31231777344666511 ) ) ;
#24452=CARTESIAN_POINT ( 'NONE',  ( -10.55019063360125742, -2.506253911140448487, 29.99999999999988631 ) ) ;
#24453=AXIS2_PLACEMENT_3D ( 'NONE', #36809, #84574, #9780 ) ;
#24454=CIRCLE ( 'NONE', #74825, 0.2500000000000002220 ) ;
#24455=CARTESIAN_POINT ( 'NONE',  ( -13.45069879557126669, -2.721908614388770964, 31.22303859784723912 ) ) ;
#24456=EDGE_CURVE ( 'NONE', #88631, #71689, #31589, .T. ) ;
#24457=CYLINDRICAL_SURFACE ( 'NONE', #37249, 0.2499999999999997502 ) ;
#24458=B_SPLINE_CURVE_WITH_KNOTS ( 'NONE', 3,
 ( #31249, #85317, #45653, #65913, #86670, #46103 ),
 .UNSPECIFIED., .F., .F.,
 ( 4, 2, 4 ),
 ( 0.0003909512603274038984, 0.0005862562993132300771, 0.0007815613382990563643 ),
 .UNSPECIFIED. ) ;
#24459=LINE ( 'NONE', #5093, #9145 ) ;
#24460=CARTESIAN_POINT ( 'NONE',  ( 15.00784301325308157, -11.76352882383564769, 32.36236540154569497 ) ) ;
#24461=EDGE_CURVE ( 'NONE', #63896, #52314, #51428, .T. ) ;
#24464=ORIENTED_EDGE ( 'NONE', *, *, #52052, .T. ) ;
#24465=VERTEX_POINT ( 'NONE', #22660 ) ;
#24466=ORIENTED_EDGE ( 'NONE', *, *, #8101, .F. ) ;
#24467=ORIENTED_EDGE ( 'NONE', *, *, #66590, .F. ) ;
#24468=ORIENTED_EDGE ( 'NONE', *, *, #11959, .T. ) ;
#24469=CARTESIAN_POINT ( 'NONE',  ( -1.318547033612945674, -3.050289026998446840, 32.03036669348366416 ) ) ;
#24470=CARTESIAN_POINT ( 'NONE',  ( 12.46153846153846168, -10.05456864172156806, 36.03766855953608683 ) ) ;
#24471=DIRECTION ( 'NONE',  ( -0.000000000000000000, 1.000000000000000000, -0.000000000000000000 ) ) ;
#24472=DIRECTION ( 'NONE',  ( -0.000000000000000000, -0.3420201433256694346, -0.9396926207859080948 ) ) ;
#24473=CARTESIAN_POINT ( 'NONE',  ( 7.596177102105255763, -12.65889640711025521, 30.72598325615533454 ) ) ;
#24474=CARTESIAN_POINT ( 'NONE',  ( 3.100622021331010725, -6.001485441113818986, 34.52039167877662607 ) ) ;
#24475=DIRECTION ( 'NONE',  ( 0.000000000000000000, 0.000000000000000000, 1.000000000000000000 ) ) ;
#24476=CARTESIAN_POINT ( 'NONE',  ( 9.692307692307695177, -9.905515769479276145, 34.41647553114623292 ) ) ;
#24477=CARTESIAN_POINT ( 'NONE',  ( 12.46153846153846168, -10.51840700105979565, 33.73612834413961536 ) ) ;
#24478=ORIENTED_EDGE ( 'NONE', *, *, #7732, .F. ) ;
#24479=ORIENTED_EDGE ( 'NONE', *, *, #83898, .T. ) ;
#24482=EDGE_LOOP ( 'NONE', ( #10033, #41029, #19713, #82106 ) ) ;
#24483=CARTESIAN_POINT ( 'NONE',  ( 6.857806922520602200, -11.67786785259541027, 32.92929555188721480 ) ) ;
#24484=DIRECTION ( 'NONE',  ( -0.000000000000000000, -0.3420201433256694901, -0.9396926207859082059 ) ) ;
#24485=CARTESIAN_POINT ( 'NONE',  ( 1.384615384615386802, -4.661471528628507777, 34.16647553114623292 ) ) ;
#24487=FACE_BOUND ( 'NONE', #9259, .T. ) ;
#24488=ORIENTED_EDGE ( 'NONE', *, *, #27145, .F. ) ;
#24490=VECTOR ( 'NONE', #16675, 1000.000000000000000 ) ;
#24491=ORIENTED_EDGE ( 'NONE', *, *, #43371, .F. ) ;
#24493=ORIENTED_EDGE ( 'NONE', *, *, #51099, .F. ) ;
#24494=ADVANCED_FACE ( 'NONE', ( #78930 ), #44236, .F. ) ;
#24495=FACE_BOUND ( 'NONE', #62669, .T. ) ;
#24497=CARTESIAN_POINT ( 'NONE',  ( -14.43784027742400689, -6.809168938359901446, 34.95455904226513866 ) ) ;
#24499=CARTESIAN_POINT ( 'NONE',  ( 14.24242186173153435, -2.892918686051582533, 31.69288490824015980 ) ) ;
#24501=EDGE_CURVE ( 'NONE', #61262, #14730, #43379, .T. ) ;
#24502=FACE_OUTER_BOUND ( 'NONE', #42203, .T. ) ;
#24503=EDGE_LOOP ( 'NONE', ( #74358, #19748 ) ) ;
#24504=B_SPLINE_CURVE_WITH_KNOTS ( 'NONE', 3,
 ( #29020, #10050, #64984, #56475, #83965, #57356, #3288, #30764, #70438, #63667 ),
 .UNSPECIFIED., .F., .F.,
 ( 4, 2, 2, 2, 4 ),
 ( 0.000000000000000000, 0.0001954339857564092904, 0.0003908679715128185808, 0.0005863019572692278712, 0.0007817359430256371616 ),
 .UNSPECIFIED. ) ;
#24505=CARTESIAN_POINT ( 'NONE',  ( -11.66915214157184622, -4.684245665217972032, 34.18127051446801090 ) ) ;
#24506=CARTESIAN_POINT ( 'NONE',  ( 2.980792499826877773, -12.17611988154120972, 31.52148481390971213 ) ) ;
#24508=CARTESIAN_POINT ( 'NONE',  ( 7.846153846153846700, -11.35647404775217417, 33.31231777344666511 ) ) ;
#24509=CARTESIAN_POINT ( 'NONE',  ( 11.53846153846153832, -13.75783147151868846, 33.36296068462461051 ) ) ;
#24511=CARTESIAN_POINT ( 'NONE',  ( 3.230769230769231726, -6.343179335718451384, 34.87096338111211935 ) ) ;
#24512=CARTESIAN_POINT ( 'NONE',  ( 14.53070365930516061, -8.239487800360276282, 34.69522927552633718 ) ) ;
#24513=CARTESIAN_POINT ( 'NONE',  ( -2.438383774359866418, -2.541943142973489778, 30.39792223712631980 ) ) ;
#24514=DIRECTION ( 'NONE',  ( 0.000000000000000000, 0.1736481776669275834, 0.9848077530122086864 ) ) ;
#24515=DIRECTION ( 'NONE',  ( 0.000000000000000000, 1.000000000000000000, 0.000000000000000000 ) ) ;
#24517=CARTESIAN_POINT ( 'NONE',  ( -1.515306851282940404, -2.729777683071817229, 31.24903638046269094 ) ) ;
#24519=CARTESIAN_POINT ( 'NONE',  ( -0.2387587925603957550, -8.540255544307065350, 34.89611431652622286 ) ) ;
#24520=LINE ( 'NONE', #64606, #81776 ) ;
#24521=DIRECTION ( 'NONE',  ( -0.000000000000000000, 1.000000000000000000, -0.000000000000000000 ) ) ;
#24524=ORIENTED_EDGE ( 'NONE', *, *, #36667, .F. ) ;
#24525=CARTESIAN_POINT ( 'NONE',  ( 0.3313912521002411737, -12.45813303252208648, 30.39737893381572675 ) ) ;
#24526=ORIENTED_EDGE ( 'NONE', *, *, #74410, .F. ) ;
#24528=VECTOR ( 'NONE', #47874, 1000.000000000000000 ) ;
#24529=EDGE_CURVE ( 'NONE', #27245, #66929, #27280, .T. ) ;
#24530=ORIENTED_EDGE ( 'NONE', *, *, #59426, .T. ) ;
#24531=CARTESIAN_POINT ( 'NONE',  ( -2.084912766423897335, -12.44528174975671853, 30.48912976160716681 ) ) ;
#24535=CARTESIAN_POINT ( 'NONE',  ( 18.00000000000000000, -12.78798330534102945, 29.74999999999997868 ) ) ;
#24537=CARTESIAN_POINT ( 'NONE',  ( 9.758376043310132530, -11.16473453929635440, 33.15142922261926373 ) ) ;
#24538=CARTESIAN_POINT ( 'NONE',  ( 13.51514082284902862, -3.068774925481848825, 32.56582465632704526 ) ) ;
#24539=CARTESIAN_POINT ( 'NONE',  ( -12.39628332202562433, -4.320704448112861584, 33.92786785259548310 ) ) ;
#24540=CARTESIAN_POINT ( 'NONE',  ( 15.00784227186238162, -8.282780595021769443, 34.94152052738834868 ) ) ;
#24541=CARTESIAN_POINT ( 'NONE',  ( -10.68065506134538545, -4.481592998940162609, 33.73612834413957984 ) ) ;
#24542=CARTESIAN_POINT ( 'NONE',  ( 0.7115928814519150158, -2.544122305571458575, 31.48381861865057729 ) ) ;
#24546=CARTESIAN_POINT ( 'NONE',  ( 1.384615384615386802, -2.721908614388771852, 31.22303859784724978 ) ) ;
#24547=CARTESIAN_POINT ( 'NONE',  ( 13.31934538405906743, -3.643525952247789412, 33.31231777344662959 ) ) ;
#24548=B_SPLINE_CURVE_WITH_KNOTS ( 'NONE', 3,
 ( #83368, #29749, #82489, #21655, #49126, #76149, #14459, #7712, #20768, #14912 ),
 .UNSPECIFIED., .F., .F.,
 ( 4, 2, 2, 2, 4 ),
 ( 0.0007817359430256252354, 0.0009771253907249902518, 0.001172514838424355051, 0.001367904286123720068, 0.001563293733823085084 ),
 .UNSPECIFIED. ) ;
#24549=FACE_OUTER_BOUND ( 'NONE', #11009, .T. ) ;
#24550=B_SPLINE_CURVE_WITH_KNOTS ( 'NONE', 3,
 ( #21679, #88835, #33431, #34304, #14480, #27105, #20791, #28437, #34749, #81617 ),
 .UNSPECIFIED., .F., .F.,
 ( 4, 2, 2, 2, 4 ),
 ( 0.000000000000000000, 0.0001954339857564091278, 0.0003908679715128182556, 0.0005863019572692274375, 0.0007817359430256365111 ),
 .UNSPECIFIED. ) ;
#24552=ORIENTED_EDGE ( 'NONE', *, *, #43371, .T. ) ;
#24553=EDGE_LOOP ( 'NONE', ( #51234, #9503, #9974, #75775 ) ) ;
#24554=DIRECTION ( 'NONE',  ( -0.000000000000000000, 1.000000000000000000, -0.000000000000000000 ) ) ;
#24556=CARTESIAN_POINT ( 'NONE',  ( 16.28437159207980045, -12.50538340440932394, 31.33453814440721885 ) ) ;
#24558=CARTESIAN_POINT ( 'NONE',  ( 8.769230769230768274, -11.69971097300155272, 32.46337939537588113 ) ) ;
#24559=DIRECTION ( 'NONE',  ( 0.000000000000000000, -0.000000000000000000, -1.000000000000000000 ) ) ;
#24560=EDGE_CURVE ( 'NONE', #2196, #34824, #43403, .T. ) ;
#24561=EDGE_CURVE ( 'NONE', #60387, #30501, #2539, .T. ) ;
#24562=ORIENTED_EDGE ( 'NONE', *, *, #61596, .F. ) ;
#24563=CARTESIAN_POINT ( 'NONE',  ( 12.46153846153833911, -12.51329471203414379, 31.30864560766407578 ) ) ;
#24564=ORIENTED_EDGE ( 'NONE', *, *, #28128, .T. ) ;
#24566=VERTEX_POINT ( 'NONE', #4612 ) ;
#24567=CARTESIAN_POINT ( 'NONE',  ( 7.596177102105255763, -10.82459398097509506, 33.81372124010185587 ) ) ;
#24568=B_SPLINE_CURVE_WITH_KNOTS ( 'NONE', 3,
 ( #80683, #87900, #40139, #19404, #54064, #61259 ),
 .UNSPECIFIED., .F., .F.,
 ( 4, 2, 4 ),
 ( 0.0003909569690057804843, 0.0005862646681846042955, 0.0007815723673634281067 ),
 .UNSPECIFIED. ) ;
#24570=CARTESIAN_POINT ( 'NONE',  ( -0.2115384615370421995, -7.500000000000154543, 35.00000000000007105 ) ) ;
#24571=CARTESIAN_POINT ( 'NONE',  ( -11.28846153846153655, -2.499999999999998668, 29.75000000000000355 ) ) ;
#24572=CARTESIAN_POINT ( 'NONE',  ( -5.143005456283213483, -8.164416787775445883, 34.95778746994557906 ) ) ;
#24573=ADVANCED_FACE ( 'NONE', ( #5056 ), #51885, .F. ) ;
#24574=B_SPLINE_CURVE_WITH_KNOTS ( 'NONE', 3,
 ( #47654, #18853, #74243, #13421, #54854, #73807 ),
 .UNSPECIFIED., .F., .F.,
 ( 4, 2, 4 ),
 ( 0.5000000000000000000, 0.7500000000000000000, 1.000000000000000000 ),
 .UNSPECIFIED. ) ;
#24575=EDGE_LOOP ( 'NONE', ( #62876, #56751, #64093, #48985 ) ) ;
#24577=B_SPLINE_CURVE_WITH_KNOTS ( 'NONE', 3,
 ( #54856, #41797, #41345, #82340, #56184, #40904, #21960, #68367, #6666, #15207 ),
 .UNSPECIFIED., .F., .F.,
 ( 4, 2, 2, 2, 4 ),
 ( 0.0007817359430256294638, 0.0009771253907249976244, 0.001172514838424365676, 0.001367904286123733729, 0.001563293733823094625 ),
 .UNSPECIFIED. ) ;
#24578=ORIENTED_EDGE ( 'NONE', *, *, #85284, .T. ) ;
#24581=CARTESIAN_POINT ( 'NONE',  ( -3.903791733932698182, -12.01375889529407281, 32.43194544308182969 ) ) ;
#24582=CARTESIAN_POINT ( 'NONE',  ( 9.822833130541338775, -2.372941743896879174, 30.88044141588253666 ) ) ;
#24583=DIRECTION ( 'NONE',  ( -0.000000000000000000, 1.000000000000000000, 3.491481338843133355E-15 ) ) ;
#24586=CARTESIAN_POINT ( 'NONE',  ( 10.48523664565292002, -5.070767119584671079, 34.40440758774516183 ) ) ;
#24587=CARTESIAN_POINT ( 'NONE',  ( -4.403869391139117795, -8.432397168068783699, 34.66272746175022945 ) ) ;
#24588=CARTESIAN_POINT ( 'NONE',  ( -1.634615384615383027, -7.500000000000001776, 34.75000000000000000 ) ) ;
#24589=EDGE_LOOP ( 'NONE', ( #54681, #3950, #16280, #82852 ) ) ;
#24590=ORIENTED_EDGE ( 'NONE', *, *, #63489, .F. ) ;
#24593=CARTESIAN_POINT ( 'NONE',  ( -13.63459212866397685, -5.643011162660950042, 34.66104346484419096 ) ) ;
#24594=VERTEX_POINT ( 'NONE', #46038 ) ;
#24595=CARTESIAN_POINT ( 'NONE',  ( -9.822998295418001291, -9.929715669179220328, 34.40415004197138416 ) ) ;
#24598=ORIENTED_EDGE ( 'NONE', *, *, #53851, .T. ) ;
#24599=B_SPLINE_CURVE_WITH_KNOTS ( 'NONE', 3,
 ( #87748, #26023, #53482, #2084, #29573, #27788, #324, #49396, #55696, #29138 ),
 .UNSPECIFIED., .F., .F.,
 ( 4, 2, 2, 2, 4 ),
 ( 0.0007817359527651132059, 0.0009771254036996528287, 0.001172514854634192560, 0.001367904305568732291, 0.001563293756503272023 ),
 .UNSPECIFIED. ) ;
#24600=FACE_OUTER_BOUND ( 'NONE', #61748, .T. ) ;
#24601=ORIENTED_EDGE ( 'NONE', *, *, #41493, .T. ) ;
#24602=CARTESIAN_POINT ( 'NONE',  ( 5.777073041093150785, -9.172386477786396597, 34.72672124145550043 ) ) ;
#24603=CARTESIAN_POINT ( 'NONE',  ( 4.153846153846154188, -3.322132147404559976, 32.92929555188717927 ) ) ;
#24604=EDGE_CURVE ( 'NONE', #46048, #38377, #78806, .T. ) ;
#24605=CARTESIAN_POINT ( 'NONE',  ( 7.596130621932389637, -4.175268141568689195, 33.81360843649122216 ) ) ;
#24606=CARTESIAN_POINT ( 'NONE',  ( -6.923076923077044142, -4.481592998941358097, 33.73612834414048933 ) ) ;
#24607=FACE_OUTER_BOUND ( 'NONE', #37461, .T. ) ;
#24608=LINE ( 'NONE', #34803, #6456 ) ;
#24609=CARTESIAN_POINT ( 'NONE',  ( -10.61538461538473399, -10.90142922262034020, 33.41473453929536674 ) ) ;
#24610=ORIENTED_EDGE ( 'NONE', *, *, #41622, .T. ) ;
#24612=EDGE_CURVE ( 'NONE', #35523, #42119, #42301, .T. ) ;
#24613=CARTESIAN_POINT ( 'NONE',  ( 15.23076923076923173, -4.098570777380720287, 33.41473453929634729 ) ) ;
#24614=ORIENTED_EDGE ( 'NONE', *, *, #36763, .T. ) ;
#24615=EDGE_CURVE ( 'NONE', #65392, #85801, #10925, .T. ) ;
#24616=B_SPLINE_CURVE_WITH_KNOTS ( 'NONE', 3,
 ( #70711, #2670, #22957, #77900, #16638, #44099, #64815, #28386, #52197, #45890 ),
 .UNSPECIFIED., .F., .F.,
 ( 4, 2, 2, 2, 4 ),
 ( 0.0007817359430256301143, 0.0009771253907249963233, 0.001172514838424362641, 0.001367904286123728958, 0.001563293733823095276 ),
 .UNSPECIFIED. ) ;
#24617=CARTESIAN_POINT ( 'NONE',  ( 6.923076923076924238, -9.780366693483667717, 34.19971097300155094 ) ) ;
#24618=VECTOR ( 'NONE', #71195, 1000.000000000000227 ) ;
#24619=CARTESIAN_POINT ( 'NONE',  ( 16.82694633287448838, -10.82459398097509862, 33.81372124010183455 ) ) ;
#24620=CARTESIAN_POINT ( 'NONE',  ( 10.36540787133602493, -8.347322224742351082, 34.93158281831414769 ) ) ;
#24622=CARTESIAN_POINT ( 'NONE',  ( 12.21156173059610772, -4.236021600441997492, 33.53823185664189310 ) ) ;
#24623=FACE_BOUND ( 'NONE', #47637, .T. ) ;
#24624=CARTESIAN_POINT ( 'NONE',  ( 12.33084699487089964, -3.062553014421049546, 32.05460306192773601 ) ) ;
#24625=CARTESIAN_POINT ( 'NONE',  ( 20.75000000000000000, -10.50000000000000000, 29.75000000000000355 ) ) ;
#24627=CARTESIAN_POINT ( 'NONE',  ( -11.31503457659996847, -7.630147231320743018, 34.74852402298682819 ) ) ;
#24628=CARTESIAN_POINT ( 'NONE',  ( -10.61538461538473577, -11.67786785259630911, 32.92929555188603530 ) ) ;
#24629=CARTESIAN_POINT ( 'NONE',  ( 3.230769230769231726, -13.20930481340135110, 34.54067556320372745 ) ) ;
#24631=EDGE_CURVE ( 'NONE', #25475, #81411, #84262, .T. ) ;
#24632=DIRECTION ( 'NONE',  ( 0.000000000000000000, 0.8660254037844377084, 0.5000000000000015543 ) ) ;
#24634=ORIENTED_EDGE ( 'NONE', *, *, #50599, .F. ) ;
#24635=CARTESIAN_POINT ( 'NONE',  ( -7.911424292114620727, -11.48612834413959582, 32.76840700105983473 ) ) ;
#24637=DIRECTION ( 'NONE',  ( 0.000000000000000000, 0.4999999999999960032, -0.8660254037844410391 ) ) ;
#24641=CARTESIAN_POINT ( 'NONE',  ( 5.207448515156719360, -12.15418822224088657, 32.17964115625579069 ) ) ;
#24643=CARTESIAN_POINT ( 'NONE',  ( -2.372962308248625973, -3.643525952247789412, 33.31231777344662959 ) ) ;
#24644=CARTESIAN_POINT ( 'NONE',  ( 8.769230769230768274, -2.486705287966279876, 31.30864560766543647 ) ) ;
#24645=CARTESIAN_POINT ( 'NONE',  ( 17.07692307692307665, -1.466349020453238561, 30.81389545987213907 ) ) ;
#24646=CARTESIAN_POINT ( 'NONE',  ( -1.384615384615505151, -12.46129190930018460, 30.37095296980731973 ) ) ;
#24647=CARTESIAN_POINT ( 'NONE',  ( 0.2380535178145138098, -11.41268669641500466, 32.86336882939237825 ) ) ;
#24648=CARTESIAN_POINT ( 'NONE',  ( -11.40766973063674961, -9.804649428959608670, 34.18742332936588468 ) ) ;
#24649=LINE ( 'NONE', #10257, #3055 ) ;
#24650=VECTOR ( 'NONE', #22210, 1000.000000000000227 ) ;
#24652=ORIENTED_EDGE ( 'NONE', *, *, #53337, .T. ) ;
#24654=FACE_OUTER_BOUND ( 'NONE', #39143, .T. ) ;
#24658=CARTESIAN_POINT ( 'NONE',  ( 18.00000000000000000, -11.35647404775217417, 33.31231777344666511 ) ) ;
#24659=CARTESIAN_POINT ( 'NONE',  ( -22.75000000000000000, -4.499999999999999112, 29.75000000000000355 ) ) ;
#24660=ORIENTED_EDGE ( 'NONE', *, *, #52361, .T. ) ;
#24661=CARTESIAN_POINT ( 'NONE',  ( -18.06527044596078113, -9.442884908240170461, 34.35708131394842013 ) ) ;
#24664=ORIENTED_EDGE ( 'NONE', *, *, #50958, .T. ) ;
#24665=CARTESIAN_POINT ( 'NONE',  ( 11.66925197942848769, -4.684288915650983043, 34.18129842949671371 ) ) ;
#24666=DIRECTION ( 'NONE',  ( -0.000000000000000000, 0.7660444431189791237, -0.6427876096865379196 ) ) ;
#24667=CARTESIAN_POINT ( 'NONE',  ( -4.853911725310227077, -9.086983370893049639, 34.49168942202179267 ) ) ;
#24668=CARTESIAN_POINT ( 'NONE',  ( -12.59168643127016196, -5.070767119584671079, 34.40440758774516183 ) ) ;
#24669=EDGE_LOOP ( 'NONE', ( #41638, #14765 ) ) ;
#24670=DIRECTION ( 'NONE',  ( 0.000000000000000000, 0.6427876096865368094, 0.7660444431189802339 ) ) ;
#24671=CARTESIAN_POINT ( 'NONE',  ( -12.71151520558705172, -2.544273027872575366, 31.48422191005632342 ) ) ;
#24673=EDGE_CURVE ( 'NONE', #54559, #66691, #39112, .T. ) ;
#24674=CARTESIAN_POINT ( 'NONE',  ( 14.98074600654777377, -10.18141759479407327, 34.26406193332782379 ) ) ;
#24675=ORIENTED_EDGE ( 'NONE', *, *, #210, .F. ) ;
#24676=VERTEX_POINT ( 'NONE', #3549 ) ;
#24677=B_SPLINE_CURVE_WITH_KNOTS ( 'NONE', 3,
 ( #40129, #82444, #458, #88765, #46863, #895, #13964, #55394, #55834, #41442 ),
 .UNSPECIFIED., .F., .F.,
 ( 4, 2, 2, 2, 4 ),
 ( 0.000000000000000000, 0.0001954311564186871184, 0.0003908623128373742367, 0.0005862934692560614093, 0.0007817246256747484735 ),
 .UNSPECIFIED. ) ;
#24678=EDGE_LOOP ( 'NONE', ( #30302, #49394 ) ) ;
#24679=FACE_OUTER_BOUND ( 'NONE', #7440, .T. ) ;
#24680=CARTESIAN_POINT ( 'NONE',  ( 6.130790440966951138, -2.295524264805589354, 30.44142389570982488 ) ) ;
#24681=B_SPLINE_CURVE_WITH_KNOTS ( 'NONE', 3,
 ( #55243, #26893, #82734, #81848, #7514, #89057, #75518, #21905, #7062, #21008 ),
 .UNSPECIFIED., .F., .F.,
 ( 4, 2, 2, 2, 4 ),
 ( 0.0007817246256747460882, 0.0009771112852218900684, 0.001172497944769033832, 0.001367884604316177595, 0.001563271263863321575 ),
 .UNSPECIFIED. ) ;
#24682=CARTESIAN_POINT ( 'NONE',  ( -18.00000000000012079, -12.27809138561165270, 31.22303859784587132 ) ) ;
#24683=EDGE_CURVE ( 'NONE', #33151, #19849, #24103, .T. ) ;
#24684=CARTESIAN_POINT ( 'NONE',  ( 15.16468581981334651, -3.513871655860377086, 32.76840700105978499 ) ) ;
#24686=ADVANCED_FACE ( 'NONE', ( #2652 ), #30145, .F. ) ;
#24687=EDGE_CURVE ( 'NONE', #18603, #30988, #53136, .T. ) ;
#24688=EDGE_LOOP ( 'NONE', ( #67699, #34871, #83534, #60631 ) ) ;
#24689=ORIENTED_EDGE ( 'NONE', *, *, #52116, .T. ) ;
#24690=CARTESIAN_POINT ( 'NONE',  ( -1.134669866267242533, -5.057305518903949526, 34.11320923018887896 ) ) ;
#24692=CARTESIAN_POINT ( 'NONE',  ( -5.142193077479396024, -2.657715359629089225, 31.77849191805834295 ) ) ;
#24694=EDGE_CURVE ( 'NONE', #60609, #55169, #55205, .T. ) ;
#24696=CARTESIAN_POINT ( 'NONE',  ( -15.23076923076922995, -2.499999999999998668, 29.75000000000001421 ) ) ;
#24697=CARTESIAN_POINT ( 'NONE',  ( -13.25382357679060519, -12.38066358083363738, 30.83685684665853444 ) ) ;
#24698=ORIENTED_EDGE ( 'NONE', *, *, #34747, .T. ) ;
#24699=ORIENTED_EDGE ( 'NONE', *, *, #49703, .T. ) ;
#24700=ORIENTED_EDGE ( 'NONE', *, *, #78758, .F. ) ;
#24701=CARTESIAN_POINT ( 'NONE',  ( -13.25457032869561402, -2.254550872974305342, 29.97347326024527092 ) ) ;
#24702=ORIENTED_EDGE ( 'NONE', *, *, #19024, .T. ) ;
#24703=LINE ( 'NONE', #38662, #86347 ) ;
#24704=CARTESIAN_POINT ( 'NONE',  ( 18.13079044096695469, -5.496552790871120031, 34.60292014791297532 ) ) ;
#24705=ORIENTED_EDGE ( 'NONE', *, *, #23423, .F. ) ;
#24706=MECHANICAL_DESIGN_GEOMETRIC_PRESENTATION_REPRESENTATION('',(#29349),#72806);
#24707=CARTESIAN_POINT ( 'NONE',  ( -8.769230769230890843, -10.90142922262034020, 33.41473453929536674 ) ) ;
#24708=DIRECTION ( 'NONE',  ( 0.000000000000000000, 0.7660444431189807890, 0.6427876096865361433 ) ) ;
#24709=CARTESIAN_POINT ( 'NONE',  ( -5.776987155906603277, -3.395485233115139057, 33.02377354290275946 ) ) ;
#24710=FACE_BOUND ( 'NONE', #78334, .T. ) ;
#24712=CARTESIAN_POINT ( 'NONE',  ( 6.000000000000001776, -10.51840700105979565, 33.73612834413961536 ) ) ;
#24713=EDGE_CURVE ( 'NONE', #49885, #3333, #63813, .T. ) ;
#24714=VECTOR ( 'NONE', #85773, 999.9999999999998863 ) ;
#24715=CARTESIAN_POINT ( 'NONE',  ( -6.923076923076922462, -12.78798330534103123, 29.99999999999997868 ) ) ;
#24716=CARTESIAN_POINT ( 'NONE',  ( 17.07692307692338218, -2.506253911140615021, 30.00000000000323297 ) ) ;
#24717=CARTESIAN_POINT ( 'NONE',  ( -8.519285359852728945, -12.07971442181322175, 32.31769673815850297 ) ) ;
#24719=CARTESIAN_POINT ( 'NONE',  ( 16.15384615384615330, -11.91647553114624181, 32.58852847137148245 ) ) ;
#24720=CARTESIAN_POINT ( 'NONE',  ( 5.299702618191482806, -2.600157965045225339, 30.74683119005207743 ) ) ;
#24721=ORIENTED_EDGE ( 'NONE', *, *, #58489, .F. ) ;
#24722=CARTESIAN_POINT ( 'NONE',  ( 8.769230769230768274, -2.538708090699994813, 30.37095296980875503 ) ) ;
#24723=CARTESIAN_POINT ( 'NONE',  ( -7.623142494540995351, -2.554770724473668153, 30.48948780036025852 ) ) ;
#24725=EDGE_LOOP ( 'NONE', ( #61101, #24468, #39342, #70009 ) ) ;
#24726=DIRECTION ( 'NONE',  ( -0.000000000000000000, 1.000000000000000000, 3.491481338843133355E-15 ) ) ;
#24727=CARTESIAN_POINT ( 'NONE',  ( 1.515405825582336607, -5.496552790871119143, 34.60292014791297532 ) ) ;
#24728=CARTESIAN_POINT ( 'NONE',  ( -0.7115384615384742206, -2.499999999999999556, 29.81609845454692120 ) ) ;
#24729=CARTESIAN_POINT ( 'NONE',  ( 3.230769230769231726, -9.905515769479276145, 34.41647553114623292 ) ) ;
#24730=DIRECTION ( 'NONE',  ( 0.000000000000000000, 0.8660254037844377084, 0.5000000000000015543 ) ) ;
#24731=ORIENTED_EDGE ( 'NONE', *, *, #38013, .T. ) ;
#24732=DIRECTION ( 'NONE',  ( -0.000000000000000000, 0.9396926207859093161, -0.3420201433256662704 ) ) ;
#24733=CARTESIAN_POINT ( 'NONE',  ( 18.24994540937804643, -4.176053281294515251, 33.81426240980091791 ) ) ;
#24734=CARTESIAN_POINT ( 'NONE',  ( 11.76124120743959978, -3.020022701398814569, 32.48759521482552515 ) ) ;
#24735=CARTESIAN_POINT ( 'NONE',  ( -9.942330929600657896, -4.335965774309648246, 33.62209801155881905 ) ) ;
#24736=CARTESIAN_POINT ( 'NONE',  ( 7.622668902429897919, -5.912607949931405038, 34.49155766932282319 ) ) ;
#24737=LINE ( 'NONE', #9887, #19444 ) ;
#24738=CARTESIAN_POINT ( 'NONE',  ( 2.373759641042384683, -5.471508081941601098, 34.59228464037088457 ) ) ;
#24741=ORIENTED_EDGE ( 'NONE', *, *, #26252, .T. ) ;
#24743=DIRECTION ( 'NONE',  ( 0.000000000000000000, 0.000000000000000000, 1.000000000000000000 ) ) ;
#24744=CARTESIAN_POINT ( 'NONE',  ( 9.692307692307572609, -10.21337939537710326, 33.94971097300076224 ) ) ;
#24745=CARTESIAN_POINT ( 'NONE',  ( -16.28453762051371356, -4.809359713505814149, 33.96456829005828837 ) ) ;
#24746=CARTESIAN_POINT ( 'NONE',  ( -0.4615384615385840772, -12.16647553114689728, 32.15551576947799362 ) ) ;
#24748=DIRECTION ( 'NONE',  ( -0.000000000000000000, 0.9396926207859092051, -0.3420201433256662704 ) ) ;
#24749=CARTESIAN_POINT ( 'NONE',  ( 1.607626736228235709, -4.887748414852792322, 34.01359900205216746 ) ) ;
#24750=EDGE_CURVE ( 'NONE', #69684, #44956, #41336, .T. ) ;
#24752=CARTESIAN_POINT ( 'NONE',  ( 13.16168842570853492, -10.01117774369187252, 34.36070679894347535 ) ) ;
#24753=DIRECTION ( 'NONE',  ( 0.000000000000000000, 0.4999999999999985567, 0.8660254037844395958 ) ) ;
#24754=CARTESIAN_POINT ( 'NONE',  ( -9.915792636031639518, -12.24155766932282496, 31.33739205006857986 ) ) ;
#24755=VECTOR ( 'NONE', #83463, 1000.000000000000114 ) ;
#24756=B_SPLINE_CURVE_WITH_KNOTS ( 'NONE', 3,
 ( #39073, #59770, #46261, #80500, #19238, #10699, #38165, #45358, #65622, #18793 ),
 .UNSPECIFIED., .F., .F.,
 ( 4, 2, 2, 2, 4 ),
 ( 0.0007817246256747464135, 0.0009771112852218902852, 0.001172497944769034265, 0.001367884604316178029, 0.001563271263863322009 ),
 .UNSPECIFIED. ) ;
#24757=FACE_OUTER_BOUND ( 'NONE', #10464, .T. ) ;
#24758=CARTESIAN_POINT ( 'NONE',  ( -2.307692307692428724, -5.941354392335915335, 34.76329471203413846 ) ) ;
#24759=CARTESIAN_POINT ( 'NONE',  ( -0.2385271099256120741, -11.24521262558773671, 33.06293181088029343 ) ) ;
#24762=ORIENTED_EDGE ( 'NONE', *, *, #42048, .F. ) ;
#24763=CARTESIAN_POINT ( 'NONE',  ( -16.21911615440247090, -9.528491918058357157, 34.59228464037090589 ) ) ;
#24764=CARTESIAN_POINT ( 'NONE',  ( 18.06525513951284267, -5.094484230520771817, 34.41647553114626845 ) ) ;
#24765=CARTESIAN_POINT ( 'NONE',  ( 5.933917620639864943, -2.486705287966279432, 31.30864560766542937 ) ) ;
#24767=LINE ( 'NONE', #58992, #30297 ) ;
#24768=DIRECTION ( 'NONE',  ( -0.000000000000000000, -0.9396926207859093161, -0.3420201433256663259 ) ) ;
#24769=CARTESIAN_POINT ( 'NONE',  ( -0.3307466537136761198, -2.541949514083463590, 30.39797389878540557 ) ) ;
#24770=VERTEX_POINT ( 'NONE', #39588 ) ;
#24772=EDGE_CURVE ( 'NONE', #81618, #2005, #59516, .T. ) ;
#24773=CARTESIAN_POINT ( 'NONE',  ( -1.449885830576159940, -10.21337939537584205, 33.94971097300158647 ) ) ;
#24774=ORIENTED_EDGE ( 'NONE', *, *, #75793, .T. ) ;
#24775=CARTESIAN_POINT ( 'NONE',  ( -4.376773112753000738, -8.282780595021769443, 34.94152052738834868 ) ) ;
#24776=ORIENTED_EDGE ( 'NONE', *, *, #24936, .T. ) ;
#24777=CYLINDRICAL_SURFACE ( 'NONE', #16149, 0.2500000000000008882 ) ;
#24778=CARTESIAN_POINT ( 'NONE',  ( -1.514763354347077096, -12.15440758774515473, 32.17923288041532004 ) ) ;
#24779=EDGE_CURVE ( 'NONE', #32972, #41920, #52018, .T. ) ;
#24780=CARTESIAN_POINT ( 'NONE',  ( -12.46153846153846168, -13.78497067705608181, 32.30358669280327177 ) ) ;
#24781=VERTEX_POINT ( 'NONE', #40471 ) ;
#24782=CARTESIAN_POINT ( 'NONE',  ( 11.40777093535123576, -11.93127051446799847, 32.56575433478202797 ) ) ;
#24783=ORIENTED_EDGE ( 'NONE', *, *, #44940, .F. ) ;
#24784=CYLINDRICAL_SURFACE ( 'NONE', #22641, 0.2500000000000009437 ) ;
#24787=CARTESIAN_POINT ( 'NONE',  ( 6.923076923076924238, -2.900454961884010974, 35.62045528018868623 ) ) ;
#24788=CARTESIAN_POINT ( 'NONE',  ( 5.076923076922953193, -5.941354392335915335, 34.76329471203413846 ) ) ;
#24789=ORIENTED_EDGE ( 'NONE', *, *, #47247, .F. ) ;
#24790=CARTESIAN_POINT ( 'NONE',  ( -10.61538461538461320, -11.91647553114624181, 32.58852847137148245 ) ) ;
#24791=CARTESIAN_POINT ( 'NONE',  ( 7.173131342990376247, -8.346898887586323923, 34.93166121998716278 ) ) ;
#24792=DIRECTION ( 'NONE',  ( 0.000000000000000000, 0.000000000000000000, 1.000000000000000000 ) ) ;
#24793=AXIS2_PLACEMENT_3D ( 'NONE', #24109, #37181, #45722 ) ;
#24796=ADVANCED_FACE ( 'NONE', ( #53063 ), #46322, .F. ) ;
#24797=ADVANCED_FACE ( 'NONE', ( #46770 ), #74244, .F. ) ;
#24798=EDGE_LOOP ( 'NONE', ( #25875, #52427 ) ) ;
#24799=EDGE_LOOP ( 'NONE', ( #40968, #73316, #3107, #83917, #77388, #4608, #51931 ) ) ;
#24801=CARTESIAN_POINT ( 'NONE',  ( 3.361559671736181976, -12.62708834333097663, 30.88030960425257021 ) ) ;
#24802=EDGE_LOOP ( 'NONE', ( #59623, #77401, #46016, #81648 ) ) ;
#24806=ORIENTED_EDGE ( 'NONE', *, *, #36402, .T. ) ;
#24807=CARTESIAN_POINT ( 'NONE',  ( -10.86536134632696715, -3.137211980971221781, 32.19342716148376837 ) ) ;
#24810=CARTESIAN_POINT ( 'NONE',  ( -9.562262636387920622, -2.254550872974305342, 29.97347326024527092 ) ) ;
#24811=CARTESIAN_POINT ( 'NONE',  ( 17.07692307692307665, -12.34228464037088635, 31.77849191805839268 ) ) ;
#24812=CARTESIAN_POINT ( 'NONE',  ( -9.915135789942574718, -7.369209533119140509, 34.99857337881830688 ) ) ;
#24813=FACE_BOUND ( 'NONE', #62357, .T. ) ;
#24814=ORIENTED_EDGE ( 'NONE', *, *, #11182, .F. ) ;
#24815=DIRECTION ( 'NONE',  ( -0.000000000000000000, -0.000000000000000000, -1.000000000000000000 ) ) ;
#24816=CARTESIAN_POINT ( 'NONE',  ( 13.44987095589141113, -9.442884908240273489, 34.35708131394835618 ) ) ;
#24818=CARTESIAN_POINT ( 'NONE',  ( 0.4615384615384611200, -13.04860791097971706, 34.73218667398347037 ) ) ;
#24819=DIRECTION ( 'NONE',  ( -0.000000000000000000, -0.7660444431189791237, -0.6427876096865379196 ) ) ;
#24820=EDGE_LOOP ( 'NONE', ( #38485, #41788, #81221, #71106 ) ) ;
#24821=LINE ( 'NONE', #58156, #23056 ) ;
#24822=EDGE_LOOP ( 'NONE', ( #74332, #73632, #47750, #30756 ) ) ;
#24823=ORIENTED_EDGE ( 'NONE', *, *, #49182, .T. ) ;
#24824=CARTESIAN_POINT ( 'NONE',  ( -0.5268089074992374776, -9.442884908240170461, 34.35708131394840592 ) ) ;
#24825=CARTESIAN_POINT ( 'NONE',  ( -9.561517251340744039, -8.191423895709840863, 34.95447573519442130 ) ) ;
#24826=LINE ( 'NONE', #64030, #70090 ) ;
#24829=CARTESIAN_POINT ( 'NONE',  ( -16.15384615384615330, -10.67929555188718282, 33.92786785259544047 ) ) ;
#24830=ORIENTED_EDGE ( 'NONE', *, *, #87105, .F. ) ;
#24831=CARTESIAN_POINT ( 'NONE',  ( -10.61538461538461320, -3.669653830205710676, 35.88435417666054406 ) ) ;
#24832=DIRECTION ( 'NONE',  ( 0.000000000000000000, 0.8660254037844377084, -0.5000000000000015543 ) ) ;
#24833=CARTESIAN_POINT ( 'NONE',  ( 2.438217745925951530, -12.70449254468099198, 30.44128974285582956 ) ) ;
#24834=CARTESIAN_POINT ( 'NONE',  ( 13.25446817517716980, -12.45813303252208648, 30.39737893381572675 ) ) ;
#24835=ORIENTED_EDGE ( 'NONE', *, *, #84389, .T. ) ;
#24836=ORIENTED_EDGE ( 'NONE', *, *, #71737, .T. ) ;
#24837=FACE_BOUND ( 'NONE', #37354, .T. ) ;
#24841=CARTESIAN_POINT ( 'NONE',  ( -17.77479207347706236, -2.251340707108580919, 29.87818027815299615 ) ) ;
#24842=CARTESIAN_POINT ( 'NONE',  ( -1.161602540521989857, -2.308499170217967134, 30.53291367094873721 ) ) ;
#24843=ORIENTED_EDGE ( 'NONE', *, *, #21032, .T. ) ;
#24844=CYLINDRICAL_SURFACE ( 'NONE', #79830, 0.2499999999999994726 ) ;
#24845=DIRECTION ( 'NONE',  ( -0.000000000000000000, -0.9848077530122085754, -0.1736481776669273613 ) ) ;
#24847=CARTESIAN_POINT ( 'NONE',  ( 4.219913487196228274, -6.343179335718452272, 34.87096338111212646 ) ) ;
#24849=CYLINDRICAL_SURFACE ( 'NONE', #18731, 0.2500000000000012212 ) ;
#24850=ORIENTED_EDGE ( 'NONE', *, *, #69818, .F. ) ;
#24851=EDGE_CURVE ( 'NONE', #26530, #43223, #12303, .T. ) ;
#24852=CARTESIAN_POINT ( 'NONE',  ( -7.846153846153965716, -10.21337939537710326, 33.94971097300076224 ) ) ;
#24853=VERTEX_POINT ( 'NONE', #67915 ) ;
#24854=CARTESIAN_POINT ( 'NONE',  ( -8.638438961405983108, -9.804649428959608670, 34.18742332936588468 ) ) ;
#24855=EDGE_CURVE ( 'NONE', #5324, #18937, #9126, .T. ) ;
#24856=CARTESIAN_POINT ( 'NONE',  ( -4.219116599806929102, -2.892918686051582089, 31.69288490824015270 ) ) ;
#24857=DIRECTION ( 'NONE',  ( 0.000000000000000000, 0.1736481776669275834, 0.9848077530122086864 ) ) ;
#24858=CARTESIAN_POINT ( 'NONE',  ( -4.023054346021368133, -12.38066358083363738, 30.83685684665853444 ) ) ;
#24859=CARTESIAN_POINT ( 'NONE',  ( 13.13463864056679853, -4.075325502946081535, 33.72974371597206300 ) ) ;
#24860=CARTESIAN_POINT ( 'NONE',  ( -15.23076923076922995, -12.48256725967547354, 35.29906147534542527 ) ) ;
#24862=ORIENTED_EDGE ( 'NONE', *, *, #45752, .F. ) ;
#24863=CARTESIAN_POINT ( 'NONE',  ( -3.296852641725109834, -3.050289026998445951, 32.03036669348365706 ) ) ;
#24864=B_SPLINE_CURVE_WITH_KNOTS ( 'NONE', 3,
 ( #44908, #79151, #52555, #19233, #24195, #11587, #25092, #74173, #80495, #72825 ),
 .UNSPECIFIED., .F., .F.,
 ( 4, 2, 2, 2, 4 ),
 ( 0.000000000000000000, 0.0001954311564186873352, 0.0003908623128373746704, 0.0005862934692560620598, 0.0007817246256747493408 ),
 .UNSPECIFIED. ) ;
#24865=DIRECTION ( 'NONE',  ( -0.000000000000000000, 0.9396926207859092051, -0.3420201433256662704 ) ) ;
#24866=CARTESIAN_POINT ( 'NONE',  ( -0.2115929431903200153, -5.057305518903948638, 34.11320923018887186 ) ) ;
#24867=EDGE_CURVE ( 'NONE', #66835, #33483, #6221, .T. ) ;
#24868=ORIENTED_EDGE ( 'NONE', *, *, #20485, .F. ) ;
#24869=ORIENTED_EDGE ( 'NONE', *, *, #82547, .F. ) ;
#24870=CARTESIAN_POINT ( 'NONE',  ( 9.757562831820530747, -3.643525952247864463, 33.31231777344670064 ) ) ;
#24872=EDGE_CURVE ( 'NONE', #69245, #3657, #79950, .T. ) ;
#24873=CARTESIAN_POINT ( 'NONE',  ( -0.3314932987036833256, -2.504778602574660340, 29.97347330155780298 ) ) ;
#24874=CARTESIAN_POINT ( 'NONE',  ( 16.02315555073584008, -9.929715669179216775, 34.40415004197138416 ) ) ;
#24875=CARTESIAN_POINT ( 'NONE',  ( 17.74997677577853850, -12.07920672191015221, 32.31858351112116168 ) ) ;
#24877=CYLINDRICAL_SURFACE ( 'NONE', #68125, 0.2499999999999997502 ) ;
#24878=ORIENTED_EDGE ( 'NONE', *, *, #16662, .T. ) ;
#24879=CARTESIAN_POINT ( 'NONE',  ( 9.692307692307695177, -10.51840700105979565, 33.73612834413961536 ) ) ;
#24880=EDGE_CURVE ( 'NONE', #66904, #39806, #11642, .T. ) ;
#24882=CARTESIAN_POINT ( 'NONE',  ( 4.087763774486018242, -8.164416787775445883, 34.95778746994557906 ) ) ;
#24883=ORIENTED_EDGE ( 'NONE', *, *, #79490, .T. ) ;
#24884=CARTESIAN_POINT ( 'NONE',  ( 15.90386940979756858, -12.41104346484419452, 31.60698883733904196 ) ) ;
#24885=B_SPLINE_CURVE_WITH_KNOTS ( 'NONE', 3,
 ( #900, #20729, #21610, #48194, #41447, #14413, #8552, #68911, #55398, #7667 ),
 .UNSPECIFIED., .F., .F.,
 ( 4, 2, 2, 2, 4 ),
 ( 0.0007817359430256322827, 0.0009771253907249989254, 0.001172514838424365676, 0.001367904286123732428, 0.001563293733823098962 ),
 .UNSPECIFIED. ) ;
#24886=ORIENTED_EDGE ( 'NONE', *, *, #67818, .F. ) ;
#24887=CARTESIAN_POINT ( 'NONE',  ( -7.846153846153844924, -2.517432740324522911, 35.29906147534542527 ) ) ;
#24888=CARTESIAN_POINT ( 'NONE',  ( -9.442307692306272315, -7.500000000000154543, 35.00000000000007105 ) ) ;
#24889=CARTESIAN_POINT ( 'NONE',  ( 17.86985203026830504, -10.31621877034669588, 34.18098118002070152 ) ) ;
#24891=CARTESIAN_POINT ( 'NONE',  ( 8.769230769230768274, -12.10708131394839349, 31.69288490824020244 ) ) ;
#24894=CARTESIAN_POINT ( 'NONE',  ( -12.46153846153846168, -3.050289026998446396, 32.03036669348365706 ) ) ;
#24896=EDGE_CURVE ( 'NONE', #66653, #85898, #77860, .T. ) ;
#24897=VERTEX_POINT ( 'NONE', #27370 ) ;
#24898=CARTESIAN_POINT ( 'NONE',  ( -4.153846153846152411, -12.34228464037088635, 31.77849191805839268 ) ) ;
#24900=VERTEX_POINT ( 'NONE', #33242 ) ;
#24901=CARTESIAN_POINT ( 'NONE',  ( 8.546304551714619890, -12.39988816332205701, 30.74660775122750778 ) ) ;
#24903=CARTESIAN_POINT ( 'NONE',  ( 5.010839665967195877, -12.10708131394839349, 31.69288490824020244 ) ) ;
#24905=CARTESIAN_POINT ( 'NONE',  ( -7.596153846152408740, -7.500000000000155431, 34.75000000000007105 ) ) ;
#24906=ADVANCED_FACE ( 'NONE', ( #87769 ), #75123, .F. ) ;
#24908=EDGE_CURVE ( 'NONE', #37386, #21487, #84270, .T. ) ;
#24910=CARTESIAN_POINT ( 'NONE',  ( -10.61538461538473577, -12.51329471203414379, 31.30864560766407578 ) ) ;
#24911=AXIS2_PLACEMENT_3D ( 'NONE', #81199, #52816, #11855 ) ;
#24912=B_SPLINE_CURVE_WITH_KNOTS ( 'NONE', 3,
 ( #30590, #70259, #72021, #10330, #84237, #22514, #2666, #70705, #57186, #37797 ),
 .UNSPECIFIED., .F., .F.,
 ( 4, 2, 2, 2, 4 ),
 ( 0.0007817246256747444619, 0.0009771112852218868158, 0.001172497944769029061, 0.001367884604316171523, 0.001563271263863313769 ),
 .UNSPECIFIED. ) ;
#24914=ORIENTED_EDGE ( 'NONE', *, *, #88415, .T. ) ;
#24915=EDGE_LOOP ( 'NONE', ( #86979, #74573, #80577, #24869 ) ) ;
#24916=B_SPLINE_CURVE_WITH_KNOTS ( 'NONE', 3,
 ( #73948, #18555, #12683, #33403, #18997, #5928, #73504, #87934, #38830, #4591 ),
 .UNSPECIFIED., .F., .F.,
 ( 4, 2, 2, 2, 4 ),
 ( 0.000000000000000000, 0.0001954311564186861968, 0.0003908623128373723936, 0.0005862934692560585904, 0.0007817246256747447872 ),
 .UNSPECIFIED. ) ;
#24917=ORIENTED_EDGE ( 'NONE', *, *, #80070, .T. ) ;
#24918=EDGE_LOOP ( 'NONE', ( #56585, #86428 ) ) ;
#24919=CARTESIAN_POINT ( 'NONE',  ( -14.30769230769230660, -2.499999999999998668, 29.50000000000001066 ) ) ;
#24920=DIRECTION ( 'NONE',  ( -0.000000000000000000, -0.8660254037844399289, -0.4999999999999980016 ) ) ;
#24922=CARTESIAN_POINT ( 'NONE',  ( -5.776988648387149539, -4.887748414852792322, 34.01359900205216746 ) ) ;
#24924=LINE ( 'NONE', #31237, #19764 ) ;
#24925=DIRECTION ( 'NONE',  ( -0.000000000000000000, 0.5000000000000011102, -0.8660254037844381525 ) ) ;
#24926=CARTESIAN_POINT ( 'NONE',  ( -17.86947429823644029, -6.852161475712352789, 34.70806712695775786 ) ) ;
#24927=DIRECTION ( 'NONE',  ( -0.000000000000000000, -0.6427876096865404731, -0.7660444431189771253 ) ) ;
#24928=ORIENTED_EDGE ( 'NONE', *, *, #70642, .T. ) ;
#24929=ORIENTED_EDGE ( 'NONE', *, *, #40150, .T. ) ;
#24930=ORIENTED_EDGE ( 'NONE', *, *, #10004, .F. ) ;
#24931=CARTESIAN_POINT ( 'NONE',  ( 0.4615384615383382183, -3.083524468854526912, 32.58852847137268327 ) ) ;
#24932=VERTEX_POINT ( 'NONE', #67475 ) ;
#24933=CARTESIAN_POINT ( 'NONE',  ( 7.715462379486287325, -3.062553014421049546, 32.05460306192773601 ) ) ;
#24934=CARTESIAN_POINT ( 'NONE',  ( -16.15384615384615330, -9.780366693483667717, 34.19971097300155094 ) ) ;
#24935=VECTOR ( 'NONE', #31338, 1000.000000000000000 ) ;
#24936=EDGE_CURVE ( 'NONE', #52162, #45, #43413, .T. ) ;
#24937=CARTESIAN_POINT ( 'NONE',  ( 1.607395053593452028, -4.989023458446560255, 34.36081565061822118 ) ) ;
#24938=CARTESIAN_POINT ( 'NONE',  ( 7.173131234715237170, -2.564540009722896752, 30.55348353981670684 ) ) ;
#24939=FACE_BOUND ( 'NONE', #39343, .T. ) ;
#24940=ORIENTED_EDGE ( 'NONE', *, *, #74221, .F. ) ;
#24942=CARTESIAN_POINT ( 'NONE',  ( -2.057692307692306599, -2.499999999999998668, 29.75000000000000355 ) ) ;
#24944=FACE_BOUND ( 'NONE', #37756, .T. ) ;
#24945=B_SPLINE_CURVE_WITH_KNOTS ( 'NONE', 3,
 ( #17424, #3005, #43557, #86349, #57071, #36802, #84565, #22840, #50303, #16975 ),
 .UNSPECIFIED., .F., .F.,
 ( 4, 2, 2, 2, 4 ),
 ( 0.000000000000000000, 0.0001954339857564074473, 0.0003908679715128148945, 0.0005863019572692223418, 0.0007817359430256297891 ),
 .UNSPECIFIED. ) ;
#24946=CARTESIAN_POINT ( 'NONE',  ( -10.68065461594093435, -3.083524468853724443, 32.58852847137143272 ) ) ;
#24949=CARTESIAN_POINT ( 'NONE',  ( 17.86985279056178300, -2.882441371585227508, 31.66841991370172238 ) ) ;
#24951=DIRECTION ( 'NONE',  ( 0.000000000000000000, 0.1736481776669275834, 0.9848077530122086864 ) ) ;
#24952=ORIENTED_EDGE ( 'NONE', *, *, #72945, .T. ) ;
#24953=CARTESIAN_POINT ( 'NONE',  ( -11.53846153846153655, -4.661471528628507777, 34.16647553114623292 ) ) ;
#24954=CARTESIAN_POINT ( 'NONE',  ( -14.53117725141625627, -5.912607949931405926, 34.49155766932282319 ) ) ;
#24956=EDGE_CURVE ( 'NONE', #8429, #40093, #82764, .T. ) ;
#24957=CARTESIAN_POINT ( 'NONE',  ( -2.557669038634660108, -11.28823185664190376, 33.01397839955799896 ) ) ;
#24958=CYLINDRICAL_SURFACE ( 'NONE', #81561, 0.2500000000000009437 ) ;
#24959=ORIENTED_EDGE ( 'NONE', *, *, #3407, .F. ) ;
#24960=CARTESIAN_POINT ( 'NONE',  ( 18.06525557127601900, -6.879047030191284051, 34.71129190930002295 ) ) ;
#24961=FACE_OUTER_BOUND ( 'NONE', #84643, .T. ) ;
#24962=CARTESIAN_POINT ( 'NONE',  ( 12.46153846153846168, -13.49023893513002648, 31.06009739812518688 ) ) ;
#24963=B_SPLINE_CURVE_WITH_KNOTS ( 'NONE', 3,
 ( #82016, #18977, #20311, #26175, #41025, #39706, #75254, #13545, #41464, #60395 ),
 .UNSPECIFIED., .F., .F.,
 ( 4, 2, 2, 2, 4 ),
 ( 0.0007817359430256317406, 0.0009771253907249982749, 0.001172514838424365026, 0.001367904286123731560, 0.001563293733823098094 ),
 .UNSPECIFIED. ) ;
#24964=DIRECTION ( 'NONE',  ( -0.000000000000000000, -0.3420201433256694346, -0.9396926207859080948 ) ) ;
#24965=CARTESIAN_POINT ( 'NONE',  ( -15.90379184220783948, -4.235687564193445276, 33.53795663066793509 ) ) ;
#24966=LINE ( 'NONE', #87587, #43810 ) ;
#24967=CARTESIAN_POINT ( 'NONE',  ( 5.076923076922954969, -12.46129190930018460, 30.37095296980731973 ) ) ;
#24968=VECTOR ( 'NONE', #26812, 1000.000000000000114 ) ;
#24969=CARTESIAN_POINT ( 'NONE',  ( -15.48074596171158390, -12.41269422305637171, 30.68257228309993323 ) ) ;
#24971=CARTESIAN_POINT ( 'NONE',  ( 6.923076923076924238, -13.53365097954675988, 30.81389545987213552 ) ) ;
#24972=DIRECTION ( 'NONE',  ( -0.000000000000000000, -0.8660254037844397068, -0.4999999999999978906 ) ) ;
#24974=ORIENTED_EDGE ( 'NONE', *, *, #61769, .F. ) ;
#24975=VECTOR ( 'NONE', #82846, 1000.000000000000227 ) ;
#24976=DIRECTION ( 'NONE',  ( 0.000000000000000000, 0.3420201433256641055, -0.9396926207859100932 ) ) ;
#24977=ORIENTED_EDGE ( 'NONE', *, *, #43709, .F. ) ;
#24978=EDGE_CURVE ( 'NONE', #69004, #88055, #28420, .T. ) ;
#24979=ORIENTED_EDGE ( 'NONE', *, *, #73193, .F. ) ;
#24980=CARTESIAN_POINT ( 'NONE',  ( -2.307692307692305711, -12.37446782046654192, 30.86335684631486131 ) ) ;
#24981=EDGE_LOOP ( 'NONE', ( #5017, #10222 ) ) ;
#24982=CARTESIAN_POINT ( 'NONE',  ( -15.00798968950081758, -5.913360116392397892, 34.49180327182771322 ) ) ;
#24984=B_SPLINE_CURVE_WITH_KNOTS ( 'NONE', 3,
 ( #26774, #46166, #39855, #5616, #4736, #11941, #88068, #6510, #13261, #24993 ),
 .UNSPECIFIED., .F., .F.,
 ( 4, 2, 2, 2, 4 ),
 ( 0.000000000000000000, 0.0001954311564186875792, 0.0003908623128373751583, 0.0005862934692560627103, 0.0007817246256747503166 ),
 .UNSPECIFIED. ) ;
#24986=CARTESIAN_POINT ( 'NONE',  ( 10.68063975489745410, -2.657715359629132301, 31.77849191805844242 ) ) ;
#24987=DIRECTION ( 'NONE',  ( -0.000000000000000000, -0.000000000000000000, -1.000000000000000000 ) ) ;
#24988=CARTESIAN_POINT ( 'NONE',  ( -12.21159305216042057, -4.176053281294518804, 33.81426240980091791 ) ) ;
#24990=DIRECTION ( 'NONE',  ( -0.000000000000000000, 0.6427876096865404731, -0.7660444431189770143 ) ) ;
#24993=CARTESIAN_POINT ( 'NONE',  ( -6.923076923077045919, -5.094484230521993062, 34.41647553114689373 ) ) ;
#24994=CARTESIAN_POINT ( 'NONE',  ( -17.93393266664992680, -2.292212530054420050, 30.41441678777543345 ) ) ;
#24995=EDGE_CURVE ( 'NONE', #42300, #14097, #41775, .T. ) ;
#24996=DIRECTION ( 'NONE',  ( -0.000000000000000000, -0.9396926207859092051, -0.3420201433256662704 ) ) ;
#24997=EDGE_CURVE ( 'NONE', #55965, #46285, #83134, .T. ) ;
#24999=ORIENTED_EDGE ( 'NONE', *, *, #10720, .T. ) ;
#25000=CARTESIAN_POINT ( 'NONE',  ( -11.53846153846153655, -5.557115091759785130, 34.35708131394839171 ) ) ;
#25001=DIRECTION ( 'NONE',  ( 0.000000000000000000, 0.3420201433256641055, -0.9396926207859100932 ) ) ;
#25002=CARTESIAN_POINT ( 'NONE',  ( 1.134638640566795642, -10.82459398097509684, 33.81372124010185587 ) ) ;
#25003=CARTESIAN_POINT ( 'NONE',  ( -15.93083480223330817, -12.39991518177334129, 30.74647679643404530 ) ) ;
#25004=EDGE_CURVE ( 'NONE', #35065, #65093, #70570, .T. ) ;
#25005=CARTESIAN_POINT ( 'NONE',  ( 17.07692307692295586, -12.51329471203414379, 31.30864560766407578 ) ) ;
#25006=CARTESIAN_POINT ( 'NONE',  ( -4.853910232829679039, -2.889357225399416862, 32.26129605718031002 ) ) ;
#25008=EDGE_CURVE ( 'NONE', #23467, #50664, #11180, .T. ) ;
#25009=EDGE_LOOP ( 'NONE', ( #67616, #43959 ) ) ;
#25010=CARTESIAN_POINT ( 'NONE',  ( 17.75002326905764605, -12.41269422305637171, 30.68257228309993323 ) ) ;
#25013=B_SPLINE_CURVE_WITH_KNOTS ( 'NONE', 3,
 ( #2492, #50677, #85373, #79506, #45260, #84937, #23658, #17807, #71846, #78162 ),
 .UNSPECIFIED., .F., .F.,
 ( 4, 2, 2, 2, 4 ),
 ( 0.0007817359430256392216, 0.0009771253907250080327, 0.001172514838424376952, 0.001367904286123745872, 0.001563293733823114791 ),
 .UNSPECIFIED. ) ;
#25014=ORIENTED_EDGE ( 'NONE', *, *, #42156, .F. ) ;
#25015=CARTESIAN_POINT ( 'NONE',  ( -5.777220458731590291, -5.913360116392398780, 34.49180327182771322 ) ) ;
#25017=CARTESIAN_POINT ( 'NONE',  ( -14.08467946359890988, -2.889357225399414197, 32.26129605718031002 ) ) ;
#25019=LINE ( 'NONE', #25912, #24935 ) ;
#25021=ORIENTED_EDGE ( 'NONE', *, *, #21337, .T. ) ;
#25022=ORIENTED_EDGE ( 'NONE', *, *, #44481, .T. ) ;
#25023=VERTEX_POINT ( 'NONE', #13846 ) ;
#25024=AXIS2_PLACEMENT_3D ( 'NONE', #39895, #17386, #4772 ) ;
#25025=CARTESIAN_POINT ( 'NONE',  ( -7.053767526187231240, -11.93127051446800024, 32.56575433478200665 ) ) ;
#25026=CARTESIAN_POINT ( 'NONE',  ( 9.915087361285756629, -2.353885683473779800, 30.79025554430704403 ) ) ;
#25028=CARTESIAN_POINT ( 'NONE',  ( 0.4615384615384611200, -12.29105614889573062, 35.45975837776705220 ) ) ;
#25029=B_SPLINE_CURVE_WITH_KNOTS ( 'NONE', 3,
 ( #57098, #23309, #21992, #3030, #1267, #9801 ),
 .UNSPECIFIED., .F., .F.,
 ( 4, 2, 4 ),
 ( 0.000000000000000000, 0.0001954784845028913534, 0.0003909569690057827069 ),
 .UNSPECIFIED. ) ;
#25031=AXIS2_PLACEMENT_3D ( 'NONE', #8445, #2993, #37675 ) ;
#25032=CARTESIAN_POINT ( 'NONE',  ( 1.384615384615386802, -3.513871655860378418, 32.76840700105978499 ) ) ;
#25033=EDGE_CURVE ( 'NONE', #10616, #54130, #27808, .T. ) ;
#25035=LINE ( 'NONE', #44848, #22142 ) ;
#25036=ORIENTED_EDGE ( 'NONE', *, *, #26654, .F. ) ;
#25040=CARTESIAN_POINT ( 'NONE',  ( 15.29602480204525605, -6.026961402152789304, 34.52809138561124769 ) ) ;
#25041=ORIENTED_EDGE ( 'NONE', *, *, #48193, .F. ) ;
#25042=CARTESIAN_POINT ( 'NONE',  ( 7.846153846153725020, -12.46129190930018460, 30.37095296980731973 ) ) ;
#25043=CARTESIAN_POINT ( 'NONE',  ( 12.52679360105129547, -8.656820664281605460, 34.87096338111211224 ) ) ;
#25044=EDGE_CURVE ( 'NONE', #27257, #1913, #32142, .T. ) ;
#25047=B_SPLINE_CURVE_WITH_KNOTS ( 'NONE', 3,
 ( #15992, #16871, #77239, #29508, #9241, #3353, #36701, #74054, #12345, #66843 ),
 .UNSPECIFIED., .F., .F.,
 ( 4, 2, 2, 2, 4 ),
 ( 0.000000000000000000, 0.0001954311564186865763, 0.0003908623128373731525, 0.0005862934692560596746, 0.0007817246256747463051 ),
 .UNSPECIFIED. ) ;
#25048=CARTESIAN_POINT ( 'NONE',  ( -13.38461538461550582, -12.27809138561165270, 31.22303859784587132 ) ) ;
#25049=ORIENTED_EDGE ( 'NONE', *, *, #25303, .T. ) ;
#25050=EDGE_CURVE ( 'NONE', #3308, #23412, #45646, .T. ) ;
#25052=CARTESIAN_POINT ( 'NONE',  ( 0.2386115026316120158, -11.43668979543635267, 33.22377378376090462 ) ) ;
#25053=CARTESIAN_POINT ( 'NONE',  ( 0.2115384615384616196, -2.499999999999998668, 29.75000000000000355 ) ) ;
#25055=CARTESIAN_POINT ( 'NONE',  ( 8.769230769230768274, -13.57706302396349152, 30.56769352161908060 ) ) ;
#25057=CARTESIAN_POINT ( 'NONE',  ( -3.007989689500821573, -6.760870238392817200, 34.69528174975672385 ) ) ;
#25058=CARTESIAN_POINT ( 'NONE',  ( -9.692307692307691624, -13.87047571288749737, 32.06866353760679544 ) ) ;
#25059=ORIENTED_EDGE ( 'NONE', *, *, #7924, .F. ) ;
#25060=CARTESIAN_POINT ( 'NONE',  ( 6.673100192134569397, -8.303909089506435137, 34.68538101551103381 ) ) ;
#25061=CARTESIAN_POINT ( 'NONE',  ( -11.28846153846010303, -7.500000000000155431, 34.75000000000007105 ) ) ;
#25062=DIRECTION ( 'NONE',  ( -0.000000000000000000, 1.000000000000000000, 3.491481338843133355E-15 ) ) ;
#25063=ORIENTED_EDGE ( 'NONE', *, *, #42900, .T. ) ;
#25065=VECTOR ( 'NONE', #83573, 1000.000000000000114 ) ;
#25068=CARTESIAN_POINT ( 'NONE',  ( -10.61538461538461320, -10.51840700105979565, 33.73612834413961536 ) ) ;
#25069=CARTESIAN_POINT ( 'NONE',  ( 10.48469314871705826, -11.71456829005830080, 32.44064028649416542 ) ) ;
#25070=FACE_BOUND ( 'NONE', #55261, .T. ) ;
#25071=CARTESIAN_POINT ( 'NONE',  ( 5.299935921016469820, -5.582272713120727481, 34.63742843783360570 ) ) ;
#25072=CARTESIAN_POINT ( 'NONE',  ( -16.15384615384615330, -13.88283147151868846, 33.14645433367849847 ) ) ;
#25073=CARTESIAN_POINT ( 'NONE',  ( 9.942307692307695177, -2.499999999999998668, 29.75000000000000355 ) ) ;
#25074=CARTESIAN_POINT ( 'NONE',  ( -1.319359813339359144, -12.27809138561124591, 31.22303859784720359 ) ) ;
#25075=DIRECTION ( 'NONE',  ( 0.000000000000000000, 0.6427876096865368094, 0.7660444431189802339 ) ) ;
#25076=CARTESIAN_POINT ( 'NONE',  ( -3.903791733932700847, -10.82426656108011720, 33.81400080652039009 ) ) ;
#25077=CARTESIAN_POINT ( 'NONE',  ( 6.249945409378045547, -4.932303261841489039, 34.32971442181322885 ) ) ;
#25079=FACE_OUTER_BOUND ( 'NONE', #9601, .T. ) ;
#25080=EDGE_LOOP ( 'NONE', ( #56467, #43330, #38851, #86512 ) ) ;
#25081=DIRECTION ( 'NONE',  ( -0.000000000000000000, -0.9396926207859093161, -0.3420201433256663259 ) ) ;
#25082=CARTESIAN_POINT ( 'NONE',  ( 8.069166690247241647, -10.01129605718032600, 34.36064277460058491 ) ) ;
#25085=CARTESIAN_POINT ( 'NONE',  ( -16.85414340794500276, -2.353885683473779356, 30.79025554430704759 ) ) ;
#25086=CARTESIAN_POINT ( 'NONE',  ( -12.52680846209478460, -6.835583212224499938, 34.95778746994557906 ) ) ;
#25088=EDGE_CURVE ( 'NONE', #24897, #14333, #37014, .T. ) ;
#25089=DIRECTION ( 'NONE',  ( -0.000000000000000000, -0.1736481776669307198, -0.9848077530122080203 ) ) ;
#25090=CARTESIAN_POINT ( 'NONE',  ( -14.43838291080261449, -11.37499894934982692, 33.29245874905763003 ) ) ;
#25091=CARTESIAN_POINT ( 'NONE',  ( 7.976945653978634532, -11.71459661697925903, 32.44059661609676937 ) ) ;
#25092=CARTESIAN_POINT ( 'NONE',  ( -0.6850233861027921201, -8.539481045369598178, 34.89627647299170832 ) ) ;
#25093=LINE ( 'NONE', #32736, #77084 ) ;
#25094=CARTESIAN_POINT ( 'NONE',  ( -9.019254006523732770, -9.271318131107980420, 34.42618302367067429 ) ) ;
#25095=B_SPLINE_CURVE_WITH_KNOTS ( 'NONE', 3,
 ( #57533, #44899, #58866, #2580, #65172, #85021, #78699, #85456, #17890, #11125 ),
 .UNSPECIFIED., .F., .F.,
 ( 4, 2, 2, 2, 4 ),
 ( 0.000000000000000000, 0.0001954311564186869015, 0.0003908623128373738030, 0.0005862934692560607588, 0.0007817246256747476061 ),
 .UNSPECIFIED. ) ;
#25096=CYLINDRICAL_SURFACE ( 'NONE', #73614, 0.2499999999999994726 ) ;
#25097=CARTESIAN_POINT ( 'NONE',  ( 17.32686848630112308, -8.476813868363244353, 34.90874843262270133 ) ) ;
#25098=ORIENTED_EDGE ( 'NONE', *, *, #64097, .F. ) ;
#25099=CARTESIAN_POINT ( 'NONE',  ( 6.988221703796556383, -7.750023224968867197, 34.99404313364389907 ) ) ;
#25100=CARTESIAN_POINT ( 'NONE',  ( -4.153846153846152411, -2.249999999999998668, 29.75000000000001776 ) ) ;
#25103=VECTOR ( 'NONE', #48341, 1000.000000000000000 ) ;
#25104=CARTESIAN_POINT ( 'NONE',  ( 6.223011351612852238, -4.187068189119697692, 33.49521262558774026 ) ) ;
#25106=EDGE_LOOP ( 'NONE', ( #45111, #33147 ) ) ;
#25107=CARTESIAN_POINT ( 'NONE',  ( 1.607394925883795622, -4.387253974876678342, 33.66317474335728832 ) ) ;
#25108=CARTESIAN_POINT ( 'NONE',  ( -12.46153846153846168, -12.62096338111211580, 30.90682066428153263 ) ) ;
#25109=CARTESIAN_POINT ( 'NONE',  ( 11.28848479441294650, -2.920706130388546651, 32.31842814019191223 ) ) ;
#25110=ORIENTED_EDGE ( 'NONE', *, *, #87812, .F. ) ;
#25111=CARTESIAN_POINT ( 'NONE',  ( 11.66898697669518192, -5.070358843744210198, 34.40418822224088302 ) ) ;
#25112=CYLINDRICAL_SURFACE ( 'NONE', #84349, 0.2499999999999986955 ) ;
#25113=FACE_OUTER_BOUND ( 'NONE', #84259, .T. ) ;
#25115=EDGE_LOOP ( 'NONE', ( #79780, #56104, #21752, #77479 ) ) ;
#25116=CARTESIAN_POINT ( 'NONE',  ( 2.557746619330623528, -12.17597550085003455, 31.52189283813461884 ) ) ;
#25117=CARTESIAN_POINT ( 'NONE',  ( 1.384615384615386802, -13.78497067705608181, 32.30358669280327177 ) ) ;
#25118=EDGE_CURVE ( 'NONE', #17226, #83191, #71310, .T. ) ;
#25119=CARTESIAN_POINT ( 'NONE',  ( 15.00728430620490350, -10.23692288466677880, 34.23039457007281072 ) ) ;
#25120=ORIENTED_EDGE ( 'NONE', *, *, #64050, .T. ) ;
#25121=ORIENTED_EDGE ( 'NONE', *, *, #22807, .T. ) ;
#25122=EDGE_CURVE ( 'NONE', #5856, #30896, #60492, .T. ) ;
#25124=CARTESIAN_POINT ( 'NONE',  ( 12.71148387091650278, -10.18230066228895758, 34.26354781536631577 ) ) ;
#25125=CARTESIAN_POINT ( 'NONE',  ( -8.546451227962359454, -3.236590943229499029, 32.36255958852954251 ) ) ;
#25126=EDGE_CURVE ( 'NONE', #11427, #42436, #4214, .T. ) ;
#25127=DIRECTION ( 'NONE',  ( -0.000000000000000000, 0.9396926207859092051, -0.3420201433256662704 ) ) ;
#25128=VECTOR ( 'NONE', #86367, 1000.000000000000227 ) ;
#25129=ADVANCED_FACE ( 'NONE', ( #60043 ), #87549, .F. ) ;
#25130=CARTESIAN_POINT ( 'NONE',  ( -10.55012904410859065, -3.300289026998473041, 32.46337939537591666 ) ) ;
#25131=B_SPLINE_CURVE_WITH_KNOTS ( 'NONE', 3,
 ( #73062, #25766, #80729, #86140, #53677, #19009, #17679, #32512, #66748, #52334 ),
 .UNSPECIFIED., .F., .F.,
 ( 4, 2, 2, 2, 4 ),
 ( 0.000000000000000000, 0.0001954311584214085934, 0.0003908623168428171867, 0.0005862934752642231509, 0.0007817246336856291692 ),
 .UNSPECIFIED. ) ;
#25132=ORIENTED_EDGE ( 'NONE', *, *, #27337, .F. ) ;
#25133=VERTEX_POINT ( 'NONE', #67256 ) ;
#25135=ORIENTED_EDGE ( 'NONE', *, *, #87534, .T. ) ;
#25138=DIRECTION ( 'NONE',  ( -0.000000000000000000, 0.5000000000000011102, -0.8660254037844381525 ) ) ;
#25139=CARTESIAN_POINT ( 'NONE',  ( 10.36538461538461675, -2.249999999999998668, 29.75000000000000355 ) ) ;
#25140=CARTESIAN_POINT ( 'NONE',  ( -13.38461538461550582, -12.46129190930018460, 30.37095296980731973 ) ) ;
#25141=ORIENTED_EDGE ( 'NONE', *, *, #73207, .F. ) ;
#25143=VERTEX_POINT ( 'NONE', #24477 ) ;
#25145=ORIENTED_EDGE ( 'NONE', *, *, #69846, .F. ) ;
#25146=CARTESIAN_POINT ( 'NONE',  ( -10.83825087844771495, -2.251424796025575326, 29.88072029997477941 ) ) ;
#25147=VECTOR ( 'NONE', #14539, 1000.000000000000000 ) ;
#25148=DIRECTION ( 'NONE',  ( 0.000000000000000000, 0.6427876096865368094, 0.7660444431189802339 ) ) ;
#25149=VERTEX_POINT ( 'NONE', #38905 ) ;
#25150=CARTESIAN_POINT ( 'NONE',  ( -8.992156986746913105, -10.61292498521070549, 33.66303323003028680 ) ) ;
#25151=CARTESIAN_POINT ( 'NONE',  ( -13.63461538461538325, -2.499999999999998668, 29.75000000000000355 ) ) ;
#25152=CARTESIAN_POINT ( 'NONE',  ( -5.749945580086545327, -3.435999193479609914, 33.07426656108010832 ) ) ;
#25153=FACE_BOUND ( 'NONE', #88586, .T. ) ;
#25156=FACE_OUTER_BOUND ( 'NONE', #35988, .T. ) ;
#25157=VECTOR ( 'NONE', #83261, 1000.000000000000114 ) ;
#25158=CARTESIAN_POINT ( 'NONE',  ( -10.55012947587177408, -11.06231777344671130, 33.60647404775212976 ) ) ;
#25159=CARTESIAN_POINT ( 'NONE',  ( 17.14211705870643243, -2.506253911140448043, 29.99999999999988631 ) ) ;
#25161=DIRECTION ( 'NONE',  ( 1.000000000000000000, 0.000000000000000000, 0.000000000000000000 ) ) ;
#25164=CARTESIAN_POINT ( 'NONE',  ( -16.02300773583338867, -7.277220443632451463, 34.74524770363009196 ) ) ;
#25165=AXIS2_PLACEMENT_3D ( 'NONE', #61240, #88753, #41432 ) ;
#25166=DIRECTION ( 'NONE',  ( -0.000000000000000000, 0.3420201433256694901, -0.9396926207859082059 ) ) ;
#25167=ORIENTED_EDGE ( 'NONE', *, *, #20165, .T. ) ;
#25168=VERTEX_POINT ( 'NONE', #10535 ) ;
#25169=CARTESIAN_POINT ( 'NONE',  ( -11.78843828251013015, -12.65889640711025521, 30.72598325615533454 ) ) ;
#25170=CARTESIAN_POINT ( 'NONE',  ( -17.07692307692307665, -11.16473453929635440, 33.15142922261926373 ) ) ;
#25171=EDGE_CURVE ( 'NONE', #65576, #23097, #14376, .T. ) ;
#25172=CARTESIAN_POINT ( 'NONE',  ( -13.44993939741969413, -7.749976730030849303, 34.74374725381503737 ) ) ;
#25173=CARTESIAN_POINT ( 'NONE',  ( -15.23076923076922995, -2.538708090699994813, 30.37095296980875503 ) ) ;
#25175=VERTEX_POINT ( 'NONE', #13199 ) ;
#25176=CARTESIAN_POINT ( 'NONE',  ( 14.37294787896833270, -9.442884908240273489, 34.35708131394835618 ) ) ;
#25177=CARTESIAN_POINT ( 'NONE',  ( 18.06606733335007675, -2.486705287966280320, 31.30864560766543647 ) ) ;
#25179=DIRECTION ( 'NONE',  ( -0.000000000000000000, -0.9848077530122086864, -0.1736481776669273613 ) ) ;
#25180=CARTESIAN_POINT ( 'NONE',  ( 5.749976775778542937, -6.652501968072646932, 34.93155406624980941 ) ) ;
#25181=FACE_OUTER_BOUND ( 'NONE', #21449, .T. ) ;
#25182=DIRECTION ( 'NONE',  ( 0.000000000000000000, 0.000000000000000000, 1.000000000000000000 ) ) ;
#25183=SURFACE_STYLE_USAGE ( .BOTH. , #24279 ) ;
#25184=CARTESIAN_POINT ( 'NONE',  ( -16.85414340794500276, -2.612705202774696200, 31.66806509827799943 ) ) ;
#25185=B_SPLINE_CURVE_WITH_KNOTS ( 'NONE', 3,
 ( #14016, #34733, #27976, #55444, #82929, #14916, #9471, #70738, #57219, #76154 ),
 .UNSPECIFIED., .F., .F.,
 ( 4, 2, 2, 2, 4 ),
 ( 0.0007817246336856284103, 0.0009771112958940092897, 0.001172497958102390169, 0.001367884620310771265, 0.001563271282519152145 ),
 .UNSPECIFIED. ) ;
#25188=EDGE_LOOP ( 'NONE', ( #58026, #5841, #81680, #65762 ) ) ;
#25189=CARTESIAN_POINT ( 'NONE',  ( -14.53117723225663838, -4.988325925672468131, 34.36044203135681130 ) ) ;
#25190=LINE ( 'NONE', #18441, #35487 ) ;
#25191=CARTESIAN_POINT ( 'NONE',  ( 10.86533013373275836, -2.587454068350148351, 30.68340429815432202 ) ) ;
#25192=CARTESIAN_POINT ( 'NONE',  ( 2.307692307692309264, -3.513871655860378418, 32.76840700105978499 ) ) ;
#25193=DIRECTION ( 'NONE',  ( 0.000000000000000000, 0.3420201433256610524, 0.9396926207859113145 ) ) ;
#25195=ADVANCED_FACE ( 'NONE', ( #20398 ), #12748, .F. ) ;
#25196=CARTESIAN_POINT ( 'NONE',  ( -7.846153846153844924, -8.120952969808772792, 34.71129190930000163 ) ) ;
#25197=CARTESIAN_POINT ( 'NONE',  ( 14.30769230769218581, -6.835583212225970762, 34.95778746994575670 ) ) ;
#25199=CARTESIAN_POINT ( 'NONE',  ( 17.07692307692307665, -12.10708131394839349, 31.69288490824020244 ) ) ;
#25200=CARTESIAN_POINT ( 'NONE',  ( 13.16113046005105680, -10.23692288466677880, 34.23039457007281072 ) ) ;
#25201=CARTESIAN_POINT ( 'NONE',  ( -10.61538461538461320, -8.164416787775445883, 34.95778746994557906 ) ) ;
#25202=CARTESIAN_POINT ( 'NONE',  ( 13.38461538461526423, -2.657715359629662544, 31.77849191805970364 ) ) ;
#25203=EDGE_CURVE ( 'NONE', #47389, #28787, #513, .T. ) ;
#25204=EDGE_CURVE ( 'NONE', #36240, #74452, #32718, .T. ) ;
#25205=CARTESIAN_POINT ( 'NONE',  ( -12.59168643127016196, -8.630895178749533159, 34.87696386517710323 ) ) ;
#25206=CARTESIAN_POINT ( 'NONE',  ( 3.903869422903798458, -12.41269422305637171, 30.68257228309993323 ) ) ;
#25207=CARTESIAN_POINT ( 'NONE',  ( 10.74617642320939837, -2.729792928343269587, 31.24908615093345077 ) ) ;
#25209=CARTESIAN_POINT ( 'NONE',  ( -15.23076923076922995, -9.780366693483667717, 34.19971097300155094 ) ) ;
#25210=EDGE_LOOP ( 'NONE', ( #49992, #76417 ) ) ;
#25211=EDGE_CURVE ( 'NONE', #72338, #14030, #21868, .T. ) ;
#25212=DIRECTION ( 'NONE',  ( -0.000000000000000000, -0.6427876096865404731, -0.7660444431189771253 ) ) ;
#25213=CYLINDRICAL_SURFACE ( 'NONE', #43187, 2.000000000000001776 ) ;
#25216=CARTESIAN_POINT ( 'NONE',  ( -14.30769230769230660, -5.471508081941601098, 34.59228464037088457 ) ) ;
#25217=CARTESIAN_POINT ( 'NONE',  ( 16.02369818411445479, -5.070767119584671079, 34.40440758774516183 ) ) ;
#25218=LINE ( 'NONE', #59887, #85700 ) ;
#25219=EDGE_LOOP ( 'NONE', ( #26134, #76689 ) ) ;
#25222=EDGE_LOOP ( 'NONE', ( #58087, #33371 ) ) ;
#25223=CARTESIAN_POINT ( 'NONE',  ( 18.06606835100243913, -8.973038597847269315, 34.52809138561122637 ) ) ;
#25225=B_SPLINE_CURVE_WITH_KNOTS ( 'NONE', 3,
 ( #85365, #16016, #70958, #2926, #84929, #77267, #50222, #78595, #71837, #78155 ),
 .UNSPECIFIED., .F., .F.,
 ( 4, 2, 2, 2, 4 ),
 ( 0.0007817246256747460882, 0.0009771112852218892010, 0.001172497944769032314, 0.001367884604316175210, 0.001563271263863318323 ),
 .UNSPECIFIED. ) ;
#25226=CARTESIAN_POINT ( 'NONE',  ( -18.00000000000012079, -11.94971097300221352, 32.03036669348236387 ) ) ;
#25227=B_SPLINE_CURVE_WITH_KNOTS ( 'NONE', 3,
 ( #69566, #83987, #43431, #70462, #62355, #7434, #83543, #8319, #49735, #77208 ),
 .UNSPECIFIED., .F., .F.,
 ( 4, 2, 2, 2, 4 ),
 ( 0.0007817359430256308733, 0.0009771253907249971907, 0.001172514838424363725, 0.001367904286123730259, 0.001563293733823096577 ),
 .UNSPECIFIED. ) ;
#25228=CARTESIAN_POINT ( 'NONE',  ( -15.48076923076922995, -7.500000000000001776, 35.04278698407183867 ) ) ;
#25229=AXIS2_PLACEMENT_3D ( 'NONE', #81918, #34155, #40050 ) ;
#25230=LINE ( 'NONE', #4514, #59892 ) ;
#25231=VERTEX_POINT ( 'NONE', #81661 ) ;
#25232=CARTESIAN_POINT ( 'NONE',  ( 0.3954560821783248969, -4.661471528628507777, 34.16647553114621871 ) ) ;
#25233=EDGE_LOOP ( 'NONE', ( #21747, #21676 ) ) ;
#25235=EDGE_CURVE ( 'NONE', #25963, #87033, #15332, .T. ) ;
#25236=ORIENTED_EDGE ( 'NONE', *, *, #53715, .F. ) ;
#25237=CARTESIAN_POINT ( 'NONE',  ( -6.923076923076922462, -11.33034616979429110, 35.88435417666054406 ) ) ;
#25238=CARTESIAN_POINT ( 'NONE',  ( 0.6845498131513102491, -11.24521262558773671, 33.06293181088029343 ) ) ;
#25240=LINE ( 'NONE', #25684, #33247 ) ;
#25241=DIRECTION ( 'NONE',  ( -0.000000000000000000, 0.6427876096865404731, -0.7660444431189770143 ) ) ;
#25242=CARTESIAN_POINT ( 'NONE',  ( -1.319360245102545237, -11.06231777344671130, 33.60647404775212976 ) ) ;
#25243=EDGE_CURVE ( 'NONE', #6016, #75911, #84091, .T. ) ;
#25244=DIRECTION ( 'NONE',  ( 0.000000000000000000, 0.7660444431189807890, 0.6427876096865361433 ) ) ;
#25245=ORIENTED_EDGE ( 'NONE', *, *, #36636, .T. ) ;
#25246=ORIENTED_EDGE ( 'NONE', *, *, #83434, .T. ) ;
#25247=ORIENTED_EDGE ( 'NONE', *, *, #67025, .T. ) ;
#25248=CARTESIAN_POINT ( 'NONE',  ( 3.361561038594017781, -3.530189275343204702, 32.79018710029569661 ) ) ;
#25249=EDGE_LOOP ( 'NONE', ( #5066, #37248, #1749, #40663 ) ) ;
#25251=CARTESIAN_POINT ( 'NONE',  ( -8.899922235898328537, -9.804603061927743113, 34.18744698557895845 ) ) ;
#25252=CARTESIAN_POINT ( 'NONE',  ( 9.468822767743365176, -5.827078755546623690, 34.72654668319379567 ) ) ;
#25253=ORIENTED_EDGE ( 'NONE', *, *, #14039, .T. ) ;
#25254=CARTESIAN_POINT ( 'NONE',  ( 16.15384615384615330, -6.386643153685126251, 34.62446782046654192 ) ) ;
#25255=B_SPLINE_CURVE_WITH_KNOTS ( 'NONE', 3,
 ( #19395, #13522, #27041, #54504, #82443, #75660, #53621, #68463, #34234, #62151 ),
 .UNSPECIFIED., .F., .F.,
 ( 4, 2, 2, 2, 4 ),
 ( 0.000000000000000000, 0.0001954311564186868473, 0.0003908623128373736946, 0.0005862934692560605419, 0.0007817246256747473893 ),
 .UNSPECIFIED. ) ;
#25256=AXIS2_PLACEMENT_3D ( 'NONE', #49257, #58540, #28099 ) ;
#25258=EDGE_LOOP ( 'NONE', ( #80079, #35342, #59026, #45954 ) ) ;
#25260=ORIENTED_EDGE ( 'NONE', *, *, #86823, .T. ) ;
#25261=B_SPLINE_CURVE_WITH_KNOTS ( 'NONE', 3,
 ( #36327, #84081, #37194, #64659, #78187, #64215, #15607, #84518, #2081, #43076 ),
 .UNSPECIFIED., .F., .F.,
 ( 4, 2, 2, 2, 4 ),
 ( 0.000000000000000000, 0.0001954339857564073388, 0.0003908679715128146777, 0.0005863019572692220165, 0.0007817359430256293554 ),
 .UNSPECIFIED. ) ;
#25262=LINE ( 'NONE', #80212, #31617 ) ;
#25263=B_SPLINE_CURVE_WITH_KNOTS ( 'NONE', 3,
 ( #88871, #27144, #82099, #67253, #47405, #68137, #33465, #46961, #32566, #25822 ),
 .UNSPECIFIED., .F., .F.,
 ( 4, 2, 2, 2, 4 ),
 ( 0.000000000000000000, 0.0001954339857564091278, 0.0003908679715128182556, 0.0005863019572692274375, 0.0007817359430256365111 ),
 .UNSPECIFIED. ) ;
#25264=DIRECTION ( 'NONE',  ( -0.000000000000000000, 0.9396926207859093161, -0.3420201433256663259 ) ) ;
#25265=FACE_OUTER_BOUND ( 'NONE', #44747, .T. ) ;
#25266=FACE_BOUND ( 'NONE', #48485, .T. ) ;
#25267=EDGE_CURVE ( 'NONE', #57235, #87613, #57278, .T. ) ;
#25269=DIRECTION ( 'NONE',  ( 0.000000000000000000, 0.6427876096865373645, -0.7660444431189797898 ) ) ;
#25271=CARTESIAN_POINT ( 'NONE',  ( -14.17690049986752321, -5.582136614379148654, 34.36778462344220486 ) ) ;
#25274=VERTEX_POINT ( 'NONE', #77109 ) ;
#25276=CARTESIAN_POINT ( 'NONE',  ( 1.514660440535158692, -2.254550872974306674, 29.97347326024527447 ) ) ;
#25277=ORIENTED_EDGE ( 'NONE', *, *, #37660, .T. ) ;
#25278=EDGE_LOOP ( 'NONE', ( #61906, #4099 ) ) ;
#25279=LINE ( 'NONE', #3659, #59044 ) ;
#25280=CARTESIAN_POINT ( 'NONE',  ( 10.86543892702292879, -5.728107161865378494, 34.42597550085002922 ) ) ;
#25281=DIRECTION ( 'NONE',  ( 0.000000000000000000, 0.9848077530122072432, 0.1736481776669354937 ) ) ;
#25282=CYLINDRICAL_SURFACE ( 'NONE', #79650, 0.2500000000000009437 ) ;
#25283=CARTESIAN_POINT ( 'NONE',  ( 17.01083966596719677, -8.120952969808774569, 34.71129190930000163 ) ) ;
#25284=CARTESIAN_POINT ( 'NONE',  ( -15.48079246806219444, -3.711651800289232028, 33.01384336483936011 ) ) ;
#25286=CARTESIAN_POINT ( 'NONE',  ( 17.01165263096229907, -6.026961402152685388, 34.52809138561120506 ) ) ;
#25287=EDGE_CURVE ( 'NONE', #70777, #48470, #74523, .T. ) ;
#25288=CARTESIAN_POINT ( 'NONE',  ( 14.17754509825408604, -11.47017969459903952, 32.78971311882035167 ) ) ;
#25289=CARTESIAN_POINT ( 'NONE',  ( -14.05769230769230660, -2.249999999999998668, 29.75000000000000355 ) ) ;
#25290=ADVANCED_FACE ( 'NONE', ( #84769 ), #64459, .F. ) ;
#25291=CARTESIAN_POINT ( 'NONE',  ( 5.326923076923011813, -7.565270445406050648, 34.75000000000000000 ) ) ;
#25293=ORIENTED_EDGE ( 'NONE', *, *, #79634, .T. ) ;
#25295=VERTEX_POINT ( 'NONE', #49636 ) ;
#25296=CARTESIAN_POINT ( 'NONE',  ( 17.75000000000000000, -7.500000000000001776, 34.75000000000000000 ) ) ;
#25297=CARTESIAN_POINT ( 'NONE',  ( -5.749999999998578915, -7.500000000000154543, 35.00000000000007105 ) ) ;
#25298=EDGE_LOOP ( 'NONE', ( #40154, #1325, #29035, #8083 ) ) ;
#25299=CARTESIAN_POINT ( 'NONE',  ( 3.230769230769108269, -12.70778746994576025, 30.41441678777401236 ) ) ;
#25300=CARTESIAN_POINT ( 'NONE',  ( 15.16468581981335007, -8.973038597847271092, 34.52809138561120506 ) ) ;
#25301=CARTESIAN_POINT ( 'NONE',  ( 0.5923302693632472860, -12.11778462344221019, 31.66786338562085135 ) ) ;
#25302=CARTESIAN_POINT ( 'NONE',  ( -13.13461538461394973, -7.500000000000155431, 34.75000000000007105 ) ) ;
#25303=EDGE_CURVE ( 'NONE', #34093, #63242, #49776, .T. ) ;
#25304=FACE_OUTER_BOUND ( 'NONE', #53633, .T. ) ;
#25305=ORIENTED_EDGE ( 'NONE', *, *, #87387, .T. ) ;
#25306=CARTESIAN_POINT ( 'NONE',  ( -0.4615384615384611200, -11.91647553114624181, 32.58852847137148245 ) ) ;
#25307=ORIENTED_EDGE ( 'NONE', *, *, #71535, .T. ) ;
#25308=DIRECTION ( 'NONE',  ( -0.000000000000000000, -0.5000000000000009992, -0.8660254037844380415 ) ) ;
#25309=CARTESIAN_POINT ( 'NONE',  ( 8.835298102580845025, -12.34228464037088813, 31.77849191805839268 ) ) ;
#25310=CARTESIAN_POINT ( 'NONE',  ( -7.623141002060449090, -3.395485233115139057, 33.02377354290275946 ) ) ;
#25311=EDGE_CURVE ( 'NONE', #23488, #28219, #61578, .T. ) ;
#25312=EDGE_CURVE ( 'NONE', #68692, #77497, #6708, .T. ) ;
#25313=CARTESIAN_POINT ( 'NONE',  ( 10.61538461538461675, -12.34228464037088635, 31.77849191805839268 ) ) ;
#25314=CARTESIAN_POINT ( 'NONE',  ( 13.16168842570853670, -4.026226216239094491, 33.68668979543634379 ) ) ;
#25315=CARTESIAN_POINT ( 'NONE',  ( -39.05038313613820122, -2.249999999999998668, 29.75000000000000355 ) ) ;
#25316=CARTESIAN_POINT ( 'NONE',  ( 9.626224281351815293, -6.386643153685125363, 34.62446782046654903 ) ) ;
#25318=ORIENTED_EDGE ( 'NONE', *, *, #43766, .F. ) ;
#25319=CARTESIAN_POINT ( 'NONE',  ( 4.853996118016227435, -11.98009711892699691, 32.48740034544075428 ) ) ;
#25320=CARTESIAN_POINT ( 'NONE',  ( -14.30769230769242917, -3.643525952248795718, 33.31231777344771672 ) ) ;
#25321=CARTESIAN_POINT ( 'NONE',  ( -0.2387589202700527991, -5.114059244376870872, 34.14424750095245997 ) ) ;
#25322=VECTOR ( 'NONE', #37368, 1000.000000000000227 ) ;
#25323=ORIENTED_EDGE ( 'NONE', *, *, #29362, .F. ) ;
#25325=DIRECTION ( 'NONE',  ( 0.000000000000000000, 0.9848077530122072432, 0.1736481776669354937 ) ) ;
#25326=CARTESIAN_POINT ( 'NONE',  ( 7.623226887246997485, -6.459968553980839800, 34.89616026154728701 ) ) ;
#25328=CARTESIAN_POINT ( 'NONE',  ( 16.15384615384615330, -9.905515769479276145, 34.41647553114623292 ) ) ;
#25331=VERTEX_POINT ( 'NONE', #56398 ) ;
#25332=CARTESIAN_POINT ( 'NONE',  ( -0.4615384615384611200, -12.78798330534102945, 29.74999999999997868 ) ) ;
#25333=CARTESIAN_POINT ( 'NONE',  ( -2.057746789344165439, -10.05730279482229683, 34.04704008940765902 ) ) ;
#25334=CARTESIAN_POINT ( 'NONE',  ( -3.296039676730006640, -11.94971097300153140, 32.03036669348370680 ) ) ;
#25335=ORIENTED_EDGE ( 'NONE', *, *, #40276, .T. ) ;
#25336=CARTESIAN_POINT ( 'NONE',  ( 15.93036122928181975, -12.47654668319379567, 31.42292124445336654 ) ) ;
#25337=B_SPLINE_CURVE_WITH_KNOTS ( 'NONE', 3,
 ( #23060, #43772, #62701, #14531, #42015, #578, #70365, #62263, #56839, #49204 ),
 .UNSPECIFIED., .F., .F.,
 ( 4, 2, 2, 2, 4 ),
 ( 0.0007817359430256372700, 0.0009771253907250052138, 0.001172514838424373266, 0.001367904286123741101, 0.001563293733823109153 ),
 .UNSPECIFIED. ) ;
#25339=CARTESIAN_POINT ( 'NONE',  ( 18.00000000000000000, -3.513871655860378418, 32.76840700105978499 ) ) ;
#25342=CARTESIAN_POINT ( 'NONE',  ( 3.164686851409094448, -2.833524468853757305, 32.15551576947924417 ) ) ;
#25343=ORIENTED_EDGE ( 'NONE', *, *, #47979, .T. ) ;
#25344=CARTESIAN_POINT ( 'NONE',  ( -11.53846153846153655, -12.37446782046654192, 30.86335684631486131 ) ) ;
#25345=CARTESIAN_POINT ( 'NONE',  ( -11.53846153846153655, -12.37446782046654192, 30.86335684631486131 ) ) ;
#25346=CARTESIAN_POINT ( 'NONE',  ( 13.38461538461538680, -12.48256725967547354, 35.29906147534542527 ) ) ;
#25347=CARTESIAN_POINT ( 'NONE',  ( -6.000000000000119904, -2.892918686052165622, 31.69288490824153470 ) ) ;
#25348=CARTESIAN_POINT ( 'NONE',  ( -4.826868657009622865, -8.346898887586323923, 34.93166121998716278 ) ) ;
#25350=EDGE_LOOP ( 'NONE', ( #55919, #86977 ) ) ;
#25351=FACE_OUTER_BOUND ( 'NONE', #38874, .T. ) ;
#25352=EDGE_LOOP ( 'NONE', ( #24789, #31500, #39548, #68317 ) ) ;
#25353=LINE ( 'NONE', #32548, #48644 ) ;
#25354=CARTESIAN_POINT ( 'NONE',  ( -10.48485917715096960, -10.31582465632705237, 34.18122507451815295 ) ) ;
#25355=CARTESIAN_POINT ( 'NONE',  ( -16.21911659980693088, -11.48612834413959582, 32.76840700105983473 ) ) ;
#25356=DIRECTION ( 'NONE',  ( -0.000000000000000000, 0.7660444431189791237, -0.6427876096865379196 ) ) ;
#25359=AXIS2_PLACEMENT_3D ( 'NONE', #41396, #74295, #81065 ) ;
#25360=CARTESIAN_POINT ( 'NONE',  ( -9.561517251340744039, -6.369690395747422684, 34.87708834333098196 ) ) ;
#25361=CARTESIAN_POINT ( 'NONE',  ( -10.86538461538461320, -2.249999999999998668, 29.75000000000000355 ) ) ;
#25362=ORIENTED_EDGE ( 'NONE', *, *, #67587, .T. ) ;
#25364=ORIENTED_EDGE ( 'NONE', *, *, #40334, .F. ) ;
#25366=ORIENTED_EDGE ( 'NONE', *, *, #37207, .F. ) ;
#25367=CARTESIAN_POINT ( 'NONE',  ( -4.377331097570101193, -5.912607949931405038, 34.49155766932282319 ) ) ;
#25368=FACE_OUTER_BOUND ( 'NONE', #4218, .T. ) ;
#25369=CARTESIAN_POINT ( 'NONE',  ( 15.10007776410167324, -4.809359713505814149, 33.96456829005828837 ) ) ;
#25370=CARTESIAN_POINT ( 'NONE',  ( 0.4615384615383396616, -5.219633306517616589, 34.19971097300220464 ) ) ;
#25371=CARTESIAN_POINT ( 'NONE',  ( 13.16113044089144068, -8.496056993536548418, 34.65000542017679663 ) ) ;
#25372=CARTESIAN_POINT ( 'NONE',  ( -5.999999999999998224, -2.833524468853757305, 32.15551576947925838 ) ) ;
#25374=VECTOR ( 'NONE', #31427, 999.9999999999998863 ) ;
#25376=CARTESIAN_POINT ( 'NONE',  ( 9.561617089197383734, -9.929715669179220328, 34.40415004197138416 ) ) ;
#25377=CARTESIAN_POINT ( 'NONE',  ( 0.4615384615384611200, -3.050289026998446396, 32.03036669348365706 ) ) ;
#25382=CARTESIAN_POINT ( 'NONE',  ( 5.999999999999878320, -12.51329471203414379, 31.30864560766407578 ) ) ;
#25383=ORIENTED_EDGE ( 'NONE', *, *, #78507, .F. ) ;
#25384=CARTESIAN_POINT ( 'NONE',  ( 7.846153846153846700, -1.466349020453238561, 30.81389545987213907 ) ) ;
#25386=B_SPLINE_CURVE_WITH_KNOTS ( 'NONE', 3,
 ( #56216, #89140, #35505, #83707, #27857, #76039, #35054, #8481, #1716, #62951 ),
 .UNSPECIFIED., .F., .F.,
 ( 4, 2, 2, 2, 4 ),
 ( 0.0007817246256747476061, 0.0009771112852218909357, 0.001172497944769034049, 0.001367884604316177161, 0.001563271263863320491 ),
 .UNSPECIFIED. ) ;
#25387=DIRECTION ( 'NONE',  ( 0.000000000000000000, 0.1736481776669267785, -0.9848077530122087975 ) ) ;
#25388=CARTESIAN_POINT ( 'NONE',  ( 6.923076923076802558, -2.625532179533778709, 30.86335684631627174 ) ) ;
#25389=FACE_BOUND ( 'NONE', #61665, .T. ) ;
#25390=ORIENTED_EDGE ( 'NONE', *, *, #85118, .F. ) ;
#25391=B_SPLINE_CURVE_WITH_KNOTS ( 'NONE', 3,
 ( #54715, #19171, #82206, #20495, #56500, #22270, #668, #55162, #27692, #63251 ),
 .UNSPECIFIED., .F., .F.,
 ( 4, 2, 2, 2, 4 ),
 ( 0.000000000000000000, 0.0001954311564186887718, 0.0003908623128373775435, 0.0005862934692560662882, 0.0007817246256747550871 ),
 .UNSPECIFIED. ) ;
#25392=ADVANCED_FACE ( 'NONE', ( #85644 ), #51833, .F. ) ;
#25393=AXIS2_PLACEMENT_3D ( 'NONE', #30605, #17550, #57640 ) ;
#25394=EDGE_LOOP ( 'NONE', ( #79036, #16066 ) ) ;
#25395=CARTESIAN_POINT ( 'NONE',  ( -5.076923076923075762, -6.681629849574314051, 35.83090037661290239 ) ) ;
#25396=VERTEX_POINT ( 'NONE', #38791 ) ;
#25397=FACE_BOUND ( 'NONE', #88188, .T. ) ;
#25398=CARTESIAN_POINT ( 'NONE',  ( -15.23076923076922995, -6.435427911321262684, 35.78748833219616898 ) ) ;
#25399=CARTESIAN_POINT ( 'NONE',  ( -13.51476259405360203, -10.88202310037935661, 33.43294751532457099 ) ) ;
#25401=CARTESIAN_POINT ( 'NONE',  ( 18.00000000000000000, -2.721908614388771852, 31.22303859784724978 ) ) ;
#25402=CARTESIAN_POINT ( 'NONE',  ( 8.992193903497444296, -7.369474539155828730, 34.99858011523957657 ) ) ;
#25403=CARTESIAN_POINT ( 'NONE',  ( -18.13069060311030611, -3.957541250942359756, 33.62499894934981626 ) ) ;
#25404=VERTEX_POINT ( 'NONE', #78876 ) ;
#25405=CARTESIAN_POINT ( 'NONE',  ( 12.46153846153846168, -4.786620604624113540, 33.94971097300155094 ) ) ;
#25406=DIRECTION ( 'NONE',  ( -1.000000000000000000, 0.000000000000000000, 0.000000000000000000 ) ) ;
#25407=CARTESIAN_POINT ( 'NONE',  ( -9.469296340694842939, -2.554770724473667265, 30.48948780036025852 ) ) ;
#25408=VERTEX_POINT ( 'NONE', #66706 ) ;
#25409=CARTESIAN_POINT ( 'NONE',  ( 2.557637717070352146, -12.45601412856602686, 31.48342859153981621 ) ) ;
#25411=EDGE_LOOP ( 'NONE', ( #76537, #42831 ) ) ;
#25412=CARTESIAN_POINT ( 'NONE',  ( -2.307692307692427391, -2.892918686052166066, 31.69288490824153470 ) ) ;
#25413=CARTESIAN_POINT ( 'NONE',  ( -12.23852710992561299, -2.554770724473667265, 30.48948780036025852 ) ) ;
#25414=CARTESIAN_POINT ( 'NONE',  ( 24.00000000000000000, -5.499999999999981348, 27.75000000000000000 ) ) ;
#25415=CARTESIAN_POINT ( 'NONE',  ( 7.976992264166607782, -7.277220443632449687, 34.74524770363009907 ) ) ;
#25416=CARTESIAN_POINT ( 'NONE',  ( -6.700113788810249105, -7.369474539155828730, 34.99858011523957657 ) ) ;
#25418=EDGE_CURVE ( 'NONE', #64011, #80539, #334, .T. ) ;
#25419=CYLINDRICAL_SURFACE ( 'NONE', #39527, 2.000000000000001776 ) ;
#25422=CARTESIAN_POINT ( 'NONE',  ( 8.899756470994333313, -12.27024696741798770, 31.24895572276497546 ) ) ;
#25425=ORIENTED_EDGE ( 'NONE', *, *, #54694, .F. ) ;
#25426=CARTESIAN_POINT ( 'NONE',  ( -12.68446467905460828, -8.239355502252617924, 34.69524867566427417 ) ) ;
#25427=EDGE_LOOP ( 'NONE', ( #41604, #36973, #2657, #6557 ) ) ;
#25428=ADVANCED_FACE ( 'NONE', ( #65798 ), #80681, .F. ) ;
#25429=ORIENTED_EDGE ( 'NONE', *, *, #35056, .T. ) ;
#25430=FACE_OUTER_BOUND ( 'NONE', #45180, .T. ) ;
#25431=VECTOR ( 'NONE', #55672, 1000.000000000000227 ) ;
#25432=ORIENTED_EDGE ( 'NONE', *, *, #2310, .F. ) ;
#25433=CARTESIAN_POINT ( 'NONE',  ( -14.98082371242109012, -5.852078868378309373, 34.47109172314383585 ) ) ;
#25436=CARTESIAN_POINT ( 'NONE',  ( 10.86543903529806876, -2.544122305571458575, 31.48381861865057729 ) ) ;
#25437=DIRECTION ( 'NONE',  ( 0.000000000000000000, 0.4999999999999960032, -0.8660254037844410391 ) ) ;
#25439=B_SPLINE_CURVE_WITH_KNOTS ( 'NONE', 3,
 ( #48674, #49124, #14910, #7710, #85904, #42386 ),
 .UNSPECIFIED., .F., .F.,
 ( 4, 2, 4 ),
 ( 4.336808689942017736E-19, 0.0001954784845028932508, 0.0003909569690057860679 ),
 .UNSPECIFIED. ) ;
#25440=B_SPLINE_CURVE_WITH_KNOTS ( 'NONE', 3,
 ( #77205, #70459, #44280, #65004, #56927, #83537, #1551, #29476, #36231, #49294 ),
 .UNSPECIFIED., .F., .F.,
 ( 4, 2, 2, 2, 4 ),
 ( 0.0007817359430256364027, 0.0009771253907250043464, 0.001172514838424372399, 0.001367904286123740234, 0.001563293733823108286 ),
 .UNSPECIFIED. ) ;
#25441=CARTESIAN_POINT ( 'NONE',  ( -5.326946301144532825, -3.520140089381497361, 33.17453946501458262 ) ) ;
#25442=LINE ( 'NONE', #46161, #21463 ) ;
#25443=CARTESIAN_POINT ( 'NONE',  ( -7.715362038329057981, -12.11778462344220841, 31.66786338562085135 ) ) ;
#25445=CARTESIAN_POINT ( 'NONE',  ( 5.207448515156718472, -3.068774925481847937, 32.56582465632704526 ) ) ;
#25447=CARTESIAN_POINT ( 'NONE',  ( -9.692307692307691624, -2.517432740324522911, 35.29906147534542527 ) ) ;
#25448=ORIENTED_EDGE ( 'NONE', *, *, #58126, .T. ) ;
#25449=EDGE_LOOP ( 'NONE', ( #52943, #13479 ) ) ;
#25451=CARTESIAN_POINT ( 'NONE',  ( -8.834501215191545853, -12.46129190929999986, 30.37095296980880832 ) ) ;
#25452=LINE ( 'NONE', #80408, #1463 ) ;
#25453=CARTESIAN_POINT ( 'NONE',  ( -2.531177232256636156, -2.353723527008296568, 30.78948104536958752 ) ) ;
#25454=CARTESIAN_POINT ( 'NONE',  ( -16.15384615384615330, -12.37446782046654192, 30.86335684631486131 ) ) ;
#25455=LINE ( 'NONE', #6078, #85234 ) ;
#25456=AXIS2_PLACEMENT_3D ( 'NONE', #1045, #49671, #7365 ) ;
#25457=FACE_OUTER_BOUND ( 'NONE', #64744, .T. ) ;
#25458=AXIS2_PLACEMENT_3D ( 'NONE', #73754, #67865, #32309 ) ;
#25461=ORIENTED_EDGE ( 'NONE', *, *, #81900, .F. ) ;
#25463=CARTESIAN_POINT ( 'NONE',  ( 7.780883845597524662, -11.06231777344662781, 33.60647404775220082 ) ) ;
#25464=B_SPLINE_CURVE_WITH_KNOTS ( 'NONE', 3,
 ( #42947, #70862, #36628, #64081, #23537, #78484, #57335, #36198, #71281, #63645 ),
 .UNSPECIFIED., .F., .F.,
 ( 4, 2, 2, 2, 4 ),
 ( 0.000000000000000000, 0.0001954311584214072652, 0.0003908623168428145304, 0.0005862934752642217414, 0.0007817246336856290608 ),
 .UNSPECIFIED. ) ;
#25465=B_SPLINE_CURVE_WITH_KNOTS ( 'NONE', 3,
 ( #67719, #32592, #47430, #52857, #60062, #25846, #74925, #38923, #88455, #11894 ),
 .UNSPECIFIED., .F., .F.,
 ( 4, 2, 2, 2, 4 ),
 ( 0.000000000000000000, 0.0001954339857564097512, 0.0003908679715128195024, 0.0005863019572692292807, 0.0007817359430256390048 ),
 .UNSPECIFIED. ) ;
#25466=CARTESIAN_POINT ( 'NONE',  ( -14.24243716817946925, -6.835583212224610072, 34.95778746994559327 ) ) ;
#25467=CARTESIAN_POINT ( 'NONE',  ( 5.076923076922953193, -12.16647553114689728, 32.15551576947799362 ) ) ;
#25468=CARTESIAN_POINT ( 'NONE',  ( 1.253924781505078689, -11.37499894934982514, 33.29245874905763003 ) ) ;
#25469=CARTESIAN_POINT ( 'NONE',  ( -2.242436736416280940, -11.94971097300157403, 32.03036669348361443 ) ) ;
#25470=EDGE_CURVE ( 'NONE', #47330, #67660, #52291, .T. ) ;
#25472=ORIENTED_EDGE ( 'NONE', *, *, #81703, .T. ) ;
#25473=B_SPLINE_CURVE_WITH_KNOTS ( 'NONE', 3,
 ( #44132, #49584, #84719, #78820, #29760, #10374, #17120, #51315, #37837, #9478 ),
 .UNSPECIFIED., .F., .F.,
 ( 4, 2, 2, 2, 4 ),
 ( 0.000000000000000000, 0.0001954339857564093175, 0.0003908679715128186350, 0.0005863019572692279796, 0.0007817359430256372700 ),
 .UNSPECIFIED. ) ;
#25475=VERTEX_POINT ( 'NONE', #45537 ) ;
#25476=CARTESIAN_POINT ( 'NONE',  ( 18.00000000000000000, -1.242168528481310874, 33.36296068462461051 ) ) ;
#25479=CARTESIAN_POINT ( 'NONE',  ( 4.376625822824220080, -3.563462043263029955, 33.22394488606062879 ) ) ;
#25480=CARTESIAN_POINT ( 'NONE',  ( 1.161130440891436466, -3.754499324213721234, 33.06261337010820256 ) ) ;
#25481=EDGE_CURVE ( 'NONE', #62418, #52040, #38341, .T. ) ;
#25483=DIRECTION ( 'NONE',  ( -0.000000000000000000, -0.9396926207859092051, -0.3420201433256662704 ) ) ;
#25484=AXIS2_PLACEMENT_3D ( 'NONE', #47718, #27892, #54469 ) ;
#25485=EDGE_LOOP ( 'NONE', ( #75435, #29832 ) ) ;
#25486=EDGE_CURVE ( 'NONE', #34572, #20451, #20748, .T. ) ;
#25487=EDGE_LOOP ( 'NONE', ( #29664, #38478 ) ) ;
#25489=DIRECTION ( 'NONE',  ( -0.000000000000000000, 1.000000000000000000, 3.491481338843133355E-15 ) ) ;
#25490=VERTEX_POINT ( 'NONE', #80224 ) ;
#25491=FACE_OUTER_BOUND ( 'NONE', #23476, .T. ) ;
#25492=CARTESIAN_POINT ( 'NONE',  ( -6.988326854851008463, -2.255955759149247619, 30.00000000000013856 ) ) ;
#25494=ORIENTED_EDGE ( 'NONE', *, *, #25171, .F. ) ;
#25497=ORIENTED_EDGE ( 'NONE', *, *, #53582, .T. ) ;
#25498=CARTESIAN_POINT ( 'NONE',  ( -13.60810030917971680, -11.60425143139329940, 33.02411095842164457 ) ) ;
#25500=DIRECTION ( 'NONE',  ( -0.000000000000000000, -0.9848077530122085754, -0.1736481776669273613 ) ) ;
#25501=CARTESIAN_POINT ( 'NONE',  ( -7.053224132515143907, -3.817052484675422797, 33.13202310037935661 ) ) ;
#25502=CARTESIAN_POINT ( 'NONE',  ( -0.4615384615384611200, -8.564572088678739092, 35.78748833219616898 ) ) ;
#25503=EDGE_CURVE ( 'NONE', #22672, #24781, #35760, .T. ) ;
#25504=AXIS2_PLACEMENT_3D ( 'NONE', #6763, #88329, #47306 ) ;
#25505=CARTESIAN_POINT ( 'NONE',  ( -6.000000000000121680, -3.083524468854526912, 32.58852847137268327 ) ) ;
#25506=VERTEX_POINT ( 'NONE', #39244 ) ;
#25508=CARTESIAN_POINT ( 'NONE',  ( -8.835313148590904220, -3.937682226553330445, 33.60647404775217240 ) ) ;
#25509=DIRECTION ( 'NONE',  ( 0.000000000000000000, 0.9396926207859126468, 0.3420201433256571111 ) ) ;
#25510=EDGE_LOOP ( 'NONE', ( #26866, #57050, #638, #61480 ) ) ;
#25511=CARTESIAN_POINT ( 'NONE',  ( 12.46153846153833911, -3.835265460704628371, 33.15142922262033665 ) ) ;
#25512=CARTESIAN_POINT ( 'NONE',  ( -6.250023237292963607, -10.76384336483936011, 33.53834819971076087 ) ) ;
#25514=CARTESIAN_POINT ( 'NONE',  ( 7.976945653978629203, -3.062576670634119758, 32.05464942895959979 ) ) ;
#25515=EDGE_CURVE ( 'NONE', #79391, #6804, #46429, .T. ) ;
#25516=FACE_BOUND ( 'NONE', #18645, .T. ) ;
#25517=CARTESIAN_POINT ( 'NONE',  ( 1.161735867877800699, -7.630690623152302621, 34.99857592706774057 ) ) ;
#25518=CYLINDRICAL_SURFACE ( 'NONE', #2846, 0.2499999999999998890 ) ;
#25521=CARTESIAN_POINT ( 'NONE',  ( 2.980792499826877329, -4.236021600441998380, 33.53823185664189310 ) ) ;
#25522=CARTESIAN_POINT ( 'NONE',  ( -5.076923076923199218, -12.70778746994576025, 30.41441678777401236 ) ) ;
#25523=CARTESIAN_POINT ( 'NONE',  ( 1.384615384615264011, -3.083524468854526912, 32.58852847137268327 ) ) ;
#25524=ADVANCED_FACE ( 'NONE', ( #61258 ), #5896, .F. ) ;
#25525=LINE ( 'NONE', #53879, #37577 ) ;
#25528=EDGE_LOOP ( 'NONE', ( #85557, #13195, #49667, #10916 ) ) ;
#25529=CARTESIAN_POINT ( 'NONE',  ( 8.769230769230647482, -12.46129190930018460, 30.37095296980731973 ) ) ;
#25530=EDGE_CURVE ( 'NONE', #18328, #21233, #41012, .T. ) ;
#25531=EDGE_CURVE ( 'NONE', #68329, #26886, #79771, .T. ) ;
#25532=CARTESIAN_POINT ( 'NONE',  ( 2.177001704582001818, -2.295517848115769421, 30.44137282052137294 ) ) ;
#25533=DIRECTION ( 'NONE',  ( -0.000000000000000000, 0.3420201433256694901, -0.9396926207859082059 ) ) ;
#25535=CARTESIAN_POINT ( 'NONE',  ( 16.85399611801622655, -12.64616026154729411, 30.79003144601914244 ) ) ;
#25536=CARTESIAN_POINT ( 'NONE',  ( 6.130790440966954691, -3.338503747796866872, 32.95102852606553512 ) ) ;
#25538=CARTESIAN_POINT ( 'NONE',  ( 14.08476609017616177, -10.61292498521070549, 33.66303323003028680 ) ) ;
#25539=CARTESIAN_POINT ( 'NONE',  ( -2.057746898314262829, -6.653508905675590945, 34.93172785388651391 ) ) ;
#25541=CARTESIAN_POINT ( 'NONE',  ( 5.011653076366756387, -9.528491918058357157, 34.59228464037090589 ) ) ;
#25542=CARTESIAN_POINT ( 'NONE',  ( 8.638539302563209787, -9.804603061927743113, 34.18744698557895845 ) ) ;
#25544=CARTESIAN_POINT ( 'NONE',  ( 9.822355298563376635, -7.723484964179501588, 34.74522123443823318 ) ) ;
#25547=CARTESIAN_POINT ( 'NONE',  ( 11.78846153846297362, -7.500000000000155431, 34.75000000000007105 ) ) ;
#25548=CARTESIAN_POINT ( 'NONE',  ( 1.384615384615386802, -1.242168528481310874, 33.36296068462461051 ) ) ;
#25549=AXIS2_PLACEMENT_3D ( 'NONE', #48979, #56179, #83671 ) ;
#25552=CARTESIAN_POINT ( 'NONE',  ( -5.207070286361294542, -2.619462340734462380, 30.83744416345203021 ) ) ;
#25553=ORIENTED_EDGE ( 'NONE', *, *, #85111, .F. ) ;
#25554=DIRECTION ( 'NONE',  ( -0.000000000000000000, -0.000000000000000000, -1.000000000000000000 ) ) ;
#25555=CARTESIAN_POINT ( 'NONE',  ( -12.39547112818838492, -12.62096338111211757, 30.90682066428152908 ) ) ;
#25556=CARTESIAN_POINT ( 'NONE',  ( 11.40777093535123043, -2.845849958028613624, 32.17971566917920967 ) ) ;
#25557=ORIENTED_EDGE ( 'NONE', *, *, #3415, .F. ) ;
#25558=CARTESIAN_POINT ( 'NONE',  ( -7.912237257109724808, -8.120952969808774569, 34.71129190930000163 ) ) ;
#25559=CARTESIAN_POINT ( 'NONE',  ( -3.007757879156381264, -3.587049720035815348, 32.86302985866382897 ) ) ;
#25560=CARTESIAN_POINT ( 'NONE',  ( -5.326923076923075762, -7.500000000000001776, 35.04278698407183867 ) ) ;
#25561=CARTESIAN_POINT ( 'NONE',  ( 11.60452988946397745, -8.973038597847271092, 34.52809138561121216 ) ) ;
#25562=EDGE_LOOP ( 'NONE', ( #58309, #62904 ) ) ;
#25565=CARTESIAN_POINT ( 'NONE',  ( -15.23076923076922995, -11.35647404775217417, 33.31231777344666511 ) ) ;
#25566=CARTESIAN_POINT ( 'NONE',  ( -11.28846153846153655, -2.249999999999998668, 29.75000000000000355 ) ) ;
#25567=ORIENTED_EDGE ( 'NONE', *, *, #74004, .F. ) ;
#25568=ORIENTED_EDGE ( 'NONE', *, *, #20448, .F. ) ;
#25569=EDGE_CURVE ( 'NONE', #21373, #39792, #54082, .T. ) ;
#25573=CARTESIAN_POINT ( 'NONE',  ( -16.21992853320628925, -3.322132147404559976, 32.92929555188719348 ) ) ;
#25575=CARTESIAN_POINT ( 'NONE',  ( -12.59168567097668756, -3.817052484675422797, 33.13202310037935661 ) ) ;
#25576=ADVANCED_FACE ( 'NONE', ( #6770 ), #88335, .F. ) ;
#25577=AXIS2_PLACEMENT_3D ( 'NONE', #70614, #31854, #51192 ) ;
#25578=CARTESIAN_POINT ( 'NONE',  ( -17.07692307692307665, -4.786620604624113540, 33.94971097300155094 ) ) ;
#25579=EDGE_LOOP ( 'NONE', ( #7885, #81734, #2014, #31600 ) ) ;
#25580=EDGE_LOOP ( 'NONE', ( #75641, #79164 ) ) ;
#25582=EDGE_LOOP ( 'NONE', ( #58487, #58670 ) ) ;
#25583=CARTESIAN_POINT ( 'NONE',  ( -1.384615384615505151, -5.219633306517616589, 34.19971097300220464 ) ) ;
#25584=ORIENTED_EDGE ( 'NONE', *, *, #59287, .F. ) ;
#25586=LINE ( 'NONE', #46300, #72409 ) ;
#25587=CARTESIAN_POINT ( 'NONE',  ( 2.557637826040450868, -3.712312575010499938, 33.01462480002815170 ) ) ;
#25588=DIRECTION ( 'NONE',  ( 0.000000000000000000, 0.7660444431189822323, -0.6427876096865344779 ) ) ;
#25589=B_SPLINE_CURVE_WITH_KNOTS ( 'NONE', 3,
 ( #41558, #1016, #34793, #76679, #9114, #49202, #50076, #28950, #28042, #70363 ),
 .UNSPECIFIED., .F., .F.,
 ( 4, 2, 2, 2, 4 ),
 ( 0.0007817359430256297891, 0.0009771253907249958896, 0.001172514838424361990, 0.001367904286123728091, 0.001563293733823094191 ),
 .UNSPECIFIED. ) ;
#25590=ORIENTED_EDGE ( 'NONE', *, *, #17848, .F. ) ;
#25592=ORIENTED_EDGE ( 'NONE', *, *, #3108, .F. ) ;
#25594=CARTESIAN_POINT ( 'NONE',  ( -13.38461538461538325, -1.044019251281081972, 31.83374038241031911 ) ) ;
#25595=CARTESIAN_POINT ( 'NONE',  ( 5.142991427925514003, -4.786620604624113540, 33.94971097300155805 ) ) ;
#25596=ORIENTED_EDGE ( 'NONE', *, *, #1303, .F. ) ;
#25597=CARTESIAN_POINT ( 'NONE',  ( 18.22301284409339672, -11.98016756924215187, 32.48728574198911190 ) ) ;
#25598=CARTESIAN_POINT ( 'NONE',  ( 15.23076923076923173, -13.20930481340135110, 34.54067556320372745 ) ) ;
#25601=CARTESIAN_POINT ( 'NONE',  ( -5.933932666649925025, -3.322132147404559976, 32.92929555188717927 ) ) ;
#25603=FACE_BOUND ( 'NONE', #13187, .T. ) ;
#25605=CARTESIAN_POINT ( 'NONE',  ( -12.52762187249433801, -8.973038597847271092, 34.52809138561120506 ) ) ;
#25606=CARTESIAN_POINT ( 'NONE',  ( -10.54931728203453822, -10.67929555188718282, 33.92786785259544757 ) ) ;
#25607=CARTESIAN_POINT ( 'NONE',  ( -17.07692307692319744, -12.70778746994576025, 30.41441678777401236 ) ) ;
#25608=CARTESIAN_POINT ( 'NONE',  ( -5.299849294439224145, -3.105860786376062332, 32.13614157043599562 ) ) ;
#25609=CARTESIAN_POINT ( 'NONE',  ( 0.4615384615383396616, -12.27809138561165270, 31.22303859784587132 ) ) ;
#25610=CARTESIAN_POINT ( 'NONE',  ( 7.053122085911702754, -2.504778602574660340, 29.97347330155780298 ) ) ;
#25611=VERTEX_POINT ( 'NONE', #34244 ) ;
#25612=AXIS2_PLACEMENT_3D ( 'NONE', #70646, #37286, #15707 ) ;
#25613=CARTESIAN_POINT ( 'NONE',  ( 2.307692307692309264, -6.386643153685126251, 34.62446782046654192 ) ) ;
#25614=CARTESIAN_POINT ( 'NONE',  ( -13.31936024510254590, -4.320704448112861584, 33.92786785259548310 ) ) ;
#25615=ORIENTED_EDGE ( 'NONE', *, *, #46223, .F. ) ;
#25616=ORIENTED_EDGE ( 'NONE', *, *, #32526, .T. ) ;
#25617=DIRECTION ( 'NONE',  ( -0.000000000000000000, 0.7660444431189791237, -0.6427876096865379196 ) ) ;
#25618=CARTESIAN_POINT ( 'NONE',  ( 15.90382292962469535, -2.341070481393820124, 30.72580821765574299 ) ) ;
#25619=CARTESIAN_POINT ( 'NONE',  ( -15.36124593888569478, -7.276988635370452485, 34.74523720219453793 ) ) ;
#25620=VERTEX_POINT ( 'NONE', #27492 ) ;
#25621=DIRECTION ( 'NONE',  ( 0.000000000000000000, 0.6427876096865373645, -0.7660444431189797898 ) ) ;
#25622=CARTESIAN_POINT ( 'NONE',  ( -9.692307692307691624, -12.78798330534102945, 29.74999999999997868 ) ) ;
#25623=EDGE_CURVE ( 'NONE', #63945, #84853, #29372, .T. ) ;
#25624=EDGE_CURVE ( 'NONE', #30118, #80116, #60383, .T. ) ;
#25625=CARTESIAN_POINT ( 'NONE',  ( 11.78840694783958298, -2.986452184633680673, 32.43230066228895225 ) ) ;
#25626=CARTESIAN_POINT ( 'NONE',  ( 17.99999999999987566, -10.33852847137269571, 34.16647553114546554 ) ) ;
#25627=CARTESIAN_POINT ( 'NONE',  ( -12.71151519248081740, -4.943428324936578910, 34.04746400365624481 ) ) ;
#25632=VERTEX_POINT ( 'NONE', #81119 ) ;
#25633=EDGE_CURVE ( 'NONE', #21841, #25408, #70210, .T. ) ;
#25634=ORIENTED_EDGE ( 'NONE', *, *, #37033, .T. ) ;
#25636=CARTESIAN_POINT ( 'NONE',  ( -9.942330916529147800, -2.588893531581426988, 31.60682220781847818 ) ) ;
#25637=ADVANCED_FACE ( 'NONE', ( #85097 ), #15311, .F. ) ;
#25638=CARTESIAN_POINT ( 'NONE',  ( 16.21910172512217585, -6.879047030191284051, 34.71129190930002295 ) ) ;
#25641=CARTESIAN_POINT ( 'NONE',  ( 15.23076923076910916, -5.941354392335915335, 34.76329471203413846 ) ) ;
#25643=FACE_OUTER_BOUND ( 'NONE', #49247, .T. ) ;
#25644=CARTESIAN_POINT ( 'NONE',  ( 14.08420738312797837, -6.716662450894489211, 34.94144148231605840 ) ) ;
#25645=AXIS2_PLACEMENT_3D ( 'NONE', #45387, #17036, #72860 ) ;
#25646=CARTESIAN_POINT ( 'NONE',  ( -13.51509209273184986, -7.276988635370452485, 34.74523720219453793 ) ) ;
#25647=CARTESIAN_POINT ( 'NONE',  ( 13.25446741488369362, -10.31621877034669588, 34.18098118002070152 ) ) ;
#25648=DIRECTION ( 'NONE',  ( 1.000000000000000000, 0.000000000000000000, 0.000000000000000000 ) ) ;
#25649=CARTESIAN_POINT ( 'NONE',  ( 13.51540582558234149, -2.494656445102012565, 31.33466734024120015 ) ) ;
#25651=CARTESIAN_POINT ( 'NONE',  ( 7.976944287120795174, -8.191423895709840863, 34.95447573519442130 ) ) ;
#25652=DIRECTION ( 'NONE',  ( -0.000000000000000000, 0.9396926207859092051, -0.3420201433256662704 ) ) ;
#25654=CARTESIAN_POINT ( 'NONE',  ( -3.361459833879537396, -12.35290016733513951, 31.75349464988449455 ) ) ;
#25655=EDGE_CURVE ( 'NONE', #59185, #37020, #42348, .T. ) ;
#25656=VERTEX_POINT ( 'NONE', #22941 ) ;
#25657=DIRECTION ( 'NONE',  ( 0.000000000000000000, 0.9848077530122072432, 0.1736481776669354937 ) ) ;
#25658=DIRECTION ( 'NONE',  ( 0.000000000000000000, 0.9848077530122072432, -0.1736481776669354937 ) ) ;
#25659=B_SPLINE_CURVE_WITH_KNOTS ( 'NONE', 3,
 ( #23224, #71852, #78610, #8838, #16472, #36312, #2067, #2499, #29551, #50238 ),
 .UNSPECIFIED., .F., .F.,
 ( 4, 2, 2, 2, 4 ),
 ( 0.0007817359430256297891, 0.0009771253907249958896, 0.001172514838424362207, 0.001367904286123728524, 0.001563293733823094625 ),
 .UNSPECIFIED. ) ;
#25660=CARTESIAN_POINT ( 'NONE',  ( 5.749976775778542049, -2.588893531581426544, 31.60682220781847818 ) ) ;
#25662=CARTESIAN_POINT ( 'NONE',  ( 13.38461538461526601, -5.219633306517616589, 34.19971097300220464 ) ) ;
#25663=CARTESIAN_POINT ( 'NONE',  ( -17.86947429823644029, -10.88167719472716577, 33.43325721877153711 ) ) ;
#25664=EDGE_CURVE ( 'NONE', #48838, #18632, #16442, .T. ) ;
#25665=CYLINDRICAL_SURFACE ( 'NONE', #84231, 0.2499999999999997502 ) ;
#25666=VERTEX_POINT ( 'NONE', #41902 ) ;
#25668=DIRECTION ( 'NONE',  ( 0.000000000000000000, 0.9396926207859126468, 0.3420201433256571111 ) ) ;
#25669=ORIENTED_EDGE ( 'NONE', *, *, #73989, .T. ) ;
#25670=CARTESIAN_POINT ( 'NONE',  ( -7.173100147298381302, -11.56360843649121861, 33.07473185843129926 ) ) ;
#25671=ORIENTED_EDGE ( 'NONE', *, *, #48750, .F. ) ;
#25672=CARTESIAN_POINT ( 'NONE',  ( -17.07692307692319744, -2.625532179533778709, 30.86335684631627174 ) ) ;
#25673=EDGE_CURVE ( 'NONE', #9337, #20097, #21613, .T. ) ;
#25674=CARTESIAN_POINT ( 'NONE',  ( -7.780898274877822374, -11.94971097300157403, 32.03036669348361443 ) ) ;
#25675=CARTESIAN_POINT ( 'NONE',  ( -1.449885830576160162, -4.481592998940161721, 33.73612834413957984 ) ) ;
#25676=VERTEX_POINT ( 'NONE', #22064 ) ;
#25677=CARTESIAN_POINT ( 'NONE',  ( 0.3313904918067641647, -5.070767119584671967, 34.40440758774516183 ) ) ;
#25678=VERTEX_POINT ( 'NONE', #56291 ) ;
#25679=ADVANCED_FACE ( 'NONE', ( #8999 ), #49538, .F. ) ;
#25680=ORIENTED_EDGE ( 'NONE', *, *, #52186, .F. ) ;
#25681=CARTESIAN_POINT ( 'NONE',  ( 3.230769230769110045, -2.892918686052166066, 31.69288490824153470 ) ) ;
#25682=DIRECTION ( 'NONE',  ( -0.000000000000000000, -0.1736481776669307198, -0.9848077530122080203 ) ) ;
#25684=CARTESIAN_POINT ( 'NONE',  ( 17.32692307692307665, -7.500000000000001776, 35.04278698407183867 ) ) ;
#25685=CARTESIAN_POINT ( 'NONE',  ( 9.942362112221147186, -10.06805714834173493, 34.32951233291982618 ) ) ;
#25687=EDGE_CURVE ( 'NONE', #26693, #49542, #77693, .T. ) ;
#25688=DIRECTION ( 'NONE',  ( -0.000000000000000000, -0.6427876096865404731, -0.7660444431189770143 ) ) ;
#25689=EDGE_LOOP ( 'NONE', ( #42599, #83804, #69649, #82322 ) ) ;
#25690=ORIENTED_EDGE ( 'NONE', *, *, #21658, .T. ) ;
#25691=ADVANCED_FACE ( 'NONE', ( #70694 ), #50402, .F. ) ;
#25692=VERTEX_POINT ( 'NONE', #77884 ) ;
#25693=DIRECTION ( 'NONE',  ( 0.000000000000000000, -6.938893903907222067E-15, 1.000000000000000000 ) ) ;
#25694=ORIENTED_EDGE ( 'NONE', *, *, #43640, .F. ) ;
#25695=CIRCLE ( 'NONE', #77444, 0.2500000000000002220 ) ;
#25696=DIRECTION ( 'NONE',  ( -0.000000000000000000, 0.8660254037844397068, -0.4999999999999978906 ) ) ;
#25697=CARTESIAN_POINT ( 'NONE',  ( 1.384615384615265343, -3.300289026999228881, 32.46337939537708905 ) ) ;
#25698=VERTEX_POINT ( 'NONE', #36895 ) ;
#25699=ADVANCED_FACE ( 'NONE', ( #64357 ), #22502, .F. ) ;
#25700=CARTESIAN_POINT ( 'NONE',  ( -7.846153846153844924, -7.500000000000001776, 35.04278698407183867 ) ) ;
#25701=B_SPLINE_CURVE_WITH_KNOTS ( 'NONE', 3,
 ( #35580, #82887, #76112, #77442, #63025, #43650, #9428, #15309, #62157, #28829 ),
 .UNSPECIFIED., .F., .F.,
 ( 4, 2, 2, 2, 4 ),
 ( 0.0007817246256747453293, 0.0009771112852218881168, 0.001172497944769031013, 0.001367884604316173692, 0.001563271263863316371 ),
 .UNSPECIFIED. ) ;
#25702=AXIS2_PLACEMENT_3D ( 'NONE', #59025, #32010, #25693 ) ;
#25703=EDGE_CURVE ( 'NONE', #53001, #89000, #15756, .T. ) ;
#25704=ORIENTED_EDGE ( 'NONE', *, *, #48823, .F. ) ;
#25706=B_SPLINE_CURVE_WITH_KNOTS ( 'NONE', 3,
 ( #43325, #83883, #22170, #48744, #49635, #42889, #69019, #7329, #70356, #36137 ),
 .UNSPECIFIED., .F., .F.,
 ( 4, 2, 2, 2, 4 ),
 ( 0.000000000000000000, 0.0001954311564186864407, 0.0003908623128373728815, 0.0005862934692560593493, 0.0007817246256747457630 ),
 .UNSPECIFIED. ) ;
#25707=ORIENTED_EDGE ( 'NONE', *, *, #14001, .F. ) ;
#25709=B_SPLINE_CURVE_WITH_KNOTS ( 'NONE', 3,
 ( #15700, #64303, #43165, #44035, #78722, #84610, #37730, #22446, #2604, #78268 ),
 .UNSPECIFIED., .F., .F.,
 ( 4, 2, 2, 2, 4 ),
 ( 0.000000000000000000, 0.0001954339857564074473, 0.0003908679715128148945, 0.0005863019572692223418, 0.0007817359430256297891 ),
 .UNSPECIFIED. ) ;
#25710=CARTESIAN_POINT ( 'NONE',  ( -9.442307692307691624, -2.249999999999998668, 29.75000000000000355 ) ) ;
#25711=VECTOR ( 'NONE', #84126, 1000.000000000000114 ) ;
#25712=CARTESIAN_POINT ( 'NONE',  ( 4.023155550735845409, -12.62707690430377383, 30.88035979386743435 ) ) ;
#25713=CARTESIAN_POINT ( 'NONE',  ( 4.088596222072069075, -2.255955759149247619, 30.00000000000013856 ) ) ;
#25714=FACE_BOUND ( 'NONE', #49605, .T. ) ;
#25715=DIRECTION ( 'NONE',  ( -0.000000000000000000, -0.1736481776669307198, -0.9848077530122080203 ) ) ;
#25716=CYLINDRICAL_SURFACE ( 'NONE', #29861, 0.2500000000000004996 ) ;
#25717=CARTESIAN_POINT ( 'NONE',  ( -1.515305987725691805, -2.295517848115769421, 30.44137282052137294 ) ) ;
#25719=CARTESIAN_POINT ( 'NONE',  ( 10.39250593295597014, -7.630691491037285168, 34.74850469731152458 ) ) ;
#25720=DIRECTION ( 'NONE',  ( -0.000000000000000000, -0.8660254037844399289, -0.4999999999999980016 ) ) ;
#25721=ORIENTED_EDGE ( 'NONE', *, *, #30154, .F. ) ;
#25722=CARTESIAN_POINT ( 'NONE',  ( -11.78843828251013015, -3.436278759898153901, 33.07459398097509506 ) ) ;
#25723=ORIENTED_EDGE ( 'NONE', *, *, #32133, .T. ) ;
#25724=ORIENTED_EDGE ( 'NONE', *, *, #75129, .F. ) ;
#25725=CARTESIAN_POINT ( 'NONE',  ( -10.61538461538461320, -1.044019251281081972, 31.83374038241031911 ) ) ;
#25726=CARTESIAN_POINT ( 'NONE',  ( -14.08491276642389423, -12.44528174975671853, 30.48912976160716681 ) ) ;
#25727=CARTESIAN_POINT ( 'NONE',  ( 15.45378207486262667, -8.282913670948747864, 34.94150082978203642 ) ) ;
#25729=CARTESIAN_POINT ( 'NONE',  ( -1.134615384615383915, -2.499999999999998668, 29.75000000000000355 ) ) ;
#25731=ORIENTED_EDGE ( 'NONE', *, *, #34115, .F. ) ;
#25732=FACE_OUTER_BOUND ( 'NONE', #63445, .T. ) ;
#25733=B_SPLINE_CURVE_WITH_KNOTS ( 'NONE', 3,
 ( #76643, #7744, #35206, #56802, #56369, #14944, #9501, #42422, #28454, #69880 ),
 .UNSPECIFIED., .F., .F.,
 ( 4, 2, 2, 2, 4 ),
 ( 0.0007817246256747451124, 0.0009771112852218881168, 0.001172497944769031230, 0.001367884604316174126, 0.001563271263863317238 ),
 .UNSPECIFIED. ) ;
#25734=CARTESIAN_POINT ( 'NONE',  ( 0.5923302693632473970, -9.804649428959606894, 34.18742332936588468 ) ) ;
#25735=CARTESIAN_POINT ( 'NONE',  ( -14.30769230769230660, -8.120952969808772792, 34.71129190930000163 ) ) ;
#25736=CARTESIAN_POINT ( 'NONE',  ( -3.296039231325549768, -12.70778746994557551, 30.41441678777548319 ) ) ;
#25737=ORIENTED_EDGE ( 'NONE', *, *, #77903, .T. ) ;
#25738=AXIS2_PLACEMENT_3D ( 'NONE', #78892, #12223, #38359 ) ;
#25739=ORIENTED_EDGE ( 'NONE', *, *, #72524, .T. ) ;
#25741=EDGE_LOOP ( 'NONE', ( #79799, #24351 ) ) ;
#25742=CARTESIAN_POINT ( 'NONE',  ( 0.4615384615383396616, -10.90142922262034020, 33.41473453929536674 ) ) ;
#25743=CARTESIAN_POINT ( 'NONE',  ( -1.384615384615383471, -2.292212530054420494, 30.41441678777542634 ) ) ;
#25744=EDGE_CURVE ( 'NONE', #24853, #86068, #32549, .T. ) ;
#25745=ORIENTED_EDGE ( 'NONE', *, *, #56477, .F. ) ;
#25746=CARTESIAN_POINT ( 'NONE',  ( -4.153846153846152411, -2.708943851104267164, 35.45975837776705220 ) ) ;
#25747=CARTESIAN_POINT ( 'NONE',  ( -9.692307692307814193, -5.094484230521993062, 34.41647553114689373 ) ) ;
#25748=FACE_OUTER_BOUND ( 'NONE', #11435, .T. ) ;
#25749=CARTESIAN_POINT ( 'NONE',  ( 1.515140822849030844, -6.808710257144161559, 34.95449254468098843 ) ) ;
#25750=DIRECTION ( 'NONE',  ( -0.000000000000000000, -0.7660444431189791237, -0.6427876096865379196 ) ) ;
#25751=ORIENTED_EDGE ( 'NONE', *, *, #37573, .T. ) ;
#25752=EDGE_CURVE ( 'NONE', #26337, #69932, #48657, .T. ) ;
#25753=CARTESIAN_POINT ( 'NONE',  ( 0.2115152242454951537, -10.05641848906368097, 34.04755513067966177 ) ) ;
#25754=ORIENTED_EDGE ( 'NONE', *, *, #52717, .T. ) ;
#25756=CARTESIAN_POINT ( 'NONE',  ( -2.307692307692427391, -9.442884908241554243, 34.35708131394783038 ) ) ;
#25757=CARTESIAN_POINT ( 'NONE',  ( -2.307692307692305711, -12.48256725967547354, 35.29906147534542527 ) ) ;
#25758=CARTESIAN_POINT ( 'NONE',  ( -4.153846153846152411, -12.37446782046654192, 30.86335684631486131 ) ) ;
#25759=CARTESIAN_POINT ( 'NONE',  ( -3.930833309752758797, -4.762714258010880997, 34.23016756924214832 ) ) ;
#25760=CARTESIAN_POINT ( 'NONE',  ( -5.207613680033383652, -10.70098750199973203, 33.91152734681376302 ) ) ;
#25761=FACE_OUTER_BOUND ( 'NONE', #60918, .T. ) ;
#25762=EDGE_CURVE ( 'NONE', #28791, #17236, #7838, .T. ) ;
#25764=ORIENTED_EDGE ( 'NONE', *, *, #62187, .F. ) ;
#25765=CARTESIAN_POINT ( 'NONE',  ( 15.16468581981335184, -8.120952969808774569, 34.71129190930000163 ) ) ;
#25766=CARTESIAN_POINT ( 'NONE',  ( 7.596153846153845812, -7.566082377512564072, 35.00000000000000711 ) ) ;
#25767=ORIENTED_EDGE ( 'NONE', *, *, #39897, .T. ) ;
#25768=ORIENTED_EDGE ( 'NONE', *, *, #75516, .T. ) ;
#25769=CARTESIAN_POINT ( 'NONE',  ( 5.076923076922953193, -9.528491918059723176, 34.59228464037033035 ) ) ;
#25770=FACE_OUTER_BOUND ( 'NONE', #62987, .T. ) ;
#25771=B_SPLINE_CURVE_WITH_KNOTS ( 'NONE', 3,
 ( #80791, #52844, #41118, #12317, #60497, #32577, #74022, #73587, #18636, #11881 ),
 .UNSPECIFIED., .F., .F.,
 ( 4, 2, 2, 2, 4 ),
 ( 0.000000000000000000, 0.0001954339857564064715, 0.0003908679715128129430, 0.0005863019572692194144, 0.0007817359430256258859 ),
 .UNSPECIFIED. ) ;
#25772=DIRECTION ( 'NONE',  ( -0.000000000000000000, 0.8660254037844399289, -0.4999999999999980016 ) ) ;
#25773=FACE_OUTER_BOUND ( 'NONE', #9806, .T. ) ;
#25774=EDGE_CURVE ( 'NONE', #40198, #67006, #79668, .T. ) ;
#25775=FACE_OUTER_BOUND ( 'NONE', #22711, .T. ) ;
#25776=VECTOR ( 'NONE', #36296, 1000.000000000000000 ) ;
#25777=CARTESIAN_POINT ( 'NONE',  ( -3.230769230769229949, -1.629998284177014645, 34.34916445242399163 ) ) ;
#25778=VERTEX_POINT ( 'NONE', #66603 ) ;
#25779=CARTESIAN_POINT ( 'NONE',  ( 5.934729554039226862, -3.835265460703609186, 33.15142922261924241 ) ) ;
#25780=AXIS2_PLACEMENT_3D ( 'NONE', #65282, #16650, #71590 ) ;
#25781=LINE ( 'NONE', #73973, #11031 ) ;
#25782=CARTESIAN_POINT ( 'NONE',  ( -2.307692307692428724, -5.941354392335915335, 34.76329471203413846 ) ) ;
#25784=CARTESIAN_POINT ( 'NONE',  ( 12.21151523731700372, -2.588893531581426988, 31.60682220781847818 ) ) ;
#25786=EDGE_LOOP ( 'NONE', ( #79362, #67559, #58179, #29574 ) ) ;
#25787=CARTESIAN_POINT ( 'NONE',  ( -0.2387589202700525215, -2.847695495035523550, 31.58253572463339509 ) ) ;
#25789=CARTESIAN_POINT ( 'NONE',  ( -13.60749490135297179, -7.630690623152299956, 34.99857592706774057 ) ) ;
#25790=VERTEX_POINT ( 'NONE', #4906 ) ;
#25793=CARTESIAN_POINT ( 'NONE',  ( -11.47239318745910097, -12.37446782046654192, 30.86335684631486842 ) ) ;
#25794=CARTESIAN_POINT ( 'NONE',  ( -9.692307692307691624, -2.538708090699994813, 30.37095296980875503 ) ) ;
#25796=CARTESIAN_POINT ( 'NONE',  ( 3.361559671736185528, -2.845873456487966635, 32.17976146951972538 ) ) ;
#25798=VERTEX_POINT ( 'NONE', #85980 ) ;
#25799=FACE_BOUND ( 'NONE', #44162, .T. ) ;
#25800=ORIENTED_EDGE ( 'NONE', *, *, #52045, .F. ) ;
#25801=CARTESIAN_POINT ( 'NONE',  ( -2.438382910802612269, -2.494641256782728966, 31.33461815524612959 ) ) ;
#25803=B_SPLINE_CURVE_WITH_KNOTS ( 'NONE', 3,
 ( #72750, #52919, #4303, #58343, #71865, #10174, #37637, #18266, #10617, #31784 ),
 .UNSPECIFIED., .F., .F.,
 ( 4, 2, 2, 2, 4 ),
 ( 0.0007817246256747442451, 0.0009771112852218865989, 0.001172497944769029061, 0.001367884604316171523, 0.001563271263863313986 ),
 .UNSPECIFIED. ) ;
#25804=CARTESIAN_POINT ( 'NONE',  ( -10.39260494640654464, -10.23759521482555357, 34.22997729860117033 ) ) ;
#25805=CARTESIAN_POINT ( 'NONE',  ( -3.165623451437267200, -7.750023238201980469, 34.74374492549440419 ) ) ;
#25806=CARTESIAN_POINT ( 'NONE',  ( 7.846153846153723244, -12.51329471203414379, 31.30864560766407578 ) ) ;
#25808=CARTESIAN_POINT ( 'NONE',  ( -6.130147209438218781, -4.460286881179643004, 33.72017969459903242 ) ) ;
#25811=ORIENTED_EDGE ( 'NONE', *, *, #59251, .T. ) ;
#25812=ORIENTED_EDGE ( 'NONE', *, *, #55258, .F. ) ;
#25813=ORIENTED_EDGE ( 'NONE', *, *, #37876, .T. ) ;
#25814=EDGE_CURVE ( 'NONE', #62595, #66445, #49081, .T. ) ;
#25817=CARTESIAN_POINT ( 'NONE',  ( -10.39260507411620793, -11.41317474335729543, 32.86274602512330034 ) ) ;
#25818=CARTESIAN_POINT ( 'NONE',  ( 11.31497661389721010, -9.417330523894424488, 34.63758898049880486 ) ) ;
#25819=CARTESIAN_POINT ( 'NONE',  ( -4.153846153846152411, -8.973038597847269315, 34.52809138561121927 ) ) ;
#25820=EDGE_CURVE ( 'NONE', #79559, #13581, #31475, .T. ) ;
#25821=CARTESIAN_POINT ( 'NONE',  ( 5.076923076923075762, -11.35647404775217417, 33.31231777344666511 ) ) ;
#25822=CARTESIAN_POINT ( 'NONE',  ( 17.99999999999987566, -10.21337939537710326, 33.94971097300076224 ) ) ;
#25824=LINE ( 'NONE', #47407, #73859 ) ;
#25825=CARTESIAN_POINT ( 'NONE',  ( -4.826977558574935045, -4.336752205174647656, 33.62275283266504289 ) ) ;
#25826=CARTESIAN_POINT ( 'NONE',  ( 0.3962680155776847624, -3.300289026998414865, 32.46337939537583139 ) ) ;
#25827=ORIENTED_EDGE ( 'NONE', *, *, #37033, .F. ) ;
#25828=ORIENTED_EDGE ( 'NONE', *, *, #23928, .T. ) ;
#25829=VECTOR ( 'NONE', #65407, 1000.000000000000114 ) ;
#25830=ORIENTED_EDGE ( 'NONE', *, *, #37566, .F. ) ;
#25831=AXIS2_PLACEMENT_3D ( 'NONE', #71107, #16175, #44512 ) ;
#25832=CARTESIAN_POINT ( 'NONE',  ( -13.38461538461550759, -12.51329471203414379, 31.30864560766407578 ) ) ;
#25833=VERTEX_POINT ( 'NONE', #11206 ) ;
#25834=FACE_OUTER_BOUND ( 'NONE', #27256, .T. ) ;
#25835=DIRECTION ( 'NONE',  ( -0.000000000000000000, 0.5000000000000011102, -0.8660254037844380415 ) ) ;
#25836=AXIS2_PLACEMENT_3D ( 'NONE', #18577, #51888, #45590 ) ;
#25837=CARTESIAN_POINT ( 'NONE',  ( -0.4615384615384611200, -2.292212530054420494, 30.41441678777542634 ) ) ;
#25838=CARTESIAN_POINT ( 'NONE',  ( -15.36145983387954139, -9.929715669179220328, 34.40415004197138416 ) ) ;
#25839=FACE_BOUND ( 'NONE', #55018, .T. ) ;
#25840=ORIENTED_EDGE ( 'NONE', *, *, #78873, .F. ) ;
#25841=B_SPLINE_CURVE_WITH_KNOTS ( 'NONE', 3,
 ( #14514, #42885, #62686, #1447, #36564, #48740, #28937, #70351, #22164, #8210 ),
 .UNSPECIFIED., .F., .F.,
 ( 4, 2, 2, 2, 4 ),
 ( 0.0007817246256747463051, 0.0009771112852218896347, 0.001172497944769033181, 0.001367884604316176728, 0.001563271263863320057 ),
 .UNSPECIFIED. ) ;
#25842=ORIENTED_EDGE ( 'NONE', *, *, #43478, .F. ) ;
#25843=CARTESIAN_POINT ( 'NONE',  ( -8.769230769230460965, -2.506253911140614576, 30.00000000000323297 ) ) ;
#25844=ORIENTED_EDGE ( 'NONE', *, *, #26545, .T. ) ;
#25845=FACE_BOUND ( 'NONE', #22503, .T. ) ;
#25846=CARTESIAN_POINT ( 'NONE',  ( 7.596130608860880429, -11.86270091957321249, 32.19358267280087915 ) ) ;
#25847=CARTESIAN_POINT ( 'NONE',  ( -13.38461538461550582, -10.90142922262034020, 33.41473453929536674 ) ) ;
#25848=ORIENTED_EDGE ( 'NONE', *, *, #82307, .T. ) ;
#25849=CARTESIAN_POINT ( 'NONE',  ( -1.161835715637317801, -5.827830569534415694, 34.72679350104403539 ) ) ;
#25850=DIRECTION ( 'NONE',  ( 0.000000000000000000, 0.4999999999999960032, -0.8660254037844410391 ) ) ;
#25852=VERTEX_POINT ( 'NONE', #38677 ) ;
#25853=CARTESIAN_POINT ( 'NONE',  ( 14.37294744720514572, -3.643525952247864463, 33.31231777344670064 ) ) ;
#25854=FACE_OUTER_BOUND ( 'NONE', #30554, .T. ) ;
#25855=CARTESIAN_POINT ( 'NONE',  ( 2.373759641042384683, -2.833524468853757750, 32.15551576947925838 ) ) ;
#25857=DIRECTION ( 'NONE',  ( 0.000000000000000000, 0.9848077530122072432, -0.1736481776669354937 ) ) ;
#25858=CARTESIAN_POINT ( 'NONE',  ( 2.373759641042383794, -3.322132147404559976, 32.92929555188717927 ) ) ;
#25860=CARTESIAN_POINT ( 'NONE',  ( -12.52680846209478460, -5.941354392334499579, 34.76329471203369792 ) ) ;
#25861=CARTESIAN_POINT ( 'NONE',  ( -10.36543909703647337, -5.057305518903948638, 34.11320923018887896 ) ) ;
#25862=CARTESIAN_POINT ( 'NONE',  ( -22.75000000000000000, -7.500000000000000000, 32.75000000000000000 ) ) ;
#25863=CARTESIAN_POINT ( 'NONE',  ( -4.946131269098287930, -8.147973898785416225, 34.70805048591653730 ) ) ;
#25864=CARTESIAN_POINT ( 'NONE',  ( 8.769230769230768274, -1.129524287112498415, 32.06866353760679544 ) ) ;
#25865=LINE ( 'NONE', #53323, #29432 ) ;
#25866=CARTESIAN_POINT ( 'NONE',  ( 0.5276057948885370941, -11.35647404775217595, 33.31231777344667222 ) ) ;
#25867=CARTESIAN_POINT ( 'NONE',  ( 9.822833130541336999, -5.070358843744210198, 34.40418822224088302 ) ) ;
#25870=VECTOR ( 'NONE', #3028, 1000.000000000000000 ) ;
#25873=CARTESIAN_POINT ( 'NONE',  ( -3.930833309752757909, -5.582272713120727481, 34.63742843783360570 ) ) ;
#25874=VERTEX_POINT ( 'NONE', #66140 ) ;
#25875=ORIENTED_EDGE ( 'NONE', *, *, #18162, .T. ) ;
#25876=CARTESIAN_POINT ( 'NONE',  ( -7.846153846153844924, -2.486705287966279876, 31.30864560766543647 ) ) ;
#25877=EDGE_LOOP ( 'NONE', ( #21982, #49947 ) ) ;
#25878=CARTESIAN_POINT ( 'NONE',  ( 3.230769230769231726, -9.780366693483667717, 34.19971097300155094 ) ) ;
#25880=CARTESIAN_POINT ( 'NONE',  ( -13.31936024510254768, -5.941354392334607049, 34.76329471203374055 ) ) ;
#25881=CARTESIAN_POINT ( 'NONE',  ( -15.45369618967607828, -12.38737895849757820, 31.66785238281580206 ) ) ;
#25882=CARTESIAN_POINT ( 'NONE',  ( -2.980714919130915685, -9.148310452688873440, 34.47095581063188519 ) ) ;
#25883=CARTESIAN_POINT ( 'NONE',  ( -10.55012947587177941, -3.643525952247864463, 33.31231777344670064 ) ) ;
#25884=CARTESIAN_POINT ( 'NONE',  ( -13.45069879557126491, -2.538708090699994813, 30.37095296980875148 ) ) ;
#25885=CARTESIAN_POINT ( 'NONE',  ( -11.60373198442231590, -5.219633306516282545, 34.19971097300152962 ) ) ;
#25886=B_SPLINE_CURVE_WITH_KNOTS ( 'NONE', 3,
 ( #47408, #74905, #40678, #29379, #57277, #7767 ),
 .UNSPECIFIED., .F., .F.,
 ( 4, 2, 4 ),
 ( 0.2500000000000000000, 0.3750000652700731796, 0.5000001305401463592 ),
 .UNSPECIFIED. ) ;
#25888=B_SPLINE_CURVE_WITH_KNOTS ( 'NONE', 3,
 ( #45010, #52663, #73845, #79261, #58976, #39175 ),
 .UNSPECIFIED., .F., .F.,
 ( 4, 2, 4 ),
 ( 4.220987180333913997E-17, 0.0001954756301637163962, 0.0003909512603273906169 ),
 .UNSPECIFIED. ) ;
#25889=CARTESIAN_POINT ( 'NONE',  ( 18.00000000000000000, -11.35647404775217417, 33.31231777344666511 ) ) ;
#25890=CARTESIAN_POINT ( 'NONE',  ( 13.38461538461526423, -3.643525952248795718, 33.31231777344771672 ) ) ;
#25892=CARTESIAN_POINT ( 'NONE',  ( 18.06519398178335578, -2.506253911140448043, 29.99999999999988631 ) ) ;
#25895=ORIENTED_EDGE ( 'NONE', *, *, #77054, .T. ) ;
#25896=ORIENTED_EDGE ( 'NONE', *, *, #49450, .T. ) ;
#25897=CARTESIAN_POINT ( 'NONE',  ( -9.626239341305252495, -3.513871655860379306, 32.76840700105978499 ) ) ;
#25898=CARTESIAN_POINT ( 'NONE',  ( -14.30769230769242739, -8.613356846316285953, 34.62446782046622218 ) ) ;
#25899=CARTESIAN_POINT ( 'NONE',  ( 1.161130460051053914, -10.97335522853832579, 33.68706563782419749 ) ) ;
#25900=CARTESIAN_POINT ( 'NONE',  ( -6.066083410955879884, -3.513871655860377086, 32.76840700105978499 ) ) ;
#25901=CARTESIAN_POINT ( 'NONE',  ( 2.307692307692309264, -12.78798330534103123, 29.99999999999997868 ) ) ;
#25903=DIRECTION ( 'NONE',  ( -0.000000000000000000, 0.3420201433256694346, -0.9396926207859080948 ) ) ;
#25904=ADVANCED_FACE ( 'NONE', ( #37332 ), #47657, .F. ) ;
#25906=CARTESIAN_POINT ( 'NONE',  ( -6.700065571464073777, -9.886259254753566594, 34.14407573483972413 ) ) ;
#25907=ORIENTED_EDGE ( 'NONE', *, *, #6661, .T. ) ;
#25908=ORIENTED_EDGE ( 'NONE', *, *, #34843, .T. ) ;
#25909=CARTESIAN_POINT ( 'NONE',  ( -14.08472940413082242, -7.369474270740069777, 34.74850911626239736 ) ) ;
#25911=CARTESIAN_POINT ( 'NONE',  ( -4.284536756956459413, -12.62707690430377383, 30.88035979386743435 ) ) ;
#25912=CARTESIAN_POINT ( 'NONE',  ( 12.46153846153846168, -8.810774026931790459, 35.74407628777942847 ) ) ;
#25913=CARTESIAN_POINT ( 'NONE',  ( -2.084680956079456582, -11.76359900205217457, 32.36225158514719880 ) ) ;
#25914=ORIENTED_EDGE ( 'NONE', *, *, #8435, .T. ) ;
#25915=VERTEX_POINT ( 'NONE', #80573 ) ;
#25916=ADVANCED_FACE ( 'NONE', ( #73810 ), #20192, .F. ) ;
#25918=EDGE_LOOP ( 'NONE', ( #76511, #10110 ) ) ;
#25919=CARTESIAN_POINT ( 'NONE',  ( 4.153846153846032507, -6.026961402154118908, 34.52809138561165270 ) ) ;
#25920=CARTESIAN_POINT ( 'NONE',  ( 11.53846153846141576, -2.379036618888197729, 30.90682066428292885 ) ) ;
#25921=CARTESIAN_POINT ( 'NONE',  ( 4.284636594813107102, -3.338503747796866872, 32.95102852606553512 ) ) ;
#25922=CARTESIAN_POINT ( 'NONE',  ( 12.46153846153833911, -2.657715359629662544, 31.77849191805970364 ) ) ;
#25924=CARTESIAN_POINT ( 'NONE',  ( -15.23076923076935252, -2.657715359629662544, 31.77849191805970364 ) ) ;
#25926=ORIENTED_EDGE ( 'NONE', *, *, #86920, .F. ) ;
#25927=CARTESIAN_POINT ( 'NONE',  ( 4.853996118016224770, -10.01117774369187252, 34.36070679894347535 ) ) ;
#25928=CARTESIAN_POINT ( 'NONE',  ( -3.480792454990688789, -2.588893531581426544, 31.60682220781847818 ) ) ;
#25929=ORIENTED_EDGE ( 'NONE', *, *, #19636, .T. ) ;
#25930=CARTESIAN_POINT ( 'NONE',  ( 7.976945653978634532, -12.38066358083363738, 30.83685684665853444 ) ) ;
#25933=ORIENTED_EDGE ( 'NONE', *, *, #26926, .F. ) ;
#25935=DIRECTION ( 'NONE',  ( -0.000000000000000000, -0.1736481776669307198, -0.9848077530122080203 ) ) ;
#25936=VERTEX_POINT ( 'NONE', #62053 ) ;
#25937=CARTESIAN_POINT ( 'NONE',  ( 2.307692307692309264, -6.386643153685126251, 34.62446782046654192 ) ) ;
#25938=DIRECTION ( 'NONE',  ( 0.000000000000000000, 0.7660444431189822323, -0.6427876096865344779 ) ) ;
#25939=CARTESIAN_POINT ( 'NONE',  ( 7.780883845597526438, -4.320704448112771878, 33.92786785259540494 ) ) ;
#25940=CARTESIAN_POINT ( 'NONE',  ( -6.923076923076922462, -3.513871655860378418, 32.76840700105978499 ) ) ;
#25942=DIRECTION ( 'NONE',  ( 0.000000000000000000, 0.000000000000000000, 1.000000000000000000 ) ) ;
#25943=VERTEX_POINT ( 'NONE', #81012 ) ;
#25944=CARTESIAN_POINT ( 'NONE',  ( -8.769230769230768274, -13.87047571288749737, 32.06866353760679544 ) ) ;
#25946=CARTESIAN_POINT ( 'NONE',  ( -14.30769230769230660, -2.721908614388771852, 31.22303859784724978 ) ) ;
#25947=ORIENTED_EDGE ( 'NONE', *, *, #83557, .F. ) ;
#25948=AXIS2_PLACEMENT_3D ( 'NONE', #14766, #42244, #69699 ) ;
#25951=CARTESIAN_POINT ( 'NONE',  ( 14.37294744720514572, -10.33852847137154107, 34.16647553114620450 ) ) ;
#25953=CARTESIAN_POINT ( 'NONE',  ( 9.692307692307572609, -10.21337939537710326, 33.94971097300076224 ) ) ;
#25954=CARTESIAN_POINT ( 'NONE',  ( 10.61538461538449596, -11.94971097300221174, 32.03036669348237098 ) ) ;
#25955=FACE_BOUND ( 'NONE', #68483, .T. ) ;
#25956=CARTESIAN_POINT ( 'NONE',  ( 1.254005729411304060, -7.722926974430166069, 34.99546784045485737 ) ) ;
#25958=CARTESIAN_POINT ( 'NONE',  ( -3.230769230769351186, -10.90142922262034020, 33.41473453929536674 ) ) ;
#25959=CARTESIAN_POINT ( 'NONE',  ( -5.776988648387149539, -9.886259254753566594, 34.14407573483972413 ) ) ;
#25960=CARTESIAN_POINT ( 'NONE',  ( -2.241624974342230736, -8.164416787775445883, 34.95778746994558617 ) ) ;
#25961=CARTESIAN_POINT ( 'NONE',  ( 8.992243613324164997, -12.64618726649961289, 30.78989965857442712 ) ) ;
#25963=VERTEX_POINT ( 'NONE', #19743 ) ;
#25964=B_SPLINE_CURVE_WITH_KNOTS ( 'NONE', 3,
 ( #36205, #29005, #83948, #62316, #49699, #15483, #55567, #88946, #21343, #42954 ),
 .UNSPECIFIED., .F., .F.,
 ( 4, 2, 2, 2, 4 ),
 ( 0.000000000000000000, 0.0001954339857564054144, 0.0003908679715128108288, 0.0005863019572692162703, 0.0007817359430256216575 ),
 .UNSPECIFIED. ) ;
#25965=CARTESIAN_POINT ( 'NONE',  ( -12.59201364661418232, -7.276987145209185215, 34.99546412871779211 ) ) ;
#25966=EDGE_LOOP ( 'NONE', ( #2990, #438 ) ) ;
#25967=CARTESIAN_POINT ( 'NONE',  ( 8.769230769230768274, -4.098570777380720287, 33.41473453929634729 ) ) ;
#25968=ORIENTED_EDGE ( 'NONE', *, *, #2524, .F. ) ;
#25969=CARTESIAN_POINT ( 'NONE',  ( 2.177544337960613863, -2.373036134822904319, 30.88089517874952250 ) ) ;
#25971=CARTESIAN_POINT ( 'NONE',  ( -2.557669038634660996, -11.79746400365624659, 32.30657167506340954 ) ) ;
#25972=ORIENTED_EDGE ( 'NONE', *, *, #63206, .F. ) ;
#25973=CARTESIAN_POINT ( 'NONE',  ( -16.85391023282967637, -2.308499170217968466, 30.53291367094874076 ) ) ;
#25974=CARTESIAN_POINT ( 'NONE',  ( -20.99999999999999645, -10.75000000000000000, 29.75000000000000355 ) ) ;
#25976=EDGE_CURVE ( 'NONE', #16582, #75011, #63657, .T. ) ;
#25977=CARTESIAN_POINT ( 'NONE',  ( 14.30769230769231015, -10.51840700105979565, 33.73612834413961536 ) ) ;
#25979=CARTESIAN_POINT ( 'NONE',  ( -12.33101302330481808, -9.503571793651731880, 34.60286762892837942 ) ) ;
#25980=CYLINDRICAL_SURFACE ( 'NONE', #11370, 0.2500000000000002220 ) ;
#25981=CARTESIAN_POINT ( 'NONE',  ( 7.173022441425065843, -4.336752205174647656, 33.62275283266504289 ) ) ;
#25982=CARTESIAN_POINT ( 'NONE',  ( -11.31545018684868786, -9.886259254753566594, 34.14407573483972413 ) ) ;
#25983=EDGE_CURVE ( 'NONE', #37000, #33880, #88229, .T. ) ;
#25985=CARTESIAN_POINT ( 'NONE',  ( 14.30769230769231015, -5.557115091759785130, 34.35708131394839171 ) ) ;
#25986=FACE_OUTER_BOUND ( 'NONE', #59922, .T. ) ;
#25987=ORIENTED_EDGE ( 'NONE', *, *, #41749, .F. ) ;
#25988=CIRCLE ( 'NONE', #76318, 2.000000000000001776 ) ;
#25989=CARTESIAN_POINT ( 'NONE',  ( 17.29993442853592711, -2.758310577978207778, 31.33698337089302299 ) ) ;
#25990=CARTESIAN_POINT ( 'NONE',  ( 15.45354889974729318, -10.97394488606064122, 33.68653795673694873 ) ) ;
#25992=EDGE_CURVE ( 'NONE', #21493, #81662, #79312, .T. ) ;
#25993=CARTESIAN_POINT ( 'NONE',  ( 2.177000841024752109, -4.118384482072085184, 33.43331474514187107 ) ) ;
#25994=CARTESIAN_POINT ( 'NONE',  ( 5.142990410273149848, -6.343179335718452272, 34.87096338111212646 ) ) ;
#25995=ORIENTED_EDGE ( 'NONE', *, *, #64136, .T. ) ;
#25996=CARTESIAN_POINT ( 'NONE',  ( 7.053868730901711182, -8.147973898785416225, 34.70805048591653730 ) ) ;
#25997=CARTESIAN_POINT ( 'NONE',  ( -12.33101302330481808, -12.70449254468099198, 30.44128974285582956 ) ) ;
#25998=CARTESIAN_POINT ( 'NONE',  ( 8.899756207464410096, -2.647132371071621471, 31.75357179365171589 ) ) ;
#26000=CARTESIAN_POINT ( 'NONE',  ( -1.384615384615383471, -6.386643153685126251, 34.62446782046654192 ) ) ;
#26001=CARTESIAN_POINT ( 'NONE',  ( 4.153846153846032507, -8.613356846316285953, 34.62446782046622218 ) ) ;
#26002=EDGE_CURVE ( 'NONE', #8955, #60703, #54857, .T. ) ;
#26003=CARTESIAN_POINT ( 'NONE',  ( -15.00798956179116317, -12.11081565061824250, 32.26097654155340422 ) ) ;
#26004=CARTESIAN_POINT ( 'NONE',  ( -15.90384615384473399, -7.500000000000154543, 35.00000000000007105 ) ) ;
#26005=EDGE_LOOP ( 'NONE', ( #78744, #22462 ) ) ;
#26006=CARTESIAN_POINT ( 'NONE',  ( 7.173076923076923350, -2.249999999999998668, 29.75000000000000355 ) ) ;
#26007=CARTESIAN_POINT ( 'NONE',  ( -18.06527044596078113, -12.27809138561121394, 31.22303859784730307 ) ) ;
#26008=B_SPLINE_CURVE_WITH_KNOTS ( 'NONE', 3,
 ( #69926, #50088, #70823, #8236, #69483, #28962, #14098, #36590, #56416, #64042 ),
 .UNSPECIFIED., .F., .F.,
 ( 4, 2, 2, 2, 4 ),
 ( 0.0007817359430256392216, 0.0009771253907250073822, 0.001172514838424375651, 0.001367904286123743920, 0.001563293733823112189 ),
 .UNSPECIFIED. ) ;
#26010=DIRECTION ( 'NONE',  ( -0.000000000000000000, -0.1736481776669307198, -0.9848077530122080203 ) ) ;
#26011=EDGE_CURVE ( 'NONE', #70591, #22567, #5758, .T. ) ;
#26012=VERTEX_POINT ( 'NONE', #74247 ) ;
#26013=ORIENTED_EDGE ( 'NONE', *, *, #77736, .T. ) ;
#26014=B_SPLINE_CURVE_WITH_KNOTS ( 'NONE', 3,
 ( #3341, #72243, #78554, #31718, #10554, #64585, #71350, #24497, #43448, #36693 ),
 .UNSPECIFIED., .F., .F.,
 ( 4, 2, 2, 2, 4 ),
 ( 0.000000000000000000, 0.0001954311564186868744, 0.0003908623128373737488, 0.0005862934692560606504, 0.0007817246256747474977 ),
 .UNSPECIFIED. ) ;
#26017=VECTOR ( 'NONE', #26512, 1000.000000000000227 ) ;
#26018=CARTESIAN_POINT ( 'NONE',  ( 12.46153846153846168, -9.905515769479276145, 34.41647553114623292 ) ) ;
#26019=CARTESIAN_POINT ( 'NONE',  ( 6.923076923076802558, -3.835265460704628371, 33.15142922262033665 ) ) ;
#26021=VECTOR ( 'NONE', #60955, 1000.000000000000000 ) ;
#26022=VECTOR ( 'NONE', #30131, 1000.000000000000114 ) ;
#26023=CARTESIAN_POINT ( 'NONE',  ( -17.74999999999992895, -7.434744429011174383, 34.75000000000000711 ) ) ;
#26024=VERTEX_POINT ( 'NONE', #67492 ) ;
#26025=EDGE_CURVE ( 'NONE', #673, #76455, #70022, .T. ) ;
#26026=ORIENTED_EDGE ( 'NONE', *, *, #77535, .F. ) ;
#26027=ORIENTED_EDGE ( 'NONE', *, *, #67301, .F. ) ;
#26028=CARTESIAN_POINT ( 'NONE',  ( -7.053767526187231240, -8.191372820521381826, 34.95448215188423546 ) ) ;
#26029=EDGE_CURVE ( 'NONE', #6055, #10508, #78638, .T. ) ;
#26030=ORIENTED_EDGE ( 'NONE', *, *, #76216, .T. ) ;
#26031=CARTESIAN_POINT ( 'NONE',  ( -9.692307692307691624, -9.905515769479276145, 34.41647553114623292 ) ) ;
#26032=DIRECTION ( 'NONE',  ( -0.000000000000000000, 1.000000000000000000, 3.491481338843133355E-15 ) ) ;
#26034=EDGE_CURVE ( 'NONE', #11784, #20954, #85036, .T. ) ;
#26035=CARTESIAN_POINT ( 'NONE',  ( 6.989144256427000990, -4.661471528628508665, 34.16647553114624003 ) ) ;
#26037=ORIENTED_EDGE ( 'NONE', *, *, #55742, .T. ) ;
#26038=ORIENTED_EDGE ( 'NONE', *, *, #63665, .T. ) ;
#26039=B_SPLINE_CURVE_WITH_KNOTS ( 'NONE', 3,
 ( #67163, #13106, #38804, #39254, #80235, #74813, #32934, #46440, #19857, #47321 ),
 .UNSPECIFIED., .F., .F.,
 ( 4, 2, 2, 2, 4 ),
 ( 0.0007817359430256293554, 0.0009771253907249941549, 0.001172514838424358954, 0.001367904286123723537, 0.001563293733823095276 ),
 .UNSPECIFIED. ) ;
#26040=VERTEX_POINT ( 'NONE', #69260 ) ;
#26041=CARTESIAN_POINT ( 'NONE',  ( -18.00000000000000000, -9.815202283848471154, 36.11096599634342397 ) ) ;
#26043=ORIENTED_EDGE ( 'NONE', *, *, #24182, .T. ) ;
#26044=B_SPLINE_CURVE_WITH_KNOTS ( 'NONE', 3,
 ( #42545, #1996, #29477, #70902, #9208, #29040, #29918, #36670, #35334, #49732 ),
 .UNSPECIFIED., .F., .F.,
 ( 4, 2, 2, 2, 4 ),
 ( 0.0007817246256747470640, 0.0009771112852218902852, 0.001172497944769033398, 0.001367884604316176728, 0.001563271263863319840 ),
 .UNSPECIFIED. ) ;
#26045=CARTESIAN_POINT ( 'NONE',  ( 3.230769230769231726, -11.69971097300155272, 32.46337939537588113 ) ) ;
#26049=AXIS2_PLACEMENT_3D ( 'NONE', #33917, #82118, #62269 ) ;
#26052=FACE_BOUND ( 'NONE', #34161, .T. ) ;
#26053=CARTESIAN_POINT ( 'NONE',  ( -0.7115616988314271696, -10.05641848906368097, 34.04755513067966177 ) ) ;
#26054=CARTESIAN_POINT ( 'NONE',  ( -1.319359813339359588, -11.94971097300157403, 32.03036669348361443 ) ) ;
#26055=CARTESIAN_POINT ( 'NONE',  ( -10.39260494640654819, -10.97394488606064122, 33.68653795673694873 ) ) ;
#26056=CARTESIAN_POINT ( 'NONE',  ( 0.2115152373170034461, -6.652501968072650484, 34.93155406624983783 ) ) ;
#26057=CARTESIAN_POINT ( 'NONE',  ( -5.300408020647025431, -3.236172620538810385, 32.36188796281390267 ) ) ;
#26059=CARTESIAN_POINT ( 'NONE',  ( 7.173076923076923350, -2.499999999999998668, 29.75000000000000355 ) ) ;
#26060=ORIENTED_EDGE ( 'NONE', *, *, #85279, .F. ) ;
#26061=CARTESIAN_POINT ( 'NONE',  ( 11.31553532094538994, -3.105860786376062332, 32.13614157043599562 ) ) ;
#26062=CARTESIAN_POINT ( 'NONE',  ( -13.63463860883683942, -9.356822207818506598, 34.66110646841856635 ) ) ;
#26063=ORIENTED_EDGE ( 'NONE', *, *, #12287, .T. ) ;
#26065=CARTESIAN_POINT ( 'NONE',  ( 5.076923076923075762, -3.937682226553329556, 33.60647404775216529 ) ) ;
#26066=CARTESIAN_POINT ( 'NONE',  ( -4.153846153846152411, -2.249999999999998668, 29.50000000000001421 ) ) ;
#26067=CARTESIAN_POINT ( 'NONE',  ( -15.23076923076935252, -9.528491918059723176, 34.59228464037033035 ) ) ;
#26068=EDGE_LOOP ( 'NONE', ( #5569, #18104, #82319, #79839 ) ) ;
#26069=EDGE_CURVE ( 'NONE', #5237, #52906, #60297, .T. ) ;
#26071=CARTESIAN_POINT ( 'NONE',  ( -7.146561866800873020, -10.11188796281391511, 34.01382737946119050 ) ) ;
#26072=CARTESIAN_POINT ( 'NONE',  ( 15.23076923076923173, -2.833524468853757305, 32.15551576947925838 ) ) ;
#26075=VECTOR ( 'NONE', #43801, 1000.000000000000227 ) ;
#26076=DIRECTION ( 'NONE',  ( -0.000000000000000000, -0.3420201433256694901, -0.9396926207859082059 ) ) ;
#26077=CARTESIAN_POINT ( 'NONE',  ( 2.242422307135989001, -11.06231777344662781, 33.60647404775220082 ) ) ;
#26080=ORIENTED_EDGE ( 'NONE', *, *, #50996, .T. ) ;
#26081=CARTESIAN_POINT ( 'NONE',  ( -9.822998295417995962, -2.494641256782728966, 31.33461815524612959 ) ) ;
#26082=CARTESIAN_POINT ( 'NONE',  ( -17.93393266664992325, -3.322132147404559088, 32.92929555188717217 ) ) ;
#26083=CYLINDRICAL_SURFACE ( 'NONE', #60354, 0.2499999999999986955 ) ;
#26084=CARTESIAN_POINT ( 'NONE',  ( -17.07692307692319744, -11.48612834414049644, 32.76840700105863391 ) ) ;
#26085=CYLINDRICAL_SURFACE ( 'NONE', #32774, 0.2500000000000012212 ) ;
#26087=EDGE_CURVE ( 'NONE', #26451, #79311, #81859, .T. ) ;
#26088=EDGE_CURVE ( 'NONE', #59796, #29766, #83222, .T. ) ;
#26089=CARTESIAN_POINT ( 'NONE',  ( 0.5266842408704249801, -7.750023238201980469, 34.74374492549440419 ) ) ;
#26090=CARTESIAN_POINT ( 'NONE',  ( -13.38461538461550582, -8.613356846316285953, 34.62446782046622218 ) ) ;
#26091=CARTESIAN_POINT ( 'NONE',  ( 17.07692307692307665, -13.57706302396349152, 30.56769352161908060 ) ) ;
#26092=CARTESIAN_POINT ( 'NONE',  ( 16.15384615384603251, -12.70778746994576025, 30.41441678777401236 ) ) ;
#26094=CARTESIAN_POINT ( 'NONE',  ( 8.769230769230647482, -12.27809138561165270, 31.22303859784587132 ) ) ;
#26095=B_SPLINE_CURVE_WITH_KNOTS ( 'NONE', 3,
 ( #24154, #78214, #58374, #36791, #23705, #29600, #50285, #16515, #2548, #58829 ),
 .UNSPECIFIED., .F., .F.,
 ( 4, 2, 2, 2, 4 ),
 ( 0.0007817359430256294638, 0.0009771253907249950223, 0.001172514838424360472, 0.001367904286123725922, 0.001563293733823091372 ),
 .UNSPECIFIED. ) ;
#26096=CARTESIAN_POINT ( 'NONE',  ( -12.71153846153846168, -7.500000000000001776, 35.00000000000000000 ) ) ;
#26097=CARTESIAN_POINT ( 'NONE',  ( 6.923076923076924238, -4.661471528628507777, 34.16647553114623292 ) ) ;
#26098=CARTESIAN_POINT ( 'NONE',  ( -6.923076923076922462, -3.322132147404559976, 32.92929555188717927 ) ) ;
#26099=CARTESIAN_POINT ( 'NONE',  ( -16.82697766754503377, -2.986452184633680229, 32.43230066228895225 ) ) ;
#26100=EDGE_LOOP ( 'NONE', ( #34362, #65670, #52825, #5437 ) ) ;
#26101=CARTESIAN_POINT ( 'NONE',  ( -16.15384615384627409, -11.94971097300221174, 32.03036669348237098 ) ) ;
#26102=CARTESIAN_POINT ( 'NONE',  ( -3.230769230769351186, -3.835265460704628371, 33.15142922262033665 ) ) ;
#26105=CARTESIAN_POINT ( 'NONE',  ( 5.207448515156721136, -10.31582465632705237, 34.18122507451815295 ) ) ;
#26106=CARTESIAN_POINT ( 'NONE',  ( 10.48469314871705649, -5.582088688514999397, 34.36776431015576350 ) ) ;
#26107=CARTESIAN_POINT ( 'NONE',  ( 5.299935921016470708, -4.026326845037961455, 33.68677907613344047 ) ) ;
#26108=ORIENTED_EDGE ( 'NONE', *, *, #18921, .F. ) ;
#26110=CARTESIAN_POINT ( 'NONE',  ( 18.00000000000000000, -11.69971097300155272, 32.46337939537588113 ) ) ;
#26111=ADVANCED_FACE ( 'NONE', ( #28719 ), #29605, .F. ) ;
#26112=EDGE_LOOP ( 'NONE', ( #21517, #6217, #52275, #23253 ) ) ;
#26113=CARTESIAN_POINT ( 'NONE',  ( 8.639083559792549494, -8.587444163452046197, 34.63053765926554206 ) ) ;
#26115=VERTEX_POINT ( 'NONE', #8891 ) ;
#26116=AXIS2_PLACEMENT_3D ( 'NONE', #64465, #3222, #79336 ) ;
#26117=DIRECTION ( 'NONE',  ( -0.000000000000000000, -0.9848077530122085754, -0.1736481776669273613 ) ) ;
#26118=CARTESIAN_POINT ( 'NONE',  ( -9.692307692307691624, -2.721908614388771852, 31.22303859784724978 ) ) ;
#26119=CARTESIAN_POINT ( 'NONE',  ( -7.911424292114618950, -3.835265460703609186, 33.15142922261924241 ) ) ;
#26120=EDGE_CURVE ( 'NONE', #41328, #4532, #36687, .T. ) ;
#26122=EDGE_LOOP ( 'NONE', ( #22558, #86043, #35527, #36031 ) ) ;
#26123=EDGE_LOOP ( 'NONE', ( #27495, #52754, #1656, #22234 ) ) ;
#26125=CARTESIAN_POINT ( 'NONE',  ( 12.21156173059610772, -12.41269422305637171, 30.68257228309993323 ) ) ;
#26126=CARTESIAN_POINT ( 'NONE',  ( -9.627052121031669074, -10.21337939537593620, 33.94971097300152252 ) ) ;
#26127=CARTESIAN_POINT ( 'NONE',  ( -8.096153846153844924, -7.500000000000001776, 35.04278698407183867 ) ) ;
#26129=CARTESIAN_POINT ( 'NONE',  ( -15.23076923076922995, -12.29105614889573062, 35.45975837776705220 ) ) ;
#26130=CARTESIAN_POINT ( 'NONE',  ( 9.692307692307695177, -9.905515769479276145, 34.41647553114623292 ) ) ;
#26131=CARTESIAN_POINT ( 'NONE',  ( 11.31553532094538994, -11.76352882383564769, 32.36236540154569497 ) ) ;
#26133=EDGE_CURVE ( 'NONE', #27372, #72596, #33520, .T. ) ;
#26134=ORIENTED_EDGE ( 'NONE', *, *, #62462, .F. ) ;
#26135=EDGE_LOOP ( 'NONE', ( #24144, #26043 ) ) ;
#26137=CARTESIAN_POINT ( 'NONE',  ( 18.06525513951284267, -9.528491918058456633, 34.59228464037085615 ) ) ;
#26138=EDGE_LOOP ( 'NONE', ( #47296, #38650 ) ) ;
#26139=B_SPLINE_CURVE_WITH_KNOTS ( 'NONE', 3,
 ( #54815, #48493, #62881, #72312, #29133, #2080, #17376, #56589, #10620, #78626 ),
 .UNSPECIFIED., .F., .F.,
 ( 4, 2, 2, 2, 4 ),
 ( 0.000000000000000000, 0.0001954339857564070949, 0.0003908679715128141898, 0.0005863019572692212576, 0.0007817359430256283796 ),
 .UNSPECIFIED. ) ;
#26140=ADVANCED_FACE ( 'NONE', ( #16969 ), #86788, .F. ) ;
#26141=AXIS2_PLACEMENT_3D ( 'NONE', #66493, #4795, #59731 ) ;
#26142=EDGE_CURVE ( 'NONE', #7620, #63664, #3446, .T. ) ;
#26143=CARTESIAN_POINT ( 'NONE',  ( 10.39251835232151677, -2.251424796025574881, 29.88072029997477230 ) ) ;
#26144=PLANE ( 'NONE',  #35261 ) ;
#26145=EDGE_LOOP ( 'NONE', ( #31601, #18861, #50000, #8322 ) ) ;
#26146=CARTESIAN_POINT ( 'NONE',  ( -14.17716660592874689, -4.459921816937791661, 33.71989282347011851 ) ) ;
#26147=CIRCLE ( 'NONE', #62145, 0.2500000000000002220 ) ;
#26149=CARTESIAN_POINT ( 'NONE',  ( -10.86540785267757947, -3.202444869320336451, 32.30641848906366675 ) ) ;
#26150=ORIENTED_EDGE ( 'NONE', *, *, #19206, .F. ) ;
#26152=CARTESIAN_POINT ( 'NONE',  ( -12.23852561744506851, -10.01129605718032600, 34.36064277460058491 ) ) ;
#26153=ADVANCED_FACE ( 'NONE', ( #30912 ), #52075, .F. ) ;
#26154=CARTESIAN_POINT ( 'NONE',  ( -16.02332071561251325, -11.04252011169590020, 33.62494198852677840 ) ) ;
#26155=FACE_BOUND ( 'NONE', #20320, .T. ) ;
#26156=DIRECTION ( 'NONE',  ( 0.000000000000000000, 0.9848077530122072432, -0.1736481776669354937 ) ) ;
#26158=CYLINDRICAL_SURFACE ( 'NONE', #16543, 0.2499999999999986955 ) ;
#26161=CARTESIAN_POINT ( 'NONE',  ( -4.153846153846152411, -8.564572088678739092, 35.78748833219616898 ) ) ;
#26162=CARTESIAN_POINT ( 'NONE',  ( -7.976301815885543434, -9.504002272028875709, 34.60269587691767867 ) ) ;
#26163=DIRECTION ( 'NONE',  ( 0.000000000000000000, 0.1736481776669267785, -0.9848077530122087975 ) ) ;
#26165=ORIENTED_EDGE ( 'NONE', *, *, #42475, .F. ) ;
#26166=CYLINDRICAL_SURFACE ( 'NONE', #51829, 0.2499999999999994726 ) ;
#26167=CARTESIAN_POINT ( 'NONE',  ( -14.30769230769242739, -12.46129190930018460, 30.37095296980731973 ) ) ;
#26169=CYLINDRICAL_SURFACE ( 'NONE', #41355, 0.2500000000000009437 ) ;
#26170=CARTESIAN_POINT ( 'NONE',  ( -0.4615384615384611200, -10.67929555188718282, 33.92786785259544047 ) ) ;
#26171=CARTESIAN_POINT ( 'NONE',  ( -17.07692307692319744, -12.51329471203414379, 31.30864560766407578 ) ) ;
#26172=LINE ( 'NONE', #40585, #14498 ) ;
#26173=ORIENTED_EDGE ( 'NONE', *, *, #34213, .T. ) ;
#26175=CARTESIAN_POINT ( 'NONE',  ( 17.29970261819148902, -3.236590943229497697, 32.36255958852954251 ) ) ;
#26177=CARTESIAN_POINT ( 'NONE',  ( -14.43783951713053249, -8.587444163452046197, 34.63053765926554206 ) ) ;
#26178=CARTESIAN_POINT ( 'NONE',  ( -13.38461538461538325, -13.87047571288749737, 32.06866353760679544 ) ) ;
#26179=VECTOR ( 'NONE', #64415, 1000.000000000000227 ) ;
#26180=ORIENTED_EDGE ( 'NONE', *, *, #53256, .T. ) ;
#26181=EDGE_CURVE ( 'NONE', #77080, #66348, #66857, .T. ) ;
#26182=ORIENTED_EDGE ( 'NONE', *, *, #57342, .F. ) ;
#26184=ORIENTED_EDGE ( 'NONE', *, *, #69232, .F. ) ;
#26185=EDGE_CURVE ( 'NONE', #8424, #6380, #76414, .T. ) ;
#26186=CARTESIAN_POINT ( 'NONE',  ( 0.2115384615384615918, -7.433931650972300353, 34.75000000000000711 ) ) ;
#26188=ORIENTED_EDGE ( 'NONE', *, *, #3817, .T. ) ;
#26190=CARTESIAN_POINT ( 'NONE',  ( -5.076923076923075762, -1.951392089020283160, 34.73218667398347748 ) ) ;
#26191=CARTESIAN_POINT ( 'NONE',  ( 4.826899839630109490, -6.695914987888143877, 34.68535235679833306 ) ) ;
#26192=CARTESIAN_POINT ( 'NONE',  ( 1.607628228708781748, -6.460100341425561332, 34.89618726649961644 ) ) ;
#26193=ADVANCED_FACE ( 'NONE', ( #4341 ), #45318, .F. ) ;
#26195=VERTEX_POINT ( 'NONE', #78667 ) ;
#26196=DIRECTION ( 'NONE',  ( 0.000000000000000000, 0.3420201433256671586, 0.9396926207859089830 ) ) ;
#26198=DIRECTION ( 'NONE',  ( -0.000000000000000000, -0.000000000000000000, -1.000000000000000000 ) ) ;
#26199=DIRECTION ( 'NONE',  ( 0.000000000000000000, 0.7660444431189807890, 0.6427876096865361433 ) ) ;
#26200=CARTESIAN_POINT ( 'NONE',  ( 17.07692307692307665, -5.180354513474913603, 36.12317359536750416 ) ) ;
#26201=CARTESIAN_POINT ( 'NONE',  ( 11.66925197942848769, -9.929761469519743144, 34.40412654351204225 ) ) ;
#26202=CARTESIAN_POINT ( 'NONE',  ( -5.934807011705343527, -2.255955759149235629, 29.99999999999988631 ) ) ;
#26203=CARTESIAN_POINT ( 'NONE',  ( -0.4615384615384611200, -12.37446782046654192, 30.86335684631486131 ) ) ;
#26206=CARTESIAN_POINT ( 'NONE',  ( -6.923076923077045919, -11.06231777344772027, 33.60647404775119895 ) ) ;
#26207=CARTESIAN_POINT ( 'NONE',  ( 2.438217745925953750, -4.299079248970732792, 33.91157788607253565 ) ) ;
#26209=VECTOR ( 'NONE', #86416, 1000.000000000000227 ) ;
#26210=CARTESIAN_POINT ( 'NONE',  ( 6.923076923076802558, -6.879047030192662504, 34.71129190930017927 ) ) ;
#26211=ORIENTED_EDGE ( 'NONE', *, *, #38397, .F. ) ;
#26212=CARTESIAN_POINT ( 'NONE',  ( 8.069166690247241647, -11.98016756924214832, 32.48728574198911190 ) ) ;
#26213=CARTESIAN_POINT ( 'NONE',  ( 11.40831356872984514, -12.70455904226513866, 30.44083106164009322 ) ) ;
#26214=EDGE_CURVE ( 'NONE', #60841, #49648, #58223, .T. ) ;
#26215=VECTOR ( 'NONE', #53364, 1000.000000000000000 ) ;
#26216=B_SPLINE_CURVE_WITH_KNOTS ( 'NONE', 3,
 ( #67707, #88444, #39361, #26715, #5118, #54617, #39799, #19952, #32583, #25837 ),
 .UNSPECIFIED., .F., .F.,
 ( 4, 2, 2, 2, 4 ),
 ( 0.0007817246256747517261, 0.0009771112852218963567, 0.001172497944769040987, 0.001367884604316185618, 0.001563271263863330249 ),
 .UNSPECIFIED. ) ;
#26217=DIRECTION ( 'NONE',  ( -0.000000000000000000, 0.6427876096865404731, -0.7660444431189771253 ) ) ;
#26218=CARTESIAN_POINT ( 'NONE',  ( -6.923076923076922462, -13.75783147151868846, 33.36296068462461051 ) ) ;
#26219=B_SPLINE_CURVE_WITH_KNOTS ( 'NONE', 3,
 ( #51928, #52823, #2851, #24460, #37529, #3751, #64997, #78969, #65889, #31221 ),
 .UNSPECIFIED., .F., .F.,
 ( 4, 2, 2, 2, 4 ),
 ( 0.000000000000000000, 0.0001954339857564097241, 0.0003908679715128194482, 0.0005863019572692291723, 0.0007817359430256388964 ),
 .UNSPECIFIED. ) ;
#26220=DIRECTION ( 'NONE',  ( 0.000000000000000000, 0.8660254037844377084, -0.5000000000000015543 ) ) ;
#26221=ORIENTED_EDGE ( 'NONE', *, *, #34619, .F. ) ;
#26222=B_SPLINE_CURVE_WITH_KNOTS ( 'NONE', 3,
 ( #64352, #37327, #2649, #23371, #78315, #64793, #85531, #23806, #51258, #58935 ),
 .UNSPECIFIED., .F., .F.,
 ( 4, 2, 2, 2, 4 ),
 ( 0.000000000000000000, 0.0001954311564186879044, 0.0003908623128373758088, 0.0005862934692560636861, 0.0007817246256747516176 ),
 .UNSPECIFIED. ) ;
#26223=CARTESIAN_POINT ( 'NONE',  ( 9.626224281351813516, -10.51840700105979387, 33.73612834413961536 ) ) ;
#26224=DIRECTION ( 'NONE',  ( -0.000000000000000000, -0.1736481776669307198, -0.9848077530122080203 ) ) ;
#26225=CARTESIAN_POINT ( 'NONE',  ( -3.361460697436787992, -11.71456829005830080, 32.44064028649416542 ) ) ;
#26226=ORIENTED_EDGE ( 'NONE', *, *, #83157, .F. ) ;
#26228=VERTEX_POINT ( 'NONE', #60165 ) ;
#26229=DIRECTION ( 'NONE',  ( 0.000000000000000000, 0.9396926207859126468, -0.3420201433256571111 ) ) ;
#26231=DIRECTION ( 'NONE',  ( 0.000000000000000000, 1.000000000000000000, -0.000000000000000000 ) ) ;
#26232=ORIENTED_EDGE ( 'NONE', *, *, #32935, .T. ) ;
#26233=CARTESIAN_POINT ( 'NONE',  ( 12.21151522424549718, -3.711651800289232028, 33.01384336483936011 ) ) ;
#26234=CARTESIAN_POINT ( 'NONE',  ( -14.30769230769199218, -2.255955759149395501, 30.00000000000324363 ) ) ;
#26235=DIRECTION ( 'NONE',  ( -0.000000000000000000, -0.7660444431189791237, -0.6427876096865379196 ) ) ;
#26237=CARTESIAN_POINT ( 'NONE',  ( 7.146089767170317408, -12.38742843783360748, 31.66772728687926985 ) ) ;
#26238=CARTESIAN_POINT ( 'NONE',  ( -5.076923076923075762, -9.819645486525091727, 36.12317359536749706 ) ) ;
#26239=EDGE_LOOP ( 'NONE', ( #18307, #55051 ) ) ;
#26240=CARTESIAN_POINT ( 'NONE',  ( -14.30769230769242739, -2.892918686052166066, 31.69288490824153470 ) ) ;
#26241=ORIENTED_EDGE ( 'NONE', *, *, #75681, .T. ) ;
#26242=CARTESIAN_POINT ( 'NONE',  ( -2.530619266599153150, -2.523278758544489353, 31.42238647778637528 ) ) ;
#26243=CARTESIAN_POINT ( 'NONE',  ( -10.54931728203453822, -9.905515769479276145, 34.41647553114623292 ) ) ;
#26244=EDGE_CURVE ( 'NONE', #88864, #25231, #73706, .T. ) ;
#26245=B_SPLINE_CURVE_WITH_KNOTS ( 'NONE', 3,
 ( #32546, #19041, #88409, #66338, #46512, #67236, #68122, #73993, #73555, #24898 ),
 .UNSPECIFIED., .F., .F.,
 ( 4, 2, 2, 2, 4 ),
 ( 0.0007817246256747519429, 0.0009771112852218970073, 0.001172497944769042288, 0.001367884604316187353, 0.001563271263863332417 ),
 .UNSPECIFIED. ) ;
#26246=CARTESIAN_POINT ( 'NONE',  ( 5.011652630962299959, -11.94971097300153140, 32.03036669348370680 ) ) ;
#26247=EDGE_CURVE ( 'NONE', #61129, #78712, #80458, .T. ) ;
#26249=DIRECTION ( 'NONE',  ( 0.000000000000000000, -6.938893903907222067E-15, 1.000000000000000000 ) ) ;
#26250=ORIENTED_EDGE ( 'NONE', *, *, #7982, .T. ) ;
#26251=ORIENTED_EDGE ( 'NONE', *, *, #9085, .F. ) ;
#26252=EDGE_CURVE ( 'NONE', #81813, #35413, #67822, .T. ) ;
#26253=ORIENTED_EDGE ( 'NONE', *, *, #1894, .T. ) ;
#26254=EDGE_LOOP ( 'NONE', ( #69238, #79070, #57196, #59788 ) ) ;
#26255=CARTESIAN_POINT ( 'NONE',  ( 2.307692307692187583, -5.219633306517616589, 34.19971097300220464 ) ) ;
#26256=CARTESIAN_POINT ( 'NONE',  ( 4.376858997939548246, -10.01129605718032778, 34.36064277460058491 ) ) ;
#26257=EDGE_CURVE ( 'NONE', #51846, #38427, #7432, .T. ) ;
#26258=CARTESIAN_POINT ( 'NONE',  ( -15.45425417449318317, -10.81261337010820256, 33.49550067578627477 ) ) ;
#26259=CARTESIAN_POINT ( 'NONE',  ( -8.069080805060693251, -3.395401636524185474, 33.02366814457250399 ) ) ;
#26260=AXIS2_PLACEMENT_3D ( 'NONE', #46476, #12691, #73955 ) ;
#26262=VECTOR ( 'NONE', #51809, 999.9999999999998863 ) ;
#26263=DIRECTION ( 'NONE',  ( 0.000000000000000000, 0.9848077530122072432, -0.1736481776669354937 ) ) ;
#26264=CARTESIAN_POINT ( 'NONE',  ( -2.176900499867520100, -3.530189275343204702, 32.79018710029569661 ) ) ;
#26265=CARTESIAN_POINT ( 'NONE',  ( 17.14299142792552288, -2.538708090699994813, 30.37095296980875503 ) ) ;
#26266=ORIENTED_EDGE ( 'NONE', *, *, #27598, .F. ) ;
#26267=ORIENTED_EDGE ( 'NONE', *, *, #31657, .F. ) ;
#26269=EDGE_LOOP ( 'NONE', ( #47499, #44506, #4201, #51858 ) ) ;
#26270=CARTESIAN_POINT ( 'NONE',  ( 2.177545098254089151, -2.619462340734462380, 30.83744416345203021 ) ) ;
#26271=EDGE_LOOP ( 'NONE', ( #83870, #73871 ) ) ;
#26272=CARTESIAN_POINT ( 'NONE',  ( 16.40390046548446534, -11.79725096376909299, 32.30694842903960762 ) ) ;
#26273=DIRECTION ( 'NONE',  ( -0.000000000000000000, -0.8660254037844397068, -0.4999999999999978906 ) ) ;
#26274=CARTESIAN_POINT ( 'NONE',  ( 15.93096747141751379, -7.630691491037286056, 34.74850469731152458 ) ) ;
#26275=CARTESIAN_POINT ( 'NONE',  ( -9.822454901745910405, -6.852621066184266141, 34.70813303252209181 ) ) ;
#26276=FACE_BOUND ( 'NONE', #27468, .T. ) ;
#26277=ORIENTED_EDGE ( 'NONE', *, *, #54639, .T. ) ;
#26278=ORIENTED_EDGE ( 'NONE', *, *, #22379, .T. ) ;
#26280=EDGE_CURVE ( 'NONE', #69003, #10584, #86163, .T. ) ;
#26281=ORIENTED_EDGE ( 'NONE', *, *, #50318, .T. ) ;
#26282=FACE_BOUND ( 'NONE', #61078, .T. ) ;
#26283=CARTESIAN_POINT ( 'NONE',  ( 9.692307692307695177, -5.471508081941601098, 34.59228464037088457 ) ) ;
#26284=CARTESIAN_POINT ( 'NONE',  ( 18.22301135161285046, -4.887748414852792322, 34.01359900205217457 ) ) ;
#26285=ORIENTED_EDGE ( 'NONE', *, *, #2061, .T. ) ;
#26287=CARTESIAN_POINT ( 'NONE',  ( 9.692307692307572609, -5.219633306517616589, 34.19971097300220464 ) ) ;
#26288=CARTESIAN_POINT ( 'NONE',  ( 3.165499230212911019, -12.16647553114622049, 32.15551576947930812 ) ) ;
#26289=VERTEX_POINT ( 'NONE', #25505 ) ;
#26291=CYLINDRICAL_SURFACE ( 'NONE', #14087, 0.2500000000000012212 ) ;
#26292=CARTESIAN_POINT ( 'NONE',  ( -3.480745961711585235, -2.779195860258149242, 31.39871582349837453 ) ) ;
#26293=DIRECTION ( 'NONE',  ( 0.000000000000000000, 0.9848077530122072432, 0.1736481776669354937 ) ) ;
#26294=ORIENTED_EDGE ( 'NONE', *, *, #7814, .F. ) ;
#26295=ADVANCED_FACE ( 'NONE', ( #39476 ), #33596, .F. ) ;
#26301=CARTESIAN_POINT ( 'NONE',  ( 0.4615384615383396616, -9.442884908241554243, 34.35708131394783038 ) ) ;
#26303=CARTESIAN_POINT ( 'NONE',  ( 0.5276057948885365390, -10.67929555188718282, 33.92786785259544757 ) ) ;
#26304=CARTESIAN_POINT ( 'NONE',  ( 12.46153846153846168, -12.34228464037088635, 31.77849191805839268 ) ) ;
#26305=CARTESIAN_POINT ( 'NONE',  ( -16.08859058257012720, -4.481592998940251427, 33.73612834413965089 ) ) ;
#26306=CARTESIAN_POINT ( 'NONE',  ( -39.05038313613820122, -2.499999999999999556, 29.75000000000000355 ) ) ;
#26307=CARTESIAN_POINT ( 'NONE',  ( -1.514762594053604250, -5.195881422630166391, 34.18770438780619259 ) ) ;
#26308=CARTESIAN_POINT ( 'NONE',  ( 8.638540166120458608, -2.845849958028613624, 32.17971566917920967 ) ) ;
#26314=VERTEX_POINT ( 'NONE', #33146 ) ;
#26315=CARTESIAN_POINT ( 'NONE',  ( -4.153846153846152411, -5.471508081941601098, 34.59228464037088457 ) ) ;
#26316=ORIENTED_EDGE ( 'NONE', *, *, #78163, .F. ) ;
#26317=ORIENTED_EDGE ( 'NONE', *, *, #37284, .T. ) ;
#26318=CARTESIAN_POINT ( 'NONE',  ( -16.82697766754503377, -4.176053281294517028, 33.81426240980091791 ) ) ;
#26319=ORIENTED_EDGE ( 'NONE', *, *, #53367, .F. ) ;
#26320=CARTESIAN_POINT ( 'NONE',  ( -5.326899820971665811, -11.47974371597207899, 33.17467449705390692 ) ) ;
#26322=CARTESIAN_POINT ( 'NONE',  ( 4.153846153846154188, -2.721908614388771852, 31.22303859784724978 ) ) ;
#26324=LINE ( 'NONE', #38509, #29478 ) ;
#26325=CARTESIAN_POINT ( 'NONE',  ( 9.942253101685738059, -9.357781135181031829, 34.66075350412533851 ) ) ;
#26326=CARTESIAN_POINT ( 'NONE',  ( 5.076923076923075762, -2.708943851104267164, 35.45975837776705220 ) ) ;
#26327=DIRECTION ( 'NONE',  ( -0.000000000000000000, -0.8660254037844397068, -0.4999999999999978906 ) ) ;
#26328=CARTESIAN_POINT ( 'NONE',  ( -11.76138775597768138, -4.887634598454295265, 34.01352882383564946 ) ) ;
#26330=ADVANCED_FACE ( 'NONE', ( #61054 ), #66935, .F. ) ;
#26331=EDGE_CURVE ( 'NONE', #66483, #22041, #88024, .T. ) ;
#26332=CARTESIAN_POINT ( 'NONE',  ( 5.207713517890027788, -2.845873456487966635, 32.17976146951972538 ) ) ;
#26333=DIRECTION ( 'NONE',  ( -0.000000000000000000, 1.000000000000000000, -0.000000000000000000 ) ) ;
#26334=CARTESIAN_POINT ( 'NONE',  ( 5.749976775778544713, -3.520140089381497361, 33.17453946501458262 ) ) ;
#26335=EDGE_CURVE ( 'NONE', #22078, #23906, #45289, .T. ) ;
#26336=AXIS2_PLACEMENT_3D ( 'NONE', #9237, #22294, #48874 ) ;
#26337=VERTEX_POINT ( 'NONE', #47980 ) ;
#26339=CARTESIAN_POINT ( 'NONE',  ( 6.700150705560774966, -2.554751324335733820, 30.48935550225260727 ) ) ;
#26341=CARTESIAN_POINT ( 'NONE',  ( 8.769230769230768274, -13.88283147151868846, 33.14645433367849847 ) ) ;
#26342=CARTESIAN_POINT ( 'NONE',  ( -5.999999999999998224, -3.513871655860378418, 32.76840700105978499 ) ) ;
#26343=CYLINDRICAL_SURFACE ( 'NONE', #80878, 0.2499999999999994726 ) ;
#26344=AXIS2_PLACEMENT_3D ( 'NONE', #55476, #76187, #75315 ) ;
#26345=CARTESIAN_POINT ( 'NONE',  ( -5.010855743573001675, -2.833524468853757750, 32.15551576947925838 ) ) ;
#26346=DIRECTION ( 'NONE',  ( 0.000000000000000000, 0.8660254037844377084, -0.5000000000000015543 ) ) ;
#26347=B_SPLINE_CURVE_WITH_KNOTS ( 'NONE', 3,
 ( #70684, #62252, #82554, #23367, #20831, #75771, #14076, #566, #50825, #16610 ),
 .UNSPECIFIED., .F., .F.,
 ( 4, 2, 2, 2, 4 ),
 ( 0.0007817359430256294638, 0.0009771253907249950223, 0.001172514838424360472, 0.001367904286123725922, 0.001563293733823091372 ),
 .UNSPECIFIED. ) ;
#26348=VERTEX_POINT ( 'NONE', #40799 ) ;
#26349=B_SPLINE_CURVE_WITH_KNOTS ( 'NONE', 3,
 ( #47042, #86739, #11502, #74530, #53363, #46614, #5625, #73657, #4288, #52472 ),
 .UNSPECIFIED., .F., .F.,
 ( 4, 2, 2, 2, 4 ),
 ( 0.000000000000000000, 0.0001954311564186864949, 0.0003908623128373729899, 0.0005862934692560594577, 0.0007817246256747459798 ),
 .UNSPECIFIED. ) ;
#26350=CARTESIAN_POINT ( 'NONE',  ( 1.384615384615265343, -5.219633306517616589, 34.19971097300220464 ) ) ;
#26351=VERTEX_POINT ( 'NONE', #6563 ) ;
#26352=B_SPLINE_CURVE_WITH_KNOTS ( 'NONE', 3,
 ( #20868, #47898, #14117, #54203, #41151, #61400, #604, #33511, #13672, #27187 ),
 .UNSPECIFIED., .F., .F.,
 ( 4, 2, 2, 2, 4 ),
 ( 0.000000000000000000, 0.0001954311564186869015, 0.0003908623128373738030, 0.0005862934692560607588, 0.0007817246256747476061 ),
 .UNSPECIFIED. ) ;
#26353=EDGE_LOOP ( 'NONE', ( #58618, #36209, #22378, #28196 ) ) ;
#26354=ADVANCED_FACE ( 'NONE', ( #88999 ), #39031, .F. ) ;
#26355=LINE ( 'NONE', #6087, #62257 ) ;
#26357=CARTESIAN_POINT ( 'NONE',  ( -7.173076923076919797, -7.566082377512563184, 35.00000000000000711 ) ) ;
#26358=CARTESIAN_POINT ( 'NONE',  ( 6.249945409378045547, -8.476813868363244353, 34.90874843262270133 ) ) ;
#26359=CYLINDRICAL_SURFACE ( 'NONE', #15074, 0.2500000000000009437 ) ;
#26360=ORIENTED_EDGE ( 'NONE', *, *, #5391, .F. ) ;
#26361=VECTOR ( 'NONE', #56172, 1000.000000000000114 ) ;
#26363=VECTOR ( 'NONE', #37640, 1000.000000000000227 ) ;
#26365=ORIENTED_EDGE ( 'NONE', *, *, #71227, .T. ) ;
#26366=ORIENTED_EDGE ( 'NONE', *, *, #72413, .T. ) ;
#26367=CARTESIAN_POINT ( 'NONE',  ( -17.07692307692307665, -10.51840700105979565, 33.73612834413961536 ) ) ;
#26368=CYLINDRICAL_SURFACE ( 'NONE', #76161, 0.2499999999999994726 ) ;
#26369=ADVANCED_FACE ( 'NONE', ( #63711 ), #69149, .F. ) ;
#26370=CARTESIAN_POINT ( 'NONE',  ( 16.08859622207207707, -2.255955759149247619, 30.00000000000014211 ) ) ;
#26371=CARTESIAN_POINT ( 'NONE',  ( 16.15384615384603251, -10.21337939537710326, 33.94971097300076224 ) ) ;
#26372=CARTESIAN_POINT ( 'NONE',  ( -16.15384615384627409, -12.16647553114689728, 32.15551576947799362 ) ) ;
#26373=DIRECTION ( 'NONE',  ( -0.000000000000000000, 0.7660444431189792347, -0.6427876096865379196 ) ) ;
#26375=VERTEX_POINT ( 'NONE', #7001 ) ;
#26376=B_SPLINE_CURVE_WITH_KNOTS ( 'NONE', 3,
 ( #67588, #7215, #26596, #2643, #36455, #83322, #21159, #21603, #22056, #28358 ),
 .UNSPECIFIED., .F., .F.,
 ( 4, 2, 2, 2, 4 ),
 ( 0.0007817246256747503166, 0.0009771112852218946220, 0.001172497944769039036, 0.001367884604316183233, 0.001563271263863327647 ),
 .UNSPECIFIED. ) ;
#26377=EDGE_CURVE ( 'NONE', #65002, #11510, #4468, .T. ) ;
#26378=CARTESIAN_POINT ( 'NONE',  ( 17.75000000000000000, -2.499999999999998668, 29.75000000000000355 ) ) ;
#26379=VERTEX_POINT ( 'NONE', #55622 ) ;
#26380=DIRECTION ( 'NONE',  ( -0.000000000000000000, 1.000000000000000000, -0.000000000000000000 ) ) ;
#26381=CARTESIAN_POINT ( 'NONE',  ( 11.53846153846153832, -3.886160181151819604, 36.00935417666054406 ) ) ;
#26382=B_SPLINE_CURVE_WITH_KNOTS ( 'NONE', 3,
 ( #37100, #42111, #29479, #7872, #48847, #83986, #15515, #8318, #22268, #56052 ),
 .UNSPECIFIED., .F., .F.,
 ( 4, 2, 2, 2, 4 ),
 ( 0.000000000000000000, 0.0001954311564186867660, 0.0003908623128373735320, 0.0005862934692560603251, 0.0007817246256747470640 ),
 .UNSPECIFIED. ) ;
#26385=CARTESIAN_POINT ( 'NONE',  ( -3.007989689500821573, -12.44528174975671853, 30.48912976160716681 ) ) ;
#26386=VERTEX_POINT ( 'NONE', #2017 ) ;
#26387=DIRECTION ( 'NONE',  ( 0.000000000000000000, 0.7660444431189807890, 0.6427876096865361433 ) ) ;
#26388=CARTESIAN_POINT ( 'NONE',  ( -9.692307692307691624, -9.780366693483667717, 34.19971097300155094 ) ) ;
#26389=TOROIDAL_SURFACE ( 'NONE', #30685, 3.000000000000000888, 2.000000000000000000 ) ;
#26394=ORIENTED_EDGE ( 'NONE', *, *, #74787, .F. ) ;
#26396=CARTESIAN_POINT ( 'NONE',  ( -4.153846153846152411, -3.050289026998446396, 32.03036669348365706 ) ) ;
#26397=CARTESIAN_POINT ( 'NONE',  ( -14.08468095607945969, -2.554770724473667265, 30.48948780036025852 ) ) ;
#26398=EDGE_CURVE ( 'NONE', #12209, #4267, #7892, .T. ) ;
#26399=CARTESIAN_POINT ( 'NONE',  ( 0.6845498131513099160, -12.39991518177334129, 30.74647679643404530 ) ) ;
#26401=CARTESIAN_POINT ( 'NONE',  ( 14.30769230769218758, -6.879047030192662504, 34.71129190930017927 ) ) ;
#26402=CARTESIAN_POINT ( 'NONE',  ( 1.515407192440173079, -8.147973898785416225, 34.70805048591653730 ) ) ;
#26404=DIRECTION ( 'NONE',  ( -0.000000000000000000, -0.6427876096865404731, -0.7660444431189770143 ) ) ;
#26405=CARTESIAN_POINT ( 'NONE',  ( -4.153846153846152411, -11.11383981884818262, 36.00935417666054406 ) ) ;
#26406=FACE_BOUND ( 'NONE', #55453, .T. ) ;
#26408=LINE ( 'NONE', #74597, #34500 ) ;
#26410=CARTESIAN_POINT ( 'NONE',  ( -9.561782254074053355, -12.15418822224088835, 32.17964115625579069 ) ) ;
#26411=CARTESIAN_POINT ( 'NONE',  ( 2.980769230769232170, -7.566083408709834757, 34.74999999999999289 ) ) ;
#26412=CARTESIAN_POINT ( 'NONE',  ( -9.561515884482908234, -10.54018710029568595, 33.71981072465678864 ) ) ;
#26413=CARTESIAN_POINT ( 'NONE',  ( 13.25392478150508069, -2.494641256782728966, 31.33461815524612959 ) ) ;
#26415=EDGE_LOOP ( 'NONE', ( #69775, #57289, #63872, #20384 ) ) ;
#26417=ORIENTED_EDGE ( 'NONE', *, *, #11749, .F. ) ;
#26418=B_SPLINE_CURVE_WITH_KNOTS ( 'NONE', 3,
 ( #46172, #73654, #42080, #20900, #6517, #76290, #22237, #69538, #49269, #69975 ),
 .UNSPECIFIED., .F., .F.,
 ( 4, 2, 2, 2, 4 ),
 ( 0.000000000000000000, 0.0001954311564186864949, 0.0003908623128373729899, 0.0005862934692560594577, 0.0007817246256747459798 ),
 .UNSPECIFIED. ) ;
#26419=CARTESIAN_POINT ( 'NONE',  ( 18.25000000000141753, -7.500000000000154543, 35.00000000000007105 ) ) ;
#26421=B_SPLINE_CURVE_WITH_KNOTS ( 'NONE', 3,
 ( #31112, #86078, #38327, #86533, #24807, #26149, #52719, #67139, #4542, #54497 ),
 .UNSPECIFIED., .F., .F.,
 ( 4, 2, 2, 2, 4 ),
 ( 0.000000000000000000, 0.0001954339857564080707, 0.0003908679715128161414, 0.0005863019572692241849, 0.0007817359430256322827 ),
 .UNSPECIFIED. ) ;
#26422=CARTESIAN_POINT ( 'NONE',  ( -15.29609324357353550, -7.749976730030849303, 34.74374725381503737 ) ) ;
#26423=FACE_OUTER_BOUND ( 'NONE', #43553, .T. ) ;
#26424=CARTESIAN_POINT ( 'NONE',  ( -2.530618525208453651, -11.76352882383564769, 32.36236540154569497 ) ) ;
#26426=CARTESIAN_POINT ( 'NONE',  ( -10.54931728203453822, -11.91647553114624358, 32.58852847137148245 ) ) ;
#26427=DIRECTION ( 'NONE',  ( -0.000000000000000000, -0.9396926207859093161, -0.3420201433256663259 ) ) ;
#26429=B_SPLINE_CURVE_WITH_KNOTS ( 'NONE', 3,
 ( #44322, #30827, #45680, #72705, #4251, #73161, #38039, #30388, #78570, #11015 ),
 .UNSPECIFIED., .F., .F.,
 ( 4, 2, 2, 2, 4 ),
 ( 0.0007817359430256316322, 0.0009771253907249980580, 0.001172514838424364592, 0.001367904286123731127, 0.001563293733823097661 ),
 .UNSPECIFIED. ) ;
#26430=DIRECTION ( 'NONE',  ( -0.000000000000000000, -0.5000000000000009992, -0.8660254037844380415 ) ) ;
#26431=CARTESIAN_POINT ( 'NONE',  ( 5.011652630962299959, -5.219633306516282545, 34.19971097300152252 ) ) ;
#26432=VECTOR ( 'NONE', #21732, 1000.000000000000000 ) ;
#26435=CARTESIAN_POINT ( 'NONE',  ( -12.33074802057151409, -8.191423895709840863, 34.95447573519442130 ) ) ;
#26439=CARTESIAN_POINT ( 'NONE',  ( 5.326977496836530435, -2.544122305571457687, 31.48381861865059150 ) ) ;
#26440=CARTESIAN_POINT ( 'NONE',  ( -1.161602540521989413, -11.98016756924215009, 32.48728574198911190 ) ) ;
#26441=EDGE_LOOP ( 'NONE', ( #15049, #14852, #41765, #22656, #44775, #2545 ) ) ;
#26442=CARTESIAN_POINT ( 'NONE',  ( 16.28437159207980045, -5.070358843744208421, 34.40418822224088302 ) ) ;
#26443=CYLINDRICAL_SURFACE ( 'NONE', #70515, 0.2499999999999994726 ) ;
#26445=CARTESIAN_POINT ( 'NONE',  ( -17.07692307692307665, -10.89733346790207413, 36.13435417666054406 ) ) ;
#26446=CARTESIAN_POINT ( 'NONE',  ( -9.019207513279361876, -3.436278759898153901, 33.07459398097509506 ) ) ;
#26447=ORIENTED_EDGE ( 'NONE', *, *, #67653, .T. ) ;
#26448=LINE ( 'NONE', #89051, #31316 ) ;
#26450=CARTESIAN_POINT ( 'NONE',  ( 8.992243613324164997, -2.523321265292115534, 31.42251411153756990 ) ) ;
#26451=VERTEX_POINT ( 'NONE', #35815 ) ;
#26452=LINE ( 'NONE', #40418, #12458 ) ;
#26453=CARTESIAN_POINT ( 'NONE',  ( 5.326923076924495071, -7.500000000000154543, 35.00000000000007105 ) ) ;
#26454=CARTESIAN_POINT ( 'NONE',  ( -11.76138849736838488, -2.523278758544489797, 31.42238647778637528 ) ) ;
#26455=ORIENTED_EDGE ( 'NONE', *, *, #3415, .T. ) ;
#26456=CARTESIAN_POINT ( 'NONE',  ( 3.164686851409095336, -2.486705287966279876, 31.30864560766542937 ) ) ;
#26457=CARTESIAN_POINT ( 'NONE',  ( 9.692307692307695177, -6.343179335718451384, 34.87096338111211935 ) ) ;
#26458=VECTOR ( 'NONE', #65006, 1000.000000000000227 ) ;
#26459=LINE ( 'NONE', #20141, #19704 ) ;
#26461=B_SPLINE_CURVE_WITH_KNOTS ( 'NONE', 3,
 ( #33762, #12610, #13926, #28326, #41858, #68428, #7176, #47717, #55796, #34649 ),
 .UNSPECIFIED., .F., .F.,
 ( 4, 2, 2, 2, 4 ),
 ( 0.0007817246256747494492, 0.0009771112852218935378, 0.001172497944769037518, 0.001367884604316181498, 0.001563271263863325695 ),
 .UNSPECIFIED. ) ;
#26462=EDGE_LOOP ( 'NONE', ( #29924, #87658, #84421, #9814 ) ) ;
#26464=B_SPLINE_CURVE_WITH_KNOTS ( 'NONE', 3,
 ( #2108, #29593, #16957, #76892, #83663, #1221, #57049, #7991, #23261, #50722 ),
 .UNSPECIFIED., .F., .F.,
 ( 4, 2, 2, 2, 4 ),
 ( 0.0007817246256747472808, 0.0009771112852218907189, 0.001172497944769034049, 0.001367884604316177595, 0.001563271263863320925 ),
 .UNSPECIFIED. ) ;
#26466=ORIENTED_EDGE ( 'NONE', *, *, #86740, .F. ) ;
#26467=VECTOR ( 'NONE', #21956, 999.9999999999998863 ) ;
#26468=CARTESIAN_POINT ( 'NONE',  ( 12.46153846153833911, -10.33852847137269571, 34.16647553114546554 ) ) ;
#26469=CARTESIAN_POINT ( 'NONE',  ( 14.24242186173153435, -4.481592998940162609, 33.73612834413957984 ) ) ;
#26470=CARTESIAN_POINT ( 'NONE',  ( -13.38461538461550759, -12.16647553114689728, 32.15551576947799362 ) ) ;
#26471=CARTESIAN_POINT ( 'NONE',  ( -7.976844449264153702, -10.70098750199973203, 33.91152734681376302 ) ) ;
#26476=CARTESIAN_POINT ( 'NONE',  ( -7.173053667125512511, -2.544273027872574922, 31.48422191005632342 ) ) ;
#26478=CARTESIAN_POINT ( 'NONE',  ( -18.00000000000000000, -1.503186988994757778, 30.80739993210377747 ) ) ;
#26479=CARTESIAN_POINT ( 'NONE',  ( 6.923076923076802558, -10.90142922262034020, 33.41473453929536674 ) ) ;
#26480=CYLINDRICAL_SURFACE ( 'NONE', #34936, 0.2500000000000012212 ) ;
#26484=VECTOR ( 'NONE', #56756, 1000.000000000000000 ) ;
#26485=VERTEX_POINT ( 'NONE', #70029 ) ;
#26486=CARTESIAN_POINT ( 'NONE',  ( -9.692307692307812417, -6.026961402154118019, 34.52809138561165270 ) ) ;
#26487=CYLINDRICAL_SURFACE ( 'NONE', #77587, 0.2500000000000008882 ) ;
#26488=VERTEX_POINT ( 'NONE', #50186 ) ;
#26489=DIRECTION ( 'NONE',  ( 0.000000000000000000, 0.9396926207859126468, -0.3420201433256571111 ) ) ;
#26490=CARTESIAN_POINT ( 'NONE',  ( 5.326923076924495071, -7.500000000000154543, 35.00000000000007105 ) ) ;
#26491=ORIENTED_EDGE ( 'NONE', *, *, #43427, .F. ) ;
#26493=CARTESIAN_POINT ( 'NONE',  ( 9.942307692307695177, -2.249999999999998668, 29.75000000000000355 ) ) ;
#26494=CARTESIAN_POINT ( 'NONE',  ( 18.25000000000143530, -7.500000000000155431, 34.75000000000007105 ) ) ;
#26495=FACE_BOUND ( 'NONE', #11029, .T. ) ;
#26496=CARTESIAN_POINT ( 'NONE',  ( -0.7115151924808155171, -9.943427161483782584, 34.11278801902876978 ) ) ;
#26497=CARTESIAN_POINT ( 'NONE',  ( -1.254089682851818877, -11.93748526763465279, 32.05452791011430946 ) ) ;
#26499=CARTESIAN_POINT ( 'NONE',  ( 11.76147289007438879, -12.39991518177334129, 30.74647679643404530 ) ) ;
#26500=CARTESIAN_POINT ( 'NONE',  ( 0.2386115026316120158, -6.459968553980840689, 34.89616026154728701 ) ) ;
#26501=CARTESIAN_POINT ( 'NONE',  ( 14.43848274865926307, -2.845873456487966635, 32.17976146951972538 ) ) ;
#26503=DIRECTION ( 'NONE',  ( -0.000000000000000000, -0.6427876096865404731, -0.7660444431189771253 ) ) ;
#26504=ORIENTED_EDGE ( 'NONE', *, *, #12023, .F. ) ;
#26505=CARTESIAN_POINT ( 'NONE',  ( 14.30769230769231015, -12.37446782046654192, 30.86335684631486131 ) ) ;
#26506=EDGE_CURVE ( 'NONE', #18801, #58277, #9889, .T. ) ;
#26507=CARTESIAN_POINT ( 'NONE',  ( -17.07692307692319744, -6.835583212225970762, 34.95778746994575670 ) ) ;
#26509=VERTEX_POINT ( 'NONE', #15096 ) ;
#26510=CARTESIAN_POINT ( 'NONE',  ( 0.5267936010512993539, -8.656820664281605460, 34.87096338111211224 ) ) ;
#26511=CARTESIAN_POINT ( 'NONE',  ( -15.29603967673000575, -2.625532179533444754, 30.86335684631481513 ) ) ;
#26512=DIRECTION ( 'NONE',  ( -0.000000000000000000, 0.6427876096865404731, -0.7660444431189771253 ) ) ;
#26513=EDGE_LOOP ( 'NONE', ( #81275, #67917 ) ) ;
#26514=CARTESIAN_POINT ( 'NONE',  ( -16.02305434602136103, -11.18335022499818621, 33.13157742990016885 ) ) ;
#26515=CARTESIAN_POINT ( 'NONE',  ( -7.053224132515143907, -10.19110544564092002, 33.96427741523702792 ) ) ;
#26516=B_SPLINE_CURVE_WITH_KNOTS ( 'NONE', 3,
 ( #83199, #70563, #71002, #29146, #42654, #43088, #29581, #75986, #42217, #8866 ),
 .UNSPECIFIED., .F., .F.,
 ( 4, 2, 2, 2, 4 ),
 ( 0.000000000000000000, 0.0001954339857564075828, 0.0003908679715128151656, 0.0005863019572692227755, 0.0007817359430256303312 ),
 .UNSPECIFIED. ) ;
#26517=VECTOR ( 'NONE', #54716, 1000.000000000000227 ) ;
#26518=FACE_BOUND ( 'NONE', #37934, .T. ) ;
#26519=CARTESIAN_POINT ( 'NONE',  ( -18.22348494372394967, -3.236172620538811717, 32.36188796281390267 ) ) ;
#26520=CARTESIAN_POINT ( 'NONE',  ( -17.07692307692307665, -8.164416787775445883, 34.95778746994557906 ) ) ;
#26521=CARTESIAN_POINT ( 'NONE',  ( 7.976945653978636308, -8.999086150933475636, 34.52020707165672775 ) ) ;
#26523=B_SPLINE_CURVE_WITH_KNOTS ( 'NONE', 3,
 ( #3159, #45484, #50889, #44582, #86040, #17124, #51778, #71618, #37841, #24317 ),
 .UNSPECIFIED., .F., .F.,
 ( 4, 2, 2, 2, 4 ),
 ( 0.0007817246256747528103, 0.0009771112852218978746, 0.001172497944769042939, 0.001367884604316188003, 0.001563271263863333068 ),
 .UNSPECIFIED. ) ;
#26524=CARTESIAN_POINT ( 'NONE',  ( 0.5923289025054098156, -4.684288915650983043, 34.18129842949671371 ) ) ;
#26526=CARTESIAN_POINT ( 'NONE',  ( -14.55769230769230660, -7.566082377512564960, 35.00000000000000711 ) ) ;
#26528=ORIENTED_EDGE ( 'NONE', *, *, #47610, .F. ) ;
#26530=VERTEX_POINT ( 'NONE', #49754 ) ;
#26531=AXIS2_PLACEMENT_3D ( 'NONE', #80156, #31057, #17108 ) ;
#26533=DIRECTION ( 'NONE',  ( -0.000000000000000000, 0.9396926207859093161, -0.3420201433256663259 ) ) ;
#26534=DIRECTION ( 'NONE',  ( 0.000000000000000000, 0.4999999999999985567, 0.8660254037844395958 ) ) ;
#26535=CARTESIAN_POINT ( 'NONE',  ( -0.3953693205758047058, -7.250054483168842268, 34.74374881642865631 ) ) ;
#26536=DIRECTION ( 'NONE',  ( 0.000000000000000000, 0.9396926207859126468, -0.3420201433256571111 ) ) ;
#26538=CARTESIAN_POINT ( 'NONE',  ( -1.634592128663975963, -4.075325502946085976, 33.72974371597207721 ) ) ;
#26539=FACE_OUTER_BOUND ( 'NONE', #29597, .T. ) ;
#26540=DIRECTION ( 'NONE',  ( -0.000000000000000000, 1.000000000000000000, -0.000000000000000000 ) ) ;
#26541=CARTESIAN_POINT ( 'NONE',  ( 10.68063975489745232, -3.643525952247864463, 33.31231777344670064 ) ) ;
#26542=CARTESIAN_POINT ( 'NONE',  ( -6.065270445960774026, -2.892918686051582089, 31.69288490824015270 ) ) ;
#26543=DIRECTION ( 'NONE',  ( -0.000000000000000000, 0.8660254037844399289, -0.4999999999999980016 ) ) ;
#26544=CARTESIAN_POINT ( 'NONE',  ( 5.776515056276052107, -12.24155766932282496, 31.33739205006857986 ) ) ;
#26545=EDGE_CURVE ( 'NONE', #29700, #66822, #77229, .T. ) ;
#26546=FACE_OUTER_BOUND ( 'NONE', #10536, .T. ) ;
#26547=CARTESIAN_POINT ( 'NONE',  ( -7.715628144390283438, -12.45806712695776319, 30.39783852428763922 ) ) ;
#26548=ADVANCED_FACE ( 'NONE', ( #48419 ), #43007, .F. ) ;
#26550=CARTESIAN_POINT ( 'NONE',  ( 1.161130440891439131, -2.599994579823203367, 30.74605699353653776 ) ) ;
#26551=CARTESIAN_POINT ( 'NONE',  ( 18.06606733335007675, -4.661471528628508665, 34.16647553114624003 ) ) ;
#26553=EDGE_CURVE ( 'NONE', #8324, #31532, #73225, .T. ) ;
#26554=EDGE_CURVE ( 'NONE', #18617, #24402, #58281, .T. ) ;
#26555=LINE ( 'NONE', #13913, #20211 ) ;
#26556=( NAMED_UNIT ( * ) PLANE_ANGLE_UNIT ( ) SI_UNIT ( $, .RADIAN. ) );
#26557=CARTESIAN_POINT ( 'NONE',  ( -0.4615384615384611200, -1.466349020453238561, 30.81389545987213907 ) ) ;
#26558=CARTESIAN_POINT ( 'NONE',  ( -18.12726022028586925, -2.249999999999999556, 29.52412087102020521 ) ) ;
#26559=VERTEX_POINT ( 'NONE', #44763 ) ;
#26563=CARTESIAN_POINT ( 'NONE',  ( -16.08859058257013430, -10.21337939537593797, 33.94971097300152252 ) ) ;
#26564=CARTESIAN_POINT ( 'NONE',  ( 0.2115152242454939047, -2.823816976329317718, 31.52131813110796443 ) ) ;
#26565=VERTEX_POINT ( 'NONE', #24054 ) ;
#26566=CARTESIAN_POINT ( 'NONE',  ( -5.076923076923075762, -11.69971097300155272, 32.46337939537588113 ) ) ;
#26567=CARTESIAN_POINT ( 'NONE',  ( -14.98076923076916422, -7.434744860731433924, 35.00000000000000711 ) ) ;
#26568=CARTESIAN_POINT ( 'NONE',  ( 2.084207383127977486, -12.69144148231606017, 30.53333754910549303 ) ) ;
#26569=ORIENTED_EDGE ( 'NONE', *, *, #431, .T. ) ;
#26570=ORIENTED_EDGE ( 'NONE', *, *, #24560, .F. ) ;
#26572=DIRECTION ( 'NONE',  ( 0.000000000000000000, 0.4999999999999985567, 0.8660254037844395958 ) ) ;
#26573=FACE_OUTER_BOUND ( 'NONE', #10734, .T. ) ;
#26574=CARTESIAN_POINT ( 'NONE',  ( 18.22301284409339672, -10.01129605718032423, 34.36064277460058491 ) ) ;
#26575=CARTESIAN_POINT ( 'NONE',  ( 9.626225312947559232, -9.058645607665454236, 34.76329471203372634 ) ) ;
#26576=CARTESIAN_POINT ( 'NONE',  ( -10.61538461538473577, -12.16647553114689728, 32.15551576947799362 ) ) ;
#26577=CARTESIAN_POINT ( 'NONE',  ( 9.757562831820530747, -10.33852847137154107, 34.16647553114620450 ) ) ;
#26578=DIRECTION ( 'NONE',  ( 0.000000000000000000, 0.000000000000000000, 1.000000000000000000 ) ) ;
#26579=CARTESIAN_POINT ( 'NONE',  ( -0.4615384615384611200, -12.34228464037088635, 31.77849191805839268 ) ) ;
#26580=EDGE_CURVE ( 'NONE', #46286, #87539, #26014, .T. ) ;
#26582=VERTEX_POINT ( 'NONE', #79005 ) ;
#26583=VERTEX_POINT ( 'NONE', #2884 ) ;
#26586=CARTESIAN_POINT ( 'NONE',  ( 11.53846153846141576, -3.643525952248795718, 33.31231777344771672 ) ) ;
#26588=ORIENTED_EDGE ( 'NONE', *, *, #65664, .T. ) ;
#26589=B_SPLINE_CURVE_WITH_KNOTS ( 'NONE', 3,
 ( #43293, #49604, #55468, #82953, #70766, #21235, #15385, #9070, #28443, #76635 ),
 .UNSPECIFIED., .F., .F.,
 ( 4, 2, 2, 2, 4 ),
 ( 0.0007817246256747460882, 0.0009771112852218892010, 0.001172497944769032314, 0.001367884604316175427, 0.001563271263863318539 ),
 .UNSPECIFIED. ) ;
#26590=CARTESIAN_POINT ( 'NONE',  ( -15.23076923076935252, -2.379036618888197729, 30.90682066428292885 ) ) ;
#26591=EDGE_CURVE ( 'NONE', #19448, #2854, #68906, .T. ) ;
#26592=ORIENTED_EDGE ( 'NONE', *, *, #39000, .T. ) ;
#26593=CARTESIAN_POINT ( 'NONE',  ( 16.82689983963011926, -10.05641848906368097, 34.04755513067966177 ) ) ;
#26594=ORIENTED_EDGE ( 'NONE', *, *, #39952, .T. ) ;
#26595=LINE ( 'NONE', #31571, #40237 ) ;
#26596=CARTESIAN_POINT ( 'NONE',  ( -6.792551484843278864, -5.070358843744210198, 34.40418822224088302 ) ) ;
#26597=CARTESIAN_POINT ( 'NONE',  ( 12.33084785842815378, -2.295517848115769421, 30.44137282052137294 ) ) ;
#26598=FACE_BOUND ( 'NONE', #58813, .T. ) ;
#26599=CARTESIAN_POINT ( 'NONE',  ( 9.692307692307695177, -2.708943851104267164, 35.45975837776705220 ) ) ;
#26601=ADVANCED_FACE ( 'NONE', ( #4235 ), #85328, .F. ) ;
#26602=CARTESIAN_POINT ( 'NONE',  ( 13.60762822870878352, -4.762714258010881885, 34.23016756924214832 ) ) ;
#26603=CARTESIAN_POINT ( 'NONE',  ( 10.48469401227430708, -9.929715669179220328, 34.40415004197138416 ) ) ;
#26604=FACE_OUTER_BOUND ( 'NONE', #75656, .T. ) ;
#26605=CARTESIAN_POINT ( 'NONE',  ( -7.912236225513983534, -9.058645607665454236, 34.76329471203372634 ) ) ;
#26606=FACE_OUTER_BOUND ( 'NONE', #31729, .T. ) ;
#26607=ADVANCED_FACE ( 'NONE', ( #51503 ), #2446, .F. ) ;
#26609=ORIENTED_EDGE ( 'NONE', *, *, #17366, .F. ) ;
#26611=CARTESIAN_POINT ( 'NONE',  ( -14.30769230769242739, -12.27809138561165270, 31.22303859784587132 ) ) ;
#26612=DIRECTION ( 'NONE',  ( -0.000000000000000000, 0.8660254037844397068, -0.4999999999999978906 ) ) ;
#26613=CARTESIAN_POINT ( 'NONE',  ( 16.40379156322419973, -11.56426240980093567, 33.07394671870546432 ) ) ;
#26614=CARTESIAN_POINT ( 'NONE',  ( -0.4615384615385840772, -11.06231777344772027, 33.60647404775119895 ) ) ;
#26616=CARTESIAN_POINT ( 'NONE',  ( -12.39547011053602610, -4.098570777380720287, 33.41473453929635440 ) ) ;
#26617=ORIENTED_EDGE ( 'NONE', *, *, #31700, .T. ) ;
#26618=DIRECTION ( 'NONE',  ( 0.000000000000000000, 0.6427876096865373645, -0.7660444431189797898 ) ) ;
#26619=B_SPLINE_CURVE_WITH_KNOTS ( 'NONE', 3,
 ( #79264, #84703, #22977, #50444, #64394, #78805, #86482, #57653, #71599, #58978 ),
 .UNSPECIFIED., .F., .F.,
 ( 4, 2, 2, 2, 4 ),
 ( 0.0007817359430256369448, 0.0009771253907250049969, 0.001172514838424373049, 0.001367904286123741101, 0.001563293733823109153 ),
 .UNSPECIFIED. ) ;
#26620=CARTESIAN_POINT ( 'NONE',  ( 14.30769230769218758, -11.48612834414049644, 32.76840700105863391 ) ) ;
#26622=ADVANCED_FACE ( 'NONE', ( #44307 ), #79460, .F. ) ;
#26623=CARTESIAN_POINT ( 'NONE',  ( -3.480792454990687457, -12.68155406624981119, 30.59749803192733708 ) ) ;
#26624=B_SPLINE_CURVE_WITH_KNOTS ( 'NONE', 3,
 ( #45131, #3257, #85687, #38384, #65839, #4140, #51415, #59089, #72605, #17218 ),
 .UNSPECIFIED., .F., .F.,
 ( 4, 2, 2, 2, 4 ),
 ( 0.0007817359430256322827, 0.0009771253907249989254, 0.001172514838424365676, 0.001367904286123732428, 0.001563293733823098962 ),
 .UNSPECIFIED. ) ;
#26625=ORIENTED_EDGE ( 'NONE', *, *, #14287, .T. ) ;
#26626=ORIENTED_EDGE ( 'NONE', *, *, #59236, .F. ) ;
#26627=EDGE_LOOP ( 'NONE', ( #41454, #22928 ) ) ;
#26629=FACE_OUTER_BOUND ( 'NONE', #65038, .T. ) ;
#26630=ORIENTED_EDGE ( 'NONE', *, *, #57587, .F. ) ;
#26631=ADVANCED_FACE ( 'NONE', ( #9233 ), #57397, .F. ) ;
#26632=FACE_OUTER_BOUND ( 'NONE', #25258, .T. ) ;
#26633=CARTESIAN_POINT ( 'NONE',  ( -5.300408020647022767, -2.847400154188068022, 31.58180166144859058 ) ) ;
#26634=CARTESIAN_POINT ( 'NONE',  ( 3.296024370282069960, -5.941354392334606160, 34.76329471203374055 ) ) ;
#26635=CARTESIAN_POINT ( 'NONE',  ( 1.634669804528839476, -6.523592122091591783, 34.90882529074906415 ) ) ;
#26637=VERTEX_POINT ( 'NONE', #16419 ) ;
#26638=CARTESIAN_POINT ( 'NONE',  ( -15.29685264172511161, -11.69971097300155272, 32.46337939537587403 ) ) ;
#26640=EDGE_LOOP ( 'NONE', ( #6989, #72844 ) ) ;
#26641=FACE_OUTER_BOUND ( 'NONE', #69806, .T. ) ;
#26642=CARTESIAN_POINT ( 'NONE',  ( -17.99999999999969447, -2.506253911140613244, 30.00000000000320455 ) ) ;
#26643=DIRECTION ( 'NONE',  ( -0.000000000000000000, -0.9396926207859092051, -0.3420201433256662704 ) ) ;
#26644=LINE ( 'NONE', #48677, #66829 ) ;
#26645=CARTESIAN_POINT ( 'NONE',  ( -4.023055712879203050, -4.684288915650984819, 34.18129842949671371 ) ) ;
#26646=EDGE_CURVE ( 'NONE', #4609, #68032, #43884, .T. ) ;
#26647=CARTESIAN_POINT ( 'NONE',  ( 18.06525557127602610, -2.625532179533470512, 30.86335684631491105 ) ) ;
#26648=CARTESIAN_POINT ( 'NONE',  ( -0.6850234052624097902, -12.44517049084099725, 30.48991314939691932 ) ) ;
#26650=ORIENTED_EDGE ( 'NONE', *, *, #79530, .T. ) ;
#26652=CARTESIAN_POINT ( 'NONE',  ( -1.384615384615506484, -3.643525952248795718, 33.31231777344771672 ) ) ;
#26653=EDGE_CURVE ( 'NONE', #74762, #85754, #69386, .T. ) ;
#26654=EDGE_CURVE ( 'NONE', #13908, #49386, #5127, .T. ) ;
#26655=EDGE_LOOP ( 'NONE', ( #40265, #82137 ) ) ;
#26656=CARTESIAN_POINT ( 'NONE',  ( -6.000000000000119904, -2.625532179533778709, 30.86335684631627174 ) ) ;
#26657=CARTESIAN_POINT ( 'NONE',  ( -2.980714919130916130, -5.728107161865378494, 34.42597550085002922 ) ) ;
#26659=B_SPLINE_CURVE_WITH_KNOTS ( 'NONE', 3,
 ( #57741, #72582, #10889, #78446, #78894, #85661, #38360, #45106, #71688, #86109 ),
 .UNSPECIFIED., .F., .F.,
 ( 4, 2, 2, 2, 4 ),
 ( 0.0007817246256747445703, 0.0009771112852218872494, 0.001172497944769030145, 0.001367884604316172825, 0.001563271263863315504 ),
 .UNSPECIFIED. ) ;
#26660=CARTESIAN_POINT ( 'NONE',  ( 7.173022441425066731, -5.852078868378311149, 34.47109172314383585 ) ) ;
#26661=CARTESIAN_POINT ( 'NONE',  ( -14.37377468705243722, -2.833524468853757305, 32.15551576947924417 ) ) ;
#26662=ORIENTED_EDGE ( 'NONE', *, *, #44820, .F. ) ;
#26664=FACE_OUTER_BOUND ( 'NONE', #4721, .T. ) ;
#26665=CARTESIAN_POINT ( 'NONE',  ( 18.25005441991345734, -12.41089969410671223, 31.60739465890703670 ) ) ;
#26666=ORIENTED_EDGE ( 'NONE', *, *, #25050, .T. ) ;
#26667=DIRECTION ( 'NONE',  ( -0.000000000000000000, -0.3420201433256694901, -0.9396926207859082059 ) ) ;
#26668=ORIENTED_EDGE ( 'NONE', *, *, #40228, .F. ) ;
#26669=CYLINDRICAL_SURFACE ( 'NONE', #16959, 0.2499999999999973355 ) ;
#26670=CARTESIAN_POINT ( 'NONE',  ( 11.76124120743959978, -6.717445702608402236, 34.94155399931962336 ) ) ;
#26671=EDGE_CURVE ( 'NONE', #76071, #7867, #22804, .T. ) ;
#26672=ORIENTED_EDGE ( 'NONE', *, *, #85279, .T. ) ;
#26673=CARTESIAN_POINT ( 'NONE',  ( -39.05038313613820122, -2.499999999999999556, 29.75000000000000355 ) ) ;
#26674=CARTESIAN_POINT ( 'NONE',  ( -6.249976744048591826, -2.318417181685854978, 30.59732222474233865 ) ) ;
#26675=DIRECTION ( 'NONE',  ( -0.000000000000000000, 0.1736481776669307198, -0.9848077530122080203 ) ) ;
#26676=VECTOR ( 'NONE', #54895, 1000.000000000000227 ) ;
#26677=CARTESIAN_POINT ( 'NONE',  ( -2.307692307692305711, -1.629998284177014645, 34.34916445242399163 ) ) ;
#26678=CARTESIAN_POINT ( 'NONE',  ( -2.241624974342230292, -10.67929555188718282, 33.92786785259544757 ) ) ;
#26679=ADVANCED_FACE ( 'NONE', ( #4689 ), #12330, .F. ) ;
#26680=B_SPLINE_CURVE_WITH_KNOTS ( 'NONE', 3,
 ( #1421, #22577, #64432, #28914, #57254, #30228, #50044, #77966, #73442, #58567 ),
 .UNSPECIFIED., .F., .F.,
 ( 4, 2, 2, 2, 4 ),
 ( 0.0007817246256747448956, 0.0009771112852218876831, 0.001172497944769030579, 0.001367884604316173475, 0.001563271263863316371 ),
 .UNSPECIFIED. ) ;
#26681=ORIENTED_EDGE ( 'NONE', *, *, #7622, .F. ) ;
#26682=DIRECTION ( 'NONE',  ( -0.000000000000000000, 0.9396926207859093161, -0.3420201433256663259 ) ) ;
#26684=DIRECTION ( 'NONE',  ( -0.000000000000000000, 0.1736481776669307198, -0.9848077530122080203 ) ) ;
#26685=ADVANCED_FACE ( 'NONE', ( #41919 ), #19525, .F. ) ;
#26688=CARTESIAN_POINT ( 'NONE',  ( -18.13069060311030611, -10.70098750199973203, 33.91152734681374881 ) ) ;
#26689=CARTESIAN_POINT ( 'NONE',  ( 3.230769230769108269, -11.67786785259630911, 32.92929555188603530 ) ) ;
#26690=CARTESIAN_POINT ( 'NONE',  ( 17.07692307692307665, -2.538708090699994813, 30.37095296980875503 ) ) ;
#26691=ORIENTED_EDGE ( 'NONE', *, *, #28535, .T. ) ;
#26692=EDGE_CURVE ( 'NONE', #9304, #31091, #2387, .T. ) ;
#26693=VERTEX_POINT ( 'NONE', #45664 ) ;
#26694=ORIENTED_EDGE ( 'NONE', *, *, #45633, .T. ) ;
#26696=CARTESIAN_POINT ( 'NONE',  ( -4.219929564802032296, -5.557115091759785130, 34.35708131394839171 ) ) ;
#26697=CARTESIAN_POINT ( 'NONE',  ( 16.40379156322419973, -10.92531984108285492, 33.72920026020278073 ) ) ;
#26698=CARTESIAN_POINT ( 'NONE',  ( -9.822784400424156459, -7.276988635370452485, 34.74523720219453793 ) ) ;
#26699=DIRECTION ( 'NONE',  ( -0.000000000000000000, 0.5000000000000011102, -0.8660254037844381525 ) ) ;
#26700=CARTESIAN_POINT ( 'NONE',  ( 4.023285562104232937, -2.504760397472873823, 29.97295953869789997 ) ) ;
#26703=CARTESIAN_POINT ( 'NONE',  ( -2.307692307692305711, -9.819645486525091727, 36.12317359536749706 ) ) ;
#26705=B_SPLINE_CURVE_WITH_KNOTS ( 'NONE', 3,
 ( #85170, #50476, #77518, #15829, #77961, #3182, #22573, #23889, #50904, #16262 ),
 .UNSPECIFIED., .F., .F.,
 ( 4, 2, 2, 2, 4 ),
 ( 0.000000000000000000, 0.0001954311564186871184, 0.0003908623128373742367, 0.0005862934692560614093, 0.0007817246256747484735 ),
 .UNSPECIFIED. ) ;
#26707=EDGE_CURVE ( 'NONE', #1158, #7863, #30136, .T. ) ;
#26708=ORIENTED_EDGE ( 'NONE', *, *, #65444, .F. ) ;
#26709=ORIENTED_EDGE ( 'NONE', *, *, #38362, .T. ) ;
#26710=CARTESIAN_POINT ( 'NONE',  ( -1.384615384615383471, -3.513871655860378418, 32.76840700105978499 ) ) ;
#26712=EDGE_CURVE ( 'NONE', #58521, #20099, #83931, .T. ) ;
#26713=CYLINDRICAL_SURFACE ( 'NONE', #8659, 0.2499999999999994726 ) ;
#26714=CARTESIAN_POINT ( 'NONE',  ( -5.934744428723973897, -3.835265460703683349, 33.15142922261929925 ) ) ;
#26715=CARTESIAN_POINT ( 'NONE',  ( -0.2387587925603951444, -2.353885683473779356, 30.79025554430704759 ) ) ;
#26716=FACE_OUTER_BOUND ( 'NONE', #46029, .T. ) ;
#26717=FACE_BOUND ( 'NONE', #47741, .T. ) ;
#26718=VERTEX_POINT ( 'NONE', #38924 ) ;
#26719=CARTESIAN_POINT ( 'NONE',  ( 17.07692307692307665, -6.386643153685126251, 34.62446782046654192 ) ) ;
#26720=FACE_OUTER_BOUND ( 'NONE', #484, .T. ) ;
#26721=VERTEX_POINT ( 'NONE', #14435 ) ;
#26722=CARTESIAN_POINT ( 'NONE',  ( 5.011653076366756387, -2.379036618887870436, 30.90682066428147934 ) ) ;
#26723=EDGE_LOOP ( 'NONE', ( #81689, #5253 ) ) ;
#26724=FACE_BOUND ( 'NONE', #22350, .T. ) ;
#26726=CARTESIAN_POINT ( 'NONE',  ( -13.63463862190834952, -10.76384336483936011, 33.53834819971076087 ) ) ;
#26727=ORIENTED_EDGE ( 'NONE', *, *, #74732, .T. ) ;
#26728=AXIS2_PLACEMENT_3D ( 'NONE', #16348, #54779, #54333 ) ;
#26729=CARTESIAN_POINT ( 'NONE',  ( -5.869161581987236254, -7.277220443632450575, 34.74524770363009196 ) ) ;
#26730=CARTESIAN_POINT ( 'NONE',  ( 17.07692307692307665, -11.91647553114624181, 32.58852847137148245 ) ) ;
#26732=ORIENTED_EDGE ( 'NONE', *, *, #14044, .T. ) ;
#26733=DIRECTION ( 'NONE',  ( 0.000000000000000000, 0.3420201433256610524, 0.9396926207859113145 ) ) ;
#26734=CARTESIAN_POINT ( 'NONE',  ( 14.43821774592595553, -3.625058011473228703, 33.29252011169590020 ) ) ;
#26735=CARTESIAN_POINT ( 'NONE',  ( 6.856993512121044354, -12.37446782046654192, 30.86335684631486487 ) ) ;
#26736=CARTESIAN_POINT ( 'NONE',  ( -17.77722033102192967, -12.69155399931963046, 30.53255429739158444 ) ) ;
#26737=ORIENTED_EDGE ( 'NONE', *, *, #35341, .T. ) ;
#26740=CARTESIAN_POINT ( 'NONE',  ( 2.307692307692309264, -3.322132147404559976, 32.92929555188717927 ) ) ;
#26741=VERTEX_POINT ( 'NONE', #62611 ) ;
#26742=LINE ( 'NONE', #74942, #14062 ) ;
#26743=CARTESIAN_POINT ( 'NONE',  ( 9.442307692307695177, -7.433932668274256805, 35.00000000000000711 ) ) ;
#26744=CARTESIAN_POINT ( 'NONE',  ( -8.069638770718178478, -12.47654668319379567, 31.42292124445336654 ) ) ;
#26745=CARTESIAN_POINT ( 'NONE',  ( 6.673076923076925127, -7.500000000000001776, 34.75000000000000000 ) ) ;
#26746=CARTESIAN_POINT ( 'NONE',  ( 7.596153846153846700, -7.500000000000001776, 35.00000000000000000 ) ) ;
#26747=CARTESIAN_POINT ( 'NONE',  ( 15.23076923076910916, -5.941354392335915335, 34.76329471203413846 ) ) ;
#26748=FACE_OUTER_BOUND ( 'NONE', #57997, .T. ) ;
#26749=CARTESIAN_POINT ( 'NONE',  ( 6.923076923077238654, -2.255955759149395501, 30.00000000000324363 ) ) ;
#26753=B_SPLINE_CURVE_WITH_KNOTS ( 'NONE', 3,
 ( #61595, #20183, #75554, #40019, #47649, #60714, #21047, #47194, #48518, #75131 ),
 .UNSPECIFIED., .F., .F.,
 ( 4, 2, 2, 2, 4 ),
 ( 0.000000000000000000, 0.0001954311564186868202, 0.0003908623128373736404, 0.0005862934692560604335, 0.0007817246256747472808 ),
 .UNSPECIFIED. ) ;
#26756=DIRECTION ( 'NONE',  ( -1.000000000000000000, 0.000000000000000000, 0.000000000000000000 ) ) ;
#26757=ORIENTED_EDGE ( 'NONE', *, *, #80077, .F. ) ;
#26758=EDGE_CURVE ( 'NONE', #64904, #34679, #19465, .T. ) ;
#26759=EDGE_LOOP ( 'NONE', ( #41238, #67805, #1560, #56385 ) ) ;
#26760=DIRECTION ( 'NONE',  ( 0.000000000000000000, 0.000000000000000000, 1.000000000000000000 ) ) ;
#26761=EDGE_CURVE ( 'NONE', #46856, #25490, #77902, .T. ) ;
#26762=ORIENTED_EDGE ( 'NONE', *, *, #30884, .F. ) ;
#26763=CARTESIAN_POINT ( 'NONE',  ( 10.61538461538461675, -5.557115091759785130, 34.35708131394839171 ) ) ;
#26765=CARTESIAN_POINT ( 'NONE',  ( 12.52770506813010343, -7.250054591869670162, 34.99404684341514127 ) ) ;
#26766=CARTESIAN_POINT ( 'NONE',  ( -11.31544869436814338, -10.01129605718032600, 34.36064277460058491 ) ) ;
#26767=CYLINDRICAL_SURFACE ( 'NONE', #57635, 0.2499999999999986955 ) ;
#26768=CARTESIAN_POINT ( 'NONE',  ( -11.66860874789975888, -11.47017969459904130, 32.78971311882034456 ) ) ;
#26769=CARTESIAN_POINT ( 'NONE',  ( 9.757562831820532523, -12.51329471203373345, 31.30864560766537963 ) ) ;
#26770=CYLINDRICAL_SURFACE ( 'NONE', #25256, 0.2499999999999998890 ) ;
#26772=CARTESIAN_POINT ( 'NONE',  ( -4.219929564802033184, -3.513871655860377086, 32.76840700105978499 ) ) ;
#26773=AXIS2_PLACEMENT_3D ( 'NONE', #84900, #15548, #42142 ) ;
#26774=CARTESIAN_POINT ( 'NONE',  ( -6.923076923076922462, -4.661471528628507777, 34.16647553114623292 ) ) ;
#26775=CARTESIAN_POINT ( 'NONE',  ( -13.25382357679059986, -6.413143153341454017, 34.63066358083362672 ) ) ;
#26776=ADVANCED_FACE ( 'NONE', ( #63048 ), #1360, .F. ) ;
#26777=CARTESIAN_POINT ( 'NONE',  ( 2.307692307692309264, -9.058645607665452459, 34.76329471203371924 ) ) ;
#26778=EDGE_LOOP ( 'NONE', ( #58667, #30999 ) ) ;
#26779=ORIENTED_EDGE ( 'NONE', *, *, #5308, .T. ) ;
#26780=CARTESIAN_POINT ( 'NONE',  ( 6.673053685783957967, -2.587272538249754117, 30.68239716806877837 ) ) ;
#26781=LINE ( 'NONE', #48817, #30212 ) ;
#26782=DIRECTION ( 'NONE',  ( -0.000000000000000000, 1.000000000000000000, -0.000000000000000000 ) ) ;
#26783=ADVANCED_FACE ( 'NONE', ( #15774 ), #63501, .F. ) ;
#26784=CARTESIAN_POINT ( 'NONE',  ( 0.3313904918067653860, -10.31621877034669232, 34.18098118002069441 ) ) ;
#26785=CARTESIAN_POINT ( 'NONE',  ( 15.23076923076910916, -12.51329471203414379, 31.30864560766407578 ) ) ;
#26786=CARTESIAN_POINT ( 'NONE',  ( -13.51530598772569292, -10.70098750199973203, 33.91152734681376302 ) ) ;
#26787=CARTESIAN_POINT ( 'NONE',  ( -3.230769230769229949, -2.499999999999998668, 29.75000000000001421 ) ) ;
#26788=EDGE_CURVE ( 'NONE', #35812, #41427, #41963, .T. ) ;
#26790=LINE ( 'NONE', #81744, #17029 ) ;
#26791=ORIENTED_EDGE ( 'NONE', *, *, #48463, .F. ) ;
#26792=B_SPLINE_CURVE_WITH_KNOTS ( 'NONE', 3,
 ( #40408, #20125, #39075, #80955, #87718, #18349, #25989, #45809, #66538, #4837 ),
 .UNSPECIFIED., .F., .F.,
 ( 4, 2, 2, 2, 4 ),
 ( 0.0007817359430256346680, 0.0009771253907250002264, 0.001172514838424365893, 0.001367904286123731560, 0.001563293733823104166 ),
 .UNSPECIFIED. ) ;
#26793=ADVANCED_FACE ( 'NONE', ( #71143 ), #23395, .F. ) ;
#26794=ORIENTED_EDGE ( 'NONE', *, *, #71323, .T. ) ;
#26795=CARTESIAN_POINT ( 'NONE',  ( 18.00000000000000000, -3.050289026998446396, 32.03036669348365706 ) ) ;
#26797=VECTOR ( 'NONE', #31076, 1000.000000000000114 ) ;
#26798=CARTESIAN_POINT ( 'NONE',  ( -0.2115929431903193214, -6.696923467548660192, 34.68552623307873972 ) ) ;
#26799=FACE_OUTER_BOUND ( 'NONE', #5898, .T. ) ;
#26801=VECTOR ( 'NONE', #20021, 1000.000000000000000 ) ;
#26802=ORIENTED_EDGE ( 'NONE', *, *, #38387, .F. ) ;
#26804=ORIENTED_EDGE ( 'NONE', *, *, #53761, .F. ) ;
#26805=PRODUCT_DEFINITION_SHAPE ( 'NONE', 'NONE',  #41349 ) ;
#26807=EDGE_LOOP ( 'NONE', ( #21588, #58624 ) ) ;
#26809=CARTESIAN_POINT ( 'NONE',  ( -14.30769230769230660, -13.04860791097971706, 34.73218667398347037 ) ) ;
#26810=DIRECTION ( 'NONE',  ( -0.000000000000000000, -0.000000000000000000, -1.000000000000000000 ) ) ;
#26812=DIRECTION ( 'NONE',  ( -0.000000000000000000, 0.5000000000000011102, -0.8660254037844380415 ) ) ;
#26813=CARTESIAN_POINT ( 'NONE',  ( -16.28399412357784826, -2.373036134822905208, 30.88089517874952250 ) ) ;
#26815=CARTESIAN_POINT ( 'NONE',  ( -15.29685161012936767, -2.486705287966279432, 31.30864560766542937 ) ) ;
#26816=ORIENTED_EDGE ( 'NONE', *, *, #26087, .F. ) ;
#26817=EDGE_CURVE ( 'NONE', #87648, #8709, #70713, .T. ) ;
#26818=ORIENTED_EDGE ( 'NONE', *, *, #21033, .T. ) ;
#26819=ORIENTED_EDGE ( 'NONE', *, *, #27521, .F. ) ;
#26820=CARTESIAN_POINT ( 'NONE',  ( -3.296039231325550212, -2.657715359629089225, 31.77849191805834295 ) ) ;
#26821=ORIENTED_EDGE ( 'NONE', *, *, #24779, .F. ) ;
#26822=EDGE_CURVE ( 'NONE', #37020, #55506, #15159, .T. ) ;
#26823=B_SPLINE_CURVE_WITH_KNOTS ( 'NONE', 3,
 ( #38340, #23921, #36996, #18075, #11311, #3214, #3652, #50938, #10427, #58152 ),
 .UNSPECIFIED., .F., .F.,
 ( 4, 2, 2, 2, 4 ),
 ( 0.0007817359430256322827, 0.0009771253907249989254, 0.001172514838424365676, 0.001367904286123732428, 0.001563293733823099179 ),
 .UNSPECIFIED. ) ;
#26824=CARTESIAN_POINT ( 'NONE',  ( 9.562159722575998444, -8.630895178749533159, 34.87696386517710323 ) ) ;
#26825=DIRECTION ( 'NONE',  ( -0.000000000000000000, -0.000000000000000000, -1.000000000000000000 ) ) ;
#26826=EDGE_CURVE ( 'NONE', #78424, #32882, #47374, .T. ) ;
#26830=CARTESIAN_POINT ( 'NONE',  ( 7.846153846153723244, -4.320704448113951379, 33.92786785259630022 ) ) ;
#26831=EDGE_LOOP ( 'NONE', ( #50317, #45161, #77044, #87356 ) ) ;
#26832=CARTESIAN_POINT ( 'NONE',  ( 2.177000841024751665, -6.413092428213692742, 34.63065189839063152 ) ) ;
#26833=FACE_BOUND ( 'NONE', #36596, .T. ) ;
#26834=CARTESIAN_POINT ( 'NONE',  ( -10.61538461538461320, -9.780366693483667717, 34.19971097300155094 ) ) ;
#26835=CARTESIAN_POINT ( 'NONE',  ( -0.4615384615384611200, -2.708943851104267164, 35.45975837776705220 ) ) ;
#26836=VERTEX_POINT ( 'NONE', #38254 ) ;
#26838=AXIS2_PLACEMENT_3D ( 'NONE', #84836, #20997, #27764 ) ;
#26839=CARTESIAN_POINT ( 'NONE',  ( 8.834485908743602067, -8.656820664281605460, 34.87096338111211224 ) ) ;
#26840=CARTESIAN_POINT ( 'NONE',  ( -17.07692307692319744, -12.70778746994576025, 30.41441678777401236 ) ) ;
#26841=CARTESIAN_POINT ( 'NONE',  ( 14.30769230769218581, -9.528491918059723176, 34.59228464037033035 ) ) ;
#26842=ORIENTED_EDGE ( 'NONE', *, *, #8488, .F. ) ;
#26844=CARTESIAN_POINT ( 'NONE',  ( -7.846153846153965716, -11.48612834414049644, 32.76840700105863391 ) ) ;
#26845=CARTESIAN_POINT ( 'NONE',  ( -16.37671241690925683, -2.251424796025575770, 29.88072029997477586 ) ) ;
#26846=CYLINDRICAL_SURFACE ( 'NONE', #65867, 0.2499999999999994726 ) ;
#26847=CARTESIAN_POINT ( 'NONE',  ( 8.069165197766695385, -3.105924265160262543, 32.13625925475356127 ) ) ;
#26848=FACE_BOUND ( 'NONE', #29126, .T. ) ;
#26849=CARTESIAN_POINT ( 'NONE',  ( 13.38461538461538680, -11.91647553114624181, 32.58852847137148245 ) ) ;
#26850=CARTESIAN_POINT ( 'NONE',  ( -17.07692307692319744, -11.06231777344772027, 33.60647404775119895 ) ) ;
#26852=CARTESIAN_POINT ( 'NONE',  ( -5.749945688361683516, -9.943054286541403997, 34.11300777759954883 ) ) ;
#26853=CARTESIAN_POINT ( 'NONE',  ( -2.176901866725357682, -12.35292014791297710, 31.75344720912887198 ) ) ;
#26854=CARTESIAN_POINT ( 'NONE',  ( -18.00000000000012079, -10.21337939537710504, 33.94971097300076224 ) ) ;
#26857=CARTESIAN_POINT ( 'NONE',  ( -7.146561866800870355, -9.331801661448606566, 34.40259984581193464 ) ) ;
#26858=ORIENTED_EDGE ( 'NONE', *, *, #77256, .F. ) ;
#26860=VECTOR ( 'NONE', #43398, 999.9999999999998863 ) ;
#26861=ORIENTED_EDGE ( 'NONE', *, *, #29886, .F. ) ;
#26862=CARTESIAN_POINT ( 'NONE',  ( 7.846153846153846700, -4.102666532097928531, 36.13435417666054406 ) ) ;
#26863=EDGE_CURVE ( 'NONE', #77695, #75748, #33347, .T. ) ;
#26864=CYLINDRICAL_SURFACE ( 'NONE', #22919, 0.2499999999999994726 ) ;
#26865=CARTESIAN_POINT ( 'NONE',  ( -10.83886953994894498, -11.60425143139329940, 33.02411095842164457 ) ) ;
#26866=ORIENTED_EDGE ( 'NONE', *, *, #760, .T. ) ;
#26867=CARTESIAN_POINT ( 'NONE',  ( 3.230769230769231726, -6.386643153685126251, 34.62446782046654192 ) ) ;
#26868=CARTESIAN_POINT ( 'NONE',  ( 5.207713517890025123, -11.93129842949671726, 32.56571108434900452 ) ) ;
#26870=CARTESIAN_POINT ( 'NONE',  ( 1.134615384615387246, -2.499999999999998668, 29.75000000000000355 ) ) ;
#26871=LINE ( 'NONE', #20114, #50392 ) ;
#26872=CARTESIAN_POINT ( 'NONE',  ( -5.076923076923075762, -11.91647553114624181, 32.58852847137148245 ) ) ;
#26874=DIRECTION ( 'NONE',  ( 0.000000000000000000, 1.000000000000000000, 0.000000000000000000 ) ) ;
#26875=CARTESIAN_POINT ( 'NONE',  ( 11.66898724022510514, -3.816742781228458448, 33.13167719472716044 ) ) ;
#26878=CARTESIAN_POINT ( 'NONE',  ( 9.561697332683166906, -7.722926236386453702, 34.74524107206102030 ) ) ;
#26880=ORIENTED_EDGE ( 'NONE', *, *, #34662, .F. ) ;
#26882=FACE_OUTER_BOUND ( 'NONE', #66447, .T. ) ;
#26884=CARTESIAN_POINT ( 'NONE',  ( -16.02332071561251325, -12.50538340440932394, 31.33453814440721885 ) ) ;
#26886=VERTEX_POINT ( 'NONE', #17543 ) ;
#26887=DIRECTION ( 'NONE',  ( -0.000000000000000000, 0.9848077530122085754, -0.1736481776669273613 ) ) ;
#26888=CARTESIAN_POINT ( 'NONE',  ( 3.007284287045282056, -3.754499324213721234, 33.06261337010820256 ) ) ;
#26889=CARTESIAN_POINT ( 'NONE',  ( 2.177545098254090927, -2.882441371585227508, 31.66841991370171527 ) ) ;
#26891=CYLINDRICAL_SURFACE ( 'NONE', #61306, 0.2499999999999995559 ) ;
#26892=CARTESIAN_POINT ( 'NONE',  ( 15.36129466900288065, -5.915461855592780260, 34.75538340440931506 ) ) ;
#26893=CARTESIAN_POINT ( 'NONE',  ( -10.55012947587177941, -9.528491918058460186, 34.59228464037086326 ) ) ;
#26895=ORIENTED_EDGE ( 'NONE', *, *, #67497, .F. ) ;
#26896=CARTESIAN_POINT ( 'NONE',  ( 2.084765348785459160, -4.026226216239095379, 33.68668979543632958 ) ) ;
#26898=AXIS2_PLACEMENT_3D ( 'NONE', #42402, #15365, #9481 ) ;
#26899=CARTESIAN_POINT ( 'NONE',  ( 8.519207545009313876, -3.520140089381495585, 33.17453946501458262 ) ) ;
#26900=ORIENTED_EDGE ( 'NONE', *, *, #4580, .T. ) ;
#26901=EDGE_LOOP ( 'NONE', ( #9146, #75746, #75602, #61027 ) ) ;
#26902=EDGE_LOOP ( 'NONE', ( #27303, #85412, #27273, #16569 ) ) ;
#26903=EDGE_CURVE ( 'NONE', #58442, #50385, #44995, .T. ) ;
#26904=VERTEX_POINT ( 'NONE', #86916 ) ;
#26905=CARTESIAN_POINT ( 'NONE',  ( -9.915233909823840008, -2.758268499246657068, 31.33685645148948140 ) ) ;
#26906=CARTESIAN_POINT ( 'NONE',  ( 0.3308469948709010233, -2.541943142973490666, 30.39792223712631980 ) ) ;
#26907=EDGE_CURVE ( 'NONE', #46529, #292, #45444, .T. ) ;
#26908=VECTOR ( 'NONE', #35085, 999.9999999999998863 ) ;
#26909=CARTESIAN_POINT ( 'NONE',  ( -13.25382494364843389, -11.93129842949671726, 32.56571108434900452 ) ) ;
#26910=DIRECTION ( 'NONE',  ( 0.000000000000000000, 0.000000000000000000, 1.000000000000000000 ) ) ;
#26911=CARTESIAN_POINT ( 'NONE',  ( -17.75000000000000355, -7.500000000000000000, 35.00000000000000000 ) ) ;
#26912=ORIENTED_EDGE ( 'NONE', *, *, #11129, .F. ) ;
#26913=ORIENTED_EDGE ( 'NONE', *, *, #60481, .T. ) ;
#26914=EDGE_CURVE ( 'NONE', #86693, #57379, #12128, .T. ) ;
#26915=ORIENTED_EDGE ( 'NONE', *, *, #49145, .F. ) ;
#26916=CARTESIAN_POINT ( 'NONE',  ( -6.989159302437059296, -8.164416787775445883, 34.95778746994557906 ) ) ;
#26918=CARTESIAN_POINT ( 'NONE',  ( -1.384615384615383471, -2.833524468853757305, 32.15551576947925838 ) ) ;
#26919=B_SPLINE_CURVE_WITH_KNOTS ( 'NONE', 3,
 ( #49378, #15153, #34968, #21461, #15594, #43061, #70535, #28210, #29555, #57010 ),
 .UNSPECIFIED., .F., .F.,
 ( 4, 2, 2, 2, 4 ),
 ( 0.0007817359430256283796, 0.0009771253907249943717, 0.001172514838424360255, 0.001367904286123726356, 0.001563293733823092240 ),
 .UNSPECIFIED. ) ;
#26920=CARTESIAN_POINT ( 'NONE',  ( -10.86538461538461320, -7.500000000000001776, 34.75000000000000000 ) ) ;
#26921=B_SPLINE_CURVE_WITH_KNOTS ( 'NONE', 3,
 ( #44462, #44916, #2162, #30087, #50339, #77820, #37274, #16563, #71067, #71951 ),
 .UNSPECIFIED., .F., .F.,
 ( 4, 2, 2, 2, 4 ),
 ( 0.000000000000000000, 0.0001954339857564086941, 0.0003908679715128173882, 0.0005863019572692261365, 0.0007817359430256347764 ),
 .UNSPECIFIED. ) ;
#26923=LINE ( 'NONE', #68788, #88206 ) ;
#26924=CARTESIAN_POINT ( 'NONE',  ( 18.00000000000000000, -10.67929555188718282, 33.92786785259544047 ) ) ;
#26925=EDGE_LOOP ( 'NONE', ( #2338, #85152 ) ) ;
#26926=EDGE_CURVE ( 'NONE', #34444, #74304, #46263, .T. ) ;
#26928=ORIENTED_EDGE ( 'NONE', *, *, #58401, .F. ) ;
#26929=CARTESIAN_POINT ( 'NONE',  ( -10.68146699474474914, -10.67929555188718460, 33.92786785259543336 ) ) ;
#26931=ORIENTED_EDGE ( 'NONE', *, *, #13889, .T. ) ;
#26932=CARTESIAN_POINT ( 'NONE',  ( 6.700150705560775855, -6.503392248772476236, 34.64988816332204635 ) ) ;
#26933=ADVANCED_FACE ( 'NONE', ( #80132 ), #23827, .F. ) ;
#26934=ADVANCED_FACE ( 'NONE', ( #38699 ), #58961, .F. ) ;
#26935=CARTESIAN_POINT ( 'NONE',  ( -17.29985003582992320, -3.395401636524186362, 33.02366814457250399 ) ) ;
#26937=CYLINDRICAL_SURFACE ( 'NONE', #53201, 0.2500000000000012212 ) ;
#26938=CARTESIAN_POINT ( 'NONE',  ( -4.023054346021368133, -4.809403383903225304, 33.96459661697924304 ) ) ;
#26939=CARTESIAN_POINT ( 'NONE',  ( -8.769230769230768274, -1.629998284177014645, 34.34916445242399163 ) ) ;
#26940=ADVANCED_FACE ( 'NONE', ( #11229 ), #66160, .F. ) ;
#26941=FACE_BOUND ( 'NONE', #41267, .T. ) ;
#26943=B_SPLINE_CURVE_WITH_KNOTS ( 'NONE', 3,
 ( #6400, #19017, #74404, #12703, #61313, #88827, #66756, #46488, #27099, #54563 ),
 .UNSPECIFIED., .F., .F.,
 ( 4, 2, 2, 2, 4 ),
 ( 0.000000000000000000, 0.0001954311564186876063, 0.0003908623128373752125, 0.0005862934692560628188, 0.0007817246256747504250 ),
 .UNSPECIFIED. ) ;
#26944=CARTESIAN_POINT ( 'NONE',  ( 6.000000000000001776, -2.708943851104267164, 35.45975837776705220 ) ) ;
#26945=CARTESIAN_POINT ( 'NONE',  ( -0.4615384615384611200, -2.249999999999998668, 29.75000000000001776 ) ) ;
#26948=CARTESIAN_POINT ( 'NONE',  ( 18.24994551834813805, -4.336752205174650321, 33.62275283266504289 ) ) ;
#26949=LINE ( 'NONE', #88228, #59614 ) ;
#26951=ORIENTED_EDGE ( 'NONE', *, *, #47102, .F. ) ;
#26954=VERTEX_POINT ( 'NONE', #7135 ) ;
#26955=CARTESIAN_POINT ( 'NONE',  ( -14.30769230769242739, -5.219633306517616589, 34.19971097300220464 ) ) ;
#26957=ORIENTED_EDGE ( 'NONE', *, *, #42757, .T. ) ;
#26958=VECTOR ( 'NONE', #57285, 1000.000000000000114 ) ;
#26959=CARTESIAN_POINT ( 'NONE',  ( 11.28848479441294650, -10.06842814019191401, 34.32929386961144758 ) ) ;
#26960=CARTESIAN_POINT ( 'NONE',  ( -15.00798956179116317, -12.69155399931963046, 30.53255429739157734 ) ) ;
#26961=FACE_BOUND ( 'NONE', #13052, .T. ) ;
#26962=B_SPLINE_CURVE_WITH_KNOTS ( 'NONE', 3,
 ( #75632, #46838, #41417, #5862, #33336, #47279, #74769, #8519, #70657, #8963 ),
 .UNSPECIFIED., .F., .F.,
 ( 4, 2, 2, 2, 4 ),
 ( 0.000000000000000000, 0.0001954311564186876063, 0.0003908623128373752125, 0.0005862934692560628188, 0.0007817246256747504250 ),
 .UNSPECIFIED. ) ;
#26963=CARTESIAN_POINT ( 'NONE',  ( -18.06527044596078113, -3.300289026998416642, 32.46337939537583139 ) ) ;
#26964=CARTESIAN_POINT ( 'NONE',  ( -17.01173008862841840, -2.255955759149234741, 29.99999999999988276 ) ) ;
#26965=CARTESIAN_POINT ( 'NONE',  ( 10.61538461538461675, -8.120952969808772792, 34.71129190930000163 ) ) ;
#26966=CARTESIAN_POINT ( 'NONE',  ( 15.23076923076923173, -2.517432740324522911, 35.29906147534542527 ) ) ;
#26968=CARTESIAN_POINT ( 'NONE',  ( -18.00000000000000000, -11.10434399251292881, 35.99290692298802696 ) ) ;
#26969=B_SPLINE_CURVE_WITH_KNOTS ( 'NONE', 3,
 ( #57082, #62500, #49881, #84577, #83694, #43136, #50314, #71043, #42698, #23293 ),
 .UNSPECIFIED., .F., .F.,
 ( 4, 2, 2, 2, 4 ),
 ( 0.0007817359430256297891, 0.0009771253907249958896, 0.001172514838424361990, 0.001367904286123728091, 0.001563293733823094191 ),
 .UNSPECIFIED. ) ;
#26973=ORIENTED_EDGE ( 'NONE', *, *, #26280, .F. ) ;
#26974=FACE_OUTER_BOUND ( 'NONE', #51605, .T. ) ;
#26975=AXIS2_PLACEMENT_3D ( 'NONE', #32088, #57779, #44239 ) ;
#26976=CARTESIAN_POINT ( 'NONE',  ( -8.769230769230768274, -4.102666532097928531, 36.13435417666054406 ) ) ;
#26977=CARTESIAN_POINT ( 'NONE',  ( -13.38461538461538325, -13.78497067705608181, 32.30358669280327177 ) ) ;
#26978=CARTESIAN_POINT ( 'NONE',  ( 6.856993512121043466, -12.10708131394839349, 31.69288490824020244 ) ) ;
#26979=FACE_OUTER_BOUND ( 'NONE', #79325, .T. ) ;
#26983=FACE_OUTER_BOUND ( 'NONE', #80056, .T. ) ;
#26984=CARTESIAN_POINT ( 'NONE',  ( -2.307692307692305711, -5.557115091759785130, 34.35708131394839171 ) ) ;
#26985=CARTESIAN_POINT ( 'NONE',  ( -5.999999999999998224, -2.721908614388771852, 31.22303859784724978 ) ) ;
#26986=DIRECTION ( 'NONE',  ( 0.000000000000000000, 0.4999999999999985567, 0.8660254037844395958 ) ) ;
#26987=DIRECTION ( 'NONE',  ( -0.000000000000000000, -0.8660254037844397068, -0.4999999999999978906 ) ) ;
#26988=CARTESIAN_POINT ( 'NONE',  ( 2.242369392200134204, -7.749976743299137993, 34.99404534957040624 ) ) ;
#26989=CARTESIAN_POINT ( 'NONE',  ( -12.68440388374210315, -2.501496062324912284, 29.88072118266895671 ) ) ;
#26990=ORIENTED_EDGE ( 'NONE', *, *, #10914, .F. ) ;
#26991=CARTESIAN_POINT ( 'NONE',  ( 1.319344938654610333, -2.625532179533444754, 30.86335684631481513 ) ) ;
#26994=CARTESIAN_POINT ( 'NONE',  ( -9.942330916529149576, -10.92453946501458795, 33.72985991061850086 ) ) ;
#26995=AXIS2_PLACEMENT_3D ( 'NONE', #76472, #54867, #6677 ) ;
#26996=DIRECTION ( 'NONE',  ( -0.000000000000000000, -0.9848077530122085754, -0.1736481776669273613 ) ) ;
#26997=CARTESIAN_POINT ( 'NONE',  ( -1.253823576790597194, -4.118422570099827595, 33.43335022499816489 ) ) ;
#26998=EDGE_LOOP ( 'NONE', ( #6447, #43203, #3537, #77746 ) ) ;
#27000=CARTESIAN_POINT ( 'NONE',  ( -15.23076923076935074, -12.46129190930018460, 30.37095296980731973 ) ) ;
#27001=EDGE_LOOP ( 'NONE', ( #25800, #22204 ) ) ;
#27002=B_SPLINE_CURVE_WITH_KNOTS ( 'NONE', 3,
 ( #84128, #43128, #51174, #64708, #22406, #83684, #9344, #2562, #64262, #49440 ),
 .UNSPECIFIED., .F., .F.,
 ( 4, 2, 2, 2, 4 ),
 ( 0.0007817246256747453293, 0.0009771112852218889842, 0.001172497944769032747, 0.001367884604316176294, 0.001563271263863320057 ),
 .UNSPECIFIED. ) ;
#27003=CARTESIAN_POINT ( 'NONE',  ( -15.90390063549801347, -10.05730279482229683, 34.04704008940765902 ) ) ;
#27004=CARTESIAN_POINT ( 'NONE',  ( -6.923076923076922462, -11.35647404775217417, 33.31231777344666511 ) ) ;
#27005=ORIENTED_EDGE ( 'NONE', *, *, #39872, .T. ) ;
#27009=CARTESIAN_POINT ( 'NONE',  ( -7.976301055592065481, -3.817052484675422797, 33.13202310037935661 ) ) ;
#27010=ORIENTED_EDGE ( 'NONE', *, *, #29496, .F. ) ;
#27011=ORIENTED_EDGE ( 'NONE', *, *, #55103, .T. ) ;
#27012=CYLINDRICAL_SURFACE ( 'NONE', #16819, 0.2500000000000002220 ) ;
#27013=EDGE_CURVE ( 'NONE', #80537, #37045, #39893, .T. ) ;
#27014=VERTEX_POINT ( 'NONE', #55310 ) ;
#27015=CARTESIAN_POINT ( 'NONE',  ( -7.846153846153967493, -2.379036618888197729, 30.90682066428292885 ) ) ;
#27016=DIRECTION ( 'NONE',  ( -0.000000000000000000, 0.9396926207859093161, -0.3420201433256663259 ) ) ;
#27017=CARTESIAN_POINT ( 'NONE',  ( -5.999999999999998224, -2.708943851104267164, 35.45975837776705220 ) ) ;
#27019=CARTESIAN_POINT ( 'NONE',  ( 15.10007776410167324, -6.413092428213692742, 34.63065189839063152 ) ) ;
#27020=CARTESIAN_POINT ( 'NONE',  ( 4.153846153846154188, -12.37446782046654192, 30.86335684631486131 ) ) ;
#27021=CARTESIAN_POINT ( 'NONE',  ( -0.3954711281883850904, -12.34228464037088813, 31.77849191805839268 ) ) ;
#27023=EDGE_CURVE ( 'NONE', #12236, #35073, #22648, .T. ) ;
#27024=EDGE_LOOP ( 'NONE', ( #4577, #28228, #62241, #8690 ) ) ;
#27025=CARTESIAN_POINT ( 'NONE',  ( -17.20707028636129721, -10.19110544564092002, 33.96427741523702792 ) ) ;
#27027=VECTOR ( 'NONE', #53060, 1000.000000000000227 ) ;
#27029=CARTESIAN_POINT ( 'NONE',  ( -8.703163435880695076, -10.67929555188718282, 33.92786785259544757 ) ) ;
#27030=FACE_OUTER_BOUND ( 'NONE', #15836, .T. ) ;
#27031=ORIENTED_EDGE ( 'NONE', *, *, #70670, .T. ) ;
#27032=CARTESIAN_POINT ( 'NONE',  ( 14.30769230769218581, -12.16647553114689728, 32.15551576947799362 ) ) ;
#27033=EDGE_LOOP ( 'NONE', ( #65760, #30814 ) ) ;
#27034=CARTESIAN_POINT ( 'NONE',  ( 0.3962874713772188695, -2.506253911140460922, 30.00000000000013856 ) ) ;
#27035=EDGE_LOOP ( 'NONE', ( #79294, #8308 ) ) ;
#27036=B_SPLINE_CURVE_WITH_KNOTS ( 'NONE', 3,
 ( #8568, #479, #56744, #15325, #21183, #63497, #69382, #71137, #1356, #42804 ),
 .UNSPECIFIED., .F., .F.,
 ( 4, 2, 2, 2, 4 ),
 ( 0.000000000000000000, 0.0001954339857564072033, 0.0003908679715128144066, 0.0005863019572692215828, 0.0007817359430256288133 ),
 .UNSPECIFIED. ) ;
#27037=CARTESIAN_POINT ( 'NONE',  ( -14.05763788777885281, -12.01375889529407281, 32.43194544308182969 ) ) ;
#27039=EDGE_CURVE ( 'NONE', #64392, #15864, #4300, .T. ) ;
#27040=ORIENTED_EDGE ( 'NONE', *, *, #87265, .F. ) ;
#27041=CARTESIAN_POINT ( 'NONE',  ( -4.284536756956462966, -3.957541250942359756, 33.62499894934981626 ) ) ;
#27042=CARTESIAN_POINT ( 'NONE',  ( 16.85343813319913053, -2.847400154188068910, 31.58180166144859768 ) ) ;
#27043=FACE_BOUND ( 'NONE', #35567, .T. ) ;
#27044=CARTESIAN_POINT ( 'NONE',  ( -14.53061926659915315, -9.172386477786396597, 34.72672124145550043 ) ) ;
#27045=CARTESIAN_POINT ( 'NONE',  ( 1.318861956302054939, -7.249945578846654470, 34.99404164642496795 ) ) ;
#27046=CARTESIAN_POINT ( 'NONE',  ( 13.38461538461526423, -5.094484230521993062, 34.41647553114689373 ) ) ;
#27047=CARTESIAN_POINT ( 'NONE',  ( 1.161130460051053692, -12.47654668319379567, 31.42292124445336654 ) ) ;
#27048=DIRECTION ( 'NONE',  ( -0.000000000000000000, -0.6427876096865404731, -0.7660444431189771253 ) ) ;
#27049=CARTESIAN_POINT ( 'NONE',  ( 15.93091993633000136, -4.186968288167451036, 33.49512374952580274 ) ) ;
#27050=FACE_OUTER_BOUND ( 'NONE', #82749, .T. ) ;
#27051=EDGE_CURVE ( 'NONE', #49709, #8288, #81477, .T. ) ;
#27052=ORIENTED_EDGE ( 'NONE', *, *, #59031, .T. ) ;
#27053=ORIENTED_EDGE ( 'NONE', *, *, #72925, .T. ) ;
#27054=VECTOR ( 'NONE', #55254, 1000.000000000000114 ) ;
#27055=CARTESIAN_POINT ( 'NONE',  ( -5.326899820971665811, -12.01397095200673881, 32.43157075238190146 ) ) ;
#27056=CARTESIAN_POINT ( 'NONE',  ( -18.25002322422145440, -10.18141759479407327, 34.26406193332782379 ) ) ;
#27057=LINE ( 'NONE', #38801, #29854 ) ;
#27058=CARTESIAN_POINT ( 'NONE',  ( 3.230769230769110045, -10.90142922262034020, 33.41473453929536674 ) ) ;
#27060=CARTESIAN_POINT ( 'NONE',  ( -12.46153846153858424, -5.094484230521993062, 34.41647553114689373 ) ) ;
#27061=ORIENTED_EDGE ( 'NONE', *, *, #74142, .F. ) ;
#27062=CARTESIAN_POINT ( 'NONE',  ( -11.60373198442231235, -12.27809138561121394, 31.22303859784730307 ) ) ;
#27064=CARTESIAN_POINT ( 'NONE',  ( 0.5276068125408998055, -9.780366693483669494, 34.19971097300155805 ) ) ;
#27065=CARTESIAN_POINT ( 'NONE',  ( -3.360917200500926239, -11.66186481527757479, 32.95055677023626117 ) ) ;
#27066=CARTESIAN_POINT ( 'NONE',  ( 7.846153846153725020, -10.90142922262034020, 33.41473453929536674 ) ) ;
#27067=ORIENTED_EDGE ( 'NONE', *, *, #21776, .T. ) ;
#27070=CARTESIAN_POINT ( 'NONE',  ( 0.4615384615384611200, -10.51840700105979565, 33.73612834413961536 ) ) ;
#27071=ORIENTED_EDGE ( 'NONE', *, *, #62570, .F. ) ;
#27073=CARTESIAN_POINT ( 'NONE',  ( 15.00784301325308157, -9.086856451489515152, 34.49173150075333183 ) ) ;
#27074=CARTESIAN_POINT ( 'NONE',  ( 3.453782074862625340, -10.01129605718032778, 34.36064277460058491 ) ) ;
#27076=CARTESIAN_POINT ( 'NONE',  ( 14.55774661933062575, -4.235687564193448829, 33.53795663066793509 ) ) ;
#27078=CARTESIAN_POINT ( 'NONE',  ( 4.376625695114563008, -4.387253974876676565, 33.66317474335728832 ) ) ;
#27079=CARTESIAN_POINT ( 'NONE',  ( -13.25408968285182176, -4.459921816937791661, 33.71989282347011851 ) ) ;
#27080=EDGE_LOOP ( 'NONE', ( #63627, #32007, #87135, #13595 ) ) ;
#27081=CARTESIAN_POINT ( 'NONE',  ( -5.207071046654771607, -2.373036134822904319, 30.88089517874952250 ) ) ;
#27082=CARTESIAN_POINT ( 'NONE',  ( 8.834485908743607396, -12.51329471203373345, 31.30864560766537963 ) ) ;
#27083=CARTESIAN_POINT ( 'NONE',  ( -11.53846153846153655, -7.500000000000001776, 35.04278698407183867 ) ) ;
#27084=CARTESIAN_POINT ( 'NONE',  ( 8.769230769230645706, -12.16647553114689728, 32.15551576947799362 ) ) ;
#27085=CARTESIAN_POINT ( 'NONE',  ( -12.46153846153846168, -2.721908614388771852, 31.22303859784724978 ) ) ;
#27086=CARTESIAN_POINT ( 'NONE',  ( -5.300408001487409315, -10.97335522853832579, 33.68706563782419749 ) ) ;
#27087=CARTESIAN_POINT ( 'NONE',  ( -0.5276218724943422256, -12.37446782046654192, 30.86335684631486487 ) ) ;
#27089=ORIENTED_EDGE ( 'NONE', *, *, #88469, .F. ) ;
#27090=AXIS2_PLACEMENT_3D ( 'NONE', #81343, #48313, #7344 ) ;
#27091=DIRECTION ( 'NONE',  ( -0.000000000000000000, 0.9848077530122086864, -0.1736481776669273891 ) ) ;
#27093=B_SPLINE_CURVE_WITH_KNOTS ( 'NONE', 3,
 ( #23544, #2821, #37958, #30314, #65426, #58661, #57783, #45149, #72625, #10933 ),
 .UNSPECIFIED., .F., .F.,
 ( 4, 2, 2, 2, 4 ),
 ( 0.0007817359430256318490, 0.0009771253907249984917, 0.001172514838424365026, 0.001367904286123731560, 0.001563293733823098094 ),
 .UNSPECIFIED. ) ;
#27094=CARTESIAN_POINT ( 'NONE',  ( 9.915087361285756629, -10.97394488606064122, 33.68653795673694873 ) ) ;
#27095=ORIENTED_EDGE ( 'NONE', *, *, #25243, .T. ) ;
#27096=CARTESIAN_POINT ( 'NONE',  ( 2.177217122616589950, -7.276987145209184327, 34.99546412871779211 ) ) ;
#27097=CARTESIAN_POINT ( 'NONE',  ( -3.099977422944443006, -5.582136614379148654, 34.36778462344220486 ) ) ;
#27098=ADVANCED_FACE ( 'NONE', ( #32833 ), #53536, .F. ) ;
#27099=CARTESIAN_POINT ( 'NONE',  ( -10.68065461594093435, -2.379036618887870436, 30.90682066428147934 ) ) ;
#27100=DIRECTION ( 'NONE',  ( -0.000000000000000000, 0.9848077530122086864, -0.1736481776669273891 ) ) ;
#27101=CARTESIAN_POINT ( 'NONE',  ( 1.384615384615386802, -6.343179335718451384, 34.87096338111211935 ) ) ;
#27102=ORIENTED_EDGE ( 'NONE', *, *, #65168, .T. ) ;
#27103=CARTESIAN_POINT ( 'NONE',  ( 17.01083966596719321, -3.050289026998445951, 32.03036669348365706 ) ) ;
#27105=CARTESIAN_POINT ( 'NONE',  ( 7.596130608860880429, -10.05641848906368097, 34.04755513067966177 ) ) ;
#27106=ORIENTED_EDGE ( 'NONE', *, *, #82211, .T. ) ;
#27108=B_SPLINE_CURVE_WITH_KNOTS ( 'NONE', 3,
 ( #50440, #44116, #36502, #70730, #63954, #58085, #37818, #71595, #1819, #23410 ),
 .UNSPECIFIED., .F., .F.,
 ( 4, 2, 2, 2, 4 ),
 ( 0.000000000000000000, 0.0001954339857564054144, 0.0003908679715128108288, 0.0005863019572692162703, 0.0007817359430256216575 ),
 .UNSPECIFIED. ) ;
#27109=EDGE_CURVE ( 'NONE', #27279, #80982, #85969, .T. ) ;
#27110=ORIENTED_EDGE ( 'NONE', *, *, #76555, .T. ) ;
#27111=AXIS2_PLACEMENT_3D ( 'NONE', #38716, #58089, #66176 ) ;
#27112=CARTESIAN_POINT ( 'NONE',  ( -16.40382288478850725, -5.728515186090277211, 34.42611988154120439 ) ) ;
#27113=CARTESIAN_POINT ( 'NONE',  ( -5.933932666649922361, -11.91647553114624358, 32.58852847137148245 ) ) ;
#27114=EDGE_LOOP ( 'NONE', ( #7747, #83113 ) ) ;
#27115=EDGE_CURVE ( 'NONE', #42284, #22567, #54876, .T. ) ;
#27116=CARTESIAN_POINT ( 'NONE',  ( 0.4615384615384611200, -11.11383981884818262, 36.00935417666054406 ) ) ;
#27117=DIRECTION ( 'NONE',  ( -0.000000000000000000, 1.000000000000000000, 3.491481338843133355E-15 ) ) ;
#27118=CARTESIAN_POINT ( 'NONE',  ( -6.673131513698879580, -12.45601412856602863, 31.48342859153981621 ) ) ;
#27119=AXIS2_PLACEMENT_3D ( 'NONE', #80978, #32335, #12074 ) ;
#27120=AXIS2_PLACEMENT_3D ( 'NONE', #16002, #14669, #43466 ) ;
#27121=CARTESIAN_POINT ( 'NONE',  ( 15.23076923076911093, -3.835265460704628371, 33.15142922262033665 ) ) ;
#27122=CARTESIAN_POINT ( 'NONE',  ( -2.176901866725355905, -10.70102852606553157, 33.91149625220312913 ) ) ;
#27124=EDGE_LOOP ( 'NONE', ( #56987, #73619, #42729, #46409 ) ) ;
#27125=B_SPLINE_CURVE_WITH_KNOTS ( 'NONE', 3,
 ( #11910, #39824, #11013, #59190, #12786, #86241, #67293, #4249, #25860, #18668 ),
 .UNSPECIFIED., .F., .F.,
 ( 4, 2, 2, 2, 4 ),
 ( 0.000000000000000000, 0.0001954311564186862781, 0.0003908623128373725562, 0.0005862934692560588072, 0.0007817246256747451124 ),
 .UNSPECIFIED. ) ;
#27126=EDGE_CURVE ( 'NONE', #26386, #72566, #54877, .T. ) ;
#27127=FACE_BOUND ( 'NONE', #66656, .T. ) ;
#27128=EDGE_LOOP ( 'NONE', ( #83722, #60807, #51211, #21551 ) ) ;
#27130=ADVANCED_FACE ( 'NONE', ( #77797 ), #76480, .F. ) ;
#27131=CARTESIAN_POINT ( 'NONE',  ( 18.13052543823364360, -6.808710257144159783, 34.95449254468098843 ) ) ;
#27132=CARTESIAN_POINT ( 'NONE',  ( 6.223012844093395834, -5.582272713120727481, 34.63742843783360570 ) ) ;
#27133=CARTESIAN_POINT ( 'NONE',  ( -6.000000000000119904, -12.27809138561165270, 31.22303859784587132 ) ) ;
#27135=VERTEX_POINT ( 'NONE', #41815 ) ;
#27136=ORIENTED_EDGE ( 'NONE', *, *, #29298, .T. ) ;
#27137=VERTEX_POINT ( 'NONE', #70604 ) ;
#27139=CARTESIAN_POINT ( 'NONE',  ( -4.854143535654666941, -5.114059244376869984, 34.14424750095245287 ) ) ;
#27141=AXIS2_PLACEMENT_3D ( 'NONE', #8353, #35827, #22303 ) ;
#27142=CARTESIAN_POINT ( 'NONE',  ( -15.23076923076935074, -10.90142922262034020, 33.41473453929536674 ) ) ;
#27143=CARTESIAN_POINT ( 'NONE',  ( -1.384615384615505151, -10.90142922262034020, 33.41473453929536674 ) ) ;
#27144=CARTESIAN_POINT ( 'NONE',  ( 17.93391658904412012, -9.780366693483667717, 34.19971097300155805 ) ) ;
#27145=EDGE_CURVE ( 'NONE', #25133, #24082, #3334, .T. ) ;
#27146=CARTESIAN_POINT ( 'NONE',  ( -0.6844646790546091708, -11.76352882383564769, 32.36236540154569497 ) ) ;
#27148=DIRECTION ( 'NONE',  ( 0.000000000000000000, 0.6427876096865368094, 0.7660444431189802339 ) ) ;
#27149=CARTESIAN_POINT ( 'NONE',  ( 11.40777007179398339, -9.804603061927743113, 34.18744698557895845 ) ) ;
#27150=ORIENTED_EDGE ( 'NONE', *, *, #77421, .F. ) ;
#27151=ORIENTED_EDGE ( 'NONE', *, *, #42999, .F. ) ;
#27152=B_SPLINE_CURVE_WITH_KNOTS ( 'NONE', 3,
 ( #63928, #77893, #16196, #44534, #43661, #71132, #37340, #3113, #85543, #30587 ),
 .UNSPECIFIED., .F., .F.,
 ( 4, 2, 2, 2, 4 ),
 ( 0.0007817359430256400890, 0.0009771253907250091169, 0.001172514838424378253, 0.001367904286123747173, 0.001563293733823116309 ),
 .UNSPECIFIED. ) ;
#27153=ORIENTED_EDGE ( 'NONE', *, *, #52963, .T. ) ;
#27154=CARTESIAN_POINT ( 'NONE',  ( -13.51476335434708709, -12.50552854090298993, 31.33409797877408920 ) ) ;
#27155=LINE ( 'NONE', #74911, #43243 ) ;
#27156=CARTESIAN_POINT ( 'NONE',  ( -9.757577692864012775, -4.320704448112771878, 33.92786785259540494 ) ) ;
#27159=FACE_BOUND ( 'NONE', #28850, .T. ) ;
#27160=ORIENTED_EDGE ( 'NONE', *, *, #81336, .T. ) ;
#27162=DIRECTION ( 'NONE',  ( 0.000000000000000000, 0.1736481776669275834, 0.9848077530122086864 ) ) ;
#27163=CARTESIAN_POINT ( 'NONE',  ( 2.980745993476265898, -10.76384336483936011, 33.53834819971076087 ) ) ;
#27164=VERTEX_POINT ( 'NONE', #28282 ) ;
#27165=LINE ( 'NONE', #53300, #34186 ) ;
#27166=ORIENTED_EDGE ( 'NONE', *, *, #57836, .T. ) ;
#27167=FACE_BOUND ( 'NONE', #2100, .T. ) ;
#27168=CARTESIAN_POINT ( 'NONE',  ( 9.442284455014730682, -5.851115903089112003, 34.47074536777953568 ) ) ;
#27169=VECTOR ( 'NONE', #18722, 1000.000000000000000 ) ;
#27170=ORIENTED_EDGE ( 'NONE', *, *, #52473, .F. ) ;
#27173=CARTESIAN_POINT ( 'NONE',  ( 1.318531973659506029, -3.050289026998445951, 32.03036669348365706 ) ) ;
#27174=EDGE_LOOP ( 'NONE', ( #14735, #53305, #20432, #75422 ) ) ;
#27175=CARTESIAN_POINT ( 'NONE',  ( -2.307692307692305711, -2.249999999999998668, 29.75000000000001776 ) ) ;
#27176=CARTESIAN_POINT ( 'NONE',  ( -7.623374177175779032, -8.540255544307065350, 34.89611431652622286 ) ) ;
#27177=CARTESIAN_POINT ( 'NONE',  ( 12.52679403281448600, -6.879047030191282275, 34.71129190930002295 ) ) ;
#27178=CARTESIAN_POINT ( 'NONE',  ( 2.557637717070351702, -2.986452184633681117, 32.43230066228895225 ) ) ;
#27179=ORIENTED_EDGE ( 'NONE', *, *, #2428, .T. ) ;
#27181=CARTESIAN_POINT ( 'NONE',  ( -5.076923076923075762, -4.661471528628507777, 34.16647553114623292 ) ) ;
#27182=CARTESIAN_POINT ( 'NONE',  ( -15.29685264172511161, -4.098570777380719399, 33.41473453929634729 ) ) ;
#27183=VECTOR ( 'NONE', #46358, 1000.000000000000114 ) ;
#27184=CARTESIAN_POINT ( 'NONE',  ( -8.769230769230890843, -3.835265460704628371, 33.15142922262033665 ) ) ;
#27185=ORIENTED_EDGE ( 'NONE', *, *, #61436, .T. ) ;
#27186=CARTESIAN_POINT ( 'NONE',  ( 2.438217745925953750, -10.31582465632705237, 34.18122507451815295 ) ) ;
#27187=CARTESIAN_POINT ( 'NONE',  ( 16.15384615384603251, -4.320704448113951379, 33.92786785259630022 ) ) ;
#27188=CARTESIAN_POINT ( 'NONE',  ( -13.31854703361294590, -4.786620604624113540, 33.94971097300155805 ) ) ;
#27189=CARTESIAN_POINT ( 'NONE',  ( -5.076923076923075762, -2.249999999999998668, 29.75000000000001776 ) ) ;
#27190=CARTESIAN_POINT ( 'NONE',  ( 3.230769230769108269, -12.51329471203414379, 31.30864560766407578 ) ) ;
#27191=EDGE_CURVE ( 'NONE', #80196, #66304, #26969, .T. ) ;
#27192=CARTESIAN_POINT ( 'NONE',  ( 16.94677510719138169, -5.070767119584671079, 34.40440758774516183 ) ) ;
#27193=CARTESIAN_POINT ( 'NONE',  ( 0.6843181305165255690, -11.60474049983370648, 33.02348890104160262 ) ) ;
#27194=CARTESIAN_POINT ( 'NONE',  ( 3.230769230769108269, -11.06231777344772027, 33.60647404775119895 ) ) ;
#27195=VECTOR ( 'NONE', #66944, 999.9999999999998863 ) ;
#27196=CARTESIAN_POINT ( 'NONE',  ( -6.700065571464075553, -2.758310577978207778, 31.33698337089303010 ) ) ;
#27198=ORIENTED_EDGE ( 'NONE', *, *, #80206, .F. ) ;
#27199=LINE ( 'NONE', #7819, #27536 ) ;
#27200=EDGE_LOOP ( 'NONE', ( #60517, #60498 ) ) ;
#27201=B_SPLINE_CURVE_WITH_KNOTS ( 'NONE', 3,
 ( #71134, #64367, #57625, #16633, #50843, #86455, #31940, #85107, #17535, #23388 ),
 .UNSPECIFIED., .F., .F.,
 ( 4, 2, 2, 2, 4 ),
 ( 0.000000000000000000, 0.0001954339857564076912, 0.0003908679715128153824, 0.0005863019572692231007, 0.0007817359430256307648 ),
 .UNSPECIFIED. ) ;
#27202=VERTEX_POINT ( 'NONE', #83239 ) ;
#27203=CARTESIAN_POINT ( 'NONE',  ( -11.31544869436814338, -2.308499170217967134, 30.53291367094873721 ) ) ;
#27204=ORIENTED_EDGE ( 'NONE', *, *, #9072, .T. ) ;
#27205=CARTESIAN_POINT ( 'NONE',  ( 1.450682717965462665, -11.91647553114624358, 32.58852847137148245 ) ) ;
#27207=CARTESIAN_POINT ( 'NONE',  ( 13.60762673622823371, -2.758310577978208666, 31.33698337089302299 ) ) ;
#27208=CARTESIAN_POINT ( 'NONE',  ( -7.846153846153844924, -8.164416787775445883, 34.95778746994557906 ) ) ;
#27209=CARTESIAN_POINT ( 'NONE',  ( 7.715593932540479649, -2.254533558242299396, 29.97296025877827930 ) ) ;
#27210=EDGE_CURVE ( 'NONE', #30445, #83962, #31256, .T. ) ;
#27211=DIRECTION ( 'NONE',  ( -0.000000000000000000, 0.6427876096865404731, -0.7660444431189770143 ) ) ;
#27212=CARTESIAN_POINT ( 'NONE',  ( -4.153846153846152411, -1.790695186598648903, 34.54067556320373455 ) ) ;
#27213=CARTESIAN_POINT ( 'NONE',  ( 2.242421861731533017, -10.21337939537584383, 33.94971097300158647 ) ) ;
#27214=DIRECTION ( 'NONE',  ( -0.000000000000000000, 0.1736481776669307198, -0.9848077530122080203 ) ) ;
#27216=CARTESIAN_POINT ( 'NONE',  ( -17.07692307692319744, -11.06231777344772027, 33.60647404775119895 ) ) ;
#27217=CARTESIAN_POINT ( 'NONE',  ( 14.55769230769231015, -2.499999999999998668, 29.75000000000000355 ) ) ;
#27218=VECTOR ( 'NONE', #40119, 1000.000000000000000 ) ;
#27219=EDGE_CURVE ( 'NONE', #47929, #33434, #21529, .T. ) ;
#27220=VERTEX_POINT ( 'NONE', #35490 ) ;
#27221=VERTEX_POINT ( 'NONE', #56205 ) ;
#27222=CARTESIAN_POINT ( 'NONE',  ( -14.98082371242109012, -8.433404298154334455, 34.66254593164985920 ) ) ;
#27223=CYLINDRICAL_SURFACE ( 'NONE', #76222, 0.2499999999999994726 ) ;
#27224=CARTESIAN_POINT ( 'NONE',  ( -6.857009589726848375, -11.91647553114624358, 32.58852847137148245 ) ) ;
#27225=CARTESIAN_POINT ( 'NONE',  ( 9.692307692307570832, -12.16647553114689728, 32.15551576947799362 ) ) ;
#27226=ADVANCED_FACE ( 'NONE', ( #21978 ), #49449, .F. ) ;
#27227=DIRECTION ( 'NONE',  ( 0.000000000000000000, 0.8660254037844377084, 0.5000000000000015543 ) ) ;
#27228=CARTESIAN_POINT ( 'NONE',  ( 11.66925197942849302, -3.957578996910242619, 33.62503395064540257 ) ) ;
#27229=DIRECTION ( 'NONE',  ( -0.000000000000000000, 0.6427876096865404731, -0.7660444431189771253 ) ) ;
#27231=ADVANCED_FACE ( 'NONE', ( #52977 ), #42028, .T. ) ;
#27232=CARTESIAN_POINT ( 'NONE',  ( 16.08776274289027342, -2.721908614388770964, 31.22303859784723912 ) ) ;
#27233=ORIENTED_EDGE ( 'NONE', *, *, #66581, .T. ) ;
#27234=CARTESIAN_POINT ( 'NONE',  ( -14.55769230769230838, -7.433931650972299465, 34.75000000000000711 ) ) ;
#27236=DIRECTION ( 'NONE',  ( -0.000000000000000000, 0.9396926207859092051, -0.3420201433256662704 ) ) ;
#27237=CARTESIAN_POINT ( 'NONE',  ( -4.284537620513710010, -4.118384482072085184, 33.43331474514187107 ) ) ;
#27238=CARTESIAN_POINT ( 'NONE',  ( 3.007284306204900837, -8.539481045369598178, 34.89627647299170832 ) ) ;
#27239=CARTESIAN_POINT ( 'NONE',  ( -7.846153846153844924, -6.681629849574314051, 35.83090037661290239 ) ) ;
#27240=AXIS2_PLACEMENT_3D ( 'NONE', #47232, #74724, #19771 ) ;
#27241=VECTOR ( 'NONE', #8540, 1000.000000000000000 ) ;
#27242=ORIENTED_EDGE ( 'NONE', *, *, #10777, .T. ) ;
#27243=AXIS2_PLACEMENT_3D ( 'NONE', #76728, #70418, #8721 ) ;
#27244=ORIENTED_EDGE ( 'NONE', *, *, #86033, .F. ) ;
#27245=VERTEX_POINT ( 'NONE', #25522 ) ;
#27246=ORIENTED_EDGE ( 'NONE', *, *, #86706, .F. ) ;
#27247=ADVANCED_FACE ( 'NONE', ( #51183 ), #16985, .F. ) ;
#27248=CYLINDRICAL_SURFACE ( 'NONE', #74640, 0.2499999999999979738 ) ;
#27249=CARTESIAN_POINT ( 'NONE',  ( -16.15384615384615330, -9.058645607665452459, 34.76329471203371924 ) ) ;
#27250=CARTESIAN_POINT ( 'NONE',  ( -3.454254174493178731, -10.11188796281391511, 34.01382737946119050 ) ) ;
#27251=EDGE_CURVE ( 'NONE', #2835, #4865, #65161, .T. ) ;
#27252=CARTESIAN_POINT ( 'NONE',  ( -15.23076923076935074, -11.48612834414049644, 32.76840700105863391 ) ) ;
#27254=ADVANCED_FACE ( 'NONE', ( #30497 ), #10677, .F. ) ;
#27255=CARTESIAN_POINT ( 'NONE',  ( 2.307692307692309264, -1.129524287112498415, 32.06866353760679544 ) ) ;
#27256=EDGE_LOOP ( 'NONE', ( #14733, #24698, #78190, #49207 ) ) ;
#27257=VERTEX_POINT ( 'NONE', #58396 ) ;
#27258=ORIENTED_EDGE ( 'NONE', *, *, #8581, .T. ) ;
#27259=CARTESIAN_POINT ( 'NONE',  ( 11.40831432902331954, -9.418419913701741919, 34.36755862841477693 ) ) ;
#27260=VERTEX_POINT ( 'NONE', #66509 ) ;
#27261=CARTESIAN_POINT ( 'NONE',  ( 17.14217821643591932, -11.06231777344670952, 33.60647404775212266 ) ) ;
#27262=CARTESIAN_POINT ( 'NONE',  ( -2.177166605928742005, -9.417988943895561960, 34.36773134775778260 ) ) ;
#27264=EDGE_LOOP ( 'NONE', ( #64888, #8714, #34499, #78342 ) ) ;
#27265=EDGE_CURVE ( 'NONE', #7759, #62397, #18348, .T. ) ;
#27266=CARTESIAN_POINT ( 'NONE',  ( -1.318548051265308274, -2.486705287966280320, 31.30864560766543647 ) ) ;
#27267=AXIS2_PLACEMENT_3D ( 'NONE', #62498, #35039, #38034 ) ;
#27268=ORIENTED_EDGE ( 'NONE', *, *, #71332, .F. ) ;
#27269=CARTESIAN_POINT ( 'NONE',  ( 7.912222197156284054, -12.10708131394839349, 31.69288490824020244 ) ) ;
#27270=FACE_BOUND ( 'NONE', #60098, .T. ) ;
#27271=CARTESIAN_POINT ( 'NONE',  ( -2.307692307692428724, -5.094484230521993062, 34.41647553114689373 ) ) ;
#27272=CARTESIAN_POINT ( 'NONE',  ( -14.30769230769199929, -2.506253911140614576, 30.00000000000323297 ) ) ;
#27273=ORIENTED_EDGE ( 'NONE', *, *, #16557, .T. ) ;
#27274=EDGE_CURVE ( 'NONE', #43614, #87443, #17219, .T. ) ;
#27275=CARTESIAN_POINT ( 'NONE',  ( 8.703148389870630552, -11.91647553114624181, 32.58852847137148245 ) ) ;
#27276=CARTESIAN_POINT ( 'NONE',  ( 6.856994543716788293, -11.91647553114624181, 32.58852847137148245 ) ) ;
#27277=CARTESIAN_POINT ( 'NONE',  ( 16.28437159207980045, -6.808710257144159783, 34.95449254468098843 ) ) ;
#27278=CARTESIAN_POINT ( 'NONE',  ( 15.29602437028206907, -6.835583212224610072, 34.95778746994559327 ) ) ;
#27279=VERTEX_POINT ( 'NONE', #24628 ) ;
#27280=B_SPLINE_CURVE_WITH_KNOTS ( 'NONE', 3,
 ( #3267, #44687, #10485, #70861, #29871, #36627, #30739, #72170, #28997, #1513 ),
 .UNSPECIFIED., .F., .F.,
 ( 4, 2, 2, 2, 4 ),
 ( 0.0007817246256747517261, 0.0009771112852218961399, 0.001172497944769040771, 0.001367884604316185401, 0.001563271263863329815 ),
 .UNSPECIFIED. ) ;
#27281=CARTESIAN_POINT ( 'NONE',  ( 15.93101946136715341, -7.369208160676171460, 34.74850200257122879 ) ) ;
#27282=CARTESIAN_POINT ( 'NONE',  ( 1.134638640566794310, -4.075325502946085976, 33.72974371597207721 ) ) ;
#27283=CARTESIAN_POINT ( 'NONE',  ( 11.53846153846141753, -6.026961402154118019, 34.52809138561165270 ) ) ;
#27284=DIRECTION ( 'NONE',  ( -0.000000000000000000, 0.7660444431189791237, -0.6427876096865379196 ) ) ;
#27285=DIRECTION ( 'NONE',  ( 0.000000000000000000, 0.9848077530122072432, -0.1736481776669354937 ) ) ;
#27286=EDGE_CURVE ( 'NONE', #85898, #66653, #50556, .T. ) ;
#27287=FACE_BOUND ( 'NONE', #59559, .T. ) ;
#27288=CARTESIAN_POINT ( 'NONE',  ( 13.25392478150508246, -11.93127051446799847, 32.56575433478202797 ) ) ;
#27289=CARTESIAN_POINT ( 'NONE',  ( 16.85399611801622299, -2.889293201056495786, 32.26117774369186009 ) ) ;
#27290=B_SPLINE_CURVE_WITH_KNOTS ( 'NONE', 3,
 ( #15108, #70489, #8351, #57408, #83123, #35825, #21414, #14662, #29510, #56963 ),
 .UNSPECIFIED., .F., .F.,
 ( 4, 2, 2, 2, 4 ),
 ( 0.0007817359430256293554, 0.0009771253907249952391, 0.001172514838424361123, 0.001367904286123726790, 0.001563293733823092673 ),
 .UNSPECIFIED. ) ;
#27292=CARTESIAN_POINT ( 'NONE',  ( 11.78851595837499211, -12.01375889529407281, 32.43194544308182969 ) ) ;
#27294=CARTESIAN_POINT ( 'NONE',  ( 17.99999999999987566, -2.892918686052165622, 31.69288490824153470 ) ) ;
#27295=CARTESIAN_POINT ( 'NONE',  ( -8.069080805060693251, -4.026226216239094491, 33.68668979543634379 ) ) ;
#27299=CARTESIAN_POINT ( 'NONE',  ( -8.546267865669285868, -7.369474270740069777, 34.74850911626239736 ) ) ;
#27300=EDGE_LOOP ( 'NONE', ( #67401, #30563 ) ) ;
#27303=ORIENTED_EDGE ( 'NONE', *, *, #19636, .F. ) ;
#27304=CARTESIAN_POINT ( 'NONE',  ( -11.47239420511146513, -6.343179335718452272, 34.87096338111212646 ) ) ;
#27305=CARTESIAN_POINT ( 'NONE',  ( -16.02305571287920571, -11.93129842949672437, 32.56571108434900452 ) ) ;
#27307=ORIENTED_EDGE ( 'NONE', *, *, #74425, .F. ) ;
#27308=CYLINDRICAL_SURFACE ( 'NONE', #41229, 0.2500000000000008882 ) ;
#27310=AXIS2_PLACEMENT_3D ( 'NONE', #25100, #12920, #66985 ) ;
#27311=CARTESIAN_POINT ( 'NONE',  ( -15.48074597481782178, -9.234221910056348293, 34.70572697212741531 ) ) ;
#27313=EDGE_CURVE ( 'NONE', #18683, #28039, #34451, .T. ) ;
#27314=CARTESIAN_POINT ( 'NONE',  ( 17.07692307692307665, -12.37446782046654192, 30.86335684631486131 ) ) ;
#27315=CARTESIAN_POINT ( 'NONE',  ( 4.023154687178596589, -11.71456829005830080, 32.44064028649416542 ) ) ;
#27316=CARTESIAN_POINT ( 'NONE',  ( -0.3962828902624369598, -4.481592998940250538, 33.73612834413965089 ) ) ;
#27317=CARTESIAN_POINT ( 'NONE',  ( 11.78840705680968171, -3.712312575010499494, 33.01462480002815170 ) ) ;
#27320=CARTESIAN_POINT ( 'NONE',  ( 13.13463864056679498, -6.524016743844655686, 34.90889640711025521 ) ) ;
#27321=CARTESIAN_POINT ( 'NONE',  ( -4.153846153846152411, -2.833524468853757305, 32.15551576947925838 ) ) ;
#27322=EDGE_CURVE ( 'NONE', #43247, #67219, #78471, .T. ) ;
#27323=ORIENTED_EDGE ( 'NONE', *, *, #5689, .F. ) ;
#27324=FACE_OUTER_BOUND ( 'NONE', #56314, .T. ) ;
#27326=CARTESIAN_POINT ( 'NONE',  ( -14.98076923076922995, -2.249999999999998668, 29.75000000000000355 ) ) ;
#27327=LINE ( 'NONE', #33643, #78589 ) ;
#27328=ORIENTED_EDGE ( 'NONE', *, *, #82885, .F. ) ;
#27329=CARTESIAN_POINT ( 'NONE',  ( 7.145856464345331283, -8.496831190052096971, 34.64984203495476578 ) ) ;
#27330=CARTESIAN_POINT ( 'NONE',  ( 16.28463659481310799, -2.494656445102014342, 31.33466734024120015 ) ) ;
#27331=FACE_OUTER_BOUND ( 'NONE', #53333, .T. ) ;
#27332=ORIENTED_EDGE ( 'NONE', *, *, #29946, .T. ) ;
#27333=CARTESIAN_POINT ( 'NONE',  ( -3.230769230769229949, -1.215029322943914858, 32.30358669280327177 ) ) ;
#27335=CARTESIAN_POINT ( 'NONE',  ( 15.48082365068267841, -5.642605341092957971, 34.66089969410670335 ) ) ;
#27336=CARTESIAN_POINT ( 'NONE',  ( 15.90382291655318880, -9.271318131107980420, 34.42618302367067429 ) ) ;
#27337=EDGE_CURVE ( 'NONE', #45031, #79887, #73057, .T. ) ;
#27338=CARTESIAN_POINT ( 'NONE',  ( 4.946775867484856093, -4.460286881179643004, 33.72017969459903242 ) ) ;
#27339=B_SPLINE_CURVE_WITH_KNOTS ( 'NONE', 3,
 ( #5922, #32951, #27519, #87930, #68071, #73943, #27074, #33398, #74379, #41478 ),
 .UNSPECIFIED., .F., .F.,
 ( 4, 2, 2, 2, 4 ),
 ( 0.0007817246256747461966, 0.0009771112852218892010, 0.001172497944769032314, 0.001367884604316175427, 0.001563271263863318323 ),
 .UNSPECIFIED. ) ;
#27340=CARTESIAN_POINT ( 'NONE',  ( 12.46153846153846168, -8.564572088678739092, 35.78748833219616898 ) ) ;
#27342=VERTEX_POINT ( 'NONE', #60182 ) ;
#27343=ORIENTED_EDGE ( 'NONE', *, *, #21347, .F. ) ;
#27345=EDGE_LOOP ( 'NONE', ( #46820, #25236 ) ) ;
#27346=CARTESIAN_POINT ( 'NONE',  ( 0.4615384615384611200, -3.937682226553329556, 33.60647404775216529 ) ) ;
#27347=CARTESIAN_POINT ( 'NONE',  ( 0.4615384615384611200, -2.538708090699994813, 30.37095296980875503 ) ) ;
#27349=DIRECTION ( 'NONE',  ( -0.000000000000000000, 0.8660254037844399289, -0.4999999999999980016 ) ) ;
#27350=CARTESIAN_POINT ( 'NONE',  ( -16.85391172531022619, -4.887748414852789658, 34.01359900205216746 ) ) ;
#27351=ORIENTED_EDGE ( 'NONE', *, *, #45934, .F. ) ;
#27352=ORIENTED_EDGE ( 'NONE', *, *, #77302, .F. ) ;
#27353=ORIENTED_EDGE ( 'NONE', *, *, #73458, .T. ) ;
#27354=CARTESIAN_POINT ( 'NONE',  ( 5.999999999999878320, -11.67786785259630911, 32.92929555188603530 ) ) ;
#27355=ORIENTED_EDGE ( 'NONE', *, *, #8452, .T. ) ;
#27356=CARTESIAN_POINT ( 'NONE',  ( -1.449885385171703955, -3.083524468853724443, 32.58852847137143272 ) ) ;
#27357=DIRECTION ( 'NONE',  ( 0.000000000000000000, 0.000000000000000000, 1.000000000000000000 ) ) ;
#27358=EDGE_CURVE ( 'NONE', #42649, #13706, #80563, .T. ) ;
#27359=B_SPLINE_CURVE_WITH_KNOTS ( 'NONE', 3,
 ( #55804, #34656, #81974, #55362, #68436, #81524, #21577, #7633, #6733, #62552 ),
 .UNSPECIFIED., .F., .F.,
 ( 4, 2, 2, 2, 4 ),
 ( 0.0007817246256747451124, 0.0009771112852218879000, 0.001172497944769030796, 0.001367884604316173692, 0.001563271263863316588 ),
 .UNSPECIFIED. ) ;
#27360=VECTOR ( 'NONE', #14685, 1000.000000000000000 ) ;
#27361=VECTOR ( 'NONE', #15972, 1000.000000000000114 ) ;
#27362=CARTESIAN_POINT ( 'NONE',  ( 5.777073041093149897, -4.026226216239095379, 33.68668979543632958 ) ) ;
#27363=CYLINDRICAL_SURFACE ( 'NONE', #6533, 0.2500000000000009437 ) ;
#27364=ADVANCED_FACE ( 'NONE', ( #19212 ), #47109, .F. ) ;
#27365=VERTEX_POINT ( 'NONE', #5688 ) ;
#27367=ORIENTED_EDGE ( 'NONE', *, *, #3043, .F. ) ;
#27368=AXIS2_PLACEMENT_3D ( 'NONE', #61046, #26825, #34898 ) ;
#27369=VERTEX_POINT ( 'NONE', #54311 ) ;
#27370=CARTESIAN_POINT ( 'NONE',  ( 0.4615384615384611200, -3.050289026998446396, 32.03036669348365706 ) ) ;
#27371=FACE_OUTER_BOUND ( 'NONE', #45525, .T. ) ;
#27372=VERTEX_POINT ( 'NONE', #27294 ) ;
#27373=EDGE_CURVE ( 'NONE', #62668, #70987, #22474, .T. ) ;
#27374=LINE ( 'NONE', #41329, #73337 ) ;
#27375=B_SPLINE_CURVE_WITH_KNOTS ( 'NONE', 3,
 ( #74957, #51420, #58202, #78923, #16342, #10020, #37487, #49682, #56445, #84821 ),
 .UNSPECIFIED., .F., .F.,
 ( 4, 2, 2, 2, 4 ),
 ( 0.0007817359430256369448, 0.0009771253907250049969, 0.001172514838424373049, 0.001367904286123741101, 0.001563293733823109153 ),
 .UNSPECIFIED. ) ;
#27376=CARTESIAN_POINT ( 'NONE',  ( -0.7115152055870529457, -6.524016743844655686, 34.90889640711025521 ) ) ;
#27377=VERTEX_POINT ( 'NONE', #34049 ) ;
#27378=CARTESIAN_POINT ( 'NONE',  ( -17.75005448165186195, -2.587454068350149239, 30.68340429815432557 ) ) ;
#27379=EDGE_CURVE ( 'NONE', #14228, #58130, #21361, .T. ) ;
#27380=CARTESIAN_POINT ( 'NONE',  ( 4.376857505459001096, -2.758310577978207778, 31.33698337089303010 ) ) ;
#27382=FACE_BOUND ( 'NONE', #10053, .T. ) ;
#27383=CARTESIAN_POINT ( 'NONE',  ( 6.923076923076924238, -12.78798330534103123, 29.99999999999997868 ) ) ;
#27384=CARTESIAN_POINT ( 'NONE',  ( 13.45068271796546178, -6.343179335718452272, 34.87096338111212646 ) ) ;
#27385=CARTESIAN_POINT ( 'NONE',  ( 3.453548772037640546, -9.332535724633405749, 34.40230450496446224 ) ) ;
#27386=CARTESIAN_POINT ( 'NONE',  ( 0.3313904918067649974, -6.809168938359898782, 34.95455904226513866 ) ) ;
#27387=CARTESIAN_POINT ( 'NONE',  ( 5.076923076922954969, -10.21337939537710326, 33.94971097300076224 ) ) ;
#27388=CARTESIAN_POINT ( 'NONE',  ( -3.230769230769352962, -3.643525952248796163, 33.31231777344771672 ) ) ;
#27390=EDGE_LOOP ( 'NONE', ( #12669, #29256 ) ) ;
#27391=CARTESIAN_POINT ( 'NONE',  ( -18.13069146666756382, -10.54014554554151140, 33.71984207302941883 ) ) ;
#27392=CARTESIAN_POINT ( 'NONE',  ( 0.2115152373170027800, -10.92453946501458439, 33.72985991061850086 ) ) ;
#27393=EDGE_LOOP ( 'NONE', ( #54171, #4394, #326, #27061 ) ) ;
#27396=ORIENTED_EDGE ( 'NONE', *, *, #44436, .T. ) ;
#27397=CARTESIAN_POINT ( 'NONE',  ( -15.93106661257773915, -11.41317474335729543, 32.86274602512330034 ) ) ;
#27398=CARTESIAN_POINT ( 'NONE',  ( -15.00775638667583678, -12.64618726649961289, 30.78989965857442712 ) ) ;
#27399=FACE_BOUND ( 'NONE', #33307, .T. ) ;
#27401=CARTESIAN_POINT ( 'NONE',  ( 4.087763774486016466, -12.34228464037088280, 31.77849191805838558 ) ) ;
#27403=CARTESIAN_POINT ( 'NONE',  ( 1.515405825582336607, -12.62708834333097663, 30.88030960425257021 ) ) ;
#27405=CARTESIAN_POINT ( 'NONE',  ( 2.177544337960610310, -11.04286588640298561, 33.62463336215343901 ) ) ;
#27406=AXIS2_PLACEMENT_3D ( 'NONE', #11131, #59764, #87258 ) ;
#27408=VERTEX_POINT ( 'NONE', #14670 ) ;
#27410=EDGE_LOOP ( 'NONE', ( #59618, #2889, #20848, #26662 ) ) ;
#27411=CARTESIAN_POINT ( 'NONE',  ( -12.33074802057151409, -5.496552790871120031, 34.60292014791297532 ) ) ;
#27412=CARTESIAN_POINT ( 'NONE',  ( -0.5922299282060184966, -2.729777683071817673, 31.24903638046269094 ) ) ;
#27413=CARTESIAN_POINT ( 'NONE',  ( 1.384615384615386802, -9.058645607665452459, 34.76329471203371924 ) ) ;
#27414=CARTESIAN_POINT ( 'NONE',  ( 10.68063975489745410, -3.083524468853784839, 32.58852847137153930 ) ) ;
#27415=CARTESIAN_POINT ( 'NONE',  ( -3.453695448285377445, -5.667676309546437530, 34.40238873228292249 ) ) ;
#27417=DIRECTION ( 'NONE',  ( 0.000000000000000000, 0.9396926207859126468, 0.3420201433256571111 ) ) ;
#27418=DIRECTION ( 'NONE',  ( 0.000000000000000000, 0.9396926207859126468, 0.3420201433256571111 ) ) ;
#27419=EDGE_CURVE ( 'NONE', #29899, #33691, #41785, .T. ) ;
#27420=CARTESIAN_POINT ( 'NONE',  ( 9.692307692307570832, -11.06231777344772027, 33.60647404775119895 ) ) ;
#27421=DIRECTION ( 'NONE',  ( 0.000000000000000000, 0.7660444431189822323, -0.6427876096865344779 ) ) ;
#27422=CARTESIAN_POINT ( 'NONE',  ( 10.86533002476265963, -3.520799739797214389, 33.17531984108286025 ) ) ;
#27423=CARTESIAN_POINT ( 'NONE',  ( -5.010855743573001675, -6.343179335718452272, 34.87096338111212646 ) ) ;
#27424=CARTESIAN_POINT ( 'NONE',  ( -3.361459833879539172, -9.929715669179220328, 34.40415004197138416 ) ) ;
#27425=CARTESIAN_POINT ( 'NONE',  ( -6.857821783564084228, -3.643525952247864463, 33.31231777344670064 ) ) ;
#27426=EDGE_CURVE ( 'NONE', #6303, #622, #50379, .T. ) ;
#27428=AXIS2_PLACEMENT_3D ( 'NONE', #74263, #53080, #82354 ) ;
#27429=CARTESIAN_POINT ( 'NONE',  ( 6.000000000000001776, -6.386643153685126251, 34.62446782046654192 ) ) ;
#27430=ORIENTED_EDGE ( 'NONE', *, *, #50471, .T. ) ;
#27431=CARTESIAN_POINT ( 'NONE',  ( -0.4615384615385826339, -3.835265460704628371, 33.15142922262033665 ) ) ;
#27432=CARTESIAN_POINT ( 'NONE',  ( 10.61538461538461675, -5.471508081941601098, 34.59228464037088457 ) ) ;
#27433=B_SPLINE_CURVE_WITH_KNOTS ( 'NONE', 3,
 ( #21430, #61965, #714, #55210, #35385, #56548, #82702, #70056, #14231, #76369 ),
 .UNSPECIFIED., .F., .F.,
 ( 4, 2, 2, 2, 4 ),
 ( 0.0007817246256747453293, 0.0009771112852218889842, 0.001172497944769032531, 0.001367884604316176294, 0.001563271263863319840 ),
 .UNSPECIFIED. ) ;
#27436=VECTOR ( 'NONE', #51728, 1000.000000000000000 ) ;
#27438=CARTESIAN_POINT ( 'NONE',  ( 5.076923076923075762, -8.164416787775445883, 34.95778746994557906 ) ) ;
#27439=CARTESIAN_POINT ( 'NONE',  ( 7.846153846153846700, -2.538708090699994813, 30.37095296980875503 ) ) ;
#27440=VERTEX_POINT ( 'NONE', #20966 ) ;
#27442=CARTESIAN_POINT ( 'NONE',  ( 12.52760579488853665, -5.471508081941601098, 34.59228464037088457 ) ) ;
#27443=EDGE_CURVE ( 'NONE', #21602, #44682, #13853, .T. ) ;
#27444=ORIENTED_EDGE ( 'NONE', *, *, #11854, .T. ) ;
#27445=CARTESIAN_POINT ( 'NONE',  ( 11.53846153846141576, -9.528491918059723176, 34.59228464037033035 ) ) ;
#27447=CARTESIAN_POINT ( 'NONE',  ( -15.23076923076922995, -1.044019251281081972, 31.83374038241031911 ) ) ;
#27449=CARTESIAN_POINT ( 'NONE',  ( 14.17700084102474811, -2.541943142973491554, 30.39792223712631980 ) ) ;
#27451=EDGE_CURVE ( 'NONE', #14199, #37091, #16103, .T. ) ;
#27452=CARTESIAN_POINT ( 'NONE',  ( -16.28445651347068335, -7.722926236386454590, 34.74524107206102030 ) ) ;
#27453=CARTESIAN_POINT ( 'NONE',  ( -15.23076923076935074, -12.46129190930018460, 30.37095296980731973 ) ) ;
#27454=ORIENTED_EDGE ( 'NONE', *, *, #22317, .F. ) ;
#27455=ORIENTED_EDGE ( 'NONE', *, *, #45330, .T. ) ;
#27456=CARTESIAN_POINT ( 'NONE',  ( 15.29683656411930848, -4.661471528628508665, 34.16647553114624003 ) ) ;
#27457=EDGE_CURVE ( 'NONE', #79057, #62627, #18174, .T. ) ;
#27458=ORIENTED_EDGE ( 'NONE', *, *, #79281, .T. ) ;
#27459=CARTESIAN_POINT ( 'NONE',  ( 7.715463243043540587, -9.084618155246140248, 34.75535874321725771 ) ) ;
#27460=CARTESIAN_POINT ( 'NONE',  ( 5.299935921016468932, -4.762714258010880997, 34.23016756924214832 ) ) ;
#27461=DIRECTION ( 'NONE',  ( -0.000000000000000000, -0.6427876096865404731, -0.7660444431189770143 ) ) ;
#27462=CARTESIAN_POINT ( 'NONE',  ( -6.673131513698880468, -11.56426240980093745, 33.07394671870546432 ) ) ;
#27463=CARTESIAN_POINT ( 'NONE',  ( 15.10062202133101295, -6.852621066184266141, 34.70813303252209181 ) ) ;
#27465=CARTESIAN_POINT ( 'NONE',  ( 15.93036122928181975, -12.69144148231606017, 30.53333754910549303 ) ) ;
#27466=AXIS2_PLACEMENT_3D ( 'NONE', #86399, #85935, #24218 ) ;
#27467=VERTEX_POINT ( 'NONE', #31291 ) ;
#27468=EDGE_LOOP ( 'NONE', ( #33786, #88447 ) ) ;
#27469=CARTESIAN_POINT ( 'NONE',  ( -0.4615384615385826339, -12.27809138561165270, 31.22303859784587132 ) ) ;
#27470=ORIENTED_EDGE ( 'NONE', *, *, #50479, .T. ) ;
#27471=B_SPLINE_CURVE_WITH_KNOTS ( 'NONE', 3,
 ( #6572, #67829, #55631, #7464, #61065, #34919, #88569, #62382, #697, #28163 ),
 .UNSPECIFIED., .F., .F.,
 ( 4, 2, 2, 2, 4 ),
 ( 0.0007817246256747473893, 0.0009771112852218905021, 0.001172497944769033615, 0.001367884604316176944, 0.001563271263863320057 ),
 .UNSPECIFIED. ) ;
#27472=B_SPLINE_CURVE_WITH_KNOTS ( 'NONE', 3,
 ( #67970, #18452, #80609, #87822, #53555, #19338, #88704, #59429, #46806, #74284 ),
 .UNSPECIFIED., .F., .F.,
 ( 4, 2, 2, 2, 4 ),
 ( 0.000000000000000000, 0.0001954339857564063089, 0.0003908679715128126177, 0.0005863019572692189808, 0.0007817359430256252354 ),
 .UNSPECIFIED. ) ;
#27473=EDGE_CURVE ( 'NONE', #82350, #9234, #34286, .T. ) ;
#27474=DIRECTION ( 'NONE',  ( -0.000000000000000000, 0.1736481776669307198, -0.9848077530122080203 ) ) ;
#27475=CARTESIAN_POINT ( 'NONE',  ( -13.60744348225026634, -7.369209533119140509, 34.99857337881830688 ) ) ;
#27476=CARTESIAN_POINT ( 'NONE',  ( 9.692307692307695177, -4.786620604624113540, 33.94971097300155094 ) ) ;
#27477=VERTEX_POINT ( 'NONE', #16881 ) ;
#27478=CARTESIAN_POINT ( 'NONE',  ( 1.384615384615265343, -3.835265460704628371, 33.15142922262033665 ) ) ;
#27479=EDGE_LOOP ( 'NONE', ( #74453, #78960 ) ) ;
#27480=CARTESIAN_POINT ( 'NONE',  ( 8.096208266067295156, -12.65882529074907126, 30.72640787790839312 ) ) ;
#27482=CARTESIAN_POINT ( 'NONE',  ( -14.24162497434223162, -11.91647553114624358, 32.58852847137148245 ) ) ;
#27483=ORIENTED_EDGE ( 'NONE', *, *, #15532, .F. ) ;
#27484=CARTESIAN_POINT ( 'NONE',  ( 1.515407192440173967, -6.413143153341454017, 34.63066358083362672 ) ) ;
#27485=CARTESIAN_POINT ( 'NONE',  ( -8.769230769230890843, -2.892918686052166066, 31.69288490824153470 ) ) ;
#27486=FACE_BOUND ( 'NONE', #16734, .T. ) ;
#27488=CARTESIAN_POINT ( 'NONE',  ( 1.134615384615387246, -7.500000000000001776, 35.00000000000000000 ) ) ;
#27489=CARTESIAN_POINT ( 'NONE',  ( 9.692307692307570832, -2.379036618888197729, 30.90682066428292885 ) ) ;
#27490=CARTESIAN_POINT ( 'NONE',  ( 1.253924781505079800, -12.35290016733513951, 31.75349464988449455 ) ) ;
#27492=CARTESIAN_POINT ( 'NONE',  ( -5.749999999998562927, -7.500000000000155431, 34.75000000000007105 ) ) ;
#27493=CARTESIAN_POINT ( 'NONE',  ( -13.38461538461538325, -6.189225973068211317, 35.74407628777942847 ) ) ;
#27494=VERTEX_POINT ( 'NONE', #3811 ) ;
#27495=ORIENTED_EDGE ( 'NONE', *, *, #30017, .F. ) ;
#27497=CARTESIAN_POINT ( 'NONE',  ( 2.084765348785459604, -2.889293201056495786, 32.26117774369186009 ) ) ;
#27498=CARTESIAN_POINT ( 'NONE',  ( 2.307692307692309264, -10.51840700105979565, 33.73612834413961536 ) ) ;
#27499=ADVANCED_FACE ( 'NONE', ( #59200 ), #45238, .F. ) ;
#27500=B_SPLINE_CURVE_WITH_KNOTS ( 'NONE', 3,
 ( #40207, #67669, #4181, #69878, #27118, #82524, #21688, #13166, #83854, #76186 ),
 .UNSPECIFIED., .F., .F.,
 ( 4, 2, 2, 2, 4 ),
 ( 0.0007817246256747519429, 0.0009771112852218970073, 0.001172497944769042288, 0.001367884604316187353, 0.001563271263863332417 ),
 .UNSPECIFIED. ) ;
#27501=CARTESIAN_POINT ( 'NONE',  ( 7.053602624840485724, -6.852161475712352789, 34.70806712695775786 ) ) ;
#27502=CARTESIAN_POINT ( 'NONE',  ( -4.023055712879202162, -9.084667340241226796, 34.75534355489798344 ) ) ;
#27503=DIRECTION ( 'NONE',  ( -0.000000000000000000, 0.9396926207859092051, -0.3420201433256662704 ) ) ;
#27504=DIRECTION ( 'NONE',  ( -0.000000000000000000, 0.6427876096865404731, -0.7660444431189771253 ) ) ;
#27505=B_SPLINE_CURVE_WITH_KNOTS ( 'NONE', 3,
 ( #41245, #27278, #7460, #20953, #7899, #34033, #19634, #54744, #89005, #6125 ),
 .UNSPECIFIED., .F., .F.,
 ( 4, 2, 2, 2, 4 ),
 ( 0.0007817246256747473893, 0.0009771112852218909357, 0.001172497944769034482, 0.001367884604316178246, 0.001563271263863321792 ),
 .UNSPECIFIED. ) ;
#27506=ORIENTED_EDGE ( 'NONE', *, *, #54803, .F. ) ;
#27507=CARTESIAN_POINT ( 'NONE',  ( 2.177545098254087819, -9.418419913701741919, 34.36755862841477693 ) ) ;
#27508=CARTESIAN_POINT ( 'NONE',  ( -6.250023237292964495, -6.695914987888143877, 34.68535235679833306 ) ) ;
#27509=CARTESIAN_POINT ( 'NONE',  ( -6.923076923077044142, -11.48612834414049644, 32.76840700105863391 ) ) ;
#27510=DIRECTION ( 'NONE',  ( -0.000000000000000000, 0.9396926207859093161, -0.3420201433256663259 ) ) ;
#27511=ORIENTED_EDGE ( 'NONE', *, *, #59222, .F. ) ;
#27512=EDGE_LOOP ( 'NONE', ( #8781, #37967 ) ) ;
#27513=ORIENTED_EDGE ( 'NONE', *, *, #15921, .F. ) ;
#27515=EDGE_CURVE ( 'NONE', #85639, #36102, #59009, .T. ) ;
#27517=CYLINDRICAL_SURFACE ( 'NONE', #52482, 0.2499999999999986955 ) ;
#27518=CARTESIAN_POINT ( 'NONE',  ( 15.23076923076923173, -3.937682226553329556, 33.60647404775216529 ) ) ;
#27519=CARTESIAN_POINT ( 'NONE',  ( 3.361294669002876656, -10.31582465632705237, 34.18122507451815295 ) ) ;
#27520=CARTESIAN_POINT ( 'NONE',  ( -17.30040800148741198, -9.417330523894424488, 34.63758898049880486 ) ) ;
#27521=EDGE_CURVE ( 'NONE', #21025, #54359, #72713, .T. ) ;
#27522=CARTESIAN_POINT ( 'NONE',  ( 9.692307692307572609, -6.026961402154118019, 34.52809138561165270 ) ) ;
#27523=EDGE_LOOP ( 'NONE', ( #47676, #84698, #43550, #75875, #19471, #30611 ) ) ;
#27524=CARTESIAN_POINT ( 'NONE',  ( 11.40790094671961796, -2.504760397472875155, 29.97295953869789997 ) ) ;
#27526=ORIENTED_EDGE ( 'NONE', *, *, #61368, .F. ) ;
#27528=FACE_OUTER_BOUND ( 'NONE', #83086, .T. ) ;
#27529=CARTESIAN_POINT ( 'NONE',  ( -11.60373153901786125, -11.06231777344662781, 33.60647404775220082 ) ) ;
#27530=AXIS2_PLACEMENT_3D ( 'NONE', #75635, #68010, #62129 ) ;
#27531=LINE ( 'NONE', #34282, #72544 ) ;
#27532=FACE_OUTER_BOUND ( 'NONE', #34448, .T. ) ;
#27533=EDGE_CURVE ( 'NONE', #78459, #79092, #83750, .T. ) ;
#27534=CARTESIAN_POINT ( 'NONE',  ( 9.469381474791545017, -9.886141570436013382, 34.14413921362392301 ) ) ;
#27535=CARTESIAN_POINT ( 'NONE',  ( -3.360916440207450506, -6.852621066184267029, 34.70813303252209181 ) ) ;
#27536=VECTOR ( 'NONE', #6922, 999.9999999999998863 ) ;
#27538=ORIENTED_EDGE ( 'NONE', *, *, #11943, .F. ) ;
#27539=CARTESIAN_POINT ( 'NONE',  ( -7.053767526187229464, -10.70098750199973203, 33.91152734681376302 ) ) ;
#27540=CARTESIAN_POINT ( 'NONE',  ( 12.71148387091650278, -4.932303261841489928, 34.32971442181322885 ) ) ;
#27541=B_SPLINE_CURVE_WITH_KNOTS ( 'NONE', 3,
 ( #54683, #48816, #68650, #20469, #56019, #83510, #75852, #21793, #62328, #82178 ),
 .UNSPECIFIED., .F., .F.,
 ( 4, 2, 2, 2, 4 ),
 ( 0.000000000000000000, 0.0001954311564186873352, 0.0003908623128373746704, 0.0005862934692560620598, 0.0007817246256747493408 ),
 .UNSPECIFIED. ) ;
#27544=B_SPLINE_CURVE_WITH_KNOTS ( 'NONE', 3,
 ( #38141, #78235, #50751, #85446, #11115, #30060, #23726, #43565, #38590, #79131 ),
 .UNSPECIFIED., .F., .F.,
 ( 4, 2, 2, 2, 4 ),
 ( 0.0007817359430256215491, 0.0009771253907249856981, 0.001172514838424349847, 0.001367904286123713779, 0.001563293733823077928 ),
 .UNSPECIFIED. ) ;
#27545=VERTEX_POINT ( 'NONE', #57866 ) ;
#27546=CARTESIAN_POINT ( 'NONE',  ( -12.46153846153846168, -11.69971097300155272, 32.46337939537588113 ) ) ;
#27547=CARTESIAN_POINT ( 'NONE',  ( -12.59222992820602371, -3.062553014421049546, 32.05460306192773601 ) ) ;
#27548=B_SPLINE_CURVE_WITH_KNOTS ( 'NONE', 3,
 ( #54129, #47828, #74873, #41518, #33868, #6838, #12717, #68111, #61772, #88400 ),
 .UNSPECIFIED., .F., .F.,
 ( 4, 2, 2, 2, 4 ),
 ( 0.000000000000000000, 0.0001954311564186861426, 0.0003908623128373722852, 0.0005862934692560583735, 0.0007817246256747445703 ),
 .UNSPECIFIED. ) ;
#27550=CARTESIAN_POINT ( 'NONE',  ( 9.442307692307693401, -7.566082377512564960, 35.00000000000000711 ) ) ;
#27551=FACE_OUTER_BOUND ( 'NONE', #50028, .T. ) ;
#27552=VERTEX_POINT ( 'NONE', #85799 ) ;
#27553=CARTESIAN_POINT ( 'NONE',  ( -15.45369544828537656, -2.758268499246657068, 31.33685645148948140 ) ) ;
#27554=ADVANCED_FACE ( 'NONE', ( #17786 ), #44786, .F. ) ;
#27555=CARTESIAN_POINT ( 'NONE',  ( 3.480714749117372886, -12.22109172314383052, 31.39792113162168263 ) ) ;
#27556=CYLINDRICAL_SURFACE ( 'NONE', #57915, 0.2500000000000008882 ) ;
#27558=CARTESIAN_POINT ( 'NONE',  ( 17.07692307692307665, -9.819645486525091727, 36.12317359536749706 ) ) ;
#27559=VERTEX_POINT ( 'NONE', #78138 ) ;
#27563=ORIENTED_EDGE ( 'NONE', *, *, #12424, .T. ) ;
#27564=CARTESIAN_POINT ( 'NONE',  ( 9.692307692307695177, -13.53365097954675988, 30.81389545987213552 ) ) ;
#27565=DIRECTION ( 'NONE',  ( -0.000000000000000000, -0.000000000000000000, -1.000000000000000000 ) ) ;
#27566=CYLINDRICAL_SURFACE ( 'NONE', #60980, 0.2499999999999986955 ) ;
#27567=VECTOR ( 'NONE', #25652, 1000.000000000000114 ) ;
#27568=LINE ( 'NONE', #21241, #20601 ) ;
#27569=CARTESIAN_POINT ( 'NONE',  ( -1.608100309179716358, -10.97335522853832579, 33.68706563782419749 ) ) ;
#27570=VERTEX_POINT ( 'NONE', #85349 ) ;
#27571=FACE_BOUND ( 'NONE', #51045, .T. ) ;
#27572=ORIENTED_EDGE ( 'NONE', *, *, #53872, .T. ) ;
#27573=CARTESIAN_POINT ( 'NONE',  ( 11.53846153846153832, -13.63283147151868846, 33.57946703557072254 ) ) ;
#27574=CARTESIAN_POINT ( 'NONE',  ( 4.946775867484854317, -11.93770438780619259, 32.05411857736982029 ) ) ;
#27575=CARTESIAN_POINT ( 'NONE',  ( 3.007842271862382955, -11.43668979543635089, 33.22377378376089752 ) ) ;
#27576=CARTESIAN_POINT ( 'NONE',  ( 6.923076923076802558, -2.625532179533778709, 30.86335684631627174 ) ) ;
#27577=EDGE_LOOP ( 'NONE', ( #59351, #38581, #67164, #11673 ) ) ;
#27578=ORIENTED_EDGE ( 'NONE', *, *, #22161, .F. ) ;
#27579=ORIENTED_EDGE ( 'NONE', *, *, #44820, .T. ) ;
#27580=VECTOR ( 'NONE', #43440, 1000.000000000000114 ) ;
#27581=CARTESIAN_POINT ( 'NONE',  ( 6.000000000000001776, -1.790695186598648903, 34.54067556320373455 ) ) ;
#27582=VERTEX_POINT ( 'NONE', #64607 ) ;
#27583=CARTESIAN_POINT ( 'NONE',  ( 15.00728430620490350, -3.562934362175799841, 33.22335522853832401 ) ) ;
#27584=VECTOR ( 'NONE', #23872, 1000.000000000000227 ) ;
#27585=CYLINDRICAL_SURFACE ( 'NONE', #69862, 0.2499999999999995559 ) ;
#27586=CARTESIAN_POINT ( 'NONE',  ( 6.066068351002443571, -12.10708131394839882, 31.69288490824020954 ) ) ;
#27587=CARTESIAN_POINT ( 'NONE',  ( 8.769230769230647482, -9.442884908241554243, 34.35708131394783038 ) ) ;
#27591=CARTESIAN_POINT ( 'NONE',  ( -8.703163435880695076, -2.833524468853757305, 32.15551576947925838 ) ) ;
#27592=ORIENTED_EDGE ( 'NONE', *, *, #10285, .F. ) ;
#27593=ORIENTED_EDGE ( 'NONE', *, *, #38191, .F. ) ;
#27594=ORIENTED_EDGE ( 'NONE', *, *, #82560, .T. ) ;
#27595=CARTESIAN_POINT ( 'NONE',  ( 3.480769230770650147, -7.500000000000154543, 35.00000000000007105 ) ) ;
#27596=CARTESIAN_POINT ( 'NONE',  ( 4.153846153846030731, -11.06231777344772027, 33.60647404775119895 ) ) ;
#27597=CARTESIAN_POINT ( 'NONE',  ( -8.069080063669991532, -4.186968288167451036, 33.49512374952580274 ) ) ;
#27598=EDGE_CURVE ( 'NONE', #2295, #26375, #77955, .T. ) ;
#27600=CARTESIAN_POINT ( 'NONE',  ( 7.846153846153846700, -8.564572088678739092, 35.78748833219616898 ) ) ;
#27601=FACE_BOUND ( 'NONE', #28812, .T. ) ;
#27602=CARTESIAN_POINT ( 'NONE',  ( -1.384615384615383471, -13.95598074871891292, 31.83374038241031911 ) ) ;
#27603=EDGE_LOOP ( 'NONE', ( #71437, #29962, #69212, #48331 ) ) ;
#27604=CARTESIAN_POINT ( 'NONE',  ( -15.23076923076892264, -2.506253911140614576, 30.00000000000323297 ) ) ;
#27605=DIRECTION ( 'NONE',  ( -0.000000000000000000, 0.9848077530122086864, -0.1736481776669273891 ) ) ;
#27606=DIRECTION ( 'NONE',  ( 0.000000000000000000, 0.8660254037844377084, -0.5000000000000015543 ) ) ;
#27607=ORIENTED_EDGE ( 'NONE', *, *, #41002, .F. ) ;
#27608=CARTESIAN_POINT ( 'NONE',  ( 6.000000000000001776, -10.67929555188718282, 33.92786785259544047 ) ) ;
#27609=ORIENTED_EDGE ( 'NONE', *, *, #59658, .T. ) ;
#27610=FACE_BOUND ( 'NONE', #40496, .T. ) ;
#27611=CARTESIAN_POINT ( 'NONE',  ( 14.30769230769218581, -12.51329471203414379, 31.30864560766407578 ) ) ;
#27613=EDGE_CURVE ( 'NONE', #8179, #72902, #16440, .T. ) ;
#27614=AXIS2_PLACEMENT_3D ( 'NONE', #76536, #43623, #27905 ) ;
#27616=CYLINDRICAL_SURFACE ( 'NONE', #69157, 0.2499999999999994726 ) ;
#27617=ORIENTED_EDGE ( 'NONE', *, *, #65855, .T. ) ;
#27618=EDGE_CURVE ( 'NONE', #49301, #39942, #56482, .T. ) ;
#27619=DIRECTION ( 'NONE',  ( 0.000000000000000000, 0.7660444431189807890, 0.6427876096865361433 ) ) ;
#27621=CARTESIAN_POINT ( 'NONE',  ( 18.06606733335007675, -10.67929555188718282, 33.92786785259544757 ) ) ;
#27622=CARTESIAN_POINT ( 'NONE',  ( -4.946397638689432164, -5.915461855592777596, 34.75538340440931506 ) ) ;
#27625=CARTESIAN_POINT ( 'NONE',  ( -12.46153846153858247, -3.300289026999228881, 32.46337939537708905 ) ) ;
#27626=CARTESIAN_POINT ( 'NONE',  ( 4.088576153289833925, -10.33852847137145048, 34.16647553114627556 ) ) ;
#27627=LINE ( 'NONE', #602, #34067 ) ;
#27628=VERTEX_POINT ( 'NONE', #4259 ) ;
#27630=CARTESIAN_POINT ( 'NONE',  ( 0.6845513056318554002, -10.77377354290276301, 33.85451476688484718 ) ) ;
#27631=DIRECTION ( 'NONE',  ( -0.000000000000000000, 1.000000000000000000, -0.000000000000000000 ) ) ;
#27632=CARTESIAN_POINT ( 'NONE',  ( -13.25382357679060519, -3.530189275343204702, 32.79018710029569661 ) ) ;
#27634=DIRECTION ( 'NONE',  ( 0.000000000000000000, 0.6427876096865368094, 0.7660444431189802339 ) ) ;
#27635=CARTESIAN_POINT ( 'NONE',  ( -2.557692307692319034, -2.499999999999999556, 29.81609845454692120 ) ) ;
#27636=ADVANCED_FACE ( 'NONE', ( #31742 ), #54211, .F. ) ;
#27639=ORIENTED_EDGE ( 'NONE', *, *, #2969, .F. ) ;
#27643=CARTESIAN_POINT ( 'NONE',  ( -8.703163435880695076, -6.343179335718452272, 34.87096338111212646 ) ) ;
#27644=EDGE_LOOP ( 'NONE', ( #42116, #31354 ) ) ;
#27645=CARTESIAN_POINT ( 'NONE',  ( -5.207613680033385428, -11.37499894934982514, 33.29245874905763003 ) ) ;
#27647=CARTESIAN_POINT ( 'NONE',  ( 14.43848411551709887, -11.18335022499818621, 33.13157742990016885 ) ) ;
#27649=CARTESIAN_POINT ( 'NONE',  ( 3.007843013253083786, -8.239355502252617924, 34.69524867566427417 ) ) ;
#27650=CARTESIAN_POINT ( 'NONE',  ( -8.769230769230892619, -12.70778746994576025, 30.41441678777401236 ) ) ;
#27651=CARTESIAN_POINT ( 'NONE',  ( -15.23076923076935252, -5.094484230521993062, 34.41647553114689373 ) ) ;
#27652=CARTESIAN_POINT ( 'NONE',  ( 4.153846153846154188, -3.513871655860378418, 32.76840700105978499 ) ) ;
#27654=CARTESIAN_POINT ( 'NONE',  ( -18.00000000000012079, -11.67786785259630733, 32.92929555188604240 ) ) ;
#27655=CARTESIAN_POINT ( 'NONE',  ( 10.61538461538461675, -2.538708090699994813, 30.37095296980875503 ) ) ;
#27656=CARTESIAN_POINT ( 'NONE',  ( -17.01085574357299990, -10.67929555188718282, 33.92786785259544757 ) ) ;
#27658=ADVANCED_FACE ( 'NONE', ( #12357 ), #88481, .F. ) ;
#27659=CARTESIAN_POINT ( 'NONE',  ( -12.46153846153858424, -11.06231777344772027, 33.60647404775119895 ) ) ;
#27660=CARTESIAN_POINT ( 'NONE',  ( 11.60371710973756443, -5.219633306516380244, 34.19971097300157936 ) ) ;
#27661=ORIENTED_EDGE ( 'NONE', *, *, #88469, .T. ) ;
#27662=ORIENTED_EDGE ( 'NONE', *, *, #2936, .T. ) ;
#27663=EDGE_CURVE ( 'NONE', #21233, #34931, #82641, .T. ) ;
#27664=CARTESIAN_POINT ( 'NONE',  ( 12.68431813051652313, -2.612705202774698421, 31.66806509827799943 ) ) ;
#27665=CARTESIAN_POINT ( 'NONE',  ( 0.5267936010512989098, -12.16647553114626490, 32.15551576947920864 ) ) ;
#27666=CYLINDRICAL_SURFACE ( 'NONE', #74253, 0.2499999999999995559 ) ;
#27667=CARTESIAN_POINT ( 'NONE',  ( 0.2115152373170036404, -10.18141759479407504, 34.26406193332783801 ) ) ;
#27668=EDGE_CURVE ( 'NONE', #83905, #8169, #4713, .T. ) ;
#27669=CARTESIAN_POINT ( 'NONE',  ( 12.21156173059610772, -9.148715823498378086, 34.47080413974185120 ) ) ;
#27670=CARTESIAN_POINT ( 'NONE',  ( -9.757577692864012775, -6.835583212224499938, 34.95778746994557906 ) ) ;
#27671=DIRECTION ( 'NONE',  ( 0.000000000000000000, 0.7660444431189822323, -0.6427876096865344779 ) ) ;
#27673=CARTESIAN_POINT ( 'NONE',  ( 18.00000000000000000, -3.322132147404559976, 32.92929555188717927 ) ) ;
#27674=VERTEX_POINT ( 'NONE', #88923 ) ;
#27676=CARTESIAN_POINT ( 'NONE',  ( 16.40390057375961064, -9.233818618650598609, 34.70587769442853698 ) ) ;
#27677=VECTOR ( 'NONE', #57025, 1000.000000000000000 ) ;
#27678=CARTESIAN_POINT ( 'NONE',  ( 8.834485908743603844, -9.528491918058460186, 34.59228464037086326 ) ) ;
#27679=CARTESIAN_POINT ( 'NONE',  ( 11.78840705680968171, -10.76462480002816235, 33.53768742498949962 ) ) ;
#27680=CARTESIAN_POINT ( 'NONE',  ( 3.903869409797562806, -6.524016743844655686, 34.90889640711025521 ) ) ;
#27681=CARTESIAN_POINT ( 'NONE',  ( 5.750023269057650488, -2.779195860258147022, 31.39871582349836743 ) ) ;
#27682=ORIENTED_EDGE ( 'NONE', *, *, #48574, .T. ) ;
#27683=ORIENTED_EDGE ( 'NONE', *, *, #36117, .T. ) ;
#27684=EDGE_CURVE ( 'NONE', #63003, #29891, #47456, .T. ) ;
#27685=ORIENTED_EDGE ( 'NONE', *, *, #55578, .T. ) ;
#27686=ORIENTED_EDGE ( 'NONE', *, *, #32996, .T. ) ;
#27687=CARTESIAN_POINT ( 'NONE',  ( -10.74553258511631348, -12.50552854090298993, 31.33409797877408920 ) ) ;
#27689=B_SPLINE_CURVE_WITH_KNOTS ( 'NONE', 3,
 ( #23457, #8637, #15834, #43301, #57255, #70773, #9079, #83409, #29788, #84746 ),
 .UNSPECIFIED., .F., .F.,
 ( 4, 2, 2, 2, 4 ),
 ( 0.0007817246256747473893, 0.0009771112852218905021, 0.001172497944769033615, 0.001367884604316176944, 0.001563271263863320057 ),
 .UNSPECIFIED. ) ;
#27690=CARTESIAN_POINT ( 'NONE',  ( 14.30769230769231015, -2.486705287966279876, 31.30864560766543647 ) ) ;
#27692=CARTESIAN_POINT ( 'NONE',  ( 17.93472999944368240, -3.083524468853725775, 32.58852847137143272 ) ) ;
#27693=FACE_OUTER_BOUND ( 'NONE', #66891, .T. ) ;
#27694=ORIENTED_EDGE ( 'NONE', *, *, #24936, .F. ) ;
#27695=B_SPLINE_CURVE_WITH_KNOTS ( 'NONE', 3,
 ( #38192, #65650, #74206, #26905, #11621, #19265, #73318, #60683, #33665, #61123 ),
 .UNSPECIFIED., .F., .F.,
 ( 4, 2, 2, 2, 4 ),
 ( 0.000000000000000000, 0.0001954339857564073388, 0.0003908679715128146777, 0.0005863019572692220165, 0.0007817359430256293554 ),
 .UNSPECIFIED. ) ;
#27697=ADVANCED_FACE ( 'NONE', ( #32184 ), #19991, .F. ) ;
#27698=ORIENTED_EDGE ( 'NONE', *, *, #84389, .F. ) ;
#27699=CARTESIAN_POINT ( 'NONE',  ( 17.29993442853592711, -12.39991518177334129, 30.74647679643404530 ) ) ;
#27700=EDGE_LOOP ( 'NONE', ( #16193, #87472 ) ) ;
#27701=FACE_OUTER_BOUND ( 'NONE', #15726, .T. ) ;
#27702=FACE_OUTER_BOUND ( 'NONE', #10276, .T. ) ;
#27703=AXIS2_PLACEMENT_3D ( 'NONE', #52101, #65606, #17441 ) ;
#27705=VERTEX_POINT ( 'NONE', #40281 ) ;
#27706=ORIENTED_EDGE ( 'NONE', *, *, #43726, .T. ) ;
#27707=FACE_OUTER_BOUND ( 'NONE', #59913, .T. ) ;
#27708=FACE_BOUND ( 'NONE', #16886, .T. ) ;
#27709=CARTESIAN_POINT ( 'NONE',  ( -2.177166869458661225, -5.070358843744209310, 34.40418822224088302 ) ) ;
#27710=ADVANCED_FACE ( 'NONE', ( #59645 ), #61411, .F. ) ;
#27711=CARTESIAN_POINT ( 'NONE',  ( -4.403869378067609475, -10.18141759479407327, 34.26406193332782379 ) ) ;
#27712=ORIENTED_EDGE ( 'NONE', *, *, #22456, .T. ) ;
#27713=CARTESIAN_POINT ( 'NONE',  ( -9.942330916529147800, -4.931416488878822335, 34.32920672191015399 ) ) ;
#27716=CARTESIAN_POINT ( 'NONE',  ( -3.230769230769229949, -4.786620604624113540, 33.94971097300155094 ) ) ;
#27717=DIRECTION ( 'NONE',  ( -0.000000000000000000, -0.9848077530122086864, -0.1736481776669273613 ) ) ;
#27718=ORIENTED_EDGE ( 'NONE', *, *, #72945, .F. ) ;
#27719=CARTESIAN_POINT ( 'NONE',  ( -0.3314910262880099157, -7.723484941389743952, 34.99544897038808955 ) ) ;
#27720=CARTESIAN_POINT ( 'NONE',  ( -7.715362038329057981, -11.18335022499818621, 33.13157742990016885 ) ) ;
#27721=CARTESIAN_POINT ( 'NONE',  ( -12.71151519248081740, -12.17611988154120972, 31.52148481390971213 ) ) ;
#27722=CARTESIAN_POINT ( 'NONE',  ( -2.307692307692427391, -10.90142922262034020, 33.41473453929536674 ) ) ;
#27723=CARTESIAN_POINT ( 'NONE',  ( -4.153846153846152411, -12.78798330534103123, 29.99999999999997868 ) ) ;
#27724=FACE_BOUND ( 'NONE', #63684, .T. ) ;
#27725=CARTESIAN_POINT ( 'NONE',  ( -8.834481759392012634, -2.506253911140460922, 30.00000000000013856 ) ) ;
#27726=CARTESIAN_POINT ( 'NONE',  ( 11.31553532094539172, -12.39988816332205701, 30.74660775122750778 ) ) ;
#27727=EDGE_CURVE ( 'NONE', #40013, #9491, #62201, .T. ) ;
#27728=CARTESIAN_POINT ( 'NONE',  ( 5.299702745901139878, -9.418065098278011860, 34.63729479722530158 ) ) ;
#27730=CARTESIAN_POINT ( 'NONE',  ( 17.86930853333243974, -11.18331474514187995, 33.13161551792790505 ) ) ;
#27731=B_SPLINE_CURVE_WITH_KNOTS ( 'NONE', 3,
 ( #56334, #14014, #22106, #76153, #20340, #48237, #47801, #55004, #75710, #508 ),
 .UNSPECIFIED., .F., .F.,
 ( 4, 2, 2, 2, 4 ),
 ( 0.000000000000000000, 0.0001954339881912783286, 0.0003908679763825566571, 0.0005863019645738349857, 0.0007817359527651133143 ),
 .UNSPECIFIED. ) ;
#27732=CARTESIAN_POINT ( 'NONE',  ( -18.24997673094235395, -9.943427161483787913, 34.11278801902876978 ) ) ;
#27734=B_SPLINE_CURVE_WITH_KNOTS ( 'NONE', 3,
 ( #36206, #37506, #71734, #56893, #15927, #72182, #37060, #49701, #3278, #44246 ),
 .UNSPECIFIED., .F., .F.,
 ( 4, 2, 2, 2, 4 ),
 ( 0.000000000000000000, 0.0001954339857564093175, 0.0003908679715128186350, 0.0005863019572692279796, 0.0007817359430256372700 ),
 .UNSPECIFIED. ) ;
#27735=ORIENTED_EDGE ( 'NONE', *, *, #65232, .T. ) ;
#27738=VERTEX_POINT ( 'NONE', #52882 ) ;
#27740=CARTESIAN_POINT ( 'NONE',  ( 0.6849144022366444595, -2.501478030877322567, 29.88021232661720816 ) ) ;
#27741=ORIENTED_EDGE ( 'NONE', *, *, #19062, .F. ) ;
#27742=CARTESIAN_POINT ( 'NONE',  ( -11.40766973063675671, -2.729792928343269587, 31.24908615093345077 ) ) ;
#27743=CARTESIAN_POINT ( 'NONE',  ( -14.30769230769230660, -3.886160181151819604, 36.00935417666054406 ) ) ;
#27745=DIRECTION ( 'NONE',  ( 0.000000000000000000, 0.3420201433256641055, -0.9396926207859100932 ) ) ;
#27746=ORIENTED_EDGE ( 'NONE', *, *, #67821, .T. ) ;
#27749=CARTESIAN_POINT ( 'NONE',  ( -10.61538461538461320, -2.499999999999998668, 29.75000000000001421 ) ) ;
#27750=CARTESIAN_POINT ( 'NONE',  ( -7.146003881983769013, -12.64616026154729411, 30.79003144601913533 ) ) ;
#27751=CARTESIAN_POINT ( 'NONE',  ( 12.21151522424549540, -2.823816976329317274, 31.52131813110795733 ) ) ;
#27753=CARTESIAN_POINT ( 'NONE',  ( 2.530471848960717640, -2.847695495035523550, 31.58253572463339154 ) ) ;
#27754=LINE ( 'NONE', #41281, #55526 ) ;
#27756=LINE ( 'NONE', #77273, #52016 ) ;
#27757=CARTESIAN_POINT ( 'NONE',  ( 10.83839596699746544, -11.24521262558773493, 33.06293181088029343 ) ) ;
#27758=EDGE_CURVE ( 'NONE', #45448, #66105, #5250, .T. ) ;
#27759=ORIENTED_EDGE ( 'NONE', *, *, #75225, .T. ) ;
#27760=CARTESIAN_POINT ( 'NONE',  ( 8.835299120233207404, -9.780366693483667717, 34.19971097300155805 ) ) ;
#27762=B_SPLINE_CURVE_WITH_KNOTS ( 'NONE', 3,
 ( #4446, #86897, #12113, #25164, #52630, #60277, #12548, #60726, #87790, #88231 ),
 .UNSPECIFIED., .F., .F.,
 ( 4, 2, 2, 2, 4 ),
 ( 0.0007817359527651132059, 0.0009771254036996528287, 0.001172514854634192560, 0.001367904305568732291, 0.001563293756503272023 ),
 .UNSPECIFIED. ) ;
#27763=LINE ( 'NONE', #13363, #13068 ) ;
#27764=DIRECTION ( 'NONE',  ( 0.000000000000000000, 0.000000000000000000, 1.000000000000000000 ) ) ;
#27766=CARTESIAN_POINT ( 'NONE',  ( 14.55774661933062397, -2.564540009722896752, 30.55348353981670684 ) ) ;
#27767=CARTESIAN_POINT ( 'NONE',  ( 3.230769230769231726, -3.513871655860378418, 32.76840700105978499 ) ) ;
#27768=LINE ( 'NONE', #13368, #21007 ) ;
#27769=ORIENTED_EDGE ( 'NONE', *, *, #70616, .F. ) ;
#27770=CARTESIAN_POINT ( 'NONE',  ( -5.076923076923075762, -5.557115091759785130, 34.35708131394839171 ) ) ;
#27771=EDGE_CURVE ( 'NONE', #7100, #63601, #62300, .T. ) ;
#27772=CARTESIAN_POINT ( 'NONE',  ( -1.515306851282940848, -10.54014554554150607, 33.71984207302941883 ) ) ;
#27773=CARTESIAN_POINT ( 'NONE',  ( 6.923076923076800782, -12.16647553114689728, 32.15551576947799362 ) ) ;
#27774=AXIS2_PLACEMENT_3D ( 'NONE', #14591, #49263, #69531 ) ;
#27775=VECTOR ( 'NONE', #17611, 1000.000000000000114 ) ;
#27776=CARTESIAN_POINT ( 'NONE',  ( -16.94639737515952049, -2.882268652242223617, 31.66798894389554064 ) ) ;
#27777=CARTESIAN_POINT ( 'NONE',  ( 0.4615384615383382183, -2.379036618888197285, 30.90682066428292885 ) ) ;
#27780=ORIENTED_EDGE ( 'NONE', *, *, #31793, .T. ) ;
#27781=EDGE_LOOP ( 'NONE', ( #60192, #71912 ) ) ;
#27782=DIRECTION ( 'NONE',  ( -0.000000000000000000, 0.5000000000000011102, -0.8660254037844380415 ) ) ;
#27783=CARTESIAN_POINT ( 'NONE',  ( 6.923076923076802558, -2.892918686052165622, 31.69288490824153470 ) ) ;
#27785=FACE_OUTER_BOUND ( 'NONE', #74538, .T. ) ;
#27786=DIRECTION ( 'NONE',  ( -0.000000000000000000, 0.8660254037844397068, -0.4999999999999978906 ) ) ;
#27787=VERTEX_POINT ( 'NONE', #82601 ) ;
#27788=CARTESIAN_POINT ( 'NONE',  ( -18.06575680251431137, -7.249945686854186278, 34.74374336980224598 ) ) ;
#27789=ORIENTED_EDGE ( 'NONE', *, *, #70891, .F. ) ;
#27790=EDGE_CURVE ( 'NONE', #37367, #53679, #69068, .T. ) ;
#27791=VERTEX_POINT ( 'NONE', #28083 ) ;
#27792=AXIS2_PLACEMENT_3D ( 'NONE', #63679, #1986, #29469 ) ;
#27793=ORIENTED_EDGE ( 'NONE', *, *, #20185, .F. ) ;
#27794=CARTESIAN_POINT ( 'NONE',  ( -7.173053667125516064, -8.347322224742351082, 34.93158281831414769 ) ) ;
#27795=ORIENTED_EDGE ( 'NONE', *, *, #33304, .T. ) ;
#27797=EDGE_CURVE ( 'NONE', #45094, #38831, #63318, .T. ) ;
#27798=CARTESIAN_POINT ( 'NONE',  ( -5.999999999999998224, -6.189225973068211317, 35.74407628777942847 ) ) ;
#27799=VECTOR ( 'NONE', #42305, 1000.000000000000000 ) ;
#27800=ADVANCED_FACE ( 'NONE', ( #48790 ), #15018, .F. ) ;
#27802=CARTESIAN_POINT ( 'NONE',  ( -12.33101275977489664, -12.27024696741798948, 31.24895572276497546 ) ) ;
#27804=ORIENTED_EDGE ( 'NONE', *, *, #65852, .T. ) ;
#27805=ORIENTED_EDGE ( 'NONE', *, *, #37842, .F. ) ;
#27808=LINE ( 'NONE', #55276, #14497 ) ;
#27809=CARTESIAN_POINT ( 'NONE',  ( -10.48459417441766206, -2.494656445102012565, 31.33466734024120015 ) ) ;
#27810=VERTEX_POINT ( 'NONE', #75821 ) ;
#27811=B_SPLINE_CURVE_WITH_KNOTS ( 'NONE', 3,
 ( #2455, #10563, #83237, #37132, #84898, #71806, #23184, #78125, #85337, #24508 ),
 .UNSPECIFIED., .F., .F.,
 ( 4, 2, 2, 2, 4 ),
 ( 0.0007817246256747466303, 0.0009771112852218900684, 0.001172497944769033398, 0.001367884604316176728, 0.001563271263863320274 ),
 .UNSPECIFIED. ) ;
#27813=CYLINDRICAL_SURFACE ( 'NONE', #33569, 0.2499999999999995559 ) ;
#27814=ORIENTED_EDGE ( 'NONE', *, *, #57939, .F. ) ;
#27815=CARTESIAN_POINT ( 'NONE',  ( 9.822352748227467956, -2.254550872974306674, 29.97347326024527092 ) ) ;
#27816=CARTESIAN_POINT ( 'NONE',  ( 12.46153846153846168, -9.058645607665452459, 34.76329471203371924 ) ) ;
#27817=ORIENTED_EDGE ( 'NONE', *, *, #57477, .T. ) ;
#27818=FACE_BOUND ( 'NONE', #62766, .T. ) ;
#27819=CARTESIAN_POINT ( 'NONE',  ( -15.45369618967607828, -8.282780595021769443, 34.94152052738834158 ) ) ;
#27821=CARTESIAN_POINT ( 'NONE',  ( 12.21151523731700550, -6.652501968072648708, 34.93155406624980941 ) ) ;
#27822=CARTESIAN_POINT ( 'NONE',  ( 7.911408985666684046, -11.06231777344671130, 33.60647404775212976 ) ) ;
#27824=LINE ( 'NONE', #35022, #82652 ) ;
#27825=CARTESIAN_POINT ( 'NONE',  ( -2.307692307692305711, -3.513871655860378418, 32.76840700105978499 ) ) ;
#27826=ORIENTED_EDGE ( 'NONE', *, *, #5953, .T. ) ;
#27827=CARTESIAN_POINT ( 'NONE',  ( -2.373774687052441212, -3.937682226553329556, 33.60647404775217240 ) ) ;
#27829=EDGE_CURVE ( 'NONE', #28684, #26115, #3171, .T. ) ;
#27830=B_SPLINE_CURVE_WITH_KNOTS ( 'NONE', 3,
 ( #70361, #76219, #8220, #36142, #14525, #1897, #83443, #77115, #29385, #56835 ),
 .UNSPECIFIED., .F., .F.,
 ( 4, 2, 2, 2, 4 ),
 ( 0.0007817359430256365111, 0.0009771253907250043464, 0.001172514838424372399, 0.001367904286123740234, 0.001563293733823108069 ),
 .UNSPECIFIED. ) ;
#27831=ORIENTED_EDGE ( 'NONE', *, *, #67377, .T. ) ;
#27832=B_SPLINE_CURVE_WITH_KNOTS ( 'NONE', 3,
 ( #5745, #54366, #75101, #33222, #46288, #60684, #47165, #13828, #41308, #68772 ),
 .UNSPECIFIED., .F., .F.,
 ( 4, 2, 2, 2, 4 ),
 ( 0.0007817359430256283796, 0.0009771253907249941549, 0.001172514838424359822, 0.001367904286123725489, 0.001563293733823091156 ),
 .UNSPECIFIED. ) ;
#27833=AXIS2_PLACEMENT_3D ( 'NONE', #78833, #10386, #59462 ) ;
#27834=AXIS2_PLACEMENT_3D ( 'NONE', #33009, #60474, #26249 ) ;
#27836=CARTESIAN_POINT ( 'NONE',  ( -7.596208436775802930, -2.341251567377310217, 30.72681386836322659 ) ) ;
#27837=VERTEX_POINT ( 'NONE', #6919 ) ;
#27838=CARTESIAN_POINT ( 'NONE',  ( 17.93391658904412012, -5.557115091759785130, 34.35708131394839171 ) ) ;
#27839=CARTESIAN_POINT ( 'NONE',  ( 2.530705151785702878, -4.762714258010882773, 34.23016756924214832 ) ) ;
#27840=FACE_BOUND ( 'NONE', #17638, .T. ) ;
#27841=CARTESIAN_POINT ( 'NONE',  ( -2.437839517130527156, -6.852621066184267029, 34.70813303252209181 ) ) ;
#27842=LINE ( 'NONE', #55307, #15731 ) ;
#27843=CARTESIAN_POINT ( 'NONE',  ( 10.36540788444226102, -8.303909089506435137, 34.68538101551103381 ) ) ;
#27844=CARTESIAN_POINT ( 'NONE',  ( -8.769230769230768274, -12.10708131394839349, 31.69288490824020244 ) ) ;
#27846=CARTESIAN_POINT ( 'NONE',  ( 0.3954550505825806250, -5.557115091759785130, 34.35708131394839171 ) ) ;
#27847=DIRECTION ( 'NONE',  ( -0.000000000000000000, 0.1736481776669307198, -0.9848077530122080203 ) ) ;
#27850=VERTEX_POINT ( 'NONE', #35281 ) ;
#27852=CARTESIAN_POINT ( 'NONE',  ( 14.53047197667037338, -12.69155399931963046, 30.53255429739157734 ) ) ;
#27853=CARTESIAN_POINT ( 'NONE',  ( 6.673076923076925127, -7.500000000000001776, 35.00000000000000000 ) ) ;
#27854=CARTESIAN_POINT ( 'NONE',  ( -0.7115152055870529457, -2.920706130388546651, 32.31842814019191223 ) ) ;
#27855=CARTESIAN_POINT ( 'NONE',  ( -6.923076923076922462, -1.422936976036506707, 30.56769352161908415 ) ) ;
#27857=CARTESIAN_POINT ( 'NONE',  ( 0.7114838709165043351, -4.176053281294515251, 33.81426240980091791 ) ) ;
#27858=CARTESIAN_POINT ( 'NONE',  ( 2.307692307692623679, -2.255955759149395501, 30.00000000000324363 ) ) ;
#27859=CARTESIAN_POINT ( 'NONE',  ( 2.307692307692309264, -13.20930481340135110, 34.54067556320372745 ) ) ;
#27860=CARTESIAN_POINT ( 'NONE',  ( 10.61538461538461675, -6.343179335718451384, 34.87096338111211935 ) ) ;
#27861=CARTESIAN_POINT ( 'NONE',  ( -15.00775787915638304, -11.24521262558773493, 33.06293181088029343 ) ) ;
#27862=CARTESIAN_POINT ( 'NONE',  ( -4.853910232829680815, -6.460100341425561332, 34.89618726649961644 ) ) ;
#27863=CARTESIAN_POINT ( 'NONE',  ( -0.4615384615385840772, -4.320704448113951379, 33.92786785259630022 ) ) ;
#27865=CARTESIAN_POINT ( 'NONE',  ( 14.43821800945587519, -11.93748526763465279, 32.05452791011430946 ) ) ;
#27866=EDGE_CURVE ( 'NONE', #55482, #1586, #39205, .T. ) ;
#27867=DIRECTION ( 'NONE',  ( -0.000000000000000000, 0.9396926207859092051, -0.3420201433256662704 ) ) ;
#27868=EDGE_LOOP ( 'NONE', ( #41662, #88876, #5795, #52769 ) ) ;
#27869=CARTESIAN_POINT ( 'NONE',  ( -0.2115929431903190994, -3.712312575010499938, 33.01462480002815170 ) ) ;
#27870=CARTESIAN_POINT ( 'NONE',  ( 10.86543903529806698, -5.642605341092957971, 34.66089969410670335 ) ) ;
#27872=B_SPLINE_CURVE_WITH_KNOTS ( 'NONE', 3,
 ( #33338, #26577, #45504, #66672, #54033, #25685, #31552, #59469, #81531, #26130 ),
 .UNSPECIFIED., .F., .F.,
 ( 4, 2, 2, 2, 4 ),
 ( 0.0007817246256747452209, 0.0009771112852218887673, 0.001172497944769032531, 0.001367884604316176294, 0.001563271263863319840 ),
 .UNSPECIFIED. ) ;
#27873=VECTOR ( 'NONE', #43609, 1000.000000000000000 ) ;
#27874=EDGE_CURVE ( 'NONE', #59207, #80088, #21767, .T. ) ;
#27875=LINE ( 'NONE', #13475, #66296 ) ;
#27876=CARTESIAN_POINT ( 'NONE',  ( -16.15384615384627409, -2.657715359629662988, 31.77849191805970364 ) ) ;
#27877=ORIENTED_EDGE ( 'NONE', *, *, #53026, .T. ) ;
#27878=CARTESIAN_POINT ( 'NONE',  ( -8.769230769230768274, -6.681629849574314051, 35.83090037661290239 ) ) ;
#27879=CARTESIAN_POINT ( 'NONE',  ( -17.07692307692307665, -13.57706302396349152, 30.56769352161908060 ) ) ;
#27880=ORIENTED_EDGE ( 'NONE', *, *, #33792, .F. ) ;
#27882=CARTESIAN_POINT ( 'NONE',  ( 17.07692307692295586, -2.657715359629662544, 31.77849191805970364 ) ) ;
#27883=EDGE_CURVE ( 'NONE', #60602, #1437, #77156, .T. ) ;
#27884=B_SPLINE_CURVE_WITH_KNOTS ( 'NONE', 3,
 ( #67106, #33759, #11721, #5406, #18913, #26564, #12605, #61215, #47264, #74755 ),
 .UNSPECIFIED., .F., .F.,
 ( 4, 2, 2, 2, 4 ),
 ( 0.000000000000000000, 0.0001954339857564127327, 0.0003908679715128183640, 0.0005863019572692239681, 0.0007817359430256295722 ),
 .UNSPECIFIED. ) ;
#27885=ORIENTED_EDGE ( 'NONE', *, *, #83287, .T. ) ;
#27886=DIRECTION ( 'NONE',  ( -0.000000000000000000, 0.8660254037844399289, -0.4999999999999980016 ) ) ;
#27888=EDGE_CURVE ( 'NONE', #18841, #9565, #50114, .T. ) ;
#27889=ORIENTED_EDGE ( 'NONE', *, *, #23249, .T. ) ;
#27890=CARTESIAN_POINT ( 'NONE',  ( 14.17754509825408960, -2.619462340734462380, 30.83744416345203021 ) ) ;
#27891=CARTESIAN_POINT ( 'NONE',  ( -15.90384615384622613, -7.565270445406050648, 34.75000000000000000 ) ) ;
#27892=DIRECTION ( 'NONE',  ( -0.000000000000000000, -0.9396926207859093161, -0.3420201433256663259 ) ) ;
#27893=ORIENTED_EDGE ( 'NONE', *, *, #60568, .F. ) ;
#27895=EDGE_CURVE ( 'NONE', #48157, #12391, #88087, .T. ) ;
#27896=CARTESIAN_POINT ( 'NONE',  ( 3.100621261037533216, -3.069018819979302926, 32.56621877034667278 ) ) ;
#27897=ORIENTED_EDGE ( 'NONE', *, *, #63299, .T. ) ;
#27898=CARTESIAN_POINT ( 'NONE',  ( -15.23076923076922995, -3.937682226553329556, 33.60647404775216529 ) ) ;
#27899=CARTESIAN_POINT ( 'NONE',  ( 5.299702745901139878, -4.989023458446560255, 34.36081565061822118 ) ) ;
#27900=CARTESIAN_POINT ( 'NONE',  ( 9.469380733400845074, -9.172386477786396597, 34.72672124145550043 ) ) ;
#27901=DIRECTION ( 'NONE',  ( -0.000000000000000000, -0.9396926207859092051, -0.3420201433256662704 ) ) ;
#27902=CARTESIAN_POINT ( 'NONE',  ( 15.00728428704528561, -6.760086850603066466, 34.69517049084099369 ) ) ;
#27903=CARTESIAN_POINT ( 'NONE',  ( 1.134638640566795420, -2.318417181685854533, 30.59732222474233865 ) ) ;
#27905=DIRECTION ( 'NONE',  ( 0.000000000000000000, 0.3420201433256610524, 0.9396926207859113145 ) ) ;
#27906=EDGE_LOOP ( 'NONE', ( #29025, #78291, #50157, #24306 ) ) ;
#27907=ORIENTED_EDGE ( 'NONE', *, *, #27618, .F. ) ;
#27908=CARTESIAN_POINT ( 'NONE',  ( -1.607494067044030528, -7.630691491037286056, 34.74850469731152458 ) ) ;
#27909=EDGE_LOOP ( 'NONE', ( #38117, #20971 ) ) ;
#27911=CARTESIAN_POINT ( 'NONE',  ( -12.46153846153846168, -1.129524287112498415, 32.06866353760679544 ) ) ;
#27912=VERTEX_POINT ( 'NONE', #78470 ) ;
#27913=EDGE_CURVE ( 'NONE', #48093, #13650, #10473, .T. ) ;
#27914=CARTESIAN_POINT ( 'NONE',  ( 11.78840694783958298, -3.520799739797214389, 33.17531984108286025 ) ) ;
#27915=CARTESIAN_POINT ( 'NONE',  ( 5.142178648199100088, -3.835265460703683349, 33.15142922261929925 ) ) ;
#27917=CARTESIAN_POINT ( 'NONE',  ( -9.915173114511331320, -2.501496062324912284, 29.88072118266895671 ) ) ;
#27918=EDGE_CURVE ( 'NONE', #6671, #50988, #64070, .T. ) ;
#27919=ORIENTED_EDGE ( 'NONE', *, *, #41033, .F. ) ;
#27920=CARTESIAN_POINT ( 'NONE',  ( -11.53846153846166089, -12.16647553114689728, 32.15551576947799362 ) ) ;
#27921=ORIENTED_EDGE ( 'NONE', *, *, #44665, .T. ) ;
#27922=CARTESIAN_POINT ( 'NONE',  ( -11.53846153846153655, -12.78798330534102945, 29.74999999999997868 ) ) ;
#27924=EDGE_CURVE ( 'NONE', #16798, #24594, #64952, .T. ) ;
#27925=CARTESIAN_POINT ( 'NONE',  ( -8.992156986746914882, -4.887634598454295265, 34.01352882383564946 ) ) ;
#27926=CARTESIAN_POINT ( 'NONE',  ( 12.21151523731700550, -2.341070481393819236, 30.72580821765574299 ) ) ;
#27927=FACE_BOUND ( 'NONE', #61307, .T. ) ;
#27928=VECTOR ( 'NONE', #48479, 1000.000000000000114 ) ;
#27929=CARTESIAN_POINT ( 'NONE',  ( 5.776515075435670887, -2.353723527008295680, 30.78948104536958752 ) ) ;
#27930=CARTESIAN_POINT ( 'NONE',  ( -17.86920819217521483, -12.11778462344220841, 31.66786338562085135 ) ) ;
#27931=AXIS2_PLACEMENT_3D ( 'NONE', #62049, #82780, #70134 ) ;
#27932=CARTESIAN_POINT ( 'NONE',  ( 9.468822767743363400, -2.353723527008296568, 30.78948104536958752 ) ) ;
#27933=CARTESIAN_POINT ( 'NONE',  ( -12.46153846153846168, -13.49023893513002648, 31.06009739812518688 ) ) ;
#27934=CARTESIAN_POINT ( 'NONE',  ( -3.100243529005665799, -3.285477652293413264, 32.44071101563363158 ) ) ;
#27935=CARTESIAN_POINT ( 'NONE',  ( -4.153846153846273204, -11.48612834414049644, 32.76840700105863391 ) ) ;
#27936=CARTESIAN_POINT ( 'NONE',  ( 8.769230769230768274, -3.050289026998446396, 32.03036669348365706 ) ) ;
#27937=ORIENTED_EDGE ( 'NONE', *, *, #8228, .F. ) ;
#27939=B_SPLINE_CURVE_WITH_KNOTS ( 'NONE', 3,
 ( #40708, #68170, #67729, #33053, #6034, #54637, #20426, #80814, #33502, #60961 ),
 .UNSPECIFIED., .F., .F.,
 ( 4, 2, 2, 2, 4 ),
 ( 0.000000000000000000, 0.0001954339857564073388, 0.0003908679715128146777, 0.0005863019572692220165, 0.0007817359430256293554 ),
 .UNSPECIFIED. ) ;
#27940=ORIENTED_EDGE ( 'NONE', *, *, #84655, .T. ) ;
#27941=CARTESIAN_POINT ( 'NONE',  ( 2.057715563643716994, -2.920706130388546651, 32.31842814019191223 ) ) ;
#27942=CARTESIAN_POINT ( 'NONE',  ( 7.976679547917406410, -10.19071101563364756, 33.96452234770658407 ) ) ;
#27943=CARTESIAN_POINT ( 'NONE',  ( -11.76194648218548622, -11.89387501736622710, 32.13663884655806413 ) ) ;
#27944=CARTESIAN_POINT ( 'NONE',  ( -18.00000000000000000, -13.18701529485372070, 34.52197243641129631 ) ) ;
#27945=EDGE_CURVE ( 'NONE', #32906, #3675, #14991, .T. ) ;
#27946=CARTESIAN_POINT ( 'NONE',  ( 15.45378058238208041, -3.587049720035815348, 32.86302985866382897 ) ) ;
#27948=EDGE_CURVE ( 'NONE', #77695, #275, #79372, .T. ) ;
#27949=VERTEX_POINT ( 'NONE', #71265 ) ;
#27950=CARTESIAN_POINT ( 'NONE',  ( 8.769230769230768274, -13.04860791097971706, 34.73218667398347037 ) ) ;
#27951=CARTESIAN_POINT ( 'NONE',  ( 3.296837581771669079, -11.16473453929635440, 33.15142922261926373 ) ) ;
#27952=CARTESIAN_POINT ( 'NONE',  ( -14.24243716817946925, -12.51329471203373700, 31.30864560766537963 ) ) ;
#27953=FACE_OUTER_BOUND ( 'NONE', #62719, .T. ) ;
#27954=ORIENTED_EDGE ( 'NONE', *, *, #62377, .T. ) ;
#27955=EDGE_CURVE ( 'NONE', #46303, #60075, #65379, .T. ) ;
#27956=ORIENTED_EDGE ( 'NONE', *, *, #67448, .T. ) ;
#27959=VERTEX_POINT ( 'NONE', #37483 ) ;
#27960=CARTESIAN_POINT ( 'NONE',  ( -9.626240358957616650, -9.905515769479276145, 34.41647553114623292 ) ) ;
#27961=CARTESIAN_POINT ( 'NONE',  ( 22.75000000000000000, -7.500000000000000000, 29.75000000000000355 ) ) ;
#27962=CARTESIAN_POINT ( 'NONE',  ( -5.999999999999998224, -12.78798330534102945, 29.74999999999997868 ) ) ;
#27964=CARTESIAN_POINT ( 'NONE',  ( 14.30769230769218758, -4.481592998941358097, 33.73612834414048933 ) ) ;
#27965=VECTOR ( 'NONE', #151, 1000.000000000000227 ) ;
#27966=ORIENTED_EDGE ( 'NONE', *, *, #73095, .F. ) ;
#27968=CARTESIAN_POINT ( 'NONE',  ( -7.846153846153844924, -1.044019251281081972, 31.83374038241031911 ) ) ;
#27969=EDGE_LOOP ( 'NONE', ( #32836, #41056 ) ) ;
#27970=CARTESIAN_POINT ( 'NONE',  ( -9.442253380669374252, -4.235687564193447052, 33.53795663066793509 ) ) ;
#27971=CARTESIAN_POINT ( 'NONE',  ( -8.899840424434849240, -7.722926974430166069, 34.99546784045485737 ) ) ;
#27972=CARTESIAN_POINT ( 'NONE',  ( 13.38461538461526423, -11.67786785259630911, 32.92929555188603530 ) ) ;
#27973=CARTESIAN_POINT ( 'NONE',  ( 11.78851595837499211, -10.06805714834173493, 34.32951233291982618 ) ) ;
#27974=CARTESIAN_POINT ( 'NONE',  ( 2.530705151785704210, -2.523321265292116422, 31.42251411153756990 ) ) ;
#27975=DIRECTION ( 'NONE',  ( 1.000000000000000000, 0.000000000000000000, 0.000000000000000000 ) ) ;
#27976=CARTESIAN_POINT ( 'NONE',  ( -3.007806096502555704, -7.369474539155830506, 34.99858011523957657 ) ) ;
#27978=ORIENTED_EDGE ( 'NONE', *, *, #55931, .F. ) ;
#27979=CARTESIAN_POINT ( 'NONE',  ( -1.384615384615383471, -1.509761064869970415, 31.06009739812519044 ) ) ;
#27981=EDGE_CURVE ( 'NONE', #56983, #8169, #26624, .T. ) ;
#27982=LINE ( 'NONE', #34739, #73449 ) ;
#27983=ORIENTED_EDGE ( 'NONE', *, *, #44412, .F. ) ;
#27984=CYLINDRICAL_SURFACE ( 'NONE', #31190, 0.2499999999999994726 ) ;
#27985=CARTESIAN_POINT ( 'NONE',  ( 11.53846153846141576, -4.320704448113951379, 33.92786785259630022 ) ) ;
#27986=CARTESIAN_POINT ( 'NONE',  ( 14.05769230769229061, -2.249999999999998668, 29.81609741502487410 ) ) ;
#27987=CARTESIAN_POINT ( 'NONE',  ( -4.377331097570101193, -10.81261337010820256, 33.49550067578627477 ) ) ;
#27988=EDGE_CURVE ( 'NONE', #50472, #4672, #35225, .T. ) ;
#27989=B_SPLINE_CURVE_WITH_KNOTS ( 'NONE', 3,
 ( #20871, #21760, #6913, #607, #76253, #55544, #75381, #34386, #48340, #83027 ),
 .UNSPECIFIED., .F., .F.,
 ( 4, 2, 2, 2, 4 ),
 ( 0.000000000000000000, 0.0001954339857564073659, 0.0003908679715128147319, 0.0005863019572692221250, 0.0007817359430256294638 ),
 .UNSPECIFIED. ) ;
#27990=EDGE_LOOP ( 'NONE', ( #39378, #53133 ) ) ;
#27991=CARTESIAN_POINT ( 'NONE',  ( -12.39547011053602610, -8.973038597847271092, 34.52809138561121216 ) ) ;
#27992=CIRCLE ( 'NONE', #32304, 0.2500000000000002220 ) ;
#27994=DIRECTION ( 'NONE',  ( -0.000000000000000000, -0.7660444431189791237, -0.6427876096865379196 ) ) ;
#27995=ORIENTED_EDGE ( 'NONE', *, *, #69096, .F. ) ;
#27996=ADVANCED_FACE ( 'NONE', ( #11808 ), #47352, .F. ) ;
#27997=DIRECTION ( 'NONE',  ( -0.000000000000000000, 0.7660444431189791237, -0.6427876096865379196 ) ) ;
#27998=VECTOR ( 'NONE', #25127, 1000.000000000000114 ) ;
#27999=VECTOR ( 'NONE', #11915, 999.9999999999998863 ) ;
#28000=ORIENTED_EDGE ( 'NONE', *, *, #72031, .T. ) ;
#28001=CARTESIAN_POINT ( 'NONE',  ( -2.438383774359869083, -12.11776431015576172, 31.66791131148498906 ) ) ;
#28003=ORIENTED_EDGE ( 'NONE', *, *, #58076, .F. ) ;
#28004=B_SPLINE_CURVE_WITH_KNOTS ( 'NONE', 3,
 ( #6415, #40644, #32539, #18147, #66330, #26233, #60014, #53700, #19909, #87515 ),
 .UNSPECIFIED., .F., .F.,
 ( 4, 2, 2, 2, 4 ),
 ( 0.000000000000000000, 0.0001954339857564093175, 0.0003908679715128186350, 0.0005863019572692279796, 0.0007817359430256372700 ),
 .UNSPECIFIED. ) ;
#28005=CARTESIAN_POINT ( 'NONE',  ( 7.846153846153846700, -12.10708131394839349, 31.69288490824020244 ) ) ;
#28006=CARTESIAN_POINT ( 'NONE',  ( 2.307692307692187583, -6.879047030192662504, 34.71129190930017927 ) ) ;
#28007=CARTESIAN_POINT ( 'NONE',  ( 13.38461538461526601, -6.879047030192662504, 34.71129190930017927 ) ) ;
#28009=EDGE_CURVE ( 'NONE', #46107, #47096, #46906, .T. ) ;
#28010=CARTESIAN_POINT ( 'NONE',  ( 11.28843831424008215, -12.45566812827425451, 31.48439005359158926 ) ) ;
#28012=ORIENTED_EDGE ( 'NONE', *, *, #77522, .T. ) ;
#28013=FACE_BOUND ( 'NONE', #32750, .T. ) ;
#28014=ORIENTED_EDGE ( 'NONE', *, *, #63111, .F. ) ;
#28015=CARTESIAN_POINT ( 'NONE',  ( -2.307692307692428724, -2.657715359629662544, 31.77849191805970364 ) ) ;
#28016=ADVANCED_FACE ( 'NONE', ( #68085 ), #19004, .F. ) ;
#28017=CARTESIAN_POINT ( 'NONE',  ( 4.403900465484466231, -11.79725096376909299, 32.30694842903960762 ) ) ;
#28018=EDGE_CURVE ( 'NONE', #23009, #14315, #71753, .T. ) ;
#28020=CARTESIAN_POINT ( 'NONE',  ( 16.85343813319912698, -2.599994579823202923, 30.74605699353653776 ) ) ;
#28021=ORIENTED_EDGE ( 'NONE', *, *, #60326, .T. ) ;
#28022=AXIS2_PLACEMENT_3D ( 'NONE', #5047, #52335, #23971 ) ;
#28023=ORIENTED_EDGE ( 'NONE', *, *, #54680, .F. ) ;
#28025=CARTESIAN_POINT ( 'NONE',  ( -3.007756386675835003, -11.43677907613345113, 33.22367315496201456 ) ) ;
#28026=ORIENTED_EDGE ( 'NONE', *, *, #59300, .T. ) ;
#28027=EDGE_CURVE ( 'NONE', #42657, #9576, #56770, .T. ) ;
#28028=CARTESIAN_POINT ( 'NONE',  ( 15.16468685140909400, -3.322132147404559532, 32.92929555188719348 ) ) ;
#28029=CARTESIAN_POINT ( 'NONE',  ( -6.699701437304502960, -2.251407671071270489, 29.88021292934942252 ) ) ;
#28030=CARTESIAN_POINT ( 'NONE',  ( -17.14219307747939425, -3.083524468853725775, 32.58852847137143272 ) ) ;
#28031=CARTESIAN_POINT ( 'NONE',  ( -8.546451100252701494, -4.226511098958373402, 33.85474049983370293 ) ) ;
#28032=B_SPLINE_CURVE_WITH_KNOTS ( 'NONE', 3,
 ( #9792, #30069, #3911, #43143, #30506, #16994, #23301, #36821, #85455, #57532 ),
 .UNSPECIFIED., .F., .F.,
 ( 4, 2, 2, 2, 4 ),
 ( 0.000000000000000000, 0.0001954311564186864949, 0.0003908623128373729899, 0.0005862934692560594577, 0.0007817246256747459798 ),
 .UNSPECIFIED. ) ;
#28033=DIRECTION ( 'NONE',  ( 0.000000000000000000, 0.8660254037844377084, -0.5000000000000015543 ) ) ;
#28034=LINE ( 'NONE', #83436, #6405 ) ;
#28035=CARTESIAN_POINT ( 'NONE',  ( -5.207070286361297207, -3.817052484675422797, 33.13202310037935661 ) ) ;
#28038=EDGE_CURVE ( 'NONE', #6878, #87412, #87041, .T. ) ;
#28039=VERTEX_POINT ( 'NONE', #83823 ) ;
#28040=DIRECTION ( 'NONE',  ( 0.000000000000000000, 0.6427876096865368094, 0.7660444431189802339 ) ) ;
#28041=DIRECTION ( 'NONE',  ( -0.000000000000000000, 0.3420201433256694901, -0.9396926207859082059 ) ) ;
#28042=CARTESIAN_POINT ( 'NONE',  ( 10.68145296638705410, -6.386643153685127139, 34.62446782046654192 ) ) ;
#28044=CARTESIAN_POINT ( 'NONE',  ( 16.15384615384615330, -2.249999999999998668, 29.50000000000001421 ) ) ;
#28045=ADVANCED_FACE ( 'NONE', ( #7716 ), #41491, .F. ) ;
#28046=FACE_BOUND ( 'NONE', #77062, .T. ) ;
#28047=CARTESIAN_POINT ( 'NONE',  ( 9.915319043920543862, -3.587049720035815348, 32.86302985866382897 ) ) ;
#28049=EDGE_LOOP ( 'NONE', ( #14040, #76654 ) ) ;
#28050=AXIS2_PLACEMENT_3D ( 'NONE', #8680, #63157, #29398 ) ;
#28051=CARTESIAN_POINT ( 'NONE',  ( -7.846153846153844924, -1.129524287112498415, 32.06866353760679544 ) ) ;
#28052=LINE ( 'NONE', #36585, #76160 ) ;
#28054=CARTESIAN_POINT ( 'NONE',  ( 3.453548899747295842, -11.60474049983370648, 33.02348890104160262 ) ) ;
#28056=CARTESIAN_POINT ( 'NONE',  ( 5.076923076923075762, -12.62096338111211580, 30.90682066428153263 ) ) ;
#28057=B_SPLINE_CURVE_WITH_KNOTS ( 'NONE', 3,
 ( #59217, #38064, #4731, #86725, #11040, #17803, #32207, #58773, #24541, #72728 ),
 .UNSPECIFIED., .F., .F.,
 ( 4, 2, 2, 2, 4 ),
 ( 0.000000000000000000, 0.0001954339857564078267, 0.0003908679715128156535, 0.0005863019572692235344, 0.0007817359430256313069 ),
 .UNSPECIFIED. ) ;
#28058=ORIENTED_EDGE ( 'NONE', *, *, #29687, .T. ) ;
#28059=FACE_BOUND ( 'NONE', #31783, .T. ) ;
#28060=CARTESIAN_POINT ( 'NONE',  ( 9.627037246346917598, -6.026961402152685388, 34.52809138561120506 ) ) ;
#28062=CARTESIAN_POINT ( 'NONE',  ( -6.989159302437059296, -9.905515769479276145, 34.41647553114623292 ) ) ;
#28063=DIRECTION ( 'NONE',  ( -0.000000000000000000, 0.3420201433256694901, -0.9396926207859082059 ) ) ;
#28064=ORIENTED_EDGE ( 'NONE', *, *, #58669, .F. ) ;
#28065=AXIS2_PLACEMENT_3D ( 'NONE', #66114, #58917, #11185 ) ;
#28066=CARTESIAN_POINT ( 'NONE',  ( -14.37296275365308418, -12.46129190929999986, 30.37095296980880832 ) ) ;
#28067=CARTESIAN_POINT ( 'NONE',  ( 15.23076923076923173, -2.292212530054420494, 30.41441678777542634 ) ) ;
#28068=CARTESIAN_POINT ( 'NONE',  ( 12.71159277317677549, -6.567000820036036579, 34.66262288849541306 ) ) ;
#28069=LINE ( 'NONE', #62284, #57636 ) ;
#28070=ORIENTED_EDGE ( 'NONE', *, *, #7197, .F. ) ;
#28071=CARTESIAN_POINT ( 'NONE',  ( 12.59158351745823445, -2.254550872974306674, 29.97347326024527092 ) ) ;
#28072=VERTEX_POINT ( 'NONE', #41053 ) ;
#28075=FACE_OUTER_BOUND ( 'NONE', #67778, .T. ) ;
#28076=CYLINDRICAL_SURFACE ( 'NONE', #59971, 0.2499999999999994726 ) ;
#28077=CARTESIAN_POINT ( 'NONE',  ( 13.16113044089144068, -9.331801661448606566, 34.40259984581193464 ) ) ;
#28078=CARTESIAN_POINT ( 'NONE',  ( -13.31935981333935359, -3.835265460703683349, 33.15142922261929925 ) ) ;
#28079=CARTESIAN_POINT ( 'NONE',  ( 3.230769230769231726, -12.09954503811598769, 35.62045528018868623 ) ) ;
#28080=CARTESIAN_POINT ( 'NONE',  ( 13.38461538461526601, -6.026961402154118019, 34.52809138561165270 ) ) ;
#28081=CARTESIAN_POINT ( 'NONE',  ( -16.28399412357784826, -8.630895178749536711, 34.87696386517710323 ) ) ;
#28082=B_SPLINE_CURVE_WITH_KNOTS ( 'NONE', 3,
 ( #4684, #16412, #17301, #44759, #9650, #10550, #37116, #64580, #2879, #30371 ),
 .UNSPECIFIED., .F., .F.,
 ( 4, 2, 2, 2, 4 ),
 ( 0.000000000000000000, 0.0001954311564186861968, 0.0003908623128373723936, 0.0005862934692560585904, 0.0007817246256747447872 ),
 .UNSPECIFIED. ) ;
#28083=CARTESIAN_POINT ( 'NONE',  ( 6.923076923076800782, -3.083524468854526912, 32.58852847137268327 ) ) ;
#28085=ORIENTED_EDGE ( 'NONE', *, *, #41772, .F. ) ;
#28086=B_SPLINE_CURVE_WITH_KNOTS ( 'NONE', 3,
 ( #65960, #31750, #59208, #53338, #86714, #39842, #67309, #60542, #40288, #28090 ),
 .UNSPECIFIED., .F., .F.,
 ( 4, 2, 2, 2, 4 ),
 ( 0.0007817246256747471724, 0.0009771112852218905021, 0.001172497944769033615, 0.001367884604316176944, 0.001563271263863320274 ),
 .UNSPECIFIED. ) ;
#28087=DIRECTION ( 'NONE',  ( 0.000000000000000000, 0.6427876096865373645, -0.7660444431189797898 ) ) ;
#28089=ORIENTED_EDGE ( 'NONE', *, *, #67908, .F. ) ;
#28090=CARTESIAN_POINT ( 'NONE',  ( -3.230769230769229949, -9.058645607665452459, 34.76329471203371924 ) ) ;
#28091=ORIENTED_EDGE ( 'NONE', *, *, #73017, .F. ) ;
#28092=FACE_OUTER_BOUND ( 'NONE', #60221, .T. ) ;
#28095=CARTESIAN_POINT ( 'NONE',  ( 3.230769230769231726, -8.120952969808772792, 34.71129190930000163 ) ) ;
#28096=VECTOR ( 'NONE', #70731, 1000.000000000000000 ) ;
#28097=DIRECTION ( 'NONE',  ( -0.000000000000000000, 0.000000000000000000, 1.000000000000000000 ) ) ;
#28098=CARTESIAN_POINT ( 'NONE',  ( 6.130525701763564150, -2.619367082507848554, 30.83698974864644171 ) ) ;
#28099=DIRECTION ( 'NONE',  ( 0.000000000000000000, 0.6427876096865373645, -0.7660444431189797898 ) ) ;
#28101=CARTESIAN_POINT ( 'NONE',  ( -4.377331097570102969, -3.754499324213721234, 33.06261337010820256 ) ) ;
#28102=CARTESIAN_POINT ( 'NONE',  ( 6.923076923076800782, -10.33852847137269571, 34.16647553114546554 ) ) ;
#28103=DIRECTION ( 'NONE',  ( -0.000000000000000000, 0.7660444431189791237, -0.6427876096865379196 ) ) ;
#28104=CARTESIAN_POINT ( 'NONE',  ( 11.53846153846141753, -5.219633306517616589, 34.19971097300220464 ) ) ;
#28105=CARTESIAN_POINT ( 'NONE',  ( -9.692307692307814193, -11.67786785259630911, 32.92929555188603530 ) ) ;
#28107=ORIENTED_EDGE ( 'NONE', *, *, #43185, .F. ) ;
#28108=FACE_OUTER_BOUND ( 'NONE', #35266, .T. ) ;
#28109=CARTESIAN_POINT ( 'NONE',  ( 1.634669804528839476, -3.435999193479609470, 33.07426656108011542 ) ) ;
#28110=CARTESIAN_POINT ( 'NONE',  ( -6.700064078983527516, -11.98016756924215009, 32.48728574198911190 ) ) ;
#28111=CARTESIAN_POINT ( 'NONE',  ( 9.915087361285756629, -12.11081565061823717, 32.26097654155341843 ) ) ;
#28112=LINE ( 'NONE', #83963, #8977 ) ;
#28113=CYLINDRICAL_SURFACE ( 'NONE', #55618, 0.2499999999999995559 ) ;
#28114=CARTESIAN_POINT ( 'NONE',  ( 5.076923076923075762, -3.886160181151819604, 36.00935417666054406 ) ) ;
#28115=EDGE_LOOP ( 'NONE', ( #83596, #14788, #8085, #39203 ) ) ;
#28116=CARTESIAN_POINT ( 'NONE',  ( 6.000000000000001776, -7.500000000000001776, 35.04278698407183867 ) ) ;
#28117=VERTEX_POINT ( 'NONE', #75282 ) ;
#28118=DIRECTION ( 'NONE',  ( -1.000000000000000000, 0.000000000000000000, 0.000000000000000000 ) ) ;
#28120=CARTESIAN_POINT ( 'NONE',  ( 10.61538461538461675, -4.098570777380720287, 33.41473453929634729 ) ) ;
#28121=CARTESIAN_POINT ( 'NONE',  ( -0.4615384615384611200, -6.386643153685126251, 34.62446782046654192 ) ) ;
#28122=CARTESIAN_POINT ( 'NONE',  ( 4.153846153846030731, -6.835583212225970762, 34.95778746994575670 ) ) ;
#28123=CARTESIAN_POINT ( 'NONE',  ( -3.453648747506816719, -7.630690623152302621, 34.99857592706774057 ) ) ;
#28125=EDGE_LOOP ( 'NONE', ( #71322, #52707 ) ) ;
#28126=EDGE_LOOP ( 'NONE', ( #29473, #62971, #51497, #17406 ) ) ;
#28127=ORIENTED_EDGE ( 'NONE', *, *, #49098, .F. ) ;
#28128=EDGE_CURVE ( 'NONE', #59563, #88887, #6811, .T. ) ;
#28129=CARTESIAN_POINT ( 'NONE',  ( 13.13463865367303463, -3.137211980971221781, 32.19342716148376837 ) ) ;
#28130=CARTESIAN_POINT ( 'NONE',  ( 7.596177115211490083, -3.627789207965226748, 32.91389620160131102 ) ) ;
#28131=CARTESIAN_POINT ( 'NONE',  ( 1.384615384615386802, -12.48256725967547354, 35.29906147534542527 ) ) ;
#28132=CARTESIAN_POINT ( 'NONE',  ( -15.23076923076922995, -11.16473453929635440, 33.15142922261926373 ) ) ;
#28133=VECTOR ( 'NONE', #11348, 1000.000000000000000 ) ;
#28135=CARTESIAN_POINT ( 'NONE',  ( -2.307692307692427391, -3.300289026999228881, 32.46337939537708905 ) ) ;
#28137=EDGE_LOOP ( 'NONE', ( #489, #28598 ) ) ;
#28138=AXIS2_PLACEMENT_3D ( 'NONE', #16020, #70521, #9272 ) ;
#28139=ORIENTED_EDGE ( 'NONE', *, *, #52356, .F. ) ;
#28140=CARTESIAN_POINT ( 'NONE',  ( 4.153846153846032507, -2.892918686052165622, 31.69288490824153470 ) ) ;
#28141=ORIENTED_EDGE ( 'NONE', *, *, #4365, .F. ) ;
#28143=CARTESIAN_POINT ( 'NONE',  ( -2.084912766423896002, -9.332535724633405749, 34.40230450496446224 ) ) ;
#28144=EDGE_CURVE ( 'NONE', #52360, #81993, #6207, .T. ) ;
#28146=EDGE_CURVE ( 'NONE', #10219, #13098, #63075, .T. ) ;
#28148=EDGE_LOOP ( 'NONE', ( #26762, #54706 ) ) ;
#28149=CARTESIAN_POINT ( 'NONE',  ( 4.087763774486017354, -3.937682226553329556, 33.60647404775217240 ) ) ;
#28150=ORIENTED_EDGE ( 'NONE', *, *, #68677, .T. ) ;
#28151=FACE_BOUND ( 'NONE', #42042, .T. ) ;
#28152=CARTESIAN_POINT ( 'NONE',  ( 6.856993512121043466, -4.098570777380720287, 33.41473453929634729 ) ) ;
#28153=EDGE_CURVE ( 'NONE', #77091, #15767, #27731, .T. ) ;
#28154=CARTESIAN_POINT ( 'NONE',  ( -4.283994123577847368, -10.31621877034669588, 34.18098118002070152 ) ) ;
#28156=CARTESIAN_POINT ( 'NONE',  ( 0.7115928814519137946, -8.346898887586323923, 34.93166121998716278 ) ) ;
#28157=CARTESIAN_POINT ( 'NONE',  ( -15.93106648486808119, -12.69155399931963046, 30.53255429739158444 ) ) ;
#28158=CARTESIAN_POINT ( 'NONE',  ( 9.019285189144222059, -8.346898887586323923, 34.93166121998716278 ) ) ;
#28159=CARTESIAN_POINT ( 'NONE',  ( 0.5267940328144852247, -6.879047030191282275, 34.71129190930002295 ) ) ;
#28160=CARTESIAN_POINT ( 'NONE',  ( -3.454254155333561283, -9.417330523894424488, 34.63758898049880486 ) ) ;
#28161=EDGE_LOOP ( 'NONE', ( #29714, #51578 ) ) ;
#28162=CARTESIAN_POINT ( 'NONE',  ( -12.33101302330481808, -2.372941743896879174, 30.88044141588253666 ) ) ;
#28163=CARTESIAN_POINT ( 'NONE',  ( -5.999999999999998224, -3.937682226553329556, 33.60647404775216529 ) ) ;
#28164=CARTESIAN_POINT ( 'NONE',  ( 0.2115152242454957365, -11.86270091957321071, 32.19358267280088626 ) ) ;
#28165=DIRECTION ( 'NONE',  ( 1.000000000000000000, 0.000000000000000000, 0.000000000000000000 ) ) ;
#28166=LINE ( 'NONE', #82690, #68874 ) ;
#28167=VECTOR ( 'NONE', #53769, 1000.000000000000227 ) ;
#28168=FACE_BOUND ( 'NONE', #29330, .T. ) ;
#28169=CARTESIAN_POINT ( 'NONE',  ( 4.853438133199128757, -11.41268669641500466, 32.86336882939237825 ) ) ;
#28170=DIRECTION ( 'NONE',  ( -0.000000000000000000, -0.3420201433256694346, -0.9396926207859080948 ) ) ;
#28171=CARTESIAN_POINT ( 'NONE',  ( 5.142990410273152513, -9.058645607665452459, 34.76329471203371924 ) ) ;
#28172=CARTESIAN_POINT ( 'NONE',  ( 3.930361229281823743, -5.827078755546623690, 34.72654668319379567 ) ) ;
#28173=CARTESIAN_POINT ( 'NONE',  ( 15.45378058238208219, -9.886259254753566594, 34.14407573483972413 ) ) ;
#28174=CARTESIAN_POINT ( 'NONE',  ( -15.23076923076922995, -3.886160181151819604, 36.00935417666054406 ) ) ;
#28177=CARTESIAN_POINT ( 'NONE',  ( 12.52679403281448600, -2.625532179533470512, 30.86335684631491105 ) ) ;
#28179=DIRECTION ( 'NONE',  ( -0.000000000000000000, -0.1736481776669307198, -0.9848077530122080203 ) ) ;
#28180=ORIENTED_EDGE ( 'NONE', *, *, #12587, .T. ) ;
#28182=CYLINDRICAL_SURFACE ( 'NONE', #34442, 0.2500000000000009437 ) ;
#28183=VECTOR ( 'NONE', #54136, 1000.000000000000227 ) ;
#28184=ORIENTED_EDGE ( 'NONE', *, *, #42226, .F. ) ;
#28185=CARTESIAN_POINT ( 'NONE',  ( -15.23076923076935074, -5.219633306517616589, 34.19971097300220464 ) ) ;
#28188=CARTESIAN_POINT ( 'NONE',  ( -5.142193077479396912, -3.083524468853724443, 32.58852847137143272 ) ) ;
#28189=CARTESIAN_POINT ( 'NONE',  ( 15.23076923076923173, -6.386643153685126251, 34.62446782046654192 ) ) ;
#28191=CARTESIAN_POINT ( 'NONE',  ( 6.989145274079363368, -4.098570777380720287, 33.41473453929635440 ) ) ;
#28192=CARTESIAN_POINT ( 'NONE',  ( 11.76124107972994537, -3.755027918224367767, 33.06320215134714857 ) ) ;
#28194=DIRECTION ( 'NONE',  ( -0.000000000000000000, 0.3420201433256694346, -0.9396926207859080948 ) ) ;
#28195=DIRECTION ( 'NONE',  ( 0.000000000000000000, -6.938893903907222067E-15, 1.000000000000000000 ) ) ;
#28196=ORIENTED_EDGE ( 'NONE', *, *, #48596, .F. ) ;
#28199=B_SPLINE_CURVE_WITH_KNOTS ( 'NONE', 3,
 ( #32759, #19252, #54351, #20135, #46718, #81404, #41299, #80516, #68319, #19687 ),
 .UNSPECIFIED., .F., .F.,
 ( 4, 2, 2, 2, 4 ),
 ( 0.000000000000000000, 0.0001954339857564082062, 0.0003908679715128164124, 0.0005863019572692246186, 0.0007817359430256328248 ),
 .UNSPECIFIED. ) ;
#28200=CARTESIAN_POINT ( 'NONE',  ( -15.93083330975275658, -12.38742843783360748, 31.66772728687926985 ) ) ;
#28201=CARTESIAN_POINT ( 'NONE',  ( -39.05038313613820122, -2.499999999999999556, 29.75000000000000355 ) ) ;
#28202=ORIENTED_EDGE ( 'NONE', *, *, #67690, .T. ) ;
#28203=B_SPLINE_CURVE_WITH_KNOTS ( 'NONE', 3,
 ( #53207, #40161, #11795, #87929, #75268, #46009, #26633, #73498, #67624, #60411 ),
 .UNSPECIFIED., .F., .F.,
 ( 4, 2, 2, 2, 4 ),
 ( 0.000000000000000000, 0.0001954339857564126514, 0.0003908679715128183098, 0.0005863019572692239681, 0.0007817359430256294638 ),
 .UNSPECIFIED. ) ;
#28205=DIRECTION ( 'NONE',  ( -0.000000000000000000, 1.000000000000000000, 3.491481338843133355E-15 ) ) ;
#28206=CARTESIAN_POINT ( 'NONE',  ( 16.15384615384615330, -8.564572088678739092, 35.78748833219616898 ) ) ;
#28207=CARTESIAN_POINT ( 'NONE',  ( 4.088576153289833925, -9.528491918058357157, 34.59228464037090589 ) ) ;
#28208=ORIENTED_EDGE ( 'NONE', *, *, #50505, .T. ) ;
#28209=CARTESIAN_POINT ( 'NONE',  ( -7.976764205778374084, -7.722926236386456367, 34.74524107206103452 ) ) ;
#28210=CARTESIAN_POINT ( 'NONE',  ( -3.099977422944444783, -4.809403383903226192, 33.96459661697924304 ) ) ;
#28211=EDGE_CURVE ( 'NONE', #54822, #77202, #53586, .T. ) ;
#28213=DIRECTION ( 'NONE',  ( -0.000000000000000000, 0.8660254037844399289, -0.4999999999999980016 ) ) ;
#28214=CARTESIAN_POINT ( 'NONE',  ( 4.826946345980720920, -4.236021600441998380, 33.53823185664189310 ) ) ;
#28215=FACE_OUTER_BOUND ( 'NONE', #53865, .T. ) ;
#28216=ORIENTED_EDGE ( 'NONE', *, *, #6301, .T. ) ;
#28217=CARTESIAN_POINT ( 'NONE',  ( 6.989144256427000101, -11.35647404775217595, 33.31231777344667222 ) ) ;
#28218=EDGE_LOOP ( 'NONE', ( #1188, #59127 ) ) ;
#28219=VERTEX_POINT ( 'NONE', #42393 ) ;
#28221=CARTESIAN_POINT ( 'NONE',  ( -16.21911615440247090, -3.643525952247790300, 33.31231777344662959 ) ) ;
#28223=EDGE_CURVE ( 'NONE', #22687, #70094, #80402, .T. ) ;
#28224=LINE ( 'NONE', #55255, #42192 ) ;
#28225=CARTESIAN_POINT ( 'NONE',  ( -17.14224599241525482, -7.749976743299138882, 34.99404534957040624 ) ) ;
#28226=VERTEX_POINT ( 'NONE', #81461 ) ;
#28228=ORIENTED_EDGE ( 'NONE', *, *, #35660, .T. ) ;
#28229=VECTOR ( 'NONE', #83366, 999.9999999999998863 ) ;
#28230=VERTEX_POINT ( 'NONE', #48987 ) ;
#28231=B_SPLINE_CURVE_WITH_KNOTS ( 'NONE', 3,
 ( #70725, #9029, #36498, #84694, #44553, #72485, #18445, #30608, #10793, #24746 ),
 .UNSPECIFIED., .F., .F.,
 ( 4, 2, 2, 2, 4 ),
 ( 0.000000000000000000, 0.0001954311564186863323, 0.0003908623128373726646, 0.0005862934692560590241, 0.0007817246256747453293 ),
 .UNSPECIFIED. ) ;
#28233=ORIENTED_EDGE ( 'NONE', *, *, #43823, .F. ) ;
#28234=CARTESIAN_POINT ( 'NONE',  ( -9.692307692307691624, -6.343179335718451384, 34.87096338111211935 ) ) ;
#28236=DIRECTION ( 'NONE',  ( -0.000000000000000000, 0.1736481776669307198, -0.9848077530122080203 ) ) ;
#28237=CARTESIAN_POINT ( 'NONE',  ( 6.130525438233644486, -2.647132371071621471, 31.75357179365173010 ) ) ;
#28238=EDGE_CURVE ( 'NONE', #41543, #79237, #68568, .T. ) ;
#28239=CARTESIAN_POINT ( 'NONE',  ( -3.007989689500820241, -4.387253974876676565, 33.66317474335728832 ) ) ;
#28241=EDGE_LOOP ( 'NONE', ( #86104, #22373, #46530, #25590 ) ) ;
#28242=VERTEX_POINT ( 'NONE', #28268 ) ;
#28243=ORIENTED_EDGE ( 'NONE', *, *, #15351, .T. ) ;
#28244=CARTESIAN_POINT ( 'NONE',  ( -9.442253380669381357, -5.728107161865378494, 34.42597550085002922 ) ) ;
#28245=CARTESIAN_POINT ( 'NONE',  ( 1.253923917947828093, -8.147922237126337563, 34.70805685702651999 ) ) ;
#28246=EDGE_LOOP ( 'NONE', ( #25567, #58198 ) ) ;
#28247=CARTESIAN_POINT ( 'NONE',  ( 2.307692307692186251, -2.657715359629662544, 31.77849191805970364 ) ) ;
#28248=CARTESIAN_POINT ( 'NONE',  ( -0.4615384615384611200, -6.343179335718451384, 34.87096338111211935 ) ) ;
#28250=EDGE_LOOP ( 'NONE', ( #4622, #73314, #20974, #40113 ) ) ;
#28251=EDGE_CURVE ( 'NONE', #9817, #88116, #40670, .T. ) ;
#28252=CARTESIAN_POINT ( 'NONE',  ( -11.47239318745910275, -4.786620604624113540, 33.94971097300155805 ) ) ;
#28253=CARTESIAN_POINT ( 'NONE',  ( -15.00798956179116317, -12.47679350104403007, 31.42216943046555855 ) ) ;
#28254=ORIENTED_EDGE ( 'NONE', *, *, #34034, .F. ) ;
#28255=FACE_BOUND ( 'NONE', #75545, .T. ) ;
#28256=CARTESIAN_POINT ( 'NONE',  ( -10.86536135943320502, -4.818429247618089661, 34.26397095200675125 ) ) ;
#28257=FACE_OUTER_BOUND ( 'NONE', #44203, .T. ) ;
#28259=DIRECTION ( 'NONE',  ( -0.000000000000000000, 0.6427876096865404731, -0.7660444431189770143 ) ) ;
#28260=CARTESIAN_POINT ( 'NONE',  ( 4.853438133199126980, -10.11188796281391511, 34.01382737946119050 ) ) ;
#28261=ADVANCED_FACE ( 'NONE', ( #75567 ), #34141, .F. ) ;
#28262=AXIS2_PLACEMENT_3D ( 'NONE', #18362, #46276, #73765 ) ;
#28263=FACE_OUTER_BOUND ( 'NONE', #63255, .T. ) ;
#28264=CARTESIAN_POINT ( 'NONE',  ( 17.99999999999987566, -2.892918686052165622, 31.69288490824153470 ) ) ;
#28265=ORIENTED_EDGE ( 'NONE', *, *, #67894, .F. ) ;
#28266=ADVANCED_FACE ( 'NONE', ( #55296 ), #82344, .F. ) ;
#28267=CARTESIAN_POINT ( 'NONE',  ( 11.47319109250076430, -3.300289026998414865, 32.46337939537583139 ) ) ;
#28268=CARTESIAN_POINT ( 'NONE',  ( 10.61538461538449596, -5.219633306517616589, 34.19971097300220464 ) ) ;
#28269=ORIENTED_EDGE ( 'NONE', *, *, #59581, .F. ) ;
#28270=B_SPLINE_CURVE_WITH_KNOTS ( 'NONE', 3,
 ( #8854, #9726, #23679, #16928, #42639, #70097, #1649, #29132, #84079, #22355 ),
 .UNSPECIFIED., .F., .F.,
 ( 4, 2, 2, 2, 4 ),
 ( 0.000000000000000000, 0.0001954311564186861968, 0.0003908623128373723936, 0.0005862934692560585904, 0.0007817246256747447872 ),
 .UNSPECIFIED. ) ;
#28271=CARTESIAN_POINT ( 'NONE',  ( -7.846153846153844924, -12.09954503811598769, 35.62045528018868623 ) ) ;
#28272=CARTESIAN_POINT ( 'NONE',  ( -7.780086512803768173, -2.292212530054420494, 30.41441678777542990 ) ) ;
#28273=EDGE_LOOP ( 'NONE', ( #58154, #35775, #25557, #11799 ) ) ;
#28275=CARTESIAN_POINT ( 'NONE',  ( 2.438482748659257737, -4.684288915650983043, 34.18129842949671371 ) ) ;
#28276=FACE_BOUND ( 'NONE', #83640, .T. ) ;
#28277=CARTESIAN_POINT ( 'NONE',  ( -1.634592128663975297, -6.524016743844655686, 34.90889640711025521 ) ) ;
#28278=CARTESIAN_POINT ( 'NONE',  ( 15.23076923076911093, -12.27809138561165270, 31.22303859784587132 ) ) ;
#28280=AXIS2_PLACEMENT_3D ( 'NONE', #84923, #64617, #37602 ) ;
#28281=DIRECTION ( 'NONE',  ( 0.000000000000000000, 0.9848077530122072432, -0.1736481776669354937 ) ) ;
#28282=CARTESIAN_POINT ( 'NONE',  ( 3.230769230769108269, -3.083524468854526912, 32.58852847137268327 ) ) ;
#28283=DIRECTION ( 'NONE',  ( -0.000000000000000000, 0.7660444431189791237, -0.6427876096865379196 ) ) ;
#28285=VERTEX_POINT ( 'NONE', #88232 ) ;
#28287=DIRECTION ( 'NONE',  ( -0.000000000000000000, 0.8660254037844397068, -0.4999999999999978906 ) ) ;
#28288=CARTESIAN_POINT ( 'NONE',  ( 17.99999999999987566, -2.379036618888197729, 30.90682066428292885 ) ) ;
#28289=CARTESIAN_POINT ( 'NONE',  ( 1.450682717965462443, -9.058645607665452459, 34.76329471203371924 ) ) ;
#28290=CARTESIAN_POINT ( 'NONE',  ( -1.515306851282944400, -3.062553014421049546, 32.05460306192773601 ) ) ;
#28291=CARTESIAN_POINT ( 'NONE',  ( -16.40386939113911779, -12.22074536777955345, 31.39888409691088356 ) ) ;
#28294=CARTESIAN_POINT ( 'NONE',  ( 6.700149964170073247, -2.308479472611653094, 30.53278059502174457 ) ) ;
#28295=CARTESIAN_POINT ( 'NONE',  ( 4.153846153846154188, -12.29105614889573062, 35.45975837776705220 ) ) ;
#28296=CARTESIAN_POINT ( 'NONE',  ( 15.36129493253280032, -11.93748526763465279, 32.05452791011430946 ) ) ;
#28297=LINE ( 'NONE', #61638, #40192 ) ;
#28298=CARTESIAN_POINT ( 'NONE',  ( -1.134615384615446976, -7.565270000091922853, 34.99999999999999289 ) ) ;
#28299=CARTESIAN_POINT ( 'NONE',  ( 16.28437185560972011, -5.195472089885680766, 34.18748526763464923 ) ) ;
#28300=LINE ( 'NONE', #55771, #25157 ) ;
#28301=EDGE_CURVE ( 'NONE', #84941, #72951, #11632, .T. ) ;
#28303=CARTESIAN_POINT ( 'NONE',  ( -14.05763799605399278, -3.136992222400443175, 32.19305428654138979 ) ) ;
#28304=FACE_OUTER_BOUND ( 'NONE', #24425, .T. ) ;
#28305=EDGE_LOOP ( 'NONE', ( #73456, #79417 ) ) ;
#28306=EDGE_CURVE ( 'NONE', #86041, #69985, #3000, .T. ) ;
#28307=CARTESIAN_POINT ( 'NONE',  ( 12.39626846098214230, -4.320704448112771878, 33.92786785259540494 ) ) ;
#28312=LINE ( 'NONE', #15254, #57017 ) ;
#28313=EDGE_LOOP ( 'NONE', ( #16704, #31585 ) ) ;
#28314=CYLINDRICAL_SURFACE ( 'NONE', #41333, 0.2500000000000009437 ) ;
#28315=CARTESIAN_POINT ( 'NONE',  ( -1.319359813339359588, -4.481592998940251427, 33.73612834413965089 ) ) ;
#28316=ORIENTED_EDGE ( 'NONE', *, *, #38878, .F. ) ;
#28318=DIRECTION ( 'NONE',  ( 0.000000000000000000, 0.1736481776669267785, -0.9848077530122087975 ) ) ;
#28319=AXIS2_PLACEMENT_3D ( 'NONE', #40096, #68430, #67113 ) ;
#28320=EDGE_LOOP ( 'NONE', ( #81306, #26818, #34203, #63173 ) ) ;
#28322=EDGE_CURVE ( 'NONE', #16142, #52128, #76072, .T. ) ;
#28323=CARTESIAN_POINT ( 'NONE',  ( 10.61538461538449418, -11.06231777344772027, 33.60647404775119895 ) ) ;
#28324=ORIENTED_EDGE ( 'NONE', *, *, #21224, .F. ) ;
#28325=CARTESIAN_POINT ( 'NONE',  ( 7.846153846153725020, -4.481592998941358097, 33.73612834414048933 ) ) ;
#28326=CARTESIAN_POINT ( 'NONE',  ( 2.530471976670374712, -8.540255544307065350, 34.89611431652622286 ) ) ;
#28327=CARTESIAN_POINT ( 'NONE',  ( 9.757562831820528970, -6.835583212224610072, 34.95778746994559327 ) ) ;
#28328=ORIENTED_EDGE ( 'NONE', *, *, #46592, .T. ) ;
#28329=EDGE_LOOP ( 'NONE', ( #35559, #61041, #56617, #60569 ) ) ;
#28330=CARTESIAN_POINT ( 'NONE',  ( 15.23076923076923173, -10.51840700105979565, 33.73612834413961536 ) ) ;
#28331=ORIENTED_EDGE ( 'NONE', *, *, #82842, .T. ) ;
#28332=CARTESIAN_POINT ( 'NONE',  ( -7.976301815885541657, -2.373036134822904319, 30.88089517874952250 ) ) ;
#28333=CARTESIAN_POINT ( 'NONE',  ( -6.923076923077045919, -2.657715359629662988, 31.77849191805970364 ) ) ;
#28334=CARTESIAN_POINT ( 'NONE',  ( -5.933932666649923249, -5.471508081941601098, 34.59228464037088457 ) ) ;
#28335=CARTESIAN_POINT ( 'NONE',  ( 23.00000000000000000, -10.75000000000000000, 27.25000000000000000 ) ) ;
#28336=CARTESIAN_POINT ( 'NONE',  ( 14.98074599347626368, -6.695914987888146541, 34.68535235679833306 ) ) ;
#28337=ADVANCED_FACE ( 'NONE', ( #63379 ), #2557, .F. ) ;
#28338=CARTESIAN_POINT ( 'NONE',  ( 0.5923767920252209773, -7.277220318596960169, 34.99547417642776992 ) ) ;
#28339=AXIS2_PLACEMENT_3D ( 'NONE', #18219, #51980, #52430 ) ;
#28342=VERTEX_POINT ( 'NONE', #23713 ) ;
#28343=DIRECTION ( 'NONE',  ( 0.000000000000000000, 0.8660254037844377084, 0.5000000000000015543 ) ) ;
#28344=ORIENTED_EDGE ( 'NONE', *, *, #72681, .T. ) ;
#28345=CARTESIAN_POINT ( 'NONE',  ( 7.715463243043541475, -2.494641256782728966, 31.33461815524612959 ) ) ;
#28346=ORIENTED_EDGE ( 'NONE', *, *, #57599, .F. ) ;
#28348=CARTESIAN_POINT ( 'NONE',  ( 2.307692307692187583, -5.219633306517616589, 34.19971097300220464 ) ) ;
#28349=EDGE_LOOP ( 'NONE', ( #76064, #45955 ) ) ;
#28350=FACE_OUTER_BOUND ( 'NONE', #43399, .T. ) ;
#28351=EDGE_LOOP ( 'NONE', ( #44396, #15811 ) ) ;
#28353=VERTEX_POINT ( 'NONE', #44421 ) ;
#28354=CARTESIAN_POINT ( 'NONE',  ( -12.46153846153846168, -3.322132147404559976, 32.92929555188717927 ) ) ;
#28355=ADVANCED_FACE ( 'NONE', ( #23280 ), #63826, .F. ) ;
#28357=ADVANCED_FACE ( 'NONE', ( #70143 ), #36799, .F. ) ;
#28358=CARTESIAN_POINT ( 'NONE',  ( -6.923076923076922462, -4.661471528628507777, 34.16647553114623292 ) ) ;
#28359=CARTESIAN_POINT ( 'NONE',  ( -16.15384615384615330, -1.044019251281081972, 31.83374038241031911 ) ) ;
#28360=B_SPLINE_CURVE_WITH_KNOTS ( 'NONE', 3,
 ( #78402, #51342, #67895, #16702, #33668, #39992, #6196, #88194, #44157, #17148 ),
 .UNSPECIFIED., .F., .F.,
 ( 4, 2, 2, 2, 4 ),
 ( 0.000000000000000000, 0.0001954311564186888531, 0.0003908623128373777062, 0.0005862934692560666135, 0.0007817246256747554124 ),
 .UNSPECIFIED. ) ;
#28362=FACE_BOUND ( 'NONE', #41161, .T. ) ;
#28363=CARTESIAN_POINT ( 'NONE',  ( 7.846153846153846700, -9.819645486525091727, 36.12317359536749706 ) ) ;
#28364=CARTESIAN_POINT ( 'NONE',  ( -5.076923076923075762, -13.53365097954675988, 30.81389545987213552 ) ) ;
#28365=EDGE_CURVE ( 'NONE', #59530, #3191, #58824, .T. ) ;
#28366=B_SPLINE_CURVE_WITH_KNOTS ( 'NONE', 3,
 ( #84158, #29212, #1724, #41834, #83262, #56665, #49021, #14806, #70179, #70624 ),
 .UNSPECIFIED., .F., .F.,
 ( 4, 2, 2, 2, 4 ),
 ( 0.0007817246256747505334, 0.0009771112852218954894, 0.001172497944769040554, 0.001367884604316185618, 0.001563271263863330682 ),
 .UNSPECIFIED. ) ;
#28367=CARTESIAN_POINT ( 'NONE',  ( 9.627037691751372250, -2.379036618887870436, 30.90682066428147934 ) ) ;
#28368=CARTESIAN_POINT ( 'NONE',  ( -17.07692307692319744, -12.51329471203414379, 31.30864560766407578 ) ) ;
#28369=CARTESIAN_POINT ( 'NONE',  ( -4.946132635956124624, -3.957578996910242619, 33.62503395064540257 ) ) ;
#28370=CARTESIAN_POINT ( 'NONE',  ( -16.15384615384615330, -2.486705287966279876, 31.30864560766543647 ) ) ;
#28371=ORIENTED_EDGE ( 'NONE', *, *, #15405, .F. ) ;
#28374=CARTESIAN_POINT ( 'NONE',  ( -14.30769230769230660, -11.16473453929635440, 33.15142922261926373 ) ) ;
#28375=VERTEX_POINT ( 'NONE', #79572 ) ;
#28376=EDGE_LOOP ( 'NONE', ( #14295, #7157 ) ) ;
#28377=CARTESIAN_POINT ( 'NONE',  ( 7.596177115211491859, -6.567427716900047230, 34.66269422305636283 ) ) ;
#28378=CARTESIAN_POINT ( 'NONE',  ( 10.61538461538449418, -12.70778746994576025, 30.41441678777401236 ) ) ;
#28379=CARTESIAN_POINT ( 'NONE',  ( 15.23076923076923173, -5.415277668671390821, 36.20867863119892149 ) ) ;
#28380=CARTESIAN_POINT ( 'NONE',  ( 7.912221179503920787, -3.322132147404559976, 32.92929555188717927 ) ) ;
#28381=CARTESIAN_POINT ( 'NONE',  ( -10.61538461538461320, -12.34228464037088635, 31.77849191805839268 ) ) ;
#28383=VERTEX_POINT ( 'NONE', #18310 ) ;
#28385=CARTESIAN_POINT ( 'NONE',  ( -15.23076923076935074, -10.21337939537710326, 33.94971097300076224 ) ) ;
#28386=CARTESIAN_POINT ( 'NONE',  ( 17.20771488474786892, -6.413143153341454017, 34.63066358083362672 ) ) ;
#28387=DIRECTION ( 'NONE',  ( 0.000000000000000000, 0.7660444431189807890, 0.6427876096865361433 ) ) ;
#28388=CARTESIAN_POINT ( 'NONE',  ( -15.36132982251114854, -2.504760397472875155, 29.97295953869789997 ) ) ;
#28392=B_SPLINE_CURVE_WITH_KNOTS ( 'NONE', 3,
 ( #42151, #35376, #15115, #15558, #42589, #22743, #50203, #70048, #8359, #36710 ),
 .UNSPECIFIED., .F., .F.,
 ( 4, 2, 2, 2, 4 ),
 ( 0.000000000000000000, 0.0001954311564186861697, 0.0003908623128373723394, 0.0005862934692560584820, 0.0007817246256747446788 ),
 .UNSPECIFIED. ) ;
#28393=EDGE_LOOP ( 'NONE', ( #27005, #72760 ) ) ;
#28395=CARTESIAN_POINT ( 'NONE',  ( -7.146561866800870355, -8.496056993536548418, 34.65000542017679663 ) ) ;
#28396=EDGE_CURVE ( 'NONE', #56689, #13581, #85823, .T. ) ;
#28398=CARTESIAN_POINT ( 'NONE',  ( 12.46153846153833911, -4.481592998941358097, 33.73612834414048933 ) ) ;
#28399=CARTESIAN_POINT ( 'NONE',  ( 15.29602437028207085, -4.320704448112861584, 33.92786785259548310 ) ) ;
#28401=CARTESIAN_POINT ( 'NONE',  ( -16.85391172531022619, -12.15243808032446005, 31.58219941686247978 ) ) ;
#28402=DIRECTION ( 'NONE',  ( 0.000000000000000000, 0.9396926207859126468, 0.3420201433256571111 ) ) ;
#28403=VERTEX_POINT ( 'NONE', #58837 ) ;
#28404=CARTESIAN_POINT ( 'NONE',  ( -14.30769230769230660, -8.564572088678739092, 35.78748833219616898 ) ) ;
#28405=CARTESIAN_POINT ( 'NONE',  ( 15.23076923076923173, -9.819645486525091727, 36.12317359536749706 ) ) ;
#28408=CARTESIAN_POINT ( 'NONE',  ( 18.00000000000000000, -9.780366693483667717, 34.19971097300155094 ) ) ;
#28409=LINE ( 'NONE', #48232, #41516 ) ;
#28410=B_SPLINE_CURVE_WITH_KNOTS ( 'NONE', 3,
 ( #15576, #9267, #16898, #30849, #16456, #85813, #64180, #43924, #57432, #43043 ),
 .UNSPECIFIED., .F., .F.,
 ( 4, 2, 2, 2, 4 ),
 ( 0.0007817246256747528103, 0.0009771112852218980915, 0.001172497944769043156, 0.001367884604316188437, 0.001563271263863333718 ),
 .UNSPECIFIED. ) ;
#28411=CARTESIAN_POINT ( 'NONE',  ( -3.360916440207450950, -5.195881422630167279, 34.18770438780618548 ) ) ;
#28412=EDGE_CURVE ( 'NONE', #59880, #45204, #17047, .T. ) ;
#28413=CARTESIAN_POINT ( 'NONE',  ( -17.74994558008654622, -10.82426656108011720, 33.81400080652039009 ) ) ;
#28414=AXIS2_PLACEMENT_3D ( 'NONE', #68418, #58655, #45143 ) ;
#28415=DIRECTION ( 'NONE',  ( 0.000000000000000000, 0.7660444431189807890, 0.6427876096865361433 ) ) ;
#28416=B_SPLINE_CURVE_WITH_KNOTS ( 'NONE', 3,
 ( #53170, #45973, #79775, #80218, #79326, #18958, #73464, #46423, #38785, #5001 ),
 .UNSPECIFIED., .F., .F.,
 ( 4, 2, 2, 2, 4 ),
 ( 0.0007817246256747486903, 0.0009771112852218918031, 0.001172497944769034699, 0.001367884604316177595, 0.001563271263863320708 ),
 .UNSPECIFIED. ) ;
#28417=CYLINDRICAL_SURFACE ( 'NONE', #60818, 0.2500000000000009437 ) ;
#28420=B_SPLINE_CURVE_WITH_KNOTS ( 'NONE', 3,
 ( #56166, #343, #21938, #63801, #76886, #49841, #7984, #14745, #35005, #14293 ),
 .UNSPECIFIED., .F., .F.,
 ( 4, 2, 2, 2, 4 ),
 ( 0.0007817246256747442451, 0.0009771112852218870326, 0.001172497944769029929, 0.001367884604316172825, 0.001563271263863315504 ),
 .UNSPECIFIED. ) ;
#28423=CARTESIAN_POINT ( 'NONE',  ( 0.5267940328144856688, -3.300289026998475705, 32.46337939537591666 ) ) ;
#28424=B_SPLINE_CURVE_WITH_KNOTS ( 'NONE', 3,
 ( #10911, #44672, #66741, #38381, #65836, #4138, #12242, #39728, #31625, #67192 ),
 .UNSPECIFIED., .F., .F.,
 ( 4, 2, 2, 2, 4 ),
 ( 0.0007817359430256320659, 0.0009771253907249987086, 0.001172514838424365460, 0.001367904286123732211, 0.001563293733823098962 ),
 .UNSPECIFIED. ) ;
#28425=CARTESIAN_POINT ( 'NONE',  ( 8.096208157792158744, -2.564540009722895419, 30.55348353981670684 ) ) ;
#28426=CARTESIAN_POINT ( 'NONE',  ( -2.980823821391186623, -10.92531984108285670, 33.72920026020278073 ) ) ;
#28427=ORIENTED_EDGE ( 'NONE', *, *, #80603, .T. ) ;
#28429=CARTESIAN_POINT ( 'NONE',  ( -3.453695448285375669, -10.61292498521070549, 33.66303323003028680 ) ) ;
#28431=EDGE_CURVE ( 'NONE', #38427, #57345, #82472, .T. ) ;
#28432=CARTESIAN_POINT ( 'NONE',  ( 10.61538461538461675, -12.37446782046654192, 30.86335684631486131 ) ) ;
#28433=VERTEX_POINT ( 'NONE', #25061 ) ;
#28434=CARTESIAN_POINT ( 'NONE',  ( 17.01165263096229907, -3.300289026998414865, 32.46337939537583139 ) ) ;
#28435=EDGE_CURVE ( 'NONE', #49386, #53248, #83590, .T. ) ;
#28436=CARTESIAN_POINT ( 'NONE',  ( 7.912222197156284054, -5.557115091759786019, 34.35708131394839882 ) ) ;
#28437=CARTESIAN_POINT ( 'NONE',  ( 7.716006636715624367, -10.19110544564092002, 33.96427741523702792 ) ) ;
#28439=CARTESIAN_POINT ( 'NONE',  ( -2.372962308248626417, -12.16647553114622049, 32.15551576947930812 ) ) ;
#28441=ORIENTED_EDGE ( 'NONE', *, *, #78966, .F. ) ;
#28442=CARTESIAN_POINT ( 'NONE',  ( -6.923076923076922462, -8.164416787775445883, 34.95778746994557906 ) ) ;
#28443=CARTESIAN_POINT ( 'NONE',  ( 0.5276057948885364279, -9.905515769479277921, 34.41647553114623292 ) ) ;
#28444=ORIENTED_EDGE ( 'NONE', *, *, #8622, .F. ) ;
#28445=AXIS2_PLACEMENT_3D ( 'NONE', #77068, #8167, #961 ) ;
#28446=FACE_OUTER_BOUND ( 'NONE', #82640, .T. ) ;
#28447=CARTESIAN_POINT ( 'NONE',  ( -14.43784027742400689, -2.373036134822904319, 30.88089517874952250 ) ) ;
#28448=EDGE_CURVE ( 'NONE', #47121, #8365, #8436, .T. ) ;
#28449=CARTESIAN_POINT ( 'NONE',  ( -11.60373198442231413, -6.879047030191174805, 34.71129190930000163 ) ) ;
#28451=B_SPLINE_CURVE_WITH_KNOTS ( 'NONE', 3,
 ( #58716, #86217, #24933, #52398, #60050, #87555, #19076, #51952, #79448, #45652 ),
 .UNSPECIFIED., .F., .F.,
 ( 4, 2, 2, 2, 4 ),
 ( 0.000000000000000000, 0.0001954339857564080165, 0.0003908679715128160329, 0.0005863019572692240765, 0.0007817359430256320659 ),
 .UNSPECIFIED. ) ;
#28453=B_SPLINE_CURVE_WITH_KNOTS ( 'NONE', 3,
 ( #85946, #72419, #3515, #51686, #79187, #11623, #18823, #72863, #66565, #73777 ),
 .UNSPECIFIED., .F., .F.,
 ( 4, 2, 2, 2, 4 ),
 ( 0.000000000000000000, 0.0001954339857564063360, 0.0003908679715128126719, 0.0005863019572692189808, 0.0007817359430256253438 ),
 .UNSPECIFIED. ) ;
#28454=CARTESIAN_POINT ( 'NONE',  ( -11.47239420511146157, -5.471508081941601098, 34.59228464037088457 ) ) ;
#28456=B_SPLINE_CURVE_WITH_KNOTS ( 'NONE', 3,
 ( #28132, #14179, #5650, #61471, #34454, #60590, #80888, #47069, #88105, #27252 ),
 .UNSPECIFIED., .F., .F.,
 ( 4, 2, 2, 2, 4 ),
 ( 0.000000000000000000, 0.0001954339857564063089, 0.0003908679715128126177, 0.0005863019572692189808, 0.0007817359430256252354 ),
 .UNSPECIFIED. ) ;
#28457=B_SPLINE_CURVE_WITH_KNOTS ( 'NONE', 3,
 ( #46995, #27177, #47441, #33052, #74936, #28068, #83016, #6033, #33501, #6903 ),
 .UNSPECIFIED., .F., .F.,
 ( 4, 2, 2, 2, 4 ),
 ( 0.0007817359430256297891, 0.0009771253907249958896, 0.001172514838424361990, 0.001367904286123728091, 0.001563293733823094191 ),
 .UNSPECIFIED. ) ;
#28458=EDGE_LOOP ( 'NONE', ( #15625, #32945, #50167, #27593 ) ) ;
#28459=ORIENTED_EDGE ( 'NONE', *, *, #1948, .F. ) ;
#28460=FACE_BOUND ( 'NONE', #77130, .T. ) ;
#28461=ORIENTED_EDGE ( 'NONE', *, *, #65193, .T. ) ;
#28462=DIRECTION ( 'NONE',  ( 0.000000000000000000, 1.000000000000000000, 0.000000000000000000 ) ) ;
#28463=AXIS2_PLACEMENT_3D ( 'NONE', #32157, #79456, #58725 ) ;
#28465=CARTESIAN_POINT ( 'NONE',  ( -2.980769230767811084, -7.500000000000154543, 35.00000000000007105 ) ) ;
#28466=CARTESIAN_POINT ( 'NONE',  ( -6.222926217516146608, -12.15238873228292071, 31.58232369045353849 ) ) ;
#28470=VERTEX_POINT ( 'NONE', #68264 ) ;
#28471=CYLINDRICAL_SURFACE ( 'NONE', #82210, 0.2499999999999995559 ) ;
#28472=EDGE_LOOP ( 'NONE', ( #8759, #81697 ) ) ;
#28474=FACE_OUTER_BOUND ( 'NONE', #63454, .T. ) ;
#28475=FACE_OUTER_BOUND ( 'NONE', #74040, .T. ) ;
#28476=CARTESIAN_POINT ( 'NONE',  ( -17.29985003582992320, -2.889293201056495786, 32.26117774369186009 ) ) ;
#28477=CARTESIAN_POINT ( 'NONE',  ( 13.38461538461538680, -10.51840700105979565, 33.73612834413961536 ) ) ;
#28479=CARTESIAN_POINT ( 'NONE',  ( -6.130147969731694069, -6.809168938359898782, 34.95455904226513866 ) ) ;
#28480=CARTESIAN_POINT ( 'NONE',  ( 14.30769230769231015, -6.386643153685126251, 34.62446782046654192 ) ) ;
#28481=CARTESIAN_POINT ( 'NONE',  ( -11.66915300512910214, -3.062553014421049546, 32.05460306192773601 ) ) ;
#28482=ORIENTED_EDGE ( 'NONE', *, *, #5439, .F. ) ;
#28483=EDGE_CURVE ( 'NONE', #26583, #81768, #67462, .T. ) ;
#28484=ORIENTED_EDGE ( 'NONE', *, *, #32138, .T. ) ;
#28486=CARTESIAN_POINT ( 'NONE',  ( 4.153846153846030731, -3.083524468854526912, 32.58852847137268327 ) ) ;
#28488=CARTESIAN_POINT ( 'NONE',  ( -3.164701897419154975, -9.905515769479277921, 34.41647553114623292 ) ) ;
#28489=CARTESIAN_POINT ( 'NONE',  ( 1.634560793993429684, -11.56426240980093567, 33.07394671870546432 ) ) ;
#28490=EDGE_CURVE ( 'NONE', #17200, #58944, #52464, .T. ) ;
#28491=B_SPLINE_CURVE_WITH_KNOTS ( 'NONE', 3,
 ( #59329, #53005, #18799, #30959, #10264, #46268, #25104, #37725, #86837, #52566 ),
 .UNSPECIFIED., .F., .F.,
 ( 4, 2, 2, 2, 4 ),
 ( 0.0007817359430256303312, 0.0009771253907249965402, 0.001172514838424362641, 0.001367904286123728958, 0.001563293733823095059 ),
 .UNSPECIFIED. ) ;
#28492=CARTESIAN_POINT ( 'NONE',  ( -6.923076923076922462, -5.180354513474913603, 36.12317359536750416 ) ) ;
#28493=CARTESIAN_POINT ( 'NONE',  ( -2.057746898314264161, -2.589246495874657938, 31.60778113518102828 ) ) ;
#28494=FACE_BOUND ( 'NONE', #20797, .T. ) ;
#28495=CARTESIAN_POINT ( 'NONE',  ( 8.769230769230645706, -11.06231777344772027, 33.60647404775119895 ) ) ;
#28496=ORIENTED_EDGE ( 'NONE', *, *, #58954, .T. ) ;
#28498=CARTESIAN_POINT ( 'NONE',  ( -9.692307692307691624, -6.189225973068211317, 35.74407628777942847 ) ) ;
#28499=FACE_OUTER_BOUND ( 'NONE', #62569, .T. ) ;
#28500=DIRECTION ( 'NONE',  ( -0.000000000000000000, 0.6427876096865404731, -0.7660444431189770143 ) ) ;
#28501=ORIENTED_EDGE ( 'NONE', *, *, #19373, .F. ) ;
#28502=EDGE_CURVE ( 'NONE', #36501, #31652, #19633, .T. ) ;
#28504=VECTOR ( 'NONE', #32044, 1000.000000000000000 ) ;
#28505=ORIENTED_EDGE ( 'NONE', *, *, #13114, .F. ) ;
#28506=FACE_BOUND ( 'NONE', #65736, .T. ) ;
#28507=CARTESIAN_POINT ( 'NONE',  ( 9.562160482869472844, -6.001485441113819874, 34.52039167877662607 ) ) ;
#28509=CARTESIAN_POINT ( 'NONE',  ( 4.403791563224195293, -2.589246495874657938, 31.60778113518102828 ) ) ;
#28510=CARTESIAN_POINT ( 'NONE',  ( -3.165513659493205623, -8.613356846314928816, 34.62446782046653482 ) ) ;
#28512=ORIENTED_EDGE ( 'NONE', *, *, #46620, .T. ) ;
#28513=CARTESIAN_POINT ( 'NONE',  ( -14.55766903863466055, -12.41269422305637171, 30.68257228309993323 ) ) ;
#28514=CARTESIAN_POINT ( 'NONE',  ( -5.999999999999998224, -9.058645607665452459, 34.76329471203371924 ) ) ;
#28515=CARTESIAN_POINT ( 'NONE',  ( -9.942284423250045577, -3.137211980971221781, 32.19342716148376837 ) ) ;
#28516=FACE_OUTER_BOUND ( 'NONE', #14171, .T. ) ;
#28517=ORIENTED_EDGE ( 'NONE', *, *, #37652, .F. ) ;
#28518=EDGE_CURVE ( 'NONE', #64799, #32448, #20255, .T. ) ;
#28519=CARTESIAN_POINT ( 'NONE',  ( -12.21148414990014963, -3.136992222400443175, 32.19305428654138979 ) ) ;
#28520=ORIENTED_EDGE ( 'NONE', *, *, #62123, .T. ) ;
#28521=CARTESIAN_POINT ( 'NONE',  ( -9.019254006523736322, -3.711651800289232028, 33.01384336483936011 ) ) ;
#28522=ORIENTED_EDGE ( 'NONE', *, *, #56450, .F. ) ;
#28523=CARTESIAN_POINT ( 'NONE',  ( -9.019230769230768274, -7.500000000000001776, 34.75000000000000000 ) ) ;
#28524=CARTESIAN_POINT ( 'NONE',  ( -10.74553182482283198, -12.45813303252208648, 30.39737893381572675 ) ) ;
#28525=DIRECTION ( 'NONE',  ( -0.000000000000000000, -0.9396926207859093161, -0.3420201433256663259 ) ) ;
#28526=DIRECTION ( 'NONE',  ( 0.000000000000000000, -0.000000000000000000, 1.000000000000000000 ) ) ;
#28527=CARTESIAN_POINT ( 'NONE',  ( 16.94623247381277054, -4.684245665217972032, 34.18127051446801090 ) ) ;
#28528=CARTESIAN_POINT ( 'NONE',  ( -3.100243792535585907, -4.299079248970732792, 33.91157788607253565 ) ) ;
#28529=CARTESIAN_POINT ( 'NONE',  ( -16.82697755857493505, -8.433404298154332679, 34.66254593164985920 ) ) ;
#28531=B_SPLINE_CURVE_WITH_KNOTS ( 'NONE', 3,
 ( #31434, #17923, #58898, #86400, #24671, #52138, #46282, #52581, #72852, #66095 ),
 .UNSPECIFIED., .F., .F.,
 ( 4, 2, 2, 2, 4 ),
 ( 0.000000000000000000, 0.0001954311564186861697, 0.0003908623128373723394, 0.0005862934692560584820, 0.0007817246256747446788 ),
 .UNSPECIFIED. ) ;
#28534=VERTEX_POINT ( 'NONE', #55185 ) ;
#28535=EDGE_CURVE ( 'NONE', #33270, #38366, #82681, .T. ) ;
#28536=CARTESIAN_POINT ( 'NONE',  ( -16.15384615384615330, -4.661471528628507777, 34.16647553114623292 ) ) ;
#28537=VERTEX_POINT ( 'NONE', #22727 ) ;
#28539=EDGE_CURVE ( 'NONE', #80310, #86521, #1135, .T. ) ;
#28540=FACE_OUTER_BOUND ( 'NONE', #37305, .T. ) ;
#28541=ORIENTED_EDGE ( 'NONE', *, *, #73003, .F. ) ;
#28542=CARTESIAN_POINT ( 'NONE',  ( 17.01083966596719677, -4.786620604624113540, 33.94971097300155805 ) ) ;
#28543=FACE_OUTER_BOUND ( 'NONE', #81867, .T. ) ;
#28544=DIRECTION ( 'NONE',  ( 0.000000000000000000, 0.8660254037844377084, 0.5000000000000015543 ) ) ;
#28546=CARTESIAN_POINT ( 'NONE',  ( 1.319345384059066539, -2.657715359629089225, 31.77849191805834295 ) ) ;
#28547=CARTESIAN_POINT ( 'NONE',  ( -4.826868765284762830, -3.627508038966690496, 32.91356715214248396 ) ) ;
#28548=CARTESIAN_POINT ( 'NONE',  ( 8.769230769230768274, -11.16473453929635440, 33.15142922261926373 ) ) ;
#28549=CARTESIAN_POINT ( 'NONE',  ( 15.93036121012220541, -11.89387501736623420, 32.13663884655804992 ) ) ;
#28550=CARTESIAN_POINT ( 'NONE',  ( 6.250000000001421085, -7.500000000000154543, 35.00000000000007105 ) ) ;
#28551=CARTESIAN_POINT ( 'NONE',  ( 10.39245839786846659, -2.554751324335735152, 30.48935550225260727 ) ) ;
#28552=CARTESIAN_POINT ( 'NONE',  ( 15.23076923076923173, -9.058645607665452459, 34.76329471203371924 ) ) ;
#28554=AXIS2_PLACEMENT_3D ( 'NONE', #48600, #69332, #76529 ) ;
#28555=CARTESIAN_POINT ( 'NONE',  ( 5.076923076922954969, -2.892918686052165622, 31.69288490824153470 ) ) ;
#28556=DIRECTION ( 'NONE',  ( -0.000000000000000000, -0.1736481776669307198, -0.9848077530122080203 ) ) ;
#28557=B_SPLINE_CURVE_WITH_KNOTS ( 'NONE', 3,
 ( #26203, #27087, #60873, #88375, #60427, #87942, #26648, #47802, #39731, #68514 ),
 .UNSPECIFIED., .F., .F.,
 ( 4, 2, 2, 2, 4 ),
 ( 0.000000000000000000, 0.0001954339857564082604, 0.0003908679715128165208, 0.0005863019572692248355, 0.0007817359430256330417 ),
 .UNSPECIFIED. ) ;
#28558=B_SPLINE_CURVE_WITH_KNOTS ( 'NONE', 3,
 ( #53204, #80707, #31610, #23945, #32056, #59964, #87024, #73495, #4582, #51396 ),
 .UNSPECIFIED., .F., .F.,
 ( 4, 2, 2, 2, 4 ),
 ( 0.0007817359430256282712, 0.0009771253907249945886, 0.001172514838424361123, 0.001367904286123727657, 0.001563293733823093975 ),
 .UNSPECIFIED. ) ;
#28559=VERTEX_POINT ( 'NONE', #56523 ) ;
#28560=VERTEX_POINT ( 'NONE', #69592 ) ;
#28561=CARTESIAN_POINT ( 'NONE',  ( -15.16470087976679437, -8.120952969808772792, 34.71129190929999453 ) ) ;
#28562=CARTESIAN_POINT ( 'NONE',  ( 1.384615384615386802, -2.517432740324522911, 35.29906147534542527 ) ) ;
#28563=DIRECTION ( 'NONE',  ( -0.000000000000000000, 0.6427876096865404731, -0.7660444431189770143 ) ) ;
#28564=ORIENTED_EDGE ( 'NONE', *, *, #1889, .T. ) ;
#28565=CARTESIAN_POINT ( 'NONE',  ( 12.46153846153833911, -9.442884908241554243, 34.35708131394783038 ) ) ;
#28566=EDGE_CURVE ( 'NONE', #45473, #86086, #35361, .T. ) ;
#28567=DIRECTION ( 'NONE',  ( 0.000000000000000000, 0.4999999999999985567, 0.8660254037844395958 ) ) ;
#28568=CARTESIAN_POINT ( 'NONE',  ( 9.019285080869083870, -4.235687564193448829, 33.53795663066793509 ) ) ;
#28570=EDGE_CURVE ( 'NONE', #16685, #21791, #63273, .T. ) ;
#28571=VERTEX_POINT ( 'NONE', #9662 ) ;
#28572=CARTESIAN_POINT ( 'NONE',  ( -14.43784027742400689, -12.70455904226513866, 30.44083106164009322 ) ) ;
#28573=ORIENTED_EDGE ( 'NONE', *, *, #41553, .T. ) ;
#28574=VECTOR ( 'NONE', #71469, 1000.000000000000114 ) ;
#28575=EDGE_CURVE ( 'NONE', #41328, #32904, #2888, .T. ) ;
#28577=CARTESIAN_POINT ( 'NONE',  ( 4.220012760437793276, -7.250054591869668386, 34.99404684341514127 ) ) ;
#28578=CARTESIAN_POINT ( 'NONE',  ( -39.05038313613820122, -2.499999999999999556, 29.75000000000000355 ) ) ;
#28579=LINE ( 'NONE', #217, #55153 ) ;
#28580=CARTESIAN_POINT ( 'NONE',  ( -6.792551484843279752, -2.647132371071621471, 31.75357179365173010 ) ) ;
#28581=ORIENTED_EDGE ( 'NONE', *, *, #5878, .T. ) ;
#28583=VERTEX_POINT ( 'NONE', #2021 ) ;
#28584=ORIENTED_EDGE ( 'NONE', *, *, #5089, .T. ) ;
#28585=CARTESIAN_POINT ( 'NONE',  ( -3.453635493832329484, -2.251424796025575770, 29.88072029997477586 ) ) ;
#28586=CARTESIAN_POINT ( 'NONE',  ( -2.531177232256636156, -10.23692288466677880, 34.23039457007281072 ) ) ;
#28587=CARTESIAN_POINT ( 'NONE',  ( -12.21159305216042057, -12.45601412856602686, 31.48342859153981621 ) ) ;
#28588=B_SPLINE_CURVE_WITH_KNOTS ( 'NONE', 3,
 ( #7933, #61095, #55226, #75070, #42175, #14244, #13356, #29869, #40837, #69188 ),
 .UNSPECIFIED., .F., .F.,
 ( 4, 2, 2, 2, 4 ),
 ( 0.0007817359430256215491, 0.0009771253907249856981, 0.001172514838424349847, 0.001367904286123713779, 0.001563293733823077928 ),
 .UNSPECIFIED. ) ;
#28589=CARTESIAN_POINT ( 'NONE',  ( -2.307692307692428724, -11.67786785259630911, 32.92929555188603530 ) ) ;
#28591=CARTESIAN_POINT ( 'NONE',  ( -18.00000000000012079, -4.481592998941359873, 33.73612834414048933 ) ) ;
#28592=CYLINDRICAL_SURFACE ( 'NONE', #12123, 0.2500000000000008882 ) ;
#28593=VERTEX_POINT ( 'NONE', #8790 ) ;
#28594=EDGE_LOOP ( 'NONE', ( #28733, #85647, #14269, #59577, #14940, #72112 ) ) ;
#28595=VERTEX_POINT ( 'NONE', #57849 ) ;
#28596=AXIS2_PLACEMENT_3D ( 'NONE', #61575, #40445, #82753 ) ;
#28597=CARTESIAN_POINT ( 'NONE',  ( -10.61538461538461320, -2.499999999999998668, 29.75000000000001421 ) ) ;
#28598=ORIENTED_EDGE ( 'NONE', *, *, #61260, .T. ) ;
#28599=CARTESIAN_POINT ( 'NONE',  ( -16.82697755857493505, -9.272278438253401589, 34.42582936511637826 ) ) ;
#28600=CARTESIAN_POINT ( 'NONE',  ( -5.299850035829924089, -12.64616026154729411, 30.79003144601913533 ) ) ;
#28601=DIRECTION ( 'NONE',  ( -0.000000000000000000, -0.3420201433256694901, -0.9396926207859082059 ) ) ;
#28604=VECTOR ( 'NONE', #78677, 1000.000000000000114 ) ;
#28605=ORIENTED_EDGE ( 'NONE', *, *, #6367, .F. ) ;
#28606=CARTESIAN_POINT ( 'NONE',  ( 4.088576153289834814, -4.320704448112771878, 33.92786785259540494 ) ) ;
#28607=ORIENTED_EDGE ( 'NONE', *, *, #26591, .F. ) ;
#28608=FACE_BOUND ( 'NONE', #81426, .T. ) ;
#28609=LINE ( 'NONE', #70028, #31667 ) ;
#28611=ORIENTED_EDGE ( 'NONE', *, *, #7938, .F. ) ;
#28612=CARTESIAN_POINT ( 'NONE',  ( 15.48076923076929567, -7.434744860731433924, 35.00000000000000711 ) ) ;
#28613=CARTESIAN_POINT ( 'NONE',  ( -9.915234651214539952, -4.762599654559228846, 34.23009711892697737 ) ) ;
#28616=CARTESIAN_POINT ( 'NONE',  ( 0.5276068125408995835, -12.37446782046654192, 30.86335684631486842 ) ) ;
#28617=ORIENTED_EDGE ( 'NONE', *, *, #36621, .T. ) ;
#28618=B_SPLINE_CURVE_WITH_KNOTS ( 'NONE', 3,
 ( #26656, #68094, #68969, #13145, #12253, #20352, #81607, #6822, #75292, #33420 ),
 .UNSPECIFIED., .F., .F.,
 ( 4, 2, 2, 2, 4 ),
 ( 0.0007817359430256399806, 0.0009771253907250089001, 0.001172514838424378036, 0.001367904286123746956, 0.001563293733823115875 ),
 .UNSPECIFIED. ) ;
#28619=B_SPLINE_CURVE_WITH_KNOTS ( 'NONE', 3,
 ( #41766, #21029, #76876, #21481, #34111, #331, #83196, #15176, #6208, #48502 ),
 .UNSPECIFIED., .F., .F.,
 ( 4, 2, 2, 2, 4 ),
 ( 0.0007817359430256282712, 0.0009771253907249939381, 0.001172514838424359822, 0.001367904286123725489, 0.001563293733823091156 ),
 .UNSPECIFIED. ) ;
#28620=EDGE_CURVE ( 'NONE', #9998, #29143, #75260, .T. ) ;
#28621=CARTESIAN_POINT ( 'NONE',  ( 6.066068351002440906, -8.120952969808772792, 34.71129190929999453 ) ) ;
#28622=CARTESIAN_POINT ( 'NONE',  ( 2.241609928332172430, -11.91647553114624181, 32.58852847137148245 ) ) ;
#28623=DIRECTION ( 'NONE',  ( -0.000000000000000000, 0.8660254037844397068, -0.4999999999999978906 ) ) ;
#28625=CARTESIAN_POINT ( 'NONE',  ( -15.23076923076922995, -2.499999999999998668, 29.75000000000001421 ) ) ;
#28626=FACE_BOUND ( 'NONE', #9496, .T. ) ;
#28627=CYLINDRICAL_SURFACE ( 'NONE', #49074, 0.2500000000000008882 ) ;
#28628=DIRECTION ( 'NONE',  ( -0.000000000000000000, -0.000000000000000000, -1.000000000000000000 ) ) ;
#28629=CARTESIAN_POINT ( 'NONE',  ( -6.923076923077044142, -12.27809138561165270, 31.22303859784587132 ) ) ;
#28630=CARTESIAN_POINT ( 'NONE',  ( -9.019230769230768274, -7.500000000000001776, 35.00000000000000000 ) ) ;
#28632=CARTESIAN_POINT ( 'NONE',  ( -18.22348494372394967, -10.11188796281392221, 34.01382737946117629 ) ) ;
#28633=VECTOR ( 'NONE', #62735, 1000.000000000000000 ) ;
#28635=ORIENTED_EDGE ( 'NONE', *, *, #63136, .F. ) ;
#28636=DIRECTION ( 'NONE',  ( -0.000000000000000000, -0.6427876096865404731, -0.7660444431189771253 ) ) ;
#28637=ORIENTED_EDGE ( 'NONE', *, *, #75606, .F. ) ;
#28638=CARTESIAN_POINT ( 'NONE',  ( -18.00000000000000000, -11.35647404775217240, 33.31231777344666511 ) ) ;
#28639=VERTEX_POINT ( 'NONE', #43888 ) ;
#28640=EDGE_CURVE ( 'NONE', #25404, #33571, #84711, .T. ) ;
#28641=LINE ( 'NONE', #26862, #6684 ) ;
#28642=CARTESIAN_POINT ( 'NONE',  ( -18.06527044596078113, -2.625532179533445198, 30.86335684631481513 ) ) ;
#28643=ORIENTED_EDGE ( 'NONE', *, *, #1187, .T. ) ;
#28644=CARTESIAN_POINT ( 'NONE',  ( -9.915186374736338237, -7.630691491037285168, 34.74850469731152458 ) ) ;
#28646=CARTESIAN_POINT ( 'NONE',  ( -6.923076923076922462, -2.538708090699994813, 30.37095296980875503 ) ) ;
#28647=FACE_OUTER_BOUND ( 'NONE', #487, .T. ) ;
#28648=CARTESIAN_POINT ( 'NONE',  ( -5.207613680033387205, -2.845849958028613624, 32.17971566917920967 ) ) ;
#28650=CYLINDRICAL_SURFACE ( 'NONE', #41586, 0.2499999999999986955 ) ;
#28651=CARTESIAN_POINT ( 'NONE',  ( -13.63463860883684120, -12.07920672191015221, 32.31858351112116168 ) ) ;
#28653=CARTESIAN_POINT ( 'NONE',  ( -18.00000000000000000, -11.35647404775217240, 33.31231777344666511 ) ) ;
#28654=DIRECTION ( 'NONE',  ( 0.000000000000000000, 0.000000000000000000, 1.000000000000000000 ) ) ;
#28658=B_SPLINE_CURVE_WITH_KNOTS ( 'NONE', 3,
 ( #22775, #85378, #29550, #29989, #10605, #17814, #37625, #43501, #50685, #57005 ),
 .UNSPECIFIED., .F., .F.,
 ( 4, 2, 2, 2, 4 ),
 ( 0.0007817359430256288133, 0.0009771253907249948054, 0.001172514838424360689, 0.001367904286123726573, 0.001563293733823092457 ),
 .UNSPECIFIED. ) ;
#28659=AXIS2_PLACEMENT_3D ( 'NONE', #34846, #27211, #47471 ) ;
#28660=B_SPLINE_CURVE_WITH_KNOTS ( 'NONE', 3,
 ( #76815, #56089, #61953, #76358, #8355, #83584, #14219, #41253, #84026, #7908 ),
 .UNSPECIFIED., .F., .F.,
 ( 4, 2, 2, 2, 4 ),
 ( 0.0007817246256747517261, 0.0009771112852218961399, 0.001172497944769040771, 0.001367884604316185401, 0.001563271263863329815 ),
 .UNSPECIFIED. ) ;
#28661=CARTESIAN_POINT ( 'NONE',  ( -14.05774678934416499, -10.76462480002816235, 33.53768742498949962 ) ) ;
#28662=AXIS2_PLACEMENT_3D ( 'NONE', #44270, #25356, #38433 ) ;
#28663=VERTEX_POINT ( 'NONE', #29504 ) ;
#28664=CARTESIAN_POINT ( 'NONE',  ( 6.700198240648278514, -7.630691491037286056, 34.74850469731152458 ) ) ;
#28665=CARTESIAN_POINT ( 'NONE',  ( 12.46153846153846168, -8.164416787775445883, 34.95778746994557906 ) ) ;
#28666=CARTESIAN_POINT ( 'NONE',  ( 1.384615384615264011, -5.941354392335915335, 34.76329471203413846 ) ) ;
#28667=CARTESIAN_POINT ( 'NONE',  ( -14.53117725141625627, -11.89387501736622710, 32.13663884655806413 ) ) ;
#28668=B_SPLINE_CURVE_WITH_KNOTS ( 'NONE', 3,
 ( #25523, #73725, #31389, #12019, #24178, #40714, #68175, #6478, #33940, #85449 ),
 .UNSPECIFIED., .F., .F.,
 ( 4, 2, 2, 2, 4 ),
 ( 0.0007817246256747450040, 0.0009771112852218876831, 0.001172497944769030579, 0.001367884604316173258, 0.001563271263863315937 ),
 .UNSPECIFIED. ) ;
#28669=CARTESIAN_POINT ( 'NONE',  ( -16.28453762051371712, -10.54014554554151140, 33.71984207302941883 ) ) ;
#28670=CARTESIAN_POINT ( 'NONE',  ( 6.923076923076924238, -11.91647553114624181, 32.58852847137148245 ) ) ;
#28671=CIRCLE ( 'NONE', #65999, 0.2500000000000002220 ) ;
#28672=DIRECTION ( 'NONE',  ( 0.000000000000000000, 0.7660444431189807890, 0.6427876096865361433 ) ) ;
#28673=CARTESIAN_POINT ( 'NONE',  ( 10.48523664565292002, -12.70455904226513866, 30.44083106164009322 ) ) ;
#28674=ADVANCED_FACE ( 'NONE', ( #50190 ), #15100, .F. ) ;
#28675=EDGE_CURVE ( 'NONE', #79746, #45649, #84453, .T. ) ;
#28676=ORIENTED_EDGE ( 'NONE', *, *, #18711, .T. ) ;
#28677=VERTEX_POINT ( 'NONE', #57401 ) ;
#28678=ORIENTED_EDGE ( 'NONE', *, *, #750, .F. ) ;
#28679=FACE_OUTER_BOUND ( 'NONE', #11391, .T. ) ;
#28680=CARTESIAN_POINT ( 'NONE',  ( -6.673131404728781746, -4.336752205174647656, 33.62275283266504289 ) ) ;
#28681=CARTESIAN_POINT ( 'NONE',  ( -15.48079245499068435, -10.92453946501458795, 33.72985991061850086 ) ) ;
#28682=CARTESIAN_POINT ( 'NONE',  ( -13.25408968285181999, -12.27024696741798948, 31.24895572276497546 ) ) ;
#28683=CARTESIAN_POINT ( 'NONE',  ( 17.99999999999987566, -9.528491918059723176, 34.59228464037033035 ) ) ;
#28684=VERTEX_POINT ( 'NONE', #50642 ) ;
#28685=CARTESIAN_POINT ( 'NONE',  ( 17.32686848630112308, -11.56426240980093567, 33.07394671870546432 ) ) ;
#28686=ORIENTED_EDGE ( 'NONE', *, *, #80126, .T. ) ;
#28687=ORIENTED_EDGE ( 'NONE', *, *, #73060, .T. ) ;
#28688=B_SPLINE_CURVE_WITH_KNOTS ( 'NONE', 3,
 ( #63120, #43310, #44949, #10738, #82968, #62674 ),
 .UNSPECIFIED., .F., .F.,
 ( 4, 2, 4 ),
 ( 4.220987180333913997E-17, 0.0001954756301637150138, 0.0003909512603273878522 ),
 .UNSPECIFIED. ) ;
#28689=ORIENTED_EDGE ( 'NONE', *, *, #77924, .F. ) ;
#28690=CARTESIAN_POINT ( 'NONE',  ( 11.53846153846153832, -3.322132147404559976, 32.92929555188717927 ) ) ;
#28692=DIRECTION ( 'NONE',  ( -0.000000000000000000, 0.5000000000000011102, -0.8660254037844380415 ) ) ;
#28693=AXIS2_PLACEMENT_3D ( 'NONE', #19977, #68610, #83472 ) ;
#28694=CARTESIAN_POINT ( 'NONE',  ( 5.934729999443683290, -12.70778746994557551, 30.41441678777548319 ) ) ;
#28695=CARTESIAN_POINT ( 'NONE',  ( -9.692307692307691624, -8.120952969808772792, 34.71129190930000163 ) ) ;
#28696=CARTESIAN_POINT ( 'NONE',  ( 14.24193887937897607, -7.249945578846651806, 34.99404164642496795 ) ) ;
#28697=VERTEX_POINT ( 'NONE', #15988 ) ;
#28698=ORIENTED_EDGE ( 'NONE', *, *, #15165, .T. ) ;
#28701=CARTESIAN_POINT ( 'NONE',  ( 4.153846153846154188, -11.16473453929635440, 33.15142922261926373 ) ) ;
#28702=ORIENTED_EDGE ( 'NONE', *, *, #63735, .F. ) ;
#28703=CARTESIAN_POINT ( 'NONE',  ( 3.230769230769108269, -3.643525952248796163, 33.31231777344771672 ) ) ;
#28704=CARTESIAN_POINT ( 'NONE',  ( 9.692307692307695177, -11.69971097300155272, 32.46337939537588113 ) ) ;
#28705=CARTESIAN_POINT ( 'NONE',  ( 10.61538461538461675, -10.05456864172156806, 36.03766855953608683 ) ) ;
#28708=DIRECTION ( 'NONE',  ( -0.000000000000000000, 0.9396926207859092051, -0.3420201433256662704 ) ) ;
#28709=ORIENTED_EDGE ( 'NONE', *, *, #46650, .F. ) ;
#28710=FACE_BOUND ( 'NONE', #65841, .T. ) ;
#28711=CARTESIAN_POINT ( 'NONE',  ( 23.00000000000000000, -2.249999999999999556, 27.25000000000000000 ) ) ;
#28712=CARTESIAN_POINT ( 'NONE',  ( 16.15384615384603251, -2.657715359629662544, 31.77849191805970364 ) ) ;
#28713=CARTESIAN_POINT ( 'NONE',  ( 3.296837581771669079, -8.973038597847269315, 34.52809138561122637 ) ) ;
#28714=CYLINDRICAL_SURFACE ( 'NONE', #76283, 0.2499999999999973355 ) ;
#28715=VECTOR ( 'NONE', #43340, 1000.000000000000227 ) ;
#28718=CARTESIAN_POINT ( 'NONE',  ( -4.826977558574934157, -10.76462480002816235, 33.53768742498949962 ) ) ;
#28719=FACE_OUTER_BOUND ( 'NONE', #55116, .T. ) ;
#28720=ORIENTED_EDGE ( 'NONE', *, *, #72957, .F. ) ;
#28722=CARTESIAN_POINT ( 'NONE',  ( -6.000000000000121680, -11.67786785259630911, 32.92929555188603530 ) ) ;
#28723=AXIS2_PLACEMENT_3D ( 'NONE', #41374, #68837, #76931 ) ;
#28724=ORIENTED_EDGE ( 'NONE', *, *, #77870, .T. ) ;
#28725=EDGE_CURVE ( 'NONE', #75886, #40515, #768, .T. ) ;
#28726=VECTOR ( 'NONE', #84434, 1000.000000000000114 ) ;
#28728=AXIS2_PLACEMENT_3D ( 'NONE', #33200, #79166, #17468 ) ;
#28729=ADVANCED_FACE ( 'NONE', ( #86685 ), #38029, .F. ) ;
#28731=CARTESIAN_POINT ( 'NONE',  ( -15.93083480223330817, -10.61302985866384141, 33.66295027996417843 ) ) ;
#28732=CARTESIAN_POINT ( 'NONE',  ( 9.627037246346919375, -2.892918686051582533, 31.69288490824015980 ) ) ;
#28733=ORIENTED_EDGE ( 'NONE', *, *, #49892, .F. ) ;
#28734=CARTESIAN_POINT ( 'NONE',  ( -10.36533019547115941, -2.920487667080175598, 32.31805714834170828 ) ) ;
#28735=CARTESIAN_POINT ( 'NONE',  ( 4.219914504848593317, -9.780366693483667717, 34.19971097300155805 ) ) ;
#28736=FACE_BOUND ( 'NONE', #72097, .T. ) ;
#28737=CARTESIAN_POINT ( 'NONE',  ( 6.857806922520604864, -4.320704448112771878, 33.92786785259540494 ) ) ;
#28738=CARTESIAN_POINT ( 'NONE',  ( -3.931066612577743147, -8.496831190052096971, 34.64984203495476578 ) ) ;
#28739=CARTESIAN_POINT ( 'NONE',  ( 1.607628228708781970, -12.64618726649961289, 30.78989965857442712 ) ) ;
#28740=CARTESIAN_POINT ( 'NONE',  ( -3.007989689500819797, -11.89424750095246175, 32.13594075562311758 ) ) ;
#28745=ORIENTED_EDGE ( 'NONE', *, *, #13550, .F. ) ;
#28746=EDGE_CURVE ( 'NONE', #49489, #68389, #66834, .T. ) ;
#28748=CARTESIAN_POINT ( 'NONE',  ( -12.33101302330481808, -6.808710257144161559, 34.95449254468098843 ) ) ;
#28749=FACE_OUTER_BOUND ( 'NONE', #29095, .T. ) ;
#28751=EDGE_CURVE ( 'NONE', #6445, #46418, #29809, .T. ) ;
#28752=DIRECTION ( 'NONE',  ( -0.000000000000000000, -0.9848077530122086864, -0.1736481776669273613 ) ) ;
#28754=CARTESIAN_POINT ( 'NONE',  ( -12.59168643127016196, -4.299443229763728169, 33.91186481527756058 ) ) ;
#28755=CARTESIAN_POINT ( 'NONE',  ( 4.023698184114460119, -12.15440758774515473, 32.17923288041532004 ) ) ;
#28756=CARTESIAN_POINT ( 'NONE',  ( 9.562159722575998444, -11.04286588640298561, 33.62463336215343901 ) ) ;
#28758=LINE ( 'NONE', #36397, #82746 ) ;
#28760=B_SPLINE_CURVE_WITH_KNOTS ( 'NONE', 3,
 ( #47554, #41693, #54756, #69166, #61508, #89015, #48434, #7015, #42586, #26850 ),
 .UNSPECIFIED., .F., .F.,
 ( 4, 2, 2, 2, 4 ),
 ( 0.000000000000000000, 0.0001954311564186870371, 0.0003908623128373740741, 0.0005862934692560610840, 0.0007817246256747481482 ),
 .UNSPECIFIED. ) ;
#28761=CARTESIAN_POINT ( 'NONE',  ( -5.869209559033047086, -11.37503395064541678, 33.29242100308974983 ) ) ;
#28762=FACE_OUTER_BOUND ( 'NONE', #31559, .T. ) ;
#28763=EDGE_CURVE ( 'NONE', #19281, #77760, #81339, .T. ) ;
#28766=VECTOR ( 'NONE', #72488, 999.9999999999998863 ) ;
#28767=CARTESIAN_POINT ( 'NONE',  ( 4.023154687178596589, -4.809359713505814149, 33.96456829005828837 ) ) ;
#28768=CARTESIAN_POINT ( 'NONE',  ( 7.596130621932389637, -4.931416488878822335, 34.32920672191015399 ) ) ;
#28770=CARTESIAN_POINT ( 'NONE',  ( 0.4615384615383382183, -3.643525952248795718, 33.31231777344771672 ) ) ;
#28771=CARTESIAN_POINT ( 'NONE',  ( 16.82694633287449193, -11.47974371597207899, 33.17467449705390692 ) ) ;
#28772=ORIENTED_EDGE ( 'NONE', *, *, #56596, .F. ) ;
#28773=CARTESIAN_POINT ( 'NONE',  ( -9.915234651214538175, -5.582147617184174848, 34.63737895849758530 ) ) ;
#28774=LINE ( 'NONE', #21561, #56885 ) ;
#28775=VERTEX_POINT ( 'NONE', #85332 ) ;
#28776=CARTESIAN_POINT ( 'NONE',  ( 8.096099364501988305, -3.712312575010499494, 33.01462480002815170 ) ) ;
#28777=CARTESIAN_POINT ( 'NONE',  ( 0.4615384615384611200, -1.466349020453238561, 30.81389545987213907 ) ) ;
#28778=EDGE_LOOP ( 'NONE', ( #24530, #3788 ) ) ;
#28779=LINE ( 'NONE', #64309, #72171 ) ;
#28780=CARTESIAN_POINT ( 'NONE',  ( 13.31934538405906743, -9.528491918058357157, 34.59228464037090589 ) ) ;
#28781=VERTEX_POINT ( 'NONE', #23615 ) ;
#28783=CARTESIAN_POINT ( 'NONE',  ( -16.02332045208259004, -3.285477652293413264, 32.44071101563363158 ) ) ;
#28784=ADVANCED_FACE ( 'NONE', ( #51065 ), #24059, .F. ) ;
#28785=VECTOR ( 'NONE', #59079, 1000.000000000000000 ) ;
#28786=CARTESIAN_POINT ( 'NONE',  ( -9.562262529472915773, -2.504778602574660340, 29.97347330155780654 ) ) ;
#28787=VERTEX_POINT ( 'NONE', #17310 ) ;
#28788=ADVANCED_FACE ( 'NONE', ( #52863 ), #58734, .F. ) ;
#28789=ORIENTED_EDGE ( 'NONE', *, *, #20410, .T. ) ;
#28790=CARTESIAN_POINT ( 'NONE',  ( -10.48459417441766561, -2.295524264805589354, 30.44142389570982488 ) ) ;
#28791=VERTEX_POINT ( 'NONE', #10105 ) ;
#28793=EDGE_CURVE ( 'NONE', #17458, #48157, #44767, .T. ) ;
#28794=CARTESIAN_POINT ( 'NONE',  ( 15.36155967173618286, -12.62708834333097663, 30.88030960425257021 ) ) ;
#28795=CARTESIAN_POINT ( 'NONE',  ( -5.934744860487159102, -5.941354392334606160, 34.76329471203374055 ) ) ;
#28796=ADVANCED_FACE ( 'NONE', ( #24502 ), #51969, .F. ) ;
#28797=B_SPLINE_CURVE_WITH_KNOTS ( 'NONE', 3,
 ( #47316, #13101, #40581, #68049, #88780, #27056, #54517, #82009, #20305, #47766 ),
 .UNSPECIFIED., .F., .F.,
 ( 4, 2, 2, 2, 4 ),
 ( 0.000000000000000000, 0.0001954311564186870099, 0.0003908623128373740199, 0.0005862934692560609756, 0.0007817246256747480398 ),
 .UNSPECIFIED. ) ;
#28798=CARTESIAN_POINT ( 'NONE',  ( 17.07692307692307665, -1.242168528481310874, 33.36296068462461051 ) ) ;
#28799=B_SPLINE_CURVE_WITH_KNOTS ( 'NONE', 3,
 ( #80095, #80560, #72885, #11191, #53052, #4428, #39576, #59377, #5329, #19287 ),
 .UNSPECIFIED., .F., .F.,
 ( 4, 2, 2, 2, 4 ),
 ( 0.000000000000000000, 0.0001954311564186868473, 0.0003908623128373736946, 0.0005862934692560605419, 0.0007817246256747473893 ),
 .UNSPECIFIED. ) ;
#28800=CARTESIAN_POINT ( 'NONE',  ( -7.596153846152408740, -7.500000000000155431, 34.75000000000007105 ) ) ;
#28801=VECTOR ( 'NONE', #11813, 1000.000000000000114 ) ;
#28802=DIRECTION ( 'NONE',  ( 0.000000000000000000, 0.1736481776669275834, 0.9848077530122086864 ) ) ;
#28803=B_SPLINE_CURVE_WITH_KNOTS ( 'NONE', 3,
 ( #9479, #8161, #48688, #76164, #41950, #36521, #29323, #63969, #22114, #7723 ),
 .UNSPECIFIED., .F., .F.,
 ( 4, 2, 2, 2, 4 ),
 ( 0.000000000000000000, 0.0001954311564186868473, 0.0003908623128373736946, 0.0005862934692560605419, 0.0007817246256747473893 ),
 .UNSPECIFIED. ) ;
#28804=ORIENTED_EDGE ( 'NONE', *, *, #73089, .F. ) ;
#28807=ORIENTED_EDGE ( 'NONE', *, *, #85642, .T. ) ;
#28808=CARTESIAN_POINT ( 'NONE',  ( -5.207071046654775159, -5.070767119584671079, 34.40440758774516183 ) ) ;
#28809=ORIENTED_EDGE ( 'NONE', *, *, #15459, .F. ) ;
#28810=LINE ( 'NONE', #8090, #56484 ) ;
#28811=CARTESIAN_POINT ( 'NONE',  ( 6.857806922520603976, -9.528491918058357157, 34.59228464037090589 ) ) ;
#28812=EDGE_LOOP ( 'NONE', ( #55714, #4754 ) ) ;
#28813=LINE ( 'NONE', #83759, #45660 ) ;
#28814=ORIENTED_EDGE ( 'NONE', *, *, #82560, .F. ) ;
#28815=CARTESIAN_POINT ( 'NONE',  ( -6.857821351800899023, -11.48612834413965977, 32.76840700105972815 ) ) ;
#28816=VERTEX_POINT ( 'NONE', #18206 ) ;
#28817=CARTESIAN_POINT ( 'NONE',  ( -10.36538461538455103, -7.434744429011176159, 34.75000000000000711 ) ) ;
#28818=EDGE_CURVE ( 'NONE', #14974, #84688, #2825, .T. ) ;
#28819=ORIENTED_EDGE ( 'NONE', *, *, #19797, .F. ) ;
#28820=CARTESIAN_POINT ( 'NONE',  ( 17.75002326905764960, -10.66389620160130036, 33.62221079203477103 ) ) ;
#28821=B_SPLINE_CURVE_WITH_KNOTS ( 'NONE', 3,
 ( #64986, #37977, #53254, #3291, #19039, #25348, #80756, #66780, #30766, #58681 ),
 .UNSPECIFIED., .F., .F.,
 ( 4, 2, 2, 2, 4 ),
 ( 0.0007817246256747491240, 0.0009771112852218931041, 0.001172497944769036867, 0.001367884604316180631, 0.001563271263863324611 ),
 .UNSPECIFIED. ) ;
#28822=VECTOR ( 'NONE', #72379, 1000.000000000000000 ) ;
#28823=CARTESIAN_POINT ( 'NONE',  ( 17.99999999999987566, -12.51329471203414379, 31.30864560766407578 ) ) ;
#28824=FACE_BOUND ( 'NONE', #41706, .T. ) ;
#28825=B_SPLINE_CURVE_WITH_KNOTS ( 'NONE', 3,
 ( #40648, #16266, #85175, #57693, #36543, #70772, #15833, #83408, #35661, #41978 ),
 .UNSPECIFIED., .F., .F.,
 ( 4, 2, 2, 2, 4 ),
 ( 0.000000000000000000, 0.0001954311564186867931, 0.0003908623128373735862, 0.0005862934692560603251, 0.0007817246256747471724 ),
 .UNSPECIFIED. ) ;
#28827=DIRECTION ( 'NONE',  ( -1.000000000000000000, 0.000000000000000000, 0.000000000000000000 ) ) ;
#28828=DIRECTION ( 'NONE',  ( -0.000000000000000000, 1.000000000000000000, 3.491481338843133355E-15 ) ) ;
#28829=CARTESIAN_POINT ( 'NONE',  ( -0.4615384615384611200, -2.833524468853757305, 32.15551576947925838 ) ) ;
#28830=CARTESIAN_POINT ( 'NONE',  ( 5.299934428535924447, -10.61302985866383963, 33.66295027996417843 ) ) ;
#28831=CARTESIAN_POINT ( 'NONE',  ( -9.757557624081776737, -2.255955759149247619, 30.00000000000013856 ) ) ;
#28832=ORIENTED_EDGE ( 'NONE', *, *, #23073, .F. ) ;
#28833=CARTESIAN_POINT ( 'NONE',  ( 15.23076923076923173, -1.466349020453238561, 30.81389545987213907 ) ) ;
#28834=ORIENTED_EDGE ( 'NONE', *, *, #29112, .T. ) ;
#28835=ORIENTED_EDGE ( 'NONE', *, *, #9287, .T. ) ;
#28836=EDGE_CURVE ( 'NONE', #83181, #19489, #71580, .T. ) ;
#28837=DIRECTION ( 'NONE',  ( 0.000000000000000000, 0.4999999999999985567, 0.8660254037844395958 ) ) ;
#28838=CARTESIAN_POINT ( 'NONE',  ( 8.068933387422251968, -10.11255958852956027, 34.01340905677048454 ) ) ;
#28839=CYLINDRICAL_SURFACE ( 'NONE', #35571, 0.2499999999999995559 ) ;
#28840=CARTESIAN_POINT ( 'NONE',  ( 17.07692307692307665, -5.415277668671390821, 36.20867863119892149 ) ) ;
#28841=CYLINDRICAL_SURFACE ( 'NONE', #34390, 0.2500000000000002220 ) ;
#28842=CARTESIAN_POINT ( 'NONE',  ( 9.915319043920543862, -2.554770724473668153, 30.48948780036025852 ) ) ;
#28843=ORIENTED_EDGE ( 'NONE', *, *, #14594, .F. ) ;
#28844=CARTESIAN_POINT ( 'NONE',  ( 1.384615384615264011, -5.094484230521993062, 34.41647553114689373 ) ) ;
#28845=CARTESIAN_POINT ( 'NONE',  ( 16.40384615384615330, -2.499999999999998668, 29.75000000000000355 ) ) ;
#28846=CARTESIAN_POINT ( 'NONE',  ( -12.52680846209478460, -11.67786785259540849, 32.92929555188721480 ) ) ;
#28847=VECTOR ( 'NONE', #15753, 1000.000000000000114 ) ;
#28848=CARTESIAN_POINT ( 'NONE',  ( -8.546217925137375104, -2.523321265292115534, 31.42251411153756990 ) ) ;
#28849=CARTESIAN_POINT ( 'NONE',  ( 13.51540582558234149, -5.496552790871120031, 34.60292014791297532 ) ) ;
#28850=EDGE_LOOP ( 'NONE', ( #17470, #59075 ) ) ;
#28851=B_SPLINE_CURVE_WITH_KNOTS ( 'NONE', 3,
 ( #301, #1179, #69202, #41736, #742, #14704, #61546, #27330, #7946, #35411 ),
 .UNSPECIFIED., .F., .F.,
 ( 4, 2, 2, 2, 4 ),
 ( 0.0007817246256747469556, 0.0009771112852218889842, 0.001172497944769031013, 0.001367884604316173041, 0.001563271263863315070 ),
 .UNSPECIFIED. ) ;
#28852=VERTEX_POINT ( 'NONE', #81245 ) ;
#28853=VECTOR ( 'NONE', #24748, 1000.000000000000114 ) ;
#28854=VECTOR ( 'NONE', #30263, 1000.000000000000227 ) ;
#28856=ADVANCED_FACE ( 'NONE', ( #81688 ), #6029, .F. ) ;
#28857=FACE_OUTER_BOUND ( 'NONE', #79984, .T. ) ;
#28858=ORIENTED_EDGE ( 'NONE', *, *, #17944, .T. ) ;
#28859=CARTESIAN_POINT ( 'NONE',  ( -1.254089682851820431, -8.586989748646450593, 34.63063291749215011 ) ) ;
#28860=CARTESIAN_POINT ( 'NONE',  ( -12.21148414990014786, -6.567000820036036579, 34.66262288849541306 ) ) ;
#28861=CARTESIAN_POINT ( 'NONE',  ( 14.05766908347085575, -10.18141759479407327, 34.26406193332782379 ) ) ;
#28862=ADVANCED_FACE ( 'NONE', ( #69824 ), #19968, .F. ) ;
#28863=CARTESIAN_POINT ( 'NONE',  ( -12.46153846153858424, -3.083524468854526912, 32.58852847137268327 ) ) ;
#28864=CARTESIAN_POINT ( 'NONE',  ( -16.85414353565465717, -12.24180327182771855, 31.33663988360758168 ) ) ;
#28865=VECTOR ( 'NONE', #65969, 1000.000000000000227 ) ;
#28866=VECTOR ( 'NONE', #18309, 1000.000000000000227 ) ;
#28867=DIRECTION ( 'NONE',  ( 0.000000000000000000, 0.7660444431189822323, -0.6427876096865344779 ) ) ;
#28868=EDGE_LOOP ( 'NONE', ( #63705, #35235 ) ) ;
#28869=CARTESIAN_POINT ( 'NONE',  ( 11.53846153846184563, -2.506253911140615021, 30.00000000000323297 ) ) ;
#28870=CARTESIAN_POINT ( 'NONE',  ( -13.16183584334697265, -4.387253974876679230, 33.66317474335728832 ) ) ;
#28871=ORIENTED_EDGE ( 'NONE', *, *, #32246, .F. ) ;
#28872=CARTESIAN_POINT ( 'NONE',  ( -9.692307692307812417, -4.481592998941358097, 33.73612834414048933 ) ) ;
#28873=LINE ( 'NONE', #50005, #71273 ) ;
#28874=CARTESIAN_POINT ( 'NONE',  ( -0.5268084620947807162, -4.320704448112771878, 33.92786785259540494 ) ) ;
#28875=CARTESIAN_POINT ( 'NONE',  ( -17.77722045873159473, -11.89424750095246175, 32.13594075562311758 ) ) ;
#28876=CARTESIAN_POINT ( 'NONE',  ( -2.084912638714239375, -2.353885683473778023, 30.79025554430704759 ) ) ;
#28877=CARTESIAN_POINT ( 'NONE',  ( -11.53846153846153655, -1.951392089020283160, 34.73218667398347748 ) ) ;
#28878=EDGE_CURVE ( 'NONE', #50472, #42433, #19531, .T. ) ;
#28879=CARTESIAN_POINT ( 'NONE',  ( -0.4615384615384611200, -12.78798330534102767, 29.49999999999997868 ) ) ;
#28881=ORIENTED_EDGE ( 'NONE', *, *, #7546, .T. ) ;
#28882=B_SPLINE_CURVE_WITH_KNOTS ( 'NONE', 3,
 ( #1962, #2826, #56463, #22232, #50579, #30317, #71290, #29445, #9596, #43392 ),
 .UNSPECIFIED., .F., .F.,
 ( 4, 2, 2, 2, 4 ),
 ( 0.0007817359430256294638, 0.0009771253907249974075, 0.001172514838424365243, 0.001367904286123733078, 0.001563293733823093758 ),
 .UNSPECIFIED. ) ;
#28883=CARTESIAN_POINT ( 'NONE',  ( -15.45369618967607828, -6.459968553980841577, 34.89616026154728701 ) ) ;
#28884=CARTESIAN_POINT ( 'NONE',  ( -1.384615384615383471, -12.10708131394839349, 31.69288490824020244 ) ) ;
#28886=CARTESIAN_POINT ( 'NONE',  ( 8.992243613324164997, -10.77377354290276124, 33.85451476688484718 ) ) ;
#28887=CARTESIAN_POINT ( 'NONE',  ( -3.230769230769229949, -10.67929555188718282, 33.92786785259544047 ) ) ;
#28888=ORIENTED_EDGE ( 'NONE', *, *, #9067, .T. ) ;
#28889=CARTESIAN_POINT ( 'NONE',  ( 0.3962684609821418569, -4.320704448112772766, 33.92786785259541915 ) ) ;
#28890=CARTESIAN_POINT ( 'NONE',  ( -2.307692307692305711, -3.050289026998446396, 32.03036669348365706 ) ) ;
#28891=EDGE_CURVE ( 'NONE', #13555, #35423, #52282, .T. ) ;
#28892=ORIENTED_EDGE ( 'NONE', *, *, #76620, .T. ) ;
#28893=CARTESIAN_POINT ( 'NONE',  ( 1.318531973659506251, -8.973038597847271092, 34.52809138561120506 ) ) ;
#28894=CARTESIAN_POINT ( 'NONE',  ( -4.403869391139117795, -10.76384336483936011, 33.53834819971076087 ) ) ;
#28895=VERTEX_POINT ( 'NONE', #74478 ) ;
#28896=CARTESIAN_POINT ( 'NONE',  ( -15.48079246806219267, -2.823816976329319051, 31.52131813110795733 ) ) ;
#28897=CARTESIAN_POINT ( 'NONE',  ( 3.903869422903798458, -3.627789207965226748, 32.91389620160131102 ) ) ;
#28899=CARTESIAN_POINT ( 'NONE',  ( -0.6844654204453110014, -10.01117774369187252, 34.36070679894347535 ) ) ;
#28900=CYLINDRICAL_SURFACE ( 'NONE', #39358, 0.2500000000000009437 ) ;
#28901=VECTOR ( 'NONE', #57113, 1000.000000000000227 ) ;
#28902=ORIENTED_EDGE ( 'NONE', *, *, #46860, .T. ) ;
#28903=CARTESIAN_POINT ( 'NONE',  ( -3.007989561791163613, -2.353885683473778023, 30.79025554430704759 ) ) ;
#28904=EDGE_CURVE ( 'NONE', #52308, #18841, #15773, .T. ) ;
#28905=B_SPLINE_CURVE_WITH_KNOTS ( 'NONE', 3,
 ( #34245, #6772, #41013, #55845, #83332, #75671, #14418, #1787, #68472, #76569 ),
 .UNSPECIFIED., .F., .F.,
 ( 4, 2, 2, 2, 4 ),
 ( 0.0007817246256747473893, 0.0009771112852218909357, 0.001172497944769034482, 0.001367884604316178246, 0.001563271263863321792 ),
 .UNSPECIFIED. ) ;
#28906=ORIENTED_EDGE ( 'NONE', *, *, #84053, .F. ) ;
#28907=DIRECTION ( 'NONE',  ( -0.000000000000000000, 0.9848077530122086864, -0.1736481776669273891 ) ) ;
#28908=DIRECTION ( 'NONE',  ( 0.000000000000000000, 0.9848077530122072432, 0.1736481776669354937 ) ) ;
#28909=EDGE_LOOP ( 'NONE', ( #77024, #83685 ) ) ;
#28911=DIRECTION ( 'NONE',  ( 0.000000000000000000, 0.8660254037844377084, 0.5000000000000015543 ) ) ;
#28912=CARTESIAN_POINT ( 'NONE',  ( -8.899377978668987055, -2.619462340734462380, 30.83744416345203021 ) ) ;
#28913=CARTESIAN_POINT ( 'NONE',  ( 0.2115617305961063344, -4.236021600441995716, 33.53823185664188600 ) ) ;
#28914=CARTESIAN_POINT ( 'NONE',  ( 13.60739505359345181, -12.11081565061823717, 32.26097654155341843 ) ) ;
#28915=CARTESIAN_POINT ( 'NONE',  ( -8.096153846153844924, -7.500000000000001776, 34.75000000000000000 ) ) ;
#28917=ORIENTED_EDGE ( 'NONE', *, *, #7836, .T. ) ;
#28918=VECTOR ( 'NONE', #71349, 1000.000000000000000 ) ;
#28919=FACE_BOUND ( 'NONE', #27512, .T. ) ;
#28920=ORIENTED_EDGE ( 'NONE', *, *, #17507, .F. ) ;
#28921=CARTESIAN_POINT ( 'NONE',  ( -8.069080805060693251, -5.582147617184174848, 34.63737895849758530 ) ) ;
#28922=EDGE_CURVE ( 'NONE', #11473, #47875, #20462, .T. ) ;
#28923=CARTESIAN_POINT ( 'NONE',  ( 4.284371855609720114, -11.93748526763465279, 32.05452791011430946 ) ) ;
#28924=EDGE_CURVE ( 'NONE', #66677, #63245, #61433, .T. ) ;
#28925=CARTESIAN_POINT ( 'NONE',  ( -11.53846153846153655, -1.367168528481310208, 33.57946703557072254 ) ) ;
#28926=CARTESIAN_POINT ( 'NONE',  ( -2.084679463598911653, -10.01129605718032778, 34.36064277460058491 ) ) ;
#28928=ORIENTED_EDGE ( 'NONE', *, *, #51658, .F. ) ;
#28929=VERTEX_POINT ( 'NONE', #53796 ) ;
#28930=VERTEX_POINT ( 'NONE', #27654 ) ;
#28931=CARTESIAN_POINT ( 'NONE',  ( 13.31929137181107947, -7.749976730030849303, 34.74374725381503737 ) ) ;
#28933=ADVANCED_FACE ( 'NONE', ( #74972 ), #41618, .F. ) ;
#28934=DIRECTION ( 'NONE',  ( -0.000000000000000000, -0.9396926207859093161, -0.3420201433256663259 ) ) ;
#28935=CARTESIAN_POINT ( 'NONE',  ( -2.557669051740897093, -12.41104346484419452, 31.60698883733904196 ) ) ;
#28936=EDGE_CURVE ( 'NONE', #33889, #51136, #85634, .T. ) ;
#28937=CARTESIAN_POINT ( 'NONE',  ( 13.60762822870878530, -11.43677907613344757, 33.22367315496202167 ) ) ;
#28939=CARTESIAN_POINT ( 'NONE',  ( -8.703163435880695076, -3.937682226553329556, 33.60647404775216529 ) ) ;
#28940=EDGE_CURVE ( 'NONE', #2419, #24282, #11468, .T. ) ;
#28941=CYLINDRICAL_SURFACE ( 'NONE', #85041, 0.2499999999999995559 ) ;
#28942=CARTESIAN_POINT ( 'NONE',  ( 6.000000000000001776, -13.88283147151868846, 33.14645433367849847 ) ) ;
#28944=EDGE_LOOP ( 'NONE', ( #31878, #65083 ) ) ;
#28945=ORIENTED_EDGE ( 'NONE', *, *, #47745, .F. ) ;
#28947=LINE ( 'NONE', #55067, #73283 ) ;
#28948=EDGE_CURVE ( 'NONE', #70346, #74779, #68410, .T. ) ;
#28950=CARTESIAN_POINT ( 'NONE',  ( 10.74617642320940369, -6.413143153341454017, 34.63066358083362672 ) ) ;
#28951=VECTOR ( 'NONE', #19472, 999.9999999999998863 ) ;
#28952=CARTESIAN_POINT ( 'NONE',  ( -17.77698715590659972, -5.582272713120728369, 34.63742843783360570 ) ) ;
#28953=CARTESIAN_POINT ( 'NONE',  ( -8.992715693795101828, -6.716662450894489211, 34.94144148231605840 ) ) ;
#28954=FACE_BOUND ( 'NONE', #62597, .T. ) ;
#28955=CARTESIAN_POINT ( 'NONE',  ( 8.703960768674447124, -11.06231777344662781, 33.60647404775220082 ) ) ;
#28956=ORIENTED_EDGE ( 'NONE', *, *, #25762, .T. ) ;
#28957=CARTESIAN_POINT ( 'NONE',  ( -8.069033362891428141, -7.630690623152299068, 34.99857592706772635 ) ) ;
#28960=CARTESIAN_POINT ( 'NONE',  ( -17.07692307692319744, -2.657715359629662988, 31.77849191805970364 ) ) ;
#28961=ORIENTED_EDGE ( 'NONE', *, *, #40453, .F. ) ;
#28962=CARTESIAN_POINT ( 'NONE',  ( 2.557746619330622639, -11.79725096376909654, 32.30694842903960762 ) ) ;
#28963=ORIENTED_EDGE ( 'NONE', *, *, #5993, .F. ) ;
#28964=FACE_BOUND ( 'NONE', #64107, .T. ) ;
#28966=CARTESIAN_POINT ( 'NONE',  ( 16.94623161025552349, -11.71456829005830080, 32.44064028649416542 ) ) ;
#28967=CARTESIAN_POINT ( 'NONE',  ( -11.47320596718551577, -11.94971097300157403, 32.03036669348361443 ) ) ;
#28968=VERTEX_POINT ( 'NONE', #56459 ) ;
#28969=CARTESIAN_POINT ( 'NONE',  ( -12.52680890749923570, -10.21337939537584383, 33.94971097300158647 ) ) ;
#28970=CARTESIAN_POINT ( 'NONE',  ( -5.777220331021931443, -9.418065098278011860, 34.63729479722530158 ) ) ;
#28971=CARTESIAN_POINT ( 'NONE',  ( -15.16551409125639260, -10.33852847137154107, 34.16647553114620450 ) ) ;
#28972=EDGE_CURVE ( 'NONE', #8816, #15450, #87738, .T. ) ;
#28973=FACE_OUTER_BOUND ( 'NONE', #10985, .T. ) ;
#28975=B_SPLINE_CURVE_WITH_KNOTS ( 'NONE', 3,
 ( #13175, #40655, #68124, #33881, #61338, #57260, #69886, #2739, #71205, #70780 ),
 .UNSPECIFIED., .F., .F.,
 ( 4, 2, 2, 2, 4 ),
 ( 0.0007817359430256313069, 0.0009771253907249971907, 0.001172514838424363074, 0.001367904286123728958, 0.001563293733823094842 ),
 .UNSPECIFIED. ) ;
#28976=CARTESIAN_POINT ( 'NONE',  ( 16.21910172512217585, -10.90142922261932057, 33.41473453929631887 ) ) ;
#28978=CARTESIAN_POINT ( 'NONE',  ( 4.153846153846154188, -2.833524468853757305, 32.15551576947925838 ) ) ;
#28979=ORIENTED_EDGE ( 'NONE', *, *, #11645, .F. ) ;
#28980=CARTESIAN_POINT ( 'NONE',  ( -8.704084989898801084, -7.750023238201979581, 34.74374492549440419 ) ) ;
#28981=CARTESIAN_POINT ( 'NONE',  ( -1.384615384615506484, -12.51329471203414379, 31.30864560766407578 ) ) ;
#28982=CARTESIAN_POINT ( 'NONE',  ( -13.38461538461538325, -13.49023893513002648, 31.06009739812518688 ) ) ;
#28983=CARTESIAN_POINT ( 'NONE',  ( -12.59222906464877134, -10.70098750199973203, 33.91152734681376302 ) ) ;
#28984=CARTESIAN_POINT ( 'NONE',  ( -5.750054590621955342, -6.653508905675592722, 34.93172785388651391 ) ) ;
#28985=CARTESIAN_POINT ( 'NONE',  ( 0.3309281019139320157, -7.722926236386453702, 34.74524107206102030 ) ) ;
#28987=CARTESIAN_POINT ( 'NONE',  ( 0.4615384615384611200, -13.49023893513002648, 31.06009739812518688 ) ) ;
#28990=CARTESIAN_POINT ( 'NONE',  ( -8.769230769230892619, -10.33852847137269571, 34.16647553114546554 ) ) ;
#28991=ORIENTED_EDGE ( 'NONE', *, *, #64087, .F. ) ;
#28992=VECTOR ( 'NONE', #26503, 1000.000000000000227 ) ;
#28993=ORIENTED_EDGE ( 'NONE', *, *, #69226, .T. ) ;
#28994=CARTESIAN_POINT ( 'NONE',  ( 11.76124107972994537, -11.89424750095246175, 32.13594075562310337 ) ) ;
#28995=EDGE_LOOP ( 'NONE', ( #70767, #88643 ) ) ;
#28996=CARTESIAN_POINT ( 'NONE',  ( -10.74607608205217346, -11.18331474514187995, 33.13161551792790505 ) ) ;
#28997=CARTESIAN_POINT ( 'NONE',  ( -5.010855743573001675, -12.62096338111211757, 30.90682066428152908 ) ) ;
#28998=AXIS2_PLACEMENT_3D ( 'NONE', #7019, #54313, #13775 ) ;
#28999=LINE ( 'NONE', #49692, #55722 ) ;
#29000=CARTESIAN_POINT ( 'NONE',  ( -3.230769230769229949, -5.415277668671390821, 36.20867863119892149 ) ) ;
#29002=CARTESIAN_POINT ( 'NONE',  ( 15.90386942290380290, -11.79746400365624659, 32.30657167506340954 ) ) ;
#29003=CARTESIAN_POINT ( 'NONE',  ( -15.10024379253558635, -8.630441415882550871, 34.87705825610312615 ) ) ;
#29004=CARTESIAN_POINT ( 'NONE',  ( 10.54930120442873331, -2.538708090699994813, 30.37095296980875148 ) ) ;
#29005=CARTESIAN_POINT ( 'NONE',  ( 11.47237812750565666, -10.51840700105979387, 33.73612834413961536 ) ) ;
#29006=ADVANCED_FACE ( 'NONE', ( #10032 ), #77614, .F. ) ;
#29007=CARTESIAN_POINT ( 'NONE',  ( -5.076923076923075762, -13.20930481340135110, 34.54067556320372745 ) ) ;
#29008=CARTESIAN_POINT ( 'NONE',  ( 7.780883845597524662, -2.379036618887870436, 30.90682066428147579 ) ) ;
#29009=EDGE_CURVE ( 'NONE', #61557, #48093, #12589, .T. ) ;
#29010=ORIENTED_EDGE ( 'NONE', *, *, #77281, .F. ) ;
#29011=VERTEX_POINT ( 'NONE', #42952 ) ;
#29012=B_SPLINE_CURVE_WITH_KNOTS ( 'NONE', 3,
 ( #5502, #5945, #27539, #32966, #33848, #60431, #40620, #33415, #87947, #26206 ),
 .UNSPECIFIED., .F., .F.,
 ( 4, 2, 2, 2, 4 ),
 ( 0.000000000000000000, 0.0001954311564186865492, 0.0003908623128373730983, 0.0005862934692560596746, 0.0007817246256747461966 ),
 .UNSPECIFIED. ) ;
#29013=DIRECTION ( 'NONE',  ( -0.000000000000000000, 0.8660254037844399289, -0.4999999999999980016 ) ) ;
#29015=CARTESIAN_POINT ( 'NONE',  ( 11.53846153846141753, -10.21337939537710326, 33.94971097300076224 ) ) ;
#29016=DIRECTION ( 'NONE',  ( 0.000000000000000000, 0.8660254037844377084, -0.5000000000000015543 ) ) ;
#29017=EDGE_LOOP ( 'NONE', ( #74252, #86234, #60031, #78735 ) ) ;
#29018=ADVANCED_FACE ( 'NONE', ( #8725 ), #63650, .F. ) ;
#29019=DIRECTION ( 'NONE',  ( -0.000000000000000000, 0.7660444431189791237, -0.6427876096865379196 ) ) ;
#29020=CARTESIAN_POINT ( 'NONE',  ( -17.07692307692307665, -3.513871655860378418, 32.76840700105978499 ) ) ;
#29021=ADVANCED_FACE ( 'NONE', ( #71284 ), #26389, .F. ) ;
#29023=ORIENTED_EDGE ( 'NONE', *, *, #69534, .T. ) ;
#29024=CARTESIAN_POINT ( 'NONE',  ( -14.37296230824862775, -12.70778746994557551, 30.41441678777548319 ) ) ;
#29025=ORIENTED_EDGE ( 'NONE', *, *, #87416, .T. ) ;
#29026=AXIS2_PLACEMENT_3D ( 'NONE', #48365, #62756, #1073 ) ;
#29027=ADVANCED_FACE ( 'NONE', ( #1956 ), #43386, .F. ) ;
#29029=DIRECTION ( 'NONE',  ( 0.000000000000000000, 0.9396926207859126468, 0.3420201433256571111 ) ) ;
#29030=CARTESIAN_POINT ( 'NONE',  ( 16.82692307692307665, -2.499999999999998668, 29.75000000000000355 ) ) ;
#29032=DIRECTION ( 'NONE',  ( 0.000000000000000000, 0.1736481776669267785, -0.9848077530122087975 ) ) ;
#29033=ORIENTED_EDGE ( 'NONE', *, *, #33731, .F. ) ;
#29034=ORIENTED_EDGE ( 'NONE', *, *, #82822, .F. ) ;
#29035=ORIENTED_EDGE ( 'NONE', *, *, #60852, .F. ) ;
#29036=B_SPLINE_CURVE_WITH_KNOTS ( 'NONE', 3,
 ( #7905, #56965, #22736, #42144, #84023, #35369, #84461, #2898, #43019, #29952 ),
 .UNSPECIFIED., .F., .F.,
 ( 4, 2, 2, 2, 4 ),
 ( 0.000000000000000000, 0.0001954339857564070678, 0.0003908679715128141356, 0.0005863019572692211492, 0.0007817359430256282712 ),
 .UNSPECIFIED. ) ;
#29037=CARTESIAN_POINT ( 'NONE',  ( -10.61538461538473577, -12.51329471203414379, 31.30864560766407578 ) ) ;
#29038=DIRECTION ( 'NONE',  ( 0.000000000000000000, 0.6427876096865373645, -0.7660444431189797898 ) ) ;
#29039=ADVANCED_FACE ( 'NONE', ( #23110 ), #85263, .F. ) ;
#29040=CARTESIAN_POINT ( 'NONE',  ( 0.7115928814519136836, -6.523592122091590895, 34.90882529074906415 ) ) ;
#29041=VECTOR ( 'NONE', #49431, 1000.000000000000000 ) ;
#29042=CARTESIAN_POINT ( 'NONE',  ( 0.2386115026316116827, -12.38737895849757820, 31.66785238281580206 ) ) ;
#29043=VECTOR ( 'NONE', #18159, 1000.000000000000227 ) ;
#29044=LINE ( 'NONE', #62790, #11946 ) ;
#29046=ORIENTED_EDGE ( 'NONE', *, *, #48198, .F. ) ;
#29047=ORIENTED_EDGE ( 'NONE', *, *, #36159, .T. ) ;
#29048=AXIS2_PLACEMENT_3D ( 'NONE', #7499, #8830, #2060 ) ;
#29050=CARTESIAN_POINT ( 'NONE',  ( 16.15384615384615330, -4.661471528628507777, 34.16647553114623292 ) ) ;
#29051=EDGE_CURVE ( 'NONE', #2574, #30732, #42508, .T. ) ;
#29052=ORIENTED_EDGE ( 'NONE', *, *, #1961, .T. ) ;
#29053=CARTESIAN_POINT ( 'NONE',  ( -13.38461538461538325, -10.89733346790207413, 36.13435417666054406 ) ) ;
#29055=CARTESIAN_POINT ( 'NONE',  ( -2.307692307692305711, -8.973038597847269315, 34.52809138561121927 ) ) ;
#29057=ORIENTED_EDGE ( 'NONE', *, *, #89162, .F. ) ;
#29058=EDGE_CURVE ( 'NONE', #58205, #33472, #44240, .T. ) ;
#29059=VERTEX_POINT ( 'NONE', #83499 ) ;
#29060=CARTESIAN_POINT ( 'NONE',  ( 13.51540582558233794, -10.70102852606553157, 33.91149625220312913 ) ) ;
#29061=ORIENTED_EDGE ( 'NONE', *, *, #77155, .F. ) ;
#29062=FACE_BOUND ( 'NONE', #10007, .T. ) ;
#29063=CARTESIAN_POINT ( 'NONE',  ( 6.673100192134569397, -4.236021600441998380, 33.53823185664189310 ) ) ;
#29064=CARTESIAN_POINT ( 'NONE',  ( -4.403822897894744237, -10.06842814019191401, 34.32929386961144758 ) ) ;
#29065=VERTEX_POINT ( 'NONE', #21785 ) ;
#29067=DIRECTION ( 'NONE',  ( 0.000000000000000000, 0.4999999999999985567, 0.8660254037844395958 ) ) ;
#29068=DIRECTION ( 'NONE',  ( -0.000000000000000000, -0.3420201433256694346, -0.9396926207859080948 ) ) ;
#29069=CARTESIAN_POINT ( 'NONE',  ( 4.088575707885378385, -11.48612834413959582, 32.76840700105983473 ) ) ;
#29070=CARTESIAN_POINT ( 'NONE',  ( -17.01166750564705410, -2.625532179533469623, 30.86335684631491105 ) ) ;
#29071=EDGE_CURVE ( 'NONE', #29311, #16242, #41621, .T. ) ;
#29074=CARTESIAN_POINT ( 'NONE',  ( 6.250054311638317373, -8.303483539816728154, 34.68545999027711702 ) ) ;
#29075=LINE ( 'NONE', #70488, #59877 ) ;
#29076=DIRECTION ( 'NONE',  ( -0.000000000000000000, 0.7660444431189791237, -0.6427876096865379196 ) ) ;
#29077=CARTESIAN_POINT ( 'NONE',  ( -0.7115616857599184053, -4.931416488878823223, 34.32920672191015399 ) ) ;
#29079=CARTESIAN_POINT ( 'NONE',  ( -14.98082371242109012, -11.86320923018887541, 32.19269448109604781 ) ) ;
#29080=ADVANCED_FACE ( 'NONE', ( #86606 ), #24877, .F. ) ;
#29081=CARTESIAN_POINT ( 'NONE',  ( 15.23076923076910916, -8.656820664282941280, 34.87096338111179961 ) ) ;
#29082=CARTESIAN_POINT ( 'NONE',  ( 13.13459214732242408, -11.86270091957321249, 32.19358267280087915 ) ) ;
#29083=FACE_OUTER_BOUND ( 'NONE', #58780, .T. ) ;
#29084=CARTESIAN_POINT ( 'NONE',  ( -14.37296230824862775, -3.643525952247789412, 33.31231777344662959 ) ) ;
#29085=FACE_OUTER_BOUND ( 'NONE', #45991, .T. ) ;
#29086=CARTESIAN_POINT ( 'NONE',  ( 2.438217745925953750, -6.808710257144159783, 34.95449254468098843 ) ) ;
#29087=AXIS2_PLACEMENT_3D ( 'NONE', #65872, #36318, #43508 ) ;
#29088=CARTESIAN_POINT ( 'NONE',  ( -5.750054481651856619, -12.43552623307873972, 30.55307653245132826 ) ) ;
#29090=ADVANCED_FACE ( 'NONE', ( #73072 ), #87057, .F. ) ;
#29092=CARTESIAN_POINT ( 'NONE',  ( 12.71159277317677549, -2.564540009722896752, 30.55348353981670684 ) ) ;
#29093=ORIENTED_EDGE ( 'NONE', *, *, #35371, .F. ) ;
#29094=CARTESIAN_POINT ( 'NONE',  ( -13.31936024510254413, -9.528491918058460186, 34.59228464037086326 ) ) ;
#29095=EDGE_LOOP ( 'NONE', ( #25253, #67430, #47826, #34014 ) ) ;
#29096=CARTESIAN_POINT ( 'NONE',  ( 15.90386942290380290, -11.28823185664190376, 33.01397839955799896 ) ) ;
#29099=CARTESIAN_POINT ( 'NONE',  ( -18.24997673094235751, -12.41269422305637171, 30.68257228309993323 ) ) ;
#29101=CYLINDRICAL_SURFACE ( 'NONE', #9867, 0.2499999999999995559 ) ;
#29102=CARTESIAN_POINT ( 'NONE',  ( -3.930470668073732909, -2.251407671071270489, 29.88021292934942252 ) ) ;
#29103=CARTESIAN_POINT ( 'NONE',  ( 15.93091919493930320, -8.282780595021769443, 34.94152052738834868 ) ) ;
#29104=CARTESIAN_POINT ( 'NONE',  ( 17.99999999999987566, -2.625532179533778709, 30.86335684631627174 ) ) ;
#29105=CARTESIAN_POINT ( 'NONE',  ( 6.000000000000001776, -5.180354513474913603, 36.12317359536750416 ) ) ;
#29108=CARTESIAN_POINT ( 'NONE',  ( -9.915792636031643070, -3.754499324213721234, 33.06261337010820256 ) ) ;
#29109=CARTESIAN_POINT ( 'NONE',  ( 14.55763782604045176, -10.76462480002816235, 33.53768742498949962 ) ) ;
#29110=CARTESIAN_POINT ( 'NONE',  ( -12.46153846153846168, -2.249999999999998668, 29.75000000000001776 ) ) ;
#29112=EDGE_CURVE ( 'NONE', #87025, #32375, #44787, .T. ) ;
#29114=CYLINDRICAL_SURFACE ( 'NONE', #17370, 0.2499999999999979738 ) ;
#29115=EDGE_LOOP ( 'NONE', ( #71616, #83473, #18618, #58024 ) ) ;
#29116=CARTESIAN_POINT ( 'NONE',  ( -3.230769230769229949, -6.435427911321262684, 35.78748833219616898 ) ) ;
#29118=CARTESIAN_POINT ( 'NONE',  ( 9.758376043310132530, -6.386643153685127139, 34.62446782046654192 ) ) ;
#29119=CARTESIAN_POINT ( 'NONE',  ( -14.30769230769230660, -11.69971097300155272, 32.46337939537588113 ) ) ;
#29121=CARTESIAN_POINT ( 'NONE',  ( -1.450698795571262689, -10.51840700105979387, 33.73612834413961536 ) ) ;
#29122=AXIS2_PLACEMENT_3D ( 'NONE', #24214, #80059, #71963 ) ;
#29123=CARTESIAN_POINT ( 'NONE',  ( -14.08491263871423449, -4.226511098958373402, 33.85474049983370293 ) ) ;
#29124=EDGE_CURVE ( 'NONE', #36170, #15837, #59999, .T. ) ;
#29125=FACE_OUTER_BOUND ( 'NONE', #62652, .T. ) ;
#29126=EDGE_LOOP ( 'NONE', ( #14232, #86708 ) ) ;
#29128=EDGE_CURVE ( 'NONE', #558, #10433, #18581, .T. ) ;
#29130=CARTESIAN_POINT ( 'NONE',  ( -13.60754160213153163, -3.586966769969701208, 32.86292498521069660 ) ) ;
#29132=CARTESIAN_POINT ( 'NONE',  ( 6.792928953345224841, -3.069018819979302926, 32.56621877034667278 ) ) ;
#29133=CARTESIAN_POINT ( 'NONE',  ( 2.057715576749954867, -5.728515186090277211, 34.42611988154120439 ) ) ;
#29135=B_SPLINE_CURVE_WITH_KNOTS ( 'NONE', 3,
 ( #38108, #11086, #52058, #86770, #18738, #58363, #31810, #17850, #11984, #57931 ),
 .UNSPECIFIED., .F., .F.,
 ( 4, 2, 2, 2, 4 ),
 ( 0.0007817359430256328248, 0.0009771253907249995759, 0.001172514838424366327, 0.001367904286123733078, 0.001563293733823099829 ),
 .UNSPECIFIED. ) ;
#29136=ORIENTED_EDGE ( 'NONE', *, *, #69105, .T. ) ;
#29137=EDGE_CURVE ( 'NONE', #49988, #6788, #60909, .T. ) ;
#29138=CARTESIAN_POINT ( 'NONE',  ( -18.25000000000000000, -7.500000000000001776, 34.75000000000000000 ) ) ;
#29140=ORIENTED_EDGE ( 'NONE', *, *, #74782, .T. ) ;
#29141=EDGE_LOOP ( 'NONE', ( #20351, #30640, #35888, #3502, #53926, #53197 ) ) ;
#29142=CARTESIAN_POINT ( 'NONE',  ( 4.284371592079798674, -12.50538340440932217, 31.33453814440721885 ) ) ;
#29143=VERTEX_POINT ( 'NONE', #24424 ) ;
#29145=CARTESIAN_POINT ( 'NONE',  ( -10.68065506134539078, -5.219633306516282545, 34.19971097300152962 ) ) ;
#29146=CARTESIAN_POINT ( 'NONE',  ( 3.930919936330006248, -4.186968288167446595, 33.49512374952580274 ) ) ;
#29147=EDGE_CURVE ( 'NONE', #83740, #81428, #7156, .T. ) ;
#29148=ORIENTED_EDGE ( 'NONE', *, *, #41033, .T. ) ;
#29152=DIRECTION ( 'NONE',  ( -0.000000000000000000, 1.000000000000000000, 3.491481338843133355E-15 ) ) ;
#29153=CYLINDRICAL_SURFACE ( 'NONE', #15738, 0.2499999999999973355 ) ;
#29154=ORIENTED_EDGE ( 'NONE', *, *, #62276, .T. ) ;
#29156=FACE_OUTER_BOUND ( 'NONE', #50837, .T. ) ;
#29157=CARTESIAN_POINT ( 'NONE',  ( -3.007757879156380820, -9.886259254753566594, 34.14407573483972413 ) ) ;
#29158=ORIENTED_EDGE ( 'NONE', *, *, #25703, .T. ) ;
#29159=ADVANCED_FACE ( 'NONE', ( #58214 ), #18135, .F. ) ;
#29161=CARTESIAN_POINT ( 'NONE',  ( -11.28840722682322273, -4.943051570960394159, 34.04725096376909477 ) ) ;
#29163=B_SPLINE_CURVE_WITH_KNOTS ( 'NONE', 3,
 ( #23031, #42873, #84312, #50492, #1436, #36554, #83420, #16710, #77975, #64892 ),
 .UNSPECIFIED., .F., .F.,
 ( 4, 2, 2, 2, 4 ),
 ( 0.0007817246256747514008, 0.0009771112852218959231, 0.001172497944769040337, 0.001367884604316184968, 0.001563271263863329381 ),
 .UNSPECIFIED. ) ;
#29164=ORIENTED_EDGE ( 'NONE', *, *, #20713, .F. ) ;
#29165=FACE_BOUND ( 'NONE', #74880, .T. ) ;
#29166=CARTESIAN_POINT ( 'NONE',  ( 11.53846153846141753, -5.219633306517616589, 34.19971097300220464 ) ) ;
#29167=DIRECTION ( 'NONE',  ( -0.000000000000000000, -0.000000000000000000, -1.000000000000000000 ) ) ;
#29168=B_SPLINE_CURVE_WITH_KNOTS ( 'NONE', 3,
 ( #25005, #52026, #38529, #86289, #78174, #30865, #43942, #3395, #10165, #72742 ),
 .UNSPECIFIED., .F., .F.,
 ( 4, 2, 2, 2, 4 ),
 ( 0.0007817246256747521597, 0.0009771112852218961399, 0.001172497944769040337, 0.001367884604316184534, 0.001563271263863328514 ),
 .UNSPECIFIED. ) ;
#29170=CARTESIAN_POINT ( 'NONE',  ( 16.15384615384615330, -13.20930481340135110, 34.54067556320372745 ) ) ;
#29171=CARTESIAN_POINT ( 'NONE',  ( -11.53846153846153655, -12.29105614889573062, 35.45975837776705220 ) ) ;
#29172=CARTESIAN_POINT ( 'NONE',  ( 14.30769230769231015, -6.435427911321262684, 35.78748833219616898 ) ) ;
#29173=VECTOR ( 'NONE', #11294, 1000.000000000000000 ) ;
#29174=B_SPLINE_CURVE_WITH_KNOTS ( 'NONE', 3,
 ( #35049, #82367, #14338, #8030, #76035, #41822, #69287, #35499, #28289, #27413 ),
 .UNSPECIFIED., .F., .F.,
 ( 4, 2, 2, 2, 4 ),
 ( 0.0007817246256747471724, 0.0009771112852218905021, 0.001172497944769033832, 0.001367884604316177161, 0.001563271263863320491 ),
 .UNSPECIFIED. ) ;
#29176=CARTESIAN_POINT ( 'NONE',  ( -4.376773112753000738, -10.77366814457252175, 33.85459836347579454 ) ) ;
#29177=ORIENTED_EDGE ( 'NONE', *, *, #59019, .T. ) ;
#29178=CARTESIAN_POINT ( 'NONE',  ( -11.47320596718551400, -4.481592998940250538, 33.73612834413965089 ) ) ;
#29179=CARTESIAN_POINT ( 'NONE',  ( -8.769230769230768274, -13.87047571288749737, 32.06866353760679544 ) ) ;
#29180=EDGE_LOOP ( 'NONE', ( #36777, #83038 ) ) ;
#29181=FACE_OUTER_BOUND ( 'NONE', #41195, .T. ) ;
#29182=CARTESIAN_POINT ( 'NONE',  ( -14.24162497434223162, -9.058645607665452459, 34.76329471203371924 ) ) ;
#29183=CARTESIAN_POINT ( 'NONE',  ( 3.453732134330715908, -7.369474270740069777, 34.74850911626239736 ) ) ;
#29184=CARTESIAN_POINT ( 'NONE',  ( -5.326946314216043810, -11.86270091957321249, 32.19358267280087915 ) ) ;
#29185=CARTESIAN_POINT ( 'NONE',  ( -0.2114841499001468561, -12.41262288849542017, 30.68299917996395010 ) ) ;
#29186=EDGE_CURVE ( 'NONE', #23103, #34892, #55024, .T. ) ;
#29187=CARTESIAN_POINT ( 'NONE',  ( 2.372947447205147053, -5.094484230520773593, 34.41647553114626845 ) ) ;
#29188=FACE_BOUND ( 'NONE', #64613, .T. ) ;
#29189=FACE_OUTER_BOUND ( 'NONE', #33449, .T. ) ;
#29191=FACE_OUTER_BOUND ( 'NONE', #42117, .T. ) ;
#29192=CARTESIAN_POINT ( 'NONE',  ( -6.673022503163469565, -10.82426656108011720, 33.81400080652039009 ) ) ;
#29193=CARTESIAN_POINT ( 'NONE',  ( 7.846153846154153122, -2.506253911140614576, 30.00000000000323297 ) ) ;
#29194=CARTESIAN_POINT ( 'NONE',  ( -14.24243716817947281, -5.941354392334607049, 34.76329471203374055 ) ) ;
#29196=EDGE_LOOP ( 'NONE', ( #74426, #28881 ) ) ;
#29197=EDGE_LOOP ( 'NONE', ( #83889, #27204, #44861, #85324 ) ) ;
#29198=CARTESIAN_POINT ( 'NONE',  ( -9.627052121031669074, -11.94971097300157403, 32.03036669348361443 ) ) ;
#29199=CARTESIAN_POINT ( 'NONE',  ( -12.21148404162500967, -6.523592122091592671, 34.90882529074906415 ) ) ;
#29200=CARTESIAN_POINT ( 'NONE',  ( 6.700248825442047362, -7.369209533119140509, 34.99857337881830688 ) ) ;
#29201=CARTESIAN_POINT ( 'NONE',  ( 9.692307692307570832, -12.70778746994576025, 30.41441678777401236 ) ) ;
#29202=LINE ( 'NONE', #69727, #18379 ) ;
#29204=DIRECTION ( 'NONE',  ( 0.000000000000000000, 0.1736481776669267785, -0.9848077530122087975 ) ) ;
#29205=CARTESIAN_POINT ( 'NONE',  ( -7.846153846153844924, -2.249999999999998668, 29.75000000000001776 ) ) ;
#29206=AXIS2_PLACEMENT_3D ( 'NONE', #51112, #51552, #10157 ) ;
#29207=CARTESIAN_POINT ( 'NONE',  ( 15.48082354240754555, -11.79725096376909654, 32.30694842903959341 ) ) ;
#29208=CARTESIAN_POINT ( 'NONE',  ( -3.230769230769229949, -11.91647553114624181, 32.58852847137148245 ) ) ;
#29210=CARTESIAN_POINT ( 'NONE',  ( -8.769230769230768274, -2.538708090699994813, 30.37095296980875503 ) ) ;
#29211=AXIS2_PLACEMENT_3D ( 'NONE', #82046, #47353, #68959 ) ;
#29212=CARTESIAN_POINT ( 'NONE',  ( 12.52679360105129724, -2.379036618887895305, 30.90682066428158592 ) ) ;
#29213=B_SPLINE_CURVE_WITH_KNOTS ( 'NONE', 3,
 ( #25843, #88020, #88452, #46982, #81678, #88893 ),
 .UNSPECIFIED., .F., .F.,
 ( 4, 2, 4 ),
 ( 0.0003909569690057804843, 0.0005862646681846042955, 0.0007815723673634281067 ),
 .UNSPECIFIED. ) ;
#29214=CARTESIAN_POINT ( 'NONE',  ( 7.911409417429874580, -6.879047030191282275, 34.71129190930002295 ) ) ;
#29215=EDGE_LOOP ( 'NONE', ( #20579, #18594 ) ) ;
#29216=CARTESIAN_POINT ( 'NONE',  ( 2.242422307135989445, -3.643525952247789412, 33.31231777344662959 ) ) ;
#29217=FACE_OUTER_BOUND ( 'NONE', #61130, .T. ) ;
#29219=CARTESIAN_POINT ( 'NONE',  ( 8.899275932065544126, -2.504778602574659896, 29.97347330155780654 ) ) ;
#29220=CARTESIAN_POINT ( 'NONE',  ( 6.923076923076924238, -4.098570777380720287, 33.41473453929634729 ) ) ;
#29221=EDGE_LOOP ( 'NONE', ( #761, #83737, #13128, #82931 ) ) ;
#29222=LINE ( 'NONE', #27878, #77329 ) ;
#29223=CARTESIAN_POINT ( 'NONE',  ( 16.15384615384603251, -3.083524468854526912, 32.58852847137268327 ) ) ;
#29225=CYLINDRICAL_SURFACE ( 'NONE', #16789, 0.2499999999999997502 ) ;
#29226=CARTESIAN_POINT ( 'NONE',  ( -18.00000000000000000, -13.45340096658850904, 31.05360187035682884 ) ) ;
#29227=VERTEX_POINT ( 'NONE', #40632 ) ;
#29228=CARTESIAN_POINT ( 'NONE',  ( 5.999999999999880096, -2.625532179533778709, 30.86335684631627174 ) ) ;
#29229=CARTESIAN_POINT ( 'NONE',  ( -6.988346923633242724, -11.67786785259541027, 32.92929555188721480 ) ) ;
#29230=VERTEX_POINT ( 'NONE', #20786 ) ;
#29231=CARTESIAN_POINT ( 'NONE',  ( 8.769230769230768274, -2.292212530054420494, 30.41441678777542634 ) ) ;
#29232=CARTESIAN_POINT ( 'NONE',  ( -16.15384615384627409, -3.300289026999228437, 32.46337939537709616 ) ) ;
#29233=CARTESIAN_POINT ( 'NONE',  ( 12.52679360105129724, -12.16647553114626490, 32.15551576947920864 ) ) ;
#29234=VERTEX_POINT ( 'NONE', #48254 ) ;
#29235=ORIENTED_EDGE ( 'NONE', *, *, #24713, .F. ) ;
#29236=AXIS2_PLACEMENT_3D ( 'NONE', #16864, #44312, #71801 ) ;
#29237=ORIENTED_EDGE ( 'NONE', *, *, #27981, .T. ) ;
#29238=AXIS2_PLACEMENT_3D ( 'NONE', #17391, #52496, #44847 ) ;
#29239=CARTESIAN_POINT ( 'NONE',  ( -6.923076923076922462, -2.292212530054420494, 30.41441678777542634 ) ) ;
#29242=B_SPLINE_CURVE_WITH_KNOTS ( 'NONE', 3,
 ( #76698, #35721, #8692, #34814, #55531, #9136, #77140, #22630, #50097, #83015 ),
 .UNSPECIFIED., .F., .F.,
 ( 4, 2, 2, 2, 4 ),
 ( 0.000000000000000000, 0.0001954339857564078267, 0.0003908679715128156535, 0.0005863019572692235344, 0.0007817359430256313069 ),
 .UNSPECIFIED. ) ;
#29243=B_SPLINE_CURVE_WITH_KNOTS ( 'NONE', 3,
 ( #63248, #56498, #15514, #50616, #71326, #56929, #23587, #49295, #16833, #16393 ),
 .UNSPECIFIED., .F., .F.,
 ( 4, 2, 2, 2, 4 ),
 ( 0.0007817359430256314154, 0.0009771253907249980580, 0.001172514838424364592, 0.001367904286123731127, 0.001563293733823097661 ),
 .UNSPECIFIED. ) ;
#29244=CARTESIAN_POINT ( 'NONE',  ( -17.32689980786543060, -6.567427716900048118, 34.66269422305636283 ) ) ;
#29245=B_SPLINE_CURVE_WITH_KNOTS ( 'NONE', 3,
 ( #32765, #60232, #53474, #59792, #46283, #26899, #53022, #61118, #18814, #88627 ),
 .UNSPECIFIED., .F., .F.,
 ( 4, 2, 2, 2, 4 ),
 ( 0.000000000000000000, 0.0001954311564186858715, 0.0003908623128373717431, 0.0005862934692560576146, 0.0007817246256747434861 ),
 .UNSPECIFIED. ) ;
#29246=B_SPLINE_CURVE_WITH_KNOTS ( 'NONE', 3,
 ( #65288, #63517, #50870, #9904, #71596, #57650, #3137, #30614, #58086, #3584 ),
 .UNSPECIFIED., .F., .F.,
 ( 4, 2, 2, 2, 4 ),
 ( 0.0007817359430256293554, 0.0009771253907249950223, 0.001172514838424360906, 0.001367904286123726790, 0.001563293733823092457 ),
 .UNSPECIFIED. ) ;
#29247=ORIENTED_EDGE ( 'NONE', *, *, #89117, .F. ) ;
#29248=VERTEX_POINT ( 'NONE', #46920 ) ;
#29249=CARTESIAN_POINT ( 'NONE',  ( -1.134615384613947953, -7.500000000000155431, 34.75000000000007105 ) ) ;
#29250=EDGE_LOOP ( 'NONE', ( #48286, #15440, #35602, #66498 ) ) ;
#29251=CARTESIAN_POINT ( 'NONE',  ( 12.46153846153833911, -11.67786785259630911, 32.92929555188603530 ) ) ;
#29252=ADVANCED_FACE ( 'NONE', ( #40193 ), #75298, .F. ) ;
#29253=ORIENTED_EDGE ( 'NONE', *, *, #85045, .T. ) ;
#29254=DIRECTION ( 'NONE',  ( -1.000000000000000000, 0.000000000000000000, 0.000000000000000000 ) ) ;
#29256=ORIENTED_EDGE ( 'NONE', *, *, #48382, .F. ) ;
#29257=CARTESIAN_POINT ( 'NONE',  ( -6.000000000000119904, -3.300289026999228881, 32.46337939537708905 ) ) ;
#29258=ORIENTED_EDGE ( 'NONE', *, *, #47068, .F. ) ;
#29259=CARTESIAN_POINT ( 'NONE',  ( -12.46153846153858247, -5.219633306517616589, 34.19971097300220464 ) ) ;
#29260=ORIENTED_EDGE ( 'NONE', *, *, #14194, .T. ) ;
#29261=VECTOR ( 'NONE', #653, 1000.000000000000000 ) ;
#29262=CARTESIAN_POINT ( 'NONE',  ( -5.933931648997561759, -8.120952969808772792, 34.71129190929999453 ) ) ;
#29263=CARTESIAN_POINT ( 'NONE',  ( -5.207614543590636913, -9.804603061927743113, 34.18744698557895845 ) ) ;
#29264=VERTEX_POINT ( 'NONE', #75726 ) ;
#29266=CARTESIAN_POINT ( 'NONE',  ( 15.23076923076923173, -3.050289026998446396, 32.03036669348365706 ) ) ;
#29267=CARTESIAN_POINT ( 'NONE',  ( 5.326868595271218254, -11.37275283266503756, 32.91324779482534524 ) ) ;
#29268=CARTESIAN_POINT ( 'NONE',  ( 6.673053698855467175, -5.765609946408404518, 34.70566812827425451 ) ) ;
#29269=FACE_BOUND ( 'NONE', #48396, .T. ) ;
#29270=CARTESIAN_POINT ( 'NONE',  ( 7.911408985666684046, -12.51329471203373700, 31.30864560766537963 ) ) ;
#29271=CARTESIAN_POINT ( 'NONE',  ( -11.76138849736838488, -6.459968553980841577, 34.89616026154728701 ) ) ;
#29272=CARTESIAN_POINT ( 'NONE',  ( 15.23076923076923173, -2.486705287966279876, 31.30864560766543647 ) ) ;
#29273=CARTESIAN_POINT ( 'NONE',  ( 3.361559671736180199, -4.684288915650983043, 34.18129842949671371 ) ) ;
#29274=CARTESIAN_POINT ( 'NONE',  ( -11.40793583669797506, -3.285477652293413264, 32.44071101563363158 ) ) ;
#29275=CARTESIAN_POINT ( 'NONE',  ( -13.38461538461538325, -8.564572088678739092, 35.78748833219616898 ) ) ;
#29276=ORIENTED_EDGE ( 'NONE', *, *, #77814, .F. ) ;
#29277=LINE ( 'NONE', #42790, #61943 ) ;
#29278=EDGE_LOOP ( 'NONE', ( #44204, #43527, #30099, #39550 ) ) ;
#29279=ORIENTED_EDGE ( 'NONE', *, *, #60408, .F. ) ;
#29280=CARTESIAN_POINT ( 'NONE',  ( 9.442307692307693401, -2.249999999999998668, 29.75000000000000355 ) ) ;
#29281=CARTESIAN_POINT ( 'NONE',  ( 16.40379167219429490, -12.22109172314383052, 31.39792113162168263 ) ) ;
#29282=CARTESIAN_POINT ( 'NONE',  ( -12.46153846153846168, -2.538708090699994813, 30.37095296980875503 ) ) ;
#29283=CARTESIAN_POINT ( 'NONE',  ( 8.096099255531889582, -3.520799739797214389, 33.17531984108286025 ) ) ;
#29284=LINE ( 'NONE', #56741, #1273 ) ;
#29285=CARTESIAN_POINT ( 'NONE',  ( -0.3307466537136754536, -11.71459661697925903, 32.44059661609676937 ) ) ;
#29286=ORIENTED_EDGE ( 'NONE', *, *, #9600, .T. ) ;
#29287=EDGE_CURVE ( 'NONE', #29866, #52292, #13703, .T. ) ;
#29288=CARTESIAN_POINT ( 'NONE',  ( -18.13069146666756382, -5.582088688514995845, 34.36776431015576350 ) ) ;
#29289=CARTESIAN_POINT ( 'NONE',  ( 1.384615384615386802, -12.10708131394839349, 31.69288490824020244 ) ) ;
#29290=LINE ( 'NONE', #57190, #80526 ) ;
#29291=CARTESIAN_POINT ( 'NONE',  ( 15.48071464014727461, -12.45601412856602686, 31.48342859153981621 ) ) ;
#29292=CARTESIAN_POINT ( 'NONE',  ( -15.29602022093047076, -2.506253911140460922, 30.00000000000013856 ) ) ;
#29294=ORIENTED_EDGE ( 'NONE', *, *, #48482, .T. ) ;
#29298=EDGE_CURVE ( 'NONE', #5455, #13666, #8283, .T. ) ;
#29299=CARTESIAN_POINT ( 'NONE',  ( -7.846153846153967493, -12.16647553114689728, 32.15551576947799362 ) ) ;
#29301=CARTESIAN_POINT ( 'NONE',  ( -9.942284423250047354, -12.41269422305637171, 30.68257228309993323 ) ) ;
#29302=CARTESIAN_POINT ( 'NONE',  ( -1.161835715637317135, -10.23759521482555357, 34.22997729860117033 ) ) ;
#29303=LINE ( 'NONE', #69833, #10665 ) ;
#29304=CARTESIAN_POINT ( 'NONE',  ( 2.373759641042384239, -9.905515769479277921, 34.41647553114623292 ) ) ;
#29305=CARTESIAN_POINT ( 'NONE',  ( -2.057637996053991003, -4.943051570960395047, 34.04725096376909477 ) ) ;
#29306=B_SPLINE_CURVE_WITH_KNOTS ( 'NONE', 3,
 ( #49961, #16184, #51260, #79221, #43649, #16616, #17520, #38227, #78766, #44970 ),
 .UNSPECIFIED., .F., .F.,
 ( 4, 2, 2, 2, 4 ),
 ( 0.0007817359430256216575, 0.0009771253907249856981, 0.001172514838424349847, 0.001367904286123713779, 0.001563293733823077928 ),
 .UNSPECIFIED. ) ;
#29307=CARTESIAN_POINT ( 'NONE',  ( 8.769230769230647482, -6.879047030192662504, 34.71129190930017927 ) ) ;
#29308=ORIENTED_EDGE ( 'NONE', *, *, #75042, .F. ) ;
#29309=LINE ( 'NONE', #44558, #71727 ) ;
#29310=CARTESIAN_POINT ( 'NONE',  ( -2.307692307692427391, -10.90142922262034020, 33.41473453929536674 ) ) ;
#29311=VERTEX_POINT ( 'NONE', #13150 ) ;
#29312=CARTESIAN_POINT ( 'NONE',  ( 2.980792499826877329, -12.41269422305637171, 30.68257228309993323 ) ) ;
#29314=CARTESIAN_POINT ( 'NONE',  ( 6.130525438233648039, -9.503571793651733657, 34.60286762892837942 ) ) ;
#29315=CARTESIAN_POINT ( 'NONE',  ( 6.699591998512594238, -3.562934362175799841, 33.22335522853832401 ) ) ;
#29316=CYLINDRICAL_SURFACE ( 'NONE', #75232, 0.2499999999999995559 ) ;
#29318=EDGE_LOOP ( 'NONE', ( #1366, #33558 ) ) ;
#29319=CARTESIAN_POINT ( 'NONE',  ( -1.134669866267241423, -11.37275283266503756, 32.91324779482534524 ) ) ;
#29320=CARTESIAN_POINT ( 'NONE',  ( -13.63463862190834952, -9.271318131107980420, 34.42618302367067429 ) ) ;
#29322=CARTESIAN_POINT ( 'NONE',  ( 0.2386115026316118215, -5.582147617184174848, 34.63737895849758530 ) ) ;
#29323=CARTESIAN_POINT ( 'NONE',  ( 9.468822767743363400, -6.716662450894489211, 34.94144148231605840 ) ) ;
#29324=EDGE_LOOP ( 'NONE', ( #74663, #65027, #10413, #3435 ) ) ;
#29325=CARTESIAN_POINT ( 'NONE',  ( 0.3313904918067645533, -4.299443229763728169, 33.91186481527756769 ) ) ;
#29326=DIRECTION ( 'NONE',  ( -0.000000000000000000, -0.3420201433256694346, -0.9396926207859080948 ) ) ;
#29327=VERTEX_POINT ( 'NONE', #27101 ) ;
#29328=VECTOR ( 'NONE', #22610, 1000.000000000000000 ) ;
#29329=CARTESIAN_POINT ( 'NONE',  ( 9.757452473027326434, -7.750023224968867197, 34.99404313364389907 ) ) ;
#29330=EDGE_LOOP ( 'NONE', ( #36914, #4963 ) ) ;
#29331=EDGE_CURVE ( 'NONE', #31770, #63430, #60907, .T. ) ;
#29333=CARTESIAN_POINT ( 'NONE',  ( -17.29985003582992320, -2.308479472611653094, 30.53278059502174457 ) ) ;
#29334=CARTESIAN_POINT ( 'NONE',  ( -12.68446542044531178, -10.01117774369187252, 34.36070679894347535 ) ) ;
#29335=DIRECTION ( 'NONE',  ( -0.000000000000000000, 0.6427876096865404731, -0.7660444431189770143 ) ) ;
#29336=VERTEX_POINT ( 'NONE', #74861 ) ;
#29337=CARTESIAN_POINT ( 'NONE',  ( -13.31936024510254413, -3.083524468853784839, 32.58852847137153930 ) ) ;
#29338=B_SPLINE_CURVE_WITH_KNOTS ( 'NONE', 3,
 ( #56920, #77197, #84416, #64996, #78520, #2850, #63235, #1544, #70449, #71760 ),
 .UNSPECIFIED., .F., .F.,
 ( 4, 2, 2, 2, 4 ),
 ( 0.000000000000000000, 0.0001954311564186871184, 0.0003908623128373742367, 0.0005862934692560614093, 0.0007817246256747484735 ),
 .UNSPECIFIED. ) ;
#29340=CARTESIAN_POINT ( 'NONE',  ( 5.999999999999878320, -5.094484230521993062, 34.41647553114689373 ) ) ;
#29341=CARTESIAN_POINT ( 'NONE',  ( -10.61538461538473399, -2.892918686052166066, 31.69288490824153470 ) ) ;
#29343=CARTESIAN_POINT ( 'NONE',  ( -6.249976744048590049, -10.82459398097509684, 33.81372124010185587 ) ) ;
#29344=CARTESIAN_POINT ( 'NONE',  ( 10.83816415665302557, -3.236590943229499029, 32.36255958852954251 ) ) ;
#29345=FACE_OUTER_BOUND ( 'NONE', #43881, .T. ) ;
#29346=ADVANCED_FACE ( 'NONE', ( #27551 ), #4447, .F. ) ;
#29348=CARTESIAN_POINT ( 'NONE',  ( -18.00000000000000000, -4.098570777380720287, 33.41473453929634729 ) ) ;
#29349=STYLED_ITEM ( 'NONE', ( #47702 ), #307 ) ;
#29352=ORIENTED_EDGE ( 'NONE', *, *, #40433, .F. ) ;
#29353=FACE_BOUND ( 'NONE', #52379, .T. ) ;
#29354=ORIENTED_EDGE ( 'NONE', *, *, #74183, .F. ) ;
#29355=CARTESIAN_POINT ( 'NONE',  ( 8.639083559792545941, -3.817052484675422797, 33.13202310037935661 ) ) ;
#29357=AXIS2_PLACEMENT_3D ( 'NONE', #12107, #5782, #87782 ) ;
#29358=EDGE_CURVE ( 'NONE', #87090, #58189, #10766, .T. ) ;
#29359=CYLINDRICAL_SURFACE ( 'NONE', #61683, 0.2499999999999995559 ) ;
#29360=CARTESIAN_POINT ( 'NONE',  ( 13.63466969625370062, -10.66356715214248752, 33.62249196103329751 ) ) ;
#29361=CARTESIAN_POINT ( 'NONE',  ( -2.176901866725357237, -9.929761469519744921, 34.40412654351204225 ) ) ;
#29362=EDGE_CURVE ( 'NONE', #922, #55479, #79229, .T. ) ;
#29363=EDGE_LOOP ( 'NONE', ( #74550, #37647 ) ) ;
#29364=VERTEX_POINT ( 'NONE', #5789 ) ;
#29365=ORIENTED_EDGE ( 'NONE', *, *, #58162, .T. ) ;
#29366=DIRECTION ( 'NONE',  ( 0.000000000000000000, 0.9848077530122072432, 0.1736481776669354937 ) ) ;
#29367=ORIENTED_EDGE ( 'NONE', *, *, #20410, .F. ) ;
#29368=B_SPLINE_CURVE_WITH_KNOTS ( 'NONE', 3,
 ( #47001, #24960, #40271, #17773, #6040, #45227, #72703, #65940, #79913, #18217 ),
 .UNSPECIFIED., .F., .F.,
 ( 4, 2, 2, 2, 4 ),
 ( 0.0007817359430256301143, 0.0009771253907249963233, 0.001172514838424362641, 0.001367904286123728958, 0.001563293733823095276 ),
 .UNSPECIFIED. ) ;
#29369=B_SPLINE_CURVE_WITH_KNOTS ( 'NONE', 3,
 ( #67386, #81354, #61946, #6573, #82237, #41249, #88570, #80918, #39928, #68271 ),
 .UNSPECIFIED., .F., .F.,
 ( 4, 2, 2, 2, 4 ),
 ( 0.0007817359430256365111, 0.0009771253907250045632, 0.001172514838424372399, 0.001367904286123740451, 0.001563293733823108503 ),
 .UNSPECIFIED. ) ;
#29370=EDGE_CURVE ( 'NONE', #81013, #25396, #64090, .T. ) ;
#29371=CYLINDRICAL_SURFACE ( 'NONE', #89109, 0.2499999999999998890 ) ;
#29372=B_SPLINE_CURVE_WITH_KNOTS ( 'NONE', 3,
 ( #82451, #39693, #20732, #32920, #75670, #55401, #62159, #41451, #467, #27935 ),
 .UNSPECIFIED., .F., .F.,
 ( 4, 2, 2, 2, 4 ),
 ( 0.000000000000000000, 0.0001954339857564064444, 0.0003908679715128128888, 0.0005863019572692193060, 0.0007817359430256257775 ),
 .UNSPECIFIED. ) ;
#29373=DIRECTION ( 'NONE',  ( -0.000000000000000000, -0.1736481776669307198, -0.9848077530122080203 ) ) ;
#29374=CARTESIAN_POINT ( 'NONE',  ( 8.769230769230768274, -1.951392089020283160, 34.73218667398347748 ) ) ;
#29375=ORIENTED_EDGE ( 'NONE', *, *, #43070, .F. ) ;
#29376=CARTESIAN_POINT ( 'NONE',  ( 16.28437159207980045, -2.372941743896878286, 30.88044141588253311 ) ) ;
#29377=EDGE_CURVE ( 'NONE', #8200, #54081, #80215, .T. ) ;
#29378=LINE ( 'NONE', #71223, #4280 ) ;
#29379=CARTESIAN_POINT ( 'NONE',  ( -17.77694319641476284, -12.75000000000000888, 29.61950345095122827 ) ) ;
#29380=CARTESIAN_POINT ( 'NONE',  ( -1.254089946381742315, -3.068774925481847493, 32.56582465632704526 ) ) ;
#29381=ORIENTED_EDGE ( 'NONE', *, *, #19799, .T. ) ;
#29382=EDGE_CURVE ( 'NONE', #62209, #76336, #85985, .T. ) ;
#29383=ORIENTED_EDGE ( 'NONE', *, *, #15560, .T. ) ;
#29385=CARTESIAN_POINT ( 'NONE',  ( -4.087777802843714170, -9.780366693483667717, 34.19971097300155805 ) ) ;
#29388=CARTESIAN_POINT ( 'NONE',  ( 10.55011461482829738, -2.379036618887870436, 30.90682066428147934 ) ) ;
#29389=FACE_OUTER_BOUND ( 'NONE', #77221, .T. ) ;
#29390=CARTESIAN_POINT ( 'NONE',  ( -3.361460697436787992, -11.18331474514187995, 33.13161551792790505 ) ) ;
#29391=FACE_BOUND ( 'NONE', #5121, .T. ) ;
#29392=CARTESIAN_POINT ( 'NONE',  ( -18.00000000000000000, -12.34228464037088635, 31.77849191805839268 ) ) ;
#29393=ORIENTED_EDGE ( 'NONE', *, *, #13930, .F. ) ;
#29394=ADVANCED_FACE ( 'NONE', ( #12114 ), #18417, .F. ) ;
#29395=CARTESIAN_POINT ( 'NONE',  ( 17.20744877868664346, -10.88167719472716399, 33.43325721877153711 ) ) ;
#29396=CARTESIAN_POINT ( 'NONE',  ( -14.30769230769242917, -12.70778746994576025, 30.41441678777401236 ) ) ;
#29397=CARTESIAN_POINT ( 'NONE',  ( 4.403900465484469784, -9.148310452688871663, 34.47095581063188519 ) ) ;
#29398=DIRECTION ( 'NONE',  ( 0.000000000000000000, 0.9848077530122072432, -0.1736481776669354937 ) ) ;
#29401=EDGE_LOOP ( 'NONE', ( #51471, #75873, #77505, #76051 ) ) ;
#29402=FACE_BOUND ( 'NONE', #42211, .T. ) ;
#29403=CARTESIAN_POINT ( 'NONE',  ( 5.010839665967196765, -5.557115091759785130, 34.35708131394839171 ) ) ;
#29404=ADVANCED_FACE ( 'NONE', ( #24262 ), #81016, .F. ) ;
#29405=CARTESIAN_POINT ( 'NONE',  ( 10.61538461538449596, -6.026961402154118019, 34.52809138561165270 ) ) ;
#29406=CARTESIAN_POINT ( 'NONE',  ( -2.980714919130914797, -8.303483539816728154, 34.68545999027711702 ) ) ;
#29407=EDGE_CURVE ( 'NONE', #67015, #25023, #9224, .T. ) ;
#29408=ORIENTED_EDGE ( 'NONE', *, *, #50007, .F. ) ;
#29409=CARTESIAN_POINT ( 'NONE',  ( -14.37377571864818648, -12.37446782046654192, 30.86335684631486487 ) ) ;
#29410=CARTESIAN_POINT ( 'NONE',  ( -17.77698715590660328, -4.026326845037963231, 33.68677907613344047 ) ) ;
#29411=CARTESIAN_POINT ( 'NONE',  ( 8.519207545009312099, -2.341070481393819236, 30.72580821765574299 ) ) ;
#29412=LINE ( 'NONE', #42036, #62010 ) ;
#29413=ORIENTED_EDGE ( 'NONE', *, *, #41435, .F. ) ;
#29416=CARTESIAN_POINT ( 'NONE',  ( 16.82689983963011926, -10.76384336483936011, 33.53834819971076087 ) ) ;
#29417=ORIENTED_EDGE ( 'NONE', *, *, #61333, .T. ) ;
#29418=CARTESIAN_POINT ( 'NONE',  ( -14.98076923076779465, -7.500000000000155431, 34.75000000000007105 ) ) ;
#29419=CARTESIAN_POINT ( 'NONE',  ( -1.449885385171703511, -12.51329471203370325, 31.30864560766548976 ) ) ;
#29420=DIRECTION ( 'NONE',  ( -0.000000000000000000, 0.5000000000000011102, -0.8660254037844381525 ) ) ;
#29421=B_SPLINE_CURVE_WITH_KNOTS ( 'NONE', 3,
 ( #50863, #31046, #37813, #24289, #9898, #18444, #78348, #16649, #44111, #71589 ),
 .UNSPECIFIED., .F., .F.,
 ( 4, 2, 2, 2, 4 ),
 ( 0.000000000000000000, 0.0001954339857564086941, 0.0003908679715128173882, 0.0005863019572692261365, 0.0007817359430256347764 ),
 .UNSPECIFIED. ) ;
#29422=CARTESIAN_POINT ( 'NONE',  ( -12.46153846153846168, -2.721908614388771852, 31.22303859784724978 ) ) ;
#29424=VECTOR ( 'NONE', #84430, 1000.000000000000000 ) ;
#29425=CARTESIAN_POINT ( 'NONE',  ( 8.769230769230645706, -4.320704448113951379, 33.92786785259630022 ) ) ;
#29426=CARTESIAN_POINT ( 'NONE',  ( 14.24242186173153435, -3.835265460703609186, 33.15142922261924241 ) ) ;
#29428=ORIENTED_EDGE ( 'NONE', *, *, #82198, .T. ) ;
#29429=CARTESIAN_POINT ( 'NONE',  ( 13.38461538461526423, -12.70778746994576025, 30.41441678777401236 ) ) ;
#29430=CARTESIAN_POINT ( 'NONE',  ( -9.442253272394237840, -11.47946981652013498, 33.17500667209847620 ) ) ;
#29431=ORIENTED_EDGE ( 'NONE', *, *, #80522, .F. ) ;
#29432=VECTOR ( 'NONE', #55105, 1000.000000000000114 ) ;
#29433=VERTEX_POINT ( 'NONE', #46776 ) ;
#29435=CARTESIAN_POINT ( 'NONE',  ( -10.83831083290076158, -11.24512374952581872, 33.06303171183252942 ) ) ;
#29436=CARTESIAN_POINT ( 'NONE',  ( -17.07692307692319744, -9.442884908241554243, 34.35708131394783038 ) ) ;
#29437=CARTESIAN_POINT ( 'NONE',  ( -14.30769230769230660, -13.63283147151868846, 33.57946703557072254 ) ) ;
#29438=CARTESIAN_POINT ( 'NONE',  ( -5.010854725920638408, -3.513871655860379306, 32.76840700105978499 ) ) ;
#29439=CARTESIAN_POINT ( 'NONE',  ( -8.834500769787091201, -2.657715359629089225, 31.77849191805832874 ) ) ;
#29441=CARTESIAN_POINT ( 'NONE',  ( 6.249999999999937828, -7.565270000091922853, 34.99999999999999289 ) ) ;
#29442=EDGE_CURVE ( 'NONE', #23776, #30732, #62961, .T. ) ;
#29445=CARTESIAN_POINT ( 'NONE',  ( 7.976945653978630979, -2.729792928343270031, 31.24908615093345077 ) ) ;
#29446=EDGE_CURVE ( 'NONE', #63242, #34093, #14641, .T. ) ;
#29449=EDGE_CURVE ( 'NONE', #76906, #1831, #26461, .T. ) ;
#29450=VERTEX_POINT ( 'NONE', #40534 ) ;
#29451=CARTESIAN_POINT ( 'NONE',  ( 8.769230769230768274, -2.833524468853757305, 32.15551576947925838 ) ) ;
#29452=CARTESIAN_POINT ( 'NONE',  ( -16.15384615384583711, -2.255955759149395501, 30.00000000000324363 ) ) ;
#29454=CYLINDRICAL_SURFACE ( 'NONE', #80085, 0.2500000000000008882 ) ;
#29455=ORIENTED_EDGE ( 'NONE', *, *, #36064, .F. ) ;
#29457=DIRECTION ( 'NONE',  ( 0.000000000000000000, 0.000000000000000000, 1.000000000000000000 ) ) ;
#29460=CARTESIAN_POINT ( 'NONE',  ( -9.019207513279360100, -9.234221910056348293, 34.70572697212741531 ) ) ;
#29461=B_SPLINE_CURVE_WITH_KNOTS ( 'NONE', 3,
 ( #65514, #58308, #29523, #44339, #71826, #64170, #37151, #10130, #37597, #24083 ),
 .UNSPECIFIED., .F., .F.,
 ( 4, 2, 2, 2, 4 ),
 ( 0.0007817359430256386795, 0.0009771253907250069485, 0.001172514838424375217, 0.001367904286123743486, 0.001563293733823111755 ),
 .UNSPECIFIED. ) ;
#29463=CARTESIAN_POINT ( 'NONE',  ( 15.90382291655318880, -2.823816976329320827, 31.52131813110797154 ) ) ;
#29464=VERTEX_POINT ( 'NONE', #69325 ) ;
#29465=CARTESIAN_POINT ( 'NONE',  ( -7.846153846153967493, -2.379036618888197729, 30.90682066428292885 ) ) ;
#29466=CARTESIAN_POINT ( 'NONE',  ( 9.019176178608812933, -9.357781135181031829, 34.66075350412533851 ) ) ;
#29467=FACE_OUTER_BOUND ( 'NONE', #16868, .T. ) ;
#29468=CARTESIAN_POINT ( 'NONE',  ( -10.61538461538461320, -2.499999999999998668, 29.50000000000001066 ) ) ;
#29469=DIRECTION ( 'NONE',  ( 0.000000000000000000, 0.1736481776669275834, 0.9848077530122086864 ) ) ;
#29470=EDGE_CURVE ( 'NONE', #10613, #2810, #82295, .T. ) ;
#29471=EDGE_LOOP ( 'NONE', ( #4506, #30806, #10207, #74665, #52118, #76508 ) ) ;
#29473=ORIENTED_EDGE ( 'NONE', *, *, #83264, .F. ) ;
#29474=AXIS2_PLACEMENT_3D ( 'NONE', #14763, #42241, #34586 ) ;
#29475=CARTESIAN_POINT ( 'NONE',  ( -3.230769230768915534, -2.255955759149395501, 30.00000000000324363 ) ) ;
#29476=CARTESIAN_POINT ( 'NONE',  ( 13.51540719244017374, -9.804649428959608670, 34.18742332936588468 ) ) ;
#29477=CARTESIAN_POINT ( 'NONE',  ( 0.5920638997721053842, -6.808710257144159783, 34.95449254468098843 ) ) ;
#29478=VECTOR ( 'NONE', #60102, 1000.000000000000227 ) ;
#29479=CARTESIAN_POINT ( 'NONE',  ( 16.94623247381276343, -9.929715669179216775, 34.40415004197138416 ) ) ;
#29480=CARTESIAN_POINT ( 'NONE',  ( 7.596153846153846700, -7.500000000000001776, 35.00000000000000000 ) ) ;
#29481=CARTESIAN_POINT ( 'NONE',  ( -7.846153846153844924, -6.386643153685126251, 34.62446782046654192 ) ) ;
#29482=EDGE_LOOP ( 'NONE', ( #57634, #18540, #19053, #55611 ) ) ;
#29484=EDGE_LOOP ( 'NONE', ( #44997, #86850, #66735, #76778 ) ) ;
#29486=VERTEX_POINT ( 'NONE', #421 ) ;
#29487=CARTESIAN_POINT ( 'NONE',  ( -9.757578138268467427, -9.442884908240170461, 34.35708131394840592 ) ) ;
#29488=CARTESIAN_POINT ( 'NONE',  ( 14.53070515178570332, -4.762714258010881885, 34.23016756924214832 ) ) ;
#29490=ORIENTED_EDGE ( 'NONE', *, *, #32205, .T. ) ;
#29492=EDGE_CURVE ( 'NONE', #38006, #64208, #15599, .T. ) ;
#29493=ORIENTED_EDGE ( 'NONE', *, *, #15095, .F. ) ;
#29494=CYLINDRICAL_SURFACE ( 'NONE', #83111, 0.2500000000000004996 ) ;
#29495=ORIENTED_EDGE ( 'NONE', *, *, #81425, .F. ) ;
#29496=EDGE_CURVE ( 'NONE', #48420, #25149, #47269, .T. ) ;
#29497=FACE_BOUND ( 'NONE', #59141, .T. ) ;
#29498=CARTESIAN_POINT ( 'NONE',  ( -6.249976730942353953, -9.148715823498378086, 34.47080413974185120 ) ) ;
#29501=CARTESIAN_POINT ( 'NONE',  ( -15.09997742294444478, -4.809403383903225304, 33.96459661697924304 ) ) ;
#29502=CARTESIAN_POINT ( 'NONE',  ( 16.37685750545900376, -4.187068189119696804, 33.49521262558774026 ) ) ;
#29503=EDGE_CURVE ( 'NONE', #5991, #328, #6727, .T. ) ;
#29504=CARTESIAN_POINT ( 'NONE',  ( -8.769230769230890843, -6.026961402154118019, 34.52809138561165270 ) ) ;
#29505=CARTESIAN_POINT ( 'NONE',  ( -11.66915300512910214, -5.582088688514999397, 34.36776431015576350 ) ) ;
#29506=CARTESIAN_POINT ( 'NONE',  ( 4.153846153846154188, -3.050289026998446396, 32.03036669348365706 ) ) ;
#29508=CARTESIAN_POINT ( 'NONE',  ( 8.546303810323916395, -11.43668979543634734, 33.22377378376089752 ) ) ;
#29509=CARTESIAN_POINT ( 'NONE',  ( -7.846153846153844924, -11.91647553114624181, 32.58852847137148245 ) ) ;
#29510=CARTESIAN_POINT ( 'NONE',  ( 16.21991450484859598, -8.973038597847269315, 34.52809138561122637 ) ) ;
#29511=CARTESIAN_POINT ( 'NONE',  ( 13.44987052412822059, -2.379036618887895305, 30.90682066428158592 ) ) ;
#29512=CARTESIAN_POINT ( 'NONE',  ( 9.469380733400845074, -12.38737895849757820, 31.66785238281580206 ) ) ;
#29513=CARTESIAN_POINT ( 'NONE',  ( 6.065255571276025215, -10.21337939537593620, 33.94971097300152252 ) ) ;
#29514=DIRECTION ( 'NONE',  ( -0.000000000000000000, -0.7660444431189791237, -0.6427876096865379196 ) ) ;
#29515=CARTESIAN_POINT ( 'NONE',  ( 11.60462814505318008, -7.250054591869670162, 34.99404684341514127 ) ) ;
#29516=CARTESIAN_POINT ( 'NONE',  ( -14.30769230769230660, -8.164416787775445883, 34.95778746994557906 ) ) ;
#29517=CARTESIAN_POINT ( 'NONE',  ( 4.023155550735844521, -5.496505350115500121, 34.60290016733514307 ) ) ;
#29518=CARTESIAN_POINT ( 'NONE',  ( 5.933916589044121892, -10.51840700105979387, 33.73612834413961536 ) ) ;
#29519=EDGE_CURVE ( 'NONE', #22275, #16729, #49406, .T. ) ;
#29520=CARTESIAN_POINT ( 'NONE',  ( 2.307692307692309264, -13.78497067705608181, 32.30358669280327177 ) ) ;
#29522=VERTEX_POINT ( 'NONE', #16579 ) ;
#29523=CARTESIAN_POINT ( 'NONE',  ( 18.13052570176355971, -11.93748526763465279, 32.05452791011430946 ) ) ;
#29526=EDGE_CURVE ( 'NONE', #14701, #17652, #86611, .T. ) ;
#29527=ORIENTED_EDGE ( 'NONE', *, *, #59358, .T. ) ;
#29528=DIRECTION ( 'NONE',  ( -0.000000000000000000, 0.5000000000000011102, -0.8660254037844380415 ) ) ;
#29529=CARTESIAN_POINT ( 'NONE',  ( -3.230769230769351186, -3.300289026999228881, 32.46337939537708905 ) ) ;
#29530=EDGE_LOOP ( 'NONE', ( #39890, #10057 ) ) ;
#29531=FACE_OUTER_BOUND ( 'NONE', #11926, .T. ) ;
#29533=CARTESIAN_POINT ( 'NONE',  ( 7.596130621932389637, -8.475808217655753651, 34.90892951860618609 ) ) ;
#29535=CARTESIAN_POINT ( 'NONE',  ( -5.299849294439222369, -4.887634598454295265, 34.01352882383564946 ) ) ;
#29537=CARTESIAN_POINT ( 'NONE',  ( 11.53846153846141753, -2.892918686052165622, 31.69288490824153470 ) ) ;
#29538=CARTESIAN_POINT ( 'NONE',  ( 6.923076923076924238, -8.120952969808772792, 34.71129190930000163 ) ) ;
#29540=B_SPLINE_CURVE_WITH_KNOTS ( 'NONE', 3,
 ( #16837, #72667, #51041, #78534, #85752, #38001, #78983, #18180, #37101, #44743 ),
 .UNSPECIFIED., .F., .F.,
 ( 4, 2, 2, 2, 4 ),
 ( 0.0007817359430256379206, 0.0009771253907250060811, 0.001172514838424374133, 0.001367904286123742185, 0.001563293733823110238 ),
 .UNSPECIFIED. ) ;
#29541=EDGE_CURVE ( 'NONE', #37415, #2917, #45743, .T. ) ;
#29543=LINE ( 'NONE', #48022, #39111 ) ;
#29544=FACE_OUTER_BOUND ( 'NONE', #48897, .T. ) ;
#29548=DIRECTION ( 'NONE',  ( 0.000000000000000000, 0.000000000000000000, 1.000000000000000000 ) ) ;
#29549=ORIENTED_EDGE ( 'NONE', *, *, #16349, .T. ) ;
#29550=CARTESIAN_POINT ( 'NONE',  ( 14.43821800945587341, -5.195472089885680766, 34.18748526763464923 ) ) ;
#29551=CARTESIAN_POINT ( 'NONE',  ( 11.60452988946397923, -5.557115091759786019, 34.35708131394839882 ) ) ;
#29552=CARTESIAN_POINT ( 'NONE',  ( -8.834501215191544077, -11.48612834413959582, 32.76840700105983473 ) ) ;
#29555=CARTESIAN_POINT ( 'NONE',  ( -3.164700879766792152, -4.786620604624113540, 33.94971097300155805 ) ) ;
#29559=EDGE_CURVE ( 'NONE', #83441, #1531, #42743, .T. ) ;
#29560=ORIENTED_EDGE ( 'NONE', *, *, #81328, .F. ) ;
#29562=ORIENTED_EDGE ( 'NONE', *, *, #18400, .F. ) ;
#29563=CARTESIAN_POINT ( 'NONE',  ( -6.066082379360133281, -12.62096338111211580, 30.90682066428152197 ) ) ;
#29564=CARTESIAN_POINT ( 'NONE',  ( 4.153846153846032507, -8.613356846316285953, 34.62446782046622218 ) ) ;
#29565=LINE ( 'NONE', #44379, #64763 ) ;
#29566=CARTESIAN_POINT ( 'NONE',  ( -6.223484943723947893, -3.236172620538810385, 32.36188796281390267 ) ) ;
#29567=CARTESIAN_POINT ( 'NONE',  ( 9.692307692307695177, -3.050289026998446396, 32.03036669348365706 ) ) ;
#29568=EDGE_CURVE ( 'NONE', #33767, #19270, #12408, .T. ) ;
#29569=B_SPLINE_CURVE_WITH_KNOTS ( 'NONE', 3,
 ( #53243, #32987, #46497, #79844, #51441, #3725, #51899, #79398, #45154, #40199 ),
 .UNSPECIFIED., .F., .F.,
 ( 4, 2, 2, 2, 4 ),
 ( 0.0007817359430256297891, 0.0009771253907249958896, 0.001172514838424361990, 0.001367904286123728091, 0.001563293733823094191 ),
 .UNSPECIFIED. ) ;
#29570=AXIS2_PLACEMENT_3D ( 'NONE', #50769, #21993, #8929 ) ;
#29571=VERTEX_POINT ( 'NONE', #76522 ) ;
#29572=EDGE_CURVE ( 'NONE', #43471, #70228, #14827, .T. ) ;
#29573=CARTESIAN_POINT ( 'NONE',  ( -17.93383085903734298, -7.250054483168842268, 34.74374881642865631 ) ) ;
#29574=ORIENTED_EDGE ( 'NONE', *, *, #20027, .F. ) ;
#29575=B_SPLINE_CURVE_WITH_KNOTS ( 'NONE', 3,
 ( #1372, #82915, #56320, #48666, #49116, #28861, #77475, #76595, #14448, #15785 ),
 .UNSPECIFIED., .F., .F.,
 ( 4, 2, 2, 2, 4 ),
 ( 0.000000000000000000, 0.0001954311564186863052, 0.0003908623128373726104, 0.0005862934692560589156, 0.0007817246256747452209 ),
 .UNSPECIFIED. ) ;
#29576=EDGE_LOOP ( 'NONE', ( #14374, #12486 ) ) ;
#29577=CARTESIAN_POINT ( 'NONE',  ( -15.23076923076935074, -12.27809138561165270, 31.22303859784587132 ) ) ;
#29578=ORIENTED_EDGE ( 'NONE', *, *, #59810, .T. ) ;
#29581=CARTESIAN_POINT ( 'NONE',  ( 3.930361210122205406, -4.386631170607603991, 33.66268669641500111 ) ) ;
#29582=CARTESIAN_POINT ( 'NONE',  ( -16.02332071561251325, -5.915461855592777596, 34.75538340440931506 ) ) ;
#29584=ORIENTED_EDGE ( 'NONE', *, *, #77311, .T. ) ;
#29586=ORIENTED_EDGE ( 'NONE', *, *, #88513, .T. ) ;
#29588=CARTESIAN_POINT ( 'NONE',  ( 1.384615384615265343, -8.613356846316285953, 34.62446782046622218 ) ) ;
#29590=DIRECTION ( 'NONE',  ( 0.000000000000000000, 0.9848077530122072432, -0.1736481776669354937 ) ) ;
#29593=CARTESIAN_POINT ( 'NONE',  ( -0.3962833220256229416, -9.528491918058460186, 34.59228464037085615 ) ) ;
#29594=ORIENTED_EDGE ( 'NONE', *, *, #64006, .T. ) ;
#29595=CARTESIAN_POINT ( 'NONE',  ( -11.28851602011339672, -5.057305518903948638, 34.11320923018887896 ) ) ;
#29596=CARTESIAN_POINT ( 'NONE',  ( 15.23076923076910916, -2.657715359629662544, 31.77849191805970364 ) ) ;
#29597=EDGE_LOOP ( 'NONE', ( #846, #1966, #27323, #81565 ) ) ;
#29598=FACE_BOUND ( 'NONE', #86666, .T. ) ;
#29599=CARTESIAN_POINT ( 'NONE',  ( -11.78848476268299628, -11.56360843649121684, 33.07473185843129926 ) ) ;
#29600=CARTESIAN_POINT ( 'NONE',  ( 10.86543892702293412, -9.148310452688876993, 34.47095581063188519 ) ) ;
#29602=CARTESIAN_POINT ( 'NONE',  ( 7.976944287120795174, -10.70102852606553157, 33.91149625220312913 ) ) ;
#29603=CARTESIAN_POINT ( 'NONE',  ( -10.61538461538461320, -5.471508081941601098, 34.59228464037088457 ) ) ;
#29605=CYLINDRICAL_SURFACE ( 'NONE', #60658, 0.2500000000000008882 ) ;
#29606=EDGE_LOOP ( 'NONE', ( #13113, #56057 ) ) ;
#29607=B_SPLINE_CURVE_WITH_KNOTS ( 'NONE', 3,
 ( #22841, #70594, #85438, #51173, #3006, #77788, #28731, #29616, #35931, #8900 ),
 .UNSPECIFIED., .F., .F.,
 ( 4, 2, 2, 2, 4 ),
 ( 0.0007817359430256221996, 0.0009771253907249863487, 0.001172514838424350498, 0.001367904286123714647, 0.001563293733823078796 ),
 .UNSPECIFIED. ) ;
#29608=DIRECTION ( 'NONE',  ( -0.000000000000000000, -0.7660444431189791237, -0.6427876096865379196 ) ) ;
#29609=EDGE_CURVE ( 'NONE', #18998, #76633, #22895, .T. ) ;
#29610=VECTOR ( 'NONE', #84321, 1000.000000000000114 ) ;
#29611=CARTESIAN_POINT ( 'NONE',  ( -16.94639763868943660, -6.808710257144159783, 34.95449254468098843 ) ) ;
#29612=ORIENTED_EDGE ( 'NONE', *, *, #2045, .F. ) ;
#29616=CARTESIAN_POINT ( 'NONE',  ( -16.02305434602136813, -10.54018710029568595, 33.71981072465678864 ) ) ;
#29617=CARTESIAN_POINT ( 'NONE',  ( 18.00000000000000000, -9.819645486525091727, 36.12317359536749706 ) ) ;
#29618=CARTESIAN_POINT ( 'NONE',  ( 8.069166690247241647, -6.460100341425561332, 34.89618726649961644 ) ) ;
#29619=FACE_OUTER_BOUND ( 'NONE', #51808, .T. ) ;
#29620=FACE_BOUND ( 'NONE', #38030, .T. ) ;
#29621=CARTESIAN_POINT ( 'NONE',  ( -1.384615384615506484, -6.835583212225970762, 34.95778746994575670 ) ) ;
#29622=FACE_OUTER_BOUND ( 'NONE', #84432, .T. ) ;
#29624=LINE ( 'NONE', #57081, #40125 ) ;
#29625=CARTESIAN_POINT ( 'NONE',  ( 6.988332494352946789, -12.46129190930001052, 30.37095296980870174 ) ) ;
#29626=EDGE_CURVE ( 'NONE', #47623, #79680, #15266, .T. ) ;
#29627=CARTESIAN_POINT ( 'NONE',  ( 1.319365452841301689, -2.255955759149247619, 30.00000000000013856 ) ) ;
#29629=ORIENTED_EDGE ( 'NONE', *, *, #39221, .F. ) ;
#29632=CARTESIAN_POINT ( 'NONE',  ( -14.30769230769242739, -6.879047030192662504, 34.71129190930017927 ) ) ;
#29633=CARTESIAN_POINT ( 'NONE',  ( -0.5276208408985961773, -3.322132147404559976, 32.92929555188719348 ) ) ;
#29634=CARTESIAN_POINT ( 'NONE',  ( 8.519230769230757616, -2.249999999999999556, 29.81609741502488120 ) ) ;
#29635=CARTESIAN_POINT ( 'NONE',  ( -4.153846153846274980, -3.083524468854526912, 32.58852847137268327 ) ) ;
#29638=CARTESIAN_POINT ( 'NONE',  ( -8.546219417617921366, -2.758310577978207778, 31.33698337089302299 ) ) ;
#29639=CARTESIAN_POINT ( 'NONE',  ( 10.61538461538461675, -1.242168528481310874, 33.36296068462461051 ) ) ;
#29640=EDGE_CURVE ( 'NONE', #32683, #10626, #79085, .T. ) ;
#29642=DIRECTION ( 'NONE',  ( 0.000000000000000000, 0.4999999999999985567, 0.8660254037844395958 ) ) ;
#29643=CARTESIAN_POINT ( 'NONE',  ( -3.360917200500926683, -4.299443229763728169, 33.91186481527756058 ) ) ;
#29644=DIRECTION ( 'NONE',  ( 0.000000000000000000, 0.8660254037844377084, 0.5000000000000015543 ) ) ;
#29645=CARTESIAN_POINT ( 'NONE',  ( -11.53846153846153655, -5.180354513474913603, 36.12317359536750416 ) ) ;
#29646=CARTESIAN_POINT ( 'NONE',  ( 7.846153846153725020, -6.879047030192662504, 34.71129190930017927 ) ) ;
#29647=EDGE_LOOP ( 'NONE', ( #57627, #67068 ) ) ;
#29649=CARTESIAN_POINT ( 'NONE',  ( -5.999999999999998224, -2.486705287966279876, 31.30864560766543647 ) ) ;
#29652=CARTESIAN_POINT ( 'NONE',  ( -2.531177232256637932, -4.988325925672468131, 34.36044203135681130 ) ) ;
#29655=CARTESIAN_POINT ( 'NONE',  ( -6.989159302437059296, -2.833524468853757305, 32.15551576947924417 ) ) ;
#29656=CARTESIAN_POINT ( 'NONE',  ( 6.923076923076924238, -1.367168528481310208, 33.57946703557072254 ) ) ;
#29657=EDGE_LOOP ( 'NONE', ( #33601, #67875 ) ) ;
#29658=CARTESIAN_POINT ( 'NONE',  ( 8.068933387422253745, -3.755027918224369099, 33.06320215134714857 ) ) ;
#29659=EDGE_CURVE ( 'NONE', #42538, #37962, #32832, .T. ) ;
#29660=CARTESIAN_POINT ( 'NONE',  ( -13.13456107297706588, -9.943054286541403997, 34.11300777759954883 ) ) ;
#29661=ORIENTED_EDGE ( 'NONE', *, *, #79507, .T. ) ;
#29662=CARTESIAN_POINT ( 'NONE',  ( -5.299849294439222369, -11.24512374952581872, 33.06303171183252942 ) ) ;
#29663=CARTESIAN_POINT ( 'NONE',  ( 8.835299120233207404, -4.786620604624113540, 33.94971097300155805 ) ) ;
#29664=ORIENTED_EDGE ( 'NONE', *, *, #27426, .T. ) ;
#29667=VECTOR ( 'NONE', #17212, 1000.000000000000000 ) ;
#29668=EDGE_CURVE ( 'NONE', #55756, #74977, #79176, .T. ) ;
#29669=CARTESIAN_POINT ( 'NONE',  ( -17.75000000000000355, -12.50000000000000000, 29.75000000000000355 ) ) ;
#29670=EDGE_LOOP ( 'NONE', ( #47206, #2065, #39206, #61753 ) ) ;
#29671=ORIENTED_EDGE ( 'NONE', *, *, #74816, .T. ) ;
#29672=B_SPLINE_CURVE_WITH_KNOTS ( 'NONE', 3,
 ( #16447, #64172, #30841, #23640, #2042, #56982, #37155, #64614, #46477, #50213 ),
 .UNSPECIFIED., .F., .F.,
 ( 4, 2, 2, 2, 4 ),
 ( 0.000000000000000000, 0.0001954311564186861697, 0.0003908623128373723394, 0.0005862934692560584820, 0.0007817246256747446788 ),
 .UNSPECIFIED. ) ;
#29673=B_SPLINE_CURVE_WITH_KNOTS ( 'NONE', 3,
 ( #73726, #19213, #80023, #67840, #6139, #39497, #25961, #46678, #74156, #39938 ),
 .UNSPECIFIED., .F., .F.,
 ( 4, 2, 2, 2, 4 ),
 ( 0.0007817246256747507503, 0.0009771112852218959231, 0.001172497944769040987, 0.001367884604316186052, 0.001563271263863331116 ),
 .UNSPECIFIED. ) ;
#29674=ORIENTED_EDGE ( 'NONE', *, *, #8433, .T. ) ;
#29675=CARTESIAN_POINT ( 'NONE',  ( 3.361294669002876212, -2.372941743896878286, 30.88044141588254377 ) ) ;
#29676=CARTESIAN_POINT ( 'NONE',  ( 2.530705151785704210, -11.43677907613345113, 33.22367315496201456 ) ) ;
#29677=CARTESIAN_POINT ( 'NONE',  ( -3.230769230769229949, -8.164416787775445883, 34.95778746994557906 ) ) ;
#29680=EDGE_CURVE ( 'NONE', #2558, #24114, #28531, .T. ) ;
#29681=EDGE_CURVE ( 'NONE', #44409, #59335, #4401, .T. ) ;
#29682=VERTEX_POINT ( 'NONE', #73310 ) ;
#29684=CARTESIAN_POINT ( 'NONE',  ( 4.376625822824220080, -8.540255544307065350, 34.89611431652622286 ) ) ;
#29685=ORIENTED_EDGE ( 'NONE', *, *, #1808, .F. ) ;
#29686=EDGE_CURVE ( 'NONE', #27365, #38356, #11613, .T. ) ;
#29687=EDGE_CURVE ( 'NONE', #84823, #35118, #4859, .T. ) ;
#29688=CARTESIAN_POINT ( 'NONE',  ( 12.68455130563185840, -11.43677907613344757, 33.22367315496202167 ) ) ;
#29690=VECTOR ( 'NONE', #24666, 1000.000000000000227 ) ;
#29691=CARTESIAN_POINT ( 'NONE',  ( -17.75005448165186195, -3.202959910592339199, 32.30730279482229150 ) ) ;
#29692=CARTESIAN_POINT ( 'NONE',  ( 5.142991427925513115, -3.513871655860379306, 32.76840700105978499 ) ) ;
#29693=ORIENTED_EDGE ( 'NONE', *, *, #23919, .F. ) ;
#29694=AXIS2_PLACEMENT_3D ( 'NONE', #73983, #33436, #81185 ) ;
#29695=EDGE_LOOP ( 'NONE', ( #55587, #76646 ) ) ;
#29697=ORIENTED_EDGE ( 'NONE', *, *, #29668, .F. ) ;
#29698=CARTESIAN_POINT ( 'NONE',  ( -0.4615384615385826339, -10.90142922262034020, 33.41473453929536674 ) ) ;
#29699=CARTESIAN_POINT ( 'NONE',  ( 14.24242230713598900, -5.941354392334499579, 34.76329471203369792 ) ) ;
#29700=VERTEX_POINT ( 'NONE', #87287 ) ;
#29701=AXIS2_PLACEMENT_3D ( 'NONE', #88256, #26533, #66627 ) ;
#29702=CARTESIAN_POINT ( 'NONE',  ( 18.00000000000000000, -10.51840700105979565, 33.73612834413961536 ) ) ;
#29703=B_SPLINE_CURVE_WITH_KNOTS ( 'NONE', 3,
 ( #957, #62212, #55455, #28429, #43276, #21223, #35186, #70750, #49588, #8612 ),
 .UNSPECIFIED., .F., .F.,
 ( 4, 2, 2, 2, 4 ),
 ( 0.000000000000000000, 0.0001954339857564054957, 0.0003908679715128109914, 0.0005863019572692164871, 0.0007817359430256219828 ),
 .UNSPECIFIED. ) ;
#29704=CARTESIAN_POINT ( 'NONE',  ( 5.207714884747862705, -11.18335022499818621, 33.13157742990016885 ) ) ;
#29705=CARTESIAN_POINT ( 'NONE',  ( 17.74997677577854205, -12.45566812827425096, 31.48439005359158926 ) ) ;
#29706=FACE_BOUND ( 'NONE', #15965, .T. ) ;
#29707=CARTESIAN_POINT ( 'NONE',  ( -11.76194648218548267, -2.599994579823203367, 30.74605699353653776 ) ) ;
#29708=CARTESIAN_POINT ( 'NONE',  ( -18.00000000000012079, -12.27809138561165270, 31.22303859784587132 ) ) ;
#29709=CARTESIAN_POINT ( 'NONE',  ( 14.30769230769218758, -12.27809138561165270, 31.22303859784587132 ) ) ;
#29710=CARTESIAN_POINT ( 'NONE',  ( 12.46153846153833911, -3.643525952248795718, 33.31231777344771672 ) ) ;
#29713=DIRECTION ( 'NONE',  ( -0.000000000000000000, 0.7660444431189791237, -0.6427876096865379196 ) ) ;
#29714=ORIENTED_EDGE ( 'NONE', *, *, #80070, .F. ) ;
#29715=CARTESIAN_POINT ( 'NONE',  ( 14.55769230769224620, -7.565270445406050648, 34.75000000000000000 ) ) ;
#29716=ORIENTED_EDGE ( 'NONE', *, *, #21331, .F. ) ;
#29717=ORIENTED_EDGE ( 'NONE', *, *, #62921, .F. ) ;
#29718=CARTESIAN_POINT ( 'NONE',  ( -23.00000000000000000, -10.75000000000000000, 29.75000000000000355 ) ) ;
#29719=CARTESIAN_POINT ( 'NONE',  ( -10.61538461538473577, -2.379036618888197729, 30.90682066428292885 ) ) ;
#29720=CARTESIAN_POINT ( 'NONE',  ( 13.16168842570853670, -11.43668979543634734, 33.22377378376089752 ) ) ;
#29721=FACE_OUTER_BOUND ( 'NONE', #30565, .T. ) ;
#29722=CARTESIAN_POINT ( 'NONE',  ( 1.634669804528838588, -10.82426656108011720, 33.81400080652039009 ) ) ;
#29723=CARTESIAN_POINT ( 'NONE',  ( 1.384615384615265343, -11.94971097300221174, 32.03036669348237098 ) ) ;
#29725=AXIS2_PLACEMENT_3D ( 'NONE', #51426, #78928, #17228 ) ;
#29726=CARTESIAN_POINT ( 'NONE',  ( -10.61538461538461320, -12.34228464037088635, 31.77849191805839268 ) ) ;
#29727=CARTESIAN_POINT ( 'NONE',  ( 14.08420738312797837, -12.69144148231606017, 30.53333754910549303 ) ) ;
#29728=CARTESIAN_POINT ( 'NONE',  ( -12.59168643127016196, -11.66186481527757302, 32.95055677023626117 ) ) ;
#29730=CARTESIAN_POINT ( 'NONE',  ( -15.48076923076922995, -2.499999999999998668, 29.75000000000000355 ) ) ;
#29732=ORIENTED_EDGE ( 'NONE', *, *, #4221, .T. ) ;
#29733=ORIENTED_EDGE ( 'NONE', *, *, #76726, .F. ) ;
#29734=CARTESIAN_POINT ( 'NONE',  ( -7.623141002060451754, -11.98016756924215009, 32.48728574198911190 ) ) ;
#29735=ORIENTED_EDGE ( 'NONE', *, *, #49622, .T. ) ;
#29736=CIRCLE ( 'NONE', #41241, 0.2500000000000002220 ) ;
#29737=CARTESIAN_POINT ( 'NONE',  ( -17.93485422066803281, -7.750023238201980469, 34.74374492549440419 ) ) ;
#29738=CARTESIAN_POINT ( 'NONE',  ( 17.86930939688969033, -11.37499894934982514, 33.29245874905763003 ) ) ;
#29739=CARTESIAN_POINT ( 'NONE',  ( 3.230769230769231726, -6.343179335718451384, 34.87096338111211935 ) ) ;
#29740=CARTESIAN_POINT ( 'NONE',  ( 2.307692307692186251, -10.33852847137269571, 34.16647553114546554 ) ) ;
#29742=B_SPLINE_CURVE_WITH_KNOTS ( 'NONE', 3,
 ( #66908, #87643, #53385, #5204, #11523, #67355, #33121, #5648, #60138, #39005 ),
 .UNSPECIFIED., .F., .F.,
 ( 4, 2, 2, 2, 4 ),
 ( 0.000000000000000000, 0.0001954311564186865763, 0.0003908623128373731525, 0.0005862934692560596746, 0.0007817246256747463051 ),
 .UNSPECIFIED. ) ;
#29743=CARTESIAN_POINT ( 'NONE',  ( 0.5923289025054114809, -9.084667340241226796, 34.75534355489798344 ) ) ;
#29744=ORIENTED_EDGE ( 'NONE', *, *, #77988, .F. ) ;
#29746=CARTESIAN_POINT ( 'NONE',  ( -2.307692307692305711, -10.51840700105979565, 33.73612834413961536 ) ) ;
#29747=EDGE_LOOP ( 'NONE', ( #64865, #83275 ) ) ;
#29748=CARTESIAN_POINT ( 'NONE',  ( 3.100621261037533216, -12.50552854090298993, 31.33409797877408920 ) ) ;
#29749=CARTESIAN_POINT ( 'NONE',  ( 17.14217864819910275, -11.48612834413965977, 32.76840700105972815 ) ) ;
#29750=CARTESIAN_POINT ( 'NONE',  ( 11.31497659473759043, -4.386631170607603991, 33.66268669641500111 ) ) ;
#29751=CARTESIAN_POINT ( 'NONE',  ( -2.176901866725357682, -2.295524264805589354, 30.44142389570982488 ) ) ;
#29752=DIRECTION ( 'NONE',  ( -0.000000000000000000, 0.7660444431189791237, -0.6427876096865379196 ) ) ;
#29753=CARTESIAN_POINT ( 'NONE',  ( -11.40793610022789828, -3.068774925481847493, 32.56582465632704526 ) ) ;
#29755=ORIENTED_EDGE ( 'NONE', *, *, #49622, .F. ) ;
#29756=CARTESIAN_POINT ( 'NONE',  ( -17.07692307692307665, -10.51840700105979565, 33.73612834413961536 ) ) ;
#29757=CARTESIAN_POINT ( 'NONE',  ( -13.63459211555773720, -9.148715823498378086, 34.47080413974185120 ) ) ;
#29759=EDGE_CURVE ( 'NONE', #12856, #20277, #83414, .T. ) ;
#29760=CARTESIAN_POINT ( 'NONE',  ( 0.2115617305961059735, -3.627789207965226748, 32.91389620160131102 ) ) ;
#29762=CARTESIAN_POINT ( 'NONE',  ( 2.372947447205147053, -12.16647553114626490, 32.15551576947920864 ) ) ;
#29763=ORIENTED_EDGE ( 'NONE', *, *, #8168, .T. ) ;
#29764=CARTESIAN_POINT ( 'NONE',  ( 7.912221179503920787, -11.91647553114624358, 32.58852847137148245 ) ) ;
#29765=CARTESIAN_POINT ( 'NONE',  ( -16.15384615384627409, -12.27809138561165270, 31.22303859784587132 ) ) ;
#29766=VERTEX_POINT ( 'NONE', #61117 ) ;
#29767=AXIS2_PLACEMENT_3D ( 'NONE', #41486, #62629, #77049 ) ;
#29768=CARTESIAN_POINT ( 'NONE',  ( -18.00000000000000000, -4.661471528628506000, 34.16647553114623292 ) ) ;
#29769=VERTEX_POINT ( 'NONE', #26457 ) ;
#29770=CARTESIAN_POINT ( 'NONE',  ( 17.86985279056177944, -6.852621066184266141, 34.70813303252209181 ) ) ;
#29771=CARTESIAN_POINT ( 'NONE',  ( 16.85405765471943695, -2.501496062324911840, 29.88072118266895671 ) ) ;
#29773=CIRCLE ( 'NONE', #70077, 0.2500000000000002220 ) ;
#29775=CARTESIAN_POINT ( 'NONE',  ( -13.38461538461550759, -12.70778746994576025, 30.41441678777401236 ) ) ;
#29776=ORIENTED_EDGE ( 'NONE', *, *, #83633, .T. ) ;
#29778=ORIENTED_EDGE ( 'NONE', *, *, #34233, .T. ) ;
#29779=CARTESIAN_POINT ( 'NONE',  ( -10.61538461538473577, -12.16647553114689728, 32.15551576947799362 ) ) ;
#29780=CARTESIAN_POINT ( 'NONE',  ( 5.777121317571356052, -7.630691491037286056, 34.74850469731152458 ) ) ;
#29781=ORIENTED_EDGE ( 'NONE', *, *, #73173, .F. ) ;
#29782=B_SPLINE_CURVE_WITH_KNOTS ( 'NONE', 3,
 ( #7472, #62390, #83587, #14221, #40814, #1149, #34047, #54757, #82244, #28629 ),
 .UNSPECIFIED., .F., .F.,
 ( 4, 2, 2, 2, 4 ),
 ( 0.000000000000000000, 0.0001954339857564081520, 0.0003908679715128163040, 0.0005863019572692244018, 0.0007817359430256326080 ),
 .UNSPECIFIED. ) ;
#29783=B_SPLINE_CURVE_WITH_KNOTS ( 'NONE', 3,
 ( #3622, #73433, #3180, #17139, #11732, #86514, #39209, #66669, #24333, #44150 ),
 .UNSPECIFIED., .F., .F.,
 ( 4, 2, 2, 2, 4 ),
 ( 0.0007817359430256334753, 0.0009771253907250058643, 0.001172514838424371098, 0.001367904286123736764, 0.001563293733823101998 ),
 .UNSPECIFIED. ) ;
#29784=CARTESIAN_POINT ( 'NONE',  ( -6.000000000000121680, -11.06231777344772027, 33.60647404775119895 ) ) ;
#29785=CARTESIAN_POINT ( 'NONE',  ( -14.37377571864818648, -10.51840700105979387, 33.73612834413961536 ) ) ;
#29786=CARTESIAN_POINT ( 'NONE',  ( -11.66860874789975888, -2.882441371585227508, 31.66841991370172238 ) ) ;
#29787=CARTESIAN_POINT ( 'NONE',  ( 2.307692307692309264, -1.466349020453238561, 30.81389545987213907 ) ) ;
#29788=CARTESIAN_POINT ( 'NONE',  ( -4.087778820496078325, -3.937682226553329556, 33.60647404775216529 ) ) ;
#29790=EDGE_CURVE ( 'NONE', #38938, #30718, #614, .T. ) ;
#29791=EDGE_CURVE ( 'NONE', #60435, #81436, #54360, .T. ) ;
#29792=ORIENTED_EDGE ( 'NONE', *, *, #55076, .F. ) ;
#29793=VERTEX_POINT ( 'NONE', #40857 ) ;
#29794=FACE_BOUND ( 'NONE', #80644, .T. ) ;
#29795=EDGE_LOOP ( 'NONE', ( #34394, #65907, #28993, #15598 ) ) ;
#29796=CARTESIAN_POINT ( 'NONE',  ( 14.98079249982687777, -12.41269422305637171, 30.68257228309993323 ) ) ;
#29798=EDGE_CURVE ( 'NONE', #16317, #28684, #13376, .T. ) ;
#29799=CARTESIAN_POINT ( 'NONE',  ( -1.634615384615383027, -7.500000000000001776, 35.04278698407183867 ) ) ;
#29801=LINE ( 'NONE', #28925, #6145 ) ;
#29802=CARTESIAN_POINT ( 'NONE',  ( -2.242437168179467033, -10.33852847137154107, 34.16647553114620450 ) ) ;
#29803=EDGE_LOOP ( 'NONE', ( #33002, #15175, #41606, #14751 ) ) ;
#29804=EDGE_LOOP ( 'NONE', ( #76328, #75524 ) ) ;
#29805=CARTESIAN_POINT ( 'NONE',  ( -1.634592115557738312, -11.79746400365624659, 32.30657167506340954 ) ) ;
#29806=ORIENTED_EDGE ( 'NONE', *, *, #40551, .T. ) ;
#29807=CARTESIAN_POINT ( 'NONE',  ( 16.08776274289027342, -9.780366693483667717, 34.19971097300155805 ) ) ;
#29808=CARTESIAN_POINT ( 'NONE',  ( 3.164685819813350953, -2.721908614388772296, 31.22303859784724622 ) ) ;
#29809=B_SPLINE_CURVE_WITH_KNOTS ( 'NONE', 3,
 ( #4239, #45218, #11899, #66386, #46119, #72695, #65034, #3791, #3345, #37571 ),
 .UNSPECIFIED., .F., .F.,
 ( 4, 2, 2, 2, 4 ),
 ( 0.000000000000000000, 0.0001954311564186869557, 0.0003908623128373739115, 0.0005862934692560608672, 0.0007817246256747478229 ),
 .UNSPECIFIED. ) ;
#29810=CARTESIAN_POINT ( 'NONE',  ( 14.24242230713599078, -12.16647553114622049, 32.15551576947930812 ) ) ;
#29811=FACE_BOUND ( 'NONE', #11207, .T. ) ;
#29812=EDGE_LOOP ( 'NONE', ( #20705, #11890, #83210, #20176 ) ) ;
#29813=CARTESIAN_POINT ( 'NONE',  ( -8.769230769230892619, -4.320704448113951379, 33.92786785259630022 ) ) ;
#29814=CARTESIAN_POINT ( 'NONE',  ( 0.6845498131513104711, -11.76359900205217457, 32.36225158514719880 ) ) ;
#29815=VECTOR ( 'NONE', #55727, 999.9999999999998863 ) ;
#29816=CYLINDRICAL_SURFACE ( 'NONE', #9222, 0.2500000000000002220 ) ;
#29818=ORIENTED_EDGE ( 'NONE', *, *, #34363, .F. ) ;
#29819=VERTEX_POINT ( 'NONE', #53920 ) ;
#29820=ORIENTED_EDGE ( 'NONE', *, *, #36418, .T. ) ;
#29821=CARTESIAN_POINT ( 'NONE',  ( 12.46153846153846168, -6.386643153685126251, 34.62446782046654192 ) ) ;
#29822=CARTESIAN_POINT ( 'NONE',  ( 17.75000000000000000, -7.500000000000001776, 35.04278698407183867 ) ) ;
#29823=CARTESIAN_POINT ( 'NONE',  ( -8.638440328263820689, -12.35292014791297710, 31.75344720912887198 ) ) ;
#29824=CARTESIAN_POINT ( 'NONE',  ( 18.00000000000000000, -6.681629849574314051, 35.83090037661290239 ) ) ;
#29825=DIRECTION ( 'NONE',  ( -1.000000000000000000, -0.000000000000000000, -0.000000000000000000 ) ) ;
#29826=CARTESIAN_POINT ( 'NONE',  ( -15.48074597481782178, -3.436278759898153901, 33.07459398097509506 ) ) ;
#29829=CARTESIAN_POINT ( 'NONE',  ( -10.61538461538461320, -1.129524287112498415, 32.06866353760679544 ) ) ;
#29830=CARTESIAN_POINT ( 'NONE',  ( 4.376625695114563008, -9.332535724633407526, 34.40230450496446224 ) ) ;
#29831=CARTESIAN_POINT ( 'NONE',  ( 3.230769230769110045, -10.90142922262034020, 33.41473453929536674 ) ) ;
#29832=ORIENTED_EDGE ( 'NONE', *, *, #34233, .F. ) ;
#29833=CARTESIAN_POINT ( 'NONE',  ( 8.546303810323914618, -12.64616026154729411, 30.79003144601914244 ) ) ;
#29834=ORIENTED_EDGE ( 'NONE', *, *, #33915, .F. ) ;
#29835=FACE_BOUND ( 'NONE', #41529, .T. ) ;
#29836=CARTESIAN_POINT ( 'NONE',  ( 5.011652630962299959, -6.026961402152685388, 34.52809138561120506 ) ) ;
#29838=CARTESIAN_POINT ( 'NONE',  ( 8.769230769230768274, -9.905515769479276145, 34.41647553114623292 ) ) ;
#29839=ORIENTED_EDGE ( 'NONE', *, *, #5472, .T. ) ;
#29840=CARTESIAN_POINT ( 'NONE',  ( 11.60371667797437567, -11.06231777344671130, 33.60647404775212976 ) ) ;
#29841=CARTESIAN_POINT ( 'NONE',  ( -3.480745974817821775, -2.318417181685854533, 30.59732222474233865 ) ) ;
#29842=CARTESIAN_POINT ( 'NONE',  ( 8.769230769230768274, -2.292212530054420494, 30.41441678777542634 ) ) ;
#29843=CARTESIAN_POINT ( 'NONE',  ( 4.376858997939548246, -6.460100341425561332, 34.89618726649961644 ) ) ;
#29844=ORIENTED_EDGE ( 'NONE', *, *, #54862, .T. ) ;
#29845=ADVANCED_FACE ( 'NONE', ( #61555 ), #74199, .F. ) ;
#29846=CYLINDRICAL_SURFACE ( 'NONE', #12864, 0.2500000000000012212 ) ;
#29847=EDGE_LOOP ( 'NONE', ( #39405, #65015 ) ) ;
#29848=B_SPLINE_CURVE_WITH_KNOTS ( 'NONE', 3,
 ( #38697, #58068, #59412, #17990, #44542, #4006, #10337, #23394, #65268, #85998 ),
 .UNSPECIFIED., .F., .F.,
 ( 4, 2, 2, 2, 4 ),
 ( 0.000000000000000000, 0.0001954311564186860884, 0.0003908623128373721767, 0.0005862934692560582651, 0.0007817246256747443535 ),
 .UNSPECIFIED. ) ;
#29849=CARTESIAN_POINT ( 'NONE',  ( 13.38461538461538680, -12.10708131394839349, 31.69288490824020244 ) ) ;
#29850=ORIENTED_EDGE ( 'NONE', *, *, #77727, .T. ) ;
#29851=CARTESIAN_POINT ( 'NONE',  ( 9.561616225640133138, -3.530157926970578952, 32.79014554554150607 ) ) ;
#29852=CARTESIAN_POINT ( 'NONE',  ( -6.673022611438609530, -11.79725096376909299, 32.30694842903960762 ) ) ;
#29853=CARTESIAN_POINT ( 'NONE',  ( 7.596177102105253987, -10.06842814019191401, 34.32929386961144758 ) ) ;
#29854=VECTOR ( 'NONE', #88343, 1000.000000000000227 ) ;
#29855=CARTESIAN_POINT ( 'NONE',  ( -15.10072179551877802, -7.723484941389743952, 34.99544897038808955 ) ) ;
#29856=CARTESIAN_POINT ( 'NONE',  ( 0.4615384615383396616, -9.442884908241554243, 34.35708131394783038 ) ) ;
#29857=DIRECTION ( 'NONE',  ( -0.000000000000000000, 0.5000000000000011102, -0.8660254037844381525 ) ) ;
#29858=CARTESIAN_POINT ( 'NONE',  ( -9.822455662039384805, -12.15440758774515473, 32.17923288041532004 ) ) ;
#29861=AXIS2_PLACEMENT_3D ( 'NONE', #53171, #88769, #54508 ) ;
#29862=DIRECTION ( 'NONE',  ( -0.000000000000000000, -0.8660254037844399289, -0.4999999999999980016 ) ) ;
#29863=LINE ( 'NONE', #20547, #20818 ) ;
#29866=VERTEX_POINT ( 'NONE', #27777 ) ;
#29867=ORIENTED_EDGE ( 'NONE', *, *, #59037, .T. ) ;
#29868=CARTESIAN_POINT ( 'NONE',  ( 3.930919936330005360, -12.15238873228292071, 31.58232369045353849 ) ) ;
#29869=CARTESIAN_POINT ( 'NONE',  ( -5.869208192175211281, -10.54018710029568595, 33.71981072465678864 ) ) ;
#29871=CARTESIAN_POINT ( 'NONE',  ( -4.826977667545032880, -12.68172785388650681, 30.59649109432439573 ) ) ;
#29872=FACE_OUTER_BOUND ( 'NONE', #76888, .T. ) ;
#29873=CARTESIAN_POINT ( 'NONE',  ( 8.992010438208831502, -11.60474049983371003, 33.02348890104160262 ) ) ;
#29874=CARTESIAN_POINT ( 'NONE',  ( -11.53846153846153655, -6.189225973068211317, 35.74407628777942847 ) ) ;
#29875=CARTESIAN_POINT ( 'NONE',  ( 6.065144780719633921, -7.750023224968867197, 34.99404313364389907 ) ) ;
#29876=ORIENTED_EDGE ( 'NONE', *, *, #49745, .T. ) ;
#29877=B_SPLINE_CURVE_WITH_KNOTS ( 'NONE', 3,
 ( #13546, #73928, #80239, #19861, #61272, #39707, #12666, #67166, #5473, #52749 ),
 .UNSPECIFIED., .F., .F.,
 ( 4, 2, 2, 2, 4 ),
 ( 0.000000000000000000, 0.0001954311564186866034, 0.0003908623128373732067, 0.0005862934692560597830, 0.0007817246256747464135 ),
 .UNSPECIFIED. ) ;
#29880=B_SPLINE_CURVE_WITH_KNOTS ( 'NONE', 3,
 ( #107, #13179, #55047, #7754, #20814, #35214, #27132, #82087, #85183, #76652 ),
 .UNSPECIFIED., .F., .F.,
 ( 4, 2, 2, 2, 4 ),
 ( 0.0007817246256747459798, 0.0009771112852218896347, 0.001172497944769033181, 0.001367884604316176728, 0.001563271263863320491 ),
 .UNSPECIFIED. ) ;
#29881=EDGE_CURVE ( 'NONE', #48748, #43361, #44609, .T. ) ;
#29883=DIRECTION ( 'NONE',  ( 0.000000000000000000, 0.9396926207859126468, -0.3420201433256571111 ) ) ;
#29884=EDGE_LOOP ( 'NONE', ( #53317, #16408 ) ) ;
#29885=LINE ( 'NONE', #57346, #6758 ) ;
#29886=EDGE_CURVE ( 'NONE', #14701, #11434, #82736, .T. ) ;
#29888=CARTESIAN_POINT ( 'NONE',  ( 8.769230769230645706, -3.083524468854526912, 32.58852847137268327 ) ) ;
#29890=FACE_OUTER_BOUND ( 'NONE', #79397, .T. ) ;
#29891=VERTEX_POINT ( 'NONE', #41744 ) ;
#29893=DIRECTION ( 'NONE',  ( 0.000000000000000000, 0.6427876096865368094, 0.7660444431189802339 ) ) ;
#29894=AXIS2_PLACEMENT_3D ( 'NONE', #37541, #65902, #78980 ) ;
#29895=B_SPLINE_CURVE_WITH_KNOTS ( 'NONE', 3,
 ( #54199, #59187, #86690, #87578, #18665, #80818, #4700, #88470, #5140, #12782 ),
 .UNSPECIFIED., .F., .F.,
 ( 4, 2, 2, 2, 4 ),
 ( 0.000000000000000000, 0.0001954339857564071491, 0.0003908679715128142982, 0.0005863019572692214744, 0.0007817359430256285964 ),
 .UNSPECIFIED. ) ;
#29896=CARTESIAN_POINT ( 'NONE',  ( -9.626240358957616650, -3.322132147404559976, 32.92929555188717927 ) ) ;
#29897=ADVANCED_FACE ( 'NONE', ( #69210 ), #62871, .F. ) ;
#29899=VERTEX_POINT ( 'NONE', #51452 ) ;
#29901=ADVANCED_FACE ( 'NONE', ( #16372 ), #85721, .F. ) ;
#29902=ORIENTED_EDGE ( 'NONE', *, *, #12951, .F. ) ;
#29904=CARTESIAN_POINT ( 'NONE',  ( -3.230769230769351186, -12.27809138561165270, 31.22303859784587132 ) ) ;
#29906=CARTESIAN_POINT ( 'NONE',  ( -7.846153846153967493, -2.657715359629662544, 31.77849191805970364 ) ) ;
#29907=EDGE_CURVE ( 'NONE', #83302, #24853, #2837, .T. ) ;
#29908=B_SPLINE_CURVE_WITH_KNOTS ( 'NONE', 3,
 ( #36144, #55510, #69472, #14980, #8222, #1899, #35698, #64029, #29388, #63147 ),
 .UNSPECIFIED., .F., .F.,
 ( 4, 2, 2, 2, 4 ),
 ( 0.000000000000000000, 0.0001954311564186876334, 0.0003908623128373752667, 0.0005862934692560629272, 0.0007817246256747505334 ),
 .UNSPECIFIED. ) ;
#29910=DIRECTION ( 'NONE',  ( -0.000000000000000000, -0.3420201433256694901, -0.9396926207859082059 ) ) ;
#29911=VERTEX_POINT ( 'NONE', #64983 ) ;
#29912=B_SPLINE_CURVE_WITH_KNOTS ( 'NONE', 3,
 ( #27469, #14393, #54937, #81538, #20706, #61236, #69345, #7643, #440, #40553 ),
 .UNSPECIFIED., .F., .F.,
 ( 4, 2, 2, 2, 4 ),
 ( 0.0007817359430256232838, 0.0009771253907249930707, 0.001172514838424355702, 0.001367904286123718550, 0.001563293733823081181 ),
 .UNSPECIFIED. ) ;
#29914=EDGE_LOOP ( 'NONE', ( #23881, #55420, #11332, #56352 ) ) ;
#29915=ORIENTED_EDGE ( 'NONE', *, *, #50058, .T. ) ;
#29917=CARTESIAN_POINT ( 'NONE',  ( -17.07692307692307665, -3.513871655860378418, 32.76840700105978499 ) ) ;
#29918=CARTESIAN_POINT ( 'NONE',  ( 0.6845513056318556222, -6.460100341425561332, 34.89618726649961644 ) ) ;
#29919=CYLINDRICAL_SURFACE ( 'NONE', #67221, 0.2499999999999979738 ) ;
#29921=CARTESIAN_POINT ( 'NONE',  ( 5.299934428535925335, -9.886259254753566594, 34.14407573483972413 ) ) ;
#29922=VERTEX_POINT ( 'NONE', #78956 ) ;
#29924=ORIENTED_EDGE ( 'NONE', *, *, #70651, .F. ) ;
#29926=EDGE_LOOP ( 'NONE', ( #63970, #73359 ) ) ;
#29927=CARTESIAN_POINT ( 'NONE',  ( -24.00000000000000000, -5.499999999999981348, 27.75000000000000000 ) ) ;
#29928=CARTESIAN_POINT ( 'NONE',  ( -18.00000000000000000, -9.780366693483671270, 34.19971097300155094 ) ) ;
#29930=DIRECTION ( 'NONE',  ( -0.000000000000000000, -0.5000000000000009992, -0.8660254037844380415 ) ) ;
#29932=VERTEX_POINT ( 'NONE', #43837 ) ;
#29933=EDGE_LOOP ( 'NONE', ( #84824, #40680, #36384, #68121 ) ) ;
#29934=CARTESIAN_POINT ( 'NONE',  ( 5.326923076924495071, -7.500000000000154543, 35.00000000000007105 ) ) ;
#29935=ORIENTED_EDGE ( 'NONE', *, *, #33229, .T. ) ;
#29936=FACE_BOUND ( 'NONE', #22561, .T. ) ;
#29938=CARTESIAN_POINT ( 'NONE',  ( 16.15384615384603251, -6.879047030192662504, 34.71129190930017927 ) ) ;
#29939=VERTEX_POINT ( 'NONE', #76407 ) ;
#29941=CARTESIAN_POINT ( 'NONE',  ( 3.480823542407545546, -3.136992222400443175, 32.19305428654138979 ) ) ;
#29942=DIRECTION ( 'NONE',  ( -0.000000000000000000, -0.3420201433256694346, -0.9396926207859080948 ) ) ;
#29943=CARTESIAN_POINT ( 'NONE',  ( -11.53846153846165912, -6.026961402154118019, 34.52809138561165270 ) ) ;
#29944=CARTESIAN_POINT ( 'NONE',  ( 1.515405825582337718, -2.494656445102013453, 31.33466734024120015 ) ) ;
#29945=EDGE_CURVE ( 'NONE', #38377, #61168, #17251, .T. ) ;
#29946=EDGE_CURVE ( 'NONE', #25295, #55459, #58665, .T. ) ;
#29948=CARTESIAN_POINT ( 'NONE',  ( -6.857821351800898135, -9.442884908240271713, 34.35708131394835618 ) ) ;
#29949=DIRECTION ( 'NONE',  ( 0.000000000000000000, 0.7660444431189822323, -0.6427876096865344779 ) ) ;
#29950=CARTESIAN_POINT ( 'NONE',  ( -7.715628144390283438, -6.852161475712352789, 34.70806712695775786 ) ) ;
#29952=CARTESIAN_POINT ( 'NONE',  ( 5.999999999999880096, -5.219633306517616589, 34.19971097300220464 ) ) ;
#29953=DIRECTION ( 'NONE',  ( -0.000000000000000000, -0.3420201433256694346, -0.9396926207859080948 ) ) ;
#29954=CARTESIAN_POINT ( 'NONE',  ( 6.249945518348141604, -10.05730279482229683, 34.04704008940765902 ) ) ;
#29955=CARTESIAN_POINT ( 'NONE',  ( -13.63463860883684120, -4.175268141568685643, 33.81360843649122216 ) ) ;
#29956=CARTESIAN_POINT ( 'NONE',  ( 11.60371710973756620, -4.481592998940250538, 33.73612834413965089 ) ) ;
#29957=CYLINDRICAL_SURFACE ( 'NONE', #18092, 0.2500000000000008882 ) ;
#29958=DIRECTION ( 'NONE',  ( -0.000000000000000000, 0.6427876096865404731, -0.7660444431189770143 ) ) ;
#29959=CARTESIAN_POINT ( 'NONE',  ( 7.846153846153846700, -13.87047571288749737, 32.06866353760679544 ) ) ;
#29960=CYLINDRICAL_SURFACE ( 'NONE', #40504, 0.2500000000000009437 ) ;
#29962=ORIENTED_EDGE ( 'NONE', *, *, #1070, .T. ) ;
#29963=CARTESIAN_POINT ( 'NONE',  ( -3.931066484868086075, -5.827830569534415694, 34.72679350104403539 ) ) ;
#29964=EDGE_LOOP ( 'NONE', ( #25754, #10407, #24036, #20606 ) ) ;
#29965=CARTESIAN_POINT ( 'NONE',  ( -9.758391103263569732, -5.557115091759785130, 34.35708131394839171 ) ) ;
#29966=EDGE_CURVE ( 'NONE', #66348, #77080, #38253, .T. ) ;
#29968=CARTESIAN_POINT ( 'NONE',  ( 16.15384615384615330, -11.16473453929635440, 33.15142922261926373 ) ) ;
#29969=ORIENTED_EDGE ( 'NONE', *, *, #80281, .T. ) ;
#29970=CARTESIAN_POINT ( 'NONE',  ( -5.076923076923075762, -1.129524287112498415, 32.06866353760679544 ) ) ;
#29972=CARTESIAN_POINT ( 'NONE',  ( -18.00000000000012079, -9.528491918059723176, 34.59228464037033035 ) ) ;
#29973=EDGE_CURVE ( 'NONE', #61122, #29364, #70473, .T. ) ;
#29974=CARTESIAN_POINT ( 'NONE',  ( 13.60739505359344825, -3.020022701398814569, 32.48759521482552515 ) ) ;
#29975=FACE_OUTER_BOUND ( 'NONE', #25352, .T. ) ;
#29976=CARTESIAN_POINT ( 'NONE',  ( -16.15384615384627409, -10.33852847137269571, 34.16647553114546554 ) ) ;
#29977=DIRECTION ( 'NONE',  ( -0.000000000000000000, 0.9396926207859092051, -0.3420201433256662704 ) ) ;
#29978=LINE ( 'NONE', #37168, #68401 ) ;
#29980=CARTESIAN_POINT ( 'NONE',  ( 1.134638653673034181, -2.779195860258146134, 31.39871582349836032 ) ) ;
#29981=CARTESIAN_POINT ( 'NONE',  ( 11.53846153846153832, -3.886160181151819604, 36.00935417666054406 ) ) ;
#29982=B_SPLINE_CURVE_WITH_KNOTS ( 'NONE', 3,
 ( #24072, #51520, #72706, #4252, #11016, #57859, #10569, #85341, #30828, #78571 ),
 .UNSPECIFIED., .F., .F.,
 ( 4, 2, 2, 2, 4 ),
 ( 0.0007817359430256297891, 0.0009771253907249961065, 0.001172514838424362424, 0.001367904286123728741, 0.001563293733823095059 ),
 .UNSPECIFIED. ) ;
#29983=ADVANCED_FACE ( 'NONE', ( #28215 ), #55683, .F. ) ;
#29984=CARTESIAN_POINT ( 'NONE',  ( 14.37376065869474751, -3.050289026998446840, 32.03036669348366416 ) ) ;
#29987=CARTESIAN_POINT ( 'NONE',  ( -10.61538461538461320, -5.471508081941601098, 34.59228464037088457 ) ) ;
#29988=ORIENTED_EDGE ( 'NONE', *, *, #18382, .T. ) ;
#29989=CARTESIAN_POINT ( 'NONE',  ( 14.53047184896071542, -5.114059244376869984, 34.14424750095245287 ) ) ;
#29990=LINE ( 'NONE', #43938, #79067 ) ;
#29991=CARTESIAN_POINT ( 'NONE',  ( 1.134592147322421640, -12.43535235679832596, 30.55408501211184813 ) ) ;
#29992=CARTESIAN_POINT ( 'NONE',  ( 18.25005431163831204, -10.66356715214248574, 33.62249196103329751 ) ) ;
#29994=CARTESIAN_POINT ( 'NONE',  ( -8.899377978668987055, -8.587444163452046197, 34.63053765926554206 ) ) ;
#29996=EDGE_CURVE ( 'NONE', #30893, #88462, #83176, .T. ) ;
#29997=ORIENTED_EDGE ( 'NONE', *, *, #9591, .T. ) ;
#29998=CARTESIAN_POINT ( 'NONE',  ( 7.622668921589514035, -3.019605429927184836, 32.48692288466676814 ) ) ;
#29999=ORIENTED_EDGE ( 'NONE', *, *, #3732, .F. ) ;
#30001=ORIENTED_EDGE ( 'NONE', *, *, #73558, .T. ) ;
#30002=CARTESIAN_POINT ( 'NONE',  ( -11.40793610022789828, -11.66157788607254098, 32.95092075102925833 ) ) ;
#30003=CARTESIAN_POINT ( 'NONE',  ( -8.899921372341079717, -2.295517848115769421, 30.44137282052137294 ) ) ;
#30005=CARTESIAN_POINT ( 'NONE',  ( 1.607626736228236375, -11.76359900205217457, 32.36225158514719880 ) ) ;
#30006=CARTESIAN_POINT ( 'NONE',  ( 14.30769230769231015, -12.78798330534102945, 29.74999999999997868 ) ) ;
#30008=VERTEX_POINT ( 'NONE', #73090 ) ;
#30009=DIRECTION ( 'NONE',  ( -0.000000000000000000, -0.9848077530122085754, -0.1736481776669273613 ) ) ;
#30010=AXIS2_PLACEMENT_3D ( 'NONE', #24971, #38046, #11023 ) ;
#30011=ORIENTED_EDGE ( 'NONE', *, *, #5431, .T. ) ;
#30012=B_SPLINE_CURVE_WITH_KNOTS ( 'NONE', 3,
 ( #16033, #43503, #44365, #15150, #2500, #70976, #65086, #71404, #29118, #77724 ),
 .UNSPECIFIED., .F., .F.,
 ( 4, 2, 2, 2, 4 ),
 ( 0.0007817359430256297891, 0.0009771253907249958896, 0.001172514838424361990, 0.001367904286123728091, 0.001563293733823094191 ),
 .UNSPECIFIED. ) ;
#30013=EDGE_LOOP ( 'NONE', ( #62305, #22854, #41000, #27089 ) ) ;
#30015=DIRECTION ( 'NONE',  ( -0.000000000000000000, -0.9848077530122085754, -0.1736481776669273613 ) ) ;
#30016=DIRECTION ( 'NONE',  ( -1.000000000000000000, 0.000000000000000000, 0.000000000000000000 ) ) ;
#30017=EDGE_CURVE ( 'NONE', #44792, #85917, #33441, .T. ) ;
#30018=DIRECTION ( 'NONE',  ( -0.000000000000000000, -0.8660254037844397068, -0.4999999999999978906 ) ) ;
#30019=EDGE_CURVE ( 'NONE', #85805, #7785, #18794, .T. ) ;
#30020=CYLINDRICAL_SURFACE ( 'NONE', #80988, 0.2499999999999986955 ) ;
#30021=CARTESIAN_POINT ( 'NONE',  ( 7.976679284387489410, -12.70449254468099198, 30.44128974285582956 ) ) ;
#30022=ORIENTED_EDGE ( 'NONE', *, *, #39397, .T. ) ;
#30023=ORIENTED_EDGE ( 'NONE', *, *, #59300, .F. ) ;
#30025=ORIENTED_EDGE ( 'NONE', *, *, #19074, .F. ) ;
#30026=CARTESIAN_POINT ( 'NONE',  ( 4.284371855609715674, -11.46989282347013095, 32.79007818306219946 ) ) ;
#30027=VERTEX_POINT ( 'NONE', #88405 ) ;
#30028=CARTESIAN_POINT ( 'NONE',  ( 13.38461538461526423, -9.528491918059723176, 34.59228464037033035 ) ) ;
#30033=CARTESIAN_POINT ( 'NONE',  ( -14.98071481085577972, -12.41089969410671223, 31.60739465890703670 ) ) ;
#30035=ORIENTED_EDGE ( 'NONE', *, *, #43878, .T. ) ;
#30036=FACE_BOUND ( 'NONE', #30304, .T. ) ;
#30037=EDGE_CURVE ( 'NONE', #37810, #10963, #53702, .T. ) ;
#30038=CARTESIAN_POINT ( 'NONE',  ( 15.45354889974729495, -11.60474049983371003, 33.02348890104160262 ) ) ;
#30039=CARTESIAN_POINT ( 'NONE',  ( 11.53846153846153832, -13.53365097954675988, 30.81389545987213552 ) ) ;
#30040=CARTESIAN_POINT ( 'NONE',  ( 2.307692307692309264, -12.34228464037088635, 31.77849191805839268 ) ) ;
#30041=CARTESIAN_POINT ( 'NONE',  ( -39.05038313613820122, -2.249999999999998668, 29.75000000000000355 ) ) ;
#30042=CARTESIAN_POINT ( 'NONE',  ( 12.46153846153846168, -9.058645607665452459, 34.76329471203371924 ) ) ;
#30043=ADVANCED_FACE ( 'NONE', ( #52364 ), #39319, .F. ) ;
#30044=CARTESIAN_POINT ( 'NONE',  ( -0.4615384615384611200, -12.34228464037088635, 31.77849191805839268 ) ) ;
#30045=CARTESIAN_POINT ( 'NONE',  ( -10.86536134632696893, -10.66389620160130036, 33.62221079203477103 ) ) ;
#30047=CARTESIAN_POINT ( 'NONE',  ( -18.00000000000012079, -10.90142922262034020, 33.41473453929536674 ) ) ;
#30048=ORIENTED_EDGE ( 'NONE', *, *, #47370, .T. ) ;
#30050=CARTESIAN_POINT ( 'NONE',  ( -12.23852561744506495, -3.395485233115139057, 33.02377354290275946 ) ) ;
#30051=CARTESIAN_POINT ( 'NONE',  ( 15.29683758177166908, -4.098570777380720287, 33.41473453929635440 ) ) ;
#30052=CARTESIAN_POINT ( 'NONE',  ( -8.519230769230768274, -2.249999999999998668, 29.75000000000000355 ) ) ;
#30053=LINE ( 'NONE', #78679, #66323 ) ;
#30054=CARTESIAN_POINT ( 'NONE',  ( 7.846153846153723244, -6.835583212225970762, 34.95778746994575670 ) ) ;
#30055=CARTESIAN_POINT ( 'NONE',  ( 7.622668902429897919, -8.496056993536548418, 34.65000542017679663 ) ) ;
#30056=FACE_BOUND ( 'NONE', #68632, .T. ) ;
#30057=EDGE_CURVE ( 'NONE', #47121, #85711, #87517, .T. ) ;
#30058=CARTESIAN_POINT ( 'NONE',  ( 12.33084785842815378, -9.929715669179220328, 34.40415004197138416 ) ) ;
#30059=CARTESIAN_POINT ( 'NONE',  ( 1.450683735617826153, -2.538708090699994813, 30.37095296980875503 ) ) ;
#30060=CARTESIAN_POINT ( 'NONE',  ( -6.673022611438608642, -10.66356715214248396, 33.62249196103329751 ) ) ;
#30061=CARTESIAN_POINT ( 'NONE',  ( -13.38461538461550582, -6.026961402154118019, 34.52809138561165270 ) ) ;
#30062=CARTESIAN_POINT ( 'NONE',  ( 7.596153846153840483, -2.499999999999999556, 29.81609845454691765 ) ) ;
#30065=VERTEX_POINT ( 'NONE', #80753 ) ;
#30067=CARTESIAN_POINT ( 'NONE',  ( -8.096177083446809419, -11.37209801155882971, 32.91403422569032955 ) ) ;
#30069=CARTESIAN_POINT ( 'NONE',  ( 5.933917620639865831, -5.471508081941601986, 34.59228464037088457 ) ) ;
#30071=CARTESIAN_POINT ( 'NONE',  ( 7.596130608860880429, -5.056417327199099532, 34.11270091957320716 ) ) ;
#30073=EDGE_CURVE ( 'NONE', #10584, #7315, #46505, .T. ) ;
#30074=CARTESIAN_POINT ( 'NONE',  ( -8.703975197954745724, -2.892918686051626498, 31.69288490824026638 ) ) ;
#30075=DIRECTION ( 'NONE',  ( -0.000000000000000000, -0.3420201433256694901, -0.9396926207859082059 ) ) ;
#30076=AXIS2_PLACEMENT_3D ( 'NONE', #10302, #72883, #73795 ) ;
#30077=CARTESIAN_POINT ( 'NONE',  ( -8.069638770718178478, -3.019605429927184836, 32.48692288466676814 ) ) ;
#30078=CARTESIAN_POINT ( 'NONE',  ( 10.36540787133602493, -6.524016743844655686, 34.90889640711025521 ) ) ;
#30079=CARTESIAN_POINT ( 'NONE',  ( 5.326923076923079314, -2.499999999999999112, 29.81604066197450109 ) ) ;
#30080=CARTESIAN_POINT ( 'NONE',  ( 12.46153846153833911, -12.70778746994576025, 30.41441678777401236 ) ) ;
#30081=VECTOR ( 'NONE', #47130, 1000.000000000000114 ) ;
#30082=CARTESIAN_POINT ( 'NONE',  ( -18.22348494372394967, -2.847400154188068022, 31.58180166144859768 ) ) ;
#30083=AXIS2_PLACEMENT_3D ( 'NONE', #87582, #51978, #88040 ) ;
#30084=DIRECTION ( 'NONE',  ( -0.000000000000000000, 1.000000000000000000, 3.491481338843133355E-15 ) ) ;
#30085=EDGE_LOOP ( 'NONE', ( #20409, #57131, #10503, #26466 ) ) ;
#30087=CARTESIAN_POINT ( 'NONE',  ( -17.29984929443922681, -2.758268499246657068, 31.33685645148948851 ) ) ;
#30090=CARTESIAN_POINT ( 'NONE',  ( 3.361294932532797208, -11.93748526763465279, 32.05452791011430946 ) ) ;
#30091=EDGE_LOOP ( 'NONE', ( #740, #41856, #39679, #59517 ) ) ;
#30092=CARTESIAN_POINT ( 'NONE',  ( -6.923076923076922462, -9.905515769479276145, 34.41647553114623292 ) ) ;
#30093=CARTESIAN_POINT ( 'NONE',  ( 7.780883400193072674, -2.625532179533445198, 30.86335684631481513 ) ) ;
#30094=EDGE_LOOP ( 'NONE', ( #40481, #69173 ) ) ;
#30096=DIRECTION ( 'NONE',  ( -0.000000000000000000, -0.1736481776669307198, -0.9848077530122080203 ) ) ;
#30097=CARTESIAN_POINT ( 'NONE',  ( 16.15384615384603251, -10.21337939537710326, 33.94971097300076224 ) ) ;
#30099=ORIENTED_EDGE ( 'NONE', *, *, #73024, .T. ) ;
#30100=FACE_OUTER_BOUND ( 'NONE', #56735, .T. ) ;
#30102=CARTESIAN_POINT ( 'NONE',  ( -0.4615384615385826339, -6.026961402154118908, 34.52809138561165270 ) ) ;
#30103=EDGE_LOOP ( 'NONE', ( #35495, #89175, #23793, #48405 ) ) ;
#30106=ADVANCED_FACE ( 'NONE', ( #12276 ), #38419, .F. ) ;
#30107=ORIENTED_EDGE ( 'NONE', *, *, #9348, .T. ) ;
#30108=FACE_OUTER_BOUND ( 'NONE', #3149, .T. ) ;
#30111=B_SPLINE_CURVE_WITH_KNOTS ( 'NONE', 3,
 ( #29768, #37847, #36949, #23437, #9058, #44139, #78826, #31079, #86042, #63974 ),
 .UNSPECIFIED., .F., .F.,
 ( 4, 2, 2, 2, 4 ),
 ( 0.000000000000000000, 0.0001954311564186876334, 0.0003908623128373752667, 0.0005862934692560629272, 0.0007817246256747505334 ),
 .UNSPECIFIED. ) ;
#30112=CARTESIAN_POINT ( 'NONE',  ( -4.023320715612507037, -12.70449254468099198, 30.44128974285582956 ) ) ;
#30113=ADVANCED_FACE ( 'NONE', ( #39761 ), #67229, .F. ) ;
#30114=CARTESIAN_POINT ( 'NONE',  ( -17.07692307692319744, -6.879047030192662504, 34.71129190930017927 ) ) ;
#30115=ORIENTED_EDGE ( 'NONE', *, *, #43751, .F. ) ;
#30116=ORIENTED_EDGE ( 'NONE', *, *, #33870, .T. ) ;
#30117=CYLINDRICAL_SURFACE ( 'NONE', #80367, 0.2499999999999994726 ) ;
#30118=VERTEX_POINT ( 'NONE', #46936 ) ;
#30119=EDGE_CURVE ( 'NONE', #31805, #78822, #27500, .T. ) ;
#30120=CARTESIAN_POINT ( 'NONE',  ( 16.40379156322419973, -8.476813868363244353, 34.90874843262270133 ) ) ;
#30121=CIRCLE ( 'NONE', #8530, 0.2500000000000002220 ) ;
#30122=DIRECTION ( 'NONE',  ( -0.000000000000000000, -0.9396926207859093161, -0.3420201433256663259 ) ) ;
#30123=CARTESIAN_POINT ( 'NONE',  ( -8.703975629717932705, -12.70778746994558439, 30.41441678777536595 ) ) ;
#30124=VERTEX_POINT ( 'NONE', #20803 ) ;
#30126=VECTOR ( 'NONE', #11300, 999.9999999999998863 ) ;
#30127=ORIENTED_EDGE ( 'NONE', *, *, #72331, .T. ) ;
#30128=CARTESIAN_POINT ( 'NONE',  ( -8.519285250882628446, -8.433404298154334455, 34.66254593164985920 ) ) ;
#30130=VECTOR ( 'NONE', #51666, 1000.000000000000227 ) ;
#30131=DIRECTION ( 'NONE',  ( -0.000000000000000000, 0.9848077530122085754, -0.1736481776669273613 ) ) ;
#30132=CARTESIAN_POINT ( 'NONE',  ( -5.076923076923075762, -9.780366693483667717, 34.19971097300155094 ) ) ;
#30133=VERTEX_POINT ( 'NONE', #14489 ) ;
#30134=B_SPLINE_CURVE_WITH_KNOTS ( 'NONE', 3,
 ( #84628, #28795, #57137, #21132, #22903, #50369, #77848, #869, #28334, #21579 ),
 .UNSPECIFIED., .F., .F.,
 ( 4, 2, 2, 2, 4 ),
 ( 0.0007817246256747459798, 0.0009771112852218896347, 0.001172497944769033181, 0.001367884604316176728, 0.001563271263863320491 ),
 .UNSPECIFIED. ) ;
#30135=CARTESIAN_POINT ( 'NONE',  ( 15.36129493253279499, -3.285477652293413264, 32.44071101563363158 ) ) ;
#30136=B_SPLINE_CURVE_WITH_KNOTS ( 'NONE', 3,
 ( #81241, #59622, #11441, #7688, #67278, #26726, #74927, #25399, #11895, #25847 ),
 .UNSPECIFIED., .F., .F.,
 ( 4, 2, 2, 2, 4 ),
 ( 0.000000000000000000, 0.0001954339857564054144, 0.0003908679715128108288, 0.0005863019572692162703, 0.0007817359430256216575 ),
 .UNSPECIFIED. ) ;
#30137=CARTESIAN_POINT ( 'NONE',  ( 5.142991427925513115, -11.16473453929635440, 33.15142922261926373 ) ) ;
#30138=CARTESIAN_POINT ( 'NONE',  ( -8.992715693795098275, -12.11044203135681840, 32.26167407432752299 ) ) ;
#30139=FACE_BOUND ( 'NONE', #74338, .T. ) ;
#30140=EDGE_CURVE ( 'NONE', #18183, #26741, #83339, .T. ) ;
#30141=CARTESIAN_POINT ( 'NONE',  ( -9.442362282929650519, -4.176053281294518804, 33.81426240980091791 ) ) ;
#30142=CARTESIAN_POINT ( 'NONE',  ( -6.700297254098854793, -9.418065098278011860, 34.63729479722530158 ) ) ;
#30143=CARTESIAN_POINT ( 'NONE',  ( 8.545745825506822158, -2.599994579823202923, 30.74605699353653776 ) ) ;
#30144=CARTESIAN_POINT ( 'NONE',  ( 3.361559671736182864, -3.338503747796865984, 32.95102852606552801 ) ) ;
#30145=CYLINDRICAL_SURFACE ( 'NONE', #30320, 0.2499999999999994726 ) ;
#30147=DIRECTION ( 'NONE',  ( -0.000000000000000000, 0.1736481776669307198, -0.9848077530122080203 ) ) ;
#30148=ORIENTED_EDGE ( 'NONE', *, *, #30391, .T. ) ;
#30149=CARTESIAN_POINT ( 'NONE',  ( 10.48469314871706182, -10.54014554554150607, 33.71984207302941883 ) ) ;
#30151=ORIENTED_EDGE ( 'NONE', *, *, #87128, .T. ) ;
#30152=CARTESIAN_POINT ( 'NONE',  ( 9.442307692307679190, -2.249999999999998668, 29.81609741502487765 ) ) ;
#30153=CARTESIAN_POINT ( 'NONE',  ( 15.00784227186237807, -2.889293201056495786, 32.26117774369186009 ) ) ;
#30154=EDGE_CURVE ( 'NONE', #17995, #56514, #52217, .T. ) ;
#30155=CARTESIAN_POINT ( 'NONE',  ( 11.40831356872984514, -8.630895178749533159, 34.87696386517710323 ) ) ;
#30156=FACE_OUTER_BOUND ( 'NONE', #29197, .T. ) ;
#30158=CARTESIAN_POINT ( 'NONE',  ( -2.307692307692305711, -11.35647404775217417, 33.31231777344666511 ) ) ;
#30159=VERTEX_POINT ( 'NONE', #48270 ) ;
#30160=CARTESIAN_POINT ( 'NONE',  ( 4.403900573759605308, -4.818054556918156095, 34.26375889529406749 ) ) ;
#30161=EDGE_CURVE ( 'NONE', #41440, #10893, #55408, .T. ) ;
#30162=EDGE_CURVE ( 'NONE', #80250, #53882, #49608, .T. ) ;
#30163=CARTESIAN_POINT ( 'NONE',  ( 14.24160992833217243, -12.62096338111211580, 30.90682066428152908 ) ) ;
#30166=DIRECTION ( 'NONE',  ( -0.000000000000000000, 1.000000000000000000, 3.491481338843133355E-15 ) ) ;
#30167=AXIS2_PLACEMENT_3D ( 'NONE', #37930, #22201, #85676 ) ;
#30169=EDGE_LOOP ( 'NONE', ( #17716, #61080, #56401, #37772 ) ) ;
#30171=CARTESIAN_POINT ( 'NONE',  ( 14.08476534878545650, -12.38737895849757820, 31.66785238281580206 ) ) ;
#30173=CARTESIAN_POINT ( 'NONE',  ( -6.923076923076922462, -2.538708090699994813, 30.37095296980875503 ) ) ;
#30174=DIRECTION ( 'NONE',  ( -0.000000000000000000, -0.3420201433256694901, -0.9396926207859082059 ) ) ;
#30175=CARTESIAN_POINT ( 'NONE',  ( 14.53047184896072075, -2.847695495035523550, 31.58253572463339154 ) ) ;
#30176=DIRECTION ( 'NONE',  ( 0.000000000000000000, 0.6427876096865368094, 0.7660444431189802339 ) ) ;
#30178=ADVANCED_FACE ( 'NONE', ( #6843 ), #27566, .F. ) ;
#30180=ORIENTED_EDGE ( 'NONE', *, *, #62429, .F. ) ;
#30181=CARTESIAN_POINT ( 'NONE',  ( -1.384615384615383471, -9.584722331328613620, 36.20867863119891439 ) ) ;
#30182=CARTESIAN_POINT ( 'NONE',  ( -16.37677237136229991, -11.76352882383564769, 32.36236540154569497 ) ) ;
#30183=EDGE_LOOP ( 'NONE', ( #63973, #69983 ) ) ;
#30184=DIRECTION ( 'NONE',  ( -0.000000000000000000, 1.000000000000000000, 3.491481338843133355E-15 ) ) ;
#30185=CARTESIAN_POINT ( 'NONE',  ( 3.480823542407545990, -2.779044189368095719, 31.39831045268885745 ) ) ;
#30186=B_SPLINE_CURVE_WITH_KNOTS ( 'NONE', 3,
 ( #59460, #31540, #86963, #59006, #86504, #80180, #73425, #11725, #13489, #61220 ),
 .UNSPECIFIED., .F., .F.,
 ( 4, 2, 2, 2, 4 ),
 ( 0.0007817359430256294638, 0.0009771253907249941549, 0.001172514838424358954, 0.001367904286123723754, 0.001563293733823095492 ),
 .UNSPECIFIED. ) ;
#30187=B_SPLINE_CURVE_WITH_KNOTS ( 'NONE', 3,
 ( #44023, #71493, #35958, #50331, #16121, #9371 ),
 .UNSPECIFIED., .F., .F.,
 ( 4, 2, 4 ),
 ( 0.0003909512603273901832, 0.0005862562993132176088, 0.0007815613382990449802 ),
 .UNSPECIFIED. ) ;
#30188=EDGE_CURVE ( 'NONE', #1645, #54361, #47922, .T. ) ;
#30189=EDGE_CURVE ( 'NONE', #49069, #4865, #63909, .T. ) ;
#30190=CARTESIAN_POINT ( 'NONE',  ( 11.47319109250076430, -4.481592998940162609, 33.73612834413957984 ) ) ;
#30191=CARTESIAN_POINT ( 'NONE',  ( 9.692307692307695177, -11.33034616979429110, 35.88435417666054406 ) ) ;
#30192=AXIS2_PLACEMENT_3D ( 'NONE', #82982, #72771, #4322 ) ;
#30193=CARTESIAN_POINT ( 'NONE',  ( 4.153846153846154188, -6.435427911321262684, 35.78748833219616898 ) ) ;
#30194=CARTESIAN_POINT ( 'NONE',  ( -7.911424292114620727, -12.46129190929999986, 30.37095296980880832 ) ) ;
#30196=ORIENTED_EDGE ( 'NONE', *, *, #73424, .F. ) ;
#30198=CARTESIAN_POINT ( 'NONE',  ( 2.307692307692309264, -2.249999999999998668, 29.75000000000001776 ) ) ;
#30199=CARTESIAN_POINT ( 'NONE',  ( -13.60754160213153163, -9.086856451489515152, 34.49173150075333183 ) ) ;
#30203=CARTESIAN_POINT ( 'NONE',  ( -13.63463862190834952, -12.43535235679832596, 30.55408501211184813 ) ) ;
#30204=CARTESIAN_POINT ( 'NONE',  ( -17.07692307692307665, -2.538708090699994813, 30.37095296980875503 ) ) ;
#30207=CARTESIAN_POINT ( 'NONE',  ( 12.21153846153846168, -2.499999999999998668, 29.75000000000000355 ) ) ;
#30208=VECTOR ( 'NONE', #46910, 1000.000000000000114 ) ;
#30209=ORIENTED_EDGE ( 'NONE', *, *, #10027, .T. ) ;
#30211=CARTESIAN_POINT ( 'NONE',  ( -4.403822897894745125, -8.347322224742351082, 34.93158281831414769 ) ) ;
#30212=VECTOR ( 'NONE', #60561, 1000.000000000000227 ) ;
#30213=ORIENTED_EDGE ( 'NONE', *, *, #61282, .F. ) ;
#30215=CARTESIAN_POINT ( 'NONE',  ( 4.088575707885378385, -3.835265460703609186, 33.15142922261924241 ) ) ;
#30216=CARTESIAN_POINT ( 'NONE',  ( -0.5922290646487698984, -9.929715669179220328, 34.40415004197138416 ) ) ;
#30217=CARTESIAN_POINT ( 'NONE',  ( -12.39547112818838492, -10.67929555188718282, 33.92786785259544757 ) ) ;
#30218=EDGE_LOOP ( 'NONE', ( #88824, #40444, #81645, #9788 ) ) ;
#30219=CARTESIAN_POINT ( 'NONE',  ( -9.019230769230768274, -2.249999999999998668, 29.75000000000000355 ) ) ;
#30220=EDGE_CURVE ( 'NONE', #47096, #998, #80153, .T. ) ;
#30221=ORIENTED_EDGE ( 'NONE', *, *, #36171, .T. ) ;
#30222=CARTESIAN_POINT ( 'NONE',  ( 2.437737470527086892, -2.504778602574659896, 29.97347330155780298 ) ) ;
#30223=CYLINDRICAL_SURFACE ( 'NONE', #10984, 0.2500000000000008882 ) ;
#30224=VERTEX_POINT ( 'NONE', #56801 ) ;
#30225=CARTESIAN_POINT ( 'NONE',  ( -6.222926958906846551, -10.77366814457252175, 33.85459836347579454 ) ) ;
#30226=DIRECTION ( 'NONE',  ( -0.000000000000000000, 0.1736481776669307198, -0.9848077530122080203 ) ) ;
#30227=CARTESIAN_POINT ( 'NONE',  ( -11.60373153901786125, -3.083524468853724443, 32.58852847137143272 ) ) ;
#30228=CARTESIAN_POINT ( 'NONE',  ( 13.63466980452883881, -12.01375889529407281, 32.43194544308182969 ) ) ;
#30229=CYLINDRICAL_SURFACE ( 'NONE', #75634, 0.2500000000000009437 ) ;
#30232=FACE_BOUND ( 'NONE', #21927, .T. ) ;
#30234=CARTESIAN_POINT ( 'NONE',  ( 15.16468581981334829, -12.37446782046654192, 30.86335684631486487 ) ) ;
#30235=AXIS2_PLACEMENT_3D ( 'NONE', #54094, #68074, #28402 ) ;
#30236=CYLINDRICAL_SURFACE ( 'NONE', #70888, 0.2499999999999998890 ) ;
#30237=CARTESIAN_POINT ( 'NONE',  ( -2.307692307692305711, -9.905515769479276145, 34.41647553114623292 ) ) ;
#30239=B_SPLINE_CURVE_WITH_KNOTS ( 'NONE', 3,
 ( #45636, #86650, #38442, #37536, #31690, #78976, #57370, #65003, #3312, #85743 ),
 .UNSPECIFIED., .F., .F.,
 ( 4, 2, 2, 2, 4 ),
 ( 0.0007817359430256388964, 0.0009771253907250073822, 0.001172514838424375868, 0.001367904286123744571, 0.001563293733823113056 ),
 .UNSPECIFIED. ) ;
#30240=VERTEX_POINT ( 'NONE', #72091 ) ;
#30241=EDGE_CURVE ( 'NONE', #33427, #2097, #7077, .T. ) ;
#30242=ORIENTED_EDGE ( 'NONE', *, *, #43074, .T. ) ;
#30243=CARTESIAN_POINT ( 'NONE',  ( 3.453780582382079967, -4.887748414852789658, 34.01359900205216746 ) ) ;
#30244=EDGE_LOOP ( 'NONE', ( #3552, #30713, #39357, #74415 ) ) ;
#30245=CARTESIAN_POINT ( 'NONE',  ( 15.93091993633000136, -9.886141570436013382, 34.14413921362392301 ) ) ;
#30246=VECTOR ( 'NONE', #19627, 1000.000000000000000 ) ;
#30247=CARTESIAN_POINT ( 'NONE',  ( -5.999999999999998224, -9.584722331328613620, 36.20867863119891439 ) ) ;
#30248=CARTESIAN_POINT ( 'NONE',  ( -11.53846153846153655, -12.62096338111211580, 30.90682066428153263 ) ) ;
#30249=FACE_BOUND ( 'NONE', #3640, .T. ) ;
#30251=CARTESIAN_POINT ( 'NONE',  ( 13.31853300525524908, -10.67929555188718460, 33.92786785259543336 ) ) ;
#30252=AXIS2_PLACEMENT_3D ( 'NONE', #68583, #129, #69471 ) ;
#30253=CARTESIAN_POINT ( 'NONE',  ( 10.61538461538461675, -2.499999999999998668, 29.75000000000001421 ) ) ;
#30254=CARTESIAN_POINT ( 'NONE',  ( -14.43783951713053249, -9.418419913701741919, 34.36755862841477693 ) ) ;
#30255=CARTESIAN_POINT ( 'NONE',  ( 11.53846153846141753, -8.613356846316285953, 34.62446782046622218 ) ) ;
#30256=EDGE_LOOP ( 'NONE', ( #4509, #10182 ) ) ;
#30257=EDGE_CURVE ( 'NONE', #23024, #30665, #59615, .T. ) ;
#30259=ORIENTED_EDGE ( 'NONE', *, *, #84287, .T. ) ;
#30260=EDGE_CURVE ( 'NONE', #47846, #81242, #9075, .T. ) ;
#30262=EDGE_LOOP ( 'NONE', ( #79648, #74371 ) ) ;
#30263=DIRECTION ( 'NONE',  ( -0.000000000000000000, -0.6427876096865404731, -0.7660444431189771253 ) ) ;
#30264=CARTESIAN_POINT ( 'NONE',  ( 4.153846153846154188, -5.557115091759785130, 34.35708131394839171 ) ) ;
#30265=CARTESIAN_POINT ( 'NONE',  ( 15.90382291655318880, -5.851115903089112003, 34.47074536777953568 ) ) ;
#30267=CARTESIAN_POINT ( 'NONE',  ( -18.25002322422145440, -5.765609946408404518, 34.70566812827425451 ) ) ;
#30268=CARTESIAN_POINT ( 'NONE',  ( -15.23076923076922995, -12.29105614889573062, 35.45975837776705220 ) ) ;
#30269=ORIENTED_EDGE ( 'NONE', *, *, #75639, .T. ) ;
#30273=DIRECTION ( 'NONE',  ( -0.000000000000000000, 0.6427876096865404731, -0.7660444431189771253 ) ) ;
#30274=CARTESIAN_POINT ( 'NONE',  ( 13.16168916709923664, -12.39988816332205701, 30.74660775122750778 ) ) ;
#30275=ORIENTED_EDGE ( 'NONE', *, *, #8581, .F. ) ;
#30276=EDGE_LOOP ( 'NONE', ( #88058, #6652 ) ) ;
#30277=FACE_BOUND ( 'NONE', #83141, .T. ) ;
#30278=CARTESIAN_POINT ( 'NONE',  ( 11.53846153846153832, -6.435427911321262684, 35.78748833219616898 ) ) ;
#30279=CARTESIAN_POINT ( 'NONE',  ( 12.46153846153833911, -12.27809138561165270, 31.22303859784587132 ) ) ;
#30280=ORIENTED_EDGE ( 'NONE', *, *, #77378, .F. ) ;
#30281=CARTESIAN_POINT ( 'NONE',  ( -16.15384615384615330, -11.35647404775217417, 33.31231777344666511 ) ) ;
#30282=CARTESIAN_POINT ( 'NONE',  ( 6.223012844093396723, -11.43677907613344757, 33.22367315496201456 ) ) ;
#30284=CARTESIAN_POINT ( 'NONE',  ( 4.219101293358989757, -6.835583212224609184, 34.95778746994559327 ) ) ;
#30285=ORIENTED_EDGE ( 'NONE', *, *, #11072, .F. ) ;
#30286=FACE_OUTER_BOUND ( 'NONE', #21920, .T. ) ;
#30287=ORIENTED_EDGE ( 'NONE', *, *, #3762, .F. ) ;
#30289=EDGE_LOOP ( 'NONE', ( #72248, #30151, #2706, #67470 ) ) ;
#30290=CARTESIAN_POINT ( 'NONE',  ( -8.638705067467212118, -10.19071101563364756, 33.96452234770658407 ) ) ;
#30291=CARTESIAN_POINT ( 'NONE',  ( 15.16549878480845770, -2.892918686051582533, 31.69288490824015980 ) ) ;
#30292=CARTESIAN_POINT ( 'NONE',  ( -11.53846153846166089, -2.657715359629662544, 31.77849191805970364 ) ) ;
#30293=ADVANCED_FACE ( 'NONE', ( #36966 ), #63558, .F. ) ;
#30294=DIRECTION ( 'NONE',  ( -0.000000000000000000, 0.7660444431189791237, -0.6427876096865379196 ) ) ;
#30296=CARTESIAN_POINT ( 'NONE',  ( -9.757577692864012775, -12.16647553114622049, 32.15551576947930812 ) ) ;
#30297=VECTOR ( 'NONE', #24312, 999.9999999999998863 ) ;
#30299=ORIENTED_EDGE ( 'NONE', *, *, #14678, .F. ) ;
#30300=CARTESIAN_POINT ( 'NONE',  ( -0.4615384615384611200, -5.557115091759785130, 34.35708131394839171 ) ) ;
#30301=CARTESIAN_POINT ( 'NONE',  ( 13.16178728698051081, -7.369209533119137845, 34.99857337881830688 ) ) ;
#30302=ORIENTED_EDGE ( 'NONE', *, *, #67457, .F. ) ;
#30304=EDGE_LOOP ( 'NONE', ( #22633, #84850 ) ) ;
#30305=CARTESIAN_POINT ( 'NONE',  ( 17.01165263096229907, -5.219633306516282545, 34.19971097300152252 ) ) ;
#30306=CARTESIAN_POINT ( 'NONE',  ( 12.52679360105129724, -4.320704448112861584, 33.92786785259548310 ) ) ;
#30308=CARTESIAN_POINT ( 'NONE',  ( 9.442284455014730682, -12.43535235679832596, 30.55408501211184813 ) ) ;
#30309=LINE ( 'NONE', #57778, #71860 ) ;
#30310=CYLINDRICAL_SURFACE ( 'NONE', #26975, 0.2500000000000008882 ) ;
#30311=CARTESIAN_POINT ( 'NONE',  ( 5.750000000000002665, -7.500000000000001776, 35.00000000000000000 ) ) ;
#30313=CARTESIAN_POINT ( 'NONE',  ( 6.249945518348142492, -10.76462480002816235, 33.53768742498949962 ) ) ;
#30314=CARTESIAN_POINT ( 'NONE',  ( -0.2387589202700521329, -8.496831190052095195, 34.64984203495477288 ) ) ;
#30315=B_SPLINE_CURVE_WITH_KNOTS ( 'NONE', 3,
 ( #68397, #48118, #54887, #33732, #66630, #81042, #47234, #6695, #13015, #87816 ),
 .UNSPECIFIED., .F., .F.,
 ( 4, 2, 2, 2, 4 ),
 ( 0.0007817246256747444619, 0.0009771112852218868158, 0.001172497944769029061, 0.001367884604316171523, 0.001563271263863313769 ),
 .UNSPECIFIED. ) ;
#30316=CARTESIAN_POINT ( 'NONE',  ( -6.000000000000119904, -6.026961402154118908, 34.52809138561165270 ) ) ;
#30317=CARTESIAN_POINT ( 'NONE',  ( 8.096208157792164073, -2.779044189368097495, 31.39831045268886456 ) ) ;
#30318=ORIENTED_EDGE ( 'NONE', *, *, #16746, .T. ) ;
#30319=CARTESIAN_POINT ( 'NONE',  ( -7.846153846153965716, -8.613356846316285953, 34.62446782046622218 ) ) ;
#30320=AXIS2_PLACEMENT_3D ( 'NONE', #64796, #78768, #65248 ) ;
#30322=VERTEX_POINT ( 'NONE', #37411 ) ;
#30323=CARTESIAN_POINT ( 'NONE',  ( -17.07692307692319744, -2.657715359629662988, 31.77849191805970364 ) ) ;
#30324=CARTESIAN_POINT ( 'NONE',  ( -3.230769230769351186, -2.892918686052166066, 31.69288490824153470 ) ) ;
#30325=FACE_OUTER_BOUND ( 'NONE', #18837, .T. ) ;
#30326=ORIENTED_EDGE ( 'NONE', *, *, #75306, .T. ) ;
#30327=CARTESIAN_POINT ( 'NONE',  ( 5.750023269057647823, -9.943427161483782584, 34.11278801902876978 ) ) ;
#30328=CARTESIAN_POINT ( 'NONE',  ( -10.48485891362104994, -10.88167719472716399, 33.43325721877153711 ) ) ;
#30329=VECTOR ( 'NONE', #43351, 1000.000000000000114 ) ;
#30330=CARTESIAN_POINT ( 'NONE',  ( -17.20748366866499879, -2.504760397472873823, 29.97295953869789997 ) ) ;
#30332=CARTESIAN_POINT ( 'NONE',  ( -12.46153846153846168, -10.51840700105979565, 33.73612834413961536 ) ) ;
#30334=CARTESIAN_POINT ( 'NONE',  ( 16.40390057375961064, -10.06805714834173138, 34.32951233291982618 ) ) ;
#30335=ORIENTED_EDGE ( 'NONE', *, *, #30653, .T. ) ;
#30336=DIRECTION ( 'NONE',  ( 0.000000000000000000, 0.9396926207859126468, 0.3420201433256571111 ) ) ;
#30337=CARTESIAN_POINT ( 'NONE',  ( 9.019285189144222059, -9.233818618650603938, 34.70587769442853698 ) ) ;
#30338=CARTESIAN_POINT ( 'NONE',  ( 7.846153846153723244, -2.657715359629662544, 31.77849191805970364 ) ) ;
#30339=CARTESIAN_POINT ( 'NONE',  ( -5.076923076923075762, -8.120952969808772792, 34.71129190930000163 ) ) ;
#30340=CARTESIAN_POINT ( 'NONE',  ( -7.596153846152425615, -7.500000000000154543, 35.00000000000007105 ) ) ;
#30341=ORIENTED_EDGE ( 'NONE', *, *, #20694, .T. ) ;
#30343=B_SPLINE_CURVE_WITH_KNOTS ( 'NONE', 3,
 ( #60588, #48401, #54267, #6544, #26370, #34005 ),
 .UNSPECIFIED., .F., .F.,
 ( 4, 2, 4 ),
 ( 5.307410501141271501E-17, 0.0001954756301637260456, 0.0003909512603273990194 ),
 .UNSPECIFIED. ) ;
#30344=AXIS2_PLACEMENT_3D ( 'NONE', #54131, #47382, #13164 ) ;
#30345=B_SPLINE_CURVE_WITH_KNOTS ( 'NONE', 3,
 ( #80742, #40635, #81616, #54123, #14479, #33861, #81, #68104, #55027, #12710 ),
 .UNSPECIFIED., .F., .F.,
 ( 4, 2, 2, 2, 4 ),
 ( 0.000000000000000000, 0.0001954339857564073388, 0.0003908679715128146777, 0.0005863019572692220165, 0.0007817359430256293554 ),
 .UNSPECIFIED. ) ;
#30347=ORIENTED_EDGE ( 'NONE', *, *, #26788, .F. ) ;
#30348=CARTESIAN_POINT ( 'NONE',  ( -10.36533030374629760, -8.303483539816728154, 34.68545999027711702 ) ) ;
#30349=DIRECTION ( 'NONE',  ( -0.000000000000000000, -0.7660444431189791237, -0.6427876096865379196 ) ) ;
#30350=VECTOR ( 'NONE', #2911, 1000.000000000000114 ) ;
#30351=CARTESIAN_POINT ( 'NONE',  ( -15.16470087976679615, -8.973038597847271092, 34.52809138561121216 ) ) ;
#30352=DIRECTION ( 'NONE',  ( -0.000000000000000000, -0.6427876096865404731, -0.7660444431189770143 ) ) ;
#30353=CARTESIAN_POINT ( 'NONE',  ( -23.00000000000000000, -9.499999999999982236, 27.25000000000000000 ) ) ;
#30354=CARTESIAN_POINT ( 'NONE',  ( 8.519254038288416098, -9.148715823498378086, 34.47080413974185120 ) ) ;
#30355=ADVANCED_FACE ( 'NONE', ( #29345 ), #78400, .F. ) ;
#30356=DIRECTION ( 'NONE',  ( 0.000000000000000000, 1.000000000000000000, 0.000000000000000000 ) ) ;
#30358=VERTEX_POINT ( 'NONE', #43298 ) ;
#30360=ORIENTED_EDGE ( 'NONE', *, *, #37624, .F. ) ;
#30363=CARTESIAN_POINT ( 'NONE',  ( 0.5267940328144846696, -8.613356846314930593, 34.62446782046653482 ) ) ;
#30364=CYLINDRICAL_SURFACE ( 'NONE', #70735, 0.2499999999999986955 ) ;
#30368=CIRCLE ( 'NONE', #37559, 0.2500000000000002220 ) ;
#30369=EDGE_CURVE ( 'NONE', #42722, #12295, #17144, .T. ) ;
#30370=VERTEX_POINT ( 'NONE', #78842 ) ;
#30371=CARTESIAN_POINT ( 'NONE',  ( -11.53846153846166089, -12.16647553114689728, 32.15551576947799362 ) ) ;
#30372=ORIENTED_EDGE ( 'NONE', *, *, #35682, .F. ) ;
#30373=FACE_BOUND ( 'NONE', #7674, .T. ) ;
#30375=AXIS2_PLACEMENT_3D ( 'NONE', #78458, #38373, #65826 ) ;
#30376=CARTESIAN_POINT ( 'NONE',  ( 15.93036121012220541, -6.760086850603066466, 34.69517049084099369 ) ) ;
#30377=EDGE_LOOP ( 'NONE', ( #28517, #9843, #58282, #17273 ) ) ;
#30379=DIRECTION ( 'NONE',  ( 0.000000000000000000, 0.000000000000000000, 1.000000000000000000 ) ) ;
#30380=DIRECTION ( 'NONE',  ( -0.000000000000000000, 0.6427876096865404731, -0.7660444431189771253 ) ) ;
#30381=ORIENTED_EDGE ( 'NONE', *, *, #19290, .F. ) ;
#30382=CARTESIAN_POINT ( 'NONE',  ( 9.692307692307695177, -7.500000000000001776, 35.04278698407183867 ) ) ;
#30383=CARTESIAN_POINT ( 'NONE',  ( -13.25408968285181821, -11.93748526763465279, 32.05452791011430946 ) ) ;
#30384=ORIENTED_EDGE ( 'NONE', *, *, #59236, .T. ) ;
#30385=CARTESIAN_POINT ( 'NONE',  ( 3.296837581771669523, -8.120952969808772792, 34.71129190929999453 ) ) ;
#30386=CARTESIAN_POINT ( 'NONE',  ( 7.053867364043873600, -2.494656445102013453, 31.33466734024120015 ) ) ;
#30387=CARTESIAN_POINT ( 'NONE',  ( -12.46153846153846168, -12.78798330534102945, 29.74999999999997868 ) ) ;
#30388=CARTESIAN_POINT ( 'NONE',  ( -16.02305434602136103, -8.147973898785416225, 34.70805048591653730 ) ) ;
#30389=CARTESIAN_POINT ( 'NONE',  ( -8.546451227962359454, -9.332535724633409302, 34.40230450496446934 ) ) ;
#30390=CARTESIAN_POINT ( 'NONE',  ( -18.13014720943822056, -6.852621066184265253, 34.70813303252209181 ) ) ;
#30391=EDGE_CURVE ( 'NONE', #221, #47746, #72641, .T. ) ;
#30392=CARTESIAN_POINT ( 'NONE',  ( 8.096208266067296933, -2.920487667080175598, 32.31805714834170828 ) ) ;
#30394=CARTESIAN_POINT ( 'NONE',  ( 7.173022441425065843, -3.202959910592335202, 32.30730279482227019 ) ) ;
#30396=CARTESIAN_POINT ( 'NONE',  ( 12.59158589678891715, -7.723484941389743952, 34.99544897038808955 ) ) ;
#30397=CARTESIAN_POINT ( 'NONE',  ( 12.46153846153833911, -5.094484230521993062, 34.41647553114689373 ) ) ;
#30398=EDGE_CURVE ( 'NONE', #52292, #29866, #59717, .T. ) ;
#30399=LINE ( 'NONE', #49775, #8857 ) ;
#30404=EDGE_LOOP ( 'NONE', ( #8559, #12069, #54275, #68797 ) ) ;
#30405=CARTESIAN_POINT ( 'NONE',  ( 9.561616225640134914, -6.413092428213692742, 34.63065189839063152 ) ) ;
#30406=EDGE_CURVE ( 'NONE', #84690, #28560, #68339, .T. ) ;
#30407=ORIENTED_EDGE ( 'NONE', *, *, #17151, .F. ) ;
#30409=CARTESIAN_POINT ( 'NONE',  ( -13.38461538461550759, -2.379036618888197729, 30.90682066428292885 ) ) ;
#30413=LINE ( 'NONE', #36725, #57328 ) ;
#30414=CARTESIAN_POINT ( 'NONE',  ( 6.923076923076802558, -11.48612834414049644, 32.76840700105863391 ) ) ;
#30416=CARTESIAN_POINT ( 'NONE',  ( -14.55771553191376633, -10.92453946501458795, 33.72985991061850086 ) ) ;
#30417=CARTESIAN_POINT ( 'NONE',  ( 7.846153846153846700, -7.500000000000001776, 35.04278698407183867 ) ) ;
#30418=CARTESIAN_POINT ( 'NONE',  ( 15.10015887114470523, -7.722926236386453702, 34.74524107206102030 ) ) ;
#30421=CARTESIAN_POINT ( 'NONE',  ( -10.61538461538461320, -2.721908614388771852, 31.22303859784724978 ) ) ;
#30422=CARTESIAN_POINT ( 'NONE',  ( 14.30769230769231015, -10.51840700105979565, 33.73612834413961536 ) ) ;
#30424=CARTESIAN_POINT ( 'NONE',  ( 13.38461538461526601, -4.481592998941358097, 33.73612834414048933 ) ) ;
#30426=EDGE_LOOP ( 'NONE', ( #40212, #74806 ) ) ;
#30427=CARTESIAN_POINT ( 'NONE',  ( -13.60754234352223335, -6.459968553980841577, 34.89616026154728701 ) ) ;
#30429=CARTESIAN_POINT ( 'NONE',  ( -39.05038313613820122, -2.249999999999998668, 29.75000000000000355 ) ) ;
#30430=CARTESIAN_POINT ( 'NONE',  ( 18.24994551834813805, -10.76462480002816413, 33.53768742498949962 ) ) ;
#30431=CARTESIAN_POINT ( 'NONE',  ( 15.45373213433071768, -7.369474270740069777, 34.74850911626239736 ) ) ;
#30432=LINE ( 'NONE', #63328, #58650 ) ;
#30433=EDGE_CURVE ( 'NONE', #61908, #10320, #73880, .T. ) ;
#30434=ORIENTED_EDGE ( 'NONE', *, *, #83886, .F. ) ;
#30437=EDGE_LOOP ( 'NONE', ( #31973, #70197, #15759, #72993 ) ) ;
#30440=LINE ( 'NONE', #36322, #61414 ) ;
#30441=CARTESIAN_POINT ( 'NONE',  ( -15.23076923076935252, -11.06231777344772027, 33.60647404775119895 ) ) ;
#30442=CARTESIAN_POINT ( 'NONE',  ( 1.515141086378952062, -11.93748526763465279, 32.05452791011430946 ) ) ;
#30443=CARTESIAN_POINT ( 'NONE',  ( 6.000000000000001776, -8.318370150425687726, 35.83090037661290239 ) ) ;
#30444=EDGE_CURVE ( 'NONE', #77110, #12785, #7818, .T. ) ;
#30445=VERTEX_POINT ( 'NONE', #5422 ) ;
#30447=ORIENTED_EDGE ( 'NONE', *, *, #43658, .F. ) ;
#30448=EDGE_LOOP ( 'NONE', ( #69098, #87420 ) ) ;
#30449=CARTESIAN_POINT ( 'NONE',  ( 13.16168842570853492, -4.762599654559228846, 34.23009711892697737 ) ) ;
#30450=CARTESIAN_POINT ( 'NONE',  ( 8.545745825506823934, -2.847400154188068022, 31.58180166144859058 ) ) ;
#30451=FACE_OUTER_BOUND ( 'NONE', #85516, .T. ) ;
#30452=EDGE_CURVE ( 'NONE', #54595, #28559, #22072, .T. ) ;
#30453=CARTESIAN_POINT ( 'NONE',  ( -11.53846153846166089, -8.656820664282941280, 34.87096338111179961 ) ) ;
#30454=CARTESIAN_POINT ( 'NONE',  ( -16.15384615384627409, -5.941354392335915335, 34.76329471203413846 ) ) ;
#30459=EDGE_LOOP ( 'NONE', ( #37530, #72012, #15708, #70788 ) ) ;
#30460=CARTESIAN_POINT ( 'NONE',  ( -13.60810030917971680, -5.827078755546623690, 34.72654668319379567 ) ) ;
#30461=ORIENTED_EDGE ( 'NONE', *, *, #4038, .T. ) ;
#30462=CARTESIAN_POINT ( 'NONE',  ( -7.173053654019277303, -12.41269422305637171, 30.68257228309993323 ) ) ;
#30463=LINE ( 'NONE', #30900, #1459 ) ;
#30464=VECTOR ( 'NONE', #20420, 1000.000000000000114 ) ;
#30466=ORIENTED_EDGE ( 'NONE', *, *, #54380, .T. ) ;
#30467=EDGE_CURVE ( 'NONE', #8934, #42078, #33340, .T. ) ;
#30469=DIRECTION ( 'NONE',  ( -0.000000000000000000, 0.9848077530122086864, -0.1736481776669273891 ) ) ;
#30470=ORIENTED_EDGE ( 'NONE', *, *, #16989, .T. ) ;
#30471=CARTESIAN_POINT ( 'NONE',  ( 5.933917620639865831, -9.058645607665454236, 34.76329471203372634 ) ) ;
#30472=LINE ( 'NONE', #3440, #70223 ) ;
#30473=B_SPLINE_CURVE_WITH_KNOTS ( 'NONE', 3,
 ( #65523, #31304, #14805, #76046, #3377, #79042, #56222, #28761, #58769, #76499 ),
 .UNSPECIFIED., .F., .F.,
 ( 4, 2, 2, 2, 4 ),
 ( 0.0007817246256747474977, 0.0009771112852218909357, 0.001172497944769034482, 0.001367884604316178029, 0.001563271263863321575 ),
 .UNSPECIFIED. ) ;
#30474=CARTESIAN_POINT ( 'NONE',  ( -2.307692307692305711, -13.87047571288749737, 32.06866353760679544 ) ) ;
#30475=CARTESIAN_POINT ( 'NONE',  ( 5.776515075435669111, -12.47654668319379567, 31.42292124445336654 ) ) ;
#30476=CARTESIAN_POINT ( 'NONE',  ( -6.857821351800899023, -2.625532179533470512, 30.86335684631491105 ) ) ;
#30477=EDGE_CURVE ( 'NONE', #70917, #10589, #60799, .T. ) ;
#30478=CARTESIAN_POINT ( 'NONE',  ( -0.5268084620947812713, -12.51329471203370325, 31.30864560766548976 ) ) ;
#30479=CARTESIAN_POINT ( 'NONE',  ( -0.3310130233048159676, -12.70449254468099198, 30.44128974285582956 ) ) ;
#30481=CARTESIAN_POINT ( 'NONE',  ( -10.83831083290076158, -9.886141570436013382, 34.14413921362392301 ) ) ;
#30482=EDGE_CURVE ( 'NONE', #13813, #19489, #72533, .T. ) ;
#30484=ORIENTED_EDGE ( 'NONE', *, *, #40138, .T. ) ;
#30485=CARTESIAN_POINT ( 'NONE',  ( 4.153846153846030731, -11.67786785259630911, 32.92929555188603530 ) ) ;
#30486=CARTESIAN_POINT ( 'NONE',  ( 16.94677510719138169, -11.04286588640298916, 33.62463336215343901 ) ) ;
#30488=CARTESIAN_POINT ( 'NONE',  ( 10.61538461538461675, -12.78798330534102767, 29.49999999999997868 ) ) ;
#30489=CYLINDRICAL_SURFACE ( 'NONE', #22674, 0.2500000000000009437 ) ;
#30490=FACE_OUTER_BOUND ( 'NONE', #46973, .T. ) ;
#30492=FACE_BOUND ( 'NONE', #71073, .T. ) ;
#30493=CARTESIAN_POINT ( 'NONE',  ( 12.46153846153833911, -3.300289026999228881, 32.46337939537708905 ) ) ;
#30494=CARTESIAN_POINT ( 'NONE',  ( -6.923076923076922462, -10.05456864172156806, 36.03766855953608683 ) ) ;
#30495=DIRECTION ( 'NONE',  ( 0.000000000000000000, 0.1736481776669275834, 0.9848077530122086864 ) ) ;
#30496=CARTESIAN_POINT ( 'NONE',  ( -11.53846153846153655, -1.466349020453238561, 30.81389545987213907 ) ) ;
#30497=FACE_OUTER_BOUND ( 'NONE', #47886, .T. ) ;
#30498=CARTESIAN_POINT ( 'NONE',  ( 1.161749121552287711, -2.251424796025575770, 29.88072029997477586 ) ) ;
#30501=VERTEX_POINT ( 'NONE', #68013 ) ;
#30502=AXIS2_PLACEMENT_3D ( 'NONE', #67012, #54370, #82304 ) ;
#30503=DIRECTION ( 'NONE',  ( -0.000000000000000000, -0.3420201433256694901, -0.9396926207859080948 ) ) ;
#30504=EDGE_CURVE ( 'NONE', #69932, #26337, #2748, .T. ) ;
#30505=CARTESIAN_POINT ( 'NONE',  ( -14.55766903863466055, -6.567427716900048118, 34.66269422305636283 ) ) ;
#30506=CARTESIAN_POINT ( 'NONE',  ( 5.750023255951410839, -5.643011162660950042, 34.66104346484419096 ) ) ;
#30507=CARTESIAN_POINT ( 'NONE',  ( -9.692307692307812417, -10.90142922262034020, 33.41473453929536674 ) ) ;
#30508=CARTESIAN_POINT ( 'NONE',  ( -4.283994123577849145, -5.070767119584671079, 34.40440758774516183 ) ) ;
#30509=CYLINDRICAL_SURFACE ( 'NONE', #9592, 0.2499999999999994726 ) ;
#30512=CARTESIAN_POINT ( 'NONE',  ( -16.21992853320628569, -5.471508081941601986, 34.59228464037088457 ) ) ;
#30514=CARTESIAN_POINT ( 'NONE',  ( -17.01166750564705055, -6.026961402152789304, 34.52809138561124769 ) ) ;
#30515=CARTESIAN_POINT ( 'NONE',  ( 17.75002325595141173, -8.347322224742351082, 34.93158281831414769 ) ) ;
#30516=CARTESIAN_POINT ( 'NONE',  ( 4.153846153846032507, -12.46129190930018460, 30.37095296980731973 ) ) ;
#30517=DIRECTION ( 'NONE',  ( -0.000000000000000000, -0.3420201433256694346, -0.9396926207859080948 ) ) ;
#30518=CARTESIAN_POINT ( 'NONE',  ( -1.384615384615505151, -11.48612834414049644, 32.76840700105863391 ) ) ;
#30519=CARTESIAN_POINT ( 'NONE',  ( -12.46153846153846168, -8.318370150425687726, 35.83090037661290239 ) ) ;
#30520=ORIENTED_EDGE ( 'NONE', *, *, #48146, .T. ) ;
#30521=CARTESIAN_POINT ( 'NONE',  ( 17.14299041027315695, -12.62096338111211757, 30.90682066428152908 ) ) ;
#30522=CARTESIAN_POINT ( 'NONE',  ( 14.30769230769231015, -12.78798330534102945, 29.74999999999997868 ) ) ;
#30524=CARTESIAN_POINT ( 'NONE',  ( 1.384615384615386802, -13.88283147151868846, 33.14645433367849847 ) ) ;
#30526=ORIENTED_EDGE ( 'NONE', *, *, #3481, .F. ) ;
#30527=EDGE_CURVE ( 'NONE', #48794, #83351, #48607, .T. ) ;
#30528=FACE_OUTER_BOUND ( 'NONE', #77530, .T. ) ;
#30529=CARTESIAN_POINT ( 'NONE',  ( -10.61538461538473577, -9.528491918059723176, 34.59228464037033035 ) ) ;
#30530=DIRECTION ( 'NONE',  ( 1.000000000000000000, 0.000000000000000000, 0.000000000000000000 ) ) ;
#30531=ORIENTED_EDGE ( 'NONE', *, *, #24612, .F. ) ;
#30532=CARTESIAN_POINT ( 'NONE',  ( 6.857806477116147548, -3.300289026998414865, 32.46337939537583139 ) ) ;
#30533=CARTESIAN_POINT ( 'NONE',  ( -2.307692307692427391, -10.90142922262034020, 33.41473453929536674 ) ) ;
#30534=CARTESIAN_POINT ( 'NONE',  ( -5.076923076923197442, -9.442884908241554243, 34.35708131394783038 ) ) ;
#30535=DIRECTION ( 'NONE',  ( 0.000000000000000000, 0.8660254037844377084, -0.5000000000000015543 ) ) ;
#30539=EDGE_CURVE ( 'NONE', #84142, #86621, #45209, .T. ) ;
#30541=CARTESIAN_POINT ( 'NONE',  ( 4.023698944407931855, -10.19110544564092002, 33.96427741523702792 ) ) ;
#30542=EDGE_LOOP ( 'NONE', ( #6689, #43314 ) ) ;
#30544=ORIENTED_EDGE ( 'NONE', *, *, #4080, .F. ) ;
#30545=ADVANCED_FACE ( 'NONE', ( #434 ), #81532, .F. ) ;
#30547=EDGE_CURVE ( 'NONE', #44265, #18436, #71518, .T. ) ;
#30548=CARTESIAN_POINT ( 'NONE',  ( -9.915233909823838232, -9.886141570436013382, 34.14413921362392301 ) ) ;
#30549=CARTESIAN_POINT ( 'NONE',  ( 9.942362112221147186, -4.074993327901527351, 33.72946981652012255 ) ) ;
#30550=FACE_OUTER_BOUND ( 'NONE', #38083, .T. ) ;
#30552=DIRECTION ( 'NONE',  ( -0.000000000000000000, -0.000000000000000000, -1.000000000000000000 ) ) ;
#30554=EDGE_LOOP ( 'NONE', ( #68961, #86534, #13185, #46654 ) ) ;
#30555=CARTESIAN_POINT ( 'NONE',  ( -1.318547033612945896, -4.786620604624113540, 33.94971097300155805 ) ) ;
#30556=EDGE_LOOP ( 'NONE', ( #61247, #34278 ) ) ;
#30557=CARTESIAN_POINT ( 'NONE',  ( 16.40384615384615330, -2.499999999999998668, 29.75000000000000355 ) ) ;
#30558=CARTESIAN_POINT ( 'NONE',  ( 1.634560902963528628, -10.76462480002816235, 33.53768742498949962 ) ) ;
#30559=CARTESIAN_POINT ( 'NONE',  ( 15.93091919493930320, -11.43668979543635089, 33.22377378376089752 ) ) ;
#30560=ORIENTED_EDGE ( 'NONE', *, *, #28144, .T. ) ;
#30561=EDGE_CURVE ( 'NONE', #54522, #62121, #82860, .T. ) ;
#30562=VECTOR ( 'NONE', #3940, 1000.000000000000114 ) ;
#30563=ORIENTED_EDGE ( 'NONE', *, *, #4631, .T. ) ;
#30564=CARTESIAN_POINT ( 'NONE',  ( -9.692307692307691624, -12.62096338111211580, 30.90682066428153263 ) ) ;
#30565=EDGE_LOOP ( 'NONE', ( #55142, #6744, #20281, #38245 ) ) ;
#30566=CARTESIAN_POINT ( 'NONE',  ( -5.869474298236436738, -8.586989748646452369, 34.63063291749215011 ) ) ;
#30567=CARTESIAN_POINT ( 'NONE',  ( -10.74553258511630993, -9.504002272028875709, 34.60269587691767867 ) ) ;
#30568=VERTEX_POINT ( 'NONE', #27020 ) ;
#30570=CARTESIAN_POINT ( 'NONE',  ( -14.30769230769230660, -12.62096338111211580, 30.90682066428153263 ) ) ;
#30571=CARTESIAN_POINT ( 'NONE',  ( -8.992157728137616601, -11.98009711892699514, 32.48740034544076138 ) ) ;
#30572=FACE_BOUND ( 'NONE', #158, .T. ) ;
#30573=CARTESIAN_POINT ( 'NONE',  ( -11.78848477575450282, -2.587272538249755893, 30.68239716806877837 ) ) ;
#30574=CARTESIAN_POINT ( 'NONE',  ( 2.307692307692187583, -8.613356846316285953, 34.62446782046622218 ) ) ;
#30575=DIRECTION ( 'NONE',  ( -0.000000000000000000, -0.9848077530122086864, -0.1736481776669273613 ) ) ;
#30576=CYLINDRICAL_SURFACE ( 'NONE', #73398, 0.2499999999999973355 ) ;
#30577=CARTESIAN_POINT ( 'NONE',  ( 6.923076923076924238, -11.69971097300155272, 32.46337939537588113 ) ) ;
#30578=CARTESIAN_POINT ( 'NONE',  ( -11.31545018684868964, -3.105924265160262543, 32.13625925475356127 ) ) ;
#30579=CARTESIAN_POINT ( 'NONE',  ( 5.142991427925516668, -2.538708090699994813, 30.37095296980875503 ) ) ;
#30580=ORIENTED_EDGE ( 'NONE', *, *, #32116, .F. ) ;
#30583=EDGE_LOOP ( 'NONE', ( #44959, #43642 ) ) ;
#30584=CARTESIAN_POINT ( 'NONE',  ( -6.700065571464073777, -8.239487800360276282, 34.69522927552633718 ) ) ;
#30585=CARTESIAN_POINT ( 'NONE',  ( 1.134592147322421418, -10.76384336483936011, 33.53834819971076087 ) ) ;
#30587=CARTESIAN_POINT ( 'NONE',  ( 2.307692307692309264, -2.538708090699994813, 30.37095296980875503 ) ) ;
#30588=CARTESIAN_POINT ( 'NONE',  ( 14.53047197667037338, -4.226511098958373402, 33.85474049983370293 ) ) ;
#30589=CYLINDRICAL_SURFACE ( 'NONE', #31491, 0.2499999999999973355 ) ;
#30590=CARTESIAN_POINT ( 'NONE',  ( -4.153846153846274980, -3.643525952248796163, 33.31231777344771672 ) ) ;
#30591=ORIENTED_EDGE ( 'NONE', *, *, #86924, .T. ) ;
#30592=CARTESIAN_POINT ( 'NONE',  ( 18.00000000000000000, -2.486705287966279876, 31.30864560766543647 ) ) ;
#30594=CARTESIAN_POINT ( 'NONE',  ( -15.16551365949320562, -10.21337939537593620, 33.94971097300152252 ) ) ;
#30595=DIRECTION ( 'NONE',  ( 0.000000000000000000, 0.7660444431189822323, -0.6427876096865344779 ) ) ;
#30596=LINE ( 'NONE', #4466, #32356 ) ;
#30597=DIRECTION ( 'NONE',  ( -0.000000000000000000, -0.6427876096865404731, -0.7660444431189771253 ) ) ;
#30599=ORIENTED_EDGE ( 'NONE', *, *, #2088, .F. ) ;
#30600=EDGE_CURVE ( 'NONE', #61210, #66121, #88781, .T. ) ;
#30601=EDGE_LOOP ( 'NONE', ( #71094, #52793 ) ) ;
#30602=CARTESIAN_POINT ( 'NONE',  ( -10.61538461538461320, -1.951392089020283160, 34.73218667398347748 ) ) ;
#30603=EDGE_CURVE ( 'NONE', #84061, #72551, #38184, .T. ) ;
#30604=ORIENTED_EDGE ( 'NONE', *, *, #2404, .F. ) ;
#30605=CARTESIAN_POINT ( 'NONE',  ( -5.076923076923075762, -1.129524287112498415, 32.06866353760679544 ) ) ;
#30606=CARTESIAN_POINT ( 'NONE',  ( 18.00000000000000000, -11.35647404775217417, 33.31231777344666511 ) ) ;
#30607=CARTESIAN_POINT ( 'NONE',  ( -14.05774678934416499, -6.696923467548660192, 34.68552623307873972 ) ) ;
#30608=CARTESIAN_POINT ( 'NONE',  ( -0.5916864312701544115, -12.15440758774515473, 32.17923288041532004 ) ) ;
#30610=DIRECTION ( 'NONE',  ( -0.000000000000000000, -0.5000000000000009992, -0.8660254037844380415 ) ) ;
#30611=ORIENTED_EDGE ( 'NONE', *, *, #73094, .T. ) ;
#30612=EDGE_CURVE ( 'NONE', #5024, #21466, #31711, .T. ) ;
#30613=LINE ( 'NONE', #77917, #80370 ) ;
#30614=CARTESIAN_POINT ( 'NONE',  ( -1.253823576790596750, -8.999086150933472084, 34.52020707165672064 ) ) ;
#30615=EDGE_LOOP ( 'NONE', ( #55865, #72183, #37294, #39889 ) ) ;
#30616=FACE_OUTER_BOUND ( 'NONE', #83104, .T. ) ;
#30617=CARTESIAN_POINT ( 'NONE',  ( 3.453780582382079078, -2.758310577978208666, 31.33698337089302299 ) ) ;
#30618=FACE_OUTER_BOUND ( 'NONE', #70130, .T. ) ;
#30619=CARTESIAN_POINT ( 'NONE',  ( 0.7114839798866022802, -2.824170634883621744, 31.52227843825337317 ) ) ;
#30620=LINE ( 'NONE', #58093, #82481 ) ;
#30621=CARTESIAN_POINT ( 'NONE',  ( -2.980714919130917462, -11.28795663066794219, 33.01431243580653785 ) ) ;
#30622=DIRECTION ( 'NONE',  ( -0.000000000000000000, 1.000000000000000000, 3.491481338843133355E-15 ) ) ;
#30625=ORIENTED_EDGE ( 'NONE', *, *, #70658, .F. ) ;
#30627=CARTESIAN_POINT ( 'NONE',  ( -12.59214882116298995, -7.722926236386453702, 34.74524107206102030 ) ) ;
#30628=LINE ( 'NONE', #70297, #56266 ) ;
#30630=B_SPLINE_CURVE_WITH_KNOTS ( 'NONE', 3,
 ( #13241, #61406, #66850, #11461, #73165, #18224, #88046, #26307, #32181, #74060 ),
 .UNSPECIFIED., .F., .F.,
 ( 4, 2, 2, 2, 4 ),
 ( 0.000000000000000000, 0.0001954339857564071220, 0.0003908679715128142440, 0.0005863019572692213660, 0.0007817359430256284880 ),
 .UNSPECIFIED. ) ;
#30631=CARTESIAN_POINT ( 'NONE',  ( -39.05038313613820122, -2.499999999999999556, 29.75000000000000355 ) ) ;
#30632=CARTESIAN_POINT ( 'NONE',  ( 7.846153846153725020, -12.46129190930018460, 30.37095296980731973 ) ) ;
#30633=EDGE_CURVE ( 'NONE', #49648, #60841, #3714, .T. ) ;
#30634=ORIENTED_EDGE ( 'NONE', *, *, #1424, .T. ) ;
#30636=CARTESIAN_POINT ( 'NONE',  ( -15.36091720050092846, -4.299443229763728169, 33.91186481527756058 ) ) ;
#30637=AXIS2_PLACEMENT_3D ( 'NONE', #2955, #71414, #85390 ) ;
#30638=EDGE_LOOP ( 'NONE', ( #8192, #78825, #72272, #27328 ) ) ;
#30639=CARTESIAN_POINT ( 'NONE',  ( -4.153846153846274980, -8.656820664282941280, 34.87096338111179961 ) ) ;
#30640=ORIENTED_EDGE ( 'NONE', *, *, #82296, .F. ) ;
#30641=CARTESIAN_POINT ( 'NONE',  ( 17.77707378248385339, -6.503392248772476236, 34.64988816332204635 ) ) ;
#30642=B_SPLINE_CURVE_WITH_KNOTS ( 'NONE', 3,
 ( #25151, #80564, #31465, #11651, #32804, #59824 ),
 .UNSPECIFIED., .F., .F.,
 ( 4, 2, 4 ),
 ( 0.000000000000000000, 0.0001954784845028902421, 0.0003909569690057804843 ),
 .UNSPECIFIED. ) ;
#30643=CARTESIAN_POINT ( 'NONE',  ( 17.01167208676183407, -2.506253911140460477, 30.00000000000013856 ) ) ;
#30645=ORIENTED_EDGE ( 'NONE', *, *, #65322, .T. ) ;
#30646=CARTESIAN_POINT ( 'NONE',  ( -12.23875879256039489, -10.97394488606064122, 33.68653795673694873 ) ) ;
#30648=CARTESIAN_POINT ( 'NONE',  ( 13.25405547100202241, -2.254533558242299396, 29.97296025877827930 ) ) ;
#30652=FACE_OUTER_BOUND ( 'NONE', #34745, .T. ) ;
#30653=EDGE_CURVE ( 'NONE', #5428, #85310, #56696, .T. ) ;
#30655=CARTESIAN_POINT ( 'NONE',  ( 11.53846153846153832, -12.62096338111211580, 30.90682066428153263 ) ) ;
#30656=CARTESIAN_POINT ( 'NONE',  ( 10.74591031714818179, -3.285477652293413264, 32.44071101563363158 ) ) ;
#30658=EDGE_CURVE ( 'NONE', #39653, #67493, #72464, .T. ) ;
#30659=AXIS2_PLACEMENT_3D ( 'NONE', #48259, #82948, #21230 ) ;
#30660=CARTESIAN_POINT ( 'NONE',  ( -14.05774689831426372, -10.18230066228895758, 34.26354781536631577 ) ) ;
#30662=ORIENTED_EDGE ( 'NONE', *, *, #68172, .F. ) ;
#30664=ADVANCED_FACE ( 'NONE', ( #30550 ), #51232, .F. ) ;
#30665=VERTEX_POINT ( 'NONE', #15277 ) ;
#30666=CARTESIAN_POINT ( 'NONE',  ( 15.23076923076911093, -2.625532179533778709, 30.86335684631627174 ) ) ;
#30667=VERTEX_POINT ( 'NONE', #23780 ) ;
#30668=DIRECTION ( 'NONE',  ( -0.000000000000000000, 0.3420201433256694901, -0.9396926207859082059 ) ) ;
#30669=CARTESIAN_POINT ( 'NONE',  ( 5.142991427925513115, -4.098570777380720287, 33.41473453929635440 ) ) ;
#30670=VERTEX_POINT ( 'NONE', #85501 ) ;
#30672=VERTEX_POINT ( 'NONE', #37300 ) ;
#30673=B_SPLINE_CURVE_WITH_KNOTS ( 'NONE', 3,
 ( #70413, #83493, #1950, #8274, #35746, #8716, #63197, #84378, #15475, #78480 ),
 .UNSPECIFIED., .F., .F.,
 ( 4, 2, 2, 2, 4 ),
 ( 0.0007817246256747483650, 0.0009771112852218926705, 0.001172497944769037084, 0.001367884604316181498, 0.001563271263863325695 ),
 .UNSPECIFIED. ) ;
#30674=EDGE_CURVE ( 'NONE', #26195, #75911, #42755, .T. ) ;
#30675=ORIENTED_EDGE ( 'NONE', *, *, #24995, .T. ) ;
#30676=CARTESIAN_POINT ( 'NONE',  ( 4.153846153846032507, -10.90142922262034020, 33.41473453929536674 ) ) ;
#30677=ORIENTED_EDGE ( 'NONE', *, *, #50763, .F. ) ;
#30678=CARTESIAN_POINT ( 'NONE',  ( 11.66925334628632882, -11.18335022499818621, 33.13157742990016885 ) ) ;
#30679=ADVANCED_FACE ( 'NONE', ( #3069 ), #78739, .F. ) ;
#30681=CARTESIAN_POINT ( 'NONE',  ( -11.78848477575450282, -3.711651800289232028, 33.01384336483936011 ) ) ;
#30683=FACE_BOUND ( 'NONE', #71076, .T. ) ;
#30684=ORIENTED_EDGE ( 'NONE', *, *, #39559, .T. ) ;
#30685=AXIS2_PLACEMENT_3D ( 'NONE', #15923, #84385, #22665 ) ;
#30686=CARTESIAN_POINT ( 'NONE',  ( -1.450372187129693513, -7.249945686854186278, 34.74374336980224598 ) ) ;
#30688=CARTESIAN_POINT ( 'NONE',  ( -14.24162395668986747, -5.557115091759786019, 34.35708131394839882 ) ) ;
#30689=CARTESIAN_POINT ( 'NONE',  ( 2.241609928332172874, -8.164416787775445883, 34.95778746994557906 ) ) ;
#30690=CARTESIAN_POINT ( 'NONE',  ( 18.00000000000000000, -8.318370150425687726, 35.83090037661290239 ) ) ;
#30691=ORIENTED_EDGE ( 'NONE', *, *, #45090, .T. ) ;
#30692=DIRECTION ( 'NONE',  ( -0.000000000000000000, 0.6427876096865404731, -0.7660444431189770143 ) ) ;
#30694=ORIENTED_EDGE ( 'NONE', *, *, #67351, .T. ) ;
#30696=CARTESIAN_POINT ( 'NONE',  ( 8.769230769230768274, -6.681629849574314051, 35.83090037661290239 ) ) ;
#30697=CARTESIAN_POINT ( 'NONE',  ( 16.08857570788537572, -6.026961402152685388, 34.52809138561120506 ) ) ;
#30698=CARTESIAN_POINT ( 'NONE',  ( -3.931066612577742259, -4.387253974876676565, 33.66317474335728832 ) ) ;
#30699=CARTESIAN_POINT ( 'NONE',  ( -18.24997674404858827, -5.643011162660949154, 34.66104346484419096 ) ) ;
#30700=CARTESIAN_POINT ( 'NONE',  ( -12.39628289026243380, -4.481592998940250538, 33.73612834413965089 ) ) ;
#30702=CARTESIAN_POINT ( 'NONE',  ( 6.923076923076924238, -1.790695186598648903, 34.54067556320373455 ) ) ;
#30703=CARTESIAN_POINT ( 'NONE',  ( 3.165499230212911908, -9.528491918058357157, 34.59228464037090589 ) ) ;
#30704=CARTESIAN_POINT ( 'NONE',  ( 4.403791672194294016, -9.272278438253401589, 34.42582936511637826 ) ) ;
#30705=CARTESIAN_POINT ( 'NONE',  ( 13.25392391794783187, -12.38065189839062263, 30.83690757178629482 ) ) ;
#30706=VERTEX_POINT ( 'NONE', #84189 ) ;
#30707=VERTEX_POINT ( 'NONE', #49932 ) ;
#30708=FACE_BOUND ( 'NONE', #50983, .T. ) ;
#30709=B_SPLINE_CURVE_WITH_KNOTS ( 'NONE', 3,
 ( #12383, #11499, #39864, #26339, #4745, #26780, #47486, #53804, #47039, #12822 ),
 .UNSPECIFIED., .F., .F.,
 ( 4, 2, 2, 2, 4 ),
 ( 0.000000000000000000, 0.0001954339857564099951, 0.0003908679715128199903, 0.0005863019572692300396, 0.0007817359430256399806 ),
 .UNSPECIFIED. ) ;
#30710=VERTEX_POINT ( 'NONE', #11170 ) ;
#30711=DIRECTION ( 'NONE',  ( -0.000000000000000000, -0.3420201433256694901, -0.9396926207859082059 ) ) ;
#30712=CARTESIAN_POINT ( 'NONE',  ( -13.16183584334697265, -10.81320215134717344, 33.49497208177562868 ) ) ;
#30713=ORIENTED_EDGE ( 'NONE', *, *, #61255, .T. ) ;
#30714=CARTESIAN_POINT ( 'NONE',  ( 6.000000000000001776, -2.249999999999998668, 29.75000000000001776 ) ) ;
#30715=CARTESIAN_POINT ( 'NONE',  ( 12.46153846153846168, -11.91647553114624181, 32.58852847137148245 ) ) ;
#30716=CARTESIAN_POINT ( 'NONE',  ( -8.519176457592452678, -6.567000820036036579, 34.66262288849541306 ) ) ;
#30717=CARTESIAN_POINT ( 'NONE',  ( 4.153846153846030731, -6.835583212225970762, 34.95778746994575670 ) ) ;
#30718=VERTEX_POINT ( 'NONE', #24682 ) ;
#30719=CARTESIAN_POINT ( 'NONE',  ( -4.153846153846273204, -6.879047030192662504, 34.71129190930017927 ) ) ;
#30720=VERTEX_POINT ( 'NONE', #32773 ) ;
#30721=ADVANCED_FACE ( 'NONE', ( #79635 ), #80076, .F. ) ;
#30722=CARTESIAN_POINT ( 'NONE',  ( 16.94623161025551639, -10.54014554554151140, 33.71984207302941883 ) ) ;
#30723=EDGE_LOOP ( 'NONE', ( #7500, #62423, #47423, #26802 ) ) ;
#30724=DIRECTION ( 'NONE',  ( 0.000000000000000000, 1.000000000000000000, 0.000000000000000000 ) ) ;
#30725=CARTESIAN_POINT ( 'NONE',  ( 14.98079248672063990, -4.818429247618089661, 34.26397095200675125 ) ) ;
#30726=LINE ( 'NONE', #58192, #84663 ) ;
#30727=CARTESIAN_POINT ( 'NONE',  ( -15.29609214626140634, -7.749976743299138882, 34.99404534957040624 ) ) ;
#30728=CYLINDRICAL_SURFACE ( 'NONE', #75002, 0.2500000000000002220 ) ;
#30729=CARTESIAN_POINT ( 'NONE',  ( 12.33139049180676494, -5.915902021225889484, 34.75552854090298638 ) ) ;
#30730=EDGE_CURVE ( 'NONE', #219, #81991, #86862, .T. ) ;
#30732=VERTEX_POINT ( 'NONE', #52145 ) ;
#30733=CARTESIAN_POINT ( 'NONE',  ( -10.61538461538473577, -3.643525952248795718, 33.31231777344771672 ) ) ;
#30734=CARTESIAN_POINT ( 'NONE',  ( -0.4615384615384611200, -4.786620604624113540, 33.94971097300155094 ) ) ;
#30735=ORIENTED_EDGE ( 'NONE', *, *, #53568, .F. ) ;
#30736=ORIENTED_EDGE ( 'NONE', *, *, #65637, .T. ) ;
#30737=CARTESIAN_POINT ( 'NONE',  ( 17.07692307692338218, -2.506253911140615021, 30.00000000000323297 ) ) ;
#30738=CARTESIAN_POINT ( 'NONE',  ( -14.05763788777885281, -2.544122305571458575, 31.48381861865057729 ) ) ;
#30739=CARTESIAN_POINT ( 'NONE',  ( -4.853910232829680815, -12.64618726649961289, 30.78989965857442712 ) ) ;
#30740=CARTESIAN_POINT ( 'NONE',  ( 9.442330961365339448, -12.41269422305637171, 30.68257228309993323 ) ) ;
#30741=CARTESIAN_POINT ( 'NONE',  ( 13.38461538461526423, -3.083524468854526912, 32.58852847137268327 ) ) ;
#30742=EDGE_CURVE ( 'NONE', #44980, #49489, #57470, .T. ) ;
#30744=CARTESIAN_POINT ( 'NONE',  ( -15.00798956179115962, -8.540255544307065350, 34.89611431652622286 ) ) ;
#30745=ORIENTED_EDGE ( 'NONE', *, *, #61928, .T. ) ;
#30746=CARTESIAN_POINT ( 'NONE',  ( 6.000000000000001776, -12.34228464037088635, 31.77849191805839268 ) ) ;
#30747=CARTESIAN_POINT ( 'NONE',  ( -17.07692307692319744, -12.27809138561165270, 31.22303859784587132 ) ) ;
#30748=VECTOR ( 'NONE', #64669, 999.9999999999998863 ) ;
#30749=CARTESIAN_POINT ( 'NONE',  ( 3.930966637108568307, -7.630690623152302621, 34.99857592706774057 ) ) ;
#30752=CARTESIAN_POINT ( 'NONE',  ( 5.076923076923075762, -2.486705287966279876, 31.30864560766543647 ) ) ;
#30753=ADVANCED_FACE ( 'NONE', ( #52592 ), #12508, .F. ) ;
#30756=ORIENTED_EDGE ( 'NONE', *, *, #83416, .F. ) ;
#30757=CARTESIAN_POINT ( 'NONE',  ( -17.93474486048716088, -8.656820664281605460, 34.87096338111211224 ) ) ;
#30758=CARTESIAN_POINT ( 'NONE',  ( 16.28389120976593318, -2.254550872974305786, 29.97347326024527092 ) ) ;
#30759=CARTESIAN_POINT ( 'NONE',  ( -2.084729404130821084, -7.369474270740069777, 34.74850911626239736 ) ) ;
#30760=VERTEX_POINT ( 'NONE', #18378 ) ;
#30761=EDGE_CURVE ( 'NONE', #75979, #62624, #28453, .T. ) ;
#30762=CARTESIAN_POINT ( 'NONE',  ( -2.531177232256636156, -6.716662450894490100, 34.94144148231605840 ) ) ;
#30763=CARTESIAN_POINT ( 'NONE',  ( -10.39237326377176451, -10.61302985866383963, 33.66295027996417843 ) ) ;
#30764=CARTESIAN_POINT ( 'NONE',  ( -17.20707028636129721, -3.817052484675422797, 33.13202310037935661 ) ) ;
#30765=LINE ( 'NONE', #73552, #19264 ) ;
#30766=CARTESIAN_POINT ( 'NONE',  ( -5.010855743573001675, -8.164416787775445883, 34.95778746994558617 ) ) ;
#30767=EDGE_CURVE ( 'NONE', #21486, #3366, #88624, .T. ) ;
#30768=EDGE_LOOP ( 'NONE', ( #19259, #74836, #10173, #30180 ) ) ;
#30769=CARTESIAN_POINT ( 'NONE',  ( 16.15384615384603251, -10.33852847137269571, 34.16647553114546554 ) ) ;
#30770=ORIENTED_EDGE ( 'NONE', *, *, #87060, .F. ) ;
#30771=CARTESIAN_POINT ( 'NONE',  ( -9.442253380669381357, -12.17597550085003633, 31.52189283813461884 ) ) ;
#30772=CARTESIAN_POINT ( 'NONE',  ( -17.01085574357300345, -3.322132147404559532, 32.92929555188717927 ) ) ;
#30773=CARTESIAN_POINT ( 'NONE',  ( 9.758375025657770152, -2.486705287966280320, 31.30864560766543647 ) ) ;
#30775=CARTESIAN_POINT ( 'NONE',  ( 12.46153846153846168, -3.513871655860378418, 32.76840700105978499 ) ) ;
#30777=ORIENTED_EDGE ( 'NONE', *, *, #48550, .F. ) ;
#30779=ORIENTED_EDGE ( 'NONE', *, *, #10578, .T. ) ;
#30780=EDGE_CURVE ( 'NONE', #23528, #86451, #13458, .T. ) ;
#30781=EDGE_CURVE ( 'NONE', #12315, #72521, #67011, .T. ) ;
#30782=ORIENTED_EDGE ( 'NONE', *, *, #1827, .F. ) ;
#30783=ORIENTED_EDGE ( 'NONE', *, *, #82288, .F. ) ;
#30784=FACE_OUTER_BOUND ( 'NONE', #43095, .T. ) ;
#30785=CARTESIAN_POINT ( 'NONE',  ( -2.307692307692427391, -3.300289026999228881, 32.46337939537708905 ) ) ;
#30786=CARTESIAN_POINT ( 'NONE',  ( -4.087778820496077437, -6.343179335718452272, 34.87096338111212646 ) ) ;
#30787=ADVANCED_FACE ( 'NONE', ( #20583 ), #13387, .F. ) ;
#30788=LINE ( 'NONE', #32135, #26458 ) ;
#30789=CARTESIAN_POINT ( 'NONE',  ( 10.61538461538449596, -12.27809138561165270, 31.22303859784587132 ) ) ;
#30790=CARTESIAN_POINT ( 'NONE',  ( -6.066082379360133281, -2.833524468853757305, 32.15551576947924417 ) ) ;
#30791=DIRECTION ( 'NONE',  ( -0.000000000000000000, 0.8660254037844399289, -0.4999999999999980016 ) ) ;
#30792=CARTESIAN_POINT ( 'NONE',  ( -7.623142494540998015, -3.105924265160262543, 32.13625925475356127 ) ) ;
#30793=ORIENTED_EDGE ( 'NONE', *, *, #38397, .T. ) ;
#30794=ORIENTED_EDGE ( 'NONE', *, *, #79960, .F. ) ;
#30796=FACE_OUTER_BOUND ( 'NONE', #83411, .T. ) ;
#30797=ORIENTED_EDGE ( 'NONE', *, *, #74137, .F. ) ;
#30798=CARTESIAN_POINT ( 'NONE',  ( 16.40379167219429846, -11.86320923018887541, 32.19269448109604781 ) ) ;
#30799=FACE_OUTER_BOUND ( 'NONE', #3161, .T. ) ;
#30800=CARTESIAN_POINT ( 'NONE',  ( -1.607542343522233130, -4.762599654559228846, 34.23009711892697737 ) ) ;
#30802=VERTEX_POINT ( 'NONE', #62014 ) ;
#30803=B_SPLINE_CURVE_WITH_KNOTS ( 'NONE', 3,
 ( #4420, #30995, #24236, #27362, #5319, #53941, #54383, #34564, #62027, #12962 ),
 .UNSPECIFIED., .F., .F.,
 ( 4, 2, 2, 2, 4 ),
 ( 0.000000000000000000, 0.0001954311564186868473, 0.0003908623128373736946, 0.0005862934692560605419, 0.0007817246256747473893 ),
 .UNSPECIFIED. ) ;
#30804=VECTOR ( 'NONE', #75772, 1000.000000000000114 ) ;
#30805=B_SPLINE_CURVE_WITH_KNOTS ( 'NONE', 3,
 ( #10026, #85697, #31179, #66308, #3265, #30738, #51884, #17684, #72617, #37047 ),
 .UNSPECIFIED., .F., .F.,
 ( 4, 2, 2, 2, 4 ),
 ( 0.0007817246256747446788, 0.0009771112852218874663, 0.001172497944769030145, 0.001367884604316172825, 0.001563271263863315720 ),
 .UNSPECIFIED. ) ;
#30806=ORIENTED_EDGE ( 'NONE', *, *, #75404, .F. ) ;
#30807=CARTESIAN_POINT ( 'NONE',  ( -2.531177251416254492, -12.44517049084099725, 30.48991314939691932 ) ) ;
#30809=EDGE_LOOP ( 'NONE', ( #13390, #58294 ) ) ;
#30810=FACE_BOUND ( 'NONE', #79905, .T. ) ;
#30811=CARTESIAN_POINT ( 'NONE',  ( -5.999999999999998224, -8.973038597847269315, 34.52809138561121927 ) ) ;
#30812=AXIS2_PLACEMENT_3D ( 'NONE', #23191, #70936, #17324 ) ;
#30813=CARTESIAN_POINT ( 'NONE',  ( -4.153846153846273204, -11.94971097300221174, 32.03036669348237098 ) ) ;
#30814=ORIENTED_EDGE ( 'NONE', *, *, #84715, .F. ) ;
#30815=CARTESIAN_POINT ( 'NONE',  ( -15.09997742294444478, -12.11778462344220841, 31.66786338562085135 ) ) ;
#30816=CARTESIAN_POINT ( 'NONE',  ( 16.37662569511456567, -4.387253974876675677, 33.66317474335728832 ) ) ;
#30817=DIRECTION ( 'NONE',  ( -0.000000000000000000, 0.9848077530122085754, -0.1736481776669273613 ) ) ;
#30818=ORIENTED_EDGE ( 'NONE', *, *, #19373, .T. ) ;
#30819=DIRECTION ( 'NONE',  ( -0.000000000000000000, -0.3420201433256694346, -0.9396926207859080948 ) ) ;
#30821=VERTEX_POINT ( 'NONE', #88635 ) ;
#30822=CARTESIAN_POINT ( 'NONE',  ( 6.250000000000063061, -7.434744860731433924, 35.00000000000000711 ) ) ;
#30823=CARTESIAN_POINT ( 'NONE',  ( -9.561782254074051579, -9.503571793651731880, 34.60286762892837942 ) ) ;
#30824=EDGE_LOOP ( 'NONE', ( #83619, #6030, #31791, #66471 ) ) ;
#30826=CARTESIAN_POINT ( 'NONE',  ( 13.13463865367303463, -2.564618984488975517, 30.55390908950641915 ) ) ;
#30827=CARTESIAN_POINT ( 'NONE',  ( -16.08859058257012720, -8.613356846314930593, 34.62446782046653482 ) ) ;
#30828=CARTESIAN_POINT ( 'NONE',  ( -10.54931626438217585, -5.557115091759786019, 34.35708131394839882 ) ) ;
#30829=DIRECTION ( 'NONE',  ( 0.000000000000000000, 0.3420201433256610524, 0.9396926207859113145 ) ) ;
#30830=CARTESIAN_POINT ( 'NONE',  ( 5.999999999999880096, -10.21337939537710326, 33.94971097300076224 ) ) ;
#30831=CARTESIAN_POINT ( 'NONE',  ( -1.450698795571264688, -2.721908614388772296, 31.22303859784725688 ) ) ;
#30832=CARTESIAN_POINT ( 'NONE',  ( 2.530471848960716752, -10.11255958852955850, 34.01340905677048454 ) ) ;
#30834=CARTESIAN_POINT ( 'NONE',  ( -15.48079246806219267, -11.86270091957321249, 32.19358267280087915 ) ) ;
#30835=CARTESIAN_POINT ( 'NONE',  ( 12.33139049180676672, -5.070767119584671079, 34.40440758774516183 ) ) ;
#30836=CARTESIAN_POINT ( 'NONE',  ( 13.44976016533501983, -7.750023224968867197, 34.99404313364389907 ) ) ;
#30838=ORIENTED_EDGE ( 'NONE', *, *, #76110, .T. ) ;
#30840=ORIENTED_EDGE ( 'NONE', *, *, #47824, .T. ) ;
#30841=CARTESIAN_POINT ( 'NONE',  ( -2.438382910802615822, -2.845849958028613624, 32.17971566917920967 ) ) ;
#30842=ORIENTED_EDGE ( 'NONE', *, *, #68437, .T. ) ;
#30843=CARTESIAN_POINT ( 'NONE',  ( 17.93472955403922242, -12.27809138561121394, 31.22303859784730307 ) ) ;
#30844=ORIENTED_EDGE ( 'NONE', *, *, #26903, .F. ) ;
#30845=LINE ( 'NONE', #49356, #67086 ) ;
#30847=FACE_OUTER_BOUND ( 'NONE', #63302, .T. ) ;
#30848=CARTESIAN_POINT ( 'NONE',  ( 9.692307692307572609, -11.48612834414049644, 32.76840700105863391 ) ) ;
#30849=CARTESIAN_POINT ( 'NONE',  ( -3.007989561791166278, -12.47679350104403007, 31.42216943046555855 ) ) ;
#30850=CARTESIAN_POINT ( 'NONE',  ( -12.23852561744506495, -4.026326845037962343, 33.68677907613344047 ) ) ;
#30851=DIRECTION ( 'NONE',  ( -0.000000000000000000, 0.9848077530122086864, -0.1736481776669273891 ) ) ;
#30852=CYLINDRICAL_SURFACE ( 'NONE', #48780, 0.2499999999999973355 ) ;
#30855=CYLINDRICAL_SURFACE ( 'NONE', #268, 0.2500000000000008882 ) ;
#30856=CARTESIAN_POINT ( 'NONE',  ( 13.38461538461538680, -3.322132147404559976, 32.92929555188717927 ) ) ;
#30857=CARTESIAN_POINT ( 'NONE',  ( 13.45068373561782415, -4.098570777380720287, 33.41473453929635440 ) ) ;
#30860=VERTEX_POINT ( 'NONE', #34983 ) ;
#30861=CARTESIAN_POINT ( 'NONE',  ( 17.29993442853592711, -12.15243808032446005, 31.58219941686247978 ) ) ;
#30862=CARTESIAN_POINT ( 'NONE',  ( -14.30769230769230660, -8.120952969808772792, 34.71129190930000163 ) ) ;
#30864=DIRECTION ( 'NONE',  ( -0.000000000000000000, 1.000000000000000000, -0.000000000000000000 ) ) ;
#30865=CARTESIAN_POINT ( 'NONE',  ( 17.32697749683652688, -12.41089969410671223, 31.60739465890703670 ) ) ;
#30866=CARTESIAN_POINT ( 'NONE',  ( -3.007989561791163169, -5.827830569534416583, 34.72679350104403539 ) ) ;
#30868=EDGE_CURVE ( 'NONE', #43223, #63578, #41311, .T. ) ;
#30869=ORIENTED_EDGE ( 'NONE', *, *, #69442, .F. ) ;
#30870=CARTESIAN_POINT ( 'NONE',  ( -1.161835843346975983, -10.11255958852956027, 34.01340905677048454 ) ) ;
#30872=B_SPLINE_CURVE_WITH_KNOTS ( 'NONE', 3,
 ( #79565, #6888, #66029, #65583, #5230, #47876, #59279, #4793, #38575, #86785 ),
 .UNSPECIFIED., .F., .F.,
 ( 4, 2, 2, 2, 4 ),
 ( 0.0007817246256747507503, 0.0009771112852218959231, 0.001172497944769040987, 0.001367884604316186052, 0.001563271263863331116 ),
 .UNSPECIFIED. ) ;
#30873=AXIS2_PLACEMENT_3D ( 'NONE', #14617, #29910, #57366 ) ;
#30875=CARTESIAN_POINT ( 'NONE',  ( 0.5920638997721079377, -12.50538340440932217, 31.33453814440721885 ) ) ;
#30876=AXIS2_PLACEMENT_3D ( 'NONE', #25746, #53206, #80709 ) ;
#30877=CARTESIAN_POINT ( 'NONE',  ( 3.453548772037639214, -5.913360116392399668, 34.49180327182771322 ) ) ;
#30878=CARTESIAN_POINT ( 'NONE',  ( -0.3307001310517008186, -7.277220318596960169, 34.99547417642776992 ) ) ;
#30879=DIRECTION ( 'NONE',  ( -0.000000000000000000, 0.1736481776669307198, -0.9848077530122080203 ) ) ;
#30880=CARTESIAN_POINT ( 'NONE',  ( -2.241623956689867025, -11.69971097300155272, 32.46337939537588113 ) ) ;
#30881=ORIENTED_EDGE ( 'NONE', *, *, #69139, .T. ) ;
#30882=ORIENTED_EDGE ( 'NONE', *, *, #87144, .F. ) ;
#30883=ADVANCED_FACE ( 'NONE', ( #55256 ), #75528, .F. ) ;
#30884=EDGE_CURVE ( 'NONE', #58039, #22897, #69301, .T. ) ;
#30885=ORIENTED_EDGE ( 'NONE', *, *, #18640, .F. ) ;
#30886=CARTESIAN_POINT ( 'NONE',  ( 12.71153846153846168, -2.499999999999998668, 29.75000000000000355 ) ) ;
#30887=CARTESIAN_POINT ( 'NONE',  ( 8.639083559792551270, -2.882441371585227508, 31.66841991370172238 ) ) ;
#30889=CARTESIAN_POINT ( 'NONE',  ( -14.98082371242109012, -3.202959910592335646, 32.30730279482227019 ) ) ;
#30890=CARTESIAN_POINT ( 'NONE',  ( -0.4615384615384611200, -10.89733346790207413, 36.13435417666054406 ) ) ;
#30891=CARTESIAN_POINT ( 'NONE',  ( 5.999999999999880096, -9.442884908241554243, 34.35708131394783038 ) ) ;
#30892=ORIENTED_EDGE ( 'NONE', *, *, #48750, .T. ) ;
#30893=VERTEX_POINT ( 'NONE', #19706 ) ;
#30896=VERTEX_POINT ( 'NONE', #758 ) ;
#30897=CARTESIAN_POINT ( 'NONE',  ( -14.30769230769230660, -11.11383981884818262, 36.00935417666054406 ) ) ;
#30898=EDGE_LOOP ( 'NONE', ( #30905, #88505 ) ) ;
#30899=CARTESIAN_POINT ( 'NONE',  ( -9.822455662039388358, -10.31621877034669588, 34.18098118002070152 ) ) ;
#30900=CARTESIAN_POINT ( 'NONE',  ( -2.307692307692305711, -13.04860791097971706, 34.73218667398347037 ) ) ;
#30901=CARTESIAN_POINT ( 'NONE',  ( 14.30769230769218758, -3.835265460704628371, 33.15142922262033665 ) ) ;
#30902=EDGE_LOOP ( 'NONE', ( #8980, #63344, #78099, #84071 ) ) ;
#30903=B_SPLINE_CURVE_WITH_KNOTS ( 'NONE', 3,
 ( #86749, #79968, #18269, #74994, #27679, #61901, #81311, #6089, #48833, #67345 ),
 .UNSPECIFIED., .F., .F.,
 ( 4, 2, 2, 2, 4 ),
 ( 0.0007817359430256216575, 0.0009771253907249856981, 0.001172514838424349630, 0.001367904286123713779, 0.001563293733823077711 ),
 .UNSPECIFIED. ) ;
#30904=DIRECTION ( 'NONE',  ( -0.000000000000000000, -0.9848077530122085754, -0.1736481776669273613 ) ) ;
#30905=ORIENTED_EDGE ( 'NONE', *, *, #3068, .F. ) ;
#30906=DIRECTION ( 'NONE',  ( 0.000000000000000000, -1.000000000000000000, 0.000000000000000000 ) ) ;
#30907=DIRECTION ( 'NONE',  ( -0.000000000000000000, 0.8660254037844397068, -0.4999999999999978906 ) ) ;
#30908=CARTESIAN_POINT ( 'NONE',  ( 2.084207383127976598, -12.47654668319379567, 31.42292124445336654 ) ) ;
#30909=CARTESIAN_POINT ( 'NONE',  ( 5.934729999443682402, -12.51329471203370325, 31.30864560766548976 ) ) ;
#30910=CARTESIAN_POINT ( 'NONE',  ( -6.923076923077044142, -2.625532179533778709, 30.86335684631627174 ) ) ;
#30911=CARTESIAN_POINT ( 'NONE',  ( -1.161835715637317801, -8.540255544307065350, 34.89611431652622286 ) ) ;
#30912=FACE_OUTER_BOUND ( 'NONE', #41150, .T. ) ;
#30913=ORIENTED_EDGE ( 'NONE', *, *, #38015, .T. ) ;
#30914=CARTESIAN_POINT ( 'NONE',  ( -10.86536134632696715, -9.943427161483782584, 34.11278801902876978 ) ) ;
#30915=CARTESIAN_POINT ( 'NONE',  ( -8.992157728137618378, -4.026226216239094491, 33.68668979543634379 ) ) ;
#30916=B_SPLINE_CURVE_WITH_KNOTS ( 'NONE', 3,
 ( #21439, #77268, #48909, #29535, #76380, #21884, #8822, #36294, #14686, #70959 ),
 .UNSPECIFIED., .F., .F.,
 ( 4, 2, 2, 2, 4 ),
 ( 0.000000000000000000, 0.0001954339857564070678, 0.0003908679715128141356, 0.0005863019572692211492, 0.0007817359430256282712 ),
 .UNSPECIFIED. ) ;
#30917=ORIENTED_EDGE ( 'NONE', *, *, #15698, .T. ) ;
#30918=CARTESIAN_POINT ( 'NONE',  ( -12.46153846153858424, -3.643525952248795718, 33.31231777344771672 ) ) ;
#30919=CARTESIAN_POINT ( 'NONE',  ( 14.24242186173153435, -10.21337939537584383, 33.94971097300158647 ) ) ;
#30920=CARTESIAN_POINT ( 'NONE',  ( -15.16470189741915320, -5.471508081941601098, 34.59228464037088457 ) ) ;
#30921=CYLINDRICAL_SURFACE ( 'NONE', #18438, 0.2499999999999995559 ) ;
#30922=DIRECTION ( 'NONE',  ( -0.000000000000000000, 0.8660254037844399289, -0.4999999999999980016 ) ) ;
#30923=FACE_BOUND ( 'NONE', #48303, .T. ) ;
#30924=CARTESIAN_POINT ( 'NONE',  ( 13.16168916709923664, -12.15238873228292071, 31.58232369045353849 ) ) ;
#30925=CARTESIAN_POINT ( 'NONE',  ( 17.74997677577854560, -10.92453946501459328, 33.72985991061849376 ) ) ;
#30926=CARTESIAN_POINT ( 'NONE',  ( 5.076923076923075762, -7.500000000000001776, 35.04278698407183867 ) ) ;
#30927=CARTESIAN_POINT ( 'NONE',  ( -11.78846153846153655, -7.566083408709835645, 34.74999999999999289 ) ) ;
#30928=CARTESIAN_POINT ( 'NONE',  ( 0.4615384615384611200, -12.29105614889573062, 35.45975837776705220 ) ) ;
#30929=CARTESIAN_POINT ( 'NONE',  ( -15.23076923076935074, -2.892918686052166066, 31.69288490824153470 ) ) ;
#30930=CARTESIAN_POINT ( 'NONE',  ( 8.900022577055551665, -10.54018710029568595, 33.71981072465678864 ) ) ;
#30932=B_SPLINE_CURVE_WITH_KNOTS ( 'NONE', 3,
 ( #38241, #72017, #22948, #57621, #37338, #50408, #79233, #84671, #52185, #65696 ),
 .UNSPECIFIED., .F., .F.,
 ( 4, 2, 2, 2, 4 ),
 ( 0.0007817246256747448956, 0.0009771112852218876831, 0.001172497944769030579, 0.001367884604316173475, 0.001563271263863316371 ),
 .UNSPECIFIED. ) ;
#30934=B_SPLINE_CURVE_WITH_KNOTS ( 'NONE', 3,
 ( #83224, #83678, #41348, #799, #49433, #7116, #8453, #55295, #62926, #61160 ),
 .UNSPECIFIED., .F., .F.,
 ( 4, 2, 2, 2, 4 ),
 ( 0.0007817359430256324996, 0.0009771253907249993591, 0.001172514838424366110, 0.001367904286123732861, 0.001563293733823099829 ),
 .UNSPECIFIED. ) ;
#30935=CARTESIAN_POINT ( 'NONE',  ( -7.976301055592065481, -11.47017969459904130, 32.78971311882034456 ) ) ;
#30936=CARTESIAN_POINT ( 'NONE',  ( -4.377331097570101193, -3.236172620538810385, 32.36188796281390267 ) ) ;
#30937=DIRECTION ( 'NONE',  ( 0.000000000000000000, 0.8660254037844377084, -0.5000000000000015543 ) ) ;
#30938=DIRECTION ( 'NONE',  ( 1.000000000000000000, 0.000000000000000000, 0.000000000000000000 ) ) ;
#30939=VECTOR ( 'NONE', #67024, 1000.000000000000114 ) ;
#30941=CARTESIAN_POINT ( 'NONE',  ( -16.82686865700962642, -8.346898887586322147, 34.93166121998716278 ) ) ;
#30943=EDGE_CURVE ( 'NONE', #58822, #59485, #22216, .T. ) ;
#30944=CARTESIAN_POINT ( 'NONE',  ( -16.40382289789473802, -5.643011162660950042, 34.66104346484419096 ) ) ;
#30945=CARTESIAN_POINT ( 'NONE',  ( -14.55771553191376633, -11.56360843649121684, 33.07473185843129926 ) ) ;
#30946=CARTESIAN_POINT ( 'NONE',  ( -7.596099426240392027, -10.06805714834173493, 34.32951233291982618 ) ) ;
#30947=CARTESIAN_POINT ( 'NONE',  ( 5.207713517890025123, -12.62708834333097663, 30.88030960425257021 ) ) ;
#30948=B_SPLINE_CURVE_WITH_KNOTS ( 'NONE', 3,
 ( #70586, #8890, #65142, #2120, #3445, #58379, #85873, #51613, #10658, #38125 ),
 .UNSPECIFIED., .F., .F.,
 ( 4, 2, 2, 2, 4 ),
 ( 0.000000000000000000, 0.0001954339857564074473, 0.0003908679715128148945, 0.0005863019572692223418, 0.0007817359430256297891 ),
 .UNSPECIFIED. ) ;
#30949=CARTESIAN_POINT ( 'NONE',  ( 0.4615384615383396616, -11.48612834414049644, 32.76840700105863391 ) ) ;
#30950=CARTESIAN_POINT ( 'NONE',  ( 7.846153846153846700, -10.67929555188718282, 33.92786785259544047 ) ) ;
#30951=B_SPLINE_CURVE_WITH_KNOTS ( 'NONE', 3,
 ( #50585, #49707, #1969, #64532, #63215, #1529, #56900, #64100, #2395, #7847 ),
 .UNSPECIFIED., .F., .F.,
 ( 4, 2, 2, 2, 4 ),
 ( 0.0007817246256747459798, 0.0009771112852218887673, 0.001172497944769031663, 0.001367884604316174559, 0.001563271263863317455 ),
 .UNSPECIFIED. ) ;
#30952=FACE_OUTER_BOUND ( 'NONE', #84357, .T. ) ;
#30953=CYLINDRICAL_SURFACE ( 'NONE', #83042, 0.2500000000000002220 ) ;
#30954=VERTEX_POINT ( 'NONE', #47167 ) ;
#30955=DIRECTION ( 'NONE',  ( -0.000000000000000000, 0.9848077530122085754, -0.1736481776669273613 ) ) ;
#30958=EDGE_CURVE ( 'NONE', #36124, #34697, #32762, .T. ) ;
#30959=CARTESIAN_POINT ( 'NONE',  ( 6.222779541268410597, -4.387253974876676565, 33.66317474335728832 ) ) ;
#30960=CARTESIAN_POINT ( 'NONE',  ( 2.307692307692309264, -8.973038597847269315, 34.52809138561121927 ) ) ;
#30962=CARTESIAN_POINT ( 'NONE',  ( 1.634669696253701510, -4.235687564193446164, 33.53795663066793509 ) ) ;
#30963=CARTESIAN_POINT ( 'NONE',  ( 2.438482748659258625, -10.70102852606553157, 33.91149625220312913 ) ) ;
#30964=CARTESIAN_POINT ( 'NONE',  ( 3.230769230769231726, -2.517432740324522911, 35.29906147534542527 ) ) ;
#30965=VERTEX_POINT ( 'NONE', #14274 ) ;
#30966=CARTESIAN_POINT ( 'NONE',  ( -12.68446542044531000, -9.172386477786396597, 34.72672124145550043 ) ) ;
#30967=CARTESIAN_POINT ( 'NONE',  ( -2.307692307692428724, -11.67786785259630911, 32.92929555188603530 ) ) ;
#30969=CARTESIAN_POINT ( 'NONE',  ( -4.854143535654666941, -9.332535724633407526, 34.40230450496446224 ) ) ;
#30971=CARTESIAN_POINT ( 'NONE',  ( -14.05774678934416499, -11.37275283266504111, 32.91324779482534524 ) ) ;
#30972=ORIENTED_EDGE ( 'NONE', *, *, #15935, .T. ) ;
#30973=LINE ( 'NONE', #38185, #62176 ) ;
#30974=CARTESIAN_POINT ( 'NONE',  ( 10.86543903529806698, -4.074993327901527351, 33.72946981652012255 ) ) ;
#30975=CARTESIAN_POINT ( 'NONE',  ( -1.161835843346975539, -5.913360116392399668, 34.49180327182771322 ) ) ;
#30977=ORIENTED_EDGE ( 'NONE', *, *, #45958, .T. ) ;
#30980=ADVANCED_FACE ( 'NONE', ( #33669 ), #75104, .F. ) ;
#30981=CARTESIAN_POINT ( 'NONE',  ( -9.692307692307691624, -9.780366693483667717, 34.19971097300155094 ) ) ;
#30982=DIRECTION ( 'NONE',  ( -0.000000000000000000, -0.5000000000000009992, -0.8660254037844380415 ) ) ;
#30983=CARTESIAN_POINT ( 'NONE',  ( -12.52762187249434156, -3.513871655860377086, 32.76840700105978499 ) ) ;
#30984=CARTESIAN_POINT ( 'NONE',  ( 11.53846153846153832, -4.102666532097928531, 36.13435417666054406 ) ) ;
#30985=AXIS2_PLACEMENT_3D ( 'NONE', #75230, #50713, #57926 ) ;
#30986=EDGE_CURVE ( 'NONE', #22049, #23792, #45676, .T. ) ;
#30987=ORIENTED_EDGE ( 'NONE', *, *, #32188, .T. ) ;
#30988=VERTEX_POINT ( 'NONE', #29567 ) ;
#30989=CARTESIAN_POINT ( 'NONE',  ( 15.48082354240754555, -4.943051570960394159, 34.04725096376909477 ) ) ;
#30991=VERTEX_POINT ( 'NONE', #22357 ) ;
#30992=CARTESIAN_POINT ( 'NONE',  ( 16.15384615384615330, -13.49023893513002648, 31.06009739812518688 ) ) ;
#30993=EDGE_CURVE ( 'NONE', #75626, #26115, #8856, .T. ) ;
#30994=EDGE_CURVE ( 'NONE', #21128, #50622, #87498, .T. ) ;
#30995=CARTESIAN_POINT ( 'NONE',  ( 5.933917620639865831, -3.937682226553329556, 33.60647404775217240 ) ) ;
#30996=CARTESIAN_POINT ( 'NONE',  ( -13.13456107297707121, -12.41262288849542017, 30.68299917996395010 ) ) ;
#30997=B_SPLINE_CURVE_WITH_KNOTS ( 'NONE', 3,
 ( #54479, #47621, #49051, #35095, #21134, #33775, #61229, #75212, #62555, #54930 ),
 .UNSPECIFIED., .F., .F.,
 ( 4, 2, 2, 2, 4 ),
 ( 0.000000000000000000, 0.0001954339857564070949, 0.0003908679715128141898, 0.0005863019572692212576, 0.0007817359430256283796 ),
 .UNSPECIFIED. ) ;
#30998=VECTOR ( 'NONE', #20289, 1000.000000000000114 ) ;
#30999=ORIENTED_EDGE ( 'NONE', *, *, #8197, .T. ) ;
#31001=B_SPLINE_CURVE_WITH_KNOTS ( 'NONE', 3,
 ( #68448, #6746, #34217, #60806, #61680, #2, #88313, #82864, #76086, #54486 ),
 .UNSPECIFIED., .F., .F.,
 ( 4, 2, 2, 2, 4 ),
 ( 0.0007817246256747517261, 0.0009771112852218961399, 0.001172497944769040771, 0.001367884604316185401, 0.001563271263863329815 ),
 .UNSPECIFIED. ) ;
#31002=ORIENTED_EDGE ( 'NONE', *, *, #29331, .T. ) ;
#31003=CARTESIAN_POINT ( 'NONE',  ( 8.992010310499177095, -2.600157965045224895, 30.74683119005207743 ) ) ;
#31005=CARTESIAN_POINT ( 'NONE',  ( -0.5268089074992374776, -10.90142922261923886, 33.41473453929638993 ) ) ;
#31006=CARTESIAN_POINT ( 'NONE',  ( -10.61538461538473577, -9.528491918059723176, 34.59228464037033035 ) ) ;
#31007=ORIENTED_EDGE ( 'NONE', *, *, #86259, .F. ) ;
#31008=CARTESIAN_POINT ( 'NONE',  ( 12.46153846153846168, -6.343179335718451384, 34.87096338111211935 ) ) ;
#31009=CARTESIAN_POINT ( 'NONE',  ( -1.634638621908349077, -8.432397168068783699, 34.66272746175022945 ) ) ;
#31010=CARTESIAN_POINT ( 'NONE',  ( 17.07692307692307665, -2.708943851104267164, 35.45975837776705220 ) ) ;
#31011=FACE_BOUND ( 'NONE', #23381, .T. ) ;
#31012=CARTESIAN_POINT ( 'NONE',  ( -5.999999999999998224, -2.499999999999998668, 29.75000000000001421 ) ) ;
#31013=CARTESIAN_POINT ( 'NONE',  ( 2.438218009455871638, -8.586989748646452369, 34.63063291749215011 ) ) ;
#31014=FACE_OUTER_BOUND ( 'NONE', #35745, .T. ) ;
#31015=CARTESIAN_POINT ( 'NONE',  ( 16.82694633287449193, -9.234221910056350069, 34.70572697212741531 ) ) ;
#31016=CARTESIAN_POINT ( 'NONE',  ( 9.942362003946010773, -3.136992222400443175, 32.19305428654138979 ) ) ;
#31017=AXIS2_PLACEMENT_3D ( 'NONE', #3480, #37266, #29644 ) ;
#31018=CARTESIAN_POINT ( 'NONE',  ( 17.93472999944368240, -6.835583212224500826, 34.95778746994557906 ) ) ;
#31020=EDGE_LOOP ( 'NONE', ( #7769, #42988 ) ) ;
#31021=CARTESIAN_POINT ( 'NONE',  ( -2.307692307692305711, -2.833524468853757305, 32.15551576947925838 ) ) ;
#31023=EDGE_LOOP ( 'NONE', ( #59647, #50856, #60892, #49755 ) ) ;
#31025=CARTESIAN_POINT ( 'NONE',  ( -6.700297381808512753, -8.496831190052096971, 34.64984203495476578 ) ) ;
#31026=CARTESIAN_POINT ( 'NONE',  ( 1.253923917947830313, -10.54014554554150607, 33.71984207302941883 ) ) ;
#31027=CARTESIAN_POINT ( 'NONE',  ( -6.700065571464073777, -6.503523203565942268, 34.64991518177335195 ) ) ;
#31028=CARTESIAN_POINT ( 'NONE',  ( -5.076923076923199218, -5.941354392335915335, 34.76329471203413846 ) ) ;
#31029=CARTESIAN_POINT ( 'NONE',  ( -16.15384615384615330, -12.10708131394839349, 31.69288490824020244 ) ) ;
#31030=ORIENTED_EDGE ( 'NONE', *, *, #56597, .T. ) ;
#31031=EDGE_CURVE ( 'NONE', #67701, #47174, #25261, .T. ) ;
#31032=CARTESIAN_POINT ( 'NONE',  ( 12.46153846153846168, -3.050289026998446396, 32.03036669348365706 ) ) ;
#31033=CARTESIAN_POINT ( 'NONE',  ( 6.923076923076802558, -3.835265460704628371, 33.15142922262033665 ) ) ;
#31034=CARTESIAN_POINT ( 'NONE',  ( -1.450697763975519194, -9.905515769479276145, 34.41647553114623292 ) ) ;
#31035=DIRECTION ( 'NONE',  ( 0.000000000000000000, 1.000000000000000000, 0.000000000000000000 ) ) ;
#31036=DIRECTION ( 'NONE',  ( 0.000000000000000000, 0.3420201433256610524, 0.9396926207859113145 ) ) ;
#31037=B_SPLINE_CURVE_WITH_KNOTS ( 'NONE', 3,
 ( #49422, #71448, #49850, #28253, #2544, #30033, #84547, #83212, #35013, #56175 ),
 .UNSPECIFIED., .F., .F.,
 ( 4, 2, 2, 2, 4 ),
 ( 0.0007817246256747530271, 0.0009771112852218978746, 0.001172497944769042939, 0.001367884604316188003, 0.001563271263863332851 ),
 .UNSPECIFIED. ) ;
#31039=EDGE_LOOP ( 'NONE', ( #57146, #87123, #62336, #17630 ) ) ;
#31041=EDGE_CURVE ( 'NONE', #52632, #49352, #50701, .T. ) ;
#31042=DIRECTION ( 'NONE',  ( 0.000000000000000000, 0.000000000000000000, 1.000000000000000000 ) ) ;
#31044=CARTESIAN_POINT ( 'NONE',  ( 17.14217821643591932, -4.320704448112858032, 33.92786785259548310 ) ) ;
#31045=CARTESIAN_POINT ( 'NONE',  ( 7.846153846153723244, -12.51329471203414379, 31.30864560766407578 ) ) ;
#31046=CARTESIAN_POINT ( 'NONE',  ( -16.21992956480203318, -2.721908614388770964, 31.22303859784723912 ) ) ;
#31047=FACE_OUTER_BOUND ( 'NONE', #49423, .T. ) ;
#31049=EDGE_CURVE ( 'NONE', #70248, #87025, #2960, .T. ) ;
#31050=CARTESIAN_POINT ( 'NONE',  ( 16.15384615384615330, -13.87047571288749737, 32.06866353760679544 ) ) ;
#31051=ORIENTED_EDGE ( 'NONE', *, *, #8596, .T. ) ;
#31052=CARTESIAN_POINT ( 'NONE',  ( -0.4615384615385840772, -3.083524468854526912, 32.58852847137268327 ) ) ;
#31053=CARTESIAN_POINT ( 'NONE',  ( -2.057746898314262385, -12.68172785388650681, 30.59649109432439218 ) ) ;
#31054=EDGE_LOOP ( 'NONE', ( #84100, #37720, #11315, #1549 ) ) ;
#31055=CARTESIAN_POINT ( 'NONE',  ( -13.44988583057615905, -11.48612834413959582, 32.76840700105983473 ) ) ;
#31056=CARTESIAN_POINT ( 'NONE',  ( -9.758391103263569732, -12.10708131394839349, 31.69288490824020244 ) ) ;
#31057=DIRECTION ( 'NONE',  ( -0.000000000000000000, -0.8660254037844399289, -0.4999999999999980016 ) ) ;
#31059=AXIS2_PLACEMENT_3D ( 'NONE', #30387, #57857, #69598 ) ;
#31060=CARTESIAN_POINT ( 'NONE',  ( -5.869474561766355514, -5.070358843744210198, 34.40418822224088302 ) ) ;
#31061=CARTESIAN_POINT ( 'NONE',  ( -4.403869391139118683, -9.271318131107980420, 34.42618302367067429 ) ) ;
#31062=CARTESIAN_POINT ( 'NONE',  ( -6.989160334032801458, -4.786620604624113540, 33.94971097300155805 ) ) ;
#31064=EDGE_LOOP ( 'NONE', ( #46758, #46812, #26316, #47000 ) ) ;
#31065=CARTESIAN_POINT ( 'NONE',  ( -4.403822884788509029, -4.943428324936578910, 34.04746400365624481 ) ) ;
#31067=B_SPLINE_CURVE_WITH_KNOTS ( 'NONE', 3,
 ( #34860, #81295, #81736, #20020, #47487, #7404, #6951, #74979, #88954, #47040 ),
 .UNSPECIFIED., .F., .F.,
 ( 4, 2, 2, 2, 4 ),
 ( 0.0007817359430256294638, 0.0009771253907249952391, 0.001172514838424361123, 0.001367904286123726790, 0.001563293733823092673 ),
 .UNSPECIFIED. ) ;
#31068=CARTESIAN_POINT ( 'NONE',  ( -4.219116154402471786, -5.941354392334500467, 34.76329471203369792 ) ) ;
#31070=ADVANCED_FACE ( 'NONE', ( #77742 ), #2515, .F. ) ;
#31071=CARTESIAN_POINT ( 'NONE',  ( -3.480792468062196221, -9.271318131107980420, 34.42618302367067429 ) ) ;
#31072=CARTESIAN_POINT ( 'NONE',  ( 14.17700170458200404, -4.684245665217972032, 34.18127051446801090 ) ) ;
#31073=CARTESIAN_POINT ( 'NONE',  ( -13.25408994638174320, -6.808710257144161559, 34.95449254468098843 ) ) ;
#31074=VERTEX_POINT ( 'NONE', #23240 ) ;
#31076=DIRECTION ( 'NONE',  ( -0.000000000000000000, 0.9396926207859092051, -0.3420201433256662704 ) ) ;
#31077=EDGE_CURVE ( 'NONE', #14975, #6775, #42641, .T. ) ;
#31078=ORIENTED_EDGE ( 'NONE', *, *, #22371, .F. ) ;
#31079=CARTESIAN_POINT ( 'NONE',  ( -18.13014796973169851, -5.070767119584671079, 34.40440758774516183 ) ) ;
#31080=VERTEX_POINT ( 'NONE', #16490 ) ;
#31081=CARTESIAN_POINT ( 'NONE',  ( 14.37294787896833448, -12.27809138561124591, 31.22303859784720359 ) ) ;
#31082=CARTESIAN_POINT ( 'NONE',  ( -1.450697763975519416, -11.91647553114624181, 32.58852847137148245 ) ) ;
#31083=CARTESIAN_POINT ( 'NONE',  ( -0.3962833220256232192, -6.835583212224609184, 34.95778746994559327 ) ) ;
#31085=CARTESIAN_POINT ( 'NONE',  ( -0.7115384615384606759, -2.249999999999998668, 29.75000000000000355 ) ) ;
#31086=ORIENTED_EDGE ( 'NONE', *, *, #8407, .F. ) ;
#31087=LINE ( 'NONE', #17134, #54261 ) ;
#31088=EDGE_LOOP ( 'NONE', ( #20500, #52447 ) ) ;
#31089=CARTESIAN_POINT ( 'NONE',  ( 2.241609928332172430, -9.058645607665454236, 34.76329471203372634 ) ) ;
#31090=CARTESIAN_POINT ( 'NONE',  ( -6.923076923076922462, -13.87047571288749737, 32.06866353760679544 ) ) ;
#31091=VERTEX_POINT ( 'NONE', #57022 ) ;
#31092=CARTESIAN_POINT ( 'NONE',  ( 11.76124120743960333, -12.69155399931963046, 30.53255429739157734 ) ) ;
#31093=CARTESIAN_POINT ( 'NONE',  ( -14.37296275365308418, -10.90142922261923886, 33.41473453929638993 ) ) ;
#31094=CARTESIAN_POINT ( 'NONE',  ( -11.53846153846153655, -2.721908614388771852, 31.22303859784724978 ) ) ;
#31095=VECTOR ( 'NONE', #19142, 1000.000000000000114 ) ;
#31096=CARTESIAN_POINT ( 'NONE',  ( 5.010839665967195877, -8.973038597847269315, 34.52809138561120506 ) ) ;
#31097=CARTESIAN_POINT ( 'NONE',  ( -11.28851612908349722, -3.520799739797214389, 33.17531984108286025 ) ) ;
#31098=EDGE_CURVE ( 'NONE', #58205, #72630, #4855, .T. ) ;
#31100=ORIENTED_EDGE ( 'NONE', *, *, #55361, .T. ) ;
#31101=ORIENTED_EDGE ( 'NONE', *, *, #69682, .F. ) ;
#31102=CARTESIAN_POINT ( 'NONE',  ( 3.100621261037536769, -5.915902021225892149, 34.75552854090298638 ) ) ;
#31103=VERTEX_POINT ( 'NONE', #11517 ) ;
#31104=EDGE_CURVE ( 'NONE', #80116, #14630, #20941, .T. ) ;
#31105=EDGE_CURVE ( 'NONE', #67886, #76288, #73618, .T. ) ;
#31106=DIRECTION ( 'NONE',  ( 0.000000000000000000, 0.6427876096865373645, -0.7660444431189797898 ) ) ;
#31107=CARTESIAN_POINT ( 'NONE',  ( 6.130525438233648039, -10.31582465632705237, 34.18122507451815295 ) ) ;
#31108=ORIENTED_EDGE ( 'NONE', *, *, #26331, .F. ) ;
#31109=B_SPLINE_CURVE_WITH_KNOTS ( 'NONE', 3,
 ( #24716, #25159, #16617, #85977, #72008, #80108 ),
 .UNSPECIFIED., .F., .F.,
 ( 4, 2, 4 ),
 ( 0.0003909569690057772317, 0.0005862646681846011513, 0.0007815723673634250709 ),
 .UNSPECIFIED. ) ;
#31110=ORIENTED_EDGE ( 'NONE', *, *, #4052, .T. ) ;
#31112=CARTESIAN_POINT ( 'NONE',  ( -10.61538461538461320, -3.050289026998446396, 32.03036669348365706 ) ) ;
#31113=VERTEX_POINT ( 'NONE', #32664 ) ;
#31114=B_SPLINE_CURVE_WITH_KNOTS ( 'NONE', 3,
 ( #69966, #86037, #48804, #83497, #77612, #45030, #35751, #14583, #7830, #1516 ),
 .UNSPECIFIED., .F., .F.,
 ( 4, 2, 2, 2, 4 ),
 ( 0.000000000000000000, 0.0001954339857564054144, 0.0003908679715128108288, 0.0005863019572692162703, 0.0007817359430256216575 ),
 .UNSPECIFIED. ) ;
#31115=CARTESIAN_POINT ( 'NONE',  ( 11.78851585009985570, -11.28795663066794575, 33.01431243580653785 ) ) ;
#31116=VECTOR ( 'NONE', #46152, 1000.000000000000000 ) ;
#31117=CYLINDRICAL_SURFACE ( 'NONE', #73331, 0.2500000000000008882 ) ;
#31118=EDGE_CURVE ( 'NONE', #36238, #18936, #540, .T. ) ;
#31120=FACE_BOUND ( 'NONE', #34707, .T. ) ;
#31121=ORIENTED_EDGE ( 'NONE', *, *, #20394, .T. ) ;
#31122=CARTESIAN_POINT ( 'NONE',  ( -5.076923076923199218, -3.643525952248796163, 33.31231777344771672 ) ) ;
#31124=FACE_OUTER_BOUND ( 'NONE', #21119, .T. ) ;
#31126=LINE ( 'NONE', #16727, #79753 ) ;
#31129=CARTESIAN_POINT ( 'NONE',  ( -7.146003140593069958, -6.503392248772476236, 34.64988816332204635 ) ) ;
#31130=ORIENTED_EDGE ( 'NONE', *, *, #13994, .T. ) ;
#31131=ORIENTED_EDGE ( 'NONE', *, *, #58604, .F. ) ;
#31132=CARTESIAN_POINT ( 'NONE',  ( -0.5916856709766823430, -9.418419913701741919, 34.36755862841477693 ) ) ;
#31133=CARTESIAN_POINT ( 'NONE',  ( 1.384615384615386802, -3.937682226553329556, 33.60647404775216529 ) ) ;
#31134=CYLINDRICAL_SURFACE ( 'NONE', #68671, 0.2499999999999998890 ) ;
#31136=CARTESIAN_POINT ( 'NONE',  ( -14.30769230769230660, -11.91647553114624181, 32.58852847137148245 ) ) ;
#31137=CARTESIAN_POINT ( 'NONE',  ( 14.30769230769231015, -2.833524468853757305, 32.15551576947925838 ) ) ;
#31138=EDGE_LOOP ( 'NONE', ( #53784, #73211 ) ) ;
#31140=CARTESIAN_POINT ( 'NONE',  ( -5.143005456283209931, -6.343179335718451384, 34.87096338111212646 ) ) ;
#31141=CARTESIAN_POINT ( 'NONE',  ( 17.77651507543566822, -3.562934362175799841, 33.22335522853832401 ) ) ;
#31142=CARTESIAN_POINT ( 'NONE',  ( -1.514762594053606692, -3.817052484675422797, 33.13202310037935661 ) ) ;
#31143=CARTESIAN_POINT ( 'NONE',  ( -13.63463860883683942, -12.68155406624981119, 30.59749803192733708 ) ) ;
#31144=ORIENTED_EDGE ( 'NONE', *, *, #67457, .T. ) ;
#31145=ADVANCED_FACE ( 'NONE', ( #86751 ), #79078, .F. ) ;
#31146=VERTEX_POINT ( 'NONE', #17830 ) ;
#31147=FACE_BOUND ( 'NONE', #38198, .T. ) ;
#31150=DIRECTION ( 'NONE',  ( 0.000000000000000000, 0.9396926207859126468, -0.3420201433256571111 ) ) ;
#31152=ORIENTED_EDGE ( 'NONE', *, *, #13427, .T. ) ;
#31153=CARTESIAN_POINT ( 'NONE',  ( -7.596099534515528440, -4.235687564193445276, 33.53795663066793509 ) ) ;
#31154=CARTESIAN_POINT ( 'NONE',  ( -10.74607608205217346, -6.413092428213692742, 34.63065189839063152 ) ) ;
#31155=CARTESIAN_POINT ( 'NONE',  ( 11.53846153846153832, -13.53365097954675988, 30.81389545987213552 ) ) ;
#31156=DIRECTION ( 'NONE',  ( -0.000000000000000000, -0.8660254037844399289, -0.4999999999999980016 ) ) ;
#31157=EDGE_LOOP ( 'NONE', ( #64251, #7757, #5524, #71593 ) ) ;
#31158=EDGE_CURVE ( 'NONE', #41427, #35812, #37054, .T. ) ;
#31159=CARTESIAN_POINT ( 'NONE',  ( -7.846153846153844924, -1.215029322943914858, 32.30358669280327177 ) ) ;
#31160=ORIENTED_EDGE ( 'NONE', *, *, #65566, .T. ) ;
#31161=CARTESIAN_POINT ( 'NONE',  ( 16.85399685940691938, -10.61292498521070549, 33.66303323003028680 ) ) ;
#31162=ORIENTED_EDGE ( 'NONE', *, *, #30444, .T. ) ;
#31163=CARTESIAN_POINT ( 'NONE',  ( 15.29683758177167086, -8.120952969808772792, 34.71129190929999453 ) ) ;
#31164=CARTESIAN_POINT ( 'NONE',  ( 24.00000000000000000, -5.499999999999981348, 27.75000000000000000 ) ) ;
#31165=CARTESIAN_POINT ( 'NONE',  ( -7.715628407920199550, -3.625058011473227815, 33.29252011169590020 ) ) ;
#31166=CARTESIAN_POINT ( 'NONE',  ( 10.36540787133602670, -12.41104346484419452, 31.60698883733904196 ) ) ;
#31167=DIRECTION ( 'NONE',  ( 0.000000000000000000, 0.9396926207859126468, 0.3420201433256571111 ) ) ;
#31168=EDGE_CURVE ( 'NONE', #12391, #48157, #79974, .T. ) ;
#31169=CIRCLE ( 'NONE', #34000, 0.2500000000000002220 ) ;
#31172=ORIENTED_EDGE ( 'NONE', *, *, #43182, .T. ) ;
#31173=CARTESIAN_POINT ( 'NONE',  ( 14.24242230713598900, -2.379036618887870436, 30.90682066428147934 ) ) ;
#31174=FACE_OUTER_BOUND ( 'NONE', #59794, .T. ) ;
#31176=ORIENTED_EDGE ( 'NONE', *, *, #19598, .T. ) ;
#31177=EDGE_LOOP ( 'NONE', ( #83754, #65165, #89066, #23673 ) ) ;
#31178=CARTESIAN_POINT ( 'NONE',  ( -4.153846153846152411, -12.78798330534102767, 29.49999999999997868 ) ) ;
#31179=CARTESIAN_POINT ( 'NONE',  ( -14.17716686945866833, -2.647132371071621471, 31.75357179365171589 ) ) ;
#31180=B_SPLINE_CURVE_WITH_KNOTS ( 'NONE', 3,
 ( #41857, #55795, #34648, #76521, #62115, #6726, #81962, #420, #8066, #40532 ),
 .UNSPECIFIED., .F., .F.,
 ( 4, 2, 2, 2, 4 ),
 ( 0.000000000000000000, 0.0001954339857564063089, 0.0003908679715128126177, 0.0005863019572692189808, 0.0007817359430256252354 ),
 .UNSPECIFIED. ) ;
#31181=EDGE_CURVE ( 'NONE', #10084, #60048, #53379, .T. ) ;
#31182=B_SPLINE_CURVE_WITH_KNOTS ( 'NONE', 3,
 ( #37768, #58466, #38659, #85960, #58924, #86430, #24241, #44958, #45856, #73340 ),
 .UNSPECIFIED., .F., .F.,
 ( 4, 2, 2, 2, 4 ),
 ( 0.000000000000000000, 0.0001954339857564097512, 0.0003908679715128195024, 0.0005863019572692292807, 0.0007817359430256390048 ),
 .UNSPECIFIED. ) ;
#31183=CARTESIAN_POINT ( 'NONE',  ( 17.20771351789003489, -3.338503747796866872, 32.95102852606552801 ) ) ;
#31185=CARTESIAN_POINT ( 'NONE',  ( 16.02369818411445834, -10.31621877034669588, 34.18098118002070152 ) ) ;
#31186=ADVANCED_FACE ( 'NONE', ( #19158 ), #26359, .F. ) ;
#31187=CARTESIAN_POINT ( 'NONE',  ( 16.28463659481310799, -3.338503747796866872, 32.95102852606552801 ) ) ;
#31190=AXIS2_PLACEMENT_3D ( 'NONE', #82503, #20781, #47361 ) ;
#31191=CARTESIAN_POINT ( 'NONE',  ( 6.223011351612851350, -10.61302985866383963, 33.66295027996417843 ) ) ;
#31192=DIRECTION ( 'NONE',  ( 0.000000000000000000, 0.000000000000000000, 1.000000000000000000 ) ) ;
#31193=CARTESIAN_POINT ( 'NONE',  ( 7.173131342990376247, -6.523592122091591783, 34.90882529074906415 ) ) ;
#31194=CARTESIAN_POINT ( 'NONE',  ( 9.469380733400841521, -2.523278758544489797, 31.42238647778637528 ) ) ;
#31195=VERTEX_POINT ( 'NONE', #61458 ) ;
#31196=CARTESIAN_POINT ( 'NONE',  ( -7.596099534515530216, -3.627508038966690496, 32.91356715214248396 ) ) ;
#31197=AXIS2_PLACEMENT_3D ( 'NONE', #6308, #27016, #54477 ) ;
#31198=ORIENTED_EDGE ( 'NONE', *, *, #47661, .T. ) ;
#31199=CARTESIAN_POINT ( 'NONE',  ( -17.20761368003338987, -2.494641256782729855, 31.33461815524612959 ) ) ;
#31202=CARTESIAN_POINT ( 'NONE',  ( 17.77707304109313924, -10.01117774369187252, 34.36070679894347535 ) ) ;
#31203=ORIENTED_EDGE ( 'NONE', *, *, #32299, .F. ) ;
#31205=CARTESIAN_POINT ( 'NONE',  ( 12.59232890250541281, -10.70102852606553157, 33.91149625220312913 ) ) ;
#31208=CARTESIAN_POINT ( 'NONE',  ( -4.946132635956127288, -10.70102852606553157, 33.91149625220312913 ) ) ;
#31209=VERTEX_POINT ( 'NONE', #19597 ) ;
#31211=VERTEX_POINT ( 'NONE', #61023 ) ;
#31212=CARTESIAN_POINT ( 'NONE',  ( -10.61538461538461320, -12.37446782046654192, 30.86335684631486131 ) ) ;
#31213=B_SPLINE_CURVE_WITH_KNOTS ( 'NONE', 3,
 ( #33895, #33461, #61353, #34781, #76663, #560 ),
 .UNSPECIFIED., .F., .F.,
 ( 4, 2, 4 ),
 ( 0.0003909569690057828153, 0.0005862646681846093912, 0.0007815723673634359129 ),
 .UNSPECIFIED. ) ;
#31214=CARTESIAN_POINT ( 'NONE',  ( 6.000000000000001776, -1.117168528481311540, 33.14645433367849847 ) ) ;
#31215=ADVANCED_FACE ( 'NONE', ( #47504 ), #34880, .F. ) ;
#31216=CARTESIAN_POINT ( 'NONE',  ( -3.007342268907659655, -7.630147231320743018, 34.74852402298682819 ) ) ;
#31218=CARTESIAN_POINT ( 'NONE',  ( 7.622668921589514035, -12.47654668319379567, 31.42292124445336654 ) ) ;
#31220=CARTESIAN_POINT ( 'NONE',  ( -6.130691466667555822, -4.118384482072085184, 33.43331474514187107 ) ) ;
#31221=CARTESIAN_POINT ( 'NONE',  ( 15.23076923076911093, -11.94971097300221174, 32.03036669348237098 ) ) ;
#31222=B_SPLINE_CURVE_WITH_KNOTS ( 'NONE', 3,
 ( #56782, #62215, #62646, #69422, #22121, #55898, #22560, #7729, #83838, #14929 ),
 .UNSPECIFIED., .F., .F.,
 ( 4, 2, 2, 2, 4 ),
 ( 0.000000000000000000, 0.0001954339857564080707, 0.0003908679715128161414, 0.0005863019572692241849, 0.0007817359430256322827 ),
 .UNSPECIFIED. ) ;
#31223=EDGE_LOOP ( 'NONE', ( #42373, #13486, #28208, #68875 ) ) ;
#31229=VERTEX_POINT ( 'NONE', #13729 ) ;
#31231=DIRECTION ( 'NONE',  ( -0.000000000000000000, -0.7660444431189791237, -0.6427876096865379196 ) ) ;
#31232=CARTESIAN_POINT ( 'NONE',  ( -1.318547033612945008, -12.37446782046654192, 30.86335684631486842 ) ) ;
#31233=EDGE_CURVE ( 'NONE', #79258, #77986, #88969, .T. ) ;
#31235=LINE ( 'NONE', #37998, #20662 ) ;
#31236=CARTESIAN_POINT ( 'NONE',  ( 7.715463243043538810, -12.62707690430377383, 30.88035979386743435 ) ) ;
#31237=CARTESIAN_POINT ( 'NONE',  ( 6.923076923076924238, -3.669653830205710676, 35.88435417666054406 ) ) ;
#31238=ADVANCED_FACE ( 'NONE', ( #20484 ), #67348, .F. ) ;
#31239=DIRECTION ( 'NONE',  ( -0.000000000000000000, 0.9396926207859093161, -0.3420201433256663259 ) ) ;
#31240=CARTESIAN_POINT ( 'NONE',  ( -5.207482990536439260, -2.254533558242299396, 29.97296025877828285 ) ) ;
#31241=CARTESIAN_POINT ( 'NONE',  ( -4.283993363284373856, -10.19110544564092002, 33.96427741523702792 ) ) ;
#31243=ORIENTED_EDGE ( 'NONE', *, *, #56904, .F. ) ;
#31244=ORIENTED_EDGE ( 'NONE', *, *, #61308, .T. ) ;
#31245=EDGE_CURVE ( 'NONE', #66835, #78733, #16630, .T. ) ;
#31246=CARTESIAN_POINT ( 'NONE',  ( 6.065255139512837346, -12.51329471203373700, 31.30864560766537963 ) ) ;
#31247=ORIENTED_EDGE ( 'NONE', *, *, #58663, .F. ) ;
#31248=DIRECTION ( 'NONE',  ( -0.000000000000000000, -0.9848077530122086864, -0.1736481776669273613 ) ) ;
#31249=CARTESIAN_POINT ( 'NONE',  ( 18.00000000000031264, -2.255955759149395501, 30.00000000000324363 ) ) ;
#31252=FACE_OUTER_BOUND ( 'NONE', #80098, .T. ) ;
#31253=ORIENTED_EDGE ( 'NONE', *, *, #43509, .F. ) ;
#31254=B_SPLINE_CURVE_WITH_KNOTS ( 'NONE', 3,
 ( #22466, #8076, #48603, #55806, #77411, #36860, #15721, #14837, #43184, #83742 ),
 .UNSPECIFIED., .F., .F.,
 ( 4, 2, 2, 2, 4 ),
 ( 0.000000000000000000, 0.0001954339857564080707, 0.0003908679715128161414, 0.0005863019572692241849, 0.0007817359430256322827 ),
 .UNSPECIFIED. ) ;
#31255=B_SPLINE_CURVE_WITH_KNOTS ( 'NONE', 3,
 ( #58276, #51498, #85767, #87117, #71346, #24942 ),
 .UNSPECIFIED., .F., .F.,
 ( 4, 2, 4 ),
 ( 0.0003909569690057874774, 0.0005862646681846157880, 0.0007815723673634440444 ),
 .UNSPECIFIED. ) ;
#31256=B_SPLINE_CURVE_WITH_KNOTS ( 'NONE', 3,
 ( #55752, #63394, #42259, #1703, #77359, #15666, #49002, #63842, #69717, #2570 ),
 .UNSPECIFIED., .F., .F.,
 ( 4, 2, 2, 2, 4 ),
 ( 0.000000000000000000, 0.0001954339857564078267, 0.0003908679715128156535, 0.0005863019572692235344, 0.0007817359430256313069 ),
 .UNSPECIFIED. ) ;
#31257=EDGE_LOOP ( 'NONE', ( #57905, #15103 ) ) ;
#31258=CARTESIAN_POINT ( 'NONE',  ( -2.307692307692427391, -12.46129190930018460, 30.37095296980731973 ) ) ;
#31259=AXIS2_PLACEMENT_3D ( 'NONE', #61357, #55058, #40227 ) ;
#31260=B_SPLINE_CURVE_WITH_KNOTS ( 'NONE', 3,
 ( #33174, #87695, #32725, #88149, #26422, #52545, #11123, #38601, #52102, #18779 ),
 .UNSPECIFIED., .F., .F.,
 ( 4, 2, 2, 2, 4 ),
 ( 0.000000000000000000, 0.0001954339881912776238, 0.0003908679763825552477, 0.0005863019645738329257, 0.0007817359527651104954 ),
 .UNSPECIFIED. ) ;
#31261=EDGE_CURVE ( 'NONE', #12327, #40886, #33114, .T. ) ;
#31262=ORIENTED_EDGE ( 'NONE', *, *, #78491, .T. ) ;
#31263=FACE_BOUND ( 'NONE', #35877, .T. ) ;
#31264=CARTESIAN_POINT ( 'NONE',  ( 15.10062202133100939, -10.19110544564092002, 33.96427741523702792 ) ) ;
#31265=DIRECTION ( 'NONE',  ( -0.000000000000000000, -0.5000000000000009992, -0.8660254037844380415 ) ) ;
#31266=VERTEX_POINT ( 'NONE', #74548 ) ;
#31267=CARTESIAN_POINT ( 'NONE',  ( 14.05766907039934033, -2.823816976329317274, 31.52131813110795733 ) ) ;
#31269=DIRECTION ( 'NONE',  ( -0.000000000000000000, -0.000000000000000000, -1.000000000000000000 ) ) ;
#31270=AXIS2_PLACEMENT_3D ( 'NONE', #51431, #38398, #71726 ) ;
#31271=CARTESIAN_POINT ( 'NONE',  ( -18.00000000000000000, -3.937682226553330445, 33.60647404775216529 ) ) ;
#31273=DIRECTION ( 'NONE',  ( -0.000000000000000000, 0.3420201433256694901, -0.9396926207859082059 ) ) ;
#31274=CARTESIAN_POINT ( 'NONE',  ( 3.164685819813350509, -12.10708131394839349, 31.69288490824020244 ) ) ;
#31275=ORIENTED_EDGE ( 'NONE', *, *, #33261, .F. ) ;
#31276=CARTESIAN_POINT ( 'NONE',  ( -6.792285115252135519, -8.999086150933472084, 34.52020707165672064 ) ) ;
#31277=FACE_OUTER_BOUND ( 'NONE', #13096, .T. ) ;
#31280=DIRECTION ( 'NONE',  ( -0.000000000000000000, -0.7660444431189791237, -0.6427876096865379196 ) ) ;
#31282=CARTESIAN_POINT ( 'NONE',  ( 7.623327153674845036, -7.369208160676173236, 34.74850200257122879 ) ) ;
#31283=CARTESIAN_POINT ( 'NONE',  ( 6.000000000000001776, -1.790695186598648903, 34.54067556320373455 ) ) ;
#31284=CARTESIAN_POINT ( 'NONE',  ( 17.20744851515672025, -5.070358843744208421, 34.40418822224088302 ) ) ;
#31285=CYLINDRICAL_SURFACE ( 'NONE', #57698, 0.2499999999999973355 ) ;
#31286=CARTESIAN_POINT ( 'NONE',  ( 8.545745844666434721, -3.019605429927184392, 32.48692288466676814 ) ) ;
#31288=EDGE_CURVE ( 'NONE', #24104, #81961, #64968, .T. ) ;
#31289=CARTESIAN_POINT ( 'NONE',  ( 1.515141086378948954, -11.46989282347013095, 32.79007818306219946 ) ) ;
#31290=CARTESIAN_POINT ( 'NONE',  ( 3.100209317155866007, -2.254533558242299396, 29.97296025877828285 ) ) ;
#31291=CARTESIAN_POINT ( 'NONE',  ( -16.15384615384627409, -10.33852847137269571, 34.16647553114546554 ) ) ;
#31295=EDGE_LOOP ( 'NONE', ( #55098, #25914, #67599, #2712 ) ) ;
#31296=AXIS2_PLACEMENT_3D ( 'NONE', #68037, #49079, #60824 ) ;
#31297=VERTEX_POINT ( 'NONE', #42100 ) ;
#31298=CARTESIAN_POINT ( 'NONE',  ( -7.846153846153967493, -2.657715359629662544, 31.77849191805970364 ) ) ;
#31299=EDGE_LOOP ( 'NONE', ( #80342, #68475, #83680, #69673 ) ) ;
#31302=CARTESIAN_POINT ( 'NONE',  ( -17.75005448165186195, -5.852078868378308485, 34.47109172314382874 ) ) ;
#31303=ADVANCED_FACE ( 'NONE', ( #1099 ), #16383, .F. ) ;
#31304=CARTESIAN_POINT ( 'NONE',  ( -5.934744860487160878, -11.67786785259547777, 32.92929555188713664 ) ) ;
#31305=CARTESIAN_POINT ( 'NONE',  ( -6.000000000000119904, -9.442884908241554243, 34.35708131394783038 ) ) ;
#31306=DIRECTION ( 'NONE',  ( -0.000000000000000000, -0.8660254037844397068, -0.4999999999999978906 ) ) ;
#31307=DIRECTION ( 'NONE',  ( -0.000000000000000000, -0.000000000000000000, -1.000000000000000000 ) ) ;
#31308=LINE ( 'NONE', #51545, #42996 ) ;
#31309=CARTESIAN_POINT ( 'NONE',  ( -7.780898274877817933, -12.27809138561124591, 31.22303859784720359 ) ) ;
#31310=B_SPLINE_CURVE_WITH_KNOTS ( 'NONE', 3,
 ( #32433, #31083, #17130, #64864, #45492, #39200, #58553, #44590, #51785, #18035 ),
 .UNSPECIFIED., .F., .F.,
 ( 4, 2, 2, 2, 4 ),
 ( 0.0007817246256747470640, 0.0009771112852218905021, 0.001172497944769033832, 0.001367884604316177161, 0.001563271263863320491 ),
 .UNSPECIFIED. ) ;
#31312=EDGE_CURVE ( 'NONE', #12423, #47330, #81106, .T. ) ;
#31313=ADVANCED_FACE ( 'NONE', ( #63236 ), #83976, .F. ) ;
#31315=CARTESIAN_POINT ( 'NONE',  ( 13.16113046005105680, -3.562934362175799841, 33.22335522853832401 ) ) ;
#31316=VECTOR ( 'NONE', #54345, 1000.000000000000227 ) ;
#31317=FACE_OUTER_BOUND ( 'NONE', #36320, .T. ) ;
#31318=EDGE_CURVE ( 'NONE', #74870, #60596, #46510, .T. ) ;
#31319=VERTEX_POINT ( 'NONE', #43851 ) ;
#31321=DIRECTION ( 'NONE',  ( -0.000000000000000000, -0.1736481776669307198, -0.9848077530122080203 ) ) ;
#31323=CARTESIAN_POINT ( 'NONE',  ( -3.230769230769229949, -12.37446782046654192, 30.86335684631486131 ) ) ;
#31324=CARTESIAN_POINT ( 'NONE',  ( 5.076923076923075762, -2.721908614388771852, 31.22303859784724978 ) ) ;
#31325=CARTESIAN_POINT ( 'NONE',  ( 8.546304551714618114, -11.76352882383564769, 32.36236540154569497 ) ) ;
#31326=CARTESIAN_POINT ( 'NONE',  ( -0.6850234052624096792, -6.760086850603068243, 34.69517049084099369 ) ) ;
#31327=AXIS2_PLACEMENT_3D ( 'NONE', #86122, #24397, #38371 ) ;
#31328=ORIENTED_EDGE ( 'NONE', *, *, #29791, .F. ) ;
#31329=CYLINDRICAL_SURFACE ( 'NONE', #12727, 0.2500000000000008882 ) ;
#31330=VERTEX_POINT ( 'NONE', #42977 ) ;
#31331=VECTOR ( 'NONE', #5338, 1000.000000000000000 ) ;
#31332=ORIENTED_EDGE ( 'NONE', *, *, #87497, .F. ) ;
#31333=ADVANCED_FACE ( 'NONE', ( #76309 ), #36225, .F. ) ;
#31334=DIRECTION ( 'NONE',  ( -0.000000000000000000, 0.6427876096865404731, -0.7660444431189771253 ) ) ;
#31335=CARTESIAN_POINT ( 'NONE',  ( 6.250000000001437961, -7.500000000000155431, 34.75000000000007105 ) ) ;
#31336=CARTESIAN_POINT ( 'NONE',  ( 0.4615384615384611200, -13.78497067705608181, 32.30358669280327177 ) ) ;
#31338=DIRECTION ( 'NONE',  ( -0.000000000000000000, 0.1736481776669307198, -0.9848077530122080203 ) ) ;
#31339=DIRECTION ( 'NONE',  ( -0.000000000000000000, 0.9848077530122086864, -0.1736481776669273891 ) ) ;
#31340=VERTEX_POINT ( 'NONE', #84417 ) ;
#31341=ORIENTED_EDGE ( 'NONE', *, *, #81092, .F. ) ;
#31342=B_SPLINE_CURVE_WITH_KNOTS ( 'NONE', 3,
 ( #24170, #79579, #64710, #71917, #31381, #71036, #30055, #51623, #10229, #44883 ),
 .UNSPECIFIED., .F., .F.,
 ( 4, 2, 2, 2, 4 ),
 ( 0.000000000000000000, 0.0001954339857564079894, 0.0003908679715128159787, 0.0005863019572692239681, 0.0007817359430256319575 ),
 .UNSPECIFIED. ) ;
#31343=EDGE_LOOP ( 'NONE', ( #37603, #52277, #83317, #24705 ) ) ;
#31344=CARTESIAN_POINT ( 'NONE',  ( 1.253923917947829203, -11.18331474514187995, 33.13161551792790505 ) ) ;
#31345=CARTESIAN_POINT ( 'NONE',  ( -16.08859101433330707, -9.528491918058456633, 34.59228464037085615 ) ) ;
#31346=CARTESIAN_POINT ( 'NONE',  ( 4.284371592079798674, -3.625058011473227815, 33.29252011169590020 ) ) ;
#31347=CARTESIAN_POINT ( 'NONE',  ( -15.16551365949320562, -3.300289026998473041, 32.46337939537591666 ) ) ;
#31349=CARTESIAN_POINT ( 'NONE',  ( -4.153846153846273204, -8.613356846316285953, 34.62446782046622218 ) ) ;
#31350=CARTESIAN_POINT ( 'NONE',  ( 17.93472955403921887, -8.613356846314824011, 34.62446782046655613 ) ) ;
#31351=VERTEX_POINT ( 'NONE', #37087 ) ;
#31352=ORIENTED_EDGE ( 'NONE', *, *, #63586, .F. ) ;
#31354=ORIENTED_EDGE ( 'NONE', *, *, #45373, .T. ) ;
#31355=ADVANCED_FACE ( 'NONE', ( #76764 ), #15950, .F. ) ;
#31356=CARTESIAN_POINT ( 'NONE',  ( -12.52680890749923570, -11.48612834413959582, 32.76840700105983473 ) ) ;
#31357=ORIENTED_EDGE ( 'NONE', *, *, #17336, .T. ) ;
#31358=CARTESIAN_POINT ( 'NONE',  ( -10.55012947587177941, -4.320704448112861584, 33.92786785259548310 ) ) ;
#31361=ORIENTED_EDGE ( 'NONE', *, *, #52920, .T. ) ;
#31362=VECTOR ( 'NONE', #62762, 1000.000000000000000 ) ;
#31363=CARTESIAN_POINT ( 'NONE',  ( -13.51530685128294529, -12.11776431015576172, 31.66791131148498906 ) ) ;
#31364=ORIENTED_EDGE ( 'NONE', *, *, #82548, .T. ) ;
#31367=CARTESIAN_POINT ( 'NONE',  ( 7.623226887246994821, -4.026226216239095379, 33.68668979543632958 ) ) ;
#31368=DIRECTION ( 'NONE',  ( -0.000000000000000000, 0.3420201433256694901, -0.9396926207859082059 ) ) ;
#31369=LINE ( 'NONE', #25055, #7110 ) ;
#31370=DIRECTION ( 'NONE',  ( 0.000000000000000000, 0.6427876096865373645, -0.7660444431189797898 ) ) ;
#31371=CARTESIAN_POINT ( 'NONE',  ( -10.74607608205217346, -10.54014554554150607, 33.71984207302941883 ) ) ;
#31372=ORIENTED_EDGE ( 'NONE', *, *, #47455, .T. ) ;
#31373=EDGE_CURVE ( 'NONE', #77667, #58446, #24125, .T. ) ;
#31375=CARTESIAN_POINT ( 'NONE',  ( 15.00784301325308157, -4.186968288167450147, 33.49512374952580274 ) ) ;
#31376=ORIENTED_EDGE ( 'NONE', *, *, #44057, .T. ) ;
#31377=CARTESIAN_POINT ( 'NONE',  ( 6.700150705560774966, -9.886141570436013382, 34.14413921362392301 ) ) ;
#31378=CARTESIAN_POINT ( 'NONE',  ( 17.07692307692295586, -11.06231777344772027, 33.60647404775119895 ) ) ;
#31379=CARTESIAN_POINT ( 'NONE',  ( -2.307692307692427391, -11.94971097300221174, 32.03036669348237098 ) ) ;
#31381=CARTESIAN_POINT ( 'NONE',  ( 7.596177115211490971, -8.303909089506435137, 34.68538101551103381 ) ) ;
#31382=FACE_BOUND ( 'NONE', #4427, .T. ) ;
#31383=CARTESIAN_POINT ( 'NONE',  ( 12.39545505058258001, -3.050289026998445951, 32.03036669348365706 ) ) ;
#31384=CARTESIAN_POINT ( 'NONE',  ( -10.68113804369794728, -7.249945578846652694, 34.99404164642496795 ) ) ;
#31385=EDGE_CURVE ( 'NONE', #4203, #7957, #17609, .T. ) ;
#31386=CARTESIAN_POINT ( 'NONE',  ( -2.307692307692305711, -13.20930481340135110, 34.54067556320372745 ) ) ;
#31387=FACE_OUTER_BOUND ( 'NONE', #3050, .T. ) ;
#31388=CARTESIAN_POINT ( 'NONE',  ( 0.5276057948885366500, -2.833524468853757750, 32.15551576947925838 ) ) ;
#31389=CARTESIAN_POINT ( 'NONE',  ( 1.515140822849028401, -3.068774925481847493, 32.56582465632704526 ) ) ;
#31390=CARTESIAN_POINT ( 'NONE',  ( 1.254055471002021971, -2.254533558242299396, 29.97296025877828285 ) ) ;
#31391=B_SPLINE_CURVE_WITH_KNOTS ( 'NONE', 3,
 ( #40117, #68453, #81542, #19829, #5876, #47291, #74784, #6750, #6326, #54944 ),
 .UNSPECIFIED., .F., .F.,
 ( 4, 2, 2, 2, 4 ),
 ( 0.0007817359430256334753, 0.0009771253907250058643, 0.001172514838424371098, 0.001367904286123736764, 0.001563293733823101998 ),
 .UNSPECIFIED. ) ;
#31393=ORIENTED_EDGE ( 'NONE', *, *, #4182, .F. ) ;
#31394=CARTESIAN_POINT ( 'NONE',  ( -15.23076923076922995, -12.78798330534102945, 29.74999999999997868 ) ) ;
#31395=B_SPLINE_CURVE_WITH_KNOTS ( 'NONE', 3,
 ( #596, #56859, #84354, #77583, #35263, #15891, #70834, #21300, #64056, #48772 ),
 .UNSPECIFIED., .F., .F.,
 ( 4, 2, 2, 2, 4 ),
 ( 0.0007817359527651090859, 0.0009771254036996478414, 0.001172514854634186489, 0.001367904305568725136, 0.001563293756503263783 ),
 .UNSPECIFIED. ) ;
#31396=CARTESIAN_POINT ( 'NONE',  ( 8.096208266067295156, -10.06805714834173315, 34.32951233291982618 ) ) ;
#31397=CARTESIAN_POINT ( 'NONE',  ( -0.7115152055870535008, -3.436278759898155233, 33.07459398097509506 ) ) ;
#31398=LINE ( 'NONE', #16112, #25128 ) ;
#31400=FACE_OUTER_BOUND ( 'NONE', #71607, .T. ) ;
#31402=CARTESIAN_POINT ( 'NONE',  ( -15.36145983387953606, -12.62707690430377383, 30.88035979386743435 ) ) ;
#31403=CARTESIAN_POINT ( 'NONE',  ( 3.230769230769231726, -2.538708090699994813, 30.37095296980875503 ) ) ;
#31404=CARTESIAN_POINT ( 'NONE',  ( 11.78846153846147793, -7.565270000091922853, 34.99999999999999289 ) ) ;
#31405=CARTESIAN_POINT ( 'NONE',  ( -16.15384615384627409, -10.21337939537710326, 33.94971097300076224 ) ) ;
#31406=CARTESIAN_POINT ( 'NONE',  ( 8.769230769230768274, -1.367168528481310208, 33.57946703557072254 ) ) ;
#31407=CYLINDRICAL_SURFACE ( 'NONE', #44011, 0.2499999999999998890 ) ;
#31408=EDGE_CURVE ( 'NONE', #61213, #16297, #13288, .T. ) ;
#31409=EDGE_CURVE ( 'NONE', #72566, #46285, #23578, .T. ) ;
#31410=CARTESIAN_POINT ( 'NONE',  ( -18.13069146666756382, -2.729777683071818117, 31.24903638046269450 ) ) ;
#31412=ORIENTED_EDGE ( 'NONE', *, *, #65264, .F. ) ;
#31414=CARTESIAN_POINT ( 'NONE',  ( 14.98074600654777377, -11.56360843649121861, 33.07473185843129926 ) ) ;
#31415=CARTESIAN_POINT ( 'NONE',  ( 7.146088274689773812, -4.887748414852792322, 34.01359900205216746 ) ) ;
#31417=B_SPLINE_CURVE_WITH_KNOTS ( 'NONE', 3,
 ( #83710, #70176, #15244, #36829, #44454, #76939, #2588, #42714, #8485, #29208 ),
 .UNSPECIFIED., .F., .F.,
 ( 4, 2, 2, 2, 4 ),
 ( 0.0007817246256747451124, 0.0009771112852218879000, 0.001172497944769030796, 0.001367884604316173692, 0.001563271263863316588 ),
 .UNSPECIFIED. ) ;
#31418=CARTESIAN_POINT ( 'NONE',  ( -10.83831157429146330, -10.01117774369187252, 34.36070679894347535 ) ) ;
#31420=CARTESIAN_POINT ( 'NONE',  ( 15.23076923076923173, -1.466349020453238561, 30.81389545987213907 ) ) ;
#31421=ORIENTED_EDGE ( 'NONE', *, *, #23884, .T. ) ;
#31422=CARTESIAN_POINT ( 'NONE',  ( 1.384615384615265343, -4.481592998941358097, 33.73612834414048933 ) ) ;
#31423=CARTESIAN_POINT ( 'NONE',  ( 6.923076923076924238, -11.33034616979429110, 35.88435417666054406 ) ) ;
#31424=CARTESIAN_POINT ( 'NONE',  ( 7.976944287120804056, -2.494656445102014342, 31.33466734024120015 ) ) ;
#31425=VERTEX_POINT ( 'NONE', #24910 ) ;
#31426=CARTESIAN_POINT ( 'NONE',  ( -12.59168643127015841, -9.504002272028875709, 34.60269587691767867 ) ) ;
#31427=DIRECTION ( 'NONE',  ( -0.000000000000000000, -0.9848077530122086864, -0.1736481776669273613 ) ) ;
#31428=LINE ( 'NONE', #25560, #69420 ) ;
#31430=CARTESIAN_POINT ( 'NONE',  ( 17.99999999999987566, -11.67786785259630911, 32.92929555188603530 ) ) ;
#31434=CARTESIAN_POINT ( 'NONE',  ( -12.46153846153846168, -2.486705287966279876, 31.30864560766543647 ) ) ;
#31435=AXIS2_PLACEMENT_3D ( 'NONE', #58790, #86293, #51563 ) ;
#31436=CARTESIAN_POINT ( 'NONE',  ( 9.692307692307695177, -13.78497067705608181, 32.30358669280327177 ) ) ;
#31437=VERTEX_POINT ( 'NONE', #25361 ) ;
#31440=CARTESIAN_POINT ( 'NONE',  ( -9.758391103263571509, -9.780366693483667717, 34.19971097300155805 ) ) ;
#31441=CARTESIAN_POINT ( 'NONE',  ( -5.076923076923075762, -3.669653830205710676, 35.88435417666054406 ) ) ;
#31442=CARTESIAN_POINT ( 'NONE',  ( 2.438218009455871638, -6.001044277235011215, 34.52024696741798948 ) ) ;
#31444=ORIENTED_EDGE ( 'NONE', *, *, #48604, .T. ) ;
#31445=ORIENTED_EDGE ( 'NONE', *, *, #11293, .T. ) ;
#31446=CARTESIAN_POINT ( 'NONE',  ( 4.153846153846030731, -5.941354392335915335, 34.76329471203413846 ) ) ;
#31448=CARTESIAN_POINT ( 'NONE',  ( -5.299850035829923200, -2.523278758544489797, 31.42238647778637528 ) ) ;
#31449=CARTESIAN_POINT ( 'NONE',  ( -3.361459833879538284, -4.684245665217971144, 34.18127051446801090 ) ) ;
#31450=CYLINDRICAL_SURFACE ( 'NONE', #62250, 0.2499999999999979738 ) ;
#31451=CARTESIAN_POINT ( 'NONE',  ( -1.253824943648434109, -12.62708834333097663, 30.88030960425257021 ) ) ;
#31452=ORIENTED_EDGE ( 'NONE', *, *, #20023, .F. ) ;
#31453=VERTEX_POINT ( 'NONE', #30775 ) ;
#31454=B_SPLINE_CURVE_WITH_KNOTS ( 'NONE', 3,
 ( #73609, #19534, #13227, #46994, #12777, #54635, #19971, #82134, #46121, #12337 ),
 .UNSPECIFIED., .F., .F.,
 ( 4, 2, 2, 2, 4 ),
 ( 0.000000000000000000, 0.0001954311564186865763, 0.0003908623128373731525, 0.0005862934692560596746, 0.0007817246256747463051 ),
 .UNSPECIFIED. ) ;
#31455=B_SPLINE_CURVE_WITH_KNOTS ( 'NONE', 3,
 ( #70367, #82998, #76226, #36149, #63152, #35243, #1020, #1467, #28955, #28495 ),
 .UNSPECIFIED., .F., .F.,
 ( 4, 2, 2, 2, 4 ),
 ( 0.000000000000000000, 0.0001954311564186862781, 0.0003908623128373725562, 0.0005862934692560588072, 0.0007817246256747451124 ),
 .UNSPECIFIED. ) ;
#31456=EDGE_LOOP ( 'NONE', ( #16604, #16780, #73417, #19540, #64000, #58724 ) ) ;
#31458=ORIENTED_EDGE ( 'NONE', *, *, #19074, .T. ) ;
#31459=EDGE_CURVE ( 'NONE', #33835, #22118, #76623, .T. ) ;
#31460=ADVANCED_FACE ( 'NONE', ( #85293 ), #51026, .F. ) ;
#31461=CARTESIAN_POINT ( 'NONE',  ( 3.165498784808455479, -11.94971097300153140, 32.03036669348370680 ) ) ;
#31462=CARTESIAN_POINT ( 'NONE',  ( 18.25005441991345378, -5.642605341092955307, 34.66089969410670335 ) ) ;
#31464=CARTESIAN_POINT ( 'NONE',  ( -8.834501215191545853, -10.90142922261923886, 33.41473453929638993 ) ) ;
#31465=CARTESIAN_POINT ( 'NONE',  ( -13.60748080681902294, -2.501496062324912284, 29.88072118266895671 ) ) ;
#31466=CARTESIAN_POINT ( 'NONE',  ( -5.869209559033046197, -3.338503747796866872, 32.95102852606553512 ) ) ;
#31467=FACE_BOUND ( 'NONE', #12057, .T. ) ;
#31468=CARTESIAN_POINT ( 'NONE',  ( 15.23076923076911093, -6.026961402154118019, 34.52809138561165270 ) ) ;
#31469=CARTESIAN_POINT ( 'NONE',  ( 9.442307692307693401, -7.433931650972300353, 34.75000000000000711 ) ) ;
#31470=EDGE_CURVE ( 'NONE', #22047, #83223, #70234, .T. ) ;
#31471=CARTESIAN_POINT ( 'NONE',  ( -7.976845312821408740, -12.11776431015576172, 31.66791131148498906 ) ) ;
#31472=CARTESIAN_POINT ( 'NONE',  ( 16.94623247381277054, -9.084618155246140248, 34.75535874321725771 ) ) ;
#31473=CARTESIAN_POINT ( 'NONE',  ( -8.703975629717930929, -12.16647553114626490, 32.15551576947920864 ) ) ;
#31474=CARTESIAN_POINT ( 'NONE',  ( -11.53846153846153655, -3.050289026998446396, 32.03036669348365706 ) ) ;
#31475=LINE ( 'NONE', #58940, #66322 ) ;
#31477=CARTESIAN_POINT ( 'NONE',  ( -5.933931648997559982, -11.69971097300155272, 32.46337939537588113 ) ) ;
#31478=EDGE_CURVE ( 'NONE', #34311, #53458, #26219, .T. ) ;
#31479=CARTESIAN_POINT ( 'NONE',  ( -7.596099534515531104, -2.564540009722895419, 30.55348353981670684 ) ) ;
#31480=ORIENTED_EDGE ( 'NONE', *, *, #51487, .F. ) ;
#31482=CIRCLE ( 'NONE', #54495, 2.000000000000001776 ) ;
#31483=CARTESIAN_POINT ( 'NONE',  ( 5.869852790561781219, -6.852621066184267029, 34.70813303252209181 ) ) ;
#31484=CARTESIAN_POINT ( 'NONE',  ( 14.98074600654777377, -2.985938066672154445, 32.43141759479405550 ) ) ;
#31485=CARTESIAN_POINT ( 'NONE',  ( 15.23076923076923173, -5.180354513474913603, 36.12317359536750416 ) ) ;
#31486=CYLINDRICAL_SURFACE ( 'NONE', #21396, 0.2500000000000008882 ) ;
#31487=CARTESIAN_POINT ( 'NONE',  ( -15.16460008980657292, -7.250054483168843156, 34.74374881642865631 ) ) ;
#31488=VERTEX_POINT ( 'NONE', #30340 ) ;
#31491=AXIS2_PLACEMENT_3D ( 'NONE', #51731, #85545, #3115 ) ;
#31493=DIRECTION ( 'NONE',  ( -0.000000000000000000, -0.7660444431189791237, -0.6427876096865379196 ) ) ;
#31494=CARTESIAN_POINT ( 'NONE',  ( 13.38461538461538680, -10.67929555188718282, 33.92786785259544047 ) ) ;
#31496=CARTESIAN_POINT ( 'NONE',  ( 10.86533013373275658, -4.336752205174649433, 33.62275283266504289 ) ) ;
#31497=CARTESIAN_POINT ( 'NONE',  ( -6.923076923076922462, -2.708943851104267164, 35.45975837776705220 ) ) ;
#31500=ORIENTED_EDGE ( 'NONE', *, *, #80431, .T. ) ;
#31501=CARTESIAN_POINT ( 'NONE',  ( -14.30769230769230660, -4.661471528628507777, 34.16647553114623292 ) ) ;
#31503=CARTESIAN_POINT ( 'NONE',  ( 10.61538461538449596, -2.625532179533778709, 30.86335684631627174 ) ) ;
#31504=CARTESIAN_POINT ( 'NONE',  ( 3.903822929624695792, -10.92453946501458439, 33.72985991061850086 ) ) ;
#31505=CARTESIAN_POINT ( 'NONE',  ( -18.00000000000000000, -12.27536236210233866, 35.44105525097462106 ) ) ;
#31507=LINE ( 'NONE', #86477, #28853 ) ;
#31508=CARTESIAN_POINT ( 'NONE',  ( -13.44988583057615905, -8.613356846314824011, 34.62446782046655613 ) ) ;
#31509=CARTESIAN_POINT ( 'NONE',  ( 16.82689983963011215, -12.22074536777955345, 31.39888409691088356 ) ) ;
#31510=CARTESIAN_POINT ( 'NONE',  ( 5.933917620639865831, -9.905515769479276145, 34.41647553114623292 ) ) ;
#31511=CARTESIAN_POINT ( 'NONE',  ( -9.442307692306272315, -7.500000000000154543, 35.00000000000007105 ) ) ;
#31513=B_SPLINE_CURVE_WITH_KNOTS ( 'NONE', 3,
 ( #51847, #23936, #78443, #37913, #37455, #65375, #4111, #79793, #3669, #51385 ),
 .UNSPECIFIED., .F., .F.,
 ( 4, 2, 2, 2, 4 ),
 ( 0.000000000000000000, 0.0001954311564186864407, 0.0003908623128373728815, 0.0005862934692560593493, 0.0007817246256747457630 ),
 .UNSPECIFIED. ) ;
#31514=CARTESIAN_POINT ( 'NONE',  ( -3.480769230769229061, -7.433931650972300353, 34.75000000000000711 ) ) ;
#31515=CARTESIAN_POINT ( 'NONE',  ( -3.165513659493203846, -11.94971097300157403, 32.03036669348361443 ) ) ;
#31516=ADVANCED_FACE ( 'NONE', ( #57808 ), #82426, .F. ) ;
#31517=CARTESIAN_POINT ( 'NONE',  ( -5.776987155906605942, -4.762714258010880997, 34.23016756924214832 ) ) ;
#31518=CARTESIAN_POINT ( 'NONE',  ( 9.562159722575998444, -5.070767119584671079, 34.40440758774516183 ) ) ;
#31519=CARTESIAN_POINT ( 'NONE',  ( -15.23076923076935074, -8.613356846316285953, 34.62446782046622218 ) ) ;
#31520=EDGE_CURVE ( 'NONE', #88008, #78911, #48695, .T. ) ;
#31521=ORIENTED_EDGE ( 'NONE', *, *, #73469, .F. ) ;
#31522=AXIS2_PLACEMENT_3D ( 'NONE', #31283, #2028, #85342 ) ;
#31523=CARTESIAN_POINT ( 'NONE',  ( -16.02305571287920571, -6.369690395747424461, 34.87708834333098196 ) ) ;
#31524=CARTESIAN_POINT ( 'NONE',  ( -5.010756470331436674, -7.250054591869668386, 34.99404684341514127 ) ) ;
#31528=CARTESIAN_POINT ( 'NONE',  ( 13.51540719244017374, -4.809403383903225304, 33.96459661697924304 ) ) ;
#31529=CARTESIAN_POINT ( 'NONE',  ( -0.4615384615384611200, -2.499999999999998668, 29.75000000000001421 ) ) ;
#31530=EDGE_CURVE ( 'NONE', #61423, #23488, #74003, .T. ) ;
#31532=VERTEX_POINT ( 'NONE', #55379 ) ;
#31534=DIRECTION ( 'NONE',  ( 0.000000000000000000, 0.8660254037844377084, 0.5000000000000015543 ) ) ;
#31536=CARTESIAN_POINT ( 'NONE',  ( 6.923076923076800782, -6.835583212225970762, 34.95778746994575670 ) ) ;
#31537=ORIENTED_EDGE ( 'NONE', *, *, #3545, .F. ) ;
#31538=CARTESIAN_POINT ( 'NONE',  ( -7.715628407920201326, -6.808710257144161559, 34.95449254468098843 ) ) ;
#31539=CARTESIAN_POINT ( 'NONE',  ( -9.469528151039279251, -2.847695495035523550, 31.58253572463339154 ) ) ;
#31540=CARTESIAN_POINT ( 'NONE',  ( 15.29602480204525428, -2.892918686051625166, 31.69288490824026638 ) ) ;
#31542=CARTESIAN_POINT ( 'NONE',  ( 0.2115617174898691555, -4.818429247618089661, 34.26397095200675125 ) ) ;
#31543=EDGE_LOOP ( 'NONE', ( #20318, #66573 ) ) ;
#31544=CARTESIAN_POINT ( 'NONE',  ( 0.4615384615384611755, -10.05456864172156806, 36.03766855953608683 ) ) ;
#31545=ORIENTED_EDGE ( 'NONE', *, *, #71436, .T. ) ;
#31547=VECTOR ( 'NONE', #36222, 1000.000000000000114 ) ;
#31548=CARTESIAN_POINT ( 'NONE',  ( -16.08859101433330707, -2.379036618887895305, 30.90682066428158592 ) ) ;
#31549=CARTESIAN_POINT ( 'NONE',  ( 0.5920641633020230499, -11.46989282347013095, 32.79007818306219946 ) ) ;
#31551=CARTESIAN_POINT ( 'NONE',  ( -6.000000000000121680, -10.33852847137269571, 34.16647553114546554 ) ) ;
#31552=CARTESIAN_POINT ( 'NONE',  ( 9.915320536401090123, -10.01129605718032600, 34.36064277460058491 ) ) ;
#31553=CARTESIAN_POINT ( 'NONE',  ( 0.3308478584281528412, -2.295517848115769421, 30.44137282052137294 ) ) ;
#31555=AXIS2_PLACEMENT_3D ( 'NONE', #28206, #75959, #74635 ) ;
#31556=DIRECTION ( 'NONE',  ( 0.000000000000000000, 1.000000000000000000, 0.000000000000000000 ) ) ;
#31558=EDGE_CURVE ( 'NONE', #6072, #52057, #34220, .T. ) ;
#31559=EDGE_LOOP ( 'NONE', ( #77657, #8417, #40598, #84533 ) ) ;
#31560=ORIENTED_EDGE ( 'NONE', *, *, #45090, .F. ) ;
#31562=FACE_OUTER_BOUND ( 'NONE', #80790, .T. ) ;
#31563=ORIENTED_EDGE ( 'NONE', *, *, #41216, .F. ) ;
#31564=CARTESIAN_POINT ( 'NONE',  ( -18.00000000000000000, -2.249999999999989786, 29.74999999999998579 ) ) ;
#31565=CARTESIAN_POINT ( 'NONE',  ( 9.627037691751372250, -5.941354392334499579, 34.76329471203369792 ) ) ;
#31567=EDGE_CURVE ( 'NONE', #46418, #81839, #55819, .T. ) ;
#31568=ORIENTED_EDGE ( 'NONE', *, *, #70782, .T. ) ;
#31569=LINE ( 'NONE', #84758, #45392 ) ;
#31570=ORIENTED_EDGE ( 'NONE', *, *, #52049, .T. ) ;
#31571=CARTESIAN_POINT ( 'NONE',  ( -12.46153846153846168, -3.669653830205710676, 35.88435417666054406 ) ) ;
#31572=CARTESIAN_POINT ( 'NONE',  ( -11.66860874789976243, -3.817052484675422797, 33.13202310037935661 ) ) ;
#31573=CARTESIAN_POINT ( 'NONE',  ( 0.3954550505825806250, -4.786620604624113540, 33.94971097300155805 ) ) ;
#31574=FACE_BOUND ( 'NONE', #20082, .T. ) ;
#31575=ORIENTED_EDGE ( 'NONE', *, *, #79717, .T. ) ;
#31577=LINE ( 'NONE', #60825, #44228 ) ;
#31579=CARTESIAN_POINT ( 'NONE',  ( 15.23076923076923173, -8.564572088678739092, 35.78748833219616898 ) ) ;
#31580=CARTESIAN_POINT ( 'NONE',  ( -14.30769230769242739, -9.442884908241554243, 34.35708131394783038 ) ) ;
#31581=CARTESIAN_POINT ( 'NONE',  ( -1.634592115557738534, -2.564618984488975961, 30.55390908950641915 ) ) ;
#31582=ORIENTED_EDGE ( 'NONE', *, *, #78782, .T. ) ;
#31584=EDGE_CURVE ( 'NONE', #84519, #80176, #65914, .T. ) ;
#31585=ORIENTED_EDGE ( 'NONE', *, *, #32423, .F. ) ;
#31586=VERTEX_POINT ( 'NONE', #56267 ) ;
#31587=CARTESIAN_POINT ( 'NONE',  ( -6.989159302437059296, -3.937682226553329556, 33.60647404775217240 ) ) ;
#31588=CARTESIAN_POINT ( 'NONE',  ( 5.777073782483851616, -3.105860786376062332, 32.13614157043599562 ) ) ;
#31589=B_SPLINE_CURVE_WITH_KNOTS ( 'NONE', 3,
 ( #85699, #85257, #42945, #16350, #64512, #58209, #15917, #83940, #78482, #37951 ),
 .UNSPECIFIED., .F., .F.,
 ( 4, 2, 2, 2, 4 ),
 ( 0.0007817359430256257775, 0.0009771253907249911191, 0.001172514838424356352, 0.001367904286123721586, 0.001563293733823086819 ),
 .UNSPECIFIED. ) ;
#31590=CARTESIAN_POINT ( 'NONE',  ( -11.53846153846153655, -1.629998284177014645, 34.34916445242399163 ) ) ;
#31591=CARTESIAN_POINT ( 'NONE',  ( -15.23076923076935074, -12.27809138561165270, 31.22303859784587132 ) ) ;
#31592=CARTESIAN_POINT ( 'NONE',  ( 1.450683735617825709, -9.780366693483669494, 34.19971097300155805 ) ) ;
#31593=CARTESIAN_POINT ( 'NONE',  ( 1.384615384615264011, -4.320704448113951379, 33.92786785259630022 ) ) ;
#31594=VERTEX_POINT ( 'NONE', #42324 ) ;
#31597=CARTESIAN_POINT ( 'NONE',  ( -1.449885830576159940, -3.835265460703609186, 33.15142922261924241 ) ) ;
#31598=EDGE_CURVE ( 'NONE', #26195, #11627, #36879, .T. ) ;
#31599=CARTESIAN_POINT ( 'NONE',  ( 10.74617642320940369, -11.71459661697925903, 32.44059661609676937 ) ) ;
#31600=ORIENTED_EDGE ( 'NONE', *, *, #44557, .F. ) ;
#31601=ORIENTED_EDGE ( 'NONE', *, *, #17879, .T. ) ;
#31602=B_SPLINE_CURVE_WITH_KNOTS ( 'NONE', 3,
 ( #21656, #71162, #29314, #43261, #62631, #42390, #22104, #44121, #76606, #9038 ),
 .UNSPECIFIED., .F., .F.,
 ( 4, 2, 2, 2, 4 ),
 ( 0.0007817246256747472808, 0.0009771112852218907189, 0.001172497944769034265, 0.001367884604316177595, 0.001563271263863321141 ),
 .UNSPECIFIED. ) ;
#31603=FACE_BOUND ( 'NONE', #60494, .T. ) ;
#31606=AXIS2_PLACEMENT_3D ( 'NONE', #20927, #81323, #41215 ) ;
#31607=ORIENTED_EDGE ( 'NONE', *, *, #15690, .T. ) ;
#31609=CARTESIAN_POINT ( 'NONE',  ( 7.846153846153846700, -2.721908614388771852, 31.22303859784724978 ) ) ;
#31610=CARTESIAN_POINT ( 'NONE',  ( -7.715628144390283438, -5.195472089885680766, 34.18748526763464923 ) ) ;
#31611=ORIENTED_EDGE ( 'NONE', *, *, #37792, .T. ) ;
#31612=EDGE_CURVE ( 'NONE', #60674, #65236, #49060, .T. ) ;
#31613=CARTESIAN_POINT ( 'NONE',  ( -7.715628144390280774, -4.459921816937788996, 33.71989282347011851 ) ) ;
#31614=CYLINDRICAL_SURFACE ( 'NONE', #6883, 0.2500000000000008882 ) ;
#31615=CARTESIAN_POINT ( 'NONE',  ( -17.07692307692307665, -13.20930481340135110, 34.54067556320372745 ) ) ;
#31616=CARTESIAN_POINT ( 'NONE',  ( -1.254089946381739429, -4.299079248970732792, 33.91157788607253565 ) ) ;
#31617=VECTOR ( 'NONE', #45967, 1000.000000000000000 ) ;
#31619=EDGE_LOOP ( 'NONE', ( #37763, #28512, #78390, #10379 ) ) ;
#31621=EDGE_LOOP ( 'NONE', ( #6613, #35863 ) ) ;
#31622=CARTESIAN_POINT ( 'NONE',  ( 14.30769230769231015, -10.89733346790207413, 36.13435417666054406 ) ) ;
#31624=CARTESIAN_POINT ( 'NONE',  ( 17.07692307692307665, -4.786620604624113540, 33.94971097300155094 ) ) ;
#31625=CARTESIAN_POINT ( 'NONE',  ( 18.06606835100243913, -8.120952969808772792, 34.71129190929999453 ) ) ;
#31626=CARTESIAN_POINT ( 'NONE',  ( -16.15384615384627409, -8.613356846316285953, 34.62446782046622218 ) ) ;
#31630=ORIENTED_EDGE ( 'NONE', *, *, #64324, .T. ) ;
#31631=LINE ( 'NONE', #80271, #1457 ) ;
#31632=CARTESIAN_POINT ( 'NONE',  ( 8.769230769231075584, -2.506253911140615021, 30.00000000000323297 ) ) ;
#31633=CARTESIAN_POINT ( 'NONE',  ( 2.307692307692309264, -13.75783147151868846, 33.36296068462461051 ) ) ;
#31634=EDGE_CURVE ( 'NONE', #63565, #63637, #71987, .T. ) ;
#31635=ORIENTED_EDGE ( 'NONE', *, *, #78394, .F. ) ;
#31637=ORIENTED_EDGE ( 'NONE', *, *, #715, .F. ) ;
#31638=CARTESIAN_POINT ( 'NONE',  ( -9.019253993452226226, -5.765609946408404518, 34.70566812827425451 ) ) ;
#31640=CARTESIAN_POINT ( 'NONE',  ( -0.3963444797551056165, -2.506253911140448487, 29.99999999999988987 ) ) ;
#31641=B_SPLINE_CURVE_WITH_KNOTS ( 'NONE', 3,
 ( #50349, #77830, #25111, #2606, #64748, #52573, #58433, #24665, #71960, #37732 ),
 .UNSPECIFIED., .F., .F.,
 ( 4, 2, 2, 2, 4 ),
 ( 0.0007817246256747484735, 0.0009771112852218931041, 0.001172497944769037735, 0.001367884604316182365, 0.001563271263863326996 ),
 .UNSPECIFIED. ) ;
#31642=CARTESIAN_POINT ( 'NONE',  ( 8.835298102580843249, -11.35647404775217595, 33.31231777344666511 ) ) ;
#31643=CARTESIAN_POINT ( 'NONE',  ( 18.00000000000000000, -11.91647553114624181, 32.58852847137148245 ) ) ;
#31644=CARTESIAN_POINT ( 'NONE',  ( -6.988347369037697376, -11.94971097300153140, 32.03036669348370680 ) ) ;
#31646=CARTESIAN_POINT ( 'NONE',  ( 5.750023269057646047, -3.627789207965226748, 32.91389620160131102 ) ) ;
#31647=CARTESIAN_POINT ( 'NONE',  ( -12.46153846153858247, -5.219633306517616589, 34.19971097300220464 ) ) ;
#31648=CARTESIAN_POINT ( 'NONE',  ( -17.07692307692319744, -9.528491918059723176, 34.59228464037033035 ) ) ;
#31649=EDGE_CURVE ( 'NONE', #48531, #77905, #72304, .T. ) ;
#31650=CARTESIAN_POINT ( 'NONE',  ( -3.454254174493178287, -11.89387501736622710, 32.13663884655806413 ) ) ;
#31652=VERTEX_POINT ( 'NONE', #2632 ) ;
#31653=CARTESIAN_POINT ( 'NONE',  ( -12.46153846153846168, -12.37446782046654192, 30.86335684631486131 ) ) ;
#31654=ORIENTED_EDGE ( 'NONE', *, *, #31997, .T. ) ;
#31655=CARTESIAN_POINT ( 'NONE',  ( -0.3954701105360229896, -2.721908614388772740, 31.22303859784725333 ) ) ;
#31656=CARTESIAN_POINT ( 'NONE',  ( -1.449885830576159940, -9.442884908240170461, 34.35708131394840592 ) ) ;
#31657=EDGE_CURVE ( 'NONE', #88418, #77943, #80949, .T. ) ;
#31658=CARTESIAN_POINT ( 'NONE',  ( 15.29602437028207085, -5.094484230520773593, 34.41647553114626845 ) ) ;
#31659=EDGE_LOOP ( 'NONE', ( #49625, #77428 ) ) ;
#31660=DIRECTION ( 'NONE',  ( -0.000000000000000000, -0.9848077530122085754, -0.1736481776669273613 ) ) ;
#31661=FACE_OUTER_BOUND ( 'NONE', #33898, .T. ) ;
#31663=CARTESIAN_POINT ( 'NONE',  ( -6.249976744048591826, -5.643011162660950042, 34.66104346484419096 ) ) ;
#31664=CARTESIAN_POINT ( 'NONE',  ( -9.692307692307691624, -13.87047571288749737, 32.06866353760679544 ) ) ;
#31665=EDGE_CURVE ( 'NONE', #27545, #64872, #3522, .T. ) ;
#31666=ORIENTED_EDGE ( 'NONE', *, *, #46138, .F. ) ;
#31667=VECTOR ( 'NONE', #35814, 1000.000000000000227 ) ;
#31668=DIRECTION ( 'NONE',  ( 0.000000000000000000, 0.4999999999999985567, 0.8660254037844395958 ) ) ;
#31669=VERTEX_POINT ( 'NONE', #17048 ) ;
#31670=CARTESIAN_POINT ( 'NONE',  ( 13.38461538461538680, -8.973038597847269315, 34.52809138561121927 ) ) ;
#31671=EDGE_CURVE ( 'NONE', #86754, #22873, #38011, .T. ) ;
#31672=CARTESIAN_POINT ( 'NONE',  ( -9.626239341305254271, -12.10708131394839882, 31.69288490824020954 ) ) ;
#31673=B_SPLINE_CURVE_WITH_KNOTS ( 'NONE', 3,
 ( #70765, #71632, #36100, #22570, #63552, #72086, #10393, #9938, #77515, #9069 ),
 .UNSPECIFIED., .F., .F.,
 ( 4, 2, 2, 2, 4 ),
 ( 0.000000000000000000, 0.0001954311564186862239, 0.0003908623128373724478, 0.0005862934692560586988, 0.0007817246256747448956 ),
 .UNSPECIFIED. ) ;
#31674=AXIS2_PLACEMENT_3D ( 'NONE', #27749, #6599, #83605 ) ;
#31675=AXIS2_PLACEMENT_3D ( 'NONE', #61147, #80562, #81447 ) ;
#31676=ADVANCED_FACE ( 'NONE', ( #23352 ), #70668, .F. ) ;
#31677=CARTESIAN_POINT ( 'NONE',  ( -13.38461538461538325, -2.721908614388771852, 31.22303859784724978 ) ) ;
#31678=FACE_OUTER_BOUND ( 'NONE', #69959, .T. ) ;
#31679=CARTESIAN_POINT ( 'NONE',  ( 14.30769230769231015, -1.117168528481311540, 33.14645433367849847 ) ) ;
#31681=AXIS2_PLACEMENT_3D ( 'NONE', #25548, #32310, #46706 ) ;
#31683=ORIENTED_EDGE ( 'NONE', *, *, #2831, .F. ) ;
#31684=EDGE_CURVE ( 'NONE', #61379, #22275, #4677, .T. ) ;
#31685=VERTEX_POINT ( 'NONE', #85510 ) ;
#31687=ORIENTED_EDGE ( 'NONE', *, *, #3573, .T. ) ;
#31688=ORIENTED_EDGE ( 'NONE', *, *, #35553, .T. ) ;
#31689=ORIENTED_EDGE ( 'NONE', *, *, #39434, .F. ) ;
#31690=CARTESIAN_POINT ( 'NONE',  ( 12.71148397988660328, -11.86320923018887719, 32.19269448109604070 ) ) ;
#31691=CARTESIAN_POINT ( 'NONE',  ( -3.296851610129365451, -6.343179335718451384, 34.87096338111212646 ) ) ;
#31692=CARTESIAN_POINT ( 'NONE',  ( -2.084265345830736305, -7.630147231320743018, 34.74852402298682819 ) ) ;
#31693=CARTESIAN_POINT ( 'NONE',  ( -7.146003140593072622, -3.105860786376062332, 32.13614157043599562 ) ) ;
#31694=CARTESIAN_POINT ( 'NONE',  ( -16.21911659980693443, -2.625532179533445198, 30.86335684631481513 ) ) ;
#31695=DIRECTION ( 'NONE',  ( 0.000000000000000000, 0.1736481776669267785, -0.9848077530122087975 ) ) ;
#31696=CYLINDRICAL_SURFACE ( 'NONE', #37836, 0.2500000000000012212 ) ;
#31697=CARTESIAN_POINT ( 'NONE',  ( -7.596208327805703320, -3.202959910592335202, 32.30730279482227019 ) ) ;
#31698=CARTESIAN_POINT ( 'NONE',  ( -4.403869391139119571, -10.05641848906368097, 34.04755513067966177 ) ) ;
#31700=EDGE_CURVE ( 'NONE', #29311, #33240, #58029, .T. ) ;
#31701=ORIENTED_EDGE ( 'NONE', *, *, #21944, .T. ) ;
#31704=ORIENTED_EDGE ( 'NONE', *, *, #73317, .F. ) ;
#31705=CARTESIAN_POINT ( 'NONE',  ( -12.46153846153846168, -1.215029322943914858, 32.30358669280327177 ) ) ;
#31706=DIRECTION ( 'NONE',  ( -0.000000000000000000, -0.9396926207859092051, -0.3420201433256662704 ) ) ;
#31707=CARTESIAN_POINT ( 'NONE',  ( -11.53846153846153655, -8.164416787775445883, 34.95778746994557906 ) ) ;
#31708=CARTESIAN_POINT ( 'NONE',  ( -14.55771554498526932, -10.05641848906368097, 34.04755513067966177 ) ) ;
#31709=FACE_BOUND ( 'NONE', #656, .T. ) ;
#31710=ORIENTED_EDGE ( 'NONE', *, *, #8228, .T. ) ;
#31711=B_SPLINE_CURVE_WITH_KNOTS ( 'NONE', 3,
 ( #28800, #49504, #83744, #9401, #78289, #43186, #2624, #9835, #16586, #2187 ),
 .UNSPECIFIED., .F., .F.,
 ( 4, 2, 2, 2, 4 ),
 ( 0.0007817359527651106038, 0.0009771254036996469741, 0.001172514854634183236, 0.001367904305568724702, 0.001563293756503266168 ),
 .UNSPECIFIED. ) ;
#31712=CIRCLE ( 'NONE', #67659, 0.2500000000000002220 ) ;
#31716=FACE_BOUND ( 'NONE', #76365, .T. ) ;
#31717=CARTESIAN_POINT ( 'NONE',  ( -9.626240358957616650, -2.292212530054420494, 30.41441678777542990 ) ) ;
#31718=CARTESIAN_POINT ( 'NONE',  ( -14.53061926659915315, -6.459968553980841577, 34.89616026154728701 ) ) ;
#31719=ORIENTED_EDGE ( 'NONE', *, *, #5740, .F. ) ;
#31721=CARTESIAN_POINT ( 'NONE',  ( 8.519230769230768274, -7.433932668274256805, 35.00000000000000711 ) ) ;
#31722=CARTESIAN_POINT ( 'NONE',  ( -18.06527000055631405, -4.320704448112774543, 33.92786785259540494 ) ) ;
#31723=ORIENTED_EDGE ( 'NONE', *, *, #78548, .F. ) ;
#31724=CARTESIAN_POINT ( 'NONE',  ( -11.53846153846166089, -5.094484230521993062, 34.41647553114689373 ) ) ;
#31725=CARTESIAN_POINT ( 'NONE',  ( -18.13014720943822056, -5.195881422630166391, 34.18770438780618548 ) ) ;
#31726=EDGE_LOOP ( 'NONE', ( #80405, #27458 ) ) ;
#31727=CYLINDRICAL_SURFACE ( 'NONE', #7158, 0.2499999999999979738 ) ;
#31728=CARTESIAN_POINT ( 'NONE',  ( -9.469294848214296678, -9.172514111537584114, 34.72667873470787470 ) ) ;
#31729=EDGE_LOOP ( 'NONE', ( #78067, #56599, #42702, #2865 ) ) ;
#31730=CYLINDRICAL_SURFACE ( 'NONE', #30083, 0.2499999999999993616 ) ;
#31731=CARTESIAN_POINT ( 'NONE',  ( -10.39237326377176451, -4.887748414852792322, 34.01359900205216746 ) ) ;
#31733=CARTESIAN_POINT ( 'NONE',  ( 8.096153846153908873, -7.434744429011177935, 34.75000000000002132 ) ) ;
#31735=DIRECTION ( 'NONE',  ( -0.000000000000000000, -0.5000000000000009992, -0.8660254037844380415 ) ) ;
#31736=CARTESIAN_POINT ( 'NONE',  ( -13.51530598772569469, -3.957541250942358424, 33.62499894934981626 ) ) ;
#31737=CARTESIAN_POINT ( 'NONE',  ( -15.36146069743678844, -12.38065189839062263, 30.83690757178629482 ) ) ;
#31738=EDGE_CURVE ( 'NONE', #52853, #71146, #35785, .T. ) ;
#31739=CIRCLE ( 'NONE', #33212, 0.2500000000000002220 ) ;
#31740=CARTESIAN_POINT ( 'NONE',  ( -15.93083480223330817, -11.76359900205217457, 32.36225158514719880 ) ) ;
#31741=CARTESIAN_POINT ( 'NONE',  ( -15.48074596171158213, -11.79746400365624659, 32.30657167506340954 ) ) ;
#31742=FACE_OUTER_BOUND ( 'NONE', #65908, .T. ) ;
#31745=CARTESIAN_POINT ( 'NONE',  ( -3.903791733932699515, -5.642605341092957083, 34.66089969410670335 ) ) ;
#31746=VERTEX_POINT ( 'NONE', #26479 ) ;
#31747=ADVANCED_FACE ( 'NONE', ( #11635 ), #39113, .F. ) ;
#31748=VECTOR ( 'NONE', #88341, 1000.000000000000227 ) ;
#31749=VERTEX_POINT ( 'NONE', #87308 ) ;
#31750=CARTESIAN_POINT ( 'NONE',  ( -3.165514091256391715, -9.528491918058460186, 34.59228464037085615 ) ) ;
#31751=EDGE_CURVE ( 'NONE', #60833, #26904, #23957, .T. ) ;
#31752=ORIENTED_EDGE ( 'NONE', *, *, #65204, .F. ) ;
#31753=CARTESIAN_POINT ( 'NONE',  ( 17.93467598719568556, -7.749976730030849303, 34.74374725381503737 ) ) ;
#31756=CARTESIAN_POINT ( 'NONE',  ( -8.835314180186649935, -3.050289026998445951, 32.03036669348365706 ) ) ;
#31757=FACE_OUTER_BOUND ( 'NONE', #19577, .T. ) ;
#31758=CARTESIAN_POINT ( 'NONE',  ( -6.130690603110307002, -2.494641256782728966, 31.33461815524612959 ) ) ;
#31759=VECTOR ( 'NONE', #57848, 1000.000000000000227 ) ;
#31760=CYLINDRICAL_SURFACE ( 'NONE', #21452, 0.2499999999999995559 ) ;
#31761=CARTESIAN_POINT ( 'NONE',  ( -9.692307692307814193, -5.941354392335915335, 34.76329471203413846 ) ) ;
#31763=ADVANCED_FACE ( 'NONE', ( #18832 ), #11181, .F. ) ;
#31764=AXIS2_PLACEMENT_3D ( 'NONE', #48242, #27091, #66747 ) ;
#31766=CARTESIAN_POINT ( 'NONE',  ( 1.634560902963529294, -3.202959910592336534, 32.30730279482227019 ) ) ;
#31769=CARTESIAN_POINT ( 'NONE',  ( 15.23076923076923173, -5.471508081941601098, 34.59228464037088457 ) ) ;
#31770=VERTEX_POINT ( 'NONE', #52602 ) ;
#31771=VERTEX_POINT ( 'NONE', #80084 ) ;
#31772=CARTESIAN_POINT ( 'NONE',  ( 14.08476534878546005, -8.282780595021769443, 34.94152052738834868 ) ) ;
#31773=CARTESIAN_POINT ( 'NONE',  ( -14.08491276642389423, -8.496831190052096971, 34.64984203495476578 ) ) ;
#31774=CARTESIAN_POINT ( 'NONE',  ( 16.40390057375961064, -12.41089969410671223, 31.60739465890703670 ) ) ;
#31776=CARTESIAN_POINT ( 'NONE',  ( 8.703960323269992472, -11.94971097300153140, 32.03036669348370680 ) ) ;
#31777=CARTESIAN_POINT ( 'NONE',  ( -5.076923076923199218, -3.083524468854526912, 32.58852847137268327 ) ) ;
#31779=CARTESIAN_POINT ( 'NONE',  ( 7.780071466793709867, -2.833524468853757305, 32.15551576947924417 ) ) ;
#31780=ORIENTED_EDGE ( 'NONE', *, *, #15508, .T. ) ;
#31782=B_SPLINE_CURVE_WITH_KNOTS ( 'NONE', 3,
 ( #67859, #59321, #6161, #53899, #59768, #32737, #19669, #38612, #11589, #46257 ),
 .UNSPECIFIED., .F., .F.,
 ( 4, 2, 2, 2, 4 ),
 ( 0.000000000000000000, 0.0001954311564186858715, 0.0003908623128373717431, 0.0005862934692560576146, 0.0007817246256747434861 ),
 .UNSPECIFIED. ) ;
#31783=EDGE_LOOP ( 'NONE', ( #67245, #12751 ) ) ;
#31784=CARTESIAN_POINT ( 'NONE',  ( -9.692307692307691624, -2.833524468853757305, 32.15551576947925838 ) ) ;
#31786=CARTESIAN_POINT ( 'NONE',  ( 9.692307692307695177, -3.513871655860378418, 32.76840700105978499 ) ) ;
#31787=CARTESIAN_POINT ( 'NONE',  ( -11.53846153846166089, -11.06231777344772027, 33.60647404775119895 ) ) ;
#31789=ORIENTED_EDGE ( 'NONE', *, *, #4479, .T. ) ;
#31790=ADVANCED_FACE ( 'NONE', ( #86869 ), #5317, .F. ) ;
#31791=ORIENTED_EDGE ( 'NONE', *, *, #48060, .T. ) ;
#31792=ORIENTED_EDGE ( 'NONE', *, *, #5472, .F. ) ;
#31793=EDGE_CURVE ( 'NONE', #15793, #73783, #62729, .T. ) ;
#31794=VECTOR ( 'NONE', #61297, 1000.000000000000227 ) ;
#31795=CARTESIAN_POINT ( 'NONE',  ( 12.46153846153876898, -2.506253911140615021, 30.00000000000323297 ) ) ;
#31796=CARTESIAN_POINT ( 'NONE',  ( 9.915320536401090123, -2.308499170217967134, 30.53291367094873721 ) ) ;
#31797=CARTESIAN_POINT ( 'NONE',  ( 4.153846153846030731, -3.643525952248796163, 33.31231777344771672 ) ) ;
#31799=VECTOR ( 'NONE', #18089, 999.9999999999998863 ) ;
#31800=CARTESIAN_POINT ( 'NONE',  ( 2.241608896736428935, -11.16473453929635440, 33.15142922261925662 ) ) ;
#31801=CARTESIAN_POINT ( 'NONE',  ( 11.53846153846141576, -11.06231777344772027, 33.60647404775119895 ) ) ;
#31802=DIRECTION ( 'NONE',  ( -0.000000000000000000, 0.1736481776669307198, -0.9848077530122080203 ) ) ;
#31803=ORIENTED_EDGE ( 'NONE', *, *, #82772, .T. ) ;
#31804=EDGE_CURVE ( 'NONE', #39107, #47910, #25586, .T. ) ;
#31805=VERTEX_POINT ( 'NONE', #32785 ) ;
#31808=B_SPLINE_CURVE_WITH_KNOTS ( 'NONE', 3,
 ( #85255, #62747, #76724, #42500, #59992, #87049, #71720, #37949, #87492, #51883 ),
 .UNSPECIFIED., .F., .F.,
 ( 4, 2, 2, 2, 4 ),
 ( 0.0007817246256747517261, 0.0009771112852218961399, 0.001172497944769040771, 0.001367884604316185401, 0.001563271263863329815 ),
 .UNSPECIFIED. ) ;
#31809=ORIENTED_EDGE ( 'NONE', *, *, #52696, .F. ) ;
#31810=CARTESIAN_POINT ( 'NONE',  ( 2.530703659305157949, -12.39991518177334129, 30.74647679643404530 ) ) ;
#31811=EDGE_LOOP ( 'NONE', ( #57367, #86686, #61142, #35729 ) ) ;
#31814=ADVANCED_FACE ( 'NONE', ( #80987 ), #58912, .F. ) ;
#31815=EDGE_CURVE ( 'NONE', #27245, #52424, #60696, .T. ) ;
#31817=EDGE_LOOP ( 'NONE', ( #55553, #35310 ) ) ;
#31821=CARTESIAN_POINT ( 'NONE',  ( -13.63459212866397507, -11.47974371597208076, 33.17467449705390692 ) ) ;
#31823=FACE_BOUND ( 'NONE', #63807, .T. ) ;
#31824=CARTESIAN_POINT ( 'NONE',  ( 10.39255792290561509, -7.369208160676172348, 34.74850200257122879 ) ) ;
#31825=CARTESIAN_POINT ( 'NONE',  ( 7.846153846153846700, -11.91647553114624181, 32.58852847137148245 ) ) ;
#31826=CARTESIAN_POINT ( 'NONE',  ( -1.384615384615506484, -3.643525952248795718, 33.31231777344771672 ) ) ;
#31827=CARTESIAN_POINT ( 'NONE',  ( 18.06606835100243558, -2.721908614388772296, 31.22303859784725333 ) ) ;
#31828=EDGE_LOOP ( 'NONE', ( #83763, #88914 ) ) ;
#31829=CARTESIAN_POINT ( 'NONE',  ( 6.673053685783957967, -8.432397168068783699, 34.66272746175022945 ) ) ;
#31831=ORIENTED_EDGE ( 'NONE', *, *, #73696, .F. ) ;
#31832=CARTESIAN_POINT ( 'NONE',  ( 6.673053685783957967, -10.05641848906368097, 34.04755513067966177 ) ) ;
#31833=VECTOR ( 'NONE', #10841, 1000.000000000000000 ) ;
#31834=DIRECTION ( 'NONE',  ( 0.000000000000000000, 0.3420201433256610524, 0.9396926207859113145 ) ) ;
#31835=CARTESIAN_POINT ( 'NONE',  ( -15.00775638667583500, -5.582272713120729257, 34.63742843783360570 ) ) ;
#31836=CARTESIAN_POINT ( 'NONE',  ( 11.47237812750566022, -5.557115091759785130, 34.35708131394839171 ) ) ;
#31837=FACE_OUTER_BOUND ( 'NONE', #37550, .T. ) ;
#31838=FACE_BOUND ( 'NONE', #29926, .T. ) ;
#31839=CARTESIAN_POINT ( 'NONE',  ( 13.31934493865461455, -12.27809138561121394, 31.22303859784730307 ) ) ;
#31840=DIRECTION ( 'NONE',  ( -0.000000000000000000, -0.1736481776669307198, -0.9848077530122080203 ) ) ;
#31841=CARTESIAN_POINT ( 'NONE',  ( -9.692307692307814193, -12.16647553114689728, 32.15551576947799362 ) ) ;
#31842=CARTESIAN_POINT ( 'NONE',  ( 1.161688425708537364, -12.64616026154729411, 30.79003144601913533 ) ) ;
#31843=CARTESIAN_POINT ( 'NONE',  ( 0.4615384615383382183, -3.083524468854526912, 32.58852847137268327 ) ) ;
#31845=CARTESIAN_POINT ( 'NONE',  ( -8.519285250882626670, -3.712312575010499049, 33.01462480002815170 ) ) ;
#31847=ADVANCED_FACE ( 'NONE', ( #55708 ), #67907, .F. ) ;
#31848=CARTESIAN_POINT ( 'NONE',  ( 16.15384615384603251, -5.094484230521993062, 34.41647553114689373 ) ) ;
#31849=ORIENTED_EDGE ( 'NONE', *, *, #53727, .F. ) ;
#31850=CARTESIAN_POINT ( 'NONE',  ( -6.923076923076922462, -13.53365097954675988, 30.81389545987213552 ) ) ;
#31851=CARTESIAN_POINT ( 'NONE',  ( 2.241609928332172430, -2.292212530054419606, 30.41441678777542634 ) ) ;
#31852=CARTESIAN_POINT ( 'NONE',  ( -1.384615384615383471, -2.721908614388771852, 31.22303859784724978 ) ) ;
#31853=CARTESIAN_POINT ( 'NONE',  ( 20.99999999999999645, -10.75000000000000000, 27.25000000000000000 ) ) ;
#31854=DIRECTION ( 'NONE',  ( 0.000000000000000000, 1.000000000000000000, 0.000000000000000000 ) ) ;
#31855=CARTESIAN_POINT ( 'NONE',  ( 6.222779668978067669, -3.563462043263029955, 33.22394488606062879 ) ) ;
#31857=CARTESIAN_POINT ( 'NONE',  ( -3.230769230769229949, -4.102666532097928531, 36.13435417666054406 ) ) ;
#31858=DIRECTION ( 'NONE',  ( -0.000000000000000000, 1.000000000000000000, -0.000000000000000000 ) ) ;
#31860=CARTESIAN_POINT ( 'NONE',  ( -9.692307692307812417, -11.48612834414049644, 32.76840700105863391 ) ) ;
#31861=DIRECTION ( 'NONE',  ( -0.000000000000000000, -0.8660254037844397068, -0.4999999999999978906 ) ) ;
#31864=CARTESIAN_POINT ( 'NONE',  ( -6.130690603110307890, -11.93127051446800024, 32.56575433478200665 ) ) ;
#31865=CYLINDRICAL_SURFACE ( 'NONE', #12572, 0.2499999999999994726 ) ;
#31866=EDGE_LOOP ( 'NONE', ( #36690, #39311, #56505, #47413 ) ) ;
#31867=EDGE_CURVE ( 'NONE', #85395, #1538, #77729, .T. ) ;
#31868=FACE_OUTER_BOUND ( 'NONE', #64237, .T. ) ;
#31869=CARTESIAN_POINT ( 'NONE',  ( 15.36129466900287532, -11.04252011169590020, 33.62494198852677130 ) ) ;
#31871=AXIS2_PLACEMENT_3D ( 'NONE', #84890, #23176, #50638 ) ;
#31872=CARTESIAN_POINT ( 'NONE',  ( 6.923076923076924238, -10.67929555188718282, 33.92786785259544047 ) ) ;
#31873=DIRECTION ( 'NONE',  ( -0.000000000000000000, 0.9396926207859093161, -0.3420201433256663259 ) ) ;
#31874=VERTEX_POINT ( 'NONE', #7086 ) ;
#31875=CARTESIAN_POINT ( 'NONE',  ( -6.700064078983529292, -10.01129605718032778, 34.36064277460058491 ) ) ;
#31876=CARTESIAN_POINT ( 'NONE',  ( -17.01166793741023042, -9.528491918058456633, 34.59228464037085615 ) ) ;
#31877=CARTESIAN_POINT ( 'NONE',  ( 11.76183702423395872, -2.251407671071270489, 29.88021292934942963 ) ) ;
#31878=ORIENTED_EDGE ( 'NONE', *, *, #77379, .T. ) ;
#31880=CARTESIAN_POINT ( 'NONE',  ( -2.980823712421087901, -3.712312575010499938, 33.01462480002815170 ) ) ;
#31881=DIRECTION ( 'NONE',  ( -0.000000000000000000, 0.1736481776669307198, -0.9848077530122080203 ) ) ;
#31882=CARTESIAN_POINT ( 'NONE',  ( 11.66898724022510514, -9.417988943895561960, 34.36773134775777550 ) ) ;
#31883=ADVANCED_FACE ( 'NONE', ( #34561 ), #62456, .F. ) ;
#31884=EDGE_LOOP ( 'NONE', ( #30196, #76756 ) ) ;
#31885=CYLINDRICAL_SURFACE ( 'NONE', #27466, 0.2499999999999995559 ) ;
#31886=CARTESIAN_POINT ( 'NONE',  ( 10.74591005361826213, -4.299079248970732792, 33.91157788607253565 ) ) ;
#31887=CARTESIAN_POINT ( 'NONE',  ( 13.38461538461538680, -13.87047571288749737, 32.06866353760679544 ) ) ;
#31888=ORIENTED_EDGE ( 'NONE', *, *, #50155, .F. ) ;
#31889=ORIENTED_EDGE ( 'NONE', *, *, #21944, .F. ) ;
#31890=B_SPLINE_CURVE_WITH_KNOTS ( 'NONE', 3,
 ( #29775, #56790, #8175, #22566, #58117, #35647, #70311, #1852, #71187, #78386 ),
 .UNSPECIFIED., .F., .F.,
 ( 4, 2, 2, 2, 4 ),
 ( 0.0007817246256747507503, 0.0009771112852218957062, 0.001172497944769040771, 0.001367884604316185835, 0.001563271263863330682 ),
 .UNSPECIFIED. ) ;
#31892=CARTESIAN_POINT ( 'NONE',  ( 5.207714884747862705, -12.11778462344220841, 31.66786338562085135 ) ) ;
#31893=CARTESIAN_POINT ( 'NONE',  ( 9.822833130541340552, -4.299079248970732792, 33.91157788607253565 ) ) ;
#31894=EDGE_CURVE ( 'NONE', #65345, #66107, #336, .T. ) ;
#31895=CARTESIAN_POINT ( 'NONE',  ( -12.68446467905460473, -3.586966769969701208, 32.86292498521069660 ) ) ;
#31896=DIRECTION ( 'NONE',  ( 0.000000000000000000, 0.9396926207859126468, 0.3420201433256571111 ) ) ;
#31898=ORIENTED_EDGE ( 'NONE', *, *, #12756, .F. ) ;
#31899=EDGE_CURVE ( 'NONE', #27135, #55920, #23674, .T. ) ;
#31900=VERTEX_POINT ( 'NONE', #54381 ) ;
#31901=EDGE_CURVE ( 'NONE', #84958, #58400, #32581, .T. ) ;
#31902=CARTESIAN_POINT ( 'NONE',  ( 4.284636594813102661, -5.496552790871117367, 34.60292014791297532 ) ) ;
#31905=CARTESIAN_POINT ( 'NONE',  ( 15.10007776410167324, -3.062553014421049546, 32.05460306192773601 ) ) ;
#31906=B_SPLINE_CURVE_WITH_KNOTS ( 'NONE', 3,
 ( #80460, #46221, #19630, #73708, #25060, #31829, #59283, #86791, #74136, #12004 ),
 .UNSPECIFIED., .F., .F.,
 ( 4, 2, 2, 2, 4 ),
 ( 0.000000000000000000, 0.0001954339857564079894, 0.0003908679715128159787, 0.0005863019572692239681, 0.0007817359430256319575 ),
 .UNSPECIFIED. ) ;
#31907=CARTESIAN_POINT ( 'NONE',  ( 2.530471848960718972, -3.755027918224367767, 33.06320215134714857 ) ) ;
#31908=CYLINDRICAL_SURFACE ( 'NONE', #62573, 0.2499999999999979738 ) ;
#31911=ORIENTED_EDGE ( 'NONE', *, *, #35341, .F. ) ;
#31912=EDGE_LOOP ( 'NONE', ( #89116, #72585 ) ) ;
#31914=ORIENTED_EDGE ( 'NONE', *, *, #50857, .F. ) ;
#31915=CARTESIAN_POINT ( 'NONE',  ( -10.68063454715869831, -2.255955759149247619, 30.00000000000013856 ) ) ;
#31916=EDGE_CURVE ( 'NONE', #17458, #73573, #64783, .T. ) ;
#31917=EDGE_CURVE ( 'NONE', #25611, #33924, #47582, .T. ) ;
#31920=CYLINDRICAL_SURFACE ( 'NONE', #54679, 0.2499999999999998890 ) ;
#31921=DIRECTION ( 'NONE',  ( -0.000000000000000000, 0.1736481776669307198, -0.9848077530122080203 ) ) ;
#31922=CARTESIAN_POINT ( 'NONE',  ( 4.153846153846032507, -2.892918686052165622, 31.69288490824153470 ) ) ;
#31923=FACE_BOUND ( 'NONE', #31912, .T. ) ;
#31924=CARTESIAN_POINT ( 'NONE',  ( -0.5922299282060179415, -4.118384482072085184, 33.43331474514187107 ) ) ;
#31925=CARTESIAN_POINT ( 'NONE',  ( -6.130147969731697621, -12.50552854090298993, 31.33409797877408920 ) ) ;
#31926=FACE_OUTER_BOUND ( 'NONE', #43738, .T. ) ;
#31927=CARTESIAN_POINT ( 'NONE',  ( 6.923076923076924238, -12.29105614889573062, 35.45975837776705220 ) ) ;
#31928=CARTESIAN_POINT ( 'NONE',  ( 6.857806922520603088, -11.06231777344662781, 33.60647404775220082 ) ) ;
#31929=AXIS2_PLACEMENT_3D ( 'NONE', #60023, #68126, #61341 ) ;
#31930=CARTESIAN_POINT ( 'NONE',  ( -4.087679547254512435, -7.250054591869667497, 34.99404684341514127 ) ) ;
#31931=CARTESIAN_POINT ( 'NONE',  ( 5.142178648199100977, -2.625532179533470512, 30.86335684631491105 ) ) ;
#31932=ORIENTED_EDGE ( 'NONE', *, *, #26244, .T. ) ;
#31933=CARTESIAN_POINT ( 'NONE',  ( -15.10024379253558635, -11.66157788607254098, 32.95092075102925833 ) ) ;
#31934=CARTESIAN_POINT ( 'NONE',  ( 12.59206389977210705, -3.625058011473228703, 33.29252011169590020 ) ) ;
#31935=EDGE_LOOP ( 'NONE', ( #42466, #13600 ) ) ;
#31936=EDGE_LOOP ( 'NONE', ( #2720, #27179 ) ) ;
#31937=CARTESIAN_POINT ( 'NONE',  ( 6.000000000000001776, -6.386643153685126251, 34.62446782046654192 ) ) ;
#31938=DIRECTION ( 'NONE',  ( 0.000000000000000000, 0.1736481776669267785, -0.9848077530122087975 ) ) ;
#31939=CARTESIAN_POINT ( 'NONE',  ( 16.15384615384603251, -4.481592998941358097, 33.73612834414048933 ) ) ;
#31940=CARTESIAN_POINT ( 'NONE',  ( 1.161130440891438464, -6.760086850603068243, 34.69517049084099369 ) ) ;
#31941=CARTESIAN_POINT ( 'NONE',  ( 12.46153846153833911, -11.06231777344772027, 33.60647404775119895 ) ) ;
#31942=ORIENTED_EDGE ( 'NONE', *, *, #58628, .T. ) ;
#31943=CARTESIAN_POINT ( 'NONE',  ( 8.545745844666436497, -12.69144148231606017, 30.53333754910549303 ) ) ;
#31944=CARTESIAN_POINT ( 'NONE',  ( 17.99999999999987566, -4.320704448113951379, 33.92786785259630022 ) ) ;
#31945=CARTESIAN_POINT ( 'NONE',  ( 11.60371667797437212, -3.083524468853784839, 32.58852847137153930 ) ) ;
#31946=DIRECTION ( 'NONE',  ( 0.000000000000000000, 0.7660444431189822323, -0.6427876096865344779 ) ) ;
#31947=CARTESIAN_POINT ( 'NONE',  ( -1.607542343522233796, -10.01117774369187252, 34.36070679894347535 ) ) ;
#31949=SHAPE_REPRESENTATION_RELATIONSHIP ( 'NONE' , 'NONE' ,  #36256, #63293 ) ;
#31950=CARTESIAN_POINT ( 'NONE',  ( -17.07692307692319744, -2.657715359629662988, 31.77849191805970364 ) ) ;
#31952=ORIENTED_EDGE ( 'NONE', *, *, #53620, .T. ) ;
#31953=EDGE_LOOP ( 'NONE', ( #50336, #72759, #82053, #62366 ) ) ;
#31954=CARTESIAN_POINT ( 'NONE',  ( 24.00000000000000000, -5.499999999999981348, 27.25000000000000000 ) ) ;
#31955=CARTESIAN_POINT ( 'NONE',  ( 12.68450136509994763, -7.369474270740069777, 34.74850911626239736 ) ) ;
#31956=CARTESIAN_POINT ( 'NONE',  ( 10.74617642320940369, -2.541949514083464479, 30.39797389878540557 ) ) ;
#31957=CARTESIAN_POINT ( 'NONE',  ( 14.30769230769218758, -2.892918686052165622, 31.69288490824153470 ) ) ;
#31958=CARTESIAN_POINT ( 'NONE',  ( 2.438530725705071678, -7.277220443632450575, 34.74524770363009196 ) ) ;
#31960=LINE ( 'NONE', #38266, #41 ) ;
#31961=CARTESIAN_POINT ( 'NONE',  ( 1.515141086378949842, -5.195472089885680766, 34.18748526763464923 ) ) ;
#31962=CARTESIAN_POINT ( 'NONE',  ( -8.834500769787091201, -12.70778746994557551, 30.41441678777548319 ) ) ;
#31963=CARTESIAN_POINT ( 'NONE',  ( 3.230769230769231726, -1.129524287112498415, 32.06866353760679544 ) ) ;
#31965=CARTESIAN_POINT ( 'NONE',  ( 14.98074600654777377, -12.45566812827425451, 31.48439005359158926 ) ) ;
#31966=VECTOR ( 'NONE', #57638, 1000.000000000000000 ) ;
#31968=DIRECTION ( 'NONE',  ( -0.000000000000000000, -0.6427876096865404731, -0.7660444431189770143 ) ) ;
#31969=CARTESIAN_POINT ( 'NONE',  ( -0.4615384615385826339, -11.48612834414049644, 32.76840700105863391 ) ) ;
#31970=CARTESIAN_POINT ( 'NONE',  ( -2.980823712421087901, -11.37275283266503756, 32.91324779482534524 ) ) ;
#31971=CARTESIAN_POINT ( 'NONE',  ( -3.360917200500928459, -12.50552854090298993, 31.33409797877408920 ) ) ;
#31973=ORIENTED_EDGE ( 'NONE', *, *, #21066, .T. ) ;
#31975=CARTESIAN_POINT ( 'NONE',  ( -12.71153846153846168, -7.566083408709835645, 34.74999999999999289 ) ) ;
#31976=CARTESIAN_POINT ( 'NONE',  ( 13.13459216039393240, -6.652501968072648708, 34.93155406624980941 ) ) ;
#31978=CARTESIAN_POINT ( 'NONE',  ( 13.38461538461538680, -4.786620604624113540, 33.94971097300155094 ) ) ;
#31979=DIRECTION ( 'NONE',  ( 0.000000000000000000, 0.3420201433256641055, -0.9396926207859100932 ) ) ;
#31980=CARTESIAN_POINT ( 'NONE',  ( 10.74622294587137361, -7.277220318596961057, 34.99547417642776992 ) ) ;
#31981=ORIENTED_EDGE ( 'NONE', *, *, #20508, .T. ) ;
#31983=CARTESIAN_POINT ( 'NONE',  ( -1.634592115557737424, -9.943427161483782584, 34.11278801902876978 ) ) ;
#31984=VERTEX_POINT ( 'NONE', #76877 ) ;
#31985=B_SPLINE_CURVE_WITH_KNOTS ( 'NONE', 3,
 ( #58911, #66110, #11633, #81429, #4416, #80083, #19716, #5315, #87755, #46742 ),
 .UNSPECIFIED., .F., .F.,
 ( 4, 2, 2, 2, 4 ),
 ( 0.0007817246256747473893, 0.0009771112852218905021, 0.001172497944769033615, 0.001367884604316176944, 0.001563271263863320057 ),
 .UNSPECIFIED. ) ;
#31987=EDGE_LOOP ( 'NONE', ( #19810, #44115 ) ) ;
#31989=LINE ( 'NONE', #46387, #50463 ) ;
#31990=CARTESIAN_POINT ( 'NONE',  ( -15.36145983387954139, -2.845849958028613624, 32.17971566917920967 ) ) ;
#31991=DIRECTION ( 'NONE',  ( -0.000000000000000000, 0.8660254037844399289, -0.4999999999999980016 ) ) ;
#31992=EDGE_LOOP ( 'NONE', ( #1215, #8440, #23449, #59023 ) ) ;
#31993=CARTESIAN_POINT ( 'NONE',  ( -10.55012904410859065, -12.46129190930001052, 30.37095296980870174 ) ) ;
#31996=VECTOR ( 'NONE', #5806, 1000.000000000000227 ) ;
#31997=EDGE_CURVE ( 'NONE', #44682, #30667, #65112, .T. ) ;
#32000=CARTESIAN_POINT ( 'NONE',  ( -0.6844646790546096149, -3.105860786376062332, 32.13614157043599562 ) ) ;
#32001=CARTESIAN_POINT ( 'NONE',  ( 2.438218009455874302, -3.285477652293413264, 32.44071101563363158 ) ) ;
#32002=DIRECTION ( 'NONE',  ( -0.000000000000000000, -0.000000000000000000, -1.000000000000000000 ) ) ;
#32003=LINE ( 'NONE', #4066, #78086 ) ;
#32004=CARTESIAN_POINT ( 'NONE',  ( 11.28843830116857383, -11.86270091957321249, 32.19358267280087915 ) ) ;
#32005=LINE ( 'NONE', #59472, #86657 ) ;
#32006=ORIENTED_EDGE ( 'NONE', *, *, #30547, .T. ) ;
#32007=ORIENTED_EDGE ( 'NONE', *, *, #46738, .T. ) ;
#32009=ORIENTED_EDGE ( 'NONE', *, *, #7040, .F. ) ;
#32010=DIRECTION ( 'NONE',  ( -0.000000000000000000, 1.000000000000000000, 3.491481338843133355E-15 ) ) ;
#32011=ORIENTED_EDGE ( 'NONE', *, *, #61443, .F. ) ;
#32012=CYLINDRICAL_SURFACE ( 'NONE', #360, 0.2499999999999997502 ) ;
#32013=DIRECTION ( 'NONE',  ( -0.000000000000000000, -0.1736481776669307198, -0.9848077530122080203 ) ) ;
#32014=EDGE_LOOP ( 'NONE', ( #19864, #87114, #59261, #38641, #82578, #60285 ) ) ;
#32015=CARTESIAN_POINT ( 'NONE',  ( -14.30769230769242739, -4.481592998941358097, 33.73612834414048933 ) ) ;
#32016=ORIENTED_EDGE ( 'NONE', *, *, #28793, .T. ) ;
#32017=CARTESIAN_POINT ( 'NONE',  ( 16.85343813319912698, -10.11188796281391511, 34.01382737946119050 ) ) ;
#32019=VECTOR ( 'NONE', #44441, 1000.000000000000000 ) ;
#32020=CARTESIAN_POINT ( 'NONE',  ( 9.758376043310132530, -8.120952969808772792, 34.71129190929999453 ) ) ;
#32021=EDGE_CURVE ( 'NONE', #66205, #57379, #84123, .T. ) ;
#32022=CARTESIAN_POINT ( 'NONE',  ( 4.153846153846154188, -12.62096338111211580, 30.90682066428153263 ) ) ;
#32023=CARTESIAN_POINT ( 'NONE',  ( -11.40793610022789828, -12.15418822224088835, 32.17964115625579069 ) ) ;
#32024=FACE_BOUND ( 'NONE', #50968, .T. ) ;
#32025=ADVANCED_FACE ( 'NONE', ( #2970 ), #70559, .F. ) ;
#32026=CARTESIAN_POINT ( 'NONE',  ( 2.531119269553878670, -7.630147231320743018, 34.74852402298682819 ) ) ;
#32027=CARTESIAN_POINT ( 'NONE',  ( 12.46153846153846168, -5.557115091759785130, 34.35708131394839171 ) ) ;
#32028=CYLINDRICAL_SURFACE ( 'NONE', #20854, 0.2500000000000004996 ) ;
#32030=CARTESIAN_POINT ( 'NONE',  ( 4.826899852701619587, -3.520140089381497361, 33.17453946501458262 ) ) ;
#32031=CARTESIAN_POINT ( 'NONE',  ( -14.43838377435986686, -8.999036380462717588, 34.52022231692819076 ) ) ;
#32032=DIRECTION ( 'NONE',  ( -0.000000000000000000, 0.1736481776669307198, -0.9848077530122080203 ) ) ;
#32034=CYLINDRICAL_SURFACE ( 'NONE', #10069, 0.2500000000000008882 ) ;
#32035=ORIENTED_EDGE ( 'NONE', *, *, #23175, .T. ) ;
#32037=CARTESIAN_POINT ( 'NONE',  ( 10.86543892702293057, -12.41262288849542017, 30.68299917996395010 ) ) ;
#32038=CARTESIAN_POINT ( 'NONE',  ( -9.692307692307691624, -8.164416787775445883, 34.95778746994557906 ) ) ;
#32039=CARTESIAN_POINT ( 'NONE',  ( 3.007842271862381178, -3.395401636524185474, 33.02366814457250399 ) ) ;
#32040=CARTESIAN_POINT ( 'NONE',  ( -13.38461538461538325, -2.833524468853757305, 32.15551576947925838 ) ) ;
#32042=CARTESIAN_POINT ( 'NONE',  ( 1.384615384615386802, -3.937682226553329556, 33.60647404775216529 ) ) ;
#32043=ORIENTED_EDGE ( 'NONE', *, *, #56622, .F. ) ;
#32044=DIRECTION ( 'NONE',  ( -0.000000000000000000, -0.5000000000000009992, -0.8660254037844380415 ) ) ;
#32045=B_SPLINE_CURVE_WITH_KNOTS ( 'NONE', 3,
 ( #24570, #32662, #3406, #30878, #79529, #4305, #17828, #60130, #58346, #66898 ),
 .UNSPECIFIED., .F., .F.,
 ( 4, 2, 2, 2, 4 ),
 ( 0.0007817246336856290608, 0.0009771112958940099402, 0.001172497958102391036, 0.001367884620310772133, 0.001563271282519153229 ),
 .UNSPECIFIED. ) ;
#32046=CARTESIAN_POINT ( 'NONE',  ( -0.2115930521604181824, -3.520799739797214389, 33.17531984108286025 ) ) ;
#32047=CARTESIAN_POINT ( 'NONE',  ( 2.438482748659258625, -12.62708834333097663, 30.88030960425257021 ) ) ;
#32048=CARTESIAN_POINT ( 'NONE',  ( 5.011599064118766655, -7.749976730030849303, 34.74374725381503737 ) ) ;
#32050=EDGE_LOOP ( 'NONE', ( #75001, #73586, #62641, #83350 ) ) ;
#32051=AXIS2_PLACEMENT_3D ( 'NONE', #77599, #70404, #14566 ) ;
#32053=ORIENTED_EDGE ( 'NONE', *, *, #14252, .T. ) ;
#32054=VECTOR ( 'NONE', #78298, 1000.000000000000000 ) ;
#32055=CARTESIAN_POINT ( 'NONE',  ( 17.77717330752099301, -7.369208160676171460, 34.74850200257122879 ) ) ;
#32056=CARTESIAN_POINT ( 'NONE',  ( -7.596208327805704208, -5.057305518903949526, 34.11320923018887896 ) ) ;
#32057=VERTEX_POINT ( 'NONE', #36335 ) ;
#32058=CARTESIAN_POINT ( 'NONE',  ( -3.480745961711584346, -12.41269422305637171, 30.68257228309993323 ) ) ;
#32059=DIRECTION ( 'NONE',  ( -0.000000000000000000, 0.5000000000000011102, -0.8660254037844380415 ) ) ;
#32060=CARTESIAN_POINT ( 'NONE',  ( -8.096130577096198877, -11.79746400365624659, 32.30657167506340954 ) ) ;
#32061=CARTESIAN_POINT ( 'NONE',  ( 8.992010438208831502, -3.563462043263030399, 33.22394488606062879 ) ) ;
#32062=DIRECTION ( 'NONE',  ( -0.000000000000000000, 0.9396926207859093161, -0.3420201433256663259 ) ) ;
#32064=CARTESIAN_POINT ( 'NONE',  ( -0.4615384615385840772, -12.16647553114689728, 32.15551576947799362 ) ) ;
#32065=EDGE_LOOP ( 'NONE', ( #66477, #37278, #42463, #88528 ) ) ;
#32066=CARTESIAN_POINT ( 'NONE',  ( -7.846153846153844924, -8.973038597847269315, 34.52809138561121927 ) ) ;
#32067=CARTESIAN_POINT ( 'NONE',  ( -2.530618525208453651, -9.086856451489515152, 34.49173150075333183 ) ) ;
#32068=CARTESIAN_POINT ( 'NONE',  ( -9.692307692307691624, -1.367168528481310208, 33.57946703557072254 ) ) ;
#32070=CARTESIAN_POINT ( 'NONE',  ( -10.61538461538461320, -3.322132147404559976, 32.92929555188717927 ) ) ;
#32071=DIRECTION ( 'NONE',  ( -0.000000000000000000, 0.8660254037844399289, -0.4999999999999980016 ) ) ;
#32072=CARTESIAN_POINT ( 'NONE',  ( -6.923076923076922462, -8.564572088678739092, 35.78748833219616898 ) ) ;
#32074=EDGE_LOOP ( 'NONE', ( #52864, #47819 ) ) ;
#32075=CARTESIAN_POINT ( 'NONE',  ( 17.29970274590113632, -3.020022701398814569, 32.48759521482552515 ) ) ;
#32076=DIRECTION ( 'NONE',  ( -0.000000000000000000, 0.8660254037844399289, -0.4999999999999980016 ) ) ;
#32078=B_SPLINE_CURVE_WITH_KNOTS ( 'NONE', 3,
 ( #40034, #59838, #31933, #52180, #53968, #67494, #46327, #59394, #67939, #47208 ),
 .UNSPECIFIED., .F., .F.,
 ( 4, 2, 2, 2, 4 ),
 ( 0.0007817246256747463051, 0.0009771112852218896347, 0.001172497944769032747, 0.001367884604316176077, 0.001563271263863319407 ),
 .UNSPECIFIED. ) ;
#32079=ORIENTED_EDGE ( 'NONE', *, *, #51343, .F. ) ;
#32080=ORIENTED_EDGE ( 'NONE', *, *, #6581, .F. ) ;
#32081=DIRECTION ( 'NONE',  ( -0.000000000000000000, 0.1736481776669307198, -0.9848077530122080203 ) ) ;
#32082=CARTESIAN_POINT ( 'NONE',  ( 12.46153846153846168, -3.937682226553329556, 33.60647404775216529 ) ) ;
#32084=EDGE_CURVE ( 'NONE', #35421, #21173, #10090, .T. ) ;
#32085=CARTESIAN_POINT ( 'NONE',  ( 10.54930120442873331, -4.098570777380720287, 33.41473453929634729 ) ) ;
#32086=VECTOR ( 'NONE', #68308, 1000.000000000000000 ) ;
#32087=B_SPLINE_CURVE_WITH_KNOTS ( 'NONE', 3,
 ( #55519, #23069, #1472, #36588, #14990, #77127, #586, #83004, #35250, #62710 ),
 .UNSPECIFIED., .F., .F.,
 ( 4, 2, 2, 2, 4 ),
 ( 0.0007817246256747472808, 0.0009771112852218907189, 0.001172497944769034265, 0.001367884604316177595, 0.001563271263863321141 ),
 .UNSPECIFIED. ) ;
#32088=CARTESIAN_POINT ( 'NONE',  ( 6.000000000000001776, -13.87047571288749737, 32.06866353760679544 ) ) ;
#32089=CARTESIAN_POINT ( 'NONE',  ( 5.999999999999880096, -8.613356846316285953, 34.62446782046622218 ) ) ;
#32090=B_SPLINE_CURVE_WITH_KNOTS ( 'NONE', 3,
 ( #60220, #87278, #79167, #74189, #10711, #67433, #12056, #31424, #53010, #46273 ),
 .UNSPECIFIED., .F., .F.,
 ( 4, 2, 2, 2, 4 ),
 ( 0.0007817246256747448956, 0.0009771112852218879000, 0.001172497944769030796, 0.001367884604316173692, 0.001563271263863316805 ),
 .UNSPECIFIED. ) ;
#32091=ORIENTED_EDGE ( 'NONE', *, *, #1628, .F. ) ;
#32092=CARTESIAN_POINT ( 'NONE',  ( -3.099978789802280144, -12.62708834333097663, 30.88030960425257021 ) ) ;
#32093=CARTESIAN_POINT ( 'NONE',  ( -2.307692307692305711, -9.780366693483667717, 34.19971097300155094 ) ) ;
#32094=CARTESIAN_POINT ( 'NONE',  ( 16.94677586748485965, -9.418419913701741919, 34.36755862841477693 ) ) ;
#32096=CARTESIAN_POINT ( 'NONE',  ( 10.39245765647776309, -9.172386477786396597, 34.72672124145550043 ) ) ;
#32098=ORIENTED_EDGE ( 'NONE', *, *, #85385, .T. ) ;
#32099=CYLINDRICAL_SURFACE ( 'NONE', #64397, 0.2499999999999986955 ) ;
#32100=CARTESIAN_POINT ( 'NONE',  ( -1.384615384615505151, -9.442884908241554243, 34.35708131394783038 ) ) ;
#32101=CARTESIAN_POINT ( 'NONE',  ( 7.846153846153846700, -13.88283147151868846, 33.14645433367849847 ) ) ;
#32102=ORIENTED_EDGE ( 'NONE', *, *, #79450, .F. ) ;
#32103=EDGE_CURVE ( 'NONE', #25666, #43394, #57033, .T. ) ;
#32104=CARTESIAN_POINT ( 'NONE',  ( -13.16160254052199008, -4.762714258010881885, 34.23016756924214832 ) ) ;
#32105=CARTESIAN_POINT ( 'NONE',  ( -11.28851602011339672, -12.43552623307873972, 30.55307653245132826 ) ) ;
#32106=CARTESIAN_POINT ( 'NONE',  ( -39.05038313613820122, -2.499999999999999556, 29.75000000000000355 ) ) ;
#32107=CARTESIAN_POINT ( 'NONE',  ( -7.596099426240391139, -4.818054556918156983, 34.26375889529406749 ) ) ;
#32108=CARTESIAN_POINT ( 'NONE',  ( 3.296024370282069516, -3.083524468853784839, 32.58852847137153930 ) ) ;
#32109=ORIENTED_EDGE ( 'NONE', *, *, #13401, .F. ) ;
#32110=ADVANCED_FACE ( 'NONE', ( #50263 ), #57924, .F. ) ;
#32111=CARTESIAN_POINT ( 'NONE',  ( 14.30769230769231015, -13.78497067705608181, 32.30358669280327177 ) ) ;
#32115=CYLINDRICAL_SURFACE ( 'NONE', #45034, 0.2499999999999986955 ) ;
#32116=EDGE_CURVE ( 'NONE', #51881, #29248, #36767, .T. ) ;
#32117=CYLINDRICAL_SURFACE ( 'NONE', #42780, 0.2500000000000004996 ) ;
#32118=LINE ( 'NONE', #10517, #83309 ) ;
#32119=ADVANCED_FACE ( 'NONE', ( #30451 ), #78641, .F. ) ;
#32121=CARTESIAN_POINT ( 'NONE',  ( 5.011672086761834066, -2.506253911140460477, 30.00000000000013856 ) ) ;
#32122=CARTESIAN_POINT ( 'NONE',  ( 15.93091919493929964, -11.98009711892700224, 32.48740034544074007 ) ) ;
#32124=EDGE_LOOP ( 'NONE', ( #53007, #62656, #86097, #53244 ) ) ;
#32125=EDGE_LOOP ( 'NONE', ( #34610, #52250, #36962, #83648 ) ) ;
#32126=ORIENTED_EDGE ( 'NONE', *, *, #5852, .T. ) ;
#32127=B_SPLINE_CURVE_WITH_KNOTS ( 'NONE', 3,
 ( #61734, #21201, #55874, #48669, #41930, #69398, #14905, #21647, #7704, #35162 ),
 .UNSPECIFIED., .F., .F.,
 ( 4, 2, 2, 2, 4 ),
 ( 0.000000000000000000, 0.0001954339857564091007, 0.0003908679715128182013, 0.0005863019572692273291, 0.0007817359430256364027 ),
 .UNSPECIFIED. ) ;
#32128=EDGE_LOOP ( 'NONE', ( #47973, #33638 ) ) ;
#32131=DIRECTION ( 'NONE',  ( 1.000000000000000000, 0.000000000000000000, 0.000000000000000000 ) ) ;
#32132=CARTESIAN_POINT ( 'NONE',  ( -3.360917200500926239, -6.809168938359898782, 34.95455904226513866 ) ) ;
#32133=EDGE_CURVE ( 'NONE', #44386, #58630, #52494, .T. ) ;
#32134=CARTESIAN_POINT ( 'NONE',  ( 15.00784301325308157, -4.887634598454295265, 34.01352882383564946 ) ) ;
#32135=CARTESIAN_POINT ( 'NONE',  ( -12.46153846153846168, -13.88283147151868846, 33.14645433367849847 ) ) ;
#32136=CARTESIAN_POINT ( 'NONE',  ( 3.230769230769231726, -1.242168528481310874, 33.36296068462461051 ) ) ;
#32137=CARTESIAN_POINT ( 'NONE',  ( 4.153846153846032507, -12.27809138561165270, 31.22303859784587132 ) ) ;
#32138=EDGE_CURVE ( 'NONE', #6007, #15407, #45324, .T. ) ;
#32140=EDGE_CURVE ( 'NONE', #14112, #52651, #87644, .T. ) ;
#32141=CARTESIAN_POINT ( 'NONE',  ( -5.326923076923097966, -2.249999999999999112, 29.81609741502488120 ) ) ;
#32142=LINE ( 'NONE', #5108, #67748 ) ;
#32143=ORIENTED_EDGE ( 'NONE', *, *, #84375, .F. ) ;
#32144=ORIENTED_EDGE ( 'NONE', *, *, #61203, .F. ) ;
#32145=ORIENTED_EDGE ( 'NONE', *, *, #84510, .F. ) ;
#32146=CARTESIAN_POINT ( 'NONE',  ( 0.2386115026316130983, -11.98009711892699691, 32.48740034544075428 ) ) ;
#32147=ORIENTED_EDGE ( 'NONE', *, *, #21835, .T. ) ;
#32148=AXIS2_PLACEMENT_3D ( 'NONE', #84124, #37685, #3452 ) ;
#32149=CARTESIAN_POINT ( 'NONE',  ( 12.46153846153833911, -3.643525952248795718, 33.31231777344771672 ) ) ;
#32150=LINE ( 'NONE', #4224, #82234 ) ;
#32151=AXIS2_PLACEMENT_3D ( 'NONE', #33113, #74547, #45735 ) ;
#32152=CARTESIAN_POINT ( 'NONE',  ( 5.076923076923075762, -1.129524287112498415, 32.06866353760679544 ) ) ;
#32153=CARTESIAN_POINT ( 'NONE',  ( -14.43783951713053249, -10.19110544564092002, 33.96427741523702792 ) ) ;
#32154=FACE_BOUND ( 'NONE', #36175, .T. ) ;
#32155=VERTEX_POINT ( 'NONE', #65561 ) ;
#32156=ORIENTED_EDGE ( 'NONE', *, *, #82230, .F. ) ;
#32157=CARTESIAN_POINT ( 'NONE',  ( 11.53846153846153832, -5.180354513474913603, 36.12317359536750416 ) ) ;
#32158=ORIENTED_EDGE ( 'NONE', *, *, #65335, .F. ) ;
#32159=FACE_BOUND ( 'NONE', #68435, .T. ) ;
#32160=CARTESIAN_POINT ( 'NONE',  ( -4.826923076921656452, -7.500000000000154543, 35.00000000000007105 ) ) ;
#32161=DIRECTION ( 'NONE',  ( -1.000000000000000000, 0.000000000000000000, 0.000000000000000000 ) ) ;
#32162=ORIENTED_EDGE ( 'NONE', *, *, #20140, .T. ) ;
#32163=CARTESIAN_POINT ( 'NONE',  ( 17.93472955403922242, -2.892918686051582533, 31.69288490824015980 ) ) ;
#32164=CARTESIAN_POINT ( 'NONE',  ( -1.384615384615506484, -8.656820664282941280, 34.87096338111179961 ) ) ;
#32165=CARTESIAN_POINT ( 'NONE',  ( -5.207532732127157615, -7.722926974430166069, 34.99546784045485737 ) ) ;
#32166=ORIENTED_EDGE ( 'NONE', *, *, #62979, .F. ) ;
#32167=CARTESIAN_POINT ( 'NONE',  ( -3.230769230769229949, -12.29105614889573062, 35.45975837776705220 ) ) ;
#32168=CARTESIAN_POINT ( 'NONE',  ( -16.15384615384615330, -1.242168528481310874, 33.36296068462461051 ) ) ;
#32171=DIRECTION ( 'NONE',  ( -0.000000000000000000, -0.9396926207859093161, -0.3420201433256663259 ) ) ;
#32172=CARTESIAN_POINT ( 'NONE',  ( 7.173022441425065843, -10.76462480002816235, 33.53768742498949962 ) ) ;
#32173=ORIENTED_EDGE ( 'NONE', *, *, #40039, .F. ) ;
#32174=CARTESIAN_POINT ( 'NONE',  ( -17.29985003582992320, -12.64616026154729411, 30.79003144601914244 ) ) ;
#32175=CARTESIAN_POINT ( 'NONE',  ( -10.55012904410859065, -5.219633306516380244, 34.19971097300157936 ) ) ;
#32176=CARTESIAN_POINT ( 'NONE',  ( 15.93036122928182330, -3.019605429927187501, 32.48692288466676814 ) ) ;
#32177=CARTESIAN_POINT ( 'NONE',  ( -8.638438961405979555, -8.999086150933475636, 34.52020707165672775 ) ) ;
#32178=CARTESIAN_POINT ( 'NONE',  ( 0.4615384615384611755, -2.499999999999998668, 29.50000000000001066 ) ) ;
#32179=ADVANCED_FACE ( 'NONE', ( #51585 ), #38551, .F. ) ;
#32180=CARTESIAN_POINT ( 'NONE',  ( 6.923076923076802558, -9.442884908241554243, 34.35708131394783038 ) ) ;
#32181=CARTESIAN_POINT ( 'NONE',  ( -1.449885830576159051, -5.219633306516282545, 34.19971097300152962 ) ) ;
#32183=CARTESIAN_POINT ( 'NONE',  ( -15.90379184220784836, -11.79725096376909299, 32.30694842903960762 ) ) ;
#32184=FACE_OUTER_BOUND ( 'NONE', #82331, .T. ) ;
#32187=ORIENTED_EDGE ( 'NONE', *, *, #70394, .F. ) ;
#32188=EDGE_CURVE ( 'NONE', #66117, #26375, #19169, .T. ) ;
#32189=B_SPLINE_CURVE_WITH_KNOTS ( 'NONE', 3,
 ( #60900, #5074, #79851, #81189, #32105, #68114, #19473, #59569, #25793, #25345 ),
 .UNSPECIFIED., .F., .F.,
 ( 4, 2, 2, 2, 4 ),
 ( 0.0007817359430256326080, 0.0009771253907249993591, 0.001172514838424366327, 0.001367904286123733078, 0.001563293733823099829 ),
 .UNSPECIFIED. ) ;
#32190=VECTOR ( 'NONE', #17973, 1000.000000000000114 ) ;
#32191=DIRECTION ( 'NONE',  ( 0.000000000000000000, 0.000000000000000000, 1.000000000000000000 ) ) ;
#32192=ORIENTED_EDGE ( 'NONE', *, *, #35179, .F. ) ;
#32195=ORIENTED_EDGE ( 'NONE', *, *, #14646, .T. ) ;
#32196=CARTESIAN_POINT ( 'NONE',  ( -2.084680956079457470, -12.39991518177334129, 30.74647679643404530 ) ) ;
#32197=ORIENTED_EDGE ( 'NONE', *, *, #67821, .F. ) ;
#32198=CARTESIAN_POINT ( 'NONE',  ( 17.86938964037546995, -7.722926236386454590, 34.74524107206102030 ) ) ;
#32200=CARTESIAN_POINT ( 'NONE',  ( 12.71153846153988098, -7.500000000000154543, 35.00000000000007105 ) ) ;
#32201=B_SPLINE_CURVE_WITH_KNOTS ( 'NONE', 3,
 ( #64646, #84067, #78175, #29123, #36317, #16037, #43507, #77288, #78615, #10166 ),
 .UNSPECIFIED., .F., .F.,
 ( 4, 2, 2, 2, 4 ),
 ( 0.0007817246256747465219, 0.0009771112852218900684, 0.001172497944769033615, 0.001367884604316177378, 0.001563271263863320925 ),
 .UNSPECIFIED. ) ;
#32202=CARTESIAN_POINT ( 'NONE',  ( -15.29603923132554932, -12.51329471203370325, 31.30864560766548976 ) ) ;
#32203=CARTESIAN_POINT ( 'NONE',  ( -3.230769230769351186, -9.442884908241554243, 34.35708131394783038 ) ) ;
#32204=CARTESIAN_POINT ( 'NONE',  ( -14.43784027742400866, -11.04286588640298561, 33.62463336215343901 ) ) ;
#32205=EDGE_CURVE ( 'NONE', #4047, #6648, #70073, .T. ) ;
#32206=DIRECTION ( 'NONE',  ( -0.000000000000000000, 1.000000000000000000, 3.491481338843133355E-15 ) ) ;
#32207=CARTESIAN_POINT ( 'NONE',  ( -10.83886955910856464, -4.386631170607603991, 33.66268669641500111 ) ) ;
#32208=CARTESIAN_POINT ( 'NONE',  ( 0.7114838709165030028, -2.589246495874657938, 31.60778113518102828 ) ) ;
#32210=CARTESIAN_POINT ( 'NONE',  ( 17.14299041027315695, -2.292212530054420050, 30.41441678777542990 ) ) ;
#32211=CARTESIAN_POINT ( 'NONE',  ( -10.48533955946484220, -2.254550872974305342, 29.97347326024527092 ) ) ;
#32212=CARTESIAN_POINT ( 'NONE',  ( 9.692307692307695177, -10.51840700105979565, 33.73612834413961536 ) ) ;
#32214=ORIENTED_EDGE ( 'NONE', *, *, #59548, .T. ) ;
#32215=CARTESIAN_POINT ( 'NONE',  ( -9.019207500173124004, -12.41269422305637171, 30.68257228309993323 ) ) ;
#32216=CARTESIAN_POINT ( 'NONE',  ( -17.20761454359063691, -8.147922237126337563, 34.70805685702651999 ) ) ;
#32217=CARTESIAN_POINT ( 'NONE',  ( -2.373774687052442545, -2.292212530054419606, 30.41441678777542634 ) ) ;
#32218=CARTESIAN_POINT ( 'NONE',  ( 8.769230769231082689, -2.255955759149395501, 30.00000000000324363 ) ) ;
#32219=EDGE_CURVE ( 'NONE', #41186, #82649, #85850, .T. ) ;
#32221=CARTESIAN_POINT ( 'NONE',  ( -9.942284436356285227, -6.524016743844655686, 34.90889640711025521 ) ) ;
#32222=AXIS2_PLACEMENT_3D ( 'NONE', #65022, #3331, #51052 ) ;
#32223=EDGE_LOOP ( 'NONE', ( #43625, #40876 ) ) ;
#32224=CARTESIAN_POINT ( 'NONE',  ( -15.23076923076922995, -4.786620604624113540, 33.94971097300155094 ) ) ;
#32226=EDGE_LOOP ( 'NONE', ( #32656, #55357, #81209, #83403 ) ) ;
#32227=CARTESIAN_POINT ( 'NONE',  ( -5.750054481651856619, -5.852078868378311149, 34.47109172314383585 ) ) ;
#32229=CARTESIAN_POINT ( 'NONE',  ( -4.153846153846274980, -12.70778746994576025, 30.41441678777401236 ) ) ;
#32230=CARTESIAN_POINT ( 'NONE',  ( 6.066067333350077639, -8.164416787775445883, 34.95778746994558617 ) ) ;
#32231=CARTESIAN_POINT ( 'NONE',  ( 13.31934538405906565, -8.656820664281498878, 34.87096338111211935 ) ) ;
#32232=ORIENTED_EDGE ( 'NONE', *, *, #51303, .F. ) ;
#32235=CIRCLE ( 'NONE', #33714, 0.2500000000000002220 ) ;
#32236=ADVANCED_FACE ( 'NONE', ( #11077 ), #86760, .F. ) ;
#32237=EDGE_CURVE ( 'NONE', #66936, #33331, #20607, .T. ) ;
#32238=CARTESIAN_POINT ( 'NONE',  ( 13.16113046005105680, -4.988325925672468131, 34.36044203135681130 ) ) ;
#32239=CARTESIAN_POINT ( 'NONE',  ( -0.2115930521604179604, -10.18230066228895758, 34.26354781536631577 ) ) ;
#32240=CARTESIAN_POINT ( 'NONE',  ( 8.900021210197719412, -5.496552790871120031, 34.60292014791297532 ) ) ;
#32242=EDGE_CURVE ( 'NONE', #88972, #56388, #62353, .T. ) ;
#32243=VECTOR ( 'NONE', #77630, 1000.000000000000000 ) ;
#32244=CYLINDRICAL_SURFACE ( 'NONE', #34158, 0.2499999999999994726 ) ;
#32245=CARTESIAN_POINT ( 'NONE',  ( -14.98082382139119062, -9.357781135181031829, 34.66075350412533851 ) ) ;
#32246=EDGE_CURVE ( 'NONE', #32412, #5555, #80773, .T. ) ;
#32247=CARTESIAN_POINT ( 'NONE',  ( -15.90379184220783593, -2.779044189368096607, 31.39831045268885035 ) ) ;
#32248=ORIENTED_EDGE ( 'NONE', *, *, #12267, .F. ) ;
#32249=ORIENTED_EDGE ( 'NONE', *, *, #69763, .T. ) ;
#32250=CARTESIAN_POINT ( 'NONE',  ( 11.66850670129631595, -2.504778602574659896, 29.97347330155780654 ) ) ;
#32251=CARTESIAN_POINT ( 'NONE',  ( -1.384615384615383471, -12.78798330534102767, 29.49999999999997868 ) ) ;
#32254=B_SPLINE_CURVE_WITH_KNOTS ( 'NONE', 3,
 ( #38790, #79329, #32031, #50511, #77991, #17634, #16295, #30254, #4097, #31580 ),
 .UNSPECIFIED., .F., .F.,
 ( 4, 2, 2, 2, 4 ),
 ( 0.000000000000000000, 0.0001954339857564073659, 0.0003908679715128147319, 0.0005863019572692221250, 0.0007817359430256294638 ),
 .UNSPECIFIED. ) ;
#32255=DIRECTION ( 'NONE',  ( 1.000000000000000000, 0.000000000000000000, 0.000000000000000000 ) ) ;
#32258=ORIENTED_EDGE ( 'NONE', *, *, #67609, .F. ) ;
#32260=CARTESIAN_POINT ( 'NONE',  ( -14.55766905174089665, -12.41104346484419452, 31.60698883733904196 ) ) ;
#32261=ORIENTED_EDGE ( 'NONE', *, *, #32138, .F. ) ;
#32262=CARTESIAN_POINT ( 'NONE',  ( 5.999999999999878320, -9.528491918059723176, 34.59228464037033035 ) ) ;
#32263=CARTESIAN_POINT ( 'NONE',  ( -8.096153846153844924, -2.249999999999998668, 29.75000000000000355 ) ) ;
#32264=FACE_BOUND ( 'NONE', #63670, .T. ) ;
#32265=CARTESIAN_POINT ( 'NONE',  ( -6.673131404728780858, -12.43552623307873972, 30.55307653245132826 ) ) ;
#32267=CARTESIAN_POINT ( 'NONE',  ( -14.24249832590895082, -2.506253911140448487, 29.99999999999988631 ) ) ;
#32269=EDGE_CURVE ( 'NONE', #7422, #76471, #42109, .T. ) ;
#32270=CARTESIAN_POINT ( 'NONE',  ( 11.31497661389721010, -11.60425143139329940, 33.02411095842164457 ) ) ;
#32271=CYLINDRICAL_SURFACE ( 'NONE', #63888, 0.2499999999999986955 ) ;
#32274=CARTESIAN_POINT ( 'NONE',  ( -6.223484943723948781, -10.81261337010820256, 33.49550067578627477 ) ) ;
#32275=CARTESIAN_POINT ( 'NONE',  ( -13.16160254052198830, -11.43677907613344757, 33.22367315496202167 ) ) ;
#32276=CARTESIAN_POINT ( 'NONE',  ( -0.7115384615384605649, -7.566083408709834757, 34.74999999999999289 ) ) ;
#32277=EDGE_CURVE ( 'NONE', #16715, #80414, #74383, .T. ) ;
#32278=FACE_BOUND ( 'NONE', #4655, .T. ) ;
#32281=CARTESIAN_POINT ( 'NONE',  ( -10.61538461538461320, -4.786620604624113540, 33.94971097300155094 ) ) ;
#32282=CARTESIAN_POINT ( 'NONE',  ( 3.230769230769231726, -4.098570777380720287, 33.41473453929634729 ) ) ;
#32285=DIRECTION ( 'NONE',  ( 0.000000000000000000, 0.9396926207859126468, 0.3420201433256571111 ) ) ;
#32288=CARTESIAN_POINT ( 'NONE',  ( -6.923076923076922462, -8.973038597847269315, 34.52809138561121927 ) ) ;
#32289=EDGE_LOOP ( 'NONE', ( #12739, #60863 ) ) ;
#32290=CARTESIAN_POINT ( 'NONE',  ( -5.999999999999998224, -3.937682226553329556, 33.60647404775216529 ) ) ;
#32291=CARTESIAN_POINT ( 'NONE',  ( -6.923076923077045919, -12.70778746994576025, 30.41441678777401236 ) ) ;
#32292=CARTESIAN_POINT ( 'NONE',  ( -1.161604033002534564, -10.61302985866383963, 33.66295027996417843 ) ) ;
#32294=CARTESIAN_POINT ( 'NONE',  ( -17.01085574357300345, -2.292212530054420494, 30.41441678777542990 ) ) ;
#32295=CARTESIAN_POINT ( 'NONE',  ( -12.71151520558705528, -6.524016743844655686, 34.90889640711025521 ) ) ;
#32297=CYLINDRICAL_SURFACE ( 'NONE', #50365, 0.2500000000000008882 ) ;
#32299=EDGE_CURVE ( 'NONE', #88887, #51951, #30343, .T. ) ;
#32301=CARTESIAN_POINT ( 'NONE',  ( 9.562159722575998444, -4.299443229763728169, 33.91186481527756058 ) ) ;
#32302=CARTESIAN_POINT ( 'NONE',  ( 8.769230769230647482, -10.21337939537710326, 33.94971097300076224 ) ) ;
#32303=FACE_OUTER_BOUND ( 'NONE', #50823, .T. ) ;
#32304=AXIS2_PLACEMENT_3D ( 'NONE', #3103, #2653, #16187 ) ;
#32305=CARTESIAN_POINT ( 'NONE',  ( 14.30769230769231015, -1.466349020453238561, 30.81389545987213907 ) ) ;
#32307=CARTESIAN_POINT ( 'NONE',  ( 16.15384615384603251, -2.657715359629662544, 31.77849191805970364 ) ) ;
#32309=DIRECTION ( 'NONE',  ( 0.000000000000000000, 0.3420201433256610524, 0.9396926207859113145 ) ) ;
#32310=DIRECTION ( 'NONE',  ( -0.000000000000000000, -0.8660254037844399289, -0.4999999999999980016 ) ) ;
#32312=VECTOR ( 'NONE', #62882, 1000.000000000000000 ) ;
#32313=VECTOR ( 'NONE', #35278, 1000.000000000000000 ) ;
#32315=CARTESIAN_POINT ( 'NONE',  ( -8.835313148590904220, -3.322132147404559532, 32.92929555188719348 ) ) ;
#32316=EDGE_LOOP ( 'NONE', ( #14534, #28520, #39162, #64895 ) ) ;
#32318=CARTESIAN_POINT ( 'NONE',  ( -12.21148404162501144, -12.65882529074907126, 30.72640787790839312 ) ) ;
#32319=CARTESIAN_POINT ( 'NONE',  ( 4.946232473812767871, -12.35290016733513951, 31.75349464988449455 ) ) ;
#32320=ORIENTED_EDGE ( 'NONE', *, *, #45740, .T. ) ;
#32321=CARTESIAN_POINT ( 'NONE',  ( -13.38461538461550759, -10.33852847137269571, 34.16647553114546554 ) ) ;
#32322=CARTESIAN_POINT ( 'NONE',  ( -2.438301962896387565, -7.722926974430166069, 34.99546784045485737 ) ) ;
#32323=EDGE_CURVE ( 'NONE', #2266, #19388, #8826, .T. ) ;
#32324=CARTESIAN_POINT ( 'NONE',  ( -8.546219417617921366, -2.554770724473667265, 30.48948780036025852 ) ) ;
#32325=CARTESIAN_POINT ( 'NONE',  ( -12.46153846153846168, -4.661471528628507777, 34.16647553114623292 ) ) ;
#32326=EDGE_CURVE ( 'NONE', #72856, #62783, #83985, .T. ) ;
#32328=CARTESIAN_POINT ( 'NONE',  ( -14.30769230769230660, -9.584722331328613620, 36.20867863119891439 ) ) ;
#32329=CARTESIAN_POINT ( 'NONE',  ( -5.076923076923075762, -12.78798330534103123, 29.99999999999997868 ) ) ;
#32332=ORIENTED_EDGE ( 'NONE', *, *, #23348, .F. ) ;
#32335=DIRECTION ( 'NONE',  ( -0.000000000000000000, 0.1736481776669307198, -0.9848077530122080203 ) ) ;
#32336=CARTESIAN_POINT ( 'NONE',  ( 2.557746619330622639, -5.728107161865378494, 34.42597550085002922 ) ) ;
#32337=FACE_OUTER_BOUND ( 'NONE', #19310, .T. ) ;
#32338=VERTEX_POINT ( 'NONE', #2860 ) ;
#32340=ORIENTED_EDGE ( 'NONE', *, *, #20337, .T. ) ;
#32341=CARTESIAN_POINT ( 'NONE',  ( 15.45354877203763522, -5.114059244376869984, 34.14424750095245287 ) ) ;
#32342=ORIENTED_EDGE ( 'NONE', *, *, #29945, .T. ) ;
#32343=CARTESIAN_POINT ( 'NONE',  ( -5.300408001487411092, -2.612411019501189813, 31.66733052389439962 ) ) ;
#32344=CARTESIAN_POINT ( 'NONE',  ( -3.360917200500926683, -5.070767119584671967, 34.40440758774516183 ) ) ;
#32345=CARTESIAN_POINT ( 'NONE',  ( -13.38461538461538325, -8.973038597847269315, 34.52809138561121927 ) ) ;
#32346=CARTESIAN_POINT ( 'NONE',  ( -13.13466986626724164, -12.43552623307873972, 30.55307653245132826 ) ) ;
#32347=ADVANCED_FACE ( 'NONE', ( #22266 ), #15073, .F. ) ;
#32348=VERTEX_POINT ( 'NONE', #85305 ) ;
#32349=ORIENTED_EDGE ( 'NONE', *, *, #44481, .F. ) ;
#32350=ORIENTED_EDGE ( 'NONE', *, *, #64657, .F. ) ;
#32351=CARTESIAN_POINT ( 'NONE',  ( -5.326923076923076650, -7.566083408709834757, 34.74999999999999289 ) ) ;
#32352=CARTESIAN_POINT ( 'NONE',  ( 5.299702618191483694, -5.114059244376869984, 34.14424750095245287 ) ) ;
#32353=EDGE_LOOP ( 'NONE', ( #7274, #85556, #1881, #78275 ) ) ;
#32355=FACE_OUTER_BOUND ( 'NONE', #4628, .T. ) ;
#32356=VECTOR ( 'NONE', #57631, 1000.000000000000227 ) ;
#32357=CARTESIAN_POINT ( 'NONE',  ( -13.45069879557126136, -6.386643153685125363, 34.62446782046654903 ) ) ;
#32358=DIRECTION ( 'NONE',  ( -0.000000000000000000, 0.1736481776669307198, -0.9848077530122080203 ) ) ;
#32359=DIRECTION ( 'NONE',  ( -0.000000000000000000, 0.3420201433256694901, -0.9396926207859082059 ) ) ;
#32360=ADVANCED_FACE ( 'NONE', ( #36233 ), #84426, .F. ) ;
#32361=CARTESIAN_POINT ( 'NONE',  ( 10.74617642320940369, -3.530189275343204702, 32.79018710029569661 ) ) ;
#32362=FACE_BOUND ( 'NONE', #48501, .T. ) ;
#32363=B_SPLINE_CURVE_WITH_KNOTS ( 'NONE', 3,
 ( #73645, #65527, #38969, #3382, #16901, #10597, #11937, #71841, #78598, #52898 ),
 .UNSPECIFIED., .F., .F.,
 ( 4, 2, 2, 2, 4 ),
 ( 0.0007817359430256293554, 0.0009771253907249971907, 0.001172514838424365026, 0.001367904286123733078, 0.001563293733823093758 ),
 .UNSPECIFIED. ) ;
#32364=CARTESIAN_POINT ( 'NONE',  ( -5.076923076923075762, -9.905515769479276145, 34.41647553114623292 ) ) ;
#32365=DIRECTION ( 'NONE',  ( -0.000000000000000000, -0.6427876096865404731, -0.7660444431189770143 ) ) ;
#32366=CYLINDRICAL_SURFACE ( 'NONE', #29357, 0.2499999999999986955 ) ;
#32367=CARTESIAN_POINT ( 'NONE',  ( 9.442284455014730682, -3.202444869320336451, 32.30641848906366675 ) ) ;
#32368=CARTESIAN_POINT ( 'NONE',  ( 6.673053698855467175, -10.92453946501458439, 33.72985991061850086 ) ) ;
#32369=CARTESIAN_POINT ( 'NONE',  ( 0.2380535178145107567, -12.24155766932282496, 31.33739205006857986 ) ) ;
#32370=CARTESIAN_POINT ( 'NONE',  ( 1.384615384615264011, -2.379036618888197285, 30.90682066428292885 ) ) ;
#32372=DIRECTION ( 'NONE',  ( 0.000000000000000000, 0.7660444431189822323, -0.6427876096865344779 ) ) ;
#32373=AXIS2_PLACEMENT_3D ( 'NONE', #38208, #52604, #3081 ) ;
#32374=CARTESIAN_POINT ( 'NONE',  ( -5.999999999999998224, -3.886160181151819604, 36.00935417666054406 ) ) ;
#32375=VERTEX_POINT ( 'NONE', #22702 ) ;
#32376=ORIENTED_EDGE ( 'NONE', *, *, #58103, .F. ) ;
#32377=CARTESIAN_POINT ( 'NONE',  ( -17.32689980786543060, -11.28823185664190376, 33.01397839955799896 ) ) ;
#32378=EDGE_CURVE ( 'NONE', #83375, #34892, #29243, .T. ) ;
#32379=CARTESIAN_POINT ( 'NONE',  ( -13.63461538461537970, -7.566083408709835645, 34.74999999999999289 ) ) ;
#32381=CARTESIAN_POINT ( 'NONE',  ( 12.23805353697412990, -10.97335522853832579, 33.68706563782419749 ) ) ;
#32382=EDGE_LOOP ( 'NONE', ( #70081, #88971, #21221, #2988, #39999, #4308 ) ) ;
#32383=FACE_OUTER_BOUND ( 'NONE', #58617, .T. ) ;
#32384=CARTESIAN_POINT ( 'NONE',  ( -4.283994123577847368, -9.504002272028875709, 34.60269587691767867 ) ) ;
#32385=CARTESIAN_POINT ( 'NONE',  ( 18.00000000000000000, -3.513871655860378418, 32.76840700105978499 ) ) ;
#32386=CARTESIAN_POINT ( 'NONE',  ( 6.000000000000001776, -9.780366693483667717, 34.19971097300155094 ) ) ;
#32387=CARTESIAN_POINT ( 'NONE',  ( -12.52762187249433978, -4.786620604624113540, 33.94971097300155805 ) ) ;
#32389=CARTESIAN_POINT ( 'NONE',  ( -8.769230769230768274, -6.435427911321262684, 35.78748833219616898 ) ) ;
#32391=VERTEX_POINT ( 'NONE', #21823 ) ;
#32392=EDGE_CURVE ( 'NONE', #40861, #73086, #86195, .T. ) ;
#32394=CARTESIAN_POINT ( 'NONE',  ( 4.853996118016225658, -10.77366814457252175, 33.85459836347579454 ) ) ;
#32396=CARTESIAN_POINT ( 'NONE',  ( 6.923076923076802558, -12.27809138561165270, 31.22303859784587132 ) ) ;
#32397=CARTESIAN_POINT ( 'NONE',  ( 16.15384615384603251, -3.083524468854526912, 32.58852847137268327 ) ) ;
#32398=CARTESIAN_POINT ( 'NONE',  ( 17.32692307692307665, -2.249999999999998668, 29.75000000000000355 ) ) ;
#32399=DIRECTION ( 'NONE',  ( 0.000000000000000000, 0.6427876096865368094, 0.7660444431189802339 ) ) ;
#32401=CARTESIAN_POINT ( 'NONE',  ( -9.692307692307691624, -1.117168528481311540, 33.14645433367849847 ) ) ;
#32402=CARTESIAN_POINT ( 'NONE',  ( 2.307692307692309264, -1.422936976036506707, 30.56769352161908415 ) ) ;
#32403=CARTESIAN_POINT ( 'NONE',  ( -13.13461538461531752, -7.434744429011176159, 34.75000000000000711 ) ) ;
#32404=CARTESIAN_POINT ( 'NONE',  ( 5.869309396889692110, -9.929715669179216775, 34.40415004197138416 ) ) ;
#32405=FACE_OUTER_BOUND ( 'NONE', #67655, .T. ) ;
#32406=DIRECTION ( 'NONE',  ( -0.000000000000000000, 0.3420201433256694901, -0.9396926207859082059 ) ) ;
#32407=CARTESIAN_POINT ( 'NONE',  ( -3.361245938885694784, -7.276988635370450709, 34.74523720219453793 ) ) ;
#32408=CYLINDRICAL_SURFACE ( 'NONE', #17079, 0.2499999999999979738 ) ;
#32409=CARTESIAN_POINT ( 'NONE',  ( 10.83816415665302557, -2.847695495035523550, 31.58253572463339154 ) ) ;
#32410=EDGE_CURVE ( 'NONE', #13761, #6434, #26044, .T. ) ;
#32411=DIRECTION ( 'NONE',  ( 0.000000000000000000, 0.000000000000000000, 1.000000000000000000 ) ) ;
#32412=VERTEX_POINT ( 'NONE', #2424 ) ;
#32413=LINE ( 'NONE', #59882, #9627 ) ;
#32414=CARTESIAN_POINT ( 'NONE',  ( -8.769230769230768274, -3.322132147404559976, 32.92929555188717927 ) ) ;
#32415=CARTESIAN_POINT ( 'NONE',  ( -0.2115384615370421995, -7.500000000000154543, 35.00000000000007105 ) ) ;
#32417=CARTESIAN_POINT ( 'NONE',  ( 13.38461538461526601, -10.90142922262034020, 33.41473453929536674 ) ) ;
#32418=DIRECTION ( 'NONE',  ( 0.000000000000000000, 0.1736481776669275834, 0.9848077530122086864 ) ) ;
#32419=DIRECTION ( 'NONE',  ( 0.000000000000000000, 0.000000000000000000, 1.000000000000000000 ) ) ;
#32420=ORIENTED_EDGE ( 'NONE', *, *, #44057, .F. ) ;
#32423=EDGE_CURVE ( 'NONE', #558, #18982, #43280, .T. ) ;
#32424=ORIENTED_EDGE ( 'NONE', *, *, #80208, .F. ) ;
#32425=CARTESIAN_POINT ( 'NONE',  ( -2.084680956079457026, -2.554770724473667709, 30.48948780036025852 ) ) ;
#32426=EDGE_LOOP ( 'NONE', ( #27053, #63144 ) ) ;
#32427=B_SPLINE_CURVE_WITH_KNOTS ( 'NONE', 3,
 ( #48563, #13020, #89145, #88703, #54441, #75174, #62089, #20659, #28298, #76497 ),
 .UNSPECIFIED., .F., .F.,
 ( 4, 2, 2, 2, 4 ),
 ( 0.000000000000000000, 0.0001954311584214073465, 0.0003908623168428146930, 0.0005862934752642220667, 0.0007817246336856293861 ),
 .UNSPECIFIED. ) ;
#32428=CARTESIAN_POINT ( 'NONE',  ( -7.623141002060451754, -6.460100341425560444, 34.89618726649961644 ) ) ;
#32429=ADVANCED_FACE ( 'NONE', ( #10976 ), #71770, .F. ) ;
#32430=EDGE_CURVE ( 'NONE', #68029, #12728, #30788, .T. ) ;
#32431=CARTESIAN_POINT ( 'NONE',  ( 13.25446817517716980, -10.19110544564092002, 33.96427741523702792 ) ) ;
#32433=CARTESIAN_POINT ( 'NONE',  ( -0.4615384615385840772, -6.835583212225970762, 34.95778746994575670 ) ) ;
#32434=ORIENTED_EDGE ( 'NONE', *, *, #81956, .T. ) ;
#32435=CARTESIAN_POINT ( 'NONE',  ( -11.53846153846153655, -11.35647404775217417, 33.31231777344666511 ) ) ;
#32436=ORIENTED_EDGE ( 'NONE', *, *, #65168, .F. ) ;
#32437=EDGE_CURVE ( 'NONE', #65096, #62997, #72216, .T. ) ;
#32438=EDGE_LOOP ( 'NONE', ( #28709, #83039, #84405, #69284 ) ) ;
#32439=CARTESIAN_POINT ( 'NONE',  ( 13.51540719244017374, -11.71459661697925903, 32.44059661609676937 ) ) ;
#32440=CARTESIAN_POINT ( 'NONE',  ( 6.000000000000001776, -1.466349020453238561, 30.81389545987213907 ) ) ;
#32441=CARTESIAN_POINT ( 'NONE',  ( -10.61538461538461320, -6.386643153685126251, 34.62446782046654192 ) ) ;
#32442=DIRECTION ( 'NONE',  ( -0.000000000000000000, -0.8660254037844399289, -0.4999999999999980016 ) ) ;
#32443=DIRECTION ( 'NONE',  ( 0.000000000000000000, 0.7660444431189807890, 0.6427876096865361433 ) ) ;
#32444=CARTESIAN_POINT ( 'NONE',  ( 11.31497659473759043, -11.89387501736622710, 32.13663884655806413 ) ) ;
#32445=DIRECTION ( 'NONE',  ( 0.000000000000000000, 0.000000000000000000, 1.000000000000000000 ) ) ;
#32446=ORIENTED_EDGE ( 'NONE', *, *, #50110, .F. ) ;
#32448=VERTEX_POINT ( 'NONE', #73116 ) ;
#32449=CARTESIAN_POINT ( 'NONE',  ( -4.153846153846274980, -8.656820664282941280, 34.87096338111179961 ) ) ;
#32450=ORIENTED_EDGE ( 'NONE', *, *, #16401, .T. ) ;
#32451=CARTESIAN_POINT ( 'NONE',  ( -9.019254006523732770, -10.05641848906368097, 34.04755513067966177 ) ) ;
#32452=CARTESIAN_POINT ( 'NONE',  ( 1.634669696253701510, -2.779044189368096607, 31.39831045268885035 ) ) ;
#32453=EDGE_LOOP ( 'NONE', ( #18900, #14732 ) ) ;
#32454=CYLINDRICAL_SURFACE ( 'NONE', #77544, 0.2500000000000002220 ) ;
#32456=VERTEX_POINT ( 'NONE', #79875 ) ;
#32457=CARTESIAN_POINT ( 'NONE',  ( 0.2115384615384550415, -2.499999999999999556, 29.81609845454691765 ) ) ;
#32458=VERTEX_POINT ( 'NONE', #17280 ) ;
#32459=CARTESIAN_POINT ( 'NONE',  ( 5.076923076923075762, -2.249999999999998668, 29.75000000000001776 ) ) ;
#32460=CYLINDRICAL_SURFACE ( 'NONE', #37383, 0.2499999999999998890 ) ;
#32461=CARTESIAN_POINT ( 'NONE',  ( -16.08777882049607655, -10.67929555188718282, 33.92786785259544757 ) ) ;
#32462=FACE_BOUND ( 'NONE', #48383, .T. ) ;
#32464=FACE_OUTER_BOUND ( 'NONE', #56947, .T. ) ;
#32466=CARTESIAN_POINT ( 'NONE',  ( 4.826946332874483936, -3.436278759898155677, 33.07459398097509506 ) ) ;
#32467=CARTESIAN_POINT ( 'NONE',  ( 10.74543222164029821, -7.723484964179501588, 34.74522123443823318 ) ) ;
#32469=ORIENTED_EDGE ( 'NONE', *, *, #6318, .T. ) ;
#32470=DIRECTION ( 'NONE',  ( -0.000000000000000000, 0.6427876096865404731, -0.7660444431189771253 ) ) ;
#32471=ORIENTED_EDGE ( 'NONE', *, *, #1781, .F. ) ;
#32472=ORIENTED_EDGE ( 'NONE', *, *, #20346, .F. ) ;
#32473=CARTESIAN_POINT ( 'NONE',  ( 10.61538461538449596, -12.46129190930018460, 30.37095296980731973 ) ) ;
#32474=FACE_OUTER_BOUND ( 'NONE', #905, .T. ) ;
#32475=CARTESIAN_POINT ( 'NONE',  ( 16.28463659481310799, -11.37503395064541678, 33.29242100308974983 ) ) ;
#32476=CARTESIAN_POINT ( 'NONE',  ( -14.53061926659915315, -11.98009711892699514, 32.48740034544076138 ) ) ;
#32477=LINE ( 'NONE', #59950, #37142 ) ;
#32478=CARTESIAN_POINT ( 'NONE',  ( -2.177166605928743781, -2.882268652242222284, 31.66798894389554064 ) ) ;
#32482=CARTESIAN_POINT ( 'NONE',  ( 0.5267940328144847806, -10.21337939537593797, 33.94971097300152252 ) ) ;
#32484=DIRECTION ( 'NONE',  ( 0.000000000000000000, 0.3420201433256610524, 0.9396926207859113145 ) ) ;
#32485=ORIENTED_EDGE ( 'NONE', *, *, #47633, .T. ) ;
#32487=EDGE_CURVE ( 'NONE', #61793, #64477, #31235, .T. ) ;
#32490=CARTESIAN_POINT ( 'NONE',  ( 15.36129493253279676, -6.852161475712352789, 34.70806712695775786 ) ) ;
#32491=CARTESIAN_POINT ( 'NONE',  ( 11.53846153846141576, -3.643525952248795718, 33.31231777344771672 ) ) ;
#32493=VECTOR ( 'NONE', #43546, 999.9999999999998863 ) ;
#32494=CARTESIAN_POINT ( 'NONE',  ( 3.100621261037534993, -12.70455904226513866, 30.44083106164009322 ) ) ;
#32495=DIRECTION ( 'NONE',  ( -0.000000000000000000, 0.5000000000000011102, -0.8660254037844381525 ) ) ;
#32496=CARTESIAN_POINT ( 'NONE',  ( 0.6843180028068707177, -12.24180327182771855, 31.33663988360758168 ) ) ;
#32497=CARTESIAN_POINT ( 'NONE',  ( 8.900021210197719412, -3.338503747796866872, 32.95102852606553512 ) ) ;
#32498=FACE_OUTER_BOUND ( 'NONE', #48842, .T. ) ;
#32499=ORIENTED_EDGE ( 'NONE', *, *, #14947, .T. ) ;
#32500=CARTESIAN_POINT ( 'NONE',  ( 0.3954550505825797924, -9.780366693483667717, 34.19971097300155805 ) ) ;
#32502=LINE ( 'NONE', #18999, #19570 ) ;
#32503=CARTESIAN_POINT ( 'NONE',  ( 15.93098073164252249, -2.501496062324911840, 29.88072118266895671 ) ) ;
#32504=CARTESIAN_POINT ( 'NONE',  ( -7.846153846153844924, -6.343179335718451384, 34.87096338111211935 ) ) ;
#32505=CARTESIAN_POINT ( 'NONE',  ( 15.23076923076911093, -12.46129190930018460, 30.37095296980731973 ) ) ;
#32506=DIRECTION ( 'NONE',  ( 0.000000000000000000, 0.000000000000000000, 1.000000000000000000 ) ) ;
#32508=DIRECTION ( 'NONE',  ( -0.000000000000000000, -0.9396926207859092051, -0.3420201433256662704 ) ) ;
#32510=VERTEX_POINT ( 'NONE', #72664 ) ;
#32511=CARTESIAN_POINT ( 'NONE',  ( 11.78840705680968348, -2.824170634883621744, 31.52227843825338738 ) ) ;
#32512=CARTESIAN_POINT ( 'NONE',  ( 8.069580245068634028, -7.630147987733840509, 34.99859428049666121 ) ) ;
#32513=CARTESIAN_POINT ( 'NONE',  ( -13.38461538461538325, -4.661471528628507777, 34.16647553114623292 ) ) ;
#32515=VERTEX_POINT ( 'NONE', #58258 ) ;
#32517=CARTESIAN_POINT ( 'NONE',  ( -11.53846153846165912, -10.90142922262034020, 33.41473453929536674 ) ) ;
#32518=CARTESIAN_POINT ( 'NONE',  ( 8.769230769230647482, -8.613356846316285953, 34.62446782046622218 ) ) ;
#32519=CARTESIAN_POINT ( 'NONE',  ( -0.2381625208402778360, -2.501478030877323011, 29.88021232661721172 ) ) ;
#32520=VECTOR ( 'NONE', #6717, 999.9999999999998863 ) ;
#32521=LINE ( 'NONE', #81610, #12842 ) ;
#32523=CARTESIAN_POINT ( 'NONE',  ( -7.173100160369890510, -11.86270091957321249, 32.19358267280087915 ) ) ;
#32524=ORIENTED_EDGE ( 'NONE', *, *, #25312, .T. ) ;
#32525=CARTESIAN_POINT ( 'NONE',  ( 9.627037246346917598, -10.90142922261923886, 33.41473453929638993 ) ) ;
#32526=EDGE_CURVE ( 'NONE', #60729, #46284, #51479, .T. ) ;
#32527=EDGE_CURVE ( 'NONE', #33691, #29899, #78675, .T. ) ;
#32528=CARTESIAN_POINT ( 'NONE',  ( -2.241623956689867470, -9.780366693483667717, 34.19971097300155805 ) ) ;
#32529=CARTESIAN_POINT ( 'NONE',  ( -5.076923076923075762, -9.058645607665452459, 34.76329471203371924 ) ) ;
#32530=ORIENTED_EDGE ( 'NONE', *, *, #36992, .T. ) ;
#32531=CARTESIAN_POINT ( 'NONE',  ( 12.46153846153846168, -2.486705287966279876, 31.30864560766543647 ) ) ;
#32532=ORIENTED_EDGE ( 'NONE', *, *, #30154, .T. ) ;
#32533=EDGE_CURVE ( 'NONE', #60409, #47762, #49643, .T. ) ;
#32534=CARTESIAN_POINT ( 'NONE',  ( 13.60739492588379740, -3.755027918224367767, 33.06320215134714857 ) ) ;
#32537=CARTESIAN_POINT ( 'NONE',  ( 15.23076923076923173, -4.661471528628507777, 34.16647553114623292 ) ) ;
#32538=ORIENTED_EDGE ( 'NONE', *, *, #64913, .T. ) ;
#32539=CARTESIAN_POINT ( 'NONE',  ( 12.33084699487089964, -3.530157926970578952, 32.79014554554150607 ) ) ;
#32540=DIRECTION ( 'NONE',  ( -0.000000000000000000, 0.3420201433256694346, -0.9396926207859080948 ) ) ;
#32541=CARTESIAN_POINT ( 'NONE',  ( -16.15384615384615330, -1.951392089020283160, 34.73218667398347748 ) ) ;
#32543=CARTESIAN_POINT ( 'NONE',  ( -5.076923076923199218, -11.06231777344772027, 33.60647404775119895 ) ) ;
#32545=B_SPLINE_CURVE_WITH_KNOTS ( 'NONE', 3,
 ( #77679, #38037, #44320, #85786, #65501, #22733, #3800, #30386, #56961, #58746 ),
 .UNSPECIFIED., .F., .F.,
 ( 4, 2, 2, 2, 4 ),
 ( 0.0007817246256747457630, 0.0009771112852218887673, 0.001172497944769031880, 0.001367884604316174993, 0.001563271263863318106 ),
 .UNSPECIFIED. ) ;
#32546=CARTESIAN_POINT ( 'NONE',  ( -4.153846153846274980, -12.51329471203414379, 31.30864560766407578 ) ) ;
#32547=ORIENTED_EDGE ( 'NONE', *, *, #34356, .F. ) ;
#32548=CARTESIAN_POINT ( 'NONE',  ( -5.076923076923075762, -9.584722331328613620, 36.20867863119891439 ) ) ;
#32549=B_SPLINE_CURVE_WITH_KNOTS ( 'NONE', 3,
 ( #43219, #14874, #8110, #35582, #63028, #44525, #86895, #16620, #9869, #45423 ),
 .UNSPECIFIED., .F., .F.,
 ( 4, 2, 2, 2, 4 ),
 ( 0.000000000000000000, 0.0001954339857564079080, 0.0003908679715128158161, 0.0005863019572692237513, 0.0007817359430256316322 ),
 .UNSPECIFIED. ) ;
#32550=B_SPLINE_CURVE_WITH_KNOTS ( 'NONE', 3,
 ( #53558, #6703, #74286, #46808, #75178, #20661, #12584, #5386, #34176, #81938 ),
 .UNSPECIFIED., .F., .F.,
 ( 4, 2, 2, 2, 4 ),
 ( 0.0007817246256747444619, 0.0009771112852218868158, 0.001172497944769029061, 0.001367884604316171523, 0.001563271263863313769 ),
 .UNSPECIFIED. ) ;
#32551=DIRECTION ( 'NONE',  ( 0.000000000000000000, 0.9396926207859126468, 0.3420201433256571111 ) ) ;
#32552=CARTESIAN_POINT ( 'NONE',  ( -3.453647913197877894, -7.630691491037286056, 34.74850469731152458 ) ) ;
#32555=DIRECTION ( 'NONE',  ( -0.000000000000000000, -0.000000000000000000, -1.000000000000000000 ) ) ;
#32558=ORIENTED_EDGE ( 'NONE', *, *, #47438, .F. ) ;
#32559=ORIENTED_EDGE ( 'NONE', *, *, #76740, .T. ) ;
#32560=ORIENTED_EDGE ( 'NONE', *, *, #68039, .F. ) ;
#32561=ORIENTED_EDGE ( 'NONE', *, *, #27126, .F. ) ;
#32562=CARTESIAN_POINT ( 'NONE',  ( -10.61538461538473399, -11.48612834414049644, 32.76840700105863391 ) ) ;
#32563=DIRECTION ( 'NONE',  ( -0.000000000000000000, 0.3420201433256694901, -0.9396926207859082059 ) ) ;
#32564=CARTESIAN_POINT ( 'NONE',  ( 8.769230769230768274, -2.249999999999998668, 29.75000000000001776 ) ) ;
#32565=CARTESIAN_POINT ( 'NONE',  ( 3.903822916553187028, -3.202444869320336451, 32.30641848906366675 ) ) ;
#32566=CARTESIAN_POINT ( 'NONE',  ( 17.93472955403921887, -10.21337939537584383, 33.94971097300158647 ) ) ;
#32567=VECTOR ( 'NONE', #71961, 1000.000000000000227 ) ;
#32569=CARTESIAN_POINT ( 'NONE',  ( 13.38461538461538680, -2.708943851104267164, 35.45975837776705220 ) ) ;
#32570=CARTESIAN_POINT ( 'NONE',  ( 0.2115617305961072503, -3.137211980971221781, 32.19342716148376837 ) ) ;
#32572=VERTEX_POINT ( 'NONE', #25370 ) ;
#32574=B_SPLINE_CURVE_WITH_KNOTS ( 'NONE', 3,
 ( #2079, #64212, #22789, #84954, #85392, #43952, #43073, #50253, #71867, #63338 ),
 .UNSPECIFIED., .F., .F.,
 ( 4, 2, 2, 2, 4 ),
 ( 0.0007817359430256346680, 0.0009771253907250002264, 0.001172514838424365893, 0.001367904286123731560, 0.001563293733823104166 ),
 .UNSPECIFIED. ) ;
#32576=ORIENTED_EDGE ( 'NONE', *, *, #18921, .T. ) ;
#32577=CARTESIAN_POINT ( 'NONE',  ( -1.634638621908349077, -11.37209801155882971, 32.91403422569032955 ) ) ;
#32578=VERTEX_POINT ( 'NONE', #37540 ) ;
#32580=DIRECTION ( 'NONE',  ( -0.000000000000000000, -0.7660444431189791237, -0.6427876096865379196 ) ) ;
#32581=B_SPLINE_CURVE_WITH_KNOTS ( 'NONE', 3,
 ( #48503, #33679, #55267, #82757, #76433, #6643, #74671, #14285, #28694, #41767 ),
 .UNSPECIFIED., .F., .F.,
 ( 4, 2, 2, 2, 4 ),
 ( 0.000000000000000000, 0.0001954311564186879315, 0.0003908623128373758630, 0.0005862934692560637946, 0.0007817246256747517261 ),
 .UNSPECIFIED. ) ;
#32582=B_SPLINE_CURVE_WITH_KNOTS ( 'NONE', 3,
 ( #10494, #72626, #4167, #67217, #52349, #31193, #72181, #65427, #38855, #3722 ),
 .UNSPECIFIED., .F., .F.,
 ( 4, 2, 2, 2, 4 ),
 ( 0.0007817246256747484735, 0.0009771112852218920199, 0.001172497944769035783, 0.001367884604316179330, 0.001563271263863322876 ),
 .UNSPECIFIED. ) ;
#32583=CARTESIAN_POINT ( 'NONE',  ( -0.3954711281883849794, -2.292212530054420494, 30.41441678777542990 ) ) ;
#32584=CARTESIAN_POINT ( 'NONE',  ( 4.153846153846154188, -2.538708090699994813, 30.37095296980875503 ) ) ;
#32585=FACE_BOUND ( 'NONE', #76375, .T. ) ;
#32588=ORIENTED_EDGE ( 'NONE', *, *, #61694, .F. ) ;
#32589=CYLINDRICAL_SURFACE ( 'NONE', #41395, 0.2500000000000002220 ) ;
#32590=EDGE_LOOP ( 'NONE', ( #71345, #21382, #57697, #47037 ) ) ;
#32591=FACE_BOUND ( 'NONE', #73127, .T. ) ;
#32592=CARTESIAN_POINT ( 'NONE',  ( 7.780070435197965040, -11.69971097300155272, 32.46337939537587403 ) ) ;
#32594=CARTESIAN_POINT ( 'NONE',  ( 8.096153846153860911, -2.249999999999999112, 29.81603969181031033 ) ) ;
#32595=VERTEX_POINT ( 'NONE', #70757 ) ;
#32596=DIRECTION ( 'NONE',  ( -0.000000000000000000, -0.9848077530122085754, -0.1736481776669273613 ) ) ;
#32598=DIRECTION ( 'NONE',  ( 0.000000000000000000, 0.7660444431189822323, -0.6427876096865344779 ) ) ;
#32599=EDGE_LOOP ( 'NONE', ( #33509, #57423 ) ) ;
#32600=ADVANCED_FACE ( 'NONE', ( #84286 ), #49594, .F. ) ;
#32601=CARTESIAN_POINT ( 'NONE',  ( 14.55763771707035303, -3.520799739797214389, 33.17531984108286025 ) ) ;
#32602=CARTESIAN_POINT ( 'NONE',  ( 7.173131342990376247, -5.642605341092957083, 34.66089969410670335 ) ) ;
#32603=CARTESIAN_POINT ( 'NONE',  ( -13.38461538461538325, -6.343179335718451384, 34.87096338111211935 ) ) ;
#32604=ORIENTED_EDGE ( 'NONE', *, *, #61591, .F. ) ;
#32606=CARTESIAN_POINT ( 'NONE',  ( -9.442253272394237840, -9.233818618650603938, 34.70587769442853698 ) ) ;
#32607=EDGE_LOOP ( 'NONE', ( #19834, #24447 ) ) ;
#32608=CARTESIAN_POINT ( 'NONE',  ( 3.361559671736181087, -6.369690395747422684, 34.87708834333098196 ) ) ;
#32609=DIRECTION ( 'NONE',  ( 0.000000000000000000, 0.6427876096865373645, -0.7660444431189797898 ) ) ;
#32610=CARTESIAN_POINT ( 'NONE',  ( -7.911423846710164298, -12.51329471203370325, 31.30864560766548976 ) ) ;
#32611=CARTESIAN_POINT ( 'NONE',  ( -11.78848477575450282, -8.432397168068783699, 34.66272746175022945 ) ) ;
#32612=DIRECTION ( 'NONE',  ( -1.000000000000000000, 0.000000000000000000, 0.000000000000000000 ) ) ;
#32614=CARTESIAN_POINT ( 'NONE',  ( 2.307692307692309264, -3.886160181151819604, 36.00935417666054406 ) ) ;
#32615=CARTESIAN_POINT ( 'NONE',  ( 6.000000000000001776, -11.69971097300155272, 32.46337939537588113 ) ) ;
#32616=CARTESIAN_POINT ( 'NONE',  ( -20.99999999999999645, -10.75000000000000000, 27.25000000000000000 ) ) ;
#32617=EDGE_CURVE ( 'NONE', #70140, #40157, #65752, .T. ) ;
#32618=CARTESIAN_POINT ( 'NONE',  ( 10.86543903529806876, -9.233818618650603938, 34.70587769442853698 ) ) ;
#32619=CARTESIAN_POINT ( 'NONE',  ( -12.23852710992561299, -11.24521262558773493, 33.06293181088029343 ) ) ;
#32621=ORIENTED_EDGE ( 'NONE', *, *, #11352, .F. ) ;
#32624=VERTEX_POINT ( 'NONE', #42846 ) ;
#32625=EDGE_CURVE ( 'NONE', #78937, #37879, #21729, .T. ) ;
#32626=VERTEX_POINT ( 'NONE', #9061 ) ;
#32627=CARTESIAN_POINT ( 'NONE',  ( -7.596099426240389363, -2.544122305571458575, 31.48381861865057729 ) ) ;
#32628=VERTEX_POINT ( 'NONE', #83843 ) ;
#32629=CARTESIAN_POINT ( 'NONE',  ( 3.453780582382081743, -9.886259254753566594, 34.14407573483972413 ) ) ;
#32631=CARTESIAN_POINT ( 'NONE',  ( 12.71153846153852385, -7.434744860731433924, 35.00000000000000711 ) ) ;
#32632=DIRECTION ( 'NONE',  ( 0.000000000000000000, 0.7660444431189822323, -0.6427876096865344779 ) ) ;
#32633=CARTESIAN_POINT ( 'NONE',  ( -7.780085495151407571, -5.557115091759786019, 34.35708131394839882 ) ) ;
#32634=CARTESIAN_POINT ( 'NONE',  ( 9.915320536401091900, -2.889357225399416418, 32.26129605718031002 ) ) ;
#32635=CARTESIAN_POINT ( 'NONE',  ( -10.36543920600657209, -3.520799739797214389, 33.17531984108286025 ) ) ;
#32636=CARTESIAN_POINT ( 'NONE',  ( 0.7114838709165038910, -5.766571408460172243, 34.70601412856602508 ) ) ;
#32637=DIRECTION ( 'NONE',  ( -0.000000000000000000, -0.000000000000000000, -1.000000000000000000 ) ) ;
#32639=CARTESIAN_POINT ( 'NONE',  ( 5.326868486301119532, -2.986452184633680673, 32.43230066228895225 ) ) ;
#32640=CARTESIAN_POINT ( 'NONE',  ( -13.13466986626724164, -6.696923467548660192, 34.68552623307873972 ) ) ;
#32641=EDGE_CURVE ( 'NONE', #60920, #83778, #77559, .T. ) ;
#32642=ADVANCED_FACE ( 'NONE', ( #44588 ), #77072, .F. ) ;
#32644=ORIENTED_EDGE ( 'NONE', *, *, #36042, .F. ) ;
#32645=ORIENTED_EDGE ( 'NONE', *, *, #60924, .F. ) ;
#32646=EDGE_CURVE ( 'NONE', #29234, #33682, #6740, .T. ) ;
#32647=AXIS2_PLACEMENT_3D ( 'NONE', #78953, #10502, #29016 ) ;
#32648=CARTESIAN_POINT ( 'NONE',  ( -11.40766973063675316, -5.582136614379148654, 34.36778462344220486 ) ) ;
#32649=DIRECTION ( 'NONE',  ( -0.000000000000000000, -0.3420201433256694346, -0.9396926207859080948 ) ) ;
#32651=CARTESIAN_POINT ( 'NONE',  ( -16.08859058257013430, -12.46129190930001052, 30.37095296980869819 ) ) ;
#32652=EDGE_CURVE ( 'NONE', #10983, #83460, #57139, .T. ) ;
#32653=DIRECTION ( 'NONE',  ( -0.000000000000000000, 0.8660254037844397068, -0.4999999999999978906 ) ) ;
#32654=CARTESIAN_POINT ( 'NONE',  ( -5.011667937410239304, -3.083524468853784839, 32.58852847137153930 ) ) ;
#32655=VECTOR ( 'NONE', #81715, 1000.000000000000000 ) ;
#32656=ORIENTED_EDGE ( 'NONE', *, *, #30994, .T. ) ;
#32657=CARTESIAN_POINT ( 'NONE',  ( 15.93091993633000847, -2.758268499246657068, 31.33685645148948851 ) ) ;
#32659=EDGE_LOOP ( 'NONE', ( #57781, #75431 ) ) ;
#32660=CARTESIAN_POINT ( 'NONE',  ( 17.99999999999987566, -3.300289026999228437, 32.46337939537709616 ) ) ;
#32661=CARTESIAN_POINT ( 'NONE',  ( -2.437840277424001556, -9.504002272028875709, 34.60269587691767867 ) ) ;
#32662=CARTESIAN_POINT ( 'NONE',  ( -0.2115384615383984479, -7.434744860731433036, 35.00000000000000000 ) ) ;
#32663=CARTESIAN_POINT ( 'NONE',  ( 4.153846153846154188, -6.343179335718451384, 34.87096338111211935 ) ) ;
#32664=CARTESIAN_POINT ( 'NONE',  ( 9.692307692307695177, -6.386643153685126251, 34.62446782046654192 ) ) ;
#32665=ORIENTED_EDGE ( 'NONE', *, *, #11464, .F. ) ;
#32666=ORIENTED_EDGE ( 'NONE', *, *, #66581, .F. ) ;
#32667=ADVANCED_FACE ( 'NONE', ( #71624 ), #9929, .F. ) ;
#32668=AXIS2_PLACEMENT_3D ( 'NONE', #11152, #64305, #66086 ) ;
#32669=ORIENTED_EDGE ( 'NONE', *, *, #29519, .T. ) ;
#32670=DIRECTION ( 'NONE',  ( -0.000000000000000000, -0.8660254037844399289, -0.4999999999999980016 ) ) ;
#32672=AXIS2_PLACEMENT_3D ( 'NONE', #14857, #68895, #70230 ) ;
#32674=CARTESIAN_POINT ( 'NONE',  ( -11.53846153846165912, -12.27809138561165270, 31.22303859784587132 ) ) ;
#32675=CARTESIAN_POINT ( 'NONE',  ( -18.00000000000000000, -8.317224813626184599, 35.82440484884453724 ) ) ;
#32676=CARTESIAN_POINT ( 'NONE',  ( -2.307692307692427391, -6.026961402154118908, 34.52809138561165270 ) ) ;
#32677=ORIENTED_EDGE ( 'NONE', *, *, #4309, .T. ) ;
#32678=EDGE_CURVE ( 'NONE', #2810, #30821, #51327, .T. ) ;
#32679=ORIENTED_EDGE ( 'NONE', *, *, #58514, .T. ) ;
#32681=EDGE_CURVE ( 'NONE', #76616, #7349, #16303, .T. ) ;
#32682=CARTESIAN_POINT ( 'NONE',  ( 11.40777007179398161, -8.999036380462717588, 34.52022231692819076 ) ) ;
#32683=VERTEX_POINT ( 'NONE', #60339 ) ;
#32684=CARTESIAN_POINT ( 'NONE',  ( 1.161689167099237974, -9.886141570436013382, 34.14413921362392301 ) ) ;
#32685=CARTESIAN_POINT ( 'NONE',  ( -9.822999158975250111, -11.71456829005830080, 32.44064028649416542 ) ) ;
#32686=ORIENTED_EDGE ( 'NONE', *, *, #61432, .T. ) ;
#32687=CARTESIAN_POINT ( 'NONE',  ( -1.254089946381740983, -11.66157788607254275, 32.95092075102925833 ) ) ;
#32688=EDGE_LOOP ( 'NONE', ( #47891, #12366 ) ) ;
#32689=CARTESIAN_POINT ( 'NONE',  ( -5.076923076923199218, -8.656820664282941280, 34.87096338111179961 ) ) ;
#32690=CYLINDRICAL_SURFACE ( 'NONE', #81746, 0.2500000000000002220 ) ;
#32691=CARTESIAN_POINT ( 'NONE',  ( 12.46153846153833911, -10.21337939537710326, 33.94971097300076224 ) ) ;
#32692=CARTESIAN_POINT ( 'NONE',  ( 16.15384615384615330, -2.708943851104267164, 35.45975837776705220 ) ) ;
#32693=EDGE_CURVE ( 'NONE', #36501, #85855, #68948, .T. ) ;
#32695=CARTESIAN_POINT ( 'NONE',  ( 4.153846153846154188, -1.215029322943914858, 32.30358669280327177 ) ) ;
#32696=VERTEX_POINT ( 'NONE', #65755 ) ;
#32697=CARTESIAN_POINT ( 'NONE',  ( -0.4615384615384611200, -2.292212530054420494, 30.41441678777542634 ) ) ;
#32698=CARTESIAN_POINT ( 'NONE',  ( 15.23076923076911093, -4.481592998941358097, 33.73612834414048933 ) ) ;
#32699=EDGE_CURVE ( 'NONE', #1879, #11337, #33377, .T. ) ;
#32700=CARTESIAN_POINT ( 'NONE',  ( -14.05774678934416677, -2.824170634883621744, 31.52227843825338738 ) ) ;
#32701=ORIENTED_EDGE ( 'NONE', *, *, #65048, .T. ) ;
#32704=CARTESIAN_POINT ( 'NONE',  ( 10.61538461538449418, -8.656820664282941280, 34.87096338111179961 ) ) ;
#32705=CARTESIAN_POINT ( 'NONE',  ( -4.023055712879203938, -2.295524264805589354, 30.44142389570982488 ) ) ;
#32706=CARTESIAN_POINT ( 'NONE',  ( 11.40831432902331954, -6.001485441113819874, 34.52039167877662607 ) ) ;
#32707=CARTESIAN_POINT ( 'NONE',  ( 8.096208157792158744, -3.136992222400443175, 32.19305428654138979 ) ) ;
#32708=FACE_BOUND ( 'NONE', #5995, .T. ) ;
#32710=CARTESIAN_POINT ( 'NONE',  ( 4.219913487196229163, -12.62096338111211757, 30.90682066428152908 ) ) ;
#32712=B_SPLINE_CURVE_WITH_KNOTS ( 'NONE', 3,
 ( #57008, #57452, #70534, #24108, #51558, #50688 ),
 .UNSPECIFIED., .F., .F.,
 ( 4, 2, 4 ),
 ( 0.0003909569690057850379, 0.0005862646681846119933, 0.0007815723673634389487 ),
 .UNSPECIFIED. ) ;
#32713=EDGE_CURVE ( 'NONE', #7735, #79114, #4513, .T. ) ;
#32714=DIRECTION ( 'NONE',  ( -0.000000000000000000, -0.9848077530122086864, -0.1736481776669273613 ) ) ;
#32715=CARTESIAN_POINT ( 'NONE',  ( -11.78846153846153832, -7.500000000000001776, 34.75000000000000000 ) ) ;
#32716=DIRECTION ( 'NONE',  ( 0.000000000000000000, 0.1736481776669267785, -0.9848077530122087975 ) ) ;
#32717=CYLINDRICAL_SURFACE ( 'NONE', #36197, 0.2499999999999986955 ) ;
#32718=B_SPLINE_CURVE_WITH_KNOTS ( 'NONE', 3,
 ( #34787, #53732, #46967, #20833, #6874, #40233, #61812, #42007, #27591, #569 ),
 .UNSPECIFIED., .F., .F.,
 ( 4, 2, 2, 2, 4 ),
 ( 0.0007817246256747442451, 0.0009771112852218865989, 0.001172497944769029061, 0.001367884604316171523, 0.001563271263863313986 ),
 .UNSPECIFIED. ) ;
#32720=ORIENTED_EDGE ( 'NONE', *, *, #25744, .F. ) ;
#32721=CARTESIAN_POINT ( 'NONE',  ( -9.692307692307691624, -13.78497067705608181, 32.30358669280327177 ) ) ;
#32723=CARTESIAN_POINT ( 'NONE',  ( 0.2115152242454954312, -6.695914987888143877, 34.68535235679833306 ) ) ;
#32724=EDGE_LOOP ( 'NONE', ( #17466, #14961, #60280, #48141 ) ) ;
#32725=CARTESIAN_POINT ( 'NONE',  ( -15.45364791319787834, -7.630691491037285168, 34.74850469731152458 ) ) ;
#32726=CARTESIAN_POINT ( 'NONE',  ( -13.44986531638946836, -2.255955759149247175, 30.00000000000013856 ) ) ;
#32727=CARTESIAN_POINT ( 'NONE',  ( -4.854143407945009869, -9.418065098278011860, 34.63729479722530158 ) ) ;
#32728=ORIENTED_EDGE ( 'NONE', *, *, #28566, .T. ) ;
#32729=CARTESIAN_POINT ( 'NONE',  ( -16.28453762051371712, -2.541943142973489334, 30.39792223712631980 ) ) ;
#32730=CARTESIAN_POINT ( 'NONE',  ( -3.230769230769352962, -6.835583212225970762, 34.95778746994575670 ) ) ;
#32732=DIRECTION ( 'NONE',  ( -0.000000000000000000, -0.8660254037844399289, -0.4999999999999980016 ) ) ;
#32735=CYLINDRICAL_SURFACE ( 'NONE', #84744, 0.2500000000000002220 ) ;
#32736=CARTESIAN_POINT ( 'NONE',  ( 15.23076923076923173, -4.945431358278436385, 36.03766855953609394 ) ) ;
#32737=CARTESIAN_POINT ( 'NONE',  ( 9.442284468086239002, -3.520140089381495585, 33.17453946501458262 ) ) ;
#32739=AXIS2_PLACEMENT_3D ( 'NONE', #13981, #42797, #20306 ) ;
#32741=EDGE_CURVE ( 'NONE', #36624, #13172, #76444, .T. ) ;
#32743=VERTEX_POINT ( 'NONE', #51784 ) ;
#32744=CARTESIAN_POINT ( 'NONE',  ( 7.173076923076861178, -7.565270000091922853, 34.99999999999999289 ) ) ;
#32745=CARTESIAN_POINT ( 'NONE',  ( 8.992010310499175318, -11.41317474335729543, 32.86274602512330034 ) ) ;
#32747=EDGE_CURVE ( 'NONE', #21625, #1947, #39925, .T. ) ;
#32748=CARTESIAN_POINT ( 'NONE',  ( 6.989144256427000990, -10.67929555188718282, 33.92786785259544757 ) ) ;
#32749=CARTESIAN_POINT ( 'NONE',  ( 17.20744877868664346, -11.93748526763465279, 32.05452791011430946 ) ) ;
#32750=EDGE_LOOP ( 'NONE', ( #7682, #78897 ) ) ;
#32752=CARTESIAN_POINT ( 'NONE',  ( 6.000000000000001776, -3.322132147404559976, 32.92929555188717927 ) ) ;
#32753=CARTESIAN_POINT ( 'NONE',  ( 4.853438152358743096, -12.47654668319379567, 31.42292124445336654 ) ) ;
#32754=VERTEX_POINT ( 'NONE', #81077 ) ;
#32755=CARTESIAN_POINT ( 'NONE',  ( 16.15384615384615330, -12.09954503811598769, 35.62045528018868623 ) ) ;
#32756=CARTESIAN_POINT ( 'NONE',  ( -2.557692307692306155, -7.566082377512563184, 35.00000000000000711 ) ) ;
#32758=AXIS2_PLACEMENT_3D ( 'NONE', #60566, #12390, #24559 ) ;
#32759=CARTESIAN_POINT ( 'NONE',  ( 2.307692307692309264, -12.37446782046654192, 30.86335684631486131 ) ) ;
#32760=CARTESIAN_POINT ( 'NONE',  ( 11.60371710973756443, -9.442884908240273489, 34.35708131394835618 ) ) ;
#32761=EDGE_LOOP ( 'NONE', ( #4228, #26594, #18704, #83008 ) ) ;
#32762=B_SPLINE_CURVE_WITH_KNOTS ( 'NONE', 3,
 ( #74660, #7075, #321, #6633, #28225, #55694, #54816, #12947, #75974, #83186 ),
 .UNSPECIFIED., .F., .F.,
 ( 4, 2, 2, 2, 4 ),
 ( 0.000000000000000000, 0.0001954311584214072923, 0.0003908623168428145846, 0.0005862934752642218498, 0.0007817246336856291692 ),
 .UNSPECIFIED. ) ;
#32763=CYLINDRICAL_SURFACE ( 'NONE', #47779, 0.2499999999999986955 ) ;
#32764=B_SPLINE_CURVE_WITH_KNOTS ( 'NONE', 3,
 ( #36168, #28971, #83468, #78022, #49227, #49665, #35264, #77141, #83915, #71252 ),
 .UNSPECIFIED., .F., .F.,
 ( 4, 2, 2, 2, 4 ),
 ( 0.0007817246256747453293, 0.0009771112852218889842, 0.001172497944769032531, 0.001367884604316176294, 0.001563271263863319840 ),
 .UNSPECIFIED. ) ;
#32765=CARTESIAN_POINT ( 'NONE',  ( 8.769230769230768274, -3.322132147404559976, 32.92929555188717927 ) ) ;
#32767=ORIENTED_EDGE ( 'NONE', *, *, #73558, .F. ) ;
#32768=ADVANCED_FACE ( 'NONE', ( #18734 ), #72327, .F. ) ;
#32769=ORIENTED_EDGE ( 'NONE', *, *, #80843, .F. ) ;
#32770=CARTESIAN_POINT ( 'NONE',  ( -16.15384615384615330, -3.322132147404559976, 32.92929555188717927 ) ) ;
#32771=CARTESIAN_POINT ( 'NONE',  ( 14.30769230769218758, -4.481592998941358097, 33.73612834414048933 ) ) ;
#32772=EDGE_CURVE ( 'NONE', #80449, #33353, #25035, .T. ) ;
#32773=CARTESIAN_POINT ( 'NONE',  ( -18.00000000000000000, -6.343179335718452272, 34.87096338111211935 ) ) ;
#32774=AXIS2_PLACEMENT_3D ( 'NONE', #40061, #74276, #12576 ) ;
#32775=CARTESIAN_POINT ( 'NONE',  ( 15.93036121012220541, -5.113361153441931428, 34.14387501736621999 ) ) ;
#32776=ORIENTED_EDGE ( 'NONE', *, *, #49260, .F. ) ;
#32777=ADVANCED_FACE ( 'NONE', ( #17844 ), #45295, .F. ) ;
#32778=ORIENTED_EDGE ( 'NONE', *, *, #18388, .T. ) ;
#32779=VECTOR ( 'NONE', #7845, 1000.000000000000000 ) ;
#32781=CARTESIAN_POINT ( 'NONE',  ( -2.980769230769226841, -2.499999999999999556, 29.81604066197450109 ) ) ;
#32782=VERTEX_POINT ( 'NONE', #11979 ) ;
#32784=EDGE_CURVE ( 'NONE', #6435, #12084, #52937, .T. ) ;
#32785=CARTESIAN_POINT ( 'NONE',  ( -6.923076923077045919, -12.51329471203414379, 31.30864560766407578 ) ) ;
#32786=B_SPLINE_CURVE_WITH_KNOTS ( 'NONE', 3,
 ( #17245, #85715, #46053, #25787, #18590, #59564, #67664, #5069, #31655, #38861 ),
 .UNSPECIFIED., .F., .F.,
 ( 4, 2, 2, 2, 4 ),
 ( 0.0007817359430256293554, 0.0009771253907249974075, 0.001172514838424365460, 0.001367904286123733512, 0.001563293733823094625 ),
 .UNSPECIFIED. ) ;
#32787=EDGE_CURVE ( 'NONE', #19289, #23594, #23781, .T. ) ;
#32788=B_SPLINE_CURVE_WITH_KNOTS ( 'NONE', 3,
 ( #18762, #80012, #3454, #59739, #24620, #3893, #51621, #66945, #72800, #32704 ),
 .UNSPECIFIED., .F., .F.,
 ( 4, 2, 2, 2, 4 ),
 ( 0.000000000000000000, 0.0001954311564186870913, 0.0003908623128373741825, 0.0005862934692560613009, 0.0007817246256747483650 ),
 .UNSPECIFIED. ) ;
#32789=CARTESIAN_POINT ( 'NONE',  ( 7.053867364043873600, -4.684288915650984819, 34.18129842949671371 ) ) ;
#32790=LINE ( 'NONE', #88648, #78396 ) ;
#32791=VERTEX_POINT ( 'NONE', #32676 ) ;
#32792=B_SPLINE_CURVE_WITH_KNOTS ( 'NONE', 3,
 ( #83477, #64065, #605, #1048, #42044, #29852, #49674, #77150, #43363, #70845 ),
 .UNSPECIFIED., .F., .F.,
 ( 4, 2, 2, 2, 4 ),
 ( 0.0007817359430256390048, 0.0009771253907250075990, 0.001172514838424376085, 0.001367904286123744571, 0.001563293733823113056 ),
 .UNSPECIFIED. ) ;
#32793=ORIENTED_EDGE ( 'NONE', *, *, #70440, .F. ) ;
#32794=EDGE_CURVE ( 'NONE', #63168, #42657, #65116, .T. ) ;
#32795=ORIENTED_EDGE ( 'NONE', *, *, #59685, .T. ) ;
#32796=CARTESIAN_POINT ( 'NONE',  ( 14.55774672760575861, -10.82426656108012075, 33.81400080652039009 ) ) ;
#32797=CARTESIAN_POINT ( 'NONE',  ( -13.13461538461538325, -2.249999999999998668, 29.75000000000000355 ) ) ;
#32799=CARTESIAN_POINT ( 'NONE',  ( 18.13079044096694759, -11.93129842949672437, 32.56571108434900452 ) ) ;
#32800=B_SPLINE_CURVE_WITH_KNOTS ( 'NONE', 3,
 ( #69611, #6588, #27299, #34934, #54763, #76824, #7917, #41263, #62396, #41701 ),
 .UNSPECIFIED., .F., .F.,
 ( 4, 2, 2, 2, 4 ),
 ( 0.0007817359527651104954, 0.0009771254036996493593, 0.001172514854634188223, 0.001367904305568727087, 0.001563293756503265951 ),
 .UNSPECIFIED. ) ;
#32802=CARTESIAN_POINT ( 'NONE',  ( 12.21151522424549718, -11.37209801155882793, 32.91403422569033665 ) ) ;
#32803=DIRECTION ( 'NONE',  ( 0.000000000000000000, 0.3420201433256641055, -0.9396926207859100932 ) ) ;
#32804=CARTESIAN_POINT ( 'NONE',  ( -13.44986637477662761, -2.506253911140460922, 30.00000000000013856 ) ) ;
#32805=CARTESIAN_POINT ( 'NONE',  ( 8.834486340506792601, -6.026961402152789304, 34.52809138561124769 ) ) ;
#32806=VECTOR ( 'NONE', #36584, 1000.000000000000114 ) ;
#32807=FACE_BOUND ( 'NONE', #19947, .T. ) ;
#32808=CARTESIAN_POINT ( 'NONE',  ( -8.546217925137375104, -2.308499170217967134, 30.53291367094873721 ) ) ;
#32809=DIRECTION ( 'NONE',  ( 0.000000000000000000, 0.000000000000000000, 1.000000000000000000 ) ) ;
#32810=DIRECTION ( 'NONE',  ( -0.000000000000000000, -0.6427876096865404731, -0.7660444431189770143 ) ) ;
#32811=FACE_OUTER_BOUND ( 'NONE', #51345, .T. ) ;
#32812=CARTESIAN_POINT ( 'NONE',  ( -5.076923076923075762, -3.050289026998446396, 32.03036669348365706 ) ) ;
#32813=CARTESIAN_POINT ( 'NONE',  ( -5.076923076923197442, -10.90142922262034020, 33.41473453929536674 ) ) ;
#32814=CARTESIAN_POINT ( 'NONE',  ( -4.088591014333314178, -11.67786785259547777, 32.92929555188713664 ) ) ;
#32815=ORIENTED_EDGE ( 'NONE', *, *, #23600, .F. ) ;
#32816=AXIS2_PLACEMENT_3D ( 'NONE', #22902, #86409, #16584 ) ;
#32817=CARTESIAN_POINT ( 'NONE',  ( -6.923076923076922462, -13.37000171582298513, 34.34916445242398453 ) ) ;
#32818=CARTESIAN_POINT ( 'NONE',  ( -13.51476335434707821, -9.504002272028875709, 34.60269587691767867 ) ) ;
#32820=EDGE_CURVE ( 'NONE', #67660, #28595, #56026, .T. ) ;
#32821=VERTEX_POINT ( 'NONE', #85853 ) ;
#32822=FACE_OUTER_BOUND ( 'NONE', #19552, .T. ) ;
#32823=CARTESIAN_POINT ( 'NONE',  ( 16.15384615384615330, -2.292212530054420494, 30.41441678777542634 ) ) ;
#32825=VERTEX_POINT ( 'NONE', #30891 ) ;
#32827=CARTESIAN_POINT ( 'NONE',  ( -6.989160334032804123, -9.780366693483667717, 34.19971097300155805 ) ) ;
#32828=CARTESIAN_POINT ( 'NONE',  ( -15.48074596171158213, -5.728515186090277211, 34.42611988154120439 ) ) ;
#32829=DIRECTION ( 'NONE',  ( -0.000000000000000000, -0.000000000000000000, -1.000000000000000000 ) ) ;
#32830=CARTESIAN_POINT ( 'NONE',  ( -13.60810030917971858, -2.353723527008296568, 30.78948104536958752 ) ) ;
#32831=CARTESIAN_POINT ( 'NONE',  ( -5.326946314216043810, -9.271318131107980420, 34.42618302367067429 ) ) ;
#32832=B_SPLINE_CURVE_WITH_KNOTS ( 'NONE', 3,
 ( #71970, #18368, #31886, #65205, #86852, #30974, #78731, #58439, #18812, #79623 ),
 .UNSPECIFIED., .F., .F.,
 ( 4, 2, 2, 2, 4 ),
 ( 0.0007817246256747464135, 0.0009771112852218900684, 0.001172497944769033615, 0.001367884604316177161, 0.001563271263863320925 ),
 .UNSPECIFIED. ) ;
#32833=FACE_OUTER_BOUND ( 'NONE', #8639, .T. ) ;
#32835=ORIENTED_EDGE ( 'NONE', *, *, #32880, .T. ) ;
#32836=ORIENTED_EDGE ( 'NONE', *, *, #18608, .T. ) ;
#32838=VECTOR ( 'NONE', #53869, 1000.000000000000114 ) ;
#32840=CARTESIAN_POINT ( 'NONE',  ( 6.000000000000001776, -13.53365097954675988, 30.81389545987213552 ) ) ;
#32842=CARTESIAN_POINT ( 'NONE',  ( 6.792385456409363087, -12.11776431015576172, 31.66791131148498906 ) ) ;
#32843=CARTESIAN_POINT ( 'NONE',  ( -3.230769230769351186, -6.026961402154118908, 34.52809138561165270 ) ) ;
#32845=CARTESIAN_POINT ( 'NONE',  ( -7.596208327805704208, -8.433404298154334455, 34.66254593164985920 ) ) ;
#32846=CARTESIAN_POINT ( 'NONE',  ( -13.45069879557126136, -8.120952969808774569, 34.71129190930000163 ) ) ;
#32847=CARTESIAN_POINT ( 'NONE',  ( -13.16165248105389907, -7.369474270740069777, 34.74850911626239736 ) ) ;
#32848=CARTESIAN_POINT ( 'NONE',  ( 12.39545608217832218, -11.35647404775217595, 33.31231777344666511 ) ) ;
#32850=DIRECTION ( 'NONE',  ( 0.000000000000000000, 0.3420201433256610524, 0.9396926207859113145 ) ) ;
#32851=LINE ( 'NONE', #61643, #61036 ) ;
#32852=CARTESIAN_POINT ( 'NONE',  ( 4.153846153846032507, -12.46129190930018460, 30.37095296980731973 ) ) ;
#32853=CARTESIAN_POINT ( 'NONE',  ( 12.46153846153846168, -1.790695186598648903, 34.54067556320373455 ) ) ;
#32855=CARTESIAN_POINT ( 'NONE',  ( -15.45425417449318317, -10.11188796281391511, 34.01382737946119050 ) ) ;
#32856=VERTEX_POINT ( 'NONE', #58812 ) ;
#32857=DIRECTION ( 'NONE',  ( -0.000000000000000000, -0.7660444431189791237, -0.6427876096865379196 ) ) ;
#32858=CARTESIAN_POINT ( 'NONE',  ( -17.07692307692319744, -6.835583212225970762, 34.95778746994575670 ) ) ;
#32859=DIRECTION ( 'NONE',  ( -0.000000000000000000, -0.9396926207859092051, -0.3420201433256662704 ) ) ;
#32861=ADVANCED_FACE ( 'NONE', ( #58358 ), #24137, .F. ) ;
#32862=B_SPLINE_CURVE_WITH_KNOTS ( 'NONE', 3,
 ( #77580, #49660, #78018, #8689, #23078, #64480, #15888, #16320, #2783, #30279 ),
 .UNSPECIFIED., .F., .F.,
 ( 4, 2, 2, 2, 4 ),
 ( 0.000000000000000000, 0.0001954339857564083688, 0.0003908679715128167377, 0.0005863019572692250523, 0.0007817359430256334753 ),
 .UNSPECIFIED. ) ;
#32863=CARTESIAN_POINT ( 'NONE',  ( 5.326977496836529546, -10.06805714834173848, 34.32951233291982618 ) ) ;
#32865=FACE_OUTER_BOUND ( 'NONE', #42195, .T. ) ;
#32866=CARTESIAN_POINT ( 'NONE',  ( 6.000000000000001776, -3.886160181151819604, 36.00935417666054406 ) ) ;
#32867=VERTEX_POINT ( 'NONE', #24588 ) ;
#32869=CARTESIAN_POINT ( 'NONE',  ( -14.43784027742400333, -5.915902021225889484, 34.75552854090298638 ) ) ;
#32870=EDGE_CURVE ( 'NONE', #33781, #87066, #43096, .T. ) ;
#32872=CARTESIAN_POINT ( 'NONE',  ( -17.74994568836168085, -3.627508038966687831, 32.91356715214246265 ) ) ;
#32873=ADVANCED_FACE ( 'NONE', ( #87204 ), #46199, .F. ) ;
#32874=EDGE_LOOP ( 'NONE', ( #58531, #556 ) ) ;
#32875=DIRECTION ( 'NONE',  ( -0.000000000000000000, -0.1736481776669307198, -0.9848077530122080203 ) ) ;
#32876=CARTESIAN_POINT ( 'NONE',  ( -9.442253380669376028, -2.779044189368095275, 31.39831045268885745 ) ) ;
#32877=FACE_OUTER_BOUND ( 'NONE', #70144, .T. ) ;
#32878=ORIENTED_EDGE ( 'NONE', *, *, #50008, .T. ) ;
#32879=ORIENTED_EDGE ( 'NONE', *, *, #47564, .T. ) ;
#32880=EDGE_CURVE ( 'NONE', #75011, #16582, #3384, .T. ) ;
#32881=AXIS2_PLACEMENT_3D ( 'NONE', #10670, #72802, #57962 ) ;
#32882=VERTEX_POINT ( 'NONE', #75010 ) ;
#32883=CARTESIAN_POINT ( 'NONE',  ( 0.4615384615384611200, -1.629998284177014645, 34.34916445242399163 ) ) ;
#32884=CARTESIAN_POINT ( 'NONE',  ( 12.33084699487090319, -12.38065189839062263, 30.83690757178629482 ) ) ;
#32885=CARTESIAN_POINT ( 'NONE',  ( 18.24994540937804643, -10.18230066228895758, 34.26354781536631577 ) ) ;
#32886=CARTESIAN_POINT ( 'NONE',  ( -1.449885385171704177, -11.67786785259541027, 32.92929555188721480 ) ) ;
#32887=FACE_OUTER_BOUND ( 'NONE', #48949, .T. ) ;
#32888=CARTESIAN_POINT ( 'NONE',  ( 1.384615384615265343, -10.90142922262034020, 33.41473453929536674 ) ) ;
#32890=CARTESIAN_POINT ( 'NONE',  ( 10.48523740594639087, -12.27039167877662251, 31.24851455888617835 ) ) ;
#32894=CARTESIAN_POINT ( 'NONE',  ( -4.153846153846152411, -8.164416787775445883, 34.95778746994557906 ) ) ;
#32895=EDGE_LOOP ( 'NONE', ( #48509, #42771, #31172, #23570 ) ) ;
#32896=ADVANCED_FACE ( 'NONE', ( #27693 ), #7436, .F. ) ;
#32897=AXIS2_PLACEMENT_3D ( 'NONE', #50873, #71161, #9468 ) ;
#32898=DIRECTION ( 'NONE',  ( -0.000000000000000000, 0.9848077530122085754, -0.1736481776669273613 ) ) ;
#32899=CARTESIAN_POINT ( 'NONE',  ( 12.71148397988660150, -3.202959910592335646, 32.30730279482227019 ) ) ;
#32900=ORIENTED_EDGE ( 'NONE', *, *, #54747, .F. ) ;
#32901=CARTESIAN_POINT ( 'NONE',  ( 17.07692307692307665, -13.04860791097971706, 34.73218667398347037 ) ) ;
#32902=VECTOR ( 'NONE', #7531, 1000.000000000000227 ) ;
#32903=EDGE_CURVE ( 'NONE', #51992, #5606, #38799, .T. ) ;
#32904=VERTEX_POINT ( 'NONE', #67359 ) ;
#32905=DIRECTION ( 'NONE',  ( -0.000000000000000000, 0.7660444431189791237, -0.6427876096865379196 ) ) ;
#32906=VERTEX_POINT ( 'NONE', #47961 ) ;
#32909=ADVANCED_FACE ( 'NONE', ( #60144 ), #12852, .F. ) ;
#32912=CARTESIAN_POINT ( 'NONE',  ( -16.21992956480203318, -6.386643153685125363, 34.62446782046654903 ) ) ;
#32913=CARTESIAN_POINT ( 'NONE',  ( -11.31568186948347154, -12.11081565061824250, 32.26097654155340422 ) ) ;
#32914=FACE_BOUND ( 'NONE', #46144, .T. ) ;
#32915=DIRECTION ( 'NONE',  ( -0.000000000000000000, 0.3420201433256694901, -0.9396926207859082059 ) ) ;
#32916=DIRECTION ( 'NONE',  ( -0.000000000000000000, 0.1736481776669307198, -0.9848077530122080203 ) ) ;
#32917=CARTESIAN_POINT ( 'NONE',  ( 13.45068271796546178, -4.661471528628508665, 34.16647553114624003 ) ) ;
#32918=CARTESIAN_POINT ( 'NONE',  ( 3.296024370282069516, -5.094484230520773593, 34.41647553114626845 ) ) ;
#32919=LINE ( 'NONE', #88772, #3534 ) ;
#32920=CARTESIAN_POINT ( 'NONE',  ( -4.376772371362299019, -11.24512374952581872, 33.06303171183252942 ) ) ;
#32922=CARTESIAN_POINT ( 'NONE',  ( -6.988347369037697376, -6.879047030191174805, 34.71129190930000163 ) ) ;
#32924=EDGE_CURVE ( 'NONE', #22118, #67341, #74117, .T. ) ;
#32926=B_SPLINE_CURVE_WITH_KNOTS ( 'NONE', 3,
 ( #26918, #54379, #47630, #75113, #13395, #40880, #61577, #89084, #27356, #82312 ),
 .UNSPECIFIED., .F., .F.,
 ( 4, 2, 2, 2, 4 ),
 ( 0.000000000000000000, 0.0001954311564186862510, 0.0003908623128373725020, 0.0005862934692560588072, 0.0007817246256747450040 ),
 .UNSPECIFIED. ) ;
#32929=CARTESIAN_POINT ( 'NONE',  ( -6.923076923077045919, -11.67786785259630911, 32.92929555188603530 ) ) ;
#32930=CARTESIAN_POINT ( 'NONE',  ( -14.30769230769230660, -2.292212530054420494, 30.41441678777542634 ) ) ;
#32931=B_SPLINE_CURVE_WITH_KNOTS ( 'NONE', 3,
 ( #87188, #25466, #80420, #19155, #18721, #46623, #12396, #39880, #19592, #47054 ),
 .UNSPECIFIED., .F., .F.,
 ( 4, 2, 2, 2, 4 ),
 ( 0.0007817246256747474977, 0.0009771112852218911526, 0.001172497944769034699, 0.001367884604316178462, 0.001563271263863322009 ),
 .UNSPECIFIED. ) ;
#32932=EDGE_CURVE ( 'NONE', #40761, #69679, #72123, .T. ) ;
#32933=CARTESIAN_POINT ( 'NONE',  ( 1.384615384615264011, -11.06231777344772027, 33.60647404775119895 ) ) ;
#32934=CARTESIAN_POINT ( 'NONE',  ( -13.16160403300253812, -2.758310577978207778, 31.33698337089302299 ) ) ;
#32935=EDGE_CURVE ( 'NONE', #61593, #44583, #78508, .T. ) ;
#32936=ORIENTED_EDGE ( 'NONE', *, *, #7468, .F. ) ;
#32937=CARTESIAN_POINT ( 'NONE',  ( -5.999999999999998224, -8.164416787775445883, 34.95778746994557906 ) ) ;
#32939=CARTESIAN_POINT ( 'NONE',  ( 10.36540788444226102, -3.137211980971221781, 32.19342716148376837 ) ) ;
#32940=CARTESIAN_POINT ( 'NONE',  ( -14.30769230769230660, -1.422936976036506707, 30.56769352161908415 ) ) ;
#32941=VERTEX_POINT ( 'NONE', #81326 ) ;
#32942=ADVANCED_FACE ( 'NONE', ( #21381 ), #28592, .F. ) ;
#32943=ORIENTED_EDGE ( 'NONE', *, *, #44423, .F. ) ;
#32945=ORIENTED_EDGE ( 'NONE', *, *, #66768, .T. ) ;
#32946=CARTESIAN_POINT ( 'NONE',  ( 0.5276068125408981402, -10.51840700105979565, 33.73612834413962247 ) ) ;
#32948=ORIENTED_EDGE ( 'NONE', *, *, #53979, .F. ) ;
#32950=CARTESIAN_POINT ( 'NONE',  ( 6.923076923076924238, -2.249999999999998668, 29.75000000000001776 ) ) ;
#32951=CARTESIAN_POINT ( 'NONE',  ( 3.296024370282069516, -10.33852847137154107, 34.16647553114620450 ) ) ;
#32952=CARTESIAN_POINT ( 'NONE',  ( -2.557715544985270650, -8.432397168068783699, 34.66272746175022945 ) ) ;
#32953=LINE ( 'NONE', #52766, #1430 ) ;
#32955=FACE_OUTER_BOUND ( 'NONE', #51123, .T. ) ;
#32956=ORIENTED_EDGE ( 'NONE', *, *, #39798, .F. ) ;
#32958=CARTESIAN_POINT ( 'NONE',  ( 11.78846153846154010, -7.500000000000001776, 35.04278698407183867 ) ) ;
#32959=DIRECTION ( 'NONE',  ( -1.000000000000000000, 0.000000000000000000, 0.000000000000000000 ) ) ;
#32960=CARTESIAN_POINT ( 'NONE',  ( -3.903791842207838148, -12.41262288849542017, 30.68299917996395010 ) ) ;
#32961=CARTESIAN_POINT ( 'NONE',  ( -3.903791733932700847, -4.818054556918156095, 34.26375889529406749 ) ) ;
#32962=CARTESIAN_POINT ( 'NONE',  ( -8.638705330997126453, -9.503571793651731880, 34.60286762892837942 ) ) ;
#32963=DIRECTION ( 'NONE',  ( -0.000000000000000000, -0.7660444431189791237, -0.6427876096865379196 ) ) ;
#32965=VERTEX_POINT ( 'NONE', #28135 ) ;
#32966=CARTESIAN_POINT ( 'NONE',  ( -7.146003881983769013, -10.77366814457252175, 33.85459836347579454 ) ) ;
#32968=ADVANCED_FACE ( 'NONE', ( #70008 ), #42114, .F. ) ;
#32969=B_SPLINE_CURVE_WITH_KNOTS ( 'NONE', 3,
 ( #1967, #64530, #31199, #9181, #58671, #16366, #58227, #56898, #79402, #30323 ),
 .UNSPECIFIED., .F., .F.,
 ( 4, 2, 2, 2, 4 ),
 ( 0.000000000000000000, 0.0001954311564186867389, 0.0003908623128373734778, 0.0005862934692560602167, 0.0007817246256747469556 ),
 .UNSPECIFIED. ) ;
#32970=B_SPLINE_CURVE_WITH_KNOTS ( 'NONE', 3,
 ( #26849, #82241, #27288, #54755, #54306, #60178, #53420, #53874, #80922, #46232 ),
 .UNSPECIFIED., .F., .F.,
 ( 4, 2, 2, 2, 4 ),
 ( 0.000000000000000000, 0.0001954311564186862239, 0.0003908623128373724478, 0.0005862934692560586988, 0.0007817246256747448956 ),
 .UNSPECIFIED. ) ;
#32971=VECTOR ( 'NONE', #75752, 1000.000000000000227 ) ;
#32972=VERTEX_POINT ( 'NONE', #1113 ) ;
#32973=B_SPLINE_CURVE_WITH_KNOTS ( 'NONE', 3,
 ( #65509, #85347, #31289, #23632, #78577, #58756, #70496, #8803, #16879, #63730 ),
 .UNSPECIFIED., .F., .F.,
 ( 4, 2, 2, 2, 4 ),
 ( 0.0007817359430256258859, 0.0009771253907249909023, 0.001172514838424355919, 0.001367904286123720935, 0.001563293733823085951 ),
 .UNSPECIFIED. ) ;
#32974=ORIENTED_EDGE ( 'NONE', *, *, #17901, .T. ) ;
#32975=CARTESIAN_POINT ( 'NONE',  ( 2.241938879378976068, -7.249945578846654470, 34.99404164642496795 ) ) ;
#32976=CARTESIAN_POINT ( 'NONE',  ( -12.46153846153858247, -3.300289026999228881, 32.46337939537708905 ) ) ;
#32977=CARTESIAN_POINT ( 'NONE',  ( -9.019253993452228002, -10.92453946501458795, 33.72985991061850086 ) ) ;
#32978=CARTESIAN_POINT ( 'NONE',  ( 6.988332494352946789, -6.026961402152789304, 34.52809138561124769 ) ) ;
#32980=DIRECTION ( 'NONE',  ( -0.000000000000000000, -0.6427876096865404731, -0.7660444431189771253 ) ) ;
#32981=VERTEX_POINT ( 'NONE', #14629 ) ;
#32982=B_SPLINE_CURVE_WITH_KNOTS ( 'NONE', 3,
 ( #35635, #55016, #75289, #27094, #82051, #20349, #47809, #68519, #6818, #70 ),
 .UNSPECIFIED., .F., .F.,
 ( 4, 2, 2, 2, 4 ),
 ( 0.0007817246256747451124, 0.0009771112852218885505, 0.001172497944769032097, 0.001367884604316175427, 0.001563271263863318973 ),
 .UNSPECIFIED. ) ;
#32983=CARTESIAN_POINT ( 'NONE',  ( -3.230769230769229949, -12.62096338111211580, 30.90682066428153263 ) ) ;
#32984=CARTESIAN_POINT ( 'NONE',  ( 15.23076923076923173, -3.886160181151819604, 36.00935417666054406 ) ) ;
#32985=CARTESIAN_POINT ( 'NONE',  ( 9.626225312947559232, -2.486705287966279432, 31.30864560766542937 ) ) ;
#32987=CARTESIAN_POINT ( 'NONE',  ( 13.44987095589141468, -6.879047030191282275, 34.71129190930002295 ) ) ;
#32988=ORIENTED_EDGE ( 'NONE', *, *, #46940, .F. ) ;
#32989=CARTESIAN_POINT ( 'NONE',  ( -5.076923076923199218, -3.083524468854526912, 32.58852847137268327 ) ) ;
#32992=ORIENTED_EDGE ( 'NONE', *, *, #83040, .F. ) ;
#32993=CARTESIAN_POINT ( 'NONE',  ( -13.13456096470193302, -4.818054556918156983, 34.26375889529406749 ) ) ;
#32994=FACE_OUTER_BOUND ( 'NONE', #50248, .T. ) ;
#32996=EDGE_CURVE ( 'NONE', #28226, #43633, #88290, .T. ) ;
#32997=DIRECTION ( 'NONE',  ( -0.000000000000000000, -0.7660444431189791237, -0.6427876096865379196 ) ) ;
#32999=B_SPLINE_CURVE_WITH_KNOTS ( 'NONE', 3,
 ( #46521, #12733, #88414, #74000, #12289, #67242, #33006, #46946, #74434, #40216 ),
 .UNSPECIFIED., .F., .F.,
 ( 4, 2, 2, 2, 4 ),
 ( 0.0007817359430256294638, 0.0009771253907249952391, 0.001172514838424361123, 0.001367904286123726790, 0.001563293733823092673 ),
 .UNSPECIFIED. ) ;
#33000=EDGE_LOOP ( 'NONE', ( #31144, #78043, #8875, #36868 ) ) ;
#33001=CARTESIAN_POINT ( 'NONE',  ( -1.384615384615383471, -12.10708131394839349, 31.69288490824020244 ) ) ;
#33002=ORIENTED_EDGE ( 'NONE', *, *, #31530, .F. ) ;
#33003=CARTESIAN_POINT ( 'NONE',  ( 5.142178216435913107, -11.67786785259547777, 32.92929555188713664 ) ) ;
#33004=VECTOR ( 'NONE', #81030, 1000.000000000000227 ) ;
#33005=LINE ( 'NONE', #87082, #9110 ) ;
#33006=CARTESIAN_POINT ( 'NONE',  ( 6.223011351612851350, -9.086983370893049639, 34.49168942202179267 ) ) ;
#33007=EDGE_CURVE ( 'NONE', #6141, #60344, #56054, .T. ) ;
#33008=CARTESIAN_POINT ( 'NONE',  ( -14.08491276642389245, -12.24180327182772388, 31.33663988360758168 ) ) ;
#33009=CARTESIAN_POINT ( 'NONE',  ( 12.46153846153846168, -12.78798330534102945, 29.74999999999997868 ) ) ;
#33011=VERTEX_POINT ( 'NONE', #22272 ) ;
#33012=ORIENTED_EDGE ( 'NONE', *, *, #57218, .F. ) ;
#33013=VERTEX_POINT ( 'NONE', #35796 ) ;
#33016=CARTESIAN_POINT ( 'NONE',  ( -5.207071046654771607, -4.299443229763728169, 33.91186481527756058 ) ) ;
#33017=CARTESIAN_POINT ( 'NONE',  ( -6.065270445960774914, -12.46129190929999986, 30.37095296980880832 ) ) ;
#33018=CARTESIAN_POINT ( 'NONE',  ( -4.023320452082588261, -9.417988943895561960, 34.36773134775778260 ) ) ;
#33019=DIRECTION ( 'NONE',  ( 0.000000000000000000, 0.3420201433256610524, 0.9396926207859113145 ) ) ;
#33020=CARTESIAN_POINT ( 'NONE',  ( 3.903846153846143530, -2.499999999999999556, 29.81609845454692120 ) ) ;
#33022=VECTOR ( 'NONE', #50615, 1000.000000000000000 ) ;
#33023=DIRECTION ( 'NONE',  ( 0.000000000000000000, 1.000000000000000000, 0.000000000000000000 ) ) ;
#33024=CARTESIAN_POINT ( 'NONE',  ( -2.307692307692305711, -3.513871655860378418, 32.76840700105978499 ) ) ;
#33027=ORIENTED_EDGE ( 'NONE', *, *, #40606, .T. ) ;
#33028=AXIS2_PLACEMENT_3D ( 'NONE', #53993, #46797, #88257 ) ;
#33029=EDGE_LOOP ( 'NONE', ( #68092, #77826, #48275, #65016 ) ) ;
#33030=VECTOR ( 'NONE', #61367, 1000.000000000000000 ) ;
#33031=CARTESIAN_POINT ( 'NONE',  ( 2.057669070399344324, -2.587272538249755449, 30.68239716806877837 ) ) ;
#33032=ORIENTED_EDGE ( 'NONE', *, *, #32392, .F. ) ;
#33033=CARTESIAN_POINT ( 'NONE',  ( 6.673100179028334189, -11.47974371597207899, 33.17467449705390692 ) ) ;
#33034=CARTESIAN_POINT ( 'NONE',  ( -7.596208436775802930, -9.357781135181033605, 34.66075350412533851 ) ) ;
#33035=DIRECTION ( 'NONE',  ( -0.000000000000000000, -0.3420201433256694346, -0.9396926207859080948 ) ) ;
#33036=DIRECTION ( 'NONE',  ( 0.000000000000000000, 0.7660444431189807890, 0.6427876096865361433 ) ) ;
#33038=FACE_BOUND ( 'NONE', #33130, .T. ) ;
#33039=ORIENTED_EDGE ( 'NONE', *, *, #87169, .T. ) ;
#33041=CARTESIAN_POINT ( 'NONE',  ( 2.307692307692309264, -9.819645486525091727, 36.12317359536749706 ) ) ;
#33042=ORIENTED_EDGE ( 'NONE', *, *, #48830, .F. ) ;
#33043=FACE_BOUND ( 'NONE', #36675, .T. ) ;
#33044=DIRECTION ( 'NONE',  ( -0.000000000000000000, -0.1736481776669307198, -0.9848077530122080203 ) ) ;
#33045=CARTESIAN_POINT ( 'NONE',  ( 8.096153846153846700, -2.249999999999998668, 29.75000000000000355 ) ) ;
#33046=ORIENTED_EDGE ( 'NONE', *, *, #87847, .F. ) ;
#33047=CARTESIAN_POINT ( 'NONE',  ( -8.096153846153844924, -2.249999999999998668, 29.75000000000000355 ) ) ;
#33049=CARTESIAN_POINT ( 'NONE',  ( 3.100621261037538545, -12.15440758774515473, 32.17923288041532004 ) ) ;
#33050=ORIENTED_EDGE ( 'NONE', *, *, #68209, .T. ) ;
#33051=CARTESIAN_POINT ( 'NONE',  ( 6.000000000000001776, -1.466349020453238561, 30.81389545987213907 ) ) ;
#33052=CARTESIAN_POINT ( 'NONE',  ( 12.68431800280686694, -6.760870238392817200, 34.69528174975672385 ) ) ;
#33053=CARTESIAN_POINT ( 'NONE',  ( -8.069080063669991532, -2.758268499246657068, 31.33685645148948140 ) ) ;
#33054=ORIENTED_EDGE ( 'NONE', *, *, #30161, .F. ) ;
#33055=DIRECTION ( 'NONE',  ( 0.000000000000000000, 0.7660444431189822323, -0.6427876096865344779 ) ) ;
#33056=CARTESIAN_POINT ( 'NONE',  ( 4.023155550735844521, -9.929715669179216775, 34.40415004197138416 ) ) ;
#33057=ORIENTED_EDGE ( 'NONE', *, *, #2186, .F. ) ;
#33058=CARTESIAN_POINT ( 'NONE',  ( 3.453782074862625340, -6.460100341425561332, 34.89618726649961644 ) ) ;
#33059=DIRECTION ( 'NONE',  ( -1.000000000000000000, 0.000000000000000000, 0.000000000000000000 ) ) ;
#33060=CARTESIAN_POINT ( 'NONE',  ( -7.846153846153844924, -12.34228464037088635, 31.77849191805839268 ) ) ;
#33061=CARTESIAN_POINT ( 'NONE',  ( -5.076923076923075762, -8.120952969808772792, 34.71129190930000163 ) ) ;
#33062=CARTESIAN_POINT ( 'NONE',  ( -6.988830351390253881, -7.249945578846651806, 34.99404164642496795 ) ) ;
#33063=CARTESIAN_POINT ( 'NONE',  ( 17.32686848630112308, -4.932303261841487263, 34.32971442181322885 ) ) ;
#33064=B_SPLINE_CURVE_WITH_KNOTS ( 'NONE', 3,
 ( #21703, #15402, #50491, #23030, #50922, #42872, #78409, #77536, #84753, #14958 ),
 .UNSPECIFIED., .F., .F.,
 ( 4, 2, 2, 2, 4 ),
 ( 0.000000000000000000, 0.0001954311564186868473, 0.0003908623128373736946, 0.0005862934692560605419, 0.0007817246256747473893 ),
 .UNSPECIFIED. ) ;
#33065=CARTESIAN_POINT ( 'NONE',  ( 6.223011351612851350, -11.76359900205217457, 32.36225158514719880 ) ) ;
#33066=CARTESIAN_POINT ( 'NONE',  ( 5.076923076923075762, -4.098570777380720287, 33.41473453929634729 ) ) ;
#33070=VERTEX_POINT ( 'NONE', #36237 ) ;
#33071=CARTESIAN_POINT ( 'NONE',  ( -12.52680890749923570, -8.613356846314824011, 34.62446782046655613 ) ) ;
#33072=VERTEX_POINT ( 'NONE', #63692 ) ;
#33073=EDGE_LOOP ( 'NONE', ( #54427, #30048, #29046, #84611 ) ) ;
#33074=CARTESIAN_POINT ( 'NONE',  ( -17.07692307692319744, -4.320704448113951379, 33.92786785259630022 ) ) ;
#33075=ORIENTED_EDGE ( 'NONE', *, *, #2520, .T. ) ;
#33076=LINE ( 'NONE', #60544, #8125 ) ;
#33079=CARTESIAN_POINT ( 'NONE',  ( -8.769230769230768274, -3.050289026998446396, 32.03036669348365706 ) ) ;
#33080=CARTESIAN_POINT ( 'NONE',  ( -3.164700879766792152, -8.973038597847269315, 34.52809138561122637 ) ) ;
#33081=CARTESIAN_POINT ( 'NONE',  ( -5.326899820971668476, -3.436278759898155677, 33.07459398097509506 ) ) ;
#33082=DIRECTION ( 'NONE',  ( -0.000000000000000000, -0.9396926207859093161, -0.3420201433256663259 ) ) ;
#33083=CARTESIAN_POINT ( 'NONE',  ( 2.373760658694747061, -11.16473453929635440, 33.15142922261926373 ) ) ;
#33084=B_SPLINE_CURVE_WITH_KNOTS ( 'NONE', 3,
 ( #27522, #88363, #41480, #54992, #75700, #20759, #6800, #934, #81587, #7255 ),
 .UNSPECIFIED., .F., .F.,
 ( 4, 2, 2, 2, 4 ),
 ( 0.0007817359430256297891, 0.0009771253907249958896, 0.001172514838424362207, 0.001367904286123728524, 0.001563293733823094625 ),
 .UNSPECIFIED. ) ;
#33086=CARTESIAN_POINT ( 'NONE',  ( 17.29970274590113632, -2.353885683473779800, 30.79025554430704759 ) ) ;
#33087=CARTESIAN_POINT ( 'NONE',  ( -10.61538461538429878, -2.255955759149395501, 30.00000000000324363 ) ) ;
#33088=CIRCLE ( 'NONE', #30375, 0.2500000000000002220 ) ;
#33090=VECTOR ( 'NONE', #4810, 1000.000000000000227 ) ;
#33091=VECTOR ( 'NONE', #51049, 1000.000000000000227 ) ;
#33092=ORIENTED_EDGE ( 'NONE', *, *, #82743, .T. ) ;
#33095=CARTESIAN_POINT ( 'NONE',  ( 15.48082365068268373, -12.01375889529407281, 32.43194544308182969 ) ) ;
#33096=CARTESIAN_POINT ( 'NONE',  ( -6.673131513698880468, -12.07971442181322352, 32.31769673815850297 ) ) ;
#33097=CARTESIAN_POINT ( 'NONE',  ( 6.065192988294654697, -2.255955759149235629, 29.99999999999988631 ) ) ;
#33098=B_SPLINE_CURVE_WITH_KNOTS ( 'NONE', 3,
 ( #86432, #66589, #25146, #67034, #31915, #72439 ),
 .UNSPECIFIED., .F., .F.,
 ( 4, 2, 4 ),
 ( 3.165870343657672947E-17, 0.0001954756301637032231, 0.0003909512603273747875 ),
 .UNSPECIFIED. ) ;
#33099=VECTOR ( 'NONE', #22875, 1000.000000000000000 ) ;
#33101=VECTOR ( 'NONE', #32470, 1000.000000000000227 ) ;
#33102=CARTESIAN_POINT ( 'NONE',  ( -0.7115616988314269475, -6.695914987888143877, 34.68535235679833306 ) ) ;
#33103=B_SPLINE_CURVE_WITH_KNOTS ( 'NONE', 3,
 ( #71538, #35103, #49939, #29684, #22910, #50377, #77858, #35558, #83748, #878 ),
 .UNSPECIFIED., .F., .F.,
 ( 4, 2, 2, 2, 4 ),
 ( 0.0007817246256747491240, 0.0009771112852218931041, 0.001172497944769036867, 0.001367884604316180631, 0.001563271263863324611 ),
 .UNSPECIFIED. ) ;
#33104=VERTEX_POINT ( 'NONE', #1999 ) ;
#33105=CARTESIAN_POINT ( 'NONE',  ( 3.230769230769108269, -6.835583212225970762, 34.95778746994575670 ) ) ;
#33106=ORIENTED_EDGE ( 'NONE', *, *, #53239, .F. ) ;
#33107=VERTEX_POINT ( 'NONE', #29481 ) ;
#33108=CYLINDRICAL_SURFACE ( 'NONE', #86596, 0.2499999999999973355 ) ;
#33109=EDGE_CURVE ( 'NONE', #74160, #16329, #15964, .T. ) ;
#33110=CARTESIAN_POINT ( 'NONE',  ( -2.438382910802615378, -9.084618155246140248, 34.75535874321725771 ) ) ;
#33111=CARTESIAN_POINT ( 'NONE',  ( 14.30769230769231015, -4.786620604624113540, 33.94971097300155094 ) ) ;
#33112=EDGE_CURVE ( 'NONE', #41653, #28230, #61265, .T. ) ;
#33113=CARTESIAN_POINT ( 'NONE',  ( 1.384615384615386802, -2.249999999999998668, 29.75000000000001776 ) ) ;
#33114=LINE ( 'NONE', #34440, #13463 ) ;
#33115=EDGE_LOOP ( 'NONE', ( #385, #21814 ) ) ;
#33117=VERTEX_POINT ( 'NONE', #78097 ) ;
#33118=ORIENTED_EDGE ( 'NONE', *, *, #35016, .F. ) ;
#33119=EDGE_CURVE ( 'NONE', #35898, #60361, #16397, .T. ) ;
#33120=CARTESIAN_POINT ( 'NONE',  ( 5.776515056276055660, -2.599994579823202923, 30.74605699353653776 ) ) ;
#33121=CARTESIAN_POINT ( 'NONE',  ( 10.39189969082028675, -11.60425143139329940, 33.02411095842164457 ) ) ;
#33122=AXIS2_PLACEMENT_3D ( 'NONE', #66424, #78596, #38511 ) ;
#33123=CARTESIAN_POINT ( 'NONE',  ( 4.153846153846154188, -11.91647553114624181, 32.58852847137148245 ) ) ;
#33124=CARTESIAN_POINT ( 'NONE',  ( 5.076923076922953193, -8.656820664282941280, 34.87096338111179961 ) ) ;
#33126=CARTESIAN_POINT ( 'NONE',  ( -15.36091720050093734, -2.647304123082328875, 31.75400227202885972 ) ) ;
#33127=ORIENTED_EDGE ( 'NONE', *, *, #2083, .F. ) ;
#33128=ORIENTED_EDGE ( 'NONE', *, *, #64727, .T. ) ;
#33129=FACE_OUTER_BOUND ( 'NONE', #7647, .T. ) ;
#33130=EDGE_LOOP ( 'NONE', ( #81572, #87749 ) ) ;
#33131=CARTESIAN_POINT ( 'NONE',  ( 17.32697749683652688, -10.82426656108011720, 33.81400080652039009 ) ) ;
#33132=CARTESIAN_POINT ( 'NONE',  ( 7.053915341089685320, -7.277220443632450575, 34.74524770363009196 ) ) ;
#33134=EDGE_CURVE ( 'NONE', #61316, #35118, #15189, .T. ) ;
#33135=VERTEX_POINT ( 'NONE', #4666 ) ;
#33136=EDGE_CURVE ( 'NONE', #48109, #1161, #7707, .T. ) ;
#33137=CARTESIAN_POINT ( 'NONE',  ( 3.480769230769230838, -2.249999999999998668, 29.75000000000000355 ) ) ;
#33138=ORIENTED_EDGE ( 'NONE', *, *, #16147, .T. ) ;
#33139=DIRECTION ( 'NONE',  ( -0.000000000000000000, 0.6427876096865404731, -0.7660444431189770143 ) ) ;
#33140=DIRECTION ( 'NONE',  ( 0.000000000000000000, -6.938893903907222067E-15, 1.000000000000000000 ) ) ;
#33141=EDGE_CURVE ( 'NONE', #66010, #32904, #60334, .T. ) ;
#33142=CARTESIAN_POINT ( 'NONE',  ( -12.21159294319032185, -12.43552623307873972, 30.55307653245132826 ) ) ;
#33143=CARTESIAN_POINT ( 'NONE',  ( -6.700065571464072889, -12.39991518177334129, 30.74647679643404530 ) ) ;
#33145=EDGE_CURVE ( 'NONE', #52583, #65133, #83967, .T. ) ;
#33146=CARTESIAN_POINT ( 'NONE',  ( -1.134615384615383915, -2.249999999999998668, 29.75000000000000355 ) ) ;
#33147=ORIENTED_EDGE ( 'NONE', *, *, #11680, .F. ) ;
#33148=CARTESIAN_POINT ( 'NONE',  ( -11.31568186948346977, -8.540255544307065350, 34.89611431652622286 ) ) ;
#33149=CARTESIAN_POINT ( 'NONE',  ( -14.24243673641627694, -2.625532179533470512, 30.86335684631491105 ) ) ;
#33150=CARTESIAN_POINT ( 'NONE',  ( 6.923076923076924238, -11.35647404775217417, 33.31231777344666511 ) ) ;
#33151=VERTEX_POINT ( 'NONE', #17286 ) ;
#33152=AXIS2_PLACEMENT_3D ( 'NONE', #22066, #25, #76116 ) ;
#33155=CARTESIAN_POINT ( 'NONE',  ( -7.780085495151407571, -11.16473453929635440, 33.15142922261926373 ) ) ;
#33156=CARTESIAN_POINT ( 'NONE',  ( 4.219913487196230939, -11.35647404775217595, 33.31231777344667222 ) ) ;
#33157=DIRECTION ( 'NONE',  ( 0.000000000000000000, 0.7660444431189822323, -0.6427876096865344779 ) ) ;
#33158=CARTESIAN_POINT ( 'NONE',  ( 10.36536137809165403, -11.86270091957321249, 32.19358267280087915 ) ) ;
#33159=FACE_BOUND ( 'NONE', #26778, .T. ) ;
#33160=CARTESIAN_POINT ( 'NONE',  ( 5.999999999999878320, -5.094484230521993062, 34.41647553114689373 ) ) ;
#33161=CARTESIAN_POINT ( 'NONE',  ( 4.403791563224197070, -12.68172785388650681, 30.59649109432439573 ) ) ;
#33162=B_SPLINE_CURVE_WITH_KNOTS ( 'NONE', 3,
 ( #51981, #52876, #18671, #17776, #79916, #58298, #18220, #45681, #38942, #37584 ),
 .UNSPECIFIED., .F., .F.,
 ( 4, 2, 2, 2, 4 ),
 ( 0.000000000000000000, 0.0001954311564186876876, 0.0003908623128373753751, 0.0005862934692560630356, 0.0007817246256747507503 ),
 .UNSPECIFIED. ) ;
#33163=LINE ( 'NONE', #66046, #49713 ) ;
#33164=CARTESIAN_POINT ( 'NONE',  ( -6.000000000000119904, -10.21337939537710326, 33.94971097300076224 ) ) ;
#33165=CARTESIAN_POINT ( 'NONE',  ( -11.53846153846153655, -10.67929555188718282, 33.92786785259544047 ) ) ;
#33166=CARTESIAN_POINT ( 'NONE',  ( 13.38461538461538680, -2.486705287966279876, 31.30864560766543647 ) ) ;
#33168=B_SPLINE_CURVE_WITH_KNOTS ( 'NONE', 3,
 ( #43933, #65533, #2062, #36304, #85374, #2494, #65080, #3835, #29984, #57888 ),
 .UNSPECIFIED., .F., .F.,
 ( 4, 2, 2, 2, 4 ),
 ( 0.0007817359430256322827, 0.0009771253907249989254, 0.001172514838424365676, 0.001367904286123732428, 0.001563293733823099179 ),
 .UNSPECIFIED. ) ;
#33169=ORIENTED_EDGE ( 'NONE', *, *, #35893, .T. ) ;
#33170=CARTESIAN_POINT ( 'NONE',  ( -12.68436655917334654, -7.369209533119140509, 34.99857337881830688 ) ) ;
#33171=ORIENTED_EDGE ( 'NONE', *, *, #82173, .T. ) ;
#33173=ORIENTED_EDGE ( 'NONE', *, *, #76329, .T. ) ;
#33174=CARTESIAN_POINT ( 'NONE',  ( -15.48076923076922995, -7.500000000000001776, 34.75000000000000000 ) ) ;
#33175=CARTESIAN_POINT ( 'NONE',  ( -13.38461538461506883, -2.255955759149395501, 30.00000000000324363 ) ) ;
#33176=FACE_OUTER_BOUND ( 'NONE', #21114, .T. ) ;
#33177=VERTEX_POINT ( 'NONE', #17738 ) ;
#33178=CARTESIAN_POINT ( 'NONE',  ( -10.61538461538461320, -11.91647553114624181, 32.58852847137148245 ) ) ;
#33179=CARTESIAN_POINT ( 'NONE',  ( -12.71156168575991785, -6.652501968072648708, 34.93155406624980941 ) ) ;
#33182=CARTESIAN_POINT ( 'NONE',  ( 0.4615384615384611200, -5.180354513474913603, 36.12317359536750416 ) ) ;
#33183=CARTESIAN_POINT ( 'NONE',  ( -12.23875879256039489, -9.418065098278013636, 34.63729479722530158 ) ) ;
#33185=CYLINDRICAL_SURFACE ( 'NONE', #61190, 0.2499999999999973355 ) ;
#33186=FACE_OUTER_BOUND ( 'NONE', #59803, .T. ) ;
#33189=CARTESIAN_POINT ( 'NONE',  ( -4.376773112753001627, -2.889293201056495786, 32.26117774369186009 ) ) ;
#33190=CARTESIAN_POINT ( 'NONE',  ( 13.38461538461526601, -2.625532179533778709, 30.86335684631627174 ) ) ;
#33191=ORIENTED_EDGE ( 'NONE', *, *, #49384, .T. ) ;
#33192=FACE_OUTER_BOUND ( 'NONE', #24315, .T. ) ;
#33193=CARTESIAN_POINT ( 'NONE',  ( 15.23076923076910916, -11.06231777344772027, 33.60647404775119895 ) ) ;
#33195=B_SPLINE_CURVE_WITH_KNOTS ( 'NONE', 3,
 ( #87213, #4782, #32685, #87655, #86323, #44857, #17404, #24146, #18290, #11537 ),
 .UNSPECIFIED., .F., .F.,
 ( 4, 2, 2, 2, 4 ),
 ( 0.000000000000000000, 0.0001954339857564097241, 0.0003908679715128194482, 0.0005863019572692291723, 0.0007817359430256388964 ),
 .UNSPECIFIED. ) ;
#33196=CARTESIAN_POINT ( 'NONE',  ( -18.00000000000012079, -12.46129190930018460, 30.37095296980731973 ) ) ;
#33197=CARTESIAN_POINT ( 'NONE',  ( 17.14299142792552288, -11.69971097300155272, 32.46337939537588113 ) ) ;
#33199=DIRECTION ( 'NONE',  ( -0.000000000000000000, 0.9396926207859092051, -0.3420201433256662704 ) ) ;
#33200=CARTESIAN_POINT ( 'NONE',  ( -0.4615384615384611200, -1.129524287112498415, 32.06866353760679544 ) ) ;
#33201=CARTESIAN_POINT ( 'NONE',  ( -7.715363405186896451, -12.35292014791297710, 31.75344720912887198 ) ) ;
#33202=EDGE_LOOP ( 'NONE', ( #63518, #22597, #86263, #9857 ) ) ;
#33204=B_SPLINE_CURVE_WITH_KNOTS ( 'NONE', 3,
 ( #14075, #18737, #41110, #25927, #11983, #73232, #52940, #39461, #82100, #41548 ),
 .UNSPECIFIED., .F., .F.,
 ( 4, 2, 2, 2, 4 ),
 ( 0.000000000000000000, 0.0001954311564186865221, 0.0003908623128373730441, 0.0005862934692560595662, 0.0007817246256747460882 ),
 .UNSPECIFIED. ) ;
#33205=LINE ( 'NONE', #33650, #43506 ) ;
#33207=CARTESIAN_POINT ( 'NONE',  ( -11.60454391782167249, -2.486705287966279432, 31.30864560766542937 ) ) ;
#33208=B_SPLINE_CURVE_WITH_KNOTS ( 'NONE', 3,
 ( #38810, #80241, #66270, #4574, #32048, #87017, #23500, #50956, #25291, #73489 ),
 .UNSPECIFIED., .F., .F.,
 ( 4, 2, 2, 2, 4 ),
 ( 0.000000000000000000, 0.0001954339881912772715, 0.0003908679763825545429, 0.0005863019645738318415, 0.0007817359527651090859 ),
 .UNSPECIFIED. ) ;
#33209=ORIENTED_EDGE ( 'NONE', *, *, #75218, .F. ) ;
#33210=DIRECTION ( 'NONE',  ( -0.000000000000000000, -0.6427876096865404731, -0.7660444431189770143 ) ) ;
#33212=AXIS2_PLACEMENT_3D ( 'NONE', #74714, #20636, #18869 ) ;
#33213=CARTESIAN_POINT ( 'NONE',  ( 1.161688425708536920, -2.889293201056495786, 32.26117774369186009 ) ) ;
#33216=ORIENTED_EDGE ( 'NONE', *, *, #44242, .F. ) ;
#33217=ORIENTED_EDGE ( 'NONE', *, *, #55076, .T. ) ;
#33218=AXIS2_PLACEMENT_3D ( 'NONE', #54667, #1066, #28544 ) ;
#33219=VECTOR ( 'NONE', #20741, 1000.000000000000114 ) ;
#33220=EDGE_CURVE ( 'NONE', #53, #59603, #79440, .T. ) ;
#33221=DIRECTION ( 'NONE',  ( 0.000000000000000000, 0.9848077530122072432, -0.1736481776669354937 ) ) ;
#33222=CARTESIAN_POINT ( 'NONE',  ( -2.084912766423897779, -5.913360116392399668, 34.49180327182771322 ) ) ;
#33223=EDGE_CURVE ( 'NONE', #64477, #17545, #22683, .T. ) ;
#33224=CARTESIAN_POINT ( 'NONE',  ( -11.53846153846153655, -3.322132147404559976, 32.92929555188717927 ) ) ;
#33225=DIRECTION ( 'NONE',  ( 0.000000000000000000, 0.9396926207859126468, -0.3420201433256571111 ) ) ;
#33226=CARTESIAN_POINT ( 'NONE',  ( -5.076923076923075762, -5.557115091759785130, 34.35708131394839171 ) ) ;
#33227=ORIENTED_EDGE ( 'NONE', *, *, #63586, .T. ) ;
#33228=ORIENTED_EDGE ( 'NONE', *, *, #75798, .F. ) ;
#33229=EDGE_CURVE ( 'NONE', #83978, #68708, #2249, .T. ) ;
#33230=EDGE_LOOP ( 'NONE', ( #86422, #11406, #58311, #27526 ) ) ;
#33231=CYLINDRICAL_SURFACE ( 'NONE', #28596, 0.2499999999999994726 ) ;
#33232=EDGE_LOOP ( 'NONE', ( #85834, #80338 ) ) ;
#33233=CARTESIAN_POINT ( 'NONE',  ( -16.40382289789473802, -12.41104346484419452, 31.60698883733904196 ) ) ;
#33234=CARTESIAN_POINT ( 'NONE',  ( 6.923076923076924238, -13.75783147151868846, 33.36296068462461051 ) ) ;
#33235=ADVANCED_FACE ( 'NONE', ( #68139 ), #6004, .F. ) ;
#33236=DIRECTION ( 'NONE',  ( -0.000000000000000000, 1.000000000000000000, -0.000000000000000000 ) ) ;
#33237=CARTESIAN_POINT ( 'NONE',  ( -5.750054481651857508, -4.336752205174647656, 33.62275283266504289 ) ) ;
#33238=ADVANCED_FACE ( 'NONE', ( #123 ), #88874, .F. ) ;
#33240=VERTEX_POINT ( 'NONE', #74016 ) ;
#33242=CARTESIAN_POINT ( 'NONE',  ( -9.442307692306256328, -7.500000000000155431, 34.75000000000007105 ) ) ;
#33243=CYLINDRICAL_SURFACE ( 'NONE', #17145, 0.2500000000000002220 ) ;
#33245=B_SPLINE_CURVE_WITH_KNOTS ( 'NONE', 3,
 ( #9988, #77569, #58170, #3232, #83901, #70372, #1471, #8679, #70820, #22617 ),
 .UNSPECIFIED., .F., .F.,
 ( 4, 2, 2, 2, 4 ),
 ( 0.0007817359527651101701, 0.0009771254036996489256, 0.001172514854634187790, 0.001367904305568726653, 0.001563293756503265517 ),
 .UNSPECIFIED. ) ;
#33246=CARTESIAN_POINT ( 'NONE',  ( 3.164685819813349177, -11.69971097300155272, 32.46337939537587403 ) ) ;
#33247=VECTOR ( 'NONE', #32002, 1000.000000000000000 ) ;
#33248=CARTESIAN_POINT ( 'NONE',  ( -17.14219307747939425, -3.643525952247790300, 33.31231777344662959 ) ) ;
#33250=ORIENTED_EDGE ( 'NONE', *, *, #56551, .T. ) ;
#33251=CARTESIAN_POINT ( 'NONE',  ( -11.47320639894870276, -4.320704448112861584, 33.92786785259548310 ) ) ;
#33252=AXIS2_PLACEMENT_3D ( 'NONE', #6492, #83037, #28087 ) ;
#33253=CARTESIAN_POINT ( 'NONE',  ( 8.992242120843620512, -12.39991518177334129, 30.74647679643404530 ) ) ;
#33254=CYLINDRICAL_SURFACE ( 'NONE', #68441, 0.2499999999999994726 ) ;
#33255=FACE_BOUND ( 'NONE', #9000, .T. ) ;
#33256=CARTESIAN_POINT ( 'NONE',  ( 18.00000000000000000, -5.557115091759785130, 34.35708131394839171 ) ) ;
#33257=CARTESIAN_POINT ( 'NONE',  ( -18.00000000000000000, -2.249999999999988898, 29.99999999999998579 ) ) ;
#33258=CARTESIAN_POINT ( 'NONE',  ( -9.019254006523732770, -4.335965774309648246, 33.62209801155881905 ) ) ;
#33259=CARTESIAN_POINT ( 'NONE',  ( 9.442330961365341224, -3.137211980971221781, 32.19342716148376837 ) ) ;
#33260=CARTESIAN_POINT ( 'NONE',  ( 15.48071464014727283, -10.18230066228895758, 34.26354781536631577 ) ) ;
#33261=EDGE_CURVE ( 'NONE', #55459, #22454, #73582, .T. ) ;
#33262=CARTESIAN_POINT ( 'NONE',  ( 0.4615384615384611200, -12.10708131394839349, 31.69288490824020244 ) ) ;
#33263=CARTESIAN_POINT ( 'NONE',  ( -0.6844646790546099480, -3.586966769969700763, 32.86292498521069660 ) ) ;
#33264=ORIENTED_EDGE ( 'NONE', *, *, #79636, .T. ) ;
#33265=EDGE_CURVE ( 'NONE', #79311, #26451, #54914, .T. ) ;
#33266=LINE ( 'NONE', #32817, #40365 ) ;
#33267=CARTESIAN_POINT ( 'NONE',  ( 0.2115617174898699049, -10.82459398097509684, 33.81372124010185587 ) ) ;
#33268=VERTEX_POINT ( 'NONE', #20832 ) ;
#33269=B_SPLINE_CURVE_WITH_KNOTS ( 'NONE', 3,
 ( #45528, #4997, #60819, #53163, #59036, #86992, #88322, #53619, #67585, #47300 ),
 .UNSPECIFIED., .F., .F.,
 ( 4, 2, 2, 2, 4 ),
 ( 0.000000000000000000, 0.0001954311564186870371, 0.0003908623128373740741, 0.0005862934692560610840, 0.0007817246256747481482 ),
 .UNSPECIFIED. ) ;
#33270=VERTEX_POINT ( 'NONE', #19941 ) ;
#33272=CARTESIAN_POINT ( 'NONE',  ( 16.02315555073584363, -2.295517848115769421, 30.44137282052136939 ) ) ;
#33273=DIRECTION ( 'NONE',  ( -0.000000000000000000, 0.3420201433256694901, -0.9396926207859082059 ) ) ;
#33274=ORIENTED_EDGE ( 'NONE', *, *, #2520, .F. ) ;
#33275=CARTESIAN_POINT ( 'NONE',  ( 11.53846153846141576, -10.33852847137269571, 34.16647553114546554 ) ) ;
#33276=CARTESIAN_POINT ( 'NONE',  ( 2.557692307693744560, -7.500000000000155431, 34.75000000000007105 ) ) ;
#33277=FACE_BOUND ( 'NONE', #35440, .T. ) ;
#33278=DIRECTION ( 'NONE',  ( 0.000000000000000000, 1.000000000000000000, 0.000000000000000000 ) ) ;
#33279=CARTESIAN_POINT ( 'NONE',  ( -9.822454901745910405, -4.460286881179643004, 33.72017969459903242 ) ) ;
#33280=CARTESIAN_POINT ( 'NONE',  ( 8.068933387422255521, -9.332535724633405749, 34.40230450496446934 ) ) ;
#33282=CARTESIAN_POINT ( 'NONE',  ( 2.557746619330623528, -4.943051570960395047, 34.04725096376909477 ) ) ;
#33284=CARTESIAN_POINT ( 'NONE',  ( 0.2380535178145126718, -5.912607949931405926, 34.49155766932282319 ) ) ;
#33286=ORIENTED_EDGE ( 'NONE', *, *, #74646, .F. ) ;
#33287=AXIS2_PLACEMENT_3D ( 'NONE', #61158, #67047, #46325 ) ;
#33288=ORIENTED_EDGE ( 'NONE', *, *, #62600, .F. ) ;
#33289=CARTESIAN_POINT ( 'NONE',  ( 9.692307692307695177, -13.75783147151868846, 33.36296068462461051 ) ) ;
#33290=ADVANCED_FACE ( 'NONE', ( #19502 ), #54606, .F. ) ;
#33291=LINE ( 'NONE', #26976, #74329 ) ;
#33292=CARTESIAN_POINT ( 'NONE',  ( -10.61538461538461320, -6.386643153685126251, 34.62446782046654192 ) ) ;
#33293=CARTESIAN_POINT ( 'NONE',  ( 6.923076923076802558, -12.27809138561165270, 31.22303859784587132 ) ) ;
#33294=CARTESIAN_POINT ( 'NONE',  ( -7.596153846153844924, -2.249999999999998668, 29.75000000000000355 ) ) ;
#33296=AXIS2_PLACEMENT_3D ( 'NONE', #77377, #42718, #63414 ) ;
#33297=CARTESIAN_POINT ( 'NONE',  ( -1.450697763975518306, -3.937682226553329556, 33.60647404775217240 ) ) ;
#33298=CARTESIAN_POINT ( 'NONE',  ( -6.249976744048591826, -8.347322224742351082, 34.93158281831414769 ) ) ;
#33299=CARTESIAN_POINT ( 'NONE',  ( 16.82694634598072270, -12.17611988154120795, 31.52148481390971213 ) ) ;
#33300=CARTESIAN_POINT ( 'NONE',  ( 13.13463864056679498, -10.06842814019191401, 34.32929386961144758 ) ) ;
#33301=DIRECTION ( 'NONE',  ( 0.000000000000000000, 0.9396926207859126468, -0.3420201433256571111 ) ) ;
#33302=CARTESIAN_POINT ( 'NONE',  ( 13.16113044089144068, -4.386631170607603991, 33.66268669641500111 ) ) ;
#33303=CYLINDRICAL_SURFACE ( 'NONE', #68310, 0.2500000000000002220 ) ;
#33304=EDGE_CURVE ( 'NONE', #9576, #42657, #50592, .T. ) ;
#33305=FACE_OUTER_BOUND ( 'NONE', #40700, .T. ) ;
#33306=CARTESIAN_POINT ( 'NONE',  ( -3.296851610129366339, -12.34228464037088280, 31.77849191805838558 ) ) ;
#33307=EDGE_LOOP ( 'NONE', ( #64882, #55209 ) ) ;
#33308=CARTESIAN_POINT ( 'NONE',  ( 1.253923917947826538, -2.541943142973489778, 30.39792223712631980 ) ) ;
#33309=EDGE_CURVE ( 'NONE', #79691, #54317, #5464, .T. ) ;
#33310=CARTESIAN_POINT ( 'NONE',  ( -16.15384615384615330, -4.786620604624113540, 33.94971097300155094 ) ) ;
#33313=DIRECTION ( 'NONE',  ( 0.000000000000000000, 0.000000000000000000, -1.000000000000000000 ) ) ;
#33314=FACE_OUTER_BOUND ( 'NONE', #67156, .T. ) ;
#33315=CARTESIAN_POINT ( 'NONE',  ( 10.36540788444226102, -5.728515186090277211, 34.42611988154120439 ) ) ;
#33316=CARTESIAN_POINT ( 'NONE',  ( -18.22629316816001932, -2.249999999999999556, 29.62232573653512446 ) ) ;
#33317=EDGE_LOOP ( 'NONE', ( #64914, #14541, #19521, #61366 ) ) ;
#33319=CARTESIAN_POINT ( 'NONE',  ( 17.74997676270703550, -3.711651800289232916, 33.01384336483936011 ) ) ;
#33320=VERTEX_POINT ( 'NONE', #81660 ) ;
#33321=CARTESIAN_POINT ( 'NONE',  ( -16.15384615384627409, -10.21337939537710326, 33.94971097300076224 ) ) ;
#33322=EDGE_CURVE ( 'NONE', #4010, #4115, #25886, .T. ) ;
#33323=CARTESIAN_POINT ( 'NONE',  ( -2.176900499867520988, -2.541949514083463590, 30.39797389878540557 ) ) ;
#33324=ORIENTED_EDGE ( 'NONE', *, *, #69763, .F. ) ;
#33325=AXIS2_PLACEMENT_3D ( 'NONE', #69375, #7676, #910 ) ;
#33326=DIRECTION ( 'NONE',  ( -0.000000000000000000, -0.7660444431189791237, -0.6427876096865379196 ) ) ;
#33328=CARTESIAN_POINT ( 'NONE',  ( 6.000000000000001776, -13.20930481340135110, 34.54067556320372745 ) ) ;
#33331=VERTEX_POINT ( 'NONE', #77550 ) ;
#33332=VERTEX_POINT ( 'NONE', #69464 ) ;
#33333=CARTESIAN_POINT ( 'NONE',  ( -17.93474486048716088, -5.094484230520770929, 34.41647553114626845 ) ) ;
#33334=CARTESIAN_POINT ( 'NONE',  ( 6.988332062589762472, -11.67786785259547777, 32.92929555188713664 ) ) ;
#33335=CARTESIAN_POINT ( 'NONE',  ( -9.626239341305252495, -9.780366693483667717, 34.19971097300155805 ) ) ;
#33336=CARTESIAN_POINT ( 'NONE',  ( -15.48074597481782178, -2.318417181685855422, 30.59732222474233865 ) ) ;
#33337=CARTESIAN_POINT ( 'NONE',  ( 13.38461538461526423, -6.835583212225970762, 34.95778746994575670 ) ) ;
#33338=CARTESIAN_POINT ( 'NONE',  ( 9.692307692307570832, -10.33852847137269571, 34.16647553114546554 ) ) ;
#33340=LINE ( 'NONE', #51800, #49531 ) ;
#33341=EDGE_CURVE ( 'NONE', #40963, #13065, #32235, .T. ) ;
#33342=LINE ( 'NONE', #14507, #37701 ) ;
#33343=ORIENTED_EDGE ( 'NONE', *, *, #55970, .T. ) ;
#33344=VERTEX_POINT ( 'NONE', #14519 ) ;
#33345=CARTESIAN_POINT ( 'NONE',  ( -17.30040802064702987, -10.11188796281391511, 34.01382737946119050 ) ) ;
#33346=VERTEX_POINT ( 'NONE', #55944 ) ;
#33347=B_SPLINE_CURVE_WITH_KNOTS ( 'NONE', 3,
 ( #11682, #4467, #52200, #18433, #72028, #79689, #51282, #17992, #59856, #17090 ),
 .UNSPECIFIED., .F., .F.,
 ( 4, 2, 2, 2, 4 ),
 ( 0.0007817246256747453293, 0.0009771112852218889842, 0.001172497944769032531, 0.001367884604316176294, 0.001563271263863319840 ),
 .UNSPECIFIED. ) ;
#33348=AXIS2_PLACEMENT_3D ( 'NONE', #84993, #72350, #79569 ) ;
#33349=CARTESIAN_POINT ( 'NONE',  ( 10.36538461538460076, -2.249999999999998668, 29.81609741502487765 ) ) ;
#33350=DIRECTION ( 'NONE',  ( -0.000000000000000000, 0.000000000000000000, 1.000000000000000000 ) ) ;
#33351=ORIENTED_EDGE ( 'NONE', *, *, #42574, .T. ) ;
#33353=VERTEX_POINT ( 'NONE', #15861 ) ;
#33354=CARTESIAN_POINT ( 'NONE',  ( 15.90384615384615330, -7.500000000000001776, 34.75000000000000000 ) ) ;
#33355=EDGE_LOOP ( 'NONE', ( #9185, #11313, #22366, #57846 ) ) ;
#33358=EDGE_CURVE ( 'NONE', #46099, #42810, #68778, .T. ) ;
#33359=CARTESIAN_POINT ( 'NONE',  ( 1.450683735617825043, -6.386643153685127139, 34.62446782046654192 ) ) ;
#33361=FACE_BOUND ( 'NONE', #26925, .T. ) ;
#33362=CARTESIAN_POINT ( 'NONE',  ( 14.30769230769231015, -13.49023893513002648, 31.06009739812518688 ) ) ;
#33363=CARTESIAN_POINT ( 'NONE',  ( 15.93091919493929964, -3.395401636524186362, 33.02366814457250399 ) ) ;
#33364=EDGE_CURVE ( 'NONE', #82738, #77091, #28034, .T. ) ;
#33365=CARTESIAN_POINT ( 'NONE',  ( -18.00000000000000000, -12.08385125132259574, 35.60175215339625510 ) ) ;
#33366=CARTESIAN_POINT ( 'NONE',  ( -6.923076923076922462, -11.69971097300155272, 32.46337939537588113 ) ) ;
#33367=CARTESIAN_POINT ( 'NONE',  ( 10.86538461538455280, -7.565270445406050648, 34.75000000000000000 ) ) ;
#33368=CARTESIAN_POINT ( 'NONE',  ( -8.069638770718176701, -9.417330523894424488, 34.63758898049880486 ) ) ;
#33369=ADVANCED_FACE ( 'NONE', ( #69904 ), #29816, .F. ) ;
#33370=CARTESIAN_POINT ( 'NONE',  ( 1.384615384615701439, -2.255955759149395501, 30.00000000000324363 ) ) ;
#33371=ORIENTED_EDGE ( 'NONE', *, *, #4938, .F. ) ;
#33372=B_SPLINE_CURVE_WITH_KNOTS ( 'NONE', 3,
 ( #30717, #30284, #85232, #65391, #86124, #36600, #29843, #52318, #24847, #10002 ),
 .UNSPECIFIED., .F., .F.,
 ( 4, 2, 2, 2, 4 ),
 ( 0.0007817246256747484735, 0.0009771112852218920199, 0.001172497944769035783, 0.001367884604316179330, 0.001563271263863322876 ),
 .UNSPECIFIED. ) ;
#33374=CARTESIAN_POINT ( 'NONE',  ( -7.846153846153844924, -12.10708131394839349, 31.69288490824020244 ) ) ;
#33375=CARTESIAN_POINT ( 'NONE',  ( -14.24243673641628050, -12.46129190930001052, 30.37095296980870174 ) ) ;
#33376=EDGE_CURVE ( 'NONE', #78512, #43106, #8661, .T. ) ;
#33377=B_SPLINE_CURVE_WITH_KNOTS ( 'NONE', 3,
 ( #38300, #24322, #4965, #52691, #72519, #80179, #39199, #32431, #10383, #59897 ),
 .UNSPECIFIED., .F., .F.,
 ( 4, 2, 2, 2, 4 ),
 ( 0.000000000000000000, 0.0001954339857564091007, 0.0003908679715128182013, 0.0005863019572692273291, 0.0007817359430256364027 ),
 .UNSPECIFIED. ) ;
#33379=CARTESIAN_POINT ( 'NONE',  ( 16.28437159207980045, -11.66157788607254275, 32.95092075102925833 ) ) ;
#33380=CARTESIAN_POINT ( 'NONE',  ( -14.55771553191376100, -12.07920672191015221, 32.31858351112116168 ) ) ;
#33382=CARTESIAN_POINT ( 'NONE',  ( -2.057746789344165439, -2.824170634883621744, 31.52227843825338738 ) ) ;
#33383=ORIENTED_EDGE ( 'NONE', *, *, #65796, .T. ) ;
#33384=CARTESIAN_POINT ( 'NONE',  ( -5.326899820971668476, -5.643011162660950042, 34.66104346484419096 ) ) ;
#33386=CARTESIAN_POINT ( 'NONE',  ( -14.30769230769242739, -8.613356846316285953, 34.62446782046622218 ) ) ;
#33389=ORIENTED_EDGE ( 'NONE', *, *, #33322, .F. ) ;
#33390=EDGE_CURVE ( 'NONE', #41890, #60580, #8214, .T. ) ;
#33392=ORIENTED_EDGE ( 'NONE', *, *, #50268, .F. ) ;
#33394=EDGE_CURVE ( 'NONE', #33011, #81813, #25706, .T. ) ;
#33396=CARTESIAN_POINT ( 'NONE',  ( 3.100078627658923835, -12.62707690430377383, 30.88035979386743435 ) ) ;
#33397=CARTESIAN_POINT ( 'NONE',  ( -8.769230769230768274, -3.669653830205710676, 35.88435417666054406 ) ) ;
#33398=CARTESIAN_POINT ( 'NONE',  ( 3.361559671736181087, -9.929761469519744921, 34.40412654351204225 ) ) ;
#33399=LINE ( 'NONE', #60859, #47478 ) ;
#33400=FACE_OUTER_BOUND ( 'NONE', #24047, .T. ) ;
#33401=ORIENTED_EDGE ( 'NONE', *, *, #28435, .F. ) ;
#33402=CARTESIAN_POINT ( 'NONE',  ( -15.36146069743679021, -11.71456829005830080, 32.44064028649416542 ) ) ;
#33403=CARTESIAN_POINT ( 'NONE',  ( -15.45369618967607828, -11.98009711892699514, 32.48740034544076138 ) ) ;
#33405=DIRECTION ( 'NONE',  ( 0.000000000000000000, 0.4999999999999960032, -0.8660254037844410391 ) ) ;
#33406=CARTESIAN_POINT ( 'NONE',  ( -9.019230769230766498, -7.566082377512564960, 35.00000000000000711 ) ) ;
#33407=CARTESIAN_POINT ( 'NONE',  ( -13.51530685128294351, -4.809359713505814149, 33.96456829005828837 ) ) ;
#33408=CARTESIAN_POINT ( 'NONE',  ( -15.90384615384473399, -7.500000000000154543, 35.00000000000007105 ) ) ;
#33409=CARTESIAN_POINT ( 'NONE',  ( -8.769230769230892619, -8.656820664282941280, 34.87096338111179961 ) ) ;
#33410=CARTESIAN_POINT ( 'NONE',  ( -8.519176349317316266, -9.233818618650603938, 34.70587769442853698 ) ) ;
#33411=CARTESIAN_POINT ( 'NONE',  ( 12.68454981315131036, -11.24521262558773493, 33.06293181088029343 ) ) ;
#33413=EDGE_LOOP ( 'NONE', ( #1761, #11002, #42037, #25059 ) ) ;
#33414=EDGE_CURVE ( 'NONE', #40774, #6072, #76277, .T. ) ;
#33415=CARTESIAN_POINT ( 'NONE',  ( -7.053224892808620083, -11.04286588640298561, 33.62463336215343901 ) ) ;
#33416=CARTESIAN_POINT ( 'NONE',  ( 1.161688425708536698, -9.172386477786396597, 34.72672124145550043 ) ) ;
#33417=VECTOR ( 'NONE', #11571, 1000.000000000000227 ) ;
#33419=ORIENTED_EDGE ( 'NONE', *, *, #49895, .F. ) ;
#33420=CARTESIAN_POINT ( 'NONE',  ( -5.999999999999998224, -2.538708090699994813, 30.37095296980875503 ) ) ;
#33421=CARTESIAN_POINT ( 'NONE',  ( 3.165518240607989142, -2.506253911140460922, 30.00000000000013856 ) ) ;
#33423=CARTESIAN_POINT ( 'NONE',  ( -8.992715693795101828, -10.97335522853832579, 33.68706563782419749 ) ) ;
#33424=ADVANCED_FACE ( 'NONE', ( #567 ), #64022, .F. ) ;
#33425=CYLINDRICAL_SURFACE ( 'NONE', #68682, 0.2499999999999997502 ) ;
#33426=CARTESIAN_POINT ( 'NONE',  ( 0.4615384615383382183, -2.379036618888197285, 30.90682066428292885 ) ) ;
#33427=VERTEX_POINT ( 'NONE', #78429 ) ;
#33428=DIRECTION ( 'NONE',  ( -0.000000000000000000, -0.5000000000000009992, -0.8660254037844380415 ) ) ;
#33429=EDGE_CURVE ( 'NONE', #84305, #50475, #4554, .T. ) ;
#33430=CARTESIAN_POINT ( 'NONE',  ( 17.07692307692295586, -6.026961402154118908, 34.52809138561165270 ) ) ;
#33431=CARTESIAN_POINT ( 'NONE',  ( 7.715462379486288214, -9.804603061927743113, 34.18744698557895845 ) ) ;
#33432=EDGE_LOOP ( 'NONE', ( #36139, #79642, #25132, #44009 ) ) ;
#33433=CARTESIAN_POINT ( 'NONE',  ( -17.01085574357299990, -11.91647553114624358, 32.58852847137148245 ) ) ;
#33434=VERTEX_POINT ( 'NONE', #64458 ) ;
#33435=CARTESIAN_POINT ( 'NONE',  ( 14.30769230769231015, -12.29105614889573062, 35.45975837776705220 ) ) ;
#33436=DIRECTION ( 'NONE',  ( -1.000000000000000000, 0.000000000000000000, 0.000000000000000000 ) ) ;
#33437=ORIENTED_EDGE ( 'NONE', *, *, #69998, .T. ) ;
#33438=LINE ( 'NONE', #81188, #28951 ) ;
#33439=CARTESIAN_POINT ( 'NONE',  ( 13.60762822870878352, -9.172514111537584114, 34.72667873470787470 ) ) ;
#33440=ADVANCED_FACE ( 'NONE', ( #17175 ), #45536, .F. ) ;
#33441=LINE ( 'NONE', #54133, #2013 ) ;
#33444=DIRECTION ( 'NONE',  ( -0.000000000000000000, -0.000000000000000000, -1.000000000000000000 ) ) ;
#33445=CARTESIAN_POINT ( 'NONE',  ( -1.384615384615506484, -11.06231777344772027, 33.60647404775119895 ) ) ;
#33446=EDGE_CURVE ( 'NONE', #1831, #76906, #11844, .T. ) ;
#33447=VERTEX_POINT ( 'NONE', #43760 ) ;
#33448=FACE_BOUND ( 'NONE', #63606, .T. ) ;
#33449=EDGE_LOOP ( 'NONE', ( #70540, #87626, #27563, #60541 ) ) ;
#33450=CARTESIAN_POINT ( 'NONE',  ( -8.899921372341076165, -12.35290016733513951, 31.75349464988449455 ) ) ;
#33451=CARTESIAN_POINT ( 'NONE',  ( 9.019230769232203571, -7.500000000000155431, 34.75000000000007105 ) ) ;
#33452=CARTESIAN_POINT ( 'NONE',  ( 18.24994551834813805, -12.22109172314383052, 31.39792113162168263 ) ) ;
#33453=CARTESIAN_POINT ( 'NONE',  ( 3.230769230769231726, -13.49023893513002648, 31.06009739812518688 ) ) ;
#33454=CARTESIAN_POINT ( 'NONE',  ( -6.249976730942353065, -12.17611988154120972, 31.52148481390971213 ) ) ;
#33455=EDGE_LOOP ( 'NONE', ( #33957, #71564, #17394, #68153 ) ) ;
#33456=ORIENTED_EDGE ( 'NONE', *, *, #88259, .T. ) ;
#33457=ORIENTED_EDGE ( 'NONE', *, *, #33429, .T. ) ;
#33460=CARTESIAN_POINT ( 'NONE',  ( -6.000000000000119904, -12.46129190930018460, 30.37095296980731973 ) ) ;
#33461=CARTESIAN_POINT ( 'NONE',  ( -17.01172909513971732, -2.506253911140448043, 29.99999999999988631 ) ) ;
#33462=CARTESIAN_POINT ( 'NONE',  ( 13.38461538461538680, -11.11383981884818262, 36.00935417666054406 ) ) ;
#33463=B_SPLINE_CURVE_WITH_KNOTS ( 'NONE', 3,
 ( #82634, #83066, #42525, #49274, #35311, #69980, #77186, #41192, #643, #35771 ),
 .UNSPECIFIED., .F., .F.,
 ( 4, 2, 2, 2, 4 ),
 ( 0.0007817246256747477145, 0.0009771112852218907189, 0.001172497944769033615, 0.001367884604316176511, 0.001563271263863319407 ),
 .UNSPECIFIED. ) ;
#33464=AXIS2_PLACEMENT_3D ( 'NONE', #47905, #13679, #88049 ) ;
#33465=CARTESIAN_POINT ( 'NONE',  ( 17.77651505627605033, -10.11188796281391511, 34.01382737946119050 ) ) ;
#33466=VECTOR ( 'NONE', #32555, 1000.000000000000000 ) ;
#33467=DIRECTION ( 'NONE',  ( -0.000000000000000000, 0.7660444431189791237, -0.6427876096865379196 ) ) ;
#33468=CARTESIAN_POINT ( 'NONE',  ( -4.946131269098287930, -4.118422570099827595, 33.43335022499816489 ) ) ;
#33469=DIRECTION ( 'NONE',  ( -0.000000000000000000, 0.3420201433256694346, -0.9396926207859080948 ) ) ;
#33470=ORIENTED_EDGE ( 'NONE', *, *, #5698, .F. ) ;
#33471=B_SPLINE_CURVE_WITH_KNOTS ( 'NONE', 3,
 ( #34179, #20664, #56227, #41387, #55332, #14350, #47695, #21998, #49472, #34627 ),
 .UNSPECIFIED., .F., .F.,
 ( 4, 2, 2, 2, 4 ),
 ( 0.000000000000000000, 0.0001954339857564100222, 0.0003908679715128200445, 0.0005863019572692300396, 0.0007817359430256400890 ),
 .UNSPECIFIED. ) ;
#33472=VERTEX_POINT ( 'NONE', #72115 ) ;
#33473=AXIS2_PLACEMENT_3D ( 'NONE', #871, #83298, #47729 ) ;
#33474=EDGE_LOOP ( 'NONE', ( #79742, #73197 ) ) ;
#33476=ORIENTED_EDGE ( 'NONE', *, *, #25044, .F. ) ;
#33477=CARTESIAN_POINT ( 'NONE',  ( -2.980714810855778385, -10.06805714834173848, 34.32951233291982618 ) ) ;
#33478=CARTESIAN_POINT ( 'NONE',  ( -5.869208192175211281, -3.530189275343204702, 32.79018710029569661 ) ) ;
#33479=EDGE_CURVE ( 'NONE', #71762, #51826, #26823, .T. ) ;
#33480=LINE ( 'NONE', #60052, #55743 ) ;
#33481=DIRECTION ( 'NONE',  ( 0.000000000000000000, 0.9848077530122072432, 0.1736481776669354937 ) ) ;
#33482=FACE_BOUND ( 'NONE', #30809, .T. ) ;
#33483=VERTEX_POINT ( 'NONE', #65362 ) ;
#33485=CARTESIAN_POINT ( 'NONE',  ( -3.007757879156380820, -6.503523203565942268, 34.64991518177335195 ) ) ;
#33486=VERTEX_POINT ( 'NONE', #78875 ) ;
#33487=EDGE_CURVE ( 'NONE', #19576, #46099, #31126, .T. ) ;
#33488=CARTESIAN_POINT ( 'NONE',  ( -4.854143535654666941, -6.760870238392817200, 34.69528174975672385 ) ) ;
#33489=B_SPLINE_CURVE_WITH_KNOTS ( 'NONE', 3,
 ( #87606, #44805, #73187, #18694, #32636, #60107, #79046, #72284, #45256, #79942 ),
 .UNSPECIFIED., .F., .F.,
 ( 4, 2, 2, 2, 4 ),
 ( 0.0007817246256747460882, 0.0009771112852218892010, 0.001172497944769032314, 0.001367884604316175643, 0.001563271263863318756 ),
 .UNSPECIFIED. ) ;
#33490=ORIENTED_EDGE ( 'NONE', *, *, #55475, .T. ) ;
#33491=FACE_BOUND ( 'NONE', #26239, .T. ) ;
#33492=CARTESIAN_POINT ( 'NONE',  ( -9.561782254074051579, -2.372941743896879174, 30.88044141588253666 ) ) ;
#33493=CARTESIAN_POINT ( 'NONE',  ( 18.24994551834813805, -5.057305518903949526, 34.11320923018887896 ) ) ;
#33494=EDGE_LOOP ( 'NONE', ( #33545, #26180, #62057, #75197 ) ) ;
#33496=CARTESIAN_POINT ( 'NONE',  ( -12.68446542044531000, -11.98009711892699514, 32.48740034544076138 ) ) ;
#33497=DIRECTION ( 'NONE',  ( -0.000000000000000000, 0.6427876096865404731, -0.7660444431189771253 ) ) ;
#33499=FACE_OUTER_BOUND ( 'NONE', #20301, .T. ) ;
#33501=CARTESIAN_POINT ( 'NONE',  ( 12.52760681254089903, -6.386643153685127139, 34.62446782046654192 ) ) ;
#33502=CARTESIAN_POINT ( 'NONE',  ( -7.911424292114620727, -2.892918686051583421, 31.69288490824015980 ) ) ;
#33503=EDGE_LOOP ( 'NONE', ( #63527, #60904 ) ) ;
#33504=EDGE_CURVE ( 'NONE', #87552, #60114, #24366, .T. ) ;
#33505=DIRECTION ( 'NONE',  ( -0.000000000000000000, -0.000000000000000000, -1.000000000000000000 ) ) ;
#33506=AXIS2_PLACEMENT_3D ( 'NONE', #23660, #71398, #16909 ) ;
#33507=CARTESIAN_POINT ( 'NONE',  ( -16.02332071561251325, -10.31582465632704704, 34.18122507451815295 ) ) ;
#33508=AXIS2_PLACEMENT_3D ( 'NONE', #16069, #85417, #29590 ) ;
#33509=ORIENTED_EDGE ( 'NONE', *, *, #60770, .F. ) ;
#33510=CARTESIAN_POINT ( 'NONE',  ( 16.15384615384615330, -1.367168528481310208, 33.57946703557072254 ) ) ;
#33511=CARTESIAN_POINT ( 'NONE',  ( 16.02369818411445834, -4.299443229763728169, 33.91186481527756058 ) ) ;
#33512=CARTESIAN_POINT ( 'NONE',  ( -14.37296230824862953, -2.657715359629089225, 31.77849191805832874 ) ) ;
#33513=CARTESIAN_POINT ( 'NONE',  ( 16.37685899793954292, -11.98016756924215187, 32.48728574198911190 ) ) ;
#33514=CARTESIAN_POINT ( 'NONE',  ( 0.2115152373170014477, -2.588893531581426988, 31.60682220781848528 ) ) ;
#33515=CARTESIAN_POINT ( 'NONE',  ( 14.98079248672064345, -5.643011162660950042, 34.66104346484419096 ) ) ;
#33516=CARTESIAN_POINT ( 'NONE',  ( 6.130791807824786943, -11.71459661697925903, 32.44059661609676937 ) ) ;
#33517=CARTESIAN_POINT ( 'NONE',  ( 5.076923076923075762, -13.04860791097971706, 34.73218667398347037 ) ) ;
#33518=B_SPLINE_CURVE_WITH_KNOTS ( 'NONE', 3,
 ( #81929, #19773, #75169, #27415, #53097, #67964, #67076, #6266, #5374, #32843 ),
 .UNSPECIFIED., .F., .F.,
 ( 4, 2, 2, 2, 4 ),
 ( 0.000000000000000000, 0.0001954339857564070949, 0.0003908679715128141898, 0.0005863019572692212576, 0.0007817359430256283796 ),
 .UNSPECIFIED. ) ;
#33520=B_SPLINE_CURVE_WITH_KNOTS ( 'NONE', 3,
 ( #28264, #1235, #1685, #48984, #76464, #11549, #79113, #57506, #31827, #59281 ),
 .UNSPECIFIED., .F., .F.,
 ( 4, 2, 2, 2, 4 ),
 ( 0.0007817359430256346680, 0.0009771253907250002264, 0.001172514838424365893, 0.001367904286123731560, 0.001563293733823104166 ),
 .UNSPECIFIED. ) ;
#33522=ORIENTED_EDGE ( 'NONE', *, *, #20039, .T. ) ;
#33523=EDGE_CURVE ( 'NONE', #21721, #68660, #32254, .T. ) ;
#33525=ORIENTED_EDGE ( 'NONE', *, *, #54802, .T. ) ;
#33526=ORIENTED_EDGE ( 'NONE', *, *, #83797, .T. ) ;
#33527=ADVANCED_FACE ( 'NONE', ( #71224 ), #57721, .F. ) ;
#33528=CARTESIAN_POINT ( 'NONE',  ( -11.47320639894870276, -2.379036618887895305, 30.90682066428158592 ) ) ;
#33529=VERTEX_POINT ( 'NONE', #9972 ) ;
#33530=CARTESIAN_POINT ( 'NONE',  ( 14.05766907039934210, -8.432397168068783699, 34.66272746175022945 ) ) ;
#33532=CARTESIAN_POINT ( 'NONE',  ( 14.30769230769231015, -11.16473453929635440, 33.15142922261926373 ) ) ;
#33533=CARTESIAN_POINT ( 'NONE',  ( 5.750023269057647823, -11.28823185664190376, 33.01397839955799896 ) ) ;
#33534=CARTESIAN_POINT ( 'NONE',  ( -0.2115929431903192381, -5.852078868378310261, 34.47109172314383585 ) ) ;
#33535=CARTESIAN_POINT ( 'NONE',  ( -8.546451227962359454, -5.114059244376869984, 34.14424750095245287 ) ) ;
#33536=CARTESIAN_POINT ( 'NONE',  ( -0.4615384615384611200, -11.91647553114624181, 32.58852847137148245 ) ) ;
#33537=FACE_OUTER_BOUND ( 'NONE', #79768, .T. ) ;
#33538=CARTESIAN_POINT ( 'NONE',  ( 6.923076923076800782, -12.51329471203414379, 31.30864560766407578 ) ) ;
#33539=CARTESIAN_POINT ( 'NONE',  ( 10.61538461538461675, -9.780366693483667717, 34.19971097300155094 ) ) ;
#33540=CARTESIAN_POINT ( 'NONE',  ( -17.07692307692319744, -4.320704448113951379, 33.92786785259630022 ) ) ;
#33541=ADVANCED_FACE ( 'NONE', ( #37439 ), #81118, .F. ) ;
#33542=CARTESIAN_POINT ( 'NONE',  ( 5.934729999443682402, -3.643525952247789412, 33.31231777344662959 ) ) ;
#33545=ORIENTED_EDGE ( 'NONE', *, *, #31598, .T. ) ;
#33546=ORIENTED_EDGE ( 'NONE', *, *, #37887, .T. ) ;
#33547=CARTESIAN_POINT ( 'NONE',  ( 14.17700170458200581, -8.191372820521381826, 34.95448215188423546 ) ) ;
#33548=DIRECTION ( 'NONE',  ( 0.000000000000000000, -6.938893903907222067E-15, 1.000000000000000000 ) ) ;
#33550=CARTESIAN_POINT ( 'NONE',  ( 12.46153846153833911, -6.026961402154118019, 34.52809138561165270 ) ) ;
#33551=CARTESIAN_POINT ( 'NONE',  ( -12.46153846153846168, -2.833524468853757305, 32.15551576947925838 ) ) ;
#33552=EDGE_CURVE ( 'NONE', #47571, #66205, #39243, .T. ) ;
#33553=VECTOR ( 'NONE', #50876, 1000.000000000000000 ) ;
#33554=CARTESIAN_POINT ( 'NONE',  ( -13.45069776397551742, -10.67929555188718460, 33.92786785259543336 ) ) ;
#33555=CARTESIAN_POINT ( 'NONE',  ( 13.38461538461526601, -6.026961402154118019, 34.52809138561165270 ) ) ;
#33558=ORIENTED_EDGE ( 'NONE', *, *, #60998, .T. ) ;
#33559=CARTESIAN_POINT ( 'NONE',  ( -7.846153846153844924, -9.780366693483667717, 34.19971097300155094 ) ) ;
#33560=VERTEX_POINT ( 'NONE', #81559 ) ;
#33561=EDGE_CURVE ( 'NONE', #34382, #77626, #35432, .T. ) ;
#33562=ORIENTED_EDGE ( 'NONE', *, *, #4202, .T. ) ;
#33563=CARTESIAN_POINT ( 'NONE',  ( 5.207448778686639024, -8.586989748646452369, 34.63063291749215011 ) ) ;
#33564=CARTESIAN_POINT ( 'NONE',  ( -7.846153846153844924, -2.721908614388771852, 31.22303859784724978 ) ) ;
#33565=CARTESIAN_POINT ( 'NONE',  ( 14.30769230769218758, -5.219633306517616589, 34.19971097300220464 ) ) ;
#33566=CARTESIAN_POINT ( 'NONE',  ( 4.023155550735846298, -6.369640206132550553, 34.87707690430378449 ) ) ;
#33567=DIRECTION ( 'NONE',  ( 0.000000000000000000, 0.4999999999999985567, 0.8660254037844395958 ) ) ;
#33568=ORIENTED_EDGE ( 'NONE', *, *, #79894, .T. ) ;
#33569=AXIS2_PLACEMENT_3D ( 'NONE', #7548, #48514, #75127 ) ;
#33570=AXIS2_PLACEMENT_3D ( 'NONE', #73564, #65888, #17266 ) ;
#33571=VERTEX_POINT ( 'NONE', #33802 ) ;
#33572=ORIENTED_EDGE ( 'NONE', *, *, #31233, .F. ) ;
#33573=ORIENTED_EDGE ( 'NONE', *, *, #79189, .T. ) ;
#33574=CARTESIAN_POINT ( 'NONE',  ( -6.065270000556319374, -5.094484230520674117, 34.41647553114621161 ) ) ;
#33575=DIRECTION ( 'NONE',  ( -1.000000000000000000, 0.000000000000000000, 0.000000000000000000 ) ) ;
#33576=CARTESIAN_POINT ( 'NONE',  ( 4.219101293358988869, -12.16647553114626490, 32.15551576947920864 ) ) ;
#33577=CYLINDRICAL_SURFACE ( 'NONE', #51350, 0.2499999999999997502 ) ;
#33578=CARTESIAN_POINT ( 'NONE',  ( -15.16470189741915675, -9.058645607665452459, 34.76329471203371924 ) ) ;
#33579=CARTESIAN_POINT ( 'NONE',  ( 12.46153846153833911, -3.083524468854526912, 32.58852847137268327 ) ) ;
#33580=ORIENTED_EDGE ( 'NONE', *, *, #21248, .T. ) ;
#33581=VERTEX_POINT ( 'NONE', #87437 ) ;
#33582=ORIENTED_EDGE ( 'NONE', *, *, #23491, .F. ) ;
#33583=CARTESIAN_POINT ( 'NONE',  ( -10.61538461538461320, -11.69971097300155272, 32.46337939537588113 ) ) ;
#33585=CARTESIAN_POINT ( 'NONE',  ( 17.32686848630112308, -10.92531984108285492, 33.72920026020278073 ) ) ;
#33586=CARTESIAN_POINT ( 'NONE',  ( -4.826977558574935045, -11.37275283266503756, 32.91324779482534524 ) ) ;
#33588=EDGE_LOOP ( 'NONE', ( #36471, #70973, #15883, #12294 ) ) ;
#33589=CARTESIAN_POINT ( 'NONE',  ( -1.319360245102545459, -11.67786785259547777, 32.92929555188713664 ) ) ;
#33590=ORIENTED_EDGE ( 'NONE', *, *, #27913, .T. ) ;
#33591=CARTESIAN_POINT ( 'NONE',  ( -14.30769230769230660, -12.78798330534102767, 29.49999999999997868 ) ) ;
#33592=AXIS2_PLACEMENT_3D ( 'NONE', #38236, #87337, #67050 ) ;
#33593=FACE_BOUND ( 'NONE', #73238, .T. ) ;
#33594=LINE ( 'NONE', #73245, #30246 ) ;
#33596=CYLINDRICAL_SURFACE ( 'NONE', #10314, 0.2499999999999994726 ) ;
#33597=ORIENTED_EDGE ( 'NONE', *, *, #37589, .F. ) ;
#33598=FACE_OUTER_BOUND ( 'NONE', #18968, .T. ) ;
#33599=CARTESIAN_POINT ( 'NONE',  ( -14.17716660592874334, -2.619367082507849442, 30.83698974864643461 ) ) ;
#33600=CARTESIAN_POINT ( 'NONE',  ( 14.17700170458200404, -9.084618155246140248, 34.75535874321725771 ) ) ;
#33601=ORIENTED_EDGE ( 'NONE', *, *, #43239, .T. ) ;
#33602=CYLINDRICAL_SURFACE ( 'NONE', #86158, 0.2500000000000008882 ) ;
#33603=CARTESIAN_POINT ( 'NONE',  ( -3.903900744468109529, -10.18230066228895758, 34.26354781536631577 ) ) ;
#33604=CARTESIAN_POINT ( 'NONE',  ( -12.68502340526241312, -12.24155766932282496, 31.33739205006857986 ) ) ;
#33605=CARTESIAN_POINT ( 'NONE',  ( 10.61538461538461675, -6.189225973068211317, 35.74407628777942847 ) ) ;
#33606=CARTESIAN_POINT ( 'NONE',  ( 8.068933387422253745, -3.236590943229497697, 32.36255958852954251 ) ) ;
#33607=FACE_BOUND ( 'NONE', #3527, .T. ) ;
#33608=CARTESIAN_POINT ( 'NONE',  ( 1.634615384615323297, -7.565270000091922853, 34.99999999999999289 ) ) ;
#33610=CARTESIAN_POINT ( 'NONE',  ( -7.846153846153844924, -1.367168528481310208, 33.57946703557072254 ) ) ;
#33611=CARTESIAN_POINT ( 'NONE',  ( -8.546219417617917813, -11.76359900205217457, 32.36225158514719880 ) ) ;
#33612=CARTESIAN_POINT ( 'NONE',  ( -2.057637887778852814, -12.41089969410671223, 31.60739465890703670 ) ) ;
#33613=CARTESIAN_POINT ( 'NONE',  ( -8.769230769230890843, -3.835265460704628371, 33.15142922262033665 ) ) ;
#33615=ORIENTED_EDGE ( 'NONE', *, *, #77302, .T. ) ;
#33616=CARTESIAN_POINT ( 'NONE',  ( -7.053768389744481837, -8.999036380462719364, 34.52022231692819076 ) ) ;
#33617=ORIENTED_EDGE ( 'NONE', *, *, #59328, .T. ) ;
#33618=EDGE_CURVE ( 'NONE', #4333, #60674, #11764, .T. ) ;
#33619=CARTESIAN_POINT ( 'NONE',  ( 0.3954550505825804030, -6.386643153685125363, 34.62446782046654903 ) ) ;
#33620=EDGE_LOOP ( 'NONE', ( #67711, #43812 ) ) ;
#33622=CARTESIAN_POINT ( 'NONE',  ( 14.05769230769230838, -7.500000000000001776, 35.00000000000000000 ) ) ;
#33623=CARTESIAN_POINT ( 'NONE',  ( 14.98076923076922995, -2.499999999999999556, 29.81609845454691765 ) ) ;
#33624=EDGE_LOOP ( 'NONE', ( #11329, #48924, #1346, #85322 ) ) ;
#33625=LINE ( 'NONE', #66523, #67316 ) ;
#33626=CARTESIAN_POINT ( 'NONE',  ( 5.933917620639864943, -10.67929555188718460, 33.92786785259543336 ) ) ;
#33628=CARTESIAN_POINT ( 'NONE',  ( 14.24242186173153435, -10.90142922261923886, 33.41473453929638993 ) ) ;
#33629=CARTESIAN_POINT ( 'NONE',  ( -7.053767526187231240, -12.62707690430377383, 30.88035979386743435 ) ) ;
#33630=DIRECTION ( 'NONE',  ( -0.000000000000000000, 0.3420201433256694901, -0.9396926207859082059 ) ) ;
#33631=CARTESIAN_POINT ( 'NONE',  ( 12.71153846153846168, -2.249999999999998668, 29.75000000000000355 ) ) ;
#33632=CARTESIAN_POINT ( 'NONE',  ( 2.307692307692309264, -1.466349020453238561, 30.81389545987213907 ) ) ;
#33635=CARTESIAN_POINT ( 'NONE',  ( 9.757453471639660592, -7.750023238201979581, 34.74374492549440419 ) ) ;
#33637=CARTESIAN_POINT ( 'NONE',  ( -9.019207513279361876, -2.920706130388546651, 32.31842814019191223 ) ) ;
#33638=ORIENTED_EDGE ( 'NONE', *, *, #19777, .F. ) ;
#33641=B_SPLINE_CURVE_WITH_KNOTS ( 'NONE', 3,
 ( #86277, #50229, #37171, #44809, #17354, #57439, #64188, #71396, #11044, #16024 ),
 .UNSPECIFIED., .F., .F.,
 ( 4, 2, 2, 2, 4 ),
 ( 0.0007817246256747451124, 0.0009771112852218879000, 0.001172497944769030796, 0.001367884604316173692, 0.001563271263863316588 ),
 .UNSPECIFIED. ) ;
#33643=CARTESIAN_POINT ( 'NONE',  ( 0.4615384615384611200, -1.044019251281081972, 31.83374038241031911 ) ) ;
#33644=ORIENTED_EDGE ( 'NONE', *, *, #6854, .F. ) ;
#33645=CARTESIAN_POINT ( 'NONE',  ( 7.053602624840485724, -8.586989748646452369, 34.63063291749215011 ) ) ;
#33647=CARTESIAN_POINT ( 'NONE',  ( 1.318533005255250634, -5.471508081941601986, 34.59228464037088457 ) ) ;
#33648=ORIENTED_EDGE ( 'NONE', *, *, #37573, .F. ) ;
#33649=CARTESIAN_POINT ( 'NONE',  ( 12.68454981315131391, -12.39991518177334129, 30.74647679643404530 ) ) ;
#33650=CARTESIAN_POINT ( 'NONE',  ( 9.692307692307695177, -8.318370150425687726, 35.83090037661290239 ) ) ;
#33651=CARTESIAN_POINT ( 'NONE',  ( -12.52680846209478460, -5.094484230520674117, 34.41647553114621161 ) ) ;
#33652=ORIENTED_EDGE ( 'NONE', *, *, #32772, .F. ) ;
#33653=CARTESIAN_POINT ( 'NONE',  ( 2.084207383127977042, -4.225889041578354544, 33.85425143139329407 ) ) ;
#33654=CARTESIAN_POINT ( 'NONE',  ( -18.00000000000012079, -12.27809138561165270, 31.22303859784587132 ) ) ;
#33655=ADVANCED_FACE ( 'NONE', ( #26604 ), #20297, .F. ) ;
#33656=ADVANCED_FACE ( 'NONE', ( #19846 ), #75242, .F. ) ;
#33658=ORIENTED_EDGE ( 'NONE', *, *, #26712, .F. ) ;
#33659=ORIENTED_EDGE ( 'NONE', *, *, #25470, .F. ) ;
#33660=VERTEX_POINT ( 'NONE', #13093 ) ;
#33661=B_SPLINE_CURVE_WITH_KNOTS ( 'NONE', 3,
 ( #76479, #76921, #70156, #84137, #15665, #43135, #52976, #66954, #5248, #24176 ),
 .UNSPECIFIED., .F., .F.,
 ( 4, 2, 2, 2, 4 ),
 ( 0.0007817359430256358606, 0.0009771253907250034790, 0.001172514838424371098, 0.001367904286123738716, 0.001563293733823106334 ),
 .UNSPECIFIED. ) ;
#33662=AXIS2_PLACEMENT_3D ( 'NONE', #38870, #26675, #66778 ) ;
#33663=VERTEX_POINT ( 'NONE', #13531 ) ;
#33665=CARTESIAN_POINT ( 'NONE',  ( -9.757578138268467427, -2.892918686051582977, 31.69288490824015980 ) ) ;
#33667=EDGE_CURVE ( 'NONE', #14549, #54915, #73912, .T. ) ;
#33668=CARTESIAN_POINT ( 'NONE',  ( -16.40382289789474157, -2.920706130388546651, 32.31842814019191223 ) ) ;
#33669=FACE_OUTER_BOUND ( 'NONE', #56253, .T. ) ;
#33670=CARTESIAN_POINT ( 'NONE',  ( -17.93129618099654010, -7.250074905162718686, 34.99404781541490195 ) ) ;
#33671=EDGE_LOOP ( 'NONE', ( #1411, #47013, #3247, #53215 ) ) ;
#33673=B_SPLINE_CURVE_WITH_KNOTS ( 'NONE', 3,
 ( #47987, #34482, #28162, #55630, #76352, #75466, #15106, #42578, #14211, #44776 ),
 .UNSPECIFIED., .F., .F.,
 ( 4, 2, 2, 2, 4 ),
 ( 0.0007817246256747504250, 0.0009771112852218954894, 0.001172497944769040554, 0.001367884604316185401, 0.001563271263863330466 ),
 .UNSPECIFIED. ) ;
#33674=B_SPLINE_CURVE_WITH_KNOTS ( 'NONE', 3,
 ( #75039, #20957, #40369, #48429, #75915, #74591, #12879, #32705, #87677, #53416 ),
 .UNSPECIFIED., .F., .F.,
 ( 4, 2, 2, 2, 4 ),
 ( 0.0007817246256747516176, 0.0009771112852218965736, 0.001172497944769041421, 0.001367884604316186269, 0.001563271263863331333 ),
 .UNSPECIFIED. ) ;
#33675=ORIENTED_EDGE ( 'NONE', *, *, #14522, .T. ) ;
#33676=CARTESIAN_POINT ( 'NONE',  ( -7.053224892808621860, -2.647304123082328875, 31.75400227202885262 ) ) ;
#33677=ORIENTED_EDGE ( 'NONE', *, *, #23485, .F. ) ;
#33678=DIRECTION ( 'NONE',  ( -0.000000000000000000, 0.9848077530122085754, -0.1736481776669273613 ) ) ;
#33679=CARTESIAN_POINT ( 'NONE',  ( 5.933917620639864943, -12.62096338111211580, 30.90682066428152197 ) ) ;
#33681=CARTESIAN_POINT ( 'NONE',  ( -5.933931648997561759, -4.098570777380720287, 33.41473453929635440 ) ) ;
#33682=VERTEX_POINT ( 'NONE', #53630 ) ;
#33683=ORIENTED_EDGE ( 'NONE', *, *, #69657, .F. ) ;
#33685=EDGE_LOOP ( 'NONE', ( #46171, #45262, #33573, #24264 ) ) ;
#33686=DIRECTION ( 'NONE',  ( -0.000000000000000000, -0.9396926207859092051, -0.3420201433256662704 ) ) ;
#33687=DIRECTION ( 'NONE',  ( -0.000000000000000000, 0.5000000000000011102, -0.8660254037844380415 ) ) ;
#33688=ORIENTED_EDGE ( 'NONE', *, *, #76926, .T. ) ;
#33689=CARTESIAN_POINT ( 'NONE',  ( -2.057746789344164995, -8.433404298154334455, 34.66254593164985920 ) ) ;
#33690=LINE ( 'NONE', #22820, #26361 ) ;
#33691=VERTEX_POINT ( 'NONE', #52731 ) ;
#33692=CARTESIAN_POINT ( 'NONE',  ( 6.000000000000001776, -1.951392089020283160, 34.73218667398347748 ) ) ;
#33693=CARTESIAN_POINT ( 'NONE',  ( 9.757500680602349874, -2.255955759149235629, 29.99999999999988987 ) ) ;
#33694=CARTESIAN_POINT ( 'NONE',  ( 12.46153846153833911, -9.528491918059723176, 34.59228464037033035 ) ) ;
#33695=FACE_BOUND ( 'NONE', #72880, .T. ) ;
#33696=CARTESIAN_POINT ( 'NONE',  ( 10.61538461538449596, -10.21337939537710326, 33.94971097300076224 ) ) ;
#33698=DIRECTION ( 'NONE',  ( -0.000000000000000000, 1.000000000000000000, 3.491481338843133355E-15 ) ) ;
#33699=CARTESIAN_POINT ( 'NONE',  ( 9.692307692307695177, -3.050289026998446396, 32.03036669348365706 ) ) ;
#33700=CARTESIAN_POINT ( 'NONE',  ( 5.076923076923075762, -9.780366693483667717, 34.19971097300155094 ) ) ;
#33701=DIRECTION ( 'NONE',  ( -0.000000000000000000, -0.1736481776669307198, -0.9848077530122080203 ) ) ;
#33702=CARTESIAN_POINT ( 'NONE',  ( -0.5922299282060231596, -3.530157926970578508, 32.79014554554150607 ) ) ;
#33703=ORIENTED_EDGE ( 'NONE', *, *, #76983, .T. ) ;
#33704=CARTESIAN_POINT ( 'NONE',  ( 2.438218009455872526, -6.852161475712352789, 34.70806712695775786 ) ) ;
#33705=ORIENTED_EDGE ( 'NONE', *, *, #1889, .F. ) ;
#33706=EDGE_CURVE ( 'NONE', #16142, #23267, #32919, .T. ) ;
#33707=B_SPLINE_CURVE_WITH_KNOTS ( 'NONE', 3,
 ( #18040, #86050, #79738, #72977, #45496, #11276, #38749, #66212, #60503, #52848 ),
 .UNSPECIFIED., .F., .F.,
 ( 4, 2, 2, 2, 4 ),
 ( 0.000000000000000000, 0.0001954339857564093175, 0.0003908679715128186350, 0.0005863019572692279796, 0.0007817359430256372700 ),
 .UNSPECIFIED. ) ;
#33708=CARTESIAN_POINT ( 'NONE',  ( -6.857008572074484221, -4.786620604624113540, 33.94971097300155805 ) ) ;
#33709=CARTESIAN_POINT ( 'NONE',  ( -14.53117725141625627, -5.113361153441934093, 34.14387501736622710 ) ) ;
#33710=CARTESIAN_POINT ( 'NONE',  ( -7.715363405186898227, -2.295524264805589354, 30.44142389570982488 ) ) ;
#33711=ORIENTED_EDGE ( 'NONE', *, *, #39736, .F. ) ;
#33712=DIRECTION ( 'NONE',  ( 0.000000000000000000, 0.7660444431189807890, 0.6427876096865361433 ) ) ;
#33713=CARTESIAN_POINT ( 'NONE',  ( -15.10024379253558635, -12.70449254468099198, 30.44128974285582956 ) ) ;
#33714=AXIS2_PLACEMENT_3D ( 'NONE', #1009, #35230, #56397 ) ;
#33715=FACE_BOUND ( 'NONE', #79491, .T. ) ;
#33716=CARTESIAN_POINT ( 'NONE',  ( -14.30769230769230660, -3.937682226553329556, 33.60647404775216529 ) ) ;
#33717=FACE_OUTER_BOUND ( 'NONE', #40683, .T. ) ;
#33718=CARTESIAN_POINT ( 'NONE',  ( -6.923076923076922462, -2.499999999999998668, 29.75000000000001421 ) ) ;
#33719=CARTESIAN_POINT ( 'NONE',  ( 0.5276057948885366500, -4.661471528628508665, 34.16647553114624003 ) ) ;
#33721=CARTESIAN_POINT ( 'NONE',  ( -14.37301522318448299, -7.749976743299138882, 34.99404534957040624 ) ) ;
#33723=VERTEX_POINT ( 'NONE', #82003 ) ;
#33724=VECTOR ( 'NONE', #42202, 1000.000000000000114 ) ;
#33726=EDGE_CURVE ( 'NONE', #22286, #86499, #22510, .T. ) ;
#33728=CARTESIAN_POINT ( 'NONE',  ( -17.77698715590660328, -3.395485233115134172, 33.02377354290275946 ) ) ;
#33729=CARTESIAN_POINT ( 'NONE',  ( -5.999999999999998224, -13.75783147151868846, 33.36296068462461051 ) ) ;
#33730=CARTESIAN_POINT ( 'NONE',  ( 6.673100192134571174, -12.17611988154120972, 31.52148481390971213 ) ) ;
#33731=EDGE_CURVE ( 'NONE', #64564, #41090, #80607, .T. ) ;
#33732=CARTESIAN_POINT ( 'NONE',  ( 5.299702745901141654, -3.563462043263029955, 33.22394488606062879 ) ) ;
#33734=CARTESIAN_POINT ( 'NONE',  ( 1.384615384615386802, -11.11383981884818262, 36.00935417666054406 ) ) ;
#33735=FACE_OUTER_BOUND ( 'NONE', #49686, .T. ) ;
#33736=CARTESIAN_POINT ( 'NONE',  ( 7.596177102105255763, -5.643011162660950042, 34.66104346484419096 ) ) ;
#33737=CARTESIAN_POINT ( 'NONE',  ( -12.46153846153846168, -1.629998284177014645, 34.34916445242399163 ) ) ;
#33738=CARTESIAN_POINT ( 'NONE',  ( 16.15384615384615330, -1.129524287112498415, 32.06866353760679544 ) ) ;
#33739=CARTESIAN_POINT ( 'NONE',  ( -17.07692307692307665, -2.499999999999998668, 29.75000000000001421 ) ) ;
#33740=CARTESIAN_POINT ( 'NONE',  ( 6.856993512121044354, -11.16473453929635440, 33.15142922261925662 ) ) ;
#33741=CARTESIAN_POINT ( 'NONE',  ( -8.769230769230892619, -11.67786785259630911, 32.92929555188603530 ) ) ;
#33743=CARTESIAN_POINT ( 'NONE',  ( 17.07692307692295586, -12.70778746994576025, 30.41441678777401236 ) ) ;
#33744=VERTEX_POINT ( 'NONE', #7225 ) ;
#33745=CARTESIAN_POINT ( 'NONE',  ( 1.254468175177166689, -2.619462340734462380, 30.83744416345203021 ) ) ;
#33746=CARTESIAN_POINT ( 'NONE',  ( -6.923076923077044142, -12.46129190930018460, 30.37095296980731973 ) ) ;
#33749=CARTESIAN_POINT ( 'NONE',  ( 5.142990410273152513, -9.905515769479277921, 34.41647553114623292 ) ) ;
#33750=LINE ( 'NONE', #4953, #65657 ) ;
#33751=CARTESIAN_POINT ( 'NONE',  ( -8.769230769230768274, -11.91647553114624181, 32.58852847137148245 ) ) ;
#33752=CARTESIAN_POINT ( 'NONE',  ( -1.161604033002534342, -4.187068189119697692, 33.49521262558774026 ) ) ;
#33753=VERTEX_POINT ( 'NONE', #83329 ) ;
#33755=DIRECTION ( 'NONE',  ( -0.000000000000000000, 0.3420201433256694346, -0.9396926207859080948 ) ) ;
#33756=ORIENTED_EDGE ( 'NONE', *, *, #47288, .T. ) ;
#33757=CARTESIAN_POINT ( 'NONE',  ( 10.61538461538461675, -2.499999999999998668, 29.50000000000001066 ) ) ;
#33759=CARTESIAN_POINT ( 'NONE',  ( 0.3954550505825801809, -2.721908614388771408, 31.22303859784724267 ) ) ;
#33760=ORIENTED_EDGE ( 'NONE', *, *, #3526, .T. ) ;
#33761=CARTESIAN_POINT ( 'NONE',  ( 3.230769230769231726, -4.786620604624113540, 33.94971097300155094 ) ) ;
#33762=CARTESIAN_POINT ( 'NONE',  ( 2.307692307692186251, -8.656820664282941280, 34.87096338111179961 ) ) ;
#33764=FACE_OUTER_BOUND ( 'NONE', #80954, .T. ) ;
#33765=EDGE_LOOP ( 'NONE', ( #71648, #23787 ) ) ;
#33766=EDGE_CURVE ( 'NONE', #22482, #58674, #78329, .T. ) ;
#33767=VERTEX_POINT ( 'NONE', #13971 ) ;
#33768=ORIENTED_EDGE ( 'NONE', *, *, #74852, .T. ) ;
#33769=CARTESIAN_POINT ( 'NONE',  ( -17.86947456176635640, -5.070358843744208421, 34.40418822224088302 ) ) ;
#33770=CARTESIAN_POINT ( 'NONE',  ( -5.076923076923075762, -6.435427911321262684, 35.78748833219616898 ) ) ;
#33772=DIRECTION ( 'NONE',  ( -0.000000000000000000, -0.9396926207859092051, -0.3420201433256662704 ) ) ;
#33773=CARTESIAN_POINT ( 'NONE',  ( -1.384615384615383471, -11.35647404775217417, 33.31231777344666511 ) ) ;
#33774=EDGE_CURVE ( 'NONE', #56271, #33346, #64448, .T. ) ;
#33775=CARTESIAN_POINT ( 'NONE',  ( -2.557715544985271094, -5.851115903089112003, 34.47074536777953568 ) ) ;
#33776=CARTESIAN_POINT ( 'NONE',  ( -4.403869391139119571, -6.695914987888143877, 34.68535235679833306 ) ) ;
#33777=CARTESIAN_POINT ( 'NONE',  ( 13.63466969625370062, -3.136992222400443175, 32.19305428654138979 ) ) ;
#33778=CARTESIAN_POINT ( 'NONE',  ( 16.08857615328983925, -12.70778746994557551, 30.41441678777548319 ) ) ;
#33779=AXIS2_PLACEMENT_3D ( 'NONE', #37228, #84992, #31370 ) ;
#33781=VERTEX_POINT ( 'NONE', #8109 ) ;
#33782=CARTESIAN_POINT ( 'NONE',  ( -17.14300648787895653, -9.780366693483667717, 34.19971097300155805 ) ) ;
#33784=DIRECTION ( 'NONE',  ( -0.000000000000000000, -0.7660444431189791237, -0.6427876096865379196 ) ) ;
#33785=CYLINDRICAL_SURFACE ( 'NONE', #25165, 0.2500000000000012212 ) ;
#33786=ORIENTED_EDGE ( 'NONE', *, *, #66473, .F. ) ;
#33787=CARTESIAN_POINT ( 'NONE',  ( 14.30769230769231015, -11.91647553114624181, 32.58852847137148245 ) ) ;
#33788=ORIENTED_EDGE ( 'NONE', *, *, #20145, .F. ) ;
#33789=CARTESIAN_POINT ( 'NONE',  ( 17.29970274590113632, -9.418065098278011860, 34.63729479722530158 ) ) ;
#33790=ORIENTED_EDGE ( 'NONE', *, *, #78457, .T. ) ;
#33791=CARTESIAN_POINT ( 'NONE',  ( -10.83821130786361664, -7.369208160676171460, 34.74850200257122879 ) ) ;
#33792=EDGE_CURVE ( 'NONE', #17306, #61727, #35581, .T. ) ;
#33793=ORIENTED_EDGE ( 'NONE', *, *, #20448, .T. ) ;
#33795=CARTESIAN_POINT ( 'NONE',  ( -8.899377978668987055, -2.882441371585227508, 31.66841991370172238 ) ) ;
#33796=FACE_BOUND ( 'NONE', #75733, .T. ) ;
#33797=CARTESIAN_POINT ( 'NONE',  ( 5.750023255951410839, -2.318417181685854978, 30.59732222474233865 ) ) ;
#33798=CARTESIAN_POINT ( 'NONE',  ( 15.90386940979756503, -3.436278759898155677, 33.07459398097509506 ) ) ;
#33801=CARTESIAN_POINT ( 'NONE',  ( 10.61538461538449418, -10.33852847137269571, 34.16647553114546554 ) ) ;
#33802=CARTESIAN_POINT ( 'NONE',  ( 10.61538461538449596, -2.892918686052165622, 31.69288490824153470 ) ) ;
#33803=CARTESIAN_POINT ( 'NONE',  ( -7.976844449264155479, -9.084618155246140248, 34.75535874321725771 ) ) ;
#33804=DIRECTION ( 'NONE',  ( -0.000000000000000000, -0.9396926207859093161, -0.3420201433256663259 ) ) ;
#33805=ORIENTED_EDGE ( 'NONE', *, *, #10063, .F. ) ;
#33806=ORIENTED_EDGE ( 'NONE', *, *, #23416, .T. ) ;
#33807=EDGE_CURVE ( 'NONE', #77497, #68692, #56960, .T. ) ;
#33808=AXIS2_PLACEMENT_3D ( 'NONE', #72045, #85132, #58520 ) ;
#33809=FACE_OUTER_BOUND ( 'NONE', #1570, .T. ) ;
#33810=CARTESIAN_POINT ( 'NONE',  ( 2.530471848960718972, -10.81320215134717344, 33.49497208177562868 ) ) ;
#33811=CARTESIAN_POINT ( 'NONE',  ( -3.903846153844733102, -7.500000000000154543, 35.00000000000007105 ) ) ;
#33812=CARTESIAN_POINT ( 'NONE',  ( -3.930833309752757909, -9.172514111537584114, 34.72667873470787470 ) ) ;
#33814=CARTESIAN_POINT ( 'NONE',  ( 13.60762673622823726, -11.24521262558773493, 33.06293181088029343 ) ) ;
#33815=ORIENTED_EDGE ( 'NONE', *, *, #60482, .F. ) ;
#33816=CARTESIAN_POINT ( 'NONE',  ( -11.76138775597768138, -12.15238873228292071, 31.58232369045353849 ) ) ;
#33817=CARTESIAN_POINT ( 'NONE',  ( 9.692307692307570832, -3.643525952248795718, 33.31231777344771672 ) ) ;
#33818=CARTESIAN_POINT ( 'NONE',  ( -3.480792454990689233, -11.56360843649121861, 33.07473185843129926 ) ) ;
#33819=CARTESIAN_POINT ( 'NONE',  ( -3.361459833879538728, -12.62707690430377383, 30.88035979386743435 ) ) ;
#33820=EDGE_LOOP ( 'NONE', ( #19027, #18663, #41221, #8311 ) ) ;
#33824=CARTESIAN_POINT ( 'NONE',  ( 10.48469401227430708, -3.957541250942358424, 33.62499894934981626 ) ) ;
#33825=ORIENTED_EDGE ( 'NONE', *, *, #71210, .T. ) ;
#33826=CARTESIAN_POINT ( 'NONE',  ( 3.930361229281821966, -11.60425143139329940, 33.02411095842164457 ) ) ;
#33827=CARTESIAN_POINT ( 'NONE',  ( 15.10062202133100939, -9.418419913701741919, 34.36755862841477693 ) ) ;
#33828=CARTESIAN_POINT ( 'NONE',  ( -5.143006487878958310, -4.098570777380720287, 33.41473453929634729 ) ) ;
#33829=EDGE_CURVE ( 'NONE', #79174, #60125, #83785, .T. ) ;
#33831=CARTESIAN_POINT ( 'NONE',  ( 14.53047184896071542, -4.387253974876679230, 33.66317474335728832 ) ) ;
#33832=EDGE_LOOP ( 'NONE', ( #16945, #14899 ) ) ;
#33833=CARTESIAN_POINT ( 'NONE',  ( 4.153846153846468603, -2.255955759149395501, 30.00000000000324363 ) ) ;
#33834=CARTESIAN_POINT ( 'NONE',  ( -13.31854703361294767, -4.098570777380720287, 33.41473453929635440 ) ) ;
#33835=VERTEX_POINT ( 'NONE', #24719 ) ;
#33836=CARTESIAN_POINT ( 'NONE',  ( -5.076923076923075762, -2.292212530054420494, 30.41441678777542634 ) ) ;
#33837=CARTESIAN_POINT ( 'NONE',  ( -2.557715544985271094, -9.271318131107980420, 34.42618302367067429 ) ) ;
#33838=CYLINDRICAL_SURFACE ( 'NONE', #14180, 0.2500000000000002220 ) ;
#33839=B_SPLINE_CURVE_WITH_KNOTS ( 'NONE', 3,
 ( #24192, #30074, #64728, #84591, #63853, #23306, #29638, #3027, #72821, #78249 ),
 .UNSPECIFIED., .F., .F.,
 ( 4, 2, 2, 2, 4 ),
 ( 0.0007817359430256293554, 0.0009771253907249941549, 0.001172514838424358954, 0.001367904286123723537, 0.001563293733823095276 ),
 .UNSPECIFIED. ) ;
#33840=CARTESIAN_POINT ( 'NONE',  ( 9.915087233576100445, -10.81320215134717344, 33.49497208177562868 ) ) ;
#33841=DIRECTION ( 'NONE',  ( 0.000000000000000000, 0.9396926207859126468, -0.3420201433256571111 ) ) ;
#33842=AXIS2_PLACEMENT_3D ( 'NONE', #83238, #20639, #83692 ) ;
#33843=CARTESIAN_POINT ( 'NONE',  ( -8.546217925137375104, -9.172514111537584114, 34.72667873470787470 ) ) ;
#33844=CARTESIAN_POINT ( 'NONE',  ( -3.361460697436787104, -6.413092428213692742, 34.63065189839063152 ) ) ;
#33846=ORIENTED_EDGE ( 'NONE', *, *, #34494, .F. ) ;
#33847=B_SPLINE_CURVE_WITH_KNOTS ( 'NONE', 3,
 ( #28523, #22205, #84812, #84363, #16333, #28980, #43362, #36176, #2799, #8256 ),
 .UNSPECIFIED., .F., .F.,
 ( 4, 2, 2, 2, 4 ),
 ( 0.000000000000000000, 0.0001954339881912776238, 0.0003908679763825552477, 0.0005863019645738329257, 0.0007817359527651104954 ),
 .UNSPECIFIED. ) ;
#33848=CARTESIAN_POINT ( 'NONE',  ( -7.173053667125515176, -10.82459398097509684, 33.81372124010185587 ) ) ;
#33849=CARTESIAN_POINT ( 'NONE',  ( 12.46153846153846168, -4.661471528628507777, 34.16647553114623292 ) ) ;
#33850=VERTEX_POINT ( 'NONE', #44973 ) ;
#33851=EDGE_LOOP ( 'NONE', ( #45380, #52767, #72850, #22942, #7002, #42246 ) ) ;
#33852=CARTESIAN_POINT ( 'NONE',  ( 2.057692307692309708, -7.500000000000001776, 35.00000000000000000 ) ) ;
#33853=CARTESIAN_POINT ( 'NONE',  ( -5.207614543590634248, -6.413092428213692742, 34.63065189839063152 ) ) ;
#33854=VECTOR ( 'NONE', #51699, 1000.000000000000114 ) ;
#33855=CARTESIAN_POINT ( 'NONE',  ( 1.384615384615386802, -3.513871655860378418, 32.76840700105978499 ) ) ;
#33856=CARTESIAN_POINT ( 'NONE',  ( 7.146088274689773812, -5.667800583137508674, 34.40243808032445827 ) ) ;
#33857=CARTESIAN_POINT ( 'NONE',  ( -14.43784027742400866, -3.069018819979302926, 32.56621877034667278 ) ) ;
#33858=ORIENTED_EDGE ( 'NONE', *, *, #3092, .T. ) ;
#33859=CARTESIAN_POINT ( 'NONE',  ( 12.39628852976437656, -2.255955759149247619, 30.00000000000013856 ) ) ;
#33860=EDGE_CURVE ( 'NONE', #45495, #67170, #27992, .T. ) ;
#33861=CARTESIAN_POINT ( 'NONE',  ( -14.55771554498527287, -2.823816976329319051, 31.52131813110795733 ) ) ;
#33862=DIRECTION ( 'NONE',  ( -0.000000000000000000, 0.9396926207859093161, -0.3420201433256663259 ) ) ;
#33863=ORIENTED_EDGE ( 'NONE', *, *, #86036, .T. ) ;
#33864=CARTESIAN_POINT ( 'NONE',  ( -9.019230769230768274, -7.433932668274256805, 35.00000000000000711 ) ) ;
#33866=ORIENTED_EDGE ( 'NONE', *, *, #22430, .T. ) ;
#33868=CARTESIAN_POINT ( 'NONE',  ( 11.28848479441295005, -2.544273027872575366, 31.48422191005632342 ) ) ;
#33869=ORIENTED_EDGE ( 'NONE', *, *, #69907, .F. ) ;
#33870=EDGE_CURVE ( 'NONE', #68708, #83978, #48362, .T. ) ;
#33871=CARTESIAN_POINT ( 'NONE',  ( 0.6843180028068700516, -4.387253974876678342, 33.66317474335728832 ) ) ;
#33872=CARTESIAN_POINT ( 'NONE',  ( 16.15384615384615330, -12.78798330534102945, 29.74999999999997868 ) ) ;
#33873=CARTESIAN_POINT ( 'NONE',  ( 1.134592147322421418, -4.335965774309649134, 33.62209801155881905 ) ) ;
#33874=VECTOR ( 'NONE', #51546, 1000.000000000000000 ) ;
#33875=CARTESIAN_POINT ( 'NONE',  ( 11.31553457955468645, -12.38737895849757820, 31.66785238281580206 ) ) ;
#33876=DIRECTION ( 'NONE',  ( 0.000000000000000000, 0.9396926207859126468, 0.3420201433256571111 ) ) ;
#33877=B_SPLINE_CURVE_WITH_KNOTS ( 'NONE', 3,
 ( #80437, #86312, #16942, #85851, #3861, #79980, #66007, #24586, #87645, #73682 ),
 .UNSPECIFIED., .F., .F.,
 ( 4, 2, 2, 2, 4 ),
 ( 0.000000000000000000, 0.0001954311564186871184, 0.0003908623128373742367, 0.0005862934692560614093, 0.0007817246256747484735 ),
 .UNSPECIFIED. ) ;
#33878=ORIENTED_EDGE ( 'NONE', *, *, #52924, .F. ) ;
#33879=FACE_BOUND ( 'NONE', #48413, .T. ) ;
#33880=VERTEX_POINT ( 'NONE', #52177 ) ;
#33881=CARTESIAN_POINT ( 'NONE',  ( -8.546451227962359454, -4.387253974876679230, 33.66317474335728832 ) ) ;
#33882=EDGE_CURVE ( 'NONE', #47735, #64358, #7525, .T. ) ;
#33883=CARTESIAN_POINT ( 'NONE',  ( -10.61538461538473577, -10.33852847137269571, 34.16647553114546554 ) ) ;
#33884=CARTESIAN_POINT ( 'NONE',  ( 18.25005441991345734, -6.523592122091590895, 34.90882529074906415 ) ) ;
#33885=EDGE_CURVE ( 'NONE', #82401, #38474, #44524, .T. ) ;
#33886=FACE_OUTER_BOUND ( 'NONE', #31223, .T. ) ;
#33887=CARTESIAN_POINT ( 'NONE',  ( -11.53846153846165912, -2.625532179533778709, 30.86335684631627174 ) ) ;
#33888=ORIENTED_EDGE ( 'NONE', *, *, #82321, .F. ) ;
#33889=VERTEX_POINT ( 'NONE', #65688 ) ;
#33890=ORIENTED_EDGE ( 'NONE', *, *, #72273, .F. ) ;
#33891=ORIENTED_EDGE ( 'NONE', *, *, #50711, .T. ) ;
#33892=EDGE_CURVE ( 'NONE', #80428, #25943, #23623, .T. ) ;
#33894=CARTESIAN_POINT ( 'NONE',  ( -17.07692307692319744, -10.33852847137269571, 34.16647553114546554 ) ) ;
#33895=CARTESIAN_POINT ( 'NONE',  ( -17.07692307692277112, -2.506253911140615021, 30.00000000000323297 ) ) ;
#33897=CARTESIAN_POINT ( 'NONE',  ( 6.000000000000001776, -12.10708131394839349, 31.69288490824020244 ) ) ;
#33898=EDGE_LOOP ( 'NONE', ( #13009, #87733, #1786, #1853 ) ) ;
#33899=CARTESIAN_POINT ( 'NONE',  ( 11.47319109250076430, -2.625532179533445198, 30.86335684631481513 ) ) ;
#33900=CARTESIAN_POINT ( 'NONE',  ( -2.557669038634660996, -4.943428324936578910, 34.04746400365624481 ) ) ;
#33901=CARTESIAN_POINT ( 'NONE',  ( -2.177166605928740672, -3.816742781228458448, 33.13167719472716044 ) ) ;
#33903=VERTEX_POINT ( 'NONE', #19300 ) ;
#33905=EDGE_LOOP ( 'NONE', ( #51346, #81857 ) ) ;
#33906=ORIENTED_EDGE ( 'NONE', *, *, #34392, .T. ) ;
#33908=ADVANCED_FACE ( 'NONE', ( #53065 ), #66139, .F. ) ;
#33909=CARTESIAN_POINT ( 'NONE',  ( 1.607626736228236819, -5.667800583137508674, 34.40243808032445827 ) ) ;
#33910=LINE ( 'NONE', #48306, #5992 ) ;
#33911=CARTESIAN_POINT ( 'NONE',  ( -1.384615384615383471, -1.215029322943914858, 32.30358669280327177 ) ) ;
#33912=CARTESIAN_POINT ( 'NONE',  ( -10.83886955910856464, -3.754499324213721234, 33.06261337010820256 ) ) ;
#33913=FACE_BOUND ( 'NONE', #18728, .T. ) ;
#33914=EDGE_LOOP ( 'NONE', ( #11221, #33825, #30287, #41925 ) ) ;
#33915=EDGE_CURVE ( 'NONE', #57709, #19174, #45870, .T. ) ;
#33916=DIRECTION ( 'NONE',  ( 0.000000000000000000, 0.9848077530122072432, 0.1736481776669354937 ) ) ;
#33917=CARTESIAN_POINT ( 'NONE',  ( -5.076923076923075762, -12.29105614889573062, 35.45975837776705220 ) ) ;
#33918=CARTESIAN_POINT ( 'NONE',  ( 3.007843013253084674, -10.61292498521070549, 33.66303323003028680 ) ) ;
#33919=ORIENTED_EDGE ( 'NONE', *, *, #68976, .F. ) ;
#33920=CARTESIAN_POINT ( 'NONE',  ( 17.20744851515672025, -5.915461855592777596, 34.75538340440931506 ) ) ;
#33921=EDGE_LOOP ( 'NONE', ( #84544, #13507, #80895, #70250 ) ) ;
#33922=FACE_BOUND ( 'NONE', #28351, .T. ) ;
#33923=LINE ( 'NONE', #82580, #74953 ) ;
#33924=VERTEX_POINT ( 'NONE', #80110 ) ;
#33925=AXIS2_PLACEMENT_3D ( 'NONE', #8040, #42716, #34623 ) ;
#33926=CARTESIAN_POINT ( 'NONE',  ( -6.923076923076922462, -9.905515769479276145, 34.41647553114623292 ) ) ;
#33928=DIRECTION ( 'NONE',  ( 0.000000000000000000, 0.3420201433256610524, 0.9396926207859113145 ) ) ;
#33930=CARTESIAN_POINT ( 'NONE',  ( -8.769230769230768274, -3.322132147404559976, 32.92929555188717927 ) ) ;
#33931=CARTESIAN_POINT ( 'NONE',  ( -4.153846153846152411, -1.129524287112498415, 32.06866353760679544 ) ) ;
#33932=CARTESIAN_POINT ( 'NONE',  ( -16.37733109757010652, -12.44517049084099725, 30.48991314939691932 ) ) ;
#33933=EDGE_CURVE ( 'NONE', #39364, #64018, #52627, .T. ) ;
#33934=CARTESIAN_POINT ( 'NONE',  ( -9.561515884482906458, -2.541949514083464479, 30.39797389878540557 ) ) ;
#33935=ORIENTED_EDGE ( 'NONE', *, *, #34268, .T. ) ;
#33938=CARTESIAN_POINT ( 'NONE',  ( -4.946397638689432164, -5.070358843744210198, 34.40418822224088302 ) ) ;
#33939=CARTESIAN_POINT ( 'NONE',  ( -15.93083330975275658, -10.01129605718032423, 34.36064277460058491 ) ) ;
#33940=CARTESIAN_POINT ( 'NONE',  ( 1.450682717965462221, -2.833524468853757750, 32.15551576947925838 ) ) ;
#33942=CARTESIAN_POINT ( 'NONE',  ( 2.372947447205146609, -10.33852847137154107, 34.16647553114620450 ) ) ;
#33944=CARTESIAN_POINT ( 'NONE',  ( -13.25382357679059986, -4.809403383903225304, 33.96459661697924304 ) ) ;
#33945=CARTESIAN_POINT ( 'NONE',  ( 13.60762673622823904, -12.39991518177334129, 30.74647679643404530 ) ) ;
#33946=CARTESIAN_POINT ( 'NONE',  ( -13.13466986626724164, -3.712312575010499049, 33.01462480002815170 ) ) ;
#33948=CARTESIAN_POINT ( 'NONE',  ( 8.769230769231082689, -2.255955759149395501, 30.00000000000324363 ) ) ;
#33950=CARTESIAN_POINT ( 'NONE',  ( -12.23875892027005108, -11.41317474335729543, 32.86274602512330034 ) ) ;
#33952=ORIENTED_EDGE ( 'NONE', *, *, #78671, .F. ) ;
#33954=ORIENTED_EDGE ( 'NONE', *, *, #8448, .T. ) ;
#33957=ORIENTED_EDGE ( 'NONE', *, *, #65614, .F. ) ;
#33958=CARTESIAN_POINT ( 'NONE',  ( 14.17700084102474989, -8.147922237126337563, 34.70805685702651999 ) ) ;
#33961=CARTESIAN_POINT ( 'NONE',  ( -11.28851612908349544, -10.18230066228895758, 34.26354781536631577 ) ) ;
#33962=DIRECTION ( 'NONE',  ( -0.000000000000000000, 0.3420201433256694346, -0.9396926207859080948 ) ) ;
#33963=CARTESIAN_POINT ( 'NONE',  ( 1.384615384615264011, -2.657715359629662544, 31.77849191805970364 ) ) ;
#33964=LINE ( 'NONE', #60551, #41651 ) ;
#33967=VECTOR ( 'NONE', #61847, 1000.000000000000227 ) ;
#33968=DIRECTION ( 'NONE',  ( -0.000000000000000000, 1.000000000000000000, 3.491481338843133355E-15 ) ) ;
#33969=CARTESIAN_POINT ( 'NONE',  ( -13.31854703361294590, -6.386643153685127139, 34.62446782046654192 ) ) ;
#33970=FACE_OUTER_BOUND ( 'NONE', #9180, .T. ) ;
#33971=B_SPLINE_CURVE_WITH_KNOTS ( 'NONE', 3,
 ( #42030, #23077, #50535, #23505, #4122, #39269, #10454, #66726, #58177, #3240 ),
 .UNSPECIFIED., .F., .F.,
 ( 4, 2, 2, 2, 4 ),
 ( 0.0007817246256747519429, 0.0009771112852218959231, 0.001172497944769039686, 0.001367884604316183667, 0.001563271263863327647 ),
 .UNSPECIFIED. ) ;
#33973=B_SPLINE_CURVE_WITH_KNOTS ( 'NONE', 3,
 ( #74601, #53425, #59301, #87245, #25077, #72811, #40380, #5690, #12020, #52540 ),
 .UNSPECIFIED., .F., .F.,
 ( 4, 2, 2, 2, 4 ),
 ( 0.0007817246256747503166, 0.0009771112852218946220, 0.001172497944769039036, 0.001367884604316183233, 0.001563271263863327647 ),
 .UNSPECIFIED. ) ;
#33974=ORIENTED_EDGE ( 'NONE', *, *, #53015, .T. ) ;
#33975=ORIENTED_EDGE ( 'NONE', *, *, #37289, .F. ) ;
#33976=CARTESIAN_POINT ( 'NONE',  ( -6.923076923076607159, -2.255955759149395501, 30.00000000000324363 ) ) ;
#33977=CARTESIAN_POINT ( 'NONE',  ( 0.6845513056318550671, -11.98016756924214832, 32.48728574198911190 ) ) ;
#33978=CARTESIAN_POINT ( 'NONE',  ( 6.923076923076924238, -8.973038597847269315, 34.52809138561121927 ) ) ;
#33979=LINE ( 'NONE', #41631, #19655 ) ;
#33980=EDGE_CURVE ( 'NONE', #31080, #19898, #18215, .T. ) ;
#33981=AXIS2_PLACEMENT_3D ( 'NONE', #72782, #30469, #64686 ) ;
#33982=CARTESIAN_POINT ( 'NONE',  ( 14.17754433796061875, -3.625366637846545892, 33.29286588640298561 ) ) ;
#33983=CARTESIAN_POINT ( 'NONE',  ( 11.53846153846153832, -3.937682226553329556, 33.60647404775216529 ) ) ;
#33984=EDGE_CURVE ( 'NONE', #16191, #70346, #60274, .T. ) ;
#33985=CARTESIAN_POINT ( 'NONE',  ( -6.923076923076922462, -3.050289026998446396, 32.03036669348365706 ) ) ;
#33987=CARTESIAN_POINT ( 'NONE',  ( -6.673022611438605978, -9.943054286541403997, 34.11300777759954883 ) ) ;
#33988=EDGE_LOOP ( 'NONE', ( #75900, #72702, #36560, #65311 ) ) ;
#33989=ADVANCED_FACE ( 'NONE', ( #40031 ), #5785, .F. ) ;
#33990=DIRECTION ( 'NONE',  ( -0.000000000000000000, 0.9848077530122085754, -0.1736481776669273613 ) ) ;
#33991=CARTESIAN_POINT ( 'NONE',  ( 3.903846153846154632, -7.500000000000001776, 35.00000000000000000 ) ) ;
#33993=CARTESIAN_POINT ( 'NONE',  ( 14.17700084102474989, -4.809359713505814149, 33.96456829005828837 ) ) ;
#33995=DIRECTION ( 'NONE',  ( -1.000000000000000000, 0.000000000000000000, 0.000000000000000000 ) ) ;
#33998=EDGE_LOOP ( 'NONE', ( #19390, #70091, #79522, #72635 ) ) ;
#33999=VERTEX_POINT ( 'NONE', #38676 ) ;
#34000=AXIS2_PLACEMENT_3D ( 'NONE', #79250, #45000, #24743 ) ;
#34001=CARTESIAN_POINT ( 'NONE',  ( -6.000000000000121680, -5.094484230521993062, 34.41647553114689373 ) ) ;
#34002=B_SPLINE_CURVE_WITH_KNOTS ( 'NONE', 3,
 ( #12702, #87954, #68524, #39297, #74402, #75293, #13583, #26213, #66753, #46486 ),
 .UNSPECIFIED., .F., .F.,
 ( 4, 2, 2, 2, 4 ),
 ( 0.000000000000000000, 0.0001954311564186876876, 0.0003908623128373753751, 0.0005862934692560630356, 0.0007817246256747507503 ),
 .UNSPECIFIED. ) ;
#34003=CARTESIAN_POINT ( 'NONE',  ( 4.853438133199127869, -10.81261337010820256, 33.49550067578627477 ) ) ;
#34004=EDGE_CURVE ( 'NONE', #24055, #84960, #26949, .T. ) ;
#34005=CARTESIAN_POINT ( 'NONE',  ( 16.15384615384646949, -2.255955759149395501, 30.00000000000324363 ) ) ;
#34007=CARTESIAN_POINT ( 'NONE',  ( -15.00798956179116317, -9.418065098278013636, 34.63729479722530158 ) ) ;
#34008=CARTESIAN_POINT ( 'NONE',  ( -15.36145983387953962, -2.494641256782728966, 31.33461815524612959 ) ) ;
#34009=ORIENTED_EDGE ( 'NONE', *, *, #23915, .F. ) ;
#34011=EDGE_LOOP ( 'NONE', ( #14260, #22698, #22165, #81745, #86065, #16843 ) ) ;
#34012=CARTESIAN_POINT ( 'NONE',  ( -10.36543909703646982, -11.86320923018887541, 32.19269448109604781 ) ) ;
#34013=EDGE_CURVE ( 'NONE', #61361, #61570, #82667, .T. ) ;
#34014=ORIENTED_EDGE ( 'NONE', *, *, #32103, .F. ) ;
#34016=CARTESIAN_POINT ( 'NONE',  ( -12.21148404162500967, -12.01375889529407281, 32.43194544308182969 ) ) ;
#34017=VECTOR ( 'NONE', #58652, 1000.000000000000000 ) ;
#34019=ORIENTED_EDGE ( 'NONE', *, *, #31158, .F. ) ;
#34021=EDGE_CURVE ( 'NONE', #17811, #42433, #4156, .T. ) ;
#34022=LINE ( 'NONE', #5223, #39716 ) ;
#34024=CARTESIAN_POINT ( 'NONE',  ( 7.976945653978634532, -12.11778462344221197, 31.66786338562085135 ) ) ;
#34025=FACE_BOUND ( 'NONE', #85185, .T. ) ;
#34026=CARTESIAN_POINT ( 'NONE',  ( 7.846153846153846700, -12.78798330534102945, 29.74999999999997868 ) ) ;
#34027=CARTESIAN_POINT ( 'NONE',  ( -14.08431636699412337, -2.501478030877323455, 29.88021232661721172 ) ) ;
#34028=ORIENTED_EDGE ( 'NONE', *, *, #20139, .T. ) ;
#34030=AXIS2_PLACEMENT_3D ( 'NONE', #24430, #86610, #46494 ) ;
#34031=CARTESIAN_POINT ( 'NONE',  ( 8.835298102580845025, -8.164416787775445883, 34.95778746994558617 ) ) ;
#34032=CARTESIAN_POINT ( 'NONE',  ( 16.15384615384615330, -2.538708090699994813, 30.37095296980875503 ) ) ;
#34033=CARTESIAN_POINT ( 'NONE',  ( 15.48082365068268373, -6.523592122091592671, 34.90882529074906415 ) ) ;
#34034=EDGE_CURVE ( 'NONE', #83533, #15199, #24577, .T. ) ;
#34035=ORIENTED_EDGE ( 'NONE', *, *, #13651, .F. ) ;
#34036=B_SPLINE_CURVE_WITH_KNOTS ( 'NONE', 3,
 ( #66866, #45248, #17796, #18237, #11033, #60099, #79039, #10590, #5607, #73638 ),
 .UNSPECIFIED., .F., .F.,
 ( 4, 2, 2, 2, 4 ),
 ( 0.0007817246256747460882, 0.0009771112852218892010, 0.001172497944769032314, 0.001367884604316175210, 0.001563271263863318323 ),
 .UNSPECIFIED. ) ;
#34037=CARTESIAN_POINT ( 'NONE',  ( 16.40384615384759215, -7.500000000000155431, 34.75000000000007105 ) ) ;
#34038=CARTESIAN_POINT ( 'NONE',  ( -7.715628144390285215, -11.46989282347013095, 32.79007818306219946 ) ) ;
#34039=CARTESIAN_POINT ( 'NONE',  ( 4.219101293358989757, -11.67786785259547777, 32.92929555188713664 ) ) ;
#34040=CARTESIAN_POINT ( 'NONE',  ( -2.177166869458661225, -9.503571793651733657, 34.60286762892837942 ) ) ;
#34041=EDGE_CURVE ( 'NONE', #83971, #56983, #27824, .T. ) ;
#34043=ADVANCED_FACE ( 'NONE', ( #22395 ), #42678, .F. ) ;
#34044=FACE_BOUND ( 'NONE', #16762, .T. ) ;
#34046=CARTESIAN_POINT ( 'NONE',  ( 11.53846153846141753, -12.46129190930018460, 30.37095296980731973 ) ) ;
#34047=CARTESIAN_POINT ( 'NONE',  ( -7.146561866800873020, -12.24155766932282496, 31.33739205006857986 ) ) ;
#34048=CARTESIAN_POINT ( 'NONE',  ( -8.769230769230768274, -11.69971097300155272, 32.46337939537588113 ) ) ;
#34049=CARTESIAN_POINT ( 'NONE',  ( 6.923076923076800782, -2.657715359629662988, 31.77849191805970364 ) ) ;
#34050=DIRECTION ( 'NONE',  ( -0.000000000000000000, 0.9848077530122085754, -0.1736481776669273613 ) ) ;
#34054=CARTESIAN_POINT ( 'NONE',  ( 1.384615384615386802, -12.10708131394839349, 31.69288490824020244 ) ) ;
#34056=CARTESIAN_POINT ( 'NONE',  ( -15.00798968950081758, -4.387253974876679230, 33.66317474335728832 ) ) ;
#34057=VECTOR ( 'NONE', #76746, 999.9999999999998863 ) ;
#34058=ORIENTED_EDGE ( 'NONE', *, *, #84303, .T. ) ;
#34060=DIRECTION ( 'NONE',  ( 0.000000000000000000, 0.8660254037844377084, -0.5000000000000015543 ) ) ;
#34061=CARTESIAN_POINT ( 'NONE',  ( -4.826977667545033768, -9.357781135181031829, 34.66075350412533851 ) ) ;
#34062=ORIENTED_EDGE ( 'NONE', *, *, #83178, .T. ) ;
#34065=CARTESIAN_POINT ( 'NONE',  ( -15.23076923076922995, -9.058645607665452459, 34.76329471203371924 ) ) ;
#34066=CARTESIAN_POINT ( 'NONE',  ( -7.173100147298380413, -12.68155406624981119, 30.59749803192733708 ) ) ;
#34067=VECTOR ( 'NONE', #8698, 1000.000000000000000 ) ;
#34068=CARTESIAN_POINT ( 'NONE',  ( 17.07692307692295586, -12.46129190930018460, 30.37095296980731973 ) ) ;
#34069=CARTESIAN_POINT ( 'NONE',  ( 1.134592160393929072, -4.931416488878823223, 34.32920672191015399 ) ) ;
#34070=CARTESIAN_POINT ( 'NONE',  ( -1.318548051265308274, -6.343179335718451384, 34.87096338111212646 ) ) ;
#34071=CARTESIAN_POINT ( 'NONE',  ( -24.00000000000000000, -5.499999999999981348, 27.25000000000000000 ) ) ;
#34073=CARTESIAN_POINT ( 'NONE',  ( 9.469429009879048564, -7.630691491037285168, 34.74850469731152458 ) ) ;
#34074=AXIS2_PLACEMENT_3D ( 'NONE', #4369, #86365, #24637 ) ;
#34075=ORIENTED_EDGE ( 'NONE', *, *, #45316, .T. ) ;
#34076=LINE ( 'NONE', #21893, #19103 ) ;
#34078=ADVANCED_FACE ( 'NONE', ( #28263 ), #13424, .F. ) ;
#34080=DIRECTION ( 'NONE',  ( -0.000000000000000000, -0.000000000000000000, -1.000000000000000000 ) ) ;
#34081=VERTEX_POINT ( 'NONE', #1684 ) ;
#34082=CARTESIAN_POINT ( 'NONE',  ( 6.923076923076802558, -8.613356846316285953, 34.62446782046622218 ) ) ;
#34083=CARTESIAN_POINT ( 'NONE',  ( -0.2115929431903202929, -10.05730279482229683, 34.04704008940765902 ) ) ;
#34084=CARTESIAN_POINT ( 'NONE',  ( -16.82692307692300915, -7.434744429011174383, 34.75000000000000711 ) ) ;
#34085=ORIENTED_EDGE ( 'NONE', *, *, #61984, .F. ) ;
#34086=DIRECTION ( 'NONE',  ( -0.000000000000000000, -0.9396926207859093161, -0.3420201433256663259 ) ) ;
#34087=CARTESIAN_POINT ( 'NONE',  ( -14.98071481085577972, -12.01375889529407281, 32.43194544308182969 ) ) ;
#34088=CARTESIAN_POINT ( 'NONE',  ( 16.08857570788537572, -9.442884908240170461, 34.35708131394840592 ) ) ;
#34089=CARTESIAN_POINT ( 'NONE',  ( -9.442253272394236063, -2.544122305571458575, 31.48381861865057729 ) ) ;
#34090=CARTESIAN_POINT ( 'NONE',  ( -18.06608341095587278, -12.10708131394839349, 31.69288490824020244 ) ) ;
#34093=VERTEX_POINT ( 'NONE', #76904 ) ;
#34094=EDGE_LOOP ( 'NONE', ( #23042, #31780 ) ) ;
#34096=AXIS2_PLACEMENT_3D ( 'NONE', #56142, #68771, #7520 ) ;
#34098=CARTESIAN_POINT ( 'NONE',  ( -9.469296340694842939, -3.105924265160262543, 32.13625925475356127 ) ) ;
#34099=DIRECTION ( 'NONE',  ( 0.000000000000000000, 0.4999999999999985567, 0.8660254037844395958 ) ) ;
#34100=VECTOR ( 'NONE', #37742, 1000.000000000000114 ) ;
#34101=CARTESIAN_POINT ( 'NONE',  ( 9.757563263583717728, -5.219633306516380244, 34.19971097300157936 ) ) ;
#34102=CARTESIAN_POINT ( 'NONE',  ( -8.769230769230768274, -13.63283147151868846, 33.57946703557072254 ) ) ;
#34103=EDGE_CURVE ( 'NONE', #76906, #7653, #56628, .T. ) ;
#34104=CARTESIAN_POINT ( 'NONE',  ( 16.08776274289027342, -4.786620604624113540, 33.94971097300155805 ) ) ;
#34105=ORIENTED_EDGE ( 'NONE', *, *, #32678, .F. ) ;
#34106=ORIENTED_EDGE ( 'NONE', *, *, #6293, .F. ) ;
#34107=B_SPLINE_CURVE_WITH_KNOTS ( 'NONE', 3,
 ( #45250, #25880, #38963, #86718, #66868, #5163, #51540, #59212, #4270, #18689 ),
 .UNSPECIFIED., .F., .F.,
 ( 4, 2, 2, 2, 4 ),
 ( 0.0007817246256747451124, 0.0009771112852218881168, 0.001172497944769031230, 0.001367884604316174126, 0.001563271263863317238 ),
 .UNSPECIFIED. ) ;
#34108=ORIENTED_EDGE ( 'NONE', *, *, #3163, .T. ) ;
#34109=FACE_OUTER_BOUND ( 'NONE', #52381, .T. ) ;
#34110=ORIENTED_EDGE ( 'NONE', *, *, #7982, .F. ) ;
#34111=CARTESIAN_POINT ( 'NONE',  ( 4.403791672194295792, -5.852078868378311149, 34.47109172314383585 ) ) ;
#34112=CARTESIAN_POINT ( 'NONE',  ( -3.230769230769229949, -11.91647553114624181, 32.58852847137148245 ) ) ;
#34113=AXIS2_PLACEMENT_3D ( 'NONE', #63370, #70132, #71451 ) ;
#34114=CARTESIAN_POINT ( 'NONE',  ( 7.146089767170317408, -4.762714258010880997, 34.23016756924214832 ) ) ;
#34115=EDGE_CURVE ( 'NONE', #5202, #36170, #14860, .T. ) ;
#34116=DIRECTION ( 'NONE',  ( 0.000000000000000000, 0.1736481776669275834, 0.9848077530122086864 ) ) ;
#34117=EDGE_LOOP ( 'NONE', ( #22605, #39074, #31575, #46407 ) ) ;
#34118=EDGE_LOOP ( 'NONE', ( #84445, #7992 ) ) ;
#34119=ORIENTED_EDGE ( 'NONE', *, *, #59357, .F. ) ;
#34120=CARTESIAN_POINT ( 'NONE',  ( -4.946875470667394303, -7.723484964179500700, 34.74522123443823318 ) ) ;
#34121=LINE ( 'NONE', #82324, #70391 ) ;
#34122=ORIENTED_EDGE ( 'NONE', *, *, #58212, .T. ) ;
#34123=CARTESIAN_POINT ( 'NONE',  ( 13.16174996241175066, -2.501496062324912284, 29.88072118266895671 ) ) ;
#34124=DIRECTION ( 'NONE',  ( -0.000000000000000000, 0.9396926207859094271, -0.3420201433256663259 ) ) ;
#34125=VERTEX_POINT ( 'NONE', #13864 ) ;
#34126=ADVANCED_FACE ( 'NONE', ( #68812 ), #7113, .F. ) ;
#34127=AXIS2_PLACEMENT_3D ( 'NONE', #71608, #11254, #59437 ) ;
#34129=CARTESIAN_POINT ( 'NONE',  ( 2.307692307692309264, -9.905515769479276145, 34.41647553114623292 ) ) ;
#34130=FACE_BOUND ( 'NONE', #46845, .T. ) ;
#34132=CARTESIAN_POINT ( 'NONE',  ( 16.15384615384615330, -2.486705287966279876, 31.30864560766543647 ) ) ;
#34133=DIRECTION ( 'NONE',  ( -0.000000000000000000, 0.1736481776669307198, -0.9848077530122080203 ) ) ;
#34134=B_SPLINE_CURVE_WITH_KNOTS ( 'NONE', 3,
 ( #35585, #61707, #82452, #36032, #84228, #1345 ),
 .UNSPECIFIED., .F., .F.,
 ( 4, 2, 4 ),
 ( 0.000000000000000000, 0.0001954784845028921395, 0.0003909569690057842790 ),
 .UNSPECIFIED. ) ;
#34135=DIRECTION ( 'NONE',  ( -0.000000000000000000, 1.000000000000000000, 3.491481338843133355E-15 ) ) ;
#34136=CARTESIAN_POINT ( 'NONE',  ( 5.010839665967194989, -9.780366693483667717, 34.19971097300155805 ) ) ;
#34138=CARTESIAN_POINT ( 'NONE',  ( 12.52679360105129724, -3.083524468853784839, 32.58852847137153930 ) ) ;
#34139=EDGE_LOOP ( 'NONE', ( #11063, #51618 ) ) ;
#34140=FACE_OUTER_BOUND ( 'NONE', #30902, .T. ) ;
#34141=CYLINDRICAL_SURFACE ( 'NONE', #75206, 0.2499999999999997502 ) ;
#34142=VERTEX_POINT ( 'NONE', #69696 ) ;
#34143=B_SPLINE_CURVE_WITH_KNOTS ( 'NONE', 3,
 ( #53534, #59855, #67065, #18873, #40921, #12127, #45891, #26524, #33719, #67953 ),
 .UNSPECIFIED., .F., .F.,
 ( 4, 2, 2, 2, 4 ),
 ( 0.0007817246256747502082, 0.0009771112852218944052, 0.001172497944769038819, 0.001367884604316183233, 0.001563271263863327430 ),
 .UNSPECIFIED. ) ;
#34144=CARTESIAN_POINT ( 'NONE',  ( 14.24160889673642849, -9.780366693483667717, 34.19971097300155805 ) ) ;
#34146=ORIENTED_EDGE ( 'NONE', *, *, #18377, .F. ) ;
#34147=AXIS2_PLACEMENT_3D ( 'NONE', #32152, #59610, #21278 ) ;
#34148=CARTESIAN_POINT ( 'NONE',  ( 11.40777093535123043, -9.929715669179220328, 34.40415004197138416 ) ) ;
#34149=ADVANCED_FACE ( 'NONE', ( #361 ), #55292, .F. ) ;
#34151=FACE_BOUND ( 'NONE', #50387, .T. ) ;
#34152=CARTESIAN_POINT ( 'NONE',  ( -18.24997673094235040, -3.137211980971222225, 32.19342716148376837 ) ) ;
#34153=CARTESIAN_POINT ( 'NONE',  ( -17.01166750564705055, -12.46129190930001052, 30.37095296980869819 ) ) ;
#34154=CARTESIAN_POINT ( 'NONE',  ( 10.39245839786846837, -8.239355502252617924, 34.69524867566427417 ) ) ;
#34155=DIRECTION ( 'NONE',  ( -0.000000000000000000, 0.6427876096865404731, -0.7660444431189770143 ) ) ;
#34157=CARTESIAN_POINT ( 'NONE',  ( -8.769230769230768274, -13.37000171582298513, 34.34916445242398453 ) ) ;
#34158=AXIS2_PLACEMENT_3D ( 'NONE', #11526, #39009, #4773 ) ;
#34160=VERTEX_POINT ( 'NONE', #48526 ) ;
#34161=EDGE_LOOP ( 'NONE', ( #6329, #34722 ) ) ;
#34164=CARTESIAN_POINT ( 'NONE',  ( -10.39237177129122003, -8.282913670948747864, 34.94150082978203642 ) ) ;
#34165=DIRECTION ( 'NONE',  ( 0.000000000000000000, 0.7660444431189822323, -0.6427876096865344779 ) ) ;
#34166=CARTESIAN_POINT ( 'NONE',  ( 10.86543903529806698, -2.920487667080175598, 32.31805714834170828 ) ) ;
#34167=CARTESIAN_POINT ( 'NONE',  ( 10.61538461538461675, -2.900454961884010974, 35.62045528018868623 ) ) ;
#34169=CARTESIAN_POINT ( 'NONE',  ( -7.846153846153965716, -8.613356846316285953, 34.62446782046622218 ) ) ;
#34170=CARTESIAN_POINT ( 'NONE',  ( 1.319345384059066539, -10.33852847137145048, 34.16647553114627556 ) ) ;
#34171=CARTESIAN_POINT ( 'NONE',  ( 17.77651507543566822, -4.225889041578354544, 33.85425143139329407 ) ) ;
#34173=LINE ( 'NONE', #89146, #58345 ) ;
#34174=CARTESIAN_POINT ( 'NONE',  ( 6.223012844093396723, -6.460100341425561332, 34.89618726649961644 ) ) ;
#34175=B_SPLINE_CURVE_WITH_KNOTS ( 'NONE', 3,
 ( #19417, #75255, #87015, #5909, #68057, #6363, #12222, #25288, #80697, #26620 ),
 .UNSPECIFIED., .F., .F.,
 ( 4, 2, 2, 2, 4 ),
 ( 0.000000000000000000, 0.0001954339857564063360, 0.0003908679715128126719, 0.0005863019572692189808, 0.0007817359430256253438 ),
 .UNSPECIFIED. ) ;
#34176=CARTESIAN_POINT ( 'NONE',  ( 6.989144256426998325, -3.322132147404559976, 32.92929555188717927 ) ) ;
#34177=B_SPLINE_CURVE_WITH_KNOTS ( 'NONE', 3,
 ( #26586, #34677, #19386, #88752, #27914, #76092, #61684, #445, #74783, #34223 ),
 .UNSPECIFIED., .F., .F.,
 ( 4, 2, 2, 2, 4 ),
 ( 0.0007817246256747434861, 0.0009771112852218861652, 0.001172497944769028844, 0.001367884604316171740, 0.001563271263863314419 ),
 .UNSPECIFIED. ) ;
#34178=CARTESIAN_POINT ( 'NONE',  ( 2.372837088411941409, -7.750023224968865421, 34.99404313364389907 ) ) ;
#34179=CARTESIAN_POINT ( 'NONE',  ( 3.230769230769231726, -2.538708090699994813, 30.37095296980875503 ) ) ;
#34180=ORIENTED_EDGE ( 'NONE', *, *, #57948, .F. ) ;
#34181=CARTESIAN_POINT ( 'NONE',  ( -4.153846153846273204, -5.219633306517616589, 34.19971097300220464 ) ) ;
#34182=CARTESIAN_POINT ( 'NONE',  ( -8.769230769230768274, -5.180354513474913603, 36.12317359536750416 ) ) ;
#34184=AXIS2_PLACEMENT_3D ( 'NONE', #81504, #40084, #32418 ) ;
#34185=DIRECTION ( 'NONE',  ( -0.000000000000000000, -0.000000000000000000, -1.000000000000000000 ) ) ;
#34186=VECTOR ( 'NONE', #12326, 1000.000000000000000 ) ;
#34187=DIRECTION ( 'NONE',  ( -0.000000000000000000, 0.5000000000000011102, -0.8660254037844381525 ) ) ;
#34189=CARTESIAN_POINT ( 'NONE',  ( -1.318547033612945452, -4.098570777380720287, 33.41473453929635440 ) ) ;
#34190=VERTEX_POINT ( 'NONE', #8003 ) ;
#34193=ORIENTED_EDGE ( 'NONE', *, *, #22907, .F. ) ;
#34194=CARTESIAN_POINT ( 'NONE',  ( -11.47326855016688185, -2.255955759149236073, 29.99999999999988987 ) ) ;
#34195=AXIS2_PLACEMENT_3D ( 'NONE', #40502, #4934, #32399 ) ;
#34196=CARTESIAN_POINT ( 'NONE',  ( 10.61538461538461675, -10.67929555188718282, 33.92786785259544047 ) ) ;
#34197=B_SPLINE_CURVE_WITH_KNOTS ( 'NONE', 3,
 ( #55749, #29948, #44773, #64152, #14779, #57854, #44318, #31276, #69714, #86238 ),
 .UNSPECIFIED., .F., .F.,
 ( 4, 2, 2, 2, 4 ),
 ( 0.0007817359430256294638, 0.0009771253907249952391, 0.001172514838424361123, 0.001367904286123726790, 0.001563293733823092673 ),
 .UNSPECIFIED. ) ;
#34198=ORIENTED_EDGE ( 'NONE', *, *, #42513, .F. ) ;
#34199=LINE ( 'NONE', #7175, #39183 ) ;
#34200=CARTESIAN_POINT ( 'NONE',  ( 8.769230769230768274, -12.09954503811598769, 35.62045528018868623 ) ) ;
#34202=ORIENTED_EDGE ( 'NONE', *, *, #7865, .T. ) ;
#34203=ORIENTED_EDGE ( 'NONE', *, *, #86586, .F. ) ;
#34204=CARTESIAN_POINT ( 'NONE',  ( 6.250054419913455561, -12.01375889529407281, 32.43194544308182969 ) ) ;
#34206=CARTESIAN_POINT ( 'NONE',  ( 7.622668921589514923, -9.417330523894422711, 34.63758898049880486 ) ) ;
#34207=CARTESIAN_POINT ( 'NONE',  ( -9.561515884482904681, -9.804649428959608670, 34.18742332936588468 ) ) ;
#34208=CARTESIAN_POINT ( 'NONE',  ( -1.514763354347081092, -11.66186481527757479, 32.95055677023626117 ) ) ;
#34209=DIRECTION ( 'NONE',  ( -0.000000000000000000, 0.1736481776669307198, -0.9848077530122080203 ) ) ;
#34210=DIRECTION ( 'NONE',  ( 0.000000000000000000, 0.000000000000000000, -1.000000000000000000 ) ) ;
#34212=CARTESIAN_POINT ( 'NONE',  ( -12.59168567097668401, -6.852621066184266141, 34.70813303252209181 ) ) ;
#34213=EDGE_CURVE ( 'NONE', #85801, #72479, #17078, .T. ) ;
#34214=VECTOR ( 'NONE', #81691, 1000.000000000000227 ) ;
#34215=EDGE_LOOP ( 'NONE', ( #10651, #22592, #28089, #22797 ) ) ;
#34216=VERTEX_POINT ( 'NONE', #63822 ) ;
#34217=CARTESIAN_POINT ( 'NONE',  ( 7.053602361310570501, -12.70449254468099198, 30.44128974285582956 ) ) ;
#34218=EDGE_LOOP ( 'NONE', ( #1389, #24741, #31888, #81626 ) ) ;
#34219=AXIS2_PLACEMENT_3D ( 'NONE', #57275, #1007, #62249 ) ;
#34220=LINE ( 'NONE', #62568, #40791 ) ;
#34221=ADVANCED_FACE ( 'NONE', ( #36795 ), #50292, .F. ) ;
#34223=CARTESIAN_POINT ( 'NONE',  ( 11.53846153846153832, -3.322132147404559976, 32.92929555188717927 ) ) ;
#34224=CARTESIAN_POINT ( 'NONE',  ( -4.153846153846152411, -13.75783147151868846, 33.36296068462461051 ) ) ;
#34225=EDGE_CURVE ( 'NONE', #17236, #28791, #40713, .T. ) ;
#34226=EDGE_LOOP ( 'NONE', ( #67584, #26779, #48349, #63707 ) ) ;
#34227=CARTESIAN_POINT ( 'NONE',  ( -16.15384615384615330, -1.129524287112498415, 32.06866353760679544 ) ) ;
#34228=ORIENTED_EDGE ( 'NONE', *, *, #79525, .F. ) ;
#34231=CARTESIAN_POINT ( 'NONE',  ( -14.17716686945866833, -12.15418822224088835, 32.17964115625579069 ) ) ;
#34233=EDGE_CURVE ( 'NONE', #23252, #87267, #15971, .T. ) ;
#34234=CARTESIAN_POINT ( 'NONE',  ( -4.219116154402471786, -4.320704448112771878, 33.92786785259540494 ) ) ;
#34235=CARTESIAN_POINT ( 'NONE',  ( 12.23861150263161335, -2.308479472611653094, 30.53278059502174457 ) ) ;
#34236=FACE_BOUND ( 'NONE', #12569, .T. ) ;
#34237=B_SPLINE_CURVE_WITH_KNOTS ( 'NONE', 3,
 ( #41084, #82960, #48717, #33875, #53703, #28010, #34318, #81191, #68548, #6844 ),
 .UNSPECIFIED., .F., .F.,
 ( 4, 2, 2, 2, 4 ),
 ( 0.000000000000000000, 0.0001954311564186881213, 0.0003908623128373762425, 0.0005862934692560643367, 0.0007817246256747524850 ),
 .UNSPECIFIED. ) ;
#34238=CARTESIAN_POINT ( 'NONE',  ( -17.75000000000000000, -2.499999999999999556, 29.75000000000000355 ) ) ;
#34239=CARTESIAN_POINT ( 'NONE',  ( 1.515453715102147658, -7.277220318596959281, 34.99547417642776992 ) ) ;
#34241=B_SPLINE_CURVE_WITH_KNOTS ( 'NONE', 3,
 ( #50630, #57386, #52400, #30800, #38461, #11431, #23601, #65481, #17750, #86220 ),
 .UNSPECIFIED., .F., .F.,
 ( 4, 2, 2, 2, 4 ),
 ( 0.000000000000000000, 0.0001954311564186875792, 0.0003908623128373751583, 0.0005862934692560627103, 0.0007817246256747503166 ),
 .UNSPECIFIED. ) ;
#34243=CARTESIAN_POINT ( 'NONE',  ( -4.854143407945009869, -4.226511098958374291, 33.85474049983370293 ) ) ;
#34244=CARTESIAN_POINT ( 'NONE',  ( -10.86538461538461320, -7.500000000000001776, 34.75000000000000000 ) ) ;
#34245=CARTESIAN_POINT ( 'NONE',  ( 14.30769230769218581, -6.835583212225970762, 34.95778746994575670 ) ) ;
#34246=B_SPLINE_CURVE_WITH_KNOTS ( 'NONE', 3,
 ( #28323, #49491, #41854, #8507, #63435, #13923, #6724, #49039, #76517, #34196 ),
 .UNSPECIFIED., .F., .F.,
 ( 4, 2, 2, 2, 4 ),
 ( 0.0007817246256747451124, 0.0009771112852218885505, 0.001172497944769032097, 0.001367884604316175427, 0.001563271263863318973 ),
 .UNSPECIFIED. ) ;
#34247=ORIENTED_EDGE ( 'NONE', *, *, #55425, .F. ) ;
#34248=ORIENTED_EDGE ( 'NONE', *, *, #3721, .T. ) ;
#34249=CARTESIAN_POINT ( 'NONE',  ( 2.084207363968360038, -10.81261337010820256, 33.49550067578627477 ) ) ;
#34250=FACE_OUTER_BOUND ( 'NONE', #6201, .T. ) ;
#34251=CARTESIAN_POINT ( 'NONE',  ( 7.173022441425065843, -6.696923467548660192, 34.68552623307873972 ) ) ;
#34252=CARTESIAN_POINT ( 'NONE',  ( 15.23076923076923173, -13.88283147151868846, 33.14645433367849847 ) ) ;
#34253=CARTESIAN_POINT ( 'NONE',  ( 6.923076923076924238, -8.564572088678739092, 35.78748833219616898 ) ) ;
#34254=DIRECTION ( 'NONE',  ( 0.000000000000000000, 0.000000000000000000, 1.000000000000000000 ) ) ;
#34256=EDGE_CURVE ( 'NONE', #71506, #64660, #48182, .T. ) ;
#34257=DIRECTION ( 'NONE',  ( 0.000000000000000000, 0.8660254037844377084, -0.5000000000000015543 ) ) ;
#34258=AXIS2_PLACEMENT_3D ( 'NONE', #65537, #31321, #58782 ) ;
#34259=CARTESIAN_POINT ( 'NONE',  ( -5.076923076923199218, -4.320704448113951379, 33.92786785259630022 ) ) ;
#34260=CARTESIAN_POINT ( 'NONE',  ( 10.61538461538461675, -13.87047571288749737, 32.06866353760679544 ) ) ;
#34262=CARTESIAN_POINT ( 'NONE',  ( -7.173100147298380413, -6.652501968072646932, 34.93155406624980941 ) ) ;
#34263=EDGE_LOOP ( 'NONE', ( #52629, #31710 ) ) ;
#34266=EDGE_CURVE ( 'NONE', #2983, #17599, #30948, .T. ) ;
#34267=CARTESIAN_POINT ( 'NONE',  ( 10.36540787133602670, -4.075325502946081535, 33.72974371597206300 ) ) ;
#34268=EDGE_CURVE ( 'NONE', #36170, #5202, #21390, .T. ) ;
#34269=ORIENTED_EDGE ( 'NONE', *, *, #19419, .T. ) ;
#34270=FACE_OUTER_BOUND ( 'NONE', #59024, .T. ) ;
#34271=CARTESIAN_POINT ( 'NONE',  ( 17.07692307692295586, -6.879047030192662504, 34.71129190930017927 ) ) ;
#34272=CARTESIAN_POINT ( 'NONE',  ( 4.826946345980721809, -6.567427716900047230, 34.66269422305636283 ) ) ;
#34273=CARTESIAN_POINT ( 'NONE',  ( -17.07692307692319744, -9.528491918059723176, 34.59228464037033035 ) ) ;
#34274=CARTESIAN_POINT ( 'NONE',  ( 14.43848411551709887, -4.118422570099828484, 33.43335022499816489 ) ) ;
#34275=EDGE_LOOP ( 'NONE', ( #26709, #68673, #28091, #2270 ) ) ;
#34276=DIRECTION ( 'NONE',  ( 0.000000000000000000, 0.9848077530122072432, 0.1736481776669354937 ) ) ;
#34277=LINE ( 'NONE', #61737, #66919 ) ;
#34278=ORIENTED_EDGE ( 'NONE', *, *, #50162, .F. ) ;
#34279=CARTESIAN_POINT ( 'NONE',  ( 0.4615384615384611200, -9.819645486525091727, 36.12317359536749706 ) ) ;
#34280=CARTESIAN_POINT ( 'NONE',  ( -8.545804370315979170, -7.630147987733840509, 34.99859428049665411 ) ) ;
#34281=FACE_OUTER_BOUND ( 'NONE', #1491, .T. ) ;
#34282=CARTESIAN_POINT ( 'NONE',  ( -39.05038313613820122, -2.249999999999998668, 29.75000000000000355 ) ) ;
#34283=DIRECTION ( 'NONE',  ( -0.000000000000000000, -0.8660254037844399289, -0.4999999999999980016 ) ) ;
#34284=CARTESIAN_POINT ( 'NONE',  ( -3.480745974817820887, -10.82459398097509684, 33.81372124010185587 ) ) ;
#34285=CARTESIAN_POINT ( 'NONE',  ( 11.53846153846153832, -12.34228464037088635, 31.77849191805839268 ) ) ;
#34286=B_SPLINE_CURVE_WITH_KNOTS ( 'NONE', 3,
 ( #72268, #37592, #78579, #79485, #10577, #38951, #10126, #51989, #65511, #9678 ),
 .UNSPECIFIED., .F., .F.,
 ( 4, 2, 2, 2, 4 ),
 ( 0.000000000000000000, 0.0001954339857564078809, 0.0003908679715128157619, 0.0005863019572692236428, 0.0007817359430256315238 ),
 .UNSPECIFIED. ) ;
#34289=VECTOR ( 'NONE', #79105, 1000.000000000000000 ) ;
#34290=CARTESIAN_POINT ( 'NONE',  ( 11.66925334628632349, -2.729792928343269587, 31.24908615093345077 ) ) ;
#34291=CARTESIAN_POINT ( 'NONE',  ( -14.30769230769230660, -10.51840700105979565, 33.73612834413961536 ) ) ;
#34292=CARTESIAN_POINT ( 'NONE',  ( 9.942362112221145409, -2.920487667080175598, 32.31805714834170828 ) ) ;
#34294=ORIENTED_EDGE ( 'NONE', *, *, #39320, .F. ) ;
#34296=CARTESIAN_POINT ( 'NONE',  ( -12.46153846153846168, -3.050289026998446396, 32.03036669348365706 ) ) ;
#34297=CARTESIAN_POINT ( 'NONE',  ( -8.834500769787089425, -11.06231777344662781, 33.60647404775220082 ) ) ;
#34298=CARTESIAN_POINT ( 'NONE',  ( 9.942307692307633005, -7.565270000091922853, 34.99999999999999289 ) ) ;
#34299=CARTESIAN_POINT ( 'NONE',  ( 17.77707304109314279, -2.523278758544490241, 31.42238647778636818 ) ) ;
#34300=ORIENTED_EDGE ( 'NONE', *, *, #35968, .T. ) ;
#34302=CARTESIAN_POINT ( 'NONE',  ( 12.33097854792509551, -2.254533558242299396, 29.97296025877828285 ) ) ;
#34304=CARTESIAN_POINT ( 'NONE',  ( 7.623227628637697428, -9.886141570436013382, 34.14413921362392301 ) ) ;
#34305=ORIENTED_EDGE ( 'NONE', *, *, #2973, .F. ) ;
#34306=CARTESIAN_POINT ( 'NONE',  ( -8.546267634964095805, -7.369474539155828730, 34.99858011523957657 ) ) ;
#34307=ORIENTED_EDGE ( 'NONE', *, *, #84672, .T. ) ;
#34308=CARTESIAN_POINT ( 'NONE',  ( 1.134615384615387246, -7.500000000000001776, 34.75000000000000000 ) ) ;
#34310=CARTESIAN_POINT ( 'NONE',  ( 5.076923076923075762, -4.786620604624113540, 33.94971097300155094 ) ) ;
#34311=VERTEX_POINT ( 'NONE', #88891 ) ;
#34312=CARTESIAN_POINT ( 'NONE',  ( 7.715462379486285549, -12.11776431015576172, 31.66791131148498906 ) ) ;
#34313=CARTESIAN_POINT ( 'NONE',  ( -14.98076923076922995, -2.499999999999998668, 29.75000000000000355 ) ) ;
#34314=CARTESIAN_POINT ( 'NONE',  ( 13.13459214732242408, -6.695914987888146541, 34.68535235679833306 ) ) ;
#34315=B_SPLINE_CURVE_WITH_KNOTS ( 'NONE', 3,
 ( #20324, #81586, #39276, #66732, #59969, #32952, #87470, #12679, #40163, #67626 ),
 .UNSPECIFIED., .F., .F.,
 ( 4, 2, 2, 2, 4 ),
 ( 0.000000000000000000, 0.0001954339857564079352, 0.0003908679715128158703, 0.0005863019572692237513, 0.0007817359430256317406 ),
 .UNSPECIFIED. ) ;
#34316=EDGE_CURVE ( 'NONE', #37130, #86943, #24608, .T. ) ;
#34317=AXIS2_PLACEMENT_3D ( 'NONE', #76981, #4414, #59807 ) ;
#34318=CARTESIAN_POINT ( 'NONE',  ( 11.31497661389720477, -12.47654668319379567, 31.42292124445336654 ) ) ;
#34319=CARTESIAN_POINT ( 'NONE',  ( -2.084679463598911653, -10.77377354290276301, 33.85451476688484718 ) ) ;
#34320=ORIENTED_EDGE ( 'NONE', *, *, #72442, .T. ) ;
#34321=FACE_BOUND ( 'NONE', #53949, .T. ) ;
#34322=ORIENTED_EDGE ( 'NONE', *, *, #42653, .F. ) ;
#34323=DIRECTION ( 'NONE',  ( 0.000000000000000000, 0.000000000000000000, 1.000000000000000000 ) ) ;
#34324=ADVANCED_FACE ( 'NONE', ( #26720 ), #82575, .F. ) ;
#34325=CARTESIAN_POINT ( 'NONE',  ( 18.22277966897806678, -6.717445702608400460, 34.94155399931962336 ) ) ;
#34326=DIRECTION ( 'NONE',  ( 0.000000000000000000, 0.4999999999999960032, -0.8660254037844410391 ) ) ;
#34327=CARTESIAN_POINT ( 'NONE',  ( 17.01165263096229907, -2.625532179533444754, 30.86335684631481513 ) ) ;
#34328=ADVANCED_FACE ( 'NONE', ( #66030 ), #61378, .F. ) ;
#34329=ORIENTED_EDGE ( 'NONE', *, *, #58595, .T. ) ;
#34330=EDGE_LOOP ( 'NONE', ( #554, #54297 ) ) ;
#34331=ORIENTED_EDGE ( 'NONE', *, *, #4221, .F. ) ;
#34332=DIRECTION ( 'NONE',  ( -0.000000000000000000, 0.6427876096865404731, -0.7660444431189771253 ) ) ;
#34334=ADVANCED_FACE ( 'NONE', ( #67713 ), #17864, .F. ) ;
#34335=CARTESIAN_POINT ( 'NONE',  ( -6.223484943723947005, -12.44517049084099725, 30.48991314939691932 ) ) ;
#34336=CARTESIAN_POINT ( 'NONE',  ( 7.846153846153723244, -10.33852847137269571, 34.16647553114546554 ) ) ;
#34337=FACE_OUTER_BOUND ( 'NONE', #47930, .T. ) ;
#34338=CARTESIAN_POINT ( 'NONE',  ( 3.453782074862625784, -9.172514111537584114, 34.72667873470787470 ) ) ;
#34339=EDGE_CURVE ( 'NONE', #58442, #17248, #64287, .T. ) ;
#34341=CARTESIAN_POINT ( 'NONE',  ( 5.076923076922954969, -11.48612834414049644, 32.76840700105863391 ) ) ;
#34342=CARTESIAN_POINT ( 'NONE',  ( 17.86985279056177944, -2.619462340734461048, 30.83744416345203021 ) ) ;
#34343=CARTESIAN_POINT ( 'NONE',  ( 7.912221179503920787, -4.661471528628508665, 34.16647553114624003 ) ) ;
#34344=ORIENTED_EDGE ( 'NONE', *, *, #54830, .T. ) ;
#34346=ORIENTED_EDGE ( 'NONE', *, *, #88259, .F. ) ;
#34347=ORIENTED_EDGE ( 'NONE', *, *, #85194, .F. ) ;
#34348=DIRECTION ( 'NONE',  ( -0.000000000000000000, 0.5000000000000011102, -0.8660254037844381525 ) ) ;
#34349=CARTESIAN_POINT ( 'NONE',  ( 11.53846153846153832, -2.499999999999998668, 29.75000000000001421 ) ) ;
#34350=CARTESIAN_POINT ( 'NONE',  ( -7.846153846153967493, -9.528491918059723176, 34.59228464037033035 ) ) ;
#34351=CARTESIAN_POINT ( 'NONE',  ( 1.449870524128224591, -12.51329471203373700, 31.30864560766537963 ) ) ;
#34352=CARTESIAN_POINT ( 'NONE',  ( -10.74553182482283198, -3.817052484675422797, 33.13202310037935661 ) ) ;
#34353=FACE_BOUND ( 'NONE', #23701, .T. ) ;
#34354=CARTESIAN_POINT ( 'NONE',  ( -7.146561847641252463, -3.562934362175799841, 33.22335522853832401 ) ) ;
#34355=ORIENTED_EDGE ( 'NONE', *, *, #30767, .F. ) ;
#34356=EDGE_CURVE ( 'NONE', #50903, #42078, #68612, .T. ) ;
#34358=CARTESIAN_POINT ( 'NONE',  ( -1.318547033612945452, -2.721908614388772740, 31.22303859784725333 ) ) ;
#34359=DIRECTION ( 'NONE',  ( 0.000000000000000000, 0.8660254037844377084, 0.5000000000000015543 ) ) ;
#34360=ORIENTED_EDGE ( 'NONE', *, *, #858, .F. ) ;
#34361=CARTESIAN_POINT ( 'NONE',  ( -5.011667505647053211, -6.879047030191282275, 34.71129190930002295 ) ) ;
#34362=ORIENTED_EDGE ( 'NONE', *, *, #18880, .T. ) ;
#34363=EDGE_CURVE ( 'NONE', #22155, #46498, #65421, .T. ) ;
#34364=FACE_BOUND ( 'NONE', #28393, .T. ) ;
#34367=LINE ( 'NONE', #12333, #30464 ) ;
#34368=CARTESIAN_POINT ( 'NONE',  ( 16.94677510719138169, -12.15440758774515473, 32.17923288041532004 ) ) ;
#34369=EDGE_CURVE ( 'NONE', #37924, #37932, #35707, .T. ) ;
#34370=ORIENTED_EDGE ( 'NONE', *, *, #18267, .T. ) ;
#34371=FACE_OUTER_BOUND ( 'NONE', #9951, .T. ) ;
#34372=DIRECTION ( 'NONE',  ( -0.000000000000000000, 0.1736481776669307198, -0.9848077530122080203 ) ) ;
#34373=CARTESIAN_POINT ( 'NONE',  ( 6.792929713638703682, -12.45813303252208648, 30.39737893381572675 ) ) ;
#34375=ORIENTED_EDGE ( 'NONE', *, *, #81799, .F. ) ;
#34376=VECTOR ( 'NONE', #62034, 1000.000000000000227 ) ;
#34377=B_SPLINE_CURVE_WITH_KNOTS ( 'NONE', 3,
 ( #2300, #1871, #58133, #15841, #56377, #49169, #64440, #29355, #83863, #14952 ),
 .UNSPECIFIED., .F., .F.,
 ( 4, 2, 2, 2, 4 ),
 ( 0.000000000000000000, 0.0001954339857564093175, 0.0003908679715128186350, 0.0005863019572692279796, 0.0007817359430256372700 ),
 .UNSPECIFIED. ) ;
#34379=CARTESIAN_POINT ( 'NONE',  ( -15.23076923076922995, -8.120952969808772792, 34.71129190930000163 ) ) ;
#34380=VECTOR ( 'NONE', #16554, 999.9999999999998863 ) ;
#34381=CARTESIAN_POINT ( 'NONE',  ( 4.376858997939550910, -2.889357225399416862, 32.26129605718031002 ) ) ;
#34382=VERTEX_POINT ( 'NONE', #9124 ) ;
#34383=CARTESIAN_POINT ( 'NONE',  ( -4.377331097570100304, -2.599994579823202923, 30.74605699353653776 ) ) ;
#34384=CARTESIAN_POINT ( 'NONE',  ( 0.6843181305165253470, -10.97394488606064122, 33.68653795673694873 ) ) ;
#34385=CARTESIAN_POINT ( 'NONE',  ( -11.53846153846165912, -8.613356846316285953, 34.62446782046622218 ) ) ;
#34386=CARTESIAN_POINT ( 'NONE',  ( 14.17754509825408960, -9.418419913701741919, 34.36755862841477693 ) ) ;
#34387=CARTESIAN_POINT ( 'NONE',  ( -13.31854805126531005, -3.322132147404559976, 32.92929555188717927 ) ) ;
#34388=CARTESIAN_POINT ( 'NONE',  ( -3.230769230769229949, -3.937682226553329556, 33.60647404775216529 ) ) ;
#34389=DIRECTION ( 'NONE',  ( 0.000000000000000000, 0.9396926207859126468, -0.3420201433256571111 ) ) ;
#34390=AXIS2_PLACEMENT_3D ( 'NONE', #1796, #9010, #13983 ) ;
#34391=DIRECTION ( 'NONE',  ( -0.000000000000000000, -0.5000000000000009992, -0.8660254037844380415 ) ) ;
#34392=EDGE_CURVE ( 'NONE', #14741, #23084, #89059, .T. ) ;
#34394=ORIENTED_EDGE ( 'NONE', *, *, #42310, .F. ) ;
#34395=DIRECTION ( 'NONE',  ( -0.000000000000000000, -0.8660254037844399289, -0.4999999999999980016 ) ) ;
#34396=ORIENTED_EDGE ( 'NONE', *, *, #1631, .F. ) ;
#34397=ADVANCED_FACE ( 'NONE', ( #15437 ), #50086, .F. ) ;
#34398=ORIENTED_EDGE ( 'NONE', *, *, #82408, .F. ) ;
#34401=CARTESIAN_POINT ( 'NONE',  ( -4.153846153846152411, -2.486705287966279876, 31.30864560766543647 ) ) ;
#34403=CARTESIAN_POINT ( 'NONE',  ( 13.45068373561782593, -2.721908614388771852, 31.22303859784725333 ) ) ;
#34405=CARTESIAN_POINT ( 'NONE',  ( 7.846153846154160227, -2.255955759149395501, 30.00000000000324363 ) ) ;
#34407=CARTESIAN_POINT ( 'NONE',  ( -13.51530685128294884, -2.541943142973491554, 30.39792223712631980 ) ) ;
#34408=CARTESIAN_POINT ( 'NONE',  ( -11.53846153846153655, -4.786620604624113540, 33.94971097300155094 ) ) ;
#34411=CARTESIAN_POINT ( 'NONE',  ( 6.792928953345229282, -10.31621877034669588, 34.18098118002070152 ) ) ;
#34412=CARTESIAN_POINT ( 'NONE',  ( -16.82697766754503377, -10.92531984108285670, 33.72920026020278073 ) ) ;
#34413=CARTESIAN_POINT ( 'NONE',  ( 10.61538461538461675, -13.04860791097971706, 34.73218667398347037 ) ) ;
#34414=B_SPLINE_CURVE_WITH_KNOTS ( 'NONE', 3,
 ( #24359, #31573, #67144, #86994, #79772, #65355, #18513, #18069, #73005, #52283 ),
 .UNSPECIFIED., .F., .F.,
 ( 4, 2, 2, 2, 4 ),
 ( 0.000000000000000000, 0.0001954339857564071491, 0.0003908679715128142982, 0.0005863019572692214744, 0.0007817359430256285964 ),
 .UNSPECIFIED. ) ;
#34415=AXIS2_PLACEMENT_3D ( 'NONE', #16433, #58750, #84904 ) ;
#34416=CARTESIAN_POINT ( 'NONE',  ( -9.915792616872021625, -3.562934362175800285, 33.22335522853832401 ) ) ;
#34418=B_SPLINE_CURVE_WITH_KNOTS ( 'NONE', 3,
 ( #86517, #60798, #88308, #87406, #66218, #24791, #74322, #45946, #87863, #39212 ),
 .UNSPECIFIED., .F., .F.,
 ( 4, 2, 2, 2, 4 ),
 ( 0.0007817246256747491240, 0.0009771112852218931041, 0.001172497944769036867, 0.001367884604316180631, 0.001563271263863324611 ),
 .UNSPECIFIED. ) ;
#34419=EDGE_CURVE ( 'NONE', #2875, #28403, #32087, .T. ) ;
#34421=ORIENTED_EDGE ( 'NONE', *, *, #67116, .T. ) ;
#34422=B_SPLINE_CURVE_WITH_KNOTS ( 'NONE', 3,
 ( #65301, #31975, #58100, #30627, #9475, #44129, #58533, #86030, #24309, #85144 ),
 .UNSPECIFIED., .F., .F.,
 ( 4, 2, 2, 2, 4 ),
 ( 0.000000000000000000, 0.0001954339881912776238, 0.0003908679763825552477, 0.0005863019645738329257, 0.0007817359527651104954 ),
 .UNSPECIFIED. ) ;
#34423=CARTESIAN_POINT ( 'NONE',  ( -15.23076923076922995, -13.75783147151868846, 33.36296068462461051 ) ) ;
#34425=FACE_OUTER_BOUND ( 'NONE', #65209, .T. ) ;
#34426=CARTESIAN_POINT ( 'NONE',  ( 5.999999999999880096, -6.026961402154118908, 34.52809138561165270 ) ) ;
#34427=CARTESIAN_POINT ( 'NONE',  ( 9.822833130541336999, -11.66157788607254098, 32.95092075102925833 ) ) ;
#34428=CARTESIAN_POINT ( 'NONE',  ( -9.442362282929646966, -10.92531984108285670, 33.72920026020278073 ) ) ;
#34431=EDGE_LOOP ( 'NONE', ( #38325, #30736, #3430, #10291 ) ) ;
#34432=CARTESIAN_POINT ( 'NONE',  ( 18.24994540937804643, -3.520799739797213501, 33.17531984108286025 ) ) ;
#34433=ORIENTED_EDGE ( 'NONE', *, *, #1520, .T. ) ;
#34434=CARTESIAN_POINT ( 'NONE',  ( -8.546451100252703270, -4.989023458446560255, 34.36081565061822118 ) ) ;
#34435=VECTOR ( 'NONE', #62497, 1000.000000000000227 ) ;
#34437=CARTESIAN_POINT ( 'NONE',  ( 0.4615384615383396616, -4.481592998941358097, 33.73612834414048933 ) ) ;
#34440=CARTESIAN_POINT ( 'NONE',  ( 6.000000000000001776, -11.33034616979429110, 35.88435417666054406 ) ) ;
#34441=ADVANCED_FACE ( 'NONE', ( #69924 ), #8234, .F. ) ;
#34442=AXIS2_PLACEMENT_3D ( 'NONE', #81817, #76374, #75485 ) ;
#34443=AXIS2_PLACEMENT_3D ( 'NONE', #27922, #81994, #892 ) ;
#34444=VERTEX_POINT ( 'NONE', #28960 ) ;
#34445=VECTOR ( 'NONE', #43817, 1000.000000000000114 ) ;
#34446=EDGE_LOOP ( 'NONE', ( #31108, #23243, #75356, #59589, #51384, #26626 ) ) ;
#34448=EDGE_LOOP ( 'NONE', ( #240, #87374, #44760, #49949 ) ) ;
#34449=CARTESIAN_POINT ( 'NONE',  ( 6.000000000000001776, -2.538708090699994813, 30.37095296980875503 ) ) ;
#34450=CARTESIAN_POINT ( 'NONE',  ( -12.68446542044531000, -12.64616026154729411, 30.79003144601914244 ) ) ;
#34451=B_SPLINE_CURVE_WITH_KNOTS ( 'NONE', 3,
 ( #71924, #52538, #80021, #59748, #87243, #10237, #40816, #61075, #267, #33165 ),
 .UNSPECIFIED., .F., .F.,
 ( 4, 2, 2, 2, 4 ),
 ( 0.0007817246256747453293, 0.0009771112852218889842, 0.001172497944769032531, 0.001367884604316176294, 0.001563271263863319840 ),
 .UNSPECIFIED. ) ;
#34452=B_SPLINE_CURVE_WITH_KNOTS ( 'NONE', 3,
 ( #30409, #71831, #23643, #64175, #50217, #58313, #1608, #15570, #43036, #85806 ),
 .UNSPECIFIED., .F., .F.,
 ( 4, 2, 2, 2, 4 ),
 ( 0.0007817246256747504250, 0.0009771112852218954894, 0.001172497944769040554, 0.001367884604316185401, 0.001563271263863330466 ),
 .UNSPECIFIED. ) ;
#34453=CARTESIAN_POINT ( 'NONE',  ( -3.360916440207451839, -10.19110544564092002, 33.96427741523702792 ) ) ;
#34454=CARTESIAN_POINT ( 'NONE',  ( -15.48074596171158390, -11.28823185664190376, 33.01397839955799896 ) ) ;
#34455=CARTESIAN_POINT ( 'NONE',  ( 5.076923076923075762, -1.367168528481310208, 33.57946703557072254 ) ) ;
#34456=CARTESIAN_POINT ( 'NONE',  ( -10.61538461538461320, -12.10708131394839349, 31.69288490824020244 ) ) ;
#34457=EDGE_LOOP ( 'NONE', ( #37874, #13482, #2109, #33250 ) ) ;
#34458=ORIENTED_EDGE ( 'NONE', *, *, #36642, .T. ) ;
#34459=ORIENTED_EDGE ( 'NONE', *, *, #38932, .F. ) ;
#34460=CARTESIAN_POINT ( 'NONE',  ( 17.07692307692295586, -12.46129190930018460, 30.37095296980731973 ) ) ;
#34462=CARTESIAN_POINT ( 'NONE',  ( 17.07692307692307665, -10.67929555188718282, 33.92786785259544047 ) ) ;
#34463=CARTESIAN_POINT ( 'NONE',  ( 4.153846153846154188, -12.62096338111211580, 30.90682066428153263 ) ) ;
#34465=VERTEX_POINT ( 'NONE', #83902 ) ;
#34466=EDGE_CURVE ( 'NONE', #13098, #23856, #979, .T. ) ;
#34467=VECTOR ( 'NONE', #33505, 1000.000000000000000 ) ;
#34470=ADVANCED_FACE ( 'NONE', ( #57293 ), #50526, .F. ) ;
#34471=FACE_BOUND ( 'NONE', #48262, .T. ) ;
#34473=CARTESIAN_POINT ( 'NONE',  ( 8.068933515131911705, -5.827830569534417471, 34.72679350104403539 ) ) ;
#34474=ORIENTED_EDGE ( 'NONE', *, *, #67381, .F. ) ;
#34475=CARTESIAN_POINT ( 'NONE',  ( -6.000000000000121680, -5.941354392335915335, 34.76329471203413846 ) ) ;
#34476=EDGE_CURVE ( 'NONE', #5555, #32412, #26659, .T. ) ;
#34477=CARTESIAN_POINT ( 'NONE',  ( 6.792928953345230170, -12.15440758774515473, 32.17923288041532004 ) ) ;
#34478=CARTESIAN_POINT ( 'NONE',  ( -17.01085574357299990, -12.62096338111211757, 30.90682066428152908 ) ) ;
#34479=CARTESIAN_POINT ( 'NONE',  ( 14.30769230769231015, -9.058645607665452459, 34.76329471203371924 ) ) ;
#34480=VERTEX_POINT ( 'NONE', #16747 ) ;
#34481=EDGE_CURVE ( 'NONE', #83601, #64427, #76099, .T. ) ;
#34482=CARTESIAN_POINT ( 'NONE',  ( -12.39628332202562433, -2.379036618887895305, 30.90682066428158592 ) ) ;
#34483=CARTESIAN_POINT ( 'NONE',  ( -6.923076923076922462, -11.16473453929635440, 33.15142922261926373 ) ) ;
#34484=CARTESIAN_POINT ( 'NONE',  ( -16.15384615384583711, -2.255955759149395501, 30.00000000000324363 ) ) ;
#34485=CARTESIAN_POINT ( 'NONE',  ( -2.372962753653082402, -10.90142922261923886, 33.41473453929638993 ) ) ;
#34486=CYLINDRICAL_SURFACE ( 'NONE', #41496, 0.2500000000000002220 ) ;
#34487=FACE_BOUND ( 'NONE', #77238, .T. ) ;
#34488=CARTESIAN_POINT ( 'NONE',  ( 5.076923076923075762, -11.16473453929635440, 33.15142922261926373 ) ) ;
#34489=CARTESIAN_POINT ( 'NONE',  ( -6.223484924564328225, -10.23692288466677880, 34.23039457007281072 ) ) ;
#34491=CARTESIAN_POINT ( 'NONE',  ( -6.923076923076922462, -9.819645486525091727, 36.12317359536749706 ) ) ;
#34492=CARTESIAN_POINT ( 'NONE',  ( -5.934744428723974785, -10.21337939537593620, 33.94971097300152252 ) ) ;
#34493=CARTESIAN_POINT ( 'NONE',  ( 17.77651505627604678, -11.41268669641499756, 32.86336882939238535 ) ) ;
#34494=EDGE_CURVE ( 'NONE', #1913, #16308, #59997, .T. ) ;
#34495=CARTESIAN_POINT ( 'NONE',  ( -18.06608341095587633, -9.780366693483671270, 34.19971097300155805 ) ) ;
#34498=CARTESIAN_POINT ( 'NONE',  ( -5.750054590621957118, -10.92531984108285670, 33.72920026020278073 ) ) ;
#34499=ORIENTED_EDGE ( 'NONE', *, *, #83793, .F. ) ;
#34500=VECTOR ( 'NONE', #59295, 1000.000000000000000 ) ;
#34502=CARTESIAN_POINT ( 'NONE',  ( 12.46153846153846168, -8.120952969808772792, 34.71129190930000163 ) ) ;
#34503=EDGE_LOOP ( 'NONE', ( #71201, #83304, #85200, #79783 ) ) ;
#34505=CARTESIAN_POINT ( 'NONE',  ( 7.846153846153846700, -5.180354513474913603, 36.12317359536750416 ) ) ;
#34506=CARTESIAN_POINT ( 'NONE',  ( 5.750023255951410839, -8.347322224742351082, 34.93158281831414769 ) ) ;
#34507=EDGE_LOOP ( 'NONE', ( #59436, #54378 ) ) ;
#34508=CARTESIAN_POINT ( 'NONE',  ( 18.06616660659164353, -7.250054591869668386, 34.99404684341514127 ) ) ;
#34511=CARTESIAN_POINT ( 'NONE',  ( -15.36091720050092846, -9.504002272028875709, 34.60269587691767867 ) ) ;
#34514=LINE ( 'NONE', #61093, #74643 ) ;
#34515=DIRECTION ( 'NONE',  ( -0.000000000000000000, 0.6427876096865404731, -0.7660444431189770143 ) ) ;
#34516=CYLINDRICAL_SURFACE ( 'NONE', #23886, 0.2500000000000004996 ) ;
#34519=DIRECTION ( 'NONE',  ( -0.000000000000000000, -0.9848077530122086864, -0.1736481776669273613 ) ) ;
#34520=CARTESIAN_POINT ( 'NONE',  ( 10.74591031714818001, -11.46989282347013095, 32.79007818306219946 ) ) ;
#34522=CARTESIAN_POINT ( 'NONE',  ( 9.019285080869083870, -9.943054286541403997, 34.11300777759954883 ) ) ;
#34524=EDGE_CURVE ( 'NONE', #798, #13779, #19162, .T. ) ;
#34525=CYLINDRICAL_SURFACE ( 'NONE', #80725, 0.2500000000000009437 ) ;
#34526=DIRECTION ( 'NONE',  ( -0.000000000000000000, 0.8660254037844399289, -0.4999999999999980016 ) ) ;
#34527=EDGE_LOOP ( 'NONE', ( #86155, #45092 ) ) ;
#34528=DIRECTION ( 'NONE',  ( 0.000000000000000000, 0.9848077530122072432, -0.1736481776669354937 ) ) ;
#34529=CYLINDRICAL_SURFACE ( 'NONE', #31555, 0.2499999999999995559 ) ;
#34530=CARTESIAN_POINT ( 'NONE',  ( 2.084766090176162212, -2.758268499246657068, 31.33685645148949561 ) ) ;
#34532=LINE ( 'NONE', #745, #41201 ) ;
#34533=CARTESIAN_POINT ( 'NONE',  ( -5.999999999999998224, -4.102666532097928531, 36.13435417666054406 ) ) ;
#34534=CARTESIAN_POINT ( 'NONE',  ( 16.08776274289027342, -8.973038597847269315, 34.52809138561120506 ) ) ;
#34535=EDGE_CURVE ( 'NONE', #24282, #2419, #57916, .T. ) ;
#34536=DIRECTION ( 'NONE',  ( -0.000000000000000000, -0.7660444431189791237, -0.6427876096865379196 ) ) ;
#34538=EDGE_CURVE ( 'NONE', #57919, #80616, #33208, .T. ) ;
#34541=VECTOR ( 'NONE', #2153, 1000.000000000000227 ) ;
#34542=VERTEX_POINT ( 'NONE', #11782 ) ;
#34543=CARTESIAN_POINT ( 'NONE',  ( -9.561515884482908234, -3.062576670634119758, 32.05464942895959979 ) ) ;
#34544=DIRECTION ( 'NONE',  ( -0.000000000000000000, 0.9848077530122085754, -0.1736481776669273613 ) ) ;
#34545=CARTESIAN_POINT ( 'NONE',  ( -13.16160403300253634, -12.15243808032446005, 31.58219941686247978 ) ) ;
#34548=B_SPLINE_CURVE_WITH_KNOTS ( 'NONE', 3,
 ( #1550, #83983, #15071, #7868, #28129, #77204, #82654, #70458, #55157, #1106 ),
 .UNSPECIFIED., .F., .F.,
 ( 4, 2, 2, 2, 4 ),
 ( 0.000000000000000000, 0.0001954339857564080707, 0.0003908679715128161414, 0.0005863019572692241849, 0.0007817359430256322827 ),
 .UNSPECIFIED. ) ;
#34549=ORIENTED_EDGE ( 'NONE', *, *, #88056, .F. ) ;
#34550=LINE ( 'NONE', #76870, #27677 ) ;
#34551=ORIENTED_EDGE ( 'NONE', *, *, #7796, .F. ) ;
#34552=ADVANCED_FACE ( 'NONE', ( #6365 ), #53194, .F. ) ;
#34554=EDGE_LOOP ( 'NONE', ( #26165, #71719 ) ) ;
#34555=VECTOR ( 'NONE', #34135, 1000.000000000000000 ) ;
#34557=FACE_OUTER_BOUND ( 'NONE', #53692, .T. ) ;
#34558=ORIENTED_EDGE ( 'NONE', *, *, #17249, .F. ) ;
#34559=CARTESIAN_POINT ( 'NONE',  ( -5.010855743572999899, -12.34228464037088813, 31.77849191805839268 ) ) ;
#34560=EDGE_CURVE ( 'NONE', #75253, #76436, #22348, .T. ) ;
#34561=FACE_OUTER_BOUND ( 'NONE', #67013, .T. ) ;
#34564=CARTESIAN_POINT ( 'NONE',  ( 5.869852030268304155, -4.299443229763728169, 33.91186481527756058 ) ) ;
#34565=CARTESIAN_POINT ( 'NONE',  ( -5.777220458731587627, -4.387253974876676565, 33.66317474335728832 ) ) ;
#34566=ORIENTED_EDGE ( 'NONE', *, *, #28575, .F. ) ;
#34570=CARTESIAN_POINT ( 'NONE',  ( -6.923076923076922462, -2.833524468853757305, 32.15551576947925838 ) ) ;
#34571=CARTESIAN_POINT ( 'NONE',  ( -2.307692307692305711, -12.62096338111211580, 30.90682066428153263 ) ) ;
#34572=VERTEX_POINT ( 'NONE', #27066 ) ;
#34573=CARTESIAN_POINT ( 'NONE',  ( -2.307692307692427391, -8.613356846316285953, 34.62446782046622218 ) ) ;
#34574=CARTESIAN_POINT ( 'NONE',  ( -17.32689982097166848, -3.436278759898155677, 33.07459398097509506 ) ) ;
#34577=CARTESIAN_POINT ( 'NONE',  ( 12.59232890250541281, -9.084667340241226796, 34.75534355489798344 ) ) ;
#34578=VERTEX_POINT ( 'NONE', #5475 ) ;
#34579=FACE_BOUND ( 'NONE', #63964, .T. ) ;
#34581=CARTESIAN_POINT ( 'NONE',  ( 13.38461538461538680, -6.343179335718451384, 34.87096338111211935 ) ) ;
#34582=EDGE_CURVE ( 'NONE', #66717, #58944, #41028, .T. ) ;
#34583=CARTESIAN_POINT ( 'NONE',  ( 12.39545608217832395, -6.343179335718451384, 34.87096338111212646 ) ) ;
#34584=CARTESIAN_POINT ( 'NONE',  ( -14.30769230769230660, -5.557115091759785130, 34.35708131394839171 ) ) ;
#34586=DIRECTION ( 'NONE',  ( 0.000000000000000000, -6.938893903907222067E-15, 1.000000000000000000 ) ) ;
#34587=CARTESIAN_POINT ( 'NONE',  ( -0.7115151924808165163, -3.627789207965226748, 32.91389620160131102 ) ) ;
#34588=EDGE_LOOP ( 'NONE', ( #70763, #11404 ) ) ;
#34589=CARTESIAN_POINT ( 'NONE',  ( -2.530619266599155370, -4.026226216239095379, 33.68668979543632958 ) ) ;
#34590=CARTESIAN_POINT ( 'NONE',  ( 13.45078452557804738, -7.250054483168843156, 34.74374881642865631 ) ) ;
#34591=VERTEX_POINT ( 'NONE', #19863 ) ;
#34592=EDGE_CURVE ( 'NONE', #88588, #74576, #42458, .T. ) ;
#34593=CYLINDRICAL_SURFACE ( 'NONE', #71732, 0.2500000000000004996 ) ;
#34594=DIRECTION ( 'NONE',  ( -0.000000000000000000, 0.9396926207859092051, -0.3420201433256662704 ) ) ;
#34595=EDGE_LOOP ( 'NONE', ( #38960, #78988 ) ) ;
#34596=DIRECTION ( 'NONE',  ( 0.000000000000000000, 0.8660254037844377084, -0.5000000000000015543 ) ) ;
#34597=DIRECTION ( 'NONE',  ( 0.000000000000000000, 0.6427876096865373645, -0.7660444431189797898 ) ) ;
#34598=FACE_BOUND ( 'NONE', #2274, .T. ) ;
#34599=CARTESIAN_POINT ( 'NONE',  ( -15.23076923076935074, -6.026961402154118019, 34.52809138561165270 ) ) ;
#34600=CARTESIAN_POINT ( 'NONE',  ( -4.088590582570128973, -8.613356846314928816, 34.62446782046653482 ) ) ;
#34601=CARTESIAN_POINT ( 'NONE',  ( -8.899377978668990608, -6.852621066184266141, 34.70813303252209181 ) ) ;
#34602=CARTESIAN_POINT ( 'NONE',  ( 12.21151523731700372, -12.45566812827425451, 31.48439005359158926 ) ) ;
#34604=CARTESIAN_POINT ( 'NONE',  ( 0.3313912521002405631, -6.001485441113819874, 34.52039167877662607 ) ) ;
#34605=AXIS2_PLACEMENT_3D ( 'NONE', #1394, #62208, #69415 ) ;
#34606=EDGE_CURVE ( 'NONE', #86693, #47571, #3031, .T. ) ;
#34607=CARTESIAN_POINT ( 'NONE',  ( -9.692307692307691624, -4.661471528628507777, 34.16647553114623292 ) ) ;
#34609=ORIENTED_EDGE ( 'NONE', *, *, #38387, .T. ) ;
#34610=ORIENTED_EDGE ( 'NONE', *, *, #76776, .F. ) ;
#34611=CARTESIAN_POINT ( 'NONE',  ( -9.942330916529147800, -2.341070481393819236, 30.72580821765574299 ) ) ;
#34612=CARTESIAN_POINT ( 'NONE',  ( -15.29603923132555110, -5.941354392334499579, 34.76329471203369792 ) ) ;
#34613=LINE ( 'NONE', #69725, #81980 ) ;
#34614=CARTESIAN_POINT ( 'NONE',  ( -8.899921372341079717, -8.191372820521381826, 34.95448215188424967 ) ) ;
#34615=CARTESIAN_POINT ( 'NONE',  ( -8.769230769230890843, -3.300289026999228881, 32.46337939537708905 ) ) ;
#34617=CARTESIAN_POINT ( 'NONE',  ( 3.903846153846154632, -7.500000000000001776, 34.75000000000000000 ) ) ;
#34618=CARTESIAN_POINT ( 'NONE',  ( 2.177132394078943545, -2.254533558242299396, 29.97296025877828285 ) ) ;
#34619=EDGE_CURVE ( 'NONE', #17855, #69894, #59957, .T. ) ;
#34620=CARTESIAN_POINT ( 'NONE',  ( 9.468822767743363400, -10.97335522853832579, 33.68706563782419749 ) ) ;
#34621=CYLINDRICAL_SURFACE ( 'NONE', #89060, 0.2499999999999979738 ) ;
#34623=DIRECTION ( 'NONE',  ( 0.000000000000000000, 0.000000000000000000, 1.000000000000000000 ) ) ;
#34624=CARTESIAN_POINT ( 'NONE',  ( -3.296039231325551100, -10.33852847137145048, 34.16647553114627556 ) ) ;
#34625=CARTESIAN_POINT ( 'NONE',  ( -8.769230769230768274, -11.35647404775217417, 33.31231777344666511 ) ) ;
#34626=VECTOR ( 'NONE', #25179, 999.9999999999998863 ) ;
#34627=CARTESIAN_POINT ( 'NONE',  ( 3.230769230769110045, -2.625532179533779154, 30.86335684631627174 ) ) ;
#34628=ORIENTED_EDGE ( 'NONE', *, *, #5914, .F. ) ;
#34629=CARTESIAN_POINT ( 'NONE',  ( 4.087762742890273415, -4.786620604624113540, 33.94971097300155805 ) ) ;
#34630=CARTESIAN_POINT ( 'NONE',  ( 0.7115927731767751618, -2.564540009722895419, 30.55348353981670684 ) ) ;
#34632=EDGE_CURVE ( 'NONE', #88595, #74089, #20283, .T. ) ;
#34633=AXIS2_PLACEMENT_3D ( 'NONE', #29617, #23719, #18210 ) ;
#34634=CARTESIAN_POINT ( 'NONE',  ( -9.019230769230768274, -7.500000000000001776, 35.04278698407183867 ) ) ;
#34635=CARTESIAN_POINT ( 'NONE',  ( 17.01165307636675905, -11.67786785259541027, 32.92929555188721480 ) ) ;
#34636=ORIENTED_EDGE ( 'NONE', *, *, #5138, .F. ) ;
#34637=CARTESIAN_POINT ( 'NONE',  ( -7.146561847641256016, -3.019605429927184836, 32.48692288466676814 ) ) ;
#34638=CARTESIAN_POINT ( 'NONE',  ( -14.53061852520844965, -12.15238873228292071, 31.58232369045353849 ) ) ;
#34639=ORIENTED_EDGE ( 'NONE', *, *, #13149, .F. ) ;
#34640=CARTESIAN_POINT ( 'NONE',  ( 9.822833130541338775, -12.70449254468099198, 30.44128974285582956 ) ) ;
#34641=ADVANCED_FACE ( 'NONE', ( #40153 ), #12224, .F. ) ;
#34642=CARTESIAN_POINT ( 'NONE',  ( -5.076923076923075762, -9.780366693483667717, 34.19971097300155094 ) ) ;
#34643=EDGE_LOOP ( 'NONE', ( #71014, #84825, #61770, #59331 ) ) ;
#34644=CARTESIAN_POINT ( 'NONE',  ( 8.519207531937803779, -8.432397168068783699, 34.66272746175022945 ) ) ;
#34645=VECTOR ( 'NONE', #1134, 1000.000000000000000 ) ;
#34647=EDGE_LOOP ( 'NONE', ( #25813, #46181, #1063, #49843 ) ) ;
#34648=CARTESIAN_POINT ( 'NONE',  ( 16.94623161025552704, -11.18331474514187995, 33.13161551792790505 ) ) ;
#34649=CARTESIAN_POINT ( 'NONE',  ( 2.307692307692309264, -8.164416787775445883, 34.95778746994557906 ) ) ;
#34651=CARTESIAN_POINT ( 'NONE',  ( 2.307692307692309264, -12.62096338111211580, 30.90682066428153263 ) ) ;
#34652=ORIENTED_EDGE ( 'NONE', *, *, #53688, .F. ) ;
#34653=ORIENTED_EDGE ( 'NONE', *, *, #13293, .T. ) ;
#34654=CARTESIAN_POINT ( 'NONE',  ( -10.48485917715097138, -2.372941743896879174, 30.88044141588253666 ) ) ;
#34656=CARTESIAN_POINT ( 'NONE',  ( 3.296024370282068627, -12.16647553114626490, 32.15551576947920864 ) ) ;
#34657=CARTESIAN_POINT ( 'NONE',  ( -1.254089682851821541, -2.619367082507848998, 30.83698974864644171 ) ) ;
#34658=CARTESIAN_POINT ( 'NONE',  ( -1.634638608836842089, -11.56360843649122216, 33.07473185843129926 ) ) ;
#34660=CARTESIAN_POINT ( 'NONE',  ( -0.4615384615384611200, -5.471508081941601098, 34.59228464037088457 ) ) ;
#34661=CARTESIAN_POINT ( 'NONE',  ( 1.318533005255250190, -2.292212530054419606, 30.41441678777542634 ) ) ;
#34662=EDGE_CURVE ( 'NONE', #3616, #7165, #72910, .T. ) ;
#34663=B_SPLINE_CURVE_WITH_KNOTS ( 'NONE', 3,
 ( #22511, #3997, #85990, #50841, #10328, #84674, #31027, #58492, #36902, #24269 ),
 .UNSPECIFIED., .F., .F.,
 ( 4, 2, 2, 2, 4 ),
 ( 0.0007817359430256308733, 0.0009771253907249971907, 0.001172514838424363725, 0.001367904286123730259, 0.001563293733823096577 ),
 .UNSPECIFIED. ) ;
#34664=B_SPLINE_CURVE_WITH_KNOTS ( 'NONE', 3,
 ( #54067, #81566, #19852, #47315, #27055, #82008, #44088, #63490, #22070, #70253 ),
 .UNSPECIFIED., .F., .F.,
 ( 4, 2, 2, 2, 4 ),
 ( 0.000000000000000000, 0.0001954311564186861697, 0.0003908623128373723394, 0.0005862934692560584820, 0.0007817246256747446788 ),
 .UNSPECIFIED. ) ;
#34665=CARTESIAN_POINT ( 'NONE',  ( 10.48469314871705649, -12.11776431015576172, 31.66791131148498906 ) ) ;
#34666=VECTOR ( 'NONE', #37740, 1000.000000000000114 ) ;
#34667=B_SPLINE_CURVE_WITH_KNOTS ( 'NONE', 3,
 ( #33430, #81178, #19463, #60890, #82947, #60444, #74865, #87963, #55461, #21229 ),
 .UNSPECIFIED., .F., .F.,
 ( 4, 2, 2, 2, 4 ),
 ( 0.0007817359430256296806, 0.0009771253907249958896, 0.001172514838424361990, 0.001367904286123728091, 0.001563293733823094408 ),
 .UNSPECIFIED. ) ;
#34668=ADVANCED_FACE ( 'NONE', ( #2234 ), #14434, .F. ) ;
#34669=ADVANCED_FACE ( 'NONE', ( #22958 ), #1803, .F. ) ;
#34670=ORIENTED_EDGE ( 'NONE', *, *, #8332, .F. ) ;
#34671=VERTEX_POINT ( 'NONE', #49553 ) ;
#34672=CARTESIAN_POINT ( 'NONE',  ( -1.634615384615382805, -7.566083408709834757, 34.74999999999999289 ) ) ;
#34675=CARTESIAN_POINT ( 'NONE',  ( 17.01084069756293715, -2.292212530054419606, 30.41441678777542634 ) ) ;
#34676=VERTEX_POINT ( 'NONE', #8129 ) ;
#34677=CARTESIAN_POINT ( 'NONE',  ( 11.60371667797437567, -3.643525952247864463, 33.31231777344670064 ) ) ;
#34678=DIRECTION ( 'NONE',  ( 0.000000000000000000, 0.4999999999999985567, 0.8660254037844395958 ) ) ;
#34679=VERTEX_POINT ( 'NONE', #49985 ) ;
#34680=CARTESIAN_POINT ( 'NONE',  ( 8.096208157792162297, -8.303483539816731707, 34.68545999027711702 ) ) ;
#34681=ORIENTED_EDGE ( 'NONE', *, *, #70552, .F. ) ;
#34682=CARTESIAN_POINT ( 'NONE',  ( -12.33149329870368405, -2.504778602574660340, 29.97347330155780654 ) ) ;
#34683=VERTEX_POINT ( 'NONE', #15772 ) ;
#34684=FACE_OUTER_BOUND ( 'NONE', #65285, .T. ) ;
#34685=ORIENTED_EDGE ( 'NONE', *, *, #36274, .T. ) ;
#34686=CARTESIAN_POINT ( 'NONE',  ( -12.46153846153846168, -9.905515769479276145, 34.41647553114623292 ) ) ;
#34687=CARTESIAN_POINT ( 'NONE',  ( -16.15384615384615330, -5.557115091759785130, 34.35708131394839171 ) ) ;
#34688=FACE_BOUND ( 'NONE', #76656, .T. ) ;
#34689=CARTESIAN_POINT ( 'NONE',  ( -14.30769230769242917, -9.528491918059723176, 34.59228464037033035 ) ) ;
#34690=CARTESIAN_POINT ( 'NONE',  ( -6.857821351800899023, -12.27809138561124591, 31.22303859784720359 ) ) ;
#34691=B_SPLINE_CURVE_WITH_KNOTS ( 'NONE', 3,
 ( #82898, #41461, #15765, #63494, #69813, #21179, #2228, #70704, #69379, #28381 ),
 .UNSPECIFIED., .F., .F.,
 ( 4, 2, 2, 2, 4 ),
 ( 0.0007817246256747530271, 0.0009771112852218978746, 0.001172497944769042939, 0.001367884604316188003, 0.001563271263863332851 ),
 .UNSPECIFIED. ) ;
#34692=CARTESIAN_POINT ( 'NONE',  ( 11.53846153846153832, -2.833524468853757305, 32.15551576947925838 ) ) ;
#34693=CARTESIAN_POINT ( 'NONE',  ( 4.376857505459002873, -8.239487800360276282, 34.69522927552633718 ) ) ;
#34694=CARTESIAN_POINT ( 'NONE',  ( -5.076923076923075762, -3.937682226553329556, 33.60647404775216529 ) ) ;
#34695=CARTESIAN_POINT ( 'NONE',  ( 16.15384615384603251, -4.481592998941358097, 33.73612834414048933 ) ) ;
#34696=DIRECTION ( 'NONE',  ( 0.000000000000000000, 0.6427876096865368094, 0.7660444431189802339 ) ) ;
#34697=VERTEX_POINT ( 'NONE', #63500 ) ;
#34698=EDGE_LOOP ( 'NONE', ( #76551, #22097, #76061, #70341 ) ) ;
#34700=CARTESIAN_POINT ( 'NONE',  ( 2.241609928332171986, -2.833524468853757305, 32.15551576947924417 ) ) ;
#34702=B_SPLINE_CURVE_WITH_KNOTS ( 'NONE', 3,
 ( #42019, #55958, #28957, #42459, #69478, #83454, #15432, #21736, #43339, #76685 ),
 .UNSPECIFIED., .F., .F.,
 ( 4, 2, 2, 2, 4 ),
 ( 0.000000000000000000, 0.0001954311584214086476, 0.0003908623168428172951, 0.0005862934752642233677, 0.0007817246336856293861 ),
 .UNSPECIFIED. ) ;
#34703=CARTESIAN_POINT ( 'NONE',  ( -12.71151519248081740, -2.564618984488975073, 30.55390908950641915 ) ) ;
#34704=DIRECTION ( 'NONE',  ( -0.000000000000000000, -0.9848077530122086864, -0.1736481776669273613 ) ) ;
#34705=FACE_OUTER_BOUND ( 'NONE', #89180, .T. ) ;
#34706=CARTESIAN_POINT ( 'NONE',  ( 9.692307692307695177, -2.538708090699994813, 30.37095296980875503 ) ) ;
#34707=EDGE_LOOP ( 'NONE', ( #30544, #52367 ) ) ;
#34708=DIRECTION ( 'NONE',  ( 0.000000000000000000, 0.9396926207859126468, 0.3420201433256571111 ) ) ;
#34709=CARTESIAN_POINT ( 'NONE',  ( 1.634669696253701066, -12.17597550085003455, 31.52189283813461884 ) ) ;
#34710=CARTESIAN_POINT ( 'NONE',  ( -14.17716686945866300, -12.50538340440932394, 31.33453814440721885 ) ) ;
#34711=CARTESIAN_POINT ( 'NONE',  ( 3.230769230769110045, -3.300289026999228881, 32.46337939537708905 ) ) ;
#34712=ORIENTED_EDGE ( 'NONE', *, *, #68195, .T. ) ;
#34713=ORIENTED_EDGE ( 'NONE', *, *, #84971, .T. ) ;
#34714=ORIENTED_EDGE ( 'NONE', *, *, #84510, .T. ) ;
#34715=DIRECTION ( 'NONE',  ( -0.000000000000000000, 0.9396926207859092051, -0.3420201433256662704 ) ) ;
#34716=ORIENTED_EDGE ( 'NONE', *, *, #52412, .F. ) ;
#34717=CARTESIAN_POINT ( 'NONE',  ( -9.561782254074048026, -10.31582465632705237, 34.18122507451815295 ) ) ;
#34718=CARTESIAN_POINT ( 'NONE',  ( -12.23852710992561299, -6.503523203565941380, 34.64991518177335195 ) ) ;
#34720=CARTESIAN_POINT ( 'NONE',  ( -8.769230769230892619, -5.094484230521993062, 34.41647553114689373 ) ) ;
#34721=CYLINDRICAL_SURFACE ( 'NONE', #30235, 0.2499999999999986955 ) ;
#34722=ORIENTED_EDGE ( 'NONE', *, *, #86116, .F. ) ;
#34723=CARTESIAN_POINT ( 'NONE',  ( 4.403846153846153300, -2.249999999999998668, 29.75000000000000355 ) ) ;
#34724=LINE ( 'NONE', #27968, #51072 ) ;
#34725=ORIENTED_EDGE ( 'NONE', *, *, #48556, .T. ) ;
#34726=CARTESIAN_POINT ( 'NONE',  ( -17.07692307692307665, -8.164416787775445883, 34.95778746994557906 ) ) ;
#34727=CARTESIAN_POINT ( 'NONE',  ( -10.55012904410858710, -3.835265460703683349, 33.15142922261929925 ) ) ;
#34729=AXIS2_PLACEMENT_3D ( 'NONE', #52260, #18491, #73437 ) ;
#34730=CARTESIAN_POINT ( 'NONE',  ( 9.019285189144222059, -12.01375889529407281, 32.43194544308182969 ) ) ;
#34731=DIRECTION ( 'NONE',  ( -0.000000000000000000, -0.3420201433256694901, -0.9396926207859082059 ) ) ;
#34732=CARTESIAN_POINT ( 'NONE',  ( 9.442284455014730682, -10.05641848906368097, 34.04755513067966177 ) ) ;
#34733=CARTESIAN_POINT ( 'NONE',  ( -2.980769230769166445, -7.434744860731434812, 35.00000000000000711 ) ) ;
#34735=ORIENTED_EDGE ( 'NONE', *, *, #85194, .T. ) ;
#34736=CARTESIAN_POINT ( 'NONE',  ( -3.230769230769229949, -6.343179335718451384, 34.87096338111211935 ) ) ;
#34737=CARTESIAN_POINT ( 'NONE',  ( 0.7114839798866033904, -3.202959910592335202, 32.30730279482227019 ) ) ;
#34739=CARTESIAN_POINT ( 'NONE',  ( -7.173076923076921574, -7.500000000000001776, 35.04278698407183867 ) ) ;
#34740=VERTEX_POINT ( 'NONE', #21187 ) ;
#34742=CARTESIAN_POINT ( 'NONE',  ( 11.40831356872984514, -4.299443229763728169, 33.91186481527756058 ) ) ;
#34743=CARTESIAN_POINT ( 'NONE',  ( -3.480769230769229061, -2.249999999999998668, 29.75000000000000355 ) ) ;
#34744=DIRECTION ( 'NONE',  ( -0.000000000000000000, -0.000000000000000000, -1.000000000000000000 ) ) ;
#34745=EDGE_LOOP ( 'NONE', ( #54996, #81304, #50600, #66032 ) ) ;
#34746=CARTESIAN_POINT ( 'NONE',  ( 3.230769230769231726, -11.91647553114624181, 32.58852847137148245 ) ) ;
#34747=EDGE_CURVE ( 'NONE', #27559, #66547, #62175, .T. ) ;
#34748=CARTESIAN_POINT ( 'NONE',  ( 3.296837581771669967, -12.10708131394839704, 31.69288490824020954 ) ) ;
#34749=CARTESIAN_POINT ( 'NONE',  ( 7.780883400193070898, -10.21337939537584383, 33.94971097300158647 ) ) ;
#34750=ORIENTED_EDGE ( 'NONE', *, *, #59703, .F. ) ;
#34752=VECTOR ( 'NONE', #8786, 1000.000000000000114 ) ;
#34753=EDGE_LOOP ( 'NONE', ( #59282, #87316, #2418, #38953 ) ) ;
#34754=CARTESIAN_POINT ( 'NONE',  ( -17.07692307692307665, -13.53365097954675988, 30.81389545987213552 ) ) ;
#34756=ORIENTED_EDGE ( 'NONE', *, *, #60146, .T. ) ;
#34757=FACE_OUTER_BOUND ( 'NONE', #26068, .T. ) ;
#34758=CARTESIAN_POINT ( 'NONE',  ( -14.53061926659915315, -2.308479472611653094, 30.53278059502174457 ) ) ;
#34759=CARTESIAN_POINT ( 'NONE',  ( -11.53846153846153655, -6.386643153685126251, 34.62446782046654192 ) ) ;
#34760=VECTOR ( 'NONE', #23314, 999.9999999999998863 ) ;
#34761=CARTESIAN_POINT ( 'NONE',  ( -1.384615384615383471, -1.242168528481310874, 33.36296068462461051 ) ) ;
#34762=CARTESIAN_POINT ( 'NONE',  ( 3.296837581771669967, -12.37446782046654192, 30.86335684631486842 ) ) ;
#34764=ORIENTED_EDGE ( 'NONE', *, *, #65649, .T. ) ;
#34765=FACE_BOUND ( 'NONE', #74785, .T. ) ;
#34766=ORIENTED_EDGE ( 'NONE', *, *, #62074, .T. ) ;
#34767=CARTESIAN_POINT ( 'NONE',  ( 7.846153846153846700, -12.29105614889573062, 35.45975837776705220 ) ) ;
#34768=ADVANCED_FACE ( 'NONE', ( #27953 ), #13989, .F. ) ;
#34769=CARTESIAN_POINT ( 'NONE',  ( 5.076923076922954969, -11.94971097300221174, 32.03036669348237098 ) ) ;
#34770=CARTESIAN_POINT ( 'NONE',  ( -2.307692307692305711, -2.499999999999998668, 29.75000000000001421 ) ) ;
#34771=CARTESIAN_POINT ( 'NONE',  ( 6.989145274079363368, -9.780366693483667717, 34.19971097300155805 ) ) ;
#34772=VERTEX_POINT ( 'NONE', #1359 ) ;
#34774=ORIENTED_EDGE ( 'NONE', *, *, #49220, .T. ) ;
#34775=B_SPLINE_CURVE_WITH_KNOTS ( 'NONE', 3,
 ( #9162, #1951, #23536, #50993, #2375, #77165, #71279, #84380, #9584, #29436 ),
 .UNSPECIFIED., .F., .F.,
 ( 4, 2, 2, 2, 4 ),
 ( 0.000000000000000000, 0.0001954339857564073388, 0.0003908679715128146777, 0.0005863019572692220165, 0.0007817359430256293554 ),
 .UNSPECIFIED. ) ;
#34776=VECTOR ( 'NONE', #86554, 1000.000000000000114 ) ;
#34777=CARTESIAN_POINT ( 'NONE',  ( -10.74553258511630993, -8.630895178749533159, 34.87696386517710323 ) ) ;
#34778=ORIENTED_EDGE ( 'NONE', *, *, #79259, .F. ) ;
#34779=DIRECTION ( 'NONE',  ( -0.000000000000000000, 0.8660254037844399289, -0.4999999999999980016 ) ) ;
#34780=AXIS2_PLACEMENT_3D ( 'NONE', #7396, #35756, #82624 ) ;
#34781=CARTESIAN_POINT ( 'NONE',  ( -16.85354713622489342, -2.501478030877323011, 29.88021232661721172 ) ) ;
#34782=FACE_OUTER_BOUND ( 'NONE', #41648, .T. ) ;
#34783=CARTESIAN_POINT ( 'NONE',  ( 16.28463659481310799, -2.295524264805589354, 30.44142389570982488 ) ) ;
#34785=CARTESIAN_POINT ( 'NONE',  ( -14.08491263871423982, -12.69155399931963046, 30.53255429739157734 ) ) ;
#34786=CARTESIAN_POINT ( 'NONE',  ( -18.22559223176555321, -7.628091957228972930, 34.99866226681163539 ) ) ;
#34787=CARTESIAN_POINT ( 'NONE',  ( -8.769230769230892619, -3.083524468854526912, 32.58852847137268327 ) ) ;
#34788=ORIENTED_EDGE ( 'NONE', *, *, #22741, .F. ) ;
#34790=VERTEX_POINT ( 'NONE', #76584 ) ;
#34791=CARTESIAN_POINT ( 'NONE',  ( -9.692307692307691624, -13.20930481340135110, 34.54067556320372745 ) ) ;
#34792=FACE_OUTER_BOUND ( 'NONE', #38298, .T. ) ;
#34793=CARTESIAN_POINT ( 'NONE',  ( 10.74591031714818179, -6.852161475712352789, 34.70806712695775786 ) ) ;
#34794=CARTESIAN_POINT ( 'NONE',  ( 1.607395053593450474, -12.47679350104403007, 31.42216943046557276 ) ) ;
#34795=LINE ( 'NONE', #29824, #29328 ) ;
#34796=FACE_OUTER_BOUND ( 'NONE', #84249, .T. ) ;
#34797=CARTESIAN_POINT ( 'NONE',  ( 9.692307692307572609, -3.835265460704628371, 33.15142922262033665 ) ) ;
#34798=ORIENTED_EDGE ( 'NONE', *, *, #6606, .T. ) ;
#34799=FACE_OUTER_BOUND ( 'NONE', #70916, .T. ) ;
#34800=CARTESIAN_POINT ( 'NONE',  ( -8.769230769230768274, -3.050289026998446396, 32.03036669348365706 ) ) ;
#34801=VECTOR ( 'NONE', #22992, 1000.000000000000000 ) ;
#34802=CARTESIAN_POINT ( 'NONE',  ( -14.30769230769230660, -13.53365097954675988, 30.81389545987213552 ) ) ;
#34803=CARTESIAN_POINT ( 'NONE',  ( -5.999999999999998224, -1.951392089020283160, 34.73218667398347748 ) ) ;
#34804=EDGE_LOOP ( 'NONE', ( #46887, #51496 ) ) ;
#34805=CARTESIAN_POINT ( 'NONE',  ( 18.24994551834813805, -12.43552623307873972, 30.55307653245132826 ) ) ;
#34806=VERTEX_POINT ( 'NONE', #69821 ) ;
#34807=FACE_BOUND ( 'NONE', #4000, .T. ) ;
#34808=CARTESIAN_POINT ( 'NONE',  ( 9.561616225640133138, -5.582088688514999397, 34.36776431015576350 ) ) ;
#34810=CARTESIAN_POINT ( 'NONE',  ( -12.23852710992561299, -8.239487800360276282, 34.69522927552633718 ) ) ;
#34811=FACE_OUTER_BOUND ( 'NONE', #3556, .T. ) ;
#34812=ORIENTED_EDGE ( 'NONE', *, *, #11464, .T. ) ;
#34814=CARTESIAN_POINT ( 'NONE',  ( -14.53061852520844965, -4.186968288167449259, 33.49512374952580274 ) ) ;
#34815=CARTESIAN_POINT ( 'NONE',  ( 6.699591979352976345, -12.44517049084099725, 30.48991314939691932 ) ) ;
#34816=CARTESIAN_POINT ( 'NONE',  ( -7.173100160369890510, -10.76384336483936011, 33.53834819971076087 ) ) ;
#34817=ORIENTED_EDGE ( 'NONE', *, *, #22136, .F. ) ;
#34818=EDGE_CURVE ( 'NONE', #29700, #84739, #38457, .T. ) ;
#34819=B_SPLINE_CURVE_WITH_KNOTS ( 'NONE', 3,
 ( #41965, #41073, #34306, #81619, #68107, #74869, #20793, #61768, #33864, #19904 ),
 .UNSPECIFIED., .F., .F.,
 ( 4, 2, 2, 2, 4 ),
 ( 0.0007817246336856291692, 0.0009771112958940105907, 0.001172497958102391904, 0.001367884620310773434, 0.001563271282519154747 ),
 .UNSPECIFIED. ) ;
#34820=B_SPLINE_CURVE_WITH_KNOTS ( 'NONE', 3,
 ( #4223, #38912, #45199, #59607, #79888, #86669, #18189, #39359, #66370, #5115 ),
 .UNSPECIFIED., .F., .F.,
 ( 4, 2, 2, 2, 4 ),
 ( 0.0007817359430256301143, 0.0009771253907249963233, 0.001172514838424362641, 0.001367904286123728958, 0.001563293733823095059 ),
 .UNSPECIFIED. ) ;
#34821=CARTESIAN_POINT ( 'NONE',  ( 16.15384615384615330, -10.51840700105979565, 33.73612834413961536 ) ) ;
#34822=CARTESIAN_POINT ( 'NONE',  ( 11.53846153846153832, -12.48256725967547354, 35.29906147534542527 ) ) ;
#34823=CARTESIAN_POINT ( 'NONE',  ( -8.834501215191544077, -3.835265460703609186, 33.15142922261924241 ) ) ;
#34824=VERTEX_POINT ( 'NONE', #22082 ) ;
#34825=CARTESIAN_POINT ( 'NONE',  ( -5.076923076923075762, -12.48256725967547354, 35.29906147534542527 ) ) ;
#34826=CARTESIAN_POINT ( 'NONE',  ( 4.153846153846154188, -13.75783147151868846, 33.36296068462461051 ) ) ;
#34827=CARTESIAN_POINT ( 'NONE',  ( 13.25392391794783009, -8.999036380462717588, 34.52022231692819076 ) ) ;
#34828=B_SPLINE_CURVE_WITH_KNOTS ( 'NONE', 3,
 ( #58478, #45417, #50397, #16183, #3544, #17518, #38671, #71558, #66134, #4439 ),
 .UNSPECIFIED., .F., .F.,
 ( 4, 2, 2, 2, 4 ),
 ( 0.000000000000000000, 0.0001954339857564079623, 0.0003908679715128159245, 0.0005863019572692238597, 0.0007817359430256318490 ),
 .UNSPECIFIED. ) ;
#34829=CARTESIAN_POINT ( 'NONE',  ( -10.39260507411620260, -2.600157965045224451, 30.74683119005207743 ) ) ;
#34830=CARTESIAN_POINT ( 'NONE',  ( 17.07692307692295586, -5.094484230521993062, 34.41647553114689373 ) ) ;
#34831=CYLINDRICAL_SURFACE ( 'NONE', #63473, 0.2499999999999997502 ) ;
#34835=EDGE_LOOP ( 'NONE', ( #81888, #42596, #54051, #70352 ) ) ;
#34836=CARTESIAN_POINT ( 'NONE',  ( 2.307692307692309264, -12.78798330534102767, 29.49999999999997868 ) ) ;
#34837=EDGE_LOOP ( 'NONE', ( #75108, #37454, #60725, #23684 ) ) ;
#34838=EDGE_CURVE ( 'NONE', #55677, #45298, #1928, .T. ) ;
#34840=CYLINDRICAL_SURFACE ( 'NONE', #84422, 0.2500000000000009437 ) ;
#34841=ORIENTED_EDGE ( 'NONE', *, *, #38878, .T. ) ;
#34842=FACE_OUTER_BOUND ( 'NONE', #42565, .T. ) ;
#34843=EDGE_CURVE ( 'NONE', #68924, #89067, #24737, .T. ) ;
#34845=CARTESIAN_POINT ( 'NONE',  ( -15.93106661257773560, -5.913360116392398780, 34.49180327182771322 ) ) ;
#34846=CARTESIAN_POINT ( 'NONE',  ( 8.769230769230768274, -12.29105614889573062, 35.45975837776705220 ) ) ;
#34847=CARTESIAN_POINT ( 'NONE',  ( -7.846153846153844924, -1.129524287112498415, 32.06866353760679544 ) ) ;
#34849=CARTESIAN_POINT ( 'NONE',  ( -4.403822884788509029, -3.627789207965226748, 32.91389620160131102 ) ) ;
#34850=CARTESIAN_POINT ( 'NONE',  ( -0.7115616988314262814, -2.587272538249754117, 30.68239716806877837 ) ) ;
#34851=CARTESIAN_POINT ( 'NONE',  ( -2.057746898314263273, -2.986452184633681117, 32.43230066228895225 ) ) ;
#34852=ADVANCED_FACE ( 'NONE', ( #37803 ), #37348, .F. ) ;
#34854=DIRECTION ( 'NONE',  ( -0.000000000000000000, -0.9848077530122086864, -0.1736481776669273613 ) ) ;
#34855=CARTESIAN_POINT ( 'NONE',  ( -7.911424292114620727, -8.613356846314824011, 34.62446782046655613 ) ) ;
#34856=EDGE_CURVE ( 'NONE', #75329, #73584, #16532, .T. ) ;
#34857=VERTEX_POINT ( 'NONE', #52198 ) ;
#34858=VERTEX_POINT ( 'NONE', #72474 ) ;
#34859=CARTESIAN_POINT ( 'NONE',  ( -15.00775787915638304, -8.239487800360276282, 34.69522927552633718 ) ) ;
#34860=CARTESIAN_POINT ( 'NONE',  ( 5.076923076922954969, -9.442884908241554243, 34.35708131394783038 ) ) ;
#34861=CARTESIAN_POINT ( 'NONE',  ( -6.857821783564084228, -12.16647553114626490, 32.15551576947920864 ) ) ;
#34862=CARTESIAN_POINT ( 'NONE',  ( 0.3962684609821410242, -10.33852847137145226, 34.16647553114627556 ) ) ;
#34863=B_SPLINE_CURVE_WITH_KNOTS ( 'NONE', 3,
 ( #66738, #45572, #30290, #10467, #11802, #71706, #11347, #24854, #37935, #65398 ),
 .UNSPECIFIED., .F., .F.,
 ( 4, 2, 2, 2, 4 ),
 ( 0.0007817359430256360774, 0.0009771253907250041296, 0.001172514838424371965, 0.001367904286123740017, 0.001563293733823108069 ),
 .UNSPECIFIED. ) ;
#34864=CARTESIAN_POINT ( 'NONE',  ( 9.758375025657770152, -11.35647404775217595, 33.31231777344666511 ) ) ;
#34865=CARTESIAN_POINT ( 'NONE',  ( -6.249976730942353953, -8.303909089506435137, 34.68538101551103381 ) ) ;
#34867=EDGE_CURVE ( 'NONE', #43627, #8235, #29848, .T. ) ;
#34869=CARTESIAN_POINT ( 'NONE',  ( -13.51476259405360203, -10.19110544564092002, 33.96427741523702792 ) ) ;
#34871=ORIENTED_EDGE ( 'NONE', *, *, #70006, .T. ) ;
#34873=CARTESIAN_POINT ( 'NONE',  ( 13.13459216039392885, -12.45566812827425451, 31.48439005359158926 ) ) ;
#34874=AXIS2_PLACEMENT_3D ( 'NONE', #67681, #88416, #69000 ) ;
#34876=EDGE_CURVE ( 'NONE', #49681, #57294, #52531, .T. ) ;
#34877=DIRECTION ( 'NONE',  ( 0.000000000000000000, 0.000000000000000000, 1.000000000000000000 ) ) ;
#34879=CARTESIAN_POINT ( 'NONE',  ( -15.23076923076935074, -3.300289026999228881, 32.46337939537708905 ) ) ;
#34880=CYLINDRICAL_SURFACE ( 'NONE', #34990, 0.2500000000000002220 ) ;
#34882=VERTEX_POINT ( 'NONE', #3121 ) ;
#34883=VERTEX_POINT ( 'NONE', #71142 ) ;
#34884=VERTEX_POINT ( 'NONE', #9449 ) ;
#34885=VERTEX_POINT ( 'NONE', #17089 ) ;
#34886=CARTESIAN_POINT ( 'NONE',  ( -16.15384615384615330, -13.49023893513002648, 31.06009739812518688 ) ) ;
#34887=CARTESIAN_POINT ( 'NONE',  ( -12.59222906464876779, -12.62707690430377383, 30.88035979386743435 ) ) ;
#34888=CARTESIAN_POINT ( 'NONE',  ( 14.05766908347084865, -2.588893531581426988, 31.60682220781847818 ) ) ;
#34889=CARTESIAN_POINT ( 'NONE',  ( 14.08481279095472694, -7.630690623152299956, 34.99857592706774057 ) ) ;
#34890=CARTESIAN_POINT ( 'NONE',  ( 7.912320452745487565, -7.250054591869670162, 34.99404684341514127 ) ) ;
#34891=CARTESIAN_POINT ( 'NONE',  ( 14.30769230769231015, -10.05456864172156806, 36.03766855953608683 ) ) ;
#34892=VERTEX_POINT ( 'NONE', #36911 ) ;
#34893=ORIENTED_EDGE ( 'NONE', *, *, #61999, .F. ) ;
#34895=DIRECTION ( 'NONE',  ( -0.000000000000000000, -0.6427876096865404731, -0.7660444431189771253 ) ) ;
#34897=CARTESIAN_POINT ( 'NONE',  ( 10.48469314871706004, -12.38065189839062263, 30.83690757178629482 ) ) ;
#34898=DIRECTION ( 'NONE',  ( -1.000000000000000000, 0.000000000000000000, 0.000000000000000000 ) ) ;
#34899=EDGE_CURVE ( 'NONE', #69130, #68662, #44994, .T. ) ;
#34901=ORIENTED_EDGE ( 'NONE', *, *, #72524, .F. ) ;
#34902=EDGE_CURVE ( 'NONE', #57842, #22025, #30596, .T. ) ;
#34903=ORIENTED_EDGE ( 'NONE', *, *, #54738, .F. ) ;
#34904=CARTESIAN_POINT ( 'NONE',  ( 4.153846153846154188, -3.937682226553329556, 33.60647404775216529 ) ) ;
#34906=FACE_BOUND ( 'NONE', #16344, .T. ) ;
#34907=B_SPLINE_CURVE_WITH_KNOTS ( 'NONE', 3,
 ( #68280, #55642, #89020, #27295, #54760, #75926, #82248, #55204, #14224, #20535 ),
 .UNSPECIFIED., .F., .F.,
 ( 4, 2, 2, 2, 4 ),
 ( 0.000000000000000000, 0.0001954311564186866305, 0.0003908623128373732609, 0.0005862934692560598914, 0.0007817246256747465219 ),
 .UNSPECIFIED. ) ;
#34908=CARTESIAN_POINT ( 'NONE',  ( -2.307692307692305711, -4.661471528628507777, 34.16647553114623292 ) ) ;
#34909=EDGE_CURVE ( 'NONE', #24019, #16297, #65709, .T. ) ;
#34911=ORIENTED_EDGE ( 'NONE', *, *, #64050, .F. ) ;
#34912=CARTESIAN_POINT ( 'NONE',  ( -16.15384615384627409, -12.70778746994576025, 30.41441678777401236 ) ) ;
#34913=CARTESIAN_POINT ( 'NONE',  ( -14.30769230769230660, -2.538708090699994813, 30.37095296980875503 ) ) ;
#34915=CARTESIAN_POINT ( 'NONE',  ( 7.846153846153846700, -12.78798330534103123, 29.99999999999997868 ) ) ;
#34916=EDGE_LOOP ( 'NONE', ( #18392, #47052 ) ) ;
#34917=EDGE_CURVE ( 'NONE', #38437, #22109, #78338, .T. ) ;
#34918=CARTESIAN_POINT ( 'NONE',  ( 16.40384615384621725, -7.434744429011175271, 34.75000000000000711 ) ) ;
#34919=CARTESIAN_POINT ( 'NONE',  ( -5.749945580086545327, -4.074993327901525575, 33.72946981652012255 ) ) ;
#34920=CYLINDRICAL_SURFACE ( 'NONE', #55649, 0.2499999999999997502 ) ;
#34921=CYLINDRICAL_SURFACE ( 'NONE', #51502, 0.2499999999999998890 ) ;
#34922=CARTESIAN_POINT ( 'NONE',  ( -13.38461538461550582, -11.48612834414049644, 32.76840700105863391 ) ) ;
#34923=FACE_BOUND ( 'NONE', #24669, .T. ) ;
#34924=LINE ( 'NONE', #55197, #1642 ) ;
#34925=FACE_OUTER_BOUND ( 'NONE', #26112, .T. ) ;
#34926=CARTESIAN_POINT ( 'NONE',  ( -17.07692307692307665, -6.386643153685126251, 34.62446782046654192 ) ) ;
#34928=CARTESIAN_POINT ( 'NONE',  ( 8.899756470994327984, -2.882268652242222284, 31.66798894389554064 ) ) ;
#34929=CARTESIAN_POINT ( 'NONE',  ( -10.61538461538473577, -6.835583212225970762, 34.95778746994575670 ) ) ;
#34931=VERTEX_POINT ( 'NONE', #51737 ) ;
#34932=B_SPLINE_CURVE_WITH_KNOTS ( 'NONE', 3,
 ( #33409, #81158, #47350, #18561, #87480, #79823, #66293, #40175, #39285, #19003 ),
 .UNSPECIFIED., .F., .F.,
 ( 4, 2, 2, 2, 4 ),
 ( 0.0007817246256747484735, 0.0009771112852218928873, 0.001172497944769037084, 0.001367884604316181498, 0.001563271263863325912 ),
 .UNSPECIFIED. ) ;
#34933=AXIS2_PLACEMENT_3D ( 'NONE', #77234, #7896, #56957 ) ;
#34934=CARTESIAN_POINT ( 'NONE',  ( -8.638392351218003640, -7.277220443632450575, 34.74524770363009196 ) ) ;
#34935=ORIENTED_EDGE ( 'NONE', *, *, #87946, .F. ) ;
#34936=AXIS2_PLACEMENT_3D ( 'NONE', #55269, #41321, #73788 ) ;
#34937=CARTESIAN_POINT ( 'NONE',  ( -13.25382494364843389, -9.084667340241226796, 34.75534355489798344 ) ) ;
#34938=EDGE_LOOP ( 'NONE', ( #73519, #29383, #11093, #47626 ) ) ;
#34940=CARTESIAN_POINT ( 'NONE',  ( -7.846153846153965716, -10.21337939537710326, 33.94971097300076224 ) ) ;
#34941=ORIENTED_EDGE ( 'NONE', *, *, #38871, .F. ) ;
#34942=CARTESIAN_POINT ( 'NONE',  ( -9.627161912975726210, -7.750023238201979581, 34.74374492549440419 ) ) ;
#34945=VECTOR ( 'NONE', #45163, 1000.000000000000114 ) ;
#34946=CARTESIAN_POINT ( 'NONE',  ( 4.023698944407932743, -9.418419913701741919, 34.36755862841477693 ) ) ;
#34947=CARTESIAN_POINT ( 'NONE',  ( -5.143005456283213483, -2.833524468853757305, 32.15551576947924417 ) ) ;
#34948=CYLINDRICAL_SURFACE ( 'NONE', #5635, 0.2499999999999973355 ) ;
#34949=CARTESIAN_POINT ( 'NONE',  ( -1.384615384615383471, -8.318370150425687726, 35.83090037661290239 ) ) ;
#34950=CARTESIAN_POINT ( 'NONE',  ( -0.2385271099256122129, -4.187068189119697692, 33.49521262558774026 ) ) ;
#34951=LINE ( 'NONE', #34071, #59834 ) ;
#34952=B_SPLINE_CURVE_WITH_KNOTS ( 'NONE', 3,
 ( #1615, #55656, #83147, #29102, #56557, #84046 ),
 .UNSPECIFIED., .F., .F.,
 ( 4, 2, 4 ),
 ( 0.0003909512603273918637, 0.0005862562993132197772, 0.0007815613382990476907 ),
 .UNSPECIFIED. ) ;
#34954=CARTESIAN_POINT ( 'NONE',  ( -9.942284423250045577, -3.627789207965226748, 32.91389620160131102 ) ) ;
#34955=CARTESIAN_POINT ( 'NONE',  ( -5.999999999999998224, -3.050289026998446396, 32.03036669348365706 ) ) ;
#34957=CARTESIAN_POINT ( 'NONE',  ( -3.230769230769351186, -3.300289026999228881, 32.46337939537708905 ) ) ;
#34958=B_SPLINE_CURVE_WITH_KNOTS ( 'NONE', 3,
 ( #56867, #2357, #29851, #15455, #48783, #22638, #49235, #15010, #76250, #57315 ),
 .UNSPECIFIED., .F., .F.,
 ( 4, 2, 2, 2, 4 ),
 ( 0.000000000000000000, 0.0001954339857564093175, 0.0003908679715128186350, 0.0005863019572692279796, 0.0007817359430256372700 ),
 .UNSPECIFIED. ) ;
#34960=CARTESIAN_POINT ( 'NONE',  ( 2.084765348785459604, -4.762599654559228846, 34.23009711892697737 ) ) ;
#34961=CARTESIAN_POINT ( 'NONE',  ( -8.899921372341079717, -11.37499894934982692, 33.29245874905763003 ) ) ;
#34962=ORIENTED_EDGE ( 'NONE', *, *, #61553, .T. ) ;
#34963=CARTESIAN_POINT ( 'NONE',  ( 14.37294787896833625, -2.625532179533470512, 30.86335684631491105 ) ) ;
#34964=CARTESIAN_POINT ( 'NONE',  ( -14.30769230769242739, -11.48612834414049644, 32.76840700105863391 ) ) ;
#34965=CARTESIAN_POINT ( 'NONE',  ( -17.20739978503954148, -7.276988635370451597, 34.74523720219453793 ) ) ;
#34966=ORIENTED_EDGE ( 'NONE', *, *, #55926, .F. ) ;
#34967=CARTESIAN_POINT ( 'NONE',  ( 8.519207545009310323, -5.765609946408404518, 34.70566812827425451 ) ) ;
#34968=CARTESIAN_POINT ( 'NONE',  ( -3.100243529005666687, -5.195472089885680766, 34.18748526763464923 ) ) ;
#34969=CARTESIAN_POINT ( 'NONE',  ( 4.153846153846154188, -12.48256725967547354, 35.29906147534542527 ) ) ;
#34971=CARTESIAN_POINT ( 'NONE',  ( -9.692307692307691624, -2.486705287966279876, 31.30864560766543647 ) ) ;
#34972=CARTESIAN_POINT ( 'NONE',  ( -18.24997673094235395, -12.17611988154120795, 31.52148481390971213 ) ) ;
#34973=EDGE_CURVE ( 'NONE', #71827, #4784, #70676, .T. ) ;
#34975=ORIENTED_EDGE ( 'NONE', *, *, #68061, .F. ) ;
#34976=VERTEX_POINT ( 'NONE', #80589 ) ;
#34977=EDGE_CURVE ( 'NONE', #56750, #27705, #34143, .T. ) ;
#34978=ORIENTED_EDGE ( 'NONE', *, *, #56606, .T. ) ;
#34979=CARTESIAN_POINT ( 'NONE',  ( -13.45069879557126491, -3.513871655860377086, 32.76840700105978499 ) ) ;
#34980=LINE ( 'NONE', #48940, #27054 ) ;
#34981=ADVANCED_FACE ( 'NONE', ( #46343 ), #74717, .F. ) ;
#34982=DIRECTION ( 'NONE',  ( -0.000000000000000000, 0.5000000000000011102, -0.8660254037844381525 ) ) ;
#34983=CARTESIAN_POINT ( 'NONE',  ( -3.230769230769229949, -2.249999999999998668, 29.50000000000001421 ) ) ;
#34984=B_SPLINE_CURVE_WITH_KNOTS ( 'NONE', 3,
 ( #70859, #2373, #9161, #29868, #57331, #78044, #35289, #43813, #7825, #71277 ),
 .UNSPECIFIED., .F., .F.,
 ( 4, 2, 2, 2, 4 ),
 ( 0.000000000000000000, 0.0001954339857564081520, 0.0003908679715128163040, 0.0005863019572692244018, 0.0007817359430256326080 ),
 .UNSPECIFIED. ) ;
#34985=VERTEX_POINT ( 'NONE', #88248 ) ;
#34987=ORIENTED_EDGE ( 'NONE', *, *, #35682, .T. ) ;
#34988=B_SPLINE_CURVE_WITH_KNOTS ( 'NONE', 3,
 ( #8564, #15320, #56301, #1795, #29283, #56740, #63929, #42357, #28380, #77458 ),
 .UNSPECIFIED., .F., .F.,
 ( 4, 2, 2, 2, 4 ),
 ( 0.0007817246256747435946, 0.0009771112852218863821, 0.001172497944769029061, 0.001367884604316171957, 0.001563271263863314636 ),
 .UNSPECIFIED. ) ;
#34989=ORIENTED_EDGE ( 'NONE', *, *, #70344, .F. ) ;
#34990=AXIS2_PLACEMENT_3D ( 'NONE', #74108, #82647, #33995 ) ;
#34991=ORIENTED_EDGE ( 'NONE', *, *, #63089, .T. ) ;
#34992=CARTESIAN_POINT ( 'NONE',  ( 8.769230769230645706, -12.51329471203414379, 31.30864560766407578 ) ) ;
#34994=CARTESIAN_POINT ( 'NONE',  ( -4.946397638689431275, -12.50538340440932217, 31.33453814440721885 ) ) ;
#34996=CARTESIAN_POINT ( 'NONE',  ( 5.999999999999878320, -2.657715359629662988, 31.77849191805970364 ) ) ;
#34998=CIRCLE ( 'NONE', #85356, 0.2500000000000002220 ) ;
#34999=EDGE_CURVE ( 'NONE', #54833, #86900, #78176, .T. ) ;
#35000=DIRECTION ( 'NONE',  ( -0.000000000000000000, 0.7660444431189791237, -0.6427876096865379196 ) ) ;
#35001=CARTESIAN_POINT ( 'NONE',  ( 6.923076923076924238, -12.48256725967547354, 35.29906147534542527 ) ) ;
#35002=ORIENTED_EDGE ( 'NONE', *, *, #21795, .T. ) ;
#35003=ORIENTED_EDGE ( 'NONE', *, *, #32784, .F. ) ;
#35004=EDGE_LOOP ( 'NONE', ( #22993, #55596, #58422, #81136 ) ) ;
#35005=CARTESIAN_POINT ( 'NONE',  ( -2.241624974342231180, -3.322132147404559976, 32.92929555188717927 ) ) ;
#35006=LINE ( 'NONE', #40891, #68896 ) ;
#35007=VERTEX_POINT ( 'NONE', #87804 ) ;
#35008=CARTESIAN_POINT ( 'NONE',  ( 9.561616225640136690, -11.71456829005830080, 32.44064028649416542 ) ) ;
#35009=ADVANCED_FACE ( 'NONE', ( #81032 ), #88688, .F. ) ;
#35010=CARTESIAN_POINT ( 'NONE',  ( 24.00000000000000000, -5.499999999999981348, 27.25000000000000000 ) ) ;
#35011=VERTEX_POINT ( 'NONE', #87351 ) ;
#35012=CARTESIAN_POINT ( 'NONE',  ( 14.98074599347626368, -10.76384336483936011, 33.53834819971076087 ) ) ;
#35013=CARTESIAN_POINT ( 'NONE',  ( -15.16470189741915320, -12.34228464037088813, 31.77849191805839268 ) ) ;
#35015=FACE_BOUND ( 'NONE', #34554, .T. ) ;
#35016=EDGE_CURVE ( 'NONE', #53989, #56689, #46789, .T. ) ;
#35017=CARTESIAN_POINT ( 'NONE',  ( -17.75005448165186195, -8.433404298154332679, 34.66254593164985920 ) ) ;
#35018=DIRECTION ( 'NONE',  ( 0.000000000000000000, 0.000000000000000000, 1.000000000000000000 ) ) ;
#35019=CARTESIAN_POINT ( 'NONE',  ( 12.23805353697412812, -6.716662450894489211, 34.94144148231605840 ) ) ;
#35021=CARTESIAN_POINT ( 'NONE',  ( 18.06606835100243913, -4.098570777380720287, 33.41473453929635440 ) ) ;
#35022=CARTESIAN_POINT ( 'NONE',  ( 5.076923076923075762, -13.57706302396349152, 30.56769352161908060 ) ) ;
#35025=CARTESIAN_POINT ( 'NONE',  ( -7.846153846153967493, -6.835583212225970762, 34.95778746994575670 ) ) ;
#35026=CARTESIAN_POINT ( 'NONE',  ( 13.51545380262814788, -7.277220443632450575, 34.74524770363009196 ) ) ;
#35027=EDGE_LOOP ( 'NONE', ( #4424, #64381, #54348, #74932 ) ) ;
#35028=ADVANCED_FACE ( 'NONE', ( #74266 ), #12563, .F. ) ;
#35029=LINE ( 'NONE', #28271, #81854 ) ;
#35030=DIRECTION ( 'NONE',  ( -0.000000000000000000, -0.000000000000000000, -1.000000000000000000 ) ) ;
#35031=B_SPLINE_CURVE_WITH_KNOTS ( 'NONE', 3,
 ( #7051, #7503, #48027, #34960, #89048, #47593, #75507, #5722, #53908, #13806 ),
 .UNSPECIFIED., .F., .F.,
 ( 4, 2, 2, 2, 4 ),
 ( 0.000000000000000000, 0.0001954311564186874978, 0.0003908623128373749957, 0.0005862934692560624935, 0.0007817246256747499913 ),
 .UNSPECIFIED. ) ;
#35032=ORIENTED_EDGE ( 'NONE', *, *, #64848, .T. ) ;
#35033=CARTESIAN_POINT ( 'NONE',  ( -9.942330916529149576, -9.356822207818506598, 34.66110646841856635 ) ) ;
#35034=CARTESIAN_POINT ( 'NONE',  ( -18.00000000000000000, -12.75000000000000888, 29.74999999999997868 ) ) ;
#35035=FACE_BOUND ( 'NONE', #34507, .T. ) ;
#35037=FACE_OUTER_BOUND ( 'NONE', #19185, .T. ) ;
#35038=CARTESIAN_POINT ( 'NONE',  ( 18.00000000000000000, -13.63283147151868846, 33.57946703557072254 ) ) ;
#35039=DIRECTION ( 'NONE',  ( -0.000000000000000000, 0.7660444431189791237, -0.6427876096865379196 ) ) ;
#35040=CARTESIAN_POINT ( 'NONE',  ( -15.45425417449318317, -9.331801661448606566, 34.40259984581193464 ) ) ;
#35043=CARTESIAN_POINT ( 'NONE',  ( -14.08491263871423982, -5.827830569534417471, 34.72679350104403539 ) ) ;
#35045=VERTEX_POINT ( 'NONE', #75158 ) ;
#35046=ORIENTED_EDGE ( 'NONE', *, *, #3721, .F. ) ;
#35048=CARTESIAN_POINT ( 'NONE',  ( -15.36091720050093024, -5.915902021225889484, 34.75552854090298638 ) ) ;
#35049=CARTESIAN_POINT ( 'NONE',  ( 1.384615384615264011, -9.528491918059723176, 34.59228464037033035 ) ) ;
#35050=CARTESIAN_POINT ( 'NONE',  ( -17.01085472592063752, -11.16473453929635440, 33.15142922261926373 ) ) ;
#35051=CARTESIAN_POINT ( 'NONE',  ( 3.007284287045284277, -11.41268669641500466, 32.86336882939237825 ) ) ;
#35053=EDGE_CURVE ( 'NONE', #19610, #53313, #41650, .T. ) ;
#35054=CARTESIAN_POINT ( 'NONE',  ( 0.6845513056318560663, -4.026326845037962343, 33.68677907613344047 ) ) ;
#35055=CARTESIAN_POINT ( 'NONE',  ( 5.869852030268303267, -3.069018819979302926, 32.56621877034667278 ) ) ;
#35056=EDGE_CURVE ( 'NONE', #77538, #44792, #85678, .T. ) ;
#35057=CARTESIAN_POINT ( 'NONE',  ( 9.626225312947561008, -10.67929555188718460, 33.92786785259543336 ) ) ;
#35058=CARTESIAN_POINT ( 'NONE',  ( 17.86930939688968678, -3.957541250942358424, 33.62499894934981626 ) ) ;
#35059=CARTESIAN_POINT ( 'NONE',  ( 16.15384615384615330, -9.058645607665452459, 34.76329471203371924 ) ) ;
#35060=CARTESIAN_POINT ( 'NONE',  ( 7.846153846153846700, -9.584722331328613620, 36.20867863119891439 ) ) ;
#35061=DIRECTION ( 'NONE',  ( -0.000000000000000000, -0.1736481776669307198, -0.9848077530122080203 ) ) ;
#35062=AXIS2_PLACEMENT_3D ( 'NONE', #35792, #8317, #1554 ) ;
#35063=CARTESIAN_POINT ( 'NONE',  ( -11.53846153846153655, -4.945431358278436385, 36.03766855953609394 ) ) ;
#35065=VERTEX_POINT ( 'NONE', #76025 ) ;
#35066=CARTESIAN_POINT ( 'NONE',  ( 12.33084785842815378, -3.957541250942358424, 33.62499894934981626 ) ) ;
#35067=CARTESIAN_POINT ( 'NONE',  ( 0.4615384615383396616, -2.625532179533779154, 30.86335684631627174 ) ) ;
#35069=AXIS2_PLACEMENT_3D ( 'NONE', #27340, #68766, #67884 ) ;
#35071=CARTESIAN_POINT ( 'NONE',  ( -5.777220331021931443, -12.47679350104403007, 31.42216943046555855 ) ) ;
#35072=CARTESIAN_POINT ( 'NONE',  ( -17.93393164899756087, -10.51840700105979387, 33.73612834413962247 ) ) ;
#35073=VERTEX_POINT ( 'NONE', #27844 ) ;
#35074=CARTESIAN_POINT ( 'NONE',  ( -16.21909714400740299, -2.506253911140460477, 30.00000000000013856 ) ) ;
#35075=CARTESIAN_POINT ( 'NONE',  ( -6.065322915492173728, -7.749976743299137993, 34.99404534957040624 ) ) ;
#35076=ORIENTED_EDGE ( 'NONE', *, *, #74588, .F. ) ;
#35077=CARTESIAN_POINT ( 'NONE',  ( 8.096208157792158744, -3.627508038966690496, 32.91356715214248396 ) ) ;
#35078=CYLINDRICAL_SURFACE ( 'NONE', #64194, 0.2500000000000008882 ) ;
#35080=CARTESIAN_POINT ( 'NONE',  ( -5.207614543590636913, -12.11776431015576172, 31.66791131148498906 ) ) ;
#35081=CARTESIAN_POINT ( 'NONE',  ( 13.13463864056679675, -9.234221910056348293, 34.70572697212741531 ) ) ;
#35083=CARTESIAN_POINT ( 'NONE',  ( -10.61538461538473577, -4.320704448113951379, 33.92786785259630022 ) ) ;
#35085=DIRECTION ( 'NONE',  ( -0.000000000000000000, -0.9848077530122086864, -0.1736481776669273613 ) ) ;
#35086=ORIENTED_EDGE ( 'NONE', *, *, #24867, .F. ) ;
#35087=ORIENTED_EDGE ( 'NONE', *, *, #81092, .T. ) ;
#35088=CARTESIAN_POINT ( 'NONE',  ( 6.065255571276025215, -6.879047030191282275, 34.71129190930002295 ) ) ;
#35089=ADVANCED_FACE ( 'NONE', ( #63840 ), #68828, .F. ) ;
#35090=ORIENTED_EDGE ( 'NONE', *, *, #69317, .F. ) ;
#35091=CARTESIAN_POINT ( 'NONE',  ( 7.846153846153723244, -9.528491918059723176, 34.59228464037033035 ) ) ;
#35092=CARTESIAN_POINT ( 'NONE',  ( 12.68431800280687050, -9.332535724633409302, 34.40230450496446934 ) ) ;
#35093=CARTESIAN_POINT ( 'NONE',  ( 2.438217745925951085, -11.66157788607254275, 32.95092075102925833 ) ) ;
#35094=EDGE_CURVE ( 'NONE', #29011, #83562, #12624, .T. ) ;
#35095=CARTESIAN_POINT ( 'NONE',  ( -2.530618525208453207, -5.667676309546437530, 34.40238873228292249 ) ) ;
#35096=CARTESIAN_POINT ( 'NONE',  ( -4.219929564802032296, -6.386643153685125363, 34.62446782046654903 ) ) ;
#35099=ADVANCED_FACE ( 'NONE', ( #43134 ), #8466, .F. ) ;
#35101=VERTEX_POINT ( 'NONE', #56643 ) ;
#35102=ORIENTED_EDGE ( 'NONE', *, *, #55268, .T. ) ;
#35103=CARTESIAN_POINT ( 'NONE',  ( 4.219101293358989757, -8.656820664281605460, 34.87096338111211224 ) ) ;
#35104=EDGE_LOOP ( 'NONE', ( #36523, #79038 ) ) ;
#35105=EDGE_CURVE ( 'NONE', #456, #31984, #1249, .T. ) ;
#35106=CARTESIAN_POINT ( 'NONE',  ( 17.01165307636676260, -2.379036618887870436, 30.90682066428148644 ) ) ;
#35107=ORIENTED_EDGE ( 'NONE', *, *, #38640, .T. ) ;
#35108=CARTESIAN_POINT ( 'NONE',  ( -17.77722045873158763, -3.236590943229503914, 32.36255958852954251 ) ) ;
#35109=CARTESIAN_POINT ( 'NONE',  ( -8.096130590202436750, -10.06842814019191401, 34.32929386961144758 ) ) ;
#35110=VERTEX_POINT ( 'NONE', #82801 ) ;
#35111=CARTESIAN_POINT ( 'NONE',  ( 7.912222197156284054, -8.120952969808772792, 34.71129190929999453 ) ) ;
#35113=ORIENTED_EDGE ( 'NONE', *, *, #70021, .F. ) ;
#35115=ORIENTED_EDGE ( 'NONE', *, *, #27790, .F. ) ;
#35116=CARTESIAN_POINT ( 'NONE',  ( -10.68114141789892102, -7.249945686854186278, 34.74374336980224598 ) ) ;
#35117=AXIS2_PLACEMENT_3D ( 'NONE', #40781, #26373, #47516 ) ;
#35118=VERTEX_POINT ( 'NONE', #13882 ) ;
#35119=CARTESIAN_POINT ( 'NONE',  ( 15.23076923076911093, -3.300289026999228881, 32.46337939537708905 ) ) ;
#35120=B_SPLINE_CURVE_WITH_KNOTS ( 'NONE', 3,
 ( #57964, #3458, #30058, #9779, #45332, #10673, #51178, #16534, #71919, #11566 ),
 .UNSPECIFIED., .F., .F.,
 ( 4, 2, 2, 2, 4 ),
 ( 0.000000000000000000, 0.0001954311564186863052, 0.0003908623128373726104, 0.0005862934692560589156, 0.0007817246256747452209 ),
 .UNSPECIFIED. ) ;
#35121=CARTESIAN_POINT ( 'NONE',  ( 16.82689983963011215, -2.823816976329320827, 31.52131813110797154 ) ) ;
#35122=FACE_BOUND ( 'NONE', #48068, .T. ) ;
#35123=EDGE_CURVE ( 'NONE', #23593, #48855, #87694, .T. ) ;
#35124=AXIS2_PLACEMENT_3D ( 'NONE', #7523, #54368, #69219 ) ;
#35125=CARTESIAN_POINT ( 'NONE',  ( -14.53117723225663482, -9.417330523894424488, 34.63758898049880486 ) ) ;
#35126=CARTESIAN_POINT ( 'NONE',  ( -6.792551221313357424, -12.27024696741798770, 31.24895572276497546 ) ) ;
#35128=CARTESIAN_POINT ( 'NONE',  ( 15.29683656411930848, -2.486705287966280320, 31.30864560766543647 ) ) ;
#35129=CARTESIAN_POINT ( 'NONE',  ( 12.23805353697412990, -3.562934362175799841, 33.22335522853832401 ) ) ;
#35130=CARTESIAN_POINT ( 'NONE',  ( 5.207448778686640800, -10.88167719472716399, 33.43325721877153711 ) ) ;
#35131=CARTESIAN_POINT ( 'NONE',  ( 10.61538461538449418, -11.06231777344772027, 33.60647404775119895 ) ) ;
#35132=ORIENTED_EDGE ( 'NONE', *, *, #58021, .T. ) ;
#35133=EDGE_CURVE ( 'NONE', #82999, #54572, #61998, .T. ) ;
#35134=CARTESIAN_POINT ( 'NONE',  ( -14.24162395668986747, -3.513871655860379306, 32.76840700105978499 ) ) ;
#35135=ORIENTED_EDGE ( 'NONE', *, *, #74705, .F. ) ;
#35136=ORIENTED_EDGE ( 'NONE', *, *, #75633, .T. ) ;
#35137=CARTESIAN_POINT ( 'NONE',  ( -1.134560964701931018, -4.818054556918156983, 34.26375889529406749 ) ) ;
#35138=CARTESIAN_POINT ( 'NONE',  ( -0.4615384615384611200, -12.37446782046654192, 30.86335684631486131 ) ) ;
#35139=CARTESIAN_POINT ( 'NONE',  ( -12.59168567097668223, -2.619462340734462380, 30.83744416345203021 ) ) ;
#35140=CARTESIAN_POINT ( 'NONE',  ( -16.82686865700962286, -10.06805714834173138, 34.32951233291982618 ) ) ;
#35141=CARTESIAN_POINT ( 'NONE',  ( 15.29602480204525783, -3.835265460703683349, 33.15142922261929925 ) ) ;
#35142=CARTESIAN_POINT ( 'NONE',  ( 18.00000000000000000, -13.20930481340135110, 34.54067556320372745 ) ) ;
#35143=ORIENTED_EDGE ( 'NONE', *, *, #35094, .T. ) ;
#35144=CARTESIAN_POINT ( 'NONE',  ( 11.31553457955469000, -3.395401636524185474, 33.02366814457250399 ) ) ;
#35145=ADVANCED_FACE ( 'NONE', ( #29191 ), #3900, .F. ) ;
#35146=DIRECTION ( 'NONE',  ( -0.000000000000000000, 0.7660444431189791237, -0.6427876096865379196 ) ) ;
#35147=CARTESIAN_POINT ( 'NONE',  ( -4.153846153846152411, -2.249999999999998668, 29.75000000000001776 ) ) ;
#35148=CARTESIAN_POINT ( 'NONE',  ( 3.100077764101671463, -3.062553014421049991, 32.05460306192774311 ) ) ;
#35149=CARTESIAN_POINT ( 'NONE',  ( -5.076923076923075762, -11.33034616979429110, 35.88435417666054406 ) ) ;
#35151=ORIENTED_EDGE ( 'NONE', *, *, #49248, .F. ) ;
#35153=EDGE_LOOP ( 'NONE', ( #84229, #61585, #36319, #8638 ) ) ;
#35155=ORIENTED_EDGE ( 'NONE', *, *, #20039, .F. ) ;
#35156=CARTESIAN_POINT ( 'NONE',  ( -9.442253272394237840, -10.06805714834173493, 34.32951233291982618 ) ) ;
#35158=LINE ( 'NONE', #22093, #79785 ) ;
#35159=CARTESIAN_POINT ( 'NONE',  ( -2.242436736416282717, -5.219633306516380244, 34.19971097300157936 ) ) ;
#35160=EDGE_CURVE ( 'NONE', #73867, #33320, #37252, .T. ) ;
#35161=B_SPLINE_CURVE_WITH_KNOTS ( 'NONE', 3,
 ( #58868, #60199, #87700, #18783, #46250, #53892, #45349, #87255, #39508, #59313 ),
 .UNSPECIFIED., .F., .F.,
 ( 4, 2, 2, 2, 4 ),
 ( 0.000000000000000000, 0.0001954311564186866305, 0.0003908623128373732609, 0.0005862934692560598914, 0.0007817246256747465219 ),
 .UNSPECIFIED. ) ;
#35162=CARTESIAN_POINT ( 'NONE',  ( 12.46153846153833911, -10.21337939537710326, 33.94971097300076224 ) ) ;
#35163=AXIS2_PLACEMENT_3D ( 'NONE', #14000, #7251, #47338 ) ;
#35164=EDGE_LOOP ( 'NONE', ( #16233, #42427 ) ) ;
#35166=DIRECTION ( 'NONE',  ( -0.000000000000000000, 0.6427876096865404731, -0.7660444431189771253 ) ) ;
#35167=ORIENTED_EDGE ( 'NONE', *, *, #32437, .T. ) ;
#35169=CYLINDRICAL_SURFACE ( 'NONE', #29767, 0.2500000000000009437 ) ;
#35170=CARTESIAN_POINT ( 'NONE',  ( 17.07692307692307665, -3.513871655860378418, 32.76840700105978499 ) ) ;
#35172=EDGE_CURVE ( 'NONE', #29433, #30896, #27544, .T. ) ;
#35173=CARTESIAN_POINT ( 'NONE',  ( 9.942362003946010773, -10.66356715214248752, 33.62249196103329751 ) ) ;
#35174=CARTESIAN_POINT ( 'NONE',  ( -17.77722033102192967, -10.97394488606064122, 33.68653795673696294 ) ) ;
#35175=CARTESIAN_POINT ( 'NONE',  ( -3.361459833879537840, -10.70098750199973203, 33.91152734681376302 ) ) ;
#35179=EDGE_CURVE ( 'NONE', #34683, #48673, #64051, .T. ) ;
#35180=CARTESIAN_POINT ( 'NONE',  ( -4.853959942656404181, -7.369474539155828730, 34.99858011523957657 ) ) ;
#35181=CARTESIAN_POINT ( 'NONE',  ( 1.134592160393928850, -9.356822207818506598, 34.66110646841856635 ) ) ;
#35182=CARTESIAN_POINT ( 'NONE',  ( -6.923076923076922462, -1.790695186598648903, 34.54067556320373455 ) ) ;
#35183=LINE ( 'NONE', #50021, #102 ) ;
#35184=EDGE_LOOP ( 'NONE', ( #76849, #16577 ) ) ;
#35186=CARTESIAN_POINT ( 'NONE',  ( -3.454254174493178731, -10.81261337010820256, 33.49550067578627477 ) ) ;
#35187=CARTESIAN_POINT ( 'NONE',  ( 14.08482604462921195, -2.251424796025574881, 29.88072029997477586 ) ) ;
#35188=CARTESIAN_POINT ( 'NONE',  ( -4.284537620513709122, -10.54014554554150607, 33.71984207302941883 ) ) ;
#35189=ORIENTED_EDGE ( 'NONE', *, *, #48054, .T. ) ;
#35190=CARTESIAN_POINT ( 'NONE',  ( 6.130525701763564150, -6.001044277235011215, 34.52024696741798948 ) ) ;
#35192=CARTESIAN_POINT ( 'NONE',  ( 7.976945653978634532, -5.582136614379148654, 34.36778462344220486 ) ) ;
#35193=CARTESIAN_POINT ( 'NONE',  ( -14.17685397720554441, -7.277220318596961057, 34.99547417642776992 ) ) ;
#35194=B_SPLINE_CURVE_WITH_KNOTS ( 'NONE', 3,
 ( #83795, #76128, #41465, #7685, #15770, #14430, #35596, #70264, #63045, #76581 ),
 .UNSPECIFIED., .F., .F.,
 ( 4, 2, 2, 2, 4 ),
 ( 0.000000000000000000, 0.0001954311564186863323, 0.0003908623128373726646, 0.0005862934692560590241, 0.0007817246256747453293 ),
 .UNSPECIFIED. ) ;
#35195=ORIENTED_EDGE ( 'NONE', *, *, #24750, .T. ) ;
#35196=DIRECTION ( 'NONE',  ( 0.000000000000000000, 0.6427876096865373645, -0.7660444431189797898 ) ) ;
#35198=AXIS2_PLACEMENT_3D ( 'NONE', #42488, #63631, #77596 ) ;
#35199=ORIENTED_EDGE ( 'NONE', *, *, #86142, .F. ) ;
#35200=CARTESIAN_POINT ( 'NONE',  ( -2.372962753653081514, -12.27809138561121394, 31.22303859784730307 ) ) ;
#35201=CARTESIAN_POINT ( 'NONE',  ( 6.130047606255684123, -7.723484964179500700, 34.74522123443823318 ) ) ;
#35202=ORIENTED_EDGE ( 'NONE', *, *, #61308, .F. ) ;
#35203=CARTESIAN_POINT ( 'NONE',  ( -17.86947456176635640, -10.31582465632705770, 34.18122507451815295 ) ) ;
#35204=CARTESIAN_POINT ( 'NONE',  ( 5.076923076923075762, -7.500000000000001776, 35.04278698407183867 ) ) ;
#35205=CARTESIAN_POINT ( 'NONE',  ( -10.68146802634049486, -5.557115091759785130, 34.35708131394839171 ) ) ;
#35206=CARTESIAN_POINT ( 'NONE',  ( -11.40793610022789650, -5.915461855592780260, 34.75538340440931506 ) ) ;
#35207=CYLINDRICAL_SURFACE ( 'NONE', #74225, 0.2500000000000002220 ) ;
#35208=ORIENTED_EDGE ( 'NONE', *, *, #5988, .T. ) ;
#35210=FACE_BOUND ( 'NONE', #38773, .T. ) ;
#35211=VERTEX_POINT ( 'NONE', #17432 ) ;
#35212=CARTESIAN_POINT ( 'NONE',  ( -8.834500769787091201, -12.51329471203370325, 31.30864560766548976 ) ) ;
#35214=CARTESIAN_POINT ( 'NONE',  ( 6.250054419913455561, -5.642605341092957083, 34.66089969410670335 ) ) ;
#35215=CARTESIAN_POINT ( 'NONE',  ( 14.43821774592595553, -8.630441415882550871, 34.87705825610312615 ) ) ;
#35218=ADVANCED_FACE ( 'NONE', ( #44887 ), #37242, .F. ) ;
#35219=ORIENTED_EDGE ( 'NONE', *, *, #45638, .T. ) ;
#35220=ORIENTED_EDGE ( 'NONE', *, *, #55422, .T. ) ;
#35221=CARTESIAN_POINT ( 'NONE',  ( -3.165514091256390827, -11.67786785259547777, 32.92929555188713664 ) ) ;
#35223=B_SPLINE_CURVE_WITH_KNOTS ( 'NONE', 3,
 ( #39847, #67313, #20885, #47024, #46596, #54224, #27207, #75833, #34403, #68635 ),
 .UNSPECIFIED., .F., .F.,
 ( 4, 2, 2, 2, 4 ),
 ( 0.0007817359430256294638, 0.0009771253907249941549, 0.001172514838424358954, 0.001367904286123723754, 0.001563293733823095492 ),
 .UNSPECIFIED. ) ;
#35224=CARTESIAN_POINT ( 'NONE',  ( -4.853911725310226188, -4.887748414852792322, 34.01359900205216746 ) ) ;
#35225=B_SPLINE_CURVE_WITH_KNOTS ( 'NONE', 3,
 ( #12245, #60426, #25760, #66743, #67639, #87941, #27086, #59984, #40176, #53672 ),
 .UNSPECIFIED., .F., .F.,
 ( 4, 2, 2, 2, 4 ),
 ( 0.000000000000000000, 0.0001954311564186865492, 0.0003908623128373730983, 0.0005862934692560596746, 0.0007817246256747461966 ),
 .UNSPECIFIED. ) ;
#35226=CARTESIAN_POINT ( 'NONE',  ( -11.60373153901785948, -5.941354392334499579, 34.76329471203369792 ) ) ;
#35227=CARTESIAN_POINT ( 'NONE',  ( -17.20761368003338987, -2.845849958028613624, 32.17971566917920967 ) ) ;
#35228=CARTESIAN_POINT ( 'NONE',  ( -12.46153846153846168, -1.242168528481310874, 33.36296068462461051 ) ) ;
#35229=FACE_OUTER_BOUND ( 'NONE', #23469, .T. ) ;
#35230=DIRECTION ( 'NONE',  ( -0.000000000000000000, 1.000000000000000000, -0.000000000000000000 ) ) ;
#35231=CARTESIAN_POINT ( 'NONE',  ( 11.31553532094539172, -9.886141570436013382, 34.14413921362392301 ) ) ;
#35232=ORIENTED_EDGE ( 'NONE', *, *, #32533, .T. ) ;
#35234=B_SPLINE_CURVE_WITH_KNOTS ( 'NONE', 3,
 ( #76837, #84047, #77710, #22760, #43925, #15577, #70069, #49793, #7929, #64181 ),
 .UNSPECIFIED., .F., .F.,
 ( 4, 2, 2, 2, 4 ),
 ( 0.0007817359430256294638, 0.0009771253907249952391, 0.001172514838424361123, 0.001367904286123726790, 0.001563293733823092673 ),
 .UNSPECIFIED. ) ;
#35235=ORIENTED_EDGE ( 'NONE', *, *, #33479, .T. ) ;
#35237=CYLINDRICAL_SURFACE ( 'NONE', #44507, 0.2499999999999995559 ) ;
#35238=CARTESIAN_POINT ( 'NONE',  ( 12.46153846153846168, -2.486705287966279876, 31.30864560766543647 ) ) ;
#35239=CARTESIAN_POINT ( 'NONE',  ( 1.607628228708781970, -11.43677907613345113, 33.22367315496201456 ) ) ;
#35240=CARTESIAN_POINT ( 'NONE',  ( 11.31497661389720832, -2.353723527008296568, 30.78948104536958752 ) ) ;
#35241=LINE ( 'NONE', #83450, #26432 ) ;
#35242=FACE_BOUND ( 'NONE', #67808, .T. ) ;
#35243=CARTESIAN_POINT ( 'NONE',  ( 8.519207545009310323, -10.92453946501458795, 33.72985991061850086 ) ) ;
#35245=AXIS2_PLACEMENT_3D ( 'NONE', #55860, #41918, #82904 ) ;
#35246=CARTESIAN_POINT ( 'NONE',  ( 17.14299041027315695, -11.91647553114624358, 32.58852847137148245 ) ) ;
#35248=CARTESIAN_POINT ( 'NONE',  ( -1.384615384615383471, -11.16473453929635440, 33.15142922261926373 ) ) ;
#35249=CARTESIAN_POINT ( 'NONE',  ( -1.134561072977068319, -2.779044189368096607, 31.39831045268885035 ) ) ;
#35250=CARTESIAN_POINT ( 'NONE',  ( 6.989144256427000101, -9.058645607665452459, 34.76329471203371924 ) ) ;
#35251=ORIENTED_EDGE ( 'NONE', *, *, #66269, .F. ) ;
#35252=CARTESIAN_POINT ( 'NONE',  ( 6.249945409378046435, -10.92531984108285670, 33.72920026020278073 ) ) ;
#35253=ORIENTED_EDGE ( 'NONE', *, *, #11981, .T. ) ;
#35254=FACE_BOUND ( 'NONE', #20690, .T. ) ;
#35255=CARTESIAN_POINT ( 'NONE',  ( -17.14300545628320904, -3.937682226553330445, 33.60647404775217240 ) ) ;
#35256=AXIS2_PLACEMENT_3D ( 'NONE', #30714, #52315, #58180 ) ;
#35257=B_SPLINE_CURVE_WITH_KNOTS ( 'NONE', 3,
 ( #70141, #27827, #21963, #34589, #76466, #75144, #56187, #13428, #62055, #1237 ),
 .UNSPECIFIED., .F., .F.,
 ( 4, 2, 2, 2, 4 ),
 ( 0.000000000000000000, 0.0001954311564186868202, 0.0003908623128373736404, 0.0005862934692560604335, 0.0007817246256747472808 ),
 .UNSPECIFIED. ) ;
#35258=CARTESIAN_POINT ( 'NONE',  ( -7.173100147298381302, -10.18141759479407327, 34.26406193332782379 ) ) ;
#35259=CARTESIAN_POINT ( 'NONE',  ( 1.384615384615386802, -2.499999999999998668, 29.75000000000001421 ) ) ;
#35260=ORIENTED_EDGE ( 'NONE', *, *, #83946, .F. ) ;
#35261=AXIS2_PLACEMENT_3D ( 'NONE', #81099, #33350, #68892 ) ;
#35262=CARTESIAN_POINT ( 'NONE',  ( -12.71156169883143150, -10.05641848906368097, 34.04755513067966177 ) ) ;
#35263=CARTESIAN_POINT ( 'NONE',  ( 5.143092217885731898, -7.250054483168843156, 34.74374881642865631 ) ) ;
#35264=CARTESIAN_POINT ( 'NONE',  ( -15.00775638667583678, -10.01129605718032600, 34.36064277460058491 ) ) ;
#35265=CARTESIAN_POINT ( 'NONE',  ( -6.988347369037697376, -10.90142922261923886, 33.41473453929638993 ) ) ;
#35266=EDGE_LOOP ( 'NONE', ( #49304, #12381, #17660, #51325 ) ) ;
#35267=CARTESIAN_POINT ( 'NONE',  ( 13.16168916709923664, -5.667676309546437530, 34.40238873228292249 ) ) ;
#35268=VERTEX_POINT ( 'NONE', #16537 ) ;
#35269=CARTESIAN_POINT ( 'NONE',  ( 15.93101805621127731, -7.369209533119136069, 34.99857337881830688 ) ) ;
#35271=CYLINDRICAL_SURFACE ( 'NONE', #2309, 0.2499999999999986955 ) ;
#35272=CARTESIAN_POINT ( 'NONE',  ( -10.68146802634049308, -12.37446782046654192, 30.86335684631486487 ) ) ;
#35273=B_SPLINE_CURVE_WITH_KNOTS ( 'NONE', 3,
 ( #29015, #71297, #43397, #36641, #84844, #36211, #56021, #76745, #77624, #9604 ),
 .UNSPECIFIED., .F., .F.,
 ( 4, 2, 2, 2, 4 ),
 ( 0.0007817359430256364027, 0.0009771253907250043464, 0.001172514838424372399, 0.001367904286123740234, 0.001563293733823108286 ),
 .UNSPECIFIED. ) ;
#35274=CARTESIAN_POINT ( 'NONE',  ( 5.010840697562940704, -2.486705287966279432, 31.30864560766542937 ) ) ;
#35275=CARTESIAN_POINT ( 'NONE',  ( -39.05038313613820122, -2.499999999999999556, 29.75000000000000355 ) ) ;
#35276=ADVANCED_FACE ( 'NONE', ( #17880 ), #23291, .F. ) ;
#35277=ADVANCED_FACE ( 'NONE', ( #44432 ), #3460, .F. ) ;
#35278=DIRECTION ( 'NONE',  ( -0.000000000000000000, 1.000000000000000000, 3.491481338843133355E-15 ) ) ;
#35279=FACE_OUTER_BOUND ( 'NONE', #31953, .T. ) ;
#35280=CARTESIAN_POINT ( 'NONE',  ( 16.37662569511456567, -5.913360116392396115, 34.49180327182771322 ) ) ;
#35281=CARTESIAN_POINT ( 'NONE',  ( -4.153846153846273204, -12.27809138561165270, 31.22303859784587132 ) ) ;
#35284=CARTESIAN_POINT ( 'NONE',  ( -17.75005448165186195, -9.272278438253398036, 34.42582936511637826 ) ) ;
#35285=VERTEX_POINT ( 'NONE', #19645 ) ;
#35286=EDGE_LOOP ( 'NONE', ( #54708, #32992 ) ) ;
#35287=CARTESIAN_POINT ( 'NONE',  ( 3.230769230769110045, -5.219633306517616589, 34.19971097300220464 ) ) ;
#35288=ORIENTED_EDGE ( 'NONE', *, *, #4881, .T. ) ;
#35289=CARTESIAN_POINT ( 'NONE',  ( 3.930361210122202742, -12.24155766932282496, 31.33739205006857986 ) ) ;
#35291=CARTESIAN_POINT ( 'NONE',  ( -7.911423846710166075, -8.656820664281498878, 34.87096338111211935 ) ) ;
#35292=CARTESIAN_POINT ( 'NONE',  ( 3.164685819813350065, -8.120952969808774569, 34.71129190930000163 ) ) ;
#35293=VECTOR ( 'NONE', #10354, 1000.000000000000114 ) ;
#35295=CARTESIAN_POINT ( 'NONE',  ( 10.86533002476265786, -6.653508905675592722, 34.93172785388651391 ) ) ;
#35296=CARTESIAN_POINT ( 'NONE',  ( -13.13456096470193302, -6.523592122091592671, 34.90882529074906415 ) ) ;
#35297=CARTESIAN_POINT ( 'NONE',  ( 17.07692307692295586, -11.48612834414049644, 32.76840700105863391 ) ) ;
#35299=B_SPLINE_CURVE_WITH_KNOTS ( 'NONE', 3,
 ( #75684, #49100, #69819, #1800, #48653, #27508, #1357, #77026, #8127, #8569 ),
 .UNSPECIFIED., .F., .F.,
 ( 4, 2, 2, 2, 4 ),
 ( 0.000000000000000000, 0.0001954339857564077183, 0.0003908679715128154366, 0.0005863019572692231007, 0.0007817359430256308733 ),
 .UNSPECIFIED. ) ;
#35300=CARTESIAN_POINT ( 'NONE',  ( -0.4615384615385826339, -2.625532179533779598, 30.86335684631627174 ) ) ;
#35301=CARTESIAN_POINT ( 'NONE',  ( 14.98074600654777377, -9.356822207818506598, 34.66110646841856635 ) ) ;
#35302=CARTESIAN_POINT ( 'NONE',  ( 5.142990410273152513, -10.67929555188718282, 33.92786785259544757 ) ) ;
#35303=CARTESIAN_POINT ( 'NONE',  ( -9.942330916529147800, -11.56360843649121684, 33.07473185843129926 ) ) ;
#35304=ORIENTED_EDGE ( 'NONE', *, *, #48830, .T. ) ;
#35305=EDGE_LOOP ( 'NONE', ( #52041, #71631 ) ) ;
#35306=CARTESIAN_POINT ( 'NONE',  ( -17.75000000000000355, -12.50000000000000000, 29.75000000000000355 ) ) ;
#35307=DIRECTION ( 'NONE',  ( 1.000000000000000000, 0.000000000000000000, 0.000000000000000000 ) ) ;
#35308=CARTESIAN_POINT ( 'NONE',  ( -2.980714919130916130, -2.779044189368095719, 31.39831045268885745 ) ) ;
#35309=CARTESIAN_POINT ( 'NONE',  ( 6.000000000000001776, -5.557115091759785130, 34.35708131394839171 ) ) ;
#35310=ORIENTED_EDGE ( 'NONE', *, *, #83898, .F. ) ;
#35311=CARTESIAN_POINT ( 'NONE',  ( -15.90390074446811042, -8.476813868363244353, 34.90874843262270133 ) ) ;
#35312=CARTESIAN_POINT ( 'NONE',  ( 11.78851595837499566, -4.074993327901527351, 33.72946981652012255 ) ) ;
#35313=B_SPLINE_CURVE_WITH_KNOTS ( 'NONE', 3,
 ( #27625, #13232, #48333, #6476, #74939, #28519, #55536, #7363, #82589, #75808 ),
 .UNSPECIFIED., .F., .F.,
 ( 4, 2, 2, 2, 4 ),
 ( 0.0007817359430256322827, 0.0009771253907249989254, 0.001172514838424365676, 0.001367904286123732428, 0.001563293733823098962 ),
 .UNSPECIFIED. ) ;
#35314=DIRECTION ( 'NONE',  ( 0.000000000000000000, 1.000000000000000000, 0.000000000000000000 ) ) ;
#35316=EDGE_LOOP ( 'NONE', ( #1214, #79570, #3969, #78357, #60765, #74111, #14808, #14601, #38051, #32669, #37044, #54337, #23682, #25121, #24022, #71955, #59209, #46294, #27470, #43764, #18776, #40016, #65397, #25145, #72736, #41588, #57598, #69841, #54159, #47529, #12283, #12211, #15881, #19040, #43869, #88007, #42878, #13733, #42164, #78303, #15840, #25830, #22637, #88892, #11194, #66796, #38537, #29902, #61302, #78862, #22825, #69346, #15090, #52225, #42424, #1059, #5621, #29594, #62450, #15315, #72991, #8810, #35883, #87867, #19618, #6191, #74251, #58945, #78111, #14543, #7980, #1101, #61044, #28021, #73933, #33227, #59003, #21965, #62803, #74330, #67459, #45757, #88933, #69919, #60662, #85333, #46381, #17379, #23785, #54598, #19075, #88398, #67284, #2830, #88339, #88387, #23501, #50959, #77069, #1806, #21568, #16300, #20819, #74680, #49946, #81292, #81082, #2819, #21671, #71784, #85739, #50635, #71209, #18572, #76765, #77566, #42040, #68931, #7357, #61281, #54492, #82900, #22998, #2417 ) ) ;
#35317=CARTESIAN_POINT ( 'NONE',  ( 18.13052543823364360, -3.625058011473227815, 33.29252011169590020 ) ) ;
#35318=EDGE_LOOP ( 'NONE', ( #10452, #39086, #19709, #44667 ) ) ;
#35319=DIRECTION ( 'NONE',  ( -0.000000000000000000, -0.7660444431189792347, -0.6427876096865379196 ) ) ;
#35320=CARTESIAN_POINT ( 'NONE',  ( 4.376809288112829321, -7.369474539155828730, 34.99858011523957657 ) ) ;
#35321=CARTESIAN_POINT ( 'NONE',  ( -1.514763354347078872, -9.504002272028875709, 34.60269587691767867 ) ) ;
#35323=CARTESIAN_POINT ( 'NONE',  ( -15.48074596171158213, -3.137211980971221781, 32.19342716148376837 ) ) ;
#35324=CARTESIAN_POINT ( 'NONE',  ( -6.923076923077045919, -2.657715359629662988, 31.77849191805970364 ) ) ;
#35325=EDGE_CURVE ( 'NONE', #22188, #61316, #20092, .T. ) ;
#35327=B_SPLINE_CURVE_WITH_KNOTS ( 'NONE', 3,
 ( #74218, #26916, #26028, #12954, #27794, #13393, #7082, #40877, #82310, #6640 ),
 .UNSPECIFIED., .F., .F.,
 ( 4, 2, 2, 2, 4 ),
 ( 0.000000000000000000, 0.0001954311564186872810, 0.0003908623128373745620, 0.0005862934692560618430, 0.0007817246256747491240 ),
 .UNSPECIFIED. ) ;
#35328=ORIENTED_EDGE ( 'NONE', *, *, #67934, .T. ) ;
#35329=EDGE_CURVE ( 'NONE', #12315, #85264, #80190, .T. ) ;
#35330=ORIENTED_EDGE ( 'NONE', *, *, #80549, .F. ) ;
#35331=ORIENTED_EDGE ( 'NONE', *, *, #9138, .F. ) ;
#35332=CYLINDRICAL_SURFACE ( 'NONE', #74703, 0.2500000000000012212 ) ;
#35333=CARTESIAN_POINT ( 'NONE',  ( -12.68502338610279523, -12.69144148231606017, 30.53333754910549303 ) ) ;
#35334=CARTESIAN_POINT ( 'NONE',  ( 0.5276057948885360949, -6.343179335718451384, 34.87096338111212646 ) ) ;
#35335=DIRECTION ( 'NONE',  ( -0.000000000000000000, 0.5000000000000011102, -0.8660254037844380415 ) ) ;
#35336=EDGE_CURVE ( 'NONE', #3335, #13990, #14614, .T. ) ;
#35338=CARTESIAN_POINT ( 'NONE',  ( -7.846153846153967493, -4.320704448113951379, 33.92786785259630022 ) ) ;
#35339=CARTESIAN_POINT ( 'NONE',  ( 14.53047184896071542, -10.11255958852956027, 34.01340905677048454 ) ) ;
#35340=ORIENTED_EDGE ( 'NONE', *, *, #3514, .F. ) ;
#35341=EDGE_CURVE ( 'NONE', #3675, #32906, #76987, .T. ) ;
#35342=ORIENTED_EDGE ( 'NONE', *, *, #21597, .T. ) ;
#35343=ORIENTED_EDGE ( 'NONE', *, *, #20611, .F. ) ;
#35344=CARTESIAN_POINT ( 'NONE',  ( 4.087762742890272527, -2.721908614388772740, 31.22303859784724622 ) ) ;
#35345=ORIENTED_EDGE ( 'NONE', *, *, #44662, .F. ) ;
#35346=CARTESIAN_POINT ( 'NONE',  ( 16.15384615384615330, -8.120952969808772792, 34.71129190930000163 ) ) ;
#35347=CARTESIAN_POINT ( 'NONE',  ( 13.38461538461526423, -4.320704448113951379, 33.92786785259630022 ) ) ;
#35348=CARTESIAN_POINT ( 'NONE',  ( 9.692307692307572609, -2.625532179533778709, 30.86335684631627174 ) ) ;
#35349=CARTESIAN_POINT ( 'NONE',  ( 13.60739492588379562, -8.496831190052093419, 34.64984203495476578 ) ) ;
#35350=ORIENTED_EDGE ( 'NONE', *, *, #81640, .F. ) ;
#35351=EDGE_CURVE ( 'NONE', #47861, #2266, #33163, .T. ) ;
#35352=EDGE_LOOP ( 'NONE', ( #35990, #21256 ) ) ;
#35353=CARTESIAN_POINT ( 'NONE',  ( 4.023698184114455678, -4.299443229763728169, 33.91186481527756058 ) ) ;
#35354=VERTEX_POINT ( 'NONE', #88580 ) ;
#35355=FACE_BOUND ( 'NONE', #17834, .T. ) ;
#35356=CARTESIAN_POINT ( 'NONE',  ( 6.792929713638703682, -4.460286881179643004, 33.72017969459903242 ) ) ;
#35357=DIRECTION ( 'NONE',  ( -0.000000000000000000, -0.1736481776669307198, -0.9848077530122080203 ) ) ;
#35358=ORIENTED_EDGE ( 'NONE', *, *, #32678, .T. ) ;
#35359=CARTESIAN_POINT ( 'NONE',  ( -14.05763788777885637, -8.346898887586323923, 34.93166121998716278 ) ) ;
#35361=LINE ( 'NONE', #56078, #53650 ) ;
#35362=B_SPLINE_CURVE_WITH_KNOTS ( 'NONE', 3,
 ( #3844, #47045, #4751, #39871, #19147, #86742, #53366, #10610, #73206, #80412 ),
 .UNSPECIFIED., .F., .F.,
 ( 4, 2, 2, 2, 4 ),
 ( 0.000000000000000000, 0.0001954339857564073388, 0.0003908679715128146777, 0.0005863019572692220165, 0.0007817359430256293554 ),
 .UNSPECIFIED. ) ;
#35363=CARTESIAN_POINT ( 'NONE',  ( 0.6843180028068696075, -6.760870238392817200, 34.69528174975672385 ) ) ;
#35364=CARTESIAN_POINT ( 'NONE',  ( 0.5920641633020236050, -12.45806712695776319, 30.39783852428763922 ) ) ;
#35367=DIRECTION ( 'NONE',  ( -0.000000000000000000, -0.9396926207859092051, -0.3420201433256662704 ) ) ;
#35368=LINE ( 'NONE', #83578, #18252 ) ;
#35369=CARTESIAN_POINT ( 'NONE',  ( 5.749976762707037281, -5.056417327199099532, 34.11270091957320716 ) ) ;
#35370=DIRECTION ( 'NONE',  ( 0.000000000000000000, -0.000000000000000000, -1.000000000000000000 ) ) ;
#35371=EDGE_CURVE ( 'NONE', #20780, #5299, #11420, .T. ) ;
#35372=FACE_BOUND ( 'NONE', #35479, .T. ) ;
#35373=CARTESIAN_POINT ( 'NONE',  ( -9.019230769230773603, -2.499999999999999556, 29.81609845454691765 ) ) ;
#35374=DIRECTION ( 'NONE',  ( -0.000000000000000000, 0.8660254037844397068, -0.4999999999999978906 ) ) ;
#35376=CARTESIAN_POINT ( 'NONE',  ( -3.296851610129365451, -2.833524468853757305, 32.15551576947924417 ) ) ;
#35378=EDGE_CURVE ( 'NONE', #27260, #19610, #39493, .T. ) ;
#35379=CARTESIAN_POINT ( 'NONE',  ( -10.68146699474474914, -6.343179335718451384, 34.87096338111212646 ) ) ;
#35381=ORIENTED_EDGE ( 'NONE', *, *, #78843, .T. ) ;
#35382=B_SPLINE_CURVE_WITH_KNOTS ( 'NONE', 3,
 ( #29452, #70431, #84396, #8736, #2394, #1081 ),
 .UNSPECIFIED., .F., .F.,
 ( 4, 2, 4 ),
 ( 0.0003909512603273650297, 0.0005862562993131907206, 0.0007815613382990164656 ),
 .UNSPECIFIED. ) ;
#35384=ORIENTED_EDGE ( 'NONE', *, *, #79544, .T. ) ;
#35385=CARTESIAN_POINT ( 'NONE',  ( -13.13466997523734037, -10.92531984108285670, 33.72920026020278073 ) ) ;
#35386=EDGE_CURVE ( 'NONE', #52135, #34125, #4358, .T. ) ;
#35388=EDGE_CURVE ( 'NONE', #4412, #83978, #66507, .T. ) ;
#35390=CARTESIAN_POINT ( 'NONE',  ( -8.069080063669991532, -9.886141570436013382, 34.14413921362392301 ) ) ;
#35391=EDGE_LOOP ( 'NONE', ( #68886, #72436, #16177, #56937 ) ) ;
#35392=CARTESIAN_POINT ( 'NONE',  ( -9.757631705111998954, -7.749976730030849303, 34.74374725381503737 ) ) ;
#35394=DIRECTION ( 'NONE',  ( -0.000000000000000000, -0.7660444431189791237, -0.6427876096865379196 ) ) ;
#35395=CARTESIAN_POINT ( 'NONE',  ( 4.153846153846154188, -7.500000000000001776, 35.04278698407183867 ) ) ;
#35396=CARTESIAN_POINT ( 'NONE',  ( -5.207070286361294542, -12.45813303252208648, 30.39737893381572675 ) ) ;
#35398=CARTESIAN_POINT ( 'NONE',  ( 5.010839665967194989, -8.120952969808774569, 34.71129190930000163 ) ) ;
#35401=CYLINDRICAL_SURFACE ( 'NONE', #77928, 0.2499999999999986955 ) ;
#35402=CARTESIAN_POINT ( 'NONE',  ( 14.37294787896832915, -10.90142922261932057, 33.41473453929631887 ) ) ;
#35403=B_SPLINE_CURVE_WITH_KNOTS ( 'NONE', 3,
 ( #82145, #55101, #61849, #88043, #81258, #14119, #33513, #19544, #40274, #47004 ),
 .UNSPECIFIED., .F., .F.,
 ( 4, 2, 2, 2, 4 ),
 ( 0.0007817246256747469556, 0.0009771112852218896347, 0.001172497944769032531, 0.001367884604316175427, 0.001563271263863318106 ),
 .UNSPECIFIED. ) ;
#35406=CARTESIAN_POINT ( 'NONE',  ( -14.17716660592874334, -10.88167719472716399, 33.43325721877153711 ) ) ;
#35407=CARTESIAN_POINT ( 'NONE',  ( -9.692307692307812417, -11.48612834414049644, 32.76840700105863391 ) ) ;
#35408=ORIENTED_EDGE ( 'NONE', *, *, #86332, .F. ) ;
#35410=CARTESIAN_POINT ( 'NONE',  ( 6.673076923076925127, -7.500000000000001776, 34.75000000000000000 ) ) ;
#35411=CARTESIAN_POINT ( 'NONE',  ( 16.15384615384615330, -2.486705287966279876, 31.30864560766543647 ) ) ;
#35412=DIRECTION ( 'NONE',  ( -0.000000000000000000, 0.000000000000000000, 1.000000000000000000 ) ) ;
#35413=VERTEX_POINT ( 'NONE', #4811 ) ;
#35414=CARTESIAN_POINT ( 'NONE',  ( -14.55766903863466055, -11.79746400365624659, 32.30657167506340954 ) ) ;
#35415=CARTESIAN_POINT ( 'NONE',  ( -1.514762594053603584, -10.88202310037936194, 33.43294751532457099 ) ) ;
#35417=CARTESIAN_POINT ( 'NONE',  ( 7.146089767170319185, -11.98016756924215009, 32.48728574198911190 ) ) ;
#35418=DIRECTION ( 'NONE',  ( 1.000000000000000000, 0.000000000000000000, 0.000000000000000000 ) ) ;
#35420=CARTESIAN_POINT ( 'NONE',  ( -10.54931626438217585, -10.51840700105979565, 33.73612834413962247 ) ) ;
#35421=VERTEX_POINT ( 'NONE', #32281 ) ;
#35422=CYLINDRICAL_SURFACE ( 'NONE', #44062, 0.2499999999999995559 ) ;
#35423=VERTEX_POINT ( 'NONE', #59746 ) ;
#35424=VERTEX_POINT ( 'NONE', #25958 ) ;
#35425=CARTESIAN_POINT ( 'NONE',  ( 5.076923076922954969, -11.94971097300221174, 32.03036669348237098 ) ) ;
#35426=CARTESIAN_POINT ( 'NONE',  ( -17.07692307692307665, -4.945431358278436385, 36.03766855953609394 ) ) ;
#35428=CARTESIAN_POINT ( 'NONE',  ( 13.25392478150507891, -8.191372820521381826, 34.95448215188423546 ) ) ;
#35429=B_SPLINE_CURVE_WITH_KNOTS ( 'NONE', 3,
 ( #5451, #32918, #60381, #87895, #53629, #14414, #36028, #29273, #48634, #1340 ),
 .UNSPECIFIED., .F., .F.,
 ( 4, 2, 2, 2, 4 ),
 ( 0.0007817246256747499913, 0.0009771112852218944052, 0.001172497944769038819, 0.001367884604316183016, 0.001563271263863327430 ),
 .UNSPECIFIED. ) ;
#35430=ADVANCED_FACE ( 'NONE', ( #54309 ), #80925, .F. ) ;
#35431=ORIENTED_EDGE ( 'NONE', *, *, #41527, .T. ) ;
#35432=B_SPLINE_CURVE_WITH_KNOTS ( 'NONE', 3,
 ( #67151, #73472, #25719, #45978, #54062, #46870, #32467, #74353, #33367, #60829 ),
 .UNSPECIFIED., .F., .F.,
 ( 4, 2, 2, 2, 4 ),
 ( 0.000000000000000000, 0.0001954339881912775425, 0.0003908679763825550850, 0.0005863019645738326005, 0.0007817359527651101701 ),
 .UNSPECIFIED. ) ;
#35433=CARTESIAN_POINT ( 'NONE',  ( 13.38461538461538680, -2.721908614388771852, 31.22303859784724978 ) ) ;
#35434=VERTEX_POINT ( 'NONE', #34926 ) ;
#35435=B_SPLINE_CURVE_WITH_KNOTS ( 'NONE', 3,
 ( #69524, #42506, #42949, #70419, #63647, #17580, #76276, #1954, #29439, #630 ),
 .UNSPECIFIED., .F., .F.,
 ( 4, 2, 2, 2, 4 ),
 ( 0.000000000000000000, 0.0001954311564186861697, 0.0003908623128373723394, 0.0005862934692560584820, 0.0007817246256747446788 ),
 .UNSPECIFIED. ) ;
#35437=ORIENTED_EDGE ( 'NONE', *, *, #1768, .T. ) ;
#35438=ORIENTED_EDGE ( 'NONE', *, *, #63015, .T. ) ;
#35439=CARTESIAN_POINT ( 'NONE',  ( 13.38461538461538680, -4.661471528628507777, 34.16647553114623292 ) ) ;
#35440=EDGE_LOOP ( 'NONE', ( #86755, #23604 ) ) ;
#35441=CARTESIAN_POINT ( 'NONE',  ( -4.826868657009623753, -12.41089969410671223, 31.60739465890703670 ) ) ;
#35443=EDGE_CURVE ( 'NONE', #33344, #59859, #29782, .T. ) ;
#35444=CARTESIAN_POINT ( 'NONE',  ( -3.230769230769229949, -4.098570777380720287, 33.41473453929634729 ) ) ;
#35445=CARTESIAN_POINT ( 'NONE',  ( -3.903900744468109973, -6.653508905675592722, 34.93172785388651391 ) ) ;
#35446=AXIS2_PLACEMENT_3D ( 'NONE', #79163, #31873, #17465 ) ;
#35451=ORIENTED_EDGE ( 'NONE', *, *, #60056, .F. ) ;
#35453=LINE ( 'NONE', #8428, #48777 ) ;
#35455=CARTESIAN_POINT ( 'NONE',  ( 11.31497659473759043, -6.760086850603066466, 34.69517049084099369 ) ) ;
#35456=CARTESIAN_POINT ( 'NONE',  ( 6.857806477116147548, -6.879047030191174805, 34.71129190930000163 ) ) ;
#35457=CARTESIAN_POINT ( 'NONE',  ( 2.557746727605761272, -9.233818618650603938, 34.70587769442853698 ) ) ;
#35458=ORIENTED_EDGE ( 'NONE', *, *, #30241, .T. ) ;
#35459=EDGE_CURVE ( 'NONE', #39506, #27738, #9361, .T. ) ;
#35460=CARTESIAN_POINT ( 'NONE',  ( 15.00728428704528561, -10.81261337010820256, 33.49550067578627477 ) ) ;
#35461=CARTESIAN_POINT ( 'NONE',  ( 3.230769230769231726, -13.95598074871891292, 31.83374038241031911 ) ) ;
#35463=FACE_BOUND ( 'NONE', #39327, .T. ) ;
#35464=LINE ( 'NONE', #28711, #8289 ) ;
#35467=CARTESIAN_POINT ( 'NONE',  ( -8.769230769230768274, -12.78798330534103123, 29.99999999999997868 ) ) ;
#35470=CARTESIAN_POINT ( 'NONE',  ( 14.55763771707035303, -2.341251567377310217, 30.72681386836322659 ) ) ;
#35471=ORIENTED_EDGE ( 'NONE', *, *, #26761, .T. ) ;
#35472=CARTESIAN_POINT ( 'NONE',  ( -18.00000000000000000, -10.51840700105979387, 33.73612834413961536 ) ) ;
#35473=EDGE_CURVE ( 'NONE', #37880, #48065, #78098, .T. ) ;
#35474=CARTESIAN_POINT ( 'NONE',  ( -6.223484924564330889, -11.60425143139329940, 33.02411095842164457 ) ) ;
#35475=ORIENTED_EDGE ( 'NONE', *, *, #13042, .T. ) ;
#35476=B_SPLINE_CURVE_WITH_KNOTS ( 'NONE', 3,
 ( #32015, #80207, #26146, #45963, #60813, #18505, #46414, #53611, #59923, #68025 ),
 .UNSPECIFIED., .F., .F.,
 ( 4, 2, 2, 2, 4 ),
 ( 0.0007817359430256313069, 0.0009771253907249971907, 0.001172514838424363074, 0.001367904286123728958, 0.001563293733823094842 ),
 .UNSPECIFIED. ) ;
#35477=CARTESIAN_POINT ( 'NONE',  ( -4.153846153846152411, -13.49023893513002648, 31.06009739812518688 ) ) ;
#35478=DIRECTION ( 'NONE',  ( -0.000000000000000000, -0.9396926207859093161, -0.3420201433256663259 ) ) ;
#35479=EDGE_LOOP ( 'NONE', ( #76862, #1644 ) ) ;
#35481=CARTESIAN_POINT ( 'NONE',  ( 4.153846153846032507, -10.21337939537710326, 33.94971097300076224 ) ) ;
#35482=EDGE_CURVE ( 'NONE', #32338, #71873, #8358, .T. ) ;
#35483=FACE_BOUND ( 'NONE', #9109, .T. ) ;
#35484=CARTESIAN_POINT ( 'NONE',  ( -6.249999999999997335, -7.500000000000001776, 35.00000000000000000 ) ) ;
#35485=CARTESIAN_POINT ( 'NONE',  ( -16.82697755857493149, -12.43552623307873972, 30.55307653245132826 ) ) ;
#35486=CARTESIAN_POINT ( 'NONE',  ( 3.361294932532794100, -8.586989748646452369, 34.63063291749215011 ) ) ;
#35487=VECTOR ( 'NONE', #45897, 1000.000000000000000 ) ;
#35488=CARTESIAN_POINT ( 'NONE',  ( 12.23861150263161157, -12.38737895849757820, 31.66785238281580206 ) ) ;
#35489=CARTESIAN_POINT ( 'NONE',  ( -7.623141002060451754, -12.64618726649961289, 30.78989965857442712 ) ) ;
#35490=CARTESIAN_POINT ( 'NONE',  ( 5.999999999999880096, -3.835265460704628371, 33.15142922262033665 ) ) ;
#35491=FACE_OUTER_BOUND ( 'NONE', #85727, .T. ) ;
#35493=VERTEX_POINT ( 'NONE', #68277 ) ;
#35494=EDGE_CURVE ( 'NONE', #11273, #57, #83382, .T. ) ;
#35495=ORIENTED_EDGE ( 'NONE', *, *, #47177, .T. ) ;
#35496=CARTESIAN_POINT ( 'NONE',  ( 5.999999999999880096, -3.300289026999228881, 32.46337939537708905 ) ) ;
#35497=EDGE_CURVE ( 'NONE', #69942, #62711, #52258, .T. ) ;
#35498=CARTESIAN_POINT ( 'NONE',  ( -10.61538461538461320, -8.164416787775445883, 34.95778746994557906 ) ) ;
#35499=CARTESIAN_POINT ( 'NONE',  ( 1.515405825582337052, -9.084667340241226796, 34.75534355489798344 ) ) ;
#35500=B_SPLINE_CURVE_WITH_KNOTS ( 'NONE', 3,
 ( #62002, #13375, #27776, #55244, #40856, #89061, #83174, #82735, #48478, #14265 ),
 .UNSPECIFIED., .F., .F.,
 ( 4, 2, 2, 2, 4 ),
 ( 0.0007817359430256347764, 0.0009771253907250036959, 0.001172514838424372832, 0.001367904286123741969, 0.001563293733823103949 ),
 .UNSPECIFIED. ) ;
#35501=CARTESIAN_POINT ( 'NONE',  ( -9.019253993452222673, -8.475808217655753651, 34.90892951860618609 ) ) ;
#35502=CARTESIAN_POINT ( 'NONE',  ( -13.13466997523734392, -2.589246495874658383, 31.60778113518102828 ) ) ;
#35504=B_SPLINE_CURVE_WITH_KNOTS ( 'NONE', 3,
 ( #74121, #40785, #32682, #66920, #88986, #55168, #68250, #27259, #54721, #47521 ),
 .UNSPECIFIED., .F., .F.,
 ( 4, 2, 2, 2, 4 ),
 ( 0.000000000000000000, 0.0001954339857564073659, 0.0003908679715128147319, 0.0005863019572692221250, 0.0007817359430256294638 ),
 .UNSPECIFIED. ) ;
#35505=CARTESIAN_POINT ( 'NONE',  ( 0.5920638997721056063, -4.299079248970732792, 33.91157788607253565 ) ) ;
#35506=CARTESIAN_POINT ( 'NONE',  ( -9.692307692307691624, -1.215029322943914858, 32.30358669280327177 ) ) ;
#35507=DIRECTION ( 'NONE',  ( -0.000000000000000000, -0.1736481776669307198, -0.9848077530122080203 ) ) ;
#35508=CARTESIAN_POINT ( 'NONE',  ( 7.596130621932389637, -5.765609946408403630, 34.70566812827425451 ) ) ;
#35510=CARTESIAN_POINT ( 'NONE',  ( 16.40390046548447245, -4.943051570960395047, 34.04725096376909477 ) ) ;
#35511=CYLINDRICAL_SURFACE ( 'NONE', #736, 0.2499999999999979738 ) ;
#35513=CARTESIAN_POINT ( 'NONE',  ( 10.48477496018053223, -7.722926974430166069, 34.99546784045485737 ) ) ;
#35514=CARTESIAN_POINT ( 'NONE',  ( -0.4615384615384611200, -9.058645607665452459, 34.76329471203371924 ) ) ;
#35515=ADVANCED_FACE ( 'NONE', ( #7016 ), #77248, .F. ) ;
#35516=VERTEX_POINT ( 'NONE', #29516 ) ;
#35517=CARTESIAN_POINT ( 'NONE',  ( -14.55766903863466055, -3.627789207965226748, 32.91389620160131102 ) ) ;
#35518=CARTESIAN_POINT ( 'NONE',  ( 7.780071466793709867, -4.661471528628507777, 34.16647553114621871 ) ) ;
#35519=AXIS2_PLACEMENT_3D ( 'NONE', #84848, #1974, #29457 ) ;
#35521=CARTESIAN_POINT ( 'NONE',  ( 6.857806922520602200, -5.094484230520674117, 34.41647553114621161 ) ) ;
#35523=VERTEX_POINT ( 'NONE', #70940 ) ;
#35524=ADVANCED_FACE ( 'NONE', ( #77689 ), #29957, .F. ) ;
#35526=LINE ( 'NONE', #27879, #45374 ) ;
#35527=ORIENTED_EDGE ( 'NONE', *, *, #67587, .F. ) ;
#35529=CARTESIAN_POINT ( 'NONE',  ( -2.530619266599154038, -10.77366814457252175, 33.85459836347579454 ) ) ;
#35532=CARTESIAN_POINT ( 'NONE',  ( -5.076923076923197442, -12.27809138561165270, 31.22303859784587132 ) ) ;
#35533=CARTESIAN_POINT ( 'NONE',  ( 13.25392478150507891, -9.084618155246140248, 34.75535874321725771 ) ) ;
#35534=EDGE_LOOP ( 'NONE', ( #58695, #57771 ) ) ;
#35535=CYLINDRICAL_SURFACE ( 'NONE', #38986, 0.2500000000000008882 ) ;
#35536=EDGE_CURVE ( 'NONE', #15565, #29065, #82429, .T. ) ;
#35537=CARTESIAN_POINT ( 'NONE',  ( 5.326923076923089084, -2.249999999999999112, 29.81603969181031033 ) ) ;
#35538=DIRECTION ( 'NONE',  ( -0.000000000000000000, 1.000000000000000000, -0.000000000000000000 ) ) ;
#35539=ORIENTED_EDGE ( 'NONE', *, *, #5117, .F. ) ;
#35541=CARTESIAN_POINT ( 'NONE',  ( 6.130791807824788719, -6.413143153341454017, 34.63066358083362672 ) ) ;
#35542=EDGE_CURVE ( 'NONE', #28852, #30322, #57688, .T. ) ;
#35543=ORIENTED_EDGE ( 'NONE', *, *, #58662, .F. ) ;
#35544=EDGE_CURVE ( 'NONE', #60075, #74684, #57415, .T. ) ;
#35545=FACE_OUTER_BOUND ( 'NONE', #59944, .T. ) ;
#35546=VECTOR ( 'NONE', #77241, 1000.000000000000227 ) ;
#35547=CARTESIAN_POINT ( 'NONE',  ( -1.161835843346975095, -2.600157965045225783, 30.74683119005207743 ) ) ;
#35548=CARTESIAN_POINT ( 'NONE',  ( 2.373759641042385127, -11.35647404775217595, 33.31231777344667222 ) ) ;
#35549=B_SPLINE_CURVE_WITH_KNOTS ( 'NONE', 3,
 ( #60885, #46919, #13148, #6401, #54564, #19896 ),
 .UNSPECIFIED., .F., .F.,
 ( 4, 2, 4 ),
 ( 0.0003909569690057842790, 0.0005862646681846108007, 0.0007815723673634373224 ),
 .UNSPECIFIED. ) ;
#35550=DIRECTION ( 'NONE',  ( -0.000000000000000000, 0.9848077530122085754, -0.1736481776669273613 ) ) ;
#35551=CARTESIAN_POINT ( 'NONE',  ( 1.161688425708537808, -2.308479472611653094, 30.53278059502174457 ) ) ;
#35553=EDGE_CURVE ( 'NONE', #4801, #44215, #50202, .T. ) ;
#35554=CARTESIAN_POINT ( 'NONE',  ( 15.23076923076953904, -2.506253911140615021, 30.00000000000323297 ) ) ;
#35555=ORIENTED_EDGE ( 'NONE', *, *, #19475, .F. ) ;
#35558=CARTESIAN_POINT ( 'NONE',  ( 4.284636594813103549, -8.191423895709842640, 34.95447573519442130 ) ) ;
#35559=ORIENTED_EDGE ( 'NONE', *, *, #88636, .T. ) ;
#35560=CARTESIAN_POINT ( 'NONE',  ( 16.82694633287449193, -2.318417181685854978, 30.59732222474233865 ) ) ;
#35561=EDGE_LOOP ( 'NONE', ( #83242, #11186 ) ) ;
#35563=CARTESIAN_POINT ( 'NONE',  ( -10.61538461538473577, -12.70778746994576025, 30.41441678777401236 ) ) ;
#35564=ORIENTED_EDGE ( 'NONE', *, *, #59345, .T. ) ;
#35565=ADVANCED_FACE ( 'NONE', ( #44784 ), #50655, .F. ) ;
#35566=CARTESIAN_POINT ( 'NONE',  ( -12.21159294319032185, -5.852078868378309373, 34.47109172314383585 ) ) ;
#35567=EDGE_LOOP ( 'NONE', ( #17502, #44241 ) ) ;
#35568=CARTESIAN_POINT ( 'NONE',  ( -8.519176457592454454, -8.303483539816728154, 34.68545999027711702 ) ) ;
#35569=EDGE_LOOP ( 'NONE', ( #39669, #7517, #57495, #13552 ) ) ;
#35570=CARTESIAN_POINT ( 'NONE',  ( -14.08491263871423982, -12.11081565061824250, 32.26097654155340422 ) ) ;
#35571=AXIS2_PLACEMENT_3D ( 'NONE', #56300, #2226, #23386 ) ;
#35572=EDGE_LOOP ( 'NONE', ( #37511, #2961 ) ) ;
#35573=DIRECTION ( 'NONE',  ( 0.000000000000000000, 0.000000000000000000, 1.000000000000000000 ) ) ;
#35574=CARTESIAN_POINT ( 'NONE',  ( -16.15384615384615330, -13.87047571288749737, 32.06866353760679544 ) ) ;
#35576=FACE_BOUND ( 'NONE', #40784, .T. ) ;
#35577=CARTESIAN_POINT ( 'NONE',  ( -11.66915300512910036, -2.541943142973491554, 30.39792223712631980 ) ) ;
#35578=CYLINDRICAL_SURFACE ( 'NONE', #65842, 0.2500000000000009437 ) ;
#35579=CARTESIAN_POINT ( 'NONE',  ( 9.468822767743363400, -11.60425143139329940, 33.02411095842164457 ) ) ;
#35580=CARTESIAN_POINT ( 'NONE',  ( -0.4615384615385840772, -3.083524468854526912, 32.58852847137268327 ) ) ;
#35581=LINE ( 'NONE', #42786, #62494 ) ;
#35582=CARTESIAN_POINT ( 'NONE',  ( -16.37677237136229991, -8.239355502252617924, 34.69524867566427417 ) ) ;
#35584=VECTOR ( 'NONE', #58421, 1000.000000000000000 ) ;
#35585=CARTESIAN_POINT ( 'NONE',  ( -6.249999999999997335, -2.499999999999998668, 29.75000000000000355 ) ) ;
#35586=ORIENTED_EDGE ( 'NONE', *, *, #55113, .F. ) ;
#35587=ORIENTED_EDGE ( 'NONE', *, *, #40950, .F. ) ;
#35588=CARTESIAN_POINT ( 'NONE',  ( -1.134669975237340811, -4.932303261841489039, 34.32971442181322885 ) ) ;
#35589=CARTESIAN_POINT ( 'NONE',  ( 15.16549878480845948, -12.27809138561121394, 31.22303859784730307 ) ) ;
#35590=FACE_OUTER_BOUND ( 'NONE', #14007, .T. ) ;
#35591=CYLINDRICAL_SURFACE ( 'NONE', #52320, 0.2500000000000008882 ) ;
#35592=CARTESIAN_POINT ( 'NONE',  ( -12.46153846153858424, -2.657715359629662544, 31.77849191805970364 ) ) ;
#35595=CARTESIAN_POINT ( 'NONE',  ( -5.142193077479396024, -5.941354392334500467, 34.76329471203369792 ) ) ;
#35596=CARTESIAN_POINT ( 'NONE',  ( -14.53117723225663660, -10.23692288466677880, 34.23039457007281072 ) ) ;
#35598=CARTESIAN_POINT ( 'NONE',  ( -8.769230769230892619, -2.657715359629662544, 31.77849191805970364 ) ) ;
#35599=CARTESIAN_POINT ( 'NONE',  ( 2.530471976670374712, -5.827830569534416583, 34.72679350104403539 ) ) ;
#35600=ORIENTED_EDGE ( 'NONE', *, *, #60319, .F. ) ;
#35601=CARTESIAN_POINT ( 'NONE',  ( -0.7115152055870527237, -2.318417181685854533, 30.59732222474233865 ) ) ;
#35602=ORIENTED_EDGE ( 'NONE', *, *, #5734, .T. ) ;
#35604=ORIENTED_EDGE ( 'NONE', *, *, #9767, .F. ) ;
#35606=CYLINDRICAL_SURFACE ( 'NONE', #52063, 0.2500000000000009437 ) ;
#35607=EDGE_CURVE ( 'NONE', #72717, #12426, #16839, .T. ) ;
#35608=ORIENTED_EDGE ( 'NONE', *, *, #36509, .T. ) ;
#35609=CARTESIAN_POINT ( 'NONE',  ( -1.134669866267242311, -8.433404298154336232, 34.66254593164985920 ) ) ;
#35610=CARTESIAN_POINT ( 'NONE',  ( -17.14300648787895653, -3.050289026998445951, 32.03036669348365706 ) ) ;
#35611=DIRECTION ( 'NONE',  ( -0.000000000000000000, 0.7660444431189791237, -0.6427876096865379196 ) ) ;
#35612=CARTESIAN_POINT ( 'NONE',  ( -4.854143407945007205, -3.563462043263029955, 33.22394488606062879 ) ) ;
#35613=FACE_OUTER_BOUND ( 'NONE', #45630, .T. ) ;
#35614=B_SPLINE_CURVE_WITH_KNOTS ( 'NONE', 3,
 ( #3227, #30700, #85654, #17186, #72128, #65373, #54072, #12219, #26616, #66716 ),
 .UNSPECIFIED., .F., .F.,
 ( 4, 2, 2, 2, 4 ),
 ( 0.0007817359430256313069, 0.0009771253907249971907, 0.001172514838424363074, 0.001367904286123728958, 0.001563293733823094842 ),
 .UNSPECIFIED. ) ;
#35615=CARTESIAN_POINT ( 'NONE',  ( 0.4615384615383382183, -9.528491918059723176, 34.59228464037033035 ) ) ;
#35617=EDGE_CURVE ( 'NONE', #47387, #81622, #32973, .T. ) ;
#35619=CARTESIAN_POINT ( 'NONE',  ( -12.23875892027004753, -11.89424750095246175, 32.13594075562311758 ) ) ;
#35620=EDGE_LOOP ( 'NONE', ( #64171, #11012, #77655, #19587 ) ) ;
#35621=CARTESIAN_POINT ( 'NONE',  ( -5.326923076923075762, -2.499999999999998668, 29.75000000000000355 ) ) ;
#35622=CARTESIAN_POINT ( 'NONE',  ( 6.000000000000001776, -8.564572088678739092, 35.78748833219616898 ) ) ;
#35623=CARTESIAN_POINT ( 'NONE',  ( -17.07692307692319744, -12.16647553114689728, 32.15551576947799362 ) ) ;
#35624=B_SPLINE_CURVE_WITH_KNOTS ( 'NONE', 3,
 ( #62985, #1297, #28786, #8954, #56251, #15713 ),
 .UNSPECIFIED., .F., .F.,
 ( 4, 2, 4 ),
 ( 0.0003909569690057804843, 0.0005862646681846042955, 0.0007815723673634281067 ),
 .UNSPECIFIED. ) ;
#35625=B_SPLINE_CURVE_WITH_KNOTS ( 'NONE', 3,
 ( #15792, #43257, #49570, #8591, #84700, #9034 ),
 .UNSPECIFIED., .F., .F.,
 ( 4, 2, 4 ),
 ( 5.648016952424533599E-17, 0.0001954756301637301926, 0.0003909512603274038984 ),
 .UNSPECIFIED. ) ;
#35626=CARTESIAN_POINT ( 'NONE',  ( -2.372962308248625529, -12.70778746994557551, 30.41441678777548319 ) ) ;
#35627=DIRECTION ( 'NONE',  ( 0.000000000000000000, 0.4999999999999960032, -0.8660254037844410391 ) ) ;
#35628=CARTESIAN_POINT ( 'NONE',  ( -3.296851610129365451, -10.67929555188718460, 33.92786785259543336 ) ) ;
#35629=LINE ( 'NONE', #28879, #17690 ) ;
#35630=EDGE_CURVE ( 'NONE', #64075, #45937, #65169, .T. ) ;
#35632=EDGE_LOOP ( 'NONE', ( #13028, #20246, #84640, #53260, #28745, #26491 ) ) ;
#35633=CARTESIAN_POINT ( 'NONE',  ( -16.85414353565466072, -10.81320215134717166, 33.49497208177562868 ) ) ;
#35634=CARTESIAN_POINT ( 'NONE',  ( -1.515306851282938849, -12.11776431015575994, 31.66791131148498906 ) ) ;
#35635=CARTESIAN_POINT ( 'NONE',  ( 9.692307692307570832, -11.06231777344772027, 33.60647404775119895 ) ) ;
#35637=ORIENTED_EDGE ( 'NONE', *, *, #58929, .T. ) ;
#35639=CARTESIAN_POINT ( 'NONE',  ( -2.557669038634660108, -3.137211980971222669, 32.19342716148376837 ) ) ;
#35640=CARTESIAN_POINT ( 'NONE',  ( 14.17713239407894044, -2.254533558242299396, 29.97296025877828285 ) ) ;
#35641=LINE ( 'NONE', #63090, #55758 ) ;
#35642=ORIENTED_EDGE ( 'NONE', *, *, #87224, .T. ) ;
#35643=VECTOR ( 'NONE', #85334, 1000.000000000000000 ) ;
#35644=CARTESIAN_POINT ( 'NONE',  ( -12.39628289026243557, -9.442884908240273489, 34.35708131394835618 ) ) ;
#35645=CARTESIAN_POINT ( 'NONE',  ( 11.53846153846153832, -7.500000000000001776, 35.04278698407183867 ) ) ;
#35646=DIRECTION ( 'NONE',  ( 0.000000000000000000, 0.1736481776669267785, -0.9848077530122087975 ) ) ;
#35647=CARTESIAN_POINT ( 'NONE',  ( -13.13456096470193302, -12.65882529074907126, 30.72640787790839312 ) ) ;
#35648=ORIENTED_EDGE ( 'NONE', *, *, #78782, .F. ) ;
#35649=CARTESIAN_POINT ( 'NONE',  ( -6.673131513698878692, -6.653508905675592722, 34.93172785388651391 ) ) ;
#35650=AXIS2_PLACEMENT_3D ( 'NONE', #12647, #67148, #87890 ) ;
#35652=ORIENTED_EDGE ( 'NONE', *, *, #36731, .T. ) ;
#35653=CARTESIAN_POINT ( 'NONE',  ( 12.68455130563185662, -12.38742843783360748, 31.66772728687926985 ) ) ;
#35654=CARTESIAN_POINT ( 'NONE',  ( -10.83886955910855932, -2.847400154188067578, 31.58180166144859058 ) ) ;
#35655=EDGE_LOOP ( 'NONE', ( #22010, #61610 ) ) ;
#35656=AXIS2_PLACEMENT_3D ( 'NONE', #42191, #8395, #69643 ) ;
#35658=CARTESIAN_POINT ( 'NONE',  ( -14.55766905174089665, -2.318417181685855422, 30.59732222474233865 ) ) ;
#35659=CARTESIAN_POINT ( 'NONE',  ( 13.16113044089144068, -6.760086850603066466, 34.69517049084099369 ) ) ;
#35660=EDGE_CURVE ( 'NONE', #78029, #19388, #11919, .T. ) ;
#35661=CARTESIAN_POINT ( 'NONE',  ( 1.319345384059066983, -6.835583212224499938, 34.95778746994557906 ) ) ;
#35663=EDGE_CURVE ( 'NONE', #10540, #59654, #8245, .T. ) ;
#35664=VERTEX_POINT ( 'NONE', #87145 ) ;
#35666=ORIENTED_EDGE ( 'NONE', *, *, #21421, .T. ) ;
#35667=FACE_BOUND ( 'NONE', #17494, .T. ) ;
#35670=AXIS2_PLACEMENT_3D ( 'NONE', #39470, #88555, #66930 ) ;
#35672=DIRECTION ( 'NONE',  ( -0.000000000000000000, -0.8660254037844399289, -0.4999999999999980016 ) ) ;
#35674=B_SPLINE_CURVE_WITH_KNOTS ( 'NONE', 3,
 ( #17588, #60337, #31538, #86502, #52690, #4964, #32428, #87393, #55352, #48150 ),
 .UNSPECIFIED., .F., .F.,
 ( 4, 2, 2, 2, 4 ),
 ( 0.0007817246256747474977, 0.0009771112852218911526, 0.001172497944769034916, 0.001367884604316178679, 0.001563271263863322443 ),
 .UNSPECIFIED. ) ;
#35675=EDGE_CURVE ( 'NONE', #40586, #14645, #20040, .T. ) ;
#35676=ORIENTED_EDGE ( 'NONE', *, *, #82110, .F. ) ;
#35677=AXIS2_PLACEMENT_3D ( 'NONE', #19938, #67252, #33019 ) ;
#35679=ORIENTED_EDGE ( 'NONE', *, *, #87460, .T. ) ;
#35680=CARTESIAN_POINT ( 'NONE',  ( -3.100243792535588128, -11.66157788607254275, 32.95092075102925833 ) ) ;
#35681=EDGE_CURVE ( 'NONE', #81564, #79445, #75867, .T. ) ;
#35682=EDGE_CURVE ( 'NONE', #9934, #79961, #39395, .T. ) ;
#35684=AXIS2_PLACEMENT_3D ( 'NONE', #34423, #29013, #41627 ) ;
#35685=CARTESIAN_POINT ( 'NONE',  ( 3.165498784808456367, -2.892918686051582533, 31.69288490824015270 ) ) ;
#35686=CARTESIAN_POINT ( 'NONE',  ( 12.21151522424549896, -2.587272538249754117, 30.68239716806877837 ) ) ;
#35688=CARTESIAN_POINT ( 'NONE',  ( -18.22292621751613950, -11.24512374952582050, 33.06303171183252942 ) ) ;
#35689=LINE ( 'NONE', #77987, #60059 ) ;
#35690=CARTESIAN_POINT ( 'NONE',  ( -6.066082379360132393, -6.343179335718451384, 34.87096338111212646 ) ) ;
#35692=CARTESIAN_POINT ( 'NONE',  ( 8.992010438208831502, -6.717445702608402236, 34.94155399931962336 ) ) ;
#35693=ORIENTED_EDGE ( 'NONE', *, *, #42620, .T. ) ;
#35695=ORIENTED_EDGE ( 'NONE', *, *, #3064, .T. ) ;
#35696=CARTESIAN_POINT ( 'NONE',  ( 3.295914011488863871, -7.750023224968865421, 34.99404313364389907 ) ) ;
#35698=CARTESIAN_POINT ( 'NONE',  ( 10.39189969082028497, -2.353723527008296568, 30.78948104536958752 ) ) ;
#35699=CARTESIAN_POINT ( 'NONE',  ( 1.634669804528839476, -12.41089969410671223, 31.60739465890703670 ) ) ;
#35700=CARTESIAN_POINT ( 'NONE',  ( 12.59206389977210705, -12.70449254468099198, 30.44128974285582956 ) ) ;
#35701=FACE_BOUND ( 'NONE', #81175, .T. ) ;
#35702=CARTESIAN_POINT ( 'NONE',  ( 16.28437185560972011, -3.285477652293413264, 32.44071101563363158 ) ) ;
#35704=CARTESIAN_POINT ( 'NONE',  ( 17.07692307692307665, -10.51840700105979565, 33.73612834413961536 ) ) ;
#35707=LINE ( 'NONE', #43779, #25147 ) ;
#35708=EDGE_LOOP ( 'NONE', ( #37117, #29490, #78, #30885 ) ) ;
#35709=CARTESIAN_POINT ( 'NONE',  ( -18.06608341095587633, -8.120952969808774569, 34.71129190930000163 ) ) ;
#35712=FACE_BOUND ( 'NONE', #9293, .T. ) ;
#35713=B_SPLINE_CURVE_WITH_KNOTS ( 'NONE', 3,
 ( #84388, #43389, #84835, #64972, #50577, #16358, #44244, #72179, #50133, #9594 ),
 .UNSPECIFIED., .F., .F.,
 ( 4, 2, 2, 2, 4 ),
 ( 0.000000000000000000, 0.0001954339857564076912, 0.0003908679715128153824, 0.0005863019572692231007, 0.0007817359430256307648 ),
 .UNSPECIFIED. ) ;
#35714=EDGE_CURVE ( 'NONE', #34892, #83375, #2784, .T. ) ;
#35715=CARTESIAN_POINT ( 'NONE',  ( -17.32694630114453105, -4.175268141568689195, 33.81360843649122216 ) ) ;
#35716=CARTESIAN_POINT ( 'NONE',  ( -7.146003881983773454, -10.01117774369187252, 34.36070679894347535 ) ) ;
#35717=CARTESIAN_POINT ( 'NONE',  ( -8.769230769230768274, -13.49023893513002648, 31.06009739812518688 ) ) ;
#35719=VERTEX_POINT ( 'NONE', #51359 ) ;
#35720=CARTESIAN_POINT ( 'NONE',  ( -12.52762187249434156, -9.780366693483667717, 34.19971097300155805 ) ) ;
#35721=CARTESIAN_POINT ( 'NONE',  ( -14.37377571864818648, -4.098570777380719399, 33.41473453929634729 ) ) ;
#35722=FACE_OUTER_BOUND ( 'NONE', #87232, .T. ) ;
#35723=CYLINDRICAL_SURFACE ( 'NONE', #15798, 0.2499999999999995559 ) ;
#35725=CARTESIAN_POINT ( 'NONE',  ( 13.13463865367303463, -5.728515186090277211, 34.42611988154120439 ) ) ;
#35726=ORIENTED_EDGE ( 'NONE', *, *, #4419, .F. ) ;
#35727=EDGE_CURVE ( 'NONE', #33332, #57312, #64898, .T. ) ;
#35728=DIRECTION ( 'NONE',  ( -0.000000000000000000, 0.8660254037844399289, -0.4999999999999980016 ) ) ;
#35729=ORIENTED_EDGE ( 'NONE', *, *, #27023, .F. ) ;
#35730=DIRECTION ( 'NONE',  ( -0.000000000000000000, -0.9396926207859092051, -0.3420201433256662704 ) ) ;
#35731=CARTESIAN_POINT ( 'NONE',  ( -1.515305987725690695, -12.35290016733513951, 31.75349464988449455 ) ) ;
#35732=FACE_OUTER_BOUND ( 'NONE', #79758, .T. ) ;
#35733=CARTESIAN_POINT ( 'NONE',  ( -12.23875892027005108, -2.847695495035523550, 31.58253572463339154 ) ) ;
#35734=CARTESIAN_POINT ( 'NONE',  ( 8.899275825150539276, -2.254550872974305342, 29.97347326024527092 ) ) ;
#35735=CARTESIAN_POINT ( 'NONE',  ( 0.2386597791098133969, -7.630691491037286056, 34.74850469731152458 ) ) ;
#35736=DIRECTION ( 'NONE',  ( 0.000000000000000000, 0.000000000000000000, -1.000000000000000000 ) ) ;
#35737=EDGE_CURVE ( 'NONE', #80445, #1486, #24354, .T. ) ;
#35740=CARTESIAN_POINT ( 'NONE',  ( -16.37733107841048863, -4.988325925672468131, 34.36044203135681130 ) ) ;
#35741=ORIENTED_EDGE ( 'NONE', *, *, #17231, .T. ) ;
#35744=CARTESIAN_POINT ( 'NONE',  ( 11.60371710973756443, -11.94971097300157403, 32.03036669348361443 ) ) ;
#35745=EDGE_LOOP ( 'NONE', ( #73886, #2949, #65144, #74066 ) ) ;
#35746=CARTESIAN_POINT ( 'NONE',  ( 10.86533002476265963, -8.476813868363244353, 34.90874843262270133 ) ) ;
#35747=CARTESIAN_POINT ( 'NONE',  ( 7.596153846153829825, -2.249999999999999112, 29.81609741502488120 ) ) ;
#35749=CARTESIAN_POINT ( 'NONE',  ( -2.307692307692305711, -1.790695186598648903, 34.54067556320373455 ) ) ;
#35750=CARTESIAN_POINT ( 'NONE',  ( 6.250054311638314708, -2.564540009722896752, 30.55348353981670684 ) ) ;
#35751=CARTESIAN_POINT ( 'NONE',  ( 12.23805351781451201, -10.81261337010820256, 33.49550067578627477 ) ) ;
#35752=EDGE_CURVE ( 'NONE', #15407, #2983, #18062, .T. ) ;
#35753=CARTESIAN_POINT ( 'NONE',  ( 7.053868730901711182, -11.18335022499818621, 33.13157742990016885 ) ) ;
#35755=CARTESIAN_POINT ( 'NONE',  ( -11.53846153846153655, -8.564572088678739092, 35.78748833219616898 ) ) ;
#35756=DIRECTION ( 'NONE',  ( -0.000000000000000000, -0.1736481776669307198, -0.9848077530122080203 ) ) ;
#35757=CARTESIAN_POINT ( 'NONE',  ( -2.084912638714241151, -3.020022701398814124, 32.48759521482552515 ) ) ;
#35758=CIRCLE ( 'NONE', #21344, 0.2500000000000002220 ) ;
#35759=CARTESIAN_POINT ( 'NONE',  ( 5.207448515156719360, -11.04252011169590020, 33.62494198852677130 ) ) ;
#35760=B_SPLINE_CURVE_WITH_KNOTS ( 'NONE', 3,
 ( #18522, #23922, #18964, #58153, #53176, #45979, #73473, #3653, #10428, #11765 ),
 .UNSPECIFIED., .F., .F.,
 ( 4, 2, 2, 2, 4 ),
 ( 0.0007817359430256293554, 0.0009771253907249952391, 0.001172514838424361123, 0.001367904286123726790, 0.001563293733823092673 ),
 .UNSPECIFIED. ) ;
#35761=CARTESIAN_POINT ( 'NONE',  ( -17.20748299053643748, -2.254533558242299396, 29.97296025877828640 ) ) ;
#35763=VERTEX_POINT ( 'NONE', #30676 ) ;
#35764=CARTESIAN_POINT ( 'NONE',  ( -14.98071491913091791, -8.303483539816728154, 34.68545999027711702 ) ) ;
#35766=CARTESIAN_POINT ( 'NONE',  ( -3.100243529005668019, -2.882268652242222284, 31.66798894389554064 ) ) ;
#35767=DIRECTION ( 'NONE',  ( 0.000000000000000000, 0.000000000000000000, 1.000000000000000000 ) ) ;
#35768=ORIENTED_EDGE ( 'NONE', *, *, #4166, .F. ) ;
#35769=EDGE_CURVE ( 'NONE', #36896, #13945, #44578, .T. ) ;
#35770=EDGE_CURVE ( 'NONE', #38055, #7411, #46839, .T. ) ;
#35771=CARTESIAN_POINT ( 'NONE',  ( -16.15384615384615330, -8.164416787775445883, 34.95778746994557906 ) ) ;
#35772=FACE_OUTER_BOUND ( 'NONE', #40552, .T. ) ;
#35773=CARTESIAN_POINT ( 'NONE',  ( 8.899756470994335089, -4.459921816937791661, 33.71989282347011851 ) ) ;
#35774=EDGE_CURVE ( 'NONE', #45628, #23088, #31569, .T. ) ;
#35775=ORIENTED_EDGE ( 'NONE', *, *, #25624, .T. ) ;
#35776=CARTESIAN_POINT ( 'NONE',  ( 0.6843180028068694964, -5.913360116392399668, 34.49180327182771322 ) ) ;
#35777=VERTEX_POINT ( 'NONE', #50497 ) ;
#35778=TOROIDAL_SURFACE ( 'NONE', #32881, 3.250000000000001332, 2.000000000000000000 ) ;
#35780=CARTESIAN_POINT ( 'NONE',  ( 18.00000000000000000, -3.322132147404559976, 32.92929555188717927 ) ) ;
#35781=CARTESIAN_POINT ( 'NONE',  ( -6.065270445960774914, -2.625532179533445198, 30.86335684631481513 ) ) ;
#35782=CARTESIAN_POINT ( 'NONE',  ( -9.692307692307814193, -6.835583212225970762, 34.95778746994575670 ) ) ;
#35783=CARTESIAN_POINT ( 'NONE',  ( 18.13079044096695469, -8.191423895709842640, 34.95447573519442130 ) ) ;
#35784=VERTEX_POINT ( 'NONE', #64447 ) ;
#35785=B_SPLINE_CURVE_WITH_KNOTS ( 'NONE', 3,
 ( #29251, #78745, #8971, #44500, #36440, #63894, #29688, #60251, #40004, #3964 ),
 .UNSPECIFIED., .F., .F.,
 ( 4, 2, 2, 2, 4 ),
 ( 0.0007817246256747463051, 0.0009771112852218896347, 0.001172497944769033181, 0.001367884604316176728, 0.001563271263863320057 ),
 .UNSPECIFIED. ) ;
#35786=ORIENTED_EDGE ( 'NONE', *, *, #69, .T. ) ;
#35787=EDGE_CURVE ( 'NONE', #12459, #12780, #38206, .T. ) ;
#35789=EDGE_LOOP ( 'NONE', ( #44278, #78539, #52826, #32588 ) ) ;
#35790=CARTESIAN_POINT ( 'NONE',  ( -17.20761454359064047, -10.54014554554151140, 33.71984207302941883 ) ) ;
#35792=CARTESIAN_POINT ( 'NONE',  ( -17.07692307692307665, -11.11383981884818262, 36.00935417666054406 ) ) ;
#35793=LINE ( 'NONE', #15962, #83035 ) ;
#35794=VECTOR ( 'NONE', #67190, 1000.000000000000000 ) ;
#35795=CARTESIAN_POINT ( 'NONE',  ( -7.596099426240392027, -4.074993327901524687, 33.72946981652012255 ) ) ;
#35796=CARTESIAN_POINT ( 'NONE',  ( 18.00000000000000000, -3.050289026998446396, 32.03036669348365706 ) ) ;
#35797=ORIENTED_EDGE ( 'NONE', *, *, #74300, .F. ) ;
#35799=VERTEX_POINT ( 'NONE', #65350 ) ;
#35800=AXIS2_PLACEMENT_3D ( 'NONE', #25476, #54264, #13734 ) ;
#35801=CARTESIAN_POINT ( 'NONE',  ( -3.007989689500820241, -10.81320215134717344, 33.49497208177562868 ) ) ;
#35803=DIRECTION ( 'NONE',  ( -0.000000000000000000, 0.8660254037844399289, -0.4999999999999980016 ) ) ;
#35804=CARTESIAN_POINT ( 'NONE',  ( -5.076923076923075762, -12.62096338111211580, 30.90682066428153263 ) ) ;
#35805=CARTESIAN_POINT ( 'NONE',  ( -17.14300648787895298, -12.37446782046654192, 30.86335684631486487 ) ) ;
#35808=ORIENTED_EDGE ( 'NONE', *, *, #45508, .T. ) ;
#35810=ORIENTED_EDGE ( 'NONE', *, *, #49892, .T. ) ;
#35811=CARTESIAN_POINT ( 'NONE',  ( 3.903822929624696680, -4.175268141568689195, 33.81360843649122216 ) ) ;
#35812=VERTEX_POINT ( 'NONE', #59034 ) ;
#35813=FACE_BOUND ( 'NONE', #20747, .T. ) ;
#35814=DIRECTION ( 'NONE',  ( -0.000000000000000000, 0.7660444431189791237, -0.6427876096865379196 ) ) ;
#35815=CARTESIAN_POINT ( 'NONE',  ( -2.307692307692305711, -3.513871655860378418, 32.76840700105978499 ) ) ;
#35816=ORIENTED_EDGE ( 'NONE', *, *, #4980, .T. ) ;
#35817=CARTESIAN_POINT ( 'NONE',  ( -14.05774689831426372, -8.476813868363244353, 34.90874843262270133 ) ) ;
#35819=CARTESIAN_POINT ( 'NONE',  ( -13.38461538461538325, -5.415277668671390821, 36.20867863119892149 ) ) ;
#35820=CARTESIAN_POINT ( 'NONE',  ( -15.29603967673000575, -6.879047030191174805, 34.71129190930000163 ) ) ;
#35821=CARTESIAN_POINT ( 'NONE',  ( 18.00000000000000000, -10.89733346790207413, 36.13435417666054406 ) ) ;
#35822=ORIENTED_EDGE ( 'NONE', *, *, #88877, .T. ) ;
#35823=CARTESIAN_POINT ( 'NONE',  ( 11.76124107972994537, -3.236590943229499029, 32.36255958852954251 ) ) ;
#35824=CARTESIAN_POINT ( 'NONE',  ( -9.692307692307691624, -2.900454961884010974, 35.62045528018868623 ) ) ;
#35825=CARTESIAN_POINT ( 'NONE',  ( 16.40390046548447245, -9.148310452688871663, 34.47095581063188519 ) ) ;
#35826=CARTESIAN_POINT ( 'NONE',  ( 15.23076923076923173, -11.33034616979429110, 35.88435417666054406 ) ) ;
#35827=DIRECTION ( 'NONE',  ( -0.000000000000000000, -0.9396926207859093161, -0.3420201433256663259 ) ) ;
#35828=CARTESIAN_POINT ( 'NONE',  ( 8.769230769230768274, -3.937682226553329556, 33.60647404775216529 ) ) ;
#35829=DIRECTION ( 'NONE',  ( -0.000000000000000000, -0.3420201433256694901, -0.9396926207859082059 ) ) ;
#35830=CARTESIAN_POINT ( 'NONE',  ( 6.923076923076802558, -3.300289026999228881, 32.46337939537708905 ) ) ;
#35831=CARTESIAN_POINT ( 'NONE',  ( -14.37377468705243722, -3.322132147404559532, 32.92929555188719348 ) ) ;
#35832=CARTESIAN_POINT ( 'NONE',  ( 5.076923076923075762, -13.37000171582298513, 34.34916445242398453 ) ) ;
#35833=CARTESIAN_POINT ( 'NONE',  ( -18.06527000055631760, -3.083524468853727551, 32.58852847137143272 ) ) ;
#35834=CARTESIAN_POINT ( 'NONE',  ( -10.83886953994894675, -6.716662450894489211, 34.94144148231605840 ) ) ;
#35835=VECTOR ( 'NONE', #2772, 1000.000000000000227 ) ;
#35837=ORIENTED_EDGE ( 'NONE', *, *, #7897, .T. ) ;
#35839=ORIENTED_EDGE ( 'NONE', *, *, #75793, .F. ) ;
#35840=DIRECTION ( 'NONE',  ( -0.000000000000000000, -0.000000000000000000, -1.000000000000000000 ) ) ;
#35841=ORIENTED_EDGE ( 'NONE', *, *, #2376, .F. ) ;
#35843=CYLINDRICAL_SURFACE ( 'NONE', #38825, 0.2499999999999986955 ) ;
#35844=VERTEX_POINT ( 'NONE', #3641 ) ;
#35845=CARTESIAN_POINT ( 'NONE',  ( -18.22292621751613950, -12.39988816332205701, 30.74660775122750778 ) ) ;
#35847=CARTESIAN_POINT ( 'NONE',  ( 1.384615384615386802, -1.117168528481311540, 33.14645433367849847 ) ) ;
#35848=B_SPLINE_CURVE_WITH_KNOTS ( 'NONE', 3,
 ( #46061, #19038, #46506, #12278, #44711, #38420, #3290, #24005, #65442, #3734 ),
 .UNSPECIFIED., .F., .F.,
 ( 4, 2, 2, 2, 4 ),
 ( 0.000000000000000000, 0.0001954339881912775425, 0.0003908679763825550850, 0.0005863019645738326005, 0.0007817359527651101701 ),
 .UNSPECIFIED. ) ;
#35849=CARTESIAN_POINT ( 'NONE',  ( 15.23076923076910916, -12.16647553114689728, 32.15551576947799362 ) ) ;
#35850=DIRECTION ( 'NONE',  ( -1.000000000000000000, 0.000000000000000000, 0.000000000000000000 ) ) ;
#35852=CARTESIAN_POINT ( 'NONE',  ( 11.28848480751918615, -2.779195860258146578, 31.39871582349836032 ) ) ;
#35853=DIRECTION ( 'NONE',  ( 1.000000000000000000, 0.000000000000000000, 0.000000000000000000 ) ) ;
#35855=CARTESIAN_POINT ( 'NONE',  ( -18.06527000055631405, -11.67786785259541205, 32.92929555188721480 ) ) ;
#35856=LINE ( 'NONE', #732, #80816 ) ;
#35859=EDGE_CURVE ( 'NONE', #74923, #1726, #26421, .T. ) ;
#35861=CARTESIAN_POINT ( 'NONE',  ( 17.07692307692295586, -2.379036618888197729, 30.90682066428292885 ) ) ;
#35863=ORIENTED_EDGE ( 'NONE', *, *, #45382, .T. ) ;
#35864=CARTESIAN_POINT ( 'NONE',  ( 1.634669804528839698, -8.346898887586323923, 34.93166121998716278 ) ) ;
#35865=CARTESIAN_POINT ( 'NONE',  ( -11.53846153846153655, -8.120952969808772792, 34.71129190930000163 ) ) ;
#35866=LINE ( 'NONE', #36313, #88675 ) ;
#35867=CARTESIAN_POINT ( 'NONE',  ( 8.769230769230768274, -5.471508081941601098, 34.59228464037088457 ) ) ;
#35870=VECTOR ( 'NONE', #24024, 1000.000000000000227 ) ;
#35871=CARTESIAN_POINT ( 'NONE',  ( 2.241608896736428491, -12.10708131394839349, 31.69288490824020244 ) ) ;
#35874=EDGE_CURVE ( 'NONE', #80757, #69974, #53615, .T. ) ;
#35875=ORIENTED_EDGE ( 'NONE', *, *, #44877, .T. ) ;
#35876=ORIENTED_EDGE ( 'NONE', *, *, #57448, .T. ) ;
#35877=EDGE_LOOP ( 'NONE', ( #41873, #81709 ) ) ;
#35878=CYLINDRICAL_SURFACE ( 'NONE', #16992, 0.2499999999999979738 ) ;
#35879=CARTESIAN_POINT ( 'NONE',  ( 11.53846153846153832, -13.49023893513002648, 31.06009739812518688 ) ) ;
#35880=CARTESIAN_POINT ( 'NONE',  ( -8.769230769230892619, -2.379036618888197729, 30.90682066428292885 ) ) ;
#35881=CARTESIAN_POINT ( 'NONE',  ( -13.31854703361294945, -12.10708131394839882, 31.69288490824020954 ) ) ;
#35882=CARTESIAN_POINT ( 'NONE',  ( 13.16113046005105680, -8.539481045369596401, 34.89627647299170832 ) ) ;
#35883=ORIENTED_EDGE ( 'NONE', *, *, #29945, .F. ) ;
#35884=CARTESIAN_POINT ( 'NONE',  ( -11.53846153846153655, -1.242168528481310874, 33.36296068462461051 ) ) ;
#35886=ADVANCED_FACE ( 'NONE', ( #46857 ), #80210, .F. ) ;
#35887=VERTEX_POINT ( 'NONE', #38775 ) ;
#35888=ORIENTED_EDGE ( 'NONE', *, *, #26025, .F. ) ;
#35889=CARTESIAN_POINT ( 'NONE',  ( -12.46153846153846168, -2.900454961884010974, 35.62045528018868623 ) ) ;
#35890=ORIENTED_EDGE ( 'NONE', *, *, #55480, .T. ) ;
#35891=CARTESIAN_POINT ( 'NONE',  ( 8.769230769230647482, -2.892918686052165622, 31.69288490824153470 ) ) ;
#35892=VECTOR ( 'NONE', #87133, 1000.000000000000114 ) ;
#35893=EDGE_CURVE ( 'NONE', #61168, #71998, #60699, .T. ) ;
#35895=B_SPLINE_CURVE_WITH_KNOTS ( 'NONE', 3,
 ( #62829, #49773, #69606, #70497, #36276, #1150, #7912, #9252, #84467, #78137 ),
 .UNSPECIFIED., .F., .F.,
 ( 4, 2, 2, 2, 4 ),
 ( 0.0007817359430256252354, 0.0009771253907249898181, 0.001172514838424354401, 0.001367904286123718983, 0.001563293733823083566 ),
 .UNSPECIFIED. ) ;
#35897=CARTESIAN_POINT ( 'NONE',  ( 2.084826885488670456, -2.501496062324912284, 29.88072118266895671 ) ) ;
#35898=VERTEX_POINT ( 'NONE', #74339 ) ;
#35899=EDGE_LOOP ( 'NONE', ( #61519, #47355, #21303, #54938 ) ) ;
#35900=ORIENTED_EDGE ( 'NONE', *, *, #62653, .T. ) ;
#35901=CARTESIAN_POINT ( 'NONE',  ( -14.24254652836034118, -7.750023238201979581, 34.74374492549440419 ) ) ;
#35903=VERTEX_POINT ( 'NONE', #33354 ) ;
#35904=CARTESIAN_POINT ( 'NONE',  ( 11.53846153846141753, -6.879047030192662504, 34.71129190930017927 ) ) ;
#35905=FACE_OUTER_BOUND ( 'NONE', #87150, .T. ) ;
#35906=B_SPLINE_CURVE_WITH_KNOTS ( 'NONE', 3,
 ( #34065, #82264, #68738, #75940, #27311, #54774, #61973, #34511, #8375, #1165 ),
 .UNSPECIFIED., .F., .F.,
 ( 4, 2, 2, 2, 4 ),
 ( 0.000000000000000000, 0.0001954311564186865221, 0.0003908623128373730441, 0.0005862934692560595662, 0.0007817246256747460882 ),
 .UNSPECIFIED. ) ;
#35907=B_SPLINE_CURVE_WITH_KNOTS ( 'NONE', 3,
 ( #205, #63222, #76751, #1537, #42967, #2839, #85283, #15053, #63669, #30332 ),
 .UNSPECIFIED., .F., .F.,
 ( 4, 2, 2, 2, 4 ),
 ( 0.0007817359430256216575, 0.0009771253907249856981, 0.001172514838424349847, 0.001367904286123713779, 0.001563293733823077928 ),
 .UNSPECIFIED. ) ;
#35908=DIRECTION ( 'NONE',  ( -0.000000000000000000, -0.3420201433256694346, -0.9396926207859080948 ) ) ;
#35909=VERTEX_POINT ( 'NONE', #12638 ) ;
#35910=B_SPLINE_CURVE_WITH_KNOTS ( 'NONE', 3,
 ( #55358, #8514, #83738, #49046, #76074, #76971, #13932, #68873, #7628, #28330 ),
 .UNSPECIFIED., .F., .F.,
 ( 4, 2, 2, 2, 4 ),
 ( 0.0007817359430256216575, 0.0009771253907249856981, 0.001172514838424349630, 0.001367904286123713779, 0.001563293733823077711 ),
 .UNSPECIFIED. ) ;
#35911=CARTESIAN_POINT ( 'NONE',  ( -11.53846153846165912, -5.219633306517616589, 34.19971097300220464 ) ) ;
#35912=DIRECTION ( 'NONE',  ( -0.000000000000000000, -0.6427876096865404731, -0.7660444431189770143 ) ) ;
#35913=ORIENTED_EDGE ( 'NONE', *, *, #19152, .T. ) ;
#35914=FACE_BOUND ( 'NONE', #1040, .T. ) ;
#35915=CARTESIAN_POINT ( 'NONE',  ( 11.31497659473759043, -5.113361153441934093, 34.14387501736622710 ) ) ;
#35916=CARTESIAN_POINT ( 'NONE',  ( -18.00000000000012079, -12.51329471203414379, 31.30864560766407578 ) ) ;
#35917=DIRECTION ( 'NONE',  ( -1.000000000000000000, 0.000000000000000000, 0.000000000000000000 ) ) ;
#35918=FACE_OUTER_BOUND ( 'NONE', #10538, .T. ) ;
#35919=AXIS2_PLACEMENT_3D ( 'NONE', #72363, #57078, #50750 ) ;
#35920=DIRECTION ( 'NONE',  ( 1.000000000000000000, 0.000000000000000000, 0.000000000000000000 ) ) ;
#35921=CARTESIAN_POINT ( 'NONE',  ( -5.076923076923075762, -10.51840700105979565, 33.73612834413961536 ) ) ;
#35922=CARTESIAN_POINT ( 'NONE',  ( -16.08777780284371772, -8.973038597847269315, 34.52809138561122637 ) ) ;
#35923=ORIENTED_EDGE ( 'NONE', *, *, #50180, .F. ) ;
#35925=CARTESIAN_POINT ( 'NONE',  ( 5.010840697562940704, -3.937682226553329556, 33.60647404775217240 ) ) ;
#35928=CIRCLE ( 'NONE', #22920, 0.2500000000000002220 ) ;
#35929=CARTESIAN_POINT ( 'NONE',  ( -16.21992853320628925, -12.62096338111211580, 30.90682066428152908 ) ) ;
#35930=CARTESIAN_POINT ( 'NONE',  ( -14.08491263871423982, -9.418065098278013636, 34.63729479722530158 ) ) ;
#35931=CARTESIAN_POINT ( 'NONE',  ( -16.08777780284372128, -10.51840700105979565, 33.73612834413962247 ) ) ;
#35932=DIRECTION ( 'NONE',  ( -0.000000000000000000, 1.000000000000000000, 3.491481338843133355E-15 ) ) ;
#35933=EDGE_CURVE ( 'NONE', #58351, #10580, #47785, .T. ) ;
#35934=CARTESIAN_POINT ( 'NONE',  ( 15.23076923076923173, -2.292212530054420494, 30.41441678777542634 ) ) ;
#35935=CARTESIAN_POINT ( 'NONE',  ( 18.00000000000000000, -5.180354513474913603, 36.12317359536750416 ) ) ;
#35936=FACE_BOUND ( 'NONE', #64129, .T. ) ;
#35937=CARTESIAN_POINT ( 'NONE',  ( -2.373775718648186928, -6.386643153685125363, 34.62446782046654903 ) ) ;
#35938=CARTESIAN_POINT ( 'NONE',  ( 15.36156103859402045, -12.11778462344221019, 31.66786338562085135 ) ) ;
#35939=CARTESIAN_POINT ( 'NONE',  ( -15.29603967673000575, -9.442884908240170461, 34.35708131394840592 ) ) ;
#35940=CYLINDRICAL_SURFACE ( 'NONE', #14191, 0.2500000000000008882 ) ;
#35941=DIRECTION ( 'NONE',  ( -0.000000000000000000, -0.6427876096865404731, -0.7660444431189770143 ) ) ;
#35942=CARTESIAN_POINT ( 'NONE',  ( -7.846153846153967493, -3.643525952248795718, 33.31231777344771672 ) ) ;
#35944=ORIENTED_EDGE ( 'NONE', *, *, #82182, .F. ) ;
#35945=ORIENTED_EDGE ( 'NONE', *, *, #27883, .F. ) ;
#35946=FACE_OUTER_BOUND ( 'NONE', #20510, .T. ) ;
#35947=FACE_OUTER_BOUND ( 'NONE', #60936, .T. ) ;
#35948=FACE_OUTER_BOUND ( 'NONE', #29482, .T. ) ;
#35949=DIRECTION ( 'NONE',  ( -0.000000000000000000, 0.5000000000000011102, -0.8660254037844380415 ) ) ;
#35952=EDGE_CURVE ( 'NONE', #31103, #32628, #85431, .T. ) ;
#35953=CARTESIAN_POINT ( 'NONE',  ( 4.284684571858915270, -7.277220443632450575, 34.74524770363009196 ) ) ;
#35954=B_SPLINE_CURVE_WITH_KNOTS ( 'NONE', 3,
 ( #12754, #61369, #75350, #88881, #42012, #40240, #82991, #69028, #55951, #74457 ),
 .UNSPECIFIED., .F., .F.,
 ( 4, 2, 2, 2, 4 ),
 ( 0.000000000000000000, 0.0001954311564186863865, 0.0003908623128373727731, 0.0005862934692560591325, 0.0007817246256747455461 ),
 .UNSPECIFIED. ) ;
#35955=DIRECTION ( 'NONE',  ( -0.000000000000000000, -0.9396926207859092051, -0.3420201433256662704 ) ) ;
#35956=DIRECTION ( 'NONE',  ( 0.000000000000000000, 0.000000000000000000, 1.000000000000000000 ) ) ;
#35957=LINE ( 'NONE', #23746, #22868 ) ;
#35958=CARTESIAN_POINT ( 'NONE',  ( 2.437737363612081598, -2.254550872974306674, 29.97347326024527447 ) ) ;
#35959=CARTESIAN_POINT ( 'NONE',  ( -4.826977667545033768, -6.653508905675592722, 34.93172785388651391 ) ) ;
#35960=DIRECTION ( 'NONE',  ( -0.000000000000000000, -0.3420201433256694901, -0.9396926207859082059 ) ) ;
#35961=CARTESIAN_POINT ( 'NONE',  ( -5.999999999999998224, -3.669653830205710676, 35.88435417666054406 ) ) ;
#35962=EDGE_LOOP ( 'NONE', ( #22444, #20181, #5122, #3815 ) ) ;
#35963=AXIS2_PLACEMENT_3D ( 'NONE', #40506, #88701, #27418 ) ;
#35964=CARTESIAN_POINT ( 'NONE',  ( 2.307692307692309264, -3.322132147404559976, 32.92929555188717927 ) ) ;
#35965=CARTESIAN_POINT ( 'NONE',  ( 10.74591005361826390, -5.915461855592780260, 34.75538340440931506 ) ) ;
#35968=EDGE_CURVE ( 'NONE', #76747, #67048, #74789, .T. ) ;
#35969=CARTESIAN_POINT ( 'NONE',  ( 6.792386319966615460, -4.684245665217972032, 34.18127051446801090 ) ) ;
#35972=FACE_OUTER_BOUND ( 'NONE', #44383, .T. ) ;
#35974=ORIENTED_EDGE ( 'NONE', *, *, #25983, .T. ) ;
#35976=CARTESIAN_POINT ( 'NONE',  ( -4.946397375159515164, -10.19071101563364756, 33.96452234770658407 ) ) ;
#35977=EDGE_CURVE ( 'NONE', #10638, #78414, #54320, .T. ) ;
#35978=EDGE_LOOP ( 'NONE', ( #75331, #85694 ) ) ;
#35979=DIRECTION ( 'NONE',  ( -0.000000000000000000, -0.7660444431189791237, -0.6427876096865379196 ) ) ;
#35980=CARTESIAN_POINT ( 'NONE',  ( 7.596153846153846700, -7.500000000000001776, 34.75000000000000000 ) ) ;
#35982=DIRECTION ( 'NONE',  ( -0.000000000000000000, 0.6427876096865404731, -0.7660444431189770143 ) ) ;
#35983=CARTESIAN_POINT ( 'NONE',  ( -15.93083480223330461, -3.105924265160262099, 32.13625925475356127 ) ) ;
#35984=AXIS2_PLACEMENT_3D ( 'NONE', #58151, #72114, #59496 ) ;
#35985=CARTESIAN_POINT ( 'NONE',  ( 18.00000000000000000, -8.564572088678739092, 35.78748833219616898 ) ) ;
#35987=ORIENTED_EDGE ( 'NONE', *, *, #88960, .F. ) ;
#35988=EDGE_LOOP ( 'NONE', ( #10040, #58621, #18091, #35923 ) ) ;
#35989=CARTESIAN_POINT ( 'NONE',  ( -6.792551484843277976, -8.630441415882550871, 34.87705825610312615 ) ) ;
#35990=ORIENTED_EDGE ( 'NONE', *, *, #25569, .T. ) ;
#35993=DIRECTION ( 'NONE',  ( -0.000000000000000000, 0.7660444431189791237, -0.6427876096865379196 ) ) ;
#35994=CARTESIAN_POINT ( 'NONE',  ( 17.07692307692307665, -12.37446782046654192, 30.86335684631486131 ) ) ;
#35995=B_SPLINE_CURVE_WITH_KNOTS ( 'NONE', 3,
 ( #82687, #75467, #76353, #20085, #258, #13764, #47098, #26402, #14661, #6129 ),
 .UNSPECIFIED., .F., .F.,
 ( 4, 2, 2, 2, 4 ),
 ( 0.0007817359430256318490, 0.0009771253907249984917, 0.001172514838424365026, 0.001367904286123731560, 0.001563293733823098311 ),
 .UNSPECIFIED. ) ;
#35997=DIRECTION ( 'NONE',  ( -0.000000000000000000, -0.000000000000000000, -1.000000000000000000 ) ) ;
#35999=CARTESIAN_POINT ( 'NONE',  ( 3.164686851409094892, -9.905515769479276145, 34.41647553114623292 ) ) ;
#36000=B_SPLINE_CURVE_WITH_KNOTS ( 'NONE', 3,
 ( #29429, #9577, #22653, #44679, #3260, #37041, #44229, #85251, #72163, #2808 ),
 .UNSPECIFIED., .F., .F.,
 ( 4, 2, 2, 2, 4 ),
 ( 0.0007817246256747507503, 0.0009771112852218959231, 0.001172497944769040987, 0.001367884604316186052, 0.001563271263863331116 ),
 .UNSPECIFIED. ) ;
#36002=VERTEX_POINT ( 'NONE', #64227 ) ;
#36003=ORIENTED_EDGE ( 'NONE', *, *, #79002, .F. ) ;
#36004=CARTESIAN_POINT ( 'NONE',  ( -2.176853977205544854, -7.277220318596959281, 34.99547417642776992 ) ) ;
#36005=ORIENTED_EDGE ( 'NONE', *, *, #21248, .F. ) ;
#36006=CARTESIAN_POINT ( 'NONE',  ( 17.07692307692307665, -4.786620604624113540, 33.94971097300155094 ) ) ;
#36007=ORIENTED_EDGE ( 'NONE', *, *, #47431, .F. ) ;
#36008=EDGE_CURVE ( 'NONE', #74006, #23956, #16678, .T. ) ;
#36009=ADVANCED_FACE ( 'NONE', ( #49837 ), #68458, .F. ) ;
#36010=CARTESIAN_POINT ( 'NONE',  ( -3.230769230769229949, -12.78798330534102767, 29.49999999999997868 ) ) ;
#36011=CARTESIAN_POINT ( 'NONE',  ( 6.000000000000001776, -2.499999999999998668, 29.75000000000001421 ) ) ;
#36012=EDGE_LOOP ( 'NONE', ( #58611, #45101, #79731, #71872 ) ) ;
#36013=CARTESIAN_POINT ( 'NONE',  ( 7.976679547917409963, -8.586989748646452369, 34.63063291749215011 ) ) ;
#36014=VERTEX_POINT ( 'NONE', #27920 ) ;
#36015=DIRECTION ( 'NONE',  ( -0.000000000000000000, 0.5000000000000011102, -0.8660254037844381525 ) ) ;
#36016=VERTEX_POINT ( 'NONE', #36769 ) ;
#36017=DIRECTION ( 'NONE',  ( 0.000000000000000000, 0.9396926207859126468, -0.3420201433256571111 ) ) ;
#36018=CARTESIAN_POINT ( 'NONE',  ( -16.08859058257013075, -3.835265460703683349, 33.15142922261929925 ) ) ;
#36020=CARTESIAN_POINT ( 'NONE',  ( 15.90386942290380290, -12.41269422305637171, 30.68257228309993323 ) ) ;
#36021=AXIS2_PLACEMENT_3D ( 'NONE', #2927, #4273, #72282 ) ;
#36022=CARTESIAN_POINT ( 'NONE',  ( 6.792386319966616348, -5.496505350115500121, 34.60290016733514307 ) ) ;
#36024=FACE_BOUND ( 'NONE', #86966, .T. ) ;
#36025=CARTESIAN_POINT ( 'NONE',  ( -1.634615384615383027, -2.249999999999998668, 29.75000000000000355 ) ) ;
#36027=CARTESIAN_POINT ( 'NONE',  ( 6.000000000000309086, -2.506253911140614576, 30.00000000000323297 ) ) ;
#36028=CARTESIAN_POINT ( 'NONE',  ( 3.453782074862624896, -4.762714258010882773, 34.23016756924214832 ) ) ;
#36030=CARTESIAN_POINT ( 'NONE',  ( -16.21992853320628925, -2.486705287966280320, 31.30864560766543647 ) ) ;
#36031=ORIENTED_EDGE ( 'NONE', *, *, #52518, .F. ) ;
#36032=CARTESIAN_POINT ( 'NONE',  ( -6.130560591741918586, -2.504760397472873823, 29.97295953869789997 ) ) ;
#36033=VERTEX_POINT ( 'NONE', #2975 ) ;
#36034=ORIENTED_EDGE ( 'NONE', *, *, #40073, .F. ) ;
#36035=CARTESIAN_POINT ( 'NONE',  ( -1.253824943648434553, -4.684288915650983043, 34.18129842949671371 ) ) ;
#36036=CARTESIAN_POINT ( 'NONE',  ( 16.15384615384615330, -12.10708131394839349, 31.69288490824020244 ) ) ;
#36037=CARTESIAN_POINT ( 'NONE',  ( 6.923076923076924238, -6.386643153685126251, 34.62446782046654192 ) ) ;
#36038=DIRECTION ( 'NONE',  ( -0.000000000000000000, -0.000000000000000000, -1.000000000000000000 ) ) ;
#36039=DIRECTION ( 'NONE',  ( 0.000000000000000000, 0.6427876096865373645, -0.7660444431189797898 ) ) ;
#36040=CARTESIAN_POINT ( 'NONE',  ( 14.53047197667037516, -11.60474049983371003, 33.02348890104160262 ) ) ;
#36041=ORIENTED_EDGE ( 'NONE', *, *, #78791, .T. ) ;
#36042=EDGE_CURVE ( 'NONE', #34976, #46832, #23783, .T. ) ;
#36043=CARTESIAN_POINT ( 'NONE',  ( -18.00000000000000000, -5.557115091759784242, 34.35708131394839171 ) ) ;
#36044=CARTESIAN_POINT ( 'NONE',  ( 1.634560902963529072, -12.22109172314383052, 31.39792113162168263 ) ) ;
#36045=CARTESIAN_POINT ( 'NONE',  ( -12.59222906464877134, -11.37499894934982692, 33.29245874905763003 ) ) ;
#36046=CARTESIAN_POINT ( 'NONE',  ( 2.980745993476265010, -3.202444869320336451, 32.30641848906366675 ) ) ;
#36047=CARTESIAN_POINT ( 'NONE',  ( 13.38461538461538680, -5.471508081941601098, 34.59228464037088457 ) ) ;
#36048=EDGE_CURVE ( 'NONE', #79283, #15980, #13498, .T. ) ;
#36049=EDGE_CURVE ( 'NONE', #23814, #12523, #9198, .T. ) ;
#36050=B_SPLINE_CURVE_WITH_KNOTS ( 'NONE', 3,
 ( #1257, #69723, #76929, #15231, #48114, #42703, #50757, #22855, #10682, #16991 ),
 .UNSPECIFIED., .F., .F.,
 ( 4, 2, 2, 2, 4 ),
 ( 0.000000000000000000, 0.0001954311564186871184, 0.0003908623128373742367, 0.0005862934692560614093, 0.0007817246256747484735 ),
 .UNSPECIFIED. ) ;
#36052=EDGE_LOOP ( 'NONE', ( #54882, #48042 ) ) ;
#36053=AXIS2_PLACEMENT_3D ( 'NONE', #47575, #32732, #20113 ) ;
#36054=VECTOR ( 'NONE', #13644, 1000.000000000000227 ) ;
#36056=ADVANCED_FACE ( 'NONE', ( #63796 ), #8867, .F. ) ;
#36059=DIRECTION ( 'NONE',  ( 0.000000000000000000, -6.938893903907222067E-15, 1.000000000000000000 ) ) ;
#36060=CARTESIAN_POINT ( 'NONE',  ( -12.21159294319032185, -6.696923467548660192, 34.68552623307873972 ) ) ;
#36061=CARTESIAN_POINT ( 'NONE',  ( -14.08491276642389423, -6.760870238392817200, 34.69528174975672385 ) ) ;
#36062=DIRECTION ( 'NONE',  ( 0.000000000000000000, 0.000000000000000000, -1.000000000000000000 ) ) ;
#36064=EDGE_CURVE ( 'NONE', #42886, #88546, #23251, .T. ) ;
#36065=CARTESIAN_POINT ( 'NONE',  ( -8.769230769230768274, -8.564572088678739092, 35.78748833219616898 ) ) ;
#36066=ORIENTED_EDGE ( 'NONE', *, *, #53227, .T. ) ;
#36067=DIRECTION ( 'NONE',  ( 0.000000000000000000, 0.3420201433256641055, -0.9396926207859100932 ) ) ;
#36068=CARTESIAN_POINT ( 'NONE',  ( -16.15384615384627409, -11.94971097300221174, 32.03036669348237098 ) ) ;
#36069=EDGE_LOOP ( 'NONE', ( #37377, #77993, #70441, #27343 ) ) ;
#36071=CARTESIAN_POINT ( 'NONE',  ( 7.846153846153846700, -12.78798330534102945, 29.74999999999997868 ) ) ;
#36072=CARTESIAN_POINT ( 'NONE',  ( 11.40777007179398339, -4.118384482072086072, 33.43331474514187107 ) ) ;
#36073=DIRECTION ( 'NONE',  ( 0.000000000000000000, 0.000000000000000000, 1.000000000000000000 ) ) ;
#36074=CYLINDRICAL_SURFACE ( 'NONE', #73818, 0.2499999999999997502 ) ;
#36076=VERTEX_POINT ( 'NONE', #43967 ) ;
#36077=CARTESIAN_POINT ( 'NONE',  ( -15.23076923076935252, -6.835583212225970762, 34.95778746994575670 ) ) ;
#36078=CARTESIAN_POINT ( 'NONE',  ( -17.07692307692319744, -5.094484230521993062, 34.41647553114689373 ) ) ;
#36080=DIRECTION ( 'NONE',  ( 1.000000000000000000, 0.000000000000000000, 0.000000000000000000 ) ) ;
#36081=CARTESIAN_POINT ( 'NONE',  ( -3.099978789802280144, -10.70102852606553157, 33.91149625220312913 ) ) ;
#36082=ORIENTED_EDGE ( 'NONE', *, *, #21722, .F. ) ;
#36083=CARTESIAN_POINT ( 'NONE',  ( 0.4615384615384611200, -3.937682226553329556, 33.60647404775216529 ) ) ;
#36084=CARTESIAN_POINT ( 'NONE',  ( -2.531177251416254936, -3.236172620538810385, 32.36188796281390267 ) ) ;
#36085=EDGE_CURVE ( 'NONE', #7957, #9491, #71432, .T. ) ;
#36086=ORIENTED_EDGE ( 'NONE', *, *, #61798, .T. ) ;
#36087=CARTESIAN_POINT ( 'NONE',  ( -1.253823576790596750, -6.413143153341454017, 34.63066358083362672 ) ) ;
#36088=EDGE_CURVE ( 'NONE', #52651, #87412, #42528, .T. ) ;
#36089=CARTESIAN_POINT ( 'NONE',  ( 9.626984776815520561, -7.749976743299138882, 34.99404534957040624 ) ) ;
#36091=B_SPLINE_CURVE_WITH_KNOTS ( 'NONE', 3,
 ( #17782, #4711, #65947, #47904, #28529, #7375, #61407, #68186, #21315, #40280 ),
 .UNSPECIFIED., .F., .F.,
 ( 4, 2, 2, 2, 4 ),
 ( 0.0007817359430256316322, 0.0009771253907249980580, 0.001172514838424364592, 0.001367904286123731127, 0.001563293733823097661 ),
 .UNSPECIFIED. ) ;
#36092=CARTESIAN_POINT ( 'NONE',  ( 0.4615384615384611200, -8.564572088678739092, 35.78748833219616898 ) ) ;
#36093=CARTESIAN_POINT ( 'NONE',  ( -5.749999999999995559, -2.499999999999999112, 29.81604066197450109 ) ) ;
#36094=LINE ( 'NONE', #63545, #9531 ) ;
#36095=CARTESIAN_POINT ( 'NONE',  ( -12.33074802057151409, -10.70102852606553157, 33.91149625220312913 ) ) ;
#36096=VECTOR ( 'NONE', #70080, 1000.000000000000000 ) ;
#36097=EDGE_LOOP ( 'NONE', ( #28611, #15406, #57927, #5692, #81519, #73338 ) ) ;
#36098=LINE ( 'NONE', #8178, #75816 ) ;
#36099=ORIENTED_EDGE ( 'NONE', *, *, #35787, .F. ) ;
#36100=CARTESIAN_POINT ( 'NONE',  ( 12.33084785842815911, -11.93127051446799847, 32.56575433478202797 ) ) ;
#36101=CARTESIAN_POINT ( 'NONE',  ( 5.934675987195693558, -7.749976730030849303, 34.74374725381503737 ) ) ;
#36102=VERTEX_POINT ( 'NONE', #30052 ) ;
#36103=DIRECTION ( 'NONE',  ( 1.000000000000000000, 0.000000000000000000, 0.000000000000000000 ) ) ;
#36104=CARTESIAN_POINT ( 'NONE',  ( -14.53117723225664015, -2.353723527008296568, 30.78948104536958752 ) ) ;
#36106=CYLINDRICAL_SURFACE ( 'NONE', #76675, 0.2499999999999973355 ) ;
#36108=EDGE_CURVE ( 'NONE', #19870, #9301, #78228, .T. ) ;
#36109=ADVANCED_FACE ( 'NONE', ( #36803 ), #9343, .F. ) ;
#36111=ORIENTED_EDGE ( 'NONE', *, *, #51099, .T. ) ;
#36112=FACE_BOUND ( 'NONE', #44591, .T. ) ;
#36113=ORIENTED_EDGE ( 'NONE', *, *, #56562, .F. ) ;
#36114=CARTESIAN_POINT ( 'NONE',  ( 15.45378058238208041, -2.554770724473668153, 30.48948780036025852 ) ) ;
#36116=CARTESIAN_POINT ( 'NONE',  ( -18.00000000000012079, -11.06231777344772027, 33.60647404775119895 ) ) ;
#36117=EDGE_CURVE ( 'NONE', #70063, #33903, #79062, .T. ) ;
#36118=CARTESIAN_POINT ( 'NONE',  ( 13.51514108637895184, -10.88167719472716399, 33.43325721877153711 ) ) ;
#36120=AXIS2_PLACEMENT_3D ( 'NONE', #78238, #23730, #58855 ) ;
#36121=ORIENTED_EDGE ( 'NONE', *, *, #16677, .F. ) ;
#36122=EDGE_LOOP ( 'NONE', ( #84668, #42539, #65750, #14483 ) ) ;
#36123=EDGE_CURVE ( 'NONE', #72614, #70706, #29607, .T. ) ;
#36124=VERTEX_POINT ( 'NONE', #56194 ) ;
#36125=FACE_OUTER_BOUND ( 'NONE', #2629, .T. ) ;
#36126=B_SPLINE_CURVE_WITH_KNOTS ( 'NONE', 3,
 ( #22254, #84411, #71757, #37526, #2848, #84856, #37983, #56485, #30772, #36656 ),
 .UNSPECIFIED., .F., .F.,
 ( 4, 2, 2, 2, 4 ),
 ( 0.0007817246256747452209, 0.0009771112852218879000, 0.001172497944769030362, 0.001367884604316172825, 0.001563271263863315504 ),
 .UNSPECIFIED. ) ;
#36127=EDGE_LOOP ( 'NONE', ( #8556, #76202 ) ) ;
#36128=B_SPLINE_CURVE_WITH_KNOTS ( 'NONE', 3,
 ( #6779, #67161, #46438, #32476, #5014, #33380, #73482, #74362, #19411, #46878 ),
 .UNSPECIFIED., .F., .F.,
 ( 4, 2, 2, 2, 4 ),
 ( 0.000000000000000000, 0.0001954311564186861968, 0.0003908623128373723936, 0.0005862934692560585904, 0.0007817246256747447872 ),
 .UNSPECIFIED. ) ;
#36129=CARTESIAN_POINT ( 'NONE',  ( 16.15384615384615330, -5.557115091759785130, 34.35708131394839171 ) ) ;
#36130=EDGE_CURVE ( 'NONE', #77977, #25611, #22405, .T. ) ;
#36131=CARTESIAN_POINT ( 'NONE',  ( 17.01084069756294781, -3.322132147404559976, 32.92929555188719348 ) ) ;
#36132=CARTESIAN_POINT ( 'NONE',  ( -18.22348492456433178, -6.716662450894492764, 34.94144148231605840 ) ) ;
#36133=ORIENTED_EDGE ( 'NONE', *, *, #55478, .T. ) ;
#36134=CARTESIAN_POINT ( 'NONE',  ( -8.519285359852728945, -4.176053281294518804, 33.81426240980091791 ) ) ;
#36137=CARTESIAN_POINT ( 'NONE',  ( 4.153846153846030731, -2.657715359629662988, 31.77849191805970364 ) ) ;
#36138=CARTESIAN_POINT ( 'NONE',  ( 11.78851585009985214, -8.303483539816731707, 34.68545999027711702 ) ) ;
#36139=ORIENTED_EDGE ( 'NONE', *, *, #40617, .T. ) ;
#36140=ORIENTED_EDGE ( 'NONE', *, *, #44557, .T. ) ;
#36141=ORIENTED_EDGE ( 'NONE', *, *, #51398, .T. ) ;
#36142=CARTESIAN_POINT ( 'NONE',  ( -3.931066612577744923, -10.11255958852956027, 34.01340905677048454 ) ) ;
#36143=CARTESIAN_POINT ( 'NONE',  ( -5.076923076923075762, -2.708943851104267164, 35.45975837776705220 ) ) ;
#36144=CARTESIAN_POINT ( 'NONE',  ( 10.61538461538461675, -2.292212530054420494, 30.41441678777542634 ) ) ;
#36145=VECTOR ( 'NONE', #76080, 1000.000000000000114 ) ;
#36147=CARTESIAN_POINT ( 'NONE',  ( -12.46153846153858247, -6.879047030192662504, 34.71129190930017927 ) ) ;
#36148=FACE_BOUND ( 'NONE', #22773, .T. ) ;
#36149=CARTESIAN_POINT ( 'NONE',  ( 8.546303810323916395, -10.77366814457252175, 33.85459836347579454 ) ) ;
#36150=ORIENTED_EDGE ( 'NONE', *, *, #81964, .T. ) ;
#36151=EDGE_CURVE ( 'NONE', #34125, #14249, #45721, .T. ) ;
#36152=CARTESIAN_POINT ( 'NONE',  ( -3.164700879766790820, -2.538708090699994813, 30.37095296980875503 ) ) ;
#36153=CARTESIAN_POINT ( 'NONE',  ( 2.307692307692309264, -1.044019251281081972, 31.83374038241031911 ) ) ;
#36154=LINE ( 'NONE', #42907, #50207 ) ;
#36155=CARTESIAN_POINT ( 'NONE',  ( -11.53846153846165912, -3.835265460704628371, 33.15142922262033665 ) ) ;
#36158=CARTESIAN_POINT ( 'NONE',  ( -18.00000000000012079, -8.613356846316285953, 34.62446782046622218 ) ) ;
#36159=EDGE_CURVE ( 'NONE', #16890, #43377, #69335, .T. ) ;
#36161=FACE_BOUND ( 'NONE', #18565, .T. ) ;
#36162=CARTESIAN_POINT ( 'NONE',  ( -16.94639737515951339, -4.459921816937789885, 33.71989282347011851 ) ) ;
#36163=CYLINDRICAL_SURFACE ( 'NONE', #50646, 0.2500000000000008882 ) ;
#36164=CARTESIAN_POINT ( 'NONE',  ( -6.673076923075486278, -7.500000000000155431, 34.75000000000007105 ) ) ;
#36165=ORIENTED_EDGE ( 'NONE', *, *, #57238, .T. ) ;
#36166=CARTESIAN_POINT ( 'NONE',  ( 0.4615384615384611200, -10.51840700105979565, 33.73612834413961536 ) ) ;
#36167=CARTESIAN_POINT ( 'NONE',  ( 15.29683656411930848, -2.292212530054420494, 30.41441678777542990 ) ) ;
#36168=CARTESIAN_POINT ( 'NONE',  ( -15.23076923076935252, -10.33852847137269571, 34.16647553114546554 ) ) ;
#36169=DIRECTION ( 'NONE',  ( 0.000000000000000000, 0.7660444431189822323, -0.6427876096865344779 ) ) ;
#36170=VERTEX_POINT ( 'NONE', #23284 ) ;
#36171=EDGE_CURVE ( 'NONE', #74862, #60729, #568, .T. ) ;
#36172=FACE_OUTER_BOUND ( 'NONE', #33073, .T. ) ;
#36173=ORIENTED_EDGE ( 'NONE', *, *, #87151, .F. ) ;
#36174=CARTESIAN_POINT ( 'NONE',  ( 13.45068271796546178, -8.164416787775445883, 34.95778746994558617 ) ) ;
#36175=EDGE_LOOP ( 'NONE', ( #73124, #38148 ) ) ;
#36176=CARTESIAN_POINT ( 'NONE',  ( -8.545803807369198424, -7.630147231320743018, 34.74852402298682819 ) ) ;
#36177=CARTESIAN_POINT ( 'NONE',  ( -10.83886955910856464, -12.44517049084099725, 30.48991314939691932 ) ) ;
#36178=CARTESIAN_POINT ( 'NONE',  ( 4.826946332874485712, -2.544273027872574922, 31.48422191005632342 ) ) ;
#36179=B_SPLINE_CURVE_WITH_KNOTS ( 'NONE', 3,
 ( #28770, #78264, #36839, #70187, #63867, #84605, #56235, #2164, #83720, #49480 ),
 .UNSPECIFIED., .F., .F.,
 ( 4, 2, 2, 2, 4 ),
 ( 0.0007817246256747443535, 0.0009771112852218868158, 0.001172497944769029278, 0.001367884604316171523, 0.001563271263863313986 ),
 .UNSPECIFIED. ) ;
#36180=CARTESIAN_POINT ( 'NONE',  ( -3.903900635498011251, -12.43552623307873972, 30.55307653245132826 ) ) ;
#36182=CARTESIAN_POINT ( 'NONE',  ( 8.703148389870632329, -3.937682226553330445, 33.60647404775217240 ) ) ;
#36185=CARTESIAN_POINT ( 'NONE',  ( 12.21153846153846168, -7.566083408709835645, 34.74999999999999289 ) ) ;
#36187=ORIENTED_EDGE ( 'NONE', *, *, #84194, .F. ) ;
#36188=LINE ( 'NONE', #50117, #74989 ) ;
#36189=CARTESIAN_POINT ( 'NONE',  ( -9.469528023329623068, -11.60474049983371003, 33.02348890104160262 ) ) ;
#36190=ORIENTED_EDGE ( 'NONE', *, *, #48127, .T. ) ;
#36192=ORIENTED_EDGE ( 'NONE', *, *, #81766, .F. ) ;
#36193=ORIENTED_EDGE ( 'NONE', *, *, #46475, .F. ) ;
#36194=CARTESIAN_POINT ( 'NONE',  ( 16.85343813319912698, -5.113361153441931428, 34.14387501736621999 ) ) ;
#36195=ADVANCED_FACE ( 'NONE', ( #65593 ), #52969, .F. ) ;
#36196=CARTESIAN_POINT ( 'NONE',  ( 3.007284287045282944, -10.11188796281391511, 34.01382737946119050 ) ) ;
#36197=AXIS2_PLACEMENT_3D ( 'NONE', #80928, #52096, #32285 ) ;
#36198=CARTESIAN_POINT ( 'NONE',  ( 0.6849648604532480034, -7.630147987733843173, 34.99859428049665411 ) ) ;
#36199=CARTESIAN_POINT ( 'NONE',  ( 10.61538461538492406, -2.506253911140615021, 30.00000000000323297 ) ) ;
#36200=CARTESIAN_POINT ( 'NONE',  ( -16.15384615384627409, -3.300289026999228437, 32.46337939537709616 ) ) ;
#36203=CARTESIAN_POINT ( 'NONE',  ( 0.2115384615384438560, -2.249999999999999112, 29.81609741502488120 ) ) ;
#36204=CARTESIAN_POINT ( 'NONE',  ( 2.980792499826877773, -6.567427716900047230, 34.66269422305636283 ) ) ;
#36205=CARTESIAN_POINT ( 'NONE',  ( 11.53846153846153832, -10.51840700105979565, 33.73612834413961536 ) ) ;
#36206=CARTESIAN_POINT ( 'NONE',  ( 2.307692307692309264, -3.513871655860378418, 32.76840700105978499 ) ) ;
#36207=CARTESIAN_POINT ( 'NONE',  ( -17.07692307692319744, -11.67786785259630911, 32.92929555188603530 ) ) ;
#36208=B_SPLINE_CURVE_WITH_KNOTS ( 'NONE', 3,
 ( #75996, #55720, #67919, #26935, #34574, #88657, #54392, #61592, #33248, #61145 ),
 .UNSPECIFIED., .F., .F.,
 ( 4, 2, 2, 2, 4 ),
 ( 0.000000000000000000, 0.0001954311564186863052, 0.0003908623128373726104, 0.0005862934692560589156, 0.0007817246256747452209 ),
 .UNSPECIFIED. ) ;
#36209=ORIENTED_EDGE ( 'NONE', *, *, #81640, .T. ) ;
#36210=CARTESIAN_POINT ( 'NONE',  ( 15.10007776410167324, -11.18331474514187995, 33.13161551792790505 ) ) ;
#36211=CARTESIAN_POINT ( 'NONE',  ( 11.78851585009985570, -9.943054286541403997, 34.11300777759954883 ) ) ;
#36212=CARTESIAN_POINT ( 'NONE',  ( -2.557692307692305267, -7.433931650972300353, 34.75000000000000711 ) ) ;
#36213=ORIENTED_EDGE ( 'NONE', *, *, #83434, .F. ) ;
#36214=LINE ( 'NONE', #56905, #50690 ) ;
#36215=CARTESIAN_POINT ( 'NONE',  ( -10.74553258511630993, -12.70455904226513866, 30.44083106164009322 ) ) ;
#36216=CARTESIAN_POINT ( 'NONE',  ( -3.164700879766793040, -12.10708131394839704, 31.69288490824020954 ) ) ;
#36217=ORIENTED_EDGE ( 'NONE', *, *, #52722, .F. ) ;
#36218=CARTESIAN_POINT ( 'NONE',  ( 18.22301284409340028, -3.395485233115139501, 33.02377354290276656 ) ) ;
#36219=ORIENTED_EDGE ( 'NONE', *, *, #33414, .T. ) ;
#36220=CARTESIAN_POINT ( 'NONE',  ( 9.915087233576100445, -11.89424750095246175, 32.13594075562310337 ) ) ;
#36221=CARTESIAN_POINT ( 'NONE',  ( 7.146089767170321849, -2.889357225399416862, 32.26129605718031002 ) ) ;
#36222=DIRECTION ( 'NONE',  ( -0.000000000000000000, -0.9396926207859092051, -0.3420201433256662704 ) ) ;
#36224=CARTESIAN_POINT ( 'NONE',  ( -9.692307692307691624, -1.951392089020283160, 34.73218667398347748 ) ) ;
#36225=CYLINDRICAL_SURFACE ( 'NONE', #27792, 0.2500000000000009437 ) ;
#36226=ORIENTED_EDGE ( 'NONE', *, *, #45459, .F. ) ;
#36227=ADVANCED_FACE ( 'NONE', ( #45327 ), #38135, .F. ) ;
#36228=VERTEX_POINT ( 'NONE', #39487 ) ;
#36229=EDGE_LOOP ( 'NONE', ( #75377, #73065, #75994, #70663 ) ) ;
#36230=CARTESIAN_POINT ( 'NONE',  ( -3.361329144382594336, -2.254533558242299396, 29.97296025877828285 ) ) ;
#36231=CARTESIAN_POINT ( 'NONE',  ( 13.45068373561782593, -9.780366693483667717, 34.19971097300155805 ) ) ;
#36232=EDGE_CURVE ( 'NONE', #82664, #8847, #32788, .T. ) ;
#36233=FACE_OUTER_BOUND ( 'NONE', #54835, .T. ) ;
#36234=CARTESIAN_POINT ( 'NONE',  ( 0.3313904918067623884, -12.50552854090298993, 31.33409797877408920 ) ) ;
#36235=AXIS2_PLACEMENT_3D ( 'NONE', #64544, #78964, #86185 ) ;
#36236=CARTESIAN_POINT ( 'NONE',  ( 15.48076923076923173, -2.249999999999998668, 29.75000000000000355 ) ) ;
#36237=CARTESIAN_POINT ( 'NONE',  ( -10.61538461538461320, -9.905515769479276145, 34.41647553114623292 ) ) ;
#36238=VERTEX_POINT ( 'NONE', #31379 ) ;
#36239=ORIENTED_EDGE ( 'NONE', *, *, #78957, .F. ) ;
#36240=VERTEX_POINT ( 'NONE', #4805 ) ;
#36242=CARTESIAN_POINT ( 'NONE',  ( 12.59233026936324684, -8.147973898785416225, 34.70805048591653730 ) ) ;
#36243=VERTEX_POINT ( 'NONE', #60172 ) ;
#36244=DIRECTION ( 'NONE',  ( -0.000000000000000000, 0.8660254037844397068, -0.4999999999999978906 ) ) ;
#36245=CARTESIAN_POINT ( 'NONE',  ( 13.45068271796546178, -3.937682226553329556, 33.60647404775216529 ) ) ;
#36246=B_SPLINE_CURVE_WITH_KNOTS ( 'NONE', 3,
 ( #69273, #27401, #68383, #1248, #48540, #21975, #54872, #76022, #14326, #42694 ),
 .UNSPECIFIED., .F., .F.,
 ( 4, 2, 2, 2, 4 ),
 ( 0.000000000000000000, 0.0001954311564186879586, 0.0003908623128373759172, 0.0005862934692560639030, 0.0007817246256747518345 ),
 .UNSPECIFIED. ) ;
#36248=ORIENTED_EDGE ( 'NONE', *, *, #37888, .F. ) ;
#36249=B_SPLINE_CURVE_WITH_KNOTS ( 'NONE', 3,
 ( #68452, #40991, #13950, #75649, #60810, #81098, #53608, #60364, #27029, #20275 ),
 .UNSPECIFIED., .F., .F.,
 ( 4, 2, 2, 2, 4 ),
 ( 0.0007817246256747453293, 0.0009771112852218889842, 0.001172497944769032531, 0.001367884604316176294, 0.001563271263863319840 ),
 .UNSPECIFIED. ) ;
#36250=EDGE_LOOP ( 'NONE', ( #67201, #73935, #64540, #39998 ) ) ;
#36251=CARTESIAN_POINT ( 'NONE',  ( 4.826923076923077538, -7.566082377512563184, 35.00000000000000711 ) ) ;
#36252=EDGE_CURVE ( 'NONE', #24676, #53273, #64995, .T. ) ;
#36254=FACE_BOUND ( 'NONE', #58215, .T. ) ;
#36255=CARTESIAN_POINT ( 'NONE',  ( -5.776987155906601501, -2.889357225399416862, 32.26129605718031002 ) ) ;
#36256=SHAPE_REPRESENTATION ( 'Ultra-Thin Hypoallergenic Micro-Foil Screen', ( #83448 ), #14453 ) ;
#36258=ORIENTED_EDGE ( 'NONE', *, *, #51487, .T. ) ;
#36259=CARTESIAN_POINT ( 'NONE',  ( -4.219097144007394107, -2.506253911140460477, 30.00000000000013856 ) ) ;
#36260=EDGE_CURVE ( 'NONE', #28816, #54248, #76829, .T. ) ;
#36261=LINE ( 'NONE', #3344, #31759 ) ;
#36262=CARTESIAN_POINT ( 'NONE',  ( 10.39245839786846837, -2.758268499246657068, 31.33685645148948140 ) ) ;
#36263=CARTESIAN_POINT ( 'NONE',  ( -15.23076923076935074, -6.879047030192662504, 34.71129190930017927 ) ) ;
#36264=CARTESIAN_POINT ( 'NONE',  ( -13.31935981333935892, -11.94971097300157403, 32.03036669348361443 ) ) ;
#36266=CARTESIAN_POINT ( 'NONE',  ( -6.923076923077044142, -11.48612834414049644, 32.76840700105863391 ) ) ;
#36267=CARTESIAN_POINT ( 'NONE',  ( -8.069080805060693251, -11.98009711892699514, 32.48740034544076138 ) ) ;
#36269=CARTESIAN_POINT ( 'NONE',  ( 13.63466980452883526, -2.318338780012835443, 30.59689888758630261 ) ) ;
#36270=CARTESIAN_POINT ( 'NONE',  ( 9.692307692307570832, -12.51329471203414379, 31.30864560766407578 ) ) ;
#36271=CARTESIAN_POINT ( 'NONE',  ( -13.16160254052199008, -12.38742843783360748, 31.66772728687926985 ) ) ;
#36272=CARTESIAN_POINT ( 'NONE',  ( 4.946775867484857869, -11.47017969459903952, 32.78971311882034456 ) ) ;
#36273=CARTESIAN_POINT ( 'NONE',  ( 3.230769230769231726, -11.35647404775217417, 33.31231777344666511 ) ) ;
#36274=EDGE_CURVE ( 'NONE', #15372, #34740, #3748, .T. ) ;
#36275=CARTESIAN_POINT ( 'NONE',  ( 8.638670177488846136, -2.504760397472875155, 29.97295953869789997 ) ) ;
#36276=CARTESIAN_POINT ( 'NONE',  ( -11.28851602011339672, -11.37275283266504111, 32.91324779482534524 ) ) ;
#36277=CARTESIAN_POINT ( 'NONE',  ( 2.373759641042384239, -6.343179335718452272, 34.87096338111212646 ) ) ;
#36279=CARTESIAN_POINT ( 'NONE',  ( 13.13461538461538680, -7.500000000000001776, 35.00000000000000000 ) ) ;
#36281=ORIENTED_EDGE ( 'NONE', *, *, #73317, .T. ) ;
#36284=CARTESIAN_POINT ( 'NONE',  ( 9.692307692307695177, -6.386643153685126251, 34.62446782046654192 ) ) ;
#36285=EDGE_LOOP ( 'NONE', ( #29744, #36714, #48683, #26184 ) ) ;
#36286=DIRECTION ( 'NONE',  ( -0.000000000000000000, -0.5000000000000009992, -0.8660254037844380415 ) ) ;
#36287=CARTESIAN_POINT ( 'NONE',  ( 17.14217821643592288, -3.083524468853783951, 32.58852847137153930 ) ) ;
#36288=VERTEX_POINT ( 'NONE', #34483 ) ;
#36289=CARTESIAN_POINT ( 'NONE',  ( 5.934729999443681514, -11.06231777344662781, 33.60647404775220082 ) ) ;
#36291=CARTESIAN_POINT ( 'NONE',  ( 7.846153846153846700, -8.164416787775445883, 34.95778746994557906 ) ) ;
#36292=EDGE_CURVE ( 'NONE', #15704, #46513, #19869, .T. ) ;
#36293=CARTESIAN_POINT ( 'NONE',  ( -5.934744428723972121, -9.442884908240271713, 34.35708131394835618 ) ) ;
#36294=CARTESIAN_POINT ( 'NONE',  ( -5.207070286361298095, -5.195881422630167279, 34.18770438780618548 ) ) ;
#36295=CARTESIAN_POINT ( 'NONE',  ( 14.98074600654777733, -8.475808217655753651, 34.90892951860618609 ) ) ;
#36296=DIRECTION ( 'NONE',  ( 0.000000000000000000, -1.000000000000000000, -8.673617379884033500E-16 ) ) ;
#36297=CARTESIAN_POINT ( 'NONE',  ( 0.4615384615384611200, -1.422936976036506707, 30.56769352161908415 ) ) ;
#36299=EDGE_CURVE ( 'NONE', #75150, #65922, #35995, .T. ) ;
#36300=EDGE_CURVE ( 'NONE', #58446, #67262, #74590, .T. ) ;
#36301=CARTESIAN_POINT ( 'NONE',  ( 11.31553457955468645, -5.582147617184174848, 34.63737895849758530 ) ) ;
#36302=CARTESIAN_POINT ( 'NONE',  ( 14.55774661933062575, -10.66356715214248752, 33.62249196103329751 ) ) ;
#36303=ADVANCED_FACE ( 'NONE', ( #81795 ), #47548, .F. ) ;
#36304=CARTESIAN_POINT ( 'NONE',  ( 14.53047184896071542, -3.236590943229499029, 32.36255958852954251 ) ) ;
#36306=EDGE_CURVE ( 'NONE', #58277, #18801, #66051, .T. ) ;
#36307=AXIS2_PLACEMENT_3D ( 'NONE', #5249, #67395, #32716 ) ;
#36309=VECTOR ( 'NONE', #30552, 1000.000000000000000 ) ;
#36311=CARTESIAN_POINT ( 'NONE',  ( 14.53070365930516061, -2.554770724473668153, 30.48948780036025852 ) ) ;
#36312=CARTESIAN_POINT ( 'NONE',  ( 11.78851585009985214, -5.728107161865378494, 34.42597550085002922 ) ) ;
#36313=CARTESIAN_POINT ( 'NONE',  ( 17.07692307692307665, -13.49023893513002648, 31.06009739812518688 ) ) ;
#36314=CARTESIAN_POINT ( 'NONE',  ( 18.13079180782478872, -10.54018710029568595, 33.71981072465678864 ) ) ;
#36315=CARTESIAN_POINT ( 'NONE',  ( -16.28399336328437386, -10.88202310037936194, 33.43294751532457099 ) ) ;
#36316=AXIS2_PLACEMENT_3D ( 'NONE', #75086, #75517, #13371 ) ;
#36317=CARTESIAN_POINT ( 'NONE',  ( -14.05774689831426372, -4.176053281294518804, 33.81426240980091791 ) ) ;
#36318=DIRECTION ( 'NONE',  ( -0.000000000000000000, 0.7660444431189791237, -0.6427876096865379196 ) ) ;
#36319=ORIENTED_EDGE ( 'NONE', *, *, #58703, .T. ) ;
#36320=EDGE_LOOP ( 'NONE', ( #24467, #22954, #37746, #66278 ) ) ;
#36321=ORIENTED_EDGE ( 'NONE', *, *, #62117, .F. ) ;
#36322=CARTESIAN_POINT ( 'NONE',  ( -1.384615384615383471, -1.117168528481311540, 33.14645433367849847 ) ) ;
#36324=CARTESIAN_POINT ( 'NONE',  ( 4.153846153846030731, -2.657715359629662988, 31.77849191805970364 ) ) ;
#36325=B_SPLINE_CURVE_WITH_KNOTS ( 'NONE', 3,
 ( #82854, #77410, #43183, #21131, #48602, #76078, #58449, #85944, #85499, #71528 ),
 .UNSPECIFIED., .F., .F.,
 ( 4, 2, 2, 2, 4 ),
 ( 0.000000000000000000, 0.0001954311564186868202, 0.0003908623128373736404, 0.0005862934692560604335, 0.0007817246256747472808 ),
 .UNSPECIFIED. ) ;
#36326=CARTESIAN_POINT ( 'NONE',  ( 4.153846153846154188, -3.513871655860378418, 32.76840700105978499 ) ) ;
#36327=CARTESIAN_POINT ( 'NONE',  ( 18.00000000000000000, -8.973038597847269315, 34.52809138561121927 ) ) ;
#36328=VERTEX_POINT ( 'NONE', #41687 ) ;
#36329=LINE ( 'NONE', #63785, #75140 ) ;
#36330=EDGE_LOOP ( 'NONE', ( #32900, #17621, #23086, #2655 ) ) ;
#36332=CARTESIAN_POINT ( 'NONE',  ( 8.639082799499071541, -12.50552854090298638, 31.33409797877408920 ) ) ;
#36333=VERTEX_POINT ( 'NONE', #53867 ) ;
#36334=LINE ( 'NONE', #70109, #47406 ) ;
#36335=CARTESIAN_POINT ( 'NONE',  ( 1.384615384615265343, -10.21337939537710326, 33.94971097300076224 ) ) ;
#36336=CARTESIAN_POINT ( 'NONE',  ( -18.00000000000000000, -10.51840700105979387, 33.73612834413961536 ) ) ;
#36337=DIRECTION ( 'NONE',  ( -0.000000000000000000, -0.7660444431189791237, -0.6427876096865379196 ) ) ;
#36338=EDGE_LOOP ( 'NONE', ( #9841, #57388 ) ) ;
#36339=ORIENTED_EDGE ( 'NONE', *, *, #8932, .T. ) ;
#36341=ORIENTED_EDGE ( 'NONE', *, *, #46319, .T. ) ;
#36343=CARTESIAN_POINT ( 'NONE',  ( 1.254468175177165357, -8.587444163452046197, 34.63053765926554206 ) ) ;
#36344=EDGE_LOOP ( 'NONE', ( #64786, #6082 ) ) ;
#36346=CARTESIAN_POINT ( 'NONE',  ( 5.011652630962299959, -3.835265460703609186, 33.15142922261924241 ) ) ;
#36347=LINE ( 'NONE', #64236, #76703 ) ;
#36348=ORIENTED_EDGE ( 'NONE', *, *, #14299, .T. ) ;
#36349=CYLINDRICAL_SURFACE ( 'NONE', #88279, 0.2499999999999997502 ) ;
#36350=CARTESIAN_POINT ( 'NONE',  ( 4.826923076923055334, -2.249999999999999112, 29.81609741502488120 ) ) ;
#36351=ORIENTED_EDGE ( 'NONE', *, *, #65458, .T. ) ;
#36352=FACE_BOUND ( 'NONE', #72583, .T. ) ;
#36353=B_SPLINE_CURVE_WITH_KNOTS ( 'NONE', 3,
 ( #51897, #79396, #86162, #87063, #17698, #66319, #11376, #32094, #10935, #12263 ),
 .UNSPECIFIED., .F., .F.,
 ( 4, 2, 2, 2, 4 ),
 ( 0.000000000000000000, 0.0001954339857564073388, 0.0003908679715128146777, 0.0005863019572692220165, 0.0007817359430256293554 ),
 .UNSPECIFIED. ) ;
#36354=CARTESIAN_POINT ( 'NONE',  ( -11.66915214157184444, -11.37499894934982692, 33.29245874905763003 ) ) ;
#36355=CARTESIAN_POINT ( 'NONE',  ( -6.988347369037698265, -2.892918686051582089, 31.69288490824015270 ) ) ;
#36356=VECTOR ( 'NONE', #50657, 1000.000000000000000 ) ;
#36357=EDGE_CURVE ( 'NONE', #84497, #17395, #27471, .T. ) ;
#36359=DIRECTION ( 'NONE',  ( -0.000000000000000000, 0.7660444431189791237, -0.6427876096865379196 ) ) ;
#36360=CARTESIAN_POINT ( 'NONE',  ( 15.23076923076954614, -2.255955759149395501, 30.00000000000324363 ) ) ;
#36361=CARTESIAN_POINT ( 'NONE',  ( 4.826946345980720032, -2.564618984488975961, 30.55390908950641915 ) ) ;
#36362=CARTESIAN_POINT ( 'NONE',  ( 14.43848274865925774, -2.295524264805589354, 30.44142389570982488 ) ) ;
#36363=ORIENTED_EDGE ( 'NONE', *, *, #13533, .F. ) ;
#36364=DIRECTION ( 'NONE',  ( 0.000000000000000000, 0.3420201433256610524, 0.9396926207859113145 ) ) ;
#36365=DIRECTION ( 'NONE',  ( -0.000000000000000000, -0.8660254037844399289, -0.4999999999999980016 ) ) ;
#36366=ORIENTED_EDGE ( 'NONE', *, *, #210, .T. ) ;
#36367=VECTOR ( 'NONE', #13165, 1000.000000000000114 ) ;
#36368=CARTESIAN_POINT ( 'NONE',  ( 11.31497661389721010, -12.11044203135681840, 32.26167407432752299 ) ) ;
#36369=CARTESIAN_POINT ( 'NONE',  ( -4.946397375159516052, -6.001044277235011215, 34.52024696741798948 ) ) ;
#36370=CARTESIAN_POINT ( 'NONE',  ( -4.153846153846273204, -2.625532179533778709, 30.86335684631627174 ) ) ;
#36371=CARTESIAN_POINT ( 'NONE',  ( 2.084765348785459604, -5.582147617184174848, 34.63737895849758530 ) ) ;
#36372=CARTESIAN_POINT ( 'NONE',  ( 16.15384615384615330, -1.790695186598648903, 34.54067556320373455 ) ) ;
#36374=FACE_BOUND ( 'NONE', #1468, .T. ) ;
#36375=CARTESIAN_POINT ( 'NONE',  ( 6.673100179028332413, -4.075325502946086864, 33.72974371597207721 ) ) ;
#36376=CARTESIAN_POINT ( 'NONE',  ( 13.38461538461538680, -2.708943851104267164, 35.45975837776705220 ) ) ;
#36377=ADVANCED_FACE ( 'NONE', ( #83122 ), #21413, .T. ) ;
#36378=CARTESIAN_POINT ( 'NONE',  ( 12.39626846098214408, -12.51329471203370325, 31.30864560766548976 ) ) ;
#36379=CARTESIAN_POINT ( 'NONE',  ( -2.980714919130917462, -11.79725096376909654, 32.30694842903960762 ) ) ;
#36380=CARTESIAN_POINT ( 'NONE',  ( 7.053868730901709405, -12.38066358083363738, 30.83685684665853444 ) ) ;
#36381=FACE_OUTER_BOUND ( 'NONE', #24116, .T. ) ;
#36384=ORIENTED_EDGE ( 'NONE', *, *, #87121, .T. ) ;
#36385=LINE ( 'NONE', #69285, #85262 ) ;
#36387=CARTESIAN_POINT ( 'NONE',  ( -7.780086512803769949, -11.35647404775217595, 33.31231777344667222 ) ) ;
#36388=CARTESIAN_POINT ( 'NONE',  ( -0.5276208408985973985, -2.833524468853757305, 32.15551576947924417 ) ) ;
#36389=CARTESIAN_POINT ( 'NONE',  ( -7.846153846153967493, -12.70778746994576025, 30.41441678777401236 ) ) ;
#36391=B_SPLINE_CURVE_WITH_KNOTS ( 'NONE', 3,
 ( #33699, #48084, #4903, #40902, #33259, #32367, #5340, #47201, #61155, #59831 ),
 .UNSPECIFIED., .F., .F.,
 ( 4, 2, 2, 2, 4 ),
 ( 0.000000000000000000, 0.0001954339857564080707, 0.0003908679715128161414, 0.0005863019572692241849, 0.0007817359430256322827 ),
 .UNSPECIFIED. ) ;
#36392=FACE_OUTER_BOUND ( 'NONE', #43196, .T. ) ;
#36394=VECTOR ( 'NONE', #42956, 1000.000000000000227 ) ;
#36395=CARTESIAN_POINT ( 'NONE',  ( -17.32694631421604115, -5.056417327199097755, 34.11270091957320716 ) ) ;
#36396=FACE_OUTER_BOUND ( 'NONE', #29964, .T. ) ;
#36397=CARTESIAN_POINT ( 'NONE',  ( 15.23076923076923173, -13.04860791097971706, 34.73218667398347037 ) ) ;
#36398=FACE_OUTER_BOUND ( 'NONE', #41710, .T. ) ;
#36399=VECTOR ( 'NONE', #32963, 1000.000000000000227 ) ;
#36400=B_SPLINE_CURVE_WITH_KNOTS ( 'NONE', 3,
 ( #67874, #33647, #2944, #85380, #57895, #84944, #16915, #37627, #50239, #28666 ),
 .UNSPECIFIED., .F., .F.,
 ( 4, 2, 2, 2, 4 ),
 ( 0.000000000000000000, 0.0001954311564186866305, 0.0003908623128373732609, 0.0005862934692560598914, 0.0007817246256747465219 ),
 .UNSPECIFIED. ) ;
#36401=EDGE_CURVE ( 'NONE', #5654, #76326, #5944, .T. ) ;
#36402=EDGE_CURVE ( 'NONE', #2497, #82763, #29075, .T. ) ;
#36403=LINE ( 'NONE', #35063, #63488 ) ;
#36404=CARTESIAN_POINT ( 'NONE',  ( -2.307692307692427391, -8.613356846316285953, 34.62446782046622218 ) ) ;
#36405=EDGE_LOOP ( 'NONE', ( #10681, #29235 ) ) ;
#36406=CARTESIAN_POINT ( 'NONE',  ( 4.023698944407932743, -5.195881422630167279, 34.18770438780618548 ) ) ;
#36407=CARTESIAN_POINT ( 'NONE',  ( -6.923076923076922462, -13.87047571288749737, 32.06866353760679544 ) ) ;
#36409=EDGE_CURVE ( 'NONE', #28375, #67914, #7049, .T. ) ;
#36410=CARTESIAN_POINT ( 'NONE',  ( 6.699591998512592461, -4.988325925672468131, 34.36044203135681130 ) ) ;
#36411=DIRECTION ( 'NONE',  ( -0.000000000000000000, 0.8660254037844397068, -0.4999999999999978906 ) ) ;
#36412=VERTEX_POINT ( 'NONE', #42579 ) ;
#36413=CARTESIAN_POINT ( 'NONE',  ( -16.40384615384615330, -2.499999999999998668, 29.75000000000000355 ) ) ;
#36414=CARTESIAN_POINT ( 'NONE',  ( 7.716006636715625255, -2.619462340734462380, 30.83744416345203021 ) ) ;
#36415=ORIENTED_EDGE ( 'NONE', *, *, #54687, .T. ) ;
#36416=LINE ( 'NONE', #16136, #19693 ) ;
#36417=CARTESIAN_POINT ( 'NONE',  ( -13.25382357679059986, -9.804649428959608670, 34.18742332936588468 ) ) ;
#36418=EDGE_CURVE ( 'NONE', #77986, #33107, #23149, .T. ) ;
#36419=ORIENTED_EDGE ( 'NONE', *, *, #20299, .T. ) ;
#36420=CARTESIAN_POINT ( 'NONE',  ( -5.076923076923075762, -12.10708131394839349, 31.69288490824020244 ) ) ;
#36421=CARTESIAN_POINT ( 'NONE',  ( 8.834486340506792601, -5.219633306516380244, 34.19971097300157936 ) ) ;
#36422=ORIENTED_EDGE ( 'NONE', *, *, #6543, .F. ) ;
#36423=CARTESIAN_POINT ( 'NONE',  ( -12.68502338610279523, -2.353723527008296568, 30.78948104536958752 ) ) ;
#36424=CARTESIAN_POINT ( 'NONE',  ( -16.15384615384615330, -3.050289026998446396, 32.03036669348365706 ) ) ;
#36425=FACE_OUTER_BOUND ( 'NONE', #74205, .T. ) ;
#36426=ORIENTED_EDGE ( 'NONE', *, *, #27219, .T. ) ;
#36428=VECTOR ( 'NONE', #33497, 1000.000000000000227 ) ;
#36429=ORIENTED_EDGE ( 'NONE', *, *, #80149, .T. ) ;
#36430=VECTOR ( 'NONE', #15180, 1000.000000000000227 ) ;
#36431=CARTESIAN_POINT ( 'NONE',  ( 5.207448515156719360, -5.070358843744210198, 34.40418822224088302 ) ) ;
#36432=CARTESIAN_POINT ( 'NONE',  ( 13.60762822870878530, -3.395485233115139057, 33.02377354290275946 ) ) ;
#36436=EDGE_LOOP ( 'NONE', ( #20588, #14486, #71830, #41819 ) ) ;
#36437=ORIENTED_EDGE ( 'NONE', *, *, #32242, .F. ) ;
#36438=FACE_OUTER_BOUND ( 'NONE', #27410, .T. ) ;
#36439=VERTEX_POINT ( 'NONE', #2025 ) ;
#36440=CARTESIAN_POINT ( 'NONE',  ( 12.71148387091650278, -11.56426240980093745, 33.07394671870546432 ) ) ;
#36441=ORIENTED_EDGE ( 'NONE', *, *, #61024, .F. ) ;
#36442=CARTESIAN_POINT ( 'NONE',  ( 15.48076923076923173, -2.249999999999998668, 29.75000000000000355 ) ) ;
#36444=EDGE_LOOP ( 'NONE', ( #2473, #65289 ) ) ;
#36446=B_SPLINE_CURVE_WITH_KNOTS ( 'NONE', 3,
 ( #18376, #73319, #85945, #44939, #24226, #72417, #11169, #71529, #3067, #45836 ),
 .UNSPECIFIED., .F., .F.,
 ( 4, 2, 2, 2, 4 ),
 ( 0.0007817246256747446788, 0.0009771112852218872494, 0.001172497944769029929, 0.001367884604316172391, 0.001563271263863315070 ),
 .UNSPECIFIED. ) ;
#36448=ORIENTED_EDGE ( 'NONE', *, *, #59694, .F. ) ;
#36449=CARTESIAN_POINT ( 'NONE',  ( -12.23852710992561299, -4.887748414852792322, 34.01359900205216746 ) ) ;
#36450=VERTEX_POINT ( 'NONE', #1141 ) ;
#36451=VECTOR ( 'NONE', #87532, 1000.000000000000114 ) ;
#36452=CARTESIAN_POINT ( 'NONE',  ( 4.376625695114563008, -5.114059244376869984, 34.14424750095245287 ) ) ;
#36453=CARTESIAN_POINT ( 'NONE',  ( -5.326899807865430603, -9.943427161483782584, 34.11278801902876978 ) ) ;
#36455=CARTESIAN_POINT ( 'NONE',  ( -6.673131513698878692, -4.932303261841489039, 34.32971442181322885 ) ) ;
#36457=CARTESIAN_POINT ( 'NONE',  ( 16.15384615384603251, -12.27809138561165270, 31.22303859784587132 ) ) ;
#36458=FACE_BOUND ( 'NONE', #46954, .T. ) ;
#36459=CARTESIAN_POINT ( 'NONE',  ( 1.515407192440172413, -12.38066358083363738, 30.83685684665853444 ) ) ;
#36460=CARTESIAN_POINT ( 'NONE',  ( -11.53846153846153655, -6.343179335718451384, 34.87096338111211935 ) ) ;
#36461=EDGE_CURVE ( 'NONE', #3816, #41163, #43477, .T. ) ;
#36462=DIRECTION ( 'NONE',  ( -0.000000000000000000, -0.000000000000000000, -1.000000000000000000 ) ) ;
#36463=FACE_OUTER_BOUND ( 'NONE', #22471, .T. ) ;
#36465=CARTESIAN_POINT ( 'NONE',  ( 11.31497659473759043, -11.41268669641499756, 32.86336882939238535 ) ) ;
#36466=CARTESIAN_POINT ( 'NONE',  ( 10.55011461482829560, -11.06231777344662781, 33.60647404775220082 ) ) ;
#36467=ORIENTED_EDGE ( 'NONE', *, *, #85408, .F. ) ;
#36468=CARTESIAN_POINT ( 'NONE',  ( 14.17708194806778010, -7.722926236386453702, 34.74524107206102030 ) ) ;
#36469=ADVANCED_FACE ( 'NONE', ( #71361 ), #2896, .F. ) ;
#36470=ORIENTED_EDGE ( 'NONE', *, *, #42893, .F. ) ;
#36471=ORIENTED_EDGE ( 'NONE', *, *, #41224, .T. ) ;
#36472=CARTESIAN_POINT ( 'NONE',  ( -1.318548051265308052, -4.661471528628508665, 34.16647553114624003 ) ) ;
#36473=CARTESIAN_POINT ( 'NONE',  ( 16.28463796167094557, -12.11778462344220841, 31.66786338562085135 ) ) ;
#36474=CARTESIAN_POINT ( 'NONE',  ( -6.000000000000119904, -6.879047030192662504, 34.71129190930017927 ) ) ;
#36475=DIRECTION ( 'NONE',  ( 0.000000000000000000, 0.3420201433256610524, 0.9396926207859113145 ) ) ;
#36476=CARTESIAN_POINT ( 'NONE',  ( 15.23076923076923173, -1.790695186598648903, 34.54067556320373455 ) ) ;
#36477=CARTESIAN_POINT ( 'NONE',  ( -2.557715531913763662, -11.56360843649121861, 33.07473185843129926 ) ) ;
#36478=EDGE_LOOP ( 'NONE', ( #27639, #24524 ) ) ;
#36479=DIRECTION ( 'NONE',  ( -0.000000000000000000, 0.3420201433256694346, -0.9396926207859080948 ) ) ;
#36481=CARTESIAN_POINT ( 'NONE',  ( -15.09997742294444478, -9.804649428959608670, 34.18742332936588468 ) ) ;
#36483=EDGE_CURVE ( 'NONE', #57772, #55252, #7903, .T. ) ;
#36484=CARTESIAN_POINT ( 'NONE',  ( 15.36155967173618286, -12.35292014791297710, 31.75344720912887198 ) ) ;
#36485=DIRECTION ( 'NONE',  ( 0.000000000000000000, 0.3420201433256641055, -0.9396926207859100932 ) ) ;
#36486=B_SPLINE_CURVE_WITH_KNOTS ( 'NONE', 3,
 ( #3437, #44407, #58825, #45309, #32260, #78658, #59722, #24151, #52511, #87217 ),
 .UNSPECIFIED., .F., .F.,
 ( 4, 2, 2, 2, 4 ),
 ( 0.000000000000000000, 0.0001954311564186882568, 0.0003908623128373765136, 0.0005862934692560647703, 0.0007817246256747530271 ),
 .UNSPECIFIED. ) ;
#36489=AXIS2_PLACEMENT_3D ( 'NONE', #35755, #69968, #57338 ) ;
#36490=ORIENTED_EDGE ( 'NONE', *, *, #59124, .F. ) ;
#36491=EDGE_CURVE ( 'NONE', #79975, #55599, #49332, .T. ) ;
#36492=B_SPLINE_CURVE_WITH_KNOTS ( 'NONE', 3,
 ( #79608, #64739, #3041, #9377, #36836, #84603, #31415, #58882, #58424, #57549 ),
 .UNSPECIFIED., .F., .F.,
 ( 4, 2, 2, 2, 4 ),
 ( 0.0007817359430256282712, 0.0009771253907249945886, 0.001172514838424360689, 0.001367904286123726790, 0.001563293733823093107 ),
 .UNSPECIFIED. ) ;
#36493=CARTESIAN_POINT ( 'NONE',  ( -7.596208436775802930, -12.07971442181322352, 32.31769673815850297 ) ) ;
#36496=CARTESIAN_POINT ( 'NONE',  ( -12.23852710992561299, -9.886259254753566594, 34.14407573483972413 ) ) ;
#36498=CARTESIAN_POINT ( 'NONE',  ( -0.5922290646487684551, -11.93127051446800024, 32.56575433478200665 ) ) ;
#36500=CARTESIAN_POINT ( 'NONE',  ( 8.545745825506822158, -6.760086850603066466, 34.69517049084099369 ) ) ;
#36501=VERTEX_POINT ( 'NONE', #72257 ) ;
#36502=CARTESIAN_POINT ( 'NONE',  ( -12.59222992820602194, -10.54014554554150607, 33.71984207302941883 ) ) ;
#36503=CARTESIAN_POINT ( 'NONE',  ( -2.084680956079457470, -10.61302985866383963, 33.66295027996417843 ) ) ;
#36504=VERTEX_POINT ( 'NONE', #11456 ) ;
#36505=CARTESIAN_POINT ( 'NONE',  ( -12.46153846153814726, -2.255955759149395501, 30.00000000000324363 ) ) ;
#36506=CARTESIAN_POINT ( 'NONE',  ( -17.07692307692307665, -11.91647553114624181, 32.58852847137148245 ) ) ;
#36507=CARTESIAN_POINT ( 'NONE',  ( -17.77698864838715309, -11.76359900205217635, 32.36225158514719169 ) ) ;
#36509=EDGE_CURVE ( 'NONE', #87198, #2477, #62858, .T. ) ;
#36510=DIRECTION ( 'NONE',  ( -0.000000000000000000, 0.3420201433256694346, -0.9396926207859080948 ) ) ;
#36511=CARTESIAN_POINT ( 'NONE',  ( -11.31544869436814338, -2.889357225399414197, 32.26129605718031002 ) ) ;
#36512=EDGE_CURVE ( 'NONE', #40093, #26721, #67098, .T. ) ;
#36514=ORIENTED_EDGE ( 'NONE', *, *, #52049, .F. ) ;
#36515=CARTESIAN_POINT ( 'NONE',  ( 13.63461538461682210, -7.500000000000155431, 34.75000000000007105 ) ) ;
#36516=B_SPLINE_CURVE_WITH_KNOTS ( 'NONE', 3,
 ( #22119, #69863, #21674, #71957, #82941, #21225, #69421, #48693, #49142, #49590 ),
 .UNSPECIFIED., .F., .F.,
 ( 4, 2, 2, 2, 4 ),
 ( 0.000000000000000000, 0.0001954311564186878502, 0.0003908623128373757004, 0.0005862934692560635777, 0.0007817246256747514008 ),
 .UNSPECIFIED. ) ;
#36517=CARTESIAN_POINT ( 'NONE',  ( -1.450698795571264021, -12.10708131394839349, 31.69288490824020244 ) ) ;
#36519=EDGE_CURVE ( 'NONE', #21173, #35421, #6955, .T. ) ;
#36520=CARTESIAN_POINT ( 'NONE',  ( -13.38461538461550582, -12.46129190930018460, 30.37095296980731973 ) ) ;
#36521=CARTESIAN_POINT ( 'NONE',  ( 9.442284468086239002, -6.652501968072648708, 34.93155406624980941 ) ) ;
#36522=EDGE_CURVE ( 'NONE', #84175, #43394, #10137, .T. ) ;
#36523=ORIENTED_EDGE ( 'NONE', *, *, #59287, .T. ) ;
#36525=CARTESIAN_POINT ( 'NONE',  ( 11.40777093535123043, -3.957541250942358424, 33.62499894934981626 ) ) ;
#36527=CARTESIAN_POINT ( 'NONE',  ( -17.07692307692307665, -8.564572088678739092, 35.78748833219616898 ) ) ;
#36529=ORIENTED_EDGE ( 'NONE', *, *, #37861, .T. ) ;
#36530=CARTESIAN_POINT ( 'NONE',  ( 6.923076923076800782, -4.320704448113951379, 33.92786785259630022 ) ) ;
#36531=CARTESIAN_POINT ( 'NONE',  ( -17.32689982097166492, -2.318417181685854978, 30.59732222474233865 ) ) ;
#36532=CARTESIAN_POINT ( 'NONE',  ( 8.069165197766697162, -5.667800583137507786, 34.40243808032445827 ) ) ;
#36533=CARTESIAN_POINT ( 'NONE',  ( -12.21159305216042057, -10.92531984108285670, 33.72920026020278073 ) ) ;
#36537=CARTESIAN_POINT ( 'NONE',  ( 2.372886289475665489, -2.506253911140448043, 29.99999999999988631 ) ) ;
#36538=CARTESIAN_POINT ( 'NONE',  ( 4.853996118016226546, -5.582147617184174848, 34.63737895849758530 ) ) ;
#36539=EDGE_LOOP ( 'NONE', ( #88034, #69213, #41738, #73687 ) ) ;
#36540=CARTESIAN_POINT ( 'NONE',  ( 11.78840694783958476, -12.68172785388650681, 30.59649109432439218 ) ) ;
#36541=CARTESIAN_POINT ( 'NONE',  ( -14.30769230769242739, -10.90142922262034020, 33.41473453929536674 ) ) ;
#36543=CARTESIAN_POINT ( 'NONE',  ( 1.134638640566794976, -6.524016743844655686, 34.90889640711025521 ) ) ;
#36544=CARTESIAN_POINT ( 'NONE',  ( -18.00000000000012079, -4.481592998941359873, 33.73612834414048933 ) ) ;
#36545=ADVANCED_FACE ( 'NONE', ( #24961 ), #87583, .F. ) ;
#36546=AXIS2_PLACEMENT_3D ( 'NONE', #17393, #11529, #86314 ) ;
#36547=ORIENTED_EDGE ( 'NONE', *, *, #69144, .F. ) ;
#36549=FACE_BOUND ( 'NONE', #79951, .T. ) ;
#36550=VERTEX_POINT ( 'NONE', #58296 ) ;
#36551=LINE ( 'NONE', #64001, #38684 ) ;
#36553=CARTESIAN_POINT ( 'NONE',  ( 9.442330961365341224, -12.17611988154120972, 31.52148481390971213 ) ) ;
#36554=CARTESIAN_POINT ( 'NONE',  ( 0.7115928814519131285, -12.65882529074907126, 30.72640787790839312 ) ) ;
#36555=EDGE_CURVE ( 'NONE', #74216, #41990, #5144, .T. ) ;
#36556=ORIENTED_EDGE ( 'NONE', *, *, #34268, .F. ) ;
#36557=ADVANCED_FACE ( 'NONE', ( #73621 ), #86242, .F. ) ;
#36558=VERTEX_POINT ( 'NONE', #60077 ) ;
#36559=CARTESIAN_POINT ( 'NONE',  ( -14.30769230769230660, -3.669653830205710676, 35.88435417666054406 ) ) ;
#36560=ORIENTED_EDGE ( 'NONE', *, *, #62043, .T. ) ;
#36561=CARTESIAN_POINT ( 'NONE',  ( 16.15384615384615330, -9.780366693483667717, 34.19971097300155094 ) ) ;
#36562=CARTESIAN_POINT ( 'NONE',  ( 13.16168916709924019, -2.758268499246657068, 31.33685645148948140 ) ) ;
#36563=CARTESIAN_POINT ( 'NONE',  ( 16.85343815235874487, -3.562934362175799841, 33.22335522853832401 ) ) ;
#36564=CARTESIAN_POINT ( 'NONE',  ( 13.63456079399342791, -11.56426240980093745, 33.07394671870546432 ) ) ;
#36566=CARTESIAN_POINT ( 'NONE',  ( -5.142193522883852452, -10.90142922261923886, 33.41473453929638993 ) ) ;
#36567=EDGE_CURVE ( 'NONE', #59816, #85420, #53319, .T. ) ;
#36568=CYLINDRICAL_SURFACE ( 'NONE', #10054, 0.2500000000000004996 ) ;
#36569=CARTESIAN_POINT ( 'NONE',  ( -18.06870381900347766, -7.749925094837281314, 34.99404781541490905 ) ) ;
#36570=DIRECTION ( 'NONE',  ( -0.000000000000000000, -0.5000000000000009992, -0.8660254037844380415 ) ) ;
#36571=ORIENTED_EDGE ( 'NONE', *, *, #49753, .F. ) ;
#36572=UNCERTAINTY_MEASURE_WITH_UNIT (LENGTH_MEASURE( 1.000000000000000082E-05 ), #18432, 'distance_accuracy_value', 'NONE');
#36573=ADVANCED_FACE ( 'NONE', ( #45679 ), #85787, .F. ) ;
#36575=EDGE_LOOP ( 'NONE', ( #37441, #17211, #88433, #38053 ) ) ;
#36577=CARTESIAN_POINT ( 'NONE',  ( 3.230769230769231726, -8.120952969808772792, 34.71129190930000163 ) ) ;
#36578=LINE ( 'NONE', #69914, #66429 ) ;
#36579=CARTESIAN_POINT ( 'NONE',  ( -1.384615384615383471, -1.790695186598648903, 34.54067556320373455 ) ) ;
#36580=CARTESIAN_POINT ( 'NONE',  ( -3.480792468062195333, -11.37209801155882971, 32.91403422569032955 ) ) ;
#36581=FACE_BOUND ( 'NONE', #2710, .T. ) ;
#36582=CARTESIAN_POINT ( 'NONE',  ( -2.307692307692427391, -10.21337939537710326, 33.94971097300076224 ) ) ;
#36583=ORIENTED_EDGE ( 'NONE', *, *, #4798, .F. ) ;
#36584=DIRECTION ( 'NONE',  ( -0.000000000000000000, 0.9396926207859092051, -0.3420201433256662704 ) ) ;
#36585=CARTESIAN_POINT ( 'NONE',  ( -14.30769230769230660, -1.951392089020283160, 34.73218667398347748 ) ) ;
#36586=DIRECTION ( 'NONE',  ( 0.000000000000000000, 0.9396926207859126468, 0.3420201433256571111 ) ) ;
#36588=CARTESIAN_POINT ( 'NONE',  ( 7.145856592054988354, -9.418065098278011860, 34.63729479722530158 ) ) ;
#36589=ORIENTED_EDGE ( 'NONE', *, *, #53568, .T. ) ;
#36590=CARTESIAN_POINT ( 'NONE',  ( 2.438484115517095319, -11.71459661697925903, 32.44059661609676937 ) ) ;
#36592=FACE_BOUND ( 'NONE', #76103, .T. ) ;
#36594=CARTESIAN_POINT ( 'NONE',  ( -6.988346923633242724, -10.33852847137145048, 34.16647553114627556 ) ) ;
#36595=CARTESIAN_POINT ( 'NONE',  ( 14.17754509825409137, -11.93770438780619259, 32.05411857736982029 ) ) ;
#36596=EDGE_LOOP ( 'NONE', ( #10939, #35328 ) ) ;
#36597=CARTESIAN_POINT ( 'NONE',  ( 5.142178648199100088, -3.300289026998475705, 32.46337939537591666 ) ) ;
#36598=CARTESIAN_POINT ( 'NONE',  ( -17.93474486048716088, -4.320704448112861584, 33.92786785259548310 ) ) ;
#36599=CARTESIAN_POINT ( 'NONE',  ( -9.692307692307812417, -3.300289026999228881, 32.46337939537708905 ) ) ;
#36600=CARTESIAN_POINT ( 'NONE',  ( 4.403900573759605308, -6.523592122091591783, 34.90882529074906415 ) ) ;
#36603=ORIENTED_EDGE ( 'NONE', *, *, #5308, .F. ) ;
#36605=ORIENTED_EDGE ( 'NONE', *, *, #28027, .T. ) ;
#36606=CARTESIAN_POINT ( 'NONE',  ( 3.453780582382079967, -2.554770724473667709, 30.48948780036025852 ) ) ;
#36607=CARTESIAN_POINT ( 'NONE',  ( -1.384615384615383471, -12.34228464037088635, 31.77849191805839268 ) ) ;
#36608=CARTESIAN_POINT ( 'NONE',  ( -5.999999999999998224, -8.120952969808772792, 34.71129190930000163 ) ) ;
#36609=CARTESIAN_POINT ( 'NONE',  ( -12.46153846153858247, -2.892918686052166066, 31.69288490824153470 ) ) ;
#36610=CARTESIAN_POINT ( 'NONE',  ( -7.912237257109724808, -8.973038597847271092, 34.52809138561120506 ) ) ;
#36614=DIRECTION ( 'NONE',  ( -0.000000000000000000, -0.000000000000000000, -1.000000000000000000 ) ) ;
#36616=ORIENTED_EDGE ( 'NONE', *, *, #7447, .T. ) ;
#36618=CARTESIAN_POINT ( 'NONE',  ( -16.15384615384615330, -3.886160181151819604, 36.00935417666054406 ) ) ;
#36620=ORIENTED_EDGE ( 'NONE', *, *, #55821, .F. ) ;
#36621=EDGE_CURVE ( 'NONE', #14768, #60046, #26352, .T. ) ;
#36622=ORIENTED_EDGE ( 'NONE', *, *, #40936, .F. ) ;
#36623=ADVANCED_FACE ( 'NONE', ( #28075 ), #74055, .F. ) ;
#36624=VERTEX_POINT ( 'NONE', #75378 ) ;
#36625=CARTESIAN_POINT ( 'NONE',  ( -15.23076923076922995, -10.05456864172156806, 36.03766855953608683 ) ) ;
#36626=B_SPLINE_CURVE_WITH_KNOTS ( 'NONE', 3,
 ( #62432, #7065, #749, #75519, #28214, #61554, #47604, #27338, #5733, #74644 ),
 .UNSPECIFIED., .F., .F.,
 ( 4, 2, 2, 2, 4 ),
 ( 0.000000000000000000, 0.0001954339857564075828, 0.0003908679715128151656, 0.0005863019572692227755, 0.0007817359430256303312 ),
 .UNSPECIFIED. ) ;
#36627=CARTESIAN_POINT ( 'NONE',  ( -4.826868657009622865, -12.65882529074907126, 30.72640787790839312 ) ) ;
#36628=CARTESIAN_POINT ( 'NONE',  ( 0.2386589448008749614, -7.630690623152302621, 34.99857592706774057 ) ) ;
#36629=CARTESIAN_POINT ( 'NONE',  ( 1.384615384615386802, -1.422936976036506707, 30.56769352161908415 ) ) ;
#36631=FACE_OUTER_BOUND ( 'NONE', #87195, .T. ) ;
#36632=CARTESIAN_POINT ( 'NONE',  ( -22.75000000000000000, -7.500000000000000000, 29.75000000000000355 ) ) ;
#36636=EDGE_CURVE ( 'NONE', #86110, #53273, #19107, .T. ) ;
#36637=FACE_OUTER_BOUND ( 'NONE', #16501, .T. ) ;
#36638=CARTESIAN_POINT ( 'NONE',  ( 12.46153846153833911, -12.70778746994576025, 30.41441678777401236 ) ) ;
#36639=ORIENTED_EDGE ( 'NONE', *, *, #45640, .T. ) ;
#36640=DIRECTION ( 'NONE',  ( -0.000000000000000000, 0.8660254037844397068, -0.4999999999999978906 ) ) ;
#36641=CARTESIAN_POINT ( 'NONE',  ( 11.76124107972994537, -10.11255958852956027, 34.01340905677048454 ) ) ;
#36642=EDGE_CURVE ( 'NONE', #30027, #18184, #82593, .T. ) ;
#36643=CARTESIAN_POINT ( 'NONE',  ( 6.222779668978067669, -12.69155399931963046, 30.53255429739158444 ) ) ;
#36644=EDGE_LOOP ( 'NONE', ( #67864, #1302 ) ) ;
#36645=CARTESIAN_POINT ( 'NONE',  ( 12.52679360105129902, -11.06231777344671130, 33.60647404775212976 ) ) ;
#36646=CARTESIAN_POINT ( 'NONE',  ( -10.86536135943320502, -12.65889640711025521, 30.72598325615533454 ) ) ;
#36649=EDGE_CURVE ( 'NONE', #14249, #34125, #2722, .T. ) ;
#36650=EDGE_LOOP ( 'NONE', ( #34110, #53023, #53154, #12360 ) ) ;
#36651=DIRECTION ( 'NONE',  ( -0.000000000000000000, 0.3420201433256694901, -0.9396926207859082059 ) ) ;
#36652=ORIENTED_EDGE ( 'NONE', *, *, #16201, .F. ) ;
#36654=CARTESIAN_POINT ( 'NONE',  ( 10.68064018666064108, -8.613356846314928816, 34.62446782046653482 ) ) ;
#36656=CARTESIAN_POINT ( 'NONE',  ( -17.07692307692307665, -3.322132147404559976, 32.92929555188717927 ) ) ;
#36657=B_SPLINE_CURVE_WITH_KNOTS ( 'NONE', 3,
 ( #56212, #47681, #49010, #75167, #68394, #40931, #7588, #29200, #82811, #27853 ),
 .UNSPECIFIED., .F., .F.,
 ( 4, 2, 2, 2, 4 ),
 ( 0.0007817246336856291692, 0.0009771112958940103739, 0.001172497958102391470, 0.001367884620310772566, 0.001563271282519153879 ),
 .UNSPECIFIED. ) ;
#36659=CARTESIAN_POINT ( 'NONE',  ( -9.469528023329623068, -6.717445702608402236, 34.94155399931962336 ) ) ;
#36660=CARTESIAN_POINT ( 'NONE',  ( -3.165624450049597360, -7.750023224968865421, 34.99404313364389907 ) ) ;
#36661=B_SPLINE_CURVE_WITH_KNOTS ( 'NONE', 3,
 ( #38484, #44774, #45675, #71807, #32172, #11011, #87579, #86691, #11453, #38035 ),
 .UNSPECIFIED., .F., .F.,
 ( 4, 2, 2, 2, 4 ),
 ( 0.0007817359430256215491, 0.0009771253907249856981, 0.001172514838424349847, 0.001367904286123713779, 0.001563293733823077928 ),
 .UNSPECIFIED. ) ;
#36662=ORIENTED_EDGE ( 'NONE', *, *, #30260, .T. ) ;
#36663=EDGE_CURVE ( 'NONE', #4672, #17811, #48337, .T. ) ;
#36664=EDGE_LOOP ( 'NONE', ( #66201, #81711 ) ) ;
#36665=ORIENTED_EDGE ( 'NONE', *, *, #54042, .F. ) ;
#36667=EDGE_CURVE ( 'NONE', #49416, #38795, #55378, .T. ) ;
#36668=CARTESIAN_POINT ( 'NONE',  ( -1.134669866267241201, -3.202959910592336534, 32.30730279482227019 ) ) ;
#36669=CARTESIAN_POINT ( 'NONE',  ( -16.94613126909828793, -3.530189275343204702, 32.79018710029569661 ) ) ;
#36670=CARTESIAN_POINT ( 'NONE',  ( 0.5923289025054111478, -6.369690395747424461, 34.87708834333098196 ) ) ;
#36671=VECTOR ( 'NONE', #88937, 1000.000000000000114 ) ;
#36672=CARTESIAN_POINT ( 'NONE',  ( 0.4615384615383382183, -12.51329471203414379, 31.30864560766407578 ) ) ;
#36673=DIRECTION ( 'NONE',  ( 0.000000000000000000, -6.938893903907222067E-15, 1.000000000000000000 ) ) ;
#36674=CARTESIAN_POINT ( 'NONE',  ( 5.299702618191482806, -10.11255958852956027, 34.01340905677048454 ) ) ;
#36675=EDGE_LOOP ( 'NONE', ( #56165, #29047 ) ) ;
#36676=VECTOR ( 'NONE', #15845, 1000.000000000000227 ) ;
#36678=VERTEX_POINT ( 'NONE', #55099 ) ;
#36679=ORIENTED_EDGE ( 'NONE', *, *, #1281, .T. ) ;
#36680=CARTESIAN_POINT ( 'NONE',  ( 4.219913487196228274, -3.937682226553329556, 33.60647404775216529 ) ) ;
#36681=ORIENTED_EDGE ( 'NONE', *, *, #80063, .T. ) ;
#36682=CARTESIAN_POINT ( 'NONE',  ( 6.923076923076924238, -13.63283147151868846, 33.57946703557072254 ) ) ;
#36683=CARTESIAN_POINT ( 'NONE',  ( -5.326946301144536378, -12.68155406624981119, 30.59749803192733708 ) ) ;
#36684=CARTESIAN_POINT ( 'NONE',  ( 13.63466969625370062, -8.303483539816731707, 34.68545999027711702 ) ) ;
#36685=VERTEX_POINT ( 'NONE', #75812 ) ;
#36686=B_SPLINE_CURVE_WITH_KNOTS ( 'NONE', 3,
 ( #60160, #87663, #19186, #74129, #1571, #42564, #50182, #29060, #84886, #14200 ),
 .UNSPECIFIED., .F., .F.,
 ( 4, 2, 2, 2, 4 ),
 ( 0.0007817246256747451124, 0.0009771112852218885505, 0.001172497944769032097, 0.001367884604316175427, 0.001563271263863318973 ),
 .UNSPECIFIED. ) ;
#36687=B_SPLINE_CURVE_WITH_KNOTS ( 'NONE', 3,
 ( #76905, #797, #83676, #29176, #22833, #77780, #55293, #43116, #8450, #82785 ),
 .UNSPECIFIED., .F., .F.,
 ( 4, 2, 2, 2, 4 ),
 ( 0.000000000000000000, 0.0001954311564186865492, 0.0003908623128373730983, 0.0005862934692560596746, 0.0007817246256747461966 ),
 .UNSPECIFIED. ) ;
#36689=CARTESIAN_POINT ( 'NONE',  ( 3.930361229281822855, -4.225889041578354544, 33.85425143139329407 ) ) ;
#36690=ORIENTED_EDGE ( 'NONE', *, *, #74210, .T. ) ;
#36691=FACE_BOUND ( 'NONE', #78206, .T. ) ;
#36692=CARTESIAN_POINT ( 'NONE',  ( -12.46153846153858247, -9.442884908241554243, 34.35708131394783038 ) ) ;
#36693=CARTESIAN_POINT ( 'NONE',  ( -14.30769230769242917, -6.835583212225970762, 34.95778746994575670 ) ) ;
#36694=ORIENTED_EDGE ( 'NONE', *, *, #64173, .T. ) ;
#36695=CARTESIAN_POINT ( 'NONE',  ( -17.07692307692319744, -10.21337939537710326, 33.94971097300076224 ) ) ;
#36696=CYLINDRICAL_SURFACE ( 'NONE', #70567, 0.2499999999999994726 ) ;
#36697=CARTESIAN_POINT ( 'NONE',  ( 1.384615384615386802, -3.322132147404559976, 32.92929555188717927 ) ) ;
#36698=CARTESIAN_POINT ( 'NONE',  ( -15.29685264172511161, -6.386643153685125363, 34.62446782046654903 ) ) ;
#36699=CARTESIAN_POINT ( 'NONE',  ( 1.634669804528840586, -2.544122305571458575, 31.48381861865057729 ) ) ;
#36700=CIRCLE ( 'NONE', #39621, 0.2500000000000002220 ) ;
#36701=CARTESIAN_POINT ( 'NONE',  ( 8.545745844666438273, -11.60425143139329940, 33.02411095842164457 ) ) ;
#36705=CARTESIAN_POINT ( 'NONE',  ( 9.468822767743359847, -12.47654668319379567, 31.42292124445336654 ) ) ;
#36706=CARTESIAN_POINT ( 'NONE',  ( 9.019176178608809380, -4.176053281294518804, 33.81426240980091791 ) ) ;
#36707=CARTESIAN_POINT ( 'NONE',  ( 4.946775867484856093, -12.45813303252208648, 30.39737893381572675 ) ) ;
#36708=CARTESIAN_POINT ( 'NONE',  ( 11.78846153846295763, -7.500000000000154543, 35.00000000000007105 ) ) ;
#36710=CARTESIAN_POINT ( 'NONE',  ( -3.230769230769352962, -3.083524468854526912, 32.58852847137268327 ) ) ;
#36711=CARTESIAN_POINT ( 'NONE',  ( -6.066083410955878108, -4.786620604624113540, 33.94971097300155805 ) ) ;
#36712=CARTESIAN_POINT ( 'NONE',  ( -5.869208192175213945, -12.38066358083363738, 30.83685684665853444 ) ) ;
#36714=ORIENTED_EDGE ( 'NONE', *, *, #21331, .T. ) ;
#36716=ORIENTED_EDGE ( 'NONE', *, *, #70562, .F. ) ;
#36717=EDGE_CURVE ( 'NONE', #20364, #60609, #78030, .T. ) ;
#36718=DIRECTION ( 'NONE',  ( -0.000000000000000000, -0.1736481776669307198, -0.9848077530122080203 ) ) ;
#36719=ORIENTED_EDGE ( 'NONE', *, *, #43407, .F. ) ;
#36720=DIRECTION ( 'NONE',  ( 0.000000000000000000, 1.000000000000000000, 0.000000000000000000 ) ) ;
#36721=EDGE_CURVE ( 'NONE', #20451, #34572, #13416, .T. ) ;
#36722=EDGE_LOOP ( 'NONE', ( #80442, #3371, #83344, #45599 ) ) ;
#36723=CARTESIAN_POINT ( 'NONE',  ( -8.069638789877792817, -5.912607949931405926, 34.49155766932282319 ) ) ;
#36725=CARTESIAN_POINT ( 'NONE',  ( 2.307692307692309264, -1.367168528481310208, 33.57946703557072254 ) ) ;
#36726=CARTESIAN_POINT ( 'NONE',  ( -5.776988648387149539, -9.086983370893049639, 34.49168942202179267 ) ) ;
#36727=CARTESIAN_POINT ( 'NONE',  ( 17.77651507543566822, -2.353723527008297012, 30.78948104536958752 ) ) ;
#36728=CARTESIAN_POINT ( 'NONE',  ( 15.16549923021291058, -8.656820664281498878, 34.87096338111211935 ) ) ;
#36729=CARTESIAN_POINT ( 'NONE',  ( 15.00789054834058511, -7.630691491037285168, 34.74850469731152458 ) ) ;
#36730=CARTESIAN_POINT ( 'NONE',  ( -13.51476335434707821, -12.15440758774515473, 32.17923288041532004 ) ) ;
#36731=EDGE_CURVE ( 'NONE', #19674, #18184, #33847, .T. ) ;
#36734=LINE ( 'NONE', #44357, #80855 ) ;
#36735=CYLINDRICAL_SURFACE ( 'NONE', #50623, 0.2500000000000009437 ) ;
#36736=ADVANCED_FACE ( 'NONE', ( #83924 ), #35271, .F. ) ;
#36737=CARTESIAN_POINT ( 'NONE',  ( 13.51540719244018263, -4.118422570099828484, 33.43335022499816489 ) ) ;
#36739=CARTESIAN_POINT ( 'NONE',  ( -39.05038313613820122, -2.499999999999999556, 29.75000000000000355 ) ) ;
#36740=ORIENTED_EDGE ( 'NONE', *, *, #83793, .T. ) ;
#36741=CARTESIAN_POINT ( 'NONE',  ( -13.38461538461550759, -6.835583212225970762, 34.95778746994575670 ) ) ;
#36742=CARTESIAN_POINT ( 'NONE',  ( 15.93036121012220185, -12.24155766932282496, 31.33739205006857986 ) ) ;
#36744=CARTESIAN_POINT ( 'NONE',  ( 15.16544631527705533, -7.749976743299138882, 34.99404534957040624 ) ) ;
#36746=CARTESIAN_POINT ( 'NONE',  ( 2.307692307692187583, -12.27809138561165270, 31.22303859784587132 ) ) ;
#36747=CARTESIAN_POINT ( 'NONE',  ( 8.519207531937803779, -10.76384336483936011, 33.53834819971076087 ) ) ;
#36748=ORIENTED_EDGE ( 'NONE', *, *, #21033, .F. ) ;
#36749=ORIENTED_EDGE ( 'NONE', *, *, #34256, .F. ) ;
#36750=EDGE_CURVE ( 'NONE', #5178, #10414, #86509, .T. ) ;
#36751=VERTEX_POINT ( 'NONE', #29418 ) ;
#36752=B_SPLINE_CURVE_WITH_KNOTS ( 'NONE', 3,
 ( #32823, #40479, #33272, #74707, #86905, #25618, #47663, #60283, #60731, #53525 ),
 .UNSPECIFIED., .F., .F.,
 ( 4, 2, 2, 2, 4 ),
 ( 0.000000000000000000, 0.0001954311564186882568, 0.0003908623128373765136, 0.0005862934692560647703, 0.0007817246256747530271 ),
 .UNSPECIFIED. ) ;
#36753=CARTESIAN_POINT ( 'NONE',  ( 6.923076923076802558, -10.21337939537710326, 33.94971097300076224 ) ) ;
#36754=CARTESIAN_POINT ( 'NONE',  ( -8.769230769230768274, -2.292212530054420494, 30.41441678777542634 ) ) ;
#36755=CARTESIAN_POINT ( 'NONE',  ( -13.25408968285182354, -9.417988943895561960, 34.36773134775777550 ) ) ;
#36757=ORIENTED_EDGE ( 'NONE', *, *, #82065, .T. ) ;
#36758=EDGE_CURVE ( 'NONE', #78695, #1002, #34958, .T. ) ;
#36760=VERTEX_POINT ( 'NONE', #62732 ) ;
#36761=B_SPLINE_CURVE_WITH_KNOTS ( 'NONE', 3,
 ( #70150, #63388, #57075, #84570, #13876, #7128, #57520, #77791, #64264, #85886 ),
 .UNSPECIFIED., .F., .F.,
 ( 4, 2, 2, 2, 4 ),
 ( 0.000000000000000000, 0.0001954339857564074473, 0.0003908679715128148945, 0.0005863019572692223418, 0.0007817359430256297891 ),
 .UNSPECIFIED. ) ;
#36762=ORIENTED_EDGE ( 'NONE', *, *, #84515, .F. ) ;
#36763=EDGE_CURVE ( 'NONE', #63786, #4010, #42464, .T. ) ;
#36764=EDGE_CURVE ( 'NONE', #5458, #19800, #83305, .T. ) ;
#36765=LINE ( 'NONE', #43521, #32902 ) ;
#36766=DIRECTION ( 'NONE',  ( -0.000000000000000000, 0.1736481776669307198, -0.9848077530122080203 ) ) ;
#36767=LINE ( 'NONE', #2523, #52348 ) ;
#36769=CARTESIAN_POINT ( 'NONE',  ( 12.46153846153846168, -12.62096338111211580, 30.90682066428153263 ) ) ;
#36770=ORIENTED_EDGE ( 'NONE', *, *, #69093, .T. ) ;
#36771=ADVANCED_FACE ( 'NONE', ( #38378 ), #44220, .F. ) ;
#36772=VERTEX_POINT ( 'NONE', #39281 ) ;
#36773=B_SPLINE_CURVE_WITH_KNOTS ( 'NONE', 3,
 ( #65463, #79432, #17731, #10970, #43856, #30348, #9628, #2857, #57817, #78526 ),
 .UNSPECIFIED., .F., .F.,
 ( 4, 2, 2, 2, 4 ),
 ( 0.0007817359430256315238, 0.0009771253907249980580, 0.001172514838424364592, 0.001367904286123730910, 0.001563293733823097444 ),
 .UNSPECIFIED. ) ;
#36775=ORIENTED_EDGE ( 'NONE', *, *, #57199, .T. ) ;
#36776=CARTESIAN_POINT ( 'NONE',  ( -2.557669038634661440, -2.779195860258149242, 31.39871582349837453 ) ) ;
#36777=ORIENTED_EDGE ( 'NONE', *, *, #80319, .T. ) ;
#36778=CARTESIAN_POINT ( 'NONE',  ( -10.61538461538461320, -5.557115091759785130, 34.35708131394839171 ) ) ;
#36779=CARTESIAN_POINT ( 'NONE',  ( 8.519230769230768274, -7.500000000000001776, 35.00000000000000000 ) ) ;
#36780=ADVANCED_FACE ( 'NONE', ( #23521 ), #44668, .F. ) ;
#36781=EDGE_CURVE ( 'NONE', #59185, #45658, #56968, .T. ) ;
#36782=VECTOR ( 'NONE', #64672, 1000.000000000000114 ) ;
#36783=CARTESIAN_POINT ( 'NONE',  ( 7.053602624840490165, -11.93748526763465279, 32.05452791011430946 ) ) ;
#36785=DIRECTION ( 'NONE',  ( -0.000000000000000000, -0.1736481776669307198, -0.9848077530122080203 ) ) ;
#36786=CARTESIAN_POINT ( 'NONE',  ( 5.011673145148991537, -2.255955759149247619, 30.00000000000013856 ) ) ;
#36787=EDGE_LOOP ( 'NONE', ( #87018, #10510, #69222, #4083 ) ) ;
#36788=FACE_BOUND ( 'NONE', #82701, .T. ) ;
#36789=EDGE_CURVE ( 'NONE', #28895, #53468, #43569, .T. ) ;
#36790=CARTESIAN_POINT ( 'NONE',  ( 15.23076923076910916, -11.67786785259630911, 32.92929555188603530 ) ) ;
#36791=CARTESIAN_POINT ( 'NONE',  ( 10.83816415665302380, -9.332535724633409302, 34.40230450496446934 ) ) ;
#36792=CARTESIAN_POINT ( 'NONE',  ( -15.16551409125639260, -3.083524468853784839, 32.58852847137153930 ) ) ;
#36793=DIRECTION ( 'NONE',  ( -0.000000000000000000, 0.7660444431189791237, -0.6427876096865379196 ) ) ;
#36795=FACE_OUTER_BOUND ( 'NONE', #4449, .T. ) ;
#36796=CARTESIAN_POINT ( 'NONE',  ( 14.53047197667037338, -2.353885683473779800, 30.79025554430704403 ) ) ;
#36797=EDGE_LOOP ( 'NONE', ( #83272, #56018, #84323, #50074 ) ) ;
#36798=CARTESIAN_POINT ( 'NONE',  ( -11.31545018684868964, -4.187068189119696804, 33.49521262558774026 ) ) ;
#36799=CYLINDRICAL_SURFACE ( 'NONE', #6211, 0.2500000000000008882 ) ;
#36800=ORIENTED_EDGE ( 'NONE', *, *, #46518, .T. ) ;
#36802=CARTESIAN_POINT ( 'NONE',  ( 10.36536137809165403, -6.695914987888146541, 34.68535235679833306 ) ) ;
#36803=FACE_OUTER_BOUND ( 'NONE', #65980, .T. ) ;
#36804=CARTESIAN_POINT ( 'NONE',  ( -6.000000000000121680, -6.835583212225970762, 34.95778746994575670 ) ) ;
#36805=CARTESIAN_POINT ( 'NONE',  ( -10.48485917715097138, -3.068774925481847493, 32.56582465632704526 ) ) ;
#36807=FACE_BOUND ( 'NONE', #24918, .T. ) ;
#36808=CARTESIAN_POINT ( 'NONE',  ( -1.634638608836841200, -6.652501968072646932, 34.93155406624980941 ) ) ;
#36809=CARTESIAN_POINT ( 'NONE',  ( 18.00000000000000000, -6.435427911321262684, 35.78748833219616898 ) ) ;
#36810=DIRECTION ( 'NONE',  ( 0.000000000000000000, 0.1736481776669275834, 0.9848077530122086864 ) ) ;
#36811=CARTESIAN_POINT ( 'NONE',  ( -6.857821783564083340, -11.06231777344671130, 33.60647404775212976 ) ) ;
#36813=CARTESIAN_POINT ( 'NONE',  ( -5.999999999999998224, -12.78798330534103123, 29.99999999999997868 ) ) ;
#36815=B_SPLINE_CURVE_WITH_KNOTS ( 'NONE', 3,
 ( #20571, #48035, #47152, #26003, #46277, #34087, #5730, #47602, #88179, #74639 ),
 .UNSPECIFIED., .F., .F.,
 ( 4, 2, 2, 2, 4 ),
 ( 0.0007817246256747447872, 0.0009771112852218876831, 0.001172497944769030579, 0.001367884604316173475, 0.001563271263863316371 ),
 .UNSPECIFIED. ) ;
#36818=CARTESIAN_POINT ( 'NONE',  ( -8.069080063669991532, -11.24512374952581872, 33.06303171183252942 ) ) ;
#36819=AXIS2_PLACEMENT_3D ( 'NONE', #66532, #52114, #79603 ) ;
#36821=CARTESIAN_POINT ( 'NONE',  ( 5.869852030268306819, -5.915902021225892149, 34.75552854090298638 ) ) ;
#36825=CARTESIAN_POINT ( 'NONE',  ( -2.557715531913761886, -3.520140089381496473, 33.17453946501458262 ) ) ;
#36826=CARTESIAN_POINT ( 'NONE',  ( -2.307692307692305711, -11.16473453929635440, 33.15142922261926373 ) ) ;
#36827=AXIS2_PLACEMENT_3D ( 'NONE', #51118, #9283, #77284 ) ;
#36828=CARTESIAN_POINT ( 'NONE',  ( -7.912236225513983534, -2.833524468853757305, 32.15551576947924417 ) ) ;
#36829=CARTESIAN_POINT ( 'NONE',  ( -3.007989561791164945, -12.11081565061823717, 32.26097654155341843 ) ) ;
#36830=CARTESIAN_POINT ( 'NONE',  ( 5.300299017621258990, -2.501478030877322567, 29.88021232661720816 ) ) ;
#36831=CARTESIAN_POINT ( 'NONE',  ( 4.153846153846032507, -10.90142922262034020, 33.41473453929536674 ) ) ;
#36832=CARTESIAN_POINT ( 'NONE',  ( 14.30769230769231015, -13.04860791097971706, 34.73218667398347037 ) ) ;
#36833=CARTESIAN_POINT ( 'NONE',  ( 8.096099364501988305, -6.696923467548660192, 34.68552623307873972 ) ) ;
#36834=ORIENTED_EDGE ( 'NONE', *, *, #84193, .F. ) ;
#36835=CARTESIAN_POINT ( 'NONE',  ( 3.361559671736180643, -12.35292014791297710, 31.75344720912887198 ) ) ;
#36836=CARTESIAN_POINT ( 'NONE',  ( 7.173022441425065843, -5.057305518903949526, 34.11320923018887896 ) ) ;
#36838=B_SPLINE_CURVE_WITH_KNOTS ( 'NONE', 3,
 ( #33833, #68947, #7258, #937, #42383, #34723 ),
 .UNSPECIFIED., .F., .F.,
 ( 4, 2, 4 ),
 ( 0.0003909512603273906169, 0.0005862562993132179340, 0.0007815613382990451970 ),
 .UNSPECIFIED. ) ;
#36839=CARTESIAN_POINT ( 'NONE',  ( 0.5920638997721061614, -3.625058011473228259, 33.29252011169590020 ) ) ;
#36840=DIRECTION ( 'NONE',  ( -0.000000000000000000, -0.1736481776669307198, -0.9848077530122080203 ) ) ;
#36841=EDGE_LOOP ( 'NONE', ( #71136, #4009 ) ) ;
#36843=FACE_OUTER_BOUND ( 'NONE', #29471, .T. ) ;
#36844=EDGE_LOOP ( 'NONE', ( #73894, #55507, #82071, #78087 ) ) ;
#36845=CARTESIAN_POINT ( 'NONE',  ( -11.28846153846153477, -2.499999999999999556, 29.81604066197449754 ) ) ;
#36846=CARTESIAN_POINT ( 'NONE',  ( 9.692307692307695177, -13.37000171582298513, 34.34916445242398453 ) ) ;
#36847=CARTESIAN_POINT ( 'NONE',  ( -5.300408020647024543, -11.41268669641500466, 32.86336882939237825 ) ) ;
#36848=CARTESIAN_POINT ( 'NONE',  ( -15.23076923076935252, -5.094484230521993062, 34.41647553114689373 ) ) ;
#36849=EDGE_CURVE ( 'NONE', #20099, #87653, #85681, .T. ) ;
#36850=ORIENTED_EDGE ( 'NONE', *, *, #44864, .F. ) ;
#36851=CARTESIAN_POINT ( 'NONE',  ( -12.59168643127016196, -2.373036134822904319, 30.88089517874952250 ) ) ;
#36852=CARTESIAN_POINT ( 'NONE',  ( -15.93106661257774270, -3.236590943229499473, 32.36255958852954251 ) ) ;
#36854=B_SPLINE_CURVE_WITH_KNOTS ( 'NONE', 3,
 ( #7665, #40132, #67591, #27044, #61700, #54507, #35125, #5889, #76108, #34689 ),
 .UNSPECIFIED., .F., .F.,
 ( 4, 2, 2, 2, 4 ),
 ( 0.000000000000000000, 0.0001954311564186865221, 0.0003908623128373730441, 0.0005862934692560595662, 0.0007817246256747460882 ),
 .UNSPECIFIED. ) ;
#36856=ORIENTED_EDGE ( 'NONE', *, *, #9836, .F. ) ;
#36858=ORIENTED_EDGE ( 'NONE', *, *, #22123, .F. ) ;
#36859=CARTESIAN_POINT ( 'NONE',  ( -9.822999158975250111, -9.804603061927743113, 34.18744698557895845 ) ) ;
#36860=CARTESIAN_POINT ( 'NONE',  ( -14.55771554498526932, -3.202444869320336451, 32.30641848906366675 ) ) ;
#36861=EDGE_CURVE ( 'NONE', #54248, #43633, #72152, .T. ) ;
#36863=EDGE_CURVE ( 'NONE', #4267, #35011, #34863, .T. ) ;
#36864=CARTESIAN_POINT ( 'NONE',  ( -3.099978789802281032, -8.191423895709840863, 34.95447573519442130 ) ) ;
#36865=CARTESIAN_POINT ( 'NONE',  ( -2.307692307692305711, -13.53365097954675988, 30.81389545987213552 ) ) ;
#36866=ORIENTED_EDGE ( 'NONE', *, *, #48820, .F. ) ;
#36867=ADVANCED_FACE ( 'NONE', ( #79366 ), #85241, .F. ) ;
#36868=ORIENTED_EDGE ( 'NONE', *, *, #45591, .F. ) ;
#36870=EDGE_LOOP ( 'NONE', ( #46124, #60455 ) ) ;
#36871=CARTESIAN_POINT ( 'NONE',  ( 16.37685899793955357, -8.282913670948747864, 34.94150082978203642 ) ) ;
#36872=CARTESIAN_POINT ( 'NONE',  ( 7.846153846153846700, -11.91647553114624181, 32.58852847137148245 ) ) ;
#36873=DIRECTION ( 'NONE',  ( -0.000000000000000000, -0.9396926207859092051, -0.3420201433256662704 ) ) ;
#36876=ORIENTED_EDGE ( 'NONE', *, *, #41973, .T. ) ;
#36877=DIRECTION ( 'NONE',  ( 0.000000000000000000, 0.4999999999999985567, 0.8660254037844395958 ) ) ;
#36878=EDGE_LOOP ( 'NONE', ( #15120, #59688 ) ) ;
#36879=B_SPLINE_CURVE_WITH_KNOTS ( 'NONE', 3,
 ( #68887, #34675, #7646, #62138, #35560, #21145, #63002, #41879, #35106, #69347 ),
 .UNSPECIFIED., .F., .F.,
 ( 4, 2, 2, 2, 4 ),
 ( 0.000000000000000000, 0.0001954311564186882568, 0.0003908623128373765136, 0.0005862934692560647703, 0.0007817246256747530271 ),
 .UNSPECIFIED. ) ;
#36880=CARTESIAN_POINT ( 'NONE',  ( 4.284371855609715674, -5.195472089885680766, 34.18748526763464923 ) ) ;
#36881=EDGE_CURVE ( 'NONE', #31211, #69454, #14444, .T. ) ;
#36882=CARTESIAN_POINT ( 'NONE',  ( -10.68146699474474914, -9.058645607665454236, 34.76329471203372634 ) ) ;
#36883=ORIENTED_EDGE ( 'NONE', *, *, #88427, .T. ) ;
#36884=VECTOR ( 'NONE', #15127, 1000.000000000000114 ) ;
#36885=CARTESIAN_POINT ( 'NONE',  ( 16.02315468717859659, -12.38065189839062263, 30.83690757178629482 ) ) ;
#36886=DIRECTION ( 'NONE',  ( -0.000000000000000000, -0.9848077530122086864, -0.1736481776669273613 ) ) ;
#36887=CARTESIAN_POINT ( 'NONE',  ( 12.46153846153833911, -2.892918686052165622, 31.69288490824153470 ) ) ;
#36888=FACE_BOUND ( 'NONE', #83144, .T. ) ;
#36889=CARTESIAN_POINT ( 'NONE',  ( 1.384615384615386802, -12.37446782046654192, 30.86335684631486131 ) ) ;
#36890=CARTESIAN_POINT ( 'NONE',  ( -4.219116599806928214, -12.27809138561121394, 31.22303859784730307 ) ) ;
#36891=CYLINDRICAL_SURFACE ( 'NONE', #82610, 0.2499999999999979738 ) ;
#36893=CARTESIAN_POINT ( 'NONE',  ( 4.153846153846154188, -2.292212530054420494, 30.41441678777542634 ) ) ;
#36894=CARTESIAN_POINT ( 'NONE',  ( 17.75002325595141173, -6.524016743844656574, 34.90889640711025521 ) ) ;
#36895=CARTESIAN_POINT ( 'NONE',  ( -7.846153846153967493, -12.51329471203414379, 31.30864560766407578 ) ) ;
#36896=VERTEX_POINT ( 'NONE', #79816 ) ;
#36897=CARTESIAN_POINT ( 'NONE',  ( -5.934744428723973897, -11.94971097300157403, 32.03036669348361443 ) ) ;
#36900=DIRECTION ( 'NONE',  ( 0.000000000000000000, 0.8660254037844377084, -0.5000000000000015543 ) ) ;
#36901=CARTESIAN_POINT ( 'NONE',  ( -5.749945688361684404, -12.17597550085003633, 31.52189283813461884 ) ) ;
#36902=CARTESIAN_POINT ( 'NONE',  ( -6.857008572074484221, -6.386643153685127139, 34.62446782046654192 ) ) ;
#36903=CARTESIAN_POINT ( 'NONE',  ( 14.30769230769218581, -4.320704448113951379, 33.92786785259630022 ) ) ;
#36904=CARTESIAN_POINT ( 'NONE',  ( 2.373759641042385571, -2.292212530054420494, 30.41441678777542990 ) ) ;
#36905=CARTESIAN_POINT ( 'NONE',  ( 1.134638653673031961, -11.79746400365624659, 32.30657167506340954 ) ) ;
#36906=ORIENTED_EDGE ( 'NONE', *, *, #71332, .T. ) ;
#36907=VECTOR ( 'NONE', #75720, 1000.000000000000227 ) ;
#36908=CARTESIAN_POINT ( 'NONE',  ( 4.153846153846154188, -4.661471528628507777, 34.16647553114623292 ) ) ;
#36909=CARTESIAN_POINT ( 'NONE',  ( 6.700150705560775855, -3.586966769969700763, 32.86292498521069660 ) ) ;
#36910=LINE ( 'NONE', #55859, #43085 ) ;
#36911=CARTESIAN_POINT ( 'NONE',  ( 17.07692307692307665, -4.098570777380720287, 33.41473453929634729 ) ) ;
#36912=DIRECTION ( 'NONE',  ( -0.000000000000000000, -0.6427876096865404731, -0.7660444431189770143 ) ) ;
#36914=ORIENTED_EDGE ( 'NONE', *, *, #48845, .T. ) ;
#36915=B_SPLINE_CURVE_WITH_KNOTS ( 'NONE', 3,
 ( #86102, #24376, #51844, #79340, #17644, #65807, #45099, #4108, #31592, #59058 ),
 .UNSPECIFIED., .F., .F.,
 ( 4, 2, 2, 2, 4 ),
 ( 0.0007817359430256366195, 0.0009771253907250045632, 0.001172514838424372615, 0.001367904286123740668, 0.001563293733823108503 ),
 .UNSPECIFIED. ) ;
#36916=ORIENTED_EDGE ( 'NONE', *, *, #36117, .F. ) ;
#36920=CARTESIAN_POINT ( 'NONE',  ( -9.692307692307814193, -6.835583212225970762, 34.95778746994575670 ) ) ;
#36922=CARTESIAN_POINT ( 'NONE',  ( 3.230769230769110045, -6.879047030192662504, 34.71129190930017927 ) ) ;
#36923=CARTESIAN_POINT ( 'NONE',  ( 16.82692307692307665, -7.500000000000001776, 35.00000000000000000 ) ) ;
#36926=ORIENTED_EDGE ( 'NONE', *, *, #3311, .T. ) ;
#36927=CARTESIAN_POINT ( 'NONE',  ( 4.403846153846090239, -7.565270445406050648, 34.75000000000000000 ) ) ;
#36928=DIRECTION ( 'NONE',  ( -0.000000000000000000, 0.3420201433256694901, -0.9396926207859082059 ) ) ;
#36929=EDGE_LOOP ( 'NONE', ( #26708, #8203 ) ) ;
#36930=CARTESIAN_POINT ( 'NONE',  ( 3.230769230769231726, -12.34228464037088635, 31.77849191805839268 ) ) ;
#36931=LINE ( 'NONE', #78359, #74631 ) ;
#36932=B_SPLINE_CURVE_WITH_KNOTS ( 'NONE', 3,
 ( #2334, #77124, #42905, #43776, #49650, #14986, #8677, #64037, #36152, #71237 ),
 .UNSPECIFIED., .F., .F.,
 ( 4, 2, 2, 2, 4 ),
 ( 0.0007817359430256400890, 0.0009771253907250091169, 0.001172514838424378253, 0.001367904286123747173, 0.001563293733823116309 ),
 .UNSPECIFIED. ) ;
#36933=CARTESIAN_POINT ( 'NONE',  ( 5.076923076923075762, -12.10708131394839349, 31.69288490824020244 ) ) ;
#36934=CARTESIAN_POINT ( 'NONE',  ( 11.76147438255493149, -8.282913670948747864, 34.94150082978203642 ) ) ;
#36935=CARTESIAN_POINT ( 'NONE',  ( -12.68446467905460828, -12.39988816332205701, 30.74660775122750778 ) ) ;
#36938=VERTEX_POINT ( 'NONE', #59531 ) ;
#36939=CARTESIAN_POINT ( 'NONE',  ( 1.161130440891438687, -5.912607949931405038, 34.49155766932282319 ) ) ;
#36940=CARTESIAN_POINT ( 'NONE',  ( -1.634592115557737646, -12.17611988154120972, 31.52148481390971213 ) ) ;
#36942=CARTESIAN_POINT ( 'NONE',  ( -16.02332071561251325, -11.66157788607254275, 32.95092075102925833 ) ) ;
#36943=VECTOR ( 'NONE', #5241, 1000.000000000000227 ) ;
#36944=CARTESIAN_POINT ( 'NONE',  ( -7.596208436775802930, -2.986452184633680229, 32.43230066228895225 ) ) ;
#36945=ORIENTED_EDGE ( 'NONE', *, *, #21888, .F. ) ;
#36947=CARTESIAN_POINT ( 'NONE',  ( 3.165498784808455923, -9.442884908240170461, 34.35708131394840592 ) ) ;
#36948=ORIENTED_EDGE ( 'NONE', *, *, #59810, .F. ) ;
#36949=CARTESIAN_POINT ( 'NONE',  ( -18.13069060311030967, -4.684245665217971144, 34.18127051446801090 ) ) ;
#36950=ORIENTED_EDGE ( 'NONE', *, *, #42763, .T. ) ;
#36951=CARTESIAN_POINT ( 'NONE',  ( 7.173022332454967120, -4.176053281294514363, 33.81426240980091791 ) ) ;
#36952=CARTESIAN_POINT ( 'NONE',  ( 3.230769230769231726, -3.937682226553329556, 33.60647404775216529 ) ) ;
#36954=CARTESIAN_POINT ( 'NONE',  ( -1.515306851282940181, -4.118384482072085184, 33.43331474514187107 ) ) ;
#36955=LINE ( 'NONE', #2278, #40769 ) ;
#36956=ORIENTED_EDGE ( 'NONE', *, *, #70331, .F. ) ;
#36957=CARTESIAN_POINT ( 'NONE',  ( -8.992097032293871806, -2.251424796025575326, 29.88072029997477941 ) ) ;
#36959=VERTEX_POINT ( 'NONE', #46468 ) ;
#36960=CARTESIAN_POINT ( 'NONE',  ( -17.77722033102192967, -12.11081565061824250, 32.26097654155340422 ) ) ;
#36961=CARTESIAN_POINT ( 'NONE',  ( -3.903846153846087574, -7.434744429011176159, 34.75000000000000711 ) ) ;
#36962=ORIENTED_EDGE ( 'NONE', *, *, #25122, .T. ) ;
#36963=EDGE_CURVE ( 'NONE', #57712, #51469, #57646, .T. ) ;
#36964=CARTESIAN_POINT ( 'NONE',  ( 11.53846153846141576, -12.70778746994576025, 30.41441678777401236 ) ) ;
#36965=CARTESIAN_POINT ( 'NONE',  ( 10.68145296638705410, -3.050289026998446840, 32.03036669348366416 ) ) ;
#36966=FACE_OUTER_BOUND ( 'NONE', #86096, .T. ) ;
#36967=LINE ( 'NONE', #84300, #46323 ) ;
#36968=CARTESIAN_POINT ( 'NONE',  ( -18.24997673094235395, -4.236021600441996604, 33.53823185664189310 ) ) ;
#36969=ORIENTED_EDGE ( 'NONE', *, *, #48723, .F. ) ;
#36970=EDGE_LOOP ( 'NONE', ( #30745, #17298, #45853, #39697 ) ) ;
#36972=FACE_BOUND ( 'NONE', #28349, .T. ) ;
#36973=ORIENTED_EDGE ( 'NONE', *, *, #54235, .T. ) ;
#36974=CARTESIAN_POINT ( 'NONE',  ( -8.096130590202436750, -5.643011162660950042, 34.66104346484419096 ) ) ;
#36975=B_SPLINE_CURVE_WITH_KNOTS ( 'NONE', 3,
 ( #74393, #510, #33844, #12692, #12246, #40177, #64, #27535, #20772, #75711 ),
 .UNSPECIFIED., .F., .F.,
 ( 4, 2, 2, 2, 4 ),
 ( 0.000000000000000000, 0.0001954339857564076641, 0.0003908679715128153282, 0.0005863019572692229923, 0.0007817359430256306564 ),
 .UNSPECIFIED. ) ;
#36976=VECTOR ( 'NONE', #9617, 1000.000000000000000 ) ;
#36977=CARTESIAN_POINT ( 'NONE',  ( 6.000000000000001776, -10.67929555188718282, 33.92786785259544047 ) ) ;
#36978=CARTESIAN_POINT ( 'NONE',  ( -14.17690049986751433, -8.999086150933475636, 34.52020707165672775 ) ) ;
#36979=VERTEX_POINT ( 'NONE', #61293 ) ;
#36980=ORIENTED_EDGE ( 'NONE', *, *, #34632, .F. ) ;
#36981=CARTESIAN_POINT ( 'NONE',  ( 16.82694634598072270, -4.236021600441997492, 33.53823185664189310 ) ) ;
#36983=FACE_OUTER_BOUND ( 'NONE', #2595, .T. ) ;
#36984=EDGE_CURVE ( 'NONE', #80414, #84227, #53667, .T. ) ;
#36985=DIRECTION ( 'NONE',  ( 0.000000000000000000, 0.3420201433256641055, -0.9396926207859100932 ) ) ;
#36987=CARTESIAN_POINT ( 'NONE',  ( -12.46153846153814726, -2.255955759149395501, 30.00000000000324363 ) ) ;
#36988=FACE_BOUND ( 'NONE', #8868, .T. ) ;
#36989=ORIENTED_EDGE ( 'NONE', *, *, #24444, .T. ) ;
#36990=B_SPLINE_CURVE_WITH_KNOTS ( 'NONE', 3,
 ( #39831, #11916, #81261, #47453, #60974, #19112, #33065, #33516, #88479, #32615 ),
 .UNSPECIFIED., .F., .F.,
 ( 4, 2, 2, 2, 4 ),
 ( 0.0007817359430256390048, 0.0009771253907250075990, 0.001172514838424376085, 0.001367904286123744571, 0.001563293733823113056 ),
 .UNSPECIFIED. ) ;
#36991=CARTESIAN_POINT ( 'NONE',  ( -9.692307692307691624, -11.33034616979429110, 35.88435417666054406 ) ) ;
#36992=EDGE_CURVE ( 'NONE', #21128, #67701, #87936, .T. ) ;
#36993=CARTESIAN_POINT ( 'NONE',  ( -6.250023224221455287, -6.652501968072646932, 34.93155406624980941 ) ) ;
#36996=CARTESIAN_POINT ( 'NONE',  ( 8.899756470994335089, -3.285477652293413264, 32.44071101563363158 ) ) ;
#36997=CARTESIAN_POINT ( 'NONE',  ( -1.319360245102545681, -3.083524468853784839, 32.58852847137153930 ) ) ;
#36999=EDGE_LOOP ( 'NONE', ( #26182, #15364 ) ) ;
#37000=VERTEX_POINT ( 'NONE', #67188 ) ;
#37002=CARTESIAN_POINT ( 'NONE',  ( 5.934729554039225974, -3.300289026998414865, 32.46337939537583139 ) ) ;
#37003=FACE_OUTER_BOUND ( 'NONE', #43316, .T. ) ;
#37004=CARTESIAN_POINT ( 'NONE',  ( -3.903900635498011251, -4.336752205174647656, 33.62275283266504289 ) ) ;
#37005=CARTESIAN_POINT ( 'NONE',  ( 7.780883400193070898, -12.46129190929999986, 30.37095296980880832 ) ) ;
#37006=CARTESIAN_POINT ( 'NONE',  ( -15.36145983387954139, -3.338472653186243644, 32.95098750199972670 ) ) ;
#37007=ORIENTED_EDGE ( 'NONE', *, *, #46527, .T. ) ;
#37008=LINE ( 'NONE', #64471, #21290 ) ;
#37009=CARTESIAN_POINT ( 'NONE',  ( -0.2114840416250089172, -3.435999193479610803, 33.07426656108012963 ) ) ;
#37010=B_SPLINE_CURVE_WITH_KNOTS ( 'NONE', 3,
 ( #50350, #77831, #16137, #9386, #80966, #74638, #80058, #53013, #87729, #26001 ),
 .UNSPECIFIED., .F., .F.,
 ( 4, 2, 2, 2, 4 ),
 ( 0.000000000000000000, 0.0001954339857564079894, 0.0003908679715128159787, 0.0005863019572692239681, 0.0007817359430256319575 ),
 .UNSPECIFIED. ) ;
#37013=EDGE_LOOP ( 'NONE', ( #54281, #24200 ) ) ;
#37014=B_SPLINE_CURVE_WITH_KNOTS ( 'NONE', 3,
 ( #25377, #11875, #65906, #52840, #32570, #39352, #39790, #46096, #25826, #73122 ),
 .UNSPECIFIED., .F., .F.,
 ( 4, 2, 2, 2, 4 ),
 ( 0.000000000000000000, 0.0001954339857564081791, 0.0003908679715128163582, 0.0005863019572692245102, 0.0007817359430256327164 ),
 .UNSPECIFIED. ) ;
#37016=B_SPLINE_CURVE_WITH_KNOTS ( 'NONE', 3,
 ( #88813, #6387, #82925, #12688, #54546, #27973, #20338, #26201, #82042, #61 ),
 .UNSPECIFIED., .F., .F.,
 ( 4, 2, 2, 2, 4 ),
 ( 0.0007817246256747452209, 0.0009771112852218887673, 0.001172497944769032531, 0.001367884604316176294, 0.001563271263863319840 ),
 .UNSPECIFIED. ) ;
#37017=FACE_BOUND ( 'NONE', #47498, .T. ) ;
#37018=DIRECTION ( 'NONE',  ( 0.000000000000000000, 0.4999999999999960032, -0.8660254037844410391 ) ) ;
#37019=CARTESIAN_POINT ( 'NONE',  ( 14.30769230769218758, -11.94971097300221174, 32.03036669348237098 ) ) ;
#37020=VERTEX_POINT ( 'NONE', #88369 ) ;
#37021=CARTESIAN_POINT ( 'NONE',  ( 4.087763774486018242, -11.35647404775217595, 33.31231777344666511 ) ) ;
#37022=CARTESIAN_POINT ( 'NONE',  ( 6.923076923076924238, -10.51840700105979565, 33.73612834413961536 ) ) ;
#37023=CARTESIAN_POINT ( 'NONE',  ( 8.638540166120462160, -8.191372820521381826, 34.95448215188423546 ) ) ;
#37024=CARTESIAN_POINT ( 'NONE',  ( -4.153846153846152411, -4.102666532097928531, 36.13435417666054406 ) ) ;
#37026=DIRECTION ( 'NONE',  ( 0.000000000000000000, 0.3420201433256641055, -0.9396926207859100932 ) ) ;
#37027=EDGE_LOOP ( 'NONE', ( #64138, #14568, #69514, #33046 ) ) ;
#37028=CARTESIAN_POINT ( 'NONE',  ( 13.51540719244017730, -12.11778462344221019, 31.66786338562085135 ) ) ;
#37030=CARTESIAN_POINT ( 'NONE',  ( -18.22305672590244896, -12.75000000000001066, 29.61950333530916168 ) ) ;
#37031=CARTESIAN_POINT ( 'NONE',  ( 14.98074599347626545, -2.823816976329317274, 31.52131813110795733 ) ) ;
#37032=DIRECTION ( 'NONE',  ( 0.000000000000000000, 0.000000000000000000, 1.000000000000000000 ) ) ;
#37033=EDGE_CURVE ( 'NONE', #17504, #20844, #32502, .T. ) ;
#37034=AXIS2_PLACEMENT_3D ( 'NONE', #21731, #62262, #48753 ) ;
#37035=CARTESIAN_POINT ( 'NONE',  ( -12.33074665371367828, -2.729792928343269587, 31.24908615093345077 ) ) ;
#37036=CARTESIAN_POINT ( 'NONE',  ( 6.923076923076924238, -12.78798330534102945, 29.74999999999997868 ) ) ;
#37037=CARTESIAN_POINT ( 'NONE',  ( 12.39626846098214052, -5.941354392334499579, 34.76329471203369792 ) ) ;
#37040=AXIS2_PLACEMENT_3D ( 'NONE', #59829, #32365, #88665 ) ;
#37041=CARTESIAN_POINT ( 'NONE',  ( 13.63466980452883526, -12.65882529074907126, 30.72640787790839312 ) ) ;
#37044=ORIENTED_EDGE ( 'NONE', *, *, #47610, .T. ) ;
#37045=VERTEX_POINT ( 'NONE', #13566 ) ;
#37047=CARTESIAN_POINT ( 'NONE',  ( -14.30769230769230660, -2.486705287966279876, 31.30864560766543647 ) ) ;
#37048=CARTESIAN_POINT ( 'NONE',  ( 2.980792499826877773, -9.943427161483782584, 34.11278801902876978 ) ) ;
#37049=ADVANCED_FACE ( 'NONE', ( #82039 ), #59976, .F. ) ;
#37050=B_SPLINE_CURVE_WITH_KNOTS ( 'NONE', 3,
 ( #21262, #41997, #60485, #40224, #67692, #48736, #34335, #5997, #33017, #33460 ),
 .UNSPECIFIED., .F., .F.,
 ( 4, 2, 2, 2, 4 ),
 ( 0.000000000000000000, 0.0001954339857564080707, 0.0003908679715128161414, 0.0005863019572692241849, 0.0007817359430256322827 ),
 .UNSPECIFIED. ) ;
#37051=CARTESIAN_POINT ( 'NONE',  ( 9.626224281351811740, -12.37446782046654192, 30.86335684631486487 ) ) ;
#37052=CARTESIAN_POINT ( 'NONE',  ( -4.826977558574935045, -3.712312575010499494, 33.01462480002815170 ) ) ;
#37053=CARTESIAN_POINT ( 'NONE',  ( -9.019254006523732770, -11.86270091957321249, 32.19358267280087915 ) ) ;
#37054=B_SPLINE_CURVE_WITH_KNOTS ( 'NONE', 3,
 ( #79970, #45282, #18272, #10179, #73217, #37641, #85842, #66456, #4762, #52926 ),
 .UNSPECIFIED., .F., .F.,
 ( 4, 2, 2, 2, 4 ),
 ( 0.000000000000000000, 0.0001954311564186862510, 0.0003908623128373725020, 0.0005862934692560588072, 0.0007817246256747450040 ),
 .UNSPECIFIED. ) ;
#37055=CARTESIAN_POINT ( 'NONE',  ( 6.130047435250454591, -7.723484941389743952, 34.99544897038808955 ) ) ;
#37058=CYLINDRICAL_SURFACE ( 'NONE', #52039, 0.2500000000000008882 ) ;
#37059=CARTESIAN_POINT ( 'NONE',  ( -8.769230769230768274, -11.35647404775217417, 33.31231777344666511 ) ) ;
#37060=CARTESIAN_POINT ( 'NONE',  ( 2.084207363968359150, -3.754499324213721234, 33.06261337010820256 ) ) ;
#37061=VERTEX_POINT ( 'NONE', #58 ) ;
#37062=DIRECTION ( 'NONE',  ( -0.000000000000000000, 0.7660444431189791237, -0.6427876096865379196 ) ) ;
#37063=ADVANCED_FACE ( 'NONE', ( #26641 ), #47796, .F. ) ;
#37064=VERTEX_POINT ( 'NONE', #68079 ) ;
#37065=AXIS2_PLACEMENT_3D ( 'NONE', #70024, #1126, #49316 ) ;
#37066=CARTESIAN_POINT ( 'NONE',  ( 14.98074599347626545, -11.37209801155882793, 32.91403422569033665 ) ) ;
#37067=CARTESIAN_POINT ( 'NONE',  ( -3.165513659493206067, -2.892918686051626498, 31.69288490824026638 ) ) ;
#37068=CARTESIAN_POINT ( 'NONE',  ( -2.438169015808770546, -7.276988635370450709, 34.74523720219453793 ) ) ;
#37069=ORIENTED_EDGE ( 'NONE', *, *, #34867, .F. ) ;
#37070=ADVANCED_FACE ( 'NONE', ( #54099 ), #6805, .F. ) ;
#37072=DIRECTION ( 'NONE',  ( 1.000000000000000000, 0.000000000000000000, 0.000000000000000000 ) ) ;
#37074=CYLINDRICAL_SURFACE ( 'NONE', #6344, 0.2500000000000012212 ) ;
#37075=AXIS2_PLACEMENT_3D ( 'NONE', #37406, #58121, #37859 ) ;
#37078=CARTESIAN_POINT ( 'NONE',  ( -0.7115616988314267255, -8.432397168068783699, 34.66272746175022945 ) ) ;
#37079=VERTEX_POINT ( 'NONE', #53216 ) ;
#37080=CARTESIAN_POINT ( 'NONE',  ( -9.692307692307812417, -12.27809138561165270, 31.22303859784587132 ) ) ;
#37081=EDGE_CURVE ( 'NONE', #21191, #3730, #83818, .T. ) ;
#37082=CARTESIAN_POINT ( 'NONE',  ( -16.28453762051371356, -11.18331474514187995, 33.13161551792790505 ) ) ;
#37083=CARTESIAN_POINT ( 'NONE',  ( -6.250023237292963607, -2.587272538249754117, 30.68239716806877837 ) ) ;
#37085=LINE ( 'NONE', #36224, #63771 ) ;
#37086=B_SPLINE_CURVE_WITH_KNOTS ( 'NONE', 3,
 ( #68508, #74841, #32503, #53668, #59977, #60868 ),
 .UNSPECIFIED., .F., .F.,
 ( 4, 2, 4 ),
 ( 0.000000000000000000, 0.0001954784845028913534, 0.0003909569690057827069 ),
 .UNSPECIFIED. ) ;
#37087=CARTESIAN_POINT ( 'NONE',  ( -13.63461538461538325, -7.500000000000001776, 35.00000000000000000 ) ) ;
#37088=EDGE_LOOP ( 'NONE', ( #69224, #50056 ) ) ;
#37089=B_SPLINE_CURVE_WITH_KNOTS ( 'NONE', 3,
 ( #13778, #28177, #76366, #1604, #48002, #29092, #82700, #49348, #56545, #1155 ),
 .UNSPECIFIED., .F., .F.,
 ( 4, 2, 2, 2, 4 ),
 ( 0.0007817359430256390048, 0.0009771253907250078159, 0.001172514838424376735, 0.001367904286123745655, 0.001563293733823114574 ),
 .UNSPECIFIED. ) ;
#37090=AXIS2_PLACEMENT_3D ( 'NONE', #32950, #60857, #46458 ) ;
#37091=VERTEX_POINT ( 'NONE', #69403 ) ;
#37092=ORIENTED_EDGE ( 'NONE', *, *, #34902, .T. ) ;
#37093=EDGE_CURVE ( 'NONE', #29234, #87291, #64725, .T. ) ;
#37094=CARTESIAN_POINT ( 'NONE',  ( 1.384615384615386802, -9.058645607665452459, 34.76329471203371924 ) ) ;
#37095=CARTESIAN_POINT ( 'NONE',  ( 11.53846153846153832, -9.058645607665452459, 34.76329471203371924 ) ) ;
#37096=AXIS2_PLACEMENT_3D ( 'NONE', #22955, #44989, #66154 ) ;
#37097=CARTESIAN_POINT ( 'NONE',  ( -15.00775787915638126, -9.086983370893049639, 34.49168942202179267 ) ) ;
#37098=DIRECTION ( 'NONE',  ( -0.000000000000000000, -0.9396926207859092051, -0.3420201433256662704 ) ) ;
#37099=CARTESIAN_POINT ( 'NONE',  ( 7.716005876422150855, -12.70455904226513866, 30.44083106164009322 ) ) ;
#37100=CARTESIAN_POINT ( 'NONE',  ( 17.07692307692307665, -9.905515769479276145, 34.41647553114623292 ) ) ;
#37101=CARTESIAN_POINT ( 'NONE',  ( -17.93393164899755732, -9.780366693483671270, 34.19971097300155805 ) ) ;
#37103=CARTESIAN_POINT ( 'NONE',  ( 9.692307692307570832, -10.33852847137269571, 34.16647553114546554 ) ) ;
#37104=ORIENTED_EDGE ( 'NONE', *, *, #74459, .F. ) ;
#37105=ORIENTED_EDGE ( 'NONE', *, *, #24529, .F. ) ;
#37106=EDGE_LOOP ( 'NONE', ( #62460, #44615 ) ) ;
#37107=CARTESIAN_POINT ( 'NONE',  ( 11.60452887181161508, -2.486705287966280320, 31.30864560766543647 ) ) ;
#37110=CARTESIAN_POINT ( 'NONE',  ( -10.48485917715097138, -6.808710257144161559, 34.95449254468098843 ) ) ;
#37111=CYLINDRICAL_SURFACE ( 'NONE', #60475, 0.2499999999999973355 ) ;
#37112=CARTESIAN_POINT ( 'NONE',  ( -10.74607608205217346, -11.71456829005830080, 32.44064028649416542 ) ) ;
#37113=ORIENTED_EDGE ( 'NONE', *, *, #41639, .T. ) ;
#37115=ORIENTED_EDGE ( 'NONE', *, *, #69892, .T. ) ;
#37116=CARTESIAN_POINT ( 'NONE',  ( -11.76194646302586477, -12.11044203135681840, 32.26167407432752299 ) ) ;
#37117=ORIENTED_EDGE ( 'NONE', *, *, #65655, .F. ) ;
#37118=FACE_BOUND ( 'NONE', #60812, .T. ) ;
#37119=CYLINDRICAL_SURFACE ( 'NONE', #40425, 0.2499999999999995559 ) ;
#37121=CARTESIAN_POINT ( 'NONE',  ( -4.153846153846152411, -11.69971097300155272, 32.46337939537588113 ) ) ;
#37122=ORIENTED_EDGE ( 'NONE', *, *, #57477, .F. ) ;
#37123=EDGE_CURVE ( 'NONE', #82411, #18197, #25439, .T. ) ;
#37124=CARTESIAN_POINT ( 'NONE',  ( -14.17690186672535901, -8.191423895709840863, 34.95447573519442130 ) ) ;
#37125=CARTESIAN_POINT ( 'NONE',  ( 3.361294932532796764, -3.285477652293413264, 32.44071101563363158 ) ) ;
#37126=DIRECTION ( 'NONE',  ( -0.000000000000000000, -0.3420201433256694346, -0.9396926207859080948 ) ) ;
#37127=ORIENTED_EDGE ( 'NONE', *, *, #11838, .F. ) ;
#37128=CARTESIAN_POINT ( 'NONE',  ( 17.86939034479591726, -7.722926974430166069, 34.99546784045485737 ) ) ;
#37129=CYLINDRICAL_SURFACE ( 'NONE', #20760, 0.2500000000000008882 ) ;
#37130=VERTEX_POINT ( 'NONE', #8148 ) ;
#37132=CARTESIAN_POINT ( 'NONE',  ( 8.068933515131909928, -11.60474049983371003, 33.02348890104160262 ) ) ;
#37133=CARTESIAN_POINT ( 'NONE',  ( -14.30769230769230660, -6.343179335718451384, 34.87096338111211935 ) ) ;
#37134=CARTESIAN_POINT ( 'NONE',  ( 3.361294932532796320, -4.459921816937789885, 33.71989282347011851 ) ) ;
#37136=CARTESIAN_POINT ( 'NONE',  ( 13.38461538461538680, -2.292212530054420494, 30.41441678777542634 ) ) ;
#37137=CYLINDRICAL_SURFACE ( 'NONE', #43029, 0.2500000000000002220 ) ;
#37138=EDGE_CURVE ( 'NONE', #14427, #49108, #3025, .T. ) ;
#37139=CARTESIAN_POINT ( 'NONE',  ( -13.38461538461550759, -12.51329471203414379, 31.30864560766407578 ) ) ;
#37140=CARTESIAN_POINT ( 'NONE',  ( -11.53846153846153655, -6.681629849574314051, 35.83090037661290239 ) ) ;
#37141=CYLINDRICAL_SURFACE ( 'NONE', #61805, 0.2499999999999979738 ) ;
#37142=VECTOR ( 'NONE', #27503, 1000.000000000000114 ) ;
#37143=CARTESIAN_POINT ( 'NONE',  ( -0.3954711281883858676, -8.164416787775445883, 34.95778746994558617 ) ) ;
#37144=CYLINDRICAL_SURFACE ( 'NONE', #30010, 0.2500000000000009437 ) ;
#37145=DIRECTION ( 'NONE',  ( -0.000000000000000000, 0.3420201433256694346, -0.9396926207859080948 ) ) ;
#37149=EDGE_CURVE ( 'NONE', #20800, #84823, #1816, .T. ) ;
#37150=B_SPLINE_CURVE_WITH_KNOTS ( 'NONE', 3,
 ( #41265, #29094, #13781, #63297, #75482, #56103, #83597, #34937, #48005, #1606 ),
 .UNSPECIFIED., .F., .F.,
 ( 4, 2, 2, 2, 4 ),
 ( 0.0007817246256747460882, 0.0009771112852218900684, 0.001172497944769033832, 0.001367884604316177595, 0.001563271263863321575 ),
 .UNSPECIFIED. ) ;
#37151=CARTESIAN_POINT ( 'NONE',  ( 18.22301135161285046, -11.76359900205217457, 32.36225158514719880 ) ) ;
#37152=ORIENTED_EDGE ( 'NONE', *, *, #7791, .F. ) ;
#37153=B_SPLINE_CURVE_WITH_KNOTS ( 'NONE', 3,
 ( #45559, #10895, #66727, #52758, #5026, #64935, #80248, #72141, #59073, #87465 ),
 .UNSPECIFIED., .F., .F.,
 ( 4, 2, 2, 2, 4 ),
 ( 0.000000000000000000, 0.0001954311564186861968, 0.0003908623128373723936, 0.0005862934692560585904, 0.0007817246256747447872 ),
 .UNSPECIFIED. ) ;
#37154=EDGE_CURVE ( 'NONE', #55599, #20857, #39483, .T. ) ;
#37155=CARTESIAN_POINT ( 'NONE',  ( -2.531177232256639709, -3.019605429927184836, 32.48692288466676814 ) ) ;
#37156=EDGE_LOOP ( 'NONE', ( #76397, #31253 ) ) ;
#37157=CARTESIAN_POINT ( 'NONE',  ( -3.931066612577743147, -11.41317474335729187, 32.86274602512330034 ) ) ;
#37158=ORIENTED_EDGE ( 'NONE', *, *, #25992, .T. ) ;
#37159=DIRECTION ( 'NONE',  ( -0.000000000000000000, -0.000000000000000000, -1.000000000000000000 ) ) ;
#37161=CARTESIAN_POINT ( 'NONE',  ( 17.29970261819148902, -8.496831190052089866, 34.64984203495476578 ) ) ;
#37162=CARTESIAN_POINT ( 'NONE',  ( -4.153846153846152411, -6.189225973068211317, 35.74407628777942847 ) ) ;
#37164=CARTESIAN_POINT ( 'NONE',  ( 17.99999999999987566, -2.379036618888197729, 30.90682066428292885 ) ) ;
#37165=EDGE_CURVE ( 'NONE', #28537, #49979, #82922, .T. ) ;
#37166=DIRECTION ( 'NONE',  ( -1.000000000000000000, 0.000000000000000000, 0.000000000000000000 ) ) ;
#37167=CARTESIAN_POINT ( 'NONE',  ( -13.51476335434707821, -8.630895178749533159, 34.87696386517710323 ) ) ;
#37168=CARTESIAN_POINT ( 'NONE',  ( -10.61538461538461320, -1.367168528481310208, 33.57946703557072254 ) ) ;
#37170=CARTESIAN_POINT ( 'NONE',  ( -11.53846153846166089, -2.657715359629662544, 31.77849191805970364 ) ) ;
#37171=CARTESIAN_POINT ( 'NONE',  ( -2.177166869458663889, -12.15418822224088657, 32.17964115625579069 ) ) ;
#37172=CARTESIAN_POINT ( 'NONE',  ( 10.36540787133602670, -5.643011162660950042, 34.66104346484419096 ) ) ;
#37173=VECTOR ( 'NONE', #12881, 1000.000000000000227 ) ;
#37175=EDGE_LOOP ( 'NONE', ( #73732, #70837, #43917, #59240 ) ) ;
#37176=CARTESIAN_POINT ( 'NONE',  ( 17.32686859527121470, -12.22109172314383052, 31.39792113162168263 ) ) ;
#37177=CARTESIAN_POINT ( 'NONE',  ( 12.39545608217832218, -8.164416787775445883, 34.95778746994557906 ) ) ;
#37178=CARTESIAN_POINT ( 'NONE',  ( -8.992156986746914882, -11.24512374952581872, 33.06303171183252942 ) ) ;
#37179=CARTESIAN_POINT ( 'NONE',  ( 5.299934428535923558, -2.758310577978207778, 31.33698337089303010 ) ) ;
#37180=ADVANCED_FACE ( 'NONE', ( #41935 ), #30509, .F. ) ;
#37181=DIRECTION ( 'NONE',  ( -0.000000000000000000, -0.1736481776669307198, -0.9848077530122080203 ) ) ;
#37182=CARTESIAN_POINT ( 'NONE',  ( -18.00000000000012079, -2.379036618888197285, 30.90682066428292885 ) ) ;
#37183=B_SPLINE_CURVE_WITH_KNOTS ( 'NONE', 3,
 ( #20597, #338, #27802, #40884, #75117, #20166, #87761, #40006, #46301, #68347 ),
 .UNSPECIFIED., .F., .F.,
 ( 4, 2, 2, 2, 4 ),
 ( 0.0007817359430256333669, 0.0009771253907250056474, 0.001172514838424370881, 0.001367904286123736331, 0.001563293733823101564 ),
 .UNSPECIFIED. ) ;
#37186=ORIENTED_EDGE ( 'NONE', *, *, #43900, .T. ) ;
#37187=B_SPLINE_CURVE_WITH_KNOTS ( 'NONE', 3,
 ( #53446, #73747, #87710, #47132, #12911, #58876, #25982, #24648, #66069, #52996 ),
 .UNSPECIFIED., .F., .F.,
 ( 4, 2, 2, 2, 4 ),
 ( 0.0007817359430256360774, 0.0009771253907250041296, 0.001172514838424371965, 0.001367904286123740017, 0.001563293733823108069 ),
 .UNSPECIFIED. ) ;
#37189=CARTESIAN_POINT ( 'NONE',  ( -5.749945688361685292, -5.728107161865375829, 34.42597550085002922 ) ) ;
#37190=CIRCLE ( 'NONE', #51568, 2.000000000000001776 ) ;
#37191=CARTESIAN_POINT ( 'NONE',  ( 3.230769230769231726, -5.557115091759785130, 34.35708131394839171 ) ) ;
#37192=CARTESIAN_POINT ( 'NONE',  ( -15.29685161012936767, -10.67929555188718460, 33.92786785259543336 ) ) ;
#37193=CARTESIAN_POINT ( 'NONE',  ( 4.219914504848592429, -3.513871655860379306, 32.76840700105978499 ) ) ;
#37194=CARTESIAN_POINT ( 'NONE',  ( 17.86930853333243618, -8.999036380462719364, 34.52022231692819076 ) ) ;
#37195=ORIENTED_EDGE ( 'NONE', *, *, #48700, .F. ) ;
#37196=CARTESIAN_POINT ( 'NONE',  ( 6.923076923076924238, -1.466349020453238561, 30.81389545987213907 ) ) ;
#37197=VECTOR ( 'NONE', #70284, 1000.000000000000227 ) ;
#37198=ORIENTED_EDGE ( 'NONE', *, *, #28435, .T. ) ;
#37199=EDGE_LOOP ( 'NONE', ( #16625, #88319, #31932, #47705 ) ) ;
#37201=EDGE_CURVE ( 'NONE', #58674, #22482, #19054, .T. ) ;
#37202=CARTESIAN_POINT ( 'NONE',  ( 18.06525513951284267, -2.379036618887895305, 30.90682066428158592 ) ) ;
#37203=CARTESIAN_POINT ( 'NONE',  ( 17.07692307692307665, -1.466349020453238561, 30.81389545987213907 ) ) ;
#37204=CARTESIAN_POINT ( 'NONE',  ( -16.37677237136229991, -4.186968288167451036, 33.49512374952580274 ) ) ;
#37205=EDGE_CURVE ( 'NONE', #85285, #88692, #75990, .T. ) ;
#37206=CARTESIAN_POINT ( 'NONE',  ( 11.31497661389720655, -10.97335522853832579, 33.68706563782419749 ) ) ;
#37207=EDGE_CURVE ( 'NONE', #74314, #68579, #87848, .T. ) ;
#37208=CARTESIAN_POINT ( 'NONE',  ( -6.923076923076922462, -1.044019251281081972, 31.83374038241031911 ) ) ;
#37209=ORIENTED_EDGE ( 'NONE', *, *, #5978, .T. ) ;
#37210=VERTEX_POINT ( 'NONE', #32730 ) ;
#37212=ORIENTED_EDGE ( 'NONE', *, *, #15160, .F. ) ;
#37213=CARTESIAN_POINT ( 'NONE',  ( -2.530618525208453651, -2.758268499246657068, 31.33685645148949561 ) ) ;
#37214=ORIENTED_EDGE ( 'NONE', *, *, #73661, .F. ) ;
#37215=ADVANCED_FACE ( 'NONE', ( #31400 ), #66061, .F. ) ;
#37216=CARTESIAN_POINT ( 'NONE',  ( -6.989160334032801458, -12.37446782046654192, 30.86335684631486487 ) ) ;
#37217=LINE ( 'NONE', #64681, #63309 ) ;
#37218=CARTESIAN_POINT ( 'NONE',  ( 9.692307692307695177, -9.819645486525091727, 36.12317359536749706 ) ) ;
#37219=EDGE_LOOP ( 'NONE', ( #45677, #54017, #18605, #75552, #40994, #87303, #36800, #28324 ) ) ;
#37220=ADVANCED_FACE ( 'NONE', ( #17892 ), #65612, .T. ) ;
#37221=CARTESIAN_POINT ( 'NONE',  ( -11.28846153846153655, -7.500000000000001776, 35.04278698407183867 ) ) ;
#37222=ORIENTED_EDGE ( 'NONE', *, *, #759, .F. ) ;
#37223=CARTESIAN_POINT ( 'NONE',  ( -10.68065461594093435, -5.094484230520674117, 34.41647553114621161 ) ) ;
#37224=CARTESIAN_POINT ( 'NONE',  ( 17.99999999999987566, -12.70778746994576025, 30.41441678777401236 ) ) ;
#37226=CARTESIAN_POINT ( 'NONE',  ( -18.00000000000000000, -13.49681301100524244, 30.80739993210377392 ) ) ;
#37227=CARTESIAN_POINT ( 'NONE',  ( 4.946231610255517275, -3.062553014421049546, 32.05460306192773601 ) ) ;
#37228=CARTESIAN_POINT ( 'NONE',  ( -8.769230769230768274, -1.790695186598648903, 34.54067556320373455 ) ) ;
#37230=VERTEX_POINT ( 'NONE', #73279 ) ;
#37231=CARTESIAN_POINT ( 'NONE',  ( 5.076923076922953193, -4.320704448113951379, 33.92786785259630022 ) ) ;
#37232=ORIENTED_EDGE ( 'NONE', *, *, #80169, .F. ) ;
#37233=CARTESIAN_POINT ( 'NONE',  ( 11.40831356872984870, -12.15440758774515473, 32.17923288041532004 ) ) ;
#37235=DIRECTION ( 'NONE',  ( -0.000000000000000000, 1.000000000000000000, 3.491481338843133355E-15 ) ) ;
#37236=CARTESIAN_POINT ( 'NONE',  ( 2.242422307135989890, -5.941354392334500467, 34.76329471203369792 ) ) ;
#37237=CARTESIAN_POINT ( 'NONE',  ( -0.3962828902624366822, -12.46129190930001052, 30.37095296980870174 ) ) ;
#37239=FACE_BOUND ( 'NONE', #85860, .T. ) ;
#37240=CARTESIAN_POINT ( 'NONE',  ( -11.53846153846153655, -13.57706302396349152, 30.56769352161908060 ) ) ;
#37241=CARTESIAN_POINT ( 'NONE',  ( 1.449870955891410906, -2.625532179533470067, 30.86335684631491105 ) ) ;
#37242=CYLINDRICAL_SURFACE ( 'NONE', #5099, 0.2500000000000009437 ) ;
#37243=CARTESIAN_POINT ( 'NONE',  ( -3.007757879156381264, -11.76359900205217457, 32.36225158514719880 ) ) ;
#37244=CARTESIAN_POINT ( 'NONE',  ( 9.942362003946010773, -4.235687564193448829, 33.53795663066793509 ) ) ;
#37245=CARTESIAN_POINT ( 'NONE',  ( 2.307692307692309264, -4.786620604624113540, 33.94971097300155094 ) ) ;
#37247=EDGE_CURVE ( 'NONE', #48006, #14278, #35161, .T. ) ;
#37248=ORIENTED_EDGE ( 'NONE', *, *, #73615, .T. ) ;
#37249=AXIS2_PLACEMENT_3D ( 'NONE', #3747, #37527, #45624 ) ;
#37250=CARTESIAN_POINT ( 'NONE',  ( -7.912237257109724808, -11.16473453929635440, 33.15142922261925662 ) ) ;
#37251=EDGE_CURVE ( 'NONE', #78822, #33344, #86369, .T. ) ;
#37252=B_SPLINE_CURVE_WITH_KNOTS ( 'NONE', 3,
 ( #58850, #86356, #71474, #10235, #2568, #78689, #9781, #72807, #22848, #37693 ),
 .UNSPECIFIED., .F., .F.,
 ( 4, 2, 2, 2, 4 ),
 ( 0.000000000000000000, 0.0001954339857564079352, 0.0003908679715128158703, 0.0005863019572692237513, 0.0007817359430256317406 ),
 .UNSPECIFIED. ) ;
#37253=CARTESIAN_POINT ( 'NONE',  ( 8.769230769230768274, -6.343179335718451384, 34.87096338111211935 ) ) ;
#37254=CARTESIAN_POINT ( 'NONE',  ( -9.442253380669374252, -9.148310452688876993, 34.47095581063188519 ) ) ;
#37255=CARTESIAN_POINT ( 'NONE',  ( -9.915233909823836456, -10.61292498521070549, 33.66303323003028680 ) ) ;
#37256=CARTESIAN_POINT ( 'NONE',  ( 3.361294932532794988, -6.852161475712352789, 34.70806712695775786 ) ) ;
#37257=CARTESIAN_POINT ( 'NONE',  ( -9.692307692307691624, -4.098570777380720287, 33.41473453929634729 ) ) ;
#37259=CARTESIAN_POINT ( 'NONE',  ( -11.28846153846160050, -7.565270000091922853, 34.99999999999999289 ) ) ;
#37260=DIRECTION ( 'NONE',  ( -0.000000000000000000, 1.000000000000000000, -0.000000000000000000 ) ) ;
#37261=VECTOR ( 'NONE', #10075, 1000.000000000000227 ) ;
#37262=EDGE_CURVE ( 'NONE', #66893, #72317, #71677, .T. ) ;
#37263=DIRECTION ( 'NONE',  ( -0.000000000000000000, -0.000000000000000000, -1.000000000000000000 ) ) ;
#37264=CARTESIAN_POINT ( 'NONE',  ( 10.54930223602447903, -6.343179335718451384, 34.87096338111212646 ) ) ;
#37266=DIRECTION ( 'NONE',  ( -0.000000000000000000, 0.5000000000000011102, -0.8660254037844381525 ) ) ;
#37267=VECTOR ( 'NONE', #65075, 1000.000000000000000 ) ;
#37268=B_SPLINE_CURVE_WITH_KNOTS ( 'NONE', 3,
 ( #49029, #40519, #19790, #42288, #69744, #67986, #6286, #1730, #15695, #43161 ),
 .UNSPECIFIED., .F., .F.,
 ( 4, 2, 2, 2, 4 ),
 ( 0.000000000000000000, 0.0001954311564186875792, 0.0003908623128373751583, 0.0005862934692560627103, 0.0007817246256747503166 ),
 .UNSPECIFIED. ) ;
#37269=CARTESIAN_POINT ( 'NONE',  ( -6.223484924564329113, -12.11044203135681840, 32.26167407432752299 ) ) ;
#37270=EDGE_CURVE ( 'NONE', #55151, #81591, #39064, .T. ) ;
#37272=EDGE_LOOP ( 'NONE', ( #76980, #53072, #55615, #36226 ) ) ;
#37273=DIRECTION ( 'NONE',  ( -0.000000000000000000, 0.5000000000000011102, -0.8660254037844381525 ) ) ;
#37274=CARTESIAN_POINT ( 'NONE',  ( -17.30040802064702632, -2.847400154188068910, 31.58180166144859768 ) ) ;
#37276=CARTESIAN_POINT ( 'NONE',  ( 6.923076923076800782, -5.094484230521993062, 34.41647553114689373 ) ) ;
#37277=CARTESIAN_POINT ( 'NONE',  ( -5.326899807865432379, -2.564618984488975961, 30.55390908950641915 ) ) ;
#37278=ORIENTED_EDGE ( 'NONE', *, *, #56870, .T. ) ;
#37279=CARTESIAN_POINT ( 'NONE',  ( -6.792286482109972212, -9.929761469519744921, 34.40412654351204225 ) ) ;
#37280=CARTESIAN_POINT ( 'NONE',  ( 4.088575707885377497, -6.026961402152685388, 34.52809138561120506 ) ) ;
#37282=CARTESIAN_POINT ( 'NONE',  ( -12.52762084089859407, -9.058645607665454236, 34.76329471203372634 ) ) ;
#37283=DIRECTION ( 'NONE',  ( -0.000000000000000000, 0.8660254037844399289, -0.4999999999999980016 ) ) ;
#37284=EDGE_CURVE ( 'NONE', #78742, #72334, #55581, .T. ) ;
#37285=CARTESIAN_POINT ( 'NONE',  ( -8.638705067467203236, -2.619367082507849442, 30.83698974864643461 ) ) ;
#37286=DIRECTION ( 'NONE',  ( -0.000000000000000000, 0.9848077530122086864, -0.1736481776669273891 ) ) ;
#37287=VERTEX_POINT ( 'NONE', #40828 ) ;
#37288=LINE ( 'NONE', #56686, #131 ) ;
#37289=EDGE_CURVE ( 'NONE', #20449, #20445, #42165, .T. ) ;
#37292=B_SPLINE_CURVE_WITH_KNOTS ( 'NONE', 3,
 ( #68556, #68127, #19927, #81202, #33452, #6427, #7309, #54591, #61790, #14057 ),
 .UNSPECIFIED., .F., .F.,
 ( 4, 2, 2, 2, 4 ),
 ( 0.0007817359430256339090, 0.0009771253907250065148, 0.001172514838424371965, 0.001367904286123737632, 0.001563293733823103299 ),
 .UNSPECIFIED. ) ;
#37293=CARTESIAN_POINT ( 'NONE',  ( -1.318547033612945896, -5.557115091759786019, 34.35708131394839882 ) ) ;
#37294=ORIENTED_EDGE ( 'NONE', *, *, #9784, .F. ) ;
#37295=EDGE_LOOP ( 'NONE', ( #31078, #30381 ) ) ;
#37296=EDGE_CURVE ( 'NONE', #60879, #24900, #66257, .T. ) ;
#37297=ORIENTED_EDGE ( 'NONE', *, *, #28018, .F. ) ;
#37298=CARTESIAN_POINT ( 'NONE',  ( 3.453548899747296730, -2.353885683473778023, 30.79025554430704759 ) ) ;
#37299=CARTESIAN_POINT ( 'NONE',  ( -8.769230769230890843, -3.300289026999228881, 32.46337939537708905 ) ) ;
#37300=CARTESIAN_POINT ( 'NONE',  ( 3.230769230769231726, -12.62096338111211580, 30.90682066428153263 ) ) ;
#37301=FACE_OUTER_BOUND ( 'NONE', #12171, .T. ) ;
#37302=ORIENTED_EDGE ( 'NONE', *, *, #48133, .F. ) ;
#37303=VERTEX_POINT ( 'NONE', #88597 ) ;
#37304=CARTESIAN_POINT ( 'NONE',  ( 11.76147438255493327, -11.43677907613344757, 33.22367315496202167 ) ) ;
#37305=EDGE_LOOP ( 'NONE', ( #30662, #81778, #62134, #72119 ) ) ;
#37306=CARTESIAN_POINT ( 'NONE',  ( 9.757563263583717728, -12.46129190930001052, 30.37095296980870174 ) ) ;
#37308=VECTOR ( 'NONE', #8420, 1000.000000000000227 ) ;
#37309=CARTESIAN_POINT ( 'NONE',  ( 10.36536137809165403, -11.37209801155882793, 32.91403422569033665 ) ) ;
#37310=CARTESIAN_POINT ( 'NONE',  ( 16.15384615384615330, -11.35647404775217417, 33.31231777344666511 ) ) ;
#37311=VERTEX_POINT ( 'NONE', #81820 ) ;
#37312=VECTOR ( 'NONE', #10917, 1000.000000000000000 ) ;
#37313=VERTEX_POINT ( 'NONE', #82708 ) ;
#37314=DIRECTION ( 'NONE',  ( -0.000000000000000000, 0.8660254037844399289, -0.4999999999999980016 ) ) ;
#37315=ORIENTED_EDGE ( 'NONE', *, *, #86831, .T. ) ;
#37316=ADVANCED_FACE ( 'NONE', ( #76376 ), #27308, .F. ) ;
#37317=VECTOR ( 'NONE', #15370, 1000.000000000000000 ) ;
#37319=CARTESIAN_POINT ( 'NONE',  ( -16.08777780284371417, -3.513871655860379306, 32.76840700105978499 ) ) ;
#37320=ORIENTED_EDGE ( 'NONE', *, *, #89058, .F. ) ;
#37321=DIRECTION ( 'NONE',  ( -0.000000000000000000, 0.9848077530122086864, -0.1736481776669273891 ) ) ;
#37322=CARTESIAN_POINT ( 'NONE',  ( -14.30769230769242917, -12.70778746994576025, 30.41441678777401236 ) ) ;
#37323=ADVANCED_FACE ( 'NONE', ( #40394 ), #56108, .F. ) ;
#37324=CARTESIAN_POINT ( 'NONE',  ( -8.835313148590907772, -11.91647553114624181, 32.58852847137148245 ) ) ;
#37325=FACE_BOUND ( 'NONE', #637, .T. ) ;
#37326=CARTESIAN_POINT ( 'NONE',  ( 8.096208266067295156, -12.41089969410671223, 31.60739465890703670 ) ) ;
#37327=CARTESIAN_POINT ( 'NONE',  ( 4.087763774486016466, -2.292212530054419606, 30.41441678777542634 ) ) ;
#37328=CARTESIAN_POINT ( 'NONE',  ( 13.38461538461538680, -10.51840700105979565, 33.73612834413961536 ) ) ;
#37329=CARTESIAN_POINT ( 'NONE',  ( 16.28463659481311154, -3.957578996910245284, 33.62503395064540257 ) ) ;
#37330=CARTESIAN_POINT ( 'NONE',  ( 6.857806477116148436, -11.94971097300153140, 32.03036669348370680 ) ) ;
#37332=FACE_OUTER_BOUND ( 'NONE', #27124, .T. ) ;
#37333=VERTEX_POINT ( 'NONE', #48011 ) ;
#37334=FACE_OUTER_BOUND ( 'NONE', #66091, .T. ) ;
#37335=ORIENTED_EDGE ( 'NONE', *, *, #30482, .F. ) ;
#37336=ORIENTED_EDGE ( 'NONE', *, *, #82986, .T. ) ;
#37337=CARTESIAN_POINT ( 'NONE',  ( 8.769230769230768274, -8.164416787775445883, 34.95778746994557906 ) ) ;
#37338=CARTESIAN_POINT ( 'NONE',  ( 10.86533002476265786, -12.07971442181322352, 32.31769673815850297 ) ) ;
#37339=EDGE_CURVE ( 'NONE', #44873, #88199, #14743, .T. ) ;
#37340=CARTESIAN_POINT ( 'NONE',  ( 2.530703659305157949, -2.554770724473667709, 30.48948780036025852 ) ) ;
#37341=CARTESIAN_POINT ( 'NONE',  ( -5.076923076923075762, -12.62096338111211580, 30.90682066428153263 ) ) ;
#37342=CARTESIAN_POINT ( 'NONE',  ( -9.692307692307691624, -11.11383981884818262, 36.00935417666054406 ) ) ;
#37343=CARTESIAN_POINT ( 'NONE',  ( 1.253923917947830091, -11.71456829005830080, 32.44064028649416542 ) ) ;
#37344=ORIENTED_EDGE ( 'NONE', *, *, #62613, .F. ) ;
#37345=CARTESIAN_POINT ( 'NONE',  ( 4.219913487196229163, -4.661471528628508665, 34.16647553114624003 ) ) ;
#37346=CARTESIAN_POINT ( 'NONE',  ( 14.08476534878545650, -12.64616026154729411, 30.79003144601914244 ) ) ;
#37348=CYLINDRICAL_SURFACE ( 'NONE', #13717, 0.2499999999999973355 ) ;
#37349=DIRECTION ( 'NONE',  ( -0.000000000000000000, 0.9396926207859092051, -0.3420201433256662704 ) ) ;
#37354=EDGE_LOOP ( 'NONE', ( #4640, #56393 ) ) ;
#37355=CARTESIAN_POINT ( 'NONE',  ( 14.24242230713598900, -12.51329471203370325, 31.30864560766548976 ) ) ;
#37356=EDGE_CURVE ( 'NONE', #17504, #48285, #72797, .T. ) ;
#37357=ORIENTED_EDGE ( 'NONE', *, *, #50321, .T. ) ;
#37358=CARTESIAN_POINT ( 'NONE',  ( -6.923076923077044142, -2.625532179533778709, 30.86335684631627174 ) ) ;
#37359=CARTESIAN_POINT ( 'NONE',  ( -1.384615384615383471, -9.905515769479276145, 34.41647553114623292 ) ) ;
#37360=FACE_OUTER_BOUND ( 'NONE', #7343, .T. ) ;
#37361=DIRECTION ( 'NONE',  ( -0.000000000000000000, 0.7660444431189791237, -0.6427876096865379196 ) ) ;
#37364=VERTEX_POINT ( 'NONE', #14236 ) ;
#37365=CARTESIAN_POINT ( 'NONE',  ( 4.153846153846030731, -12.51329471203414379, 31.30864560766407578 ) ) ;
#37366=CARTESIAN_POINT ( 'NONE',  ( -2.057637887778853703, -12.65882529074907126, 30.72640787790839312 ) ) ;
#37367=VERTEX_POINT ( 'NONE', #6153 ) ;
#37368=DIRECTION ( 'NONE',  ( -0.000000000000000000, 0.7660444431189791237, -0.6427876096865379196 ) ) ;
#37369=DIRECTION ( 'NONE',  ( 0.000000000000000000, -6.938893903907222067E-15, 1.000000000000000000 ) ) ;
#37370=CARTESIAN_POINT ( 'NONE',  ( -3.230769230769229949, -9.905515769479276145, 34.41647553114623292 ) ) ;
#37371=CARTESIAN_POINT ( 'NONE',  ( 6.923076923076800782, -3.643525952248796163, 33.31231777344771672 ) ) ;
#37372=CARTESIAN_POINT ( 'NONE',  ( -6.250023237292966272, -10.05641848906368097, 34.04755513067966177 ) ) ;
#37373=EDGE_CURVE ( 'NONE', #58562, #44876, #79191, .T. ) ;
#37374=CARTESIAN_POINT ( 'NONE',  ( -4.377331097570100304, -9.331801661448606566, 34.40259984581193464 ) ) ;
#37375=CARTESIAN_POINT ( 'NONE',  ( -8.069638789877792817, -12.44517049084099725, 30.48991314939691932 ) ) ;
#37377=ORIENTED_EDGE ( 'NONE', *, *, #18067, .T. ) ;
#37378=CARTESIAN_POINT ( 'NONE',  ( -4.284537620513710010, -4.809359713505814149, 33.96456829005828837 ) ) ;
#37379=LINE ( 'NONE', #51311, #67627 ) ;
#37380=CARTESIAN_POINT ( 'NONE',  ( -1.161602540521987859, -3.395485233115138168, 33.02377354290276656 ) ) ;
#37383=AXIS2_PLACEMENT_3D ( 'NONE', #38779, #85633, #18068 ) ;
#37384=DIRECTION ( 'NONE',  ( -0.000000000000000000, -0.5000000000000009992, -0.8660254037844380415 ) ) ;
#37385=CARTESIAN_POINT ( 'NONE',  ( 8.519254025182176449, -10.06842814019191401, 34.32929386961144758 ) ) ;
#37386=VERTEX_POINT ( 'NONE', #57876 ) ;
#37388=CARTESIAN_POINT ( 'NONE',  ( -15.36145983387954139, -3.957541250942358424, 33.62499894934981626 ) ) ;
#37390=EDGE_CURVE ( 'NONE', #8057, #17639, #68501, .T. ) ;
#37391=EDGE_LOOP ( 'NONE', ( #62018, #33050, #19406, #45651 ) ) ;
#37392=AXIS2_PLACEMENT_3D ( 'NONE', #67155, #33804, #5457 ) ;
#37393=CARTESIAN_POINT ( 'NONE',  ( -4.284536756956459413, -8.191372820521381826, 34.95448215188423546 ) ) ;
#37394=VECTOR ( 'NONE', #14152, 1000.000000000000227 ) ;
#37395=EDGE_LOOP ( 'NONE', ( #1735, #80715, #32349, #13544, #2681, #3082 ) ) ;
#37396=CARTESIAN_POINT ( 'NONE',  ( -13.38461538461538325, -2.517432740324522911, 35.29906147534542527 ) ) ;
#37397=EDGE_CURVE ( 'NONE', #44468, #54188, #30845, .T. ) ;
#37398=ADVANCED_FACE ( 'NONE', ( #43039 ), #16894, .F. ) ;
#37399=CARTESIAN_POINT ( 'NONE',  ( -0.4615384615384611200, -6.435427911321262684, 35.78748833219616898 ) ) ;
#37400=CYLINDRICAL_SURFACE ( 'NONE', #2451, 0.2499999999999993616 ) ;
#37402=DIRECTION ( 'NONE',  ( 0.000000000000000000, 0.1736481776669275834, 0.9848077530122086864 ) ) ;
#37403=ORIENTED_EDGE ( 'NONE', *, *, #72075, .T. ) ;
#37404=DIRECTION ( 'NONE',  ( -0.000000000000000000, 0.3420201433256694901, -0.9396926207859082059 ) ) ;
#37405=ORIENTED_EDGE ( 'NONE', *, *, #45747, .F. ) ;
#37406=CARTESIAN_POINT ( 'NONE',  ( 18.00000000000000000, -9.819645486525091727, 36.12317359536749706 ) ) ;
#37407=CARTESIAN_POINT ( 'NONE',  ( 2.373760658694747061, -3.050289026998446840, 32.03036669348366416 ) ) ;
#37408=VERTEX_POINT ( 'NONE', #71384 ) ;
#37409=CARTESIAN_POINT ( 'NONE',  ( -5.999999999999998224, -10.67929555188718282, 33.92786785259544047 ) ) ;
#37410=DIRECTION ( 'NONE',  ( -0.000000000000000000, 0.1736481776669307198, -0.9848077530122080203 ) ) ;
#37411=CARTESIAN_POINT ( 'NONE',  ( -1.384615384615383471, -9.058645607665452459, 34.76329471203371924 ) ) ;
#37412=CYLINDRICAL_SURFACE ( 'NONE', #67933, 0.2499999999999979738 ) ;
#37413=DIRECTION ( 'NONE',  ( 0.000000000000000000, 0.000000000000000000, 1.000000000000000000 ) ) ;
#37414=ORIENTED_EDGE ( 'NONE', *, *, #4863, .T. ) ;
#37415=VERTEX_POINT ( 'NONE', #57429 ) ;
#37416=FACE_BOUND ( 'NONE', #3620, .T. ) ;
#37417=EDGE_LOOP ( 'NONE', ( #32621, #36571 ) ) ;
#37418=CARTESIAN_POINT ( 'NONE',  ( 15.10062202133100939, -12.45813303252208648, 30.39737893381572675 ) ) ;
#37419=ORIENTED_EDGE ( 'NONE', *, *, #37284, .F. ) ;
#37421=B_SPLINE_CURVE_WITH_KNOTS ( 'NONE', 3,
 ( #79420, #24903, #51463, #65883, #43847, #58244, #3744, #11396, #38879, #17260 ),
 .UNSPECIFIED., .F., .F.,
 ( 4, 2, 2, 2, 4 ),
 ( 0.000000000000000000, 0.0001954339857564081520, 0.0003908679715128163040, 0.0005863019572692244018, 0.0007817359430256326080 ),
 .UNSPECIFIED. ) ;
#37422=CARTESIAN_POINT ( 'NONE',  ( 6.065255139512839122, -3.083524468853784839, 32.58852847137153930 ) ) ;
#37423=CARTESIAN_POINT ( 'NONE',  ( 5.142178648199100088, -4.481592998940251427, 33.73612834413965089 ) ) ;
#37424=ORIENTED_EDGE ( 'NONE', *, *, #19517, .T. ) ;
#37425=ORIENTED_EDGE ( 'NONE', *, *, #62093, .F. ) ;
#37426=ORIENTED_EDGE ( 'NONE', *, *, #38683, .F. ) ;
#37427=CARTESIAN_POINT ( 'NONE',  ( 17.01083966596719321, -4.098570777380720287, 33.41473453929634729 ) ) ;
#37428=ORIENTED_EDGE ( 'NONE', *, *, #23564, .T. ) ;
#37429=CARTESIAN_POINT ( 'NONE',  ( 11.53846153846141753, -11.48612834414049644, 32.76840700105863391 ) ) ;
#37430=CARTESIAN_POINT ( 'NONE',  ( -11.53846153846153655, -3.513871655860378418, 32.76840700105978499 ) ) ;
#37433=FACE_BOUND ( 'NONE', #17421, .T. ) ;
#37434=ORIENTED_EDGE ( 'NONE', *, *, #13168, .F. ) ;
#37435=CARTESIAN_POINT ( 'NONE',  ( 13.51540719244018263, -8.999086150933475636, 34.52020707165672775 ) ) ;
#37437=AXIS2_PLACEMENT_3D ( 'NONE', #17531, #24726, #72461 ) ;
#37438=CARTESIAN_POINT ( 'NONE',  ( 5.010840697562940704, -3.322132147404559976, 32.92929555188719348 ) ) ;
#37439=FACE_OUTER_BOUND ( 'NONE', #39876, .T. ) ;
#37440=DIRECTION ( 'NONE',  ( -0.000000000000000000, -0.6427876096865404731, -0.7660444431189771253 ) ) ;
#37441=ORIENTED_EDGE ( 'NONE', *, *, #86303, .F. ) ;
#37442=CARTESIAN_POINT ( 'NONE',  ( -6.923076923076922462, -6.386643153685126251, 34.62446782046654192 ) ) ;
#37443=ORIENTED_EDGE ( 'NONE', *, *, #1182, .T. ) ;
#37444=AXIS2_PLACEMENT_3D ( 'NONE', #63410, #83709, #35956 ) ;
#37445=ORIENTED_EDGE ( 'NONE', *, *, #48241, .T. ) ;
#37446=AXIS2_PLACEMENT_3D ( 'NONE', #44084, #84667, #15758 ) ;
#37447=CARTESIAN_POINT ( 'NONE',  ( -18.25000000000000711, -2.249999999999999556, 29.81919447696817471 ) ) ;
#37448=CARTESIAN_POINT ( 'NONE',  ( -9.469294848214296678, -8.282913670948747864, 34.94150082978203642 ) ) ;
#37450=CARTESIAN_POINT ( 'NONE',  ( -8.769230769230892619, -12.51329471203414379, 31.30864560766407578 ) ) ;
#37451=DIRECTION ( 'NONE',  ( -0.000000000000000000, -0.3420201433256694346, -0.9396926207859080948 ) ) ;
#37453=CARTESIAN_POINT ( 'NONE',  ( 14.24160992833217065, -2.833524468853757305, 32.15551576947924417 ) ) ;
#37454=ORIENTED_EDGE ( 'NONE', *, *, #5138, .T. ) ;
#37455=CARTESIAN_POINT ( 'NONE',  ( 6.673100179028335077, -2.544273027872574922, 31.48422191005632342 ) ) ;
#37456=CARTESIAN_POINT ( 'NONE',  ( -0.4615384615385840772, -3.643525952248795718, 33.31231777344771672 ) ) ;
#37457=CARTESIAN_POINT ( 'NONE',  ( 4.219101725122178514, -9.442884908240271713, 34.35708131394835618 ) ) ;
#37458=CARTESIAN_POINT ( 'NONE',  ( 10.68064018666063930, -11.94971097300157403, 32.03036669348361443 ) ) ;
#37459=EDGE_LOOP ( 'NONE', ( #46898, #75628 ) ) ;
#37460=B_SPLINE_CURVE_WITH_KNOTS ( 'NONE', 3,
 ( #62758, #41623, #76735, #54676, #54234, #15040, #13264, #83503, #6512, #55568 ),
 .UNSPECIFIED., .F., .F.,
 ( 4, 2, 2, 2, 4 ),
 ( 0.000000000000000000, 0.0001954311564186868744, 0.0003908623128373737488, 0.0005862934692560606504, 0.0007817246256747474977 ),
 .UNSPECIFIED. ) ;
#37461=EDGE_LOOP ( 'NONE', ( #62439, #419, #69940, #61278 ) ) ;
#37462=FACE_BOUND ( 'NONE', #12801, .T. ) ;
#37463=EDGE_CURVE ( 'NONE', #25475, #37415, #71833, .T. ) ;
#37464=ORIENTED_EDGE ( 'NONE', *, *, #26069, .T. ) ;
#37465=CARTESIAN_POINT ( 'NONE',  ( 18.22296290356148418, -7.369474270740072441, 34.74850911626239736 ) ) ;
#37466=CARTESIAN_POINT ( 'NONE',  ( -13.25382357679060519, -10.54018710029568595, 33.71981072465678864 ) ) ;
#37467=VERTEX_POINT ( 'NONE', #44346 ) ;
#37468=FACE_OUTER_BOUND ( 'NONE', #81884, .T. ) ;
#37469=CARTESIAN_POINT ( 'NONE',  ( -10.86540785267757947, -6.695914987888146541, 34.68535235679833306 ) ) ;
#37471=FACE_OUTER_BOUND ( 'NONE', #31054, .T. ) ;
#37472=ORIENTED_EDGE ( 'NONE', *, *, #79490, .F. ) ;
#37473=CARTESIAN_POINT ( 'NONE',  ( -7.846153846153844924, -8.120952969808772792, 34.71129190930000163 ) ) ;
#37475=CARTESIAN_POINT ( 'NONE',  ( -20.74999999999999645, -10.50000000000000000, 29.75000000000000355 ) ) ;
#37476=ORIENTED_EDGE ( 'NONE', *, *, #59107, .F. ) ;
#37477=DIRECTION ( 'NONE',  ( -0.000000000000000000, -0.3420201433256694901, -0.9396926207859082059 ) ) ;
#37478=CARTESIAN_POINT ( 'NONE',  ( 3.930919936330005360, -6.503392248772476236, 34.64988816332204635 ) ) ;
#37479=CARTESIAN_POINT ( 'NONE',  ( 11.53846153846153832, -13.37000171582298513, 34.34916445242398453 ) ) ;
#37480=CARTESIAN_POINT ( 'NONE',  ( -12.33101275977490019, -2.882268652242222284, 31.66798894389554064 ) ) ;
#37482=ADVANCED_FACE ( 'NONE', ( #29531 ), #43481, .F. ) ;
#37483=CARTESIAN_POINT ( 'NONE',  ( 0.4615384615383396616, -6.879047030192662504, 34.71129190930017927 ) ) ;
#37484=VECTOR ( 'NONE', #34185, 1000.000000000000000 ) ;
#37486=VERTEX_POINT ( 'NONE', #23206 ) ;
#37487=CARTESIAN_POINT ( 'NONE',  ( -15.00775787915638304, -3.587049720035815348, 32.86302985866382897 ) ) ;
#37488=CARTESIAN_POINT ( 'NONE',  ( 13.13461538461538680, -7.433932668274256805, 35.00000000000000711 ) ) ;
#37489=EDGE_LOOP ( 'NONE', ( #52799, #59010 ) ) ;
#37490=ORIENTED_EDGE ( 'NONE', *, *, #67558, .T. ) ;
#37491=CARTESIAN_POINT ( 'NONE',  ( -11.66915300512909504, -10.54014554554150607, 33.71984207302941883 ) ) ;
#37494=B_SPLINE_CURVE_WITH_KNOTS ( 'NONE', 3,
 ( #7223, #61703, #26603, #68041, #22, #46869, #40574, #6346, #74352, #33801 ),
 .UNSPECIFIED., .F., .F.,
 ( 4, 2, 2, 2, 4 ),
 ( 0.000000000000000000, 0.0001954311564186863052, 0.0003908623128373726104, 0.0005862934692560589156, 0.0007817246256747452209 ),
 .UNSPECIFIED. ) ;
#37495=CARTESIAN_POINT ( 'NONE',  ( 9.561616225640136690, -12.38065189839062263, 30.83690757178629482 ) ) ;
#37496=LINE ( 'NONE', #58211, #56044 ) ;
#37498=CARTESIAN_POINT ( 'NONE',  ( 0.4615384615387756462, -2.255955759149395501, 30.00000000000324363 ) ) ;
#37499=ORIENTED_EDGE ( 'NONE', *, *, #3194, .T. ) ;
#37500=DIRECTION ( 'NONE',  ( -0.000000000000000000, -0.9396926207859092051, -0.3420201433256662704 ) ) ;
#37501=EDGE_CURVE ( 'NONE', #87990, #51727, #21116, .T. ) ;
#37505=CARTESIAN_POINT ( 'NONE',  ( 3.903846153846154632, -7.500000000000001776, 35.00000000000000000 ) ) ;
#37506=CARTESIAN_POINT ( 'NONE',  ( 2.241608896736428047, -3.513871655860377086, 32.76840700105978499 ) ) ;
#37507=ORIENTED_EDGE ( 'NONE', *, *, #26506, .F. ) ;
#37511=ORIENTED_EDGE ( 'NONE', *, *, #61056, .F. ) ;
#37512=EDGE_CURVE ( 'NONE', #38908, #6875, #22245, .T. ) ;
#37513=CARTESIAN_POINT ( 'NONE',  ( 0.6843180028068702736, -9.332535724633405749, 34.40230450496446224 ) ) ;
#37514=CARTESIAN_POINT ( 'NONE',  ( -1.384615384615383471, -8.973038597847269315, 34.52809138561121927 ) ) ;
#37515=CARTESIAN_POINT ( 'NONE',  ( -3.230769230769229949, -8.564572088678739092, 35.78748833219616898 ) ) ;
#37516=ORIENTED_EDGE ( 'NONE', *, *, #87452, .T. ) ;
#37518=CARTESIAN_POINT ( 'NONE',  ( 10.39189967166066531, -3.754499324213721234, 33.06261337010820256 ) ) ;
#37520=CARTESIAN_POINT ( 'NONE',  ( 14.30769230769231015, -11.91647553114624181, 32.58852847137148245 ) ) ;
#37521=CARTESIAN_POINT ( 'NONE',  ( 8.900022577055558770, -4.118422570099828484, 33.43335022499816489 ) ) ;
#37522=ORIENTED_EDGE ( 'NONE', *, *, #35769, .F. ) ;
#37523=CARTESIAN_POINT ( 'NONE',  ( 18.00000000000000000, -11.16473453929635440, 33.15142922261926373 ) ) ;
#37524=ORIENTED_EDGE ( 'NONE', *, *, #73588, .T. ) ;
#37526=CARTESIAN_POINT ( 'NONE',  ( -16.85414340794500276, -3.563462043263029955, 33.22394488606062879 ) ) ;
#37527=DIRECTION ( 'NONE',  ( -0.000000000000000000, 0.7660444431189791237, -0.6427876096865379196 ) ) ;
#37528=CARTESIAN_POINT ( 'NONE',  ( -14.17690049986752321, -9.804649428959608670, 34.18742332936588468 ) ) ;
#37529=CARTESIAN_POINT ( 'NONE',  ( 14.98079249982687777, -11.79746400365624659, 32.30657167506340954 ) ) ;
#37530=ORIENTED_EDGE ( 'NONE', *, *, #55584, .F. ) ;
#37531=ORIENTED_EDGE ( 'NONE', *, *, #87442, .T. ) ;
#37532=B_SPLINE_CURVE_WITH_KNOTS ( 'NONE', 3,
 ( #4113, #86107, #24833, #39708, #66268, #4572, #52305, #32047, #45105, #79796 ),
 .UNSPECIFIED., .F., .F.,
 ( 4, 2, 2, 2, 4 ),
 ( 0.0007817246256747511840, 0.0009771112852218952725, 0.001172497944769039470, 0.001367884604316183667, 0.001563271263863327864 ),
 .UNSPECIFIED. ) ;
#37533=AXIS2_PLACEMENT_3D ( 'NONE', #27116, #75739, #28911 ) ;
#37534=VERTEX_POINT ( 'NONE', #72721 ) ;
#37535=VERTEX_POINT ( 'NONE', #86264 ) ;
#37536=CARTESIAN_POINT ( 'NONE',  ( 12.68431800280686694, -11.89424750095246175, 32.13594075562310337 ) ) ;
#37537=CARTESIAN_POINT ( 'NONE',  ( 15.93036122928182330, -5.827078755546626354, 34.72654668319379567 ) ) ;
#37538=VECTOR ( 'NONE', #83003, 1000.000000000000000 ) ;
#37539=CARTESIAN_POINT ( 'NONE',  ( -4.153846153846274980, -6.835583212225970762, 34.95778746994575670 ) ) ;
#37540=CARTESIAN_POINT ( 'NONE',  ( -4.153846153846152411, -2.833524468853757305, 32.15551576947925838 ) ) ;
#37541=CARTESIAN_POINT ( 'NONE',  ( -15.23076923076922995, -12.78798330534102945, 29.74999999999997868 ) ) ;
#37542=CARTESIAN_POINT ( 'NONE',  ( 8.519207531937803779, -9.271318131107980420, 34.42618302367067429 ) ) ;
#37543=CARTESIAN_POINT ( 'NONE',  ( -3.230769230769229949, -13.75783147151868846, 33.36296068462461051 ) ) ;
#37544=CARTESIAN_POINT ( 'NONE',  ( -17.75005448165186195, -6.696923467548661968, 34.68552623307873972 ) ) ;
#37545=ORIENTED_EDGE ( 'NONE', *, *, #25744, .T. ) ;
#37546=B_SPLINE_CURVE_WITH_KNOTS ( 'NONE', 3,
 ( #35347, #7882, #56510, #42995, #8774, #1121, #62798, #83995, #36245, #84437 ),
 .UNSPECIFIED., .F., .F.,
 ( 4, 2, 2, 2, 4 ),
 ( 0.0007817246256747464135, 0.0009771112852218900684, 0.001172497944769033615, 0.001367884604316177161, 0.001563271263863320925 ),
 .UNSPECIFIED. ) ;
#37548=B_SPLINE_CURVE_WITH_KNOTS ( 'NONE', 3,
 ( #12196, #46859, #19835, #74791, #13079, #40566, #73002, #38777, #32020, #59486 ),
 .UNSPECIFIED., .F., .F.,
 ( 4, 2, 2, 2, 4 ),
 ( 0.0007817359430256318490, 0.0009771253907249984917, 0.001172514838424365026, 0.001367904286123731560, 0.001563293733823098311 ),
 .UNSPECIFIED. ) ;
#37550=EDGE_LOOP ( 'NONE', ( #5156, #3595, #84522, #72761 ) ) ;
#37551=CARTESIAN_POINT ( 'NONE',  ( 11.76124120743959978, -2.612705202774698421, 31.66806509827799943 ) ) ;
#37552=ORIENTED_EDGE ( 'NONE', *, *, #11397, .T. ) ;
#37553=B_SPLINE_CURVE_WITH_KNOTS ( 'NONE', 3,
 ( #38644, #66102, #31893, #66563, #44488, #30549, #59353, #50801, #37748, #65216 ),
 .UNSPECIFIED., .F., .F.,
 ( 4, 2, 2, 2, 4 ),
 ( 0.0007817246256747464135, 0.0009771112852218900684, 0.001172497944769033615, 0.001367884604316177161, 0.001563271263863320925 ),
 .UNSPECIFIED. ) ;
#37554=CARTESIAN_POINT ( 'NONE',  ( 16.21910172512217585, -11.94971097300157403, 32.03036669348361443 ) ) ;
#37555=DIRECTION ( 'NONE',  ( 0.000000000000000000, 0.8660254037844377084, -0.5000000000000015543 ) ) ;
#37556=CARTESIAN_POINT ( 'NONE',  ( 9.019230769232203571, -7.500000000000155431, 34.75000000000007105 ) ) ;
#37557=CARTESIAN_POINT ( 'NONE',  ( -14.30769230769230660, -9.780366693483667717, 34.19971097300155094 ) ) ;
#37559=AXIS2_PLACEMENT_3D ( 'NONE', #46474, #13135, #32506 ) ;
#37560=ORIENTED_EDGE ( 'NONE', *, *, #46847, .T. ) ;
#37561=CYLINDRICAL_SURFACE ( 'NONE', #28463, 0.2499999999999986955 ) ;
#37562=EDGE_LOOP ( 'NONE', ( #29258, #44529 ) ) ;
#37563=FACE_BOUND ( 'NONE', #3274, .T. ) ;
#37564=CARTESIAN_POINT ( 'NONE',  ( 13.38461538461526423, -12.51329471203414379, 31.30864560766407578 ) ) ;
#37565=VECTOR ( 'NONE', #61706, 1000.000000000000114 ) ;
#37566=EDGE_CURVE ( 'NONE', #83933, #74576, #65520, .T. ) ;
#37567=CARTESIAN_POINT ( 'NONE',  ( 16.02369894440793630, -6.852621066184266141, 34.70813303252209181 ) ) ;
#37568=ORIENTED_EDGE ( 'NONE', *, *, #27883, .T. ) ;
#37569=CARTESIAN_POINT ( 'NONE',  ( -15.16551365949320562, -12.27809138561124591, 31.22303859784720359 ) ) ;
#37570=CARTESIAN_POINT ( 'NONE',  ( 3.453548772037641434, -3.236590943229497253, 32.36255958852954251 ) ) ;
#37571=CARTESIAN_POINT ( 'NONE',  ( 2.307692307692186251, -11.67786785259630911, 32.92929555188603530 ) ) ;
#37572=EDGE_LOOP ( 'NONE', ( #71749, #86713, #34714, #84624 ) ) ;
#37573=EDGE_CURVE ( 'NONE', #2295, #52380, #58766, .T. ) ;
#37574=DIRECTION ( 'NONE',  ( 0.000000000000000000, 0.1736481776669267785, -0.9848077530122087975 ) ) ;
#37575=DIRECTION ( 'NONE',  ( -0.000000000000000000, 0.5000000000000011102, -0.8660254037844381525 ) ) ;
#37577=VECTOR ( 'NONE', #12451, 1000.000000000000114 ) ;
#37578=DIRECTION ( 'NONE',  ( -0.000000000000000000, 0.9848077530122086864, -0.1736481776669273891 ) ) ;
#37579=CARTESIAN_POINT ( 'NONE',  ( -9.626240358957616650, -9.058645607665452459, 34.76329471203371924 ) ) ;
#37580=EDGE_LOOP ( 'NONE', ( #28928, #2635, #68212, #88300 ) ) ;
#37581=CARTESIAN_POINT ( 'NONE',  ( -13.38461538461538325, -12.78798330534102945, 29.74999999999997868 ) ) ;
#37582=CARTESIAN_POINT ( 'NONE',  ( 10.61538461538461675, -2.708943851104267164, 35.45975837776705220 ) ) ;
#37584=CARTESIAN_POINT ( 'NONE',  ( 15.23076923076910916, -12.70778746994576025, 30.41441678777401236 ) ) ;
#37585=CARTESIAN_POINT ( 'NONE',  ( 9.561617089197389063, -12.35290016733513951, 31.75349464988449455 ) ) ;
#37586=FACE_BOUND ( 'NONE', #53475, .T. ) ;
#37587=CARTESIAN_POINT ( 'NONE',  ( 4.403900465484466231, -12.17597550085003633, 31.52189283813461884 ) ) ;
#37588=LINE ( 'NONE', #51082, #60402 ) ;
#37589=EDGE_CURVE ( 'NONE', #14975, #60707, #34036, .T. ) ;
#37590=CARTESIAN_POINT ( 'NONE',  ( -1.134560964701931018, -9.233818618650603938, 34.70587769442853698 ) ) ;
#37591=CARTESIAN_POINT ( 'NONE',  ( 12.71153846153840128, -7.565270000091922853, 34.99999999999999289 ) ) ;
#37592=CARTESIAN_POINT ( 'NONE',  ( -10.68146802634049308, -8.120952969808774569, 34.71129190930000163 ) ) ;
#37593=LINE ( 'NONE', #70499, #5972 ) ;
#37595=VERTEX_POINT ( 'NONE', #24089 ) ;
#37596=B_SPLINE_CURVE_WITH_KNOTS ( 'NONE', 3,
 ( #47941, #6530, #82191, #34434, #19154, #20480, #67783, #80872, #41199, #46622 ),
 .UNSPECIFIED., .F., .F.,
 ( 4, 2, 2, 2, 4 ),
 ( 0.0007817246256747484735, 0.0009771112852218922368, 0.001172497944769036217, 0.001367884604316180197, 0.001563271263863323960 ),
 .UNSPECIFIED. ) ;
#37597=CARTESIAN_POINT ( 'NONE',  ( 18.06606835100244268, -11.69971097300155272, 32.46337939537588113 ) ) ;
#37598=ORIENTED_EDGE ( 'NONE', *, *, #48048, .T. ) ;
#37600=CARTESIAN_POINT ( 'NONE',  ( 4.153846153846154188, -1.044019251281081972, 31.83374038241031911 ) ) ;
#37602=DIRECTION ( 'NONE',  ( 0.000000000000000000, 0.8660254037844377084, -0.5000000000000015543 ) ) ;
#37603=ORIENTED_EDGE ( 'NONE', *, *, #47212, .T. ) ;
#37604=CARTESIAN_POINT ( 'NONE',  ( -7.912237257109728361, -5.557115091759785130, 34.35708131394839171 ) ) ;
#37606=CARTESIAN_POINT ( 'NONE',  ( 3.100078627658923391, -2.295517848115769421, 30.44137282052137294 ) ) ;
#37607=B_SPLINE_CURVE_WITH_KNOTS ( 'NONE', 3,
 ( #19673, #8279, #2379, #49695, #50129, #22228, #67863, #35753, #12917, #63202 ),
 .UNSPECIFIED., .F., .F.,
 ( 4, 2, 2, 2, 4 ),
 ( 0.0007817359430256257775, 0.0009771253907249911191, 0.001172514838424356352, 0.001367904286123721586, 0.001563293733823086819 ),
 .UNSPECIFIED. ) ;
#37608=CARTESIAN_POINT ( 'NONE',  ( -9.758390071667825794, -12.62096338111211580, 30.90682066428152908 ) ) ;
#37609=CARTESIAN_POINT ( 'NONE',  ( -5.869208192175211281, -8.999086150933472084, 34.52020707165672064 ) ) ;
#37610=CARTESIAN_POINT ( 'NONE',  ( -12.39547112818838670, -3.937682226553329556, 33.60647404775216529 ) ) ;
#37611=CARTESIAN_POINT ( 'NONE',  ( -23.00000000000000000, -5.499999999999981348, 27.75000000000000000 ) ) ;
#37612=CARTESIAN_POINT ( 'NONE',  ( -39.05038313613820122, -2.499999999999999556, 29.75000000000000355 ) ) ;
#37613=CARTESIAN_POINT ( 'NONE',  ( 5.869852790561781219, -4.460286881179643004, 33.72017969459903242 ) ) ;
#37614=AXIS2_PLACEMENT_3D ( 'NONE', #49973, #69810, #8117 ) ;
#37616=CARTESIAN_POINT ( 'NONE',  ( 1.134592147322419420, -2.823816976329317718, 31.52131813110795733 ) ) ;
#37618=EDGE_CURVE ( 'NONE', #87573, #20844, #13619, .T. ) ;
#37619=EDGE_CURVE ( 'NONE', #23459, #46284, #82397, .T. ) ;
#37620=CIRCLE ( 'NONE', #66356, 0.2500000000000002220 ) ;
#37621=CARTESIAN_POINT ( 'NONE',  ( 13.63466969625370240, -4.235687564193448829, 33.53795663066793509 ) ) ;
#37623=VERTEX_POINT ( 'NONE', #4724 ) ;
#37624=EDGE_CURVE ( 'NONE', #32743, #73490, #9316, .T. ) ;
#37625=CARTESIAN_POINT ( 'NONE',  ( 14.53070365930516061, -4.887748414852792322, 34.01359900205216746 ) ) ;
#37626=CARTESIAN_POINT ( 'NONE',  ( 4.153846153846154188, -9.819645486525091727, 36.12317359536749706 ) ) ;
#37627=CARTESIAN_POINT ( 'NONE',  ( 1.254467414883692289, -5.915902021225892149, 34.75552854090298638 ) ) ;
#37628=CARTESIAN_POINT ( 'NONE',  ( 5.076923076922954969, -2.892918686052165622, 31.69288490824153470 ) ) ;
#37629=EDGE_CURVE ( 'NONE', #60953, #23257, #53340, .T. ) ;
#37630=CARTESIAN_POINT ( 'NONE',  ( 8.519207531937803779, -11.86270091957321249, 32.19358267280087915 ) ) ;
#37631=CARTESIAN_POINT ( 'NONE',  ( -3.100243792535585463, -5.915461855592777596, 34.75538340440931506 ) ) ;
#37632=VERTEX_POINT ( 'NONE', #74073 ) ;
#37633=CARTESIAN_POINT ( 'NONE',  ( 7.716005876422148191, -3.069018819979302926, 32.56621877034667278 ) ) ;
#37634=EDGE_LOOP ( 'NONE', ( #88544, #51579, #57718, #13834 ) ) ;
#37635=EDGE_LOOP ( 'NONE', ( #71973, #29237 ) ) ;
#37636=AXIS2_PLACEMENT_3D ( 'NONE', #75904, #14204, #71796 ) ;
#37637=CARTESIAN_POINT ( 'NONE',  ( -9.469294848214296678, -2.889357225399414197, 32.26129605718031002 ) ) ;
#37638=CARTESIAN_POINT ( 'NONE',  ( -6.223484924564330889, -12.69144148231606017, 30.53333754910549303 ) ) ;
#37639=CARTESIAN_POINT ( 'NONE',  ( -9.019253993452226226, -2.341070481393819236, 30.72580821765574299 ) ) ;
#37640=DIRECTION ( 'NONE',  ( -0.000000000000000000, 0.7660444431189791237, -0.6427876096865379196 ) ) ;
#37641=CARTESIAN_POINT ( 'NONE',  ( 13.13459216039392885, -5.765609946408404518, 34.70566812827425451 ) ) ;
#37642=AXIS2_PLACEMENT_3D ( 'NONE', #29981, #9702, #4279 ) ;
#37643=ORIENTED_EDGE ( 'NONE', *, *, #33119, .F. ) ;
#37644=CARTESIAN_POINT ( 'NONE',  ( 8.992010310499178871, -3.755027918224367767, 33.06320215134714857 ) ) ;
#37645=ORIENTED_EDGE ( 'NONE', *, *, #8544, .T. ) ;
#37646=EDGE_CURVE ( 'NONE', #72317, #66893, #11559, .T. ) ;
#37647=ORIENTED_EDGE ( 'NONE', *, *, #88787, .F. ) ;
#37648=CARTESIAN_POINT ( 'NONE',  ( 13.31934538405906565, -5.094484230520674117, 34.41647553114621161 ) ) ;
#37650=ADVANCED_FACE ( 'NONE', ( #34842 ), #19559, .F. ) ;
#37652=EDGE_CURVE ( 'NONE', #58112, #54935, #47913, .T. ) ;
#37653=CARTESIAN_POINT ( 'NONE',  ( -8.638440328263820689, -9.929761469519743144, 34.40412654351204225 ) ) ;
#37654=CARTESIAN_POINT ( 'NONE',  ( -4.284537620513711786, -8.147922237126337563, 34.70805685702651999 ) ) ;
#37655=CARTESIAN_POINT ( 'NONE',  ( -16.08777780284371772, -2.721908614388772740, 31.22303859784725333 ) ) ;
#37656=ORIENTED_EDGE ( 'NONE', *, *, #2297, .F. ) ;
#37659=B_SPLINE_CURVE_WITH_KNOTS ( 'NONE', 3,
 ( #23285, #42689, #8460, #11449, #84567, #29184, #38933, #16529, #77789, #43559 ),
 .UNSPECIFIED., .F., .F.,
 ( 4, 2, 2, 2, 4 ),
 ( 0.000000000000000000, 0.0001954339857564097512, 0.0003908679715128195024, 0.0005863019572692292807, 0.0007817359430256390048 ),
 .UNSPECIFIED. ) ;
#37660=EDGE_CURVE ( 'NONE', #14030, #72338, #58581, .T. ) ;
#37661=EDGE_LOOP ( 'NONE', ( #39248, #82719, #24835, #69557 ) ) ;
#37663=VERTEX_POINT ( 'NONE', #625 ) ;
#37664=CARTESIAN_POINT ( 'NONE',  ( 7.846153846153846700, -12.37446782046654192, 30.86335684631486131 ) ) ;
#37666=VECTOR ( 'NONE', #88900, 1000.000000000000114 ) ;
#37667=B_SPLINE_CURVE_WITH_KNOTS ( 'NONE', 3,
 ( #3483, #77817, #43590, #85469, #16560, #2594, #44026, #23315, #64735, #71498 ),
 .UNSPECIFIED., .F., .F.,
 ( 4, 2, 2, 2, 4 ),
 ( 0.0007817246256747469556, 0.0009771112852218889842, 0.001172497944769031013, 0.001367884604316173041, 0.001563271263863315070 ),
 .UNSPECIFIED. ) ;
#37669=EDGE_LOOP ( 'NONE', ( #44140, #71236, #7256, #1354 ) ) ;
#37671=FACE_OUTER_BOUND ( 'NONE', #61107, .T. ) ;
#37672=VERTEX_POINT ( 'NONE', #26763 ) ;
#37673=CARTESIAN_POINT ( 'NONE',  ( -9.019253993452222673, -4.931416488878822335, 34.32920672191015399 ) ) ;
#37674=CARTESIAN_POINT ( 'NONE',  ( 17.93391762063986050, -12.62096338111211580, 30.90682066428152908 ) ) ;
#37675=DIRECTION ( 'NONE',  ( 0.000000000000000000, 0.1736481776669267785, -0.9848077530122087975 ) ) ;
#37676=DIRECTION ( 'NONE',  ( -0.000000000000000000, 0.9848077530122086864, -0.1736481776669273891 ) ) ;
#37677=CARTESIAN_POINT ( 'NONE',  ( -39.05038313613820122, -2.499999999999999556, 29.75000000000000355 ) ) ;
#37678=CARTESIAN_POINT ( 'NONE',  ( -1.134669975237340811, -8.476813868363244353, 34.90874843262270133 ) ) ;
#37680=VERTEX_POINT ( 'NONE', #6056 ) ;
#37682=CARTESIAN_POINT ( 'NONE',  ( 11.28846153846152411, -2.249999999999998668, 29.81609741502487765 ) ) ;
#37685=DIRECTION ( 'NONE',  ( -0.000000000000000000, -0.8660254037844399289, -0.4999999999999980016 ) ) ;
#37686=CARTESIAN_POINT ( 'NONE',  ( 16.85343815235874487, -10.97335522853832934, 33.68706563782419749 ) ) ;
#37687=DIRECTION ( 'NONE',  ( -0.000000000000000000, 0.6427876096865404731, -0.7660444431189771253 ) ) ;
#37688=CARTESIAN_POINT ( 'NONE',  ( -16.21911615440247090, -12.16647553114622049, 32.15551576947930812 ) ) ;
#37689=CARTESIAN_POINT ( 'NONE',  ( 12.21151522424549896, -4.335965774309649134, 33.62209801155881905 ) ) ;
#37690=FACE_BOUND ( 'NONE', #11967, .T. ) ;
#37691=CARTESIAN_POINT ( 'NONE',  ( 13.31853197365950692, -12.10708131394839349, 31.69288490824020244 ) ) ;
#37692=CARTESIAN_POINT ( 'NONE',  ( -10.86538461538461320, -7.433932668274256805, 35.00000000000000711 ) ) ;
#37693=CARTESIAN_POINT ( 'NONE',  ( 16.15384615384603251, -3.300289026999228437, 32.46337939537709616 ) ) ;
#37694=CARTESIAN_POINT ( 'NONE',  ( -1.134561072977069873, -12.17597550085003455, 31.52189283813461884 ) ) ;
#37695=DIRECTION ( 'NONE',  ( 0.000000000000000000, 0.000000000000000000, -1.000000000000000000 ) ) ;
#37696=FACE_OUTER_BOUND ( 'NONE', #73248, .T. ) ;
#37697=CARTESIAN_POINT ( 'NONE',  ( 9.019176287578909879, -10.76462480002816235, 33.53768742498949962 ) ) ;
#37700=ORIENTED_EDGE ( 'NONE', *, *, #86722, .F. ) ;
#37701=VECTOR ( 'NONE', #75638, 1000.000000000000114 ) ;
#37702=CARTESIAN_POINT ( 'NONE',  ( -15.23076923076935074, -11.48612834414049644, 32.76840700105863391 ) ) ;
#37703=CARTESIAN_POINT ( 'NONE',  ( 5.076923076922953193, -3.083524468854526912, 32.58852847137268327 ) ) ;
#37705=LINE ( 'NONE', #16547, #66873 ) ;
#37706=CARTESIAN_POINT ( 'NONE',  ( 7.622668902429897919, -5.113361153441932316, 34.14387501736621999 ) ) ;
#37707=CARTESIAN_POINT ( 'NONE',  ( 3.230769230769231726, -11.11383981884818262, 36.00935417666054406 ) ) ;
#37710=CARTESIAN_POINT ( 'NONE',  ( -11.60378445395371472, -7.749976743299138882, 34.99404534957040624 ) ) ;
#37711=CARTESIAN_POINT ( 'NONE',  ( 0.7115927731767749398, -3.627508038966689163, 32.91356715214248396 ) ) ;
#37712=CARTESIAN_POINT ( 'NONE',  ( -7.596208436775802930, -10.18230066228895758, 34.26354781536631577 ) ) ;
#37713=CARTESIAN_POINT ( 'NONE',  ( 9.468822767743363400, -4.225889041578353655, 33.85425143139329407 ) ) ;
#37714=CARTESIAN_POINT ( 'NONE',  ( 14.30769230769231015, -5.557115091759785130, 34.35708131394839171 ) ) ;
#37715=DIRECTION ( 'NONE',  ( 0.000000000000000000, 0.6427876096865368094, 0.7660444431189802339 ) ) ;
#37717=EDGE_CURVE ( 'NONE', #26721, #40093, #20007, .T. ) ;
#37718=EDGE_CURVE ( 'NONE', #49073, #43765, #43604, .T. ) ;
#37719=CARTESIAN_POINT ( 'NONE',  ( 8.096208157792160520, -6.567000820036036579, 34.66262288849541306 ) ) ;
#37720=ORIENTED_EDGE ( 'NONE', *, *, #73500, .T. ) ;
#37721=CARTESIAN_POINT ( 'NONE',  ( 15.10062126103753322, -11.66186481527757302, 32.95055677023626117 ) ) ;
#37722=CARTESIAN_POINT ( 'NONE',  ( 1.384615384615386802, -6.189225973068211317, 35.74407628777942847 ) ) ;
#37724=ADVANCED_FACE ( 'NONE', ( #48354 ), #14133, .F. ) ;
#37725=CARTESIAN_POINT ( 'NONE',  ( 6.130791807824788719, -4.118422570099827595, 33.43335022499816489 ) ) ;
#37726=CARTESIAN_POINT ( 'NONE',  ( 3.230769230769110045, -11.94971097300221174, 32.03036669348237098 ) ) ;
#37727=ORIENTED_EDGE ( 'NONE', *, *, #59902, .T. ) ;
#37728=CARTESIAN_POINT ( 'NONE',  ( -6.700297254098854793, -10.23759521482555357, 34.22997729860117033 ) ) ;
#37729=CARTESIAN_POINT ( 'NONE',  ( 2.373759641042385127, -10.67929555188718282, 33.92786785259544757 ) ) ;
#37730=CARTESIAN_POINT ( 'NONE',  ( 12.23805351781451201, -5.912607949931405926, 34.49155766932282319 ) ) ;
#37731=ORIENTED_EDGE ( 'NONE', *, *, #36008, .F. ) ;
#37732=CARTESIAN_POINT ( 'NONE',  ( 11.53846153846153832, -4.661471528628507777, 34.16647553114623292 ) ) ;
#37733=CARTESIAN_POINT ( 'NONE',  ( -16.15384615384615330, -9.819645486525091727, 36.12317359536749706 ) ) ;
#37734=ADVANCED_FACE ( 'NONE', ( #28092 ), #83044, .F. ) ;
#37735=B_SPLINE_CURVE_WITH_KNOTS ( 'NONE', 3,
 ( #8760, #75877, #28585, #36230, #41656, #29475 ),
 .UNSPECIFIED., .F., .F.,
 ( 4, 2, 4 ),
 ( 4.220987180333914613E-17, 0.0001954756301637168027, 0.0003909512603273914300 ),
 .UNSPECIFIED. ) ;
#37736=LINE ( 'NONE', #17023, #1767 ) ;
#37737=CARTESIAN_POINT ( 'NONE',  ( -15.48076923076923528, -2.249999999999999556, 29.81609741502490607 ) ) ;
#37738=ORIENTED_EDGE ( 'NONE', *, *, #5852, .F. ) ;
#37739=VECTOR ( 'NONE', #54765, 1000.000000000000000 ) ;
#37740=DIRECTION ( 'NONE',  ( -0.000000000000000000, 0.9848077530122085754, -0.1736481776669273613 ) ) ;
#37742=DIRECTION ( 'NONE',  ( -0.000000000000000000, 0.9396926207859092051, -0.3420201433256662704 ) ) ;
#37743=ORIENTED_EDGE ( 'NONE', *, *, #26142, .F. ) ;
#37744=ORIENTED_EDGE ( 'NONE', *, *, #13391, .F. ) ;
#37745=EDGE_CURVE ( 'NONE', #22022, #55623, #33076, .T. ) ;
#37746=ORIENTED_EDGE ( 'NONE', *, *, #986, .T. ) ;
#37747=CARTESIAN_POINT ( 'NONE',  ( -18.25002323729296805, -3.711651800289232028, 33.01384336483935300 ) ) ;
#37748=CARTESIAN_POINT ( 'NONE',  ( 9.758375025657770152, -3.937682226553329556, 33.60647404775216529 ) ) ;
#37749=EDGE_CURVE ( 'NONE', #8847, #82664, #30673, .T. ) ;
#37750=CARTESIAN_POINT ( 'NONE',  ( -3.931066484868085187, -12.69155399931963046, 30.53255429739158444 ) ) ;
#37752=EDGE_CURVE ( 'NONE', #77905, #48531, #80146, .T. ) ;
#37753=ORIENTED_EDGE ( 'NONE', *, *, #23163, .F. ) ;
#37755=CARTESIAN_POINT ( 'NONE',  ( 10.86538461538461675, -2.249999999999998668, 29.75000000000000355 ) ) ;
#37756=EDGE_LOOP ( 'NONE', ( #66016, #49371 ) ) ;
#37757=EDGE_CURVE ( 'NONE', #26530, #81582, #49688, .T. ) ;
#37758=CARTESIAN_POINT ( 'NONE',  ( 9.942253210655836781, -12.43552623307873972, 30.55307653245132826 ) ) ;
#37759=VECTOR ( 'NONE', #60087, 1000.000000000000114 ) ;
#37760=B_SPLINE_CURVE_WITH_KNOTS ( 'NONE', 3,
 ( #12461, #80032, #47119, #72816, #32726, #33175 ),
 .UNSPECIFIED., .F., .F.,
 ( 4, 2, 4 ),
 ( 2.453269466693398621E-17, 0.0001954756301636960945, 0.0003909512603273676860 ),
 .UNSPECIFIED. ) ;
#37761=CARTESIAN_POINT ( 'NONE',  ( -8.638438961405983108, -12.38066358083363738, 30.83685684665853444 ) ) ;
#37762=CARTESIAN_POINT ( 'NONE',  ( 13.44987052412822237, -10.33852847137154107, 34.16647553114620450 ) ) ;
#37763=ORIENTED_EDGE ( 'NONE', *, *, #14946, .F. ) ;
#37764=B_SPLINE_CURVE_WITH_KNOTS ( 'NONE', 3,
 ( #12149, #33306, #25654, #38722, #47249, #66183, #67977, #31971, #59435, #58984 ),
 .UNSPECIFIED., .F., .F.,
 ( 4, 2, 2, 2, 4 ),
 ( 0.000000000000000000, 0.0001954311564186882026, 0.0003908623128373764051, 0.0005862934692560646619, 0.0007817246256747528103 ),
 .UNSPECIFIED. ) ;
#37765=ORIENTED_EDGE ( 'NONE', *, *, #57673, .T. ) ;
#37766=EDGE_CURVE ( 'NONE', #82473, #48855, #84826, .T. ) ;
#37767=VERTEX_POINT ( 'NONE', #69960 ) ;
#37768=CARTESIAN_POINT ( 'NONE',  ( 15.23076923076923173, -2.538708090699994813, 30.37095296980875503 ) ) ;
#37769=ORIENTED_EDGE ( 'NONE', *, *, #2281, .T. ) ;
#37770=CARTESIAN_POINT ( 'NONE',  ( -0.4615384615384611200, -10.51840700105979565, 33.73612834413961536 ) ) ;
#37771=CARTESIAN_POINT ( 'NONE',  ( -5.142193522883852452, -10.21337939537584383, 33.94971097300158647 ) ) ;
#37772=ORIENTED_EDGE ( 'NONE', *, *, #23238, .F. ) ;
#37773=EDGE_CURVE ( 'NONE', #4310, #61816, #75837, .T. ) ;
#37774=DIRECTION ( 'NONE',  ( 0.000000000000000000, 0.6427876096865373645, -0.7660444431189797898 ) ) ;
#37775=CARTESIAN_POINT ( 'NONE',  ( 10.61538461538461675, -5.471508081941601098, 34.59228464037088457 ) ) ;
#37776=DIRECTION ( 'NONE',  ( -0.000000000000000000, 0.9848077530122085754, -0.1736481776669273613 ) ) ;
#37777=FACE_BOUND ( 'NONE', #11740, .T. ) ;
#37778=CARTESIAN_POINT ( 'NONE',  ( -0.7115616988314267255, -4.335965774309649134, 33.62209801155881905 ) ) ;
#37779=CARTESIAN_POINT ( 'NONE',  ( 9.758476833270350426, -7.250054483168843156, 34.74374881642865631 ) ) ;
#37780=DIRECTION ( 'NONE',  ( -0.000000000000000000, -0.1736481776669307198, -0.9848077530122080203 ) ) ;
#37781=CARTESIAN_POINT ( 'NONE',  ( 6.250000000000000888, -2.499999999999998668, 29.75000000000000355 ) ) ;
#37782=CARTESIAN_POINT ( 'NONE',  ( 6.923076923076802558, -11.94971097300221174, 32.03036669348237098 ) ) ;
#37783=CARTESIAN_POINT ( 'NONE',  ( 17.86930939688969033, -6.369640206132551441, 34.87707690430378449 ) ) ;
#37785=EDGE_LOOP ( 'NONE', ( #35151, #8471, #86766, #5728 ) ) ;
#37786=CARTESIAN_POINT ( 'NONE',  ( -5.999999999999998224, -11.69971097300155272, 32.46337939537588113 ) ) ;
#37787=ORIENTED_EDGE ( 'NONE', *, *, #33304, .F. ) ;
#37788=ADVANCED_FACE ( 'NONE', ( #42944 ), #50123, .F. ) ;
#37789=ORIENTED_EDGE ( 'NONE', *, *, #56043, .T. ) ;
#37790=CYLINDRICAL_SURFACE ( 'NONE', #37437, 0.2500000000000002220 ) ;
#37791=CARTESIAN_POINT ( 'NONE',  ( 15.23076923076910916, -3.083524468854526912, 32.58852847137268327 ) ) ;
#37792=EDGE_CURVE ( 'NONE', #33486, #5632, #34984, .T. ) ;
#37793=VECTOR ( 'NONE', #79508, 1000.000000000000114 ) ;
#37794=AXIS2_PLACEMENT_3D ( 'NONE', #320, #34982, #75103 ) ;
#37795=CARTESIAN_POINT ( 'NONE',  ( 13.13459216039392707, -11.56360843649121861, 33.07473185843129926 ) ) ;
#37796=CARTESIAN_POINT ( 'NONE',  ( 7.846153846153846700, -9.905515769479276145, 34.41647553114623292 ) ) ;
#37797=CARTESIAN_POINT ( 'NONE',  ( -4.153846153846152411, -3.322132147404559976, 32.92929555188717927 ) ) ;
#37800=CARTESIAN_POINT ( 'NONE',  ( 14.17754433796061875, -12.70455904226513866, 30.44083106164009322 ) ) ;
#37801=B_SPLINE_CURVE_WITH_KNOTS ( 'NONE', 3,
 ( #53748, #63160, #1911, #84345, #35252, #14542, #1028, #42465, #49214, #27608 ),
 .UNSPECIFIED., .F., .F.,
 ( 4, 2, 2, 2, 4 ),
 ( 0.0007817246256747461966, 0.0009771112852218892010, 0.001172497944769032314, 0.001367884604316175427, 0.001563271263863318323 ),
 .UNSPECIFIED. ) ;
#37802=CARTESIAN_POINT ( 'NONE',  ( -12.59222992820602194, -4.809359713505814149, 33.96456829005828837 ) ) ;
#37803=FACE_OUTER_BOUND ( 'NONE', #52611, .T. ) ;
#37806=ORIENTED_EDGE ( 'NONE', *, *, #53561, .F. ) ;
#37807=B_SPLINE_CURVE_WITH_KNOTS ( 'NONE', 3,
 ( #74377, #54534, #82030, #68496, #46893, #87928, #47787, #46008, #18549, #67623 ),
 .UNSPECIFIED., .F., .F.,
 ( 4, 2, 2, 2, 4 ),
 ( 0.0007817359430256285964, 0.0009771253907249945886, 0.001172514838424360472, 0.001367904286123726356, 0.001563293733823092457 ),
 .UNSPECIFIED. ) ;
#37808=EDGE_LOOP ( 'NONE', ( #27592, #42811 ) ) ;
#37809=CARTESIAN_POINT ( 'NONE',  ( -14.43784027742400689, -5.070767119584671079, 34.40440758774516183 ) ) ;
#37810=VERTEX_POINT ( 'NONE', #9582 ) ;
#37812=CARTESIAN_POINT ( 'NONE',  ( 17.93391762063986050, -11.35647404775217595, 33.31231777344666511 ) ) ;
#37813=CARTESIAN_POINT ( 'NONE',  ( -16.28453762051371356, -2.729777683071817229, 31.24903638046269450 ) ) ;
#37814=DIRECTION ( 'NONE',  ( -0.000000000000000000, 0.6427876096865404731, -0.7660444431189770143 ) ) ;
#37816=CARTESIAN_POINT ( 'NONE',  ( 1.384615384615386802, -9.905515769479276145, 34.41647553114623292 ) ) ;
#37818=CARTESIAN_POINT ( 'NONE',  ( -12.68502340526241312, -10.81261337010820256, 33.49550067578627477 ) ) ;
#37819=CARTESIAN_POINT ( 'NONE',  ( -16.40382288478850725, -11.79746400365624659, 32.30657167506340954 ) ) ;
#37821=CARTESIAN_POINT ( 'NONE',  ( -9.562260257057236146, -7.723484941389743952, 34.99544897038808955 ) ) ;
#37822=FACE_OUTER_BOUND ( 'NONE', #19504, .T. ) ;
#37823=CARTESIAN_POINT ( 'NONE',  ( -8.769230769230768274, -6.343179335718451384, 34.87096338111211935 ) ) ;
#37824=DIRECTION ( 'NONE',  ( -0.000000000000000000, 0.5000000000000011102, -0.8660254037844380415 ) ) ;
#37825=DIRECTION ( 'NONE',  ( -0.000000000000000000, -0.3420201433256694901, -0.9396926207859082059 ) ) ;
#37826=CARTESIAN_POINT ( 'NONE',  ( 9.442330948259101575, -4.818429247618089661, 34.26397095200675125 ) ) ;
#37831=CARTESIAN_POINT ( 'NONE',  ( -13.38461538461538325, -9.905515769479276145, 34.41647553114623292 ) ) ;
#37832=CARTESIAN_POINT ( 'NONE',  ( -12.46153846153858247, -11.94971097300221174, 32.03036669348237098 ) ) ;
#37836=AXIS2_PLACEMENT_3D ( 'NONE', #2427, #65011, #59154 ) ;
#37837=CARTESIAN_POINT ( 'NONE',  ( 0.3962680155776850399, -3.835265460703609186, 33.15142922261924241 ) ) ;
#37838=CARTESIAN_POINT ( 'NONE',  ( 8.545745844666440050, -10.23692288466677880, 34.23039457007281072 ) ) ;
#37839=ORIENTED_EDGE ( 'NONE', *, *, #24956, .T. ) ;
#37841=CARTESIAN_POINT ( 'NONE',  ( -1.318548051265307386, -12.34228464037088813, 31.77849191805839268 ) ) ;
#37842=EDGE_CURVE ( 'NONE', #78742, #31319, #15027, .T. ) ;
#37844=ORIENTED_EDGE ( 'NONE', *, *, #18373, .T. ) ;
#37845=B_SPLINE_CURVE_WITH_KNOTS ( 'NONE', 3,
 ( #49759, #36698, #49327, #15544, #43013, #76805, #70485, #15101, #35820, #36263 ),
 .UNSPECIFIED., .F., .F.,
 ( 4, 2, 2, 2, 4 ),
 ( 0.000000000000000000, 0.0001954339857564074473, 0.0003908679715128148945, 0.0005863019572692223418, 0.0007817359430256297891 ),
 .UNSPECIFIED. ) ;
#37846=B_SPLINE_CURVE_WITH_KNOTS ( 'NONE', 3,
 ( #11219, #44987, #18424, #12119, #53975, #67502, #5794, #38244, #58950, #66614 ),
 .UNSPECIFIED., .F., .F.,
 ( 4, 2, 2, 2, 4 ),
 ( 0.000000000000000000, 0.0001954311564186863323, 0.0003908623128373726646, 0.0005862934692560590241, 0.0007817246256747453293 ),
 .UNSPECIFIED. ) ;
#37847=CARTESIAN_POINT ( 'NONE',  ( -18.06608237936013595, -4.661471528628505112, 34.16647553114621871 ) ) ;
#37848=EDGE_CURVE ( 'NONE', #80960, #24436, #31808, .T. ) ;
#37849=ORIENTED_EDGE ( 'NONE', *, *, #50533, .F. ) ;
#37850=LINE ( 'NONE', #15375, #79418 ) ;
#37851=CARTESIAN_POINT ( 'NONE',  ( -7.715362038329056205, -11.71459661697926080, 32.44059661609675516 ) ) ;
#37852=CARTESIAN_POINT ( 'NONE',  ( 9.692307692307570832, -8.656820664282941280, 34.87096338111179961 ) ) ;
#37855=ORIENTED_EDGE ( 'NONE', *, *, #55764, .T. ) ;
#37857=CARTESIAN_POINT ( 'NONE',  ( -5.934744860487159102, -2.379036618887895305, 30.90682066428159303 ) ) ;
#37858=ORIENTED_EDGE ( 'NONE', *, *, #24115, .F. ) ;
#37859=DIRECTION ( 'NONE',  ( 0.000000000000000000, 0.9396926207859126468, 0.3420201433256571111 ) ) ;
#37860=CARTESIAN_POINT ( 'NONE',  ( 0.6843180028068690524, -11.41317474335729187, 32.86274602512330034 ) ) ;
#37861=EDGE_CURVE ( 'NONE', #38356, #35065, #8201, .T. ) ;
#37864=FACE_OUTER_BOUND ( 'NONE', #44061, .T. ) ;
#37865=CARTESIAN_POINT ( 'NONE',  ( -11.78848476268299628, -2.985938066672154445, 32.43141759479405550 ) ) ;
#37866=EDGE_CURVE ( 'NONE', #18168, #45741, #86599, .T. ) ;
#37868=DIRECTION ( 'NONE',  ( 0.000000000000000000, 1.000000000000000000, 0.000000000000000000 ) ) ;
#37869=CARTESIAN_POINT ( 'NONE',  ( -7.912236225513979981, -12.62096338111211580, 30.90682066428152908 ) ) ;
#37870=ORIENTED_EDGE ( 'NONE', *, *, #75008, .F. ) ;
#37872=ORIENTED_EDGE ( 'NONE', *, *, #4017, .T. ) ;
#37873=CARTESIAN_POINT ( 'NONE',  ( -4.023055712879202162, -8.191423895709842640, 34.95447573519442130 ) ) ;
#37874=ORIENTED_EDGE ( 'NONE', *, *, #17262, .F. ) ;
#37875=EDGE_CURVE ( 'NONE', #22236, #18827, #84457, .T. ) ;
#37876=EDGE_CURVE ( 'NONE', #41430, #60227, #2744, .T. ) ;
#37877=CARTESIAN_POINT ( 'NONE',  ( -14.30769230769230660, -10.67929555188718282, 33.92786785259544047 ) ) ;
#37878=CARTESIAN_POINT ( 'NONE',  ( 6.065255139512838234, -10.33852847137154107, 34.16647553114620450 ) ) ;
#37879=VERTEX_POINT ( 'NONE', #30737 ) ;
#37880=VERTEX_POINT ( 'NONE', #25769 ) ;
#37882=CARTESIAN_POINT ( 'NONE',  ( 16.85399685940691938, -4.186968288167451036, 33.49512374952580274 ) ) ;
#37883=EDGE_LOOP ( 'NONE', ( #26912, #82090 ) ) ;
#37884=B_SPLINE_CURVE_WITH_KNOTS ( 'NONE', 3,
 ( #74711, #82352, #12998, #53980, #60287, #87799, #74261, #40483, #67948, #6251 ),
 .UNSPECIFIED., .F., .F.,
 ( 4, 2, 2, 2, 4 ),
 ( 0.000000000000000000, 0.0001954311564186872810, 0.0003908623128373745620, 0.0005862934692560618430, 0.0007817246256747491240 ),
 .UNSPECIFIED. ) ;
#37886=VECTOR ( 'NONE', #49515, 1000.000000000000227 ) ;
#37887=EDGE_CURVE ( 'NONE', #72513, #4656, #19013, .T. ) ;
#37888=EDGE_CURVE ( 'NONE', #39612, #80371, #3868, .T. ) ;
#37889=CARTESIAN_POINT ( 'NONE',  ( -11.66915300512910214, -3.530157926970578952, 32.79014554554150607 ) ) ;
#37890=CARTESIAN_POINT ( 'NONE',  ( -15.93083330975275658, -10.77377354290276301, 33.85451476688484718 ) ) ;
#37891=FACE_BOUND ( 'NONE', #18393, .T. ) ;
#37892=ORIENTED_EDGE ( 'NONE', *, *, #60697, .F. ) ;
#37893=DIRECTION ( 'NONE',  ( 0.000000000000000000, 0.000000000000000000, 1.000000000000000000 ) ) ;
#37894=CARTESIAN_POINT ( 'NONE',  ( 13.51514108637895006, -9.417988943895561960, 34.36773134775777550 ) ) ;
#37895=CARTESIAN_POINT ( 'NONE',  ( -4.153846153846273204, -2.892918686052165622, 31.69288490824153470 ) ) ;
#37897=CARTESIAN_POINT ( 'NONE',  ( 13.38461538461538680, -1.242168528481310874, 33.36296068462461051 ) ) ;
#37898=ORIENTED_EDGE ( 'NONE', *, *, #82981, .F. ) ;
#37899=DIRECTION ( 'NONE',  ( -0.000000000000000000, -0.000000000000000000, -1.000000000000000000 ) ) ;
#37900=B_SPLINE_CURVE_WITH_KNOTS ( 'NONE', 3,
 ( #71611, #84272, #78817, #9918, #58101, #8604, #50018, #23859, #63082, #36078 ),
 .UNSPECIFIED., .F., .F.,
 ( 4, 2, 2, 2, 4 ),
 ( 0.000000000000000000, 0.0001954311564186878502, 0.0003908623128373757004, 0.0005862934692560635777, 0.0007817246256747514008 ),
 .UNSPECIFIED. ) ;
#37901=EDGE_LOOP ( 'NONE', ( #81983, #42092, #33419, #42914 ) ) ;
#37902=ADVANCED_FACE ( 'NONE', ( #39296 ), #85696, .F. ) ;
#37903=ORIENTED_EDGE ( 'NONE', *, *, #61255, .F. ) ;
#37904=DIRECTION ( 'NONE',  ( -0.000000000000000000, -0.9396926207859092051, -0.3420201433256662704 ) ) ;
#37905=CARTESIAN_POINT ( 'NONE',  ( -1.608100309179714360, -5.827078755546626354, 34.72654668319379567 ) ) ;
#37906=CARTESIAN_POINT ( 'NONE',  ( -10.86540785267757947, -12.22074536777954989, 31.39888409691088356 ) ) ;
#37907=CARTESIAN_POINT ( 'NONE',  ( -13.63459212866397685, -2.920706130388546651, 32.31842814019191223 ) ) ;
#37908=ADVANCED_FACE ( 'NONE', ( #64960 ), #23974, .F. ) ;
#37910=CARTESIAN_POINT ( 'NONE',  ( 14.08420738312797482, -3.019605429927184392, 32.48692288466676814 ) ) ;
#37912=ORIENTED_EDGE ( 'NONE', *, *, #69690, .T. ) ;
#37913=CARTESIAN_POINT ( 'NONE',  ( 6.700149964170075023, -2.523278758544489797, 31.42238647778637528 ) ) ;
#37915=CARTESIAN_POINT ( 'NONE',  ( 10.55011416942384095, -3.300289026998414865, 32.46337939537583139 ) ) ;
#37916=CARTESIAN_POINT ( 'NONE',  ( -13.44988538517170440, -12.70778746994557551, 30.41441678777548319 ) ) ;
#37918=EDGE_CURVE ( 'NONE', #49110, #12728, #65121, .T. ) ;
#37919=ORIENTED_EDGE ( 'NONE', *, *, #85776, .F. ) ;
#37920=FACE_BOUND ( 'NONE', #1893, .T. ) ;
#37921=VERTEX_POINT ( 'NONE', #41061 ) ;
#37922=CARTESIAN_POINT ( 'NONE',  ( 11.53846153846141576, -12.51329471203414379, 31.30864560766407578 ) ) ;
#37923=CARTESIAN_POINT ( 'NONE',  ( -8.769230769230768274, -5.415277668671390821, 36.20867863119892149 ) ) ;
#37924=VERTEX_POINT ( 'NONE', #520 ) ;
#37925=CARTESIAN_POINT ( 'NONE',  ( -3.230769230769229949, -12.37446782046654192, 30.86335684631486131 ) ) ;
#37926=CARTESIAN_POINT ( 'NONE',  ( -2.307692307692305711, -4.098570777380720287, 33.41473453929634729 ) ) ;
#37927=CARTESIAN_POINT ( 'NONE',  ( 0.5276068125408989173, -12.10708131394839704, 31.69288490824020954 ) ) ;
#37928=CARTESIAN_POINT ( 'NONE',  ( -1.318548051265309162, -3.937682226553329556, 33.60647404775216529 ) ) ;
#37929=EDGE_LOOP ( 'NONE', ( #35900, #21003, #22834, #13108 ) ) ;
#37930=CARTESIAN_POINT ( 'NONE',  ( -17.07692307692307665, -6.435427911321262684, 35.78748833219616898 ) ) ;
#37932=VERTEX_POINT ( 'NONE', #12701 ) ;
#37934=EDGE_LOOP ( 'NONE', ( #72147, #60571 ) ) ;
#37935=CARTESIAN_POINT ( 'NONE',  ( -8.703162418228330921, -9.780366693483667717, 34.19971097300155805 ) ) ;
#37936=CARTESIAN_POINT ( 'NONE',  ( -12.68446542044531178, -2.889293201056495786, 32.26117774369186009 ) ) ;
#37937=FACE_OUTER_BOUND ( 'NONE', #39266, .T. ) ;
#37938=DIRECTION ( 'NONE',  ( -0.000000000000000000, 0.3420201433256694901, -0.9396926207859082059 ) ) ;
#37939=CARTESIAN_POINT ( 'NONE',  ( -14.53117723225663838, -8.539481045369596401, 34.89627647299170832 ) ) ;
#37940=DIRECTION ( 'NONE',  ( -0.000000000000000000, 0.3420201433256694901, -0.9396926207859082059 ) ) ;
#37942=VERTEX_POINT ( 'NONE', #61310 ) ;
#37943=B_SPLINE_CURVE_WITH_KNOTS ( 'NONE', 3,
 ( #80422, #59696, #25468, #52925, #53823, #39884, #80876, #52037, #17829, #18723 ),
 .UNSPECIFIED., .F., .F.,
 ( 4, 2, 2, 2, 4 ),
 ( 0.000000000000000000, 0.0001954311564186869286, 0.0003908623128373738573, 0.0005862934692560607588, 0.0007817246256747477145 ),
 .UNSPECIFIED. ) ;
#37944=CARTESIAN_POINT ( 'NONE',  ( 4.946775107191381693, -12.15440758774515473, 32.17923288041532004 ) ) ;
#37945=LINE ( 'NONE', #65408, #62041 ) ;
#37947=VERTEX_POINT ( 'NONE', #46914 ) ;
#37948=ORIENTED_EDGE ( 'NONE', *, *, #9223, .T. ) ;
#37949=CARTESIAN_POINT ( 'NONE',  ( -5.869209559033047974, -12.62708834333097663, 30.88030960425257021 ) ) ;
#37950=CARTESIAN_POINT ( 'NONE',  ( 7.715463243043539698, -6.369640206132550553, 34.87707690430378449 ) ) ;
#37951=CARTESIAN_POINT ( 'NONE',  ( 6.000000000000001776, -11.16473453929635440, 33.15142922261926373 ) ) ;
#37953=CARTESIAN_POINT ( 'NONE',  ( 2.307692307692309264, -5.415277668671390821, 36.20867863119892149 ) ) ;
#37954=CARTESIAN_POINT ( 'NONE',  ( -17.01166793741023753, -11.67786785259547777, 32.92929555188713664 ) ) ;
#37955=CARTESIAN_POINT ( 'NONE',  ( 5.869308533332442401, -8.147922237126337563, 34.70805685702651999 ) ) ;
#37957=CARTESIAN_POINT ( 'NONE',  ( -4.023320452082591814, -6.001044277235011215, 34.52024696741798948 ) ) ;
#37958=CARTESIAN_POINT ( 'NONE',  ( -0.3310127597748976358, -8.586989748646448817, 34.63063291749215011 ) ) ;
#37960=CARTESIAN_POINT ( 'NONE',  ( -5.776573038138430150, -7.630147231320743018, 34.74852402298682819 ) ) ;
#37961=CARTESIAN_POINT ( 'NONE',  ( 12.33139125210024289, -11.93770438780619259, 32.05411857736982029 ) ) ;
#37962=VERTEX_POINT ( 'NONE', #19453 ) ;
#37963=CARTESIAN_POINT ( 'NONE',  ( 10.48523664565292179, -9.504002272028875709, 34.60269587691767867 ) ) ;
#37964=B_SPLINE_CURVE_WITH_KNOTS ( 'NONE', 3,
 ( #23292, #56204, #50752, #21527, #15225, #78236, #21977, #16538, #63393, #69716 ),
 .UNSPECIFIED., .F., .F.,
 ( 4, 2, 2, 2, 4 ),
 ( 0.0007817246256747460882, 0.0009771112852218892010, 0.001172497944769032314, 0.001367884604316175210, 0.001563271263863318323 ),
 .UNSPECIFIED. ) ;
#37965=AXIS2_PLACEMENT_3D ( 'NONE', #48934, #58233, #21909 ) ;
#37966=VECTOR ( 'NONE', #33698, 1000.000000000000000 ) ;
#37967=ORIENTED_EDGE ( 'NONE', *, *, #82316, .F. ) ;
#37968=CARTESIAN_POINT ( 'NONE',  ( 14.98079249982687777, -11.28823185664190376, 33.01397839955799896 ) ) ;
#37970=CARTESIAN_POINT ( 'NONE',  ( 10.36540787133602493, -3.436278759898153901, 33.07459398097509506 ) ) ;
#37971=CARTESIAN_POINT ( 'NONE',  ( 15.48082365068268373, -4.818054556918156983, 34.26375889529406749 ) ) ;
#37973=CARTESIAN_POINT ( 'NONE',  ( 12.46153846153833911, -11.06231777344772027, 33.60647404775119895 ) ) ;
#37975=EDGE_CURVE ( 'NONE', #73916, #47875, #28618, .T. ) ;
#37976=CARTESIAN_POINT ( 'NONE',  ( -6.222926958906846551, -5.582147617184174848, 34.63737895849758530 ) ) ;
#37977=CARTESIAN_POINT ( 'NONE',  ( -5.011667937410237528, -8.656820664281605460, 34.87096338111211224 ) ) ;
#37979=DIRECTION ( 'NONE',  ( -0.000000000000000000, 0.8660254037844399289, -0.4999999999999980016 ) ) ;
#37982=CYLINDRICAL_SURFACE ( 'NONE', #36235, 0.2499999999999995559 ) ;
#37983=CARTESIAN_POINT ( 'NONE',  ( -16.85391023282967637, -3.395485233115139501, 33.02377354290276656 ) ) ;
#37984=LINE ( 'NONE', #11399, #24331 ) ;
#37986=CARTESIAN_POINT ( 'NONE',  ( 6.923076923076802558, -10.21337939537710326, 33.94971097300076224 ) ) ;
#37987=CARTESIAN_POINT ( 'NONE',  ( 9.442330961365339448, -8.303909089506435137, 34.68538101551103381 ) ) ;
#37992=ORIENTED_EDGE ( 'NONE', *, *, #66318, .T. ) ;
#37993=VERTEX_POINT ( 'NONE', #73 ) ;
#37994=ADVANCED_FACE ( 'NONE', ( #55019 ), #27984, .F. ) ;
#37995=CARTESIAN_POINT ( 'NONE',  ( -12.46153846153814726, -2.255955759149395501, 30.00000000000324363 ) ) ;
#37996=CARTESIAN_POINT ( 'NONE',  ( 11.47319153790521717, -9.528491918058357157, 34.59228464037090589 ) ) ;
#37997=CARTESIAN_POINT ( 'NONE',  ( -3.930833309752757021, -6.460100341425561332, 34.89618726649961644 ) ) ;
#37998=CARTESIAN_POINT ( 'NONE',  ( -18.00000000000000000, -6.682775186373817178, 35.82440484884453724 ) ) ;
#37999=CARTESIAN_POINT ( 'NONE',  ( -13.60754234352223335, -3.395401636524185474, 33.02366814457250399 ) ) ;
#38000=CARTESIAN_POINT ( 'NONE',  ( 0.5276068125408989173, -4.786620604624113540, 33.94971097300155805 ) ) ;
#38001=CARTESIAN_POINT ( 'NONE',  ( -17.74994568836168440, -9.943054286541400444, 34.11300777759954883 ) ) ;
#38002=CARTESIAN_POINT ( 'NONE',  ( -17.93474442872397034, -6.879047030191283163, 34.71129190930002295 ) ) ;
#38003=CARTESIAN_POINT ( 'NONE',  ( -4.377331097570101193, -10.11188796281391511, 34.01382737946119050 ) ) ;
#38004=ORIENTED_EDGE ( 'NONE', *, *, #5208, .T. ) ;
#38005=ORIENTED_EDGE ( 'NONE', *, *, #79497, .T. ) ;
#38006=VERTEX_POINT ( 'NONE', #88825 ) ;
#38007=CYLINDRICAL_SURFACE ( 'NONE', #18635, 0.2500000000000004996 ) ;
#38008=ORIENTED_EDGE ( 'NONE', *, *, #58741, .T. ) ;
#38009=CARTESIAN_POINT ( 'NONE',  ( -15.23076923076922995, -13.87047571288749737, 32.06866353760679544 ) ) ;
#38010=CARTESIAN_POINT ( 'NONE',  ( 1.384615384615386802, -2.538708090699994813, 30.37095296980875503 ) ) ;
#38011=B_SPLINE_CURVE_WITH_KNOTS ( 'NONE', 3,
 ( #24234, #49942, #43195, #50380, #30120, #77861, #36871, #16164, #51696, #79202 ),
 .UNSPECIFIED., .F., .F.,
 ( 4, 2, 2, 2, 4 ),
 ( 0.0007817246256747476061, 0.0009771112852218902852, 0.001172497944769033181, 0.001367884604316175860, 0.001563271263863318539 ),
 .UNSPECIFIED. ) ;
#38013=EDGE_CURVE ( 'NONE', #6050, #8255, #48247, .T. ) ;
#38014=CARTESIAN_POINT ( 'NONE',  ( -10.68065506134539078, -11.94971097300153140, 32.03036669348370680 ) ) ;
#38015=EDGE_CURVE ( 'NONE', #45914, #68800, #71513, .T. ) ;
#38016=ORIENTED_EDGE ( 'NONE', *, *, #23568, .T. ) ;
#38018=ORIENTED_EDGE ( 'NONE', *, *, #57121, .T. ) ;
#38019=CARTESIAN_POINT ( 'NONE',  ( -17.14219307747939780, -11.67786785259541027, 32.92929555188721480 ) ) ;
#38020=AXIS2_PLACEMENT_3D ( 'NONE', #52703, #59018, #24792 ) ;
#38021=EDGE_LOOP ( 'NONE', ( #33677, #89068 ) ) ;
#38022=FACE_BOUND ( 'NONE', #29606, .T. ) ;
#38023=CARTESIAN_POINT ( 'NONE',  ( 17.07692307692295586, -8.656820664282941280, 34.87096338111179961 ) ) ;
#38024=CIRCLE ( 'NONE', #88397, 0.2500000000000002220 ) ;
#38025=CARTESIAN_POINT ( 'NONE',  ( -3.903900635498009919, -11.86320923018887719, 32.19269448109604781 ) ) ;
#38026=VERTEX_POINT ( 'NONE', #74401 ) ;
#38027=CARTESIAN_POINT ( 'NONE',  ( -15.00775787915638126, -12.15243808032446005, 31.58219941686247978 ) ) ;
#38028=CARTESIAN_POINT ( 'NONE',  ( -6.857821783564084228, -2.379036618887895305, 30.90682066428159303 ) ) ;
#38029=CYLINDRICAL_SURFACE ( 'NONE', #72343, 0.2499999999999979738 ) ;
#38030=EDGE_LOOP ( 'NONE', ( #76429, #24652 ) ) ;
#38031=CARTESIAN_POINT ( 'NONE',  ( 17.93467708450782183, -7.749976743299138882, 34.99404534957040624 ) ) ;
#38032=CARTESIAN_POINT ( 'NONE',  ( 6.000000000000001776, -12.78798330534102945, 29.74999999999997868 ) ) ;
#38034=DIRECTION ( 'NONE',  ( 0.000000000000000000, 0.6427876096865368094, 0.7660444431189802339 ) ) ;
#38035=CARTESIAN_POINT ( 'NONE',  ( 6.923076923076924238, -10.51840700105979565, 33.73612834413961536 ) ) ;
#38036=ORIENTED_EDGE ( 'NONE', *, *, #21023, .T. ) ;
#38037=CARTESIAN_POINT ( 'NONE',  ( 6.988332062589762472, -2.657715359629131857, 31.77849191805844242 ) ) ;
#38038=CARTESIAN_POINT ( 'NONE',  ( -12.23875892027004753, -2.600157965045224451, 30.74683119005207743 ) ) ;
#38039=CARTESIAN_POINT ( 'NONE',  ( -15.93083480223330817, -8.239487800360276282, 34.69522927552633718 ) ) ;
#38040=CARTESIAN_POINT ( 'NONE',  ( 7.780397043639536214, -7.249945686854188942, 34.74374336980223887 ) ) ;
#38041=CARTESIAN_POINT ( 'NONE',  ( 9.562159722575998444, -12.50552854090298638, 31.33409797877408920 ) ) ;
#38042=CYLINDRICAL_SURFACE ( 'NONE', #56726, 0.2499999999999994726 ) ;
#38043=LINE ( 'NONE', #37140, #83630 ) ;
#38044=CARTESIAN_POINT ( 'NONE',  ( -15.23076923076935074, -12.46129190930018460, 30.37095296980731973 ) ) ;
#38045=CARTESIAN_POINT ( 'NONE',  ( -0.3962833220256229416, -8.656820664281605460, 34.87096338111211224 ) ) ;
#38046=DIRECTION ( 'NONE',  ( -0.000000000000000000, 0.9848077530122086864, -0.1736481776669273891 ) ) ;
#38047=CARTESIAN_POINT ( 'NONE',  ( -8.545855283458346108, -2.251407671071268712, 29.88021292934943673 ) ) ;
#38049=ORIENTED_EDGE ( 'NONE', *, *, #13427, .F. ) ;
#38051=ORIENTED_EDGE ( 'NONE', *, *, #60428, .F. ) ;
#38052=B_SPLINE_CURVE_WITH_KNOTS ( 'NONE', 3,
 ( #76755, #69984, #42969, #35776, #56479, #48384, #1978, #70442, #83970, #22250 ),
 .UNSPECIFIED., .F., .F.,
 ( 4, 2, 2, 2, 4 ),
 ( 0.0007817359430256289217, 0.0009771253907249950223, 0.001172514838424361123, 0.001367904286123727007, 0.001563293733823093107 ),
 .UNSPECIFIED. ) ;
#38053=ORIENTED_EDGE ( 'NONE', *, *, #40624, .F. ) ;
#38054=CARTESIAN_POINT ( 'NONE',  ( -17.01166793741023042, -4.320704448112858032, 33.92786785259548310 ) ) ;
#38055=VERTEX_POINT ( 'NONE', #5950 ) ;
#38056=CARTESIAN_POINT ( 'NONE',  ( 3.296024802045255164, -10.21337939537593797, 33.94971097300152252 ) ) ;
#38058=DIRECTION ( 'NONE',  ( -0.000000000000000000, 0.8660254037844399289, -0.4999999999999980016 ) ) ;
#38059=CARTESIAN_POINT ( 'NONE',  ( 17.07692307692307665, -2.721908614388771852, 31.22303859784724978 ) ) ;
#38060=CARTESIAN_POINT ( 'NONE',  ( -0.3962828902624371263, -6.026961402152789304, 34.52809138561124769 ) ) ;
#38061=CYLINDRICAL_SURFACE ( 'NONE', #33122, 0.2500000000000009437 ) ;
#38062=AXIS2_PLACEMENT_3D ( 'NONE', #71717, #78040, #27745 ) ;
#38063=CARTESIAN_POINT ( 'NONE',  ( -8.769230769230890843, -5.219633306517616589, 34.19971097300220464 ) ) ;
#38064=CARTESIAN_POINT ( 'NONE',  ( -10.68146802634049308, -4.098570777380719399, 33.41473453929634729 ) ) ;
#38065=CARTESIAN_POINT ( 'NONE',  ( 0.5923289025054128132, -2.494656445102013453, 31.33466734024120015 ) ) ;
#38067=CARTESIAN_POINT ( 'NONE',  ( -11.31568186948347154, -2.612705202774698421, 31.66806509827799943 ) ) ;
#38070=ORIENTED_EDGE ( 'NONE', *, *, #2176, .F. ) ;
#38071=ORIENTED_EDGE ( 'NONE', *, *, #20197, .F. ) ;
#38072=CARTESIAN_POINT ( 'NONE',  ( 17.14299142792551933, -12.10708131394839882, 31.69288490824020954 ) ) ;
#38073=CARTESIAN_POINT ( 'NONE',  ( 18.00000000000000000, -1.422936976036506707, 30.56769352161908415 ) ) ;
#38074=FACE_OUTER_BOUND ( 'NONE', #77513, .T. ) ;
#38075=CARTESIAN_POINT ( 'NONE',  ( 16.21899093456577745, -7.750023224968865421, 34.99404313364389907 ) ) ;
#38077=CYLINDRICAL_SURFACE ( 'NONE', #71565, 0.2500000000000008882 ) ;
#38078=EDGE_CURVE ( 'NONE', #46711, #21870, #51070, .T. ) ;
#38079=ADVANCED_FACE ( 'NONE', ( #8611 ), #22994, .F. ) ;
#38080=VECTOR ( 'NONE', #59391, 1000.000000000000114 ) ;
#38081=ORIENTED_EDGE ( 'NONE', *, *, #58854, .T. ) ;
#38082=CARTESIAN_POINT ( 'NONE',  ( -10.39195821646982587, -7.630147987733840509, 34.99859428049665411 ) ) ;
#38083=EDGE_LOOP ( 'NONE', ( #81523, #19055, #23507, #63828 ) ) ;
#38084=ORIENTED_EDGE ( 'NONE', *, *, #19312, .T. ) ;
#38085=CARTESIAN_POINT ( 'NONE',  ( -5.933931648997561759, -5.557115091759786019, 34.35708131394839882 ) ) ;
#38086=CIRCLE ( 'NONE', #35256, 0.2500000000000002220 ) ;
#38087=EDGE_CURVE ( 'NONE', #4529, #2835, #67230, .T. ) ;
#38088=CARTESIAN_POINT ( 'NONE',  ( -23.00000000000000000, -12.50000000000000000, 27.25000000000000000 ) ) ;
#38089=CARTESIAN_POINT ( 'NONE',  ( 9.757563263583723057, -12.27809138561124591, 31.22303859784720359 ) ) ;
#38090=EDGE_CURVE ( 'NONE', #24436, #33117, #14925, .T. ) ;
#38091=CARTESIAN_POINT ( 'NONE',  ( -6.249976730942353953, -3.137211980971221781, 32.19342716148376837 ) ) ;
#38093=VERTEX_POINT ( 'NONE', #69418 ) ;
#38095=EDGE_LOOP ( 'NONE', ( #27789, #73298 ) ) ;
#38097=CARTESIAN_POINT ( 'NONE',  ( -1.384615384615505151, -3.300289026999228881, 32.46337939537708905 ) ) ;
#38098=DIRECTION ( 'NONE',  ( 0.000000000000000000, 0.8660254037844377084, -0.5000000000000015543 ) ) ;
#38100=CARTESIAN_POINT ( 'NONE',  ( -15.23076923076922995, -3.050289026998446396, 32.03036669348365706 ) ) ;
#38101=CARTESIAN_POINT ( 'NONE',  ( 1.384615384615386802, -12.10708131394839349, 31.69288490824020244 ) ) ;
#38102=CARTESIAN_POINT ( 'NONE',  ( 17.93391658904412012, -8.120952969808774569, 34.71129190930000163 ) ) ;
#38103=ORIENTED_EDGE ( 'NONE', *, *, #56372, .T. ) ;
#38104=ORIENTED_EDGE ( 'NONE', *, *, #73434, .T. ) ;
#38106=VECTOR ( 'NONE', #46359, 1000.000000000000227 ) ;
#38107=ORIENTED_EDGE ( 'NONE', *, *, #61330, .T. ) ;
#38108=CARTESIAN_POINT ( 'NONE',  ( 2.307692307692187583, -12.46129190930018460, 30.37095296980731973 ) ) ;
#38109=EDGE_LOOP ( 'NONE', ( #5345, #75449, #9991, #27578 ) ) ;
#38110=CARTESIAN_POINT ( 'NONE',  ( 1.161130440891437132, -10.11188796281391333, 34.01382737946119050 ) ) ;
#38111=CARTESIAN_POINT ( 'NONE',  ( 12.68455130563185662, -8.282913670948747864, 34.94150082978203642 ) ) ;
#38113=ADVANCED_FACE ( 'NONE', ( #43707 ), #16243, .F. ) ;
#38115=EDGE_CURVE ( 'NONE', #1316, #83223, #56347, .T. ) ;
#38116=CARTESIAN_POINT ( 'NONE',  ( -1.319360245102546347, -2.657715359629131857, 31.77849191805844242 ) ) ;
#38117=ORIENTED_EDGE ( 'NONE', *, *, #22169, .F. ) ;
#38118=CARTESIAN_POINT ( 'NONE',  ( -8.769230769230892619, -5.094484230521993062, 34.41647553114689373 ) ) ;
#38119=CARTESIAN_POINT ( 'NONE',  ( -7.173053654019277303, -2.779195860258147022, 31.39871582349836743 ) ) ;
#38120=B_SPLINE_CURVE_WITH_KNOTS ( 'NONE', 3,
 ( #85793, #4255, #31736, #59196, #52434, #29955, #43463, #57412, #23192, #50653 ),
 .UNSPECIFIED., .F., .F.,
 ( 4, 2, 2, 2, 4 ),
 ( 0.000000000000000000, 0.0001954311564186866305, 0.0003908623128373732609, 0.0005862934692560598914, 0.0007817246256747465219 ),
 .UNSPECIFIED. ) ;
#38121=FACE_BOUND ( 'NONE', #79973, .T. ) ;
#38122=CARTESIAN_POINT ( 'NONE',  ( 10.54962781287031071, -7.249945686854186278, 34.74374336980224598 ) ) ;
#38123=CARTESIAN_POINT ( 'NONE',  ( 9.692307692307695177, -3.669653830205710676, 35.88435417666054406 ) ) ;
#38125=CARTESIAN_POINT ( 'NONE',  ( 8.769230769230647482, -6.026961402154118019, 34.52809138561165270 ) ) ;
#38126=CARTESIAN_POINT ( 'NONE',  ( -3.480792454990687457, -8.475808217655753651, 34.90892951860618609 ) ) ;
#38127=ORIENTED_EDGE ( 'NONE', *, *, #750, .T. ) ;
#38129=CARTESIAN_POINT ( 'NONE',  ( 13.38461538461538680, -13.04860791097971706, 34.73218667398347037 ) ) ;
#38131=ORIENTED_EDGE ( 'NONE', *, *, #45902, .F. ) ;
#38133=B_SPLINE_CURVE_WITH_KNOTS ( 'NONE', 3,
 ( #44905, #30512, #78703, #16551, #30944, #44018, #11130, #9797, #85906, #22861 ),
 .UNSPECIFIED., .F., .F.,
 ( 4, 2, 2, 2, 4 ),
 ( 0.000000000000000000, 0.0001954311564186867660, 0.0003908623128373735320, 0.0005862934692560603251, 0.0007817246256747470640 ),
 .UNSPECIFIED. ) ;
#38134=CARTESIAN_POINT ( 'NONE',  ( 14.17754509825408960, -10.19110544564092002, 33.96427741523702792 ) ) ;
#38135=CYLINDRICAL_SURFACE ( 'NONE', #49768, 0.2499999999999986955 ) ;
#38136=CARTESIAN_POINT ( 'NONE',  ( 11.28843830116857383, -5.851115903089112003, 34.47074536777953568 ) ) ;
#38137=LINE ( 'NONE', #43999, #28574 ) ;
#38138=FACE_BOUND ( 'NONE', #86955, .T. ) ;
#38139=DIRECTION ( 'NONE',  ( -0.000000000000000000, 0.9848077530122085754, -0.1736481776669273613 ) ) ;
#38141=CARTESIAN_POINT ( 'NONE',  ( -6.923076923077044142, -10.90142922262034020, 33.41473453929536674 ) ) ;
#38142=DIRECTION ( 'NONE',  ( 0.000000000000000000, 0.3420201433256610524, 0.9396926207859113145 ) ) ;
#38143=CARTESIAN_POINT ( 'NONE',  ( 9.758376043310132530, -4.098570777380720287, 33.41473453929635440 ) ) ;
#38144=CARTESIAN_POINT ( 'NONE',  ( 15.90386942290380290, -10.66389620160130036, 33.62221079203477103 ) ) ;
#38145=DIRECTION ( 'NONE',  ( -0.000000000000000000, 0.5000000000000011102, -0.8660254037844381525 ) ) ;
#38147=B_SPLINE_CURVE_WITH_KNOTS ( 'NONE', 3,
 ( #73510, #80722, #18118, #87037, #5497, #45128, #17216, #11805, #3694, #23963 ),
 .UNSPECIFIED., .F., .F.,
 ( 4, 2, 2, 2, 4 ),
 ( 0.0007817359430256324996, 0.0009771253907249993591, 0.001172514838424366110, 0.001367904286123732861, 0.001563293733823099829 ),
 .UNSPECIFIED. ) ;
#38148=ORIENTED_EDGE ( 'NONE', *, *, #52222, .F. ) ;
#38149=CARTESIAN_POINT ( 'NONE',  ( -18.00000000000000000, -5.184797716151534175, 36.11096599634342397 ) ) ;
#38150=CARTESIAN_POINT ( 'NONE',  ( 8.068933515131909928, -10.23759521482555357, 34.22997729860117033 ) ) ;
#38151=CARTESIAN_POINT ( 'NONE',  ( -7.780898706641008467, -11.67786785259547777, 32.92929555188713664 ) ) ;
#38153=AXIS2_PLACEMENT_3D ( 'NONE', #36011, #78299, #71101 ) ;
#38154=CARTESIAN_POINT ( 'NONE',  ( 6.923076923076924238, -12.62096338111211580, 30.90682066428153263 ) ) ;
#38155=CARTESIAN_POINT ( 'NONE',  ( -12.68502338610279523, -6.716662450894489211, 34.94144148231605840 ) ) ;
#38157=CARTESIAN_POINT ( 'NONE',  ( -1.450368812928716000, -7.249945578846654470, 34.99404164642496795 ) ) ;
#38158=FACE_OUTER_BOUND ( 'NONE', #30289, .T. ) ;
#38159=CARTESIAN_POINT ( 'NONE',  ( -7.623141002060450866, -10.01129605718032600, 34.36064277460058491 ) ) ;
#38160=CARTESIAN_POINT ( 'NONE',  ( 5.142178216435913107, -12.70778746994558439, 30.41441678777537305 ) ) ;
#38161=CARTESIAN_POINT ( 'NONE',  ( 12.46153846153833911, -12.46129190930018460, 30.37095296980731973 ) ) ;
#38162=CYLINDRICAL_SURFACE ( 'NONE', #41136, 0.2499999999999997502 ) ;
#38163=EDGE_CURVE ( 'NONE', #47709, #83085, #5973, .T. ) ;
#38164=CARTESIAN_POINT ( 'NONE',  ( -14.30769230769230660, -3.050289026998446396, 32.03036669348365706 ) ) ;
#38165=CARTESIAN_POINT ( 'NONE',  ( 8.069166690247241647, -9.172514111537584114, 34.72667873470787470 ) ) ;
#38166=ORIENTED_EDGE ( 'NONE', *, *, #49998, .T. ) ;
#38167=CARTESIAN_POINT ( 'NONE',  ( 3.361294669002873992, -12.50538340440932217, 31.33453814440721885 ) ) ;
#38168=CARTESIAN_POINT ( 'NONE',  ( 8.834486340506794377, -11.48612834413965977, 32.76840700105972815 ) ) ;
#38170=CARTESIAN_POINT ( 'NONE',  ( -10.61538461538461320, -2.486705287966279876, 31.30864560766543647 ) ) ;
#38171=CARTESIAN_POINT ( 'NONE',  ( -12.46153846153858424, -12.51329471203414379, 31.30864560766407578 ) ) ;
#38172=ORIENTED_EDGE ( 'NONE', *, *, #45342, .F. ) ;
#38173=CARTESIAN_POINT ( 'NONE',  ( -6.673131513698878692, -10.18230066228895758, 34.26354781536631577 ) ) ;
#38174=LINE ( 'NONE', #31423, #38762 ) ;
#38175=CARTESIAN_POINT ( 'NONE',  ( 8.835298102580843249, -2.486705287966280320, 31.30864560766543647 ) ) ;
#38176=EDGE_LOOP ( 'NONE', ( #22352, #12955, #75738, #42758 ) ) ;
#38177=CARTESIAN_POINT ( 'NONE',  ( -13.51530598772569469, -9.929715669179220328, 34.40415004197138416 ) ) ;
#38178=LINE ( 'NONE', #43602, #46963 ) ;
#38180=ADVANCED_FACE ( 'NONE', ( #21563 ), #29225, .F. ) ;
#38181=CIRCLE ( 'NONE', #75594, 0.2500000000000002220 ) ;
#38182=CARTESIAN_POINT ( 'NONE',  ( -14.05763799605399633, -11.28795663066794575, 33.01431243580653785 ) ) ;
#38184=B_SPLINE_CURVE_WITH_KNOTS ( 'NONE', 3,
 ( #69338, #62557, #873, #28338, #55810, #14840, #21582, #76535, #42317, #10286 ),
 .UNSPECIFIED., .F., .F.,
 ( 4, 2, 2, 2, 4 ),
 ( 0.0007817246336856290608, 0.0009771112958940101571, 0.001172497958102391036, 0.001367884620310772133, 0.001563271282519153446 ),
 .UNSPECIFIED. ) ;
#38185=CARTESIAN_POINT ( 'NONE',  ( -16.15384615384615330, -13.37000171582298513, 34.34916445242398453 ) ) ;
#38186=CARTESIAN_POINT ( 'NONE',  ( -11.76132780152463830, -2.251424796025575326, 29.88072029997477941 ) ) ;
#38187=CARTESIAN_POINT ( 'NONE',  ( 3.930919936330004472, -9.886141570436013382, 34.14413921362392301 ) ) ;
#38188=VERTEX_POINT ( 'NONE', #49486 ) ;
#38189=ORIENTED_EDGE ( 'NONE', *, *, #70528, .F. ) ;
#38190=ORIENTED_EDGE ( 'NONE', *, *, #59658, .F. ) ;
#38191=EDGE_CURVE ( 'NONE', #26565, #44547, #22069, .T. ) ;
#38192=CARTESIAN_POINT ( 'NONE',  ( -9.692307692307691624, -2.721908614388771852, 31.22303859784724978 ) ) ;
#38193=LINE ( 'NONE', #65651, #86076 ) ;
#38194=EDGE_CURVE ( 'NONE', #68109, #83936, #74729, .T. ) ;
#38195=CARTESIAN_POINT ( 'NONE',  ( 2.307692307692309264, -5.557115091759785130, 34.35708131394839171 ) ) ;
#38196=DIRECTION ( 'NONE',  ( -0.000000000000000000, -0.5000000000000009992, -0.8660254037844380415 ) ) ;
#38197=AXIS2_PLACEMENT_3D ( 'NONE', #84969, #36337, #2094 ) ;
#38198=EDGE_LOOP ( 'NONE', ( #23170, #75073 ) ) ;
#38199=EDGE_CURVE ( 'NONE', #75748, #62404, #36416, .T. ) ;
#38201=CARTESIAN_POINT ( 'NONE',  ( 15.36156103859402222, -4.809403383903225304, 33.96459661697924304 ) ) ;
#38202=ORIENTED_EDGE ( 'NONE', *, *, #88861, .T. ) ;
#38203=CARTESIAN_POINT ( 'NONE',  ( -18.22348492456433178, -10.97335522853832934, 33.68706563782419749 ) ) ;
#38206=B_SPLINE_CURVE_WITH_KNOTS ( 'NONE', 3,
 ( #77978, #23907, #2746, #16282, #45073, #9516, #72550, #44618, #10417, #10861 ),
 .UNSPECIFIED., .F., .F.,
 ( 4, 2, 2, 2, 4 ),
 ( 0.000000000000000000, 0.0001954311564186873894, 0.0003908623128373747788, 0.0005862934692560621682, 0.0007817246256747495577 ),
 .UNSPECIFIED. ) ;
#38207=CARTESIAN_POINT ( 'NONE',  ( 1.515141086378950952, -10.88167719472716399, 33.43325721877153711 ) ) ;
#38208=CARTESIAN_POINT ( 'NONE',  ( 20.75000000000001066, -7.500000000000000000, 29.75000000000000355 ) ) ;
#38210=EDGE_LOOP ( 'NONE', ( #53202, #10195, #85080, #30447 ) ) ;
#38213=CARTESIAN_POINT ( 'NONE',  ( 5.142178648199100977, -5.219633306516380244, 34.19971097300157936 ) ) ;
#38214=EDGE_LOOP ( 'NONE', ( #58264, #83438, #57309, #16804 ) ) ;
#38215=CARTESIAN_POINT ( 'NONE',  ( 18.06525513951284267, -12.16647553114626490, 32.15551576947920864 ) ) ;
#38216=B_SPLINE_CURVE_WITH_KNOTS ( 'NONE', 3,
 ( #76687, #55518, #6889, #21286, #40691, #35249, #68154, #6457, #34358, #48760 ),
 .UNSPECIFIED., .F., .F.,
 ( 4, 2, 2, 2, 4 ),
 ( 0.0007817359430256293554, 0.0009771253907249974075, 0.001172514838424365460, 0.001367904286123733512, 0.001563293733823094625 ),
 .UNSPECIFIED. ) ;
#38217=CARTESIAN_POINT ( 'NONE',  ( 12.46153846153846168, -11.16473453929635440, 33.15142922261926373 ) ) ;
#38218=EDGE_CURVE ( 'NONE', #60596, #12315, #56527, .T. ) ;
#38219=VERTEX_POINT ( 'NONE', #70640 ) ;
#38220=DIRECTION ( 'NONE',  ( -0.000000000000000000, -0.7660444431189791237, -0.6427876096865379196 ) ) ;
#38221=CARTESIAN_POINT ( 'NONE',  ( -1.515306851282942624, -8.147922237126337563, 34.70805685702651999 ) ) ;
#38222=CARTESIAN_POINT ( 'NONE',  ( 8.769230769230647482, -6.026961402154118019, 34.52809138561165270 ) ) ;
#38223=FACE_BOUND ( 'NONE', #23829, .T. ) ;
#38224=CARTESIAN_POINT ( 'NONE',  ( -5.076923076923199218, -10.33852847137269571, 34.16647553114546554 ) ) ;
#38225=CARTESIAN_POINT ( 'NONE',  ( -6.923076923076922462, -9.058645607665452459, 34.76329471203371924 ) ) ;
#38226=EDGE_CURVE ( 'NONE', #40782, #441, #77392, .T. ) ;
#38227=CARTESIAN_POINT ( 'NONE',  ( -15.09997742294444834, -10.54018710029568595, 33.71981072465678864 ) ) ;
#38228=CARTESIAN_POINT ( 'NONE',  ( 17.01084069756293715, -9.058645607665454236, 34.76329471203372634 ) ) ;
#38229=CARTESIAN_POINT ( 'NONE',  ( -6.000000000000119904, -2.892918686052165622, 31.69288490824153470 ) ) ;
#38230=AXIS2_PLACEMENT_3D ( 'NONE', #18341, #4833, #46697 ) ;
#38231=CARTESIAN_POINT ( 'NONE',  ( 17.74997677577853850, -6.652501968072647820, 34.93155406624980941 ) ) ;
#38232=CARTESIAN_POINT ( 'NONE',  ( 16.15384615384615330, -2.249999999999998668, 29.75000000000001776 ) ) ;
#38233=EDGE_LOOP ( 'NONE', ( #63800, #3181 ) ) ;
#38234=EDGE_CURVE ( 'NONE', #6887, #63695, #31641, .T. ) ;
#38235=CARTESIAN_POINT ( 'NONE',  ( -18.00000000000012079, -6.026961402154117131, 34.52809138561165270 ) ) ;
#38236=CARTESIAN_POINT ( 'NONE',  ( 11.53846153846153832, -11.11383981884818262, 36.00935417666054406 ) ) ;
#38239=AXIS2_PLACEMENT_3D ( 'NONE', #33632, #727, #56996 ) ;
#38240=LINE ( 'NONE', #58490, #27436 ) ;
#38241=CARTESIAN_POINT ( 'NONE',  ( 10.61538461538449418, -12.16647553114689728, 32.15551576947799362 ) ) ;
#38242=CARTESIAN_POINT ( 'NONE',  ( -6.923076923076922462, -9.058645607665452459, 34.76329471203371924 ) ) ;
#38243=FACE_OUTER_BOUND ( 'NONE', #8749, .T. ) ;
#38244=CARTESIAN_POINT ( 'NONE',  ( -11.66860950819323328, -10.31621877034669588, 34.18098118002070152 ) ) ;
#38245=ORIENTED_EDGE ( 'NONE', *, *, #15929, .F. ) ;
#38249=CARTESIAN_POINT ( 'NONE',  ( -9.822999158975250111, -4.118384482072085184, 33.43331474514187107 ) ) ;
#38250=DIRECTION ( 'NONE',  ( -0.000000000000000000, -0.6427876096865404731, -0.7660444431189770143 ) ) ;
#38251=CARTESIAN_POINT ( 'NONE',  ( 10.83816415665302380, -4.387253974876679230, 33.66317474335728832 ) ) ;
#38253=B_SPLINE_CURVE_WITH_KNOTS ( 'NONE', 3,
 ( #79409, #17711, #30328, #7954, #56136, #21465, #30763, #51013, #35420, #78504 ),
 .UNSPECIFIED., .F., .F.,
 ( 4, 2, 2, 2, 4 ),
 ( 0.0007817359430256216575, 0.0009771253907249856981, 0.001172514838424349847, 0.001367904286123713779, 0.001563293733823077928 ),
 .UNSPECIFIED. ) ;
#38254=CARTESIAN_POINT ( 'NONE',  ( 5.076923076922953193, -11.67786785259630911, 32.92929555188603530 ) ) ;
#38255=ADVANCED_FACE ( 'NONE', ( #65198 ), #52129, .F. ) ;
#38257=VERTEX_POINT ( 'NONE', #58002 ) ;
#38258=ORIENTED_EDGE ( 'NONE', *, *, #80880, .F. ) ;
#38259=CARTESIAN_POINT ( 'NONE',  ( 14.24160992833216888, -12.34228464037088280, 31.77849191805838558 ) ) ;
#38260=EDGE_CURVE ( 'NONE', #53380, #54393, #80057, .T. ) ;
#38261=CARTESIAN_POINT ( 'NONE',  ( -17.75000000000006750, -7.565270445406050648, 34.75000000000000000 ) ) ;
#38263=CARTESIAN_POINT ( 'NONE',  ( -16.21911659980693443, -5.219633306516282545, 34.19971097300152252 ) ) ;
#38264=FACE_OUTER_BOUND ( 'NONE', #30768, .T. ) ;
#38266=CARTESIAN_POINT ( 'NONE',  ( 7.173076923076923350, -7.500000000000001776, 35.04278698407183867 ) ) ;
#38267=CARTESIAN_POINT ( 'NONE',  ( 8.769230769230647482, -10.90142922262034020, 33.41473453929536674 ) ) ;
#38270=CARTESIAN_POINT ( 'NONE',  ( -18.25000000000000355, -12.50000000000000000, 29.75000000000000355 ) ) ;
#38271=CARTESIAN_POINT ( 'NONE',  ( -9.822917347511772590, -7.722926974430166069, 34.99546784045485737 ) ) ;
#38272=LINE ( 'NONE', #3587, #48707 ) ;
#38273=CARTESIAN_POINT ( 'NONE',  ( -3.164600089806574257, -7.250054483168843156, 34.74374881642865631 ) ) ;
#38275=CARTESIAN_POINT ( 'NONE',  ( 4.023154687178596589, -12.38065189839062263, 30.83690757178629482 ) ) ;
#38276=VECTOR ( 'NONE', #63279, 1000.000000000000227 ) ;
#38277=CARTESIAN_POINT ( 'NONE',  ( -5.750054590621955342, -4.932303261841489039, 34.32971442181322885 ) ) ;
#38278=CARTESIAN_POINT ( 'NONE',  ( -3.164700879766792152, -11.16473453929635440, 33.15142922261926373 ) ) ;
#38279=CARTESIAN_POINT ( 'NONE',  ( -11.40767109749459074, -2.845873456487965747, 32.17976146951972538 ) ) ;
#38281=CARTESIAN_POINT ( 'NONE',  ( -16.08777882049607655, -6.343179335718451384, 34.87096338111212646 ) ) ;
#38283=CARTESIAN_POINT ( 'NONE',  ( -9.692307692307691624, -2.486705287966279876, 31.30864560766543647 ) ) ;
#38284=B_SPLINE_CURVE_WITH_KNOTS ( 'NONE', 3,
 ( #29299, #43245, #70720, #9023, #36493, #2239, #29734, #84689, #22964, #50428 ),
 .UNSPECIFIED., .F., .F.,
 ( 4, 2, 2, 2, 4 ),
 ( 0.0007817246256747447872, 0.0009771112852218879000, 0.001172497944769031013, 0.001367884604316173909, 0.001563271263863317022 ),
 .UNSPECIFIED. ) ;
#38285=CARTESIAN_POINT ( 'NONE',  ( 13.31934538405906565, -6.835583212224499938, 34.95778746994557906 ) ) ;
#38289=FILL_AREA_STYLE ('',( #45029 ) ) ;
#38290=CARTESIAN_POINT ( 'NONE',  ( 8.546304551714619890, -11.24512374952581872, 33.06303171183252942 ) ) ;
#38291=EDGE_LOOP ( 'NONE', ( #14682, #40998 ) ) ;
#38293=CARTESIAN_POINT ( 'NONE',  ( 2.980745993476265898, -9.271318131107980420, 34.42618302367067429 ) ) ;
#38294=VECTOR ( 'NONE', #50045, 1000.000000000000000 ) ;
#38295=ORIENTED_EDGE ( 'NONE', *, *, #48036, .F. ) ;
#38296=EDGE_CURVE ( 'NONE', #69130, #34806, #40266, .T. ) ;
#38297=CARTESIAN_POINT ( 'NONE',  ( -4.088591014333314178, -2.657715359629131857, 31.77849191805844242 ) ) ;
#38298=EDGE_LOOP ( 'NONE', ( #78522, #35136, #21042, #44297 ) ) ;
#38299=FACE_OUTER_BOUND ( 'NONE', #19554, .T. ) ;
#38300=CARTESIAN_POINT ( 'NONE',  ( 13.38461538461538680, -9.780366693483667717, 34.19971097300155094 ) ) ;
#38301=DIRECTION ( 'NONE',  ( -0.000000000000000000, 0.9396926207859092051, -0.3420201433256662704 ) ) ;
#38302=ORIENTED_EDGE ( 'NONE', *, *, #67661, .T. ) ;
#38304=VERTEX_POINT ( 'NONE', #79169 ) ;
#38305=CARTESIAN_POINT ( 'NONE',  ( -12.46153846153846168, -13.20930481340135110, 34.54067556320372745 ) ) ;
#38306=VERTEX_POINT ( 'NONE', #45370 ) ;
#38307=CARTESIAN_POINT ( 'NONE',  ( -15.90379173393269596, -2.318338780012836775, 30.59689888758630616 ) ) ;
#38308=DIRECTION ( 'NONE',  ( -0.000000000000000000, -0.3420201433256694901, -0.9396926207859082059 ) ) ;
#38309=AXIS2_PLACEMENT_3D ( 'NONE', #6292, #33755, #25668 ) ;
#38310=EDGE_LOOP ( 'NONE', ( #82771, #1347 ) ) ;
#38311=CARTESIAN_POINT ( 'NONE',  ( 9.442330961365341224, -9.148715823498378086, 34.47080413974185120 ) ) ;
#38312=CARTESIAN_POINT ( 'NONE',  ( 7.846153846153846700, -2.499999999999998668, 29.50000000000001066 ) ) ;
#38313=EDGE_CURVE ( 'NONE', #66445, #88887, #67142, .T. ) ;
#38314=CARTESIAN_POINT ( 'NONE',  ( -1.254089946381741427, -11.04252011169590020, 33.62494198852677130 ) ) ;
#38315=AXIS2_PLACEMENT_3D ( 'NONE', #6616, #35412, #41737 ) ;
#38316=CARTESIAN_POINT ( 'NONE',  ( 5.076923076923075762, -8.973038597847269315, 34.52809138561121927 ) ) ;
#38317=CARTESIAN_POINT ( 'NONE',  ( -13.38461538461538325, -11.91647553114624181, 32.58852847137148245 ) ) ;
#38318=ORIENTED_EDGE ( 'NONE', *, *, #61298, .T. ) ;
#38320=ORIENTED_EDGE ( 'NONE', *, *, #76437, .T. ) ;
#38321=CARTESIAN_POINT ( 'NONE',  ( 3.230769230769108269, -5.941354392335915335, 34.76329471203413846 ) ) ;
#38322=ORIENTED_EDGE ( 'NONE', *, *, #6606, .F. ) ;
#38323=CARTESIAN_POINT ( 'NONE',  ( -8.899377978668987055, -10.19110544564092002, 33.96427741523702792 ) ) ;
#38324=CARTESIAN_POINT ( 'NONE',  ( 1.450683735617825709, -2.721908614388772740, 31.22303859784725333 ) ) ;
#38325=ORIENTED_EDGE ( 'NONE', *, *, #69296, .F. ) ;
#38326=ORIENTED_EDGE ( 'NONE', *, *, #56224, .T. ) ;
#38327=CARTESIAN_POINT ( 'NONE',  ( -10.74607608205217346, -3.062553014421049546, 32.05460306192773601 ) ) ;
#38328=VERTEX_POINT ( 'NONE', #50784 ) ;
#38329=CARTESIAN_POINT ( 'NONE',  ( -10.39237326377176451, -9.086983370893049639, 34.49168942202179267 ) ) ;
#38330=VECTOR ( 'NONE', #57773, 1000.000000000000227 ) ;
#38331=EDGE_CURVE ( 'NONE', #34679, #18725, #3709, .T. ) ;
#38333=CARTESIAN_POINT ( 'NONE',  ( 12.23805351781451201, -2.599994579823202923, 30.74605699353653776 ) ) ;
#38334=FACE_BOUND ( 'NONE', #9091, .T. ) ;
#38336=CARTESIAN_POINT ( 'NONE',  ( 2.057692307692309708, -7.566083408709834757, 34.74999999999999289 ) ) ;
#38337=DIRECTION ( 'NONE',  ( -0.000000000000000000, -0.1736481776669307198, -0.9848077530122080203 ) ) ;
#38338=EDGE_CURVE ( 'NONE', #55087, #2893, #82212, .T. ) ;
#38339=CARTESIAN_POINT ( 'NONE',  ( -14.24243673641628050, -6.026961402152789304, 34.52809138561124769 ) ) ;
#38340=CARTESIAN_POINT ( 'NONE',  ( 8.769230769230647482, -3.300289026999228881, 32.46337939537708905 ) ) ;
#38341=LINE ( 'NONE', #45088, #4472 ) ;
#38342=EDGE_LOOP ( 'NONE', ( #18081, #81543, #79183, #57026 ) ) ;
#38343=EDGE_CURVE ( 'NONE', #33560, #7422, #56367, .T. ) ;
#38344=B_SPLINE_CURVE_WITH_KNOTS ( 'NONE', 3,
 ( #84450, #85330, #50188, #63271, #15986, #2886, #22292, #70925, #9235, #2449 ),
 .UNSPECIFIED., .F., .F.,
 ( 4, 2, 2, 2, 4 ),
 ( 0.0007817359430256252354, 0.0009771253907249902518, 0.001172514838424355051, 0.001367904286123720068, 0.001563293733823085084 ),
 .UNSPECIFIED. ) ;
#38345=VECTOR ( 'NONE', #23987, 1000.000000000000227 ) ;
#38346=CARTESIAN_POINT ( 'NONE',  ( -7.173053654019277303, -6.567427716900047230, 34.66269422305636283 ) ) ;
#38347=ORIENTED_EDGE ( 'NONE', *, *, #7455, .T. ) ;
#38349=CARTESIAN_POINT ( 'NONE',  ( -7.173100147298380413, -4.175268141568689195, 33.81360843649122216 ) ) ;
#38350=CARTESIAN_POINT ( 'NONE',  ( -7.846153846153844924, -5.415277668671390821, 36.20867863119892149 ) ) ;
#38351=EDGE_CURVE ( 'NONE', #64930, #79014, #11213, .T. ) ;
#38352=DIRECTION ( 'NONE',  ( 0.000000000000000000, 0.6427876096865373645, -0.7660444431189797898 ) ) ;
#38353=CARTESIAN_POINT ( 'NONE',  ( -2.241623956689868802, -12.10708131394839704, 31.69288490824020954 ) ) ;
#38354=CARTESIAN_POINT ( 'NONE',  ( 17.32692307692451195, -7.500000000000155431, 34.75000000000007105 ) ) ;
#38355=CARTESIAN_POINT ( 'NONE',  ( -3.230769230769352962, -11.06231777344772027, 33.60647404775119895 ) ) ;
#38356=VERTEX_POINT ( 'NONE', #69532 ) ;
#38357=CARTESIAN_POINT ( 'NONE',  ( 17.01083966596719321, -5.557115091759785130, 34.35708131394839171 ) ) ;
#38358=CARTESIAN_POINT ( 'NONE',  ( 17.75002325595140817, -3.436278759898155677, 33.07459398097509506 ) ) ;
#38359=DIRECTION ( 'NONE',  ( 0.000000000000000000, 0.000000000000000000, 1.000000000000000000 ) ) ;
#38360=CARTESIAN_POINT ( 'NONE',  ( 14.53070515178570865, -2.523321265292115534, 31.42251411153756990 ) ) ;
#38362=EDGE_CURVE ( 'NONE', #1867, #57235, #44530, .T. ) ;
#38363=ORIENTED_EDGE ( 'NONE', *, *, #44201, .T. ) ;
#38364=FACE_BOUND ( 'NONE', #74441, .T. ) ;
#38366=VERTEX_POINT ( 'NONE', #26000 ) ;
#38367=CARTESIAN_POINT ( 'NONE',  ( 11.78840694783958298, -12.45601412856602686, 31.48342859153981621 ) ) ;
#38368=CARTESIAN_POINT ( 'NONE',  ( -7.173076923076921574, -7.500000000000001776, 34.75000000000000000 ) ) ;
#38369=ORIENTED_EDGE ( 'NONE', *, *, #11590, .T. ) ;
#38370=CARTESIAN_POINT ( 'NONE',  ( -7.846153846153965716, -4.481592998941358097, 33.73612834414048933 ) ) ;
#38371=DIRECTION ( 'NONE',  ( 0.000000000000000000, 0.3420201433256641055, -0.9396926207859100932 ) ) ;
#38372=CARTESIAN_POINT ( 'NONE',  ( -7.976301055592065481, -11.93770438780619259, 32.05411857736982029 ) ) ;
#38373=DIRECTION ( 'NONE',  ( -0.000000000000000000, 1.000000000000000000, -0.000000000000000000 ) ) ;
#38374=LINE ( 'NONE', #19435, #20069 ) ;
#38375=ORIENTED_EDGE ( 'NONE', *, *, #10285, .T. ) ;
#38376=CARTESIAN_POINT ( 'NONE',  ( -15.00775638667583678, -2.308499170217967134, 30.53291367094873721 ) ) ;
#38377=VERTEX_POINT ( 'NONE', #76286 ) ;
#38378=FACE_OUTER_BOUND ( 'NONE', #9480, .T. ) ;
#38379=DIRECTION ( 'NONE',  ( 0.000000000000000000, 0.7660444431189822323, -0.6427876096865344779 ) ) ;
#38380=CARTESIAN_POINT ( 'NONE',  ( -12.46153846153846168, -13.53365097954675988, 30.81389545987213552 ) ) ;
#38381=CARTESIAN_POINT ( 'NONE',  ( 18.22277954126840172, -8.496831190052089866, 34.64984203495476578 ) ) ;
#38382=CARTESIAN_POINT ( 'NONE',  ( 7.846153846153723244, -11.67786785259630911, 32.92929555188603530 ) ) ;
#38383=AXIS2_PLACEMENT_3D ( 'NONE', #48007, #48448, #75484 ) ;
#38384=CARTESIAN_POINT ( 'NONE',  ( 5.299702618191483694, -12.44528174975671853, 30.48912976160716681 ) ) ;
#38387=EDGE_CURVE ( 'NONE', #6352, #20065, #5288, .T. ) ;
#38388=CARTESIAN_POINT ( 'NONE',  ( -3.480745961711583458, -3.137211980971222669, 32.19342716148376837 ) ) ;
#38389=CARTESIAN_POINT ( 'NONE',  ( -9.692307692307691624, -8.120952969808772792, 34.71129190930000163 ) ) ;
#38390=CARTESIAN_POINT ( 'NONE',  ( 6.250000000000004441, -2.499999999999999112, 29.81604066197450109 ) ) ;
#38391=ORIENTED_EDGE ( 'NONE', *, *, #20807, .F. ) ;
#38392=ORIENTED_EDGE ( 'NONE', *, *, #66195, .F. ) ;
#38393=CARTESIAN_POINT ( 'NONE',  ( -9.019207513279360100, -5.643011162660950042, 34.66104346484419096 ) ) ;
#38394=CARTESIAN_POINT ( 'NONE',  ( 11.28848479441294650, -4.818429247618089661, 34.26397095200675125 ) ) ;
#38395=CARTESIAN_POINT ( 'NONE',  ( 17.07692307692295586, -3.643525952248796163, 33.31231777344771672 ) ) ;
#38396=CARTESIAN_POINT ( 'NONE',  ( 8.900021210197717636, -11.37503395064541678, 33.29242100308974273 ) ) ;
#38397=EDGE_CURVE ( 'NONE', #2182, #49089, #635, .T. ) ;
#38398=DIRECTION ( 'NONE',  ( -0.000000000000000000, -0.1736481776669307198, -0.9848077530122080203 ) ) ;
#38399=CARTESIAN_POINT ( 'NONE',  ( 5.776515056276054771, -8.496056993536548418, 34.65000542017679663 ) ) ;
#38400=ORIENTED_EDGE ( 'NONE', *, *, #18150, .T. ) ;
#38401=AXIS2_PLACEMENT_3D ( 'NONE', #15485, #50135, #2389 ) ;
#38402=CARTESIAN_POINT ( 'NONE',  ( 10.61538461538461675, -13.53365097954675988, 30.81389545987213552 ) ) ;
#38403=CARTESIAN_POINT ( 'NONE',  ( 8.769230769230768274, -8.120952969808772792, 34.71129190930000163 ) ) ;
#38404=EDGE_CURVE ( 'NONE', #86388, #23968, #69292, .T. ) ;
#38405=CARTESIAN_POINT ( 'NONE',  ( 4.218990934565787221, -7.750023224968867197, 34.99404313364389907 ) ) ;
#38406=CARTESIAN_POINT ( 'NONE',  ( -3.453695448285377445, -11.76352882383564769, 32.36236540154569497 ) ) ;
#38407=ORIENTED_EDGE ( 'NONE', *, *, #31181, .T. ) ;
#38408=CARTESIAN_POINT ( 'NONE',  ( -7.780085495151406683, -3.513871655860379306, 32.76840700105978499 ) ) ;
#38409=VECTOR ( 'NONE', #41752, 1000.000000000000114 ) ;
#38410=ORIENTED_EDGE ( 'NONE', *, *, #81522, .T. ) ;
#38411=DIRECTION ( 'NONE',  ( 0.000000000000000000, 0.9396926207859126468, -0.3420201433256571111 ) ) ;
#38413=CYLINDRICAL_SURFACE ( 'NONE', #74374, 0.2500000000000002220 ) ;
#38415=CIRCLE ( 'NONE', #78646, 0.2500000000000002220 ) ;
#38416=FACE_OUTER_BOUND ( 'NONE', #24088, .T. ) ;
#38417=LINE ( 'NONE', #3286, #34945 ) ;
#38418=EDGE_CURVE ( 'NONE', #7925, #79557, #77890, .T. ) ;
#38419=CYLINDRICAL_SURFACE ( 'NONE', #86921, 0.2500000000000004996 ) ;
#38420=CARTESIAN_POINT ( 'NONE',  ( 8.834376548562733689, -7.750023238201979581, 34.74374492549440419 ) ) ;
#38422=EDGE_CURVE ( 'NONE', #9533, #67226, #60671, .T. ) ;
#38423=EDGE_CURVE ( 'NONE', #39262, #32155, #50581, .T. ) ;
#38424=B_SPLINE_CURVE_WITH_KNOTS ( 'NONE', 3,
 ( #36291, #61642, #78152, #57878, #16453, #29533, #70956, #64621, #2923, #9266 ),
 .UNSPECIFIED., .F., .F.,
 ( 4, 2, 2, 2, 4 ),
 ( 0.000000000000000000, 0.0001954311564186870642, 0.0003908623128373741283, 0.0005862934692560611925, 0.0007817246256747482566 ),
 .UNSPECIFIED. ) ;
#38425=ORIENTED_EDGE ( 'NONE', *, *, #61409, .T. ) ;
#38426=CYLINDRICAL_SURFACE ( 'NONE', #70262, 0.2500000000000009437 ) ;
#38427=VERTEX_POINT ( 'NONE', #63210 ) ;
#38428=CARTESIAN_POINT ( 'NONE',  ( 5.299702745901138101, -11.60474049983371003, 33.02348890104160262 ) ) ;
#38429=EDGE_CURVE ( 'NONE', #34985, #16890, #29885, .T. ) ;
#38430=DIRECTION ( 'NONE',  ( -0.000000000000000000, -0.9848077530122085754, -0.1736481776669273613 ) ) ;
#38431=CARTESIAN_POINT ( 'NONE',  ( -7.846153846153844924, -1.242168528481310874, 33.36296068462461051 ) ) ;
#38433=DIRECTION ( 'NONE',  ( 0.000000000000000000, 0.6427876096865368094, 0.7660444431189802339 ) ) ;
#38435=DIRECTION ( 'NONE',  ( -0.000000000000000000, -0.8660254037844399289, -0.4999999999999980016 ) ) ;
#38436=ORIENTED_EDGE ( 'NONE', *, *, #44581, .F. ) ;
#38437=VERTEX_POINT ( 'NONE', #57787 ) ;
#38438=VERTEX_POINT ( 'NONE', #15928 ) ;
#38439=ORIENTED_EDGE ( 'NONE', *, *, #88427, .F. ) ;
#38440=ORIENTED_EDGE ( 'NONE', *, *, #3674, .F. ) ;
#38442=CARTESIAN_POINT ( 'NONE',  ( 12.59206416330202671, -11.93748526763465279, 32.05452791011430946 ) ) ;
#38443=CARTESIAN_POINT ( 'NONE',  ( -3.480745974817821331, -6.524016743844655686, 34.90889640711025521 ) ) ;
#38444=CARTESIAN_POINT ( 'NONE',  ( -10.55012947587177941, -5.094484230520773593, 34.41647553114626845 ) ) ;
#38445=CARTESIAN_POINT ( 'NONE',  ( -15.23076923076922995, -4.945431358278436385, 36.03766855953609394 ) ) ;
#38446=CARTESIAN_POINT ( 'NONE',  ( 13.38461538461538680, -8.120952969808772792, 34.71129190930000163 ) ) ;
#38448=CARTESIAN_POINT ( 'NONE',  ( 8.769230769230768274, -8.973038597847269315, 34.52809138561121927 ) ) ;
#38449=CYLINDRICAL_SURFACE ( 'NONE', #40797, 0.2500000000000009437 ) ;
#38450=CARTESIAN_POINT ( 'NONE',  ( -3.903791842207838148, -10.66356715214248396, 33.62249196103329751 ) ) ;
#38452=VERTEX_POINT ( 'NONE', #49264 ) ;
#38453=ORIENTED_EDGE ( 'NONE', *, *, #68513, .T. ) ;
#38454=EDGE_LOOP ( 'NONE', ( #9474, #33590, #41664, #54214 ) ) ;
#38455=CARTESIAN_POINT ( 'NONE',  ( 6.130790440966951138, -12.35292014791297710, 31.75344720912887198 ) ) ;
#38456=ORIENTED_EDGE ( 'NONE', *, *, #84122, .T. ) ;
#38457=B_SPLINE_CURVE_WITH_KNOTS ( 'NONE', 3,
 ( #35598, #63047, #41468, #70712, #14891, #42364, #28848, #84684, #56309, #83798 ),
 .UNSPECIFIED., .F., .F.,
 ( 4, 2, 2, 2, 4 ),
 ( 0.0007817246256747446788, 0.0009771112852218874663, 0.001172497944769030145, 0.001367884604316172825, 0.001563271263863315720 ),
 .UNSPECIFIED. ) ;
#38458=LINE ( 'NONE', #31705, #77700 ) ;
#38459=CARTESIAN_POINT ( 'NONE',  ( 10.55011416942384095, -9.442884908240170461, 34.35708131394840592 ) ) ;
#38461=CARTESIAN_POINT ( 'NONE',  ( -1.634592128663975741, -4.818429247618089661, 34.26397095200675125 ) ) ;
#38462=VECTOR ( 'NONE', #51842, 1000.000000000000227 ) ;
#38464=FACE_BOUND ( 'NONE', #39738, .T. ) ;
#38466=ORIENTED_EDGE ( 'NONE', *, *, #23312, .F. ) ;
#38467=EDGE_CURVE ( 'NONE', #67881, #36002, #70873, .T. ) ;
#38468=CARTESIAN_POINT ( 'NONE',  ( -17.20761368003338632, -11.37499894934982514, 33.29245874905763003 ) ) ;
#38469=VECTOR ( 'NONE', #78642, 1000.000000000000000 ) ;
#38470=EDGE_LOOP ( 'NONE', ( #60247, #47611, #88212, #71333 ) ) ;
#38471=FACE_BOUND ( 'NONE', #58360, .T. ) ;
#38472=CARTESIAN_POINT ( 'NONE',  ( 13.38461538461538680, -8.810774026931790459, 35.74407628777942847 ) ) ;
#38473=DIRECTION ( 'NONE',  ( 0.000000000000000000, 0.6427876096865368094, 0.7660444431189802339 ) ) ;
#38474=VERTEX_POINT ( 'NONE', #43393 ) ;
#38475=CARTESIAN_POINT ( 'NONE',  ( -15.23076923076935074, -12.27809138561165270, 31.22303859784587132 ) ) ;
#38477=CARTESIAN_POINT ( 'NONE',  ( -18.13014796973170206, -4.299443229763728169, 33.91186481527756058 ) ) ;
#38478=ORIENTED_EDGE ( 'NONE', *, *, #13308, .T. ) ;
#38479=FACE_OUTER_BOUND ( 'NONE', #32590, .T. ) ;
#38480=CARTESIAN_POINT ( 'NONE',  ( 3.230769230769108269, -5.094484230521993062, 34.41647553114689373 ) ) ;
#38481=VERTEX_POINT ( 'NONE', #36638 ) ;
#38482=ADVANCED_FACE ( 'NONE', ( #63658 ), #43827, .F. ) ;
#38483=DIRECTION ( 'NONE',  ( 0.000000000000000000, 0.3420201433256641055, -0.9396926207859100932 ) ) ;
#38484=CARTESIAN_POINT ( 'NONE',  ( 6.923076923076802558, -10.90142922262034020, 33.41473453929536674 ) ) ;
#38485=ORIENTED_EDGE ( 'NONE', *, *, #16956, .T. ) ;
#38486=CARTESIAN_POINT ( 'NONE',  ( 0.2115152242454953480, -9.271318131107980420, 34.42618302367067429 ) ) ;
#38487=CARTESIAN_POINT ( 'NONE',  ( 14.55763782604044998, -8.433404298154334455, 34.66254593164985920 ) ) ;
#38488=CARTESIAN_POINT ( 'NONE',  ( 16.02369818411445834, -3.069018819979304702, 32.56621877034667278 ) ) ;
#38489=LINE ( 'NONE', #66846, #44306 ) ;
#38490=CARTESIAN_POINT ( 'NONE',  ( 18.00000000000000000, -7.500000000000001776, 35.04278698407183867 ) ) ;
#38491=CARTESIAN_POINT ( 'NONE',  ( 6.673053685783957967, -9.271318131107980420, 34.42618302367067429 ) ) ;
#38492=CARTESIAN_POINT ( 'NONE',  ( 11.53846153846153832, -12.29105614889573062, 35.45975837776705220 ) ) ;
#38493=CARTESIAN_POINT ( 'NONE',  ( 8.769230769230645706, -3.083524468854526912, 32.58852847137268327 ) ) ;
#38495=CARTESIAN_POINT ( 'NONE',  ( -15.23076923076922995, -11.69971097300155272, 32.46337939537588113 ) ) ;
#38496=CARTESIAN_POINT ( 'NONE',  ( -14.30769230769230660, -2.499999999999998668, 29.75000000000001421 ) ) ;
#38498=ORIENTED_EDGE ( 'NONE', *, *, #67609, .T. ) ;
#38499=CARTESIAN_POINT ( 'NONE',  ( 16.15384615384615330, -2.721908614388771852, 31.22303859784724978 ) ) ;
#38500=VERTEX_POINT ( 'NONE', #30752 ) ;
#38502=ORIENTED_EDGE ( 'NONE', *, *, #78629, .T. ) ;
#38503=EDGE_CURVE ( 'NONE', #57712, #7553, #69972, .T. ) ;
#38504=CARTESIAN_POINT ( 'NONE',  ( -2.177166605928743337, -12.45806712695776319, 30.39783852428763922 ) ) ;
#38508=DIRECTION ( 'NONE',  ( -0.000000000000000000, 1.000000000000000000, 3.491481338843133355E-15 ) ) ;
#38509=CARTESIAN_POINT ( 'NONE',  ( -6.923076923076922462, -13.88283147151868846, 33.14645433367849847 ) ) ;
#38510=CARTESIAN_POINT ( 'NONE',  ( -7.715362038329057981, -5.582136614379148654, 34.36778462344220486 ) ) ;
#38511=DIRECTION ( 'NONE',  ( 0.000000000000000000, 0.4999999999999985567, 0.8660254037844395958 ) ) ;
#38512=CARTESIAN_POINT ( 'NONE',  ( -5.299850035829926753, -3.395401636524186362, 33.02366814457250399 ) ) ;
#38513=FACE_OUTER_BOUND ( 'NONE', #43673, .T. ) ;
#38514=CARTESIAN_POINT ( 'NONE',  ( 6.000000000000309086, -2.506253911140614576, 30.00000000000323297 ) ) ;
#38516=CARTESIAN_POINT ( 'NONE',  ( -11.28851612908349722, -2.589246495874658383, 31.60778113518102828 ) ) ;
#38517=CARTESIAN_POINT ( 'NONE',  ( 14.53070365930516061, -10.61302985866384141, 33.66295027996417843 ) ) ;
#38518=EDGE_CURVE ( 'NONE', #24368, #25168, #53159, .T. ) ;
#38519=VECTOR ( 'NONE', #10486, 999.9999999999998863 ) ;
#38520=EDGE_CURVE ( 'NONE', #12295, #27221, #4851, .T. ) ;
#38521=CARTESIAN_POINT ( 'NONE',  ( -2.437839517130526712, -4.460286881179643004, 33.72017969459903242 ) ) ;
#38522=ORIENTED_EDGE ( 'NONE', *, *, #51990, .T. ) ;
#38523=ORIENTED_EDGE ( 'NONE', *, *, #40562, .F. ) ;
#38525=CARTESIAN_POINT ( 'NONE',  ( -14.24243673641628050, -8.613356846314928816, 34.62446782046653482 ) ) ;
#38526=CARTESIAN_POINT ( 'NONE',  ( -11.53846153846153655, -3.669653830205710676, 35.88435417666054406 ) ) ;
#38527=CARTESIAN_POINT ( 'NONE',  ( 14.30769230769231015, -4.945431358278436385, 36.03766855953609394 ) ) ;
#38528=B_SPLINE_CURVE_WITH_KNOTS ( 'NONE', 3,
 ( #43874, #22713, #37110, #48857, #21392, #83101, #63701, #9642, #70015, #64571 ),
 .UNSPECIFIED., .F., .F.,
 ( 4, 2, 2, 2, 4 ),
 ( 0.0007817246256747474977, 0.0009771112852218911526, 0.001172497944769034699, 0.001367884604316178462, 0.001563271263863322009 ),
 .UNSPECIFIED. ) ;
#38529=CARTESIAN_POINT ( 'NONE',  ( 17.20744851515672025, -12.50538340440932394, 31.33453814440721885 ) ) ;
#38530=CARTESIAN_POINT ( 'NONE',  ( -3.230769230769229949, -5.471508081941601098, 34.59228464037088457 ) ) ;
#38531=B_SPLINE_CURVE_WITH_KNOTS ( 'NONE', 3,
 ( #25583, #85507, #72868, #66108, #24690, #79198, #71985, #11176, #30555, #18384 ),
 .UNSPECIFIED., .F., .F.,
 ( 4, 2, 2, 2, 4 ),
 ( 0.0007817359430256284880, 0.0009771253907249941549, 0.001172514838424359822, 0.001367904286123725489, 0.001563293733823091156 ),
 .UNSPECIFIED. ) ;
#38532=B_SPLINE_CURVE_WITH_KNOTS ( 'NONE', 3,
 ( #2265, #29762, #57227, #16241, #43705, #11260, #4040, #86035, #85148, #65305 ),
 .UNSPECIFIED., .F., .F.,
 ( 4, 2, 2, 2, 4 ),
 ( 0.0007817246256747451124, 0.0009771112852218879000, 0.001172497944769030796, 0.001367884604316173692, 0.001563271263863316588 ),
 .UNSPECIFIED. ) ;
#38533=AXIS2_PLACEMENT_3D ( 'NONE', #31485, #58948, #62817 ) ;
#38535=ORIENTED_EDGE ( 'NONE', *, *, #68499, .T. ) ;
#38536=CARTESIAN_POINT ( 'NONE',  ( 17.86985279056177944, -12.45813303252208648, 30.39737893381572675 ) ) ;
#38537=ORIENTED_EDGE ( 'NONE', *, *, #34876, .T. ) ;
#38539=EDGE_LOOP ( 'NONE', ( #75876, #16844, #57259, #11164 ) ) ;
#38540=CARTESIAN_POINT ( 'NONE',  ( 7.846153846153723244, -11.06231777344772027, 33.60647404775119895 ) ) ;
#38541=CARTESIAN_POINT ( 'NONE',  ( -2.307692307692305711, -9.058645607665452459, 34.76329471203371924 ) ) ;
#38542=CARTESIAN_POINT ( 'NONE',  ( -9.692307692307812417, -6.879047030192662504, 34.71129190930017927 ) ) ;
#38543=CARTESIAN_POINT ( 'NONE',  ( -10.61538461538461320, -10.05456864172156806, 36.03766855953608683 ) ) ;
#38544=CARTESIAN_POINT ( 'NONE',  ( -2.177166605928741117, -11.93748526763465279, 32.05452791011430946 ) ) ;
#38545=ORIENTED_EDGE ( 'NONE', *, *, #4365, .T. ) ;
#38546=ORIENTED_EDGE ( 'NONE', *, *, #3661, .F. ) ;
#38547=EDGE_LOOP ( 'NONE', ( #41425, #47250, #79870, #76334 ) ) ;
#38549=CARTESIAN_POINT ( 'NONE',  ( 9.942362112221147186, -2.318338780012835443, 30.59689888758630261 ) ) ;
#38550=B_SPLINE_CURVE_WITH_KNOTS ( 'NONE', 3,
 ( #2989, #79558, #65132, #65577, #38568, #66484, #79995, #45763, #11541, #51156 ),
 .UNSPECIFIED., .F., .F.,
 ( 4, 2, 2, 2, 4 ),
 ( 0.0007817246256747505334, 0.0009771112852218954894, 0.001172497944769040554, 0.001367884604316185618, 0.001563271263863330682 ),
 .UNSPECIFIED. ) ;
#38551=CYLINDRICAL_SURFACE ( 'NONE', #25024, 0.2499999999999979738 ) ;
#38552=CARTESIAN_POINT ( 'NONE',  ( -8.546217925137375104, -10.01129605718032600, 34.36064277460058491 ) ) ;
#38553=B_SPLINE_CURVE_WITH_KNOTS ( 'NONE', 3,
 ( #64285, #36828, #17896, #57983, #17451, #2154, #30077, #77810, #43583, #9800 ),
 .UNSPECIFIED., .F., .F.,
 ( 4, 2, 2, 2, 4 ),
 ( 0.000000000000000000, 0.0001954311564186860613, 0.0003908623128373721225, 0.0005862934692560581567, 0.0007817246256747442451 ),
 .UNSPECIFIED. ) ;
#38554=DIRECTION ( 'NONE',  ( -0.000000000000000000, 0.8660254037844397068, -0.4999999999999978906 ) ) ;
#38555=CARTESIAN_POINT ( 'NONE',  ( 5.933916589044120116, -12.37446782046654192, 30.86335684631486487 ) ) ;
#38556=ORIENTED_EDGE ( 'NONE', *, *, #8794, .T. ) ;
#38557=ORIENTED_EDGE ( 'NONE', *, *, #89130, .F. ) ;
#38559=VERTEX_POINT ( 'NONE', #42957 ) ;
#38560=AXIS2_PLACEMENT_3D ( 'NONE', #5983, #28462, #34323 ) ;
#38561=CARTESIAN_POINT ( 'NONE',  ( -5.750054481651857508, -3.202959910592335202, 32.30730279482227019 ) ) ;
#38564=CARTESIAN_POINT ( 'NONE',  ( -7.173076923076942002, -2.249999999999999112, 29.81609741502488120 ) ) ;
#38565=CARTESIAN_POINT ( 'NONE',  ( -2.307692307691991296, -2.255955759149395501, 30.00000000000324363 ) ) ;
#38567=AXIS2_PLACEMENT_3D ( 'NONE', #48372, #83958, #55572 ) ;
#38568=CARTESIAN_POINT ( 'NONE',  ( 10.86533002476265963, -2.341251567377310217, 30.72681386836322659 ) ) ;
#38569=VERTEX_POINT ( 'NONE', #44249 ) ;
#38571=CARTESIAN_POINT ( 'NONE',  ( -8.769230769230768274, -4.661471528628507777, 34.16647553114623292 ) ) ;
#38572=CARTESIAN_POINT ( 'NONE',  ( 0.4615384615383382183, -11.67786785259630911, 32.92929555188603530 ) ) ;
#38573=FACE_BOUND ( 'NONE', #29576, .T. ) ;
#38574=CARTESIAN_POINT ( 'NONE',  ( -0.2114840416250085564, -11.47946981652013498, 33.17500667209846910 ) ) ;
#38575=CARTESIAN_POINT ( 'NONE',  ( 7.912221179503920787, -2.292212530054420494, 30.41441678777542990 ) ) ;
#38576=CARTESIAN_POINT ( 'NONE',  ( -1.608100309179714360, -3.562934362175799841, 33.22335522853832401 ) ) ;
#38577=CARTESIAN_POINT ( 'NONE',  ( -3.296039231325549324, -8.656820664281497102, 34.87096338111211935 ) ) ;
#38578=ORIENTED_EDGE ( 'NONE', *, *, #74004, .T. ) ;
#38579=CARTESIAN_POINT ( 'NONE',  ( 11.40777093535123399, -11.37499894934982692, 33.29245874905763003 ) ) ;
#38580=CARTESIAN_POINT ( 'NONE',  ( 8.992242120843620512, -6.503523203565941380, 34.64991518177335195 ) ) ;
#38581=ORIENTED_EDGE ( 'NONE', *, *, #78565, .T. ) ;
#38582=CARTESIAN_POINT ( 'NONE',  ( -8.703975629717930929, -3.643525952247864463, 33.31231777344670064 ) ) ;
#38583=CARTESIAN_POINT ( 'NONE',  ( 16.15384615384615330, -11.16473453929635440, 33.15142922261926373 ) ) ;
#38584=CARTESIAN_POINT ( 'NONE',  ( -6.065270445960775803, -10.90142922261923886, 33.41473453929638993 ) ) ;
#38587=FACE_BOUND ( 'NONE', #68004, .T. ) ;
#38588=CARTESIAN_POINT ( 'NONE',  ( 5.326868486301119532, -5.766571408460171355, 34.70601412856602508 ) ) ;
#38589=FACE_OUTER_BOUND ( 'NONE', #29324, .T. ) ;
#38590=CARTESIAN_POINT ( 'NONE',  ( -6.857008572074485109, -10.51840700105979565, 33.73612834413962247 ) ) ;
#38591=CYLINDRICAL_SURFACE ( 'NONE', #64517, 0.2500000000000008882 ) ;
#38592=CARTESIAN_POINT ( 'NONE',  ( -11.53846153846153655, -5.180354513474913603, 36.12317359536750416 ) ) ;
#38593=CARTESIAN_POINT ( 'NONE',  ( -3.931066484868087851, -10.97394488606064122, 33.68653795673694873 ) ) ;
#38595=VECTOR ( 'NONE', #22079, 999.9999999999998863 ) ;
#38597=B_SPLINE_CURVE_WITH_KNOTS ( 'NONE', 3,
 ( #52119, #64738, #79607, #17904, #23317, #50774, #78260, #9807, #30521, #54338 ),
 .UNSPECIFIED., .F., .F.,
 ( 4, 2, 2, 2, 4 ),
 ( 0.0007817246256747519429, 0.0009771112852218959231, 0.001172497944769039686, 0.001367884604316183667, 0.001563271263863327647 ),
 .UNSPECIFIED. ) ;
#38598=VERTEX_POINT ( 'NONE', #36207 ) ;
#38601=CARTESIAN_POINT ( 'NONE',  ( -15.00734226890766188, -7.630147231320743018, 34.74852402298682819 ) ) ;
#38602=CARTESIAN_POINT ( 'NONE',  ( -1.319359813339359366, -10.90142922261932057, 33.41473453929631887 ) ) ;
#38603=CARTESIAN_POINT ( 'NONE',  ( -10.83831157429145975, -11.43668979543635089, 33.22377378376089752 ) ) ;
#38604=CARTESIAN_POINT ( 'NONE',  ( -4.153846153846152411, -4.661471528628507777, 34.16647553114623292 ) ) ;
#38605=CARTESIAN_POINT ( 'NONE',  ( 6.223012844093396723, -3.395485233115139057, 33.02377354290275946 ) ) ;
#38607=CARTESIAN_POINT ( 'NONE',  ( 14.08420736396836226, -10.81261337010820256, 33.49550067578627477 ) ) ;
#38608=CARTESIAN_POINT ( 'NONE',  ( -14.43784027742400333, -11.66186481527757302, 32.95055677023626117 ) ) ;
#38609=CARTESIAN_POINT ( 'NONE',  ( 8.096099364501986528, -11.86320923018887719, 32.19269448109604070 ) ) ;
#38610=CARTESIAN_POINT ( 'NONE',  ( 5.299935921016470708, -12.64618726649961289, 30.78989965857442712 ) ) ;
#38611=CARTESIAN_POINT ( 'NONE',  ( 8.639083559792549494, -10.19110544564092002, 33.96427741523702792 ) ) ;
#38612=CARTESIAN_POINT ( 'NONE',  ( 9.562159722576001997, -3.625366637846545892, 33.29286588640298561 ) ) ;
#38613=CARTESIAN_POINT ( 'NONE',  ( -3.230769230769229949, -5.471508081941601098, 34.59228464037088457 ) ) ;
#38615=DIRECTION ( 'NONE',  ( 0.000000000000000000, 0.8660254037844377084, -0.5000000000000015543 ) ) ;
#38616=ORIENTED_EDGE ( 'NONE', *, *, #22796, .F. ) ;
#38617=CARTESIAN_POINT ( 'NONE',  ( -5.076923076923075762, -11.11383981884818262, 36.00935417666054406 ) ) ;
#38618=LINE ( 'NONE', #86835, #84860 ) ;
#38620=CARTESIAN_POINT ( 'NONE',  ( -10.74607521849492464, -9.929715669179220328, 34.40415004197138416 ) ) ;
#38621=CARTESIAN_POINT ( 'NONE',  ( -5.326946314216041145, -2.587272538249754117, 30.68239716806877837 ) ) ;
#38622=ORIENTED_EDGE ( 'NONE', *, *, #24501, .T. ) ;
#38625=CARTESIAN_POINT ( 'NONE',  ( -7.596099426240392027, -12.41089969410671223, 31.60739465890703670 ) ) ;
#38626=ORIENTED_EDGE ( 'NONE', *, *, #33007, .T. ) ;
#38628=CARTESIAN_POINT ( 'NONE',  ( 12.52679403281448600, -12.46129190930001052, 30.37095296980870174 ) ) ;
#38629=FACE_OUTER_BOUND ( 'NONE', #36970, .T. ) ;
#38631=CARTESIAN_POINT ( 'NONE',  ( -16.21959958215948916, -7.249945578846654470, 34.99404164642496795 ) ) ;
#38632=VERTEX_POINT ( 'NONE', #64976 ) ;
#38633=CARTESIAN_POINT ( 'NONE',  ( 10.61538461538461675, -13.20930481340135110, 34.54067556320372745 ) ) ;
#38634=CARTESIAN_POINT ( 'NONE',  ( -11.60371147023562344, -2.255955759149247619, 30.00000000000013856 ) ) ;
#38635=EDGE_CURVE ( 'NONE', #64411, #28677, #57467, .T. ) ;
#38636=CIRCLE ( 'NONE', #63044, 0.2500000000000002220 ) ;
#38637=CARTESIAN_POINT ( 'NONE',  ( 4.153846153846032507, -10.21337939537710326, 33.94971097300076224 ) ) ;
#38638=EDGE_LOOP ( 'NONE', ( #13115, #11407, #77735, #526 ) ) ;
#38640=EDGE_CURVE ( 'NONE', #81137, #5354, #72460, .T. ) ;
#38641=ORIENTED_EDGE ( 'NONE', *, *, #30781, .T. ) ;
#38643=CARTESIAN_POINT ( 'NONE',  ( 0.3954550505825804030, -8.120952969808774569, 34.71129190930000163 ) ) ;
#38644=CARTESIAN_POINT ( 'NONE',  ( 9.692307692307570832, -4.320704448113951379, 33.92786785259630022 ) ) ;
#38646=CARTESIAN_POINT ( 'NONE',  ( -10.39260507411620438, -3.236590943229499029, 32.36255958852954251 ) ) ;
#38647=VERTEX_POINT ( 'NONE', #31653 ) ;
#38649=CARTESIAN_POINT ( 'NONE',  ( 4.376625822824220080, -5.827830569534416583, 34.72679350104403539 ) ) ;
#38650=ORIENTED_EDGE ( 'NONE', *, *, #76556, .T. ) ;
#38651=CARTESIAN_POINT ( 'NONE',  ( -16.21992853320628925, -12.34228464037088280, 31.77849191805838558 ) ) ;
#38652=AXIS2_PLACEMENT_3D ( 'NONE', #28625, #7012, #56087 ) ;
#38654=CARTESIAN_POINT ( 'NONE',  ( -8.546451227962359454, -12.44528174975671853, 30.48912976160716681 ) ) ;
#38655=LINE ( 'NONE', #51241, #33854 ) ;
#38657=ORIENTED_EDGE ( 'NONE', *, *, #23379, .T. ) ;
#38659=CARTESIAN_POINT ( 'NONE',  ( 15.10007776410167502, -2.541943142973491554, 30.39792223712631980 ) ) ;
#38661=B_SPLINE_CURVE_WITH_KNOTS ( 'NONE', 3,
 ( #79687, #17541, #24277, #51736, #44993, #58958, #24736, #17989, #45442, #4464 ),
 .UNSPECIFIED., .F., .F.,
 ( 4, 2, 2, 2, 4 ),
 ( 0.000000000000000000, 0.0001954339857564070678, 0.0003908679715128141356, 0.0005863019572692211492, 0.0007817359430256282712 ),
 .UNSPECIFIED. ) ;
#38662=CARTESIAN_POINT ( 'NONE',  ( 2.307692307692309264, -13.04860791097971706, 34.73218667398347037 ) ) ;
#38663=EDGE_CURVE ( 'NONE', #59654, #10540, #71334, .T. ) ;
#38664=CARTESIAN_POINT ( 'NONE',  ( -13.60810032833933469, -6.760086850603066466, 34.69517049084099369 ) ) ;
#38667=CARTESIAN_POINT ( 'NONE',  ( 16.15384615384615330, -12.34228464037088635, 31.77849191805839268 ) ) ;
#38668=CARTESIAN_POINT ( 'NONE',  ( 4.219101725122175850, -2.892918686051625166, 31.69288490824025928 ) ) ;
#38669=FACE_BOUND ( 'NONE', #28909, .T. ) ;
#38670=CARTESIAN_POINT ( 'NONE',  ( -5.999999999999998224, -10.05456864172156806, 36.03766855953608683 ) ) ;
#38671=CARTESIAN_POINT ( 'NONE',  ( 11.31497659473759043, -8.496056993536548418, 34.65000542017679663 ) ) ;
#38672=CARTESIAN_POINT ( 'NONE',  ( -8.769230769230768274, -4.098570777380720287, 33.41473453929634729 ) ) ;
#38673=CARTESIAN_POINT ( 'NONE',  ( 17.07692307692307665, -9.058645607665452459, 34.76329471203371924 ) ) ;
#38674=CARTESIAN_POINT ( 'NONE',  ( 14.30769230769231015, -2.833524468853757305, 32.15551576947925838 ) ) ;
#38675=CIRCLE ( 'NONE', #51636, 0.2500000000000002220 ) ;
#38676=CARTESIAN_POINT ( 'NONE',  ( 6.000000000000317080, -2.255955759149395501, 30.00000000000324363 ) ) ;
#38677=CARTESIAN_POINT ( 'NONE',  ( 8.769230769230647482, -3.835265460704628371, 33.15142922262033665 ) ) ;
#38678=ORIENTED_EDGE ( 'NONE', *, *, #83520, .F. ) ;
#38679=CARTESIAN_POINT ( 'NONE',  ( -17.07692307692319744, -5.941354392335915335, 34.76329471203413846 ) ) ;
#38680=CARTESIAN_POINT ( 'NONE',  ( -13.38461538461538325, -9.058645607665452459, 34.76329471203371924 ) ) ;
#38681=ORIENTED_EDGE ( 'NONE', *, *, #20068, .F. ) ;
#38682=ORIENTED_EDGE ( 'NONE', *, *, #16212, .T. ) ;
#38683=EDGE_CURVE ( 'NONE', #59958, #1686, #15523, .T. ) ;
#38684=VECTOR ( 'NONE', #16274, 1000.000000000000000 ) ;
#38685=FACE_OUTER_BOUND ( 'NONE', #7585, .T. ) ;
#38686=CARTESIAN_POINT ( 'NONE',  ( 10.86543903529806876, -12.65882529074907126, 30.72640787790839312 ) ) ;
#38687=CARTESIAN_POINT ( 'NONE',  ( 16.40379167219429846, -2.587454068350149239, 30.68340429815432557 ) ) ;
#38689=CARTESIAN_POINT ( 'NONE',  ( -10.61538461538473399, -11.94971097300221174, 32.03036669348237098 ) ) ;
#38690=ORIENTED_EDGE ( 'NONE', *, *, #13519, .F. ) ;
#38692=CARTESIAN_POINT ( 'NONE',  ( 18.13052543823364360, -4.299079248970731015, 33.91157788607253565 ) ) ;
#38693=AXIS2_PLACEMENT_3D ( 'NONE', #78568, #71360, #9668 ) ;
#38694=CARTESIAN_POINT ( 'NONE',  ( 4.826899839630109490, -5.851115903089112003, 34.47074536777953568 ) ) ;
#38696=CARTESIAN_POINT ( 'NONE',  ( -12.46153846153846168, -4.786620604624113540, 33.94971097300155094 ) ) ;
#38697=CARTESIAN_POINT ( 'NONE',  ( 0.4615384615384611200, -3.322132147404559976, 32.92929555188717927 ) ) ;
#38698=( NAMED_UNIT ( * ) SI_UNIT ( $, .STERADIAN. ) SOLID_ANGLE_UNIT ( ) );
#38699=FACE_OUTER_BOUND ( 'NONE', #29278, .T. ) ;
#38701=ORIENTED_EDGE ( 'NONE', *, *, #48382, .T. ) ;
#38702=ORIENTED_EDGE ( 'NONE', *, *, #18150, .F. ) ;
#38703=EDGE_CURVE ( 'NONE', #46051, #31453, #539, .T. ) ;
#38704=LINE ( 'NONE', #30602, #82305 ) ;
#38705=CARTESIAN_POINT ( 'NONE',  ( -4.403869391139118683, -12.43535235679832596, 30.55408501211184813 ) ) ;
#38706=CARTESIAN_POINT ( 'NONE',  ( 10.86543892702293057, -2.564540009722896752, 30.55348353981670684 ) ) ;
#38707=CARTESIAN_POINT ( 'NONE',  ( 4.087763774486018242, -10.67929555188718460, 33.92786785259543336 ) ) ;
#38708=EDGE_CURVE ( 'NONE', #10893, #41440, #29569, .T. ) ;
#38709=CARTESIAN_POINT ( 'NONE',  ( 17.32692307692314415, -7.434744860731433924, 35.00000000000000711 ) ) ;
#38711=LINE ( 'NONE', #8263, #60470 ) ;
#38712=DIRECTION ( 'NONE',  ( -0.000000000000000000, 0.9396926207859092051, -0.3420201433256662704 ) ) ;
#38713=CARTESIAN_POINT ( 'NONE',  ( -8.992715693795103604, -12.69144148231606017, 30.53333754910549303 ) ) ;
#38714=LINE ( 'NONE', #66174, #88495 ) ;
#38716=CARTESIAN_POINT ( 'NONE',  ( 16.15384615384615330, -1.242168528481310874, 33.36296068462461051 ) ) ;
#38717=CARTESIAN_POINT ( 'NONE',  ( 2.177545098254088263, -3.285722584762969856, 32.44110544564090759 ) ) ;
#38718=CARTESIAN_POINT ( 'NONE',  ( 8.068933515131911705, -8.540255544307065350, 34.89611431652622286 ) ) ;
#38719=CARTESIAN_POINT ( 'NONE',  ( -6.223484943723947893, -10.11188796281391511, 34.01382737946119050 ) ) ;
#38720=EDGE_CURVE ( 'NONE', #59530, #64959, #60893, .T. ) ;
#38721=CARTESIAN_POINT ( 'NONE',  ( -4.153846153846152411, -8.973038597847269315, 34.52809138561121927 ) ) ;
#38722=CARTESIAN_POINT ( 'NONE',  ( -3.453696189676078276, -12.38737895849757820, 31.66785238281580206 ) ) ;
#38723=ORIENTED_EDGE ( 'NONE', *, *, #44384, .F. ) ;
#38724=B_SPLINE_CURVE_WITH_KNOTS ( 'NONE', 3,
 ( #80782, #19061, #67251, #59150, #60486, #87999, #26258, #10974, #65900, #27142 ),
 .UNSPECIFIED., .F., .F.,
 ( 4, 2, 2, 2, 4 ),
 ( 0.000000000000000000, 0.0001954339857564054144, 0.0003908679715128108288, 0.0005863019572692162703, 0.0007817359430256216575 ),
 .UNSPECIFIED. ) ;
#38726=CARTESIAN_POINT ( 'NONE',  ( 11.53846153846141753, -11.94971097300221174, 32.03036669348237098 ) ) ;
#38727=DIRECTION ( 'NONE',  ( 0.000000000000000000, 0.000000000000000000, 1.000000000000000000 ) ) ;
#38728=CARTESIAN_POINT ( 'NONE',  ( 13.31853300525525086, -6.343179335718451384, 34.87096338111212646 ) ) ;
#38730=ADVANCED_FACE ( 'NONE', ( #82950 ), #82070, .F. ) ;
#38731=B_SPLINE_CURVE_WITH_KNOTS ( 'NONE', 3,
 ( #33193, #74628, #31869, #25990, #11597, #80048, #53453, #74181, #46265, #12482 ),
 .UNSPECIFIED., .F., .F.,
 ( 4, 2, 2, 2, 4 ),
 ( 0.0007817246256747451124, 0.0009771112852218885505, 0.001172497944769032097, 0.001367884604316175427, 0.001563271263863318973 ),
 .UNSPECIFIED. ) ;
#38732=CARTESIAN_POINT ( 'NONE',  ( -18.22286542220362904, -2.501496062324911396, 29.88072118266894250 ) ) ;
#38733=CARTESIAN_POINT ( 'NONE',  ( 14.17754433796061875, -5.070767119584671079, 34.40440758774516183 ) ) ;
#38734=CARTESIAN_POINT ( 'NONE',  ( 5.142178216435913107, -4.320704448112861584, 33.92786785259548310 ) ) ;
#38735=ORIENTED_EDGE ( 'NONE', *, *, #52820, .T. ) ;
#38737=CARTESIAN_POINT ( 'NONE',  ( 2.980792499826877773, -9.148715823498378086, 34.47080413974185120 ) ) ;
#38738=ADVANCED_FACE ( 'NONE', ( #40638 ), #55030, .F. ) ;
#38739=ORIENTED_EDGE ( 'NONE', *, *, #16825, .F. ) ;
#38740=DIRECTION ( 'NONE',  ( 0.000000000000000000, 0.6427876096865373645, -0.7660444431189797898 ) ) ;
#38741=EDGE_LOOP ( 'NONE', ( #6894, #17915 ) ) ;
#38742=CARTESIAN_POINT ( 'NONE',  ( 15.23076923076923173, -2.486705287966279876, 31.30864560766543647 ) ) ;
#38744=EDGE_CURVE ( 'NONE', #11362, #61129, #55242, .T. ) ;
#38745=CARTESIAN_POINT ( 'NONE',  ( 16.15384615384615330, -8.120952969808772792, 34.71129190930000163 ) ) ;
#38746=EDGE_LOOP ( 'NONE', ( #18265, #76134, #7518, #16646 ) ) ;
#38747=FACE_OUTER_BOUND ( 'NONE', #8061, .T. ) ;
#38749=CARTESIAN_POINT ( 'NONE',  ( 11.31497659473758866, -3.754499324213721234, 33.06261337010820256 ) ) ;
#38750=B_SPLINE_CURVE_WITH_KNOTS ( 'NONE', 3,
 ( #60219, #17913, #87277, #80510, #18803, #66993, #46713, #60664, #88174, #45367 ),
 .UNSPECIFIED., .F., .F.,
 ( 4, 2, 2, 2, 4 ),
 ( 0.000000000000000000, 0.0001954311564186876876, 0.0003908623128373753751, 0.0005862934692560630356, 0.0007817246256747507503 ),
 .UNSPECIFIED. ) ;
#38751=ORIENTED_EDGE ( 'NONE', *, *, #32533, .F. ) ;
#38752=CARTESIAN_POINT ( 'NONE',  ( 2.307692307692186251, -9.528491918059723176, 34.59228464037033035 ) ) ;
#38753=CARTESIAN_POINT ( 'NONE',  ( 0.4615384615383396616, -11.48612834414049644, 32.76840700105863391 ) ) ;
#38754=ADVANCED_FACE ( 'NONE', ( #69429 ), #41514, .F. ) ;
#38756=EDGE_CURVE ( 'NONE', #30027, #86745, #34819, .T. ) ;
#38757=CARTESIAN_POINT ( 'NONE',  ( -5.326923076923075762, -7.500000000000001776, 35.00000000000000000 ) ) ;
#38759=CARTESIAN_POINT ( 'NONE',  ( 12.59206416330202671, -5.195472089885680766, 34.18748526763464923 ) ) ;
#38760=AXIS2_PLACEMENT_3D ( 'NONE', #33729, #46351, #26534 ) ;
#38762=VECTOR ( 'NONE', #58889, 1000.000000000000114 ) ;
#38764=EDGE_LOOP ( 'NONE', ( #54925, #56317 ) ) ;
#38765=EDGE_LOOP ( 'NONE', ( #29999, #63953, #70358, #88142 ) ) ;
#38766=B_SPLINE_CURVE_WITH_KNOTS ( 'NONE', 3,
 ( #16585, #51229, #3954, #58904, #86410, #64765, #79186, #24680, #58020, #80074 ),
 .UNSPECIFIED., .F., .F.,
 ( 4, 2, 2, 2, 4 ),
 ( 0.0007817246256747516176, 0.0009771112852218965736, 0.001172497944769041421, 0.001367884604316186269, 0.001563271263863331333 ),
 .UNSPECIFIED. ) ;
#38767=VERTEX_POINT ( 'NONE', #61321 ) ;
#38768=CARTESIAN_POINT ( 'NONE',  ( 3.296024370282069071, -12.70778746994558439, 30.41441678777536595 ) ) ;
#38769=ORIENTED_EDGE ( 'NONE', *, *, #609, .F. ) ;
#38770=B_SPLINE_CURVE_WITH_KNOTS ( 'NONE', 3,
 ( #50758, #57531, #3469, #51189, #30505, #58404, #85900, #50322, #8919, #29632 ),
 .UNSPECIFIED., .F., .F.,
 ( 4, 2, 2, 2, 4 ),
 ( 0.000000000000000000, 0.0001954339857564074473, 0.0003908679715128148945, 0.0005863019572692223418, 0.0007817359430256297891 ),
 .UNSPECIFIED. ) ;
#38771=CARTESIAN_POINT ( 'NONE',  ( -14.30769230769242917, -11.06231777344772027, 33.60647404775119895 ) ) ;
#38773=EDGE_LOOP ( 'NONE', ( #30797, #39779 ) ) ;
#38774=EDGE_LOOP ( 'NONE', ( #83646, #78004, #86855, #3157 ) ) ;
#38775=CARTESIAN_POINT ( 'NONE',  ( -7.846153846153967493, -11.67786785259630911, 32.92929555188603530 ) ) ;
#38777=CARTESIAN_POINT ( 'NONE',  ( 9.823099500132480344, -8.147973898785416225, 34.70805048591653730 ) ) ;
#38779=CARTESIAN_POINT ( 'NONE',  ( -4.153846153846152411, -1.790695186598648903, 34.54067556320373455 ) ) ;
#38781=AXIS2_PLACEMENT_3D ( 'NONE', #3797, #57405, #85783 ) ;
#38782=CARTESIAN_POINT ( 'NONE',  ( -11.47239420511146513, -11.91647553114624358, 32.58852847137148245 ) ) ;
#38784=FACE_BOUND ( 'NONE', #15847, .T. ) ;
#38785=CARTESIAN_POINT ( 'NONE',  ( 17.14299041027315695, -6.343179335718452272, 34.87096338111212646 ) ) ;
#38786=CARTESIAN_POINT ( 'NONE',  ( -1.318446243652726890, -7.250054483168843156, 34.74374881642865631 ) ) ;
#38787=ADVANCED_FACE ( 'NONE', ( #48261 ), #47825, .F. ) ;
#38789=DIRECTION ( 'NONE',  ( -0.000000000000000000, 0.1736481776669307198, -0.9848077530122080203 ) ) ;
#38790=CARTESIAN_POINT ( 'NONE',  ( -14.30769230769230660, -8.973038597847269315, 34.52809138561121927 ) ) ;
#38791=CARTESIAN_POINT ( 'NONE',  ( 12.46153846153846168, -3.322132147404559976, 32.92929555188717927 ) ) ;
#38792=ORIENTED_EDGE ( 'NONE', *, *, #86903, .T. ) ;
#38793=CARTESIAN_POINT ( 'NONE',  ( -11.60373153901785948, -3.643525952247789412, 33.31231777344662959 ) ) ;
#38794=VERTEX_POINT ( 'NONE', #531 ) ;
#38795=VERTEX_POINT ( 'NONE', #75304 ) ;
#38796=ADVANCED_FACE ( 'NONE', ( #21232 ), #48704, .F. ) ;
#38797=CARTESIAN_POINT ( 'NONE',  ( 12.46153846153846168, -10.67929555188718282, 33.92786785259544047 ) ) ;
#38798=CARTESIAN_POINT ( 'NONE',  ( -1.634638608836841200, -5.765609946408405406, 34.70566812827424741 ) ) ;
#38799=B_SPLINE_CURVE_WITH_KNOTS ( 'NONE', 3,
 ( #6105, #75444, #55163, #88107, #41220, #81767, #47072, #82661, #20932, #48404 ),
 .UNSPECIFIED., .F., .F.,
 ( 4, 2, 2, 2, 4 ),
 ( 0.000000000000000000, 0.0001954339857564081249, 0.0003908679715128162498, 0.0005863019572692244018, 0.0007817359430256324996 ),
 .UNSPECIFIED. ) ;
#38800=B_SPLINE_CURVE_WITH_KNOTS ( 'NONE', 3,
 ( #79152, #87262, #66977, #80042, #25981, #53445, #17453, #44909, #28191, #7038 ),
 .UNSPECIFIED., .F., .F.,
 ( 4, 2, 2, 2, 4 ),
 ( 0.0007817359430256303312, 0.0009771253907249965402, 0.001172514838424362641, 0.001367904286123728958, 0.001563293733823095059 ),
 .UNSPECIFIED. ) ;
#38801=CARTESIAN_POINT ( 'NONE',  ( 6.000000000000001776, -13.63283147151868846, 33.57946703557072254 ) ) ;
#38802=DIRECTION ( 'NONE',  ( 0.000000000000000000, 0.4999999999999985567, 0.8660254037844395958 ) ) ;
#38804=CARTESIAN_POINT ( 'NONE',  ( -13.25408968285182532, -2.882268652242222284, 31.66798894389554064 ) ) ;
#38805=VERTEX_POINT ( 'NONE', #63548 ) ;
#38806=CARTESIAN_POINT ( 'NONE',  ( 16.85399685940691938, -5.667676309546437530, 34.40238873228292249 ) ) ;
#38807=CARTESIAN_POINT ( 'NONE',  ( -0.4615384615384611200, -3.322132147404559976, 32.92929555188717927 ) ) ;
#38808=CARTESIAN_POINT ( 'NONE',  ( -1.384615384615505151, -3.835265460704628371, 33.15142922262033665 ) ) ;
#38809=AXIS2_PLACEMENT_3D ( 'NONE', #31579, #38789, #3651 ) ;
#38810=CARTESIAN_POINT ( 'NONE',  ( 4.826923076923076650, -7.500000000000001776, 34.75000000000000000 ) ) ;
#38811=ORIENTED_EDGE ( 'NONE', *, *, #63531, .T. ) ;
#38812=ORIENTED_EDGE ( 'NONE', *, *, #55059, .T. ) ;
#38813=AXIS2_PLACEMENT_3D ( 'NONE', #16982, #44431, #58849 ) ;
#38815=AXIS2_PLACEMENT_3D ( 'NONE', #2968, #56600, #30016 ) ;
#38816=VERTEX_POINT ( 'NONE', #76631 ) ;
#38817=CARTESIAN_POINT ( 'NONE',  ( 18.06616914096265702, -7.250054483168842268, 34.74374881642865631 ) ) ;
#38818=LINE ( 'NONE', #86118, #20303 ) ;
#38819=ORIENTED_EDGE ( 'NONE', *, *, #5963, .T. ) ;
#38820=CARTESIAN_POINT ( 'NONE',  ( -2.307692307692428724, -12.51329471203414379, 31.30864560766407578 ) ) ;
#38821=CARTESIAN_POINT ( 'NONE',  ( 6.699591979352975457, -10.81261337010820256, 33.49550067578627477 ) ) ;
#38822=CARTESIAN_POINT ( 'NONE',  ( 0.5920641633020261585, -12.27024696741798770, 31.24895572276497546 ) ) ;
#38823=EDGE_CURVE ( 'NONE', #30118, #76426, #70415, .T. ) ;
#38824=CARTESIAN_POINT ( 'NONE',  ( 5.076923076923075762, -6.343179335718451384, 34.87096338111211935 ) ) ;
#38825=AXIS2_PLACEMENT_3D ( 'NONE', #85690, #4143, #11356 ) ;
#38826=AXIS2_PLACEMENT_3D ( 'NONE', #87553, #34348, #13203 ) ;
#38827=CARTESIAN_POINT ( 'NONE',  ( -0.4615384615385826339, -11.48612834414049644, 32.76840700105863391 ) ) ;
#38828=ORIENTED_EDGE ( 'NONE', *, *, #27379, .T. ) ;
#38830=CARTESIAN_POINT ( 'NONE',  ( -15.29603923132555110, -12.16647553114622049, 32.15551576947930812 ) ) ;
#38831=VERTEX_POINT ( 'NONE', #50470 ) ;
#38832=CARTESIAN_POINT ( 'NONE',  ( 15.23076923076923173, -8.120952969808772792, 34.71129190930000163 ) ) ;
#38833=CARTESIAN_POINT ( 'NONE',  ( 14.98074600654777733, -4.931416488878822335, 34.32920672191015399 ) ) ;
#38834=DIRECTION ( 'NONE',  ( -0.000000000000000000, 0.1736481776669307198, -0.9848077530122080203 ) ) ;
#38836=CARTESIAN_POINT ( 'NONE',  ( 6.923076923076924238, -8.164416787775445883, 34.95778746994557906 ) ) ;
#38837=CARTESIAN_POINT ( 'NONE',  ( 18.13079180782478872, -2.541949514083464479, 30.39797389878540557 ) ) ;
#38839=EDGE_LOOP ( 'NONE', ( #77621, #22817, #79468, #50361 ) ) ;
#38840=CARTESIAN_POINT ( 'NONE',  ( 17.07692307692295586, -3.083524468854526912, 32.58852847137268327 ) ) ;
#38841=CARTESIAN_POINT ( 'NONE',  ( 2.372947447205147942, -4.320704448112861584, 33.92786785259548310 ) ) ;
#38843=EDGE_LOOP ( 'NONE', ( #49315, #27579 ) ) ;
#38844=EDGE_LOOP ( 'NONE', ( #15633, #34903 ) ) ;
#38845=CARTESIAN_POINT ( 'NONE',  ( -11.76194648218548622, -10.81261337010820256, 33.49550067578627477 ) ) ;
#38847=CARTESIAN_POINT ( 'NONE',  ( -10.61538461538461320, -13.75783147151868846, 33.36296068462461051 ) ) ;
#38848=DIRECTION ( 'NONE',  ( -0.000000000000000000, 0.3420201433256694901, -0.9396926207859082059 ) ) ;
#38849=CARTESIAN_POINT ( 'NONE',  ( 17.99999999999987566, -12.16647553114689728, 32.15551576947799362 ) ) ;
#38850=CARTESIAN_POINT ( 'NONE',  ( 12.46153846153846168, -11.11383981884818262, 36.00935417666054406 ) ) ;
#38851=ORIENTED_EDGE ( 'NONE', *, *, #42333, .F. ) ;
#38852=CARTESIAN_POINT ( 'NONE',  ( 5.869852790561777667, -3.817052484675422797, 33.13202310037935661 ) ) ;
#38853=EDGE_CURVE ( 'NONE', #519, #64802, #36098, .T. ) ;
#38854=EDGE_CURVE ( 'NONE', #28470, #85639, #9163, .T. ) ;
#38855=CARTESIAN_POINT ( 'NONE',  ( 6.989144256426998325, -6.343179335718452272, 34.87096338111212646 ) ) ;
#38856=CARTESIAN_POINT ( 'NONE',  ( -12.46153846153846168, -2.499999999999998668, 29.75000000000001421 ) ) ;
#38857=ORIENTED_EDGE ( 'NONE', *, *, #38423, .F. ) ;
#38858=CARTESIAN_POINT ( 'NONE',  ( -7.623374304885432551, -3.755027918224367767, 33.06320215134714857 ) ) ;
#38859=EDGE_CURVE ( 'NONE', #69859, #68982, #57310, .T. ) ;
#38860=ORIENTED_EDGE ( 'NONE', *, *, #63206, .T. ) ;
#38861=CARTESIAN_POINT ( 'NONE',  ( -0.4615384615384611200, -2.721908614388771852, 31.22303859784724978 ) ) ;
#38863=CARTESIAN_POINT ( 'NONE',  ( -1.634638621908349077, -9.271318131107980420, 34.42618302367067429 ) ) ;
#38864=CARTESIAN_POINT ( 'NONE',  ( 3.230769230769231726, -2.833524468853757305, 32.15551576947925838 ) ) ;
#38865=EDGE_LOOP ( 'NONE', ( #22908, #15563 ) ) ;
#38866=ADVANCED_FACE ( 'NONE', ( #62654 ), #84291, .F. ) ;
#38867=B_SPLINE_CURVE_WITH_KNOTS ( 'NONE', 3,
 ( #80177, #86044, #59457, #24321, #73868, #86959, #39198, #12165, #59004, #25226 ),
 .UNSPECIFIED., .F., .F.,
 ( 4, 2, 2, 2, 4 ),
 ( 0.000000000000000000, 0.0001954339857564067696, 0.0003908679715128135393, 0.0005863019572692202818, 0.0007817359430256270785 ),
 .UNSPECIFIED. ) ;
#38868=CARTESIAN_POINT ( 'NONE',  ( -13.38461538461550759, -5.094484230521993062, 34.41647553114689373 ) ) ;
#38869=CARTESIAN_POINT ( 'NONE',  ( -14.55769230769230660, -7.500000000000001776, 34.75000000000000000 ) ) ;
#38870=CARTESIAN_POINT ( 'NONE',  ( -1.384615384615383471, -8.564572088678739092, 35.78748833219616898 ) ) ;
#38871=EDGE_CURVE ( 'NONE', #76436, #75253, #20783, .T. ) ;
#38872=CARTESIAN_POINT ( 'NONE',  ( 11.53846153846153832, -1.242168528481310874, 33.36296068462461051 ) ) ;
#38873=CARTESIAN_POINT ( 'NONE',  ( -2.057746898314262385, -10.92531984108285670, 33.72920026020278073 ) ) ;
#38874=EDGE_LOOP ( 'NONE', ( #32248, #79279, #50738, #45072, #12753, #16043 ) ) ;
#38875=FACE_BOUND ( 'NONE', #23561, .T. ) ;
#38876=ORIENTED_EDGE ( 'NONE', *, *, #68157, .F. ) ;
#38877=CARTESIAN_POINT ( 'NONE',  ( 5.326868486301118644, -11.56426240980093745, 33.07394671870546432 ) ) ;
#38878=EDGE_CURVE ( 'NONE', #26509, #53886, #83172, .T. ) ;
#38879=CARTESIAN_POINT ( 'NONE',  ( 5.011652630962300847, -12.27809138561121394, 31.22303859784730307 ) ) ;
#38881=AXIS2_PLACEMENT_3D ( 'NONE', #38009, #53289, #19511 ) ;
#38882=FACE_OUTER_BOUND ( 'NONE', #74400, .T. ) ;
#38883=CARTESIAN_POINT ( 'NONE',  ( 9.942253101685734507, -2.589246495874658383, 31.60778113518102828 ) ) ;
#38889=ORIENTED_EDGE ( 'NONE', *, *, #25235, .T. ) ;
#38890=EDGE_LOOP ( 'NONE', ( #20173, #34817 ) ) ;
#38893=VERTEX_POINT ( 'NONE', #57244 ) ;
#38894=EDGE_CURVE ( 'NONE', #63694, #8816, #51863, .T. ) ;
#38895=ORIENTED_EDGE ( 'NONE', *, *, #60141, .T. ) ;
#38897=CARTESIAN_POINT ( 'NONE',  ( -11.78848477575450282, -9.271318131107980420, 34.42618302367067429 ) ) ;
#38898=DIRECTION ( 'NONE',  ( 0.000000000000000000, 0.000000000000000000, 1.000000000000000000 ) ) ;
#38899=EDGE_CURVE ( 'NONE', #37767, #11473, #73440, .T. ) ;
#38900=CARTESIAN_POINT ( 'NONE',  ( -7.053224132515142131, -3.285722584762969856, 32.44110544564090759 ) ) ;
#38901=CARTESIAN_POINT ( 'NONE',  ( 13.13459214732242408, -8.432397168068783699, 34.66272746175022945 ) ) ;
#38902=CARTESIAN_POINT ( 'NONE',  ( -12.68502338610279523, -12.47654668319379567, 31.42292124445336654 ) ) ;
#38903=CARTESIAN_POINT ( 'NONE',  ( -0.7115616988314266145, -11.86270091957321071, 32.19358267280088626 ) ) ;
#38904=CARTESIAN_POINT ( 'NONE',  ( -7.780085495151406683, -3.050289026998446840, 32.03036669348366416 ) ) ;
#38905=CARTESIAN_POINT ( 'NONE',  ( 12.46153846153833911, -11.94971097300221174, 32.03036669348237098 ) ) ;
#38906=ORIENTED_EDGE ( 'NONE', *, *, #6975, .T. ) ;
#38907=EDGE_LOOP ( 'NONE', ( #75259, #60702, #1742, #60329 ) ) ;
#38908=VERTEX_POINT ( 'NONE', #52697 ) ;
#38909=CARTESIAN_POINT ( 'NONE',  ( 0.3313904918067679950, -12.15440758774515473, 32.17923288041532004 ) ) ;
#38912=CARTESIAN_POINT ( 'NONE',  ( -16.08859058257012720, -6.879047030191284051, 34.71129190930002295 ) ) ;
#38913=CARTESIAN_POINT ( 'NONE',  ( 6.000000000000001776, -6.435427911321262684, 35.78748833219616898 ) ) ;
#38914=DIRECTION ( 'NONE',  ( 0.000000000000000000, 0.7660444431189807890, 0.6427876096865361433 ) ) ;
#38915=CARTESIAN_POINT ( 'NONE',  ( 4.403791672194295792, -2.587454068350147462, 30.68340429815432202 ) ) ;
#38916=FACE_BOUND ( 'NONE', #25877, .T. ) ;
#38917=ORIENTED_EDGE ( 'NONE', *, *, #20179, .F. ) ;
#38919=EDGE_LOOP ( 'NONE', ( #87562, #49940 ) ) ;
#38921=EDGE_LOOP ( 'NONE', ( #85523, #44608 ) ) ;
#38922=FACE_BOUND ( 'NONE', #26005, .T. ) ;
#38923=CARTESIAN_POINT ( 'NONE',  ( 7.716006636715625255, -11.93770438780619259, 32.05411857736982029 ) ) ;
#38924=CARTESIAN_POINT ( 'NONE',  ( -2.307692307692427391, -11.48612834414049644, 32.76840700105863391 ) ) ;
#38925=ORIENTED_EDGE ( 'NONE', *, *, #10410, .T. ) ;
#38926=CARTESIAN_POINT ( 'NONE',  ( 17.93391658904412012, -2.721908614388770964, 31.22303859784723912 ) ) ;
#38927=CARTESIAN_POINT ( 'NONE',  ( -1.634638608836840978, -8.475808217655753651, 34.90892951860618609 ) ) ;
#38928=DIRECTION ( 'NONE',  ( -0.000000000000000000, 0.9848077530122086864, -0.1736481776669273891 ) ) ;
#38929=ORIENTED_EDGE ( 'NONE', *, *, #40551, .F. ) ;
#38930=CARTESIAN_POINT ( 'NONE',  ( 9.692307692307695177, -11.91647553114624181, 32.58852847137148245 ) ) ;
#38931=CARTESIAN_POINT ( 'NONE',  ( -18.06527044596078113, -5.219633306516281657, 34.19971097300152252 ) ) ;
#38932=EDGE_CURVE ( 'NONE', #22144, #85987, #51789, .T. ) ;
#38933=CARTESIAN_POINT ( 'NONE',  ( -5.300408020647025431, -11.89387501736622710, 32.13663884655806413 ) ) ;
#38934=ORIENTED_EDGE ( 'NONE', *, *, #22721, .T. ) ;
#38935=ADVANCED_FACE ( 'NONE', ( #59464 ), #52251, .F. ) ;
#38936=CARTESIAN_POINT ( 'NONE',  ( 8.769230769230768274, -10.89733346790207413, 36.13435417666054406 ) ) ;
#38937=CARTESIAN_POINT ( 'NONE',  ( -17.01166750564705055, -11.94971097300157403, 32.03036669348361443 ) ) ;
#38938=VERTEX_POINT ( 'NONE', #65321 ) ;
#38939=CARTESIAN_POINT ( 'NONE',  ( -17.20761368003338632, -12.62707690430377383, 30.88035979386743435 ) ) ;
#38940=CARTESIAN_POINT ( 'NONE',  ( 14.37376065869474751, -8.120952969808772792, 34.71129190929999453 ) ) ;
#38941=CARTESIAN_POINT ( 'NONE',  ( -2.307692307692305711, -2.538708090699994813, 30.37095296980875503 ) ) ;
#38942=CARTESIAN_POINT ( 'NONE',  ( 15.16549923021291058, -12.70778746994557551, 30.41441678777548319 ) ) ;
#38943=DIRECTION ( 'NONE',  ( -0.000000000000000000, 0.1736481776669307198, -0.9848077530122080203 ) ) ;
#38945=CARTESIAN_POINT ( 'NONE',  ( 0.4615384615383382183, -11.67786785259630911, 32.92929555188603530 ) ) ;
#38946=CARTESIAN_POINT ( 'NONE',  ( -15.23076923076922995, -12.37446782046654192, 30.86335684631486131 ) ) ;
#38947=B_SPLINE_CURVE_WITH_KNOTS ( 'NONE', 3,
 ( #40571, #55836, #6342, #62154, #33797, #462, #27929, #83325, #61253, #44076 ),
 .UNSPECIFIED., .F., .F.,
 ( 4, 2, 2, 2, 4 ),
 ( 0.000000000000000000, 0.0001954311564186879044, 0.0003908623128373758088, 0.0005862934692560636861, 0.0007817246256747516176 ),
 .UNSPECIFIED. ) ;
#38948=VECTOR ( 'NONE', #5801, 1000.000000000000114 ) ;
#38949=CARTESIAN_POINT ( 'NONE',  ( 10.68145194873469173, -9.058645607665452459, 34.76329471203371924 ) ) ;
#38950=CARTESIAN_POINT ( 'NONE',  ( -14.98082382139119062, -2.589246495874658383, 31.60778113518102828 ) ) ;
#38951=CARTESIAN_POINT ( 'NONE',  ( -10.86540785267757947, -8.432397168068783699, 34.66272746175022945 ) ) ;
#38953=ORIENTED_EDGE ( 'NONE', *, *, #30260, .F. ) ;
#38955=ORIENTED_EDGE ( 'NONE', *, *, #11943, .T. ) ;
#38957=AXIS2_PLACEMENT_3D ( 'NONE', #4450, #44981, #85541 ) ;
#38959=DIRECTION ( 'NONE',  ( -0.000000000000000000, 0.9848077530122085754, -0.1736481776669273613 ) ) ;
#38960=ORIENTED_EDGE ( 'NONE', *, *, #8008, .T. ) ;
#38963=CARTESIAN_POINT ( 'NONE',  ( -13.25408994638174143, -5.915461855592780260, 34.75538340440931506 ) ) ;
#38964=CARTESIAN_POINT ( 'NONE',  ( 5.933916589044121892, -11.16473453929635440, 33.15142922261925662 ) ) ;
#38965=CYLINDRICAL_SURFACE ( 'NONE', #80675, 0.2500000000000004996 ) ;
#38966=CARTESIAN_POINT ( 'NONE',  ( -14.30769230769242917, -11.06231777344772027, 33.60647404775119895 ) ) ;
#38969=CARTESIAN_POINT ( 'NONE',  ( -7.715628144390285215, -2.882268652242222728, 31.66798894389554064 ) ) ;
#38970=CARTESIAN_POINT ( 'NONE',  ( -14.17690186672535901, -4.684288915650983043, 34.18129842949671371 ) ) ;
#38971=CARTESIAN_POINT ( 'NONE',  ( 1.384615384615386802, -1.367168528481310208, 33.57946703557072254 ) ) ;
#38973=CARTESIAN_POINT ( 'NONE',  ( 10.74591005361826213, -12.50538340440932394, 31.33453814440721885 ) ) ;
#38974=CARTESIAN_POINT ( 'NONE',  ( -17.74994558008654622, -2.318338780012836331, 30.59689888758630616 ) ) ;
#38975=CARTESIAN_POINT ( 'NONE',  ( -2.531177251416254936, -4.386631170607603991, 33.66268669641500111 ) ) ;
#38977=VERTEX_POINT ( 'NONE', #78835 ) ;
#38978=CARTESIAN_POINT ( 'NONE',  ( -9.561781990544126586, -3.816742781228458004, 33.13167719472716044 ) ) ;
#38979=DIRECTION ( 'NONE',  ( -0.000000000000000000, -0.9848077530122086864, -0.1736481776669273613 ) ) ;
#38980=CARTESIAN_POINT ( 'NONE',  ( -2.307692307692305711, -12.34228464037088635, 31.77849191805839268 ) ) ;
#38982=EDGE_CURVE ( 'NONE', #75052, #27477, #31087, .T. ) ;
#38983=CARTESIAN_POINT ( 'NONE',  ( 4.153846153846030731, -3.643525952248796163, 33.31231777344771672 ) ) ;
#38984=CARTESIAN_POINT ( 'NONE',  ( -0.4615384615385826339, -6.879047030192662504, 34.71129190930017927 ) ) ;
#38986=AXIS2_PLACEMENT_3D ( 'NONE', #84180, #15709, #8950 ) ;
#38987=B_SPLINE_CURVE_WITH_KNOTS ( 'NONE', 3,
 ( #4894, #32357, #3975, #73343, #11193, #51710, #38664, #46757, #40015, #86434 ),
 .UNSPECIFIED., .F., .F.,
 ( 4, 2, 2, 2, 4 ),
 ( 0.000000000000000000, 0.0001954339857564074473, 0.0003908679715128148945, 0.0005863019572692223418, 0.0007817359430256297891 ),
 .UNSPECIFIED. ) ;
#38988=ORIENTED_EDGE ( 'NONE', *, *, #45057, .T. ) ;
#38989=CARTESIAN_POINT ( 'NONE',  ( 3.165499230212911908, -6.835583212224499938, 34.95778746994557906 ) ) ;
#38990=EDGE_LOOP ( 'NONE', ( #18716, #18876 ) ) ;
#38991=VECTOR ( 'NONE', #55233, 1000.000000000000114 ) ;
#38992=ADVANCED_FACE ( 'NONE', ( #86508 ), #24784, .F. ) ;
#38993=ORIENTED_EDGE ( 'NONE', *, *, #33141, .F. ) ;
#38995=CARTESIAN_POINT ( 'NONE',  ( 5.777173307520998335, -7.369208160676172348, 34.74850200257122879 ) ) ;
#38996=CARTESIAN_POINT ( 'NONE',  ( 9.915087233576102221, -12.24180327182771855, 31.33663988360758879 ) ) ;
#38997=CARTESIAN_POINT ( 'NONE',  ( 6.223012844093396723, -8.282913670948747864, 34.94150082978203642 ) ) ;
#38998=DIRECTION ( 'NONE',  ( 0.000000000000000000, 0.1736481776669275834, 0.9848077530122086864 ) ) ;
#38999=ORIENTED_EDGE ( 'NONE', *, *, #85698, .T. ) ;
#39000=EDGE_CURVE ( 'NONE', #83351, #89000, #33707, .T. ) ;
#39002=ORIENTED_EDGE ( 'NONE', *, *, #67974, .F. ) ;
#39004=CARTESIAN_POINT ( 'NONE',  ( 1.134592147322421196, -11.37209801155882971, 32.91403422569032955 ) ) ;
#39005=CARTESIAN_POINT ( 'NONE',  ( 10.61538461538449418, -11.67786785259630911, 32.92929555188603530 ) ) ;
#39007=CARTESIAN_POINT ( 'NONE',  ( 9.019176178608811156, -5.766571408460171355, 34.70601412856602508 ) ) ;
#39008=VECTOR ( 'NONE', #76470, 999.9999999999998863 ) ;
#39009=DIRECTION ( 'NONE',  ( -0.000000000000000000, -0.5000000000000009992, -0.8660254037844380415 ) ) ;
#39010=CARTESIAN_POINT ( 'NONE',  ( -3.930419191984583005, -7.630147231320743018, 34.74852402298682819 ) ) ;
#39011=ADVANCED_FACE ( 'NONE', ( #87111 ), #73592, .F. ) ;
#39012=CARTESIAN_POINT ( 'NONE',  ( 5.934729554039225974, -12.46129190929999986, 30.37095296980880832 ) ) ;
#39013=ORIENTED_EDGE ( 'NONE', *, *, #36984, .F. ) ;
#39014=ORIENTED_EDGE ( 'NONE', *, *, #78657, .F. ) ;
#39015=CYLINDRICAL_SURFACE ( 'NONE', #30192, 0.2499999999999986955 ) ;
#39016=VECTOR ( 'NONE', #27847, 1000.000000000000000 ) ;
#39017=CARTESIAN_POINT ( 'NONE',  ( -12.68502340526241134, -11.41268669641500466, 32.86336882939237825 ) ) ;
#39018=ORIENTED_EDGE ( 'NONE', *, *, #30539, .F. ) ;
#39019=CYLINDRICAL_SURFACE ( 'NONE', #16265, 0.2499999999999994726 ) ;
#39020=CARTESIAN_POINT ( 'NONE',  ( -2.241624974342231180, -3.937682226553329556, 33.60647404775216529 ) ) ;
#39022=ORIENTED_EDGE ( 'NONE', *, *, #68440, .F. ) ;
#39023=EDGE_CURVE ( 'NONE', #35903, #81809, #62725, .T. ) ;
#39024=CARTESIAN_POINT ( 'NONE',  ( -13.63463862190834952, -12.22074536777954989, 31.39888409691088356 ) ) ;
#39026=CARTESIAN_POINT ( 'NONE',  ( 5.934729999443682402, -9.528491918058357157, 34.59228464037090589 ) ) ;
#39028=CARTESIAN_POINT ( 'NONE',  ( -12.33074665371367651, -12.38066358083363738, 30.83685684665853444 ) ) ;
#39029=CARTESIAN_POINT ( 'NONE',  ( -6.988347369037697376, -3.835265460703609186, 33.15142922261924241 ) ) ;
#39030=CARTESIAN_POINT ( 'NONE',  ( -15.10072406793445765, -2.504778602574660340, 29.97347330155780654 ) ) ;
#39031=CYLINDRICAL_SURFACE ( 'NONE', #26141, 0.2499999999999994726 ) ;
#39032=EDGE_LOOP ( 'NONE', ( #52235, #45775, #55075, #77280 ) ) ;
#39033=CARTESIAN_POINT ( 'NONE',  ( 11.53846153846141576, -11.67786785259630911, 32.92929555188603530 ) ) ;
#39034=DIRECTION ( 'NONE',  ( 0.000000000000000000, 0.000000000000000000, 1.000000000000000000 ) ) ;
#39035=DIRECTION ( 'NONE',  ( -0.000000000000000000, 0.5000000000000011102, -0.8660254037844380415 ) ) ;
#39036=EDGE_CURVE ( 'NONE', #72151, #65829, #33480, .T. ) ;
#39037=VERTEX_POINT ( 'NONE', #53742 ) ;
#39038=CIRCLE ( 'NONE', #204, 0.2500000000000002220 ) ;
#39039=CARTESIAN_POINT ( 'NONE',  ( -18.22348492456433178, -12.69144148231606017, 30.53333754910549303 ) ) ;
#39040=CARTESIAN_POINT ( 'NONE',  ( -12.46153846153846168, -9.819645486525091727, 36.12317359536749706 ) ) ;
#39043=LINE ( 'NONE', #68273, #4116 ) ;
#39045=FACE_BOUND ( 'NONE', #12336, .T. ) ;
#39046=CARTESIAN_POINT ( 'NONE',  ( 12.46153846153846168, -3.050289026998446396, 32.03036669348365706 ) ) ;
#39047=CARTESIAN_POINT ( 'NONE',  ( 4.284371592079800450, -12.70449254468099198, 30.44128974285582956 ) ) ;
#39048=CARTESIAN_POINT ( 'NONE',  ( 2.307692307692186251, -10.33852847137269571, 34.16647553114546554 ) ) ;
#39049=CARTESIAN_POINT ( 'NONE',  ( 1.384615384615386802, -12.62096338111211580, 30.90682066428153263 ) ) ;
#39050=DIRECTION ( 'NONE',  ( 0.000000000000000000, 0.7660444431189807890, 0.6427876096865361433 ) ) ;
#39051=CARTESIAN_POINT ( 'NONE',  ( 16.02369894440793630, -10.88202310037936194, 33.43294751532457099 ) ) ;
#39052=VECTOR ( 'NONE', #82497, 999.9999999999998863 ) ;
#39054=CARTESIAN_POINT ( 'NONE',  ( 13.25446741488368296, -2.647304123082328875, 31.75400227202885972 ) ) ;
#39056=EDGE_CURVE ( 'NONE', #75394, #76215, #13206, .T. ) ;
#39057=CARTESIAN_POINT ( 'NONE',  ( -8.703162418228330921, -5.557115091759786019, 34.35708131394839882 ) ) ;
#39058=ORIENTED_EDGE ( 'NONE', *, *, #65264, .T. ) ;
#39059=DIRECTION ( 'NONE',  ( 0.000000000000000000, 0.4999999999999985567, 0.8660254037844395958 ) ) ;
#39060=CARTESIAN_POINT ( 'NONE',  ( 16.15384615384603251, -12.70778746994576025, 30.41441678777401236 ) ) ;
#39062=FACE_OUTER_BOUND ( 'NONE', #43274, .T. ) ;
#39063=CARTESIAN_POINT ( 'NONE',  ( -8.769230769230768274, -5.557115091759785130, 34.35708131394839171 ) ) ;
#39064=LINE ( 'NONE', #39950, #22516 ) ;
#39066=CARTESIAN_POINT ( 'NONE',  ( 2.177545098254086930, -11.93770438780619259, 32.05411857736982029 ) ) ;
#39067=DIRECTION ( 'NONE',  ( -0.000000000000000000, 0.1736481776669307198, -0.9848077530122080203 ) ) ;
#39068=LINE ( 'NONE', #66529, #84928 ) ;
#39069=CARTESIAN_POINT ( 'NONE',  ( 5.326868486301119532, -12.68172785388650681, 30.59649109432439573 ) ) ;
#39072=CARTESIAN_POINT ( 'NONE',  ( 14.24242186173153435, -6.026961402152685388, 34.52809138561120506 ) ) ;
#39073=CARTESIAN_POINT ( 'NONE',  ( 7.846153846153723244, -9.528491918059723176, 34.59228464037033035 ) ) ;
#39074=ORIENTED_EDGE ( 'NONE', *, *, #61282, .T. ) ;
#39075=CARTESIAN_POINT ( 'NONE',  ( 17.20744877868662925, -2.882268652242222728, 31.66798894389554064 ) ) ;
#39076=CARTESIAN_POINT ( 'NONE',  ( 9.019176287578911655, -11.37275283266504111, 32.91324779482534524 ) ) ;
#39078=B_SPLINE_CURVE_WITH_KNOTS ( 'NONE', 3,
 ( #52460, #80401, #54233, #47033, #61001, #40743 ),
 .UNSPECIFIED., .F., .F.,
 ( 4, 2, 4 ),
 ( 0.000000000000000000, 0.0001954784845028902421, 0.0003909569690057804843 ),
 .UNSPECIFIED. ) ;
#39080=CARTESIAN_POINT ( 'NONE',  ( -15.23076923076891553, -2.255955759149395501, 30.00000000000324363 ) ) ;
#39081=CARTESIAN_POINT ( 'NONE',  ( 17.07692307692295586, -11.94971097300221174, 32.03036669348237098 ) ) ;
#39082=EDGE_LOOP ( 'NONE', ( #69131, #54319 ) ) ;
#39083=CARTESIAN_POINT ( 'NONE',  ( 7.173131234715238946, -8.303483539816728154, 34.68545999027711702 ) ) ;
#39085=CARTESIAN_POINT ( 'NONE',  ( 5.011653076366756387, -12.51329471203370325, 31.30864560766548976 ) ) ;
#39086=ORIENTED_EDGE ( 'NONE', *, *, #59387, .T. ) ;
#39087=CARTESIAN_POINT ( 'NONE',  ( -13.25382357679059986, -11.18335022499818621, 33.13157742990016885 ) ) ;
#39088=DIRECTION ( 'NONE',  ( 0.000000000000000000, 0.9848077530122072432, -0.1736481776669354937 ) ) ;
#39089=CARTESIAN_POINT ( 'NONE',  ( -12.46153846153858424, -8.656820664282941280, 34.87096338111179961 ) ) ;
#39090=VECTOR ( 'NONE', #21867, 1000.000000000000000 ) ;
#39091=CARTESIAN_POINT ( 'NONE',  ( -16.08767954725451332, -7.250054591869668386, 34.99404684341514127 ) ) ;
#39093=CARTESIAN_POINT ( 'NONE',  ( 2.373760658694747061, -12.10708131394839704, 31.69288490824020954 ) ) ;
#39094=CARTESIAN_POINT ( 'NONE',  ( -39.05038313613820122, -2.499999999999999556, 29.75000000000000355 ) ) ;
#39095=CARTESIAN_POINT ( 'NONE',  ( 3.903822916553186584, -10.05641848906368097, 34.04755513067966177 ) ) ;
#39096=VERTEX_POINT ( 'NONE', #40243 ) ;
#39097=ORIENTED_EDGE ( 'NONE', *, *, #48367, .T. ) ;
#39098=B_SPLINE_CURVE_WITH_KNOTS ( 'NONE', 3,
 ( #72050, #16660, #84707, #16229, #9470, #24301, #36934, #79266, #10361, #64396 ),
 .UNSPECIFIED., .F., .F.,
 ( 4, 2, 2, 2, 4 ),
 ( 0.0007817246256747483650, 0.0009771112852218926705, 0.001172497944769037084, 0.001367884604316181498, 0.001563271263863325695 ),
 .UNSPECIFIED. ) ;
#39099=EDGE_LOOP ( 'NONE', ( #5790, #18615, #9590, #56128, #23796, #21395 ) ) ;
#39100=DIRECTION ( 'NONE',  ( 0.000000000000000000, 0.000000000000000000, 1.000000000000000000 ) ) ;
#39101=CARTESIAN_POINT ( 'NONE',  ( -8.703162418228330921, -3.050289026998446840, 32.03036669348366416 ) ) ;
#39102=CARTESIAN_POINT ( 'NONE',  ( -12.71151519248081740, -3.627789207965226748, 32.91389620160131102 ) ) ;
#39103=CARTESIAN_POINT ( 'NONE',  ( 15.00728428704528383, -3.754499324213721234, 33.06261337010820256 ) ) ;
#39104=ORIENTED_EDGE ( 'NONE', *, *, #37792, .F. ) ;
#39105=B_SPLINE_CURVE_WITH_KNOTS ( 'NONE', 3,
 ( #4635, #11846, #64985, #24445, #59571, #32107, #60017, #17712, #87520, #59125 ),
 .UNSPECIFIED., .F., .F.,
 ( 4, 2, 2, 2, 4 ),
 ( 0.0007817246256747484735, 0.0009771112852218928873, 0.001172497944769037518, 0.001367884604316181932, 0.001563271263863326346 ),
 .UNSPECIFIED. ) ;
#39107=VERTEX_POINT ( 'NONE', #46547 ) ;
#39108=CARTESIAN_POINT ( 'NONE',  ( 4.376858997939548246, -5.582272713120727481, 34.63742843783360570 ) ) ;
#39109=VERTEX_POINT ( 'NONE', #6013 ) ;
#39110=CARTESIAN_POINT ( 'NONE',  ( 9.442307692307693401, -7.500000000000001776, 34.75000000000000000 ) ) ;
#39111=VECTOR ( 'NONE', #34519, 999.9999999999998863 ) ;
#39112=B_SPLINE_CURVE_WITH_KNOTS ( 'NONE', 3,
 ( #58481, #44080, #23375, #43651, #22939, #15754, #71561, #24256, #63919, #36893 ),
 .UNSPECIFIED., .F., .F.,
 ( 4, 2, 2, 2, 4 ),
 ( 0.0007817246256747516176, 0.0009771112852218965736, 0.001172497944769041421, 0.001367884604316186269, 0.001563271263863331333 ),
 .UNSPECIFIED. ) ;
#39113=CYLINDRICAL_SURFACE ( 'NONE', #14888, 0.2499999999999994726 ) ;
#39114=EDGE_CURVE ( 'NONE', #37680, #16668, #6452, .T. ) ;
#39115=CARTESIAN_POINT ( 'NONE',  ( 10.36540788444226102, -11.28823185664190376, 33.01397839955799896 ) ) ;
#39116=CARTESIAN_POINT ( 'NONE',  ( 16.08776377448601735, -11.35647404775217595, 33.31231777344666511 ) ) ;
#39117=ORIENTED_EDGE ( 'NONE', *, *, #31318, .F. ) ;
#39120=DIRECTION ( 'NONE',  ( -0.000000000000000000, 0.7660444431189791237, -0.6427876096865379196 ) ) ;
#39121=CARTESIAN_POINT ( 'NONE',  ( 5.207448778686639024, -5.195472089885680766, 34.18748526763464923 ) ) ;
#39122=EDGE_LOOP ( 'NONE', ( #38876, #33906, #31458, #21816 ) ) ;
#39123=CARTESIAN_POINT ( 'NONE',  ( 2.980745993476266342, -11.86270091957321249, 32.19358267280087915 ) ) ;
#39125=EDGE_CURVE ( 'NONE', #18841, #52308, #26216, .T. ) ;
#39126=CARTESIAN_POINT ( 'NONE',  ( 12.52679360105129724, -6.835583212224610072, 34.95778746994559327 ) ) ;
#39128=CARTESIAN_POINT ( 'NONE',  ( -17.07692307692307665, -12.10708131394839349, 31.69288490824020244 ) ) ;
#39129=FACE_BOUND ( 'NONE', #71254, .T. ) ;
#39130=CARTESIAN_POINT ( 'NONE',  ( -5.326946301144532825, -10.18141759479407327, 34.26406193332782379 ) ) ;
#39131=CARTESIAN_POINT ( 'NONE',  ( -6.065270000556318486, -12.51329471203370325, 31.30864560766548976 ) ) ;
#39132=AXIS2_PLACEMENT_3D ( 'NONE', #31497, #87352, #65270 ) ;
#39133=CARTESIAN_POINT ( 'NONE',  ( -8.834501215191544077, -4.481592998940162609, 33.73612834413957984 ) ) ;
#39134=DIRECTION ( 'NONE',  ( -0.000000000000000000, -0.9848077530122085754, -0.1736481776669273613 ) ) ;
#39135=CARTESIAN_POINT ( 'NONE',  ( 14.43821774592595375, -3.068774925481848825, 32.56582465632704526 ) ) ;
#39136=VECTOR ( 'NONE', #86976, 1000.000000000000000 ) ;
#39137=CARTESIAN_POINT ( 'NONE',  ( 0.3308469948709059638, -12.11776431015575994, 31.66791131148498906 ) ) ;
#39139=ORIENTED_EDGE ( 'NONE', *, *, #64949, .F. ) ;
#39140=CARTESIAN_POINT ( 'NONE',  ( 11.31497659473759043, -3.236172620538810385, 32.36188796281390267 ) ) ;
#39141=CARTESIAN_POINT ( 'NONE',  ( 12.71159288145191013, -3.435999193479609914, 33.07426656108010832 ) ) ;
#39142=VERTEX_POINT ( 'NONE', #67266 ) ;
#39143=EDGE_LOOP ( 'NONE', ( #49166, #40537, #46116, #64102, #26694, #31162 ) ) ;
#39144=AXIS2_PLACEMENT_3D ( 'NONE', #81072, #27886, #88288 ) ;
#39145=B_SPLINE_CURVE_WITH_KNOTS ( 'NONE', 3,
 ( #54394, #42557, #59823, #87324, #39578, #12533, #62797, #5332, #19291, #35346 ),
 .UNSPECIFIED., .F., .F.,
 ( 4, 2, 2, 2, 4 ),
 ( 0.0007817359430256320659, 0.0009771253907249987086, 0.001172514838424365460, 0.001367904286123732211, 0.001563293733823098962 ),
 .UNSPECIFIED. ) ;
#39146=CARTESIAN_POINT ( 'NONE',  ( -11.60373153901785948, -12.70778746994557551, 30.41441678777548319 ) ) ;
#39148=DIRECTION ( 'NONE',  ( 0.000000000000000000, 0.8660254037844377084, -0.5000000000000015543 ) ) ;
#39149=CARTESIAN_POINT ( 'NONE',  ( -13.38461538461550759, -5.094484230521993062, 34.41647553114689373 ) ) ;
#39150=LINE ( 'NONE', #59846, #80676 ) ;
#39151=ORIENTED_EDGE ( 'NONE', *, *, #49875, .T. ) ;
#39152=CARTESIAN_POINT ( 'NONE',  ( 14.37376065869474751, -8.973038597847271092, 34.52809138561121216 ) ) ;
#39154=ADVANCED_FACE ( 'NONE', ( #41121 ), #4678, .F. ) ;
#39155=CARTESIAN_POINT ( 'NONE',  ( -0.4615384615384611200, -13.53365097954675988, 30.81389545987213552 ) ) ;
#39158=CARTESIAN_POINT ( 'NONE',  ( -39.05038313613820122, -2.249999999999998668, 29.75000000000000355 ) ) ;
#39159=DIRECTION ( 'NONE',  ( 0.000000000000000000, 0.9396926207859126468, -0.3420201433256571111 ) ) ;
#39162=ORIENTED_EDGE ( 'NONE', *, *, #51673, .F. ) ;
#39163=EDGE_LOOP ( 'NONE', ( #16444, #62453, #25907, #49783 ) ) ;
#39165=ADVANCED_FACE ( 'NONE', ( #82566 ), #83449, .F. ) ;
#39166=CARTESIAN_POINT ( 'NONE',  ( 5.076923076923075762, -10.67929555188718282, 33.92786785259544047 ) ) ;
#39167=CARTESIAN_POINT ( 'NONE',  ( -17.93474486048716088, -3.643525952247861355, 33.31231777344670064 ) ) ;
#39168=CYLINDRICAL_SURFACE ( 'NONE', #38760, 0.2500000000000009437 ) ;
#39169=CARTESIAN_POINT ( 'NONE',  ( -0.3307000435256987059, -7.277220443632451463, 34.74524770363009196 ) ) ;
#39170=FACE_OUTER_BOUND ( 'NONE', #40728, .T. ) ;
#39172=CARTESIAN_POINT ( 'NONE',  ( -12.59222906464877134, -3.957541250942358424, 33.62499894934981626 ) ) ;
#39173=CARTESIAN_POINT ( 'NONE',  ( 1.634560902963528184, -5.057305518903949526, 34.11320923018887896 ) ) ;
#39174=CARTESIAN_POINT ( 'NONE',  ( 16.94677586748485609, -12.27039167877662251, 31.24851455888617835 ) ) ;
#39175=CARTESIAN_POINT ( 'NONE',  ( -5.999999999999683808, -2.255955759149395501, 30.00000000000324363 ) ) ;
#39176=CARTESIAN_POINT ( 'NONE',  ( -10.61538461538461320, -4.945431358278436385, 36.03766855953609394 ) ) ;
#39177=CARTESIAN_POINT ( 'NONE',  ( 15.00728430620489995, -12.47654668319379567, 31.42292124445336654 ) ) ;
#39178=AXIS2_PLACEMENT_3D ( 'NONE', #23944, #30711, #31150 ) ;
#39179=CARTESIAN_POINT ( 'NONE',  ( -2.980769230767794653, -7.500000000000155431, 34.75000000000007105 ) ) ;
#39180=CARTESIAN_POINT ( 'NONE',  ( -4.153846153846152411, -2.708943851104267164, 35.45975837776705220 ) ) ;
#39181=CYLINDRICAL_SURFACE ( 'NONE', #68073, 0.2499999999999986955 ) ;
#39182=LINE ( 'NONE', #88272, #18283 ) ;
#39183=VECTOR ( 'NONE', #54021, 1000.000000000000227 ) ;
#39184=ORIENTED_EDGE ( 'NONE', *, *, #26252, .F. ) ;
#39185=CARTESIAN_POINT ( 'NONE',  ( 8.835298102580845025, -4.661471528628508665, 34.16647553114624003 ) ) ;
#39186=CARTESIAN_POINT ( 'NONE',  ( 18.24994540937804643, -4.932303261841487263, 34.32971442181322885 ) ) ;
#39187=CARTESIAN_POINT ( 'NONE',  ( 13.25392478150507891, -6.369640206132551441, 34.87707690430378449 ) ) ;
#39189=CARTESIAN_POINT ( 'NONE',  ( 13.51514108637895006, -5.195472089885680766, 34.18748526763464923 ) ) ;
#39190=CARTESIAN_POINT ( 'NONE',  ( 14.05766908347085042, -4.931416488878822335, 34.32920672191015399 ) ) ;
#39191=CARTESIAN_POINT ( 'NONE',  ( -0.3310127597748989681, -2.619367082507848998, 30.83698974864644171 ) ) ;
#39194=CARTESIAN_POINT ( 'NONE',  ( 18.00000000000000000, -3.513871655860378418, 32.76840700105978499 ) ) ;
#39195=ORIENTED_EDGE ( 'NONE', *, *, #52394, .T. ) ;
#39196=CYLINDRICAL_SURFACE ( 'NONE', #65848, 0.2499999999999998890 ) ;
#39198=CARTESIAN_POINT ( 'NONE',  ( -18.22348494372394967, -11.89387501736623243, 32.13663884655804992 ) ) ;
#39199=CARTESIAN_POINT ( 'NONE',  ( 13.16113044089144068, -10.11188796281391511, 34.01382737946119050 ) ) ;
#39200=CARTESIAN_POINT ( 'NONE',  ( -0.2114840416250086119, -6.523592122091592671, 34.90882529074906415 ) ) ;
#39201=ORIENTED_EDGE ( 'NONE', *, *, #21835, .F. ) ;
#39203=ORIENTED_EDGE ( 'NONE', *, *, #20291, .F. ) ;
#39205=CIRCLE ( 'NONE', #72292, 0.2500000000000002220 ) ;
#39206=ORIENTED_EDGE ( 'NONE', *, *, #85141, .T. ) ;
#39207=VECTOR ( 'NONE', #48174, 1000.000000000000227 ) ;
#39208=LINE ( 'NONE', #25237, #73096 ) ;
#39209=CARTESIAN_POINT ( 'NONE',  ( 12.68454981315131214, -12.15243808032445827, 31.58219941686247978 ) ) ;
#39210=CARTESIAN_POINT ( 'NONE',  ( -10.48459280755982803, -6.413143153341454017, 34.63066358083362672 ) ) ;
#39211=CARTESIAN_POINT ( 'NONE',  ( 2.307692307692309264, -13.57706302396349152, 30.56769352161908060 ) ) ;
#39212=CARTESIAN_POINT ( 'NONE',  ( 6.923076923076924238, -8.164416787775445883, 34.95778746994557906 ) ) ;
#39213=CARTESIAN_POINT ( 'NONE',  ( 11.40831432902331954, -11.93770438780619259, 32.05411857736982029 ) ) ;
#39214=EDGE_CURVE ( 'NONE', #60261, #58859, #54115, .T. ) ;
#39215=CARTESIAN_POINT ( 'NONE',  ( -16.15384615384627409, -6.835583212225970762, 34.95778746994575670 ) ) ;
#39216=ORIENTED_EDGE ( 'NONE', *, *, #7224, .T. ) ;
#39217=EDGE_LOOP ( 'NONE', ( #66352, #50141 ) ) ;
#39218=ORIENTED_EDGE ( 'NONE', *, *, #86541, .T. ) ;
#39219=CARTESIAN_POINT ( 'NONE',  ( 3.480823542407545546, -3.627508038966689163, 32.91356715214248396 ) ) ;
#39220=VERTEX_POINT ( 'NONE', #14530 ) ;
#39221=EDGE_CURVE ( 'NONE', #68176, #32696, #70364, .T. ) ;
#39222=LINE ( 'NONE', #17618, #42096 ) ;
#39223=CARTESIAN_POINT ( 'NONE',  ( 9.561617089197383734, -5.496505350115501010, 34.60290016733514307 ) ) ;
#39225=VERTEX_POINT ( 'NONE', #84335 ) ;
#39226=CARTESIAN_POINT ( 'NONE',  ( -12.39628332202562433, -11.67786785259547777, 32.92929555188713664 ) ) ;
#39227=ORIENTED_EDGE ( 'NONE', *, *, #51825, .F. ) ;
#39229=EDGE_LOOP ( 'NONE', ( #18293, #52337, #29693, #70304 ) ) ;
#39230=VECTOR ( 'NONE', #13342, 999.9999999999998863 ) ;
#39231=CARTESIAN_POINT ( 'NONE',  ( -7.846153846153844924, -9.584722331328613620, 36.20867863119891439 ) ) ;
#39232=ADVANCED_FACE ( 'NONE', ( #7339 ), #41559, .F. ) ;
#39233=CARTESIAN_POINT ( 'NONE',  ( -11.53846153846165912, -10.90142922262034020, 33.41473453929536674 ) ) ;
#39234=CARTESIAN_POINT ( 'NONE',  ( -6.000000000000121680, -2.657715359629662988, 31.77849191805970364 ) ) ;
#39235=B_SPLINE_CURVE_WITH_KNOTS ( 'NONE', 3,
 ( #21874, #48899, #82255, #34056, #83140, #14677, #70507, #41705, #69176, #42160 ),
 .UNSPECIFIED., .F., .F.,
 ( 4, 2, 2, 2, 4 ),
 ( 0.0007817359430256313069, 0.0009771253907249971907, 0.001172514838424363291, 0.001367904286123729392, 0.001563293733823095276 ),
 .UNSPECIFIED. ) ;
#39236=FACE_BOUND ( 'NONE', #68248, .T. ) ;
#39237=CARTESIAN_POINT ( 'NONE',  ( -16.15384615384615330, -9.905515769479276145, 34.41647553114623292 ) ) ;
#39238=FACE_OUTER_BOUND ( 'NONE', #77178, .T. ) ;
#39239=B_SPLINE_CURVE_WITH_KNOTS ( 'NONE', 3,
 ( #43910, #23197, #57867, #10127, #29088, #2468, #22311, #36712, #44336, #3364 ),
 .UNSPECIFIED., .F., .F.,
 ( 4, 2, 2, 2, 4 ),
 ( 0.0007817359430256322827, 0.0009771253907249989254, 0.001172514838424365676, 0.001367904286123732428, 0.001563293733823098962 ),
 .UNSPECIFIED. ) ;
#39240=EDGE_CURVE ( 'NONE', #48079, #79735, #8978, .T. ) ;
#39242=CARTESIAN_POINT ( 'NONE',  ( 5.076923076923075762, -3.322132147404559976, 32.92929555188717927 ) ) ;
#39243=LINE ( 'NONE', #87896, #63904 ) ;
#39244=CARTESIAN_POINT ( 'NONE',  ( -5.076923076923075762, -2.721908614388771852, 31.22303859784724978 ) ) ;
#39245=ORIENTED_EDGE ( 'NONE', *, *, #65346, .T. ) ;
#39246=DIRECTION ( 'NONE',  ( -0.000000000000000000, -0.8660254037844399289, -0.4999999999999980016 ) ) ;
#39248=ORIENTED_EDGE ( 'NONE', *, *, #78781, .F. ) ;
#39249=CARTESIAN_POINT ( 'NONE',  ( -0.7115616988314267255, -9.271318131107980420, 34.42618302367067429 ) ) ;
#39250=CARTESIAN_POINT ( 'NONE',  ( 2.557746619330623528, -10.66356715214248396, 33.62249196103329751 ) ) ;
#39251=CARTESIAN_POINT ( 'NONE',  ( 3.230769230769108269, -3.643525952248796163, 33.31231777344771672 ) ) ;
#39252=CARTESIAN_POINT ( 'NONE',  ( 4.153846153846154188, -2.292212530054420494, 30.41441678777542634 ) ) ;
#39254=CARTESIAN_POINT ( 'NONE',  ( -13.16183584334697443, -2.847695495035523550, 31.58253572463339154 ) ) ;
#39255=ORIENTED_EDGE ( 'NONE', *, *, #47770, .F. ) ;
#39257=DIRECTION ( 'NONE',  ( 0.000000000000000000, 0.9848077530122072432, 0.1736481776669354937 ) ) ;
#39258=CARTESIAN_POINT ( 'NONE',  ( -5.076923076923197442, -2.625532179533778709, 30.86335684631627174 ) ) ;
#39259=CARTESIAN_POINT ( 'NONE',  ( 10.48523740594639619, -3.285722584762969856, 32.44110544564090759 ) ) ;
#39260=ADVANCED_FACE ( 'NONE', ( #15427 ), #63597, .F. ) ;
#39261=CARTESIAN_POINT ( 'NONE',  ( -3.453696189676078276, -12.64616026154729411, 30.79003144601913533 ) ) ;
#39262=VERTEX_POINT ( 'NONE', #83893 ) ;
#39263=ORIENTED_EDGE ( 'NONE', *, *, #59844, .T. ) ;
#39266=EDGE_LOOP ( 'NONE', ( #58910, #67888, #32195, #21999 ) ) ;
#39267=CIRCLE ( 'NONE', #43547, 0.2500000000000002220 ) ;
#39268=ADVANCED_FACE ( 'NONE', ( #29389 ), #22609, .F. ) ;
#39269=CARTESIAN_POINT ( 'NONE',  ( 18.25005441991345734, -12.65882529074907126, 30.72640787790838601 ) ) ;
#39270=CARTESIAN_POINT ( 'NONE',  ( -6.130475185075718869, -7.276987145209185215, 34.99546412871779211 ) ) ;
#39271=EDGE_CURVE ( 'NONE', #24035, #44409, #82056, .T. ) ;
#39272=EDGE_LOOP ( 'NONE', ( #57474, #22172 ) ) ;
#39273=CARTESIAN_POINT ( 'NONE',  ( -15.23076923076922995, -12.62096338111211580, 30.90682066428153263 ) ) ;
#39274=DIRECTION ( 'NONE',  ( 0.000000000000000000, 1.000000000000000000, 0.000000000000000000 ) ) ;
#39275=CARTESIAN_POINT ( 'NONE',  ( -8.769230769230890843, -6.879047030192662504, 34.71129190930017927 ) ) ;
#39276=CARTESIAN_POINT ( 'NONE',  ( -2.438383774359864198, -8.147922237126337563, 34.70805685702651999 ) ) ;
#39277=CARTESIAN_POINT ( 'NONE',  ( 6.000000000000001776, -2.499999999999998668, 29.75000000000001421 ) ) ;
#39279=CARTESIAN_POINT ( 'NONE',  ( -15.00798956179116317, -2.353885683473779800, 30.79025554430704403 ) ) ;
#39280=ORIENTED_EDGE ( 'NONE', *, *, #26133, .T. ) ;
#39281=CARTESIAN_POINT ( 'NONE',  ( -24.00000000000000000, -9.499999999999982236, 27.74999999999999645 ) ) ;
#39283=CARTESIAN_POINT ( 'NONE',  ( -13.60810032833933469, -5.113361153441934093, 34.14387501736622710 ) ) ;
#39284=CARTESIAN_POINT ( 'NONE',  ( 10.48469401227431419, -12.35290016733513951, 31.75349464988449455 ) ) ;
#39285=CARTESIAN_POINT ( 'NONE',  ( -8.703163435880695076, -8.164416787775445883, 34.95778746994558617 ) ) ;
#39287=B_SPLINE_CURVE_WITH_KNOTS ( 'NONE', 3,
 ( #26342, #25900, #19143, #67335, #18708, #11053, #59233, #60119, #53807, #88078 ),
 .UNSPECIFIED., .F., .F.,
 ( 4, 2, 2, 2, 4 ),
 ( 0.000000000000000000, 0.0001954339857564093175, 0.0003908679715128186350, 0.0005863019572692279796, 0.0007817359430256372700 ),
 .UNSPECIFIED. ) ;
#39288=DIRECTION ( 'NONE',  ( -0.000000000000000000, -0.5000000000000009992, -0.8660254037844380415 ) ) ;
#39290=ORIENTED_EDGE ( 'NONE', *, *, #70057, .F. ) ;
#39291=CARTESIAN_POINT ( 'NONE',  ( -8.769230769230768274, -5.471508081941601098, 34.59228464037088457 ) ) ;
#39292=CARTESIAN_POINT ( 'NONE',  ( -9.626239341305252495, -8.120952969808772792, 34.71129190929999453 ) ) ;
#39294=ORIENTED_EDGE ( 'NONE', *, *, #71828, .T. ) ;
#39295=ORIENTED_EDGE ( 'NONE', *, *, #46698, .F. ) ;
#39296=FACE_OUTER_BOUND ( 'NONE', #33000, .T. ) ;
#39297=CARTESIAN_POINT ( 'NONE',  ( 11.31553457955468645, -12.64616026154729411, 30.79003144601914244 ) ) ;
#39298=CARTESIAN_POINT ( 'NONE',  ( -0.6844654204453112234, -9.172386477786396597, 34.72672124145550043 ) ) ;
#39299=CARTESIAN_POINT ( 'NONE',  ( -7.146561866800870355, -5.912607949931405038, 34.49155766932282319 ) ) ;
#39300=AXIS2_PLACEMENT_3D ( 'NONE', #72627, #59558, #18586 ) ;
#39303=CARTESIAN_POINT ( 'NONE',  ( -6.989160334032803235, -11.69971097300155272, 32.46337939537587403 ) ) ;
#39304=ORIENTED_EDGE ( 'NONE', *, *, #29519, .F. ) ;
#39305=EDGE_CURVE ( 'NONE', #64026, #47786, #63149, .T. ) ;
#39306=CARTESIAN_POINT ( 'NONE',  ( -3.007756386675835447, -12.64618726649961289, 30.78989965857442712 ) ) ;
#39307=DIRECTION ( 'NONE',  ( -0.000000000000000000, 0.9848077530122086864, -0.1736481776669273891 ) ) ;
#39308=CARTESIAN_POINT ( 'NONE',  ( 4.088576153289833925, -8.656820664281497102, 34.87096338111211935 ) ) ;
#39309=ORIENTED_EDGE ( 'NONE', *, *, #83753, .F. ) ;
#39310=CARTESIAN_POINT ( 'NONE',  ( 12.71148397988660328, -3.712312575010499494, 33.01462480002815170 ) ) ;
#39311=ORIENTED_EDGE ( 'NONE', *, *, #77988, .T. ) ;
#39312=CARTESIAN_POINT ( 'NONE',  ( 13.44987095589141468, -3.835265460703683349, 33.15142922261929925 ) ) ;
#39313=CYLINDRICAL_SURFACE ( 'NONE', #2352, 0.2499999999999993616 ) ;
#39314=CARTESIAN_POINT ( 'NONE',  ( 15.48071464014727283, -4.932303261841489928, 34.32971442181322885 ) ) ;
#39316=CARTESIAN_POINT ( 'NONE',  ( -13.16183571563731647, -4.989023458446560255, 34.36081565061822118 ) ) ;
#39317=CYLINDRICAL_SURFACE ( 'NONE', #53601, 0.2500000000000002220 ) ;
#39318=ADVANCED_FACE ( 'NONE', ( #9537 ), #31134, .F. ) ;
#39319=CYLINDRICAL_SURFACE ( 'NONE', #33662, 0.2499999999999995559 ) ;
#39320=EDGE_CURVE ( 'NONE', #43306, #36328, #15368, .T. ) ;
#39321=B_SPLINE_CURVE_WITH_KNOTS ( 'NONE', 3,
 ( #35119, #22491, #30135, #42778, #57161, #1776, #2208, #63908, #49076, #29266 ),
 .UNSPECIFIED., .F., .F.,
 ( 4, 2, 2, 2, 4 ),
 ( 0.0007817359430256322827, 0.0009771253907249989254, 0.001172514838424365676, 0.001367904286123732428, 0.001563293733823099179 ),
 .UNSPECIFIED. ) ;
#39322=CARTESIAN_POINT ( 'NONE',  ( -6.066082379360133281, -5.471508081941601986, 34.59228464037088457 ) ) ;
#39323=CARTESIAN_POINT ( 'NONE',  ( -4.853910232829682592, -10.77377354290276301, 33.85451476688484718 ) ) ;
#39324=VECTOR ( 'NONE', #44272, 1000.000000000000000 ) ;
#39325=ORIENTED_EDGE ( 'NONE', *, *, #89058, .T. ) ;
#39326=CARTESIAN_POINT ( 'NONE',  ( -4.153846153846274980, -5.941354392335915335, 34.76329471203413846 ) ) ;
#39327=EDGE_LOOP ( 'NONE', ( #41921, #85826 ) ) ;
#39328=CARTESIAN_POINT ( 'NONE',  ( -15.16551409125639260, -6.835583212224610072, 34.95778746994559327 ) ) ;
#39330=CYLINDRICAL_SURFACE ( 'NONE', #31929, 0.2499999999999986955 ) ;
#39331=VECTOR ( 'NONE', #38554, 1000.000000000000227 ) ;
#39332=DIRECTION ( 'NONE',  ( -0.000000000000000000, 0.8660254037844399289, -0.4999999999999980016 ) ) ;
#39333=ADVANCED_FACE ( 'NONE', ( #23059 ), #52298, .F. ) ;
#39334=CARTESIAN_POINT ( 'NONE',  ( 5.076923076923075762, -11.69971097300155272, 32.46337939537588113 ) ) ;
#39335=CARTESIAN_POINT ( 'NONE',  ( -14.05763799605399278, -12.17597550085003633, 31.52189283813461884 ) ) ;
#39336=CARTESIAN_POINT ( 'NONE',  ( 4.946362485181154511, -2.504760397472873823, 29.97295953869789997 ) ) ;
#39337=CARTESIAN_POINT ( 'NONE',  ( 9.627037246346917598, -8.613356846314824011, 34.62446782046655613 ) ) ;
#39338=EDGE_CURVE ( 'NONE', #51322, #23856, #58607, .T. ) ;
#39339=EDGE_LOOP ( 'NONE', ( #73608, #77571, #61309, #68236 ) ) ;
#39340=ORIENTED_EDGE ( 'NONE', *, *, #48036, .T. ) ;
#39342=ORIENTED_EDGE ( 'NONE', *, *, #69703, .F. ) ;
#39343=EDGE_LOOP ( 'NONE', ( #39373, #78433 ) ) ;
#39346=CARTESIAN_POINT ( 'NONE',  ( -11.53846153846165912, -9.442884908241554243, 34.35708131394783038 ) ) ;
#39347=CARTESIAN_POINT ( 'NONE',  ( 15.23076923076923173, -4.786620604624113540, 33.94971097300155094 ) ) ;
#39348=CARTESIAN_POINT ( 'NONE',  ( 4.153846153846154188, -3.050289026998446396, 32.03036669348365706 ) ) ;
#39349=CARTESIAN_POINT ( 'NONE',  ( 0.5267940328144847806, -5.219633306516380244, 34.19971097300157936 ) ) ;
#39350=DIRECTION ( 'NONE',  ( 0.000000000000000000, 0.6427876096865368094, 0.7660444431189802339 ) ) ;
#39351=CARTESIAN_POINT ( 'NONE',  ( 17.93472955403921887, -2.625532179533444754, 30.86335684631481513 ) ) ;
#39352=CARTESIAN_POINT ( 'NONE',  ( 0.2115152242454947096, -3.202444869320336451, 32.30641848906366675 ) ) ;
#39353=ORIENTED_EDGE ( 'NONE', *, *, #33414, .F. ) ;
#39354=ORIENTED_EDGE ( 'NONE', *, *, #39881, .F. ) ;
#39355=ORIENTED_EDGE ( 'NONE', *, *, #72651, .F. ) ;
#39356=CARTESIAN_POINT ( 'NONE',  ( 24.00000000000000000, -9.499999999999982236, 27.25000000000000000 ) ) ;
#39357=ORIENTED_EDGE ( 'NONE', *, *, #40772, .T. ) ;
#39358=AXIS2_PLACEMENT_3D ( 'NONE', #44145, #57678, #37402 ) ;
#39359=CARTESIAN_POINT ( 'NONE',  ( -16.02305434602136103, -6.413143153341451352, 34.63066358083362672 ) ) ;
#39360=CARTESIAN_POINT ( 'NONE',  ( 10.48469314871706182, -8.999036380462717588, 34.52022231692819076 ) ) ;
#39361=CARTESIAN_POINT ( 'NONE',  ( -0.3310130233048166892, -2.372941743896879618, 30.88044141588254377 ) ) ;
#39362=CARTESIAN_POINT ( 'NONE',  ( 3.230769230769231726, -5.557115091759785130, 34.35708131394839171 ) ) ;
#39363=FACE_BOUND ( 'NONE', #36878, .T. ) ;
#39364=VERTEX_POINT ( 'NONE', #85651 ) ;
#39365=ADVANCED_FACE ( 'NONE', ( #37003 ), #78438, .F. ) ;
#39366=ORIENTED_EDGE ( 'NONE', *, *, #20674, .F. ) ;
#39367=LINE ( 'NONE', #80800, #21249 ) ;
#39368=ORIENTED_EDGE ( 'NONE', *, *, #65771, .F. ) ;
#39369=EDGE_CURVE ( 'NONE', #59454, #64208, #24826, .T. ) ;
#39370=FACE_BOUND ( 'NONE', #17870, .T. ) ;
#39371=CARTESIAN_POINT ( 'NONE',  ( -9.442253272394237840, -2.318338780012835443, 30.59689888758630261 ) ) ;
#39372=CARTESIAN_POINT ( 'NONE',  ( 18.13052570176355971, -5.195472089885680766, 34.18748526763464923 ) ) ;
#39373=ORIENTED_EDGE ( 'NONE', *, *, #75939, .F. ) ;
#39374=CARTESIAN_POINT ( 'NONE',  ( 2.057669070399343880, -8.432397168068783699, 34.66272746175022945 ) ) ;
#39375=CARTESIAN_POINT ( 'NONE',  ( -1.450697763975519194, -8.164416787775445883, 34.95778746994557906 ) ) ;
#39376=ADVANCED_FACE ( 'NONE', ( #9981 ), #79788, .F. ) ;
#39377=CARTESIAN_POINT ( 'NONE',  ( -18.06608237936013239, -3.937682226553330445, 33.60647404775217240 ) ) ;
#39378=ORIENTED_EDGE ( 'NONE', *, *, #29759, .F. ) ;
#39379=CARTESIAN_POINT ( 'NONE',  ( -7.715628407920200438, -8.630441415882550871, 34.87705825610312615 ) ) ;
#39380=CARTESIAN_POINT ( 'NONE',  ( 7.053602361310569613, -5.915461855592777596, 34.75538340440931506 ) ) ;
#39381=DIRECTION ( 'NONE',  ( -0.000000000000000000, 0.5000000000000011102, -0.8660254037844381525 ) ) ;
#39382=ORIENTED_EDGE ( 'NONE', *, *, #60698, .T. ) ;
#39383=CARTESIAN_POINT ( 'NONE',  ( 2.372947447205147942, -12.51329471203373700, 31.30864560766537963 ) ) ;
#39384=CARTESIAN_POINT ( 'NONE',  ( -17.07692307692307665, -11.69971097300155272, 32.46337939537588113 ) ) ;
#39385=VERTEX_POINT ( 'NONE', #86100 ) ;
#39386=CARTESIAN_POINT ( 'NONE',  ( 3.480714640147274164, -6.653508905675590945, 34.93172785388651391 ) ) ;
#39387=CARTESIAN_POINT ( 'NONE',  ( 14.37294787896833270, -8.613356846314928816, 34.62446782046653482 ) ) ;
#39388=CARTESIAN_POINT ( 'NONE',  ( -14.55766905174089665, -2.544273027872575366, 31.48422191005632342 ) ) ;
#39389=CARTESIAN_POINT ( 'NONE',  ( -4.153846153846152411, -11.33034616979429110, 35.88435417666054406 ) ) ;
#39390=DIRECTION ( 'NONE',  ( 0.000000000000000000, 0.9848077530122072432, -0.1736481776669354937 ) ) ;
#39391=CARTESIAN_POINT ( 'NONE',  ( 17.07692307692307665, -4.661471528628507777, 34.16647553114623292 ) ) ;
#39392=CARTESIAN_POINT ( 'NONE',  ( -8.769230769230768274, -4.098570777380720287, 33.41473453929634729 ) ) ;
#39393=CARTESIAN_POINT ( 'NONE',  ( 20.99999999999999645, -2.249999999999999556, 27.25000000000000000 ) ) ;
#39394=B_SPLINE_CURVE_WITH_KNOTS ( 'NONE', 3,
 ( #42212, #75984, #76432, #48952, #6642, #14283, #69231, #7533, #55706, #14736 ),
 .UNSPECIFIED., .F., .F.,
 ( 4, 2, 2, 2, 4 ),
 ( 0.000000000000000000, 0.0001954339857564071762, 0.0003908679715128143524, 0.0005863019572692215828, 0.0007817359430256287049 ),
 .UNSPECIFIED. ) ;
#39395=LINE ( 'NONE', #66854, #7990 ) ;
#39396=DIRECTION ( 'NONE',  ( 0.000000000000000000, 0.4999999999999985567, 0.8660254037844395958 ) ) ;
#39397=EDGE_CURVE ( 'NONE', #80197, #16713, #1487, .T. ) ;
#39399=B_SPLINE_CURVE_WITH_KNOTS ( 'NONE', 3,
 ( #15974, #8331, #7884, #35349, #84881, #36684, #64134, #62801, #1123, #70018 ),
 .UNSPECIFIED., .F., .F.,
 ( 4, 2, 2, 2, 4 ),
 ( 0.0007817359430256318490, 0.0009771253907249984917, 0.001172514838424365026, 0.001367904286123731560, 0.001563293733823098311 ),
 .UNSPECIFIED. ) ;
#39400=EDGE_LOOP ( 'NONE', ( #6900, #81018 ) ) ;
#39401=VECTOR ( 'NONE', #66556, 1000.000000000000000 ) ;
#39402=CARTESIAN_POINT ( 'NONE',  ( 5.011653076366756387, -6.835583212224499938, 34.95778746994557906 ) ) ;
#39403=ORIENTED_EDGE ( 'NONE', *, *, #13149, .T. ) ;
#39404=EDGE_CURVE ( 'NONE', #69679, #40761, #17608, .T. ) ;
#39405=ORIENTED_EDGE ( 'NONE', *, *, #9784, .T. ) ;
#39406=DIRECTION ( 'NONE',  ( -0.000000000000000000, -0.5000000000000009992, -0.8660254037844380415 ) ) ;
#39408=CARTESIAN_POINT ( 'NONE',  ( 18.25000000000143530, -7.500000000000155431, 34.75000000000007105 ) ) ;
#39410=CARTESIAN_POINT ( 'NONE',  ( -17.74994568836168440, -5.728107161865374941, 34.42597550085002922 ) ) ;
#39411=CARTESIAN_POINT ( 'NONE',  ( 5.869852790561783884, -11.47017969459903952, 32.78971311882034456 ) ) ;
#39412=CARTESIAN_POINT ( 'NONE',  ( -0.3310127597748990791, -6.001044277235011215, 34.52024696741798948 ) ) ;
#39413=FACE_OUTER_BOUND ( 'NONE', #38210, .T. ) ;
#39414=CARTESIAN_POINT ( 'NONE',  ( -4.946397638689434828, -2.647132371071621471, 31.75357179365173010 ) ) ;
#39415=CARTESIAN_POINT ( 'NONE',  ( -7.846153846153844924, -5.557115091759785130, 34.35708131394839171 ) ) ;
#39416=CARTESIAN_POINT ( 'NONE',  ( -7.715628144390278997, -12.27024696741798770, 31.24895572276497546 ) ) ;
#39418=EDGE_CURVE ( 'NONE', #80757, #19260, #41205, .T. ) ;
#39420=CARTESIAN_POINT ( 'NONE',  ( -4.283994123577847368, -12.15440758774515473, 32.17923288041532004 ) ) ;
#39421=CARTESIAN_POINT ( 'NONE',  ( 6.000000000000001776, -8.810774026931790459, 35.74407628777942847 ) ) ;
#39422=EDGE_CURVE ( 'NONE', #27582, #62474, #27057, .T. ) ;
#39423=EDGE_CURVE ( 'NONE', #14877, #37595, #60836, .T. ) ;
#39424=ORIENTED_EDGE ( 'NONE', *, *, #53715, .T. ) ;
#39425=ORIENTED_EDGE ( 'NONE', *, *, #40882, .T. ) ;
#39426=CARTESIAN_POINT ( 'NONE',  ( -9.561515884482908234, -3.530189275343204702, 32.79018710029569661 ) ) ;
#39427=CARTESIAN_POINT ( 'NONE',  ( 7.780883400193070898, -11.48612834413959582, 32.76840700105983473 ) ) ;
#39429=CARTESIAN_POINT ( 'NONE',  ( 15.48076923076917133, -7.565270000091922853, 34.99999999999999289 ) ) ;
#39430=CARTESIAN_POINT ( 'NONE',  ( -10.61538461538461320, -11.11383981884818262, 36.00935417666054406 ) ) ;
#39431=CARTESIAN_POINT ( 'NONE',  ( -9.692307692307691624, -6.343179335718451384, 34.87096338111211935 ) ) ;
#39432=EDGE_CURVE ( 'NONE', #19898, #31080, #16476, .T. ) ;
#39434=EDGE_CURVE ( 'NONE', #40036, #18264, #85235, .T. ) ;
#39435=ORIENTED_EDGE ( 'NONE', *, *, #22314, .T. ) ;
#39437=ORIENTED_EDGE ( 'NONE', *, *, #38663, .F. ) ;
#39438=ORIENTED_EDGE ( 'NONE', *, *, #30037, .F. ) ;
#39439=CARTESIAN_POINT ( 'NONE',  ( 5.142178648199100088, -8.613356846314928816, 34.62446782046653482 ) ) ;
#39440=CARTESIAN_POINT ( 'NONE',  ( -0.4615384615385840772, -5.094484230521993062, 34.41647553114689373 ) ) ;
#39441=CARTESIAN_POINT ( 'NONE',  ( 9.758376043310134307, -12.10708131394839704, 31.69288490824020954 ) ) ;
#39442=CARTESIAN_POINT ( 'NONE',  ( 11.78851595837499211, -2.318338780012835443, 30.59689888758630261 ) ) ;
#39443=CARTESIAN_POINT ( 'NONE',  ( -13.25382357679060519, -3.062576670634119758, 32.05464942895959979 ) ) ;
#39444=EDGE_CURVE ( 'NONE', #68800, #9134, #39700, .T. ) ;
#39445=ORIENTED_EDGE ( 'NONE', *, *, #27771, .F. ) ;
#39446=ORIENTED_EDGE ( 'NONE', *, *, #48726, .F. ) ;
#39447=B_SPLINE_CURVE_WITH_KNOTS ( 'NONE', 3,
 ( #16934, #44385, #71871, #37644, #65106, #4648, #60027, #87531, #48283, #82539 ),
 .UNSPECIFIED., .F., .F.,
 ( 4, 2, 2, 2, 4 ),
 ( 0.0007817359430256372700, 0.0009771253907250054306, 0.001172514838424373483, 0.001367904286123741535, 0.001563293733823109804 ),
 .UNSPECIFIED. ) ;
#39450=CARTESIAN_POINT ( 'NONE',  ( 17.20771351789002424, -9.929761469519743144, 34.40412654351204225 ) ) ;
#39451=CARTESIAN_POINT ( 'NONE',  ( 9.692307692307695177, -2.292212530054420494, 30.41441678777542634 ) ) ;
#39452=APPLICATION_CONTEXT ( 'automotive_design' ) ;
#39453=CARTESIAN_POINT ( 'NONE',  ( 8.835298102580843249, -5.471508081941601098, 34.59228464037088457 ) ) ;
#39454=VECTOR ( 'NONE', #77404, 1000.000000000000227 ) ;
#39455=VECTOR ( 'NONE', #6080, 1000.000000000000000 ) ;
#39456=CARTESIAN_POINT ( 'NONE',  ( -8.769230769230892619, -10.33852847137269571, 34.16647553114546554 ) ) ;
#39457=CARTESIAN_POINT ( 'NONE',  ( 17.93391658904412012, -4.786620604624113540, 33.94971097300155805 ) ) ;
#39458=CARTESIAN_POINT ( 'NONE',  ( -16.08859058257013430, -2.892918686051626054, 31.69288490824025928 ) ) ;
#39459=ORIENTED_EDGE ( 'NONE', *, *, #59045, .T. ) ;
#39460=ORIENTED_EDGE ( 'NONE', *, *, #461, .T. ) ;
#39461=CARTESIAN_POINT ( 'NONE',  ( 4.946775107191381693, -10.31621877034669588, 34.18098118002070152 ) ) ;
#39462=CARTESIAN_POINT ( 'NONE',  ( -4.826923076923076650, -2.249999999999998668, 29.75000000000000355 ) ) ;
#39463=ORIENTED_EDGE ( 'NONE', *, *, #10938, .T. ) ;
#39464=CARTESIAN_POINT ( 'NONE',  ( 8.096208157792160520, -12.41262288849542017, 30.68299917996395010 ) ) ;
#39467=VERTEX_POINT ( 'NONE', #32929 ) ;
#39468=CARTESIAN_POINT ( 'NONE',  ( 7.912221179503920787, -3.937682226553329556, 33.60647404775216529 ) ) ;
#39469=EDGE_LOOP ( 'NONE', ( #42940, #81270 ) ) ;
#39470=CARTESIAN_POINT ( 'NONE',  ( 7.846153846153846700, -6.435427911321262684, 35.78748833219616898 ) ) ;
#39471=CARTESIAN_POINT ( 'NONE',  ( 14.55763771707035126, -12.45601412856602686, 31.48342859153981621 ) ) ;
#39472=ADVANCED_FACE ( 'NONE', ( #60390 ), #59505, .F. ) ;
#39473=CARTESIAN_POINT ( 'NONE',  ( -12.46153846153858247, -12.46129190930018460, 30.37095296980731973 ) ) ;
#39474=CYLINDRICAL_SURFACE ( 'NONE', #40347, 0.2500000000000002220 ) ;
#39475=CARTESIAN_POINT ( 'NONE',  ( -9.692307692307691624, -8.564572088678739092, 35.78748833219616898 ) ) ;
#39476=FACE_OUTER_BOUND ( 'NONE', #70319, .T. ) ;
#39477=ORIENTED_EDGE ( 'NONE', *, *, #7844, .F. ) ;
#39478=CARTESIAN_POINT ( 'NONE',  ( 16.15384615384615330, -13.04860791097971706, 34.73218667398347037 ) ) ;
#39479=ADVANCED_FACE ( 'NONE', ( #5466 ), #26169, .F. ) ;
#39481=CYLINDRICAL_SURFACE ( 'NONE', #10611, 2.000000000000001776 ) ;
#39482=VERTEX_POINT ( 'NONE', #45987 ) ;
#39483=B_SPLINE_CURVE_WITH_KNOTS ( 'NONE', 3,
 ( #28872, #51642, #500, #77048, #1381, #27970, #62628, #16549, #44016, #37257 ),
 .UNSPECIFIED., .F., .F.,
 ( 4, 2, 2, 2, 4 ),
 ( 0.0007817359430256313069, 0.0009771253907249971907, 0.001172514838424363074, 0.001367904286123728958, 0.001563293733823094842 ),
 .UNSPECIFIED. ) ;
#39485=ADVANCED_FACE ( 'NONE', ( #5903 ), #73481, .F. ) ;
#39486=CARTESIAN_POINT ( 'NONE',  ( -9.692307692307814193, -5.094484230521993062, 34.41647553114689373 ) ) ;
#39487=CARTESIAN_POINT ( 'NONE',  ( -0.4615384615384611200, -5.471508081941601098, 34.59228464037088457 ) ) ;
#39488=CARTESIAN_POINT ( 'NONE',  ( 11.31553532094538994, -5.667676309546437530, 34.40238873228292249 ) ) ;
#39489=CARTESIAN_POINT ( 'NONE',  ( 8.992243613324164997, -10.01129605718032600, 34.36064277460058491 ) ) ;
#39490=FACE_BOUND ( 'NONE', #56060, .T. ) ;
#39492=CARTESIAN_POINT ( 'NONE',  ( -3.230769230769229949, -13.53365097954675988, 30.81389545987213552 ) ) ;
#39493=LINE ( 'NONE', #67836, #10885 ) ;
#39494=CARTESIAN_POINT ( 'NONE',  ( 1.384615384615264011, -12.70778746994576025, 30.41441678777401236 ) ) ;
#39495=CARTESIAN_POINT ( 'NONE',  ( -9.561781990544128362, -10.88167719472716399, 33.43325721877153711 ) ) ;
#39496=EDGE_CURVE ( 'NONE', #61245, #19826, #44368, .T. ) ;
#39497=CARTESIAN_POINT ( 'NONE',  ( 9.019285189144222059, -12.65882529074907126, 30.72640787790839312 ) ) ;
#39499=EDGE_LOOP ( 'NONE', ( #73520, #31121, #31244, #58880 ) ) ;
#39501=ORIENTED_EDGE ( 'NONE', *, *, #6543, .T. ) ;
#39502=CARTESIAN_POINT ( 'NONE',  ( 1.384615384615693667, -2.506253911140615021, 30.00000000000323297 ) ) ;
#39503=CARTESIAN_POINT ( 'NONE',  ( -3.931066612577741370, -12.24180327182771855, 31.33663988360758168 ) ) ;
#39505=CARTESIAN_POINT ( 'NONE',  ( -2.438383774359863754, -11.71456829005830080, 32.44064028649416542 ) ) ;
#39506=VERTEX_POINT ( 'NONE', #15319 ) ;
#39507=CARTESIAN_POINT ( 'NONE',  ( -9.942307692307691624, -7.500000000000001776, 35.00000000000000000 ) ) ;
#39508=CARTESIAN_POINT ( 'NONE',  ( -11.60373153901785770, -4.320704448112771878, 33.92786785259540494 ) ) ;
#39510=CARTESIAN_POINT ( 'NONE',  ( 15.10062126103754210, -12.15440758774515473, 32.17923288041532004 ) ) ;
#39511=CARTESIAN_POINT ( 'NONE',  ( 8.545745844666436497, -2.612411019501189369, 31.66733052389439962 ) ) ;
#39513=CARTESIAN_POINT ( 'NONE',  ( 5.299702745901141654, -12.69155399931963046, 30.53255429739158444 ) ) ;
#39514=CARTESIAN_POINT ( 'NONE',  ( -7.146561866800870355, -4.386631170607603991, 33.66268669641500111 ) ) ;
#39515=CARTESIAN_POINT ( 'NONE',  ( 1.384615384615386802, -9.905515769479276145, 34.41647553114623292 ) ) ;
#39517=VECTOR ( 'NONE', #78769, 1000.000000000000114 ) ;
#39518=CARTESIAN_POINT ( 'NONE',  ( -4.377331078410485077, -3.019605429927184836, 32.48692288466676814 ) ) ;
#39519=FACE_OUTER_BOUND ( 'NONE', #82629, .T. ) ;
#39520=ORIENTED_EDGE ( 'NONE', *, *, #87422, .T. ) ;
#39521=B_SPLINE_CURVE_WITH_KNOTS ( 'NONE', 3,
 ( #53400, #33589, #32687, #19184, #80902, #54283, #60158, #88553, #81340, #11992 ),
 .UNSPECIFIED., .F., .F.,
 ( 4, 2, 2, 2, 4 ),
 ( 0.0007817246256747477145, 0.0009771112852218909357, 0.001172497944769034265, 0.001367884604316177595, 0.001563271263863320708 ),
 .UNSPECIFIED. ) ;
#39522=DIRECTION ( 'NONE',  ( -0.000000000000000000, 0.5000000000000011102, -0.8660254037844381525 ) ) ;
#39523=CARTESIAN_POINT ( 'NONE',  ( 8.835299120233205628, -11.16473453929635440, 33.15142922261926373 ) ) ;
#39525=EDGE_CURVE ( 'NONE', #43394, #84175, #60495, .T. ) ;
#39526=VECTOR ( 'NONE', #27786, 1000.000000000000227 ) ;
#39527=AXIS2_PLACEMENT_3D ( 'NONE', #52433, #4254, #18223 ) ;
#39528=B_SPLINE_CURVE_WITH_KNOTS ( 'NONE', 3,
 ( #65488, #22720, #70922, #3786, #71795, #57395, #50637, #31264, #86228, #78116 ),
 .UNSPECIFIED., .F., .F.,
 ( 4, 2, 2, 2, 4 ),
 ( 0.000000000000000000, 0.0001954339857564091007, 0.0003908679715128182013, 0.0005863019572692273291, 0.0007817359430256364027 ),
 .UNSPECIFIED. ) ;
#39529=CARTESIAN_POINT ( 'NONE',  ( -10.83831157429146508, -2.523278758544489797, 31.42238647778637528 ) ) ;
#39530=CARTESIAN_POINT ( 'NONE',  ( -16.15384615384615330, -10.67929555188718282, 33.92786785259544047 ) ) ;
#39531=ORIENTED_EDGE ( 'NONE', *, *, #53932, .T. ) ;
#39532=CARTESIAN_POINT ( 'NONE',  ( 6.989145274079363368, -8.120952969808772792, 34.71129190929999453 ) ) ;
#39534=CARTESIAN_POINT ( 'NONE',  ( 11.28843831424008393, -2.985938066672154445, 32.43141759479405550 ) ) ;
#39535=VERTEX_POINT ( 'NONE', #82458 ) ;
#39536=CARTESIAN_POINT ( 'NONE',  ( -13.31935981333936070, -11.48612834413965977, 32.76840700105972815 ) ) ;
#39538=B_SPLINE_CURVE_WITH_KNOTS ( 'NONE', 3,
 ( #39431, #18258, #45723, #81300, #32221, #59682, #66889, #14157, #27670, #56025 ),
 .UNSPECIFIED., .F., .F.,
 ( 4, 2, 2, 2, 4 ),
 ( 0.000000000000000000, 0.0001954311564186868744, 0.0003908623128373737488, 0.0005862934692560606504, 0.0007817246256747474977 ),
 .UNSPECIFIED. ) ;
#39539=CARTESIAN_POINT ( 'NONE',  ( 15.36155967173618286, -5.496552790871120031, 34.60292014791297532 ) ) ;
#39540=CARTESIAN_POINT ( 'NONE',  ( -14.24162395668986747, -11.16473453929635440, 33.15142922261926373 ) ) ;
#39541=EDGE_CURVE ( 'NONE', #88546, #54362, #56190, .T. ) ;
#39542=VERTEX_POINT ( 'NONE', #8563 ) ;
#39543=CARTESIAN_POINT ( 'NONE',  ( 7.053121978996697017, -2.254550872974306674, 29.97347326024527447 ) ) ;
#39544=CARTESIAN_POINT ( 'NONE',  ( -15.45369618967607828, -11.43668979543635089, 33.22377378376089752 ) ) ;
#39545=EDGE_CURVE ( 'NONE', #3, #39385, #88435, .T. ) ;
#39546=EDGE_CURVE ( 'NONE', #44275, #2005, #63492, .T. ) ;
#39547=LINE ( 'NONE', #61556, #58510 ) ;
#39548=ORIENTED_EDGE ( 'NONE', *, *, #9409, .T. ) ;
#39549=ORIENTED_EDGE ( 'NONE', *, *, #5266, .F. ) ;
#39550=ORIENTED_EDGE ( 'NONE', *, *, #85621, .F. ) ;
#39551=CARTESIAN_POINT ( 'NONE',  ( -7.846153846153967493, -3.083524468854526912, 32.58852847137268327 ) ) ;
#39553=CARTESIAN_POINT ( 'NONE',  ( -12.46153846153858247, -3.835265460704628371, 33.15142922262033665 ) ) ;
#39554=EDGE_CURVE ( 'NONE', #46850, #83826, #62558, .T. ) ;
#39555=AXIS2_PLACEMENT_3D ( 'NONE', #31853, #79143, #30938 ) ;
#39556=CARTESIAN_POINT ( 'NONE',  ( 5.142178648199100977, -6.026961402152789304, 34.52809138561124769 ) ) ;
#39557=VERTEX_POINT ( 'NONE', #69377 ) ;
#39558=ADVANCED_FACE ( 'NONE', ( #30 ), #21621, .F. ) ;
#39559=EDGE_CURVE ( 'NONE', #46752, #31330, #911, .T. ) ;
#39561=EDGE_LOOP ( 'NONE', ( #63989, #66324 ) ) ;
#39563=ORIENTED_EDGE ( 'NONE', *, *, #31245, .T. ) ;
#39564=CARTESIAN_POINT ( 'NONE',  ( -16.28453675695646652, -12.35290016733513951, 31.75349464988449455 ) ) ;
#39565=ADVANCED_FACE ( 'NONE', ( #14881 ), #63038, .F. ) ;
#39567=CARTESIAN_POINT ( 'NONE',  ( 7.173022332454967120, -4.932303261841489039, 34.32971442181322885 ) ) ;
#39568=CARTESIAN_POINT ( 'NONE',  ( 16.08857615328983570, -11.67786785259541027, 32.92929555188721480 ) ) ;
#39569=EDGE_LOOP ( 'NONE', ( #14053, #38018, #10856, #54643 ) ) ;
#39570=B_SPLINE_CURVE_WITH_KNOTS ( 'NONE', 3,
 ( #84930, #34947, #28648, #50671, #78156, #83606, #70517, #62408, #28188, #55657 ),
 .UNSPECIFIED., .F., .F.,
 ( 4, 2, 2, 2, 4 ),
 ( 0.000000000000000000, 0.0001954311564186861968, 0.0003908623128373723936, 0.0005862934692560585904, 0.0007817246256747447872 ),
 .UNSPECIFIED. ) ;
#39571=ORIENTED_EDGE ( 'NONE', *, *, #45524, .T. ) ;
#39572=EDGE_LOOP ( 'NONE', ( #77953, #75000 ) ) ;
#39573=CARTESIAN_POINT ( 'NONE',  ( 14.43821774592595197, -11.04252011169590020, 33.62494198852677130 ) ) ;
#39574=CARTESIAN_POINT ( 'NONE',  ( -8.769230769230768274, -12.37446782046654192, 30.86335684631486131 ) ) ;
#39576=CARTESIAN_POINT ( 'NONE',  ( 16.85343815235874132, -5.827078755546626354, 34.72654668319379567 ) ) ;
#39577=CARTESIAN_POINT ( 'NONE',  ( 3.230769230769231726, -12.34228464037088635, 31.77849191805839268 ) ) ;
#39578=CARTESIAN_POINT ( 'NONE',  ( 16.40379167219429490, -8.433404298154332679, 34.66254593164985920 ) ) ;
#39579=LINE ( 'NONE', #45861, #42216 ) ;
#39580=CARTESIAN_POINT ( 'NONE',  ( -2.057746789344163663, -11.37275283266503756, 32.91324779482534524 ) ) ;
#39581=FACE_BOUND ( 'NONE', #5258, .T. ) ;
#39582=CARTESIAN_POINT ( 'NONE',  ( -5.300408001487407539, -10.23692288466677880, 34.23039457007281072 ) ) ;
#39583=CARTESIAN_POINT ( 'NONE',  ( -18.06608237936013595, -12.34228464037088280, 31.77849191805838558 ) ) ;
#39584=ADVANCED_FACE ( 'NONE', ( #35590 ), #28839, .F. ) ;
#39586=CARTESIAN_POINT ( 'NONE',  ( 11.66898724022510514, -12.45806712695776319, 30.39783852428763922 ) ) ;
#39587=DIRECTION ( 'NONE',  ( 0.000000000000000000, 0.1736481776669267785, -0.9848077530122087975 ) ) ;
#39588=CARTESIAN_POINT ( 'NONE',  ( -18.00000000000012079, -10.90142922262034020, 33.41473453929536674 ) ) ;
#39589=CARTESIAN_POINT ( 'NONE',  ( 0.3313912521002370104, -12.27039167877662251, 31.24851455888617835 ) ) ;
#39590=CARTESIAN_POINT ( 'NONE',  ( -0.5276218724943423366, -3.513871655860377086, 32.76840700105978499 ) ) ;
#39591=ORIENTED_EDGE ( 'NONE', *, *, #29298, .F. ) ;
#39592=CARTESIAN_POINT ( 'NONE',  ( 2.557746619330622639, -6.567000820036038355, 34.66262288849541306 ) ) ;
#39593=CARTESIAN_POINT ( 'NONE',  ( -13.13456096470193124, -4.074993327901527351, 33.72946981652012255 ) ) ;
#39594=ORIENTED_EDGE ( 'NONE', *, *, #54569, .F. ) ;
#39595=ORIENTED_EDGE ( 'NONE', *, *, #81406, .T. ) ;
#39597=EDGE_CURVE ( 'NONE', #25676, #43597, #34663, .T. ) ;
#39598=B_SPLINE_CURVE_WITH_KNOTS ( 'NONE', 3,
 ( #65633, #5286, #25556, #87726, #25109, #39534, #18804, #88175, #80511, #80963 ),
 .UNSPECIFIED., .F., .F.,
 ( 4, 2, 2, 2, 4 ),
 ( 0.000000000000000000, 0.0001954311564186860071, 0.0003908623128373720141, 0.0005862934692560580483, 0.0007817246256747440282 ),
 .UNSPECIFIED. ) ;
#39599=CARTESIAN_POINT ( 'NONE',  ( 15.93036121012220541, -3.754499324213721234, 33.06261337010820256 ) ) ;
#39600=CARTESIAN_POINT ( 'NONE',  ( 12.33084785842815378, -10.70098750199973203, 33.91152734681376302 ) ) ;
#39601=ORIENTED_EDGE ( 'NONE', *, *, #29331, .F. ) ;
#39603=CARTESIAN_POINT ( 'NONE',  ( -6.988347369037697376, -10.21337939537584383, 33.94971097300158647 ) ) ;
#39604=CARTESIAN_POINT ( 'NONE',  ( -15.48079246806219267, -5.851115903089112003, 34.47074536777953568 ) ) ;
#39606=CARTESIAN_POINT ( 'NONE',  ( -3.230769230769229949, -6.343179335718451384, 34.87096338111211935 ) ) ;
#39609=CARTESIAN_POINT ( 'NONE',  ( -16.15384615384615330, -2.900454961884010974, 35.62045528018868623 ) ) ;
#39611=ORIENTED_EDGE ( 'NONE', *, *, #46588, .T. ) ;
#39612=VERTEX_POINT ( 'NONE', #64806 ) ;
#39613=DIRECTION ( 'NONE',  ( 0.000000000000000000, 0.4999999999999985567, 0.8660254037844395958 ) ) ;
#39614=CARTESIAN_POINT ( 'NONE',  ( -17.75005459062195712, -3.520799739797213501, 33.17531984108286025 ) ) ;
#39615=CARTESIAN_POINT ( 'NONE',  ( 4.219040135629509081, -2.506253911140448487, 29.99999999999988631 ) ) ;
#39616=DIRECTION ( 'NONE',  ( -0.000000000000000000, 0.6427876096865404731, -0.7660444431189770143 ) ) ;
#39617=DIRECTION ( 'NONE',  ( -0.000000000000000000, -0.6427876096865404731, -0.7660444431189771253 ) ) ;
#39619=LINE ( 'NONE', #11695, #73407 ) ;
#39620=CARTESIAN_POINT ( 'NONE',  ( 14.17754433796061875, -6.809168938359901446, 34.95455904226513866 ) ) ;
#39621=AXIS2_PLACEMENT_3D ( 'NONE', #82485, #55877, #48672 ) ;
#39622=EDGE_CURVE ( 'NONE', #8848, #78089, #47574, .T. ) ;
#39623=CARTESIAN_POINT ( 'NONE',  ( -13.63461538461538680, -7.433931650972299465, 34.75000000000000711 ) ) ;
#39624=CARTESIAN_POINT ( 'NONE',  ( 5.934729999443682402, -10.33852847137145048, 34.16647553114627556 ) ) ;
#39625=CARTESIAN_POINT ( 'NONE',  ( 18.13052570176356326, -10.19071101563364401, 33.96452234770658407 ) ) ;
#39626=CARTESIAN_POINT ( 'NONE',  ( 8.519207531937805555, -12.22074536777954989, 31.39888409691088356 ) ) ;
#39628=LINE ( 'NONE', #65732, #63037 ) ;
#39630=DIRECTION ( 'NONE',  ( -0.000000000000000000, 1.000000000000000000, -0.000000000000000000 ) ) ;
#39631=ORIENTED_EDGE ( 'NONE', *, *, #48921, .F. ) ;
#39632=CARTESIAN_POINT ( 'NONE',  ( 1.384615384615386802, -2.538708090699994813, 30.37095296980875503 ) ) ;
#39633=DIRECTION ( 'NONE',  ( -1.000000000000000000, 0.000000000000000000, 0.000000000000000000 ) ) ;
#39634=CARTESIAN_POINT ( 'NONE',  ( 13.16113046005105680, -6.716662450894489211, 34.94144148231605840 ) ) ;
#39636=DIRECTION ( 'NONE',  ( -0.000000000000000000, -0.7660444431189791237, -0.6427876096865379196 ) ) ;
#39638=DIRECTION ( 'NONE',  ( -0.000000000000000000, -0.9848077530122085754, -0.1736481776669273613 ) ) ;
#39639=CARTESIAN_POINT ( 'NONE',  ( -18.06973409430282729, -2.249999999999999556, 29.49970722874968843 ) ) ;
#39640=ORIENTED_EDGE ( 'NONE', *, *, #44247, .T. ) ;
#39642=EDGE_CURVE ( 'NONE', #2951, #66107, #70067, .T. ) ;
#39643=CARTESIAN_POINT ( 'NONE',  ( 3.230769230769231726, -8.164416787775445883, 34.95778746994557906 ) ) ;
#39644=EDGE_CURVE ( 'NONE', #14452, #61423, #11055, .T. ) ;
#39645=ORIENTED_EDGE ( 'NONE', *, *, #75056, .T. ) ;
#39646=CARTESIAN_POINT ( 'NONE',  ( -2.084912766423896446, -2.600157965045225783, 30.74683119005207743 ) ) ;
#39647=VERTEX_POINT ( 'NONE', #38242 ) ;
#39648=CARTESIAN_POINT ( 'NONE',  ( 0.4615384615383382183, -6.835583212225970762, 34.95778746994575670 ) ) ;
#39649=CARTESIAN_POINT ( 'NONE',  ( -9.627052121031669074, -2.892918686051626498, 31.69288490824026638 ) ) ;
#39650=VECTOR ( 'NONE', #5247, 1000.000000000000227 ) ;
#39652=CARTESIAN_POINT ( 'NONE',  ( 2.307692307692186251, -12.70778746994576025, 30.41441678777401236 ) ) ;
#39653=VERTEX_POINT ( 'NONE', #58059 ) ;
#39654=ORIENTED_EDGE ( 'NONE', *, *, #69804, .T. ) ;
#39655=ORIENTED_EDGE ( 'NONE', *, *, #12544, .F. ) ;
#39656=CARTESIAN_POINT ( 'NONE',  ( -15.93083330975275658, -2.308499170217968466, 30.53291367094874076 ) ) ;
#39657=CARTESIAN_POINT ( 'NONE',  ( 7.173022332454966232, -11.56426240980093745, 33.07394671870546432 ) ) ;
#39659=CARTESIAN_POINT ( 'NONE',  ( -10.68146802634049486, -2.538708090699994813, 30.37095296980875148 ) ) ;
#39660=B_SPLINE_CURVE_WITH_KNOTS ( 'NONE', 3,
 ( #10396, #72531, #65327, #24335, #3625, #63556, #44152, #9497, #9941, #43295 ),
 .UNSPECIFIED., .F., .F.,
 ( 4, 2, 2, 2, 4 ),
 ( 0.0007817359430256257775, 0.0009771253907249911191, 0.001172514838424356352, 0.001367904286123721586, 0.001563293733823086819 ),
 .UNSPECIFIED. ) ;
#39661=VECTOR ( 'NONE', #72003, 1000.000000000000000 ) ;
#39662=DIRECTION ( 'NONE',  ( -0.000000000000000000, 0.6427876096865404731, -0.7660444431189770143 ) ) ;
#39663=CARTESIAN_POINT ( 'NONE',  ( -3.164701897419154530, -4.661471528628508665, 34.16647553114624003 ) ) ;
#39664=CARTESIAN_POINT ( 'NONE',  ( 0.2386115026316118215, -2.308479472611653094, 30.53278059502174457 ) ) ;
#39665=B_SPLINE_CURVE_WITH_KNOTS ( 'NONE', 3,
 ( #77749, #1657, #69229, #21928, #49402, #76874, #70555, #36332, #15174, #34992 ),
 .UNSPECIFIED., .F., .F.,
 ( 4, 2, 2, 2, 4 ),
 ( 0.000000000000000000, 0.0001954311564186881213, 0.0003908623128373762425, 0.0005862934692560643367, 0.0007817246256747524850 ),
 .UNSPECIFIED. ) ;
#39666=LINE ( 'NONE', #81091, #73669 ) ;
#39669=ORIENTED_EDGE ( 'NONE', *, *, #31665, .F. ) ;
#39670=ORIENTED_EDGE ( 'NONE', *, *, #74043, .T. ) ;
#39673=AXIS2_PLACEMENT_3D ( 'NONE', #25414, #51077, #51519 ) ;
#39674=FACE_OUTER_BOUND ( 'NONE', #17651, .T. ) ;
#39675=CARTESIAN_POINT ( 'NONE',  ( -8.769230769230768274, -9.905515769479276145, 34.41647553114623292 ) ) ;
#39676=EDGE_LOOP ( 'NONE', ( #65641, #10282, #2795, #47986 ) ) ;
#39677=CARTESIAN_POINT ( 'NONE',  ( 14.30769230769218581, -8.656820664282941280, 34.87096338111179961 ) ) ;
#39679=ORIENTED_EDGE ( 'NONE', *, *, #9098, .F. ) ;
#39680=CARTESIAN_POINT ( 'NONE',  ( 0.3309778697965401473, -2.504760397472875155, 29.97295953869789997 ) ) ;
#39681=ORIENTED_EDGE ( 'NONE', *, *, #47092, .T. ) ;
#39683=CARTESIAN_POINT ( 'NONE',  ( -8.992715712954719720, -5.113361153441934093, 34.14387501736622710 ) ) ;
#39684=B_SPLINE_CURVE_WITH_KNOTS ( 'NONE', 3,
 ( #38222, #32805, #11197, #78761, #53057, #80565, #11652, #44517, #5334, #44965 ),
 .UNSPECIFIED., .F., .F.,
 ( 4, 2, 2, 2, 4 ),
 ( 0.0007817359430256297891, 0.0009771253907249958896, 0.001172514838424362207, 0.001367904286123728524, 0.001563293733823094625 ),
 .UNSPECIFIED. ) ;
#39685=CARTESIAN_POINT ( 'NONE',  ( 1.384615384615386802, -6.435427911321262684, 35.78748833219616898 ) ) ;
#39686=FACE_BOUND ( 'NONE', #83725, .T. ) ;
#39687=B_SPLINE_CURVE_WITH_KNOTS ( 'NONE', 3,
 ( #50905, #29785, #22574, #10397, #71196, #23890, #64430, #16698, #31093, #36541 ),
 .UNSPECIFIED., .F., .F.,
 ( 4, 2, 2, 2, 4 ),
 ( 0.000000000000000000, 0.0001954339857564054144, 0.0003908679715128108288, 0.0005863019572692162703, 0.0007817359430256216575 ),
 .UNSPECIFIED. ) ;
#39688=DIRECTION ( 'NONE',  ( -1.000000000000000000, 0.000000000000000000, 0.000000000000000000 ) ) ;
#39689=LINE ( 'NONE', #59935, #6893 ) ;
#39690=CARTESIAN_POINT ( 'NONE',  ( -1.450697763975520083, -2.292212530054419606, 30.41441678777542634 ) ) ;
#39691=CARTESIAN_POINT ( 'NONE',  ( 4.403791672194294904, -8.433404298154334455, 34.66254593164985920 ) ) ;
#39692=DIRECTION ( 'NONE',  ( 0.000000000000000000, -1.000000000000000000, -8.673617379884033500E-16 ) ) ;
#39693=CARTESIAN_POINT ( 'NONE',  ( -4.219929564802032296, -11.16473453929635440, 33.15142922261925662 ) ) ;
#39694=EDGE_LOOP ( 'NONE', ( #4264, #70237, #29260, #28501 ) ) ;
#39695=LINE ( 'NONE', #5008, #33101 ) ;
#39696=ORIENTED_EDGE ( 'NONE', *, *, #69196, .T. ) ;
#39697=ORIENTED_EDGE ( 'NONE', *, *, #2312, .F. ) ;
#39699=CARTESIAN_POINT ( 'NONE',  ( -3.230769230769229949, -3.513871655860378418, 32.76840700105978499 ) ) ;
#39700=LINE ( 'NONE', #67160, #58569 ) ;
#39703=CARTESIAN_POINT ( 'NONE',  ( 12.46153846153833911, -10.33852847137269571, 34.16647553114546554 ) ) ;
#39704=ORIENTED_EDGE ( 'NONE', *, *, #20541, .F. ) ;
#39705=VECTOR ( 'NONE', #44321, 1000.000000000000114 ) ;
#39706=CARTESIAN_POINT ( 'NONE',  ( 17.32697738856139580, -3.136992222400443175, 32.19305428654138979 ) ) ;
#39707=CARTESIAN_POINT ( 'NONE',  ( 14.98074600654777377, -4.175268141568685643, 33.81360843649122216 ) ) ;
#39708=CARTESIAN_POINT ( 'NONE',  ( 2.530471976670372936, -12.69155399931963046, 30.53255429739157734 ) ) ;
#39711=EDGE_LOOP ( 'NONE', ( #68516, #88434, #31101, #48353 ) ) ;
#39712=ORIENTED_EDGE ( 'NONE', *, *, #16714, .F. ) ;
#39713=CARTESIAN_POINT ( 'NONE',  ( 4.153846153846030731, -12.16647553114689728, 32.15551576947799362 ) ) ;
#39714=CARTESIAN_POINT ( 'NONE',  ( -14.05763788777885281, -5.642605341092957971, 34.66089969410670335 ) ) ;
#39715=VERTEX_POINT ( 'NONE', #84234 ) ;
#39716=VECTOR ( 'NONE', #87660, 1000.000000000000000 ) ;
#39717=CARTESIAN_POINT ( 'NONE',  ( 3.230769230769231726, -12.62096338111211580, 30.90682066428153263 ) ) ;
#39718=CARTESIAN_POINT ( 'NONE',  ( 15.23076923076911093, -9.442884908241554243, 34.35708131394783038 ) ) ;
#39719=FACE_OUTER_BOUND ( 'NONE', #73815, .T. ) ;
#39720=CARTESIAN_POINT ( 'NONE',  ( 14.53065521125379611, -7.369474270740069777, 34.74850911626239736 ) ) ;
#39721=DIRECTION ( 'NONE',  ( -0.000000000000000000, -0.9396926207859093161, -0.3420201433256663259 ) ) ;
#39722=ORIENTED_EDGE ( 'NONE', *, *, #36049, .F. ) ;
#39723=CARTESIAN_POINT ( 'NONE',  ( -7.596208327805704208, -10.05730279482229683, 34.04704008940765902 ) ) ;
#39725=CARTESIAN_POINT ( 'NONE',  ( 2.307692307692309264, -13.20930481340135110, 34.54067556320372745 ) ) ;
#39727=LINE ( 'NONE', #47798, #35794 ) ;
#39728=CARTESIAN_POINT ( 'NONE',  ( 18.13079180782478872, -8.147973898785416225, 34.70805048591653730 ) ) ;
#39729=CARTESIAN_POINT ( 'NONE',  ( 2.438217745925951530, -2.647132371071621471, 31.75357179365173010 ) ) ;
#39730=CARTESIAN_POINT ( 'NONE',  ( -8.703975629717932705, -9.528491918058460186, 34.59228464037086326 ) ) ;
#39731=CARTESIAN_POINT ( 'NONE',  ( -0.5268089074992375886, -12.46129190929999986, 30.37095296980880832 ) ) ;
#39733=ORIENTED_EDGE ( 'NONE', *, *, #50588, .T. ) ;
#39735=CARTESIAN_POINT ( 'NONE',  ( 1.384615384615386802, -3.669653830205710676, 35.88435417666054406 ) ) ;
#39736=EDGE_CURVE ( 'NONE', #15629, #5929, #27152, .T. ) ;
#39737=VECTOR ( 'NONE', #55329, 1000.000000000000000 ) ;
#39738=EDGE_LOOP ( 'NONE', ( #42205, #60187 ) ) ;
#39739=ORIENTED_EDGE ( 'NONE', *, *, #73799, .T. ) ;
#39741=FACE_OUTER_BOUND ( 'NONE', #63507, .T. ) ;
#39742=ADVANCED_FACE ( 'NONE', ( #23819 ), #72019, .F. ) ;
#39743=CARTESIAN_POINT ( 'NONE',  ( 13.16113044089143713, -3.754499324213721234, 33.06261337010820256 ) ) ;
#39745=CARTESIAN_POINT ( 'NONE',  ( -0.4615384615385826339, -2.892918686052166066, 31.69288490824153470 ) ) ;
#39747=DIRECTION ( 'NONE',  ( -0.000000000000000000, 0.9396926207859092051, -0.3420201433256662704 ) ) ;
#39750=EDGE_CURVE ( 'NONE', #84034, #42820, #82988, .T. ) ;
#39751=CARTESIAN_POINT ( 'NONE',  ( 11.53846153846153832, -13.88283147151868846, 33.14645433367849847 ) ) ;
#39752=CARTESIAN_POINT ( 'NONE',  ( -3.360916440207452283, -11.93770438780619259, 32.05411857736982029 ) ) ;
#39753=ORIENTED_EDGE ( 'NONE', *, *, #64153, .F. ) ;
#39754=CARTESIAN_POINT ( 'NONE',  ( 15.93091919493930320, -12.38737895849757820, 31.66785238281580206 ) ) ;
#39755=ORIENTED_EDGE ( 'NONE', *, *, #53833, .F. ) ;
#39756=CARTESIAN_POINT ( 'NONE',  ( 13.38461538461526601, -3.300289026999228881, 32.46337939537708905 ) ) ;
#39757=CARTESIAN_POINT ( 'NONE',  ( 6.000000000000001776, -11.16473453929635440, 33.15142922261926373 ) ) ;
#39758=EDGE_LOOP ( 'NONE', ( #47335, #13562, #60957, #65694 ) ) ;
#39759=DIRECTION ( 'NONE',  ( 0.000000000000000000, 0.3420201433256641055, -0.9396926207859100932 ) ) ;
#39760=CARTESIAN_POINT ( 'NONE',  ( 13.51540582558233794, -9.084667340241226796, 34.75534355489798344 ) ) ;
#39761=FACE_OUTER_BOUND ( 'NONE', #12938, .T. ) ;
#39763=CARTESIAN_POINT ( 'NONE',  ( -0.7115616857599196265, -11.56360843649122216, 33.07473185843129926 ) ) ;
#39764=VECTOR ( 'NONE', #52448, 1000.000000000000000 ) ;
#39766=EDGE_LOOP ( 'NONE', ( #43699, #6117 ) ) ;
#39767=DIRECTION ( 'NONE',  ( -0.000000000000000000, 0.9396926207859092051, -0.3420201433256662704 ) ) ;
#39768=EDGE_CURVE ( 'NONE', #38893, #46048, #2415, .T. ) ;
#39769=ORIENTED_EDGE ( 'NONE', *, *, #75948, .F. ) ;
#39770=CARTESIAN_POINT ( 'NONE',  ( 8.769230769230647482, -12.46129190930018460, 30.37095296980731973 ) ) ;
#39771=EDGE_CURVE ( 'NONE', #1868, #83195, #68944, .T. ) ;
#39772=CARTESIAN_POINT ( 'NONE',  ( -12.33074802057151409, -2.845873456487965747, 32.17976146951972538 ) ) ;
#39774=EDGE_CURVE ( 'NONE', #72479, #85801, #59372, .T. ) ;
#39775=CYLINDRICAL_SURFACE ( 'NONE', #71774, 0.2499999999999979738 ) ;
#39776=VECTOR ( 'NONE', #82280, 1000.000000000000227 ) ;
#39777=CARTESIAN_POINT ( 'NONE',  ( -6.923076923077044142, -6.026961402154118908, 34.52809138561165270 ) ) ;
#39779=ORIENTED_EDGE ( 'NONE', *, *, #2412, .F. ) ;
#39780=ORIENTED_EDGE ( 'NONE', *, *, #63381, .T. ) ;
#39781=EDGE_LOOP ( 'NONE', ( #76438, #17179, #79001, #242 ) ) ;
#39782=EDGE_LOOP ( 'NONE', ( #62226, #47117, #88618, #81545 ) ) ;
#39783=CARTESIAN_POINT ( 'NONE',  ( -16.40382288478850725, -3.627789207965226304, 32.91389620160131102 ) ) ;
#39786=CARTESIAN_POINT ( 'NONE',  ( 3.930361210122205406, -3.236172620538810385, 32.36188796281390267 ) ) ;
#39787=CARTESIAN_POINT ( 'NONE',  ( -5.076923076923075762, -10.51840700105979565, 33.73612834413961536 ) ) ;
#39788=CARTESIAN_POINT ( 'NONE',  ( -5.143006487878958310, -8.120952969808774569, 34.71129190930000163 ) ) ;
#39790=CARTESIAN_POINT ( 'NONE',  ( 0.2380535178145122277, -3.236172620538810829, 32.36188796281390267 ) ) ;
#39791=ORIENTED_EDGE ( 'NONE', *, *, #35607, .T. ) ;
#39792=VERTEX_POINT ( 'NONE', #31939 ) ;
#39793=ORIENTED_EDGE ( 'NONE', *, *, #79530, .F. ) ;
#39794=CARTESIAN_POINT ( 'NONE',  ( 2.307692307692309264, -2.538708090699994813, 30.37095296980875503 ) ) ;
#39797=CARTESIAN_POINT ( 'NONE',  ( -7.911424292114620727, -4.481592998940162609, 33.73612834413957984 ) ) ;
#39798=EDGE_CURVE ( 'NONE', #33903, #70063, #50740, .T. ) ;
#39799=CARTESIAN_POINT ( 'NONE',  ( -0.2385256174450677280, -2.308499170217967134, 30.53291367094873721 ) ) ;
#39800=CARTESIAN_POINT ( 'NONE',  ( -15.45369618967607828, -10.01117774369187252, 34.36070679894347535 ) ) ;
#39801=FACE_BOUND ( 'NONE', #74525, .T. ) ;
#39802=ORIENTED_EDGE ( 'NONE', *, *, #50777, .F. ) ;
#39803=AXIS2_PLACEMENT_3D ( 'NONE', #50861, #85561, #84691 ) ;
#39804=EDGE_LOOP ( 'NONE', ( #88693, #60135 ) ) ;
#39805=CARTESIAN_POINT ( 'NONE',  ( -4.826977558574935045, -6.696923467548660192, 34.68552623307873972 ) ) ;
#39806=VERTEX_POINT ( 'NONE', #80119 ) ;
#39807=FACE_BOUND ( 'NONE', #42684, .T. ) ;
#39808=CARTESIAN_POINT ( 'NONE',  ( 9.692307692307570832, -5.941354392335915335, 34.76329471203413846 ) ) ;
#39809=CARTESIAN_POINT ( 'NONE',  ( 7.846153846154160227, -2.255955759149395501, 30.00000000000324363 ) ) ;
#39810=ORIENTED_EDGE ( 'NONE', *, *, #20494, .T. ) ;
#39811=LINE ( 'NONE', #46989, #47767 ) ;
#39813=CARTESIAN_POINT ( 'NONE',  ( -4.826923076923140599, -7.565270000091922853, 34.99999999999999289 ) ) ;
#39814=ORIENTED_EDGE ( 'NONE', *, *, #33261, .T. ) ;
#39815=B_SPLINE_CURVE_WITH_KNOTS ( 'NONE', 3,
 ( #49920, #44042, #23769, #57565, #85490, #64312, #51221, #57126, #70648, #43608 ),
 .UNSPECIFIED., .F., .F.,
 ( 4, 2, 2, 2, 4 ),
 ( 0.000000000000000000, 0.0001954339857564078267, 0.0003908679715128156535, 0.0005863019572692235344, 0.0007817359430256313069 ),
 .UNSPECIFIED. ) ;
#39816=CARTESIAN_POINT ( 'NONE',  ( -8.769230769230890843, -4.481592998941358097, 33.73612834414048933 ) ) ;
#39817=CARTESIAN_POINT ( 'NONE',  ( -3.453695448285377889, -2.758268499246657068, 31.33685645148949561 ) ) ;
#39818=CARTESIAN_POINT ( 'NONE',  ( 2.438482748659261734, -2.845873456487966635, 32.17976146951972538 ) ) ;
#39819=ORIENTED_EDGE ( 'NONE', *, *, #83296, .F. ) ;
#39820=ADVANCED_FACE ( 'NONE', ( #68705 ), #75909, .F. ) ;
#39821=CARTESIAN_POINT ( 'NONE',  ( -2.437839517130524492, -11.47017969459903952, 32.78971311882034456 ) ) ;
#39822=CARTESIAN_POINT ( 'NONE',  ( 2.557637717070352146, -3.520799739797214389, 33.17531984108286025 ) ) ;
#39823=ORIENTED_EDGE ( 'NONE', *, *, #18566, .T. ) ;
#39824=CARTESIAN_POINT ( 'NONE',  ( -12.52762084089859407, -5.471508081941602875, 34.59228464037088457 ) ) ;
#39825=CARTESIAN_POINT ( 'NONE',  ( -4.153846153846273204, -2.625532179533778709, 30.86335684631627174 ) ) ;
#39826=CARTESIAN_POINT ( 'NONE',  ( -14.43784027742400866, -2.647304123082328875, 31.75400227202885972 ) ) ;
#39827=CARTESIAN_POINT ( 'NONE',  ( -11.66915300512910214, -8.147922237126337563, 34.70805685702651999 ) ) ;
#39828=CARTESIAN_POINT ( 'NONE',  ( 0.3962684609821413018, -2.657715359629089669, 31.77849191805833584 ) ) ;
#39829=VECTOR ( 'NONE', #9176, 1000.000000000000000 ) ;
#39830=CARTESIAN_POINT ( 'NONE',  ( -0.3963454732438077555, -2.255955759149235185, 29.99999999999988987 ) ) ;
#39831=CARTESIAN_POINT ( 'NONE',  ( 5.999999999999880096, -11.94971097300221174, 32.03036669348237098 ) ) ;
#39832=DIRECTION ( 'NONE',  ( 0.000000000000000000, 0.7660444431189822323, -0.6427876096865344779 ) ) ;
#39833=CARTESIAN_POINT ( 'NONE',  ( 8.835299120233209180, -12.10708131394839704, 31.69288490824020954 ) ) ;
#39834=CARTESIAN_POINT ( 'NONE',  ( -12.39547011053602610, -11.16473453929635440, 33.15142922261926373 ) ) ;
#39836=VERTEX_POINT ( 'NONE', #27716 ) ;
#39837=VECTOR ( 'NONE', #33772, 1000.000000000000114 ) ;
#39838=CARTESIAN_POINT ( 'NONE',  ( 4.826946332874483936, -6.524016743844655686, 34.90889640711025521 ) ) ;
#39839=ORIENTED_EDGE ( 'NONE', *, *, #22253, .T. ) ;
#39840=ADVANCED_FACE ( 'NONE', ( #55186 ), #82682, .F. ) ;
#39842=CARTESIAN_POINT ( 'NONE',  ( -2.980714810855777497, -9.233818618650603938, 34.70587769442853698 ) ) ;
#39843=AXIS2_PLACEMENT_3D ( 'NONE', #35985, #43176, #2180 ) ;
#39844=ORIENTED_EDGE ( 'NONE', *, *, #26069, .F. ) ;
#39845=CARTESIAN_POINT ( 'NONE',  ( 1.449870524128224814, -12.16647553114626490, 32.15551576947920864 ) ) ;
#39847=CARTESIAN_POINT ( 'NONE',  ( 13.38461538461526601, -2.892918686052165622, 31.69288490824153470 ) ) ;
#39849=CARTESIAN_POINT ( 'NONE',  ( -18.22348492456433178, -12.11044203135682018, 32.26167407432752299 ) ) ;
#39850=CARTESIAN_POINT ( 'NONE',  ( -7.596099534515530216, -5.728107161865378494, 34.42597550085002922 ) ) ;
#39851=CARTESIAN_POINT ( 'NONE',  ( -8.546219417617919589, -4.887748414852792322, 34.01359900205216746 ) ) ;
#39853=CARTESIAN_POINT ( 'NONE',  ( -10.61538461538461320, -12.78798330534103123, 29.99999999999997868 ) ) ;
#39855=CARTESIAN_POINT ( 'NONE',  ( -7.053767526187232129, -4.684245665217972032, 34.18127051446801090 ) ) ;
#39856=CARTESIAN_POINT ( 'NONE',  ( -4.403869378067612139, -12.07920672191015221, 32.31858351112116168 ) ) ;
#39858=CARTESIAN_POINT ( 'NONE',  ( -16.15384615384615330, -1.215029322943914858, 32.30358669280327177 ) ) ;
#39860=ORIENTED_EDGE ( 'NONE', *, *, #66275, .T. ) ;
#39861=ORIENTED_EDGE ( 'NONE', *, *, #87230, .T. ) ;
#39862=B_SPLINE_CURVE_WITH_KNOTS ( 'NONE', 3,
 ( #72609, #56985, #3700, #25319, #56552, #63301, #59540, #37944, #45582, #18567 ),
 .UNSPECIFIED., .F., .F.,
 ( 4, 2, 2, 2, 4 ),
 ( 0.000000000000000000, 0.0001954311564186861697, 0.0003908623128373723394, 0.0005862934692560584820, 0.0007817246256747446788 ),
 .UNSPECIFIED. ) ;
#39863=AXIS2_PLACEMENT_3D ( 'NONE', #1142, #1590, #49333 ) ;
#39864=CARTESIAN_POINT ( 'NONE',  ( 6.792385456409365752, -2.541943142973490666, 30.39792223712631980 ) ) ;
#39865=CARTESIAN_POINT ( 'NONE',  ( 13.38461538461526423, -3.643525952248795718, 33.31231777344771672 ) ) ;
#39866=CARTESIAN_POINT ( 'NONE',  ( 16.37662582282421653, -12.47679350104403007, 31.42216943046555855 ) ) ;
#39867=DIRECTION ( 'NONE',  ( -0.000000000000000000, -0.9848077530122085754, -0.1736481776669273613 ) ) ;
#39869=LINE ( 'NONE', #46615, #79444 ) ;
#39870=CIRCLE ( 'NONE', #22559, 5.250000000000000888 ) ;
#39871=CARTESIAN_POINT ( 'NONE',  ( -16.37677237136229991, -9.086856451489516928, 34.49173150075333183 ) ) ;
#39872=EDGE_CURVE ( 'NONE', #53910, #44756, #77555, .T. ) ;
#39873=AXIS2_PLACEMENT_3D ( 'NONE', #51659, #71500, #77819 ) ;
#39874=VERTEX_POINT ( 'NONE', #77236 ) ;
#39875=CARTESIAN_POINT ( 'NONE',  ( -6.857008572074483332, -9.780366693483667717, 34.19971097300155805 ) ) ;
#39876=EDGE_LOOP ( 'NONE', ( #54098, #16283, #65546, #65647 ) ) ;
#39877=B_SPLINE_CURVE_WITH_KNOTS ( 'NONE', 3,
 ( #80847, #25884, #34407, #60995, #13257, #54228, #68204, #81725, #75402, #12374 ),
 .UNSPECIFIED., .F., .F.,
 ( 4, 2, 2, 2, 4 ),
 ( 0.000000000000000000, 0.0001954339857564098054, 0.0003908679715128196108, 0.0005863019572692293891, 0.0007817359430256392216 ),
 .UNSPECIFIED. ) ;
#39878=VERTEX_POINT ( 'NONE', #43890 ) ;
#39879=CARTESIAN_POINT ( 'NONE',  ( -14.17685388967953664, -7.277220443632450575, 34.74524770363009196 ) ) ;
#39880=CARTESIAN_POINT ( 'NONE',  ( -14.17690186672535901, -6.369690395747422684, 34.87708834333098196 ) ) ;
#39881=EDGE_CURVE ( 'NONE', #27959, #58891, #46462, .T. ) ;
#39884=CARTESIAN_POINT ( 'NONE',  ( 1.134592160393928406, -11.56360843649122216, 33.07473185843129926 ) ) ;
#39886=VERTEX_POINT ( 'NONE', #21851 ) ;
#39887=ORIENTED_EDGE ( 'NONE', *, *, #76776, .T. ) ;
#39889=ORIENTED_EDGE ( 'NONE', *, *, #1768, .F. ) ;
#39890=ORIENTED_EDGE ( 'NONE', *, *, #87918, .F. ) ;
#39891=CARTESIAN_POINT ( 'NONE',  ( 5.749976762707036393, -2.587272538249754117, 30.68239716806877837 ) ) ;
#39892=CARTESIAN_POINT ( 'NONE',  ( 9.823098133274644539, -2.295524264805589354, 30.44142389570982488 ) ) ;
#39893=B_SPLINE_CURVE_WITH_KNOTS ( 'NONE', 3,
 ( #12565, #27846, #53987, #382, #54424, #14330, #33284, #34604, #81034, #40052 ),
 .UNSPECIFIED., .F., .F.,
 ( 4, 2, 2, 2, 4 ),
 ( 0.000000000000000000, 0.0001954339857564072304, 0.0003908679715128144608, 0.0005863019572692216913, 0.0007817359430256289217 ),
 .UNSPECIFIED. ) ;
#39895=CARTESIAN_POINT ( 'NONE',  ( -15.23076923076922995, -2.708943851104267164, 35.45975837776705220 ) ) ;
#39897=EDGE_CURVE ( 'NONE', #66304, #80196, #37845, .T. ) ;
#39899=CARTESIAN_POINT ( 'NONE',  ( -10.39260507411620083, -12.24180327182772388, 31.33663988360758168 ) ) ;
#39900=VECTOR ( 'NONE', #76501, 1000.000000000000227 ) ;
#39902=EDGE_LOOP ( 'NONE', ( #12972, #62784, #20302, #84087 ) ) ;
#39903=CARTESIAN_POINT ( 'NONE',  ( 17.32686859527121825, -12.43552623307873972, 30.55307653245132826 ) ) ;
#39904=ORIENTED_EDGE ( 'NONE', *, *, #57231, .T. ) ;
#39905=CARTESIAN_POINT ( 'NONE',  ( 10.61538461538461675, -11.11383981884818262, 36.00935417666054406 ) ) ;
#39906=CARTESIAN_POINT ( 'NONE',  ( 7.976199008988623440, -2.504778602574660340, 29.97347330155780654 ) ) ;
#39907=EDGE_CURVE ( 'NONE', #4994, #45619, #73253, .T. ) ;
#39909=EDGE_LOOP ( 'NONE', ( #48172, #34685 ) ) ;
#39913=DIRECTION ( 'NONE',  ( -0.000000000000000000, -0.5000000000000009992, -0.8660254037844380415 ) ) ;
#39914=CARTESIAN_POINT ( 'NONE',  ( 14.43848274865925774, -12.35292014791297710, 31.75344720912887198 ) ) ;
#39916=CARTESIAN_POINT ( 'NONE',  ( -7.053768389744485390, -3.530157926970578508, 32.79014554554150607 ) ) ;
#39917=ADVANCED_FACE ( 'NONE', ( #38479 ), #10107, .F. ) ;
#39918=CARTESIAN_POINT ( 'NONE',  ( -17.07692307692307665, -13.63283147151868846, 33.57946703557072254 ) ) ;
#39922=CYLINDRICAL_SURFACE ( 'NONE', #40888, 0.2500000000000009437 ) ;
#39923=ORIENTED_EDGE ( 'NONE', *, *, #78427, .F. ) ;
#39924=EDGE_CURVE ( 'NONE', #48285, #17504, #42168, .T. ) ;
#39925=B_SPLINE_CURVE_WITH_KNOTS ( 'NONE', 3,
 ( #12166, #39649, #45491, #31539, #5409, #32876, #72971, #79288, #87853, #26118 ),
 .UNSPECIFIED., .F., .F.,
 ( 4, 2, 2, 2, 4 ),
 ( 0.0007817359430256293554, 0.0009771253907249941549, 0.001172514838424358954, 0.001367904286123723537, 0.001563293733823095276 ),
 .UNSPECIFIED. ) ;
#39928=CARTESIAN_POINT ( 'NONE',  ( 17.14299142792552288, -9.780366693483667717, 34.19971097300155805 ) ) ;
#39929=CARTESIAN_POINT ( 'NONE',  ( -2.373775718648185595, -10.51840700105979387, 33.73612834413961536 ) ) ;
#39930=CARTESIAN_POINT ( 'NONE',  ( 0.4615384615384611200, -13.63283147151868846, 33.57946703557072254 ) ) ;
#39931=FACE_BOUND ( 'NONE', #24387, .T. ) ;
#39932=CARTESIAN_POINT ( 'NONE',  ( -7.146003881983771677, -12.38737895849757820, 31.66785238281580206 ) ) ;
#39934=VECTOR ( 'NONE', #84381, 1000.000000000000227 ) ;
#39935=CARTESIAN_POINT ( 'NONE',  ( -9.469528023329626620, -12.11081565061824250, 32.26097654155340422 ) ) ;
#39936=CARTESIAN_POINT ( 'NONE',  ( -8.703162418228330921, -11.69971097300155272, 32.46337939537588113 ) ) ;
#39937=CARTESIAN_POINT ( 'NONE',  ( 17.77707378248385339, -11.24512374952581872, 33.06303171183252942 ) ) ;
#39938=CARTESIAN_POINT ( 'NONE',  ( 8.769230769230768274, -12.62096338111211580, 30.90682066428153263 ) ) ;
#39941=CARTESIAN_POINT ( 'NONE',  ( 10.48469401227431419, -11.93127051446799847, 32.56575433478202797 ) ) ;
#39942=VERTEX_POINT ( 'NONE', #79012 ) ;
#39944=VERTEX_POINT ( 'NONE', #38930 ) ;
#39945=CARTESIAN_POINT ( 'NONE',  ( 7.716006636715625255, -9.418419913701741919, 34.36755862841477693 ) ) ;
#39946=CARTESIAN_POINT ( 'NONE',  ( -7.846153846153844924, -11.35647404775217417, 33.31231777344666511 ) ) ;
#39947=CARTESIAN_POINT ( 'NONE',  ( 6.000000000000001776, -9.058645607665452459, 34.76329471203371924 ) ) ;
#39948=ORIENTED_EDGE ( 'NONE', *, *, #69732, .F. ) ;
#39949=CARTESIAN_POINT ( 'NONE',  ( -17.07692307692307665, -2.292212530054420494, 30.41441678777542634 ) ) ;
#39950=CARTESIAN_POINT ( 'NONE',  ( -7.846153846153844924, -13.78497067705608181, 32.30358669280327177 ) ) ;
#39952=EDGE_CURVE ( 'NONE', #71524, #24900, #3793, .T. ) ;
#39953=CARTESIAN_POINT ( 'NONE',  ( 2.177000841024752109, -11.71456829005830080, 32.44064028649416542 ) ) ;
#39954=DIRECTION ( 'NONE',  ( -0.000000000000000000, 0.3420201433256694346, -0.9396926207859080948 ) ) ;
#39956=CARTESIAN_POINT ( 'NONE',  ( -11.53846153846153655, -11.33034616979429110, 35.88435417666054406 ) ) ;
#39957=CARTESIAN_POINT ( 'NONE',  ( -1.384615384615506484, -6.835583212225970762, 34.95778746994575670 ) ) ;
#39958=FACE_OUTER_BOUND ( 'NONE', #78999, .T. ) ;
#39960=CARTESIAN_POINT ( 'NONE',  ( 9.915734654169265028, -7.630147231320743018, 34.74852402298682819 ) ) ;
#39961=DIRECTION ( 'NONE',  ( -0.000000000000000000, 0.5000000000000011102, -0.8660254037844381525 ) ) ;
#39965=AXIS2_PLACEMENT_3D ( 'NONE', #5449, #32916, #61701 ) ;
#39968=CARTESIAN_POINT ( 'NONE',  ( -8.992157728137618378, -3.395401636524185474, 33.02366814457250399 ) ) ;
#39969=ORIENTED_EDGE ( 'NONE', *, *, #44983, .T. ) ;
#39970=CARTESIAN_POINT ( 'NONE',  ( 3.230769230769231726, -12.10708131394839349, 31.69288490824020244 ) ) ;
#39972=CARTESIAN_POINT ( 'NONE',  ( 5.010840697562939816, -12.34228464037088280, 31.77849191805838558 ) ) ;
#39973=ORIENTED_EDGE ( 'NONE', *, *, #20438, .T. ) ;
#39974=CARTESIAN_POINT ( 'NONE',  ( 12.59206416330202671, -12.45806712695776319, 30.39783852428763922 ) ) ;
#39976=CARTESIAN_POINT ( 'NONE',  ( -17.32692307692307665, -7.433932668274255917, 35.00000000000000711 ) ) ;
#39977=DIRECTION ( 'NONE',  ( 1.000000000000000000, 0.000000000000000000, 0.000000000000000000 ) ) ;
#39978=VERTEX_POINT ( 'NONE', #86687 ) ;
#39979=CYLINDRICAL_SURFACE ( 'NONE', #56390, 0.2499999999999979738 ) ;
#39981=ADVANCED_FACE ( 'NONE', ( #23617 ), #51067, .F. ) ;
#39982=EDGE_CURVE ( 'NONE', #73792, #77192, #18208, .T. ) ;
#39983=CARTESIAN_POINT ( 'NONE',  ( -13.13466997523734037, -8.476813868363244353, 34.90874843262270133 ) ) ;
#39984=ORIENTED_EDGE ( 'NONE', *, *, #67974, .T. ) ;
#39985=EDGE_LOOP ( 'NONE', ( #8913, #84872, #8419, #42634 ) ) ;
#39986=EDGE_CURVE ( 'NONE', #84435, #67271, #45670, .T. ) ;
#39987=ORIENTED_EDGE ( 'NONE', *, *, #23262, .T. ) ;
#39989=CARTESIAN_POINT ( 'NONE',  ( 0.2115617305961063066, -8.303909089506435137, 34.68538101551103381 ) ) ;
#39990=FACE_OUTER_BOUND ( 'NONE', #767, .T. ) ;
#39991=EDGE_CURVE ( 'NONE', #28559, #54595, #5627, .T. ) ;
#39992=CARTESIAN_POINT ( 'NONE',  ( -16.40386937806761125, -2.985938066672154445, 32.43141759479405550 ) ) ;
#39994=B_SPLINE_CURVE_WITH_KNOTS ( 'NONE', 3,
 ( #80778, #59593, #5100, #53724, #19495, #81211, #18620, #33016, #12740, #11868 ),
 .UNSPECIFIED., .F., .F.,
 ( 4, 2, 2, 2, 4 ),
 ( 0.000000000000000000, 0.0001954311564186868473, 0.0003908623128373736946, 0.0005862934692560605419, 0.0007817246256747473893 ),
 .UNSPECIFIED. ) ;
#39995=EDGE_CURVE ( 'NONE', #67434, #67903, #84121, .T. ) ;
#39996=CARTESIAN_POINT ( 'NONE',  ( -16.94639737515951339, -5.195472089885680766, 34.18748526763464923 ) ) ;
#39997=EDGE_LOOP ( 'NONE', ( #9562, #43762 ) ) ;
#39998=ORIENTED_EDGE ( 'NONE', *, *, #49325, .F. ) ;
#39999=ORIENTED_EDGE ( 'NONE', *, *, #84173, .F. ) ;
#40000=CARTESIAN_POINT ( 'NONE',  ( -8.069638789877792817, -5.113361153441934093, 34.14387501736622710 ) ) ;
#40001=ORIENTED_EDGE ( 'NONE', *, *, #44604, .F. ) ;
#40003=ADVANCED_FACE ( 'NONE', ( #10560 ), #79466, .F. ) ;
#40004=CARTESIAN_POINT ( 'NONE',  ( 12.52760579488853665, -11.35647404775217595, 33.31231777344666511 ) ) ;
#40005=ADVANCED_FACE ( 'NONE', ( #4696 ), #45220, .F. ) ;
#40006=CARTESIAN_POINT ( 'NONE',  ( -12.33074665371367651, -12.11778462344220841, 31.66786338562085135 ) ) ;
#40008=ORIENTED_EDGE ( 'NONE', *, *, #51307, .F. ) ;
#40009=EDGE_LOOP ( 'NONE', ( #43258, #59975 ) ) ;
#40010=ORIENTED_EDGE ( 'NONE', *, *, #51268, .F. ) ;
#40011=CARTESIAN_POINT ( 'NONE',  ( -10.61538461538461320, -10.67929555188718282, 33.92786785259544047 ) ) ;
#40012=CARTESIAN_POINT ( 'NONE',  ( -1.384615384615383471, -3.669653830205710676, 35.88435417666054406 ) ) ;
#40013=VERTEX_POINT ( 'NONE', #52865 ) ;
#40014=CARTESIAN_POINT ( 'NONE',  ( 2.242422307135989001, -2.657715359629089225, 31.77849191805834295 ) ) ;
#40015=CARTESIAN_POINT ( 'NONE',  ( -13.44988583057615905, -6.879047030191174805, 34.71129190930000163 ) ) ;
#40016=ORIENTED_EDGE ( 'NONE', *, *, #17407, .T. ) ;
#40017=DIRECTION ( 'NONE',  ( -0.000000000000000000, -0.5000000000000009992, -0.8660254037844380415 ) ) ;
#40018=CARTESIAN_POINT ( 'NONE',  ( 8.992010310499175318, -12.44528174975671853, 30.48912976160716681 ) ) ;
#40019=CARTESIAN_POINT ( 'NONE',  ( 0.2386115026316108223, -9.172386477786396597, 34.72672124145550043 ) ) ;
#40020=B_SPLINE_CURVE_WITH_KNOTS ( 'NONE', 3,
 ( #14855, #30123, #42767, #22917, #57590, #2198, #2634, #43199, #85077, #49945 ),
 .UNSPECIFIED., .F., .F.,
 ( 4, 2, 2, 2, 4 ),
 ( 0.0007817246256747507503, 0.0009771112852218957062, 0.001172497944769040771, 0.001367884604316185835, 0.001563271263863330682 ),
 .UNSPECIFIED. ) ;
#40021=AXIS2_PLACEMENT_3D ( 'NONE', #30702, #65811, #59511 ) ;
#40022=FACE_BOUND ( 'NONE', #39400, .T. ) ;
#40023=ADVANCED_FACE ( 'NONE', ( #47440 ), #87574, .F. ) ;
#40024=CARTESIAN_POINT ( 'NONE',  ( -0.5922299282060213832, -9.804603061927743113, 34.18744698557895845 ) ) ;
#40025=LINE ( 'NONE', #33257, #31331 ) ;
#40026=CARTESIAN_POINT ( 'NONE',  ( -10.61538461538461320, -10.67929555188718282, 33.92786785259544047 ) ) ;
#40027=CARTESIAN_POINT ( 'NONE',  ( -7.145955605505568187, -7.630691491037286056, 34.74850469731152458 ) ) ;
#40028=CARTESIAN_POINT ( 'NONE',  ( -5.999999999999998224, -2.721908614388771852, 31.22303859784724978 ) ) ;
#40030=B_SPLINE_CURVE_WITH_KNOTS ( 'NONE', 3,
 ( #56319, #77038, #1812, #29302, #56755, #84251, #22530, #49994, #77474, #37359 ),
 .UNSPECIFIED., .F., .F.,
 ( 4, 2, 2, 2, 4 ),
 ( 0.0007817246256747457630, 0.0009771112852218887673, 0.001172497944769031663, 0.001367884604316174559, 0.001563271263863317672 ),
 .UNSPECIFIED. ) ;
#40031=FACE_OUTER_BOUND ( 'NONE', #20070, .T. ) ;
#40032=CARTESIAN_POINT ( 'NONE',  ( 12.46153846153846168, -2.833524468853757305, 32.15551576947925838 ) ) ;
#40033=ORIENTED_EDGE ( 'NONE', *, *, #60948, .T. ) ;
#40034=CARTESIAN_POINT ( 'NONE',  ( -15.23076923076935252, -11.67786785259630911, 32.92929555188603530 ) ) ;
#40035=CARTESIAN_POINT ( 'NONE',  ( -13.16183571563731469, -4.226511098958373402, 33.85474049983370293 ) ) ;
#40036=VERTEX_POINT ( 'NONE', #40262 ) ;
#40037=ORIENTED_EDGE ( 'NONE', *, *, #16464, .T. ) ;
#40038=FACE_OUTER_BOUND ( 'NONE', #37669, .T. ) ;
#40039=EDGE_CURVE ( 'NONE', #47287, #51433, #68015, .T. ) ;
#40040=CARTESIAN_POINT ( 'NONE',  ( -15.23076923076935074, -2.625532179533778709, 30.86335684631627174 ) ) ;
#40042=ORIENTED_EDGE ( 'NONE', *, *, #70797, .T. ) ;
#40044=CARTESIAN_POINT ( 'NONE',  ( -6.923076923077045919, -9.528491918059723176, 34.59228464037033035 ) ) ;
#40045=FACE_BOUND ( 'NONE', #8472, .T. ) ;
#40046=ADVANCED_FACE ( 'NONE', ( #61391 ), #26291, .F. ) ;
#40048=CARTESIAN_POINT ( 'NONE',  ( 5.776515075435670887, -6.716662450894490100, 34.94144148231605840 ) ) ;
#40049=CARTESIAN_POINT ( 'NONE',  ( 14.30769230769231015, -3.050289026998446396, 32.03036669348365706 ) ) ;
#40050=DIRECTION ( 'NONE',  ( 0.000000000000000000, 0.7660444431189807890, 0.6427876096865361433 ) ) ;
#40052=CARTESIAN_POINT ( 'NONE',  ( 0.4615384615383396616, -6.026961402154118908, 34.52809138561165270 ) ) ;
#40054=EDGE_LOOP ( 'NONE', ( #32350, #41412 ) ) ;
#40056=VECTOR ( 'NONE', #84365, 1000.000000000000114 ) ;
#40058=CARTESIAN_POINT ( 'NONE',  ( 16.15384615384615330, -6.386643153685126251, 34.62446782046654192 ) ) ;
#40060=CARTESIAN_POINT ( 'NONE',  ( 17.32692307692309797, -2.249999999999997780, 29.81603969181029612 ) ) ;
#40061=CARTESIAN_POINT ( 'NONE',  ( -15.23076923076922995, -1.129524287112498415, 32.06866353760679544 ) ) ;
#40063=EDGE_CURVE ( 'NONE', #88099, #7820, #31454, .T. ) ;
#40064=CARTESIAN_POINT ( 'NONE',  ( -15.23076923076922995, -8.973038597847269315, 34.52809138561121927 ) ) ;
#40065=CARTESIAN_POINT ( 'NONE',  ( -6.065270000556318486, -8.656820664281497102, 34.87096338111211935 ) ) ;
#40066=VECTOR ( 'NONE', #14722, 1000.000000000000227 ) ;
#40068=CARTESIAN_POINT ( 'NONE',  ( 17.01165263096230262, -12.27809138561121394, 31.22303859784730307 ) ) ;
#40069=CARTESIAN_POINT ( 'NONE',  ( 12.33084785842815378, -11.37499894934982692, 33.29245874905763003 ) ) ;
#40070=DIRECTION ( 'NONE',  ( -0.000000000000000000, -0.9396926207859093161, -0.3420201433256663259 ) ) ;
#40071=VECTOR ( 'NONE', #56973, 1000.000000000000227 ) ;
#40072=CARTESIAN_POINT ( 'NONE',  ( 8.703960323269996024, -12.27809138561121394, 31.22303859784730307 ) ) ;
#40073=EDGE_CURVE ( 'NONE', #19302, #6432, #60959, .T. ) ;
#40074=CARTESIAN_POINT ( 'NONE',  ( -0.3310130233048168558, -4.299079248970732792, 33.91157788607253565 ) ) ;
#40075=CARTESIAN_POINT ( 'NONE',  ( 14.98076923076923173, -2.249999999999998668, 29.75000000000000355 ) ) ;
#40077=B_SPLINE_CURVE_WITH_KNOTS ( 'NONE', 3,
 ( #62820, #7008, #1140, #55190, #83121, #29074, #41247, #21412, #28621, #69597 ),
 .UNSPECIFIED., .F., .F.,
 ( 4, 2, 2, 2, 4 ),
 ( 0.0007817359430256319575, 0.0009771253907249984917, 0.001172514838424365026, 0.001367904286123731343, 0.001563293733823097878 ),
 .UNSPECIFIED. ) ;
#40078=CARTESIAN_POINT ( 'NONE',  ( -17.07692307692307665, -2.833524468853757305, 32.15551576947925838 ) ) ;
#40079=EDGE_LOOP ( 'NONE', ( #83383, #69572, #15258, #43973 ) ) ;
#40080=CYLINDRICAL_SURFACE ( 'NONE', #80099, 0.2499999999999995559 ) ;
#40081=CARTESIAN_POINT ( 'NONE',  ( -17.32689982097166492, -6.524016743844656574, 34.90889640711025521 ) ) ;
#40083=DIRECTION ( 'NONE',  ( 0.000000000000000000, 0.6427876096865373645, -0.7660444431189797898 ) ) ;
#40084=DIRECTION ( 'NONE',  ( -0.000000000000000000, 0.9848077530122086864, -0.1736481776669273891 ) ) ;
#40085=FACE_OUTER_BOUND ( 'NONE', #84864, .T. ) ;
#40086=CARTESIAN_POINT ( 'NONE',  ( 5.326977496836527770, -4.074993327901525575, 33.72946981652012255 ) ) ;
#40087=ORIENTED_EDGE ( 'NONE', *, *, #77870, .F. ) ;
#40089=CARTESIAN_POINT ( 'NONE',  ( -3.230769230769229949, -6.681629849574314051, 35.83090037661290239 ) ) ;
#40090=ORIENTED_EDGE ( 'NONE', *, *, #80630, .T. ) ;
#40091=CARTESIAN_POINT ( 'NONE',  ( 8.703960323269994248, -8.613356846314824011, 34.62446782046655613 ) ) ;
#40092=CARTESIAN_POINT ( 'NONE',  ( -17.86947429823644029, -3.816742781228455783, 33.13167719472716044 ) ) ;
#40093=VERTEX_POINT ( 'NONE', #82585 ) ;
#40094=CARTESIAN_POINT ( 'NONE',  ( 4.153846153846154188, -12.78798330534102945, 29.74999999999997868 ) ) ;
#40095=CARTESIAN_POINT ( 'NONE',  ( -16.37672483627479636, -7.630691491037286056, 34.74850469731152458 ) ) ;
#40096=CARTESIAN_POINT ( 'NONE',  ( 20.74999999999999645, -7.500000000000000000, 29.75000000000000355 ) ) ;
#40097=ORIENTED_EDGE ( 'NONE', *, *, #21815, .F. ) ;
#40099=ORIENTED_EDGE ( 'NONE', *, *, #78363, .T. ) ;
#40100=LINE ( 'NONE', #24787, #9755 ) ;
#40101=DIRECTION ( 'NONE',  ( -0.000000000000000000, -0.9848077530122085754, -0.1736481776669273613 ) ) ;
#40102=CARTESIAN_POINT ( 'NONE',  ( 18.22277966897806678, -10.23759521482555357, 34.22997729860117033 ) ) ;
#40104=DIRECTION ( 'NONE',  ( -0.000000000000000000, 0.8660254037844397068, -0.4999999999999978906 ) ) ;
#40105=CYLINDRICAL_SURFACE ( 'NONE', #43554, 0.2499999999999973355 ) ;
#40108=CARTESIAN_POINT ( 'NONE',  ( -12.52680890749923570, -6.879047030191174805, 34.71129190930000163 ) ) ;
#40109=ORIENTED_EDGE ( 'NONE', *, *, #51871, .T. ) ;
#40111=ORIENTED_EDGE ( 'NONE', *, *, #5495, .F. ) ;
#40112=CARTESIAN_POINT ( 'NONE',  ( 1.384615384615386802, -12.78798330534102945, 29.74999999999997868 ) ) ;
#40113=ORIENTED_EDGE ( 'NONE', *, *, #25126, .F. ) ;
#40114=EDGE_CURVE ( 'NONE', #34882, #65891, #86191, .T. ) ;
#40115=AXIS2_PLACEMENT_3D ( 'NONE', #3823, #24091, #80392 ) ;
#40116=CARTESIAN_POINT ( 'NONE',  ( -13.13461538461532108, -7.434744860731433924, 35.00000000000000711 ) ) ;
#40117=CARTESIAN_POINT ( 'NONE',  ( 11.53846153846141753, -12.27809138561165270, 31.22303859784587132 ) ) ;
#40118=VERTEX_POINT ( 'NONE', #39816 ) ;
#40119=DIRECTION ( 'NONE',  ( -0.000000000000000000, 0.1736481776669307198, -0.9848077530122080203 ) ) ;
#40120=VECTOR ( 'NONE', #17941, 1000.000000000000000 ) ;
#40121=EDGE_CURVE ( 'NONE', #33177, #37079, #75370, .T. ) ;
#40123=CARTESIAN_POINT ( 'NONE',  ( 11.78840705680968171, -2.587454068350148351, 30.68340429815432202 ) ) ;
#40124=VERTEX_POINT ( 'NONE', #55089 ) ;
#40125=VECTOR ( 'NONE', #71042, 1000.000000000000000 ) ;
#40126=CARTESIAN_POINT ( 'NONE',  ( -12.33149102628801153, -7.723484941389743952, 34.99544897038808955 ) ) ;
#40127=AXIS2_PLACEMENT_3D ( 'NONE', #67828, #81794, #59289 ) ;
#40128=CARTESIAN_POINT ( 'NONE',  ( 1.384615384615386802, -6.386643153685126251, 34.62446782046654192 ) ) ;
#40129=CARTESIAN_POINT ( 'NONE',  ( -4.153846153846152411, -6.343179335718451384, 34.87096338111211935 ) ) ;
#40130=FACE_BOUND ( 'NONE', #32074, .T. ) ;
#40131=ADVANCED_FACE ( 'NONE', ( #67286 ), #5579, .F. ) ;
#40132=CARTESIAN_POINT ( 'NONE',  ( -14.37377468705243722, -9.058645607665454236, 34.76329471203372634 ) ) ;
#40133=CYLINDRICAL_SURFACE ( 'NONE', #54339, 0.2499999999999994726 ) ;
#40134=CARTESIAN_POINT ( 'NONE',  ( 13.44987052412822059, -5.094484230520773593, 34.41647553114626845 ) ) ;
#40137=DIRECTION ( 'NONE',  ( 0.000000000000000000, 0.3420201433256641055, -0.9396926207859100932 ) ) ;
#40138=EDGE_CURVE ( 'NONE', #82649, #52040, #29242, .T. ) ;
#40139=CARTESIAN_POINT ( 'NONE',  ( -13.25457022178060562, -2.504778602574660340, 29.97347330155780654 ) ) ;
#40140=ORIENTED_EDGE ( 'NONE', *, *, #6791, .F. ) ;
#40142=CARTESIAN_POINT ( 'NONE',  ( 2.177544337960609866, -3.069018819979302926, 32.56621877034667278 ) ) ;
#40143=CARTESIAN_POINT ( 'NONE',  ( 2.438218009455872970, -10.88167719472716399, 33.43325721877153711 ) ) ;
#40144=CARTESIAN_POINT ( 'NONE',  ( 15.36155967173618286, -8.191423895709840863, 34.95447573519442130 ) ) ;
#40145=DIRECTION ( 'NONE',  ( -0.000000000000000000, 0.9848077530122085754, -0.1736481776669273613 ) ) ;
#40146=CARTESIAN_POINT ( 'NONE',  ( -17.07692307692307665, -12.34228464037088635, 31.77849191805839268 ) ) ;
#40147=CARTESIAN_POINT ( 'NONE',  ( 8.096153846153846700, -2.499999999999998668, 29.75000000000000355 ) ) ;
#40148=ORIENTED_EDGE ( 'NONE', *, *, #34419, .T. ) ;
#40149=CARTESIAN_POINT ( 'NONE',  ( -11.76194648218548444, -12.24155766932282496, 31.33739205006857986 ) ) ;
#40150=EDGE_CURVE ( 'NONE', #53886, #26509, #81879, .T. ) ;
#40152=CARTESIAN_POINT ( 'NONE',  ( -8.899922235898330314, -12.11776431015576172, 31.66791131148498906 ) ) ;
#40153=FACE_OUTER_BOUND ( 'NONE', #41293, .T. ) ;
#40154=ORIENTED_EDGE ( 'NONE', *, *, #28448, .T. ) ;
#40155=ORIENTED_EDGE ( 'NONE', *, *, #68224, .T. ) ;
#40157=VERTEX_POINT ( 'NONE', #42477 ) ;
#40158=CARTESIAN_POINT ( 'NONE',  ( 0.5920641633020254924, -10.88167719472716399, 33.43325721877153711 ) ) ;
#40159=ORIENTED_EDGE ( 'NONE', *, *, #60778, .F. ) ;
#40160=CARTESIAN_POINT ( 'NONE',  ( 4.088576153289833037, -11.67786785259541027, 32.92929555188721480 ) ) ;
#40161=CARTESIAN_POINT ( 'NONE',  ( -5.143006487878958310, -2.721908614388772740, 31.22303859784724622 ) ) ;
#40162=CYLINDRICAL_SURFACE ( 'NONE', #81207, 0.2499999999999986955 ) ;
#40163=CARTESIAN_POINT ( 'NONE',  ( -2.372962753653082402, -8.613356846314824011, 34.62446782046655613 ) ) ;
#40164=EDGE_CURVE ( 'NONE', #79737, #21202, #16299, .T. ) ;
#40166=ORIENTED_EDGE ( 'NONE', *, *, #87128, .F. ) ;
#40167=CARTESIAN_POINT ( 'NONE',  ( -0.3962833220256234967, -12.16647553114626490, 32.15551576947920864 ) ) ;
#40168=ORIENTED_EDGE ( 'NONE', *, *, #23874, .F. ) ;
#40169=DIRECTION ( 'NONE',  ( 0.000000000000000000, 0.6427876096865368094, 0.7660444431189802339 ) ) ;
#40170=CARTESIAN_POINT ( 'NONE',  ( 8.769230769230645706, -12.51329471203414379, 31.30864560766407578 ) ) ;
#40171=CARTESIAN_POINT ( 'NONE',  ( 9.692307692307695177, -12.37446782046654192, 30.86335684631486131 ) ) ;
#40172=EDGE_CURVE ( 'NONE', #86079, #77001, #57249, .T. ) ;
#40173=EDGE_CURVE ( 'NONE', #77760, #19281, #43197, .T. ) ;
#40174=CARTESIAN_POINT ( 'NONE',  ( -16.40384615384615330, -7.566082377512564960, 35.00000000000000711 ) ) ;
#40175=CARTESIAN_POINT ( 'NONE',  ( -8.638440328263820689, -8.191423895709840863, 34.95447573519442130 ) ) ;
#40176=CARTESIAN_POINT ( 'NONE',  ( -5.142193077479396912, -11.06231777344662781, 33.60647404775220082 ) ) ;
#40177=CARTESIAN_POINT ( 'NONE',  ( -3.480792468062196221, -6.695914987888143877, 34.68535235679833306 ) ) ;
#40179=VERTEX_POINT ( 'NONE', #1921 ) ;
#40180=EDGE_CURVE ( 'NONE', #80616, #57919, #31395, .T. ) ;
#40181=LINE ( 'NONE', #6393, #57512 ) ;
#40182=CARTESIAN_POINT ( 'NONE',  ( 1.384615384615386802, -4.945431358278436385, 36.03766855953609394 ) ) ;
#40183=VECTOR ( 'NONE', #21450, 1000.000000000000227 ) ;
#40186=ORIENTED_EDGE ( 'NONE', *, *, #45992, .F. ) ;
#40187=CARTESIAN_POINT ( 'NONE',  ( 7.911408985666682270, -12.16647553114626490, 32.15551576947920864 ) ) ;
#40188=DIRECTION ( 'NONE',  ( -0.000000000000000000, 1.000000000000000000, 3.491481338843133355E-15 ) ) ;
#40189=AXIS2_PLACEMENT_3D ( 'NONE', #44064, #36015, #64340 ) ;
#40190=CARTESIAN_POINT ( 'NONE',  ( 6.923076923076924238, -8.564572088678739092, 35.78748833219616898 ) ) ;
#40191=DIRECTION ( 'NONE',  ( 0.000000000000000000, 0.4999999999999985567, 0.8660254037844395958 ) ) ;
#40192=VECTOR ( 'NONE', #55768, 999.9999999999998863 ) ;
#40193=FACE_OUTER_BOUND ( 'NONE', #48747, .T. ) ;
#40194=VERTEX_POINT ( 'NONE', #76242 ) ;
#40195=CARTESIAN_POINT ( 'NONE',  ( 6.000000000000001776, -3.513871655860378418, 32.76840700105978499 ) ) ;
#40196=DIRECTION ( 'NONE',  ( 0.000000000000000000, 0.6427876096865373645, -0.7660444431189797898 ) ) ;
#40197=CARTESIAN_POINT ( 'NONE',  ( 18.00000000000000000, -12.34228464037088635, 31.77849191805839268 ) ) ;
#40198=VERTEX_POINT ( 'NONE', #30715 ) ;
#40199=CARTESIAN_POINT ( 'NONE',  ( 13.38461538461538680, -6.386643153685126251, 34.62446782046654192 ) ) ;
#40200=B_SPLINE_CURVE_WITH_KNOTS ( 'NONE', 3,
 ( #20013, #5174, #53799, #74974, #32640, #6511, #80854, #26775, #33969, #68208 ),
 .UNSPECIFIED., .F., .F.,
 ( 4, 2, 2, 2, 4 ),
 ( 0.0007817359430256297891, 0.0009771253907249958896, 0.001172514838424361990, 0.001367904286123728091, 0.001563293733823094191 ),
 .UNSPECIFIED. ) ;
#40201=ORIENTED_EDGE ( 'NONE', *, *, #57195, .T. ) ;
#40202=FACE_OUTER_BOUND ( 'NONE', #86, .T. ) ;
#40203=CARTESIAN_POINT ( 'NONE',  ( 11.66898697669518548, -6.808710257144161559, 34.95449254468098843 ) ) ;
#40205=CARTESIAN_POINT ( 'NONE',  ( 0.4615384615383396616, -4.481592998941358097, 33.73612834414048933 ) ) ;
#40206=CARTESIAN_POINT ( 'NONE',  ( -6.066082379360135945, -2.292212530054419606, 30.41441678777542634 ) ) ;
#40207=CARTESIAN_POINT ( 'NONE',  ( -6.923076923077045919, -12.51329471203414379, 31.30864560766407578 ) ) ;
#40208=DIRECTION ( 'NONE',  ( -0.000000000000000000, -0.8660254037844399289, -0.4999999999999980016 ) ) ;
#40209=DIRECTION ( 'NONE',  ( -0.000000000000000000, 0.3420201433256694346, -0.9396926207859080948 ) ) ;
#40211=FACE_BOUND ( 'NONE', #13216, .T. ) ;
#40212=ORIENTED_EDGE ( 'NONE', *, *, #23919, .T. ) ;
#40213=CARTESIAN_POINT ( 'NONE',  ( 17.07692307692307665, -3.513871655860378418, 32.76840700105978499 ) ) ;
#40215=CARTESIAN_POINT ( 'NONE',  ( -12.33101302330481808, -3.068774925481847493, 32.56582465632704526 ) ) ;
#40216=CARTESIAN_POINT ( 'NONE',  ( 6.000000000000001776, -8.973038597847269315, 34.52809138561121927 ) ) ;
#40217=CARTESIAN_POINT ( 'NONE',  ( 8.769230769230768274, -1.117168528481311540, 33.14645433367849847 ) ) ;
#40218=DIRECTION ( 'NONE',  ( 0.000000000000000000, 0.7660444431189822323, -0.6427876096865344779 ) ) ;
#40219=VERTEX_POINT ( 'NONE', #65389 ) ;
#40220=EDGE_LOOP ( 'NONE', ( #81422, #88755 ) ) ;
#40221=ORIENTED_EDGE ( 'NONE', *, *, #9040, .F. ) ;
#40222=ORIENTED_EDGE ( 'NONE', *, *, #61599, .F. ) ;
#40224=CARTESIAN_POINT ( 'NONE',  ( -6.222926217516146608, -12.39988816332205701, 30.74660775122750778 ) ) ;
#40225=CARTESIAN_POINT ( 'NONE',  ( -7.846153846153965716, -10.21337939537710326, 33.94971097300076224 ) ) ;
#40226=CARTESIAN_POINT ( 'NONE',  ( -7.846153846153844924, -3.322132147404559976, 32.92929555188717927 ) ) ;
#40227=DIRECTION ( 'NONE',  ( 0.000000000000000000, 0.9848077530122072432, -0.1736481776669354937 ) ) ;
#40228=EDGE_CURVE ( 'NONE', #8255, #15080, #75427, .T. ) ;
#40229=VECTOR ( 'NONE', #2669, 1000.000000000000000 ) ;
#40231=CARTESIAN_POINT ( 'NONE',  ( -5.300408020647025431, -8.496056993536548418, 34.65000542017679663 ) ) ;
#40233=CARTESIAN_POINT ( 'NONE',  ( -8.519176349317316266, -2.920487667080175598, 32.31805714834170828 ) ) ;
#40234=ORIENTED_EDGE ( 'NONE', *, *, #45402, .F. ) ;
#40235=VERTEX_POINT ( 'NONE', #59077 ) ;
#40236=ORIENTED_EDGE ( 'NONE', *, *, #27051, .F. ) ;
#40237=VECTOR ( 'NONE', #87426, 1000.000000000000000 ) ;
#40238=CARTESIAN_POINT ( 'NONE',  ( -11.53846153846153655, -12.37446782046654192, 30.86335684631486131 ) ) ;
#40240=CARTESIAN_POINT ( 'NONE',  ( -1.634638608836843421, -2.588893531581426544, 31.60682220781847818 ) ) ;
#40241=CARTESIAN_POINT ( 'NONE',  ( -9.915234651214539952, -4.026226216239094491, 33.68668979543634379 ) ) ;
#40242=AXIS2_PLACEMENT_3D ( 'NONE', #23664, #56573, #84063 ) ;
#40243=CARTESIAN_POINT ( 'NONE',  ( -11.53846153846153655, -4.786620604624113540, 33.94971097300155094 ) ) ;
#40244=CARTESIAN_POINT ( 'NONE',  ( -15.36091720050092846, -10.31621877034669588, 34.18098118002070152 ) ) ;
#40245=FACE_BOUND ( 'NONE', #60524, .T. ) ;
#40246=EDGE_LOOP ( 'NONE', ( #17928, #65871, #44148, #76882 ) ) ;
#40247=EDGE_CURVE ( 'NONE', #48730, #11070, #85168, .T. ) ;
#40249=DIRECTION ( 'NONE',  ( -0.000000000000000000, -0.7660444431189791237, -0.6427876096865379196 ) ) ;
#40250=EDGE_LOOP ( 'NONE', ( #8968, #23993 ) ) ;
#40251=DIRECTION ( 'NONE',  ( -0.000000000000000000, 0.8660254037844397068, -0.4999999999999978906 ) ) ;
#40253=FACE_BOUND ( 'NONE', #33232, .T. ) ;
#40254=CARTESIAN_POINT ( 'NONE',  ( -10.83831157429146330, -2.889293201056495786, 32.26117774369186009 ) ) ;
#40258=DIRECTION ( 'NONE',  ( -0.000000000000000000, 0.5000000000000011102, -0.8660254037844381525 ) ) ;
#40259=CARTESIAN_POINT ( 'NONE',  ( -0.5916864312701585193, -2.373036134822905208, 30.88089517874951540 ) ) ;
#40260=ORIENTED_EDGE ( 'NONE', *, *, #62348, .T. ) ;
#40262=CARTESIAN_POINT ( 'NONE',  ( 3.230769230769231726, -3.322132147404559976, 32.92929555188717927 ) ) ;
#40263=CARTESIAN_POINT ( 'NONE',  ( 18.24994540937804643, -10.92531984108285492, 33.72920026020278073 ) ) ;
#40264=CYLINDRICAL_SURFACE ( 'NONE', #11686, 0.2499999999999979738 ) ;
#40265=ORIENTED_EDGE ( 'NONE', *, *, #47490, .F. ) ;
#40266=B_SPLINE_CURVE_WITH_KNOTS ( 'NONE', 3,
 ( #59336, #37282, #72845, #30966, #17916, #17021, #9818, #31426, #86393, #51669 ),
 .UNSPECIFIED., .F., .F.,
 ( 4, 2, 2, 2, 4 ),
 ( 0.000000000000000000, 0.0001954311564186865221, 0.0003908623128373730441, 0.0005862934692560595662, 0.0007817246256747460882 ),
 .UNSPECIFIED. ) ;
#40267=B_SPLINE_CURVE_WITH_KNOTS ( 'NONE', 3,
 ( #58269, #30363, #2435, #23160, #57833, #78543, #78105, #77658, #50627, #83994 ),
 .UNSPECIFIED., .F., .F.,
 ( 4, 2, 2, 2, 4 ),
 ( 0.0007817359430256320659, 0.0009771253907249987086, 0.001172514838424365243, 0.001367904286123731994, 0.001563293733823098528 ),
 .UNSPECIFIED. ) ;
#40268=CARTESIAN_POINT ( 'NONE',  ( -2.307692307692305711, -13.37000171582298513, 34.34916445242398453 ) ) ;
#40269=CARTESIAN_POINT ( 'NONE',  ( 2.530471976670375600, -3.563462043263030399, 33.22394488606062879 ) ) ;
#40271=CARTESIAN_POINT ( 'NONE',  ( 18.13052570176355971, -6.852161475712351013, 34.70806712695775786 ) ) ;
#40273=CARTESIAN_POINT ( 'NONE',  ( -14.55771553191376633, -2.588893531581426988, 31.60682220781847818 ) ) ;
#40274=CARTESIAN_POINT ( 'NONE',  ( 16.21991348719623360, -11.91647553114624358, 32.58852847137148245 ) ) ;
#40275=CARTESIAN_POINT ( 'NONE',  ( 0.2386115026316125431, -2.523278758544489797, 31.42238647778637528 ) ) ;
#40276=EDGE_CURVE ( 'NONE', #47301, #72614, #50965, .T. ) ;
#40277=EDGE_CURVE ( 'NONE', #36504, #1046, #65824, .T. ) ;
#40278=DIRECTION ( 'NONE',  ( 1.000000000000000000, 0.000000000000000000, 0.000000000000000000 ) ) ;
#40280=CARTESIAN_POINT ( 'NONE',  ( -17.07692307692307665, -8.120952969808772792, 34.71129190930000163 ) ) ;
#40281=CARTESIAN_POINT ( 'NONE',  ( 0.4615384615384611200, -4.661471528628507777, 34.16647553114623292 ) ) ;
#40282=VECTOR ( 'NONE', #83708, 1000.000000000000000 ) ;
#40284=ORIENTED_EDGE ( 'NONE', *, *, #34899, .T. ) ;
#40285=DIRECTION ( 'NONE',  ( -0.000000000000000000, 1.000000000000000000, -0.000000000000000000 ) ) ;
#40286=ORIENTED_EDGE ( 'NONE', *, *, #11829, .T. ) ;
#40288=CARTESIAN_POINT ( 'NONE',  ( -3.164701897419154530, -9.058645607665452459, 34.76329471203371924 ) ) ;
#40289=VERTEX_POINT ( 'NONE', #23948 ) ;
#40292=CARTESIAN_POINT ( 'NONE',  ( -14.05774689831426372, -2.986452184633680229, 32.43230066228895225 ) ) ;
#40293=CARTESIAN_POINT ( 'NONE',  ( -15.23076923076935252, -12.51329471203414379, 31.30864560766407578 ) ) ;
#40294=CYLINDRICAL_SURFACE ( 'NONE', #50425, 0.2500000000000004996 ) ;
#40295=CARTESIAN_POINT ( 'NONE',  ( -5.010855743573001675, -2.486705287966279876, 31.30864560766543647 ) ) ;
#40296=CARTESIAN_POINT ( 'NONE',  ( -15.29685161012936589, -4.661471528628507777, 34.16647553114621871 ) ) ;
#40297=CYLINDRICAL_SURFACE ( 'NONE', #16627, 0.2499999999999995559 ) ;
#40298=CARTESIAN_POINT ( 'NONE',  ( 6.673053698855467175, -12.45566812827425096, 31.48439005359158926 ) ) ;
#40299=DIRECTION ( 'NONE',  ( -0.000000000000000000, -0.5000000000000009992, -0.8660254037844380415 ) ) ;
#40300=CARTESIAN_POINT ( 'NONE',  ( -4.153846153846274980, -12.16647553114689728, 32.15551576947799362 ) ) ;
#40301=CARTESIAN_POINT ( 'NONE',  ( 6.000000000000001776, -3.322132147404559976, 32.92929555188717927 ) ) ;
#40302=B_SPLINE_CURVE_WITH_KNOTS ( 'NONE', 3,
 ( #72527, #31548, #19366, #17601, #12172, #38307, #39656, #67118, #5416, #87858 ),
 .UNSPECIFIED., .F., .F.,
 ( 4, 2, 2, 2, 4 ),
 ( 0.0007817246256747528103, 0.0009771112852218970073, 0.001172497944769041421, 0.001367884604316185835, 0.001563271263863330032 ),
 .UNSPECIFIED. ) ;
#40304=VECTOR ( 'NONE', #31248, 999.9999999999998863 ) ;
#40305=EDGE_LOOP ( 'NONE', ( #908, #72 ) ) ;
#40306=VERTEX_POINT ( 'NONE', #10458 ) ;
#40307=CARTESIAN_POINT ( 'NONE',  ( -8.769230769230768274, -12.37446782046654192, 30.86335684631486131 ) ) ;
#40308=CARTESIAN_POINT ( 'NONE',  ( 15.36129466900287532, -12.15418822224088657, 32.17964115625579069 ) ) ;
#40310=CARTESIAN_POINT ( 'NONE',  ( 6.223375485772421278, -2.251407671071270489, 29.88021292934942252 ) ) ;
#40311=AXIS2_PLACEMENT_3D ( 'NONE', #88275, #19347, #25658 ) ;
#40312=CARTESIAN_POINT ( 'NONE',  ( 6.065255571276025215, -5.219633306516380244, 34.19971097300157936 ) ) ;
#40313=CARTESIAN_POINT ( 'NONE',  ( -6.065270445960775803, -8.613356846314824011, 34.62446782046655613 ) ) ;
#40314=DIRECTION ( 'NONE',  ( -0.000000000000000000, -0.3420201433256694346, -0.9396926207859080948 ) ) ;
#40315=ORIENTED_EDGE ( 'NONE', *, *, #13935, .T. ) ;
#40316=CARTESIAN_POINT ( 'NONE',  ( 1.318531973659506251, -4.786620604624113540, 33.94971097300155805 ) ) ;
#40317=EDGE_LOOP ( 'NONE', ( #10448, #67140 ) ) ;
#40319=CARTESIAN_POINT ( 'NONE',  ( -14.53051900017131359, -7.369208160676171460, 34.74850200257122879 ) ) ;
#40320=CARTESIAN_POINT ( 'NONE',  ( 0.4615384615384611200, -12.09954503811598769, 35.62045528018868623 ) ) ;
#40321=CARTESIAN_POINT ( 'NONE',  ( -17.07692307692319744, -10.90142922262034020, 33.41473453929536674 ) ) ;
#40322=CARTESIAN_POINT ( 'NONE',  ( 6.250054419913455561, -8.346898887586323923, 34.93166121998716278 ) ) ;
#40323=CARTESIAN_POINT ( 'NONE',  ( -17.93474486048716088, -12.51329471203373700, 31.30864560766537963 ) ) ;
#40324=EDGE_CURVE ( 'NONE', #72998, #31746, #64624, .T. ) ;
#40325=EDGE_LOOP ( 'NONE', ( #12416, #2605 ) ) ;
#40326=ORIENTED_EDGE ( 'NONE', *, *, #41996, .T. ) ;
#40327=ORIENTED_EDGE ( 'NONE', *, *, #15778, .F. ) ;
#40328=ORIENTED_EDGE ( 'NONE', *, *, #81286, .T. ) ;
#40329=FACE_OUTER_BOUND ( 'NONE', #85479, .T. ) ;
#40330=CARTESIAN_POINT ( 'NONE',  ( 17.99999999999987566, -11.48612834414049644, 32.76840700105863391 ) ) ;
#40331=AXIS2_PLACEMENT_3D ( 'NONE', #73282, #11585, #3917 ) ;
#40332=CARTESIAN_POINT ( 'NONE',  ( 4.219913487196229163, -11.91647553114624358, 32.58852847137148245 ) ) ;
#40333=CARTESIAN_POINT ( 'NONE',  ( -16.15384615384615330, -2.292212530054420494, 30.41441678777542634 ) ) ;
#40334=EDGE_CURVE ( 'NONE', #40827, #40441, #80769, .T. ) ;
#40336=CARTESIAN_POINT ( 'NONE',  ( -10.36533030374630293, -12.17597550085003633, 31.52189283813461884 ) ) ;
#40337=ORIENTED_EDGE ( 'NONE', *, *, #55873, .F. ) ;
#40338=ADVANCED_FACE ( 'NONE', ( #58626 ), #45116, .F. ) ;
#40339=ORIENTED_EDGE ( 'NONE', *, *, #60659, .F. ) ;
#40340=ORIENTED_EDGE ( 'NONE', *, *, #5689, .T. ) ;
#40341=DIRECTION ( 'NONE',  ( -0.000000000000000000, 0.3420201433256694346, -0.9396926207859080948 ) ) ;
#40342=EDGE_LOOP ( 'NONE', ( #410, #16748 ) ) ;
#40343=CYLINDRICAL_SURFACE ( 'NONE', #21801, 0.2499999999999994726 ) ;
#40344=CARTESIAN_POINT ( 'NONE',  ( -12.21159305216042057, -12.07971442181322175, 32.31769673815850297 ) ) ;
#40347=AXIS2_PLACEMENT_3D ( 'NONE', #34026, #87222, #61491 ) ;
#40348=ADVANCED_FACE ( 'NONE', ( #4126 ), #31614, .F. ) ;
#40349=CARTESIAN_POINT ( 'NONE',  ( -12.46153846153858247, -11.48612834414049644, 32.76840700105863391 ) ) ;
#40350=ORIENTED_EDGE ( 'NONE', *, *, #10864, .T. ) ;
#40351=CYLINDRICAL_SURFACE ( 'NONE', #1079, 0.2499999999999994726 ) ;
#40352=FACE_BOUND ( 'NONE', #46942, .T. ) ;
#40353=B_SPLINE_CURVE_WITH_KNOTS ( 'NONE', 3,
 ( #14785, #29194, #53655, #35043, #82804, #39714, #62071, #8023, #69718, #81142 ),
 .UNSPECIFIED., .F., .F.,
 ( 4, 2, 2, 2, 4 ),
 ( 0.0007817246256747451124, 0.0009771112852218881168, 0.001172497944769031230, 0.001367884604316174126, 0.001563271263863317238 ),
 .UNSPECIFIED. ) ;
#40354=FACE_OUTER_BOUND ( 'NONE', #55905, .T. ) ;
#40356=AXIS2_PLACEMENT_3D ( 'NONE', #49206, #7779, #48756 ) ;
#40357=ADVANCED_FACE ( 'NONE', ( #73043 ), #11339, .F. ) ;
#40358=DIRECTION ( 'NONE',  ( 0.000000000000000000, 1.000000000000000000, 0.000000000000000000 ) ) ;
#40360=DIRECTION ( 'NONE',  ( -1.000000000000000000, 0.000000000000000000, 0.000000000000000000 ) ) ;
#40362=AXIS2_PLACEMENT_3D ( 'NONE', #79451, #4225, #59164 ) ;
#40363=CARTESIAN_POINT ( 'NONE',  ( -3.230769230769229949, -9.058645607665452459, 34.76329471203371924 ) ) ;
#40364=ORIENTED_EDGE ( 'NONE', *, *, #12940, .T. ) ;
#40365=VECTOR ( 'NONE', #53069, 1000.000000000000227 ) ;
#40367=CYLINDRICAL_SURFACE ( 'NONE', #40127, 0.2500000000000012212 ) ;
#40368=CARTESIAN_POINT ( 'NONE',  ( -3.903791733932700847, -10.06805714834173848, 34.32951233291982618 ) ) ;
#40369=CARTESIAN_POINT ( 'NONE',  ( -4.023320715612507925, -2.372941743896878286, 30.88044141588254377 ) ) ;
#40370=CARTESIAN_POINT ( 'NONE',  ( -2.437839517130526268, -10.88202310037936194, 33.43294751532457099 ) ) ;
#40371=CARTESIAN_POINT ( 'NONE',  ( 8.900021210197715860, -9.929761469519743144, 34.40412654351204225 ) ) ;
#40372=EDGE_CURVE ( 'NONE', #78354, #33346, #88802, .T. ) ;
#40373=FACE_BOUND ( 'NONE', #43746, .T. ) ;
#40374=CARTESIAN_POINT ( 'NONE',  ( 5.776515075435670887, -4.988325925672468131, 34.36044203135681130 ) ) ;
#40375=CARTESIAN_POINT ( 'NONE',  ( 4.153846153846030731, -12.70778746994576025, 30.41441678777401236 ) ) ;
#40376=CARTESIAN_POINT ( 'NONE',  ( 2.057715563643717438, -10.06842814019191401, 34.32929386961144758 ) ) ;
#40377=CARTESIAN_POINT ( 'NONE',  ( 7.846153846153846700, -6.435427911321262684, 35.78748833219616898 ) ) ;
#40379=EDGE_CURVE ( 'NONE', #9486, #34081, #75947, .T. ) ;
#40380=CARTESIAN_POINT ( 'NONE',  ( 6.223012844093394946, -4.762714258010880997, 34.23016756924214832 ) ) ;
#40382=ORIENTED_EDGE ( 'NONE', *, *, #74200, .T. ) ;
#40383=CARTESIAN_POINT ( 'NONE',  ( -5.076923076923075762, -12.34228464037088635, 31.77849191805839268 ) ) ;
#40384=EDGE_LOOP ( 'NONE', ( #66902, #32258 ) ) ;
#40386=EDGE_CURVE ( 'NONE', #45661, #35777, #3468, .T. ) ;
#40388=EDGE_CURVE ( 'NONE', #21202, #79737, #19593, .T. ) ;
#40389=CARTESIAN_POINT ( 'NONE',  ( 16.40390057375961064, -12.65882529074907126, 30.72640787790838601 ) ) ;
#40391=CARTESIAN_POINT ( 'NONE',  ( -5.076923076923075762, -9.058645607665452459, 34.76329471203371924 ) ) ;
#40392=ORIENTED_EDGE ( 'NONE', *, *, #43621, .F. ) ;
#40393=DIRECTION ( 'NONE',  ( -0.000000000000000000, 1.000000000000000000, -0.000000000000000000 ) ) ;
#40394=FACE_OUTER_BOUND ( 'NONE', #37391, .T. ) ;
#40397=CARTESIAN_POINT ( 'NONE',  ( 2.307692307692187583, -9.442884908241554243, 34.35708131394783038 ) ) ;
#40399=CARTESIAN_POINT ( 'NONE',  ( 4.088575707885377497, -11.94971097300153140, 32.03036669348370680 ) ) ;
#40400=CARTESIAN_POINT ( 'NONE',  ( -12.46153846153846168, -8.164416787775445883, 34.95778746994557906 ) ) ;
#40401=CARTESIAN_POINT ( 'NONE',  ( 1.449870524128224591, -10.33852847137154107, 34.16647553114620450 ) ) ;
#40402=B_SPLINE_CURVE_WITH_KNOTS ( 'NONE', 3,
 ( #36708, #79025, #85346, #22740, #29515, #71818, #1595, #84027, #23631, #43906 ),
 .UNSPECIFIED., .F., .F.,
 ( 4, 2, 2, 2, 4 ),
 ( 0.0007817246336856289524, 0.0009771112958940101571, 0.001172497958102391253, 0.001367884620310772350, 0.001563271282519153446 ),
 .UNSPECIFIED. ) ;
#40404=CARTESIAN_POINT ( 'NONE',  ( -24.00000000000000000, -9.499999999999982236, 27.25000000000000000 ) ) ;
#40405=CYLINDRICAL_SURFACE ( 'NONE', #47073, 0.2499999999999994726 ) ;
#40406=VERTEX_POINT ( 'NONE', #25747 ) ;
#40407=VECTOR ( 'NONE', #84940, 1000.000000000000114 ) ;
#40408=CARTESIAN_POINT ( 'NONE',  ( 17.07692307692295586, -2.892918686052165622, 31.69288490824153470 ) ) ;
#40411=CARTESIAN_POINT ( 'NONE',  ( -17.77722045873158763, -12.44528174975671853, 30.48912976160715615 ) ) ;
#40412=CYLINDRICAL_SURFACE ( 'NONE', #51231, 0.2499999999999994726 ) ;
#40413=EDGE_LOOP ( 'NONE', ( #39860, #24216 ) ) ;
#40414=CYLINDRICAL_SURFACE ( 'NONE', #45711, 0.2499999999999995559 ) ;
#40415=CARTESIAN_POINT ( 'NONE',  ( -14.53117725141625094, -11.41268669641500466, 32.86336882939237825 ) ) ;
#40416=CARTESIAN_POINT ( 'NONE',  ( -16.15384615384615330, -12.34228464037088635, 31.77849191805839268 ) ) ;
#40417=ORIENTED_EDGE ( 'NONE', *, *, #34034, .T. ) ;
#40418=CARTESIAN_POINT ( 'NONE',  ( -6.923076923076922462, -4.102666532097928531, 36.13435417666054406 ) ) ;
#40419=CARTESIAN_POINT ( 'NONE',  ( 5.143089683514715738, -7.250054591869668386, 34.99404684341514127 ) ) ;
#40420=CARTESIAN_POINT ( 'NONE',  ( -12.59222906464877134, -4.684245665217972032, 34.18127051446801090 ) ) ;
#40421=EDGE_LOOP ( 'NONE', ( #68197, #78652 ) ) ;
#40422=CARTESIAN_POINT ( 'NONE',  ( 2.241609928332173762, -3.937682226553329556, 33.60647404775217240 ) ) ;
#40423=EDGE_CURVE ( 'NONE', #75445, #28787, #68070, .T. ) ;
#40424=CARTESIAN_POINT ( 'NONE',  ( 6.792385456409367528, -4.809359713505814149, 33.96456829005828837 ) ) ;
#40425=AXIS2_PLACEMENT_3D ( 'NONE', #25398, #33044, #46556 ) ;
#40426=CARTESIAN_POINT ( 'NONE',  ( -13.31936024510254768, -8.656820664281605460, 34.87096338111211224 ) ) ;
#40429=EDGE_LOOP ( 'NONE', ( #6203, #39424, #37912, #15782 ) ) ;
#40430=EDGE_LOOP ( 'NONE', ( #66209, #55844, #70530, #16754 ) ) ;
#40431=VECTOR ( 'NONE', #23976, 1000.000000000000227 ) ;
#40432=VECTOR ( 'NONE', #22953, 1000.000000000000000 ) ;
#40433=EDGE_CURVE ( 'NONE', #25506, #85233, #28203, .T. ) ;
#40434=CARTESIAN_POINT ( 'NONE',  ( 5.076923076923075762, -12.34228464037088635, 31.77849191805839268 ) ) ;
#40439=EDGE_CURVE ( 'NONE', #74505, #66117, #9775, .T. ) ;
#40440=CARTESIAN_POINT ( 'NONE',  ( 5.299934428535925335, -5.667800583137508674, 34.40243808032445827 ) ) ;
#40441=VERTEX_POINT ( 'NONE', #74830 ) ;
#40442=B_SPLINE_CURVE_WITH_KNOTS ( 'NONE', 3,
 ( #50842, #78331, #5236, #87673, #32700, #64807, #5675, #23387, #71133, #25946 ),
 .UNSPECIFIED., .F., .F.,
 ( 4, 2, 2, 2, 4 ),
 ( 0.0007817359430256293554, 0.0009771253907249941549, 0.001172514838424358954, 0.001367904286123723537, 0.001563293733823095276 ),
 .UNSPECIFIED. ) ;
#40443=ORIENTED_EDGE ( 'NONE', *, *, #14812, .F. ) ;
#40444=ORIENTED_EDGE ( 'NONE', *, *, #44490, .T. ) ;
#40445=DIRECTION ( 'NONE',  ( -0.000000000000000000, -0.5000000000000009992, -0.8660254037844380415 ) ) ;
#40446=EDGE_LOOP ( 'NONE', ( #2998, #62054, #10047, #41783 ) ) ;
#40447=CYLINDRICAL_SURFACE ( 'NONE', #43055, 0.2500000000000008882 ) ;
#40448=CARTESIAN_POINT ( 'NONE',  ( -3.361459833879538284, -11.93127051446800024, 32.56575433478200665 ) ) ;
#40449=EDGE_CURVE ( 'NONE', #13183, #42562, #59523, .T. ) ;
#40450=FACE_OUTER_BOUND ( 'NONE', #50405, .T. ) ;
#40451=CARTESIAN_POINT ( 'NONE',  ( 15.90382292962469535, -11.56360843649121861, 33.07473185843129926 ) ) ;
#40452=ORIENTED_EDGE ( 'NONE', *, *, #4573, .T. ) ;
#40453=EDGE_CURVE ( 'NONE', #45514, #23762, #7792, .T. ) ;
#40454=VERTEX_POINT ( 'NONE', #13557 ) ;
#40455=VERTEX_POINT ( 'NONE', #6374 ) ;
#40456=CARTESIAN_POINT ( 'NONE',  ( -10.74553258511631348, -11.04286588640298561, 33.62463336215343901 ) ) ;
#40457=LINE ( 'NONE', #40012, #18576 ) ;
#40458=EDGE_LOOP ( 'NONE', ( #26417, #26737, #50187, #66287 ) ) ;
#40459=CARTESIAN_POINT ( 'NONE',  ( 9.442284455014730682, -11.86270091957321249, 32.19358267280087915 ) ) ;
#40461=ORIENTED_EDGE ( 'NONE', *, *, #23163, .T. ) ;
#40462=CARTESIAN_POINT ( 'NONE',  ( -17.07692307692307665, -8.973038597847269315, 34.52809138561121927 ) ) ;
#40464=CARTESIAN_POINT ( 'NONE',  ( -17.77698864838715309, -2.554770724473667709, 30.48948780036025852 ) ) ;
#40465=CARTESIAN_POINT ( 'NONE',  ( 4.403900465484468896, -2.779044189368096163, 31.39831045268886456 ) ) ;
#40466=FACE_BOUND ( 'NONE', #84618, .T. ) ;
#40467=CARTESIAN_POINT ( 'NONE',  ( 17.07692307692295586, -2.892918686052165622, 31.69288490824153470 ) ) ;
#40468=CARTESIAN_POINT ( 'NONE',  ( -6.222926958906846551, -12.38737895849757820, 31.66785238281580206 ) ) ;
#40469=CARTESIAN_POINT ( 'NONE',  ( -10.48485917715097138, -11.04252011169590020, 33.62494198852677130 ) ) ;
#40470=LINE ( 'NONE', #12541, #34555 ) ;
#40471=CARTESIAN_POINT ( 'NONE',  ( 17.07692307692307665, -8.973038597847269315, 34.52809138561121927 ) ) ;
#40472=DIRECTION ( 'NONE',  ( -0.000000000000000000, 0.9848077530122086864, -0.1736481776669273891 ) ) ;
#40473=CARTESIAN_POINT ( 'NONE',  ( 6.923076923077231548, -2.506253911140614576, 30.00000000000323297 ) ) ;
#40476=CARTESIAN_POINT ( 'NONE',  ( 0.2380535369741281215, -10.97335522853832579, 33.68706563782419749 ) ) ;
#40477=ORIENTED_EDGE ( 'NONE', *, *, #75668, .T. ) ;
#40478=CARTESIAN_POINT ( 'NONE',  ( -6.700065571464073777, -4.887748414852792322, 34.01359900205216746 ) ) ;
#40479=CARTESIAN_POINT ( 'NONE',  ( 16.08776377448601735, -2.292212530054419606, 30.41441678777542634 ) ) ;
#40480=CARTESIAN_POINT ( 'NONE',  ( -7.780898706641008467, -2.379036618887895305, 30.90682066428158592 ) ) ;
#40481=ORIENTED_EDGE ( 'NONE', *, *, #47455, .F. ) ;
#40482=CARTESIAN_POINT ( 'NONE',  ( -16.08777780284371772, -11.16473453929635440, 33.15142922261926373 ) ) ;
#40483=CARTESIAN_POINT ( 'NONE',  ( 6.792928953345229282, -8.630895178749536711, 34.87696386517710323 ) ) ;
#40484=EDGE_CURVE ( 'NONE', #13555, #24183, #87027, .T. ) ;
#40485=FACE_BOUND ( 'NONE', #45195, .T. ) ;
#40486=CARTESIAN_POINT ( 'NONE',  ( -18.22292621751613240, -3.105860786376063221, 32.13614157043599562 ) ) ;
#40487=CARTESIAN_POINT ( 'NONE',  ( -17.07692307692276046, -2.255955759149395501, 30.00000000000324363 ) ) ;
#40488=CARTESIAN_POINT ( 'NONE',  ( 8.096099364501986528, -9.272278438253398036, 34.42582936511637115 ) ) ;
#40491=CARTESIAN_POINT ( 'NONE',  ( -14.53057182442989337, -7.630690623152299956, 34.99857592706774057 ) ) ;
#40493=ORIENTED_EDGE ( 'NONE', *, *, #74804, .T. ) ;
#40495=AXIS2_PLACEMENT_3D ( 'NONE', #87787, #81458, #81902 ) ;
#40496=EDGE_LOOP ( 'NONE', ( #30917, #78220 ) ) ;
#40497=CARTESIAN_POINT ( 'NONE',  ( 5.010840697562940704, -10.67929555188718460, 33.92786785259543336 ) ) ;
#40498=EDGE_CURVE ( 'NONE', #79559, #53989, #23885, .T. ) ;
#40499=CARTESIAN_POINT ( 'NONE',  ( -17.77722033102192967, -3.563462043263028178, 33.22394488606062879 ) ) ;
#40500=CARTESIAN_POINT ( 'NONE',  ( 16.28437159207979334, -3.068774925481847937, 32.56582465632704526 ) ) ;
#40501=CARTESIAN_POINT ( 'NONE',  ( 10.86533002476265786, -2.986452184633680673, 32.43230066228895225 ) ) ;
#40502=CARTESIAN_POINT ( 'NONE',  ( -15.23076923076922995, -13.20930481340135110, 34.54067556320372745 ) ) ;
#40504=AXIS2_PLACEMENT_3D ( 'NONE', #23635, #57418, #16882 ) ;
#40505=CARTESIAN_POINT ( 'NONE',  ( 5.076923076923075762, -1.629998284177014645, 34.34916445242399163 ) ) ;
#40506=CARTESIAN_POINT ( 'NONE',  ( 8.769230769230768274, -9.819645486525091727, 36.12317359536749706 ) ) ;
#40508=CARTESIAN_POINT ( 'NONE',  ( -18.00000000000012079, -11.94971097300221352, 32.03036669348236387 ) ) ;
#40509=CARTESIAN_POINT ( 'NONE',  ( -17.07692307692307665, -1.044019251281081972, 31.83374038241031911 ) ) ;
#40510=CARTESIAN_POINT ( 'NONE',  ( -2.307692307692305711, -13.75783147151868846, 33.36296068462461051 ) ) ;
#40512=CARTESIAN_POINT ( 'NONE',  ( -8.703163435880695076, -11.35647404775217595, 33.31231777344666511 ) ) ;
#40513=CARTESIAN_POINT ( 'NONE',  ( -16.82686865700962642, -2.920487667080175154, 32.31805714834170828 ) ) ;
#40515=VERTEX_POINT ( 'NONE', #82914 ) ;
#40516=CARTESIAN_POINT ( 'NONE',  ( -4.946397375159510723, -11.93748526763465279, 32.05452791011430946 ) ) ;
#40519=CARTESIAN_POINT ( 'NONE',  ( 4.087763774486018242, -4.661471528628507777, 34.16647553114621871 ) ) ;
#40520=CYLINDRICAL_SURFACE ( 'NONE', #47591, 0.2499999999999994726 ) ;
#40521=EDGE_CURVE ( 'NONE', #40709, #77395, #55812, .T. ) ;
#40522=CARTESIAN_POINT ( 'NONE',  ( -2.307692307692428724, -8.656820664282941280, 34.87096338111179961 ) ) ;
#40523=CARTESIAN_POINT ( 'NONE',  ( -5.750000000000062172, -7.565270000091922853, 34.99999999999999289 ) ) ;
#40524=ORIENTED_EDGE ( 'NONE', *, *, #77846, .T. ) ;
#40526=CARTESIAN_POINT ( 'NONE',  ( 17.75002326905764960, -3.627789207965226304, 32.91389620160131102 ) ) ;
#40528=CARTESIAN_POINT ( 'NONE',  ( 11.78840694783958476, -9.357781135181031829, 34.66075350412533851 ) ) ;
#40529=DIRECTION ( 'NONE',  ( -0.000000000000000000, -0.8660254037844397068, -0.4999999999999978906 ) ) ;
#40530=ORIENTED_EDGE ( 'NONE', *, *, #61583, .F. ) ;
#40531=AXIS2_PLACEMENT_3D ( 'NONE', #47211, #83114, #31938 ) ;
#40532=CARTESIAN_POINT ( 'NONE',  ( 17.07692307692295586, -11.48612834414049644, 32.76840700105863391 ) ) ;
#40533=EDGE_CURVE ( 'NONE', #66377, #10085, #76545, .T. ) ;
#40534=CARTESIAN_POINT ( 'NONE',  ( 0.4615384615384611200, -2.721908614388771852, 31.22303859784724978 ) ) ;
#40535=DIRECTION ( 'NONE',  ( 0.000000000000000000, 0.6427876096865368094, 0.7660444431189802339 ) ) ;
#40536=ORIENTED_EDGE ( 'NONE', *, *, #77379, .F. ) ;
#40537=ORIENTED_EDGE ( 'NONE', *, *, #81186, .F. ) ;
#40538=EDGE_CURVE ( 'NONE', #84649, #14645, #42815, .T. ) ;
#40539=B_SPLINE_CURVE_WITH_KNOTS ( 'NONE', 3,
 ( #23279, #85877, #44874, #30481, #30914, #16087, #64700, #51616, #43551, #72352 ),
 .UNSPECIFIED., .F., .F.,
 ( 4, 2, 2, 2, 4 ),
 ( 0.000000000000000000, 0.0001954339857564090194, 0.0003908679715128180387, 0.0005863019572692270039, 0.0007817359430256360774 ),
 .UNSPECIFIED. ) ;
#40540=ORIENTED_EDGE ( 'NONE', *, *, #50599, .T. ) ;
#40541=CARTESIAN_POINT ( 'NONE',  ( -15.09997878980228059, -3.957578996910242619, 33.62503395064540257 ) ) ;
#40543=CARTESIAN_POINT ( 'NONE',  ( 9.627037691751372250, -3.083524468853724443, 32.58852847137143272 ) ) ;
#40544=CARTESIAN_POINT ( 'NONE',  ( -17.14300648787895653, -5.557115091759785130, 34.35708131394839171 ) ) ;
#40545=CARTESIAN_POINT ( 'NONE',  ( -6.700297254098857458, -11.60474049983371003, 33.02348890104160262 ) ) ;
#40546=CARTESIAN_POINT ( 'NONE',  ( 15.23076923076923173, -13.95598074871891292, 31.83374038241031911 ) ) ;
#40547=CARTESIAN_POINT ( 'NONE',  ( 13.45068373561782593, -3.050289026998446840, 32.03036669348366416 ) ) ;
#40548=EDGE_CURVE ( 'NONE', #1790, #34883, #65835, .T. ) ;
#40549=CARTESIAN_POINT ( 'NONE',  ( 16.08776377448601735, -12.62096338111211580, 30.90682066428152908 ) ) ;
#40550=VERTEX_POINT ( 'NONE', #34271 ) ;
#40551=EDGE_CURVE ( 'NONE', #6432, #3401, #87250, .T. ) ;
#40552=EDGE_LOOP ( 'NONE', ( #44838, #14366, #24952, #57264 ) ) ;
#40553=CARTESIAN_POINT ( 'NONE',  ( -0.4615384615384611200, -12.10708131394839349, 31.69288490824020244 ) ) ;
#40555=VECTOR ( 'NONE', #88849, 1000.000000000000227 ) ;
#40556=CARTESIAN_POINT ( 'NONE',  ( -13.16165225034871078, -7.369474539155828730, 34.99858011523957657 ) ) ;
#40557=CARTESIAN_POINT ( 'NONE',  ( 6.130790440966950250, -9.929761469519744921, 34.40412654351204225 ) ) ;
#40558=ORIENTED_EDGE ( 'NONE', *, *, #15608, .F. ) ;
#40559=ADVANCED_FACE ( 'NONE', ( #69832 ), #491, .F. ) ;
#40560=LINE ( 'NONE', #4539, #27218 ) ;
#40561=AXIS2_PLACEMENT_3D ( 'NONE', #42614, #56123, #62416 ) ;
#40562=EDGE_CURVE ( 'NONE', #41231, #47411, #40030, .T. ) ;
#40563=ORIENTED_EDGE ( 'NONE', *, *, #16777, .T. ) ;
#40564=CARTESIAN_POINT ( 'NONE',  ( 1.384615384615386802, -12.09954503811598769, 35.62045528018868623 ) ) ;
#40565=ORIENTED_EDGE ( 'NONE', *, *, #67576, .F. ) ;
#40566=CARTESIAN_POINT ( 'NONE',  ( 9.942362003946010773, -8.303483539816731707, 34.68545999027711702 ) ) ;
#40567=ORIENTED_EDGE ( 'NONE', *, *, #47979, .F. ) ;
#40568=CARTESIAN_POINT ( 'NONE',  ( -16.15384615384615330, -6.386643153685126251, 34.62446782046654192 ) ) ;
#40569=CARTESIAN_POINT ( 'NONE',  ( 10.86533013373275658, -5.057305518903948638, 34.11320923018887896 ) ) ;
#40570=FACE_BOUND ( 'NONE', #79884, .T. ) ;
#40571=CARTESIAN_POINT ( 'NONE',  ( 6.000000000000001776, -2.292212530054420494, 30.41441678777542634 ) ) ;
#40573=CARTESIAN_POINT ( 'NONE',  ( -1.384615384615383471, -2.249999999999998668, 29.50000000000001421 ) ) ;
#40574=CARTESIAN_POINT ( 'NONE',  ( 10.39189969082028675, -10.23692288466677880, 34.23039457007281072 ) ) ;
#40575=CARTESIAN_POINT ( 'NONE',  ( -8.769230769230768274, -12.09954503811598769, 35.62045528018868623 ) ) ;
#40577=CARTESIAN_POINT ( 'NONE',  ( -10.61538461538473399, -4.481592998941358097, 33.73612834414048933 ) ) ;
#40578=VERTEX_POINT ( 'NONE', #71151 ) ;
#40579=ORIENTED_EDGE ( 'NONE', *, *, #67426, .T. ) ;
#40580=CARTESIAN_POINT ( 'NONE',  ( 2.307692307692309264, -10.51840700105979565, 33.73612834413961536 ) ) ;
#40581=CARTESIAN_POINT ( 'NONE',  ( -18.13069060311030611, -9.929715669179222104, 34.40415004197138416 ) ) ;
#40582=CARTESIAN_POINT ( 'NONE',  ( -4.403846153846151523, -7.500000000000001776, 35.00000000000000000 ) ) ;
#40584=DIRECTION ( 'NONE',  ( -0.000000000000000000, 1.000000000000000000, -0.000000000000000000 ) ) ;
#40585=CARTESIAN_POINT ( 'NONE',  ( -13.38461538461538325, -13.95598074871891292, 31.83374038241031911 ) ) ;
#40586=VERTEX_POINT ( 'NONE', #10791 ) ;
#40587=DIRECTION ( 'NONE',  ( -0.000000000000000000, -0.7660444431189791237, -0.6427876096865379196 ) ) ;
#40588=CARTESIAN_POINT ( 'NONE',  ( 11.60360731779350374, -7.750023238201979581, 34.74374492549440419 ) ) ;
#40589=CARTESIAN_POINT ( 'NONE',  ( -14.17690186672535901, -12.35292014791297710, 31.75344720912887198 ) ) ;
#40591=VECTOR ( 'NONE', #71184, 1000.000000000000114 ) ;
#40592=ORIENTED_EDGE ( 'NONE', *, *, #77504, .T. ) ;
#40593=EDGE_LOOP ( 'NONE', ( #44195, #22021 ) ) ;
#40594=EDGE_CURVE ( 'NONE', #18500, #86292, #63613, .T. ) ;
#40596=CARTESIAN_POINT ( 'NONE',  ( 10.39245765647776309, -4.026226216239094491, 33.68668979543634379 ) ) ;
#40597=EDGE_CURVE ( 'NONE', #85310, #75827, #55015, .T. ) ;
#40598=ORIENTED_EDGE ( 'NONE', *, *, #54037, .T. ) ;
#40599=CYLINDRICAL_SURFACE ( 'NONE', #30876, 0.2499999999999979738 ) ;
#40600=CARTESIAN_POINT ( 'NONE',  ( 15.23076923076923173, -8.973038597847269315, 34.52809138561121927 ) ) ;
#40601=CARTESIAN_POINT ( 'NONE',  ( 3.296836564119306701, -5.471508081941601098, 34.59228464037088457 ) ) ;
#40602=CARTESIAN_POINT ( 'NONE',  ( 8.835298102580843249, -3.322132147404559976, 32.92929555188717927 ) ) ;
#40603=B_SPLINE_CURVE_WITH_KNOTS ( 'NONE', 3,
 ( #26045, #33246, #10749, #4893, #65675, #39123, #59821, #60708, #31461, #18842 ),
 .UNSPECIFIED., .F., .F.,
 ( 4, 2, 2, 2, 4 ),
 ( 0.000000000000000000, 0.0001954339857564098054, 0.0003908679715128196108, 0.0005863019572692293891, 0.0007817359430256392216 ),
 .UNSPECIFIED. ) ;
#40606=EDGE_CURVE ( 'NONE', #69003, #59070, #63947, .T. ) ;
#40607=CARTESIAN_POINT ( 'NONE',  ( -11.76128963609641964, -7.369209533119140509, 34.99857337881830688 ) ) ;
#40608=CARTESIAN_POINT ( 'NONE',  ( -0.5268084620947810492, -5.941354392334500467, 34.76329471203369792 ) ) ;
#40609=ORIENTED_EDGE ( 'NONE', *, *, #54738, .T. ) ;
#40610=CARTESIAN_POINT ( 'NONE',  ( -5.142193077479395136, -2.379036618887870436, 30.90682066428147934 ) ) ;
#40611=CARTESIAN_POINT ( 'NONE',  ( -2.437839517130527156, -9.418419913701741919, 34.36755862841477693 ) ) ;
#40612=CARTESIAN_POINT ( 'NONE',  ( -3.230769230769352962, -10.33852847137269571, 34.16647553114546554 ) ) ;
#40613=CARTESIAN_POINT ( 'NONE',  ( 9.942253210655835005, -10.76462480002816235, 33.53768742498949962 ) ) ;
#40614=CARTESIAN_POINT ( 'NONE',  ( 13.31934538405906565, -4.320704448112771878, 33.92786785259540494 ) ) ;
#40615=CARTESIAN_POINT ( 'NONE',  ( 18.22301135161285046, -2.554770724473668597, 30.48948780036025852 ) ) ;
#40616=CARTESIAN_POINT ( 'NONE',  ( -0.5276208408985966214, -2.486705287966279876, 31.30864560766542937 ) ) ;
#40617=EDGE_CURVE ( 'NONE', #11323, #3349, #72222, .T. ) ;
#40620=CARTESIAN_POINT ( 'NONE',  ( -7.146561847641256016, -10.97335522853832579, 33.68706563782419749 ) ) ;
#40621=CARTESIAN_POINT ( 'NONE',  ( 1.384615384615386802, -9.058645607665452459, 34.76329471203371924 ) ) ;
#40623=AXIS2_PLACEMENT_3D ( 'NONE', #56260, #42318, #22906 ) ;
#40624=EDGE_CURVE ( 'NONE', #77202, #54822, #18489, .T. ) ;
#40625=CARTESIAN_POINT ( 'NONE',  ( 5.076923076923075762, -2.292212530054420494, 30.41441678777542634 ) ) ;
#40627=CARTESIAN_POINT ( 'NONE',  ( -12.59222992820601839, -11.71456829005830080, 32.44064028649416542 ) ) ;
#40628=CARTESIAN_POINT ( 'NONE',  ( -12.68502340526241312, -3.236172620538810385, 32.36188796281390267 ) ) ;
#40629=AXIS2_PLACEMENT_3D ( 'NONE', #78727, #11609, #4850 ) ;
#40630=CARTESIAN_POINT ( 'NONE',  ( 10.61538461538461675, -4.661471528628507777, 34.16647553114623292 ) ) ;
#40631=CARTESIAN_POINT ( 'NONE',  ( -7.846153846153844924, -2.900454961884010974, 35.62045528018868623 ) ) ;
#40632=CARTESIAN_POINT ( 'NONE',  ( -0.4615384615384611200, -2.499999999999998668, 29.50000000000001066 ) ) ;
#40633=ORIENTED_EDGE ( 'NONE', *, *, #78644, .F. ) ;
#40634=CYLINDRICAL_SURFACE ( 'NONE', #66433, 0.2499999999999995559 ) ;
#40635=CARTESIAN_POINT ( 'NONE',  ( -14.37377571864818648, -2.721908614388770964, 31.22303859784723912 ) ) ;
#40636=CARTESIAN_POINT ( 'NONE',  ( -14.24152570110066307, -7.250054591869670162, 34.99404684341514127 ) ) ;
#40637=VERTEX_POINT ( 'NONE', #31045 ) ;
#40638=FACE_OUTER_BOUND ( 'NONE', #20521, .T. ) ;
#40639=ADVANCED_FACE ( 'NONE', ( #2683 ), #17551, .F. ) ;
#40640=EDGE_LOOP ( 'NONE', ( #32340, #10547 ) ) ;
#40641=CARTESIAN_POINT ( 'NONE',  ( 12.59232890250541281, -12.35292014791297710, 31.75344720912887198 ) ) ;
#40642=CARTESIAN_POINT ( 'NONE',  ( 11.60452887181161330, -6.343179335718452272, 34.87096338111212646 ) ) ;
#40644=CARTESIAN_POINT ( 'NONE',  ( 12.39545505058257824, -3.513871655860377086, 32.76840700105978499 ) ) ;
#40645=CARTESIAN_POINT ( 'NONE',  ( -14.55769230769230660, -2.249999999999998668, 29.75000000000000355 ) ) ;
#40646=CARTESIAN_POINT ( 'NONE',  ( 13.38461538461538680, -6.386643153685126251, 34.62446782046654192 ) ) ;
#40648=CARTESIAN_POINT ( 'NONE',  ( 1.384615384615386802, -6.343179335718451384, 34.87096338111211935 ) ) ;
#40651=ORIENTED_EDGE ( 'NONE', *, *, #23986, .F. ) ;
#40652=EDGE_CURVE ( 'NONE', #9053, #70948, #65720, .T. ) ;
#40653=DIRECTION ( 'NONE',  ( -0.000000000000000000, 1.000000000000000000, -0.000000000000000000 ) ) ;
#40654=ORIENTED_EDGE ( 'NONE', *, *, #27945, .T. ) ;
#40655=CARTESIAN_POINT ( 'NONE',  ( -8.703975197954740395, -4.481592998940250538, 33.73612834413965089 ) ) ;
#40656=CARTESIAN_POINT ( 'NONE',  ( -12.39628332202562433, -3.083524468853784839, 32.58852847137153930 ) ) ;
#40658=CYLINDRICAL_SURFACE ( 'NONE', #46393, 0.2499999999999986955 ) ;
#40659=CARTESIAN_POINT ( 'NONE',  ( 5.999999999999880096, -5.219633306517616589, 34.19971097300220464 ) ) ;
#40660=EDGE_CURVE ( 'NONE', #83423, #53882, #51795, .T. ) ;
#40661=VERTEX_POINT ( 'NONE', #81927 ) ;
#40662=ORIENTED_EDGE ( 'NONE', *, *, #52045, .T. ) ;
#40663=ORIENTED_EDGE ( 'NONE', *, *, #66937, .F. ) ;
#40666=EDGE_CURVE ( 'NONE', #87523, #74505, #79745, .T. ) ;
#40667=ORIENTED_EDGE ( 'NONE', *, *, #13462, .T. ) ;
#40668=CARTESIAN_POINT ( 'NONE',  ( 11.28846153846153832, -2.249999999999998668, 29.75000000000000355 ) ) ;
#40669=CARTESIAN_POINT ( 'NONE',  ( -17.30040800148741198, -10.23692288466677880, 34.23039457007281072 ) ) ;
#40670=B_SPLINE_CURVE_WITH_KNOTS ( 'NONE', 3,
 ( #62056, #55737, #21510, #6670, #54860, #6241 ),
 .UNSPECIFIED., .F., .F.,
 ( 4, 2, 4 ),
 ( 0.000000000000000000, 0.0001954784845028895374, 0.0003909569690057790748 ),
 .UNSPECIFIED. ) ;
#40671=CARTESIAN_POINT ( 'NONE',  ( 1.515141086378952506, -3.816742781228458448, 33.13167719472716044 ) ) ;
#40673=CARTESIAN_POINT ( 'NONE',  ( -7.846153846153967493, -3.643525952248795718, 33.31231777344771672 ) ) ;
#40674=VECTOR ( 'NONE', #27975, 1000.000000000000000 ) ;
#40675=CARTESIAN_POINT ( 'NONE',  ( -5.207614543590632472, -10.54014554554150607, 33.71984207302941883 ) ) ;
#40677=CARTESIAN_POINT ( 'NONE',  ( -2.373775718648186484, -4.786620604624113540, 33.94971097300155805 ) ) ;
#40678=CARTESIAN_POINT ( 'NONE',  ( -17.86950326799833633, -12.75000000000001066, 29.52694330344912643 ) ) ;
#40679=CARTESIAN_POINT ( 'NONE',  ( -5.143006487878956534, -3.513871655860377086, 32.76840700105978499 ) ) ;
#40680=ORIENTED_EDGE ( 'NONE', *, *, #85300, .T. ) ;
#40681=EDGE_LOOP ( 'NONE', ( #50059, #37297 ) ) ;
#40682=VECTOR ( 'NONE', #37410, 1000.000000000000000 ) ;
#40683=EDGE_LOOP ( 'NONE', ( #13078, #84924, #23461, #57267 ) ) ;
#40684=CARTESIAN_POINT ( 'NONE',  ( -8.769230769230768274, -1.044019251281081972, 31.83374038241031911 ) ) ;
#40685=DIRECTION ( 'NONE',  ( 1.000000000000000000, 0.000000000000000000, 0.000000000000000000 ) ) ;
#40686=CARTESIAN_POINT ( 'NONE',  ( -9.692307692307814193, -4.320704448113951379, 33.92786785259630022 ) ) ;
#40687=DIRECTION ( 'NONE',  ( -0.000000000000000000, 0.5000000000000011102, -0.8660254037844380415 ) ) ;
#40688=CARTESIAN_POINT ( 'NONE',  ( -15.23076923076935252, -10.33852847137269571, 34.16647553114546554 ) ) ;
#40689=FACE_BOUND ( 'NONE', #42230, .T. ) ;
#40690=EDGE_LOOP ( 'NONE', ( #47016, #18251 ) ) ;
#40691=CARTESIAN_POINT ( 'NONE',  ( -1.134669866267242311, -2.824170634883621744, 31.52227843825337317 ) ) ;
#40692=CARTESIAN_POINT ( 'NONE',  ( 3.164685819813352285, -10.51840700105979387, 33.73612834413961536 ) ) ;
#40694=FACE_OUTER_BOUND ( 'NONE', #47949, .T. ) ;
#40696=FACE_BOUND ( 'NONE', #49291, .T. ) ;
#40697=ADVANCED_FACE ( 'NONE', ( #19330 ), #80598, .F. ) ;
#40698=CARTESIAN_POINT ( 'NONE',  ( -5.076923076922769340, -2.506253911140614576, 30.00000000000323297 ) ) ;
#40699=B_SPLINE_CURVE_WITH_KNOTS ( 'NONE', 3,
 ( #81120, #87440, #60831, #6350, #25722, #53632, #18525, #74356, #38793, #11314 ),
 .UNSPECIFIED., .F., .F.,
 ( 4, 2, 2, 2, 4 ),
 ( 0.000000000000000000, 0.0001954311564186858715, 0.0003908623128373717431, 0.0005862934692560576146, 0.0007817246256747434861 ),
 .UNSPECIFIED. ) ;
#40700=EDGE_LOOP ( 'NONE', ( #587, #14476, #28906, #58056 ) ) ;
#40701=CARTESIAN_POINT ( 'NONE',  ( -12.33074665371367651, -8.147973898785416225, 34.70805048591653730 ) ) ;
#40703=CARTESIAN_POINT ( 'NONE',  ( -4.946875641672624724, -7.723484941389743952, 34.99544897038808955 ) ) ;
#40705=CARTESIAN_POINT ( 'NONE',  ( 6.792385456409363975, -5.582088688514999397, 34.36776431015576350 ) ) ;
#40706=CARTESIAN_POINT ( 'NONE',  ( -7.596099426240392027, -8.346898887586323923, 34.93166121998716278 ) ) ;
#40707=CARTESIAN_POINT ( 'NONE',  ( 6.923076923076924238, -12.37446782046654192, 30.86335684631486131 ) ) ;
#40708=CARTESIAN_POINT ( 'NONE',  ( -7.846153846153844924, -2.721908614388771852, 31.22303859784724978 ) ) ;
#40709=VERTEX_POINT ( 'NONE', #72934 ) ;
#40710=B_SPLINE_CURVE_WITH_KNOTS ( 'NONE', 3,
 ( #84112, #27822, #49857, #77337, #15644, #48981, #2118, #29602, #358, #55290 ),
 .UNSPECIFIED., .F., .F.,
 ( 4, 2, 2, 2, 4 ),
 ( 0.0007817246256747453293, 0.0009771112852218889842, 0.001172497944769032531, 0.001367884604316176294, 0.001563271263863319840 ),
 .UNSPECIFIED. ) ;
#40711=CARTESIAN_POINT ( 'NONE',  ( -5.076923076923199218, -5.094484230521993062, 34.41647553114689373 ) ) ;
#40712=CARTESIAN_POINT ( 'NONE',  ( -15.23076923076922995, -4.098570777380720287, 33.41473453929634729 ) ) ;
#40713=B_SPLINE_CURVE_WITH_KNOTS ( 'NONE', 3,
 ( #58833, #78666, #16084, #16520, #36361, #44416, #9335, #23275, #17415, #64249 ),
 .UNSPECIFIED., .F., .F.,
 ( 4, 2, 2, 2, 4 ),
 ( 0.000000000000000000, 0.0001954339857564099951, 0.0003908679715128199903, 0.0005863019572692300396, 0.0007817359430256399806 ),
 .UNSPECIFIED. ) ;
#40714=CARTESIAN_POINT ( 'NONE',  ( 1.634669804528839476, -2.920487667080174710, 32.31805714834170828 ) ) ;
#40715=ORIENTED_EDGE ( 'NONE', *, *, #59340, .T. ) ;
#40716=LINE ( 'NONE', #68177, #8348 ) ;
#40718=CARTESIAN_POINT ( 'NONE',  ( -14.43838291080261271, -2.494641256782728966, 31.33461815524612959 ) ) ;
#40719=CARTESIAN_POINT ( 'NONE',  ( -4.854143535654666941, -8.496831190052096971, 34.64984203495476578 ) ) ;
#40721=CARTESIAN_POINT ( 'NONE',  ( 17.07692307692307665, -4.661471528628507777, 34.16647553114623292 ) ) ;
#40723=CARTESIAN_POINT ( 'NONE',  ( -2.557692307692305267, -2.499999999999998668, 29.75000000000000355 ) ) ;
#40724=CARTESIAN_POINT ( 'NONE',  ( -6.923076923076922462, -2.721908614388771852, 31.22303859784724978 ) ) ;
#40726=EDGE_LOOP ( 'NONE', ( #6084, #41388, #42603, #322 ) ) ;
#40727=FACE_OUTER_BOUND ( 'NONE', #53783, .T. ) ;
#40728=EDGE_LOOP ( 'NONE', ( #36856, #74190, #67016, #59674 ) ) ;
#40730=DIRECTION ( 'NONE',  ( 0.000000000000000000, 0.1736481776669275834, 0.9848077530122086864 ) ) ;
#40731=VERTEX_POINT ( 'NONE', #87360 ) ;
#40732=CARTESIAN_POINT ( 'NONE',  ( -5.076923076923075762, -11.35647404775217417, 33.31231777344666511 ) ) ;
#40734=CARTESIAN_POINT ( 'NONE',  ( 17.77651507543566112, -4.988325925672468131, 34.36044203135681130 ) ) ;
#40735=LINE ( 'NONE', #42063, #36671 ) ;
#40736=CARTESIAN_POINT ( 'NONE',  ( 11.53846153846153832, -8.973038597847269315, 34.52809138561121927 ) ) ;
#40737=DIRECTION ( 'NONE',  ( 0.000000000000000000, 0.4999999999999960032, -0.8660254037844410391 ) ) ;
#40738=FACE_OUTER_BOUND ( 'NONE', #31295, .T. ) ;
#40739=CARTESIAN_POINT ( 'NONE',  ( 2.177000841024749889, -9.804603061927743113, 34.18744698557895845 ) ) ;
#40742=CARTESIAN_POINT ( 'NONE',  ( 17.07692307692307665, -2.292212530054420494, 30.41441678777542634 ) ) ;
#40743=CARTESIAN_POINT ( 'NONE',  ( -14.30769230769199929, -2.506253911140614576, 30.00000000000323297 ) ) ;
#40744=CARTESIAN_POINT ( 'NONE',  ( 5.299935921016469820, -10.77377354290276301, 33.85451476688484718 ) ) ;
#40745=AXIS2_PLACEMENT_3D ( 'NONE', #79464, #38928, #24951 ) ;
#40746=VECTOR ( 'NONE', #58810, 1000.000000000000114 ) ;
#40747=ORIENTED_EDGE ( 'NONE', *, *, #71798, .T. ) ;
#40749=DIRECTION ( 'NONE',  ( -0.000000000000000000, 0.8660254037844399289, -0.4999999999999980016 ) ) ;
#40750=CARTESIAN_POINT ( 'NONE',  ( 15.45378207486262667, -11.98016756924215009, 32.48728574198911190 ) ) ;
#40752=CARTESIAN_POINT ( 'NONE',  ( 0.2115617174898691277, -10.06842814019191401, 34.32929386961144758 ) ) ;
#40753=ADVANCED_FACE ( 'NONE', ( #53095 ), #39168, .F. ) ;
#40754=CYLINDRICAL_SURFACE ( 'NONE', #367, 0.2500000000000009437 ) ;
#40755=CIRCLE ( 'NONE', #47738, 0.2500000000000002220 ) ;
#40756=CARTESIAN_POINT ( 'NONE',  ( -9.692307692307691624, -10.67929555188718282, 33.92786785259544047 ) ) ;
#40757=DIRECTION ( 'NONE',  ( -0.000000000000000000, -0.3420201433256694901, -0.9396926207859082059 ) ) ;
#40758=ADVANCED_FACE ( 'NONE', ( #12136 ), #26083, .F. ) ;
#40759=ORIENTED_EDGE ( 'NONE', *, *, #77562, .F. ) ;
#40760=CYLINDRICAL_SURFACE ( 'NONE', #15615, 0.2499999999999994726 ) ;
#40761=VERTEX_POINT ( 'NONE', #81484 ) ;
#40762=CARTESIAN_POINT ( 'NONE',  ( -14.05769230769087130, -7.500000000000155431, 34.75000000000007105 ) ) ;
#40763=CARTESIAN_POINT ( 'NONE',  ( 15.45378207486262667, -3.395485233115139057, 33.02377354290275946 ) ) ;
#40765=B_SPLINE_CURVE_WITH_KNOTS ( 'NONE', 3,
 ( #37409, #1860, #84297, #30225, #29343, #17142, #64876, #85608, #17604, #29784 ),
 .UNSPECIFIED., .F., .F.,
 ( 4, 2, 2, 2, 4 ),
 ( 0.000000000000000000, 0.0001954311564186865492, 0.0003908623128373730983, 0.0005862934692560596746, 0.0007817246256747461966 ),
 .UNSPECIFIED. ) ;
#40766=CARTESIAN_POINT ( 'NONE',  ( 14.30769230769231015, -1.129524287112498415, 32.06866353760679544 ) ) ;
#40767=CARTESIAN_POINT ( 'NONE',  ( 5.999999999999880096, -2.892918686052165622, 31.69288490824153470 ) ) ;
#40768=ORIENTED_EDGE ( 'NONE', *, *, #76895, .T. ) ;
#40769=VECTOR ( 'NONE', #9064, 1000.000000000000114 ) ;
#40771=ORIENTED_EDGE ( 'NONE', *, *, #36461, .T. ) ;
#40772=EDGE_CURVE ( 'NONE', #4390, #9985, #73838, .T. ) ;
#40774=VERTEX_POINT ( 'NONE', #12574 ) ;
#40775=EDGE_LOOP ( 'NONE', ( #81773, #74203, #82559, #51332 ) ) ;
#40776=DIRECTION ( 'NONE',  ( -0.000000000000000000, -0.6427876096865404731, -0.7660444431189770143 ) ) ;
#40777=CARTESIAN_POINT ( 'NONE',  ( -2.307692307692428724, -10.33852847137269571, 34.16647553114546554 ) ) ;
#40778=CARTESIAN_POINT ( 'NONE',  ( 4.376625822824220080, -12.11081565061823717, 32.26097654155341843 ) ) ;
#40779=CARTESIAN_POINT ( 'NONE',  ( -16.15384615384627409, -2.379036618888197285, 30.90682066428292885 ) ) ;
#40781=CARTESIAN_POINT ( 'NONE',  ( -18.00000000000000000, -13.18701529485372070, 34.52197243641129631 ) ) ;
#40782=VERTEX_POINT ( 'NONE', #67518 ) ;
#40783=VERTEX_POINT ( 'NONE', #5815 ) ;
#40784=EDGE_LOOP ( 'NONE', ( #83728, #12181 ) ) ;
#40785=CARTESIAN_POINT ( 'NONE',  ( 11.47237812750566022, -8.973038597847271092, 34.52809138561120506 ) ) ;
#40786=ORIENTED_EDGE ( 'NONE', *, *, #58741, .F. ) ;
#40787=CARTESIAN_POINT ( 'NONE',  ( 10.61538461538461675, -12.37446782046654192, 30.86335684631486131 ) ) ;
#40788=CARTESIAN_POINT ( 'NONE',  ( -12.23875879256039667, -12.11081565061824250, 32.26097654155340422 ) ) ;
#40791=VECTOR ( 'NONE', #46524, 1000.000000000000000 ) ;
#40792=FACE_OUTER_BOUND ( 'NONE', #63538, .T. ) ;
#40795=FACE_BOUND ( 'NONE', #73753, .T. ) ;
#40796=CARTESIAN_POINT ( 'NONE',  ( -18.00000000000000000, -9.058645607665452459, 34.76329471203371924 ) ) ;
#40797=AXIS2_PLACEMENT_3D ( 'NONE', #37543, #30791, #79439 ) ;
#40798=B_SPLINE_CURVE_WITH_KNOTS ( 'NONE', 3,
 ( #9045, #2261, #8157, #35633, #63081, #83827, #50017, #515, #76158, #29756 ),
 .UNSPECIFIED., .F., .F.,
 ( 4, 2, 2, 2, 4 ),
 ( 0.0007817359430256221996, 0.0009771253907249863487, 0.001172514838424350498, 0.001367904286123714647, 0.001563293733823078796 ),
 .UNSPECIFIED. ) ;
#40799=CARTESIAN_POINT ( 'NONE',  ( 3.230769230769231726, -9.058645607665452459, 34.76329471203371924 ) ) ;
#40801=CARTESIAN_POINT ( 'NONE',  ( -9.692307692307691624, -4.661471528628507777, 34.16647553114623292 ) ) ;
#40803=CARTESIAN_POINT ( 'NONE',  ( -13.16118842275381340, -7.630147231320743018, 34.74852402298682819 ) ) ;
#40804=CARTESIAN_POINT ( 'NONE',  ( 14.05771556364371833, -9.234221910056348293, 34.70572697212741531 ) ) ;
#40805=ORIENTED_EDGE ( 'NONE', *, *, #55195, .T. ) ;
#40806=CARTESIAN_POINT ( 'NONE',  ( -1.384615384615383471, -4.786620604624113540, 33.94971097300155094 ) ) ;
#40807=CARTESIAN_POINT ( 'NONE',  ( -7.596099534515530216, -11.28795663066794575, 33.01431243580653785 ) ) ;
#40808=CARTESIAN_POINT ( 'NONE',  ( 4.153846153846154188, -11.35647404775217417, 33.31231777344666511 ) ) ;
#40809=CARTESIAN_POINT ( 'NONE',  ( -2.438383774359862866, -10.54014554554150607, 33.71984207302941883 ) ) ;
#40810=LINE ( 'NONE', #87679, #22824 ) ;
#40811=FACE_BOUND ( 'NONE', #11212, .T. ) ;
#40812=CARTESIAN_POINT ( 'NONE',  ( -7.173100147298380413, -12.45566812827425096, 31.48439005359158926 ) ) ;
#40813=CARTESIAN_POINT ( 'NONE',  ( 6.673076923076925127, -2.249999999999998668, 29.75000000000000355 ) ) ;
#40814=CARTESIAN_POINT ( 'NONE',  ( -7.173053654019276415, -12.17611988154120972, 31.52148481390971213 ) ) ;
#40815=CARTESIAN_POINT ( 'NONE',  ( -18.13014796973169851, -2.373036134822904319, 30.88089517874953316 ) ) ;
#40816=CARTESIAN_POINT ( 'NONE',  ( -11.31544869436814338, -10.77377354290276124, 33.85451476688484718 ) ) ;
#40817=CARTESIAN_POINT ( 'NONE',  ( -5.300408001487409315, -12.47654668319379567, 31.42292124445336654 ) ) ;
#40819=ORIENTED_EDGE ( 'NONE', *, *, #37646, .T. ) ;
#40820=CYLINDRICAL_SURFACE ( 'NONE', #46182, 0.2499999999999998890 ) ;
#40823=ORIENTED_EDGE ( 'NONE', *, *, #10778, .F. ) ;
#40824=DIRECTION ( 'NONE',  ( -0.000000000000000000, 0.9848077530122086864, -0.1736481776669273891 ) ) ;
#40825=DIRECTION ( 'NONE',  ( 0.000000000000000000, 0.9396926207859126468, -0.3420201433256571111 ) ) ;
#40826=CARTESIAN_POINT ( 'NONE',  ( 5.076923076923075762, -1.242168528481310874, 33.36296068462461051 ) ) ;
#40827=VERTEX_POINT ( 'NONE', #33292 ) ;
#40828=CARTESIAN_POINT ( 'NONE',  ( -18.00000000000012079, -2.625532179533778709, 30.86335684631627174 ) ) ;
#40830=LINE ( 'NONE', #20983, #27360 ) ;
#40831=CYLINDRICAL_SURFACE ( 'NONE', #83, 0.2499999999999986955 ) ;
#40832=AXIS2_PLACEMENT_3D ( 'NONE', #27600, #60504, #33481 ) ;
#40833=CARTESIAN_POINT ( 'NONE',  ( 16.85399685940693004, -12.39988816332205701, 30.74660775122750778 ) ) ;
#40834=CARTESIAN_POINT ( 'NONE',  ( 10.54930223602447903, -2.486705287966279432, 31.30864560766542937 ) ) ;
#40835=DIRECTION ( 'NONE',  ( 0.000000000000000000, 0.000000000000000000, 1.000000000000000000 ) ) ;
#40836=ADVANCED_FACE ( 'NONE', ( #73383 ), #11690, .F. ) ;
#40837=CARTESIAN_POINT ( 'NONE',  ( -5.933931648997560870, -10.51840700105979565, 33.73612834413962247 ) ) ;
#40838=EDGE_CURVE ( 'NONE', #70678, #19537, #69047, .T. ) ;
#40840=CARTESIAN_POINT ( 'NONE',  ( 14.30769230769218758, -6.026961402154118019, 34.52809138561165270 ) ) ;
#40841=ORIENTED_EDGE ( 'NONE', *, *, #74086, .T. ) ;
#40844=ADVANCED_FACE ( 'NONE', ( #35948 ), #84147, .F. ) ;
#40845=CARTESIAN_POINT ( 'NONE',  ( -16.02305571287920571, -12.35292014791297710, 31.75344720912887198 ) ) ;
#40846=CARTESIAN_POINT ( 'NONE',  ( 17.14217864819909920, -11.94971097300157403, 32.03036669348361443 ) ) ;
#40848=CARTESIAN_POINT ( 'NONE',  ( -18.00000000000012079, -2.892918686052166066, 31.69288490824153470 ) ) ;
#40849=CARTESIAN_POINT ( 'NONE',  ( 3.165498784808455479, -3.835265460703609186, 33.15142922261924241 ) ) ;
#40851=VERTEX_POINT ( 'NONE', #21083 ) ;
#40852=CARTESIAN_POINT ( 'NONE',  ( 8.703148389870632329, -5.471508081941602875, 34.59228464037088457 ) ) ;
#40853=EDGE_CURVE ( 'NONE', #61249, #20169, #36657, .T. ) ;
#40855=CARTESIAN_POINT ( 'NONE',  ( 6.988332062589762472, -12.16647553114626490, 32.15551576947920864 ) ) ;
#40856=CARTESIAN_POINT ( 'NONE',  ( -16.82697755857492794, -2.824170634883621744, 31.52227843825337317 ) ) ;
#40857=CARTESIAN_POINT ( 'NONE',  ( -18.00000000000000711, -12.74702886152665471, 29.99985851721553587 ) ) ;
#40858=AXIS2_PLACEMENT_3D ( 'NONE', #48954, #6210, #27357 ) ;
#40859=CARTESIAN_POINT ( 'NONE',  ( -8.769230769230768274, -2.249999999999998668, 29.75000000000001776 ) ) ;
#40860=ADVANCED_FACE ( 'NONE', ( #28749 ), #21536, .F. ) ;
#40861=VERTEX_POINT ( 'NONE', #61631 ) ;
#40862=ORIENTED_EDGE ( 'NONE', *, *, #3500, .F. ) ;
#40863=EDGE_LOOP ( 'NONE', ( #59144, #59033, #59858, #60962 ) ) ;
#40867=DIRECTION ( 'NONE',  ( 0.000000000000000000, 0.7660444431189822323, -0.6427876096865344779 ) ) ;
#40869=CARTESIAN_POINT ( 'NONE',  ( 9.823099500132483897, -4.809403383903225304, 33.96459661697924304 ) ) ;
#40870=CARTESIAN_POINT ( 'NONE',  ( -7.846153846153967493, -11.06231777344772027, 33.60647404775119895 ) ) ;
#40871=LINE ( 'NONE', #67455, #21896 ) ;
#40872=B_SPLINE_CURVE_WITH_KNOTS ( 'NONE', 3,
 ( #40712, #27182, #54641, #20430, #80819, #47894, #19104, #46568, #75375, #13669 ),
 .UNSPECIFIED., .F., .F.,
 ( 4, 2, 2, 2, 4 ),
 ( 0.000000000000000000, 0.0001954339857564078267, 0.0003908679715128156535, 0.0005863019572692235344, 0.0007817359430256313069 ),
 .UNSPECIFIED. ) ;
#40873=ORIENTED_EDGE ( 'NONE', *, *, #37918, .T. ) ;
#40874=ADVANCED_FACE ( 'NONE', ( #56653 ), #89136, .F. ) ;
#40875=ORIENTED_EDGE ( 'NONE', *, *, #59031, .F. ) ;
#40876=ORIENTED_EDGE ( 'NONE', *, *, #69768, .T. ) ;
#40877=CARTESIAN_POINT ( 'NONE',  ( -7.053224892808618307, -8.630895178749536711, 34.87696386517710323 ) ) ;
#40878=EDGE_CURVE ( 'NONE', #57134, #49278, #29174, .T. ) ;
#40879=ORIENTED_EDGE ( 'NONE', *, *, #19484, .T. ) ;
#40880=CARTESIAN_POINT ( 'NONE',  ( -1.634638608836841200, -2.985938066672154445, 32.43141759479405550 ) ) ;
#40881=DIRECTION ( 'NONE',  ( -0.000000000000000000, 0.6427876096865404731, -0.7660444431189770143 ) ) ;
#40882=EDGE_CURVE ( 'NONE', #35898, #79443, #9848, .T. ) ;
#40883=EDGE_CURVE ( 'NONE', #35887, #15372, #34613, .T. ) ;
#40884=CARTESIAN_POINT ( 'NONE',  ( -12.23875892027004930, -12.24180327182772388, 31.33663988360758168 ) ) ;
#40885=FACE_OUTER_BOUND ( 'NONE', #13636, .T. ) ;
#40886=VERTEX_POINT ( 'NONE', #1259 ) ;
#40887=ORIENTED_EDGE ( 'NONE', *, *, #31158, .T. ) ;
#40888=AXIS2_PLACEMENT_3D ( 'NONE', #18311, #3114, #46664 ) ;
#40889=ORIENTED_EDGE ( 'NONE', *, *, #45579, .T. ) ;
#40890=CARTESIAN_POINT ( 'NONE',  ( -5.299801759351723263, -7.630691491037286056, 34.74850469731152458 ) ) ;
#40891=CARTESIAN_POINT ( 'NONE',  ( -39.05038313613820122, -2.499999999999999556, 29.75000000000000355 ) ) ;
#40892=ORIENTED_EDGE ( 'NONE', *, *, #38899, .F. ) ;
#40893=CARTESIAN_POINT ( 'NONE',  ( -12.46153846153858247, -2.892918686052166066, 31.69288490824153470 ) ) ;
#40894=DIRECTION ( 'NONE',  ( 0.000000000000000000, 0.3420201433256671586, 0.9396926207859089830 ) ) ;
#40895=EDGE_LOOP ( 'NONE', ( #75970, #40382, #86427, #27694 ) ) ;
#40896=CARTESIAN_POINT ( 'NONE',  ( -4.087777802843713282, -4.786620604624113540, 33.94971097300155805 ) ) ;
#40897=CARTESIAN_POINT ( 'NONE',  ( 12.52679360105129724, -9.528491918058460186, 34.59228464037086326 ) ) ;
#40898=FACE_BOUND ( 'NONE', #52055, .T. ) ;
#40900=DIRECTION ( 'NONE',  ( -0.000000000000000000, -0.8660254037844397068, -0.4999999999999978906 ) ) ;
#40902=CARTESIAN_POINT ( 'NONE',  ( 9.469381474791543241, -3.105860786376062332, 32.13614157043599562 ) ) ;
#40903=CARTESIAN_POINT ( 'NONE',  ( 4.946775867484853428, -10.19110544564092002, 33.96427741523702792 ) ) ;
#40904=CARTESIAN_POINT ( 'NONE',  ( -3.903791842207838148, -2.779044189368096163, 31.39831045268886456 ) ) ;
#40905=CARTESIAN_POINT ( 'NONE',  ( 12.71148387091650278, -2.986452184633680673, 32.43230066228895225 ) ) ;
#40906=ORIENTED_EDGE ( 'NONE', *, *, #70455, .T. ) ;
#40907=CYLINDRICAL_SURFACE ( 'NONE', #25948, 0.2499999999999973355 ) ;
#40910=CARTESIAN_POINT ( 'NONE',  ( 15.90386942290380290, -3.627789207965226304, 32.91389620160131102 ) ) ;
#40911=CYLINDRICAL_SURFACE ( 'NONE', #13090, 0.2500000000000012212 ) ;
#40912=ORIENTED_EDGE ( 'NONE', *, *, #68039, .T. ) ;
#40913=ADVANCED_FACE ( 'NONE', ( #83702 ), #21985, .F. ) ;
#40914=FACE_OUTER_BOUND ( 'NONE', #62451, .T. ) ;
#40915=CARTESIAN_POINT ( 'NONE',  ( -15.23076923076922995, -12.62096338111211580, 30.90682066428153263 ) ) ;
#40916=VECTOR ( 'NONE', #51832, 1000.000000000000114 ) ;
#40917=FACE_BOUND ( 'NONE', #83432, .T. ) ;
#40918=LINE ( 'NONE', #89124, #60533 ) ;
#40920=CARTESIAN_POINT ( 'NONE',  ( 5.076923076923075762, -12.48256725967547354, 35.29906147534542527 ) ) ;
#40921=CARTESIAN_POINT ( 'NONE',  ( 0.7114838709165038910, -4.932303261841488151, 34.32971442181322885 ) ) ;
#40923=CARTESIAN_POINT ( 'NONE',  ( -10.61538461538461320, -11.35647404775217417, 33.31231777344666511 ) ) ;
#40926=VECTOR ( 'NONE', #76423, 1000.000000000000000 ) ;
#40928=VECTOR ( 'NONE', #40278, 1000.000000000000000 ) ;
#40929=CARTESIAN_POINT ( 'NONE',  ( -9.692307692307814193, -2.657715359629662544, 31.77849191805970364 ) ) ;
#40930=CYLINDRICAL_SURFACE ( 'NONE', #55600, 0.2500000000000002220 ) ;
#40931=CARTESIAN_POINT ( 'NONE',  ( 6.857323494763590155, -7.249945578846651806, 34.99404164642496795 ) ) ;
#40932=B_SPLINE_CURVE_WITH_KNOTS ( 'NONE', 3,
 ( #22666, #72177, #37957, #77616, #15924, #16357, #43821, #71286, #10034, #9593 ),
 .UNSPECIFIED., .F., .F.,
 ( 4, 2, 2, 2, 4 ),
 ( 0.0007817359430256282712, 0.0009771253907249941549, 0.001172514838424359822, 0.001367904286123725706, 0.001563293733823091589 ),
 .UNSPECIFIED. ) ;
#40933=CARTESIAN_POINT ( 'NONE',  ( -1.384615384615383471, -13.75783147151868846, 33.36296068462461051 ) ) ;
#40934=CARTESIAN_POINT ( 'NONE',  ( 7.846153846153723244, -12.16647553114689728, 32.15551576947799362 ) ) ;
#40936=EDGE_CURVE ( 'NONE', #58918, #37595, #46396, .T. ) ;
#40937=CARTESIAN_POINT ( 'NONE',  ( -12.71151520558705172, -4.075325502946081535, 33.72974371597206300 ) ) ;
#40938=CARTESIAN_POINT ( 'NONE',  ( 1.161688425708536032, -10.01117774369187252, 34.36070679894347535 ) ) ;
#40940=CARTESIAN_POINT ( 'NONE',  ( 10.86543903529806521, -3.435999193479609914, 33.07426656108010832 ) ) ;
#40941=CARTESIAN_POINT ( 'NONE',  ( -4.946132635956126400, -6.369690395747422684, 34.87708834333098196 ) ) ;
#40942=CARTESIAN_POINT ( 'NONE',  ( 13.16168916709923664, -4.186968288167450147, 33.49512374952580274 ) ) ;
#40943=CARTESIAN_POINT ( 'NONE',  ( -3.360917200500924906, -10.31621877034669588, 34.18098118002070152 ) ) ;
#40944=CARTESIAN_POINT ( 'NONE',  ( -3.480745961711584346, -8.303909089506435137, 34.68538101551103381 ) ) ;
#40947=CARTESIAN_POINT ( 'NONE',  ( 1.161689167099237752, -2.554751324335734264, 30.48935550225260727 ) ) ;
#40948=CARTESIAN_POINT ( 'NONE',  ( -3.296039676730006640, -3.835265460703609186, 33.15142922261924241 ) ) ;
#40950=EDGE_CURVE ( 'NONE', #79461, #72151, #28032, .T. ) ;
#40951=CARTESIAN_POINT ( 'NONE',  ( -9.915792616872023402, -10.97335522853832579, 33.68706563782419749 ) ) ;
#40952=CARTESIAN_POINT ( 'NONE',  ( 5.076923076923075762, -11.16473453929635440, 33.15142922261926373 ) ) ;
#40953=CARTESIAN_POINT ( 'NONE',  ( 10.55011416942384095, -6.026961402152685388, 34.52809138561120506 ) ) ;
#40954=DIRECTION ( 'NONE',  ( -0.000000000000000000, 0.8660254037844397068, -0.4999999999999978906 ) ) ;
#40957=CARTESIAN_POINT ( 'NONE',  ( 17.99999999999987566, -3.835265460704628815, 33.15142922262033665 ) ) ;
#40958=EDGE_CURVE ( 'NONE', #42418, #42284, #3300, .T. ) ;
#40959=ORIENTED_EDGE ( 'NONE', *, *, #21630, .F. ) ;
#40960=CARTESIAN_POINT ( 'NONE',  ( -11.40841648254176732, -2.254550872974305342, 29.97347326024527092 ) ) ;
#40961=AXIS2_PLACEMENT_3D ( 'NONE', #86927, #52656, #80143 ) ;
#40962=CARTESIAN_POINT ( 'NONE',  ( -11.53846153846153655, -6.343179335718451384, 34.87096338111211935 ) ) ;
#40963=VERTEX_POINT ( 'NONE', #49888 ) ;
#40964=CARTESIAN_POINT ( 'NONE',  ( 7.716006636715624367, -4.460286881179643004, 33.72017969459903242 ) ) ;
#40965=CARTESIAN_POINT ( 'NONE',  ( 12.46153846153846168, -13.88283147151868846, 33.14645433367849847 ) ) ;
#40967=ADVANCED_FACE ( 'NONE', ( #85901 ), #71049, .F. ) ;
#40968=ORIENTED_EDGE ( 'NONE', *, *, #72138, .T. ) ;
#40969=ORIENTED_EDGE ( 'NONE', *, *, #5655, .T. ) ;
#40970=CARTESIAN_POINT ( 'NONE',  ( 17.86930939688968678, -9.929715669179216775, 34.40415004197138416 ) ) ;
#40971=B_SPLINE_CURVE_WITH_KNOTS ( 'NONE', 3,
 ( #62430, #56577, #14262, #55241, #84066, #43505, #49809, #747, #42627, #83624 ),
 .UNSPECIFIED., .F., .F.,
 ( 4, 2, 2, 2, 4 ),
 ( 0.0007817359430256390048, 0.0009771253907250078159, 0.001172514838424376735, 0.001367904286123745655, 0.001563293733823114574 ),
 .UNSPECIFIED. ) ;
#40972=VERTEX_POINT ( 'NONE', #3022 ) ;
#40974=CARTESIAN_POINT ( 'NONE',  ( 6.000000000000001776, -12.09954503811598769, 35.62045528018868623 ) ) ;
#40975=DIRECTION ( 'NONE',  ( 0.000000000000000000, 0.8660254037844377084, 0.5000000000000015543 ) ) ;
#40976=CARTESIAN_POINT ( 'NONE',  ( -10.61538461538473399, -2.625532179533778709, 30.86335684631627174 ) ) ;
#40977=ADVANCED_FACE ( 'NONE', ( #2146 ), #57974, .F. ) ;
#40978=CARTESIAN_POINT ( 'NONE',  ( -6.792551484843279752, -11.66157788607254275, 32.95092075102925833 ) ) ;
#40979=LINE ( 'NONE', #13940, #47864 ) ;
#40980=CARTESIAN_POINT ( 'NONE',  ( -13.38461538461538325, -2.249999999999998668, 29.75000000000001776 ) ) ;
#40981=CARTESIAN_POINT ( 'NONE',  ( 16.15384615384615330, -12.62096338111211580, 30.90682066428153263 ) ) ;
#40983=ADVANCED_FACE ( 'NONE', ( #51190 ), #71934, .F. ) ;
#40985=ORIENTED_EDGE ( 'NONE', *, *, #39125, .T. ) ;
#40986=DIRECTION ( 'NONE',  ( -0.000000000000000000, 0.6427876096865404731, -0.7660444431189771253 ) ) ;
#40987=ORIENTED_EDGE ( 'NONE', *, *, #7212, .T. ) ;
#40989=CARTESIAN_POINT ( 'NONE',  ( -5.326899820971668476, -4.818429247618089661, 34.26397095200675125 ) ) ;
#40990=EDGE_CURVE ( 'NONE', #88116, #9579, #45264, .T. ) ;
#40991=CARTESIAN_POINT ( 'NONE',  ( -8.703975629717929152, -11.06231777344671130, 33.60647404775212976 ) ) ;
#40992=DIRECTION ( 'NONE',  ( -0.000000000000000000, -0.3420201433256694346, -0.9396926207859080948 ) ) ;
#40993=CIRCLE ( 'NONE', #32373, 5.000000000000000888 ) ;
#40994=ORIENTED_EDGE ( 'NONE', *, *, #30477, .T. ) ;
#40995=CARTESIAN_POINT ( 'NONE',  ( 9.692307692307695177, -12.34228464037088635, 31.77849191805839268 ) ) ;
#40996=EDGE_LOOP ( 'NONE', ( #34962, #42836, #6972, #34105 ) ) ;
#40997=CARTESIAN_POINT ( 'NONE',  ( 7.911408985666682270, -12.70778746994558439, 30.41441678777536595 ) ) ;
#40998=ORIENTED_EDGE ( 'NONE', *, *, #50958, .F. ) ;
#40999=CARTESIAN_POINT ( 'NONE',  ( -10.54921547442195795, -7.250054483168843156, 34.74374881642865631 ) ) ;
#41000=ORIENTED_EDGE ( 'NONE', *, *, #40324, .F. ) ;
#41001=CARTESIAN_POINT ( 'NONE',  ( -16.37733109757010652, -6.760086850603066466, 34.69517049084099369 ) ) ;
#41002=EDGE_CURVE ( 'NONE', #35887, #73980, #15125, .T. ) ;
#41003=CARTESIAN_POINT ( 'NONE',  ( 10.61538461538461675, -4.786620604624113540, 33.94971097300155094 ) ) ;
#41004=FACE_BOUND ( 'NONE', #88086, .T. ) ;
#41005=B_SPLINE_CURVE_WITH_KNOTS ( 'NONE', 3,
 ( #24286, #2682, #45452, #72482, #44109, #29737, #10790, #58967, #38261, #52207 ),
 .UNSPECIFIED., .F., .F.,
 ( 4, 2, 2, 2, 4 ),
 ( 0.000000000000000000, 0.0001954339881912783015, 0.0003908679763825566029, 0.0005863019645738348773, 0.0007817359527651132059 ),
 .UNSPECIFIED. ) ;
#41007=CARTESIAN_POINT ( 'NONE',  ( 17.07692307692295586, -2.625532179533778709, 30.86335684631627174 ) ) ;
#41008=FACE_OUTER_BOUND ( 'NONE', #64076, .T. ) ;
#41011=CARTESIAN_POINT ( 'NONE',  ( -5.011667937410237528, -4.320704448112861584, 33.92786785259548310 ) ) ;
#41012=LINE ( 'NONE', #47760, #63479 ) ;
#41013=CARTESIAN_POINT ( 'NONE',  ( 14.43821774592595197, -6.808710257144161559, 34.95449254468098843 ) ) ;
#41014=EDGE_LOOP ( 'NONE', ( #36429, #31952 ) ) ;
#41017=CARTESIAN_POINT ( 'NONE',  ( 2.177545098254088707, -10.88202310037936194, 33.43294751532457099 ) ) ;
#41018=CARTESIAN_POINT ( 'NONE',  ( -7.846153846153844924, -13.63283147151868846, 33.57946703557072254 ) ) ;
#41019=CARTESIAN_POINT ( 'NONE',  ( 7.053868730901711182, -6.413143153341454017, 34.63066358083362672 ) ) ;
#41020=DIRECTION ( 'NONE',  ( -0.000000000000000000, 0.8660254037844397068, -0.4999999999999978906 ) ) ;
#41022=DIRECTION ( 'NONE',  ( -0.000000000000000000, 0.9848077530122085754, -0.1736481776669273613 ) ) ;
#41024=EDGE_CURVE ( 'NONE', #20214, #48033, #73736, .T. ) ;
#41025=CARTESIAN_POINT ( 'NONE',  ( 17.32686859527121470, -3.202959910592336090, 32.30730279482227019 ) ) ;
#41026=CARTESIAN_POINT ( 'NONE',  ( -4.946397375159516052, -2.619367082507848554, 30.83698974864644171 ) ) ;
#41027=CYLINDRICAL_SURFACE ( 'NONE', #74670, 0.2499999999999973355 ) ;
#41028=LINE ( 'NONE', #32940, #48236 ) ;
#41029=ORIENTED_EDGE ( 'NONE', *, *, #79066, .T. ) ;
#41031=VERTEX_POINT ( 'NONE', #19658 ) ;
#41032=ORIENTED_EDGE ( 'NONE', *, *, #29496, .T. ) ;
#41033=EDGE_CURVE ( 'NONE', #70251, #76766, #53435, .T. ) ;
#41034=CARTESIAN_POINT ( 'NONE',  ( 15.48082354240754555, -6.567000820036036579, 34.66262288849541306 ) ) ;
#41035=VERTEX_POINT ( 'NONE', #33622 ) ;
#41036=FACE_OUTER_BOUND ( 'NONE', #60276, .T. ) ;
#41037=DIRECTION ( 'NONE',  ( -0.000000000000000000, -0.7660444431189791237, -0.6427876096865379196 ) ) ;
#41039=CARTESIAN_POINT ( 'NONE',  ( -2.307692307692305711, -4.786620604624113540, 33.94971097300155094 ) ) ;
#41040=B_SPLINE_CURVE_WITH_KNOTS ( 'NONE', 3,
 ( #50950, #4109, #78003, #56841, #16307, #17645, #64469, #50080, #77564, #9540 ),
 .UNSPECIFIED., .F., .F.,
 ( 4, 2, 2, 2, 4 ),
 ( 0.000000000000000000, 0.0001954311564186876063, 0.0003908623128373752125, 0.0005862934692560628188, 0.0007817246256747504250 ),
 .UNSPECIFIED. ) ;
#41042=CARTESIAN_POINT ( 'NONE',  ( 14.30769230769231015, -4.098570777380720287, 33.41473453929634729 ) ) ;
#41045=CARTESIAN_POINT ( 'NONE',  ( -12.21148414990014963, -11.79725096376909299, 32.30694842903960762 ) ) ;
#41046=ORIENTED_EDGE ( 'NONE', *, *, #66343, .T. ) ;
#41048=CARTESIAN_POINT ( 'NONE',  ( 18.00000000000000000, -2.721908614388771852, 31.22303859784724978 ) ) ;
#41049=DIRECTION ( 'NONE',  ( 0.000000000000000000, 0.9396926207859126468, -0.3420201433256571111 ) ) ;
#41050=DIRECTION ( 'NONE',  ( -0.000000000000000000, -0.9396926207859092051, -0.3420201433256662704 ) ) ;
#41051=FACE_OUTER_BOUND ( 'NONE', #73219, .T. ) ;
#41053=CARTESIAN_POINT ( 'NONE',  ( -0.4615384615384611200, -12.10708131394839349, 31.69288490824020244 ) ) ;
#41054=CARTESIAN_POINT ( 'NONE',  ( -2.307692307692428724, -5.094484230521993062, 34.41647553114689373 ) ) ;
#41056=ORIENTED_EDGE ( 'NONE', *, *, #49941, .T. ) ;
#41057=CARTESIAN_POINT ( 'NONE',  ( 15.00728428704528561, -8.496056993536548418, 34.65000542017679663 ) ) ;
#41058=CARTESIAN_POINT ( 'NONE',  ( -9.692307692307814193, -9.528491918059723176, 34.59228464037033035 ) ) ;
#41059=DIRECTION ( 'NONE',  ( -0.000000000000000000, -0.000000000000000000, -1.000000000000000000 ) ) ;
#41060=ORIENTED_EDGE ( 'NONE', *, *, #82508, .F. ) ;
#41061=CARTESIAN_POINT ( 'NONE',  ( -4.153846153846152411, -6.343179335718451384, 34.87096338111211935 ) ) ;
#41064=EDGE_CURVE ( 'NONE', #77857, #998, #87252, .T. ) ;
#41065=CARTESIAN_POINT ( 'NONE',  ( 10.86543903529806876, -4.818054556918156983, 34.26375889529406749 ) ) ;
#41067=CARTESIAN_POINT ( 'NONE',  ( -14.55766905174090020, -2.920706130388546651, 32.31842814019191223 ) ) ;
#41069=LINE ( 'NONE', #42407, #59225 ) ;
#41070=CARTESIAN_POINT ( 'NONE',  ( -5.076923076923075762, -9.780366693483667717, 34.19971097300155094 ) ) ;
#41071=CARTESIAN_POINT ( 'NONE',  ( -14.55769230769230838, -7.433932668274256805, 35.00000000000000711 ) ) ;
#41073=CARTESIAN_POINT ( 'NONE',  ( -8.519230769230702549, -7.434744860731433924, 35.00000000000000711 ) ) ;
#41074=B_SPLINE_CURVE_WITH_KNOTS ( 'NONE', 3,
 ( #39486, #5239, #11107, #66499, #12877, #5677, #19637, #88568, #73255, #81352 ),
 .UNSPECIFIED., .F., .F.,
 ( 4, 2, 2, 2, 4 ),
 ( 0.0007817246256747484735, 0.0009771112852218922368, 0.001172497944769036217, 0.001367884604316180197, 0.001563271263863323960 ),
 .UNSPECIFIED. ) ;
#41076=CARTESIAN_POINT ( 'NONE',  ( -16.21992956480203318, -5.557115091759785130, 34.35708131394839171 ) ) ;
#41079=ORIENTED_EDGE ( 'NONE', *, *, #78657, .T. ) ;
#41080=CYLINDRICAL_SURFACE ( 'NONE', #44731, 0.2500000000000004996 ) ;
#41081=CARTESIAN_POINT ( 'NONE',  ( -8.899922235898330314, -2.541943142973491554, 30.39792223712631980 ) ) ;
#41082=CARTESIAN_POINT ( 'NONE',  ( -10.61538461538473399, -6.026961402154118019, 34.52809138561165270 ) ) ;
#41083=VECTOR ( 'NONE', #35853, 1000.000000000000000 ) ;
#41084=CARTESIAN_POINT ( 'NONE',  ( 11.53846153846153832, -12.34228464037088635, 31.77849191805839268 ) ) ;
#41085=CARTESIAN_POINT ( 'NONE',  ( -1.449885385171704399, -11.06231777344662781, 33.60647404775220082 ) ) ;
#41086=B_SPLINE_CURVE_WITH_KNOTS ( 'NONE', 3,
 ( #35481, #21068, #22408, #48994, #62933, #1245, #15219, #8903, #28735, #75574 ),
 .UNSPECIFIED., .F., .F.,
 ( 4, 2, 2, 2, 4 ),
 ( 0.0007817359430256367279, 0.0009771253907250045632, 0.001172514838424372615, 0.001367904286123740668, 0.001563293733823108503 ),
 .UNSPECIFIED. ) ;
#41089=FACE_BOUND ( 'NONE', #4911, .T. ) ;
#41090=VERTEX_POINT ( 'NONE', #52546 ) ;
#41093=FACE_OUTER_BOUND ( 'NONE', #54824, .T. ) ;
#41095=DIRECTION ( 'NONE',  ( -0.000000000000000000, -0.9396926207859092051, -0.3420201433256662704 ) ) ;
#41096=CARTESIAN_POINT ( 'NONE',  ( 17.01083966596718611, -2.538708090699995257, 30.37095296980875148 ) ) ;
#41097=B_SPLINE_CURVE_WITH_KNOTS ( 'NONE', 3,
 ( #12353, #39830, #65945, #79480, #45233, #3806 ),
 .UNSPECIFIED., .F., .F.,
 ( 4, 2, 4 ),
 ( 0.0003909512603273928937, 0.0005862562993132217288, 0.0007815613382990504012 ),
 .UNSPECIFIED. ) ;
#41098=ORIENTED_EDGE ( 'NONE', *, *, #15801, .T. ) ;
#41101=EDGE_LOOP ( 'NONE', ( #84449, #61082 ) ) ;
#41102=CARTESIAN_POINT ( 'NONE',  ( -3.099978789802278367, -11.37503395064541678, 33.29242100308974983 ) ) ;
#41104=AXIS2_PLACEMENT_3D ( 'NONE', #19210, #21863, #6582 ) ;
#41105=CARTESIAN_POINT ( 'NONE',  ( 4.376625822824220080, -10.23759521482555357, 34.22997729860117033 ) ) ;
#41106=EDGE_CURVE ( 'NONE', #8808, #67806, #46686, .T. ) ;
#41107=CARTESIAN_POINT ( 'NONE',  ( -11.53846153846166089, -5.941354392335915335, 34.76329471203413846 ) ) ;
#41108=CARTESIAN_POINT ( 'NONE',  ( 4.023698944407932743, -3.285722584762969856, 32.44110544564090759 ) ) ;
#41109=CARTESIAN_POINT ( 'NONE',  ( 4.088595163684911604, -2.506253911140460477, 30.00000000000013856 ) ) ;
#41110=CARTESIAN_POINT ( 'NONE',  ( 4.946232473812766095, -9.929715669179216775, 34.40415004197138416 ) ) ;
#41111=CARTESIAN_POINT ( 'NONE',  ( -4.219096085620237524, -2.255955759149247619, 30.00000000000013856 ) ) ;
#41112=CARTESIAN_POINT ( 'NONE',  ( -2.084680956079456582, -3.587049720035815348, 32.86302985866382897 ) ) ;
#41113=CARTESIAN_POINT ( 'NONE',  ( 11.53846153846141753, -10.21337939537710326, 33.94971097300076224 ) ) ;
#41116=ORIENTED_EDGE ( 'NONE', *, *, #1423, .T. ) ;
#41117=ORIENTED_EDGE ( 'NONE', *, *, #73017, .T. ) ;
#41118=CARTESIAN_POINT ( 'NONE',  ( -1.515306851282941292, -11.18331474514187995, 33.13161551792790505 ) ) ;
#41119=CARTESIAN_POINT ( 'NONE',  ( 1.515141086378948954, -6.001044277235011215, 34.52024696741798948 ) ) ;
#41120=CARTESIAN_POINT ( 'NONE',  ( 13.63461538461538680, -2.249999999999998668, 29.75000000000000355 ) ) ;
#41121=FACE_OUTER_BOUND ( 'NONE', #57390, .T. ) ;
#41122=CARTESIAN_POINT ( 'NONE',  ( 10.61538461538461675, -12.29105614889573062, 35.45975837776705220 ) ) ;
#41123=FACE_BOUND ( 'NONE', #59841, .T. ) ;
#41124=CARTESIAN_POINT ( 'NONE',  ( -7.146003881983771677, -3.395401636524186362, 33.02366814457250399 ) ) ;
#41125=EDGE_LOOP ( 'NONE', ( #36193, #66185 ) ) ;
#41127=CYLINDRICAL_SURFACE ( 'NONE', #47588, 0.2499999999999993616 ) ;
#41129=EDGE_LOOP ( 'NONE', ( #19379, #14521, #6525, #4518 ) ) ;
#41130=CARTESIAN_POINT ( 'NONE',  ( 4.826899852701618698, -2.341070481393820124, 30.72580821765574299 ) ) ;
#41131=EDGE_CURVE ( 'NONE', #85190, #19800, #11124, .T. ) ;
#41132=VERTEX_POINT ( 'NONE', #31852 ) ;
#41133=FACE_BOUND ( 'NONE', #23833, .T. ) ;
#41134=B_SPLINE_CURVE_WITH_KNOTS ( 'NONE', 3,
 ( #60669, #61551, #26892, #61113, #89056, #27335, #80967, #39539, #12060, #18808 ),
 .UNSPECIFIED., .F., .F.,
 ( 4, 2, 2, 2, 4 ),
 ( 0.0007817246256747450040, 0.0009771112852218881168, 0.001172497944769031230, 0.001367884604316174342, 0.001563271263863317455 ),
 .UNSPECIFIED. ) ;
#41135=DIRECTION ( 'NONE',  ( -0.000000000000000000, -0.7660444431189792347, -0.6427876096865379196 ) ) ;
#41136=AXIS2_PLACEMENT_3D ( 'NONE', #43152, #70622, #37715 ) ;
#41138=LINE ( 'NONE', #35717, #30329 ) ;
#41139=EDGE_LOOP ( 'NONE', ( #41306, #5211, #38819, #4118 ) ) ;
#41141=DIRECTION ( 'NONE',  ( 0.000000000000000000, 0.3420201433256641055, -0.9396926207859100932 ) ) ;
#41142=LINE ( 'NONE', #60519, #27965 ) ;
#41143=DIRECTION ( 'NONE',  ( 1.000000000000000000, 0.000000000000000000, 0.000000000000000000 ) ) ;
#41144=ORIENTED_EDGE ( 'NONE', *, *, #27322, .T. ) ;
#41146=ADVANCED_FACE ( 'NONE', ( #26423 ), #74164, .F. ) ;
#41147=CARTESIAN_POINT ( 'NONE',  ( -6.923076923076922462, -11.11383981884818262, 36.00935417666054406 ) ) ;
#41149=CARTESIAN_POINT ( 'NONE',  ( 14.30769230769218581, -12.70778746994576025, 30.41441678777401236 ) ) ;
#41150=EDGE_LOOP ( 'NONE', ( #31809, #55381, #2076, #17095 ) ) ;
#41151=CARTESIAN_POINT ( 'NONE',  ( 15.90386940979756503, -4.075325502946085976, 33.72974371597207721 ) ) ;
#41152=CARTESIAN_POINT ( 'NONE',  ( 5.933916589044120116, -8.973038597847269315, 34.52809138561120506 ) ) ;
#41153=CARTESIAN_POINT ( 'NONE',  ( -11.76194648218548622, -8.496056993536548418, 34.65000542017679663 ) ) ;
#41154=CARTESIAN_POINT ( 'NONE',  ( -4.153846153846152411, -6.681629849574314051, 35.83090037661290239 ) ) ;
#41155=CARTESIAN_POINT ( 'NONE',  ( -13.16160254052198830, -3.395485233115139057, 33.02377354290275946 ) ) ;
#41156=CARTESIAN_POINT ( 'NONE',  ( 12.46153846153846168, -2.517432740324522911, 35.29906147534542527 ) ) ;
#41158=EDGE_CURVE ( 'NONE', #86621, #63322, #37760, .T. ) ;
#41159=CARTESIAN_POINT ( 'NONE',  ( 5.076923076923075762, -13.49023893513002648, 31.06009739812518688 ) ) ;
#41161=EDGE_LOOP ( 'NONE', ( #10352, #9314 ) ) ;
#41162=DIRECTION ( 'NONE',  ( -0.000000000000000000, 1.000000000000000000, 3.491481338843133355E-15 ) ) ;
#41163=VERTEX_POINT ( 'NONE', #60637 ) ;
#41164=ORIENTED_EDGE ( 'NONE', *, *, #85063, .F. ) ;
#41166=EDGE_LOOP ( 'NONE', ( #26672, #26794, #19685, #3968 ) ) ;
#41167=CARTESIAN_POINT ( 'NONE',  ( 14.08476609017615644, -8.239355502252617924, 34.69524867566427417 ) ) ;
#41169=CARTESIAN_POINT ( 'NONE',  ( -14.17716686945866655, -3.068774925481847493, 32.56582465632704526 ) ) ;
#41170=EDGE_CURVE ( 'NONE', #47265, #65473, #20542, .T. ) ;
#41172=CARTESIAN_POINT ( 'NONE',  ( 6.223011351612850461, -3.105924265160262543, 32.13625925475356127 ) ) ;
#41173=CARTESIAN_POINT ( 'NONE',  ( -11.76138775597768138, -11.24512374952581872, 33.06303171183252942 ) ) ;
#41174=CARTESIAN_POINT ( 'NONE',  ( -15.36145983387954139, -4.684245665217972032, 34.18127051446801090 ) ) ;
#41175=CARTESIAN_POINT ( 'NONE',  ( -10.61538461538461320, -12.78798330534102945, 29.74999999999997868 ) ) ;
#41177=ADVANCED_FACE ( 'NONE', ( #62841 ), #26864, .F. ) ;
#41178=EDGE_CURVE ( 'NONE', #6173, #37287, #62481, .T. ) ;
#41179=FACE_OUTER_BOUND ( 'NONE', #78659, .T. ) ;
#41181=B_SPLINE_CURVE_WITH_KNOTS ( 'NONE', 3,
 ( #79474, #53768, #81255, #53318, #39386, #5587, #33058, #32608, #80821, #24511 ),
 .UNSPECIFIED., .F., .F.,
 ( 4, 2, 2, 2, 4 ),
 ( 0.0007817246256747469556, 0.0009771112852218902852, 0.001172497944769033615, 0.001367884604316176728, 0.001563271263863320057 ),
 .UNSPECIFIED. ) ;
#41182=CYLINDRICAL_SURFACE ( 'NONE', #23454, 0.2499999999999986955 ) ;
#41183=CARTESIAN_POINT ( 'NONE',  ( -13.25408968285182532, -11.46989282347013095, 32.79007818306219946 ) ) ;
#41184=EDGE_CURVE ( 'NONE', #6648, #70140, #7029, .T. ) ;
#41185=B_SPLINE_CURVE_WITH_KNOTS ( 'NONE', 3,
 ( #5610, #45701, #11036, #65966, #12370, #60547, #39849, #18690, #52893, #47025 ),
 .UNSPECIFIED., .F., .F.,
 ( 4, 2, 2, 2, 4 ),
 ( 0.000000000000000000, 0.0001954311564186856818, 0.0003908623128373713636, 0.0005862934692560570725, 0.0007817246256747427272 ),
 .UNSPECIFIED. ) ;
#41186=VERTEX_POINT ( 'NONE', #61522 ) ;
#41187=ORIENTED_EDGE ( 'NONE', *, *, #26758, .F. ) ;
#41188=FACE_OUTER_BOUND ( 'NONE', #78656, .T. ) ;
#41189=CARTESIAN_POINT ( 'NONE',  ( 1.384615384615264011, -3.643525952248795718, 33.31231777344771672 ) ) ;
#41190=CARTESIAN_POINT ( 'NONE',  ( -6.923076923076922462, -11.91647553114624181, 32.58852847137148245 ) ) ;
#41191=CARTESIAN_POINT ( 'NONE',  ( -11.47229239749887952, -7.250054483168843156, 34.74374881642865631 ) ) ;
#41192=CARTESIAN_POINT ( 'NONE',  ( -16.02305571287920216, -8.191423895709842640, 34.95447573519442130 ) ) ;
#41193=CARTESIAN_POINT ( 'NONE',  ( 11.76147438255493327, -4.026326845037962343, 33.68677907613344047 ) ) ;
#41195=EDGE_LOOP ( 'NONE', ( #17682, #51595, #1199, #15735 ) ) ;
#41197=ORIENTED_EDGE ( 'NONE', *, *, #25687, .T. ) ;
#41198=ADVANCED_FACE ( 'NONE', ( #54322 ), #28182, .F. ) ;
#41199=CARTESIAN_POINT ( 'NONE',  ( -8.703163435880695076, -4.661471528628508665, 34.16647553114624003 ) ) ;
#41200=CARTESIAN_POINT ( 'NONE',  ( 3.931018056211275535, -7.369209533119140509, 34.99857337881830688 ) ) ;
#41201=VECTOR ( 'NONE', #41739, 1000.000000000000000 ) ;
#41202=CARTESIAN_POINT ( 'NONE',  ( 14.24160889673642849, -4.786620604624113540, 33.94971097300155805 ) ) ;
#41203=CARTESIAN_POINT ( 'NONE',  ( -15.45369544828538011, -3.105860786376062332, 32.13614157043599562 ) ) ;
#41205=B_SPLINE_CURVE_WITH_KNOTS ( 'NONE', 3,
 ( #45097, #73921, #33379, #4564, #26613, #6356, #11319, #32475, #13102, #88782 ),
 .UNSPECIFIED., .F., .F.,
 ( 4, 2, 2, 2, 4 ),
 ( 0.0007817246256747489071, 0.0009771112852218922368, 0.001172497944769035350, 0.001367884604316178679, 0.001563271263863322009 ),
 .UNSPECIFIED. ) ;
#41207=ORIENTED_EDGE ( 'NONE', *, *, #58722, .F. ) ;
#41208=ADVANCED_FACE ( 'NONE', ( #68733 ), #21878, .F. ) ;
#41209=VERTEX_POINT ( 'NONE', #89029 ) ;
#41212=EDGE_LOOP ( 'NONE', ( #57153, #33343, #13076, #29455 ) ) ;
#41213=VECTOR ( 'NONE', #36286, 1000.000000000000000 ) ;
#41214=CARTESIAN_POINT ( 'NONE',  ( -6.249976744048591826, -4.818429247618089661, 34.26397095200675125 ) ) ;
#41215=DIRECTION ( 'NONE',  ( 0.000000000000000000, 0.1736481776669267785, -0.9848077530122087975 ) ) ;
#41216=EDGE_CURVE ( 'NONE', #59376, #37064, #67768, .T. ) ;
#41219=CARTESIAN_POINT ( 'NONE',  ( -15.16551409125639260, -9.528491918058460186, 34.59228464037086326 ) ) ;
#41220=CARTESIAN_POINT ( 'NONE',  ( 14.05771557674995442, -12.41269422305637171, 30.68257228309993323 ) ) ;
#41221=ORIENTED_EDGE ( 'NONE', *, *, #10470, .T. ) ;
#41223=ORIENTED_EDGE ( 'NONE', *, *, #75090, .F. ) ;
#41224=EDGE_CURVE ( 'NONE', #25798, #57772, #55941, .T. ) ;
#41225=CARTESIAN_POINT ( 'NONE',  ( -10.48459280755982803, -11.71459661697925903, 32.44059661609676937 ) ) ;
#41226=ORIENTED_EDGE ( 'NONE', *, *, #4682, .T. ) ;
#41227=DIRECTION ( 'NONE',  ( 0.000000000000000000, 0.1736481776669275834, 0.9848077530122086864 ) ) ;
#41228=CARTESIAN_POINT ( 'NONE',  ( -12.46153846153846168, -11.91647553114624181, 32.58852847137148245 ) ) ;
#41229=AXIS2_PLACEMENT_3D ( 'NONE', #20109, #41711, #7488 ) ;
#41231=VERTEX_POINT ( 'NONE', #41269 ) ;
#41232=ORIENTED_EDGE ( 'NONE', *, *, #5566, .F. ) ;
#41233=CARTESIAN_POINT ( 'NONE',  ( 7.846153846153725020, -12.27809138561165270, 31.22303859784587132 ) ) ;
#41234=EDGE_CURVE ( 'NONE', #44863, #20097, #78608, .T. ) ;
#41235=FACE_BOUND ( 'NONE', #38921, .T. ) ;
#41236=CARTESIAN_POINT ( 'NONE',  ( 6.792385456409367528, -4.118384482072085184, 33.43331474514187107 ) ) ;
#41237=CARTESIAN_POINT ( 'NONE',  ( -4.153846153846152411, -9.905515769479276145, 34.41647553114623292 ) ) ;
#41238=ORIENTED_EDGE ( 'NONE', *, *, #22159, .T. ) ;
#41239=EDGE_CURVE ( 'NONE', #77888, #46688, #719, .T. ) ;
#41240=CARTESIAN_POINT ( 'NONE',  ( -9.915792616872025178, -4.988325925672468131, 34.36044203135681130 ) ) ;
#41241=AXIS2_PLACEMENT_3D ( 'NONE', #63095, #49147, #9063 ) ;
#41242=AXIS2_PLACEMENT_3D ( 'NONE', #48138, #60325, #12596 ) ;
#41243=CARTESIAN_POINT ( 'NONE',  ( 9.019176178608812933, -8.476813868363244353, 34.90874843262270133 ) ) ;
#41244=CARTESIAN_POINT ( 'NONE',  ( 16.28463659481310444, -6.369690395747422684, 34.87708834333098196 ) ) ;
#41245=CARTESIAN_POINT ( 'NONE',  ( 15.23076923076910916, -6.835583212225970762, 34.95778746994575670 ) ) ;
#41246=ORIENTED_EDGE ( 'NONE', *, *, #61436, .F. ) ;
#41247=CARTESIAN_POINT ( 'NONE',  ( 6.223011351612851350, -8.239487800360276282, 34.69522927552633718 ) ) ;
#41248=CARTESIAN_POINT ( 'NONE',  ( 15.23076923076923173, -11.11383981884818262, 36.00935417666054406 ) ) ;
#41249=CARTESIAN_POINT ( 'NONE',  ( 17.32697738856138869, -9.943054286541403997, 34.11300777759954883 ) ) ;
#41250=CARTESIAN_POINT ( 'NONE',  ( -2.057637887778853703, -9.233818618650603938, 34.70587769442853698 ) ) ;
#41251=CARTESIAN_POINT ( 'NONE',  ( -15.10024352900566846, -11.93748526763465279, 32.05452791011430946 ) ) ;
#41252=FACE_BOUND ( 'NONE', #43091, .T. ) ;
#41253=CARTESIAN_POINT ( 'NONE',  ( -6.792286482109971324, -12.62708834333097663, 30.88030960425257021 ) ) ;
#41254=CARTESIAN_POINT ( 'NONE',  ( -6.250023224221455287, -10.18141759479407327, 34.26406193332782379 ) ) ;
#41255=EDGE_CURVE ( 'NONE', #81196, #9998, #51878, .T. ) ;
#41256=EDGE_CURVE ( 'NONE', #41090, #64564, #76370, .T. ) ;
#41257=CARTESIAN_POINT ( 'NONE',  ( 11.60371667797437567, -12.16647553114626490, 32.15551576947920864 ) ) ;
#41258=CARTESIAN_POINT ( 'NONE',  ( 3.454196192630801576, -7.630147231320743018, 34.74852402298682819 ) ) ;
#41260=CARTESIAN_POINT ( 'NONE',  ( -5.207613680033384540, -12.35290016733513951, 31.75349464988449455 ) ) ;
#41263=CARTESIAN_POINT ( 'NONE',  ( -8.992057461709771715, -7.369208160676171460, 34.74850200257122879 ) ) ;
#41264=ORIENTED_EDGE ( 'NONE', *, *, #77054, .F. ) ;
#41265=CARTESIAN_POINT ( 'NONE',  ( -13.38461538461550759, -9.528491918059723176, 34.59228464037033035 ) ) ;
#41266=VECTOR ( 'NONE', #66886, 1000.000000000000114 ) ;
#41267=EDGE_LOOP ( 'NONE', ( #28023, #48779 ) ) ;
#41268=LINE ( 'NONE', #70061, #36884 ) ;
#41269=CARTESIAN_POINT ( 'NONE',  ( -1.384615384615506484, -10.33852847137269571, 34.16647553114546554 ) ) ;
#41270=CARTESIAN_POINT ( 'NONE',  ( -9.692307692307814193, -11.67786785259630911, 32.92929555188603530 ) ) ;
#41271=EDGE_LOOP ( 'NONE', ( #39733, #79639, #47509, #17059 ) ) ;
#41272=CARTESIAN_POINT ( 'NONE',  ( 5.142990410273151625, -11.91647553114624358, 32.58852847137148245 ) ) ;
#41274=EDGE_CURVE ( 'NONE', #72334, #78742, #39862, .T. ) ;
#41275=CARTESIAN_POINT ( 'NONE',  ( -10.39260494640654819, -12.69155399931963046, 30.53255429739157734 ) ) ;
#41276=CARTESIAN_POINT ( 'NONE',  ( -7.146561847641255127, -12.69144148231606017, 30.53333754910549303 ) ) ;
#41279=LINE ( 'NONE', #68741, #1270 ) ;
#41280=CARTESIAN_POINT ( 'NONE',  ( 2.530703659305157061, -2.758310577978208666, 31.33698337089302299 ) ) ;
#41281=CARTESIAN_POINT ( 'NONE',  ( -18.00000000000000000, -13.54022505542197408, 30.56119799385072255 ) ) ;
#41284=EDGE_CURVE ( 'NONE', #57930, #11539, #49785, .T. ) ;
#41285=CARTESIAN_POINT ( 'NONE',  ( 11.40831356872984514, -5.915902021225889484, 34.75552854090298638 ) ) ;
#41286=CARTESIAN_POINT ( 'NONE',  ( 10.83816415665302202, -11.41317474335729543, 32.86274602512330034 ) ) ;
#41287=AXIS2_PLACEMENT_3D ( 'NONE', #74071, #66864, #52888 ) ;
#41291=DIRECTION ( 'NONE',  ( 0.000000000000000000, 1.000000000000000000, 0.000000000000000000 ) ) ;
#41292=CARTESIAN_POINT ( 'NONE',  ( 4.023236498642070558, -7.722926974430166069, 34.99546784045485737 ) ) ;
#41293=EDGE_LOOP ( 'NONE', ( #36770, #43968, #3169, #26842 ) ) ;
#41294=FACE_OUTER_BOUND ( 'NONE', #4323, .T. ) ;
#41295=CARTESIAN_POINT ( 'NONE',  ( -14.37377571864818293, -11.16473453929635440, 33.15142922261925662 ) ) ;
#41296=LINE ( 'NONE', #7057, #46917 ) ;
#41298=CARTESIAN_POINT ( 'NONE',  ( -5.299849294439224145, -5.667676309546437530, 34.40238873228292249 ) ) ;
#41299=CARTESIAN_POINT ( 'NONE',  ( 2.084207363968360482, -12.44517049084099725, 30.48991314939691932 ) ) ;
#41300=FACE_OUTER_BOUND ( 'NONE', #33921, .T. ) ;
#41301=LINE ( 'NONE', #68765, #85001 ) ;
#41302=CARTESIAN_POINT ( 'NONE',  ( 6.673053685783958855, -5.056417327199099532, 34.11270091957320716 ) ) ;
#41303=ORIENTED_EDGE ( 'NONE', *, *, #69442, .T. ) ;
#41304=ORIENTED_EDGE ( 'NONE', *, *, #12075, .F. ) ;
#41305=B_SPLINE_CURVE_WITH_KNOTS ( 'NONE', 3,
 ( #37429, #10863, #84317, #58144, #64900, #31115, #3205, #30678, #4085, #85631 ),
 .UNSPECIFIED., .F., .F.,
 ( 4, 2, 2, 2, 4 ),
 ( 0.0007817359430256253438, 0.0009771253907249898181, 0.001172514838424354401, 0.001367904286123718983, 0.001563293733823083566 ),
 .UNSPECIFIED. ) ;
#41306=ORIENTED_EDGE ( 'NONE', *, *, #15723, .F. ) ;
#41307=DIRECTION ( 'NONE',  ( 0.000000000000000000, 0.000000000000000000, 1.000000000000000000 ) ) ;
#41308=CARTESIAN_POINT ( 'NONE',  ( -2.241623956689868358, -5.557115091759786019, 34.35708131394839882 ) ) ;
#41311=LINE ( 'NONE', #34102, #39526 ) ;
#41312=CARTESIAN_POINT ( 'NONE',  ( -17.07692307692319744, -4.481592998941358097, 33.73612834414048933 ) ) ;
#41313=ORIENTED_EDGE ( 'NONE', *, *, #58628, .F. ) ;
#41314=ORIENTED_EDGE ( 'NONE', *, *, #29568, .F. ) ;
#41315=ORIENTED_EDGE ( 'NONE', *, *, #48700, .T. ) ;
#41318=CARTESIAN_POINT ( 'NONE',  ( -5.011667937410238416, -12.51329471203373700, 31.30864560766537963 ) ) ;
#41320=AXIS2_PLACEMENT_3D ( 'NONE', #5666, #33139, #26387 ) ;
#41321=DIRECTION ( 'NONE',  ( -0.000000000000000000, -0.9396926207859093161, -0.3420201433256663259 ) ) ;
#41322=CARTESIAN_POINT ( 'NONE',  ( -18.00000000000000000, -1.077559353945483744, 31.82153278338624602 ) ) ;
#41324=EDGE_LOOP ( 'NONE', ( #28441, #47186 ) ) ;
#41325=ORIENTED_EDGE ( 'NONE', *, *, #44800, .F. ) ;
#41327=CARTESIAN_POINT ( 'NONE',  ( -10.48485917715097138, -2.647132371071621471, 31.75357179365171589 ) ) ;
#41328=VERTEX_POINT ( 'NONE', #79827 ) ;
#41329=CARTESIAN_POINT ( 'NONE',  ( -4.153846153846152411, -1.422936976036506707, 30.56769352161908415 ) ) ;
#41330=B_SPLINE_CURVE_WITH_KNOTS ( 'NONE', 3,
 ( #74236, #33693, #27815, #81890, #87777, #26493 ),
 .UNSPECIFIED., .F., .F.,
 ( 4, 2, 4 ),
 ( 0.0003909512603273880690, 0.0005862562993132132720, 0.0007815613382990384750 ),
 .UNSPECIFIED. ) ;
#41331=LINE ( 'NONE', #74683, #55152 ) ;
#41333=AXIS2_PLACEMENT_3D ( 'NONE', #42291, #21107, #76059 ) ;
#41334=CARTESIAN_POINT ( 'NONE',  ( 9.019285080869085647, -12.41262288849542017, 30.68299917996395010 ) ) ;
#41335=CARTESIAN_POINT ( 'NONE',  ( -5.326923076923075762, -2.499999999999998668, 29.75000000000000355 ) ) ;
#41336=B_SPLINE_CURVE_WITH_KNOTS ( 'NONE', 3,
 ( #11204, #86893, #39135, #45420, #72899, #80109, #52625, #26501, #60272, #38674 ),
 .UNSPECIFIED., .F., .F.,
 ( 4, 2, 2, 2, 4 ),
 ( 0.0007817246256747440282, 0.0009771112852218863821, 0.001172497944769028844, 0.001367884604316171307, 0.001563271263863313769 ),
 .UNSPECIFIED. ) ;
#41337=ORIENTED_EDGE ( 'NONE', *, *, #31671, .F. ) ;
#41338=FACE_BOUND ( 'NONE', #84213, .T. ) ;
#41340=CARTESIAN_POINT ( 'NONE',  ( 15.93091919493929609, -2.523278758544490241, 31.42238647778636818 ) ) ;
#41341=EDGE_CURVE ( 'NONE', #20954, #11784, #72062, .T. ) ;
#41342=CARTESIAN_POINT ( 'NONE',  ( 3.361561038594018225, -8.999086150933472084, 34.52020707165672064 ) ) ;
#41343=CARTESIAN_POINT ( 'NONE',  ( 1.384615384615386802, -2.249999999999998668, 29.50000000000001421 ) ) ;
#41345=CARTESIAN_POINT ( 'NONE',  ( -4.023320452082589149, -2.882268652242224505, 31.66798894389554064 ) ) ;
#41346=CARTESIAN_POINT ( 'NONE',  ( -4.153846153846152411, -11.35647404775217417, 33.31231777344666511 ) ) ;
#41347=VERTEX_POINT ( 'NONE', #44678 ) ;
#41348=CARTESIAN_POINT ( 'NONE',  ( 14.43821800945587341, -12.45806712695776319, 30.39783852428763922 ) ) ;
#41349=PRODUCT_DEFINITION ( 'UNKNOWN', '', #15939, #9532 ) ;
#41351=EDGE_LOOP ( 'NONE', ( #70219, #37403, #73001, #4187 ) ) ;
#41352=DIRECTION ( 'NONE',  ( -0.000000000000000000, -0.8660254037844399289, -0.4999999999999980016 ) ) ;
#41354=ORIENTED_EDGE ( 'NONE', *, *, #62673, .T. ) ;
#41355=AXIS2_PLACEMENT_3D ( 'NONE', #52741, #19410, #18531 ) ;
#41356=DIRECTION ( 'NONE',  ( -0.000000000000000000, -0.7660444431189791237, -0.6427876096865379196 ) ) ;
#41357=CARTESIAN_POINT ( 'NONE',  ( -4.153846153846152411, -2.292212530054420494, 30.41441678777542634 ) ) ;
#41358=FACE_BOUND ( 'NONE', #43291, .T. ) ;
#41359=CARTESIAN_POINT ( 'NONE',  ( 8.769230769230768274, -3.322132147404559976, 32.92929555188717927 ) ) ;
#41360=LINE ( 'NONE', #20637, #4211 ) ;
#41361=CARTESIAN_POINT ( 'NONE',  ( 10.36536137809165403, -8.432397168068783699, 34.66272746175022945 ) ) ;
#41362=ADVANCED_FACE ( 'NONE', ( #84041 ), #35843, .F. ) ;
#41363=CARTESIAN_POINT ( 'NONE',  ( 12.46153846153846168, -12.34228464037088635, 31.77849191805839268 ) ) ;
#41365=CARTESIAN_POINT ( 'NONE',  ( -8.519176457592454454, -12.17597550085003633, 31.52189283813461884 ) ) ;
#41369=ORIENTED_EDGE ( 'NONE', *, *, #82435, .T. ) ;
#41370=EDGE_LOOP ( 'NONE', ( #51488, #55814 ) ) ;
#41371=CARTESIAN_POINT ( 'NONE',  ( -14.30769230769242739, -2.625532179533778709, 30.86335684631627174 ) ) ;
#41373=CARTESIAN_POINT ( 'NONE',  ( -10.36543920600657209, -8.476813868363244353, 34.90874843262270133 ) ) ;
#41374=CARTESIAN_POINT ( 'NONE',  ( -5.999999999999998224, -13.87047571288749737, 32.06866353760679544 ) ) ;
#41375=CARTESIAN_POINT ( 'NONE',  ( -0.6850233861027947846, -3.019605429927184836, 32.48692288466676814 ) ) ;
#41376=CARTESIAN_POINT ( 'NONE',  ( 3.007843013253084230, -11.24512374952581872, 33.06303171183252942 ) ) ;
#41378=CARTESIAN_POINT ( 'NONE',  ( -12.52680846209478460, -4.320704448112771878, 33.92786785259540494 ) ) ;
#41379=DIRECTION ( 'NONE',  ( 0.000000000000000000, 0.6427876096865368094, 0.7660444431189802339 ) ) ;
#41380=CARTESIAN_POINT ( 'NONE',  ( 15.36156103859402222, -11.71459661697925903, 32.44059661609676937 ) ) ;
#41382=LINE ( 'NONE', #7597, #45300 ) ;
#41383=CARTESIAN_POINT ( 'NONE',  ( 5.299702745901139878, -8.540255544307065350, 34.89611431652622286 ) ) ;
#41384=CARTESIAN_POINT ( 'NONE',  ( -16.15384615384615330, -12.78798330534102945, 29.74999999999997868 ) ) ;
#41385=EDGE_CURVE ( 'NONE', #77968, #33107, #31631, .T. ) ;
#41386=CARTESIAN_POINT ( 'NONE',  ( -6.857009589726848375, -3.322132147404559976, 32.92929555188717927 ) ) ;
#41387=CARTESIAN_POINT ( 'NONE',  ( 3.007843013253082010, -2.554751324335734264, 30.48935550225260727 ) ) ;
#41388=ORIENTED_EDGE ( 'NONE', *, *, #37289, .T. ) ;
#41389=FACE_OUTER_BOUND ( 'NONE', #30615, .T. ) ;
#41393=EDGE_CURVE ( 'NONE', #26228, #80339, #73198, .T. ) ;
#41394=LINE ( 'NONE', #34634, #37484 ) ;
#41395=AXIS2_PLACEMENT_3D ( 'NONE', #74033, #60508, #142 ) ;
#41396=CARTESIAN_POINT ( 'NONE',  ( -4.153846153846152411, -1.129524287112498415, 32.06866353760679544 ) ) ;
#41397=CARTESIAN_POINT ( 'NONE',  ( -9.757577692864012775, -5.941354392334499579, 34.76329471203369792 ) ) ;
#41398=CARTESIAN_POINT ( 'NONE',  ( 7.715462379486288214, -2.541943142973490666, 30.39792223712631980 ) ) ;
#41399=ORIENTED_EDGE ( 'NONE', *, *, #53826, .T. ) ;
#41401=CARTESIAN_POINT ( 'NONE',  ( -9.561517251340742263, -5.496552790871120031, 34.60292014791297532 ) ) ;
#41403=CARTESIAN_POINT ( 'NONE',  ( -4.153846153846152411, -2.517432740324522911, 35.29906147534542527 ) ) ;
#41404=AXIS2_PLACEMENT_3D ( 'NONE', #81487, #53549, #87362 ) ;
#41405=CARTESIAN_POINT ( 'NONE',  ( 7.596153846153846700, -7.566083408709834757, 34.74999999999999289 ) ) ;
#41406=ORIENTED_EDGE ( 'NONE', *, *, #63050, .F. ) ;
#41407=CARTESIAN_POINT ( 'NONE',  ( 7.596177115211490971, -4.236021600441998380, 33.53823185664189310 ) ) ;
#41408=CARTESIAN_POINT ( 'NONE',  ( 8.703148389870632329, -6.343179335718451384, 34.87096338111212646 ) ) ;
#41409=VECTOR ( 'NONE', #51793, 1000.000000000000227 ) ;
#41410=DIRECTION ( 'NONE',  ( 0.000000000000000000, 0.000000000000000000, 1.000000000000000000 ) ) ;
#41411=ORIENTED_EDGE ( 'NONE', *, *, #39872, .F. ) ;
#41412=ORIENTED_EDGE ( 'NONE', *, *, #41968, .F. ) ;
#41413=CARTESIAN_POINT ( 'NONE',  ( -6.792286482109971324, -8.191423895709842640, 34.95447573519442130 ) ) ;
#41414=EDGE_LOOP ( 'NONE', ( #41315, #82275, #2775, #66882 ) ) ;
#41415=LINE ( 'NONE', #40974, #60112 ) ;
#41416=CARTESIAN_POINT ( 'NONE',  ( 5.142178216435913107, -5.094484230520773593, 34.41647553114626845 ) ) ;
#41417=CARTESIAN_POINT ( 'NONE',  ( -15.36145983387954139, -2.295517848115769421, 30.44137282052137294 ) ) ;
#41418=DIRECTION ( 'NONE',  ( 0.000000000000000000, 0.9848077530122072432, -0.1736481776669354937 ) ) ;
#41419=DIRECTION ( 'NONE',  ( 0.000000000000000000, 0.4999999999999960032, -0.8660254037844410391 ) ) ;
#41421=CARTESIAN_POINT ( 'NONE',  ( -5.076923076923199218, -12.16647553114689728, 32.15551576947799362 ) ) ;
#41422=B_SPLINE_CURVE_WITH_KNOTS ( 'NONE', 3,
 ( #33196, #12923, #48468, #40411, #54788, #61990, #20563, #81836, #67868, #81396 ),
 .UNSPECIFIED., .F., .F.,
 ( 4, 2, 2, 2, 4 ),
 ( 0.0007817359430256326080, 0.0009771253907249993591, 0.001172514838424366110, 0.001367904286123732861, 0.001563293733823099612 ),
 .UNSPECIFIED. ) ;
#41423=VECTOR ( 'NONE', #32059, 1000.000000000000114 ) ;
#41424=ORIENTED_EDGE ( 'NONE', *, *, #25623, .F. ) ;
#41425=ORIENTED_EDGE ( 'NONE', *, *, #64913, .F. ) ;
#41426=CARTESIAN_POINT ( 'NONE',  ( -10.61538461538461320, -2.833524468853757305, 32.15551576947925838 ) ) ;
#41427=VERTEX_POINT ( 'NONE', #20347 ) ;
#41429=CARTESIAN_POINT ( 'NONE',  ( 7.623226887246997485, -2.523278758544489797, 31.42238647778637528 ) ) ;
#41430=VERTEX_POINT ( 'NONE', #39291 ) ;
#41431=CARTESIAN_POINT ( 'NONE',  ( -4.153846153846152411, -1.629998284177014645, 34.34916445242399163 ) ) ;
#41432=DIRECTION ( 'NONE',  ( 0.000000000000000000, 0.3420201433256641055, -0.9396926207859100932 ) ) ;
#41433=ORIENTED_EDGE ( 'NONE', *, *, #7447, .F. ) ;
#41434=CARTESIAN_POINT ( 'NONE',  ( 2.307692307692186251, -10.33852847137269571, 34.16647553114546554 ) ) ;
#41435=EDGE_CURVE ( 'NONE', #53468, #28895, #74317, .T. ) ;
#41436=ORIENTED_EDGE ( 'NONE', *, *, #48568, .T. ) ;
#41437=CARTESIAN_POINT ( 'NONE',  ( 7.912221179503920787, -12.62096338111211757, 30.90682066428152908 ) ) ;
#41438=VERTEX_POINT ( 'NONE', #61303 ) ;
#41439=CARTESIAN_POINT ( 'NONE',  ( -14.30769230769242917, -2.379036618888197729, 30.90682066428292885 ) ) ;
#41440=VERTEX_POINT ( 'NONE', #19449 ) ;
#41441=CARTESIAN_POINT ( 'NONE',  ( -16.40386939113911779, -6.695914987888146541, 34.68535235679833306 ) ) ;
#41442=CARTESIAN_POINT ( 'NONE',  ( -4.153846153846274980, -6.835583212225970762, 34.95778746994575670 ) ) ;
#41443=FACE_BOUND ( 'NONE', #5097, .T. ) ;
#41444=FACE_OUTER_BOUND ( 'NONE', #24822, .T. ) ;
#41445=CARTESIAN_POINT ( 'NONE',  ( -6.673022611438610419, -12.17597550085003633, 31.52189283813461884 ) ) ;
#41446=ADVANCED_FACE ( 'NONE', ( #82496 ), #80728, .F. ) ;
#41447=CARTESIAN_POINT ( 'NONE',  ( 4.403791672194296680, -12.43552623307873972, 30.55307653245132826 ) ) ;
#41448=CARTESIAN_POINT ( 'NONE',  ( -3.480745961711584346, -4.236021600441998380, 33.53823185664189310 ) ) ;
#41449=AXIS2_PLACEMENT_3D ( 'NONE', #75469, #54303, #62384 ) ;
#41451=CARTESIAN_POINT ( 'NONE',  ( -4.283993363284372080, -11.47017969459903952, 32.78971311882034456 ) ) ;
#41452=CARTESIAN_POINT ( 'NONE',  ( -17.07692307692307665, -12.37446782046654192, 30.86335684631486131 ) ) ;
#41453=EDGE_CURVE ( 'NONE', #45729, #40586, #68517, .T. ) ;
#41454=ORIENTED_EDGE ( 'NONE', *, *, #53478, .T. ) ;
#41455=VERTEX_POINT ( 'NONE', #55011 ) ;
#41456=VECTOR ( 'NONE', #990, 1000.000000000000227 ) ;
#41457=CARTESIAN_POINT ( 'NONE',  ( 2.307692307692187583, -10.90142922262034020, 33.41473453929536674 ) ) ;
#41458=CARTESIAN_POINT ( 'NONE',  ( -3.230769230769352962, -5.941354392335915335, 34.76329471203413846 ) ) ;
#41459=CARTESIAN_POINT ( 'NONE',  ( -11.66860874789975888, -11.93770438780619259, 32.05411857736982029 ) ) ;
#41460=CARTESIAN_POINT ( 'NONE',  ( -7.846153846153844924, -13.95598074871891292, 31.83374038241031911 ) ) ;
#41461=CARTESIAN_POINT ( 'NONE',  ( -10.55012947587177408, -12.51329471203373700, 31.30864560766537963 ) ) ;
#41462=CARTESIAN_POINT ( 'NONE',  ( 7.846153846153725020, -6.026961402154118019, 34.52809138561165270 ) ) ;
#41463=ORIENTED_EDGE ( 'NONE', *, *, #49395, .T. ) ;
#41464=CARTESIAN_POINT ( 'NONE',  ( 17.14299142792551578, -3.050289026998446840, 32.03036669348366416 ) ) ;
#41465=CARTESIAN_POINT ( 'NONE',  ( -14.43838291080261627, -9.929715669179220328, 34.40415004197138416 ) ) ;
#41466=CARTESIAN_POINT ( 'NONE',  ( -14.37296275365308418, -8.613356846314824011, 34.62446782046655613 ) ) ;
#41468=CARTESIAN_POINT ( 'NONE',  ( -8.638705330997128229, -2.647132371071621471, 31.75357179365171589 ) ) ;
#41469=EDGE_LOOP ( 'NONE', ( #50756, #66097 ) ) ;
#41470=ORIENTED_EDGE ( 'NONE', *, *, #3068, .T. ) ;
#41471=B_SPLINE_CURVE_WITH_KNOTS ( 'NONE', 3,
 ( #77360, #70606, #30498, #31390, #29627, #71926 ),
 .UNSPECIFIED., .F., .F.,
 ( 4, 2, 4 ),
 ( 4.224605973302673136E-17, 0.0001954756301637161251, 0.0003909512603273899664 ),
 .UNSPECIFIED. ) ;
#41473=EDGE_CURVE ( 'NONE', #38026, #38006, #40181, .T. ) ;
#41474=CARTESIAN_POINT ( 'NONE',  ( 0.5923768795512234231, -7.277220443632451463, 34.74524770363009196 ) ) ;
#41475=ORIENTED_EDGE ( 'NONE', *, *, #15289, .T. ) ;
#41476=CARTESIAN_POINT ( 'NONE',  ( -9.692307692307814193, -10.33852847137269571, 34.16647553114546554 ) ) ;
#41477=CARTESIAN_POINT ( 'NONE',  ( 15.23076923076910916, -4.320704448113951379, 33.92786785259630022 ) ) ;
#41478=CARTESIAN_POINT ( 'NONE',  ( 3.230769230769231726, -9.905515769479276145, 34.41647553114623292 ) ) ;
#41480=CARTESIAN_POINT ( 'NONE',  ( 9.822833394071261992, -6.001044277235009439, 34.52024696741798948 ) ) ;
#41482=CARTESIAN_POINT ( 'NONE',  ( -11.60421496677487063, -7.249945578846652694, 34.99404164642496795 ) ) ;
#41483=CARTESIAN_POINT ( 'NONE',  ( -12.33074665371367651, -11.71459661697925903, 32.44059661609676937 ) ) ;
#41484=VERTEX_POINT ( 'NONE', #74396 ) ;
#41486=CARTESIAN_POINT ( 'NONE',  ( 16.15384615384615330, -13.53365097954675988, 30.81389545987213552 ) ) ;
#41488=CARTESIAN_POINT ( 'NONE',  ( 8.992010438208831502, -12.11081565061823717, 32.26097654155341843 ) ) ;
#41491=CYLINDRICAL_SURFACE ( 'NONE', #6142, 0.2499999999999973355 ) ;
#41492=CARTESIAN_POINT ( 'NONE',  ( -0.7115616857599206257, -2.588893531581426988, 31.60682220781847818 ) ) ;
#41493=EDGE_CURVE ( 'NONE', #72231, #5606, #81164, .T. ) ;
#41496=AXIS2_PLACEMENT_3D ( 'NONE', #20959, #83581, #21858 ) ;
#41497=DIRECTION ( 'NONE',  ( 1.000000000000000000, 0.000000000000000000, 0.000000000000000000 ) ) ;
#41498=CARTESIAN_POINT ( 'NONE',  ( 1.384615384615264011, -9.528491918059723176, 34.59228464037033035 ) ) ;
#41500=CARTESIAN_POINT ( 'NONE',  ( -15.23076923076922995, -8.318370150425687726, 35.83090037661290239 ) ) ;
#41501=CARTESIAN_POINT ( 'NONE',  ( -13.25382357679060519, -8.147973898785416225, 34.70805048591653730 ) ) ;
#41502=EDGE_CURVE ( 'NONE', #76098, #22173, #18304, .T. ) ;
#41503=ORIENTED_EDGE ( 'NONE', *, *, #61789, .F. ) ;
#41504=CARTESIAN_POINT ( 'NONE',  ( -12.68446467905461006, -11.76352882383564769, 32.36236540154569497 ) ) ;
#41505=CARTESIAN_POINT ( 'NONE',  ( -15.93106661257773915, -12.24180327182771855, 31.33663988360758168 ) ) ;
#41506=CARTESIAN_POINT ( 'NONE',  ( 1.384615384615265343, -9.442884908241554243, 34.35708131394783038 ) ) ;
#41507=DIRECTION ( 'NONE',  ( -0.000000000000000000, -0.9848077530122085754, -0.1736481776669273613 ) ) ;
#41509=ORIENTED_EDGE ( 'NONE', *, *, #38520, .T. ) ;
#41510=CARTESIAN_POINT ( 'NONE',  ( -15.29603967673000575, -2.892918686051582977, 31.69288490824015980 ) ) ;
#41511=CARTESIAN_POINT ( 'NONE',  ( 3.480823542407545101, -12.17597550085003455, 31.52189283813461884 ) ) ;
#41512=CARTESIAN_POINT ( 'NONE',  ( 5.207448515156721136, -12.50538340440932217, 31.33453814440721885 ) ) ;
#41513=VERTEX_POINT ( 'NONE', #61749 ) ;
#41514=CYLINDRICAL_SURFACE ( 'NONE', #11071, 0.2499999999999998890 ) ;
#41515=ORIENTED_EDGE ( 'NONE', *, *, #88412, .T. ) ;
#41516=VECTOR ( 'NONE', #43260, 999.9999999999998863 ) ;
#41517=CARTESIAN_POINT ( 'NONE',  ( -7.846153846153844924, -5.471508081941601098, 34.59228464037088457 ) ) ;
#41518=CARTESIAN_POINT ( 'NONE',  ( 11.31553457955468467, -2.523278758544489797, 31.42238647778637528 ) ) ;
#41520=CARTESIAN_POINT ( 'NONE',  ( 7.780883400193071786, -12.27809138561121394, 31.22303859784730307 ) ) ;
#41521=DIRECTION ( 'NONE',  ( -0.000000000000000000, 0.9396926207859092051, -0.3420201433256662704 ) ) ;
#41522=DIRECTION ( 'NONE',  ( -0.000000000000000000, 0.3420201433256694346, -0.9396926207859080948 ) ) ;
#41523=VECTOR ( 'NONE', #48843, 1000.000000000000227 ) ;
#41524=VECTOR ( 'NONE', #16223, 1000.000000000000227 ) ;
#41525=CARTESIAN_POINT ( 'NONE',  ( -7.846153846153967493, -5.094484230521993062, 34.41647553114689373 ) ) ;
#41526=CARTESIAN_POINT ( 'NONE',  ( 3.480823542407545546, -12.41262288849542017, 30.68299917996395010 ) ) ;
#41527=EDGE_CURVE ( 'NONE', #5856, #88899, #29012, .T. ) ;
#41528=VECTOR ( 'NONE', #4914, 1000.000000000000114 ) ;
#41529=EDGE_LOOP ( 'NONE', ( #75791, #35637 ) ) ;
#41530=FACE_BOUND ( 'NONE', #60156, .T. ) ;
#41531=ORIENTED_EDGE ( 'NONE', *, *, #15305, .T. ) ;
#41532=LINE ( 'NONE', #83415, #65875 ) ;
#41533=EDGE_CURVE ( 'NONE', #1706, #17127, #69828, .T. ) ;
#41535=CYLINDRICAL_SURFACE ( 'NONE', #66055, 0.2500000000000012212 ) ;
#41536=CARTESIAN_POINT ( 'NONE',  ( 11.53846153846141753, -2.625532179533778709, 30.86335684631627174 ) ) ;
#41537=CARTESIAN_POINT ( 'NONE',  ( -11.47320596718551045, -2.625532179533470512, 30.86335684631491105 ) ) ;
#41538=ORIENTED_EDGE ( 'NONE', *, *, #85486, .T. ) ;
#41539=EDGE_CURVE ( 'NONE', #51846, #58941, #14919, .T. ) ;
#41540=ORIENTED_EDGE ( 'NONE', *, *, #45959, .F. ) ;
#41541=EDGE_LOOP ( 'NONE', ( #76925, #60691, #35543, #66213 ) ) ;
#41542=CARTESIAN_POINT ( 'NONE',  ( -10.61538461538461320, -8.164416787775445883, 34.95778746994557906 ) ) ;
#41543=VERTEX_POINT ( 'NONE', #36515 ) ;
#41544=CYLINDRICAL_SURFACE ( 'NONE', #15808, 0.2500000000000009437 ) ;
#41545=CARTESIAN_POINT ( 'NONE',  ( -9.915134384786696842, -7.369208160676171460, 34.74850200257122879 ) ) ;
#41546=FACE_OUTER_BOUND ( 'NONE', #1942, .T. ) ;
#41547=CARTESIAN_POINT ( 'NONE',  ( 11.28848480751918437, -2.564618984488975517, 30.55390908950641915 ) ) ;
#41548=CARTESIAN_POINT ( 'NONE',  ( 5.076923076922953193, -10.33852847137269571, 34.16647553114546554 ) ) ;
#41550=CARTESIAN_POINT ( 'NONE',  ( 14.43848411551709709, -6.413143153341454017, 34.63066358083362672 ) ) ;
#41551=CARTESIAN_POINT ( 'NONE',  ( 17.32697738856138869, -2.564540009722896752, 30.55348353981672105 ) ) ;
#41552=ORIENTED_EDGE ( 'NONE', *, *, #57121, .F. ) ;
#41553=EDGE_CURVE ( 'NONE', #54188, #22025, #11762, .T. ) ;
#41554=ORIENTED_EDGE ( 'NONE', *, *, #85118, .T. ) ;
#41555=ORIENTED_EDGE ( 'NONE', *, *, #21148, .F. ) ;
#41556=CARTESIAN_POINT ( 'NONE',  ( 3.165446315277056222, -7.749976743299137993, 34.99404534957040624 ) ) ;
#41558=CARTESIAN_POINT ( 'NONE',  ( 10.61538461538449596, -6.879047030192662504, 34.71129190930017927 ) ) ;
#41559=CYLINDRICAL_SURFACE ( 'NONE', #57158, 0.2500000000000009437 ) ;
#41560=CARTESIAN_POINT ( 'NONE',  ( -10.61538461538473399, -3.835265460704628371, 33.15142922262033665 ) ) ;
#41561=FACE_BOUND ( 'NONE', #55466, .T. ) ;
#41562=CARTESIAN_POINT ( 'NONE',  ( 9.915087233576105774, -3.755027918224367767, 33.06320215134714857 ) ) ;
#41563=VERTEX_POINT ( 'NONE', #42832 ) ;
#41564=CARTESIAN_POINT ( 'NONE',  ( 0.3962684609821406911, -11.67786785259540672, 32.92929555188720059 ) ) ;
#41565=DIRECTION ( 'NONE',  ( -0.000000000000000000, 0.7660444431189791237, -0.6427876096865379196 ) ) ;
#41566=CARTESIAN_POINT ( 'NONE',  ( 16.85399685940693004, -6.503392248772476236, 34.64988816332204635 ) ) ;
#41568=ORIENTED_EDGE ( 'NONE', *, *, #73588, .F. ) ;
#41569=CARTESIAN_POINT ( 'NONE',  ( 17.99999999999987566, -12.46129190930018460, 30.37095296980731973 ) ) ;
#41571=FACE_BOUND ( 'NONE', #74938, .T. ) ;
#41572=CARTESIAN_POINT ( 'NONE',  ( -17.20707104665477161, -4.299443229763728169, 33.91186481527756058 ) ) ;
#41573=B_SPLINE_CURVE_WITH_KNOTS ( 'NONE', 3,
 ( #25940, #53858, #39916, #11546, #5229, #81345, #67376, #25501, #39029, #88558 ),
 .UNSPECIFIED., .F., .F.,
 ( 4, 2, 2, 2, 4 ),
 ( 0.000000000000000000, 0.0001954339857564093175, 0.0003908679715128186350, 0.0005863019572692279796, 0.0007817359430256372700 ),
 .UNSPECIFIED. ) ;
#41575=CARTESIAN_POINT ( 'NONE',  ( -8.069020109216943126, -2.251424796025575770, 29.88072029997477230 ) ) ;
#41576=CARTESIAN_POINT ( 'NONE',  ( -12.68502338610278990, -12.11044203135681840, 32.26167407432752299 ) ) ;
#41577=ORIENTED_EDGE ( 'NONE', *, *, #64417, .T. ) ;
#41578=B_SPLINE_CURVE_WITH_KNOTS ( 'NONE', 3,
 ( #3903, #18771, #85895, #38593, #59299, #25076, #45786, #59749, #4813, #46238 ),
 .UNSPECIFIED., .F., .F.,
 ( 4, 2, 2, 2, 4 ),
 ( 0.0007817246256747461966, 0.0009771112852218892010, 0.001172497944769032314, 0.001367884604316175427, 0.001563271263863318323 ),
 .UNSPECIFIED. ) ;
#41579=CARTESIAN_POINT ( 'NONE',  ( 0.3954550505825812912, -10.51840700105979387, 33.73612834413961536 ) ) ;
#41580=CARTESIAN_POINT ( 'NONE',  ( -3.230769230769352962, -2.379036618888197285, 30.90682066428292885 ) ) ;
#41581=CARTESIAN_POINT ( 'NONE',  ( -3.230769230769229949, -2.721908614388771852, 31.22303859784724978 ) ) ;
#41582=DIRECTION ( 'NONE',  ( 0.000000000000000000, 0.9848077530122072432, -0.1736481776669354937 ) ) ;
#41584=CARTESIAN_POINT ( 'NONE',  ( 16.37662569511456567, -10.81320215134717166, 33.49497208177562868 ) ) ;
#41585=CARTESIAN_POINT ( 'NONE',  ( 3.903869409797563250, -10.06842814019191401, 34.32929386961144758 ) ) ;
#41586=AXIS2_PLACEMENT_3D ( 'NONE', #29105, #49795, #70520 ) ;
#41587=CARTESIAN_POINT ( 'NONE',  ( 14.30769230769231015, -11.16473453929635440, 33.15142922261926373 ) ) ;
#41588=ORIENTED_EDGE ( 'NONE', *, *, #81159, .T. ) ;
#41589=CARTESIAN_POINT ( 'NONE',  ( -4.153846153846152411, -2.538708090699994813, 30.37095296980875503 ) ) ;
#41590=DIRECTION ( 'NONE',  ( -0.000000000000000000, 0.8660254037844399289, -0.4999999999999980016 ) ) ;
#41591=CARTESIAN_POINT ( 'NONE',  ( 13.51540719244017730, -12.38066358083363738, 30.83685684665853444 ) ) ;
#41592=B_SPLINE_CURVE_WITH_KNOTS ( 'NONE', 3,
 ( #5836, #79722, #38732, #52232, #12594, #5396 ),
 .UNSPECIFIED., .F., .F.,
 ( 4, 2, 4 ),
 ( 0.000000000000000000, 0.0001954784845028772859, 0.0003909569690057545718 ),
 .UNSPECIFIED. ) ;
#41593=CARTESIAN_POINT ( 'NONE',  ( -13.38461538461538325, -3.513871655860378418, 32.76840700105978499 ) ) ;
#41594=CARTESIAN_POINT ( 'NONE',  ( 9.758376043310132530, -8.973038597847271092, 34.52809138561121216 ) ) ;
#41595=CARTESIAN_POINT ( 'NONE',  ( -9.692307692307691624, -2.538708090699994813, 30.37095296980875503 ) ) ;
#41597=ADVANCED_FACE ( 'NONE', ( #70296 ), #21216, .F. ) ;
#41598=AXIS2_PLACEMENT_3D ( 'NONE', #48989, #21967, #48094 ) ;
#41599=EDGE_CURVE ( 'NONE', #78839, #34884, #40798, .T. ) ;
#41600=CARTESIAN_POINT ( 'NONE',  ( 12.39621444873415257, -7.749976730030849303, 34.74374725381503737 ) ) ;
#41602=VERTEX_POINT ( 'NONE', #22110 ) ;
#41603=CARTESIAN_POINT ( 'NONE',  ( 2.307692307692309264, -11.16473453929635440, 33.15142922261926373 ) ) ;
#41604=ORIENTED_EDGE ( 'NONE', *, *, #38429, .F. ) ;
#41605=EDGE_CURVE ( 'NONE', #37210, #8934, #50509, .T. ) ;
#41606=ORIENTED_EDGE ( 'NONE', *, *, #56180, .T. ) ;
#41607=CARTESIAN_POINT ( 'NONE',  ( -8.638440328263818913, -6.369690395747422684, 34.87708834333098196 ) ) ;
#41608=EDGE_CURVE ( 'NONE', #36439, #80539, #62204, .T. ) ;
#41609=EDGE_LOOP ( 'NONE', ( #58495, #7737, #25305, #69830 ) ) ;
#41610=CARTESIAN_POINT ( 'NONE',  ( -15.23076923076922995, -6.435427911321262684, 35.78748833219616898 ) ) ;
#41612=CARTESIAN_POINT ( 'NONE',  ( 0.4615384615384611755, -8.810774026931790459, 35.74407628777942847 ) ) ;
#41613=CARTESIAN_POINT ( 'NONE',  ( -15.93083480223330817, -5.667800583137506898, 34.40243808032445827 ) ) ;
#41614=CARTESIAN_POINT ( 'NONE',  ( -5.999999999999998224, -2.499999999999998668, 29.75000000000001421 ) ) ;
#41615=DIRECTION ( 'NONE',  ( -0.000000000000000000, -0.000000000000000000, -1.000000000000000000 ) ) ;
#41616=CARTESIAN_POINT ( 'NONE',  ( 2.084766090176159992, -9.886141570436013382, 34.14413921362392301 ) ) ;
#41617=EDGE_CURVE ( 'NONE', #39653, #10726, #14467, .T. ) ;
#41618=CYLINDRICAL_SURFACE ( 'NONE', #43674, 0.2499999999999995559 ) ;
#41619=FACE_OUTER_BOUND ( 'NONE', #83631, .T. ) ;
#41620=CARTESIAN_POINT ( 'NONE',  ( -5.076923076923197442, -8.613356846316285953, 34.62446782046622218 ) ) ;
#41621=B_SPLINE_CURVE_WITH_KNOTS ( 'NONE', 3,
 ( #63203, #1519, #29003, #30744, #51432, #85705, #11371, #80283, #45146, #4616 ),
 .UNSPECIFIED., .F., .F.,
 ( 4, 2, 2, 2, 4 ),
 ( 0.0007817246256747484735, 0.0009771112852218928873, 0.001172497944769037084, 0.001367884604316181498, 0.001563271263863325912 ),
 .UNSPECIFIED. ) ;
#41622=EDGE_CURVE ( 'NONE', #84688, #14974, #84841, .T. ) ;
#41623=CARTESIAN_POINT ( 'NONE',  ( 5.933917620639864943, -11.35647404775217595, 33.31231777344666511 ) ) ;
#41624=CARTESIAN_POINT ( 'NONE',  ( -9.692307692307691624, -3.322132147404559976, 32.92929555188717927 ) ) ;
#41625=ORIENTED_EDGE ( 'NONE', *, *, #14594, .T. ) ;
#41627=DIRECTION ( 'NONE',  ( 0.000000000000000000, 0.4999999999999985567, 0.8660254037844395958 ) ) ;
#41628=CARTESIAN_POINT ( 'NONE',  ( 15.45354889974729495, -12.11081565061823717, 32.26097654155341843 ) ) ;
#41630=EDGE_CURVE ( 'NONE', #7422, #33560, #66649, .T. ) ;
#41631=CARTESIAN_POINT ( 'NONE',  ( -11.53846153846153655, -12.48256725967547354, 35.29906147534542527 ) ) ;
#41632=CARTESIAN_POINT ( 'NONE',  ( 12.39626801557768587, -9.442884908240170461, 34.35708131394840592 ) ) ;
#41633=CARTESIAN_POINT ( 'NONE',  ( -13.38461538461538325, -10.67929555188718282, 33.92786785259544047 ) ) ;
#41634=CARTESIAN_POINT ( 'NONE',  ( -2.307692307692428724, -8.656820664282941280, 34.87096338111179961 ) ) ;
#41636=ORIENTED_EDGE ( 'NONE', *, *, #26247, .T. ) ;
#41637=CARTESIAN_POINT ( 'NONE',  ( 16.02369894440793985, -2.882441371585227508, 31.66841991370172238 ) ) ;
#41638=ORIENTED_EDGE ( 'NONE', *, *, #67908, .T. ) ;
#41639=EDGE_CURVE ( 'NONE', #52419, #41861, #34422, .T. ) ;
#41640=CARTESIAN_POINT ( 'NONE',  ( 9.758376043310132530, -11.69971097300155272, 32.46337939537588113 ) ) ;
#41641=AXIS2_PLACEMENT_3D ( 'NONE', #29829, #9121, #14537 ) ;
#41642=AXIS2_PLACEMENT_3D ( 'NONE', #50063, #28934, #36985 ) ;
#41643=LINE ( 'NONE', #49283, #60007 ) ;
#41644=CARTESIAN_POINT ( 'NONE',  ( -4.153846153846152411, -4.098570777380720287, 33.41473453929634729 ) ) ;
#41645=CYLINDRICAL_SURFACE ( 'NONE', #62346, 0.2500000000000012212 ) ;
#41648=EDGE_LOOP ( 'NONE', ( #49637, #53990, #86049, #65927 ) ) ;
#41649=EDGE_CURVE ( 'NONE', #87319, #41602, #46217, .T. ) ;
#41650=B_SPLINE_CURVE_WITH_KNOTS ( 'NONE', 3,
 ( #89127, #6685, #67510, #80131, #68385, #33282, #52647, #60741, #53985, #81475 ),
 .UNSPECIFIED., .F., .F.,
 ( 4, 2, 2, 2, 4 ),
 ( 0.0007817359430256283796, 0.0009771253907249943717, 0.001172514838424360255, 0.001367904286123726356, 0.001563293733823092240 ),
 .UNSPECIFIED. ) ;
#41651=VECTOR ( 'NONE', #26327, 1000.000000000000227 ) ;
#41653=VERTEX_POINT ( 'NONE', #71170 ) ;
#41655=EDGE_CURVE ( 'NONE', #13933, #17114, #37379, .T. ) ;
#41656=CARTESIAN_POINT ( 'NONE',  ( -3.296019162543315062, -2.255955759149247619, 30.00000000000013856 ) ) ;
#41657=CARTESIAN_POINT ( 'NONE',  ( -2.307692307692305711, -9.905515769479276145, 34.41647553114623292 ) ) ;
#41658=CARTESIAN_POINT ( 'NONE',  ( -3.361460697436789768, -9.804603061927743113, 34.18744698557895845 ) ) ;
#41659=FACE_OUTER_BOUND ( 'NONE', #7301, .T. ) ;
#41660=CARTESIAN_POINT ( 'NONE',  ( 7.596153846153847589, -7.433932668274256805, 35.00000000000000711 ) ) ;
#41661=CARTESIAN_POINT ( 'NONE',  ( -15.48079245499068612, -2.588893531581426988, 31.60682220781847818 ) ) ;
#41662=ORIENTED_EDGE ( 'NONE', *, *, #76005, .T. ) ;
#41663=EDGE_CURVE ( 'NONE', #68176, #40963, #63306, .T. ) ;
#41664=ORIENTED_EDGE ( 'NONE', *, *, #71709, .F. ) ;
#41665=EDGE_LOOP ( 'NONE', ( #67937, #55423 ) ) ;
#41666=CARTESIAN_POINT ( 'NONE',  ( 8.769230769230768274, -2.517432740324522911, 35.29906147534542527 ) ) ;
#41667=EDGE_LOOP ( 'NONE', ( #5724, #43281 ) ) ;
#41668=EDGE_CURVE ( 'NONE', #34542, #65424, #48281, .T. ) ;
#41669=CARTESIAN_POINT ( 'NONE',  ( 17.07692307692295586, -11.06231777344772027, 33.60647404775119895 ) ) ;
#41670=CYLINDRICAL_SURFACE ( 'NONE', #54690, 0.2499999999999994726 ) ;
#41672=ORIENTED_EDGE ( 'NONE', *, *, #15284, .T. ) ;
#41673=VECTOR ( 'NONE', #85996, 1000.000000000000000 ) ;
#41674=ORIENTED_EDGE ( 'NONE', *, *, #49188, .T. ) ;
#41675=CARTESIAN_POINT ( 'NONE',  ( -17.74994558008654622, -2.920487667080175154, 32.31805714834172960 ) ) ;
#41676=VERTEX_POINT ( 'NONE', #38283 ) ;
#41677=FACE_BOUND ( 'NONE', #73556, .T. ) ;
#41679=CARTESIAN_POINT ( 'NONE',  ( -4.219116154402471786, -10.33852847137145048, 34.16647553114627556 ) ) ;
#41680=EDGE_LOOP ( 'NONE', ( #69610, #72715, #9212, #76031 ) ) ;
#41681=LINE ( 'NONE', #54292, #48964 ) ;
#41684=LINE ( 'NONE', #34915, #9269 ) ;
#41685=ORIENTED_EDGE ( 'NONE', *, *, #60141, .F. ) ;
#41686=CARTESIAN_POINT ( 'NONE',  ( 11.66898724022510159, -3.285477652293413264, 32.44071101563363158 ) ) ;
#41687=CARTESIAN_POINT ( 'NONE',  ( -8.769230769230768274, -12.34228464037088635, 31.77849191805839268 ) ) ;
#41688=CARTESIAN_POINT ( 'NONE',  ( -12.46153846153858247, -12.27809138561165270, 31.22303859784587132 ) ) ;
#41689=DIRECTION ( 'NONE',  ( -0.000000000000000000, -0.8660254037844399289, -0.4999999999999980016 ) ) ;
#41690=FACE_OUTER_BOUND ( 'NONE', #57593, .T. ) ;
#41691=FACE_BOUND ( 'NONE', #11922, .T. ) ;
#41692=DIRECTION ( 'NONE',  ( -0.000000000000000000, -0.9848077530122085754, -0.1736481776669273613 ) ) ;
#41693=CARTESIAN_POINT ( 'NONE',  ( -17.14300545628321260, -10.67929555188718460, 33.92786785259543336 ) ) ;
#41694=CIRCLE ( 'NONE', #57493, 0.2500000000000002220 ) ;
#41695=CARTESIAN_POINT ( 'NONE',  ( 11.78840694783958298, -12.07971442181322352, 32.31769673815850297 ) ) ;
#41696=CARTESIAN_POINT ( 'NONE',  ( 2.307692307692309264, -13.87047571288749737, 32.06866353760679544 ) ) ;
#41698=CARTESIAN_POINT ( 'NONE',  ( -10.83831157429146330, -6.459968553980841577, 34.89616026154728701 ) ) ;
#41700=ORIENTED_EDGE ( 'NONE', *, *, #69326, .T. ) ;
#41701=CARTESIAN_POINT ( 'NONE',  ( -9.019230769230768274, -7.500000000000001776, 34.75000000000000000 ) ) ;
#41702=VERTEX_POINT ( 'NONE', #58987 ) ;
#41703=AXIS2_PLACEMENT_3D ( 'NONE', #55637, #28628, #7909 ) ;
#41705=CARTESIAN_POINT ( 'NONE',  ( -15.09997742294443945, -4.118422570099827595, 33.43335022499816489 ) ) ;
#41706=EDGE_LOOP ( 'NONE', ( #55995, #62660 ) ) ;
#41707=CARTESIAN_POINT ( 'NONE',  ( 17.93391658904412012, -12.10708131394839349, 31.69288490824020244 ) ) ;
#41708=EDGE_CURVE ( 'NONE', #82006, #23503, #49407, .T. ) ;
#41709=CARTESIAN_POINT ( 'NONE',  ( -7.976301055592065481, -10.19110544564092002, 33.96427741523702792 ) ) ;
#41710=EDGE_LOOP ( 'NONE', ( #45808, #52488, #57349, #10769 ) ) ;
#41711=DIRECTION ( 'NONE',  ( -0.000000000000000000, -0.9848077530122085754, -0.1736481776669273613 ) ) ;
#41713=B_SPLINE_CURVE_WITH_KNOTS ( 'NONE', 3,
 ( #86881, #73797, #45858, #60262, #53501, #46753, #74232, #12530, #40014, #28247 ),
 .UNSPECIFIED., .F., .F.,
 ( 4, 2, 2, 2, 4 ),
 ( 0.000000000000000000, 0.0001954311564186863865, 0.0003908623128373727731, 0.0005862934692560591325, 0.0007817246256747455461 ),
 .UNSPECIFIED. ) ;
#41714=AXIS2_PLACEMENT_3D ( 'NONE', #34182, #4949, #53114 ) ;
#41715=FACE_OUTER_BOUND ( 'NONE', #78913, .T. ) ;
#41716=CARTESIAN_POINT ( 'NONE',  ( 4.826946345980720032, -4.943428324936578910, 34.04746400365624481 ) ) ;
#41717=AXIS2_PLACEMENT_3D ( 'NONE', #81886, #13849, #42228 ) ;
#41718=B_SPLINE_CURVE_WITH_KNOTS ( 'NONE', 3,
 ( #31446, #79641, #44496, #38649, #64773, #11630, #39108, #31902, #52149, #86866 ),
 .UNSPECIFIED., .F., .F.,
 ( 4, 2, 2, 2, 4 ),
 ( 0.0007817246256747459798, 0.0009771112852218896347, 0.001172497944769033181, 0.001367884604316176728, 0.001563271263863320491 ),
 .UNSPECIFIED. ) ;
#41719=CARTESIAN_POINT ( 'NONE',  ( -2.980769230769215739, -2.249999999999999112, 29.81603969181031033 ) ) ;
#41721=CARTESIAN_POINT ( 'NONE',  ( -1.384615384615383471, -3.937682226553329556, 33.60647404775216529 ) ) ;
#41722=CARTESIAN_POINT ( 'NONE',  ( 5.076923076923075762, -8.810774026931790459, 35.74407628777942847 ) ) ;
#41727=CARTESIAN_POINT ( 'NONE',  ( -6.130147969731693181, -3.625366637846544560, 33.29286588640298561 ) ) ;
#41728=VERTEX_POINT ( 'NONE', #33310 ) ;
#41729=ADVANCED_FACE ( 'NONE', ( #52674 ), #12152, .F. ) ;
#41730=DIRECTION ( 'NONE',  ( -0.000000000000000000, -0.8660254037844397068, -0.4999999999999978906 ) ) ;
#41732=CARTESIAN_POINT ( 'NONE',  ( -15.90379173393269951, -12.41089969410671223, 31.60739465890703670 ) ) ;
#41733=CYLINDRICAL_SURFACE ( 'NONE', #18235, 0.2500000000000009437 ) ;
#41734=VERTEX_POINT ( 'NONE', #18902 ) ;
#41735=CARTESIAN_POINT ( 'NONE',  ( -18.00000000000000000, -2.721908614388771852, 31.22303859784724978 ) ) ;
#41736=CARTESIAN_POINT ( 'NONE',  ( 16.37662582282421653, -2.612705202774696200, 31.66806509827799943 ) ) ;
#41737=DIRECTION ( 'NONE',  ( 1.000000000000000000, 0.000000000000000000, 0.000000000000000000 ) ) ;
#41738=ORIENTED_EDGE ( 'NONE', *, *, #15634, .F. ) ;
#41739=DIRECTION ( 'NONE',  ( 1.000000000000000000, 0.000000000000000000, 0.000000000000000000 ) ) ;
#41740=CARTESIAN_POINT ( 'NONE',  ( -1.384615384615505151, -4.481592998941358097, 33.73612834414048933 ) ) ;
#41741=CARTESIAN_POINT ( 'NONE',  ( 7.173131342990377135, -12.01375889529407281, 32.43194544308182969 ) ) ;
#41742=ADVANCED_FACE ( 'NONE', ( #67535 ), #25213, .T. ) ;
#41743=CARTESIAN_POINT ( 'NONE',  ( 3.007842271862382066, -2.523278758544489353, 31.42238647778637528 ) ) ;
#41744=CARTESIAN_POINT ( 'NONE',  ( -9.692307692307812417, -6.879047030192662504, 34.71129190930017927 ) ) ;
#41746=EDGE_LOOP ( 'NONE', ( #3813, #15183, #43069, #47981 ) ) ;
#41747=VECTOR ( 'NONE', #25750, 1000.000000000000227 ) ;
#41748=B_SPLINE_CURVE_WITH_KNOTS ( 'NONE', 3,
 ( #84410, #2407, #14166, #36220, #63674, #83972, #62339, #14610, #41640, #1981 ),
 .UNSPECIFIED., .F., .F.,
 ( 4, 2, 2, 2, 4 ),
 ( 0.0007817359430256388964, 0.0009771253907250073822, 0.001172514838424375868, 0.001367904286123744571, 0.001563293733823113056 ),
 .UNSPECIFIED. ) ;
#41749=EDGE_CURVE ( 'NONE', #72951, #84941, #41923, .T. ) ;
#41752=DIRECTION ( 'NONE',  ( -0.000000000000000000, -0.3420201433256694346, -0.9396926207859080948 ) ) ;
#41753=CARTESIAN_POINT ( 'NONE',  ( -6.700065571464073777, -4.187068189119697692, 33.49521262558774026 ) ) ;
#41754=ADVANCED_FACE ( 'NONE', ( #13030 ), #60322, .F. ) ;
#41755=B_SPLINE_CURVE_WITH_KNOTS ( 'NONE', 3,
 ( #54691, #76298, #88959, #68656, #34428, #75857, #61892, #74983, #62769, #40756 ),
 .UNSPECIFIED., .F., .F.,
 ( 4, 2, 2, 2, 4 ),
 ( 0.0007817246256747453293, 0.0009771112852218889842, 0.001172497944769032531, 0.001367884604316176294, 0.001563271263863319840 ),
 .UNSPECIFIED. ) ;
#41756=CYLINDRICAL_SURFACE ( 'NONE', #81021, 0.2499999999999995559 ) ;
#41758=VERTEX_POINT ( 'NONE', #33746 ) ;
#41759=CARTESIAN_POINT ( 'NONE',  ( 17.32697749683652688, -11.47946981652013498, 33.17500667209846910 ) ) ;
#41760=EDGE_LOOP ( 'NONE', ( #2037, #3574 ) ) ;
#41761=EDGE_LOOP ( 'NONE', ( #56429, #74607 ) ) ;
#41762=EDGE_CURVE ( 'NONE', #83278, #82873, #61201, .T. ) ;
#41763=ORIENTED_EDGE ( 'NONE', *, *, #819, .F. ) ;
#41764=CARTESIAN_POINT ( 'NONE',  ( -7.911424292114620727, -5.219633306516282545, 34.19971097300152962 ) ) ;
#41765=ORIENTED_EDGE ( 'NONE', *, *, #69096, .T. ) ;
#41766=CARTESIAN_POINT ( 'NONE',  ( 4.153846153846032507, -6.026961402154118908, 34.52809138561165270 ) ) ;
#41767=CARTESIAN_POINT ( 'NONE',  ( 5.999999999999878320, -12.70778746994576025, 30.41441678777401236 ) ) ;
#41769=CARTESIAN_POINT ( 'NONE',  ( 2.307692307692615685, -2.506253911140615021, 30.00000000000323297 ) ) ;
#41770=DIRECTION ( 'NONE',  ( -0.000000000000000000, 0.1736481776669307198, -0.9848077530122080203 ) ) ;
#41771=ORIENTED_EDGE ( 'NONE', *, *, #44662, .T. ) ;
#41772=EDGE_CURVE ( 'NONE', #15837, #83400, #63447, .T. ) ;
#41773=EDGE_LOOP ( 'NONE', ( #29154, #73599 ) ) ;
#41774=ORIENTED_EDGE ( 'NONE', *, *, #53015, .F. ) ;
#41775=LINE ( 'NONE', #21040, #83565 ) ;
#41776=CARTESIAN_POINT ( 'NONE',  ( -10.61538461538461320, -11.11383981884818262, 36.00935417666054406 ) ) ;
#41777=ORIENTED_EDGE ( 'NONE', *, *, #48048, .F. ) ;
#41779=CARTESIAN_POINT ( 'NONE',  ( -11.47239420511146513, -12.62096338111211757, 30.90682066428152908 ) ) ;
#41781=EDGE_CURVE ( 'NONE', #32578, #52323, #81946, .T. ) ;
#41782=CARTESIAN_POINT ( 'NONE',  ( -14.53061852520844965, -2.554751324335734708, 30.48935550225260727 ) ) ;
#41783=ORIENTED_EDGE ( 'NONE', *, *, #970, .F. ) ;
#41784=B_SPLINE_CURVE_WITH_KNOTS ( 'NONE', 3,
 ( #19984, #20870, #39827, #13674, #47450, #32611, #41153, #5590, #74945, #34385 ),
 .UNSPECIFIED., .F., .F.,
 ( 4, 2, 2, 2, 4 ),
 ( 0.000000000000000000, 0.0001954339857564078538, 0.0003908679715128157077, 0.0005863019572692235344, 0.0007817359430256314154 ),
 .UNSPECIFIED. ) ;
#41785=B_SPLINE_CURVE_WITH_KNOTS ( 'NONE', 3,
 ( #49342, #36711, #43467, #707, #21424, #83132, #76362, #22310, #83589, #42152 ),
 .UNSPECIFIED., .F., .F.,
 ( 4, 2, 2, 2, 4 ),
 ( 0.000000000000000000, 0.0001954339857564070678, 0.0003908679715128141356, 0.0005863019572692211492, 0.0007817359430256282712 ),
 .UNSPECIFIED. ) ;
#41786=CARTESIAN_POINT ( 'NONE',  ( -17.77722045873159473, -2.600157965045223563, 30.74683119005207033 ) ) ;
#41788=ORIENTED_EDGE ( 'NONE', *, *, #81451, .T. ) ;
#41789=FACE_BOUND ( 'NONE', #18038, .T. ) ;
#41790=ADVANCED_FACE ( 'NONE', ( #20235 ), #47698, .F. ) ;
#41791=B_SPLINE_CURVE_WITH_KNOTS ( 'NONE', 3,
 ( #40301, #6070, #79949, #18249, #19134, #26334, #67326, #4738, #33542, #52465 ),
 .UNSPECIFIED., .F., .F.,
 ( 4, 2, 2, 2, 4 ),
 ( 0.000000000000000000, 0.0001954311564186861155, 0.0003908623128373722310, 0.0005862934692560583735, 0.0007817246256747444619 ),
 .UNSPECIFIED. ) ;
#41792=CARTESIAN_POINT ( 'NONE',  ( 10.86533013373275658, -10.05730279482229683, 34.04704008940765902 ) ) ;
#41793=LINE ( 'NONE', #69253, #2509 ) ;
#41794=CARTESIAN_POINT ( 'NONE',  ( 3.453780582382082631, -9.086983370893047862, 34.49168942202179267 ) ) ;
#41795=CARTESIAN_POINT ( 'NONE',  ( 13.38461538461538680, -11.91647553114624181, 32.58852847137148245 ) ) ;
#41796=FACE_OUTER_BOUND ( 'NONE', #7423, .T. ) ;
#41797=CARTESIAN_POINT ( 'NONE',  ( -4.088590582570128973, -2.892918686051625166, 31.69288490824025928 ) ) ;
#41798=CARTESIAN_POINT ( 'NONE',  ( -16.15384615384615330, -8.973038597847269315, 34.52809138561121927 ) ) ;
#41799=EDGE_LOOP ( 'NONE', ( #78403, #25448, #29674, #64590 ) ) ;
#41800=CARTESIAN_POINT ( 'NONE',  ( -18.25000000000000000, -7.500000000000001776, 34.75000000000000000 ) ) ;
#41801=CARTESIAN_POINT ( 'NONE',  ( 13.31885858210107898, -7.249945686854186278, 34.74374336980224598 ) ) ;
#41802=B_SPLINE_CURVE_WITH_KNOTS ( 'NONE', 3,
 ( #84152, #22428, #43148, #50328, #44019, #77372, #21541, #77809, #76494, #70618 ),
 .UNSPECIFIED., .F., .F.,
 ( 4, 2, 2, 2, 4 ),
 ( 0.0007817359430256317406, 0.0009771253907249982749, 0.001172514838424365026, 0.001367904286123731560, 0.001563293733823098094 ),
 .UNSPECIFIED. ) ;
#41806=VERTEX_POINT ( 'NONE', #32414 ) ;
#41807=CARTESIAN_POINT ( 'NONE',  ( 17.77707378248384629, -5.667676309546437530, 34.40238873228292249 ) ) ;
#41808=FACE_OUTER_BOUND ( 'NONE', #60805, .T. ) ;
#41809=FACE_BOUND ( 'NONE', #80558, .T. ) ;
#41812=CARTESIAN_POINT ( 'NONE',  ( 5.750000000000002665, -7.500000000000001776, 35.00000000000000000 ) ) ;
#41813=CARTESIAN_POINT ( 'NONE',  ( 12.39545608217832395, -12.34228464037088280, 31.77849191805838558 ) ) ;
#41815=CARTESIAN_POINT ( 'NONE',  ( 15.48076923076923173, -2.499999999999998668, 29.75000000000000355 ) ) ;
#41818=ORIENTED_EDGE ( 'NONE', *, *, #7090, .T. ) ;
#41819=ORIENTED_EDGE ( 'NONE', *, *, #67104, .F. ) ;
#41820=CARTESIAN_POINT ( 'NONE',  ( -10.61538461538461320, -1.466349020453238561, 30.81389545987213907 ) ) ;
#41821=CARTESIAN_POINT ( 'NONE',  ( 13.38461538461538680, -12.78798330534102945, 29.74999999999997868 ) ) ;
#41822=CARTESIAN_POINT ( 'NONE',  ( 1.634669804528839254, -9.233818618650603938, 34.70587769442853698 ) ) ;
#41823=CARTESIAN_POINT ( 'NONE',  ( -16.85391172531022619, -11.24521262558773493, 33.06293181088029343 ) ) ;
#41824=CARTESIAN_POINT ( 'NONE',  ( -4.088591014333315066, -3.083524468853784839, 32.58852847137153930 ) ) ;
#41826=DIRECTION ( 'NONE',  ( -0.000000000000000000, -0.9848077530122085754, -0.1736481776669273613 ) ) ;
#41828=CARTESIAN_POINT ( 'NONE',  ( -17.32689980786543060, -4.943428324936578910, 34.04746400365624481 ) ) ;
#41829=CARTESIAN_POINT ( 'NONE',  ( 7.846153846153846700, -5.471508081941601098, 34.59228464037088457 ) ) ;
#41830=CARTESIAN_POINT ( 'NONE',  ( 9.692307692307695177, -12.78798330534102767, 29.49999999999997868 ) ) ;
#41832=B_SPLINE_CURVE_WITH_KNOTS ( 'NONE', 3,
 ( #47704, #62104, #48580, #34638, #69314, #14817, #55344, #1286, #68419, #67989 ),
 .UNSPECIFIED., .F., .F.,
 ( 4, 2, 2, 2, 4 ),
 ( 0.000000000000000000, 0.0001954339857564083417, 0.0003908679715128166835, 0.0005863019572692250523, 0.0007817359430256333669 ),
 .UNSPECIFIED. ) ;
#41833=CARTESIAN_POINT ( 'NONE',  ( 9.942253210655838558, -11.37275283266504111, 32.91324779482534524 ) ) ;
#41834=CARTESIAN_POINT ( 'NONE',  ( 12.68431813051652668, -2.353885683473779800, 30.79025554430704403 ) ) ;
#41836=CARTESIAN_POINT ( 'NONE',  ( 12.52679403281448423, -2.892918686051625166, 31.69288490824026638 ) ) ;
#41837=ORIENTED_EDGE ( 'NONE', *, *, #10389, .F. ) ;
#41838=CARTESIAN_POINT ( 'NONE',  ( -14.55771554498527642, -3.711651800289232028, 33.01384336483936011 ) ) ;
#41839=CARTESIAN_POINT ( 'NONE',  ( 10.86533002476265786, -5.766571408460171355, 34.70601412856602508 ) ) ;
#41841=AXIS2_PLACEMENT_3D ( 'NONE', #38847, #25772, #79385 ) ;
#41842=CIRCLE ( 'NONE', #79246, 0.2500000000000002220 ) ;
#41843=CARTESIAN_POINT ( 'NONE',  ( -0.4615384615384611200, -10.67929555188718282, 33.92786785259544047 ) ) ;
#41844=CARTESIAN_POINT ( 'NONE',  ( 16.94623247381277054, -11.37499894934982514, 33.29245874905763003 ) ) ;
#41845=ORIENTED_EDGE ( 'NONE', *, *, #83582, .T. ) ;
#41846=CYLINDRICAL_SURFACE ( 'NONE', #48516, 0.2500000000000002220 ) ;
#41850=FACE_OUTER_BOUND ( 'NONE', #24482, .T. ) ;
#41851=VERTEX_POINT ( 'NONE', #62966 ) ;
#41852=DIRECTION ( 'NONE',  ( -0.000000000000000000, 0.7660444431189791237, -0.6427876096865379196 ) ) ;
#41853=CIRCLE ( 'NONE', #184, 0.2500000000000002220 ) ;
#41854=CARTESIAN_POINT ( 'NONE',  ( 10.74591005361826035, -11.04252011169590020, 33.62494198852677130 ) ) ;
#41855=DIRECTION ( 'NONE',  ( -1.000000000000000000, 0.000000000000000000, 0.000000000000000000 ) ) ;
#41856=ORIENTED_EDGE ( 'NONE', *, *, #59911, .T. ) ;
#41857=CARTESIAN_POINT ( 'NONE',  ( 17.07692307692307665, -11.16473453929635440, 33.15142922261926373 ) ) ;
#41858=CARTESIAN_POINT ( 'NONE',  ( 2.557637717070351258, -8.476813868363244353, 34.90874843262270133 ) ) ;
#41859=CARTESIAN_POINT ( 'NONE',  ( -15.23076923076922995, -12.37446782046654192, 30.86335684631486131 ) ) ;
#41860=ORIENTED_EDGE ( 'NONE', *, *, #21133, .T. ) ;
#41861=VERTEX_POINT ( 'NONE', #69742 ) ;
#41862=CARTESIAN_POINT ( 'NONE',  ( 6.249945518348142492, -6.696923467548660192, 34.68552623307873972 ) ) ;
#41863=EDGE_LOOP ( 'NONE', ( #35330, #80892 ) ) ;
#41864=CARTESIAN_POINT ( 'NONE',  ( -15.00798956179115962, -4.226511098958373402, 33.85474049983370293 ) ) ;
#41865=CARTESIAN_POINT ( 'NONE',  ( 15.48071464014727283, -12.68172785388650681, 30.59649109432439218 ) ) ;
#41866=CARTESIAN_POINT ( 'NONE',  ( 13.38461538461526423, -3.643525952248795718, 33.31231777344771672 ) ) ;
#41867=CYLINDRICAL_SURFACE ( 'NONE', #27530, 0.2499999999999986955 ) ;
#41868=DIRECTION ( 'NONE',  ( -0.000000000000000000, 0.6427876096865404731, -0.7660444431189770143 ) ) ;
#41869=CARTESIAN_POINT ( 'NONE',  ( -2.557692307692330136, -2.249999999999999112, 29.81609741502488120 ) ) ;
#41870=CYLINDRICAL_SURFACE ( 'NONE', #55014, 0.2500000000000009437 ) ;
#41871=B_SPLINE_CURVE_WITH_KNOTS ( 'NONE', 3,
 ( #38696, #32387, #37802, #59853, #25627, #87350, #80588, #3565, #12126, #3120 ),
 .UNSPECIFIED., .F., .F.,
 ( 4, 2, 2, 2, 4 ),
 ( 0.000000000000000000, 0.0001954339857564071762, 0.0003908679715128143524, 0.0005863019572692215828, 0.0007817359430256287049 ),
 .UNSPECIFIED. ) ;
#41872=VECTOR ( 'NONE', #73087, 1000.000000000000000 ) ;
#41873=ORIENTED_EDGE ( 'NONE', *, *, #14731, .T. ) ;
#41875=ORIENTED_EDGE ( 'NONE', *, *, #31558, .T. ) ;
#41876=CARTESIAN_POINT ( 'NONE',  ( -17.32689980786543060, -9.943427161483782584, 34.11278801902876978 ) ) ;
#41877=ORIENTED_EDGE ( 'NONE', *, *, #29377, .F. ) ;
#41879=CARTESIAN_POINT ( 'NONE',  ( 16.94677510719138169, -2.373036134822905208, 30.88089517874952250 ) ) ;
#41880=VERTEX_POINT ( 'NONE', #20668 ) ;
#41881=DIRECTION ( 'NONE',  ( -0.000000000000000000, 0.8660254037844399289, -0.4999999999999980016 ) ) ;
#41882=CARTESIAN_POINT ( 'NONE',  ( 6.223012844093395834, -10.01129605718032778, 34.36064277460058491 ) ) ;
#41883=VERTEX_POINT ( 'NONE', #56230 ) ;
#41885=ORIENTED_EDGE ( 'NONE', *, *, #83385, .T. ) ;
#41886=ORIENTED_EDGE ( 'NONE', *, *, #43754, .T. ) ;
#41887=CARTESIAN_POINT ( 'NONE',  ( -12.68446542044531178, -3.395401636524185474, 33.02366814457250399 ) ) ;
#41888=EDGE_CURVE ( 'NONE', #23097, #65576, #54829, .T. ) ;
#41889=EDGE_CURVE ( 'NONE', #6007, #17599, #83718, .T. ) ;
#41890=VERTEX_POINT ( 'NONE', #14810 ) ;
#41891=AXIS2_PLACEMENT_3D ( 'NONE', #87940, #45576, #67194 ) ;
#41892=CARTESIAN_POINT ( 'NONE',  ( -7.846153846153844924, -13.04860791097971706, 34.73218667398347037 ) ) ;
#41894=FACE_BOUND ( 'NONE', #22363, .T. ) ;
#41895=CYLINDRICAL_SURFACE ( 'NONE', #62896, 0.2499999999999986955 ) ;
#41896=CARTESIAN_POINT ( 'NONE',  ( -6.673131404728779970, -12.22109172314383052, 31.39792113162168263 ) ) ;
#41898=AXIS2_PLACEMENT_3D ( 'NONE', #57720, #14518, #55942 ) ;
#41900=CARTESIAN_POINT ( 'NONE',  ( -13.38461538461538325, -12.37446782046654192, 30.86335684631486131 ) ) ;
#41902=CARTESIAN_POINT ( 'NONE',  ( -12.46153846153846168, -2.292212530054420494, 30.41441678777542634 ) ) ;
#41904=CARTESIAN_POINT ( 'NONE',  ( 10.61538461538449596, -10.21337939537710326, 33.94971097300076224 ) ) ;
#41905=VERTEX_POINT ( 'NONE', #22001 ) ;
#41906=EDGE_LOOP ( 'NONE', ( #69580, #85616, #2086, #80820 ) ) ;
#41908=CARTESIAN_POINT ( 'NONE',  ( -5.999999999999998224, -11.11383981884818262, 36.00935417666054406 ) ) ;
#41909=CARTESIAN_POINT ( 'NONE',  ( 15.10062202133100939, -12.27039167877662251, 31.24851455888617835 ) ) ;
#41910=CARTESIAN_POINT ( 'NONE',  ( -11.60373198442231590, -11.94971097300153140, 32.03036669348370680 ) ) ;
#41911=CARTESIAN_POINT ( 'NONE',  ( -17.01166793741023042, -10.33852847137154107, 34.16647553114620450 ) ) ;
#41912=CARTESIAN_POINT ( 'NONE',  ( 15.36156103859402045, -3.530189275343204702, 32.79018710029569661 ) ) ;
#41913=CARTESIAN_POINT ( 'NONE',  ( -12.33074802057151409, -4.684288915650983043, 34.18129842949671371 ) ) ;
#41914=VERTEX_POINT ( 'NONE', #8936 ) ;
#41915=CARTESIAN_POINT ( 'NONE',  ( -18.22348494372394967, -5.912607949931402374, 34.49155766932282319 ) ) ;
#41916=CARTESIAN_POINT ( 'NONE',  ( 1.515407192440173745, -12.11778462344221019, 31.66786338562085135 ) ) ;
#41917=DIRECTION ( 'NONE',  ( -0.000000000000000000, 0.9396926207859093161, -0.3420201433256663259 ) ) ;
#41918=DIRECTION ( 'NONE',  ( -0.000000000000000000, -0.6427876096865404731, -0.7660444431189770143 ) ) ;
#41919=FACE_OUTER_BOUND ( 'NONE', #23940, .T. ) ;
#41920=VERTEX_POINT ( 'NONE', #62098 ) ;
#41921=ORIENTED_EDGE ( 'NONE', *, *, #72745, .F. ) ;
#41923=B_SPLINE_CURVE_WITH_KNOTS ( 'NONE', 3,
 ( #46372, #67092, #54450, #60767, #40081, #87376, #6710, #75184, #5393, #32858 ),
 .UNSPECIFIED., .F., .F.,
 ( 4, 2, 2, 2, 4 ),
 ( 0.000000000000000000, 0.0001954311564186870371, 0.0003908623128373740741, 0.0005862934692560610840, 0.0007817246256747481482 ),
 .UNSPECIFIED. ) ;
#41924=CARTESIAN_POINT ( 'NONE',  ( -7.053768389744481837, -8.147922237126337563, 34.70805685702651999 ) ) ;
#41925=ORIENTED_EDGE ( 'NONE', *, *, #315, .F. ) ;
#41926=CARTESIAN_POINT ( 'NONE',  ( -9.469294848214296678, -10.01129605718032600, 34.36064277460058491 ) ) ;
#41927=DIRECTION ( 'NONE',  ( -1.000000000000000000, -0.000000000000000000, -0.000000000000000000 ) ) ;
#41928=CARTESIAN_POINT ( 'NONE',  ( -5.999999999999998224, -8.810774026931790459, 35.74407628777942847 ) ) ;
#41930=CARTESIAN_POINT ( 'NONE',  ( 12.21156173059610772, -9.943427161483782584, 34.11278801902876978 ) ) ;
#41931=ORIENTED_EDGE ( 'NONE', *, *, #9653, .F. ) ;
#41932=CARTESIAN_POINT ( 'NONE',  ( -11.78846153846153832, -7.500000000000001776, 35.00000000000000000 ) ) ;
#41933=CARTESIAN_POINT ( 'NONE',  ( -12.39547011053602432, -11.69971097300155272, 32.46337939537588113 ) ) ;
#41934=ORIENTED_EDGE ( 'NONE', *, *, #79069, .F. ) ;
#41935=FACE_OUTER_BOUND ( 'NONE', #72314, .T. ) ;
#41936=CARTESIAN_POINT ( 'NONE',  ( -10.61538461538461320, -3.513871655860378418, 32.76840700105978499 ) ) ;
#41937=CARTESIAN_POINT ( 'NONE',  ( -10.61538461538461320, -9.058645607665452459, 34.76329471203371924 ) ) ;
#41939=CARTESIAN_POINT ( 'NONE',  ( -15.93041975493136597, -7.630147987733843173, 34.99859428049665411 ) ) ;
#41940=CARTESIAN_POINT ( 'NONE',  ( 2.373759641042383794, -2.486705287966280320, 31.30864560766543647 ) ) ;
#41941=CARTESIAN_POINT ( 'NONE',  ( -39.05038313613820122, -2.249999999999998668, 29.75000000000000355 ) ) ;
#41942=CARTESIAN_POINT ( 'NONE',  ( -12.59222992820602371, -12.38065189839062263, 30.83690757178629482 ) ) ;
#41943=VECTOR ( 'NONE', #32859, 1000.000000000000114 ) ;
#41945=ORIENTED_EDGE ( 'NONE', *, *, #84756, .F. ) ;
#41946=CARTESIAN_POINT ( 'NONE',  ( -4.153846153846152411, -13.57706302396349152, 30.56769352161908060 ) ) ;
#41947=B_SPLINE_CURVE_WITH_KNOTS ( 'NONE', 3,
 ( #82058, #20354, #47815, #75294, #13584, #68526, #42840, #30963, #37729, #3494 ),
 .UNSPECIFIED., .F., .F.,
 ( 4, 2, 2, 2, 4 ),
 ( 0.0007817246256747459798, 0.0009771112852218887673, 0.001172497944769031663, 0.001367884604316174559, 0.001563271263863317455 ),
 .UNSPECIFIED. ) ;
#41948=CARTESIAN_POINT ( 'NONE',  ( 1.318533005255250856, -9.058645607665454236, 34.76329471203372634 ) ) ;
#41949=DIRECTION ( 'NONE',  ( 0.000000000000000000, 0.9848077530122072432, 0.1736481776669354937 ) ) ;
#41950=CARTESIAN_POINT ( 'NONE',  ( 9.442330948259101575, -6.524016743844655686, 34.90889640711025521 ) ) ;
#41953=CARTESIAN_POINT ( 'NONE',  ( -2.438383774359866418, -3.062553014421049991, 32.05460306192774311 ) ) ;
#41954=ADVANCED_FACE ( 'NONE', ( #29217 ), #49475, .F. ) ;
#41955=CARTESIAN_POINT ( 'NONE',  ( -1.384615384615505151, -6.879047030192662504, 34.71129190930017927 ) ) ;
#41956=CARTESIAN_POINT ( 'NONE',  ( 8.769230769230768274, -5.557115091759785130, 34.35708131394839171 ) ) ;
#41957=ADVANCED_FACE ( 'NONE', ( #76053 ), #15251, .F. ) ;
#41958=VERTEX_POINT ( 'NONE', #69307 ) ;
#41959=CARTESIAN_POINT ( 'NONE',  ( 6.065255571276025215, -6.026961402152789304, 34.52809138561124769 ) ) ;
#41960=B_SPLINE_CURVE_WITH_KNOTS ( 'NONE', 3,
 ( #41866, #76975, #71089, #49050, #43620, #56257, #36432, #7635, #64322, #70215 ),
 .UNSPECIFIED., .F., .F.,
 ( 4, 2, 2, 2, 4 ),
 ( 0.0007817246256747434861, 0.0009771112852218861652, 0.001172497944769028844, 0.001367884604316171740, 0.001563271263863314419 ),
 .UNSPECIFIED. ) ;
#41961=CARTESIAN_POINT ( 'NONE',  ( -11.53846153846165912, -2.892918686052166066, 31.69288490824153470 ) ) ;
#41963=B_SPLINE_CURVE_WITH_KNOTS ( 'NONE', 3,
 ( #43671, #1804, #14892, #57632, #85115, #70267, #9017, #28849, #43238, #36047 ),
 .UNSPECIFIED., .F., .F.,
 ( 4, 2, 2, 2, 4 ),
 ( 0.0007817246256747450040, 0.0009771112852218881168, 0.001172497944769031230, 0.001367884604316174342, 0.001563271263863317455 ),
 .UNSPECIFIED. ) ;
#41964=EDGE_LOOP ( 'NONE', ( #19382, #10965 ) ) ;
#41965=CARTESIAN_POINT ( 'NONE',  ( -8.519230769229348965, -7.500000000000154543, 35.00000000000007105 ) ) ;
#41966=B_SPLINE_CURVE_WITH_KNOTS ( 'NONE', 3,
 ( #14680, #56105, #61967, #62840, #83599, #276, #8368, #27742, #1159, #61083 ),
 .UNSPECIFIED., .F., .F.,
 ( 4, 2, 2, 2, 4 ),
 ( 0.0007817359430256293554, 0.0009771253907249941549, 0.001172514838424358954, 0.001367904286123723537, 0.001563293733823095276 ),
 .UNSPECIFIED. ) ;
#41968=EDGE_CURVE ( 'NONE', #52756, #60044, #59135, .T. ) ;
#41971=CARTESIAN_POINT ( 'NONE',  ( 4.946232473812766983, -5.496505350115500121, 34.60290016733514307 ) ) ;
#41973=EDGE_CURVE ( 'NONE', #45581, #38569, #65516, .T. ) ;
#41974=DIRECTION ( 'NONE',  ( -0.000000000000000000, 0.9848077530122086864, -0.1736481776669273891 ) ) ;
#41975=FACE_OUTER_BOUND ( 'NONE', #37634, .T. ) ;
#41976=CARTESIAN_POINT ( 'NONE',  ( 1.253923917947830757, -4.118384482072085184, 33.43331474514187107 ) ) ;
#41978=CARTESIAN_POINT ( 'NONE',  ( 1.384615384615264011, -6.835583212225970762, 34.95778746994575670 ) ) ;
#41979=DIRECTION ( 'NONE',  ( -0.000000000000000000, 0.9848077530122086864, -0.1736481776669273891 ) ) ;
#41980=VERTEX_POINT ( 'NONE', #82828 ) ;
#41981=ORIENTED_EDGE ( 'NONE', *, *, #79701, .T. ) ;
#41983=FACE_BOUND ( 'NONE', #23864, .T. ) ;
#41984=ORIENTED_EDGE ( 'NONE', *, *, #82463, .T. ) ;
#41985=CARTESIAN_POINT ( 'NONE',  ( 3.230769230769231726, -1.509761064869970415, 31.06009739812519044 ) ) ;
#41986=DIRECTION ( 'NONE',  ( 0.000000000000000000, 0.000000000000000000, -1.000000000000000000 ) ) ;
#41987=CARTESIAN_POINT ( 'NONE',  ( 3.230769230769231726, -1.044019251281081972, 31.83374038241031911 ) ) ;
#41988=CARTESIAN_POINT ( 'NONE',  ( 7.146088274689774700, -9.886259254753566594, 34.14407573483972413 ) ) ;
#41989=B_SPLINE_CURVE_WITH_KNOTS ( 'NONE', 3,
 ( #63621, #1923, #27622, #48330, #1039, #55533, #21302, #56861, #15449, #14553 ),
 .UNSPECIFIED., .F., .F.,
 ( 4, 2, 2, 2, 4 ),
 ( 0.0007817246256747459798, 0.0009771112852218896347, 0.001172497944769033181, 0.001367884604316176728, 0.001563271263863320491 ),
 .UNSPECIFIED. ) ;
#41990=VERTEX_POINT ( 'NONE', #21100 ) ;
#41991=ORIENTED_EDGE ( 'NONE', *, *, #17818, .T. ) ;
#41993=AXIS2_PLACEMENT_3D ( 'NONE', #75799, #82581, #13222 ) ;
#41995=ORIENTED_EDGE ( 'NONE', *, *, #86924, .F. ) ;
#41996=EDGE_CURVE ( 'NONE', #84941, #57639, #14353, .T. ) ;
#41997=CARTESIAN_POINT ( 'NONE',  ( -6.066083410955879884, -12.37446782046654192, 30.86335684631486487 ) ) ;
#41998=EDGE_CURVE ( 'NONE', #29327, #54013, #11141, .T. ) ;
#41999=CARTESIAN_POINT ( 'NONE',  ( -11.76194646302587010, -5.827078755546623690, 34.72654668319379567 ) ) ;
#42000=CARTESIAN_POINT ( 'NONE',  ( -18.13014720943822056, -11.47017969459903597, 32.78971311882035167 ) ) ;
#42001=ORIENTED_EDGE ( 'NONE', *, *, #33892, .T. ) ;
#42002=CARTESIAN_POINT ( 'NONE',  ( 8.992010310499175318, -9.332535724633409302, 34.40230450496446934 ) ) ;
#42004=DIRECTION ( 'NONE',  ( -0.000000000000000000, 0.7660444431189791237, -0.6427876096865379196 ) ) ;
#42005=ADVANCED_FACE ( 'NONE', ( #24654 ), #85472, .F. ) ;
#42006=CARTESIAN_POINT ( 'NONE',  ( 14.55774661933062397, -6.567000820036036579, 34.66262288849541306 ) ) ;
#42007=CARTESIAN_POINT ( 'NONE',  ( -8.638440328263820689, -2.845873456487965747, 32.17976146951972538 ) ) ;
#42008=EDGE_LOOP ( 'NONE', ( #55421, #65918 ) ) ;
#42010=ORIENTED_EDGE ( 'NONE', *, *, #18714, .T. ) ;
#42011=CARTESIAN_POINT ( 'NONE',  ( 3.007889714031644957, -7.630690623152302621, 34.99857592706774057 ) ) ;
#42012=CARTESIAN_POINT ( 'NONE',  ( -1.634592128663973076, -2.544273027872574922, 31.48422191005632342 ) ) ;
#42013=CARTESIAN_POINT ( 'NONE',  ( -16.15384615384615330, -6.386643153685126251, 34.62446782046654192 ) ) ;
#42014=CARTESIAN_POINT ( 'NONE',  ( -17.86920955903304886, -5.496552790871120031, 34.60292014791297532 ) ) ;
#42015=CARTESIAN_POINT ( 'NONE',  ( -6.673131404728781746, -3.712312575010499494, 33.01462480002815170 ) ) ;
#42016=FACE_BOUND ( 'NONE', #19969, .T. ) ;
#42017=CARTESIAN_POINT ( 'NONE',  ( 16.21991450484859243, -3.050289026998446840, 32.03036669348366416 ) ) ;
#42019=CARTESIAN_POINT ( 'NONE',  ( -8.096153846153844924, -7.500000000000001776, 35.00000000000000000 ) ) ;
#42020=DIRECTION ( 'NONE',  ( -0.000000000000000000, -0.1736481776669307198, -0.9848077530122080203 ) ) ;
#42022=CARTESIAN_POINT ( 'NONE',  ( 3.361294669002873992, -11.66157788607254275, 32.95092075102925833 ) ) ;
#42024=CARTESIAN_POINT ( 'NONE',  ( 10.61538461538461675, -8.973038597847269315, 34.52809138561121927 ) ) ;
#42026=FACE_BOUND ( 'NONE', #7519, .T. ) ;
#42028=TOROIDAL_SURFACE ( 'NONE', #60718, 3.250000000000001332, 2.000000000000000000 ) ;
#42029=VECTOR ( 'NONE', #1653, 1000.000000000000227 ) ;
#42030=CARTESIAN_POINT ( 'NONE',  ( 17.99999999999987566, -12.70778746994576025, 30.41441678777401236 ) ) ;
#42033=CARTESIAN_POINT ( 'NONE',  ( 5.076923076923075762, -3.050289026998446396, 32.03036669348365706 ) ) ;
#42034=CARTESIAN_POINT ( 'NONE',  ( 15.48082365068268018, -2.318338780012835443, 30.59689888758630261 ) ) ;
#42035=DIRECTION ( 'NONE',  ( -0.000000000000000000, -0.6427876096865404731, -0.7660444431189771253 ) ) ;
#42036=CARTESIAN_POINT ( 'NONE',  ( 5.076923076923075762, -3.669653830205710676, 35.88435417666054406 ) ) ;
#42037=ORIENTED_EDGE ( 'NONE', *, *, #41655, .T. ) ;
#42038=AXIS2_PLACEMENT_3D ( 'NONE', #4397, #31881, #86847 ) ;
#42039=CARTESIAN_POINT ( 'NONE',  ( -5.010855743573000787, -4.661471528628508665, 34.16647553114624003 ) ) ;
#42040=ORIENTED_EDGE ( 'NONE', *, *, #18171, .F. ) ;
#42041=CARTESIAN_POINT ( 'NONE',  ( -8.899922235898330314, -3.530157926970578952, 32.79014554554150607 ) ) ;
#42042=EDGE_LOOP ( 'NONE', ( #1634, #30972 ) ) ;
#42043=CARTESIAN_POINT ( 'NONE',  ( -18.24999999999999289, -12.75000000000000711, 29.68455015305019273 ) ) ;
#42044=CARTESIAN_POINT ( 'NONE',  ( -6.673131404728780858, -11.86320923018887541, 32.19269448109604781 ) ) ;
#42045=B_SPLINE_CURVE_WITH_KNOTS ( 'NONE', 3,
 ( #80376, #46574, #49238, #34829, #75815, #6484, #88919, #61850, #13675, #13239 ),
 .UNSPECIFIED., .F., .F.,
 ( 4, 2, 2, 2, 4 ),
 ( 0.0007817359430256392216, 0.0009771253907250080327, 0.001172514838424376952, 0.001367904286123745872, 0.001563293733823114791 ),
 .UNSPECIFIED. ) ;
#42046=CYLINDRICAL_SURFACE ( 'NONE', #54364, 0.2499999999999994726 ) ;
#42047=DIRECTION ( 'NONE',  ( 1.000000000000000000, 0.000000000000000000, 0.000000000000000000 ) ) ;
#42048=EDGE_CURVE ( 'NONE', #75687, #65093, #8579, .T. ) ;
#42049=CARTESIAN_POINT ( 'NONE',  ( -39.05038313613820122, -2.249999999999998668, 29.75000000000000355 ) ) ;
#42051=CARTESIAN_POINT ( 'NONE',  ( 15.23076923076923173, -13.75783147151868846, 33.36296068462461051 ) ) ;
#42052=CARTESIAN_POINT ( 'NONE',  ( 7.911409417429874580, -4.481592998940250538, 33.73612834413965089 ) ) ;
#42054=ORIENTED_EDGE ( 'NONE', *, *, #65965, .F. ) ;
#42058=VERTEX_POINT ( 'NONE', #65625 ) ;
#42059=CARTESIAN_POINT ( 'NONE',  ( -8.546217925137376881, -6.460100341425560444, 34.89618726649961644 ) ) ;
#42060=VERTEX_POINT ( 'NONE', #86384 ) ;
#42061=DIRECTION ( 'NONE',  ( -0.000000000000000000, -0.9848077530122085754, -0.1736481776669273613 ) ) ;
#42062=EDGE_CURVE ( 'NONE', #20364, #40851, #56897, .T. ) ;
#42063=CARTESIAN_POINT ( 'NONE',  ( 11.53846153846153832, -13.57706302396349152, 30.56769352161908060 ) ) ;
#42064=CARTESIAN_POINT ( 'NONE',  ( -16.08777780284371772, -5.557115091759786019, 34.35708131394839882 ) ) ;
#42065=ADVANCED_FACE ( 'NONE', ( #72390 ), #17011, .F. ) ;
#42066=CARTESIAN_POINT ( 'NONE',  ( -11.66915300512910214, -11.18331474514187995, 33.13161551792790505 ) ) ;
#42067=CARTESIAN_POINT ( 'NONE',  ( 10.61538461538449418, -6.835583212225970762, 34.95778746994575670 ) ) ;
#42068=CARTESIAN_POINT ( 'NONE',  ( -13.13466997523734214, -6.653508905675592722, 34.93172785388651391 ) ) ;
#42069=DIRECTION ( 'NONE',  ( -0.000000000000000000, -0.1736481776669307198, -0.9848077530122080203 ) ) ;
#42072=CARTESIAN_POINT ( 'NONE',  ( -0.5916856709766814548, -2.619462340734461048, 30.83744416345203021 ) ) ;
#42073=CARTESIAN_POINT ( 'NONE',  ( -16.82686865700962286, -10.82426656108011720, 33.81400080652039009 ) ) ;
#42075=CARTESIAN_POINT ( 'NONE',  ( 14.43773747052708778, -2.504778602574659896, 29.97347330155780654 ) ) ;
#42076=CARTESIAN_POINT ( 'NONE',  ( -13.38461538461538325, -6.681629849574314051, 35.83090037661290239 ) ) ;
#42077=EDGE_CURVE ( 'NONE', #56304, #45063, #26921, .T. ) ;
#42078=VERTEX_POINT ( 'NONE', #10262 ) ;
#42079=ORIENTED_EDGE ( 'NONE', *, *, #57836, .F. ) ;
#42080=CARTESIAN_POINT ( 'NONE',  ( 3.100078627658924280, -10.70098750199973203, 33.91152734681376302 ) ) ;
#42083=CARTESIAN_POINT ( 'NONE',  ( -11.76128823094054354, -7.369208160676171460, 34.74850200257122879 ) ) ;
#42084=ORIENTED_EDGE ( 'NONE', *, *, #20611, .T. ) ;
#42085=EDGE_CURVE ( 'NONE', #81436, #60435, #36492, .T. ) ;
#42086=DIRECTION ( 'NONE',  ( -0.000000000000000000, 0.9848077530122085754, -0.1736481776669273613 ) ) ;
#42088=LINE ( 'NONE', #74534, #22150 ) ;
#42089=ORIENTED_EDGE ( 'NONE', *, *, #72745, .T. ) ;
#42091=CARTESIAN_POINT ( 'NONE',  ( 17.99999999999987566, -3.643525952248796163, 33.31231777344771672 ) ) ;
#42092=ORIENTED_EDGE ( 'NONE', *, *, #25530, .T. ) ;
#42093=B_SPLINE_CURVE_WITH_KNOTS ( 'NONE', 3,
 ( #61658, #34194, #40960, #19356, #60780, #68424 ),
 .UNSPECIFIED., .F., .F.,
 ( 4, 2, 4 ),
 ( 0.0003909512603273759801, 0.0005862562993132019963, 0.0007815613382990279582 ),
 .UNSPECIFIED. ) ;
#42096=VECTOR ( 'NONE', #30668, 999.9999999999998863 ) ;
#42097=CARTESIAN_POINT ( 'NONE',  ( 15.36155967173618286, -3.338503747796866872, 32.95102852606553512 ) ) ;
#42098=CARTESIAN_POINT ( 'NONE',  ( -1.607542343522233352, -9.172386477786396597, 34.72672124145550043 ) ) ;
#42100=CARTESIAN_POINT ( 'NONE',  ( 11.53846153846153832, -4.098570777380720287, 33.41473453929634729 ) ) ;
#42101=AXIS2_PLACEMENT_3D ( 'NONE', #65200, #3499, #85932 ) ;
#42102=VERTEX_POINT ( 'NONE', #10702 ) ;
#42103=ORIENTED_EDGE ( 'NONE', *, *, #50335, .F. ) ;
#42104=EDGE_LOOP ( 'NONE', ( #31421, #26250, #53521, #75307 ) ) ;
#42105=EDGE_LOOP ( 'NONE', ( #47271, #88951, #67449, #16920 ) ) ;
#42106=EDGE_CURVE ( 'NONE', #53666, #14815, #16060, .T. ) ;
#42107=CARTESIAN_POINT ( 'NONE',  ( -17.32694631421604115, -10.76384336483936011, 33.53834819971076087 ) ) ;
#42108=CARTESIAN_POINT ( 'NONE',  ( 7.716006636715624367, -3.817052484675424129, 33.13202310037935661 ) ) ;
#42109=LINE ( 'NONE', #76319, #24968 ) ;
#42111=CARTESIAN_POINT ( 'NONE',  ( 17.01084069756293715, -9.905515769479276145, 34.41647553114623292 ) ) ;
#42112=CARTESIAN_POINT ( 'NONE',  ( -17.77722045873158763, -4.387253974876677454, 33.66317474335728832 ) ) ;
#42113=ADVANCED_FACE ( 'NONE', ( #60656 ), #26443, .F. ) ;
#42114=CYLINDRICAL_SURFACE ( 'NONE', #73972, 0.2499999999999986955 ) ;
#42115=ORIENTED_EDGE ( 'NONE', *, *, #9346, .F. ) ;
#42116=ORIENTED_EDGE ( 'NONE', *, *, #28153, .T. ) ;
#42117=EDGE_LOOP ( 'NONE', ( #64491, #37948, #66254, #24493 ) ) ;
#42118=CARTESIAN_POINT ( 'NONE',  ( -0.4615384615384611200, -13.20930481340135110, 34.54067556320372745 ) ) ;
#42119=VERTEX_POINT ( 'NONE', #73755 ) ;
#42120=CARTESIAN_POINT ( 'NONE',  ( -11.53846153846166089, -4.320704448113951379, 33.92786785259630022 ) ) ;
#42121=CARTESIAN_POINT ( 'NONE',  ( 14.55763771707034948, -4.932303261841489928, 34.32971442181322885 ) ) ;
#42122=CARTESIAN_POINT ( 'NONE',  ( 3.230769230769231726, -2.499999999999998668, 29.75000000000001421 ) ) ;
#42123=VECTOR ( 'NONE', #89026, 1000.000000000000000 ) ;
#42125=EDGE_LOOP ( 'NONE', ( #16375, #87593 ) ) ;
#42126=ADVANCED_FACE ( 'NONE', ( #60213 ), #66539, .F. ) ;
#42127=VERTEX_POINT ( 'NONE', #80956 ) ;
#42128=CARTESIAN_POINT ( 'NONE',  ( -17.77698715590659972, -2.889357225399417306, 32.26129605718031712 ) ) ;
#42129=ORIENTED_EDGE ( 'NONE', *, *, #39444, .F. ) ;
#42130=FACE_BOUND ( 'NONE', #36841, .T. ) ;
#42131=CARTESIAN_POINT ( 'NONE',  ( 4.853438152358743984, -4.988325925672468131, 34.36044203135681130 ) ) ;
#42132=CARTESIAN_POINT ( 'NONE',  ( 7.846153846153846700, -5.471508081941601098, 34.59228464037088457 ) ) ;
#42133=ORIENTED_EDGE ( 'NONE', *, *, #2408, .F. ) ;
#42134=ADVANCED_FACE ( 'NONE', ( #53905 ), #53003, .F. ) ;
#42135=DIRECTION ( 'NONE',  ( 0.000000000000000000, 0.6427876096865368094, 0.7660444431189802339 ) ) ;
#42136=CARTESIAN_POINT ( 'NONE',  ( -16.08777882049607655, -12.62096338111211757, 30.90682066428152908 ) ) ;
#42137=CARTESIAN_POINT ( 'NONE',  ( 10.36536137809164870, -2.823816976329317274, 31.52131813110795733 ) ) ;
#42139=CARTESIAN_POINT ( 'NONE',  ( 14.24242230713598900, -9.528491918058357157, 34.59228464037090589 ) ) ;
#42140=ORIENTED_EDGE ( 'NONE', *, *, #13397, .F. ) ;
#42141=CARTESIAN_POINT ( 'NONE',  ( -11.40793610022789473, -12.50538340440932394, 31.33453814440721885 ) ) ;
#42142=DIRECTION ( 'NONE',  ( 0.000000000000000000, 0.000000000000000000, -1.000000000000000000 ) ) ;
#42143=CARTESIAN_POINT ( 'NONE',  ( 0.4615384615383396616, -11.94971097300221174, 32.03036669348237098 ) ) ;
#42144=CARTESIAN_POINT ( 'NONE',  ( 5.777073782483852504, -4.887634598454295265, 34.01352882383564946 ) ) ;
#42145=DIRECTION ( 'NONE',  ( -0.000000000000000000, -0.1736481776669307198, -0.9848077530122080203 ) ) ;
#42146=EDGE_CURVE ( 'NONE', #57707, #59177, #18350, .T. ) ;
#42147=FACE_BOUND ( 'NONE', #1203, .T. ) ;
#42148=CARTESIAN_POINT ( 'NONE',  ( -4.153846153846152411, -5.180354513474913603, 36.12317359536750416 ) ) ;
#42149=FACE_OUTER_BOUND ( 'NONE', #42978, .T. ) ;
#42150=CARTESIAN_POINT ( 'NONE',  ( 5.207713517890025123, -2.295524264805589354, 30.44142389570982488 ) ) ;
#42151=CARTESIAN_POINT ( 'NONE',  ( -3.230769230769229949, -2.833524468853757305, 32.15551576947925838 ) ) ;
#42152=CARTESIAN_POINT ( 'NONE',  ( -6.000000000000119904, -5.219633306517616589, 34.19971097300220464 ) ) ;
#42155=ORIENTED_EDGE ( 'NONE', *, *, #8922, .T. ) ;
#42156=EDGE_CURVE ( 'NONE', #45741, #74119, #15865, .T. ) ;
#42157=CARTESIAN_POINT ( 'NONE',  ( 1.253923917947832312, -12.11776431015575994, 31.66791131148498906 ) ) ;
#42158=ORIENTED_EDGE ( 'NONE', *, *, #72862, .F. ) ;
#42159=EDGE_CURVE ( 'NONE', #87108, #1750, #5279, .T. ) ;
#42160=CARTESIAN_POINT ( 'NONE',  ( -15.23076923076922995, -4.098570777380720287, 33.41473453929634729 ) ) ;
#42161=ORIENTED_EDGE ( 'NONE', *, *, #46928, .F. ) ;
#42162=CARTESIAN_POINT ( 'NONE',  ( -3.930834802233301950, -12.15243808032446005, 31.58219941686247978 ) ) ;
#42163=CARTESIAN_POINT ( 'NONE',  ( -18.13069146666756382, -2.541943142973489778, 30.39792223712632335 ) ) ;
#42164=ORIENTED_EDGE ( 'NONE', *, *, #14947, .F. ) ;
#42165=LINE ( 'NONE', #20549, #85791 ) ;
#42167=AXIS2_PLACEMENT_3D ( 'NONE', #7742, #14047, #49607 ) ;
#42168=B_SPLINE_CURVE_WITH_KNOTS ( 'NONE', 3,
 ( #72697, #2891, #79906, #37128, #38031, #80363, #44314, #52422, #44769, #65495 ),
 .UNSPECIFIED., .F., .F.,
 ( 4, 2, 2, 2, 4 ),
 ( 0.000000000000000000, 0.0001954311584214072381, 0.0003908623168428144762, 0.0005862934752642217414, 0.0007817246336856289524 ),
 .UNSPECIFIED. ) ;
#42169=DIRECTION ( 'NONE',  ( 0.000000000000000000, 0.6427876096865373645, -0.7660444431189797898 ) ) ;
#42170=CARTESIAN_POINT ( 'NONE',  ( 17.77707304109314634, -2.308479472611653094, 30.53278059502174457 ) ) ;
#42171=EDGE_CURVE ( 'NONE', #63925, #72548, #38731, .T. ) ;
#42172=CARTESIAN_POINT ( 'NONE',  ( 12.46153846153833911, -2.892918686052165622, 31.69288490824153470 ) ) ;
#42173=CARTESIAN_POINT ( 'NONE',  ( 15.36081683702491674, -7.723484964179501588, 34.74522123443823318 ) ) ;
#42174=DIRECTION ( 'NONE',  ( -0.000000000000000000, -0.1736481776669307198, -0.9848077530122080203 ) ) ;
#42175=CARTESIAN_POINT ( 'NONE',  ( -5.750054481651856619, -10.76462480002816235, 33.53768742498949962 ) ) ;
#42177=DIRECTION ( 'NONE',  ( 1.000000000000000000, 0.000000000000000000, 0.000000000000000000 ) ) ;
#42178=CARTESIAN_POINT ( 'NONE',  ( 14.30769230769218758, -10.90142922262034020, 33.41473453929536674 ) ) ;
#42179=DIRECTION ( 'NONE',  ( -0.000000000000000000, -0.5000000000000009992, -0.8660254037844380415 ) ) ;
#42181=DIRECTION ( 'NONE',  ( -0.000000000000000000, -0.6427876096865404731, -0.7660444431189770143 ) ) ;
#42183=VERTEX_POINT ( 'NONE', #19676 ) ;
#42184=CARTESIAN_POINT ( 'NONE',  ( 1.515405825582336607, -8.191423895709840863, 34.95447573519442130 ) ) ;
#42185=CARTESIAN_POINT ( 'NONE',  ( -0.3307466537136748985, -9.804649428959606894, 34.18742332936587047 ) ) ;
#42186=DIRECTION ( 'NONE',  ( -0.000000000000000000, -0.9396926207859092051, -0.3420201433256662704 ) ) ;
#42187=ORIENTED_EDGE ( 'NONE', *, *, #22696, .F. ) ;
#42188=CARTESIAN_POINT ( 'NONE',  ( -14.37377571864818648, -11.69971097300155272, 32.46337939537587403 ) ) ;
#42191=CARTESIAN_POINT ( 'NONE',  ( -9.692307692307691624, -12.78798330534102945, 29.74999999999997868 ) ) ;
#42192=VECTOR ( 'NONE', #13829, 1000.000000000000000 ) ;
#42193=DIRECTION ( 'NONE',  ( 0.000000000000000000, 0.1736481776669267785, -0.9848077530122087975 ) ) ;
#42194=CARTESIAN_POINT ( 'NONE',  ( 10.48469401227430886, -12.62707690430377383, 30.88035979386743435 ) ) ;
#42195=EDGE_LOOP ( 'NONE', ( #15129, #40985, #41845, #42773 ) ) ;
#42196=CYLINDRICAL_SURFACE ( 'NONE', #45507, 0.2500000000000008882 ) ;
#42197=ORIENTED_EDGE ( 'NONE', *, *, #72273, .T. ) ;
#42198=ORIENTED_EDGE ( 'NONE', *, *, #20337, .F. ) ;
#42199=CARTESIAN_POINT ( 'NONE',  ( -9.442362173959550020, -3.202959910592335646, 32.30730279482227019 ) ) ;
#42200=CARTESIAN_POINT ( 'NONE',  ( 6.673053685783957079, -2.823816976329319495, 31.52131813110795733 ) ) ;
#42201=CARTESIAN_POINT ( 'NONE',  ( -12.46153846153858247, -10.21337939537710326, 33.94971097300076224 ) ) ;
#42202=DIRECTION ( 'NONE',  ( -0.000000000000000000, 0.5000000000000011102, -0.8660254037844380415 ) ) ;
#42203=EDGE_LOOP ( 'NONE', ( #11361, #24601, #86617, #23935 ) ) ;
#42204=DIRECTION ( 'NONE',  ( -0.000000000000000000, -0.6427876096865404731, -0.7660444431189770143 ) ) ;
#42205=ORIENTED_EDGE ( 'NONE', *, *, #38362, .F. ) ;
#42206=B_SPLINE_CURVE_WITH_KNOTS ( 'NONE', 3,
 ( #79562, #44866, #10653, #57498, #38119, #84987, #8886, #23269, #36355, #63817 ),
 .UNSPECIFIED., .F., .F.,
 ( 4, 2, 2, 2, 4 ),
 ( 0.000000000000000000, 0.0001954339857564126514, 0.0003908679715128183098, 0.0005863019572692239681, 0.0007817359430256294638 ),
 .UNSPECIFIED. ) ;
#42209=ORIENTED_EDGE ( 'NONE', *, *, #63400, .F. ) ;
#42211=EDGE_LOOP ( 'NONE', ( #42368, #46326 ) ) ;
#42212=CARTESIAN_POINT ( 'NONE',  ( -0.4615384615384611200, -4.786620604624113540, 33.94971097300155094 ) ) ;
#42213=DIRECTION ( 'NONE',  ( 0.000000000000000000, 0.6427876096865368094, 0.7660444431189802339 ) ) ;
#42214=VECTOR ( 'NONE', #631, 1000.000000000000227 ) ;
#42215=EDGE_CURVE ( 'NONE', #35812, #60430, #38618, .T. ) ;
#42216=VECTOR ( 'NONE', #66594, 1000.000000000000227 ) ;
#42217=CARTESIAN_POINT ( 'NONE',  ( 4.088575707885377497, -4.481592998940161721, 33.73612834413957984 ) ) ;
#42218=CARTESIAN_POINT ( 'NONE',  ( -5.010753935960420513, -7.250054483168843156, 34.74374881642865631 ) ) ;
#42219=ADVANCED_FACE ( 'NONE', ( #72234 ), #37111, .F. ) ;
#42221=ORIENTED_EDGE ( 'NONE', *, *, #46861, .T. ) ;
#42222=ORIENTED_EDGE ( 'NONE', *, *, #82740, .F. ) ;
#42223=CARTESIAN_POINT ( 'NONE',  ( -6.857821783564085116, -3.083524468853784839, 32.58852847137153930 ) ) ;
#42224=CARTESIAN_POINT ( 'NONE',  ( 4.153846153846032507, -11.48612834414049644, 32.76840700105863391 ) ) ;
#42225=VERTEX_POINT ( 'NONE', #45201 ) ;
#42226=EDGE_CURVE ( 'NONE', #86676, #79746, #34241, .T. ) ;
#42227=DIRECTION ( 'NONE',  ( -1.000000000000000000, 0.000000000000000000, 0.000000000000000000 ) ) ;
#42228=DIRECTION ( 'NONE',  ( 0.000000000000000000, 0.9848077530122072432, -0.1736481776669354937 ) ) ;
#42229=LINE ( 'NONE', #13850, #85384 ) ;
#42230=EDGE_LOOP ( 'NONE', ( #47426, #25615 ) ) ;
#42231=CARTESIAN_POINT ( 'NONE',  ( 15.16549878480845770, -10.90142922261923886, 33.41473453929638993 ) ) ;
#42232=EDGE_CURVE ( 'NONE', #7100, #37311, #80529, .T. ) ;
#42233=LINE ( 'NONE', #35461, #800 ) ;
#42234=ORIENTED_EDGE ( 'NONE', *, *, #66514, .T. ) ;
#42235=FACE_BOUND ( 'NONE', #69510, .T. ) ;
#42236=FACE_OUTER_BOUND ( 'NONE', #32065, .T. ) ;
#42237=CARTESIAN_POINT ( 'NONE',  ( 1.384615384615386802, -1.509761064869970415, 31.06009739812519044 ) ) ;
#42238=CARTESIAN_POINT ( 'NONE',  ( 12.33139049180676672, -6.809168938359901446, 34.95455904226513866 ) ) ;
#42239=CARTESIAN_POINT ( 'NONE',  ( 7.846153846153846700, -13.37000171582298513, 34.34916445242398453 ) ) ;
#42240=CARTESIAN_POINT ( 'NONE',  ( 18.25005431163831204, -4.235687564193445276, 33.53795663066793509 ) ) ;
#42241=DIRECTION ( 'NONE',  ( -0.000000000000000000, 1.000000000000000000, 3.491481338843133355E-15 ) ) ;
#42242=CARTESIAN_POINT ( 'NONE',  ( -15.93083480223330817, -9.086983370893049639, 34.49168942202179267 ) ) ;
#42243=ORIENTED_EDGE ( 'NONE', *, *, #66158, .F. ) ;
#42244=DIRECTION ( 'NONE',  ( -0.000000000000000000, 0.6427876096865404731, -0.7660444431189770143 ) ) ;
#42245=DIRECTION ( 'NONE',  ( -0.000000000000000000, 0.7660444431189791237, -0.6427876096865379196 ) ) ;
#42246=ORIENTED_EDGE ( 'NONE', *, *, #20014, .F. ) ;
#42247=VECTOR ( 'NONE', #64683, 999.9999999999998863 ) ;
#42248=CARTESIAN_POINT ( 'NONE',  ( 8.519207531937803779, -3.202444869320336451, 32.30641848906366675 ) ) ;
#42249=CARTESIAN_POINT ( 'NONE',  ( -4.403822897894744237, -3.436278759898155677, 33.07459398097509506 ) ) ;
#42250=EDGE_LOOP ( 'NONE', ( #25739, #63797, #67270, #52307 ) ) ;
#42251=DIRECTION ( 'NONE',  ( -0.000000000000000000, -0.8660254037844397068, -0.4999999999999978906 ) ) ;
#42252=CARTESIAN_POINT ( 'NONE',  ( 2.530471976670374712, -4.989023458446561143, 34.36081565061822118 ) ) ;
#42253=FACE_BOUND ( 'NONE', #35104, .T. ) ;
#42255=CARTESIAN_POINT ( 'NONE',  ( 15.29602480204525961, -12.27809138561124591, 31.22303859784720359 ) ) ;
#42256=FACE_OUTER_BOUND ( 'NONE', #80891, .T. ) ;
#42257=CARTESIAN_POINT ( 'NONE',  ( 1.384615384615386802, -12.62096338111211580, 30.90682066428153263 ) ) ;
#42258=CARTESIAN_POINT ( 'NONE',  ( -7.780898706641008467, -12.70778746994558439, 30.41441678777536595 ) ) ;
#42259=CARTESIAN_POINT ( 'NONE',  ( -12.59222992820602371, -4.118384482072085184, 33.43331474514187107 ) ) ;
#42262=ORIENTED_EDGE ( 'NONE', *, *, #61521, .F. ) ;
#42264=B_SPLINE_CURVE_WITH_KNOTS ( 'NONE', 3,
 ( #14248, #61983, #34520, #41286, #7937, #62854, #27757, #14693, #63757, #13801 ),
 .UNSPECIFIED., .F., .F.,
 ( 4, 2, 2, 2, 4 ),
 ( 0.0007817359430256253438, 0.0009771253907249898181, 0.001172514838424354401, 0.001367904286123718983, 0.001563293733823083566 ),
 .UNSPECIFIED. ) ;
#42265=ORIENTED_EDGE ( 'NONE', *, *, #72554, .T. ) ;
#42267=CARTESIAN_POINT ( 'NONE',  ( 14.55763771707035303, -12.68172785388650681, 30.59649109432439218 ) ) ;
#42268=DIRECTION ( 'NONE',  ( -0.000000000000000000, 0.1736481776669307198, -0.9848077530122080203 ) ) ;
#42269=CARTESIAN_POINT ( 'NONE',  ( -0.5922290646487710086, -2.845849958028613624, 32.17971566917920967 ) ) ;
#42270=CARTESIAN_POINT ( 'NONE',  ( -3.903791733932699515, -2.920487667080175154, 32.31805714834170828 ) ) ;
#42272=CARTESIAN_POINT ( 'NONE',  ( 3.903846153846154632, -7.433931650972300353, 34.75000000000000711 ) ) ;
#42273=DIRECTION ( 'NONE',  ( -0.000000000000000000, -0.8660254037844399289, -0.4999999999999980016 ) ) ;
#42274=EDGE_CURVE ( 'NONE', #57045, #32941, #12715, .T. ) ;
#42275=CARTESIAN_POINT ( 'NONE',  ( -17.07692307692307665, -4.786620604624113540, 33.94971097300155094 ) ) ;
#42276=CARTESIAN_POINT ( 'NONE',  ( -4.826977667545033768, -2.341251567377310217, 30.72681386836322659 ) ) ;
#42277=LINE ( 'NONE', #33737, #87075 ) ;
#42279=CARTESIAN_POINT ( 'NONE',  ( -4.946131269098293259, -2.729792928343270919, 31.24908615093345077 ) ) ;
#42280=CARTESIAN_POINT ( 'NONE',  ( 10.74543205063506868, -7.723484941389743952, 34.99544897038808955 ) ) ;
#42281=EDGE_CURVE ( 'NONE', #65093, #26314, #66468, .T. ) ;
#42282=ADVANCED_FACE ( 'NONE', ( #66373 ), #58272, .F. ) ;
#42283=LINE ( 'NONE', #83265, #72995 ) ;
#42284=VERTEX_POINT ( 'NONE', #16850 ) ;
#42285=CARTESIAN_POINT ( 'NONE',  ( -14.30769230769242739, -3.835265460704628371, 33.15142922262033665 ) ) ;
#42288=CARTESIAN_POINT ( 'NONE',  ( 3.930919194939304084, -4.762599654559228846, 34.23009711892697737 ) ) ;
#42289=LINE ( 'NONE', #8939, #81520 ) ;
#42291=CARTESIAN_POINT ( 'NONE',  ( -4.153846153846152411, -13.53365097954675988, 30.81389545987213552 ) ) ;
#42292=CARTESIAN_POINT ( 'NONE',  ( -9.561781990544128362, -5.195472089885680766, 34.18748526763464923 ) ) ;
#42293=ORIENTED_EDGE ( 'NONE', *, *, #31867, .T. ) ;
#42294=CARTESIAN_POINT ( 'NONE',  ( 9.915087361285756629, -12.69155399931963046, 30.53255429739157734 ) ) ;
#42295=CARTESIAN_POINT ( 'NONE',  ( -4.854143535654668717, -10.11255958852956027, 34.01340905677048454 ) ) ;
#42299=CARTESIAN_POINT ( 'NONE',  ( -2.307692307692305711, -6.343179335718451384, 34.87096338111211935 ) ) ;
#42300=VERTEX_POINT ( 'NONE', #31707 ) ;
#42301=B_SPLINE_CURVE_WITH_KNOTS ( 'NONE', 3,
 ( #52340, #53232, #72618, #87494, #80735, #19015, #39743, #46487, #73965, #12255 ),
 .UNSPECIFIED., .F., .F.,
 ( 4, 2, 2, 2, 4 ),
 ( 0.000000000000000000, 0.0001954339857564093175, 0.0003908679715128186350, 0.0005863019572692279796, 0.0007817359430256372700 ),
 .UNSPECIFIED. ) ;
#42302=CARTESIAN_POINT ( 'NONE',  ( -10.86540783960607115, -4.175268141568685643, 33.81360843649122216 ) ) ;
#42304=ADVANCED_FACE ( 'NONE', ( #85763 ), #58718, .F. ) ;
#42305=DIRECTION ( 'NONE',  ( -0.000000000000000000, 1.000000000000000000, 3.491481338843133355E-15 ) ) ;
#42306=CARTESIAN_POINT ( 'NONE',  ( -10.61538461538461320, -2.249999999999998668, 29.75000000000001776 ) ) ;
#42307=ORIENTED_EDGE ( 'NONE', *, *, #30017, .T. ) ;
#42309=CARTESIAN_POINT ( 'NONE',  ( -10.61538461538473577, -2.379036618888197729, 30.90682066428292885 ) ) ;
#42310=EDGE_CURVE ( 'NONE', #87005, #58712, #42713, .T. ) ;
#42312=CARTESIAN_POINT ( 'NONE',  ( -17.77698715590660328, -4.762714258010878332, 34.23016756924214832 ) ) ;
#42313=CARTESIAN_POINT ( 'NONE',  ( -1.319359813339359588, -2.625532179533470067, 30.86335684631491105 ) ) ;
#42315=FACE_OUTER_BOUND ( 'NONE', #2172, .T. ) ;
#42317=CARTESIAN_POINT ( 'NONE',  ( 0.2115384615384615363, -7.433932668274254141, 35.00000000000001421 ) ) ;
#42318=DIRECTION ( 'NONE',  ( -0.000000000000000000, -0.3420201433256694901, -0.9396926207859082059 ) ) ;
#42320=ORIENTED_EDGE ( 'NONE', *, *, #62462, .T. ) ;
#42321=CARTESIAN_POINT ( 'NONE',  ( 9.692307692307695177, -4.098570777380720287, 33.41473453929634729 ) ) ;
#42322=VERTEX_POINT ( 'NONE', #43149 ) ;
#42323=EDGE_CURVE ( 'NONE', #57930, #40306, #65342, .T. ) ;
#42324=CARTESIAN_POINT ( 'NONE',  ( -16.15384615384615330, -11.16473453929635440, 33.15142922261926373 ) ) ;
#42325=ORIENTED_EDGE ( 'NONE', *, *, #87428, .F. ) ;
#42326=CARTESIAN_POINT ( 'NONE',  ( -18.00000000000012079, -3.300289026999231545, 32.46337939537709616 ) ) ;
#42327=CARTESIAN_POINT ( 'NONE',  ( 3.903846153846154632, -2.249999999999998668, 29.75000000000000355 ) ) ;
#42328=VERTEX_POINT ( 'NONE', #397 ) ;
#42329=DIRECTION ( 'NONE',  ( -0.000000000000000000, -0.1736481776669307198, -0.9848077530122080203 ) ) ;
#42330=ORIENTED_EDGE ( 'NONE', *, *, #57128, .F. ) ;
#42331=CARTESIAN_POINT ( 'NONE',  ( -8.638705067467206788, -8.586989748646452369, 34.63063291749215011 ) ) ;
#42332=EDGE_LOOP ( 'NONE', ( #15701, #63574 ) ) ;
#42333=EDGE_CURVE ( 'NONE', #60048, #48024, #75099, .T. ) ;
#42334=CARTESIAN_POINT ( 'NONE',  ( -12.71151520558705528, -3.436278759898153901, 33.07459398097509506 ) ) ;
#42335=B_SPLINE_CURVE_WITH_KNOTS ( 'NONE', 3,
 ( #60751, #75168, #81485, #20652, #40060, #32398 ),
 .UNSPECIFIED., .F., .F.,
 ( 4, 2, 4 ),
 ( 0.0003909512603273935984, 0.0005862562993132163077, 0.0007815613382990390171 ),
 .UNSPECIFIED. ) ;
#42336=VECTOR ( 'NONE', #62356, 999.9999999999998863 ) ;
#42337=ORIENTED_EDGE ( 'NONE', *, *, #70263, .F. ) ;
#42338=CARTESIAN_POINT ( 'NONE',  ( 16.08776274289027342, -12.37446782046654192, 30.86335684631486487 ) ) ;
#42339=CARTESIAN_POINT ( 'NONE',  ( -14.30769230769230660, -11.33034616979429110, 35.88435417666054406 ) ) ;
#42341=FACE_BOUND ( 'NONE', #33503, .T. ) ;
#42342=AXIS2_PLACEMENT_3D ( 'NONE', #71869, #31339, #38998 ) ;
#42343=CARTESIAN_POINT ( 'NONE',  ( 1.634669696253701288, -12.41262288849542017, 30.68299917996395010 ) ) ;
#42344=CARTESIAN_POINT ( 'NONE',  ( -6.700297381808510089, -12.24180327182771855, 31.33663988360758168 ) ) ;
#42345=LINE ( 'NONE', #76564, #49601 ) ;
#42348=LINE ( 'NONE', #69802, #7382 ) ;
#42349=ORIENTED_EDGE ( 'NONE', *, *, #74545, .T. ) ;
#42350=LINE ( 'NONE', #55402, #43253 ) ;
#42351=ORIENTED_EDGE ( 'NONE', *, *, #85294, .T. ) ;
#42352=VERTEX_POINT ( 'NONE', #7595 ) ;
#42353=CARTESIAN_POINT ( 'NONE',  ( -5.076923076923075762, -3.050289026998446396, 32.03036669348365706 ) ) ;
#42354=CARTESIAN_POINT ( 'NONE',  ( -16.15384615384627409, -11.48612834414049644, 32.76840700105863391 ) ) ;
#42355=EDGE_CURVE ( 'NONE', #42183, #78937, #50, .T. ) ;
#42356=CARTESIAN_POINT ( 'NONE',  ( 6.000000000000001776, -1.242168528481310874, 33.36296068462461051 ) ) ;
#42357=CARTESIAN_POINT ( 'NONE',  ( 7.976944287120798727, -3.338503747796866872, 32.95102852606553512 ) ) ;
#42358=FACE_OUTER_BOUND ( 'NONE', #29250, .T. ) ;
#42359=DIRECTION ( 'NONE',  ( -0.000000000000000000, 0.7660444431189791237, -0.6427876096865379196 ) ) ;
#42360=ORIENTED_EDGE ( 'NONE', *, *, #73024, .F. ) ;
#42361=LINE ( 'NONE', #49099, #38595 ) ;
#42364=CARTESIAN_POINT ( 'NONE',  ( -8.519176349317316266, -2.544122305571458575, 31.48381861865057729 ) ) ;
#42365=DIRECTION ( 'NONE',  ( 0.000000000000000000, 0.7660444431189822323, -0.6427876096865344779 ) ) ;
#42366=VERTEX_POINT ( 'NONE', #21991 ) ;
#42367=CARTESIAN_POINT ( 'NONE',  ( 5.076923076923075762, -13.87047571288749737, 32.06866353760679544 ) ) ;
#42368=ORIENTED_EDGE ( 'NONE', *, *, #27013, .T. ) ;
#42369=B_SPLINE_CURVE_WITH_KNOTS ( 'NONE', 3,
 ( #85387, #19588, #61015, #45728, #11957, #33987, #25906, #47049, #39875, #46180 ),
 .UNSPECIFIED., .F., .F.,
 ( 4, 2, 2, 2, 4 ),
 ( 0.0007817359430256365111, 0.0009771253907250043464, 0.001172514838424372399, 0.001367904286123740234, 0.001563293733823108069 ),
 .UNSPECIFIED. ) ;
#42370=ORIENTED_EDGE ( 'NONE', *, *, #81290, .F. ) ;
#42371=CARTESIAN_POINT ( 'NONE',  ( 7.846153846153846700, -13.78497067705608181, 32.30358669280327177 ) ) ;
#42372=EDGE_CURVE ( 'NONE', #519, #22135, #78263, .T. ) ;
#42373=ORIENTED_EDGE ( 'NONE', *, *, #75433, .F. ) ;
#42375=CARTESIAN_POINT ( 'NONE',  ( -17.14219352288385778, -3.300289026998414865, 32.46337939537583850 ) ) ;
#42376=CYLINDRICAL_SURFACE ( 'NONE', #49506, 0.2500000000000002220 ) ;
#42377=CARTESIAN_POINT ( 'NONE',  ( -4.946132635956123735, -3.338503747796866872, 32.95102852606553512 ) ) ;
#42378=CYLINDRICAL_SURFACE ( 'NONE', #2841, 0.2500000000000002220 ) ;
#42379=ADVANCED_FACE ( 'NONE', ( #49465 ), #8037, .F. ) ;
#42380=CARTESIAN_POINT ( 'NONE',  ( 8.638539302563209787, -6.413092428213692742, 34.63065189839063152 ) ) ;
#42381=VECTOR ( 'NONE', #35611, 1000.000000000000227 ) ;
#42382=VERTEX_POINT ( 'NONE', #76042 ) ;
#42383=CARTESIAN_POINT ( 'NONE',  ( 4.403846153846169287, -2.249999999999999112, 29.81603969181031033 ) ) ;
#42384=CARTESIAN_POINT ( 'NONE',  ( -12.46153846153846168, -9.058645607665452459, 34.76329471203371924 ) ) ;
#42385=ORIENTED_EDGE ( 'NONE', *, *, #28251, .F. ) ;
#42386=CARTESIAN_POINT ( 'NONE',  ( -3.230769230768923084, -2.506253911140615021, 30.00000000000323297 ) ) ;
#42387=DIRECTION ( 'NONE',  ( -0.000000000000000000, -0.3420201433256694346, -0.9396926207859080948 ) ) ;
#42388=CARTESIAN_POINT ( 'NONE',  ( -0.5922290646487706756, -3.957541250942359756, 33.62499894934981626 ) ) ;
#42389=B_SPLINE_CURVE_WITH_KNOTS ( 'NONE', 3,
 ( #85802, #79033, #3814, #22748, #86257, #57422, #17334, #24525, #44791, #51994 ),
 .UNSPECIFIED., .F., .F.,
 ( 4, 2, 2, 2, 4 ),
 ( 0.000000000000000000, 0.0001954339857564081791, 0.0003908679715128163582, 0.0005863019572692245102, 0.0007817359430256327164 ),
 .UNSPECIFIED. ) ;
#42390=CARTESIAN_POINT ( 'NONE',  ( 6.250054419913455561, -9.233818618650603938, 34.70587769442853698 ) ) ;
#42391=LINE ( 'NONE', #88814, #4465 ) ;
#42392=EDGE_CURVE ( 'NONE', #82786, #2951, #62515, .T. ) ;
#42393=CARTESIAN_POINT ( 'NONE',  ( 11.53846153846153832, -8.120952969808772792, 34.71129190930000163 ) ) ;
#42394=DIRECTION ( 'NONE',  ( -0.000000000000000000, -0.9848077530122085754, -0.1736481776669273613 ) ) ;
#42397=CARTESIAN_POINT ( 'NONE',  ( -1.319359813339359588, -11.48612834413965977, 32.76840700105972815 ) ) ;
#42398=CARTESIAN_POINT ( 'NONE',  ( 12.46153846153833911, -5.094484230521993062, 34.41647553114689373 ) ) ;
#42399=CARTESIAN_POINT ( 'NONE',  ( 7.846153846153725020, -2.625532179533779154, 30.86335684631627174 ) ) ;
#42400=DIRECTION ( 'NONE',  ( 0.000000000000000000, 0.9848077530122072432, 0.1736481776669354937 ) ) ;
#42401=ORIENTED_EDGE ( 'NONE', *, *, #35977, .F. ) ;
#42402=CARTESIAN_POINT ( 'NONE',  ( 10.61538461538461675, -1.790695186598648903, 34.54067556320373455 ) ) ;
#42403=CARTESIAN_POINT ( 'NONE',  ( -2.372962753653082402, -3.300289026998414865, 32.46337939537583139 ) ) ;
#42404=CARTESIAN_POINT ( 'NONE',  ( -1.254089682851820209, -6.852161475712352789, 34.70806712695775786 ) ) ;
#42405=CARTESIAN_POINT ( 'NONE',  ( -4.219929564802032296, -10.51840700105979387, 33.73612834413961536 ) ) ;
#42407=CARTESIAN_POINT ( 'NONE',  ( -16.15384615384615330, -12.78798330534103123, 29.99999999999997868 ) ) ;
#42408=EDGE_CURVE ( 'NONE', #53458, #34311, #21324, .T. ) ;
#42410=FACE_OUTER_BOUND ( 'NONE', #16159, .T. ) ;
#42411=CYLINDRICAL_SURFACE ( 'NONE', #17746, 0.2499999999999973355 ) ;
#42412=ORIENTED_EDGE ( 'NONE', *, *, #4052, .F. ) ;
#42413=CARTESIAN_POINT ( 'NONE',  ( -8.769230769230455635, -2.255955759149395501, 30.00000000000324363 ) ) ;
#42417=DIRECTION ( 'NONE',  ( 0.000000000000000000, 0.8660254037844377084, -0.5000000000000015543 ) ) ;
#42418=VERTEX_POINT ( 'NONE', #84154 ) ;
#42419=CARTESIAN_POINT ( 'NONE',  ( 10.68145194873469350, -11.35647404775217595, 33.31231777344666511 ) ) ;
#42420=CARTESIAN_POINT ( 'NONE',  ( -9.019207500173124004, -2.564618984488975073, 30.55390908950641915 ) ) ;
#42421=CARTESIAN_POINT ( 'NONE',  ( -10.83886955910856464, -5.912607949931405926, 34.49155766932282319 ) ) ;
#42422=CARTESIAN_POINT ( 'NONE',  ( -11.40767109749458541, -5.496552790871120031, 34.60292014791297532 ) ) ;
#42423=DIRECTION ( 'NONE',  ( 0.000000000000000000, 0.1736481776669275834, 0.9848077530122086864 ) ) ;
#42424=ORIENTED_EDGE ( 'NONE', *, *, #4545, .T. ) ;
#42425=ORIENTED_EDGE ( 'NONE', *, *, #5838, .T. ) ;
#42426=FACE_BOUND ( 'NONE', #9111, .T. ) ;
#42427=ORIENTED_EDGE ( 'NONE', *, *, #41599, .T. ) ;
#42428=CARTESIAN_POINT ( 'NONE',  ( 15.23076923076923173, -12.37446782046654192, 30.86335684631486131 ) ) ;
#42429=B_SPLINE_CURVE_WITH_KNOTS ( 'NONE', 3,
 ( #17403, #24145, #24595, #59268, #86773, #16953, #79990, #30899, #46206, #73691 ),
 .UNSPECIFIED., .F., .F.,
 ( 4, 2, 2, 2, 4 ),
 ( 0.000000000000000000, 0.0001954311564186863323, 0.0003908623128373726646, 0.0005862934692560590241, 0.0007817246256747453293 ),
 .UNSPECIFIED. ) ;
#42430=CARTESIAN_POINT ( 'NONE',  ( -14.24243716817946925, -11.67786785259547777, 32.92929555188713664 ) ) ;
#42431=CARTESIAN_POINT ( 'NONE',  ( 9.562160482869471068, -12.27039167877662251, 31.24851455888617835 ) ) ;
#42432=CARTESIAN_POINT ( 'NONE',  ( -10.61538461538461320, -12.09954503811598769, 35.62045528018868623 ) ) ;
#42433=VERTEX_POINT ( 'NONE', #75595 ) ;
#42435=EDGE_LOOP ( 'NONE', ( #28184, #35350 ) ) ;
#42436=VERTEX_POINT ( 'NONE', #68845 ) ;
#42437=CARTESIAN_POINT ( 'NONE',  ( 13.13461538461538858, -7.566083408709835645, 34.74999999999999289 ) ) ;
#42438=EDGE_LOOP ( 'NONE', ( #56850, #76625 ) ) ;
#42439=FACE_OUTER_BOUND ( 'NONE', #29115, .T. ) ;
#42440=CARTESIAN_POINT ( 'NONE',  ( -6.673076923076909139, -2.249999999999999112, 29.81603969181031033 ) ) ;
#42441=LINE ( 'NONE', #29374, #11171 ) ;
#42442=CARTESIAN_POINT ( 'NONE',  ( 9.019176287578908102, -9.272278438253398036, 34.42582936511637115 ) ) ;
#42443=CARTESIAN_POINT ( 'NONE',  ( 6.000000000000001776, -8.564572088678739092, 35.78748833219616898 ) ) ;
#42444=CARTESIAN_POINT ( 'NONE',  ( 14.37294787896833448, -6.879047030191282275, 34.71129190930002295 ) ) ;
#42445=CARTESIAN_POINT ( 'NONE',  ( -1.134669975237340811, -2.986452184633681117, 32.43230066228895225 ) ) ;
#42447=ORIENTED_EDGE ( 'NONE', *, *, #37390, .F. ) ;
#42448=ORIENTED_EDGE ( 'NONE', *, *, #64002, .T. ) ;
#42449=CARTESIAN_POINT ( 'NONE',  ( 2.980769230769232170, -7.500000000000001776, 35.00000000000000000 ) ) ;
#42450=CARTESIAN_POINT ( 'NONE',  ( -6.000000000000119904, -9.442884908241554243, 34.35708131394783038 ) ) ;
#42451=CARTESIAN_POINT ( 'NONE',  ( -13.51530685128294529, -5.582088688514999397, 34.36776431015576350 ) ) ;
#42452=B_SPLINE_CURVE_WITH_KNOTS ( 'NONE', 3,
 ( #10594, #38060, #39412, #59660, #33534, #72725, #60103, #4728, #53344, #60548 ),
 .UNSPECIFIED., .F., .F.,
 ( 4, 2, 2, 2, 4 ),
 ( 0.0007817359430256288133, 0.0009771253907249945886, 0.001172514838424360472, 0.001367904286123726356, 0.001563293733823092240 ),
 .UNSPECIFIED. ) ;
#42453=CARTESIAN_POINT ( 'NONE',  ( 1.384615384615386802, -12.34228464037088635, 31.77849191805839268 ) ) ;
#42454=CARTESIAN_POINT ( 'NONE',  ( 12.68431813051652668, -12.69155399931963046, 30.53255429739157734 ) ) ;
#42455=FACE_BOUND ( 'NONE', #25582, .T. ) ;
#42456=CARTESIAN_POINT ( 'NONE',  ( 8.068933387422250192, -11.41317474335729543, 32.86274602512330034 ) ) ;
#42457=ORIENTED_EDGE ( 'NONE', *, *, #76324, .F. ) ;
#42458=CIRCLE ( 'NONE', #46756, 0.2500000000000002220 ) ;
#42459=CARTESIAN_POINT ( 'NONE',  ( -7.976763501357926778, -7.722926974430166069, 34.99546784045486447 ) ) ;
#42460=CARTESIAN_POINT ( 'NONE',  ( 9.627037691751372250, -12.16647553114622049, 32.15551576947930812 ) ) ;
#42463=ORIENTED_EDGE ( 'NONE', *, *, #4243, .F. ) ;
#42464=B_SPLINE_CURVE_WITH_KNOTS ( 'NONE', 3,
 ( #9568, #42043, #37030, #69501, #42485, #69943 ),
 .UNSPECIFIED., .F., .F.,
 ( 4, 2, 4 ),
 ( 0.000000000000000000, 0.1250000000000000000, 0.2500000000000000000 ),
 .UNSPECIFIED. ) ;
#42465=CARTESIAN_POINT ( 'NONE',  ( 6.130790440966950250, -10.70102852606553157, 33.91149625220312913 ) ) ;
#42466=ORIENTED_EDGE ( 'NONE', *, *, #2613, .T. ) ;
#42467=B_SPLINE_CURVE_WITH_KNOTS ( 'NONE', 3,
 ( #1269, #48125, #28299, #21545, #49019, #35510, #70178, #76941, #13902, #7151 ),
 .UNSPECIFIED., .F., .F.,
 ( 4, 2, 2, 2, 4 ),
 ( 0.0007817359430256285964, 0.0009771253907249948054, 0.001172514838424360906, 0.001367904286123727223, 0.001563293733823093324 ),
 .UNSPECIFIED. ) ;
#42468=FACE_BOUND ( 'NONE', #47345, .T. ) ;
#42470=EDGE_CURVE ( 'NONE', #83460, #10983, #60094, .T. ) ;
#42471=CARTESIAN_POINT ( 'NONE',  ( 17.07692307692295586, -11.94971097300221174, 32.03036669348237098 ) ) ;
#42472=CARTESIAN_POINT ( 'NONE',  ( 12.46153846153833911, -11.67786785259630911, 32.92929555188603530 ) ) ;
#42473=ORIENTED_EDGE ( 'NONE', *, *, #39771, .F. ) ;
#42474=VECTOR ( 'NONE', #10528, 1000.000000000000114 ) ;
#42475=EDGE_CURVE ( 'NONE', #9551, #4412, #38553, .T. ) ;
#42477=CARTESIAN_POINT ( 'NONE',  ( 4.153846153846032507, -3.835265460704628371, 33.15142922262033665 ) ) ;
#42479=DIRECTION ( 'NONE',  ( -0.000000000000000000, 0.6427876096865404731, -0.7660444431189771253 ) ) ;
#42481=CARTESIAN_POINT ( 'NONE',  ( 13.31853197365950692, -5.557115091759785130, 34.35708131394839171 ) ) ;
#42482=ORIENTED_EDGE ( 'NONE', *, *, #30884, .T. ) ;
#42483=CARTESIAN_POINT ( 'NONE',  ( 4.376625822824218304, -3.020022701398814124, 32.48759521482552515 ) ) ;
#42484=ORIENTED_EDGE ( 'NONE', *, *, #3173, .F. ) ;
#42485=CARTESIAN_POINT ( 'NONE',  ( -18.06544984694978595, -12.75000000000000888, 29.49999999999998224 ) ) ;
#42487=CARTESIAN_POINT ( 'NONE',  ( 4.853996118016228323, -2.523278758544489797, 31.42238647778637528 ) ) ;
#42488=CARTESIAN_POINT ( 'NONE',  ( -8.769230769230768274, -5.180354513474913603, 36.12317359536750416 ) ) ;
#42490=CYLINDRICAL_SURFACE ( 'NONE', #74886, 0.2499999999999994726 ) ;
#42492=DIRECTION ( 'NONE',  ( -0.000000000000000000, 0.000000000000000000, 1.000000000000000000 ) ) ;
#42494=ORIENTED_EDGE ( 'NONE', *, *, #45740, .F. ) ;
#42495=CARTESIAN_POINT ( 'NONE',  ( -16.40382289789474513, -4.818429247618091438, 34.26397095200675125 ) ) ;
#42496=ORIENTED_EDGE ( 'NONE', *, *, #28751, .F. ) ;
#42497=ORIENTED_EDGE ( 'NONE', *, *, #65048, .F. ) ;
#42498=CARTESIAN_POINT ( 'NONE',  ( 15.23076923076910916, -11.06231777344772027, 33.60647404775119895 ) ) ;
#42499=ORIENTED_EDGE ( 'NONE', *, *, #21898, .F. ) ;
#42500=CARTESIAN_POINT ( 'NONE',  ( -5.777220331021931443, -12.69155399931963046, 30.53255429739158444 ) ) ;
#42501=FACE_OUTER_BOUND ( 'NONE', #74068, .T. ) ;
#42502=B_SPLINE_CURVE_WITH_KNOTS ( 'NONE', 3,
 ( #43318, #23039, #15411, #36562, #70795, #63580, #63129, #49629, #1882, #23473 ),
 .UNSPECIFIED., .F., .F.,
 ( 4, 2, 2, 2, 4 ),
 ( 0.000000000000000000, 0.0001954339857564073659, 0.0003908679715128147319, 0.0005863019572692221250, 0.0007817359430256294638 ),
 .UNSPECIFIED. ) ;
#42503=VECTOR ( 'NONE', #36928, 999.9999999999998863 ) ;
#42504=LINE ( 'NONE', #74969, #67489 ) ;
#42505=CYLINDRICAL_SURFACE ( 'NONE', #12912, 0.2500000000000009437 ) ;
#42506=CARTESIAN_POINT ( 'NONE',  ( -8.835313148590902443, -2.486705287966279432, 31.30864560766542937 ) ) ;
#42508=LINE ( 'NONE', #78487, #69533 ) ;
#42509=B_SPLINE_CURVE_WITH_KNOTS ( 'NONE', 3,
 ( #38448, #18178, #80334, #73580, #30354, #37542, #65009, #3318, #75768, #27587 ),
 .UNSPECIFIED., .F., .F.,
 ( 4, 2, 2, 2, 4 ),
 ( 0.000000000000000000, 0.0001954339857564073659, 0.0003908679715128147319, 0.0005863019572692221250, 0.0007817359430256294638 ),
 .UNSPECIFIED. ) ;
#42510=CARTESIAN_POINT ( 'NONE',  ( 6.699591998512593349, -10.23692288466677880, 34.23039457007281072 ) ) ;
#42511=CARTESIAN_POINT ( 'NONE',  ( -2.307692307692428724, -3.083524468854526912, 32.58852847137268327 ) ) ;
#42512=EDGE_CURVE ( 'NONE', #58364, #2406, #79401, .T. ) ;
#42513=EDGE_CURVE ( 'NONE', #39107, #89080, #23556, .T. ) ;
#42514=LINE ( 'NONE', #75847, #17688 ) ;
#42515=DIRECTION ( 'NONE',  ( -0.000000000000000000, -0.000000000000000000, -1.000000000000000000 ) ) ;
#42516=ADVANCED_FACE ( 'NONE', ( #78251 ), #72381, .F. ) ;
#42517=ORIENTED_EDGE ( 'NONE', *, *, #55493, .T. ) ;
#42518=ORIENTED_EDGE ( 'NONE', *, *, #28891, .F. ) ;
#42519=EDGE_CURVE ( 'NONE', #80969, #57045, #23745, .T. ) ;
#42520=CARTESIAN_POINT ( 'NONE',  ( 12.71159288145191901, -2.544122305571458575, 31.48381861865057729 ) ) ;
#42522=CARTESIAN_POINT ( 'NONE',  ( 10.61538461538461675, -13.95598074871891292, 31.83374038241031911 ) ) ;
#42524=ORIENTED_EDGE ( 'NONE', *, *, #39768, .F. ) ;
#42525=CARTESIAN_POINT ( 'NONE',  ( -16.02332071561251325, -8.630441415882549094, 34.87705825610312615 ) ) ;
#42526=CARTESIAN_POINT ( 'NONE',  ( -13.44988538517170795, -11.06231777344662781, 33.60647404775220082 ) ) ;
#42528=CIRCLE ( 'NONE', #61219, 0.2500000000000002220 ) ;
#42530=CARTESIAN_POINT ( 'NONE',  ( -13.45069879557126669, -9.780366693483667717, 34.19971097300155805 ) ) ;
#42532=CARTESIAN_POINT ( 'NONE',  ( 4.153846153846032507, -9.442884908241554243, 34.35708131394783038 ) ) ;
#42534=CARTESIAN_POINT ( 'NONE',  ( -8.069080805060693251, -2.523278758544489797, 31.42238647778637528 ) ) ;
#42536=CARTESIAN_POINT ( 'NONE',  ( -14.05763799605399456, -11.79725096376909299, 32.30694842903960762 ) ) ;
#42537=DIRECTION ( 'NONE',  ( -0.000000000000000000, 0.9396926207859093161, -0.3420201433256663259 ) ) ;
#42538=VERTEX_POINT ( 'NONE', #78705 ) ;
#42539=ORIENTED_EDGE ( 'NONE', *, *, #12553, .T. ) ;
#42540=EDGE_CURVE ( 'NONE', #9337, #67157, #81481, .T. ) ;
#42541=ORIENTED_EDGE ( 'NONE', *, *, #31049, .F. ) ;
#42542=ORIENTED_EDGE ( 'NONE', *, *, #18455, .F. ) ;
#42543=CARTESIAN_POINT ( 'NONE',  ( -10.86536135943320502, -12.41104346484419452, 31.60698883733904196 ) ) ;
#42544=CARTESIAN_POINT ( 'NONE',  ( -16.85414353565466783, -3.755027918224367767, 33.06320215134714857 ) ) ;
#42545=CARTESIAN_POINT ( 'NONE',  ( 0.4615384615383382183, -6.835583212225970762, 34.95778746994575670 ) ) ;
#42548=CARTESIAN_POINT ( 'NONE',  ( -7.623374177175779032, -4.226511098958374291, 33.85474049983370293 ) ) ;
#42550=ORIENTED_EDGE ( 'NONE', *, *, #81703, .F. ) ;
#42551=ORIENTED_EDGE ( 'NONE', *, *, #32924, .F. ) ;
#42553=VECTOR ( 'NONE', #10255, 999.9999999999998863 ) ;
#42554=VERTEX_POINT ( 'NONE', #6157 ) ;
#42555=CARTESIAN_POINT ( 'NONE',  ( -3.100243529005665799, -10.88167719472716399, 33.43325721877153711 ) ) ;
#42557=CARTESIAN_POINT ( 'NONE',  ( 16.21910172512217585, -8.613356846314930593, 34.62446782046653482 ) ) ;
#42558=CARTESIAN_POINT ( 'NONE',  ( -8.769230769230890843, -11.48612834414049644, 32.76840700105863391 ) ) ;
#42559=DIRECTION ( 'NONE',  ( 0.000000000000000000, 0.7660444431189807890, 0.6427876096865361433 ) ) ;
#42560=CARTESIAN_POINT ( 'NONE',  ( -10.74553182482283198, -11.93770438780619259, 32.05411857736982029 ) ) ;
#42561=ORIENTED_EDGE ( 'NONE', *, *, #54042, .T. ) ;
#42562=VERTEX_POINT ( 'NONE', #18787 ) ;
#42563=B_SPLINE_CURVE_WITH_KNOTS ( 'NONE', 3,
 ( #25388, #78995, #11432, #86672, #79452, #24938, #59611, #65916, #46105, #17297 ),
 .UNSPECIFIED., .F., .F.,
 ( 4, 2, 2, 2, 4 ),
 ( 0.0007817359430256399806, 0.0009771253907250089001, 0.001172514838424378036, 0.001367904286123746956, 0.001563293733823115875 ),
 .UNSPECIFIED. ) ;
#42564=CARTESIAN_POINT ( 'NONE',  ( 13.63466980452883526, -10.82426656108012075, 33.81400080652039009 ) ) ;
#42565=EDGE_LOOP ( 'NONE', ( #1116, #30127, #83677, #15337 ) ) ;
#42566=FACE_BOUND ( 'NONE', #72964, .T. ) ;
#42567=CARTESIAN_POINT ( 'NONE',  ( -1.254570221780606287, -2.504778602574659896, 29.97347330155780298 ) ) ;
#42570=ORIENTED_EDGE ( 'NONE', *, *, #83868, .T. ) ;
#42571=CARTESIAN_POINT ( 'NONE',  ( 15.16501580245589764, -7.249945578846651806, 34.99404164642496795 ) ) ;
#42572=CARTESIAN_POINT ( 'NONE',  ( 11.28843831424008926, -6.652501968072648708, 34.93155406624980941 ) ) ;
#42573=CARTESIAN_POINT ( 'NONE',  ( 10.61538461538449596, -2.892918686052165622, 31.69288490824153470 ) ) ;
#42574=EDGE_CURVE ( 'NONE', #58249, #55087, #12037, .T. ) ;
#42576=CARTESIAN_POINT ( 'NONE',  ( 1.634560793993428796, -2.589246495874657938, 31.60778113518102828 ) ) ;
#42577=EDGE_LOOP ( 'NONE', ( #33042, #39355 ) ) ;
#42578=CARTESIAN_POINT ( 'NONE',  ( -12.33074802057151409, -2.295524264805589354, 30.44142389570982488 ) ) ;
#42579=CARTESIAN_POINT ( 'NONE',  ( 17.07692307692295586, -12.46129190930018460, 30.37095296980731973 ) ) ;
#42580=DIRECTION ( 'NONE',  ( -0.000000000000000000, -0.8660254037844397068, -0.4999999999999978906 ) ) ;
#42581=CARTESIAN_POINT ( 'NONE',  ( 13.38461538461526423, -2.379036618888197729, 30.90682066428292885 ) ) ;
#42582=FACE_OUTER_BOUND ( 'NONE', #81782, .T. ) ;
#42583=AXIS2_PLACEMENT_3D ( 'NONE', #37582, #52429, #46131 ) ;
#42584=FACE_BOUND ( 'NONE', #59806, .T. ) ;
#42585=CARTESIAN_POINT ( 'NONE',  ( 17.32686859527121825, -3.712312575010499494, 33.01462480002815170 ) ) ;
#42586=CARTESIAN_POINT ( 'NONE',  ( -17.14219307747939069, -11.06231777344663136, 33.60647404775220082 ) ) ;
#42587=EDGE_CURVE ( 'NONE', #16922, #74826, #5844, .T. ) ;
#42588=CARTESIAN_POINT ( 'NONE',  ( 11.76147438255493327, -11.98016756924215009, 32.48728574198911190 ) ) ;
#42589=CARTESIAN_POINT ( 'NONE',  ( -3.480745974817821775, -2.920706130388546651, 32.31842814019191223 ) ) ;
#42590=CARTESIAN_POINT ( 'NONE',  ( -18.00000000000000000, -2.833524468853757305, 32.15551576947926549 ) ) ;
#42591=CYLINDRICAL_SURFACE ( 'NONE', #21780, 0.2499999999999994726 ) ;
#42594=B_SPLINE_CURVE_WITH_KNOTS ( 'NONE', 3,
 ( #31609, #59072, #65820, #59519, #44654, #44207, #71694, #72140, #86571, #50961 ),
 .UNSPECIFIED., .F., .F.,
 ( 4, 2, 2, 2, 4 ),
 ( 0.000000000000000000, 0.0001954339857564126514, 0.0003908679715128183098, 0.0005863019572692239681, 0.0007817359430256294638 ),
 .UNSPECIFIED. ) ;
#42595=CARTESIAN_POINT ( 'NONE',  ( -5.777220331021934108, -10.97394488606064122, 33.68653795673694873 ) ) ;
#42596=ORIENTED_EDGE ( 'NONE', *, *, #83767, .T. ) ;
#42597=EDGE_CURVE ( 'NONE', #34806, #69130, #55779, .T. ) ;
#42598=CARTESIAN_POINT ( 'NONE',  ( 14.30769230769231015, -12.78798330534103123, 29.99999999999997868 ) ) ;
#42599=ORIENTED_EDGE ( 'NONE', *, *, #11324, .T. ) ;
#42600=CARTESIAN_POINT ( 'NONE',  ( -11.47320639894870276, -6.835583212224610072, 34.95778746994559327 ) ) ;
#42601=CARTESIAN_POINT ( 'NONE',  ( -18.24997673094235395, -2.564618984488975961, 30.55390908950641915 ) ) ;
#42602=EDGE_CURVE ( 'NONE', #37879, #65133, #39068, .T. ) ;
#42603=ORIENTED_EDGE ( 'NONE', *, *, #74545, .F. ) ;
#42604=CARTESIAN_POINT ( 'NONE',  ( -18.06608341095587633, -12.37446782046654192, 30.86335684631486487 ) ) ;
#42606=CARTESIAN_POINT ( 'NONE',  ( 6.222779668978068557, -6.717445702608402236, 34.94155399931962336 ) ) ;
#42607=CARTESIAN_POINT ( 'NONE',  ( -10.39237177129122003, -12.64618726649961289, 30.78989965857442712 ) ) ;
#42609=CARTESIAN_POINT ( 'NONE',  ( -5.326899807865431491, -12.41269422305637171, 30.68257228309993323 ) ) ;
#42610=CARTESIAN_POINT ( 'NONE',  ( 0.4615384615383382183, -12.16647553114689728, 32.15551576947799362 ) ) ;
#42611=CARTESIAN_POINT ( 'NONE',  ( -14.08467946359891165, -4.762714258010881885, 34.23016756924214832 ) ) ;
#42613=CARTESIAN_POINT ( 'NONE',  ( -18.24997674404858827, -11.47974371597207899, 33.17467449705390692 ) ) ;
#42614=CARTESIAN_POINT ( 'NONE',  ( 2.307692307692309264, -2.708943851104267164, 35.45975837776705220 ) ) ;
#42615=EDGE_CURVE ( 'NONE', #39647, #56424, #74619, .T. ) ;
#42616=CARTESIAN_POINT ( 'NONE',  ( 8.769230769230647482, -10.21337939537710326, 33.94971097300076224 ) ) ;
#42618=CARTESIAN_POINT ( 'NONE',  ( -15.23076923076922995, -13.49023893513002648, 31.06009739812518688 ) ) ;
#42619=EDGE_LOOP ( 'NONE', ( #51564, #6814, #16961, #75392 ) ) ;
#42620=EDGE_CURVE ( 'NONE', #57617, #79299, #70783, .T. ) ;
#42621=AXIS2_PLACEMENT_3D ( 'NONE', #17917, #37283, #45371 ) ;
#42622=CARTESIAN_POINT ( 'NONE',  ( -17.93474442872397745, -2.892918686051626498, 31.69288490824025928 ) ) ;
#42623=CARTESIAN_POINT ( 'NONE',  ( 15.93091993633000136, -12.15238873228291716, 31.58232369045353849 ) ) ;
#42624=DIRECTION ( 'NONE',  ( -0.000000000000000000, -0.6427876096865404731, -0.7660444431189770143 ) ) ;
#42625=CARTESIAN_POINT ( 'NONE',  ( -8.096153846153844924, -7.500000000000001776, 34.75000000000000000 ) ) ;
#42627=CARTESIAN_POINT ( 'NONE',  ( 13.45068373561782593, -2.538708090699994813, 30.37095296980875503 ) ) ;
#42629=DIRECTION ( 'NONE',  ( 0.000000000000000000, 0.8660254037844377084, -0.5000000000000015543 ) ) ;
#42631=B_SPLINE_CURVE_WITH_KNOTS ( 'NONE', 3,
 ( #3422, #59259, #37654, #65115, #10636, #24587, #3862, #4774, #23690, #31349 ),
 .UNSPECIFIED., .F., .F.,
 ( 4, 2, 2, 2, 4 ),
 ( 0.000000000000000000, 0.0001954339857564079894, 0.0003908679715128159787, 0.0005863019572692239681, 0.0007817359430256319575 ),
 .UNSPECIFIED. ) ;
#42633=B_SPLINE_CURVE_WITH_KNOTS ( 'NONE', 3,
 ( #15813, #7276, #36525, #70303, #521, #22117, #15366, #34742, #76618, #27985 ),
 .UNSPECIFIED., .F., .F.,
 ( 4, 2, 2, 2, 4 ),
 ( 0.000000000000000000, 0.0001954311564186866034, 0.0003908623128373732067, 0.0005862934692560597830, 0.0007817246256747464135 ),
 .UNSPECIFIED. ) ;
#42634=ORIENTED_EDGE ( 'NONE', *, *, #51685, .F. ) ;
#42635=ORIENTED_EDGE ( 'NONE', *, *, #3661, .T. ) ;
#42636=CARTESIAN_POINT ( 'NONE',  ( -9.442253380669379581, -3.136992222400443175, 32.19305428654138979 ) ) ;
#42637=DIRECTION ( 'NONE',  ( -0.000000000000000000, 0.9396926207859093161, -0.3420201433256663259 ) ) ;
#42638=EDGE_CURVE ( 'NONE', #19405, #49519, #901, .T. ) ;
#42639=CARTESIAN_POINT ( 'NONE',  ( 6.673100179028331524, -2.920706130388546651, 32.31842814019191223 ) ) ;
#42640=FACE_OUTER_BOUND ( 'NONE', #67369, .T. ) ;
#42641=LINE ( 'NONE', #21919, #33724 ) ;
#42642=EDGE_LOOP ( 'NONE', ( #51017, #82424 ) ) ;
#42644=VERTEX_POINT ( 'NONE', #68297 ) ;
#42645=ADVANCED_FACE ( 'NONE', ( #69625 ), #34948, .F. ) ;
#42646=ORIENTED_EDGE ( 'NONE', *, *, #5978, .F. ) ;
#42647=ORIENTED_EDGE ( 'NONE', *, *, #81328, .T. ) ;
#42649=VERTEX_POINT ( 'NONE', #6601 ) ;
#42650=CARTESIAN_POINT ( 'NONE',  ( 16.21910172512217585, -12.46129190930001052, 30.37095296980869819 ) ) ;
#42651=EDGE_CURVE ( 'NONE', #42644, #52424, #53542, .T. ) ;
#42652=DIRECTION ( 'NONE',  ( 0.000000000000000000, -6.938893903907222067E-15, 1.000000000000000000 ) ) ;
#42653=EDGE_CURVE ( 'NONE', #47496, #36412, #46052, .T. ) ;
#42654=CARTESIAN_POINT ( 'NONE',  ( 3.903869422903799347, -4.236021600441998380, 33.53823185664189310 ) ) ;
#42655=CARTESIAN_POINT ( 'NONE',  ( -5.326923076923075762, -7.500000000000001776, 34.75000000000000000 ) ) ;
#42656=AXIS2_PLACEMENT_3D ( 'NONE', #61318, #88834, #54570 ) ;
#42657=VERTEX_POINT ( 'NONE', #29104 ) ;
#42658=ORIENTED_EDGE ( 'NONE', *, *, #26181, .F. ) ;
#42660=ORIENTED_EDGE ( 'NONE', *, *, #5670, .F. ) ;
#42661=DIRECTION ( 'NONE',  ( -0.000000000000000000, 0.1736481776669307198, -0.9848077530122080203 ) ) ;
#42662=DIRECTION ( 'NONE',  ( 0.000000000000000000, 0.7660444431189807890, 0.6427876096865361433 ) ) ;
#42663=ORIENTED_EDGE ( 'NONE', *, *, #31567, .T. ) ;
#42664=CARTESIAN_POINT ( 'NONE',  ( 1.384615384615265343, -9.442884908241554243, 34.35708131394783038 ) ) ;
#42665=DIRECTION ( 'NONE',  ( 0.000000000000000000, 0.9396926207859126468, 0.3420201433256571111 ) ) ;
#42666=CARTESIAN_POINT ( 'NONE',  ( -3.007989689500821573, -10.11255958852955850, 34.01340905677048454 ) ) ;
#42667=VERTEX_POINT ( 'NONE', #7930 ) ;
#42668=DIRECTION ( 'NONE',  ( -0.000000000000000000, -0.6427876096865404731, -0.7660444431189770143 ) ) ;
#42669=CARTESIAN_POINT ( 'NONE',  ( -16.15384615384627409, -12.70778746994576025, 30.41441678777401236 ) ) ;
#42671=FACE_BOUND ( 'NONE', #75286, .T. ) ;
#42672=CARTESIAN_POINT ( 'NONE',  ( 11.53846153846153832, -4.786620604624113540, 33.94971097300155094 ) ) ;
#42673=CARTESIAN_POINT ( 'NONE',  ( -18.22292695890684655, -12.38737895849757820, 31.66785238281580206 ) ) ;
#42674=CARTESIAN_POINT ( 'NONE',  ( -11.53846153846153655, -4.098570777380720287, 33.41473453929634729 ) ) ;
#42677=VECTOR ( 'NONE', #47549, 1000.000000000000227 ) ;
#42678=CYLINDRICAL_SURFACE ( 'NONE', #63979, 0.2500000000000008882 ) ;
#42680=VERTEX_POINT ( 'NONE', #28189 ) ;
#42681=CARTESIAN_POINT ( 'NONE',  ( -8.069080805060693251, -6.459968553980841577, 34.89616026154728701 ) ) ;
#42682=DIRECTION ( 'NONE',  ( 0.000000000000000000, 0.9848077530122072432, -0.1736481776669354937 ) ) ;
#42683=EDGE_CURVE ( 'NONE', #8176, #70654, #69185, .T. ) ;
#42684=EDGE_LOOP ( 'NONE', ( #21306, #9932 ) ) ;
#42685=VECTOR ( 'NONE', #2833, 1000.000000000000114 ) ;
#42687=CARTESIAN_POINT ( 'NONE',  ( 8.545745825506822158, -3.236172620538810385, 32.36188796281390267 ) ) ;
#42688=CARTESIAN_POINT ( 'NONE',  ( -4.023054346021367245, -2.541949514083464479, 30.39797389878540557 ) ) ;
#42689=CARTESIAN_POINT ( 'NONE',  ( -5.143006487878958310, -11.69971097300155272, 32.46337939537587403 ) ) ;
#42690=CARTESIAN_POINT ( 'NONE',  ( 6.923076923076924238, -13.57706302396349152, 30.56769352161908060 ) ) ;
#42692=FACE_BOUND ( 'NONE', #70697, .T. ) ;
#42694=CARTESIAN_POINT ( 'NONE',  ( 4.153846153846030731, -12.51329471203414379, 31.30864560766407578 ) ) ;
#42695=AXIS2_PLACEMENT_3D ( 'NONE', #32840, #12573, #61630 ) ;
#42696=CARTESIAN_POINT ( 'NONE',  ( 1.607395053593452694, -12.69155399931963046, 30.53255429739158444 ) ) ;
#42697=CARTESIAN_POINT ( 'NONE',  ( -6.923076923076922462, -10.67929555188718282, 33.92786785259544047 ) ) ;
#42698=CARTESIAN_POINT ( 'NONE',  ( -15.16470087976679437, -6.386643153685127139, 34.62446782046654192 ) ) ;
#42699=DIRECTION ( 'NONE',  ( 1.000000000000000000, 0.000000000000000000, 0.000000000000000000 ) ) ;
#42701=EDGE_LOOP ( 'NONE', ( #38557, #16590, #34609, #83989 ) ) ;
#42702=ORIENTED_EDGE ( 'NONE', *, *, #67426, .F. ) ;
#42703=CARTESIAN_POINT ( 'NONE',  ( 15.90382292962469535, -9.356822207818511927, 34.66110646841856635 ) ) ;
#42704=CARTESIAN_POINT ( 'NONE',  ( -0.5276218724943421146, -2.721908614388772296, 31.22303859784725688 ) ) ;
#42705=CARTESIAN_POINT ( 'NONE',  ( -9.561781990544128362, -9.417988943895561960, 34.36773134775777550 ) ) ;
#42706=CARTESIAN_POINT ( 'NONE',  ( -16.94639737515951694, -11.46989282347013095, 32.79007818306219946 ) ) ;
#42707=B_SPLINE_CURVE_WITH_KNOTS ( 'NONE', 3,
 ( #84402, #50143, #77629, #78070, #23128, #15938, #16373, #60794, #40543, #47726 ),
 .UNSPECIFIED., .F., .F.,
 ( 4, 2, 2, 2, 4 ),
 ( 0.000000000000000000, 0.0001954311564186860071, 0.0003908623128373720141, 0.0005862934692560580483, 0.0007817246256747440282 ),
 .UNSPECIFIED. ) ;
#42708=CARTESIAN_POINT ( 'NONE',  ( -16.82697755857493505, -6.696923467548659303, 34.68552623307873972 ) ) ;
#42710=B_SPLINE_CURVE_WITH_KNOTS ( 'NONE', 3,
 ( #4973, #60793, #76412, #69650, #60348, #87403, #14717, #46395, #88302, #61225 ),
 .UNSPECIFIED., .F., .F.,
 ( 4, 2, 2, 2, 4 ),
 ( 0.0007817359430256218744, 0.0009771253907249859150, 0.001172514838424350064, 0.001367904286123714213, 0.001563293733823078145 ),
 .UNSPECIFIED. ) ;
#42711=CARTESIAN_POINT ( 'NONE',  ( -11.78846153846153832, -7.500000000000001776, 35.00000000000000000 ) ) ;
#42712=DIRECTION ( 'NONE',  ( -0.000000000000000000, -0.000000000000000000, -1.000000000000000000 ) ) ;
#42713=LINE ( 'NONE', #83256, #2924 ) ;
#42714=CARTESIAN_POINT ( 'NONE',  ( -3.099978789802282364, -11.93129842949671726, 32.56571108434900452 ) ) ;
#42715=CARTESIAN_POINT ( 'NONE',  ( -3.453696189676080053, -4.026226216239095379, 33.68668979543632958 ) ) ;
#42716=DIRECTION ( 'NONE',  ( -0.000000000000000000, 1.000000000000000000, -0.000000000000000000 ) ) ;
#42718=DIRECTION ( 'NONE',  ( -0.000000000000000000, -0.8660254037844399289, -0.4999999999999980016 ) ) ;
#42719=EDGE_CURVE ( 'NONE', #13624, #20560, #85772, .T. ) ;
#42720=EDGE_CURVE ( 'NONE', #64611, #10442, #67594, .T. ) ;
#42721=CYLINDRICAL_SURFACE ( 'NONE', #44165, 0.2500000000000009437 ) ;
#42722=VERTEX_POINT ( 'NONE', #48911 ) ;
#42723=CARTESIAN_POINT ( 'NONE',  ( -14.53061852520844965, -3.586966769969701208, 32.86292498521069660 ) ) ;
#42724=DIRECTION ( 'NONE',  ( -0.000000000000000000, -0.5000000000000009992, -0.8660254037844380415 ) ) ;
#42727=LINE ( 'NONE', #30524, #28901 ) ;
#42728=DIRECTION ( 'NONE',  ( -0.000000000000000000, -0.6427876096865404731, -0.7660444431189771253 ) ) ;
#42729=ORIENTED_EDGE ( 'NONE', *, *, #75681, .F. ) ;
#42730=DIRECTION ( 'NONE',  ( -0.000000000000000000, 0.5000000000000011102, -0.8660254037844380415 ) ) ;
#42731=DIRECTION ( 'NONE',  ( -0.000000000000000000, -0.6427876096865404731, -0.7660444431189771253 ) ) ;
#42733=CARTESIAN_POINT ( 'NONE',  ( 9.757562831820528970, -12.70778746994558439, 30.41441678777536595 ) ) ;
#42734=DIRECTION ( 'NONE',  ( 1.000000000000000000, -0.000000000000000000, -0.000000000000000000 ) ) ;
#42737=ORIENTED_EDGE ( 'NONE', *, *, #15179, .T. ) ;
#42738=CARTESIAN_POINT ( 'NONE',  ( -13.16183584334697265, -2.600157965045224451, 30.74683119005207743 ) ) ;
#42740=EDGE_CURVE ( 'NONE', #31080, #66517, #77711, .T. ) ;
#42741=EDGE_LOOP ( 'NONE', ( #915, #30818 ) ) ;
#42742=CYLINDRICAL_SURFACE ( 'NONE', #75114, 0.2499999999999973355 ) ;
#42743=LINE ( 'NONE', #56687, #55178 ) ;
#42744=CYLINDRICAL_SURFACE ( 'NONE', #39843, 0.2499999999999995559 ) ;
#42745=ORIENTED_EDGE ( 'NONE', *, *, #72681, .F. ) ;
#42747=ADVANCED_FACE ( 'NONE', ( #50672 ), #9696, .F. ) ;
#42748=CARTESIAN_POINT ( 'NONE',  ( 6.130525701763564150, -6.852161475712352789, 34.70806712695775786 ) ) ;
#42749=ORIENTED_EDGE ( 'NONE', *, *, #78970, .T. ) ;
#42750=VECTOR ( 'NONE', #75134, 999.9999999999998863 ) ;
#42751=CARTESIAN_POINT ( 'NONE',  ( 15.45354889974729318, -12.69155399931963046, 30.53255429739157734 ) ) ;
#42752=CYLINDRICAL_SURFACE ( 'NONE', #6935, 0.2499999999999995559 ) ;
#42753=EDGE_CURVE ( 'NONE', #36102, #6730, #78157, .T. ) ;
#42754=B_SPLINE_CURVE_WITH_KNOTS ( 'NONE', 3,
 ( #63751, #56992, #84485, #42170, #50223, #9268, #36727, #65073, #3827, #37164 ),
 .UNSPECIFIED., .F., .F.,
 ( 4, 2, 2, 2, 4 ),
 ( 0.000000000000000000, 0.0001954311564186882568, 0.0003908623128373765136, 0.0005862934692560647703, 0.0007817246256747530271 ),
 .UNSPECIFIED. ) ;
#42755=LINE ( 'NONE', #64767, #13597 ) ;
#42756=CARTESIAN_POINT ( 'NONE',  ( -2.307692307692305711, -5.471508081941601098, 34.59228464037088457 ) ) ;
#42757=EDGE_CURVE ( 'NONE', #75394, #27467, #58965, .T. ) ;
#42758=ORIENTED_EDGE ( 'NONE', *, *, #79634, .F. ) ;
#42759=AXIS2_PLACEMENT_3D ( 'NONE', #11927, #39406, #81273 ) ;
#42761=DIRECTION ( 'NONE',  ( 1.000000000000000000, 0.000000000000000000, 0.000000000000000000 ) ) ;
#42762=ORIENTED_EDGE ( 'NONE', *, *, #35172, .T. ) ;
#42763=EDGE_CURVE ( 'NONE', #19730, #42722, #66303, .T. ) ;
#42764=CARTESIAN_POINT ( 'NONE',  ( 16.15384615384645883, -2.506253911140615021, 30.00000000000323297 ) ) ;
#42765=ORIENTED_EDGE ( 'NONE', *, *, #50429, .F. ) ;
#42766=CARTESIAN_POINT ( 'NONE',  ( -17.74994568836168440, -3.136992222400446728, 32.19305428654138268 ) ) ;
#42767=CARTESIAN_POINT ( 'NONE',  ( -8.638705330997126453, -12.70449254468099198, 30.44128974285582956 ) ) ;
#42768=ORIENTED_EDGE ( 'NONE', *, *, #49289, .F. ) ;
#42769=CARTESIAN_POINT ( 'NONE',  ( -16.15384615384627409, -9.442884908241554243, 34.35708131394783038 ) ) ;
#42770=EDGE_CURVE ( 'NONE', #19826, #61245, #82427, .T. ) ;
#42771=ORIENTED_EDGE ( 'NONE', *, *, #20911, .T. ) ;
#42772=CARTESIAN_POINT ( 'NONE',  ( 14.30769230769231015, -13.75783147151868846, 33.36296068462461051 ) ) ;
#42773=ORIENTED_EDGE ( 'NONE', *, *, #70405, .F. ) ;
#42775=CARTESIAN_POINT ( 'NONE',  ( -12.46153846153846168, -8.973038597847269315, 34.52809138561121927 ) ) ;
#42776=EDGE_LOOP ( 'NONE', ( #38522, #70477, #32558, #23004 ) ) ;
#42778=CARTESIAN_POINT ( 'NONE',  ( 15.45354877203763522, -3.236590943229499029, 32.36255958852954251 ) ) ;
#42780=AXIS2_PLACEMENT_3D ( 'NONE', #38431, #18160, #45623 ) ;
#42781=FACE_BOUND ( 'NONE', #43473, .T. ) ;
#42782=CARTESIAN_POINT ( 'NONE',  ( 7.846153846153723244, -12.51329471203414379, 31.30864560766407578 ) ) ;
#42783=CARTESIAN_POINT ( 'NONE',  ( -6.792551484843277976, -9.503571793651733657, 34.60286762892837942 ) ) ;
#42784=CARTESIAN_POINT ( 'NONE',  ( -16.08777882049607655, -4.661471528628508665, 34.16647553114624003 ) ) ;
#42785=CARTESIAN_POINT ( 'NONE',  ( -16.94613263595612906, -12.35292014791297710, 31.75344720912887198 ) ) ;
#42786=CARTESIAN_POINT ( 'NONE',  ( -3.230769230769229949, -10.05456864172156806, 36.03766855953608683 ) ) ;
#42787=CARTESIAN_POINT ( 'NONE',  ( -16.40382289789474157, -2.544273027872574922, 31.48422191005632342 ) ) ;
#42788=VERTEX_POINT ( 'NONE', #10149 ) ;
#42789=VECTOR ( 'NONE', #47816, 1000.000000000000000 ) ;
#42790=CARTESIAN_POINT ( 'NONE',  ( -5.076923076923075762, -1.215029322943914858, 32.30358669280327177 ) ) ;
#42791=ORIENTED_EDGE ( 'NONE', *, *, #76632, .T. ) ;
#42793=VERTEX_POINT ( 'NONE', #15578 ) ;
#42794=CARTESIAN_POINT ( 'NONE',  ( 14.30769230769231015, -3.513871655860378418, 32.76840700105978499 ) ) ;
#42795=CARTESIAN_POINT ( 'NONE',  ( -3.296851610129365007, -5.471508081941601986, 34.59228464037088457 ) ) ;
#42796=EDGE_CURVE ( 'NONE', #2346, #60982, #71840, .T. ) ;
#42797=DIRECTION ( 'NONE',  ( -0.000000000000000000, 1.000000000000000000, 3.491481338843133355E-15 ) ) ;
#42798=B_SPLINE_CURVE_WITH_KNOTS ( 'NONE', 3,
 ( #15878, #22616, #70819, #21285, #64038, #69479, #55959, #1470, #42460, #2335 ),
 .UNSPECIFIED., .F., .F.,
 ( 4, 2, 2, 2, 4 ),
 ( 0.000000000000000000, 0.0001954311564186862239, 0.0003908623128373724478, 0.0005862934692560586988, 0.0007817246256747448956 ),
 .UNSPECIFIED. ) ;
#42799=DIRECTION ( 'NONE',  ( 0.000000000000000000, 0.3420201433256610524, 0.9396926207859113145 ) ) ;
#42800=CARTESIAN_POINT ( 'NONE',  ( -12.39547112818838670, -2.486705287966280320, 31.30864560766543647 ) ) ;
#42801=CARTESIAN_POINT ( 'NONE',  ( 13.60739492588379385, -11.41317474335729543, 32.86274602512330034 ) ) ;
#42802=ADVANCED_FACE ( 'NONE', ( #77269 ), #65526, .F. ) ;
#42803=ORIENTED_EDGE ( 'NONE', *, *, #88896, .F. ) ;
#42804=CARTESIAN_POINT ( 'NONE',  ( 13.38461538461526601, -5.219633306517616589, 34.19971097300220464 ) ) ;
#42807=CARTESIAN_POINT ( 'NONE',  ( 15.36129466900287888, -12.50538340440932394, 31.33453814440721885 ) ) ;
#42809=CARTESIAN_POINT ( 'NONE',  ( -5.076923076923075762, -12.09954503811598769, 35.62045528018868623 ) ) ;
#42810=VERTEX_POINT ( 'NONE', #51544 ) ;
#42811=ORIENTED_EDGE ( 'NONE', *, *, #32277, .F. ) ;
#42812=CARTESIAN_POINT ( 'NONE',  ( -9.469296340694842939, -12.39991518177334129, 30.74647679643404530 ) ) ;
#42813=ORIENTED_EDGE ( 'NONE', *, *, #13208, .F. ) ;
#42814=CARTESIAN_POINT ( 'NONE',  ( -5.076923076923075762, -13.87047571288749737, 32.06866353760679544 ) ) ;
#42815=LINE ( 'NONE', #63509, #54335 ) ;
#42816=CARTESIAN_POINT ( 'NONE',  ( -14.17716660592874689, -6.852161475712352789, 34.70806712695775786 ) ) ;
#42817=CARTESIAN_POINT ( 'NONE',  ( 1.384615384615264011, -4.320704448113951379, 33.92786785259630022 ) ) ;
#42820=VERTEX_POINT ( 'NONE', #2487 ) ;
#42821=CARTESIAN_POINT ( 'NONE',  ( 4.403846153847589484, -7.500000000000155431, 34.75000000000007105 ) ) ;
#42822=CARTESIAN_POINT ( 'NONE',  ( -10.61538461538461320, -2.517432740324522911, 35.29906147534542527 ) ) ;
#42823=EDGE_LOOP ( 'NONE', ( #10826, #49966, #15848, #74814 ) ) ;
#42824=FACE_OUTER_BOUND ( 'NONE', #61615, .T. ) ;
#42825=B_SPLINE_CURVE_WITH_KNOTS ( 'NONE', 3,
 ( #53663, #10903, #81149, #45567, #12235, #46897, #53211, #65828, #5487, #38827 ),
 .UNSPECIFIED., .F., .F.,
 ( 4, 2, 2, 2, 4 ),
 ( 0.000000000000000000, 0.0001954339857564064444, 0.0003908679715128128888, 0.0005863019572692193060, 0.0007817359430256257775 ),
 .UNSPECIFIED. ) ;
#42826=CARTESIAN_POINT ( 'NONE',  ( -17.32694630114453105, -12.07920672191015221, 32.31858351112116168 ) ) ;
#42827=CARTESIAN_POINT ( 'NONE',  ( -17.86920819217521483, -11.71459661697926258, 32.44059661609676937 ) ) ;
#42828=DIRECTION ( 'NONE',  ( -0.000000000000000000, 0.8660254037844399289, -0.4999999999999980016 ) ) ;
#42829=CARTESIAN_POINT ( 'NONE',  ( -12.52680890749923570, -12.46129190929999986, 30.37095296980880832 ) ) ;
#42831=ORIENTED_EDGE ( 'NONE', *, *, #27274, .F. ) ;
#42832=CARTESIAN_POINT ( 'NONE',  ( -15.23076923076935074, -10.21337939537710326, 33.94971097300076224 ) ) ;
#42833=CARTESIAN_POINT ( 'NONE',  ( -5.076923076923075762, -2.708943851104267164, 35.45975837776705220 ) ) ;
#42834=DIRECTION ( 'NONE',  ( -0.000000000000000000, -0.3420201433256694346, -0.9396926207859080948 ) ) ;
#42836=ORIENTED_EDGE ( 'NONE', *, *, #54231, .T. ) ;
#42838=CARTESIAN_POINT ( 'NONE',  ( -16.02305434602136813, -12.11778462344220841, 31.66786338562085135 ) ) ;
#42840=CARTESIAN_POINT ( 'NONE',  ( 2.530705151785703322, -10.77377354290276301, 33.85451476688484718 ) ) ;
#42841=DIRECTION ( 'NONE',  ( 0.000000000000000000, 0.1736481776669267785, -0.9848077530122087975 ) ) ;
#42842=EDGE_CURVE ( 'NONE', #72489, #42562, #11599, .T. ) ;
#42843=EDGE_LOOP ( 'NONE', ( #2611, #37765, #54407, #62146 ) ) ;
#42844=AXIS2_PLACEMENT_3D ( 'NONE', #27961, #41927, #21197 ) ;
#42846=CARTESIAN_POINT ( 'NONE',  ( -3.230769230769351186, -8.613356846316285953, 34.62446782046622218 ) ) ;
#42847=CARTESIAN_POINT ( 'NONE',  ( -15.23076923076922995, -1.466349020453238561, 30.81389545987213907 ) ) ;
#42848=LINE ( 'NONE', #77952, #4829 ) ;
#42849=ORIENTED_EDGE ( 'NONE', *, *, #82926, .T. ) ;
#42850=EDGE_CURVE ( 'NONE', #12394, #70222, #78095, .T. ) ;
#42851=CARTESIAN_POINT ( 'NONE',  ( -3.165514091256391271, -2.379036618887895305, 30.90682066428159303 ) ) ;
#42852=AXIS2_PLACEMENT_3D ( 'NONE', #59043, #65794, #4094 ) ;
#42854=CARTESIAN_POINT ( 'NONE',  ( -17.75005459062195712, -12.07971442181322352, 32.31769673815850297 ) ) ;
#42855=CARTESIAN_POINT ( 'NONE',  ( 6.249999999999937828, -7.565270445406050648, 34.75000000000000000 ) ) ;
#42856=VERTEX_POINT ( 'NONE', #5612 ) ;
#42857=AXIS2_PLACEMENT_3D ( 'NONE', #50461, #78380, #16684 ) ;
#42858=CYLINDRICAL_SURFACE ( 'NONE', #37533, 0.2499999999999994726 ) ;
#42859=CARTESIAN_POINT ( 'NONE',  ( -14.30769230769230660, -2.292212530054420494, 30.41441678777542634 ) ) ;
#42860=CARTESIAN_POINT ( 'NONE',  ( -3.903846153846149303, -2.499999999999999112, 29.81604066197450109 ) ) ;
#42862=FACE_OUTER_BOUND ( 'NONE', #37580, .T. ) ;
#42864=ORIENTED_EDGE ( 'NONE', *, *, #7080, .F. ) ;
#42865=ORIENTED_EDGE ( 'NONE', *, *, #47833, .T. ) ;
#42866=FACE_BOUND ( 'NONE', #36405, .T. ) ;
#42867=EDGE_LOOP ( 'NONE', ( #72882, #72542 ) ) ;
#42868=CARTESIAN_POINT ( 'NONE',  ( 15.48071474911737333, -2.587454068350148351, 30.68340429815432202 ) ) ;
#42869=EDGE_CURVE ( 'NONE', #30240, #84116, #66425, .T. ) ;
#42872=CARTESIAN_POINT ( 'NONE',  ( 17.74997677577853850, -5.765609946408405406, 34.70566812827424741 ) ) ;
#42873=CARTESIAN_POINT ( 'NONE',  ( 0.5267936010512993539, -12.70778746994558439, 30.41441678777537305 ) ) ;
#42874=B_SPLINE_CURVE_WITH_KNOTS ( 'NONE', 3,
 ( #51219, #72405, #44477, #3501, #30971, #38182, #58436, #65640, #39540, #80968 ),
 .UNSPECIFIED., .F., .F.,
 ( 4, 2, 2, 2, 4 ),
 ( 0.0007817359430256252354, 0.0009771253907249898181, 0.001172514838424354401, 0.001367904286123718983, 0.001563293733823083566 ),
 .UNSPECIFIED. ) ;
#42875=ORIENTED_EDGE ( 'NONE', *, *, #35630, .F. ) ;
#42877=ORIENTED_EDGE ( 'NONE', *, *, #61807, .F. ) ;
#42878=ORIENTED_EDGE ( 'NONE', *, *, #57128, .T. ) ;
#42879=CARTESIAN_POINT ( 'NONE',  ( -10.86536135943320502, -8.347322224742351082, 34.93158281831414058 ) ) ;
#42880=EDGE_LOOP ( 'NONE', ( #15817, #61128, #87535, #37127 ) ) ;
#42882=AXIS2_PLACEMENT_3D ( 'NONE', #59230, #40749, #66883 ) ;
#42883=CARTESIAN_POINT ( 'NONE',  ( -17.07692307692307665, -13.37000171582298513, 34.34916445242398453 ) ) ;
#42884=CARTESIAN_POINT ( 'NONE',  ( 16.94623247381276698, -3.338472653186243200, 32.95098750199972670 ) ) ;
#42885=CARTESIAN_POINT ( 'NONE',  ( 13.44987052412822059, -11.67786785259547777, 32.92929555188713664 ) ) ;
#42886=VERTEX_POINT ( 'NONE', #81283 ) ;
#42887=CARTESIAN_POINT ( 'NONE',  ( 12.46153846153833911, -9.528491918059723176, 34.59228464037033035 ) ) ;
#42889=CARTESIAN_POINT ( 'NONE',  ( 3.903822929624694904, -2.588893531581426544, 31.60682220781847818 ) ) ;
#42890=CARTESIAN_POINT ( 'NONE',  ( -1.384615384615506484, -3.083524468854526912, 32.58852847137268327 ) ) ;
#42891=ORIENTED_EDGE ( 'NONE', *, *, #69579, .T. ) ;
#42892=ORIENTED_EDGE ( 'NONE', *, *, #58544, .T. ) ;
#42893=EDGE_CURVE ( 'NONE', #19715, #78412, #87161, .T. ) ;
#42894=ORIENTED_EDGE ( 'NONE', *, *, #50794, .T. ) ;
#42895=DIRECTION ( 'NONE',  ( 0.000000000000000000, 0.000000000000000000, 1.000000000000000000 ) ) ;
#42896=CARTESIAN_POINT ( 'NONE',  ( 12.33084699487090319, -6.413092428213692742, 34.63065189839063152 ) ) ;
#42898=CARTESIAN_POINT ( 'NONE',  ( -18.00000000000012079, -5.941354392335914447, 34.76329471203413846 ) ) ;
#42899=CARTESIAN_POINT ( 'NONE',  ( -2.084679463598911209, -2.523321265292116422, 31.42251411153756990 ) ) ;
#42900=EDGE_CURVE ( 'NONE', #41883, #75445, #87874, .T. ) ;
#42901=FACE_BOUND ( 'NONE', #25222, .T. ) ;
#42902=CARTESIAN_POINT ( 'NONE',  ( 9.758376043310132530, -3.513871655860379306, 32.76840700105978499 ) ) ;
#42903=EDGE_CURVE ( 'NONE', #27494, #47764, #7290, .T. ) ;
#42904=ORIENTED_EDGE ( 'NONE', *, *, #36849, .F. ) ;
#42905=CARTESIAN_POINT ( 'NONE',  ( -3.100243529005667575, -2.619367082507848998, 30.83698974864644171 ) ) ;
#42906=CARTESIAN_POINT ( 'NONE',  ( 18.00000000000000000, -13.20930481340135110, 34.54067556320372745 ) ) ;
#42907=CARTESIAN_POINT ( 'NONE',  ( -12.46153846153846168, -12.78798330534102767, 29.49999999999997868 ) ) ;
#42909=VERTEX_POINT ( 'NONE', #80846 ) ;
#42910=ADVANCED_FACE ( 'NONE', ( #12373 ), #74514, .F. ) ;
#42911=CARTESIAN_POINT ( 'NONE',  ( 5.076923076922953193, -12.70778746994576025, 30.41441678777401236 ) ) ;
#42912=ADVANCED_FACE ( 'NONE', ( #60994 ), #31760, .F. ) ;
#42913=B_SPLINE_CURVE_WITH_KNOTS ( 'NONE', 3,
 ( #12591, #80617, #40516, #67534, #19786, #47697, #5392, #54007, #13468, #87831 ),
 .UNSPECIFIED., .F., .F.,
 ( 4, 2, 2, 2, 4 ),
 ( 0.0007817359430256390048, 0.0009771253907250075990, 0.001172514838424376085, 0.001367904286123744571, 0.001563293733823113056 ),
 .UNSPECIFIED. ) ;
#42914=ORIENTED_EDGE ( 'NONE', *, *, #87978, .F. ) ;
#42915=FACE_BOUND ( 'NONE', #41761, .T. ) ;
#42916=CARTESIAN_POINT ( 'NONE',  ( 18.13079180782478872, -3.530189275343204702, 32.79018710029569661 ) ) ;
#42917=CARTESIAN_POINT ( 'NONE',  ( 4.403900573759607973, -2.544122305571457687, 31.48381861865059150 ) ) ;
#42918=CARTESIAN_POINT ( 'NONE',  ( -3.230769230769229949, -8.120952969808772792, 34.71129190930000163 ) ) ;
#42919=ORIENTED_EDGE ( 'NONE', *, *, #38013, .F. ) ;
#42920=CARTESIAN_POINT ( 'NONE',  ( 5.142991427925514891, -3.050289026998446840, 32.03036669348366416 ) ) ;
#42921=CARTESIAN_POINT ( 'NONE',  ( -3.454254155333561283, -2.353723527008296568, 30.78948104536958752 ) ) ;
#42922=CARTESIAN_POINT ( 'NONE',  ( 8.769230769230645706, -8.656820664282941280, 34.87096338111179961 ) ) ;
#42923=CARTESIAN_POINT ( 'NONE',  ( 3.230769230769231726, -1.790695186598648903, 34.54067556320373455 ) ) ;
#42924=ORIENTED_EDGE ( 'NONE', *, *, #53086, .T. ) ;
#42925=CARTESIAN_POINT ( 'NONE',  ( -4.153846153846152411, -6.386643153685126251, 34.62446782046654192 ) ) ;
#42927=DIRECTION ( 'NONE',  ( -0.000000000000000000, 0.3420201433256694901, -0.9396926207859082059 ) ) ;
#42928=EDGE_LOOP ( 'NONE', ( #81413, #19249, #68980, #28720 ) ) ;
#42929=CARTESIAN_POINT ( 'NONE',  ( 11.53846153846141753, -6.879047030192662504, 34.71129190930017927 ) ) ;
#42930=CARTESIAN_POINT ( 'NONE',  ( -10.74607608205217346, -12.38065189839062263, 30.83690757178629482 ) ) ;
#42931=CARTESIAN_POINT ( 'NONE',  ( 7.846153846153723244, -10.33852847137269571, 34.16647553114546554 ) ) ;
#42932=CARTESIAN_POINT ( 'NONE',  ( -15.48076923076922995, -7.500000000000001776, 35.00000000000000000 ) ) ;
#42933=CARTESIAN_POINT ( 'NONE',  ( -2.980823821391186623, -4.176053281294514363, 33.81426240980091791 ) ) ;
#42934=CARTESIAN_POINT ( 'NONE',  ( 8.519207545009310323, -4.175268141568685643, 33.81360843649122216 ) ) ;
#42935=CARTESIAN_POINT ( 'NONE',  ( -17.07692307692307665, -13.95598074871891292, 31.83374038241031911 ) ) ;
#42937=ORIENTED_EDGE ( 'NONE', *, *, #12816, .T. ) ;
#42938=DIRECTION ( 'NONE',  ( 0.000000000000000000, 0.4999999999999960032, -0.8660254037844410391 ) ) ;
#42940=ORIENTED_EDGE ( 'NONE', *, *, #36401, .F. ) ;
#42942=ORIENTED_EDGE ( 'NONE', *, *, #51046, .T. ) ;
#42943=VERTEX_POINT ( 'NONE', #27650 ) ;
#42944=FACE_OUTER_BOUND ( 'NONE', #85967, .T. ) ;
#42945=CARTESIAN_POINT ( 'NONE',  ( 6.130525701763564150, -11.46989282347013095, 32.79007818306219946 ) ) ;
#42947=CARTESIAN_POINT ( 'NONE',  ( 0.2115384615384615641, -7.500000000000001776, 35.00000000000000000 ) ) ;
#42948=CARTESIAN_POINT ( 'NONE',  ( 10.74617505635156611, -6.369690395747422684, 34.87708834333098196 ) ) ;
#42949=CARTESIAN_POINT ( 'NONE',  ( -8.899921372341076165, -2.494641256782728966, 31.33461815524612959 ) ) ;
#42950=CARTESIAN_POINT ( 'NONE',  ( -12.46153846153846168, -2.486705287966279876, 31.30864560766543647 ) ) ;
#42951=VECTOR ( 'NONE', #21203, 1000.000000000000114 ) ;
#42952=CARTESIAN_POINT ( 'NONE',  ( 1.384615384615264011, -12.70778746994576025, 30.41441678777401236 ) ) ;
#42953=LINE ( 'NONE', #49698, #3147 ) ;
#42954=CARTESIAN_POINT ( 'NONE',  ( 11.53846153846141753, -10.90142922262034020, 33.41473453929536674 ) ) ;
#42956=DIRECTION ( 'NONE',  ( -0.000000000000000000, 0.8660254037844397068, -0.4999999999999978906 ) ) ;
#42957=CARTESIAN_POINT ( 'NONE',  ( 7.846153846153723244, -9.528491918059723176, 34.59228464037033035 ) ) ;
#42958=ORIENTED_EDGE ( 'NONE', *, *, #82498, .F. ) ;
#42960=CARTESIAN_POINT ( 'NONE',  ( 8.992010438208827949, -3.020022701398814569, 32.48759521482552515 ) ) ;
#42963=CARTESIAN_POINT ( 'NONE',  ( -2.057692307690870415, -7.500000000000155431, 34.75000000000007105 ) ) ;
#42964=VERTEX_POINT ( 'NONE', #20458 ) ;
#42966=CARTESIAN_POINT ( 'NONE',  ( -10.68146699474474914, -12.62096338111211580, 30.90682066428152908 ) ) ;
#42967=CARTESIAN_POINT ( 'NONE',  ( -12.21159294319032185, -10.76462480002816235, 33.53768742498949962 ) ) ;
#42968=ORIENTED_EDGE ( 'NONE', *, *, #63050, .T. ) ;
#42969=CARTESIAN_POINT ( 'NONE',  ( 0.5920641633020238270, -6.001044277235011215, 34.52024696741798948 ) ) ;
#42970=EDGE_LOOP ( 'NONE', ( #70390, #66366, #46741, #28809 ) ) ;
#42972=CARTESIAN_POINT ( 'NONE',  ( 10.83839596699746544, -8.239487800360276282, 34.69522927552633718 ) ) ;
#42973=EDGE_CURVE ( 'NONE', #84284, #88629, #61989, .T. ) ;
#42974=CARTESIAN_POINT ( 'NONE',  ( 8.835298102580845025, -9.058645607665452459, 34.76329471203371924 ) ) ;
#42975=LINE ( 'NONE', #70448, #31547 ) ;
#42976=CARTESIAN_POINT ( 'NONE',  ( -9.561782254074051579, -6.808710257144161559, 34.95449254468098843 ) ) ;
#42977=CARTESIAN_POINT ( 'NONE',  ( 15.23076923076911093, -6.026961402154118019, 34.52809138561165270 ) ) ;
#42978=EDGE_LOOP ( 'NONE', ( #27307, #63158, #65239, #5051 ) ) ;
#42979=ORIENTED_EDGE ( 'NONE', *, *, #55361, .F. ) ;
#42980=ORIENTED_EDGE ( 'NONE', *, *, #9040, .T. ) ;
#42981=EDGE_CURVE ( 'NONE', #39647, #7402, #22269, .T. ) ;
#42982=CARTESIAN_POINT ( 'NONE',  ( -6.223484943723947005, -11.41268669641500466, 32.86336882939237825 ) ) ;
#42984=CARTESIAN_POINT ( 'NONE',  ( -4.219928533206290133, -12.34228464037088280, 31.77849191805838558 ) ) ;
#42985=CARTESIAN_POINT ( 'NONE',  ( -2.176901866725354573, -11.37503395064541678, 33.29242100308974983 ) ) ;
#42986=CARTESIAN_POINT ( 'NONE',  ( -7.623141002060451754, -4.026326845037962343, 33.68677907613344047 ) ) ;
#42987=CARTESIAN_POINT ( 'NONE',  ( 14.55763782604044998, -10.05730279482229683, 34.04704008940765902 ) ) ;
#42988=ORIENTED_EDGE ( 'NONE', *, *, #88145, .F. ) ;
#42989=EDGE_LOOP ( 'NONE', ( #7642, #11717, #82648, #64922 ) ) ;
#42991=VECTOR ( 'NONE', #1994, 999.9999999999998863 ) ;
#42992=CARTESIAN_POINT ( 'NONE',  ( 4.219101293358989757, -4.320704448112861584, 33.92786785259548310 ) ) ;
#42993=ORIENTED_EDGE ( 'NONE', *, *, #18407, .F. ) ;
#42994=CARTESIAN_POINT ( 'NONE',  ( 8.992242120843616959, -8.239487800360276282, 34.69522927552633718 ) ) ;
#42995=CARTESIAN_POINT ( 'NONE',  ( 13.60739505359345536, -4.226511098958373402, 33.85474049983370293 ) ) ;
#42996=VECTOR ( 'NONE', #10150, 1000.000000000000227 ) ;
#42997=EDGE_CURVE ( 'NONE', #68861, #40709, #82620, .T. ) ;
#42999=EDGE_CURVE ( 'NONE', #14363, #69353, #14450, .T. ) ;
#43000=VERTEX_POINT ( 'NONE', #21781 ) ;
#43001=VECTOR ( 'NONE', #79576, 999.9999999999998863 ) ;
#43002=VERTEX_POINT ( 'NONE', #55559 ) ;
#43003=CARTESIAN_POINT ( 'NONE',  ( 4.153846153846030731, -4.320704448113951379, 33.92786785259630022 ) ) ;
#43005=FACE_BOUND ( 'NONE', #75583, .T. ) ;
#43006=CARTESIAN_POINT ( 'NONE',  ( -2.084912638714239819, -4.989023458446561143, 34.36081565061822118 ) ) ;
#43007=CYLINDRICAL_SURFACE ( 'NONE', #37636, 0.2500000000000002220 ) ;
#43008=ORIENTED_EDGE ( 'NONE', *, *, #66434, .T. ) ;
#43009=CARTESIAN_POINT ( 'NONE',  ( 14.98076923076923350, -7.433932668274256805, 35.00000000000000711 ) ) ;
#43012=ADVANCED_FACE ( 'NONE', ( #76727 ), #7392, .F. ) ;
#43013=CARTESIAN_POINT ( 'NONE',  ( -15.48074596171158390, -6.567427716900048118, 34.66269422305636283 ) ) ;
#43014=CARTESIAN_POINT ( 'NONE',  ( -16.82686876528476105, -2.564540009722896752, 30.55348353981672105 ) ) ;
#43015=EDGE_LOOP ( 'NONE', ( #88321, #64847, #17378, #81153 ) ) ;
#43017=CARTESIAN_POINT ( 'NONE',  ( 3.453780582382080411, -4.187068189119697692, 33.49521262558774026 ) ) ;
#43018=CARTESIAN_POINT ( 'NONE',  ( -6.673076923076923350, -2.249999999999998668, 29.75000000000000355 ) ) ;
#43019=CARTESIAN_POINT ( 'NONE',  ( 5.934729554039226862, -5.219633306516282545, 34.19971097300152252 ) ) ;
#43020=DIRECTION ( 'NONE',  ( -0.000000000000000000, 0.7660444431189791237, -0.6427876096865379196 ) ) ;
#43021=CARTESIAN_POINT ( 'NONE',  ( 6.000000000000001776, -9.780366693483667717, 34.19971097300155094 ) ) ;
#43022=CARTESIAN_POINT ( 'NONE',  ( -1.384615384615506484, -6.835583212225970762, 34.95778746994575670 ) ) ;
#43023=CARTESIAN_POINT ( 'NONE',  ( 11.76147289007438701, -4.187068189119697692, 33.49521262558774026 ) ) ;
#43024=CARTESIAN_POINT ( 'NONE',  ( 16.15384615384615330, -8.564572088678739092, 35.78748833219616898 ) ) ;
#43025=CARTESIAN_POINT ( 'NONE',  ( 3.480769230770666578, -7.500000000000155431, 34.75000000000007105 ) ) ;
#43026=CARTESIAN_POINT ( 'NONE',  ( 15.36156103859402222, -9.804649428959608670, 34.18742332936588468 ) ) ;
#43027=CARTESIAN_POINT ( 'NONE',  ( -2.557715531913763662, -5.765609946408404518, 34.70566812827425451 ) ) ;
#43028=B_SPLINE_CURVE_WITH_KNOTS ( 'NONE', 3,
 ( #22162, #36131, #42884, #64453, #49630, #9522, #36563, #63131, #2753, #77103 ),
 .UNSPECIFIED., .F., .F.,
 ( 4, 2, 2, 2, 4 ),
 ( 0.000000000000000000, 0.0001954311564186862510, 0.0003908623128373725020, 0.0005862934692560588072, 0.0007817246256747450040 ),
 .UNSPECIFIED. ) ;
#43029=AXIS2_PLACEMENT_3D ( 'NONE', #51521, #64601, #2899 ) ;
#43031=ORIENTED_EDGE ( 'NONE', *, *, #42323, .F. ) ;
#43032=CARTESIAN_POINT ( 'NONE',  ( -4.088591014333315066, -5.941354392334606160, 34.76329471203374055 ) ) ;
#43033=ORIENTED_EDGE ( 'NONE', *, *, #14588, .T. ) ;
#43035=ORIENTED_EDGE ( 'NONE', *, *, #24163, .T. ) ;
#43036=CARTESIAN_POINT ( 'NONE',  ( -13.31854805126531005, -2.292212530054420494, 30.41441678777542990 ) ) ;
#43037=CARTESIAN_POINT ( 'NONE',  ( 17.20771351789003489, -2.845873456487966635, 32.17976146951972538 ) ) ;
#43039=FACE_OUTER_BOUND ( 'NONE', #59521, .T. ) ;
#43041=CARTESIAN_POINT ( 'NONE',  ( 6.249945409378045547, -6.653508905675592722, 34.93172785388651391 ) ) ;
#43042=B_SPLINE_CURVE_WITH_KNOTS ( 'NONE', 3,
 ( #10825, #38297, #24319, #44585, #9926, #72070, #43712, #3610, #2711, #23870 ),
 .UNSPECIFIED., .F., .F.,
 ( 4, 2, 2, 2, 4 ),
 ( 0.0007817246256747457630, 0.0009771112852218887673, 0.001172497944769031880, 0.001367884604316174993, 0.001563271263863318106 ),
 .UNSPECIFIED. ) ;
#43043=CARTESIAN_POINT ( 'NONE',  ( -3.230769230769229949, -12.34228464037088635, 31.77849191805839268 ) ) ;
#43044=DIRECTION ( 'NONE',  ( 0.000000000000000000, 0.8660254037844377084, 0.5000000000000015543 ) ) ;
#43046=CARTESIAN_POINT ( 'NONE',  ( 15.29591501010119892, -7.750023238201979581, 34.74374492549440419 ) ) ;
#43047=LINE ( 'NONE', #1619, #41083 ) ;
#43050=FACE_OUTER_BOUND ( 'NONE', #81163, .T. ) ;
#43051=CARTESIAN_POINT ( 'NONE',  ( 13.38461538461538680, -4.098570777380720287, 33.41473453929634729 ) ) ;
#43053=AXIS2_PLACEMENT_3D ( 'NONE', #47220, #74715, #13001 ) ;
#43054=CARTESIAN_POINT ( 'NONE',  ( 16.15384615384615330, -6.189225973068211317, 35.74407628777942847 ) ) ;
#43055=AXIS2_PLACEMENT_3D ( 'NONE', #26478, #4880, #73786 ) ;
#43056=ORIENTED_EDGE ( 'NONE', *, *, #22904, .T. ) ;
#43058=CARTESIAN_POINT ( 'NONE',  ( 16.02315468717859304, -12.11776431015576172, 31.66791131148498906 ) ) ;
#43059=CARTESIAN_POINT ( 'NONE',  ( 1.253923917947828537, -12.38065189839062263, 30.83690757178629482 ) ) ;
#43061=CARTESIAN_POINT ( 'NONE',  ( -2.980714919130914353, -4.943051570960395047, 34.04725096376909477 ) ) ;
#43062=ADVANCED_FACE ( 'NONE', ( #628 ), #15031, .F. ) ;
#43063=CARTESIAN_POINT ( 'NONE',  ( -8.834501215191545853, -8.613356846314824011, 34.62446782046655613 ) ) ;
#43065=DIRECTION ( 'NONE',  ( 1.000000000000000000, 0.000000000000000000, 0.000000000000000000 ) ) ;
#43066=B_SPLINE_CURVE_WITH_KNOTS ( 'NONE', 3,
 ( #83295, #63886, #35093, #2185, #62554, #22028, #29676, #49503, #35548, #82855 ),
 .UNSPECIFIED., .F., .F.,
 ( 4, 2, 2, 2, 4 ),
 ( 0.0007817246256747478229, 0.0009771112852218913694, 0.001172497944769034916, 0.001367884604316178679, 0.001563271263863322226 ),
 .UNSPECIFIED. ) ;
#43067=EDGE_LOOP ( 'NONE', ( #10461, #56763, #41636, #28459 ) ) ;
#43068=EDGE_LOOP ( 'NONE', ( #76192, #40892 ) ) ;
#43069=ORIENTED_EDGE ( 'NONE', *, *, #34266, .F. ) ;
#43070=EDGE_CURVE ( 'NONE', #4983, #58791, #42504, .T. ) ;
#43071=CARTESIAN_POINT ( 'NONE',  ( 3.230769230769110045, -6.026961402154118908, 34.52809138561165270 ) ) ;
#43072=CARTESIAN_POINT ( 'NONE',  ( 6.700150705560778519, -2.758268499246657957, 31.33685645148948140 ) ) ;
#43073=CARTESIAN_POINT ( 'NONE',  ( 16.37685750545900731, -2.758310577978207778, 31.33698337089302299 ) ) ;
#43074=EDGE_CURVE ( 'NONE', #79653, #88101, #10479, .T. ) ;
#43075=CARTESIAN_POINT ( 'NONE',  ( 4.403791672194295792, -3.712312575010499494, 33.01462480002815170 ) ) ;
#43076=CARTESIAN_POINT ( 'NONE',  ( 17.99999999999987566, -9.442884908241554243, 34.35708131394783038 ) ) ;
#43077=ORIENTED_EDGE ( 'NONE', *, *, #19375, .F. ) ;
#43078=CARTESIAN_POINT ( 'NONE',  ( -8.769230769230768274, -2.900454961884010974, 35.62045528018868623 ) ) ;
#43079=ORIENTED_EDGE ( 'NONE', *, *, #60289, .T. ) ;
#43081=ADVANCED_FACE ( 'NONE', ( #75401 ), #14581, .F. ) ;
#43082=CARTESIAN_POINT ( 'NONE',  ( -15.23076923076935074, -9.442884908241554243, 34.35708131394783038 ) ) ;
#43083=ORIENTED_EDGE ( 'NONE', *, *, #39924, .T. ) ;
#43084=FACE_OUTER_BOUND ( 'NONE', #62461, .T. ) ;
#43085=VECTOR ( 'NONE', #63936, 1000.000000000000000 ) ;
#43086=CARTESIAN_POINT ( 'NONE',  ( -10.36538461538317790, -7.500000000000155431, 34.75000000000007105 ) ) ;
#43087=EDGE_CURVE ( 'NONE', #148, #84960, #47106, .T. ) ;
#43088=CARTESIAN_POINT ( 'NONE',  ( 3.903822916553187472, -4.335965774309649134, 33.62209801155881905 ) ) ;
#43089=CARTESIAN_POINT ( 'NONE',  ( -16.02305571287920216, -5.496552790871120031, 34.60292014791297532 ) ) ;
#43090=ORIENTED_EDGE ( 'NONE', *, *, #45271, .F. ) ;
#43091=EDGE_LOOP ( 'NONE', ( #23484, #45273 ) ) ;
#43092=ORIENTED_EDGE ( 'NONE', *, *, #40652, .T. ) ;
#43093=DIRECTION ( 'NONE',  ( -0.000000000000000000, 0.1736481776669307198, -0.9848077530122080203 ) ) ;
#43094=CARTESIAN_POINT ( 'NONE',  ( 4.219914504848592429, -11.16473453929635440, 33.15142922261926373 ) ) ;
#43095=EDGE_LOOP ( 'NONE', ( #53924, #15728, #52939, #18063 ) ) ;
#43096=B_SPLINE_CURVE_WITH_KNOTS ( 'NONE', 3,
 ( #52053, #38555, #66009, #86765, #52497, #79983, #18282, #45750, #39012, #4775 ),
 .UNSPECIFIED., .F., .F.,
 ( 4, 2, 2, 2, 4 ),
 ( 0.000000000000000000, 0.0001954339857564080707, 0.0003908679715128161414, 0.0005863019572692241849, 0.0007817359430256322827 ),
 .UNSPECIFIED. ) ;
#43097=CARTESIAN_POINT ( 'NONE',  ( 1.634669696253702176, -9.148310452688873440, 34.47095581063188519 ) ) ;
#43098=CARTESIAN_POINT ( 'NONE',  ( 4.946231610255514610, -3.530157926970578508, 32.79014554554150607 ) ) ;
#43099=B_SPLINE_CURVE_WITH_KNOTS ( 'NONE', 3,
 ( #58416, #17898, #45804, #58875, #46256, #59320, #52556, #45355, #11588, #37714 ),
 .UNSPECIFIED., .F., .F.,
 ( 4, 2, 2, 2, 4 ),
 ( 0.0007817359430256297891, 0.0009771253907249958896, 0.001172514838424362207, 0.001367904286123728524, 0.001563293733823094625 ),
 .UNSPECIFIED. ) ;
#43100=DIRECTION ( 'NONE',  ( 0.000000000000000000, 0.9396926207859126468, 0.3420201433256571111 ) ) ;
#43101=ADVANCED_FACE ( 'NONE', ( #29872 ), #15477, .F. ) ;
#43104=DIRECTION ( 'NONE',  ( -0.000000000000000000, -0.9848077530122086864, -0.1736481776669273613 ) ) ;
#43105=CYLINDRICAL_SURFACE ( 'NONE', #10898, 0.2499999999999998890 ) ;
#43106=VERTEX_POINT ( 'NONE', #85258 ) ;
#43107=FACE_BOUND ( 'NONE', #79784, .T. ) ;
#43108=CARTESIAN_POINT ( 'NONE',  ( 11.47319109250076430, -5.219633306516282545, 34.19971097300152962 ) ) ;
#43110=CARTESIAN_POINT ( 'NONE',  ( 2.177544337960610754, -12.50552854090298993, 31.33409797877408920 ) ) ;
#43112=VECTOR ( 'NONE', #24077, 1000.000000000000114 ) ;
#43113=CARTESIAN_POINT ( 'NONE',  ( -10.61538461538473577, -5.941354392335915335, 34.76329471203413846 ) ) ;
#43114=EDGE_CURVE ( 'NONE', #48549, #58504, #28999, .T. ) ;
#43115=CARTESIAN_POINT ( 'NONE',  ( -1.319360245102545015, -8.656820664281605460, 34.87096338111211224 ) ) ;
#43116=CARTESIAN_POINT ( 'NONE',  ( -4.283994123577851809, -11.04286588640298561, 33.62463336215343901 ) ) ;
#43117=ORIENTED_EDGE ( 'NONE', *, *, #80323, .F. ) ;
#43119=CARTESIAN_POINT ( 'NONE',  ( -18.13014720943822056, -10.88202310037936194, 33.43294751532457099 ) ) ;
#43120=CARTESIAN_POINT ( 'NONE',  ( -17.01166793741023042, -6.835583212224605631, 34.95778746994559327 ) ) ;
#43122=VERTEX_POINT ( 'NONE', #10029 ) ;
#43123=AXIS2_PLACEMENT_3D ( 'NONE', #32459, #54052, #80667 ) ;
#43125=CARTESIAN_POINT ( 'NONE',  ( -12.21148404162501144, -3.435999193479609914, 33.07426656108010832 ) ) ;
#43127=CARTESIAN_POINT ( 'NONE',  ( 15.90382292962469535, -6.652501968072647820, 34.93155406624980941 ) ) ;
#43128=CARTESIAN_POINT ( 'NONE',  ( -7.780898706641008467, -11.06231777344671130, 33.60647404775212976 ) ) ;
#43129=DIRECTION ( 'NONE',  ( -0.000000000000000000, 0.8660254037844399289, -0.4999999999999980016 ) ) ;
#43130=CARTESIAN_POINT ( 'NONE',  ( -4.153846153846274980, -2.379036618888197729, 30.90682066428292885 ) ) ;
#43131=FACE_BOUND ( 'NONE', #73292, .T. ) ;
#43132=CARTESIAN_POINT ( 'NONE',  ( -2.557669038634660108, -6.567427716900047230, 34.66269422305636283 ) ) ;
#43133=CARTESIAN_POINT ( 'NONE',  ( 1.607394925883794068, -2.600157965045225783, 30.74683119005207743 ) ) ;
#43134=FACE_OUTER_BOUND ( 'NONE', #54921, .T. ) ;
#43135=CARTESIAN_POINT ( 'NONE',  ( -17.74994568836168440, -11.28795663066794575, 33.01431243580655206 ) ) ;
#43136=CARTESIAN_POINT ( 'NONE',  ( -14.98071491913091791, -6.567000820036036579, 34.66262288849541306 ) ) ;
#43139=ORIENTED_EDGE ( 'NONE', *, *, #51201, .F. ) ;
#43140=ORIENTED_EDGE ( 'NONE', *, *, #81102, .T. ) ;
#43141=CARTESIAN_POINT ( 'NONE',  ( 5.299934428535925335, -6.503523203565942268, 34.64991518177335195 ) ) ;
#43142=CARTESIAN_POINT ( 'NONE',  ( -4.826977558574935045, -3.202959910592335202, 32.30730279482227019 ) ) ;
#43143=CARTESIAN_POINT ( 'NONE',  ( 5.777073041093152561, -5.582147617184174848, 34.63737895849758530 ) ) ;
#43144=CARTESIAN_POINT ( 'NONE',  ( 8.769230769231082689, -2.255955759149395501, 30.00000000000324363 ) ) ;
#43145=CARTESIAN_POINT ( 'NONE',  ( -4.153846153846152411, -2.833524468853757305, 32.15551576947925838 ) ) ;
#43147=CARTESIAN_POINT ( 'NONE',  ( 6.699591998512592461, -2.353723527008295680, 30.78948104536958752 ) ) ;
#43148=CARTESIAN_POINT ( 'NONE',  ( 18.13052570176355971, -3.285477652293413264, 32.44071101563363158 ) ) ;
#43149=CARTESIAN_POINT ( 'NONE',  ( -17.07692307692319744, -10.33852847137269571, 34.16647553114546554 ) ) ;
#43150=CARTESIAN_POINT ( 'NONE',  ( -1.608100328339332030, -12.44517049084099725, 30.48991314939691932 ) ) ;
#43151=FACE_OUTER_BOUND ( 'NONE', #82766, .T. ) ;
#43152=CARTESIAN_POINT ( 'NONE',  ( 6.000000000000001776, -13.20930481340135110, 34.54067556320372745 ) ) ;
#43154=CARTESIAN_POINT ( 'NONE',  ( 14.55763782604045176, -11.86320923018887719, 32.19269448109604070 ) ) ;
#43155=CARTESIAN_POINT ( 'NONE',  ( 14.08420736396836226, -6.760086850603066466, 34.69517049084099369 ) ) ;
#43156=EDGE_LOOP ( 'NONE', ( #50684, #63100 ) ) ;
#43157=AXIS2_PLACEMENT_3D ( 'NONE', #82816, #21089, #48560 ) ;
#43158=DIRECTION ( 'NONE',  ( -0.000000000000000000, 0.9396926207859092051, -0.3420201433256662704 ) ) ;
#43159=DIRECTION ( 'NONE',  ( 0.000000000000000000, 0.8660254037844377084, -0.5000000000000015543 ) ) ;
#43161=CARTESIAN_POINT ( 'NONE',  ( 4.153846153846030731, -5.094484230521993062, 34.41647553114689373 ) ) ;
#43162=CARTESIAN_POINT ( 'NONE',  ( -16.15384615384615330, -2.486705287966279876, 31.30864560766543647 ) ) ;
#43163=ORIENTED_EDGE ( 'NONE', *, *, #63073, .T. ) ;
#43164=CARTESIAN_POINT ( 'NONE',  ( -7.053767526187232129, -2.845849958028613624, 32.17971566917920967 ) ) ;
#43165=CARTESIAN_POINT ( 'NONE',  ( 12.33084699487089964, -5.582088688514999397, 34.36776431015576350 ) ) ;
#43166=ORIENTED_EDGE ( 'NONE', *, *, #5177, .F. ) ;
#43167=CARTESIAN_POINT ( 'NONE',  ( 7.976945653978629203, -3.530189275343204702, 32.79018710029569661 ) ) ;
#43168=CARTESIAN_POINT ( 'NONE',  ( 16.85399611801622299, -2.523278758544490241, 31.42238647778636818 ) ) ;
#43169=ORIENTED_EDGE ( 'NONE', *, *, #15846, .T. ) ;
#43173=ORIENTED_EDGE ( 'NONE', *, *, #75205, .F. ) ;
#43174=CARTESIAN_POINT ( 'NONE',  ( 8.835298102580845025, -2.292212530054420494, 30.41441678777542990 ) ) ;
#43175=CARTESIAN_POINT ( 'NONE',  ( -11.60373153901785948, -12.51329471203370325, 31.30864560766548976 ) ) ;
#43176=DIRECTION ( 'NONE',  ( -0.000000000000000000, 0.1736481776669307198, -0.9848077530122080203 ) ) ;
#43177=VERTEX_POINT ( 'NONE', #50994 ) ;
#43178=ORIENTED_EDGE ( 'NONE', *, *, #85734, .T. ) ;
#43179=ORIENTED_EDGE ( 'NONE', *, *, #84303, .F. ) ;
#43181=VECTOR ( 'NONE', #83552, 1000.000000000000227 ) ;
#43182=EDGE_CURVE ( 'NONE', #11993, #37408, #56454, .T. ) ;
#43183=CARTESIAN_POINT ( 'NONE',  ( -5.207613680033384540, -9.084618155246140248, 34.75535874321725771 ) ) ;
#43184=CARTESIAN_POINT ( 'NONE',  ( -14.37296275365308418, -3.300289026998414865, 32.46337939537583139 ) ) ;
#43185=EDGE_CURVE ( 'NONE', #56880, #23776, #2377, .T. ) ;
#43186=CARTESIAN_POINT ( 'NONE',  ( -7.911910648668153634, -7.249945686854186278, 34.74374336980223887 ) ) ;
#43187=AXIS2_PLACEMENT_3D ( 'NONE', #45917, #18463, #12592 ) ;
#43189=CARTESIAN_POINT ( 'NONE',  ( -5.076923076923075762, -2.292212530054420494, 30.41441678777542634 ) ) ;
#43190=EDGE_LOOP ( 'NONE', ( #34106, #75321 ) ) ;
#43191=EDGE_CURVE ( 'NONE', #72551, #84061, #25464, .T. ) ;
#43192=VERTEX_POINT ( 'NONE', #1514 ) ;
#43193=CARTESIAN_POINT ( 'NONE',  ( -1.515225744239911521, -7.722926236386453702, 34.74524107206102030 ) ) ;
#43195=CARTESIAN_POINT ( 'NONE',  ( 16.28437159207980045, -8.630441415882549094, 34.87705825610312615 ) ) ;
#43196=EDGE_LOOP ( 'NONE', ( #69666, #78734, #12738, #9083 ) ) ;
#43197=B_SPLINE_CURVE_WITH_KNOTS ( 'NONE', 3,
 ( #8248, #36598, #7359, #48328, #43354, #21749, #29410, #75803, #69492, #63618 ),
 .UNSPECIFIED., .F., .F.,
 ( 4, 2, 2, 2, 4 ),
 ( 0.0007817246256747505334, 0.0009771112852218941883, 0.001172497944769037952, 0.001367884604316181498, 0.001563271263863325261 ),
 .UNSPECIFIED. ) ;
#43199=CARTESIAN_POINT ( 'NONE',  ( -8.638440328263820689, -12.62708834333097663, 30.88030960425257021 ) ) ;
#43200=ORIENTED_EDGE ( 'NONE', *, *, #13570, .T. ) ;
#43201=ORIENTED_EDGE ( 'NONE', *, *, #22136, .T. ) ;
#43202=CARTESIAN_POINT ( 'NONE',  ( -8.769230769230768274, -8.120952969808772792, 34.71129190930000163 ) ) ;
#43203=ORIENTED_EDGE ( 'NONE', *, *, #26029, .T. ) ;
#43204=CARTESIAN_POINT ( 'NONE',  ( -3.230769230769351186, -6.879047030192662504, 34.71129190930017927 ) ) ;
#43205=CARTESIAN_POINT ( 'NONE',  ( -0.4615384615385840772, -5.094484230521993062, 34.41647553114689373 ) ) ;
#43206=EDGE_CURVE ( 'NONE', #45365, #65338, #1952, .T. ) ;
#43207=ORIENTED_EDGE ( 'NONE', *, *, #80149, .F. ) ;
#43208=LINE ( 'NONE', #41892, #80547 ) ;
#43209=CARTESIAN_POINT ( 'NONE',  ( -14.05774689831426372, -12.68172785388650681, 30.59649109432439218 ) ) ;
#43210=CARTESIAN_POINT ( 'NONE',  ( 18.00000000000000000, -12.34228464037088635, 31.77849191805839268 ) ) ;
#43211=FACE_BOUND ( 'NONE', #38095, .T. ) ;
#43212=CARTESIAN_POINT ( 'NONE',  ( 1.449870955891411350, -12.46129190930001052, 30.37095296980870174 ) ) ;
#43214=ADVANCED_FACE ( 'NONE', ( #64965 ), #15918, .F. ) ;
#43215=CYLINDRICAL_SURFACE ( 'NONE', #46589, 0.2500000000000002220 ) ;
#43216=CARTESIAN_POINT ( 'NONE',  ( 0.4615384615387756462, -2.255955759149395501, 30.00000000000324363 ) ) ;
#43217=CARTESIAN_POINT ( 'NONE',  ( 9.757563263583719504, -3.300289026998473041, 32.46337939537591666 ) ) ;
#43218=CARTESIAN_POINT ( 'NONE',  ( -3.007989689500818464, -3.236590943229497253, 32.36255958852954251 ) ) ;
#43219=CARTESIAN_POINT ( 'NONE',  ( -16.15384615384615330, -8.120952969808772792, 34.71129190930000163 ) ) ;
#43220=VERTEX_POINT ( 'NONE', #16784 ) ;
#43221=EDGE_CURVE ( 'NONE', #77943, #88418, #59919, .T. ) ;
#43222=CARTESIAN_POINT ( 'NONE',  ( 10.61538461538461675, -10.51840700105979565, 33.73612834413961536 ) ) ;
#43223=VERTEX_POINT ( 'NONE', #33751 ) ;
#43224=VERTEX_POINT ( 'NONE', #27438 ) ;
#43226=CARTESIAN_POINT ( 'NONE',  ( 7.846153846153846700, -9.780366693483667717, 34.19971097300155094 ) ) ;
#43227=CARTESIAN_POINT ( 'NONE',  ( 11.53846153846153832, -8.164416787775445883, 34.95778746994557906 ) ) ;
#43228=CARTESIAN_POINT ( 'NONE',  ( 0.2115384615384615641, -7.500000000000001776, 35.04278698407183867 ) ) ;
#43229=CARTESIAN_POINT ( 'NONE',  ( -12.46153846153846168, -2.486705287966279876, 31.30864560766543647 ) ) ;
#43230=CARTESIAN_POINT ( 'NONE',  ( 1.384615384615386802, -1.215029322943914858, 32.30358669280327177 ) ) ;
#43231=ORIENTED_EDGE ( 'NONE', *, *, #52356, .T. ) ;
#43232=CARTESIAN_POINT ( 'NONE',  ( -9.692307692307691624, -9.819645486525091727, 36.12317359536749706 ) ) ;
#43233=CARTESIAN_POINT ( 'NONE',  ( 3.230769230769110045, -11.48612834414049644, 32.76840700105863391 ) ) ;
#43234=B_SPLINE_CURVE_WITH_KNOTS ( 'NONE', 3,
 ( #36790, #64243, #2547, #30038, #57497, #83216, #49425, #16514, #43981, #21498 ),
 .UNSPECIFIED., .F., .F.,
 ( 4, 2, 2, 2, 4 ),
 ( 0.0007817246256747463051, 0.0009771112852218896347, 0.001172497944769033181, 0.001367884604316176728, 0.001563271263863320057 ),
 .UNSPECIFIED. ) ;
#43235=DIRECTION ( 'NONE',  ( 0.000000000000000000, 0.9396926207859126468, -0.3420201433256571111 ) ) ;
#43237=DIRECTION ( 'NONE',  ( -0.000000000000000000, 0.9396926207859092051, -0.3420201433256662704 ) ) ;
#43238=CARTESIAN_POINT ( 'NONE',  ( 13.45068271796546178, -5.471508081941601098, 34.59228464037088457 ) ) ;
#43239=EDGE_CURVE ( 'NONE', #37672, #16542, #13656, .T. ) ;
#43241=ORIENTED_EDGE ( 'NONE', *, *, #43555, .F. ) ;
#43243=VECTOR ( 'NONE', #40685, 1000.000000000000000 ) ;
#43245=CARTESIAN_POINT ( 'NONE',  ( -7.780898706641008467, -12.16647553114626490, 32.15551576947920864 ) ) ;
#43246=ADVANCED_FACE ( 'NONE', ( #13915 ), #81505, .F. ) ;
#43247=VERTEX_POINT ( 'NONE', #40522 ) ;
#43248=CARTESIAN_POINT ( 'NONE',  ( -9.692307692307812417, -12.46129190930018460, 30.37095296980731973 ) ) ;
#43249=CARTESIAN_POINT ( 'NONE',  ( 15.45354889974729673, -4.226511098958373402, 33.85474049983370293 ) ) ;
#43250=LINE ( 'NONE', #41928, #22176 ) ;
#43251=DIRECTION ( 'NONE',  ( 1.000000000000000000, 0.000000000000000000, 0.000000000000000000 ) ) ;
#43253=VECTOR ( 'NONE', #47761, 1000.000000000000114 ) ;
#43254=FACE_OUTER_BOUND ( 'NONE', #82320, .T. ) ;
#43255=VERTEX_POINT ( 'NONE', #17686 ) ;
#43256=CARTESIAN_POINT ( 'NONE',  ( 4.283893760101836534, -7.723484964179500700, 34.74522123443823318 ) ) ;
#43257=CARTESIAN_POINT ( 'NONE',  ( 17.74999999999998224, -2.249999999999998668, 29.81609741502487054 ) ) ;
#43258=ORIENTED_EDGE ( 'NONE', *, *, #78343, .T. ) ;
#43259=CARTESIAN_POINT ( 'NONE',  ( -10.54931626438217585, -3.513871655860379306, 32.76840700105978499 ) ) ;
#43260=DIRECTION ( 'NONE',  ( -0.000000000000000000, 0.3420201433256694901, -0.9396926207859082059 ) ) ;
#43261=CARTESIAN_POINT ( 'NONE',  ( 6.222779668978068557, -9.418065098278011860, 34.63729479722530158 ) ) ;
#43262=ADVANCED_FACE ( 'NONE', ( #20675 ), #54906, .F. ) ;
#43263=CARTESIAN_POINT ( 'NONE',  ( -2.084679463598912097, -2.308499170217967134, 30.53291367094873721 ) ) ;
#43265=CARTESIAN_POINT ( 'NONE',  ( -0.4615384615384611200, -12.78798330534103123, 29.99999999999997868 ) ) ;
#43268=ADVANCED_FACE ( 'NONE', ( #40085 ), #74296, .F. ) ;
#43269=CARTESIAN_POINT ( 'NONE',  ( -3.165514091256391271, -6.835583212224609184, 34.95778746994559327 ) ) ;
#43270=CARTESIAN_POINT ( 'NONE',  ( -1.384615384615505151, -12.27809138561165270, 31.22303859784587132 ) ) ;
#43272=CARTESIAN_POINT ( 'NONE',  ( 14.30769230769231015, -5.415277668671390821, 36.20867863119892149 ) ) ;
#43273=CARTESIAN_POINT ( 'NONE',  ( -2.980714810855778829, -10.82426656108011720, 33.81400080652039009 ) ) ;
#43274=EDGE_LOOP ( 'NONE', ( #83645, #68285, #59049, #6494 ) ) ;
#43275=CARTESIAN_POINT ( 'NONE',  ( 0.4615384615383382183, -4.320704448113951379, 33.92786785259630022 ) ) ;
#43276=CARTESIAN_POINT ( 'NONE',  ( -3.480745961711583902, -10.66389620160130036, 33.62221079203477103 ) ) ;
#43277=ORIENTED_EDGE ( 'NONE', *, *, #11939, .T. ) ;
#43278=EDGE_CURVE ( 'NONE', #7349, #7411, #60773, .T. ) ;
#43279=DIRECTION ( 'NONE',  ( -0.000000000000000000, 1.000000000000000000, 3.491481338843133355E-15 ) ) ;
#43280=B_SPLINE_CURVE_WITH_KNOTS ( 'NONE', 3,
 ( #57372, #84867, #43859, #62788, #28587, #9631, #23150, #56051, #70004, #3315 ),
 .UNSPECIFIED., .F., .F.,
 ( 4, 2, 2, 2, 4 ),
 ( 0.0007817246256747530271, 0.0009771112852218978746, 0.001172497944769042939, 0.001367884604316188003, 0.001563271263863332851 ),
 .UNSPECIFIED. ) ;
#43281=ORIENTED_EDGE ( 'NONE', *, *, #50072, .T. ) ;
#43282=B_SPLINE_CURVE_WITH_KNOTS ( 'NONE', 3,
 ( #39081, #40846, #32749, #68312, #54789, #18800, #6172, #45815, #33197, #89049 ),
 .UNSPECIFIED., .F., .F.,
 ( 4, 2, 2, 2, 4 ),
 ( 0.0007817359430256386795, 0.0009771253907250069485, 0.001172514838424375217, 0.001367904286123743486, 0.001563293733823111755 ),
 .UNSPECIFIED. ) ;
#43283=CARTESIAN_POINT ( 'NONE',  ( 7.053867364043876265, -3.957578996910242619, 33.62503395064540257 ) ) ;
#43284=CARTESIAN_POINT ( 'NONE',  ( 16.94636248518114741, -2.504760397472873823, 29.97295953869789997 ) ) ;
#43285=ADVANCED_FACE ( 'NONE', ( #47703 ), #53571, .F. ) ;
#43286=CARTESIAN_POINT ( 'NONE',  ( -8.769230769230768274, -5.471508081941601098, 34.59228464037088457 ) ) ;
#43287=DIRECTION ( 'NONE',  ( 0.000000000000000000, 0.7660444431189807890, 0.6427876096865361433 ) ) ;
#43289=ORIENTED_EDGE ( 'NONE', *, *, #10065, .F. ) ;
#43290=CARTESIAN_POINT ( 'NONE',  ( -3.100243792535585907, -2.372941743896878286, 30.88044141588254377 ) ) ;
#43291=EDGE_LOOP ( 'NONE', ( #50898, #43008 ) ) ;
#43293=CARTESIAN_POINT ( 'NONE',  ( 0.4615384615383382183, -10.33852847137269571, 34.16647553114546554 ) ) ;
#43294=ORIENTED_EDGE ( 'NONE', *, *, #84200, .F. ) ;
#43295=CARTESIAN_POINT ( 'NONE',  ( -5.999999999999998224, -11.16473453929635440, 33.15142922261926373 ) ) ;
#43296=DIRECTION ( 'NONE',  ( 0.000000000000000000, 0.000000000000000000, -1.000000000000000000 ) ) ;
#43297=ADVANCED_FACE ( 'NONE', ( #32865 ), #6288, .F. ) ;
#43298=CARTESIAN_POINT ( 'NONE',  ( 8.769230769230768274, -2.249999999999998668, 29.50000000000001421 ) ) ;
#43301=CARTESIAN_POINT ( 'NONE',  ( -3.931066484868084299, -4.226511098958374291, 33.85474049983370293 ) ) ;
#43302=ORIENTED_EDGE ( 'NONE', *, *, #30162, .F. ) ;
#43303=ORIENTED_EDGE ( 'NONE', *, *, #22167, .T. ) ;
#43304=AXIS2_PLACEMENT_3D ( 'NONE', #82491, #34731, #33841 ) ;
#43305=FACE_BOUND ( 'NONE', #64337, .T. ) ;
#43306=VERTEX_POINT ( 'NONE', #86151 ) ;
#43307=CARTESIAN_POINT ( 'NONE',  ( 15.23076923076911093, -12.46129190930018460, 30.37095296980731973 ) ) ;
#43308=VECTOR ( 'NONE', #904, 1000.000000000000114 ) ;
#43309=VECTOR ( 'NONE', #60520, 1000.000000000000227 ) ;
#43310=CARTESIAN_POINT ( 'NONE',  ( 6.673076923076905587, -2.249999999999999112, 29.81609741502488120 ) ) ;
#43311=FACE_OUTER_BOUND ( 'NONE', #46219, .T. ) ;
#43312=CARTESIAN_POINT ( 'NONE',  ( -2.057746898314262385, -10.18230066228895758, 34.26354781536631577 ) ) ;
#43314=ORIENTED_EDGE ( 'NONE', *, *, #20534, .T. ) ;
#43315=ORIENTED_EDGE ( 'NONE', *, *, #59387, .F. ) ;
#43316=EDGE_LOOP ( 'NONE', ( #60005, #74828, #71908, #24590, #7540, #32187 ) ) ;
#43317=CARTESIAN_POINT ( 'NONE',  ( 6.923076923076924238, -13.87047571288749737, 32.06866353760679544 ) ) ;
#43318=CARTESIAN_POINT ( 'NONE',  ( 13.38461538461538680, -2.721908614388771852, 31.22303859784724978 ) ) ;
#43319=CARTESIAN_POINT ( 'NONE',  ( 14.05766908347085042, -12.07920672191015221, 32.31858351112116168 ) ) ;
#43320=CARTESIAN_POINT ( 'NONE',  ( -18.00000000000012079, -6.835583212225971650, 34.95778746994575670 ) ) ;
#43321=EDGE_LOOP ( 'NONE', ( #3528, #45498, #43747, #63007 ) ) ;
#43322=CARTESIAN_POINT ( 'NONE',  ( 16.37662582282421653, -2.353885683473779800, 30.79025554430704759 ) ) ;
#43323=EDGE_CURVE ( 'NONE', #67903, #67434, #63101, .T. ) ;
#43324=CARTESIAN_POINT ( 'NONE',  ( 10.61538461538449596, -2.625532179533778709, 30.86335684631627174 ) ) ;
#43325=CARTESIAN_POINT ( 'NONE',  ( 4.153846153846154188, -2.486705287966279876, 31.30864560766543647 ) ) ;
#43328=ADVANCED_FACE ( 'NONE', ( #61652 ), #89158, .F. ) ;
#43329=ORIENTED_EDGE ( 'NONE', *, *, #69050, .F. ) ;
#43330=ORIENTED_EDGE ( 'NONE', *, *, #58099, .T. ) ;
#43331=CARTESIAN_POINT ( 'NONE',  ( 12.33139125210024112, -6.852621066184266141, 34.70813303252209181 ) ) ;
#43332=CARTESIAN_POINT ( 'NONE',  ( 1.634669804528839476, -11.47946981652013498, 33.17500667209846910 ) ) ;
#43333=EDGE_CURVE ( 'NONE', #19690, #88317, #4075, .T. ) ;
#43334=CARTESIAN_POINT ( 'NONE',  ( 16.02315468717859304, -5.582088688514999397, 34.36776431015576350 ) ) ;
#43336=CARTESIAN_POINT ( 'NONE',  ( 15.23076923076923173, -12.34228464037088635, 31.77849191805839268 ) ) ;
#43337=CARTESIAN_POINT ( 'NONE',  ( -2.530618525208453651, -9.886141570436013382, 34.14413921362392301 ) ) ;
#43338=ORIENTED_EDGE ( 'NONE', *, *, #56315, .T. ) ;
#43339=CARTESIAN_POINT ( 'NONE',  ( -7.596153846153909761, -7.565270000091922853, 34.99999999999999289 ) ) ;
#43340=DIRECTION ( 'NONE',  ( -0.000000000000000000, -0.8660254037844397068, -0.4999999999999978906 ) ) ;
#43341=LINE ( 'NONE', #78445, #12818 ) ;
#43342=CARTESIAN_POINT ( 'NONE',  ( -11.40766973063675493, -3.530189275343204702, 32.79018710029569661 ) ) ;
#43344=ORIENTED_EDGE ( 'NONE', *, *, #51805, .T. ) ;
#43346=CARTESIAN_POINT ( 'NONE',  ( -18.25002323729296450, -8.432397168068783699, 34.66272746175022945 ) ) ;
#43348=FACE_BOUND ( 'NONE', #10071, .T. ) ;
#43349=CARTESIAN_POINT ( 'NONE',  ( -16.85391172531022619, -4.187068189119696804, 33.49521262558774026 ) ) ;
#43351=DIRECTION ( 'NONE',  ( -0.000000000000000000, 0.9848077530122085754, -0.1736481776669273613 ) ) ;
#43352=ORIENTED_EDGE ( 'NONE', *, *, #64115, .T. ) ;
#43354=CARTESIAN_POINT ( 'NONE',  ( -17.75005459062195712, -4.176053281294518804, 33.81426240980091791 ) ) ;
#43355=CARTESIAN_POINT ( 'NONE',  ( 8.639082799499073317, -8.630895178749533159, 34.87696386517710323 ) ) ;
#43356=CARTESIAN_POINT ( 'NONE',  ( -7.173053654019277303, -10.66389620160130036, 33.62221079203477103 ) ) ;
#43357=ORIENTED_EDGE ( 'NONE', *, *, #6285, .F. ) ;
#43358=CARTESIAN_POINT ( 'NONE',  ( -9.822998295418001291, -2.845849958028613624, 32.17971566917920967 ) ) ;
#43359=ORIENTED_EDGE ( 'NONE', *, *, #65055, .T. ) ;
#43361=VERTEX_POINT ( 'NONE', #62103 ) ;
#43362=CARTESIAN_POINT ( 'NONE',  ( -8.639183162975086816, -7.723484964179501588, 34.74522123443823318 ) ) ;
#43363=CARTESIAN_POINT ( 'NONE',  ( -6.857008572074483332, -11.69971097300155272, 32.46337939537588113 ) ) ;
#43364=CARTESIAN_POINT ( 'NONE',  ( 4.946775107191377252, -2.647304123082328875, 31.75400227202885262 ) ) ;
#43365=CARTESIAN_POINT ( 'NONE',  ( 12.71159277317677549, -4.235687564193448829, 33.53795663066793509 ) ) ;
#43366=CARTESIAN_POINT ( 'NONE',  ( -14.30769230769230660, -8.164416787775445883, 34.95778746994557906 ) ) ;
#43367=CARTESIAN_POINT ( 'NONE',  ( -15.23076923076935074, -6.026961402154118019, 34.52809138561165270 ) ) ;
#43368=CARTESIAN_POINT ( 'NONE',  ( 5.999999999999880096, -2.892918686052165622, 31.69288490824153470 ) ) ;
#43370=ORIENTED_EDGE ( 'NONE', *, *, #1090, .T. ) ;
#43371=EDGE_CURVE ( 'NONE', #50664, #23467, #56728, .T. ) ;
#43372=CARTESIAN_POINT ( 'NONE',  ( 11.53846153846141576, -4.320704448113951379, 33.92786785259630022 ) ) ;
#43373=LINE ( 'NONE', #23531, #87006 ) ;
#43374=EDGE_LOOP ( 'NONE', ( #26278, #38036, #84408, #52406 ) ) ;
#43375=B_SPLINE_CURVE_WITH_KNOTS ( 'NONE', 3,
 ( #47135, #46701, #13359, #80952, #19237, #26439, #67862, #19671, #81830, #89043 ),
 .UNSPECIFIED., .F., .F.,
 ( 4, 2, 2, 2, 4 ),
 ( 0.0007817246256747457630, 0.0009771112852218887673, 0.001172497944769031880, 0.001367884604316174993, 0.001563271263863318106 ),
 .UNSPECIFIED. ) ;
#43376=ORIENTED_EDGE ( 'NONE', *, *, #2088, .T. ) ;
#43377=VERTEX_POINT ( 'NONE', #83273 ) ;
#43378=DIRECTION ( 'NONE',  ( -0.000000000000000000, 0.8660254037844397068, -0.4999999999999978906 ) ) ;
#43379=LINE ( 'NONE', #78046, #44701 ) ;
#43380=AXIS2_PLACEMENT_3D ( 'NONE', #43317, #78864, #79321 ) ;
#43381=DIRECTION ( 'NONE',  ( -0.000000000000000000, -0.000000000000000000, -1.000000000000000000 ) ) ;
#43382=CARTESIAN_POINT ( 'NONE',  ( 8.899756207464411872, -11.66157788607254098, 32.95092075102925833 ) ) ;
#43384=ADVANCED_FACE ( 'NONE', ( #68859 ), #28314, .F. ) ;
#43386=CYLINDRICAL_SURFACE ( 'NONE', #53712, 0.2499999999999995559 ) ;
#43387=EDGE_LOOP ( 'NONE', ( #81080, #57068, #9280, #83190 ) ) ;
#43389=CARTESIAN_POINT ( 'NONE',  ( -1.450698795571264021, -6.386643153685125363, 34.62446782046654903 ) ) ;
#43391=EDGE_CURVE ( 'NONE', #56650, #36450, #49483, .T. ) ;
#43392=CARTESIAN_POINT ( 'NONE',  ( 7.846153846153846700, -2.721908614388771852, 31.22303859784724978 ) ) ;
#43393=CARTESIAN_POINT ( 'NONE',  ( 17.99999999999987566, -12.27809138561165270, 31.22303859784587132 ) ) ;
#43394=VERTEX_POINT ( 'NONE', #55783 ) ;
#43395=CARTESIAN_POINT ( 'NONE',  ( 12.33139049180676672, -9.504002272028875709, 34.60269587691767867 ) ) ;
#43397=CARTESIAN_POINT ( 'NONE',  ( 11.66898724022509981, -10.19071101563364756, 33.96452234770658407 ) ) ;
#43398=DIRECTION ( 'NONE',  ( -0.000000000000000000, -0.9848077530122086864, -0.1736481776669273613 ) ) ;
#43399=EDGE_LOOP ( 'NONE', ( #41197, #84765, #39002, #24868 ) ) ;
#43400=CARTESIAN_POINT ( 'NONE',  ( -2.373774687052440768, -6.343179335718451384, 34.87096338111212646 ) ) ;
#43401=EDGE_CURVE ( 'NONE', #85626, #87991, #72837, .T. ) ;
#43402=CARTESIAN_POINT ( 'NONE',  ( -12.59201516965492473, -7.276988635370452485, 34.74523720219453793 ) ) ;
#43403=B_SPLINE_CURVE_WITH_KNOTS ( 'NONE', 3,
 ( #67208, #80279, #5509, #39298, #4152, #18132, #3708, #66754, #18575, #87053 ),
 .UNSPECIFIED., .F., .F.,
 ( 4, 2, 2, 2, 4 ),
 ( 0.000000000000000000, 0.0001954311564186868202, 0.0003908623128373736404, 0.0005862934692560604335, 0.0007817246256747472808 ),
 .UNSPECIFIED. ) ;
#43404=VECTOR ( 'NONE', #22178, 1000.000000000000000 ) ;
#43405=CARTESIAN_POINT ( 'NONE',  ( -8.769230769230892619, -9.528491918059723176, 34.59228464037033035 ) ) ;
#43406=ADVANCED_FACE ( 'NONE', ( #35972 ), #41846, .F. ) ;
#43407=EDGE_CURVE ( 'NONE', #5574, #82155, #29222, .T. ) ;
#43409=B_SPLINE_CURVE_WITH_KNOTS ( 'NONE', 3,
 ( #72634, #79405, #47723, #52804, #17706, #34204, #45160, #80297, #81969, #46055 ),
 .UNSPECIFIED., .F., .F.,
 ( 4, 2, 2, 2, 4 ),
 ( 0.0007817246256747446788, 0.0009771112852218879000, 0.001172497944769031013, 0.001367884604316174126, 0.001563271263863317238 ),
 .UNSPECIFIED. ) ;
#43410=CARTESIAN_POINT ( 'NONE',  ( -10.74594520712653534, -2.504760397472875155, 29.97295953869789997 ) ) ;
#43411=VERTEX_POINT ( 'NONE', #76952 ) ;
#43413=B_SPLINE_CURVE_WITH_KNOTS ( 'NONE', 3,
 ( #26486, #53947, #89093, #15627, #62033, #28244, #56609, #49414, #69677, #63359 ),
 .UNSPECIFIED., .F., .F.,
 ( 4, 2, 2, 2, 4 ),
 ( 0.0007817359430256297891, 0.0009771253907249961065, 0.001172514838424362424, 0.001367904286123728741, 0.001563293733823095059 ),
 .UNSPECIFIED. ) ;
#43414=ADVANCED_FACE ( 'NONE', ( #82834 ), #77389, .F. ) ;
#43415=B_SPLINE_CURVE_WITH_KNOTS ( 'NONE', 3,
 ( #59431, #52666, #18009, #59875, #79265, #45464, #72049, #38717, #3142, #58090 ),
 .UNSPECIFIED., .F., .F.,
 ( 4, 2, 2, 2, 4 ),
 ( 0.000000000000000000, 0.0001954339857564081791, 0.0003908679715128163582, 0.0005863019572692245102, 0.0007817359430256327164 ),
 .UNSPECIFIED. ) ;
#43416=DIRECTION ( 'NONE',  ( -0.000000000000000000, -0.000000000000000000, -1.000000000000000000 ) ) ;
#43417=CARTESIAN_POINT ( 'NONE',  ( 7.173131342990374471, -2.920487667080175154, 32.31805714834170828 ) ) ;
#43418=CARTESIAN_POINT ( 'NONE',  ( -8.096177070375304652, -2.588893531581426988, 31.60682220781847818 ) ) ;
#43419=CARTESIAN_POINT ( 'NONE',  ( 1.384615384615264011, -8.656820664282941280, 34.87096338111179961 ) ) ;
#43420=CARTESIAN_POINT ( 'NONE',  ( -3.480769230769229061, -7.500000000000001776, 35.00000000000000000 ) ) ;
#43421=ORIENTED_EDGE ( 'NONE', *, *, #1312, .F. ) ;
#43422=ORIENTED_EDGE ( 'NONE', *, *, #34535, .F. ) ;
#43423=EDGE_LOOP ( 'NONE', ( #87285, #22786 ) ) ;
#43424=CYLINDRICAL_SURFACE ( 'NONE', #73218, 0.2499999999999979738 ) ;
#43425=CARTESIAN_POINT ( 'NONE',  ( 15.93091919493930320, -5.582147617184174848, 34.63737895849758530 ) ) ;
#43427=EDGE_CURVE ( 'NONE', #54250, #54586, #52413, .T. ) ;
#43429=CARTESIAN_POINT ( 'NONE',  ( -2.177166869458664333, -11.66157788607254275, 32.95092075102925833 ) ) ;
#43431=CARTESIAN_POINT ( 'NONE',  ( 4.284371855609715674, -6.852161475712352789, 34.70806712695775786 ) ) ;
#43432=CARTESIAN_POINT ( 'NONE',  ( 5.207448778686637247, -10.19071101563364756, 33.96452234770658407 ) ) ;
#43433=ORIENTED_EDGE ( 'NONE', *, *, #47154, .T. ) ;
#43434=ORIENTED_EDGE ( 'NONE', *, *, #26554, .T. ) ;
#43435=B_SPLINE_CURVE_WITH_KNOTS ( 'NONE', 3,
 ( #65912, #59162, #80343, #72232, #33033, #3775, #88011, #66817, #24483, #11883 ),
 .UNSPECIFIED., .F., .F.,
 ( 4, 2, 2, 2, 4 ),
 ( 0.000000000000000000, 0.0001954311564186868744, 0.0003908623128373737488, 0.0005862934692560606504, 0.0007817246256747474977 ),
 .UNSPECIFIED. ) ;
#43436=ORIENTED_EDGE ( 'NONE', *, *, #40666, .F. ) ;
#43437=CARTESIAN_POINT ( 'NONE',  ( 12.52679403281448600, -8.613356846314928816, 34.62446782046653482 ) ) ;
#43438=ORIENTED_EDGE ( 'NONE', *, *, #53817, .T. ) ;
#43439=CARTESIAN_POINT ( 'NONE',  ( 8.900022577055551665, -8.147973898785416225, 34.70805048591653730 ) ) ;
#43440=DIRECTION ( 'NONE',  ( -0.000000000000000000, -0.3420201433256694346, -0.9396926207859080948 ) ) ;
#43442=VERTEX_POINT ( 'NONE', #51665 ) ;
#43443=EDGE_LOOP ( 'NONE', ( #35555, #10615, #74761, #35768 ) ) ;
#43444=CARTESIAN_POINT ( 'NONE',  ( 13.38461538461569411, -2.506253911140615021, 30.00000000000323297 ) ) ;
#43445=VERTEX_POINT ( 'NONE', #16133 ) ;
#43446=FACE_BOUND ( 'NONE', #57178, .T. ) ;
#43447=CARTESIAN_POINT ( 'NONE',  ( 13.60762822870878352, -12.38742843783360748, 31.66772728687926985 ) ) ;
#43448=CARTESIAN_POINT ( 'NONE',  ( -14.37296230824862775, -6.835583212224499938, 34.95778746994557906 ) ) ;
#43449=ORIENTED_EDGE ( 'NONE', *, *, #6928, .T. ) ;
#43450=CARTESIAN_POINT ( 'NONE',  ( -14.24243716817947281, -8.656820664281605460, 34.87096338111211224 ) ) ;
#43451=CARTESIAN_POINT ( 'NONE',  ( 16.21910172512217585, -4.481592998940251427, 33.73612834413965089 ) ) ;
#43453=CARTESIAN_POINT ( 'NONE',  ( -11.78848477575450460, -5.851115903089112003, 34.47074536777953568 ) ) ;
#43454=FACE_OUTER_BOUND ( 'NONE', #68194, .T. ) ;
#43455=EDGE_CURVE ( 'NONE', #56514, #17995, #84659, .T. ) ;
#43456=CIRCLE ( 'NONE', #4634, 0.2500000000000002220 ) ;
#43458=CARTESIAN_POINT ( 'NONE',  ( -7.596099534515530216, -6.567000820036036579, 34.66262288849541306 ) ) ;
#43459=CARTESIAN_POINT ( 'NONE',  ( 0.3954550505825793483, -11.69971097300155272, 32.46337939537587403 ) ) ;
#43460=CARTESIAN_POINT ( 'NONE',  ( 13.45068271796546178, -2.292212530054420494, 30.41441678777542990 ) ) ;
#43461=CYLINDRICAL_SURFACE ( 'NONE', #47329, 0.2500000000000008882 ) ;
#43462=FACE_BOUND ( 'NONE', #71545, .T. ) ;
#43463=CARTESIAN_POINT ( 'NONE',  ( -13.60810030917971858, -4.225889041578353655, 33.85425143139329407 ) ) ;
#43464=CARTESIAN_POINT ( 'NONE',  ( 2.307692307692309264, -9.780366693483667717, 34.19971097300155094 ) ) ;
#43465=CARTESIAN_POINT ( 'NONE',  ( -0.2115930521604184600, -8.476813868363244353, 34.90874843262270133 ) ) ;
#43466=DIRECTION ( 'NONE',  ( 0.000000000000000000, 0.1736481776669267785, -0.9848077530122087975 ) ) ;
#43467=CARTESIAN_POINT ( 'NONE',  ( -6.130691466667557599, -4.809359713505814149, 33.96456829005828837 ) ) ;
#43468=VECTOR ( 'NONE', #2072, 1000.000000000000227 ) ;
#43469=CARTESIAN_POINT ( 'NONE',  ( -2.531177232256636156, -5.827078755546623690, 34.72654668319379567 ) ) ;
#43471=VERTEX_POINT ( 'NONE', #24208 ) ;
#43472=CARTESIAN_POINT ( 'NONE',  ( -4.153846153846274980, -5.941354392335915335, 34.76329471203413846 ) ) ;
#43473=EDGE_LOOP ( 'NONE', ( #79764, #28963 ) ) ;
#43474=B_SPLINE_CURVE_WITH_KNOTS ( 'NONE', 3,
 ( #57247, #78391, #16693, #36960, #42854, #44149, #8628, #15826, #51335, #3179 ),
 .UNSPECIFIED., .F., .F.,
 ( 4, 2, 2, 2, 4 ),
 ( 0.0007817246256747427272, 0.0009771112852218844305, 0.001172497944769026242, 0.001367884604316168054, 0.001563271263863309649 ),
 .UNSPECIFIED. ) ;
#43475=DIRECTION ( 'NONE',  ( 0.000000000000000000, 0.8660254037844377084, 0.5000000000000015543 ) ) ;
#43476=EDGE_LOOP ( 'NONE', ( #12193, #73686 ) ) ;
#43477=B_SPLINE_CURVE_WITH_KNOTS ( 'NONE', 3,
 ( #23186, #28622, #50648, #22300, #78127, #77240, #16430, #43897, #9669, #64598 ),
 .UNSPECIFIED., .F., .F.,
 ( 4, 2, 2, 2, 4 ),
 ( 0.000000000000000000, 0.0001954311564186862781, 0.0003908623128373725562, 0.0005862934692560588072, 0.0007817246256747451124 ),
 .UNSPECIFIED. ) ;
#43478=EDGE_CURVE ( 'NONE', #61793, #30720, #48113, .T. ) ;
#43479=DIRECTION ( 'NONE',  ( 0.000000000000000000, 0.000000000000000000, 1.000000000000000000 ) ) ;
#43480=EDGE_LOOP ( 'NONE', ( #77665, #9035 ) ) ;
#43481=CYLINDRICAL_SURFACE ( 'NONE', #54137, 0.2499999999999993616 ) ;
#43483=CARTESIAN_POINT ( 'NONE',  ( 17.14299142792551578, -8.120952969808772792, 34.71129190929999453 ) ) ;
#43484=EDGE_CURVE ( 'NONE', #47571, #86693, #6170, .T. ) ;
#43485=CARTESIAN_POINT ( 'NONE',  ( 13.38461538461538680, -2.833524468853757305, 32.15551576947925838 ) ) ;
#43486=CARTESIAN_POINT ( 'NONE',  ( 16.08776377448601735, -8.164416787775445883, 34.95778746994557906 ) ) ;
#43487=CARTESIAN_POINT ( 'NONE',  ( -16.37733107841048508, -10.23692288466677880, 34.23039457007281072 ) ) ;
#43488=CARTESIAN_POINT ( 'NONE',  ( -13.60754234352223158, -8.282780595021769443, 34.94152052738834158 ) ) ;
#43489=CARTESIAN_POINT ( 'NONE',  ( 4.826899839630110378, -8.432397168068783699, 34.66272746175022945 ) ) ;
#43491=B_SPLINE_CURVE_WITH_KNOTS ( 'NONE', 3,
 ( #30300, #83934, #77159, #23098, #22217, #64955, #57767, #63638, #50561, #2368 ),
 .UNSPECIFIED., .F., .F.,
 ( 4, 2, 2, 2, 4 ),
 ( 0.000000000000000000, 0.0001954339857564072033, 0.0003908679715128144066, 0.0005863019572692215828, 0.0007817359430256288133 ),
 .UNSPECIFIED. ) ;
#43492=FACE_OUTER_BOUND ( 'NONE', #55978, .T. ) ;
#43495=CARTESIAN_POINT ( 'NONE',  ( 6.923076923076924238, -2.486705287966279876, 31.30864560766543647 ) ) ;
#43497=VECTOR ( 'NONE', #36614, 1000.000000000000000 ) ;
#43498=CARTESIAN_POINT ( 'NONE',  ( -14.30769230769230660, -10.51840700105979565, 33.73612834413961536 ) ) ;
#43500=ORIENTED_EDGE ( 'NONE', *, *, #86178, .T. ) ;
#43501=CARTESIAN_POINT ( 'NONE',  ( 14.43848411551709709, -4.809403383903225304, 33.96459661697924304 ) ) ;
#43502=CARTESIAN_POINT ( 'NONE',  ( -11.28840722682322628, -8.303483539816728154, 34.68545999027711702 ) ) ;
#43503=CARTESIAN_POINT ( 'NONE',  ( 9.757563263583719504, -6.879047030191282275, 34.71129190930002295 ) ) ;
#43504=CARTESIAN_POINT ( 'NONE',  ( 15.00788971403164496, -7.630690623152299956, 34.99857592706774057 ) ) ;
#43505=CARTESIAN_POINT ( 'NONE',  ( 13.63466969625370062, -2.564540009722896752, 30.55348353981670684 ) ) ;
#43506=VECTOR ( 'NONE', #53916, 1000.000000000000000 ) ;
#43507=CARTESIAN_POINT ( 'NONE',  ( -14.08467946359890988, -4.026326845037962343, 33.68677907613344047 ) ) ;
#43508=DIRECTION ( 'NONE',  ( 0.000000000000000000, 0.6427876096865368094, 0.7660444431189802339 ) ) ;
#43509=EDGE_CURVE ( 'NONE', #33104, #56650, #19088, .T. ) ;
#43511=EDGE_LOOP ( 'NONE', ( #11425, #15283, #37787, #8600 ) ) ;
#43512=EDGE_LOOP ( 'NONE', ( #52927, #37560 ) ) ;
#43513=CARTESIAN_POINT ( 'NONE',  ( 6.222962903561486847, -7.369474270740069777, 34.74850911626239736 ) ) ;
#43514=CYLINDRICAL_SURFACE ( 'NONE', #60471, 0.2499999999999997502 ) ;
#43515=CARTESIAN_POINT ( 'NONE',  ( 1.384615384615265343, -12.46129190930018460, 30.37095296980731973 ) ) ;
#43516=CARTESIAN_POINT ( 'NONE',  ( 10.74617505635156789, -9.929761469519743144, 34.40412654351204225 ) ) ;
#43517=VERTEX_POINT ( 'NONE', #3933 ) ;
#43518=LINE ( 'NONE', #80316, #68005 ) ;
#43519=EDGE_LOOP ( 'NONE', ( #11422, #29997 ) ) ;
#43520=VERTEX_POINT ( 'NONE', #57555 ) ;
#43521=CARTESIAN_POINT ( 'NONE',  ( 0.4615384615384611755, -1.367168528481310208, 33.57946703557072254 ) ) ;
#43523=B_SPLINE_CURVE_WITH_KNOTS ( 'NONE', 3,
 ( #36284, #25316, #30405, #63741, #44341, #57872, #46027, #11809, #2916, #87482 ),
 .UNSPECIFIED., .F., .F.,
 ( 4, 2, 2, 2, 4 ),
 ( 0.000000000000000000, 0.0001954339857564074473, 0.0003908679715128148945, 0.0005863019572692223418, 0.0007817359430256297891 ),
 .UNSPECIFIED. ) ;
#43525=DIRECTION ( 'NONE',  ( 0.000000000000000000, 0.6427876096865368094, 0.7660444431189802339 ) ) ;
#43526=CARTESIAN_POINT ( 'NONE',  ( -12.46153846153815437, -2.506253911140614576, 30.00000000000323297 ) ) ;
#43527=ORIENTED_EDGE ( 'NONE', *, *, #48854, .T. ) ;
#43528=ORIENTED_EDGE ( 'NONE', *, *, #84415, .T. ) ;
#43531=CARTESIAN_POINT ( 'NONE',  ( 1.319344938654610999, -8.613356846314824011, 34.62446782046655613 ) ) ;
#43534=CARTESIAN_POINT ( 'NONE',  ( 4.853996859406925601, -3.586966769969700763, 32.86292498521069660 ) ) ;
#43535=CARTESIAN_POINT ( 'NONE',  ( 2.307692307692309264, -9.058645607665452459, 34.76329471203371924 ) ) ;
#43536=EDGE_LOOP ( 'NONE', ( #25429, #42307, #72915, #52916 ) ) ;
#43537=CARTESIAN_POINT ( 'NONE',  ( -16.15384615384615330, -6.681629849574314051, 35.83090037661290239 ) ) ;
#43538=CARTESIAN_POINT ( 'NONE',  ( 4.946363163309711375, -2.254533558242299396, 29.97296025877828285 ) ) ;
#43539=ORIENTED_EDGE ( 'NONE', *, *, #25814, .F. ) ;
#43540=FACE_BOUND ( 'NONE', #657, .T. ) ;
#43541=CARTESIAN_POINT ( 'NONE',  ( 11.28843830116857383, -5.056417327199099532, 34.11270091957321426 ) ) ;
#43544=CARTESIAN_POINT ( 'NONE',  ( -17.77722033102192967, -2.612705202774696200, 31.66806509827799943 ) ) ;
#43545=FACE_OUTER_BOUND ( 'NONE', #58307, .T. ) ;
#43546=DIRECTION ( 'NONE',  ( -0.000000000000000000, 0.3420201433256694901, -0.9396926207859082059 ) ) ;
#43547=AXIS2_PLACEMENT_3D ( 'NONE', #34770, #61791, #74435 ) ;
#43548=CARTESIAN_POINT ( 'NONE',  ( -1.318548051265307830, -8.164416787775445883, 34.95778746994558617 ) ) ;
#43549=CARTESIAN_POINT ( 'NONE',  ( -39.05038313613820122, -2.499999999999999556, 29.75000000000000355 ) ) ;
#43550=ORIENTED_EDGE ( 'NONE', *, *, #20204, .F. ) ;
#43551=CARTESIAN_POINT ( 'NONE',  ( -10.68065506134539078, -10.21337939537584383, 33.94971097300158647 ) ) ;
#43552=CARTESIAN_POINT ( 'NONE',  ( 5.076923076922953193, -4.320704448113951379, 33.92786785259630022 ) ) ;
#43553=EDGE_LOOP ( 'NONE', ( #71379, #85278, #68672, #26294 ) ) ;
#43554=AXIS2_PLACEMENT_3D ( 'NONE', #19371, #79748, #32443 ) ;
#43555=EDGE_CURVE ( 'NONE', #67271, #40972, #43629, .T. ) ;
#43557=CARTESIAN_POINT ( 'NONE',  ( 10.48469314871705826, -6.413092428213692742, 34.63065189839063152 ) ) ;
#43558=CARTESIAN_POINT ( 'NONE',  ( 18.00000000000000000, -12.09954503811598769, 35.62045528018868623 ) ) ;
#43559=CARTESIAN_POINT ( 'NONE',  ( -5.076923076923197442, -11.94971097300221174, 32.03036669348237098 ) ) ;
#43560=CARTESIAN_POINT ( 'NONE',  ( -10.55012947587177941, -3.083524468853784839, 32.58852847137153930 ) ) ;
#43561=CARTESIAN_POINT ( 'NONE',  ( -8.068981943788728017, -7.369209533119140509, 34.99857337881830688 ) ) ;
#43562=FACE_BOUND ( 'NONE', #57850, .T. ) ;
#43563=CARTESIAN_POINT ( 'NONE',  ( 14.30769230769231015, -8.564572088678739092, 35.78748833219616898 ) ) ;
#43564=CARTESIAN_POINT ( 'NONE',  ( 17.07692307692307665, -6.435427911321262684, 35.78748833219616898 ) ) ;
#43565=CARTESIAN_POINT ( 'NONE',  ( -6.792285115252136407, -10.54018710029568595, 33.71981072465678864 ) ) ;
#43567=CARTESIAN_POINT ( 'NONE',  ( 6.923076923076924238, -12.37446782046654192, 30.86335684631486131 ) ) ;
#43569=B_SPLINE_CURVE_WITH_KNOTS ( 'NONE', 3,
 ( #45124, #72599, #23960, #58636, #18557, #78464, #57759, #52770, #31163, #38832 ),
 .UNSPECIFIED., .F., .F.,
 ( 4, 2, 2, 2, 4 ),
 ( 0.0007817359430256318490, 0.0009771253907249984917, 0.001172514838424365026, 0.001367904286123731560, 0.001563293733823098311 ),
 .UNSPECIFIED. ) ;
#43571=EDGE_LOOP ( 'NONE', ( #77833, #35143, #66958, #80974 ) ) ;
#43573=CARTESIAN_POINT ( 'NONE',  ( -4.403822884788507253, -11.79746400365624659, 32.30657167506340954 ) ) ;
#43574=LINE ( 'NONE', #9791, #51252 ) ;
#43575=CARTESIAN_POINT ( 'NONE',  ( -7.623374177175780808, -11.60474049983371003, 33.02348890104160262 ) ) ;
#43576=CARTESIAN_POINT ( 'NONE',  ( 10.86538461538461675, -2.499999999999998668, 29.75000000000000355 ) ) ;
#43577=ADVANCED_FACE ( 'NONE', ( #30528 ), #6174, .F. ) ;
#43580=CARTESIAN_POINT ( 'NONE',  ( -11.66907119366561396, -7.722926974430166069, 34.99546784045485737 ) ) ;
#43583=CARTESIAN_POINT ( 'NONE',  ( -7.911423846710166075, -3.083524468853724443, 32.58852847137143272 ) ) ;
#43584=DIRECTION ( 'NONE',  ( -0.000000000000000000, -0.6427876096865404731, -0.7660444431189771253 ) ) ;
#43586=CARTESIAN_POINT ( 'NONE',  ( 3.930919936330007136, -10.61292498521070549, 33.66303323003028680 ) ) ;
#43588=CARTESIAN_POINT ( 'NONE',  ( 10.83881101429940408, -7.630147987733840509, 34.99859428049665411 ) ) ;
#43589=EDGE_CURVE ( 'NONE', #78986, #69985, #62918, .T. ) ;
#43590=CARTESIAN_POINT ( 'NONE',  ( 17.20744851515672025, -2.647132371071621471, 31.75357179365173010 ) ) ;
#43592=CARTESIAN_POINT ( 'NONE',  ( 3.480823650682684622, -12.41089969410671223, 31.60739465890703670 ) ) ;
#43593=CARTESIAN_POINT ( 'NONE',  ( -5.776987155906605054, -2.523321265292115090, 31.42251411153756280 ) ) ;
#43595=CARTESIAN_POINT ( 'NONE',  ( 6.673053698855467175, -4.931416488878822335, 34.32920672191015399 ) ) ;
#43596=CARTESIAN_POINT ( 'NONE',  ( -16.94639763868943660, -5.915461855592777596, 34.75538340440931506 ) ) ;
#43597=VERTEX_POINT ( 'NONE', #61545 ) ;
#43598=CARTESIAN_POINT ( 'NONE',  ( -17.86947456176635640, -6.808710257144159783, 34.95449254468098843 ) ) ;
#43599=CARTESIAN_POINT ( 'NONE',  ( 3.903869422903799347, -5.728515186090277211, 34.42611988154120439 ) ) ;
#43602=CARTESIAN_POINT ( 'NONE',  ( -12.46153846153846168, -1.367168528481310208, 33.57946703557072254 ) ) ;
#43603=CARTESIAN_POINT ( 'NONE',  ( -5.076923076923197442, -11.48612834414049644, 32.76840700105863391 ) ) ;
#43604=B_SPLINE_CURVE_WITH_KNOTS ( 'NONE', 3,
 ( #34401, #61863, #55117, #82614, #60988, #12804, #20883, #76271, #88490, #54222 ),
 .UNSPECIFIED., .F., .F.,
 ( 4, 2, 2, 2, 4 ),
 ( 0.000000000000000000, 0.0001954311564186864407, 0.0003908623128373728815, 0.0005862934692560593493, 0.0007817246256747457630 ),
 .UNSPECIFIED. ) ;
#43605=B_SPLINE_CURVE_WITH_KNOTS ( 'NONE', 3,
 ( #76661, #29808, #57271, #85195, #64015, #2751, #84761, #69898, #35685, #57715 ),
 .UNSPECIFIED., .F., .F.,
 ( 4, 2, 2, 2, 4 ),
 ( 0.000000000000000000, 0.0001954339857564126514, 0.0003908679715128183098, 0.0005863019572692239681, 0.0007817359430256294638 ),
 .UNSPECIFIED. ) ;
#43606=CARTESIAN_POINT ( 'NONE',  ( 12.46153846153833911, -8.613356846316285953, 34.62446782046622218 ) ) ;
#43608=CARTESIAN_POINT ( 'NONE',  ( -11.53846153846165912, -4.481592998941358097, 33.73612834414048933 ) ) ;
#43609=DIRECTION ( 'NONE',  ( -0.000000000000000000, -0.1736481776669307198, -0.9848077530122080203 ) ) ;
#43610=EDGE_CURVE ( 'NONE', #58985, #41090, #18357, .T. ) ;
#43611=CARTESIAN_POINT ( 'NONE',  ( 9.915320536401090123, -6.460100341425560444, 34.89618726649961644 ) ) ;
#43613=ADVANCED_FACE ( 'NONE', ( #73299 ), #53459, .F. ) ;
#43614=VERTEX_POINT ( 'NONE', #11603 ) ;
#43615=AXIS2_PLACEMENT_3D ( 'NONE', #86792, #3450, #39034 ) ;
#43616=VERTEX_POINT ( 'NONE', #39970 ) ;
#43619=CARTESIAN_POINT ( 'NONE',  ( 7.846153846153846700, -1.242168528481310874, 33.36296068462461051 ) ) ;
#43620=CARTESIAN_POINT ( 'NONE',  ( 13.63456079399343146, -3.520799739797214389, 33.17531984108286025 ) ) ;
#43621=EDGE_CURVE ( 'NONE', #20169, #77592, #20130, .T. ) ;
#43623=DIRECTION ( 'NONE',  ( -0.000000000000000000, 0.9396926207859093161, -0.3420201433256663259 ) ) ;
#43624=VERTEX_POINT ( 'NONE', #67431 ) ;
#43625=ORIENTED_EDGE ( 'NONE', *, *, #84515, .T. ) ;
#43626=CARTESIAN_POINT ( 'NONE',  ( -1.449939397419692355, -7.749976730030849303, 34.74374725381503737 ) ) ;
#43627=VERTEX_POINT ( 'NONE', #88615 ) ;
#43628=CARTESIAN_POINT ( 'NONE',  ( 9.822833394071260216, -12.45806712695776319, 30.39783852428763922 ) ) ;
#43629=B_SPLINE_CURVE_WITH_KNOTS ( 'NONE', 3,
 ( #72841, #85480, #11148, #10709, #85046, #17017, #65194, #3493, #24661, #79613 ),
 .UNSPECIFIED., .F., .F.,
 ( 4, 2, 2, 2, 4 ),
 ( 0.000000000000000000, 0.0001954339857564072304, 0.0003908679715128144608, 0.0005863019572692216913, 0.0007817359430256289217 ),
 .UNSPECIFIED. ) ;
#43630=B_SPLINE_CURVE_WITH_KNOTS ( 'NONE', 3,
 ( #76021, #57077, #55306, #8905, #36375, #14325, #15662, #83235, #28737, #21071 ),
 .UNSPECIFIED., .F., .F.,
 ( 4, 2, 2, 2, 4 ),
 ( 0.000000000000000000, 0.0001954311564186868473, 0.0003908623128373736946, 0.0005862934692560605419, 0.0007817246256747473893 ),
 .UNSPECIFIED. ) ;
#43631=CARTESIAN_POINT ( 'NONE',  ( -17.93393164899755732, -3.050289026998447728, 32.03036669348366416 ) ) ;
#43633=VERTEX_POINT ( 'NONE', #53911 ) ;
#43634=B_SPLINE_CURVE_WITH_KNOTS ( 'NONE', 3,
 ( #74056, #6042, #12347, #34384, #160, #19543, #27630, #19108, #26303, #67295 ),
 .UNSPECIFIED., .F., .F.,
 ( 4, 2, 2, 2, 4 ),
 ( 0.0007817246256747461966, 0.0009771112852218889842, 0.001172497944769031880, 0.001367884604316174776, 0.001563271263863317672 ),
 .UNSPECIFIED. ) ;
#43635=ORIENTED_EDGE ( 'NONE', *, *, #50449, .T. ) ;
#43636=CARTESIAN_POINT ( 'NONE',  ( -39.05038313613820122, -12.75000000000000178, 27.25000000000000000 ) ) ;
#43637=ORIENTED_EDGE ( 'NONE', *, *, #21445, .T. ) ;
#43639=CARTESIAN_POINT ( 'NONE',  ( -6.000000000000119904, -8.613356846316285953, 34.62446782046622218 ) ) ;
#43640=EDGE_CURVE ( 'NONE', #83562, #34160, #60663, .T. ) ;
#43642=ORIENTED_EDGE ( 'NONE', *, *, #63704, .F. ) ;
#43643=CARTESIAN_POINT ( 'NONE',  ( 17.93391658904412012, -10.51840700105979565, 33.73612834413961536 ) ) ;
#43645=CARTESIAN_POINT ( 'NONE',  ( 10.68064018666064285, -3.835265460703683349, 33.15142922261929925 ) ) ;
#43646=FACE_BOUND ( 'NONE', #78077, .T. ) ;
#43647=LINE ( 'NONE', #58044, #70058 ) ;
#43648=CARTESIAN_POINT ( 'NONE',  ( -4.376772371362299019, -12.15238873228292071, 31.58232369045353849 ) ) ;
#43649=CARTESIAN_POINT ( 'NONE',  ( -14.98082371242109012, -10.76462480002816235, 33.53768742498949962 ) ) ;
#43650=CARTESIAN_POINT ( 'NONE',  ( -0.2114840416250086119, -2.920487667080175154, 32.31805714834172250 ) ) ;
#43651=CARTESIAN_POINT ( 'NONE',  ( 4.376625822824220080, -2.353885683473779800, 30.79025554430704759 ) ) ;
#43652=CARTESIAN_POINT ( 'NONE',  ( 8.769230769230768274, -9.058645607665452459, 34.76329471203371924 ) ) ;
#43653=CARTESIAN_POINT ( 'NONE',  ( 10.39189969082028675, -10.97335522853832579, 33.68706563782419749 ) ) ;
#43654=ORIENTED_EDGE ( 'NONE', *, *, #73434, .F. ) ;
#43655=CARTESIAN_POINT ( 'NONE',  ( -15.93083330975275658, -3.395485233115139501, 33.02377354290276656 ) ) ;
#43656=VERTEX_POINT ( 'NONE', #60218 ) ;
#43657=VERTEX_POINT ( 'NONE', #53008 ) ;
#43658=EDGE_CURVE ( 'NONE', #51433, #9533, #66992, .T. ) ;
#43659=CARTESIAN_POINT ( 'NONE',  ( 7.780883400193072674, -6.879047030191174805, 34.71129190930000163 ) ) ;
#43660=LINE ( 'NONE', #71131, #72124 ) ;
#43661=CARTESIAN_POINT ( 'NONE',  ( 2.557637826040451312, -2.587454068350147907, 30.68340429815432202 ) ) ;
#43662=DIRECTION ( 'NONE',  ( -0.000000000000000000, 0.6427876096865404731, -0.7660444431189770143 ) ) ;
#43663=CARTESIAN_POINT ( 'NONE',  ( -15.23076923076922995, -3.937682226553329556, 33.60647404775216529 ) ) ;
#43664=CARTESIAN_POINT ( 'NONE',  ( -0.2115929431903184610, -11.86320923018887719, 32.19269448109604781 ) ) ;
#43665=ORIENTED_EDGE ( 'NONE', *, *, #10745, .T. ) ;
#43666=CARTESIAN_POINT ( 'NONE',  ( -18.00000000000012079, -6.026961402154117131, 34.52809138561165270 ) ) ;
#43668=CARTESIAN_POINT ( 'NONE',  ( 14.98079248672064345, -10.82459398097509329, 33.81372124010185587 ) ) ;
#43669=CARTESIAN_POINT ( 'NONE',  ( 7.846153846153846700, -13.49023893513002648, 31.06009739812518688 ) ) ;
#43670=DIRECTION ( 'NONE',  ( -0.000000000000000000, -0.5000000000000009992, -0.8660254037844380415 ) ) ;
#43671=CARTESIAN_POINT ( 'NONE',  ( 13.38461538461526423, -5.941354392335915335, 34.76329471203413846 ) ) ;
#43673=EDGE_LOOP ( 'NONE', ( #36883, #65062, #88201, #60985 ) ) ;
#43674=AXIS2_PLACEMENT_3D ( 'NONE', #13260, #27214, #81287 ) ;
#43675=ORIENTED_EDGE ( 'NONE', *, *, #29470, .T. ) ;
#43676=AXIS2_PLACEMENT_3D ( 'NONE', #83666, #42668, #27671 ) ;
#43677=EDGE_CURVE ( 'NONE', #46850, #13379, #80509, .T. ) ;
#43678=CARTESIAN_POINT ( 'NONE',  ( -9.561781990544128362, -12.45806712695776319, 30.39783852428763922 ) ) ;
#43679=EDGE_LOOP ( 'NONE', ( #79512, #11286 ) ) ;
#43681=CARTESIAN_POINT ( 'NONE',  ( 9.915319043920545639, -9.886259254753566594, 34.14407573483972413 ) ) ;
#43684=CARTESIAN_POINT ( 'NONE',  ( -8.546219417617919589, -10.61302985866383963, 33.66295027996417843 ) ) ;
#43686=LINE ( 'NONE', #84697, #80592 ) ;
#43687=VERTEX_POINT ( 'NONE', #19682 ) ;
#43688=CARTESIAN_POINT ( 'NONE',  ( 1.384615384615386802, -13.95598074871891292, 31.83374038241031911 ) ) ;
#43689=CARTESIAN_POINT ( 'NONE',  ( -2.084679463598910765, -12.64618726649961289, 30.78989965857442712 ) ) ;
#43690=ORIENTED_EDGE ( 'NONE', *, *, #23750, .T. ) ;
#43691=CYLINDRICAL_SURFACE ( 'NONE', #2285, 0.2500000000000009437 ) ;
#43692=CYLINDRICAL_SURFACE ( 'NONE', #32897, 0.2499999999999997502 ) ;
#43693=CARTESIAN_POINT ( 'NONE',  ( 3.230769230769231726, -13.20930481340135110, 34.54067556320372745 ) ) ;
#43694=CARTESIAN_POINT ( 'NONE',  ( 0.6845498131513093609, -2.758310577978207334, 31.33698337089302299 ) ) ;
#43696=CARTESIAN_POINT ( 'NONE',  ( -12.71151519248081740, -12.41269422305637171, 30.68257228309993323 ) ) ;
#43697=CARTESIAN_POINT ( 'NONE',  ( -11.47320639894870276, -3.083524468853784839, 32.58852847137153930 ) ) ;
#43699=ORIENTED_EDGE ( 'NONE', *, *, #18930, .F. ) ;
#43700=CARTESIAN_POINT ( 'NONE',  ( 1.134638653673032849, -5.728515186090277211, 34.42611988154120439 ) ) ;
#43701=CARTESIAN_POINT ( 'NONE',  ( 4.376858997939548246, -10.77377354290276301, 33.85451476688484718 ) ) ;
#43703=ADVANCED_FACE ( 'NONE', ( #12926 ), #40414, .F. ) ;
#43704=CARTESIAN_POINT ( 'NONE',  ( -15.23076923076922995, -8.120952969808772792, 34.71129190930000163 ) ) ;
#43705=CARTESIAN_POINT ( 'NONE',  ( 2.557637717070351258, -12.07971442181321997, 32.31769673815850297 ) ) ;
#43706=EDGE_LOOP ( 'NONE', ( #79247, #77259 ) ) ;
#43707=FACE_OUTER_BOUND ( 'NONE', #14023, .T. ) ;
#43708=CARTESIAN_POINT ( 'NONE',  ( -17.07692307692307665, -2.499999999999998668, 29.50000000000001066 ) ) ;
#43709=EDGE_CURVE ( 'NONE', #40731, #24676, #26448, .T. ) ;
#43710=VERTEX_POINT ( 'NONE', #13366 ) ;
#43712=CARTESIAN_POINT ( 'NONE',  ( -3.930833309752757909, -2.523321265292115090, 31.42251411153756280 ) ) ;
#43714=EDGE_LOOP ( 'NONE', ( #39591, #40633 ) ) ;
#43715=CARTESIAN_POINT ( 'NONE',  ( 6.923076923076924238, -10.89733346790207413, 36.13435417666054406 ) ) ;
#43716=CARTESIAN_POINT ( 'NONE',  ( 2.980746006547775107, -4.175268141568689195, 33.81360843649122216 ) ) ;
#43717=EDGE_CURVE ( 'NONE', #40179, #24050, #2778, .T. ) ;
#43718=CARTESIAN_POINT ( 'NONE',  ( -1.384615384615383471, -4.098570777380720287, 33.41473453929634729 ) ) ;
#43719=CARTESIAN_POINT ( 'NONE',  ( -4.219928533206288357, -11.35647404775217595, 33.31231777344666511 ) ) ;
#43720=ORIENTED_EDGE ( 'NONE', *, *, #81722, .F. ) ;
#43721=CARTESIAN_POINT ( 'NONE',  ( -3.230769230769352962, -2.379036618888197285, 30.90682066428292885 ) ) ;
#43722=VERTEX_POINT ( 'NONE', #62424 ) ;
#43723=CARTESIAN_POINT ( 'NONE',  ( -39.05038313613820122, -12.50000000000000000, 29.75000000000000355 ) ) ;
#43724=CARTESIAN_POINT ( 'NONE',  ( 9.692307692307695177, -3.886160181151819604, 36.00935417666054406 ) ) ;
#43726=EDGE_CURVE ( 'NONE', #5488, #11611, #44741, .T. ) ;
#43728=CARTESIAN_POINT ( 'NONE',  ( 5.076923076922954969, -10.90142922262034020, 33.41473453929536674 ) ) ;
#43729=CARTESIAN_POINT ( 'NONE',  ( -39.05038313613820122, -2.249999999999998668, 29.75000000000000355 ) ) ;
#43731=CARTESIAN_POINT ( 'NONE',  ( -14.30769230769230660, -12.78798330534102945, 29.74999999999997868 ) ) ;
#43732=B_SPLINE_CURVE_WITH_KNOTS ( 'NONE', 3,
 ( #85995, #10780, #38249, #58957, #86461, #24735, #5802, #33279, #46340, #59410 ),
 .UNSPECIFIED., .F., .F.,
 ( 4, 2, 2, 2, 4 ),
 ( 0.000000000000000000, 0.0001954339857564078267, 0.0003908679715128156535, 0.0005863019572692235344, 0.0007817359430256313069 ),
 .UNSPECIFIED. ) ;
#43733=B_SPLINE_CURVE_WITH_KNOTS ( 'NONE', 3,
 ( #5, #40116, #40556, #7203, #13071, #68022, #47739, #27475, #6749, #54489 ),
 .UNSPECIFIED., .F., .F.,
 ( 4, 2, 2, 2, 4 ),
 ( 0.0007817246336856291692, 0.0009771112958940105907, 0.001172497958102391904, 0.001367884620310773434, 0.001563271282519154747 ),
 .UNSPECIFIED. ) ;
#43734=ORIENTED_EDGE ( 'NONE', *, *, #3194, .F. ) ;
#43736=FACE_BOUND ( 'NONE', #76586, .T. ) ;
#43737=B_SPLINE_CURVE_WITH_KNOTS ( 'NONE', 3,
 ( #78686, #24173, #72362, #64712, #38588, #86354, #25071, #51625, #65157, #3011 ),
 .UNSPECIFIED., .F., .F.,
 ( 4, 2, 2, 2, 4 ),
 ( 0.0007817246256747459798, 0.0009771112852218896347, 0.001172497944769033181, 0.001367884604316176728, 0.001563271263863320491 ),
 .UNSPECIFIED. ) ;
#43738=EDGE_LOOP ( 'NONE', ( #26625, #6327, #53576, #66751 ) ) ;
#43740=EDGE_CURVE ( 'NONE', #42183, #53607, #63763, .T. ) ;
#43742=VECTOR ( 'NONE', #59830, 1000.000000000000000 ) ;
#43744=CARTESIAN_POINT ( 'NONE',  ( 9.626224281351813516, -12.10708131394839349, 31.69288490824020244 ) ) ;
#43745=CARTESIAN_POINT ( 'NONE',  ( -14.30769230769242739, -9.442884908241554243, 34.35708131394783038 ) ) ;
#43746=EDGE_LOOP ( 'NONE', ( #76767, #44957 ) ) ;
#43747=ORIENTED_EDGE ( 'NONE', *, *, #44950, .T. ) ;
#43748=CARTESIAN_POINT ( 'NONE',  ( 16.82689983963011926, -4.335965774309648246, 33.62209801155881905 ) ) ;
#43750=CARTESIAN_POINT ( 'NONE',  ( 2.057692307692309708, -7.566082377512563184, 35.00000000000000711 ) ) ;
#43751=EDGE_CURVE ( 'NONE', #77592, #1771, #8241, .T. ) ;
#43752=CARTESIAN_POINT ( 'NONE',  ( -5.076923076923199218, -5.094484230521993062, 34.41647553114689373 ) ) ;
#43753=CARTESIAN_POINT ( 'NONE',  ( 14.05771556364372188, -12.01397095200674059, 32.43157075238190146 ) ) ;
#43754=EDGE_CURVE ( 'NONE', #21774, #44514, #68364, .T. ) ;
#43755=FACE_BOUND ( 'NONE', #63932, .T. ) ;
#43756=VERTEX_POINT ( 'NONE', #49372 ) ;
#43757=CARTESIAN_POINT ( 'NONE',  ( 12.68454981315131391, -5.667800583137506010, 34.40243808032445827 ) ) ;
#43758=ADVANCED_FACE ( 'NONE', ( #41294 ), #56572, .F. ) ;
#43760=CARTESIAN_POINT ( 'NONE',  ( 10.61538461538449418, -5.094484230521993062, 34.41647553114689373 ) ) ;
#43761=CARTESIAN_POINT ( 'NONE',  ( -1.318548051265308052, -2.833524468853757750, 32.15551576947925838 ) ) ;
#43762=ORIENTED_EDGE ( 'NONE', *, *, #47770, .T. ) ;
#43764=ORIENTED_EDGE ( 'NONE', *, *, #43087, .T. ) ;
#43765=VERTEX_POINT ( 'NONE', #7055 ) ;
#43766=EDGE_CURVE ( 'NONE', #25678, #58364, #15148, .T. ) ;
#43767=B_SPLINE_CURVE_WITH_KNOTS ( 'NONE', 3,
 ( #12085, #18386, #3962, #31448, #86423, #45846, #32343, #59809, #24692, #52151 ),
 .UNSPECIFIED., .F., .F.,
 ( 4, 2, 2, 2, 4 ),
 ( 0.000000000000000000, 0.0001954311564186864407, 0.0003908623128373728815, 0.0005862934692560593493, 0.0007817246256747457630 ),
 .UNSPECIFIED. ) ;
#43768=VECTOR ( 'NONE', #14109, 1000.000000000000114 ) ;
#43769=CARTESIAN_POINT ( 'NONE',  ( -6.923076923077044142, -10.21337939537710326, 33.94971097300076224 ) ) ;
#43770=CARTESIAN_POINT ( 'NONE',  ( -18.00000000000000000, -4.112162358433185005, 36.11790692298802696 ) ) ;
#43771=CARTESIAN_POINT ( 'NONE',  ( -10.86536134632696715, -12.17611988154120972, 31.52148481390971213 ) ) ;
#43772=CARTESIAN_POINT ( 'NONE',  ( -6.857821351800897247, -3.835265460703683349, 33.15142922261929925 ) ) ;
#43773=FACE_OUTER_BOUND ( 'NONE', #77255, .T. ) ;
#43774=CARTESIAN_POINT ( 'NONE',  ( -15.48079245499068435, -3.520140089381495585, 33.17453946501458262 ) ) ;
#43775=ORIENTED_EDGE ( 'NONE', *, *, #46014, .F. ) ;
#43776=CARTESIAN_POINT ( 'NONE',  ( -3.007989689500820241, -2.600157965045225783, 30.74683119005207743 ) ) ;
#43777=CARTESIAN_POINT ( 'NONE',  ( 3.230769230769231726, -9.058645607665452459, 34.76329471203371924 ) ) ;
#43778=CARTESIAN_POINT ( 'NONE',  ( -17.14219352288385778, -11.94971097300153140, 32.03036669348370680 ) ) ;
#43779=CARTESIAN_POINT ( 'NONE',  ( -4.153846153846152411, -3.669653830205710676, 35.88435417666054406 ) ) ;
#43780=ORIENTED_EDGE ( 'NONE', *, *, #20179, .T. ) ;
#43781=DIRECTION ( 'NONE',  ( 0.000000000000000000, 0.9848077530122072432, 0.1736481776669354937 ) ) ;
#43782=ORIENTED_EDGE ( 'NONE', *, *, #6205, .F. ) ;
#43783=FACE_BOUND ( 'NONE', #16225, .T. ) ;
#43784=CARTESIAN_POINT ( 'NONE',  ( 4.153846153846154188, -2.486705287966279876, 31.30864560766543647 ) ) ;
#43786=ORIENTED_EDGE ( 'NONE', *, *, #61024, .T. ) ;
#43787=CARTESIAN_POINT ( 'NONE',  ( -7.623142494540996239, -4.187068189119696804, 33.49521262558774026 ) ) ;
#43788=CARTESIAN_POINT ( 'NONE',  ( -2.176900499867519212, -4.118422570099827595, 33.43335022499816489 ) ) ;
#43789=CARTESIAN_POINT ( 'NONE',  ( 5.076923076923075762, -2.900454961884010974, 35.62045528018868623 ) ) ;
#43790=ADVANCED_FACE ( 'NONE', ( #1635 ), #8389, .F. ) ;
#43791=CYLINDRICAL_SURFACE ( 'NONE', #76206, 0.2500000000000004996 ) ;
#43793=CYLINDRICAL_SURFACE ( 'NONE', #30167, 0.2499999999999995559 ) ;
#43794=ORIENTED_EDGE ( 'NONE', *, *, #60360, .T. ) ;
#43795=DIRECTION ( 'NONE',  ( -0.000000000000000000, 0.8660254037844397068, -0.4999999999999978906 ) ) ;
#43797=CARTESIAN_POINT ( 'NONE',  ( 3.230769230769110045, -2.625532179533779154, 30.86335684631627174 ) ) ;
#43798=CARTESIAN_POINT ( 'NONE',  ( 15.00784301325307979, -2.758268499246657068, 31.33685645148948140 ) ) ;
#43799=CARTESIAN_POINT ( 'NONE',  ( -7.715363405186892898, -3.338503747796866872, 32.95102852606553512 ) ) ;
#43800=CARTESIAN_POINT ( 'NONE',  ( -12.59168643127016374, -11.04286588640298561, 33.62463336215343901 ) ) ;
#43801=DIRECTION ( 'NONE',  ( -0.000000000000000000, -0.6427876096865404731, -0.7660444431189771253 ) ) ;
#43802=AXIS2_PLACEMENT_3D ( 'NONE', #14096, #54180, #34359 ) ;
#43805=ORIENTED_EDGE ( 'NONE', *, *, #49102, .F. ) ;
#43807=CARTESIAN_POINT ( 'NONE',  ( 6.923076923076924238, -1.129524287112498415, 32.06866353760679544 ) ) ;
#43809=ORIENTED_EDGE ( 'NONE', *, *, #12844, .T. ) ;
#43810=VECTOR ( 'NONE', #52878, 1000.000000000000227 ) ;
#43811=ORIENTED_EDGE ( 'NONE', *, *, #84070, .F. ) ;
#43812=ORIENTED_EDGE ( 'NONE', *, *, #47227, .T. ) ;
#43813=CARTESIAN_POINT ( 'NONE',  ( 4.023698944407930078, -12.27039167877662251, 31.24851455888617835 ) ) ;
#43814=CARTESIAN_POINT ( 'NONE',  ( 3.230769230769231726, -1.951392089020283160, 34.73218667398347748 ) ) ;
#43817=DIRECTION ( 'NONE',  ( -0.000000000000000000, -0.3420201433256694346, -0.9396926207859080948 ) ) ;
#43818=CARTESIAN_POINT ( 'NONE',  ( -17.01085574357300345, -11.35647404775217595, 33.31231777344667222 ) ) ;
#43819=CARTESIAN_POINT ( 'NONE',  ( 6.223426398914789992, -7.630147987733840509, 34.99859428049665411 ) ) ;
#43820=ORIENTED_EDGE ( 'NONE', *, *, #85776, .T. ) ;
#43821=CARTESIAN_POINT ( 'NONE',  ( -3.930834802233303282, -5.667800583137508674, 34.40243808032445827 ) ) ;
#43822=CARTESIAN_POINT ( 'NONE',  ( -17.14219352288385423, -12.27809138561121394, 31.22303859784730307 ) ) ;
#43823=EDGE_CURVE ( 'NONE', #47862, #66121, #9707, .T. ) ;
#43824=CARTESIAN_POINT ( 'NONE',  ( -8.834500769787091201, -11.67786785259540849, 32.92929555188721480 ) ) ;
#43825=CARTESIAN_POINT ( 'NONE',  ( 12.46153846153846168, -11.69971097300155272, 32.46337939537588113 ) ) ;
#43827=CYLINDRICAL_SURFACE ( 'NONE', #38401, 0.2499999999999979738 ) ;
#43828=EDGE_CURVE ( 'NONE', #72161, #46109, #71541, .T. ) ;
#43830=CARTESIAN_POINT ( 'NONE',  ( 8.899756207464410096, -3.068774925481848825, 32.56582465632704526 ) ) ;
#43831=CARTESIAN_POINT ( 'NONE',  ( -7.846153846153844924, -13.75783147151868846, 33.36296068462461051 ) ) ;
#43833=CARTESIAN_POINT ( 'NONE',  ( 12.52760681254089903, -10.51840700105979565, 33.73612834413962247 ) ) ;
#43834=ORIENTED_EDGE ( 'NONE', *, *, #8168, .F. ) ;
#43837=CARTESIAN_POINT ( 'NONE',  ( 9.692307692307695177, -5.557115091759785130, 34.35708131394839171 ) ) ;
#43838=CARTESIAN_POINT ( 'NONE',  ( -12.21153846153702638, -7.500000000000155431, 34.75000000000007105 ) ) ;
#43839=VECTOR ( 'NONE', #50562, 999.9999999999998863 ) ;
#43840=EDGE_CURVE ( 'NONE', #62614, #27628, #64639, .T. ) ;
#43841=CARTESIAN_POINT ( 'NONE',  ( -8.992715693795100051, -9.417330523894424488, 34.63758898049880486 ) ) ;
#43842=B_SPLINE_CURVE_WITH_KNOTS ( 'NONE', 3,
 ( #29972, #2050, #56990, #57431, #23208, #77707, #49790, #84482, #83604, #50669 ),
 .UNSPECIFIED., .F., .F.,
 ( 4, 2, 2, 2, 4 ),
 ( 0.0007817246256747481482, 0.0009771112852218911526, 0.001172497944769034049, 0.001367884604316176944, 0.001563271263863319840 ),
 .UNSPECIFIED. ) ;
#43843=ORIENTED_EDGE ( 'NONE', *, *, #70057, .T. ) ;
#43844=CARTESIAN_POINT ( 'NONE',  ( 16.40379156322419973, -10.18230066228895758, 34.26354781536631577 ) ) ;
#43845=ORIENTED_EDGE ( 'NONE', *, *, #43978, .F. ) ;
#43847=CARTESIAN_POINT ( 'NONE',  ( 4.826946345980721809, -12.17611988154120972, 31.52148481390971213 ) ) ;
#43848=CARTESIAN_POINT ( 'NONE',  ( 7.053602361310566948, -3.068774925481847937, 32.56582465632704526 ) ) ;
#43849=CARTESIAN_POINT ( 'NONE',  ( -6.066083410955879884, -2.538708090699994813, 30.37095296980875148 ) ) ;
#43850=CARTESIAN_POINT ( 'NONE',  ( 1.253924781505079356, -8.191372820521381826, 34.95448215188423546 ) ) ;
#43851=CARTESIAN_POINT ( 'NONE',  ( 5.076923076922954969, -11.94971097300221174, 32.03036669348237098 ) ) ;
#43852=ORIENTED_EDGE ( 'NONE', *, *, #29382, .T. ) ;
#43853=ORIENTED_EDGE ( 'NONE', *, *, #45342, .T. ) ;
#43854=ORIENTED_EDGE ( 'NONE', *, *, #20083, .F. ) ;
#43856=CARTESIAN_POINT ( 'NONE',  ( -10.36543909703647337, -8.433404298154334455, 34.66254593164985920 ) ) ;
#43858=EDGE_CURVE ( 'NONE', #11982, #8529, #28658, .T. ) ;
#43859=CARTESIAN_POINT ( 'NONE',  ( -12.33101302330481985, -12.50538340440932394, 31.33453814440721885 ) ) ;
#43860=CARTESIAN_POINT ( 'NONE',  ( -13.31935981333936070, -6.026961402152789304, 34.52809138561124769 ) ) ;
#43862=FACE_OUTER_BOUND ( 'NONE', #84318, .T. ) ;
#43863=EDGE_CURVE ( 'NONE', #82908, #2182, #81308, .T. ) ;
#43864=CARTESIAN_POINT ( 'NONE',  ( 10.61538461538461675, -9.058645607665452459, 34.76329471203371924 ) ) ;
#43865=DIRECTION ( 'NONE',  ( 0.000000000000000000, 0.9396926207859126468, -0.3420201433256571111 ) ) ;
#43866=ORIENTED_EDGE ( 'NONE', *, *, #72651, .T. ) ;
#43868=ORIENTED_EDGE ( 'NONE', *, *, #71932, .T. ) ;
#43869=ORIENTED_EDGE ( 'NONE', *, *, #2376, .T. ) ;
#43870=CARTESIAN_POINT ( 'NONE',  ( 11.76147438255493327, -2.523321265292115534, 31.42251411153756990 ) ) ;
#43872=ORIENTED_EDGE ( 'NONE', *, *, #37149, .T. ) ;
#43873=CARTESIAN_POINT ( 'NONE',  ( -9.942284423250045577, -9.148715823498378086, 34.47080413974185120 ) ) ;
#43874=CARTESIAN_POINT ( 'NONE',  ( -10.61538461538473577, -6.835583212225970762, 34.95778746994575670 ) ) ;
#43875=CARTESIAN_POINT ( 'NONE',  ( 8.835399910193425299, -7.250054483168843156, 34.74374881642865631 ) ) ;
#43878=EDGE_CURVE ( 'NONE', #41031, #65326, #44816, .T. ) ;
#43879=ORIENTED_EDGE ( 'NONE', *, *, #20145, .T. ) ;
#43881=EDGE_LOOP ( 'NONE', ( #51758, #5460, #72615, #51360 ) ) ;
#43882=FACE_BOUND ( 'NONE', #40305, .T. ) ;
#43883=CARTESIAN_POINT ( 'NONE',  ( 13.60739505359344825, -12.47679350104403007, 31.42216943046555855 ) ) ;
#43884=LINE ( 'NONE', #47432, #70689 ) ;
#43885=ORIENTED_EDGE ( 'NONE', *, *, #1424, .F. ) ;
#43886=CARTESIAN_POINT ( 'NONE',  ( -4.403846153846151523, -2.499999999999998668, 29.75000000000000355 ) ) ;
#43887=CARTESIAN_POINT ( 'NONE',  ( 3.361561038594016004, -3.062576670634119758, 32.05464942895959979 ) ) ;
#43888=CARTESIAN_POINT ( 'NONE',  ( 18.00000000000030553, -2.506253911140615021, 30.00000000000323297 ) ) ;
#43889=ORIENTED_EDGE ( 'NONE', *, *, #33726, .T. ) ;
#43890=CARTESIAN_POINT ( 'NONE',  ( 1.634615384615386580, -2.249999999999998668, 29.75000000000000355 ) ) ;
#43891=CARTESIAN_POINT ( 'NONE',  ( -13.16183584334697443, -11.89424750095246175, 32.13594075562311758 ) ) ;
#43892=ADVANCED_FACE ( 'NONE', ( #64195 ), #9281, .F. ) ;
#43893=VERTEX_POINT ( 'NONE', #86284 ) ;
#43894=VECTOR ( 'NONE', #24296, 1000.000000000000227 ) ;
#43895=CARTESIAN_POINT ( 'NONE',  ( 3.230769230769231726, -8.120952969808772792, 34.71129190930000163 ) ) ;
#43896=PLANE ( 'NONE',  #38693 ) ;
#43897=CARTESIAN_POINT ( 'NONE',  ( 2.177544337960616527, -12.15440758774515473, 32.17923288041532004 ) ) ;
#43898=CARTESIAN_POINT ( 'NONE',  ( 15.93091919493929964, -2.889293201056495786, 32.26117774369186009 ) ) ;
#43899=CARTESIAN_POINT ( 'NONE',  ( -0.4615384615384611200, -4.661471528628507777, 34.16647553114623292 ) ) ;
#43900=EDGE_CURVE ( 'NONE', #26375, #19635, #24150, .T. ) ;
#43902=EDGE_CURVE ( 'NONE', #45619, #4994, #88821, .T. ) ;
#43903=CARTESIAN_POINT ( 'NONE',  ( 7.911408985666682270, -3.083524468853784839, 32.58852847137153930 ) ) ;
#43904=B_SPLINE_CURVE_WITH_KNOTS ( 'NONE', 3,
 ( #38316, #31096, #85611, #80195, #51341, #64880, #78844, #86060, #18495, #11738 ),
 .UNSPECIFIED., .F., .F.,
 ( 4, 2, 2, 2, 4 ),
 ( 0.000000000000000000, 0.0001954339857564073659, 0.0003908679715128147319, 0.0005863019572692221250, 0.0007817359430256294638 ),
 .UNSPECIFIED. ) ;
#43905=CARTESIAN_POINT ( 'NONE',  ( 4.153846153846154188, -12.10708131394839349, 31.69288490824020244 ) ) ;
#43906=CARTESIAN_POINT ( 'NONE',  ( 11.28846153846153832, -7.500000000000001776, 35.00000000000000000 ) ) ;
#43908=CARTESIAN_POINT ( 'NONE',  ( 4.153846153846030731, -5.941354392335915335, 34.76329471203413846 ) ) ;
#43909=CARTESIAN_POINT ( 'NONE',  ( -8.639185713310999049, -2.254550872974305342, 29.97347326024527092 ) ) ;
#43910=CARTESIAN_POINT ( 'NONE',  ( -6.000000000000119904, -12.46129190930018460, 30.37095296980731973 ) ) ;
#43912=ADVANCED_FACE ( 'NONE', ( #20019 ), #19578, .F. ) ;
#43913=ORIENTED_EDGE ( 'NONE', *, *, #72828, .F. ) ;
#43915=EDGE_LOOP ( 'NONE', ( #36437, #35808, #34300, #14893 ) ) ;
#43916=CARTESIAN_POINT ( 'NONE',  ( -9.822999158975251888, -5.582088688514999397, 34.36776431015576350 ) ) ;
#43917=ORIENTED_EDGE ( 'NONE', *, *, #85740, .F. ) ;
#43918=CARTESIAN_POINT ( 'NONE',  ( 16.08857570788537927, -11.48612834413959582, 32.76840700105983473 ) ) ;
#43919=ORIENTED_EDGE ( 'NONE', *, *, #62582, .T. ) ;
#43923=CARTESIAN_POINT ( 'NONE',  ( 6.673053685783957967, -11.37209801155882971, 32.91403422569032955 ) ) ;
#43924=CARTESIAN_POINT ( 'NONE',  ( -3.099978789802281920, -12.35292014791297710, 31.75344720912887198 ) ) ;
#43925=CARTESIAN_POINT ( 'NONE',  ( 7.173022441425063178, -9.272278438253401589, 34.42582936511637826 ) ) ;
#43926=CARTESIAN_POINT ( 'NONE',  ( 15.10062126103753855, -8.630895178749533159, 34.87696386517710323 ) ) ;
#43928=CARTESIAN_POINT ( 'NONE',  ( 6.000000000000001776, -6.189225973068211317, 35.74407628777942847 ) ) ;
#43931=CARTESIAN_POINT ( 'NONE',  ( 1.319344938654611443, -2.892918686051582977, 31.69288490824016691 ) ) ;
#43932=CARTESIAN_POINT ( 'NONE',  ( 11.53846153846141576, -12.70778746994576025, 30.41441678777401236 ) ) ;
#43933=CARTESIAN_POINT ( 'NONE',  ( 14.30769230769218758, -3.300289026999228881, 32.46337939537708905 ) ) ;
#43935=EDGE_CURVE ( 'NONE', #25274, #38093, #58620, .T. ) ;
#43938=CARTESIAN_POINT ( 'NONE',  ( -11.53846153846153655, -12.78798330534102767, 29.49999999999997868 ) ) ;
#43939=CARTESIAN_POINT ( 'NONE',  ( -8.769230769230768274, -11.16473453929635440, 33.15142922261926373 ) ) ;
#43940=CARTESIAN_POINT ( 'NONE',  ( 15.90384615384615330, -7.566082377512564960, 35.00000000000000711 ) ) ;
#43941=VECTOR ( 'NONE', #70129, 1000.000000000000000 ) ;
#43942=CARTESIAN_POINT ( 'NONE',  ( 17.29993592101647337, -12.38742843783360748, 31.66772728687926985 ) ) ;
#43943=DIRECTION ( 'NONE',  ( -0.000000000000000000, -0.1736481776669307198, -0.9848077530122080203 ) ) ;
#43944=ADVANCED_FACE ( 'NONE', ( #87615 ), #5622, .F. ) ;
#43945=ORIENTED_EDGE ( 'NONE', *, *, #57618, .T. ) ;
#43946=CARTESIAN_POINT ( 'NONE',  ( -1.384615384615505151, -10.21337939537710326, 33.94971097300076224 ) ) ;
#43947=ORIENTED_EDGE ( 'NONE', *, *, #16268, .F. ) ;
#43948=EDGE_CURVE ( 'NONE', #65065, #8429, #24329, .T. ) ;
#43949=EDGE_LOOP ( 'NONE', ( #21742, #60030, #49970, #41540 ) ) ;
#43950=DIRECTION ( 'NONE',  ( -0.000000000000000000, -0.9396926207859092051, -0.3420201433256662704 ) ) ;
#43951=DIRECTION ( 'NONE',  ( 0.000000000000000000, 1.000000000000000000, -0.000000000000000000 ) ) ;
#43952=CARTESIAN_POINT ( 'NONE',  ( 16.40390046548446534, -2.779044189368097051, 31.39831045268885745 ) ) ;
#43953=CARTESIAN_POINT ( 'NONE',  ( 4.376857505459002873, -3.587049720035815792, 32.86302985866382897 ) ) ;
#43954=CARTESIAN_POINT ( 'NONE',  ( 17.77651507543566822, -9.417330523894424488, 34.63758898049880486 ) ) ;
#43957=DIRECTION ( 'NONE',  ( -0.000000000000000000, -0.3420201433256694901, -0.9396926207859082059 ) ) ;
#43958=VERTEX_POINT ( 'NONE', #74090 ) ;
#43959=ORIENTED_EDGE ( 'NONE', *, *, #85508, .F. ) ;
#43960=CARTESIAN_POINT ( 'NONE',  ( 12.52673244332181568, -2.506253911140448043, 29.99999999999988631 ) ) ;
#43962=B_SPLINE_CURVE_WITH_KNOTS ( 'NONE', 3,
 ( #58794, #11064, #52033, #25015, #32227, #37189, #3850, #64654, #38085, #66451 ),
 .UNSPECIFIED., .F., .F.,
 ( 4, 2, 2, 2, 4 ),
 ( 0.0007817359430256282712, 0.0009771253907249941549, 0.001172514838424359822, 0.001367904286123725489, 0.001563293733823091372 ),
 .UNSPECIFIED. ) ;
#43963=EDGE_CURVE ( 'NONE', #42436, #19174, #30709, .T. ) ;
#43964=CARTESIAN_POINT ( 'NONE',  ( -10.48533700912893174, -7.723484964179501588, 34.74522123443823318 ) ) ;
#43965=LINE ( 'NONE', #30890, #40746 ) ;
#43966=EDGE_CURVE ( 'NONE', #49557, #72270, #84495, .T. ) ;
#43967=CARTESIAN_POINT ( 'NONE',  ( -7.846153846153965716, -12.27809138561165270, 31.22303859784587132 ) ) ;
#43968=ORIENTED_EDGE ( 'NONE', *, *, #35737, .T. ) ;
#43969=ORIENTED_EDGE ( 'NONE', *, *, #68408, .T. ) ;
#43971=EDGE_LOOP ( 'NONE', ( #74231, #88312 ) ) ;
#43972=CARTESIAN_POINT ( 'NONE',  ( -14.08467946359890988, -2.308499170217967134, 30.53291367094873721 ) ) ;
#43973=ORIENTED_EDGE ( 'NONE', *, *, #4658, .F. ) ;
#43974=CYLINDRICAL_SURFACE ( 'NONE', #33508, 0.2499999999999995559 ) ;
#43975=CARTESIAN_POINT ( 'NONE',  ( 6.222779541268409709, -12.44528174975671853, 30.48912976160716681 ) ) ;
#43976=CARTESIAN_POINT ( 'NONE',  ( 2.372947447205147942, -9.528491918058460186, 34.59228464037085615 ) ) ;
#43977=ORIENTED_EDGE ( 'NONE', *, *, #72789, .T. ) ;
#43978=EDGE_CURVE ( 'NONE', #25915, #23361, #26418, .T. ) ;
#43979=CARTESIAN_POINT ( 'NONE',  ( 14.98079248672064345, -2.544273027872575366, 31.48422191005632342 ) ) ;
#43980=ORIENTED_EDGE ( 'NONE', *, *, #46074, .F. ) ;
#43981=CARTESIAN_POINT ( 'NONE',  ( 15.29683656411930848, -11.35647404775217595, 33.31231777344666511 ) ) ;
#43982=FACE_OUTER_BOUND ( 'NONE', #63029, .T. ) ;
#43983=CARTESIAN_POINT ( 'NONE',  ( -18.00000000000000000, -2.486705287966279876, 31.30864560766543647 ) ) ;
#43984=CARTESIAN_POINT ( 'NONE',  ( -0.2385256174450662847, -11.43677907613345113, 33.22367315496201456 ) ) ;
#43985=CARTESIAN_POINT ( 'NONE',  ( -10.86540783960607293, -5.765609946408404518, 34.70566812827425451 ) ) ;
#43986=CARTESIAN_POINT ( 'NONE',  ( 16.08857570788537572, -2.625532179533444754, 30.86335684631481513 ) ) ;
#43987=CARTESIAN_POINT ( 'NONE',  ( -0.3962833220256231082, -12.70778746994558439, 30.41441678777537305 ) ) ;
#43988=ORIENTED_EDGE ( 'NONE', *, *, #63726, .F. ) ;
#43989=CARTESIAN_POINT ( 'NONE',  ( -11.47320596718551400, -12.27809138561124591, 31.22303859784720359 ) ) ;
#43990=CARTESIAN_POINT ( 'NONE',  ( -6.249976744048589161, -11.47974371597207899, 33.17467449705390692 ) ) ;
#43991=ADVANCED_FACE ( 'NONE', ( #28108 ), #56468, .F. ) ;
#43992=ORIENTED_EDGE ( 'NONE', *, *, #31997, .F. ) ;
#43993=CARTESIAN_POINT ( 'NONE',  ( -1.384615384615383471, -10.51840700105979565, 33.73612834413961536 ) ) ;
#43994=CARTESIAN_POINT ( 'NONE',  ( -4.854143535654667829, -5.913360116392398780, 34.49180327182771322 ) ) ;
#43995=CARTESIAN_POINT ( 'NONE',  ( 3.296938371731887862, -7.250054483168843156, 34.74374881642865631 ) ) ;
#43996=CARTESIAN_POINT ( 'NONE',  ( 2.057669083470851756, -5.765609946408404518, 34.70566812827425451 ) ) ;
#43997=CARTESIAN_POINT ( 'NONE',  ( 17.93472955403921887, -6.026961402152685388, 34.52809138561120506 ) ) ;
#43998=EDGE_CURVE ( 'NONE', #19270, #82252, #14597, .T. ) ;
#43999=CARTESIAN_POINT ( 'NONE',  ( 13.38461538461538680, -13.95598074871891292, 31.83374038241031911 ) ) ;
#44000=ADVANCED_FACE ( 'NONE', ( #41188 ), #69099, .F. ) ;
#44001=FACE_BOUND ( 'NONE', #24123, .T. ) ;
#44002=DIRECTION ( 'NONE',  ( -0.000000000000000000, 0.9396926207859092051, -0.3420201433256662704 ) ) ;
#44003=FACE_OUTER_BOUND ( 'NONE', #19811, .T. ) ;
#44004=DIRECTION ( 'NONE',  ( -0.000000000000000000, 0.7660444431189791237, -0.6427876096865379196 ) ) ;
#44005=CARTESIAN_POINT ( 'NONE',  ( -6.792286482109972212, -10.70102852606553157, 33.91149625220312913 ) ) ;
#44006=CARTESIAN_POINT ( 'NONE',  ( 9.823099500132483897, -4.118422570099828484, 33.43335022499816489 ) ) ;
#44007=DIRECTION ( 'NONE',  ( -0.000000000000000000, 0.3420201433256694346, -0.9396926207859080948 ) ) ;
#44009=ORIENTED_EDGE ( 'NONE', *, *, #78246, .F. ) ;
#44010=CARTESIAN_POINT ( 'NONE',  ( 18.00000000000000000, -3.669653830205710676, 35.88435417666054406 ) ) ;
#44011=AXIS2_PLACEMENT_3D ( 'NONE', #85029, #84157, #2157 ) ;
#44012=CARTESIAN_POINT ( 'NONE',  ( -12.33074802057151409, -6.369690395747422684, 34.87708834333098196 ) ) ;
#44013=CARTESIAN_POINT ( 'NONE',  ( -0.7115616857599182943, -3.520140089381497361, 33.17453946501458262 ) ) ;
#44014=CARTESIAN_POINT ( 'NONE',  ( -10.86536135943320502, -11.47974371597208076, 33.17467449705390692 ) ) ;
#44015=CARTESIAN_POINT ( 'NONE',  ( 6.700149964170075023, -12.64616026154729411, 30.79003144601913533 ) ) ;
#44016=CARTESIAN_POINT ( 'NONE',  ( -9.626239341305254271, -4.098570777380720287, 33.41473453929635440 ) ) ;
#44018=CARTESIAN_POINT ( 'NONE',  ( -16.40386937806761125, -5.765609946408405406, 34.70566812827424741 ) ) ;
#44019=CARTESIAN_POINT ( 'NONE',  ( 18.24994551834813805, -3.202959910592336090, 32.30730279482227019 ) ) ;
#44020=VECTOR ( 'NONE', #48032, 1000.000000000000227 ) ;
#44021=DIRECTION ( 'NONE',  ( 0.000000000000000000, 0.1736481776669267785, -0.9848077530122087975 ) ) ;
#44022=CARTESIAN_POINT ( 'NONE',  ( 10.48469401227430708, -6.369640206132551441, 34.87707690430378449 ) ) ;
#44023=CARTESIAN_POINT ( 'NONE',  ( 2.307692307692623679, -2.255955759149395501, 30.00000000000324363 ) ) ;
#44024=CARTESIAN_POINT ( 'NONE',  ( 6.000000000000001776, -13.87047571288749737, 32.06866353760679544 ) ) ;
#44025=FACE_OUTER_BOUND ( 'NONE', #24222, .T. ) ;
#44026=CARTESIAN_POINT ( 'NONE',  ( 17.29993592101647693, -2.523321265292116866, 31.42251411153756990 ) ) ;
#44027=EDGE_LOOP ( 'NONE', ( #41984, #84002, #71096, #19932 ) ) ;
#44028=CARTESIAN_POINT ( 'NONE',  ( -15.90384615384471800, -7.500000000000155431, 34.75000000000007105 ) ) ;
#44031=CARTESIAN_POINT ( 'NONE',  ( 7.145856592054987466, -10.97394488606064122, 33.68653795673694873 ) ) ;
#44032=CARTESIAN_POINT ( 'NONE',  ( -8.769230769230892619, -8.656820664282941280, 34.87096338111179961 ) ) ;
#44034=CARTESIAN_POINT ( 'NONE',  ( -16.21992853320628925, -3.937682226553330445, 33.60647404775217240 ) ) ;
#44035=CARTESIAN_POINT ( 'NONE',  ( 12.23861224402230619, -5.667676309546437530, 34.40238873228292249 ) ) ;
#44036=ORIENTED_EDGE ( 'NONE', *, *, #52575, .F. ) ;
#44037=CARTESIAN_POINT ( 'NONE',  ( 6.699591979352975457, -3.236172620538810385, 32.36188796281390267 ) ) ;
#44038=CARTESIAN_POINT ( 'NONE',  ( -13.16160403300253279, -9.886259254753566594, 34.14407573483972413 ) ) ;
#44039=LINE ( 'NONE', #23765, #44836 ) ;
#44040=DIRECTION ( 'NONE',  ( -0.000000000000000000, 0.9396926207859093161, -0.3420201433256663259 ) ) ;
#44041=ORIENTED_EDGE ( 'NONE', *, *, #874, .T. ) ;
#44042=CARTESIAN_POINT ( 'NONE',  ( -11.60454494941741999, -4.098570777380719399, 33.41473453929634729 ) ) ;
#44044=CARTESIAN_POINT ( 'NONE',  ( -1.384615384615505151, -6.026961402154118908, 34.52809138561165270 ) ) ;
#44045=ORIENTED_EDGE ( 'NONE', *, *, #23416, .F. ) ;
#44046=VERTEX_POINT ( 'NONE', #33976 ) ;
#44047=VERTEX_POINT ( 'NONE', #49706 ) ;
#44048=CARTESIAN_POINT ( 'NONE',  ( -8.769230769230890843, -10.21337939537710326, 33.94971097300076224 ) ) ;
#44049=CARTESIAN_POINT ( 'NONE',  ( -8.638438961405983108, -3.062576670634119758, 32.05464942895959979 ) ) ;
#44050=CARTESIAN_POINT ( 'NONE',  ( -3.930833309752757021, -12.64618726649961289, 30.78989965857442712 ) ) ;
#44051=CARTESIAN_POINT ( 'NONE',  ( -10.39237326377176451, -3.105924265160262543, 32.13625925475356127 ) ) ;
#44052=VERTEX_POINT ( 'NONE', #197 ) ;
#44054=CARTESIAN_POINT ( 'NONE',  ( -2.057692307690886846, -7.500000000000154543, 35.00000000000007105 ) ) ;
#44055=ORIENTED_EDGE ( 'NONE', *, *, #24394, .F. ) ;
#44056=CARTESIAN_POINT ( 'NONE',  ( 9.692307692307695177, -12.37446782046654192, 30.86335684631486131 ) ) ;
#44057=EDGE_CURVE ( 'NONE', #1586, #8757, #83378, .T. ) ;
#44059=CARTESIAN_POINT ( 'NONE',  ( 2.307692307692309264, -3.513871655860378418, 32.76840700105978499 ) ) ;
#44060=DIRECTION ( 'NONE',  ( -0.000000000000000000, -0.6427876096865404731, -0.7660444431189770143 ) ) ;
#44061=EDGE_LOOP ( 'NONE', ( #21709, #13201, #20030, #32767 ) ) ;
#44062=AXIS2_PLACEMENT_3D ( 'NONE', #33770, #25682, #48936 ) ;
#44064=CARTESIAN_POINT ( 'NONE',  ( -16.15384615384615330, -11.11383981884818262, 36.00935417666054406 ) ) ;
#44065=ORIENTED_EDGE ( 'NONE', *, *, #10210, .T. ) ;
#44066=B_SPLINE_CURVE_WITH_KNOTS ( 'NONE', 3,
 ( #87880, #61242, #59482, #81101, #73453, #88318, #13513, #67137, #6328, #81990 ),
 .UNSPECIFIED., .F., .F.,
 ( 4, 2, 2, 2, 4 ),
 ( 0.0007817246256747459798, 0.0009771112852218896347, 0.001172497944769033398, 0.001367884604316177161, 0.001563271263863320708 ),
 .UNSPECIFIED. ) ;
#44068=CARTESIAN_POINT ( 'NONE',  ( -16.02332045208259004, -3.816742781228458448, 33.13167719472716044 ) ) ;
#44069=ORIENTED_EDGE ( 'NONE', *, *, #69534, .F. ) ;
#44070=EDGE_CURVE ( 'NONE', #17127, #80196, #77181, .T. ) ;
#44071=AXIS2_PLACEMENT_3D ( 'NONE', #55651, #6592, #7027 ) ;
#44072=CARTESIAN_POINT ( 'NONE',  ( 12.52760579488853665, -6.343179335718452272, 34.87096338111212646 ) ) ;
#44073=LINE ( 'NONE', #13630, #45085 ) ;
#44074=LINE ( 'NONE', #42339, #87103 ) ;
#44075=FACE_BOUND ( 'NONE', #25411, .T. ) ;
#44076=CARTESIAN_POINT ( 'NONE',  ( 5.999999999999878320, -2.379036618888197729, 30.90682066428292885 ) ) ;
#44077=CARTESIAN_POINT ( 'NONE',  ( 2.307692307692309264, -8.120952969808772792, 34.71129190930000163 ) ) ;
#44078=CARTESIAN_POINT ( 'NONE',  ( 8.769230769230768274, -2.708943851104267164, 35.45975837776705220 ) ) ;
#44079=CARTESIAN_POINT ( 'NONE',  ( 3.361294669002876656, -3.625058011473228259, 33.29252011169590020 ) ) ;
#44080=CARTESIAN_POINT ( 'NONE',  ( 4.219101293358989757, -2.379036618887895305, 30.90682066428159303 ) ) ;
#44081=CARTESIAN_POINT ( 'NONE',  ( -7.976845312821408740, -3.062553014421049546, 32.05460306192773601 ) ) ;
#44083=EDGE_LOOP ( 'NONE', ( #45832, #63739, #83321, #73064 ) ) ;
#44084=CARTESIAN_POINT ( 'NONE',  ( -5.076923076923075762, -3.886160181151819604, 36.00935417666054406 ) ) ;
#44085=B_SPLINE_CURVE_WITH_KNOTS ( 'NONE', 3,
 ( #40205, #87072, #11841, #33871, #52806, #18595, #59568, #67667, #67227, #60457 ),
 .UNSPECIFIED., .F., .F.,
 ( 4, 2, 2, 2, 4 ),
 ( 0.0007817359430256304396, 0.0009771253907249963233, 0.001172514838424362424, 0.001367904286123728308, 0.001563293733823094191 ),
 .UNSPECIFIED. ) ;
#44086=ORIENTED_EDGE ( 'NONE', *, *, #59201, .F. ) ;
#44087=ORIENTED_EDGE ( 'NONE', *, *, #85675, .F. ) ;
#44088=CARTESIAN_POINT ( 'NONE',  ( -5.300408001487405762, -12.11044203135681840, 32.26167407432752299 ) ) ;
#44089=CARTESIAN_POINT ( 'NONE',  ( 10.74591005361826035, -12.70449254468099198, 30.44128974285582956 ) ) ;
#44090=CARTESIAN_POINT ( 'NONE',  ( -5.749945688361685292, -6.567000820036038355, 34.66262288849541306 ) ) ;
#44091=CARTESIAN_POINT ( 'NONE',  ( 14.37375964104238335, -3.937682226553329556, 33.60647404775216529 ) ) ;
#44092=CARTESIAN_POINT ( 'NONE',  ( -16.15384615384615330, -2.499999999999998668, 29.50000000000001066 ) ) ;
#44095=EDGE_CURVE ( 'NONE', #33240, #10922, #16836, .T. ) ;
#44096=EDGE_CURVE ( 'NONE', #84840, #79197, #27541, .T. ) ;
#44097=CARTESIAN_POINT ( 'NONE',  ( 18.00000000000000000, -3.937682226553329556, 33.60647404775216529 ) ) ;
#44098=CARTESIAN_POINT ( 'NONE',  ( 6.792385456409363087, -3.530157926970578508, 32.79014554554150607 ) ) ;
#44099=CARTESIAN_POINT ( 'NONE',  ( 17.32697738856138869, -6.567000820036036579, 34.66262288849541306 ) ) ;
#44104=ORIENTED_EDGE ( 'NONE', *, *, #75165, .F. ) ;
#44105=EDGE_CURVE ( 'NONE', #5354, #81137, #23220, .T. ) ;
#44106=CARTESIAN_POINT ( 'NONE',  ( -7.846153846153844924, -11.35647404775217417, 33.31231777344666511 ) ) ;
#44107=ORIENTED_EDGE ( 'NONE', *, *, #67088, .T. ) ;
#44108=AXIS2_PLACEMENT_3D ( 'NONE', #40859, #60677, #6624 ) ;
#44109=CARTESIAN_POINT ( 'NONE',  ( -18.06532401280430733, -7.749976730030849303, 34.74374725381503737 ) ) ;
#44110=CARTESIAN_POINT ( 'NONE',  ( 9.692307692307695177, -9.780366693483667717, 34.19971097300155094 ) ) ;
#44111=CARTESIAN_POINT ( 'NONE',  ( -16.21911659980692733, -2.892918686051582089, 31.69288490824015980 ) ) ;
#44112=CARTESIAN_POINT ( 'NONE',  ( 5.777133736936903574, -2.251424796025575770, 29.88072029997477586 ) ) ;
#44115=ORIENTED_EDGE ( 'NONE', *, *, #77511, .T. ) ;
#44116=CARTESIAN_POINT ( 'NONE',  ( -12.52762187249433978, -10.51840700105979387, 33.73612834413961536 ) ) ;
#44117=CARTESIAN_POINT ( 'NONE',  ( -16.40386939113912135, -11.86270091957321071, 32.19358267280088626 ) ) ;
#44119=LINE ( 'NONE', #2692, #13809 ) ;
#44120=DIRECTION ( 'NONE',  ( 0.000000000000000000, 0.9848077530122072432, 0.1736481776669354937 ) ) ;
#44121=CARTESIAN_POINT ( 'NONE',  ( 6.130790440966952026, -9.084667340241226796, 34.75534355489798344 ) ) ;
#44122=CARTESIAN_POINT ( 'NONE',  ( -2.307692307692305711, -2.292212530054420494, 30.41441678777542634 ) ) ;
#44123=CARTESIAN_POINT ( 'NONE',  ( -6.000000000000119904, -10.21337939537710326, 33.94971097300076224 ) ) ;
#44124=CARTESIAN_POINT ( 'NONE',  ( 11.28848480751918437, -6.567427716900048118, 34.66269422305636283 ) ) ;
#44125=CARTESIAN_POINT ( 'NONE',  ( -7.053768389744481837, -4.809359713505814149, 33.96456829005828837 ) ) ;
#44127=ORIENTED_EDGE ( 'NONE', *, *, #4741, .T. ) ;
#44129=CARTESIAN_POINT ( 'NONE',  ( -12.39639268220649271, -7.750023238201979581, 34.74374492549440419 ) ) ;
#44130=DIRECTION ( 'NONE',  ( -0.000000000000000000, 0.3420201433256694901, -0.9396926207859082059 ) ) ;
#44132=CARTESIAN_POINT ( 'NONE',  ( 0.4615384615384611200, -3.513871655860378418, 32.76840700105978499 ) ) ;
#44133=VECTOR ( 'NONE', #86171, 1000.000000000000227 ) ;
#44134=CARTESIAN_POINT ( 'NONE',  ( -17.32689980786543060, -2.564618984488975517, 30.55390908950641915 ) ) ;
#44135=ORIENTED_EDGE ( 'NONE', *, *, #17173, .T. ) ;
#44137=LINE ( 'NONE', #18027, #48389 ) ;
#44138=EDGE_LOOP ( 'NONE', ( #28346, #50040 ) ) ;
#44139=CARTESIAN_POINT ( 'NONE',  ( -18.25002322422145085, -4.931416488878823223, 34.32920672191015399 ) ) ;
#44140=ORIENTED_EDGE ( 'NONE', *, *, #8742, .T. ) ;
#44141=CARTESIAN_POINT ( 'NONE',  ( 17.75002326905764605, -6.567427716900048118, 34.66269422305636283 ) ) ;
#44142=CARTESIAN_POINT ( 'NONE',  ( 3.230769230769108269, -4.320704448113951379, 33.92786785259630022 ) ) ;
#44143=AXIS2_PLACEMENT_3D ( 'NONE', #10261, #37273, #58881 ) ;
#44144=CARTESIAN_POINT ( 'NONE',  ( -0.7115616857599186273, -10.18141759479407327, 34.26406193332782379 ) ) ;
#44145=CARTESIAN_POINT ( 'NONE',  ( -12.46153846153846168, -13.53365097954675988, 30.81389545987213552 ) ) ;
#44146=EDGE_LOOP ( 'NONE', ( #79100, #29778, #69516, #9229 ) ) ;
#44147=CARTESIAN_POINT ( 'NONE',  ( -13.38461538461538325, -2.833524468853757305, 32.15551576947925838 ) ) ;
#44148=ORIENTED_EDGE ( 'NONE', *, *, #33561, .F. ) ;
#44149=CARTESIAN_POINT ( 'NONE',  ( -17.74994558008654622, -12.01375889529407992, 32.43194544308182969 ) ) ;
#44150=CARTESIAN_POINT ( 'NONE',  ( 12.46153846153846168, -12.10708131394839349, 31.69288490824020244 ) ) ;
#44151=ORIENTED_EDGE ( 'NONE', *, *, #78893, .T. ) ;
#44152=CARTESIAN_POINT ( 'NONE',  ( -5.776988648387149539, -11.24521262558773671, 33.06293181088029343 ) ) ;
#44153=CARTESIAN_POINT ( 'NONE',  ( 10.83839596699746544, -3.105924265160262543, 32.13625925475356127 ) ) ;
#44154=CARTESIAN_POINT ( 'NONE',  ( -4.023800991011373895, -2.504778602574660340, 29.97347330155780298 ) ) ;
#44155=EDGE_CURVE ( 'NONE', #84107, #43411, #6950, .T. ) ;
#44156=CARTESIAN_POINT ( 'NONE',  ( -14.17716686945866300, -10.31582465632705237, 34.18122507451815295 ) ) ;
#44157=CARTESIAN_POINT ( 'NONE',  ( -16.21911615440247090, -3.083524468853725775, 32.58852847137143272 ) ) ;
#44158=VECTOR ( 'NONE', #8163, 1000.000000000000114 ) ;
#44159=EDGE_LOOP ( 'NONE', ( #19149, #36341, #73445, #46063 ) ) ;
#44160=ORIENTED_EDGE ( 'NONE', *, *, #81193, .T. ) ;
#44161=FACE_BOUND ( 'NONE', #72205, .T. ) ;
#44162=EDGE_LOOP ( 'NONE', ( #11640, #81351 ) ) ;
#44164=EDGE_CURVE ( 'NONE', #87031, #79680, #69487, .T. ) ;
#44165=AXIS2_PLACEMENT_3D ( 'NONE', #61645, #49023, #54899 ) ;
#44166=CARTESIAN_POINT ( 'NONE',  ( 13.44987095589141290, -10.90142922261932057, 33.41473453929631887 ) ) ;
#44168=EDGE_CURVE ( 'NONE', #21769, #5830, #79054, .T. ) ;
#44169=ORIENTED_EDGE ( 'NONE', *, *, #24687, .F. ) ;
#44171=ORIENTED_EDGE ( 'NONE', *, *, #19585, .T. ) ;
#44172=CARTESIAN_POINT ( 'NONE',  ( -1.515306851282940626, -11.71456829005830080, 32.44064028649416542 ) ) ;
#44174=CARTESIAN_POINT ( 'NONE',  ( 2.438218009455873858, -4.459921816937789885, 33.71989282347011851 ) ) ;
#44175=EDGE_CURVE ( 'NONE', #74304, #34444, #32969, .T. ) ;
#44176=CARTESIAN_POINT ( 'NONE',  ( -7.912237257109728361, -2.538708090699994813, 30.37095296980875148 ) ) ;
#44177=CARTESIAN_POINT ( 'NONE',  ( -5.076923076923075762, -13.20930481340135110, 34.54067556320372745 ) ) ;
#44178=FACE_BOUND ( 'NONE', #49120, .T. ) ;
#44180=CARTESIAN_POINT ( 'NONE',  ( 5.076923076923075762, -3.513871655860378418, 32.76840700105978499 ) ) ;
#44181=EDGE_CURVE ( 'NONE', #2618, #10136, #23044, .T. ) ;
#44182=CYLINDRICAL_SURFACE ( 'NONE', #38809, 0.2499999999999995559 ) ;
#44184=CARTESIAN_POINT ( 'NONE',  ( -11.60454494941741999, -3.050289026998445951, 32.03036669348365706 ) ) ;
#44185=EDGE_LOOP ( 'NONE', ( #17274, #53122, #16214, #69097 ) ) ;
#44186=CARTESIAN_POINT ( 'NONE',  ( -2.557692307692305267, -7.500000000000001776, 35.00000000000000000 ) ) ;
#44188=ORIENTED_EDGE ( 'NONE', *, *, #86637, .F. ) ;
#44190=DIRECTION ( 'NONE',  ( -0.000000000000000000, -0.5000000000000011102, -0.8660254037844380415 ) ) ;
#44191=CARTESIAN_POINT ( 'NONE',  ( -8.546217925137375104, -12.38742843783360748, 31.66772728687926985 ) ) ;
#44192=CARTESIAN_POINT ( 'NONE',  ( -4.087777802843714170, -4.098570777380720287, 33.41473453929635440 ) ) ;
#44193=CARTESIAN_POINT ( 'NONE',  ( 17.20776149493583773, -7.277220443632451463, 34.74524770363009196 ) ) ;
#44194=CARTESIAN_POINT ( 'NONE',  ( -2.373775718648187372, -9.780366693483667717, 34.19971097300155805 ) ) ;
#44195=ORIENTED_EDGE ( 'NONE', *, *, #45992, .T. ) ;
#44196=EDGE_CURVE ( 'NONE', #85987, #22316, #20972, .T. ) ;
#44197=CARTESIAN_POINT ( 'NONE',  ( -5.207613680033384540, -6.369640206132550553, 34.87707690430378449 ) ) ;
#44199=CARTESIAN_POINT ( 'NONE',  ( -11.60454494941741999, -9.780366693483667717, 34.19971097300155805 ) ) ;
#44200=LINE ( 'NONE', #78007, #8515 ) ;
#44201=EDGE_CURVE ( 'NONE', #48673, #34683, #68211, .T. ) ;
#44202=CARTESIAN_POINT ( 'NONE',  ( -13.63459212866397685, -12.65889640711025521, 30.72598325615533454 ) ) ;
#44203=EDGE_LOOP ( 'NONE', ( #65042, #88215, #45107, #14185 ) ) ;
#44204=ORIENTED_EDGE ( 'NONE', *, *, #69170, .F. ) ;
#44205=FACE_BOUND ( 'NONE', #36644, .T. ) ;
#44206=EDGE_CURVE ( 'NONE', #88485, #64018, #32786, .T. ) ;
#44207=CARTESIAN_POINT ( 'NONE',  ( 7.596130608860879541, -2.823816976329319495, 31.52131813110795733 ) ) ;
#44208=CARTESIAN_POINT ( 'NONE',  ( -6.792238505064159604, -7.277220443632450575, 34.74524770363009196 ) ) ;
#44210=EDGE_LOOP ( 'NONE', ( #6279, #54238 ) ) ;
#44211=CARTESIAN_POINT ( 'NONE',  ( 3.903869409797563250, -11.47974371597208076, 33.17467449705390692 ) ) ;
#44212=CARTESIAN_POINT ( 'NONE',  ( 6.222779668978065004, -11.60474049983371003, 33.02348890104160262 ) ) ;
#44213=CARTESIAN_POINT ( 'NONE',  ( 0.7115927731767749398, -12.17597550085003455, 31.52189283813461884 ) ) ;
#44215=VERTEX_POINT ( 'NONE', #25339 ) ;
#44216=CYLINDRICAL_SURFACE ( 'NONE', #47391, 0.2499999999999998890 ) ;
#44219=EDGE_LOOP ( 'NONE', ( #55082, #55702 ) ) ;
#44220=CYLINDRICAL_SURFACE ( 'NONE', #52668, 0.2500000000000009437 ) ;
#44221=CARTESIAN_POINT ( 'NONE',  ( 15.23076923076911093, -2.892918686052165622, 31.69288490824153470 ) ) ;
#44222=DIRECTION ( 'NONE',  ( 0.000000000000000000, 0.000000000000000000, -1.000000000000000000 ) ) ;
#44223=DIRECTION ( 'NONE',  ( 0.000000000000000000, 0.000000000000000000, 1.000000000000000000 ) ) ;
#44224=CARTESIAN_POINT ( 'NONE',  ( -14.43784027742400689, -8.630895178749533159, 34.87696386517710323 ) ) ;
#44225=CARTESIAN_POINT ( 'NONE',  ( 12.39545608217832395, -5.471508081941602875, 34.59228464037088457 ) ) ;
#44227=ORIENTED_EDGE ( 'NONE', *, *, #6984, .T. ) ;
#44228=VECTOR ( 'NONE', #68467, 1000.000000000000114 ) ;
#44229=CARTESIAN_POINT ( 'NONE',  ( 13.60762822870878352, -12.64618726649961289, 30.78989965857442712 ) ) ;
#44232=VECTOR ( 'NONE', #67548, 1000.000000000000114 ) ;
#44233=ORIENTED_EDGE ( 'NONE', *, *, #30406, .T. ) ;
#44234=CARTESIAN_POINT ( 'NONE',  ( -10.83886955910856109, -11.41268669641500466, 32.86336882939237825 ) ) ;
#44235=CARTESIAN_POINT ( 'NONE',  ( -7.596208436775802930, -5.766571408460171355, 34.70601412856602508 ) ) ;
#44236=CYLINDRICAL_SURFACE ( 'NONE', #69147, 0.2499999999999973355 ) ;
#44238=CARTESIAN_POINT ( 'NONE',  ( 13.38461538461538680, -2.833524468853757305, 32.15551576947925838 ) ) ;
#44239=DIRECTION ( 'NONE',  ( 0.000000000000000000, 0.3420201433256610524, 0.9396926207859113145 ) ) ;
#44240=LINE ( 'NONE', #8280, #14896 ) ;
#44241=ORIENTED_EDGE ( 'NONE', *, *, #62026, .F. ) ;
#44242=EDGE_CURVE ( 'NONE', #24932, #87868, #87969, .T. ) ;
#44243=CARTESIAN_POINT ( 'NONE',  ( 6.250054311638314708, -10.66356715214248396, 33.62249196103329751 ) ) ;
#44244=CARTESIAN_POINT ( 'NONE',  ( -1.608100328339332252, -6.760086850603068243, 34.69517049084099369 ) ) ;
#44245=FACE_OUTER_BOUND ( 'NONE', #42619, .T. ) ;
#44246=CARTESIAN_POINT ( 'NONE',  ( 2.307692307692187583, -3.835265460704628371, 33.15142922262033665 ) ) ;
#44247=EDGE_CURVE ( 'NONE', #42119, #35523, #64992, .T. ) ;
#44248=ORIENTED_EDGE ( 'NONE', *, *, #67285, .F. ) ;
#44249=CARTESIAN_POINT ( 'NONE',  ( 0.4615384615384611200, -2.538708090699994813, 30.37095296980875503 ) ) ;
#44250=ADVANCED_FACE ( 'NONE', ( #53245 ), #46499, .F. ) ;
#44252=AXIS2_PLACEMENT_3D ( 'NONE', #62492, #13436, #55301 ) ;
#44253=CARTESIAN_POINT ( 'NONE',  ( -17.77722033102192967, -8.540255544307065350, 34.89611431652622286 ) ) ;
#44256=DIRECTION ( 'NONE',  ( -0.000000000000000000, 0.1736481776669307198, -0.9848077530122080203 ) ) ;
#44257=ORIENTED_EDGE ( 'NONE', *, *, #34524, .F. ) ;
#44258=CARTESIAN_POINT ( 'NONE',  ( 5.749976762707036393, -10.05641848906368097, 34.04755513067966177 ) ) ;
#44259=B_SPLINE_CURVE_WITH_KNOTS ( 'NONE', 3,
 ( #16495, #51583, #31344, #24129, #65110, #39004, #64665, #72320, #3416, #45287 ),
 .UNSPECIFIED., .F., .F.,
 ( 4, 2, 2, 2, 4 ),
 ( 0.000000000000000000, 0.0001954339857564064715, 0.0003908679715128129430, 0.0005863019572692194144, 0.0007817359430256258859 ),
 .UNSPECIFIED. ) ;
#44260=CARTESIAN_POINT ( 'NONE',  ( 10.39189969082028497, -12.69144148231606017, 30.53333754910549303 ) ) ;
#44261=CARTESIAN_POINT ( 'NONE',  ( -10.86540783960607293, -12.68155406624981119, 30.59749803192733708 ) ) ;
#44262=ADVANCED_FACE ( 'NONE', ( #79846 ), #26669, .F. ) ;
#44263=AXIS2_PLACEMENT_3D ( 'NONE', #31505, #37814, #10348 ) ;
#44265=VERTEX_POINT ( 'NONE', #39756 ) ;
#44266=CARTESIAN_POINT ( 'NONE',  ( 7.596130621932387861, -11.56360843649121861, 33.07473185843129926 ) ) ;
#44268=LINE ( 'NONE', #73559, #60860 ) ;
#44269=CARTESIAN_POINT ( 'NONE',  ( 8.992010438208831502, -9.418065098278013636, 34.63729479722530158 ) ) ;
#44270=CARTESIAN_POINT ( 'NONE',  ( -0.4615384615384611200, -13.20930481340135110, 34.54067556320372745 ) ) ;
#44271=CARTESIAN_POINT ( 'NONE',  ( -14.24162395668986747, -9.780366693483667717, 34.19971097300155805 ) ) ;
#44272=DIRECTION ( 'NONE',  ( -0.000000000000000000, -0.000000000000000000, -1.000000000000000000 ) ) ;
#44274=EDGE_LOOP ( 'NONE', ( #18480, #72699, #850, #54363 ) ) ;
#44275=VERTEX_POINT ( 'NONE', #32989 ) ;
#44277=EDGE_LOOP ( 'NONE', ( #17743, #72210, #56834, #63455 ) ) ;
#44278=ORIENTED_EDGE ( 'NONE', *, *, #37718, .T. ) ;
#44279=CARTESIAN_POINT ( 'NONE',  ( -1.384615384615383471, -3.050289026998446396, 32.03036669348365706 ) ) ;
#44280=CARTESIAN_POINT ( 'NONE',  ( 13.51514108637894829, -10.19071101563364756, 33.96452234770658407 ) ) ;
#44281=CARTESIAN_POINT ( 'NONE',  ( -7.053637514818842824, -2.504760397472873823, 29.97295953869789997 ) ) ;
#44282=CARTESIAN_POINT ( 'NONE',  ( -5.933931648997560870, -4.786620604624113540, 33.94971097300155805 ) ) ;
#44283=FACE_OUTER_BOUND ( 'NONE', #62808, .T. ) ;
#44284=CARTESIAN_POINT ( 'NONE',  ( -6.065270000556318486, -3.083524468853724443, 32.58852847137143272 ) ) ;
#44285=CARTESIAN_POINT ( 'NONE',  ( 12.46153846153846168, -4.102666532097928531, 36.13435417666054406 ) ) ;
#44286=CARTESIAN_POINT ( 'NONE',  ( -17.93393164899756087, -6.386643153685127139, 34.62446782046654192 ) ) ;
#44287=AXIS2_PLACEMENT_3D ( 'NONE', #43619, #78736, #63885 ) ;
#44288=ORIENTED_EDGE ( 'NONE', *, *, #13280, .F. ) ;
#44290=ORIENTED_EDGE ( 'NONE', *, *, #839, .F. ) ;
#44292=ORIENTED_EDGE ( 'NONE', *, *, #53582, .F. ) ;
#44293=CARTESIAN_POINT ( 'NONE',  ( -16.15384615384615330, -4.661471528628507777, 34.16647553114623292 ) ) ;
#44294=CARTESIAN_POINT ( 'NONE',  ( 10.36536137809165403, -9.271318131107980420, 34.42618302367067429 ) ) ;
#44297=ORIENTED_EDGE ( 'NONE', *, *, #17285, .F. ) ;
#44298=ADVANCED_FACE ( 'NONE', ( #60452 ), #12716, .F. ) ;
#44299=ADVANCED_FACE ( 'NONE', ( #40202 ), #45158, .F. ) ;
#44300=ORIENTED_EDGE ( 'NONE', *, *, #68476, .F. ) ;
#44301=FACE_OUTER_BOUND ( 'NONE', #10073, .T. ) ;
#44303=ADVANCED_FACE ( 'NONE', ( #72631 ), #32099, .F. ) ;
#44304=FACE_BOUND ( 'NONE', #4172, .T. ) ;
#44305=LINE ( 'NONE', #15982, #50359 ) ;
#44306=VECTOR ( 'NONE', #24964, 1000.000000000000114 ) ;
#44307=FACE_OUTER_BOUND ( 'NONE', #36787, .T. ) ;
#44308=ORIENTED_EDGE ( 'NONE', *, *, #34662, .T. ) ;
#44309=CYLINDRICAL_SURFACE ( 'NONE', #3141, 0.2500000000000008882 ) ;
#44310=CARTESIAN_POINT ( 'NONE',  ( 16.40390046548447245, -4.235687564193445276, 33.53795663066793509 ) ) ;
#44311=EDGE_CURVE ( 'NONE', #64217, #25231, #82253, .T. ) ;
#44312=DIRECTION ( 'NONE',  ( -0.000000000000000000, 1.000000000000000000, 3.491481338843133355E-15 ) ) ;
#44313=VERTEX_POINT ( 'NONE', #41517 ) ;
#44314=CARTESIAN_POINT ( 'NONE',  ( 18.13004743525045370, -7.723484941389743952, 34.99544897038808955 ) ) ;
#44315=DIRECTION ( 'NONE',  ( 0.000000000000000000, 0.1736481776669267785, -0.9848077530122087975 ) ) ;
#44316=ORIENTED_EDGE ( 'NONE', *, *, #81418, .F. ) ;
#44318=CARTESIAN_POINT ( 'NONE',  ( -6.700065571464073777, -9.086983370893049639, 34.49168942202179267 ) ) ;
#44320=CARTESIAN_POINT ( 'NONE',  ( 7.053602361310566948, -2.647132371071621471, 31.75357179365173010 ) ) ;
#44321=DIRECTION ( 'NONE',  ( -0.000000000000000000, 0.9848077530122085754, -0.1736481776669273613 ) ) ;
#44322=CARTESIAN_POINT ( 'NONE',  ( -16.15384615384627409, -8.613356846316285953, 34.62446782046622218 ) ) ;
#44323=CARTESIAN_POINT ( 'NONE',  ( 7.596153846153846700, -7.500000000000001776, 34.75000000000000000 ) ) ;
#44324=LINE ( 'NONE', #71813, #45915 ) ;
#44326=CARTESIAN_POINT ( 'NONE',  ( -6.923076923076922462, -13.57706302396349152, 30.56769352161908060 ) ) ;
#44327=CARTESIAN_POINT ( 'NONE',  ( 4.376625695114563008, -12.24180327182771855, 31.33663988360758168 ) ) ;
#44328=CARTESIAN_POINT ( 'NONE',  ( 2.557637826040449980, -10.05730279482229683, 34.04704008940765902 ) ) ;
#44329=AXIS2_PLACEMENT_3D ( 'NONE', #83451, #22181, #78002 ) ;
#44330=B_SPLINE_CURVE_WITH_KNOTS ( 'NONE', 3,
 ( #2685, #38709, #66169, #65722, #51750, #52210, #79699, #17553, #58971, #36923 ),
 .UNSPECIFIED., .F., .F.,
 ( 4, 2, 2, 2, 4 ),
 ( 0.0007817246336856289524, 0.0009771112958940099402, 0.001172497958102391036, 0.001367884620310772133, 0.001563271282519153229 ),
 .UNSPECIFIED. ) ;
#44331=B_SPLINE_CURVE_WITH_KNOTS ( 'NONE', 3,
 ( #85423, #30471, #11543, #24602, #65134, #59274, #79561, #11094, #39026, #32262 ),
 .UNSPECIFIED., .F., .F.,
 ( 4, 2, 2, 2, 4 ),
 ( 0.000000000000000000, 0.0001954311564186868202, 0.0003908623128373736404, 0.0005862934692560604335, 0.0007817246256747472808 ),
 .UNSPECIFIED. ) ;
#44332=DIRECTION ( 'NONE',  ( 0.000000000000000000, 0.3420201433256610524, 0.9396926207859113145 ) ) ;
#44333=FACE_OUTER_BOUND ( 'NONE', #66251, .T. ) ;
#44334=CARTESIAN_POINT ( 'NONE',  ( 12.46153846153846168, -4.661471528628507777, 34.16647553114623292 ) ) ;
#44336=CARTESIAN_POINT ( 'NONE',  ( -5.933931648997560870, -12.37446782046654192, 30.86335684631486842 ) ) ;
#44338=ORIENTED_EDGE ( 'NONE', *, *, #72002, .F. ) ;
#44339=CARTESIAN_POINT ( 'NONE',  ( 18.22277954126840172, -11.89424750095246175, 32.13594075562311758 ) ) ;
#44340=ORIENTED_EDGE ( 'NONE', *, *, #16842, .T. ) ;
#44341=CARTESIAN_POINT ( 'NONE',  ( 9.442330961365339448, -6.567427716900048118, 34.66269422305636283 ) ) ;
#44342=EDGE_CURVE ( 'NONE', #20467, #50087, #564, .T. ) ;
#44343=ORIENTED_EDGE ( 'NONE', *, *, #1290, .F. ) ;
#44344=CARTESIAN_POINT ( 'NONE',  ( 16.15384615384615330, -12.62096338111211580, 30.90682066428153263 ) ) ;
#44346=CARTESIAN_POINT ( 'NONE',  ( -2.307692307692305711, -2.292212530054420494, 30.41441678777542634 ) ) ;
#44348=CARTESIAN_POINT ( 'NONE',  ( 6.130525438233648039, -6.808710257144159783, 34.95449254468098843 ) ) ;
#44349=CARTESIAN_POINT ( 'NONE',  ( 9.823099500132483897, -11.18335022499818621, 33.13157742990016885 ) ) ;
#44350=CARTESIAN_POINT ( 'NONE',  ( 4.153846153846154188, -6.386643153685126251, 34.62446782046654192 ) ) ;
#44351=DIRECTION ( 'NONE',  ( -0.000000000000000000, 0.1736481776669307198, -0.9848077530122080203 ) ) ;
#44352=CARTESIAN_POINT ( 'NONE',  ( -17.93026593459031659, -2.250000000000000000, 29.50029277152256668 ) ) ;
#44353=CARTESIAN_POINT ( 'NONE',  ( -17.07692307692307665, -12.29105614889573062, 35.45975837776705220 ) ) ;
#44354=CARTESIAN_POINT ( 'NONE',  ( 0.5276057948885359838, -2.486705287966280320, 31.30864560766543647 ) ) ;
#44357=CARTESIAN_POINT ( 'NONE',  ( -39.05038313613820122, -2.499999999999999556, 29.75000000000000355 ) ) ;
#44358=CARTESIAN_POINT ( 'NONE',  ( -2.307692307692305711, -6.189225973068211317, 35.74407628777942847 ) ) ;
#44359=DIRECTION ( 'NONE',  ( 0.000000000000000000, 0.3420201433256641055, -0.9396926207859100932 ) ) ;
#44362=EDGE_LOOP ( 'NONE', ( #73138, #53237 ) ) ;
#44363=CARTESIAN_POINT ( 'NONE',  ( 17.29970261819148902, -12.24180327182771855, 31.33663988360758168 ) ) ;
#44365=CARTESIAN_POINT ( 'NONE',  ( 9.822833394071258439, -6.852161475712352789, 34.70806712695775786 ) ) ;
#44366=CARTESIAN_POINT ( 'NONE',  ( 5.207714884747860040, -2.729792928343270919, 31.24908615093345077 ) ) ;
#44368=B_SPLINE_CURVE_WITH_KNOTS ( 'NONE', 3,
 ( #59948, #87447, #53638, #81126, #74361, #12659, #25727, #40144, #67604, #70256 ),
 .UNSPECIFIED., .F., .F.,
 ( 4, 2, 2, 2, 4 ),
 ( 0.0007817246256747483650, 0.0009771112852218926705, 0.001172497944769037084, 0.001367884604316181498, 0.001563271263863325695 ),
 .UNSPECIFIED. ) ;
#44369=CARTESIAN_POINT ( 'NONE',  ( 2.307692307692309264, -12.10708131394839349, 31.69288490824020244 ) ) ;
#44370=ADVANCED_FACE ( 'NONE', ( #48708 ), #14484, .F. ) ;
#44372=ORIENTED_EDGE ( 'NONE', *, *, #32641, .F. ) ;
#44373=CARTESIAN_POINT ( 'NONE',  ( 17.93391658904412012, -12.37446782046654192, 30.86335684631486487 ) ) ;
#44374=ORIENTED_EDGE ( 'NONE', *, *, #68976, .T. ) ;
#44375=EDGE_LOOP ( 'NONE', ( #21696, #58274 ) ) ;
#44376=CARTESIAN_POINT ( 'NONE',  ( 7.596130621932386973, -10.92453946501458795, 33.72985991061850086 ) ) ;
#44378=CARTESIAN_POINT ( 'NONE',  ( -6.222926958906846551, -12.64616026154729411, 30.79003144601913533 ) ) ;
#44379=CARTESIAN_POINT ( 'NONE',  ( -16.15384615384615330, -9.584722331328613620, 36.20867863119891439 ) ) ;
#44380=CARTESIAN_POINT ( 'NONE',  ( -5.999999999999998224, -3.050289026998446396, 32.03036669348365706 ) ) ;
#44383=EDGE_LOOP ( 'NONE', ( #78181, #38453, #2868, #12456, #78852, #64899 ) ) ;
#44384=EDGE_CURVE ( 'NONE', #76146, #32981, #53198, .T. ) ;
#44385=CARTESIAN_POINT ( 'NONE',  ( 8.834486340506796154, -3.835265460703683349, 33.15142922261929925 ) ) ;
#44386=VERTEX_POINT ( 'NONE', #28442 ) ;
#44387=EDGE_LOOP ( 'NONE', ( #34305, #5470, #48988, #78563, #77916, #4515 ) ) ;
#44389=CARTESIAN_POINT ( 'NONE',  ( 18.24994540937804643, -2.341251567377310217, 30.72681386836322659 ) ) ;
#44390=CARTESIAN_POINT ( 'NONE',  ( 16.40390046548447245, -12.41262288849542017, 30.68299917996395010 ) ) ;
#44392=B_SPLINE_CURVE_WITH_KNOTS ( 'NONE', 3,
 ( #87625, #40316, #46618, #67340, #47497, #52915, #60570, #88085, #54696, #26350 ),
 .UNSPECIFIED., .F., .F.,
 ( 4, 2, 2, 2, 4 ),
 ( 0.000000000000000000, 0.0001954339857564071220, 0.0003908679715128142440, 0.0005863019572692213660, 0.0007817359430256284880 ),
 .UNSPECIFIED. ) ;
#44393=CARTESIAN_POINT ( 'NONE',  ( 1.384615384615265343, -3.835265460704628371, 33.15142922262033665 ) ) ;
#44394=CARTESIAN_POINT ( 'NONE',  ( -4.023798547590470065, -7.723484964179500700, 34.74522123443823318 ) ) ;
#44395=CARTESIAN_POINT ( 'NONE',  ( -15.93083480223330284, -2.758310577978207334, 31.33698337089302299 ) ) ;
#44396=ORIENTED_EDGE ( 'NONE', *, *, #70101, .T. ) ;
#44397=ORIENTED_EDGE ( 'NONE', *, *, #58792, .T. ) ;
#44399=ORIENTED_EDGE ( 'NONE', *, *, #72386, .F. ) ;
#44400=CARTESIAN_POINT ( 'NONE',  ( 15.45378058238208219, -5.667800583137506010, 34.40243808032445827 ) ) ;
#44401=ORIENTED_EDGE ( 'NONE', *, *, #48735, .T. ) ;
#44402=CARTESIAN_POINT ( 'NONE',  ( -10.39237177129121825, -4.026326845037962343, 33.68677907613344047 ) ) ;
#44403=CYLINDRICAL_SURFACE ( 'NONE', #59000, 0.2499999999999986955 ) ;
#44404=B_SPLINE_CURVE_WITH_KNOTS ( 'NONE', 3,
 ( #60604, #19623, #4335, #83000, #39471, #87664, #14092, #39914, #45312, #87220 ),
 .UNSPECIFIED., .F., .F.,
 ( 4, 2, 2, 2, 4 ),
 ( 0.0007817246256747524850, 0.0009771112852218972241, 0.001172497944769042072, 0.001367884604316186702, 0.001563271263863331550 ),
 .UNSPECIFIED. ) ;
#44405=CARTESIAN_POINT ( 'NONE',  ( -3.165513659493206067, -10.21337939537593797, 33.94971097300152252 ) ) ;
#44406=ORIENTED_EDGE ( 'NONE', *, *, #89162, .T. ) ;
#44407=CARTESIAN_POINT ( 'NONE',  ( -14.37377468705244077, -12.34228464037088280, 31.77849191805838558 ) ) ;
#44408=VECTOR ( 'NONE', #50085, 1000.000000000000227 ) ;
#44409=VERTEX_POINT ( 'NONE', #63103 ) ;
#44410=CARTESIAN_POINT ( 'NONE',  ( 2.307692307692309264, -8.973038597847269315, 34.52809138561121927 ) ) ;
#44411=CARTESIAN_POINT ( 'NONE',  ( 17.75002325595141173, -12.65889640711025521, 30.72598325615533454 ) ) ;
#44412=EDGE_CURVE ( 'NONE', #44792, #77538, #16673, .T. ) ;
#44413=CARTESIAN_POINT ( 'NONE',  ( -17.93393266664992680, -2.486705287966280320, 31.30864560766543647 ) ) ;
#44414=CYLINDRICAL_SURFACE ( 'NONE', #86401, 0.2500000000000009437 ) ;
#44415=CARTESIAN_POINT ( 'NONE',  ( -6.700065571464074665, -2.554770724473668153, 30.48948780036025852 ) ) ;
#44416=CARTESIAN_POINT ( 'NONE',  ( 4.826899839630110378, -2.587272538249754117, 30.68239716806877837 ) ) ;
#44417=DIRECTION ( 'NONE',  ( 0.000000000000000000, 0.3420201433256610524, 0.9396926207859113145 ) ) ;
#44418=ORIENTED_EDGE ( 'NONE', *, *, #85975, .F. ) ;
#44419=CARTESIAN_POINT ( 'NONE',  ( -9.692307692307812417, -6.026961402154118019, 34.52809138561165270 ) ) ;
#44421=CARTESIAN_POINT ( 'NONE',  ( 2.307692307692309264, -2.833524468853757305, 32.15551576947925838 ) ) ;
#44422=ORIENTED_EDGE ( 'NONE', *, *, #6810, .T. ) ;
#44423=EDGE_CURVE ( 'NONE', #58471, #29571, #82519, .T. ) ;
#44424=CARTESIAN_POINT ( 'NONE',  ( 11.47319153790522073, -12.16647553114622049, 32.15551576947930812 ) ) ;
#44425=CARTESIAN_POINT ( 'NONE',  ( 15.29602480204525605, -4.481592998940250538, 33.73612834413965089 ) ) ;
#44426=CARTESIAN_POINT ( 'NONE',  ( -3.931066612577743147, -2.600157965045225339, 30.74683119005207743 ) ) ;
#44427=CARTESIAN_POINT ( 'NONE',  ( -5.999999999999998224, -5.557115091759785130, 34.35708131394839171 ) ) ;
#44428=CARTESIAN_POINT ( 'NONE',  ( -7.976629031229566458, -7.276987145209185215, 34.99546412871779211 ) ) ;
#44429=FACE_BOUND ( 'NONE', #15147, .T. ) ;
#44430=CARTESIAN_POINT ( 'NONE',  ( 13.38461538461526423, -2.379036618888197729, 30.90682066428292885 ) ) ;
#44431=DIRECTION ( 'NONE',  ( -0.000000000000000000, -0.3420201433256694901, -0.9396926207859082059 ) ) ;
#44432=FACE_OUTER_BOUND ( 'NONE', #84713, .T. ) ;
#44433=CARTESIAN_POINT ( 'NONE',  ( -1.384615384615383471, -12.10708131394839349, 31.69288490824020244 ) ) ;
#44434=CARTESIAN_POINT ( 'NONE',  ( 14.17754433796061342, -11.04286588640298561, 33.62463336215343901 ) ) ;
#44435=DIRECTION ( 'NONE',  ( -0.000000000000000000, 0.1736481776669307198, -0.9848077530122080203 ) ) ;
#44436=EDGE_CURVE ( 'NONE', #17506, #12547, #84737, .T. ) ;
#44437=CARTESIAN_POINT ( 'NONE',  ( 9.019285080869085647, -10.66356715214248752, 33.62249196103329751 ) ) ;
#44439=VERTEX_POINT ( 'NONE', #29779 ) ;
#44441=DIRECTION ( 'NONE',  ( -0.000000000000000000, -0.1736481776669307198, -0.9848077530122080203 ) ) ;
#44442=EDGE_CURVE ( 'NONE', #16132, #83475, #22112, .T. ) ;
#44445=CARTESIAN_POINT ( 'NONE',  ( -9.758391103263571509, -10.51840700105979387, 33.73612834413961536 ) ) ;
#44446=CARTESIAN_POINT ( 'NONE',  ( 10.68064018666064641, -12.27809138561124591, 31.22303859784720359 ) ) ;
#44447=DIRECTION ( 'NONE',  ( 0.000000000000000000, 0.8660254037844377084, 0.5000000000000015543 ) ) ;
#44449=CARTESIAN_POINT ( 'NONE',  ( -15.23076923076922995, -12.62096338111211580, 30.90682066428153263 ) ) ;
#44450=CARTESIAN_POINT ( 'NONE',  ( -2.177166869458661669, -6.808710257144159783, 34.95449254468098843 ) ) ;
#44451=AXIS2_PLACEMENT_3D ( 'NONE', #64554, #72661, #58255 ) ;
#44452=ADVANCED_FACE ( 'NONE', ( #56361 ), #57685, .F. ) ;
#44453=CARTESIAN_POINT ( 'NONE',  ( -16.94639737515951339, -6.001044277235011215, 34.52024696741798948 ) ) ;
#44454=CARTESIAN_POINT ( 'NONE',  ( -2.980823821391187955, -12.07971442181321997, 32.31769673815850297 ) ) ;
#44455=LINE ( 'NONE', #85028, #20935 ) ;
#44456=CARTESIAN_POINT ( 'NONE',  ( 12.33084785842815734, -12.62707690430377383, 30.88035979386743435 ) ) ;
#44457=AXIS2_PLACEMENT_3D ( 'NONE', #12580, #67524, #51756 ) ;
#44458=CARTESIAN_POINT ( 'NONE',  ( -18.00000000000000000, -2.721908614388771852, 31.22303859784724978 ) ) ;
#44459=CARTESIAN_POINT ( 'NONE',  ( 14.17700084102474989, -6.413092428213692742, 34.63065189839063152 ) ) ;
#44460=ORIENTED_EDGE ( 'NONE', *, *, #58038, .T. ) ;
#44461=LINE ( 'NONE', #17459, #78688 ) ;
#44462=CARTESIAN_POINT ( 'NONE',  ( -17.07692307692307665, -2.721908614388771852, 31.22303859784724978 ) ) ;
#44465=B_SPLINE_CURVE_WITH_KNOTS ( 'NONE', 3,
 ( #15561, #8806, #50206, #51087, #71822, #43027, #43469, #78580, #64167, #1600 ),
 .UNSPECIFIED., .F., .F.,
 ( 4, 2, 2, 2, 4 ),
 ( 0.000000000000000000, 0.0001954311564186864678, 0.0003908623128373729357, 0.0005862934692560594577, 0.0007817246256747458714 ),
 .UNSPECIFIED. ) ;
#44466=CARTESIAN_POINT ( 'NONE',  ( 6.792928953345226617, -5.070767119584671079, 34.40440758774516183 ) ) ;
#44467=CARTESIAN_POINT ( 'NONE',  ( -5.300408020647024543, -2.599994579823202923, 30.74605699353653776 ) ) ;
#44468=VERTEX_POINT ( 'NONE', #9494 ) ;
#44469=CARTESIAN_POINT ( 'NONE',  ( 1.450683735617825043, -4.098570777380720287, 33.41473453929635440 ) ) ;
#44470=DIRECTION ( 'NONE',  ( 0.000000000000000000, 1.000000000000000000, 0.000000000000000000 ) ) ;
#44471=CARTESIAN_POINT ( 'NONE',  ( -12.21153846153704237, -7.500000000000154543, 35.00000000000007105 ) ) ;
#44475=CYLINDRICAL_SURFACE ( 'NONE', #71401, 0.2499999999999986955 ) ;
#44476=CYLINDRICAL_SURFACE ( 'NONE', #29122, 0.2500000000000002220 ) ;
#44477=CARTESIAN_POINT ( 'NONE',  ( -14.17716660592875044, -11.46989282347013095, 32.79007818306219946 ) ) ;
#44478=VERTEX_POINT ( 'NONE', #29340 ) ;
#44480=CARTESIAN_POINT ( 'NONE',  ( -11.53846153846122391, -2.255955759149395501, 30.00000000000324363 ) ) ;
#44481=EDGE_CURVE ( 'NONE', #64117, #73491, #74763, .T. ) ;
#44482=CARTESIAN_POINT ( 'NONE',  ( 16.15384615384603251, -12.51329471203414379, 31.30864560766407578 ) ) ;
#44483=EDGE_LOOP ( 'NONE', ( #68431, #86127 ) ) ;
#44484=VERTEX_POINT ( 'NONE', #70317 ) ;
#44485=AXIS2_PLACEMENT_3D ( 'NONE', #9667, #37578, #65039 ) ;
#44487=CARTESIAN_POINT ( 'NONE',  ( 3.296024370282069071, -2.379036618887895305, 30.90682066428159303 ) ) ;
#44488=CARTESIAN_POINT ( 'NONE',  ( 9.942253101685736283, -4.176053281294518804, 33.81426240980091791 ) ) ;
#44489=DIRECTION ( 'NONE',  ( -1.000000000000000000, 0.000000000000000000, 0.000000000000000000 ) ) ;
#44490=EDGE_CURVE ( 'NONE', #61936, #35844, #43474, .T. ) ;
#44491=LINE ( 'NONE', #30984, #10392 ) ;
#44493=ADVANCED_FACE ( 'NONE', ( #2726 ), #78837, .F. ) ;
#44494=ORIENTED_EDGE ( 'NONE', *, *, #61757, .F. ) ;
#44495=ORIENTED_EDGE ( 'NONE', *, *, #53365, .T. ) ;
#44496=CARTESIAN_POINT ( 'NONE',  ( 4.284371592079798674, -5.915461855592777596, 34.75538340440931506 ) ) ;
#44497=EDGE_LOOP ( 'NONE', ( #47162, #44151 ) ) ;
#44498=EDGE_CURVE ( 'NONE', #40198, #48420, #31673, .T. ) ;
#44499=B_SPLINE_CURVE_WITH_KNOTS ( 'NONE', 3,
 ( #87939, #14011, #506, #33840, #40613, #35173, #88372, #74389, #62196, #55002 ),
 .UNSPECIFIED., .F., .F.,
 ( 4, 2, 2, 2, 4 ),
 ( 0.0007817359430256216575, 0.0009771253907249856981, 0.001172514838424349630, 0.001367904286123713779, 0.001563293733823077711 ),
 .UNSPECIFIED. ) ;
#44500=CARTESIAN_POINT ( 'NONE',  ( 12.68431813051652846, -11.60474049983371003, 33.02348890104160262 ) ) ;
#44501=VECTOR ( 'NONE', #73370, 1000.000000000000000 ) ;
#44502=AXIS2_PLACEMENT_3D ( 'NONE', #15513, #10076, #57371 ) ;
#44503=CARTESIAN_POINT ( 'NONE',  ( 2.438218009455874746, -3.816742781228458448, 33.13167719472716044 ) ) ;
#44504=CARTESIAN_POINT ( 'NONE',  ( -17.99999999841483955, -2.249999999999995115, 29.50000000010503953 ) ) ;
#44506=ORIENTED_EDGE ( 'NONE', *, *, #45523, .T. ) ;
#44507=AXIS2_PLACEMENT_3D ( 'NONE', #62696, #1014, #55950 ) ;
#44508=ORIENTED_EDGE ( 'NONE', *, *, #60924, .T. ) ;
#44510=ORIENTED_EDGE ( 'NONE', *, *, #6347, .T. ) ;
#44511=AXIS2_PLACEMENT_3D ( 'NONE', #37626, #22776, #77723 ) ;
#44512=DIRECTION ( 'NONE',  ( 0.000000000000000000, 0.4999999999999960032, -0.8660254037844410391 ) ) ;
#44514=VERTEX_POINT ( 'NONE', #85604 ) ;
#44515=CARTESIAN_POINT ( 'NONE',  ( -8.769230769230768274, -10.51840700105979565, 33.73612834413961536 ) ) ;
#44516=DIRECTION ( 'NONE',  ( -0.000000000000000000, -0.9396926207859093161, -0.3420201433256663259 ) ) ;
#44517=CARTESIAN_POINT ( 'NONE',  ( 8.900022577055556994, -5.582136614379148654, 34.36778462344220486 ) ) ;
#44518=FACE_BOUND ( 'NONE', #77930, .T. ) ;
#44519=CARTESIAN_POINT ( 'NONE',  ( 15.10062202133100939, -6.001485441113819874, 34.52039167877662607 ) ) ;
#44520=CARTESIAN_POINT ( 'NONE',  ( -6.700064078983528404, -9.172514111537584114, 34.72667873470787470 ) ) ;
#44521=CARTESIAN_POINT ( 'NONE',  ( 13.31934538405906565, -12.70778746994557551, 30.41441678777548319 ) ) ;
#44522=CARTESIAN_POINT ( 'NONE',  ( 5.076923076922953193, -12.70778746994576025, 30.41441678777401236 ) ) ;
#44523=CARTESIAN_POINT ( 'NONE',  ( 9.692307692307572609, -3.300289026999228881, 32.46337939537708905 ) ) ;
#44524=LINE ( 'NONE', #10318, #39517 ) ;
#44525=CARTESIAN_POINT ( 'NONE',  ( -16.40386939113911779, -8.432397168068783699, 34.66272746175022945 ) ) ;
#44527=CARTESIAN_POINT ( 'NONE',  ( -16.02332071561251325, -3.625058011473227815, 33.29252011169590020 ) ) ;
#44528=ORIENTED_EDGE ( 'NONE', *, *, #42796, .F. ) ;
#44529=ORIENTED_EDGE ( 'NONE', *, *, #64284, .F. ) ;
#44530=B_SPLINE_CURVE_WITH_KNOTS ( 'NONE', 3,
 ( #21346, #59783, #53012, #82627, #80513, #35303, #12058, #48811, #68646, #28105 ),
 .UNSPECIFIED., .F., .F.,
 ( 4, 2, 2, 2, 4 ),
 ( 0.000000000000000000, 0.0001954311564186865763, 0.0003908623128373731525, 0.0005862934692560596746, 0.0007817246256747463051 ),
 .UNSPECIFIED. ) ;
#44531=B_SPLINE_CURVE_WITH_KNOTS ( 'NONE', 3,
 ( #29821, #77557, #42896, #22607, #15868, #21727, #70362, #43331, #9535, #49201 ),
 .UNSPECIFIED., .F., .F.,
 ( 4, 2, 2, 2, 4 ),
 ( 0.000000000000000000, 0.0001954339857564074473, 0.0003908679715128148945, 0.0005863019572692223418, 0.0007817359430256297891 ),
 .UNSPECIFIED. ) ;
#44532=LINE ( 'NONE', #65255, #10133 ) ;
#44533=CARTESIAN_POINT ( 'NONE',  ( -5.776988648387147762, -12.15243808032446005, 31.58219941686247978 ) ) ;
#44534=CARTESIAN_POINT ( 'NONE',  ( 2.530471848960717640, -2.600157965045225783, 30.74683119005207743 ) ) ;
#44535=B_SPLINE_CURVE_WITH_KNOTS ( 'NONE', 3,
 ( #76774, #64560, #63690, #49296, #16395, #49734, #76320, #83541, #2862, #21825 ),
 .UNSPECIFIED., .F., .F.,
 ( 4, 2, 2, 2, 4 ),
 ( 0.000000000000000000, 0.0001954339857564083688, 0.0003908679715128167377, 0.0005863019572692250523, 0.0007817359430256334753 ),
 .UNSPECIFIED. ) ;
#44536=FACE_OUTER_BOUND ( 'NONE', #63399, .T. ) ;
#44537=CARTESIAN_POINT ( 'NONE',  ( -0.4615384615384611200, -11.69971097300155272, 32.46337939537588113 ) ) ;
#44539=CARTESIAN_POINT ( 'NONE',  ( 18.25005441991345378, -2.544122305571458575, 31.48381861865057729 ) ) ;
#44540=CARTESIAN_POINT ( 'NONE',  ( 15.16549923021291058, -11.06231777344662781, 33.60647404775220082 ) ) ;
#44541=CARTESIAN_POINT ( 'NONE',  ( -1.449885385171703955, -10.33852847137145048, 34.16647553114627556 ) ) ;
#44542=CARTESIAN_POINT ( 'NONE',  ( 0.2115617174898687114, -3.436278759898155233, 33.07459398097509506 ) ) ;
#44544=VECTOR ( 'NONE', #35955, 1000.000000000000114 ) ;
#44547=VERTEX_POINT ( 'NONE', #46394 ) ;
#44548=CARTESIAN_POINT ( 'NONE',  ( -14.43838291080261627, -4.684245665217972032, 34.18127051446801090 ) ) ;
#44549=ORIENTED_EDGE ( 'NONE', *, *, #43484, .F. ) ;
#44550=CARTESIAN_POINT ( 'NONE',  ( -13.38461538461538325, -11.11383981884818262, 36.00935417666054406 ) ) ;
#44551=CARTESIAN_POINT ( 'NONE',  ( -12.33074665371367651, -9.804649428959608670, 34.18742332936588468 ) ) ;
#44552=CARTESIAN_POINT ( 'NONE',  ( 14.37376065869474751, -2.721908614388771852, 31.22303859784725333 ) ) ;
#44553=CARTESIAN_POINT ( 'NONE',  ( -0.7115152055870517245, -12.01397095200673881, 32.43157075238190146 ) ) ;
#44555=CARTESIAN_POINT ( 'NONE',  ( 1.449870955891410684, -5.219633306516380244, 34.19971097300157936 ) ) ;
#44556=ORIENTED_EDGE ( 'NONE', *, *, #29071, .F. ) ;
#44557=EDGE_CURVE ( 'NONE', #43627, #11372, #59466, .T. ) ;
#44558=CARTESIAN_POINT ( 'NONE',  ( -12.46153846153846168, -12.48256725967547354, 35.29906147534542527 ) ) ;
#44559=CYLINDRICAL_SURFACE ( 'NONE', #33808, 0.2500000000000008882 ) ;
#44561=CARTESIAN_POINT ( 'NONE',  ( -9.627162911588058591, -7.750023224968867197, 34.99404313364389907 ) ) ;
#44562=CARTESIAN_POINT ( 'NONE',  ( 14.24242186173153613, -12.27809138561121394, 31.22303859784730307 ) ) ;
#44563=CARTESIAN_POINT ( 'NONE',  ( 17.07692307692307665, -10.89733346790207413, 36.13435417666054406 ) ) ;
#44564=CARTESIAN_POINT ( 'NONE',  ( -2.241624974342229848, -2.292212530054420494, 30.41441678777542990 ) ) ;
#44565=CARTESIAN_POINT ( 'NONE',  ( -0.2115929431903188496, -11.37275283266503756, 32.91324779482534524 ) ) ;
#44566=CARTESIAN_POINT ( 'NONE',  ( -3.007989689500822017, -11.41317474335729187, 32.86274602512330034 ) ) ;
#44567=CARTESIAN_POINT ( 'NONE',  ( 15.29683758177167086, -11.16473453929635440, 33.15142922261926373 ) ) ;
#44570=CARTESIAN_POINT ( 'NONE',  ( -12.46153846153846168, -10.67929555188718282, 33.92786785259544047 ) ) ;
#44571=CARTESIAN_POINT ( 'NONE',  ( -5.326923076923075762, -7.433932668274256805, 35.00000000000000711 ) ) ;
#44572=LINE ( 'NONE', #72060, #17498 ) ;
#44576=CARTESIAN_POINT ( 'NONE',  ( -13.60810032833933469, -12.44517049084099725, 30.48991314939691932 ) ) ;
#44577=CARTESIAN_POINT ( 'NONE',  ( 8.638540166120458608, -9.929715669179220328, 34.40415004197138416 ) ) ;
#44578=B_SPLINE_CURVE_WITH_KNOTS ( 'NONE', 3,
 ( #57711, #50927, #78861, #79767, #79319, #78415, #30243, #58142, #52276, #71213 ),
 .UNSPECIFIED., .F., .F.,
 ( 4, 2, 2, 2, 4 ),
 ( 0.0007817359430256283796, 0.0009771253907249943717, 0.001172514838424360255, 0.001367904286123726356, 0.001563293733823092240 ),
 .UNSPECIFIED. ) ;
#44579=ORIENTED_EDGE ( 'NONE', *, *, #76754, .T. ) ;
#44581=EDGE_CURVE ( 'NONE', #530, #13588, #40100, .T. ) ;
#44582=CARTESIAN_POINT ( 'NONE',  ( -1.161835715637319577, -12.47679350104403007, 31.42216943046557276 ) ) ;
#44583=VERTEX_POINT ( 'NONE', #72979 ) ;
#44584=AXIS2_PLACEMENT_3D ( 'NONE', #87003, #39246, #66708 ) ;
#44585=CARTESIAN_POINT ( 'NONE',  ( -3.931066484868086963, -2.612705202774697533, 31.66806509827799943 ) ) ;
#44587=CARTESIAN_POINT ( 'NONE',  ( -9.692307692307691624, -10.51840700105979565, 33.73612834413961536 ) ) ;
#44588=FACE_OUTER_BOUND ( 'NONE', #32050, .T. ) ;
#44589=EDGE_CURVE ( 'NONE', #57339, #43411, #19866, .T. ) ;
#44590=CARTESIAN_POINT ( 'NONE',  ( -0.3307480205715113697, -6.369690395747422684, 34.87708834333098196 ) ) ;
#44591=EDGE_LOOP ( 'NONE', ( #44748, #83188 ) ) ;
#44593=ORIENTED_EDGE ( 'NONE', *, *, #42869, .T. ) ;
#44594=DIRECTION ( 'NONE',  ( -0.000000000000000000, 0.9848077530122086864, -0.1736481776669273891 ) ) ;
#44595=ORIENTED_EDGE ( 'NONE', *, *, #68647, .T. ) ;
#44596=CARTESIAN_POINT ( 'NONE',  ( 2.307692307692615685, -2.506253911140615021, 30.00000000000323297 ) ) ;
#44597=DIRECTION ( 'NONE',  ( -0.000000000000000000, 0.8660254037844399289, -0.4999999999999980016 ) ) ;
#44598=ORIENTED_EDGE ( 'NONE', *, *, #84572, .F. ) ;
#44599=LINE ( 'NONE', #64429, #31833 ) ;
#44600=CYLINDRICAL_SURFACE ( 'NONE', #3306, 0.2499999999999994726 ) ;
#44601=CARTESIAN_POINT ( 'NONE',  ( -11.60454494941741999, -2.721908614388770964, 31.22303859784723912 ) ) ;
#44602=CARTESIAN_POINT ( 'NONE',  ( 7.846153846153846700, -1.951392089020283160, 34.73218667398347748 ) ) ;
#44603=CARTESIAN_POINT ( 'NONE',  ( -13.13466997523734392, -12.07971442181322175, 32.31769673815850297 ) ) ;
#44604=EDGE_CURVE ( 'NONE', #33104, #81317, #39208, .T. ) ;
#44605=EDGE_CURVE ( 'NONE', #64975, #25175, #1681, .T. ) ;
#44606=VERTEX_POINT ( 'NONE', #4521 ) ;
#44607=ORIENTED_EDGE ( 'NONE', *, *, #18303, .F. ) ;
#44608=ORIENTED_EDGE ( 'NONE', *, *, #13721, .T. ) ;
#44609=B_SPLINE_CURVE_WITH_KNOTS ( 'NONE', 3,
 ( #6187, #60676, #68322, #74645, #55247, #47605, #75091, #7066, #62004, #310 ),
 .UNSPECIFIED., .F., .F.,
 ( 4, 2, 2, 2, 4 ),
 ( 0.000000000000000000, 0.0001954339857564097241, 0.0003908679715128194482, 0.0005863019572692291723, 0.0007817359430256388964 ),
 .UNSPECIFIED. ) ;
#44610=CARTESIAN_POINT ( 'NONE',  ( 3.100078627658922503, -5.496505350115500121, 34.60290016733514307 ) ) ;
#44611=EDGE_LOOP ( 'NONE', ( #2222, #87959 ) ) ;
#44612=VECTOR ( 'NONE', #44351, 1000.000000000000000 ) ;
#44613=CARTESIAN_POINT ( 'NONE',  ( -14.24243716817946570, -11.06231777344671130, 33.60647404775212976 ) ) ;
#44614=CARTESIAN_POINT ( 'NONE',  ( 5.076923076923075762, -4.098570777380720287, 33.41473453929634729 ) ) ;
#44615=ORIENTED_EDGE ( 'NONE', *, *, #32378, .T. ) ;
#44617=ORIENTED_EDGE ( 'NONE', *, *, #22803, .F. ) ;
#44618=CARTESIAN_POINT ( 'NONE',  ( 0.3313904918067661076, -8.630895178749536711, 34.87696386517710323 ) ) ;
#44619=ORIENTED_EDGE ( 'NONE', *, *, #67033, .T. ) ;
#44620=CARTESIAN_POINT ( 'NONE',  ( 2.438484115517095763, -4.118422570099827595, 33.43335022499816489 ) ) ;
#44621=CARTESIAN_POINT ( 'NONE',  ( 16.94677510719138169, -12.50552854090298638, 31.33409797877408920 ) ) ;
#44622=LINE ( 'NONE', #83876, #29610 ) ;
#44623=B_SPLINE_CURVE_WITH_KNOTS ( 'NONE', 3,
 ( #1709, #29198, #57088, #56210, #83246, #15673, #84145, #49456, #76033, #82809 ),
 .UNSPECIFIED., .F., .F.,
 ( 4, 2, 2, 2, 4 ),
 ( 0.0007817359430256388964, 0.0009771253907250075990, 0.001172514838424376085, 0.001367904286123744571, 0.001563293733823113273 ),
 .UNSPECIFIED. ) ;
#44624=FACE_BOUND ( 'NONE', #8697, .T. ) ;
#44625=ORIENTED_EDGE ( 'NONE', *, *, #64417, .F. ) ;
#44626=CARTESIAN_POINT ( 'NONE',  ( 12.71148397988660328, -5.852078868378309373, 34.47109172314383585 ) ) ;
#44627=B_SPLINE_CURVE_WITH_KNOTS ( 'NONE', 3,
 ( #10455, #18988, #11336, #30712, #66277, #46006, #46454, #37466, #17659, #58178 ),
 .UNSPECIFIED., .F., .F.,
 ( 4, 2, 2, 2, 4 ),
 ( 0.0007817359430256216575, 0.0009771253907249856981, 0.001172514838424349847, 0.001367904286123713779, 0.001563293733823077928 ),
 .UNSPECIFIED. ) ;
#44628=AXIS2_PLACEMENT_3D ( 'NONE', #76256, #75385, #34389 ) ;
#44630=DIRECTION ( 'NONE',  ( -0.000000000000000000, -0.3420201433256694901, -0.9396926207859082059 ) ) ;
#44631=CARTESIAN_POINT ( 'NONE',  ( 7.911409417429871027, -10.90142922261932057, 33.41473453929631887 ) ) ;
#44632=VERTEX_POINT ( 'NONE', #25681 ) ;
#44634=EDGE_LOOP ( 'NONE', ( #34558, #41945 ) ) ;
#44635=AXIS2_PLACEMENT_3D ( 'NONE', #30417, #86271, #37166 ) ;
#44636=ORIENTED_EDGE ( 'NONE', *, *, #17908, .F. ) ;
#44637=VECTOR ( 'NONE', #14313, 1000.000000000000114 ) ;
#44638=CARTESIAN_POINT ( 'NONE',  ( -0.5276218724943415594, -8.973038597847271092, 34.52809138561120506 ) ) ;
#44639=CARTESIAN_POINT ( 'NONE',  ( -1.515305987725692027, -5.496505350115500121, 34.60290016733514307 ) ) ;
#44641=CARTESIAN_POINT ( 'NONE',  ( -10.68146802634049486, -12.10708131394839349, 31.69288490824020244 ) ) ;
#44642=CARTESIAN_POINT ( 'NONE',  ( -2.057746789344164107, -12.22109172314383052, 31.39792113162168263 ) ) ;
#44643=CARTESIAN_POINT ( 'NONE',  ( -18.06527000055631760, -5.941354392334500467, 34.76329471203369792 ) ) ;
#44644=CARTESIAN_POINT ( 'NONE',  ( -6.923076923077045919, -3.643525952248796163, 33.31231777344771672 ) ) ;
#44645=EDGE_LOOP ( 'NONE', ( #38172, #54138 ) ) ;
#44646=LINE ( 'NONE', #24831, #28504 ) ;
#44647=CARTESIAN_POINT ( 'NONE',  ( 17.86930939688968678, -3.338472653186243200, 32.95098750199972670 ) ) ;
#44648=CARTESIAN_POINT ( 'NONE',  ( 10.55011461482829560, -3.083524468853724443, 32.58852847137143272 ) ) ;
#44649=CARTESIAN_POINT ( 'NONE',  ( 13.38461538461526601, -12.46129190930018460, 30.37095296980731973 ) ) ;
#44651=ORIENTED_EDGE ( 'NONE', *, *, #72418, .T. ) ;
#44652=FACE_BOUND ( 'NONE', #9831, .T. ) ;
#44654=CARTESIAN_POINT ( 'NONE',  ( 7.596177115211495412, -2.779195860258147022, 31.39871582349836743 ) ) ;
#44655=LINE ( 'NONE', #37923, #76350 ) ;
#44656=ORIENTED_EDGE ( 'NONE', *, *, #31312, .F. ) ;
#44657=CARTESIAN_POINT ( 'NONE',  ( -3.360916440207450506, -12.45813303252208648, 30.39737893381572675 ) ) ;
#44658=CARTESIAN_POINT ( 'NONE',  ( -2.084912766423896446, -4.387253974876676565, 33.66317474335728832 ) ) ;
#44659=DIRECTION ( 'NONE',  ( 0.000000000000000000, 0.1736481776669275834, 0.9848077530122086864 ) ) ;
#44661=ORIENTED_EDGE ( 'NONE', *, *, #80924, .T. ) ;
#44662=EDGE_CURVE ( 'NONE', #21693, #81733, #57500, .T. ) ;
#44663=CARTESIAN_POINT ( 'NONE',  ( -6.923076923076922462, -2.721908614388771852, 31.22303859784724978 ) ) ;
#44664=ORIENTED_EDGE ( 'NONE', *, *, #55803, .F. ) ;
#44665=EDGE_CURVE ( 'NONE', #65223, #86258, #40302, .T. ) ;
#44666=CARTESIAN_POINT ( 'NONE',  ( -2.307692307692428724, -12.16647553114689728, 32.15551576947799362 ) ) ;
#44667=ORIENTED_EDGE ( 'NONE', *, *, #19997, .F. ) ;
#44668=CYLINDRICAL_SURFACE ( 'NONE', #87214, 0.2499999999999994726 ) ;
#44670=CARTESIAN_POINT ( 'NONE',  ( 15.10007862765892206, -4.684245665217972032, 34.18127051446801090 ) ) ;
#44671=CARTESIAN_POINT ( 'NONE',  ( 2.307692307692309264, -1.790695186598648903, 34.54067556320373455 ) ) ;
#44672=CARTESIAN_POINT ( 'NONE',  ( 18.06525557127601900, -8.613356846314930593, 34.62446782046653482 ) ) ;
#44674=CARTESIAN_POINT ( 'NONE',  ( 12.33084785842815378, -5.496505350115501010, 34.60290016733514307 ) ) ;
#44675=B_SPLINE_CURVE_WITH_KNOTS ( 'NONE', 3,
 ( #55347, #49915, #8945, #62536, #89163, #62107, #69318, #21111, #27442, #62976 ),
 .UNSPECIFIED., .F., .F.,
 ( 4, 2, 2, 2, 4 ),
 ( 0.0007817246256747450040, 0.0009771112852218881168, 0.001172497944769031230, 0.001367884604316174342, 0.001563271263863317455 ),
 .UNSPECIFIED. ) ;
#44678=CARTESIAN_POINT ( 'NONE',  ( -16.15384615384615330, -12.37446782046654192, 30.86335684631486131 ) ) ;
#44679=CARTESIAN_POINT ( 'NONE',  ( 13.60739505359345181, -12.69155399931963046, 30.53255429739157734 ) ) ;
#44681=ADVANCED_FACE ( 'NONE', ( #12617 ), #10837, .F. ) ;
#44682=VERTEX_POINT ( 'NONE', #89179 ) ;
#44683=ORIENTED_EDGE ( 'NONE', *, *, #69170, .T. ) ;
#44684=CARTESIAN_POINT ( 'NONE',  ( -11.76138775597768316, -10.61292498521070549, 33.66303323003028680 ) ) ;
#44685=CARTESIAN_POINT ( 'NONE',  ( 7.596130621932389637, -6.652501968072646932, 34.93155406624980941 ) ) ;
#44686=EDGE_CURVE ( 'NONE', #21246, #38559, #3745, .T. ) ;
#44687=CARTESIAN_POINT ( 'NONE',  ( -5.011667937410237528, -12.70778746994558439, 30.41441678777537305 ) ) ;
#44688=DIRECTION ( 'NONE',  ( -0.000000000000000000, -0.9848077530122086864, -0.1736481776669273613 ) ) ;
#44689=CARTESIAN_POINT ( 'NONE',  ( 10.36540788444226102, -4.236021600441997492, 33.53823185664189310 ) ) ;
#44690=CARTESIAN_POINT ( 'NONE',  ( -16.94613263595612551, -11.37503395064541678, 33.29242100308974983 ) ) ;
#44692=ORIENTED_EDGE ( 'NONE', *, *, #24694, .F. ) ;
#44693=CARTESIAN_POINT ( 'NONE',  ( -14.30769230769230660, -6.681629849574314051, 35.83090037661290239 ) ) ;
#44696=EDGE_CURVE ( 'NONE', #2574, #56880, #45714, .T. ) ;
#44697=FACE_OUTER_BOUND ( 'NONE', #17911, .T. ) ;
#44700=CARTESIAN_POINT ( 'NONE',  ( 12.23805353697412635, -2.612411019501189369, 31.66733052389439962 ) ) ;
#44701=VECTOR ( 'NONE', #71722, 1000.000000000000114 ) ;
#44703=EDGE_LOOP ( 'NONE', ( #75110, #11190, #47587, #85706 ) ) ;
#44704=CARTESIAN_POINT ( 'NONE',  ( 13.38461538461538680, -13.63283147151868846, 33.57946703557072254 ) ) ;
#44705=CARTESIAN_POINT ( 'NONE',  ( 10.39245765647776309, -3.395401636524185474, 33.02366814457250399 ) ) ;
#44706=DIRECTION ( 'NONE',  ( -0.000000000000000000, -0.9848077530122085754, -0.1736481776669273613 ) ) ;
#44707=VERTEX_POINT ( 'NONE', #76077 ) ;
#44708=LINE ( 'NONE', #57355, #62213 ) ;
#44709=CARTESIAN_POINT ( 'NONE',  ( 10.61538461538449596, -3.835265460704628371, 33.15142922262033665 ) ) ;
#44711=CARTESIAN_POINT ( 'NONE',  ( 8.703906756426460944, -7.749976730030849303, 34.74374725381503737 ) ) ;
#44712=DIRECTION ( 'NONE',  ( -0.000000000000000000, 0.9396926207859093161, -0.3420201433256663259 ) ) ;
#44713=B_SPLINE_CURVE_WITH_KNOTS ( 'NONE', 3,
 ( #38541, #67785, #33110, #87631, #60575, #11962, #88093, #32661, #5637, #4759 ),
 .UNSPECIFIED., .F., .F.,
 ( 4, 2, 2, 2, 4 ),
 ( 0.000000000000000000, 0.0001954311564186867931, 0.0003908623128373735862, 0.0005862934692560603251, 0.0007817246256747471724 ),
 .UNSPECIFIED. ) ;
#44714=B_SPLINE_CURVE_WITH_KNOTS ( 'NONE', 3,
 ( #34479, #68706, #33600, #13760, #40804, #81350, #68266, #76348, #42139, #26841 ),
 .UNSPECIFIED., .F., .F.,
 ( 4, 2, 2, 2, 4 ),
 ( 0.000000000000000000, 0.0001954311564186864949, 0.0003908623128373729899, 0.0005862934692560594577, 0.0007817246256747459798 ),
 .UNSPECIFIED. ) ;
#44715=EDGE_CURVE ( 'NONE', #58562, #6303, #41415, .T. ) ;
#44716=ORIENTED_EDGE ( 'NONE', *, *, #52633, .T. ) ;
#44717=CARTESIAN_POINT ( 'NONE',  ( -1.134561072977069651, -3.627508038966689163, 32.91356715214248396 ) ) ;
#44718=EDGE_CURVE ( 'NONE', #17646, #78512, #84325, .T. ) ;
#44720=CYLINDRICAL_SURFACE ( 'NONE', #18449, 0.2500000000000008882 ) ;
#44721=DIRECTION ( 'NONE',  ( -0.000000000000000000, 0.9396926207859093161, -0.3420201433256663259 ) ) ;
#44722=CARTESIAN_POINT ( 'NONE',  ( -16.28399336328438096, -11.47017969459903952, 32.78971311882035167 ) ) ;
#44723=EDGE_CURVE ( 'NONE', #35423, #13555, #27359, .T. ) ;
#44724=CARTESIAN_POINT ( 'NONE',  ( 11.53846153846141576, -5.941354392335915335, 34.76329471203413846 ) ) ;
#44725=EDGE_CURVE ( 'NONE', #16932, #45628, #77935, .T. ) ;
#44727=CARTESIAN_POINT ( 'NONE',  ( 15.90386940979756503, -12.01397095200673881, 32.43157075238190146 ) ) ;
#44730=ORIENTED_EDGE ( 'NONE', *, *, #76368, .F. ) ;
#44731=AXIS2_PLACEMENT_3D ( 'NONE', #68545, #7741, #536 ) ;
#44732=ORIENTED_EDGE ( 'NONE', *, *, #80015, .F. ) ;
#44733=VERTEX_POINT ( 'NONE', #867 ) ;
#44734=CARTESIAN_POINT ( 'NONE',  ( -12.59209837515182784, -2.254533558242299396, 29.97296025877828285 ) ) ;
#44735=CARTESIAN_POINT ( 'NONE',  ( -2.241623956689868358, -3.050289026998446840, 32.03036669348366416 ) ) ;
#44737=CARTESIAN_POINT ( 'NONE',  ( -7.145942345280561270, -2.501496062324911840, 29.88072118266895671 ) ) ;
#44738=CARTESIAN_POINT ( 'NONE',  ( -6.989160334032800570, -3.050289026998445951, 32.03036669348365706 ) ) ;
#44739=CARTESIAN_POINT ( 'NONE',  ( -13.38461538461550582, -6.026961402154118019, 34.52809138561165270 ) ) ;
#44741=B_SPLINE_CURVE_WITH_KNOTS ( 'NONE', 3,
 ( #75958, #34963, #84062, #1178, #14703, #27766, #36311, #15590, #14257, #741 ),
 .UNSPECIFIED., .F., .F.,
 ( 4, 2, 2, 2, 4 ),
 ( 0.0007817359430256390048, 0.0009771253907250078159, 0.001172514838424376735, 0.001367904286123745655, 0.001563293733823114574 ),
 .UNSPECIFIED. ) ;
#44742=B_SPLINE_CURVE_WITH_KNOTS ( 'NONE', 3,
 ( #7014, #35373, #14666, #77245, #27725, #55636 ),
 .UNSPECIFIED., .F., .F.,
 ( 4, 2, 4 ),
 ( 0.000000000000000000, 0.0001954784845028902421, 0.0003909569690057804843 ),
 .UNSPECIFIED. ) ;
#44743=CARTESIAN_POINT ( 'NONE',  ( -18.00000000000000000, -9.780366693483671270, 34.19971097300155094 ) ) ;
#44745=CARTESIAN_POINT ( 'NONE',  ( -4.284537620513712675, -9.804603061927743113, 34.18744698557895845 ) ) ;
#44747=EDGE_LOOP ( 'NONE', ( #47881, #15188, #19378, #29431 ) ) ;
#44748=ORIENTED_EDGE ( 'NONE', *, *, #53472, .F. ) ;
#44749=CARTESIAN_POINT ( 'NONE',  ( 0.4615384615384611200, -2.833524468853757305, 32.15551576947925838 ) ) ;
#44750=EDGE_LOOP ( 'NONE', ( #47144, #57661 ) ) ;
#44751=CYLINDRICAL_SURFACE ( 'NONE', #51772, 0.2500000000000012212 ) ;
#44752=CARTESIAN_POINT ( 'NONE',  ( 10.54930120442873687, -8.973038597847271092, 34.52809138561120506 ) ) ;
#44753=ADVANCED_FACE ( 'NONE', ( #21130 ), #49048, .F. ) ;
#44754=DIRECTION ( 'NONE',  ( -0.000000000000000000, -0.3420201433256694346, -0.9396926207859080948 ) ) ;
#44755=CYLINDRICAL_SURFACE ( 'NONE', #32222, 0.2499999999999997502 ) ;
#44756=VERTEX_POINT ( 'NONE', #64650 ) ;
#44758=ORIENTED_EDGE ( 'NONE', *, *, #65218, .F. ) ;
#44759=CARTESIAN_POINT ( 'NONE',  ( -11.76138849736838132, -11.98009711892699514, 32.48740034544076138 ) ) ;
#44760=ORIENTED_EDGE ( 'NONE', *, *, #5641, .F. ) ;
#44761=FACE_BOUND ( 'NONE', #40009, .T. ) ;
#44762=LINE ( 'NONE', #10999, #51894 ) ;
#44763=CARTESIAN_POINT ( 'NONE',  ( 11.53846153846141753, -3.300289026999228881, 32.46337939537708905 ) ) ;
#44764=EDGE_LOOP ( 'NONE', ( #58907, #37898 ) ) ;
#44765=CARTESIAN_POINT ( 'NONE',  ( 14.08476609017615822, -2.758268499246657068, 31.33685645148948140 ) ) ;
#44766=CARTESIAN_POINT ( 'NONE',  ( 8.835397375822410027, -7.250054591869670162, 34.99404684341514127 ) ) ;
#44767=LINE ( 'NONE', #45668, #17718 ) ;
#44768=ORIENTED_EDGE ( 'NONE', *, *, #36008, .T. ) ;
#44769=CARTESIAN_POINT ( 'NONE',  ( 18.24999999999993250, -7.565270000091922853, 34.99999999999999289 ) ) ;
#44770=DIRECTION ( 'NONE',  ( 0.000000000000000000, 0.8660254037844377084, 0.5000000000000015543 ) ) ;
#44771=ORIENTED_EDGE ( 'NONE', *, *, #75162, .T. ) ;
#44772=ADVANCED_FACE ( 'NONE', ( #24113 ), #23672, .F. ) ;
#44773=CARTESIAN_POINT ( 'NONE',  ( -6.792551221313359200, -9.417988943895561960, 34.36773134775778260 ) ) ;
#44774=CARTESIAN_POINT ( 'NONE',  ( 6.988332494352947677, -10.90142922261932057, 33.41473453929631887 ) ) ;
#44775=ORIENTED_EDGE ( 'NONE', *, *, #67001, .F. ) ;
#44776=CARTESIAN_POINT ( 'NONE',  ( -12.46153846153846168, -2.292212530054420494, 30.41441678777542634 ) ) ;
#44777=CARTESIAN_POINT ( 'NONE',  ( 14.43821800945587341, -8.586989748646452369, 34.63063291749215011 ) ) ;
#44778=FACE_OUTER_BOUND ( 'NONE', #997, .T. ) ;
#44781=CARTESIAN_POINT ( 'NONE',  ( 8.992243613324164997, -4.026326845037962343, 33.68677907613344047 ) ) ;
#44782=CARTESIAN_POINT ( 'NONE',  ( -1.449885830576159496, -2.892918686051582977, 31.69288490824016691 ) ) ;
#44783=CARTESIAN_POINT ( 'NONE',  ( 6.923076923076924238, -3.050289026998446396, 32.03036669348365706 ) ) ;
#44784=FACE_OUTER_BOUND ( 'NONE', #26122, .T. ) ;
#44785=CARTESIAN_POINT ( 'NONE',  ( 3.360814393604009354, -2.504778602574659896, 29.97347330155780298 ) ) ;
#44786=CYLINDRICAL_SURFACE ( 'NONE', #295, 0.2499999999999986955 ) ;
#44787=B_SPLINE_CURVE_WITH_KNOTS ( 'NONE', 3,
 ( #73968, #79838, #37955, #59105, #52343, #45593, #38399, #51890, #52792, #32089 ),
 .UNSPECIFIED., .F., .F.,
 ( 4, 2, 2, 2, 4 ),
 ( 0.000000000000000000, 0.0001954339857564079894, 0.0003908679715128159787, 0.0005863019572692239681, 0.0007817359430256319575 ),
 .UNSPECIFIED. ) ;
#44789=B_SPLINE_CURVE_WITH_KNOTS ( 'NONE', 3,
 ( #49225, #29409, #63169, #2347, #28513, #14107, #76697, #55974, #28066, #20859 ),
 .UNSPECIFIED., .F., .F.,
 ( 4, 2, 2, 2, 4 ),
 ( 0.000000000000000000, 0.0001954339857564081520, 0.0003908679715128163040, 0.0005863019572692244018, 0.0007817359430256326080 ),
 .UNSPECIFIED. ) ;
#44790=EDGE_LOOP ( 'NONE', ( #1769, #40452 ) ) ;
#44791=CARTESIAN_POINT ( 'NONE',  ( 0.3962680155776847624, -12.46129190929999986, 30.37095296980880832 ) ) ;
#44792=VERTEX_POINT ( 'NONE', #24563 ) ;
#44793=ADVANCED_FACE ( 'NONE', ( #35545 ), #2950, .F. ) ;
#44794=ORIENTED_EDGE ( 'NONE', *, *, #29124, .F. ) ;
#44795=FACE_OUTER_BOUND ( 'NONE', #36330, .T. ) ;
#44796=EDGE_LOOP ( 'NONE', ( #19510, #39595, #1476, #16171 ) ) ;
#44797=CARTESIAN_POINT ( 'NONE',  ( 3.230769230769110045, -10.21337939537710326, 33.94971097300076224 ) ) ;
#44799=CARTESIAN_POINT ( 'NONE',  ( 3.007284306204901281, -2.353723527008296568, 30.78948104536958752 ) ) ;
#44800=EDGE_CURVE ( 'NONE', #77977, #59461, #6947, .T. ) ;
#44801=CARTESIAN_POINT ( 'NONE',  ( -5.076923076923075762, -2.721908614388771852, 31.22303859784724978 ) ) ;
#44803=CARTESIAN_POINT ( 'NONE',  ( -12.23875879256039312, -4.226511098958373402, 33.85474049983370293 ) ) ;
#44804=CARTESIAN_POINT ( 'NONE',  ( -16.37677311275300340, -10.01117774369187252, 34.36070679894347535 ) ) ;
#44805=CARTESIAN_POINT ( 'NONE',  ( 0.5267936010512993539, -5.941354392334606160, 34.76329471203374055 ) ) ;
#44806=CARTESIAN_POINT ( 'NONE',  ( -14.24162497434223162, -4.661471528628508665, 34.16647553114624003 ) ) ;
#44808=CARTESIAN_POINT ( 'NONE',  ( 18.22301284409340028, -11.43677907613345113, 33.22367315496201456 ) ) ;
#44809=CARTESIAN_POINT ( 'NONE',  ( -2.084912638714241151, -12.11081565061823717, 32.26097654155341843 ) ) ;
#44810=EDGE_CURVE ( 'NONE', #85360, #33072, #4883, .T. ) ;
#44812=DIRECTION ( 'NONE',  ( 0.000000000000000000, 0.000000000000000000, -1.000000000000000000 ) ) ;
#44813=EDGE_CURVE ( 'NONE', #41031, #3673, #13494, .T. ) ;
#44814=ORIENTED_EDGE ( 'NONE', *, *, #78394, .T. ) ;
#44815=ORIENTED_EDGE ( 'NONE', *, *, #66787, .T. ) ;
#44816=LINE ( 'NONE', #72296, #48593 ) ;
#44817=CARTESIAN_POINT ( 'NONE',  ( -14.17690049986752143, -8.147973898785416225, 34.70805048591653730 ) ) ;
#44819=CARTESIAN_POINT ( 'NONE',  ( 15.23076923076923173, -1.044019251281081972, 31.83374038241031911 ) ) ;
#44820=EDGE_CURVE ( 'NONE', #30159, #2090, #46659, .T. ) ;
#44821=FACE_OUTER_BOUND ( 'NONE', #33914, .T. ) ;
#44822=CARTESIAN_POINT ( 'NONE',  ( -3.099978789802280144, -5.496552790871119143, 34.60292014791297532 ) ) ;
#44823=ADVANCED_FACE ( 'NONE', ( #86744 ), #31329, .F. ) ;
#44824=ORIENTED_EDGE ( 'NONE', *, *, #27419, .T. ) ;
#44825=CARTESIAN_POINT ( 'NONE',  ( 18.00000000000000000, -12.37446782046654192, 30.86335684631486131 ) ) ;
#44826=EDGE_LOOP ( 'NONE', ( #25704, #43665, #19766, #35676 ) ) ;
#44828=EDGE_LOOP ( 'NONE', ( #73034, #40109, #80046, #10644 ) ) ;
#44830=CARTESIAN_POINT ( 'NONE',  ( 0.7115928814519140166, -12.41089969410671223, 31.60739465890703670 ) ) ;
#44831=CARTESIAN_POINT ( 'NONE',  ( -11.47320639894870276, -11.67786785259547777, 32.92929555188713664 ) ) ;
#44832=CARTESIAN_POINT ( 'NONE',  ( -14.30769230769230660, -2.833524468853757305, 32.15551576947925838 ) ) ;
#44834=CARTESIAN_POINT ( 'NONE',  ( 9.692307692307572609, -3.300289026999228881, 32.46337939537708905 ) ) ;
#44835=CARTESIAN_POINT ( 'NONE',  ( -2.307692307692427391, -11.94971097300221174, 32.03036669348237098 ) ) ;
#44836=VECTOR ( 'NONE', #45824, 1000.000000000000000 ) ;
#44838=ORIENTED_EDGE ( 'NONE', *, *, #67670, .F. ) ;
#44839=B_SPLINE_CURVE_WITH_KNOTS ( 'NONE', 3,
 ( #70046, #20530, #55198, #27726, #14667, #6579, #7471, #75045, #47994, #34046 ),
 .UNSPECIFIED., .F., .F.,
 ( 4, 2, 2, 2, 4 ),
 ( 0.000000000000000000, 0.0001954339857564081249, 0.0003908679715128162498, 0.0005863019572692244018, 0.0007817359430256324996 ),
 .UNSPECIFIED. ) ;
#44840=ORIENTED_EDGE ( 'NONE', *, *, #47063, .F. ) ;
#44841=CARTESIAN_POINT ( 'NONE',  ( 13.25446741488368829, -5.070767119584671079, 34.40440758774516183 ) ) ;
#44842=CARTESIAN_POINT ( 'NONE',  ( 9.692307692307570832, -2.379036618888197729, 30.90682066428292885 ) ) ;
#44843=EDGE_CURVE ( 'NONE', #81317, #36450, #42369, .T. ) ;
#44844=CARTESIAN_POINT ( 'NONE',  ( 4.153846153846154188, -12.78798330534102767, 29.49999999999997868 ) ) ;
#44845=CARTESIAN_POINT ( 'NONE',  ( -15.00775787915638304, -3.105924265160262543, 32.13625925475356127 ) ) ;
#44847=DIRECTION ( 'NONE',  ( 0.000000000000000000, 0.8660254037844377084, -0.5000000000000015543 ) ) ;
#44848=CARTESIAN_POINT ( 'NONE',  ( 4.153846153846154188, -12.09954503811598769, 35.62045528018868623 ) ) ;
#44849=ORIENTED_EDGE ( 'NONE', *, *, #53331, .T. ) ;
#44853=CARTESIAN_POINT ( 'NONE',  ( 15.48082354240754555, -5.728107161865378494, 34.42597550085002922 ) ) ;
#44856=B_SPLINE_CURVE_WITH_KNOTS ( 'NONE', 3,
 ( #81932, #54891, #5820, #81490, #14343, #20223, #19776, #35055, #13018, #89141 ),
 .UNSPECIFIED., .F., .F.,
 ( 4, 2, 2, 2, 4 ),
 ( 0.000000000000000000, 0.0001954311564186861968, 0.0003908623128373723936, 0.0005862934692560585904, 0.0007817246256747447872 ),
 .UNSPECIFIED. ) ;
#44857=CARTESIAN_POINT ( 'NONE',  ( -9.942330929600657896, -11.86270091957321249, 32.19358267280087915 ) ) ;
#44859=EDGE_CURVE ( 'NONE', #67881, #9159, #9020, .T. ) ;
#44861=ORIENTED_EDGE ( 'NONE', *, *, #79878, .F. ) ;
#44862=CARTESIAN_POINT ( 'NONE',  ( -39.05038313613820122, -2.249999999999998668, 29.75000000000000355 ) ) ;
#44863=VERTEX_POINT ( 'NONE', #33559 ) ;
#44864=EDGE_CURVE ( 'NONE', #3680, #37287, #4755, .T. ) ;
#44865=DIRECTION ( 'NONE',  ( -0.000000000000000000, -0.8660254037844397068, -0.4999999999999978906 ) ) ;
#44866=CARTESIAN_POINT ( 'NONE',  ( -6.989160334032804123, -2.721908614388772740, 31.22303859784724622 ) ) ;
#44867=CARTESIAN_POINT ( 'NONE',  ( -12.46153846153846168, -12.37446782046654192, 30.86335684631486131 ) ) ;
#44868=CARTESIAN_POINT ( 'NONE',  ( -15.23076923076922995, -13.37000171582298513, 34.34916445242398453 ) ) ;
#44869=CARTESIAN_POINT ( 'NONE',  ( 4.153846153846154188, -3.669653830205710676, 35.88435417666054406 ) ) ;
#44870=EDGE_CURVE ( 'NONE', #20057, #63601, #44392, .T. ) ;
#44871=CARTESIAN_POINT ( 'NONE',  ( -0.5276208408985981757, -12.34228464037088280, 31.77849191805838558 ) ) ;
#44872=CARTESIAN_POINT ( 'NONE',  ( -3.453696189676077832, -8.282780595021769443, 34.94152052738834868 ) ) ;
#44873=VERTEX_POINT ( 'NONE', #32224 ) ;
#44874=CARTESIAN_POINT ( 'NONE',  ( -10.74607608205217346, -9.804603061927743113, 34.18744698557895845 ) ) ;
#44876=VERTEX_POINT ( 'NONE', #74099 ) ;
#44877=EDGE_CURVE ( 'NONE', #52424, #42644, #4719, .T. ) ;
#44879=CARTESIAN_POINT ( 'NONE',  ( 14.30769230769218758, -10.21337939537710326, 33.94971097300076224 ) ) ;
#44881=DIRECTION ( 'NONE',  ( 0.000000000000000000, 0.9396926207859126468, 0.3420201433256571111 ) ) ;
#44883=CARTESIAN_POINT ( 'NONE',  ( 7.846153846153725020, -8.613356846316285953, 34.62446782046622218 ) ) ;
#44884=FACE_BOUND ( 'NONE', #41760, .T. ) ;
#44885=CARTESIAN_POINT ( 'NONE',  ( 13.13463865367303463, -12.17611988154120972, 31.52148481390971213 ) ) ;
#44886=DIRECTION ( 'NONE',  ( -0.000000000000000000, -0.1736481776669307198, -0.9848077530122080203 ) ) ;
#44887=FACE_OUTER_BOUND ( 'NONE', #36436, .T. ) ;
#44888=CARTESIAN_POINT ( 'NONE',  ( 3.100622021331010725, -4.460286881179643004, 33.72017969459903242 ) ) ;
#44889=DIRECTION ( 'NONE',  ( 1.000000000000000000, 0.000000000000000000, 0.000000000000000000 ) ) ;
#44890=DIRECTION ( 'NONE',  ( -0.000000000000000000, 0.9396926207859092051, -0.3420201433256662704 ) ) ;
#44891=CARTESIAN_POINT ( 'NONE',  ( 11.53846153846153832, -12.78798330534102767, 29.49999999999997868 ) ) ;
#44893=AXIS2_PLACEMENT_3D ( 'NONE', #30928, #73264, #39050 ) ;
#44896=DIRECTION ( 'NONE',  ( -0.000000000000000000, 0.8660254037844397068, -0.4999999999999978906 ) ) ;
#44897=CARTESIAN_POINT ( 'NONE',  ( 7.911408985666682270, -10.33852847137154107, 34.16647553114620450 ) ) ;
#44899=CARTESIAN_POINT ( 'NONE',  ( 17.01084069756293715, -8.164416787775445883, 34.95778746994557906 ) ) ;
#44901=CARTESIAN_POINT ( 'NONE',  ( 5.142178216435913107, -12.16647553114626490, 32.15551576947920864 ) ) ;
#44904=AXIS2_PLACEMENT_3D ( 'NONE', #78955, #86174, #71301 ) ;
#44905=CARTESIAN_POINT ( 'NONE',  ( -16.15384615384615330, -5.471508081941601098, 34.59228464037088457 ) ) ;
#44906=CARTESIAN_POINT ( 'NONE',  ( 0.5267940328144861128, -3.835265460703683349, 33.15142922261929925 ) ) ;
#44907=CARTESIAN_POINT ( 'NONE',  ( 11.31558202172395511, -7.630690623152299956, 34.99857592706774057 ) ) ;
#44908=CARTESIAN_POINT ( 'NONE',  ( -0.4615384615384611200, -8.164416787775445883, 34.95778746994557906 ) ) ;
#44909=CARTESIAN_POINT ( 'NONE',  ( 7.053868730901711182, -4.118422570099827595, 33.43335022499816489 ) ) ;
#44910=FACE_OUTER_BOUND ( 'NONE', #54858, .T. ) ;
#44911=CARTESIAN_POINT ( 'NONE',  ( 4.153846153846032507, -4.481592998941358097, 33.73612834414048933 ) ) ;
#44912=CARTESIAN_POINT ( 'NONE',  ( 17.20744851515672025, -8.630441415882549094, 34.87705825610312615 ) ) ;
#44913=ORIENTED_EDGE ( 'NONE', *, *, #45952, .F. ) ;
#44914=B_SPLINE_CURVE_WITH_KNOTS ( 'NONE', 3,
 ( #67371, #61487, #88993, #26385, #6116, #51915, #11390, #73553, #66335, #86628 ),
 .UNSPECIFIED., .F., .F.,
 ( 4, 2, 2, 2, 4 ),
 ( 0.0007817359430256328248, 0.0009771253907249995759, 0.001172514838424366327, 0.001367904286123733078, 0.001563293733823099829 ),
 .UNSPECIFIED. ) ;
#44915=CARTESIAN_POINT ( 'NONE',  ( 1.634615384616822320, -7.500000000000155431, 34.75000000000007105 ) ) ;
#44916=CARTESIAN_POINT ( 'NONE',  ( -17.14300648787895298, -2.721908614388770964, 31.22303859784723912 ) ) ;
#44918=CARTESIAN_POINT ( 'NONE',  ( -10.86540783960607293, -10.18141759479407327, 34.26406193332782379 ) ) ;
#44919=CARTESIAN_POINT ( 'NONE',  ( 1.384615384615265343, -9.442884908241554243, 34.35708131394783038 ) ) ;
#44920=ORIENTED_EDGE ( 'NONE', *, *, #31804, .F. ) ;
#44921=CARTESIAN_POINT ( 'NONE',  ( -17.77722033102192967, -6.717445702608402236, 34.94155399931962336 ) ) ;
#44922=CARTESIAN_POINT ( 'NONE',  ( 1.384615384615264011, -2.657715359629662544, 31.77849191805970364 ) ) ;
#44923=CARTESIAN_POINT ( 'NONE',  ( -7.596208436775802930, -12.45601412856602686, 31.48342859153981621 ) ) ;
#44924=VERTEX_POINT ( 'NONE', #6083 ) ;
#44925=CARTESIAN_POINT ( 'NONE',  ( -11.28846153846153655, -2.499999999999998668, 29.75000000000000355 ) ) ;
#44926=CARTESIAN_POINT ( 'NONE',  ( 16.85404356018549521, -7.630690623152299956, 34.99857592706774057 ) ) ;
#44927=CARTESIAN_POINT ( 'NONE',  ( -7.846153846153844924, -12.34228464037088635, 31.77849191805839268 ) ) ;
#44928=CARTESIAN_POINT ( 'NONE',  ( 6.000000000000001776, -3.886160181151819604, 36.00935417666054406 ) ) ;
#44931=FACE_OUTER_BOUND ( 'NONE', #88381, .T. ) ;
#44932=EDGE_CURVE ( 'NONE', #50951, #26741, #26790, .T. ) ;
#44933=DIRECTION ( 'NONE',  ( -1.000000000000000000, 0.000000000000000000, 0.000000000000000000 ) ) ;
#44935=ORIENTED_EDGE ( 'NONE', *, *, #68089, .T. ) ;
#44936=ADVANCED_FACE ( 'NONE', ( #13275 ), #40760, .F. ) ;
#44937=EDGE_LOOP ( 'NONE', ( #14440, #21853 ) ) ;
#44938=CARTESIAN_POINT ( 'NONE',  ( -10.61538461538461320, -11.16473453929635440, 33.15142922261926373 ) ) ;
#44939=CARTESIAN_POINT ( 'NONE',  ( -3.007989561791165389, -3.020022701398814124, 32.48759521482552515 ) ) ;
#44940=EDGE_CURVE ( 'NONE', #12084, #82763, #86406, .T. ) ;
#44941=CARTESIAN_POINT ( 'NONE',  ( -9.561517251340744039, -12.62708834333097663, 30.88030960425257021 ) ) ;
#44942=EDGE_CURVE ( 'NONE', #16715, #53257, #77191, .T. ) ;
#44943=CARTESIAN_POINT ( 'NONE',  ( -10.61538461538461320, -3.050289026998446396, 32.03036669348365706 ) ) ;
#44944=VERTEX_POINT ( 'NONE', #61897 ) ;
#44945=B_SPLINE_CURVE_WITH_KNOTS ( 'NONE', 3,
 ( #55543, #8702, #83926, #2359, #29853, #21311, #22207, #8258, #57317, #42931 ),
 .UNSPECIFIED., .F., .F.,
 ( 4, 2, 2, 2, 4 ),
 ( 0.000000000000000000, 0.0001954311564186863052, 0.0003908623128373726104, 0.0005862934692560589156, 0.0007817246256747452209 ),
 .UNSPECIFIED. ) ;
#44946=ORIENTED_EDGE ( 'NONE', *, *, #22796, .T. ) ;
#44947=CARTESIAN_POINT ( 'NONE',  ( 11.76124120743959978, -11.60474049983371003, 33.02348890104160262 ) ) ;
#44948=ORIENTED_EDGE ( 'NONE', *, *, #33134, .T. ) ;
#44949=CARTESIAN_POINT ( 'NONE',  ( 6.700210660013824260, -2.251424796025575770, 29.88072029997477586 ) ) ;
#44950=EDGE_CURVE ( 'NONE', #6564, #71441, #83075, .T. ) ;
#44952=VECTOR ( 'NONE', #37940, 999.9999999999998863 ) ;
#44953=DIRECTION ( 'NONE',  ( 0.000000000000000000, 0.7660444431189822323, -0.6427876096865344779 ) ) ;
#44954=CARTESIAN_POINT ( 'NONE',  ( -1.254089946381738319, -12.70449254468099198, 30.44128974285582956 ) ) ;
#44955=ORIENTED_EDGE ( 'NONE', *, *, #54830, .F. ) ;
#44956=VERTEX_POINT ( 'NONE', #83524 ) ;
#44957=ORIENTED_EDGE ( 'NONE', *, *, #88896, .T. ) ;
#44958=CARTESIAN_POINT ( 'NONE',  ( 15.10062202133101295, -2.619462340734462380, 30.83744416345203021 ) ) ;
#44959=ORIENTED_EDGE ( 'NONE', *, *, #84784, .F. ) ;
#44960=CARTESIAN_POINT ( 'NONE',  ( -10.61538461538473577, -5.941354392335915335, 34.76329471203413846 ) ) ;
#44961=CARTESIAN_POINT ( 'NONE',  ( 18.13052543823364360, -5.915461855592777596, 34.75538340440931506 ) ) ;
#44962=ORIENTED_EDGE ( 'NONE', *, *, #20076, .T. ) ;
#44963=CARTESIAN_POINT ( 'NONE',  ( -13.44988583057615905, -4.481592998940162609, 33.73612834413957984 ) ) ;
#44964=FACE_OUTER_BOUND ( 'NONE', #34457, .T. ) ;
#44965=CARTESIAN_POINT ( 'NONE',  ( 8.769230769230768274, -5.557115091759785130, 34.35708131394839171 ) ) ;
#44966=FACE_BOUND ( 'NONE', #53564, .T. ) ;
#44967=ADVANCED_FACE ( 'NONE', ( #209 ), #1539, .F. ) ;
#44968=CARTESIAN_POINT ( 'NONE',  ( -5.142193077479396024, -10.33852847137145048, 34.16647553114627556 ) ) ;
#44969=CARTESIAN_POINT ( 'NONE',  ( -4.377331097570102969, -12.24155766932282496, 31.33739205006857986 ) ) ;
#44970=CARTESIAN_POINT ( 'NONE',  ( -15.23076923076922995, -10.51840700105979565, 33.73612834413961536 ) ) ;
#44971=CARTESIAN_POINT ( 'NONE',  ( 16.28437159207980045, -4.299079248970731015, 33.91157788607253565 ) ) ;
#44973=CARTESIAN_POINT ( 'NONE',  ( 5.076923076922954969, -12.27809138561165270, 31.22303859784587132 ) ) ;
#44974=CARTESIAN_POINT ( 'NONE',  ( 1.634560793993430128, -2.341251567377310217, 30.72681386836322659 ) ) ;
#44975=ORIENTED_EDGE ( 'NONE', *, *, #44164, .F. ) ;
#44976=CARTESIAN_POINT ( 'NONE',  ( -9.692307692307691624, -1.129524287112498415, 32.06866353760679544 ) ) ;
#44977=CARTESIAN_POINT ( 'NONE',  ( -7.715628144390286103, -2.619367082507848554, 30.83698974864644171 ) ) ;
#44978=ORIENTED_EDGE ( 'NONE', *, *, #20140, .F. ) ;
#44979=B_SPLINE_CURVE_WITH_KNOTS ( 'NONE', 3,
 ( #66475, #4778, #59710, #87208, #56828, #57276, #29814, #76669, #84326, #50068 ),
 .UNSPECIFIED., .F., .F.,
 ( 4, 2, 2, 2, 4 ),
 ( 0.0007817359430256394385, 0.0009771253907250078159, 0.001172514838424376085, 0.001367904286123744571, 0.001563293733823112840 ),
 .UNSPECIFIED. ) ;
#44980=VERTEX_POINT ( 'NONE', #21805 ) ;
#44981=DIRECTION ( 'NONE',  ( -0.000000000000000000, -0.6427876096865404731, -0.7660444431189770143 ) ) ;
#44982=CARTESIAN_POINT ( 'NONE',  ( 10.86533002476265963, -12.68172785388650681, 30.59649109432439218 ) ) ;
#44983=EDGE_CURVE ( 'NONE', #86342, #76471, #58447, .T. ) ;
#44984=AXIS2_PLACEMENT_3D ( 'NONE', #55693, #70099, #21918 ) ;
#44985=CARTESIAN_POINT ( 'NONE',  ( -5.750054481651856619, -6.696923467548660192, 34.68552623307873972 ) ) ;
#44986=CARTESIAN_POINT ( 'NONE',  ( -10.61538461538473577, -5.094484230521993062, 34.41647553114689373 ) ) ;
#44987=CARTESIAN_POINT ( 'NONE',  ( -11.60454391782167427, -9.905515769479276145, 34.41647553114623292 ) ) ;
#44988=EDGE_LOOP ( 'NONE', ( #27907, #2658, #38008, #81237, #594, #18914 ) ) ;
#44989=DIRECTION ( 'NONE',  ( -0.000000000000000000, -0.7660444431189791237, -0.6427876096865379196 ) ) ;
#44992=CARTESIAN_POINT ( 'NONE',  ( -3.230769230769229949, -1.790695186598648903, 34.54067556320373455 ) ) ;
#44993=CARTESIAN_POINT ( 'NONE',  ( 7.596177115211492747, -5.728515186090277211, 34.42611988154120439 ) ) ;
#44994=LINE ( 'NONE', #64373, #12244 ) ;
#44995=LINE ( 'NONE', #72475, #85162 ) ;
#44997=ORIENTED_EDGE ( 'NONE', *, *, #10164, .T. ) ;
#44998=ORIENTED_EDGE ( 'NONE', *, *, #86161, .T. ) ;
#44999=CARTESIAN_POINT ( 'NONE',  ( -7.596153846153844924, -2.249999999999998668, 29.75000000000000355 ) ) ;
#45000=DIRECTION ( 'NONE',  ( -0.000000000000000000, 1.000000000000000000, -0.000000000000000000 ) ) ;
#45001=DIRECTION ( 'NONE',  ( 0.000000000000000000, 0.9396926207859126468, -0.3420201433256571111 ) ) ;
#45002=FACE_OUTER_BOUND ( 'NONE', #43536, .T. ) ;
#45003=CARTESIAN_POINT ( 'NONE',  ( 0.4615384615384611200, -13.87047571288749737, 32.06866353760679544 ) ) ;
#45005=EDGE_CURVE ( 'NONE', #40289, #4801, #57348, .T. ) ;
#45007=CARTESIAN_POINT ( 'NONE',  ( -13.38461538461538325, -13.53365097954675988, 30.81389545987213552 ) ) ;
#45008=ORIENTED_EDGE ( 'NONE', *, *, #60326, .F. ) ;
#45009=DIRECTION ( 'NONE',  ( -0.000000000000000000, 1.000000000000000000, 3.491481338843133355E-15 ) ) ;
#45010=CARTESIAN_POINT ( 'NONE',  ( -6.249999999999997335, -2.249999999999998668, 29.75000000000000355 ) ) ;
#45011=ORIENTED_EDGE ( 'NONE', *, *, #55538, .F. ) ;
#45012=CARTESIAN_POINT ( 'NONE',  ( -9.942307692307691624, -7.500000000000001776, 35.00000000000000000 ) ) ;
#45013=FACE_OUTER_BOUND ( 'NONE', #69388, .T. ) ;
#45014=EDGE_CURVE ( 'NONE', #66369, #22022, #85273, .T. ) ;
#45015=EDGE_CURVE ( 'NONE', #37045, #80537, #38052, .T. ) ;
#45016=CARTESIAN_POINT ( 'NONE',  ( -3.296526033283539991, -7.249945686854185389, 34.74374336980224598 ) ) ;
#45017=CARTESIAN_POINT ( 'NONE',  ( 7.053602361310569613, -2.372941743896878286, 30.88044141588254377 ) ) ;
#45018=LINE ( 'NONE', #72497, #33553 ) ;
#45019=CARTESIAN_POINT ( 'NONE',  ( 9.469380733400843297, -4.762599654559228846, 34.23009711892697737 ) ) ;
#45020=LINE ( 'NONE', #43265, #62875 ) ;
#45021=ORIENTED_EDGE ( 'NONE', *, *, #54483, .T. ) ;
#45022=EDGE_CURVE ( 'NONE', #43002, #57014, #48724, .T. ) ;
#45023=CARTESIAN_POINT ( 'NONE',  ( 11.60452988946397923, -11.69971097300155272, 32.46337939537588113 ) ) ;
#45024=CARTESIAN_POINT ( 'NONE',  ( -13.31936024510254590, -10.33852847137154107, 34.16647553114620450 ) ) ;
#45025=CARTESIAN_POINT ( 'NONE',  ( -18.00000000000000000, -1.163064389776900187, 32.05645593858272235 ) ) ;
#45028=DIRECTION ( 'NONE',  ( 0.000000000000000000, -1.000000000000000000, 0.000000000000000000 ) ) ;
#45029=FILL_AREA_STYLE_COLOUR ( '', #68183 ) ;
#45030=CARTESIAN_POINT ( 'NONE',  ( 12.21151522424549896, -10.76384336483936011, 33.53834819971076087 ) ) ;
#45031=VERTEX_POINT ( 'NONE', #37523 ) ;
#45033=CARTESIAN_POINT ( 'NONE',  ( -15.45369618967607828, -4.026226216239094491, 33.68668979543634379 ) ) ;
#45034=AXIS2_PLACEMENT_3D ( 'NONE', #74432, #59579, #32551 ) ;
#45035=ORIENTED_EDGE ( 'NONE', *, *, #25126, .T. ) ;
#45037=ORIENTED_EDGE ( 'NONE', *, *, #13168, .T. ) ;
#45038=DIRECTION ( 'NONE',  ( 0.000000000000000000, 0.1736481776669275834, 0.9848077530122086864 ) ) ;
#45039=CARTESIAN_POINT ( 'NONE',  ( -15.45369618967607828, -2.889293201056495786, 32.26117774369186009 ) ) ;
#45040=CARTESIAN_POINT ( 'NONE',  ( 16.85343815235874132, -6.716662450894490988, 34.94144148231605840 ) ) ;
#45041=ORIENTED_EDGE ( 'NONE', *, *, #28322, .T. ) ;
#45043=ORIENTED_EDGE ( 'NONE', *, *, #4714, .F. ) ;
#45044=CARTESIAN_POINT ( 'NONE',  ( -5.869474561766354626, -2.372941743896878286, 30.88044141588254377 ) ) ;
#45045=ADVANCED_FACE ( 'NONE', ( #72196 ), #38426, .F. ) ;
#45046=ORIENTED_EDGE ( 'NONE', *, *, #79140, .F. ) ;
#45047=CARTESIAN_POINT ( 'NONE',  ( 13.60739492588379385, -11.89424750095246175, 32.13594075562310337 ) ) ;
#45048=FACE_OUTER_BOUND ( 'NONE', #4617, .T. ) ;
#45049=VERTEX_POINT ( 'NONE', #51018 ) ;
#45050=B_SPLINE_CURVE_WITH_KNOTS ( 'NONE', 3,
 ( #35804, #69574, #9219, #28600, #71340, #36683, #83553, #64133, #2436, #49307 ),
 .UNSPECIFIED., .F., .F.,
 ( 4, 2, 2, 2, 4 ),
 ( 0.000000000000000000, 0.0001954311564186879315, 0.0003908623128373758630, 0.0005862934692560637946, 0.0007817246256747517261 ),
 .UNSPECIFIED. ) ;
#45052=LINE ( 'NONE', #78398, #40682 ) ;
#45053=B_SPLINE_CURVE_WITH_KNOTS ( 'NONE', 3,
 ( #25382, #31246, #71337, #58267, #85759, #24037, #10986, #38455, #51490, #64568 ),
 .UNSPECIFIED., .F., .F.,
 ( 4, 2, 2, 2, 4 ),
 ( 0.0007817246256747519429, 0.0009771112852218970073, 0.001172497944769042288, 0.001367884604316187353, 0.001563271263863332417 ),
 .UNSPECIFIED. ) ;
#45054=DIRECTION ( 'NONE',  ( 0.000000000000000000, 0.000000000000000000, 1.000000000000000000 ) ) ;
#45055=B_SPLINE_CURVE_WITH_KNOTS ( 'NONE', 3,
 ( #42428, #30234, #76650, #77531, #29796, #22584, #63566, #37418, #63119, #43307 ),
 .UNSPECIFIED., .F., .F.,
 ( 4, 2, 2, 2, 4 ),
 ( 0.000000000000000000, 0.0001954339857564081249, 0.0003908679715128162498, 0.0005863019572692244018, 0.0007817359430256324996 ),
 .UNSPECIFIED. ) ;
#45056=AXIS2_PLACEMENT_3D ( 'NONE', #37218, #78209, #43100 ) ;
#45057=EDGE_CURVE ( 'NONE', #17031, #27837, #86180, .T. ) ;
#45058=VECTOR ( 'NONE', #51927, 1000.000000000000227 ) ;
#45059=FACE_OUTER_BOUND ( 'NONE', #69910, .T. ) ;
#45060=CARTESIAN_POINT ( 'NONE',  ( -11.47239420511146157, -3.322132147404559976, 32.92929555188717927 ) ) ;
#45061=VERTEX_POINT ( 'NONE', #10953 ) ;
#45063=VERTEX_POINT ( 'NONE', #10055 ) ;
#45064=CARTESIAN_POINT ( 'NONE',  ( 15.36156103859401867, -2.541949514083464479, 30.39797389878540557 ) ) ;
#45066=EDGE_CURVE ( 'NONE', #4986, #85950, #83198, .T. ) ;
#45067=LINE ( 'NONE', #13510, #86733 ) ;
#45068=CARTESIAN_POINT ( 'NONE',  ( -10.83831083290076158, -9.086856451489515152, 34.49173150075333183 ) ) ;
#45070=ORIENTED_EDGE ( 'NONE', *, *, #76162, .T. ) ;
#45072=ORIENTED_EDGE ( 'NONE', *, *, #55704, .T. ) ;
#45073=CARTESIAN_POINT ( 'NONE',  ( 0.2115617174898693220, -8.347322224742351082, 34.93158281831414769 ) ) ;
#45074=ORIENTED_EDGE ( 'NONE', *, *, #69093, .F. ) ;
#45075=CARTESIAN_POINT ( 'NONE',  ( 16.02315468717859304, -9.804603061927743113, 34.18744698557895845 ) ) ;
#45076=AXIS2_PLACEMENT_3D ( 'NONE', #49726, #70450, #29032 ) ;
#45077=CARTESIAN_POINT ( 'NONE',  ( -8.096130577096198877, -2.564618984488975073, 30.55390908950641915 ) ) ;
#45078=B_SPLINE_CURVE_WITH_KNOTS ( 'NONE', 3,
 ( #83769, #37324, #49077, #30571, #71113, #76559, #30138, #14867, #77004, #77874 ),
 .UNSPECIFIED., .F., .F.,
 ( 4, 2, 2, 2, 4 ),
 ( 0.000000000000000000, 0.0001954311564186861968, 0.0003908623128373723936, 0.0005862934692560585904, 0.0007817246256747447872 ),
 .UNSPECIFIED. ) ;
#45080=FACE_BOUND ( 'NONE', #6190, .T. ) ;
#45081=ORIENTED_EDGE ( 'NONE', *, *, #82770, .T. ) ;
#45083=CARTESIAN_POINT ( 'NONE',  ( 3.230769230769231726, -7.500000000000001776, 35.04278698407183867 ) ) ;
#45084=CARTESIAN_POINT ( 'NONE',  ( 13.16168842570853670, -10.77366814457252175, 33.85459836347579454 ) ) ;
#45085=VECTOR ( 'NONE', #36886, 999.9999999999998863 ) ;
#45086=CARTESIAN_POINT ( 'NONE',  ( 14.30769230769231015, -6.435427911321262684, 35.78748833219616898 ) ) ;
#45087=CARTESIAN_POINT ( 'NONE',  ( 2.084765348785460048, -8.282780595021769443, 34.94152052738834868 ) ) ;
#45088=CARTESIAN_POINT ( 'NONE',  ( -14.30769230769230660, -2.900454961884010974, 35.62045528018868623 ) ) ;
#45090=EDGE_CURVE ( 'NONE', #27014, #63342, #54143, .T. ) ;
#45091=CARTESIAN_POINT ( 'NONE',  ( -2.084680956079455250, -9.086983370893047862, 34.49168942202179267 ) ) ;
#45092=ORIENTED_EDGE ( 'NONE', *, *, #40882, .F. ) ;
#45093=EDGE_CURVE ( 'NONE', #67353, #50385, #65958, .T. ) ;
#45094=VERTEX_POINT ( 'NONE', #22688 ) ;
#45095=CARTESIAN_POINT ( 'NONE',  ( 1.384615384615386802, -2.721908614388771852, 31.22303859784724978 ) ) ;
#45096=DIRECTION ( 'NONE',  ( -0.000000000000000000, -0.3420201433256694901, -0.9396926207859082059 ) ) ;
#45097=CARTESIAN_POINT ( 'NONE',  ( 16.15384615384603251, -11.67786785259630911, 32.92929555188603530 ) ) ;
#45098=CARTESIAN_POINT ( 'NONE',  ( 18.00000000000000000, -2.517432740324522911, 35.29906147534542527 ) ) ;
#45099=CARTESIAN_POINT ( 'NONE',  ( 1.607626736228236375, -9.886259254753564818, 34.14407573483972413 ) ) ;
#45100=LINE ( 'NONE', #23934, #56158 ) ;
#45101=ORIENTED_EDGE ( 'NONE', *, *, #27115, .T. ) ;
#45102=CARTESIAN_POINT ( 'NONE',  ( -5.076923076923075762, -6.343179335718451384, 34.87096338111211935 ) ) ;
#45103=EDGE_CURVE ( 'NONE', #52344, #50406, #67095, .T. ) ;
#45104=CARTESIAN_POINT ( 'NONE',  ( 3.007842271862380290, -9.172386477786396597, 34.72672124145550043 ) ) ;
#45105=CARTESIAN_POINT ( 'NONE',  ( 2.373759641042385127, -12.62096338111211757, 30.90682066428152908 ) ) ;
#45106=CARTESIAN_POINT ( 'NONE',  ( 14.43848274865926129, -2.494656445102012565, 31.33466734024120015 ) ) ;
#45107=ORIENTED_EDGE ( 'NONE', *, *, #85566, .T. ) ;
#45108=B_SPLINE_CURVE_WITH_KNOTS ( 'NONE', 3,
 ( #4392, #31876, #59333, #86841, #75082, #21001, #53912, #48472, #6175, #62425 ),
 .UNSPECIFIED., .F., .F.,
 ( 4, 2, 2, 2, 4 ),
 ( 0.0007817246256747481482, 0.0009771112852218911526, 0.001172497944769034049, 0.001367884604316176944, 0.001563271263863319840 ),
 .UNSPECIFIED. ) ;
#45109=EDGE_LOOP ( 'NONE', ( #77214, #49632 ) ) ;
#45110=FACE_BOUND ( 'NONE', #20028, .T. ) ;
#45111=ORIENTED_EDGE ( 'NONE', *, *, #21764, .F. ) ;
#45112=DIRECTION ( 'NONE',  ( -0.000000000000000000, -0.5000000000000009992, -0.8660254037844380415 ) ) ;
#45113=CARTESIAN_POINT ( 'NONE',  ( -5.749999999999936051, -7.434744860731433924, 35.00000000000000711 ) ) ;
#45115=DIRECTION ( 'NONE',  ( 0.000000000000000000, 1.000000000000000000, 0.000000000000000000 ) ) ;
#45116=CYLINDRICAL_SURFACE ( 'NONE', #31327, 0.2500000000000012212 ) ;
#45117=CARTESIAN_POINT ( 'NONE',  ( -8.069638789877792817, -11.89387501736622710, 32.13663884655806413 ) ) ;
#45122=CARTESIAN_POINT ( 'NONE',  ( 17.07692307692307665, -10.51840700105979565, 33.73612834413961536 ) ) ;
#45123=ORIENTED_EDGE ( 'NONE', *, *, #11046, .T. ) ;
#45124=CARTESIAN_POINT ( 'NONE',  ( 15.23076923076911093, -8.613356846316285953, 34.62446782046622218 ) ) ;
#45125=CARTESIAN_POINT ( 'NONE',  ( -12.68502338610279523, -3.019605429927184836, 32.48692288466676814 ) ) ;
#45126=DIRECTION ( 'NONE',  ( -0.000000000000000000, 0.3420201433256694901, -0.9396926207859082059 ) ) ;
#45127=EDGE_CURVE ( 'NONE', #34142, #683, #12282, .T. ) ;
#45128=CARTESIAN_POINT ( 'NONE',  ( 15.48082354240754555, -12.41262288849542017, 30.68299917996395010 ) ) ;
#45129=CARTESIAN_POINT ( 'NONE',  ( -7.976845312821404299, -8.999036380462717588, 34.52022231692819076 ) ) ;
#45130=B_SPLINE_CURVE_WITH_KNOTS ( 'NONE', 3,
 ( #67831, #81797, #34040, #13766, #14214, #41250, #81355, #47100, #69162, #12442 ),
 .UNSPECIFIED., .F., .F.,
 ( 4, 2, 2, 2, 4 ),
 ( 0.0007817246256747471724, 0.0009771112852218905021, 0.001172497944769033615, 0.001367884604316176944, 0.001563271263863320274 ),
 .UNSPECIFIED. ) ;
#45131=CARTESIAN_POINT ( 'NONE',  ( 5.076923076922954969, -12.46129190930018460, 30.37095296980731973 ) ) ;
#45133=ORIENTED_EDGE ( 'NONE', *, *, #81970, .F. ) ;
#45134=B_SPLINE_CURVE_WITH_KNOTS ( 'NONE', 3,
 ( #56229, #8048, #49474, #42723, #35517, #41838, #14809, #75603, #70183, #42285 ),
 .UNSPECIFIED., .F., .F.,
 ( 4, 2, 2, 2, 4 ),
 ( 0.000000000000000000, 0.0001954339857564092362, 0.0003908679715128184724, 0.0005863019572692276544, 0.0007817359430256369448 ),
 .UNSPECIFIED. ) ;
#45135=CARTESIAN_POINT ( 'NONE',  ( -3.296039676730006196, -3.300289026998414865, 32.46337939537583139 ) ) ;
#45137=CARTESIAN_POINT ( 'NONE',  ( 6.130045162834781181, -2.504778602574660340, 29.97347330155780298 ) ) ;
#45139=VERTEX_POINT ( 'NONE', #39326 ) ;
#45141=CARTESIAN_POINT ( 'NONE',  ( -7.596099426240391139, -5.642605341092958859, 34.66089969410670335 ) ) ;
#45142=CARTESIAN_POINT ( 'NONE',  ( -0.2115384615384616196, -2.499999999999998668, 29.75000000000000355 ) ) ;
#45143=DIRECTION ( 'NONE',  ( 0.000000000000000000, 0.3420201433256641055, -0.9396926207859100932 ) ) ;
#45144=CARTESIAN_POINT ( 'NONE',  ( 10.61538461538461675, -4.098570777380720287, 33.41473453929634729 ) ) ;
#45145=CARTESIAN_POINT ( 'NONE',  ( -8.899377978668988831, -11.93770438780619259, 32.05411857736982029 ) ) ;
#45146=CARTESIAN_POINT ( 'NONE',  ( -15.16470189741915675, -8.164416787775445883, 34.95778746994558617 ) ) ;
#45147=ORIENTED_EDGE ( 'NONE', *, *, #80851, .F. ) ;
#45148=CYLINDRICAL_SURFACE ( 'NONE', #72198, 0.2499999999999979738 ) ;
#45149=CARTESIAN_POINT ( 'NONE',  ( -0.3307466537136752871, -8.147973898785416225, 34.70805048591653730 ) ) ;
#45151=CARTESIAN_POINT ( 'NONE',  ( -6.249999999999997335, -7.500000000000001776, 34.75000000000000000 ) ) ;
#45152=CARTESIAN_POINT ( 'NONE',  ( 9.692307692307570832, -2.657715359629662544, 31.77849191805970364 ) ) ;
#45153=EDGE_LOOP ( 'NONE', ( #40667, #37336 ) ) ;
#45154=CARTESIAN_POINT ( 'NONE',  ( 13.45068373561782593, -6.386643153685127139, 34.62446782046654192 ) ) ;
#45156=VECTOR ( 'NONE', #8887, 1000.000000000000000 ) ;
#45157=ORIENTED_EDGE ( 'NONE', *, *, #10334, .T. ) ;
#45158=CYLINDRICAL_SURFACE ( 'NONE', #52903, 0.2500000000000004996 ) ;
#45159=CARTESIAN_POINT ( 'NONE',  ( -1.515306851282941958, -8.999036380462717588, 34.52022231692819076 ) ) ;
#45160=CARTESIAN_POINT ( 'NONE',  ( 6.223012844093396723, -11.98016756924215009, 32.48728574198911190 ) ) ;
#45161=ORIENTED_EDGE ( 'NONE', *, *, #85298, .T. ) ;
#45162=CARTESIAN_POINT ( 'NONE',  ( 3.230769230769108269, -12.70778746994576025, 30.41441678777401236 ) ) ;
#45163=DIRECTION ( 'NONE',  ( -0.000000000000000000, -0.3420201433256694346, -0.9396926207859080948 ) ) ;
#45164=CARTESIAN_POINT ( 'NONE',  ( 10.61538461538461675, -3.513871655860378418, 32.76840700105978499 ) ) ;
#45165=DIRECTION ( 'NONE',  ( -0.000000000000000000, -0.6427876096865404731, -0.7660444431189771253 ) ) ;
#45167=B_SPLINE_CURVE_WITH_KNOTS ( 'NONE', 3,
 ( #72285, #10598, #73188, #18695, #32208, #24542, #78599, #38065, #44354, #46162 ),
 .UNSPECIFIED., .F., .F.,
 ( 4, 2, 2, 2, 4 ),
 ( 0.0007817246256747452209, 0.0009771112852218879000, 0.001172497944769030579, 0.001367884604316173258, 0.001563271263863315937 ),
 .UNSPECIFIED. ) ;
#45169=CARTESIAN_POINT ( 'NONE',  ( -0.6850234052624101233, -8.496056993536548418, 34.65000542017679663 ) ) ;
#45170=EDGE_LOOP ( 'NONE', ( #53720, #24378, #48216, #77919 ) ) ;
#45172=CYLINDRICAL_SURFACE ( 'NONE', #17523, 0.2500000000000008882 ) ;
#45173=CARTESIAN_POINT ( 'NONE',  ( -13.60810032833933114, -2.847400154188067578, 31.58180166144859058 ) ) ;
#45174=CARTESIAN_POINT ( 'NONE',  ( 9.823098133274648092, -2.494656445102012565, 31.33466734024120015 ) ) ;
#45175=CARTESIAN_POINT ( 'NONE',  ( 6.988332494352946789, -10.21337939537593620, 33.94971097300152252 ) ) ;
#45177=VERTEX_POINT ( 'NONE', #87079 ) ;
#45178=AXIS2_PLACEMENT_3D ( 'NONE', #38032, #65496, #3794 ) ;
#45179=ORIENTED_EDGE ( 'NONE', *, *, #48045, .F. ) ;
#45180=EDGE_LOOP ( 'NONE', ( #4910, #17180, #22658, #52059, #50037, #72396 ) ) ;
#45181=ORIENTED_EDGE ( 'NONE', *, *, #66937, .T. ) ;
#45182=EDGE_LOOP ( 'NONE', ( #72769, #52693, #57228, #58902 ) ) ;
#45183=LINE ( 'NONE', #2422, #37261 ) ;
#45184=FACE_OUTER_BOUND ( 'NONE', #18940, .T. ) ;
#45185=CARTESIAN_POINT ( 'NONE',  ( 15.23076923076910916, -6.835583212225970762, 34.95778746994575670 ) ) ;
#45186=CARTESIAN_POINT ( 'NONE',  ( -5.999999999999998224, -4.786620604624113540, 33.94971097300155094 ) ) ;
#45187=CARTESIAN_POINT ( 'NONE',  ( -13.38461538461550759, -3.643525952248795718, 33.31231777344771672 ) ) ;
#45189=ADVANCED_FACE ( 'NONE', ( #25351 ), #18604, .F. ) ;
#45190=CARTESIAN_POINT ( 'NONE',  ( -0.5276218724943428917, -11.69971097300155272, 32.46337939537587403 ) ) ;
#45191=CARTESIAN_POINT ( 'NONE',  ( -17.77698864838715309, -6.503523203565942268, 34.64991518177335195 ) ) ;
#45192=CARTESIAN_POINT ( 'NONE',  ( -4.153846153846273204, -10.21337939537710326, 33.94971097300076224 ) ) ;
#45195=EDGE_LOOP ( 'NONE', ( #24064, #76323 ) ) ;
#45196=VERTEX_POINT ( 'NONE', #26240 ) ;
#45197=CARTESIAN_POINT ( 'NONE',  ( 0.3954560821783248414, -11.91647553114624181, 32.58852847137148245 ) ) ;
#45198=ORIENTED_EDGE ( 'NONE', *, *, #54616, .F. ) ;
#45199=CARTESIAN_POINT ( 'NONE',  ( -16.02332045208259359, -6.852161475712351013, 34.70806712695775786 ) ) ;
#45200=CYLINDRICAL_SURFACE ( 'NONE', #23260, 0.2499999999999995559 ) ;
#45201=CARTESIAN_POINT ( 'NONE',  ( -13.38461538461550759, -3.643525952248795718, 33.31231777344771672 ) ) ;
#45202=LINE ( 'NONE', #52401, #48015 ) ;
#45203=FACE_BOUND ( 'NONE', #49938, .T. ) ;
#45204=VERTEX_POINT ( 'NONE', #59128 ) ;
#45205=VECTOR ( 'NONE', #66249, 1000.000000000000227 ) ;
#45206=ADVANCED_FACE ( 'NONE', ( #52813 ), #4639, .F. ) ;
#45207=EDGE_LOOP ( 'NONE', ( #88964, #16387 ) ) ;
#45208=DIRECTION ( 'NONE',  ( -0.000000000000000000, -0.7660444431189791237, -0.6427876096865379196 ) ) ;
#45209=CIRCLE ( 'NONE', #58135, 0.2500000000000002220 ) ;
#45210=ORIENTED_EDGE ( 'NONE', *, *, #65297, .T. ) ;
#45211=FACE_BOUND ( 'NONE', #75310, .T. ) ;
#45212=CARTESIAN_POINT ( 'NONE',  ( -6.065270445960775803, -9.442884908240170461, 34.35708131394840592 ) ) ;
#45213=VECTOR ( 'NONE', #26987, 1000.000000000000227 ) ;
#45214=CARTESIAN_POINT ( 'NONE',  ( -4.023320452082587373, -11.93748526763465279, 32.05452791011430946 ) ) ;
#45215=VERTEX_POINT ( 'NONE', #53259 ) ;
#45218=CARTESIAN_POINT ( 'NONE',  ( 2.241609928332172874, -11.35647404775217595, 33.31231777344666511 ) ) ;
#45219=ORIENTED_EDGE ( 'NONE', *, *, #68647, .F. ) ;
#45220=CYLINDRICAL_SURFACE ( 'NONE', #1102, 0.2499999999999973355 ) ;
#45221=CARTESIAN_POINT ( 'NONE',  ( 6.988332062589762472, -5.941354392334606160, 34.76329471203374055 ) ) ;
#45223=B_SPLINE_CURVE_WITH_KNOTS ( 'NONE', 3,
 ( #82214, #75016, #75448, #13744, #67364, #25928, #53394, #60150, #26820, #81772 ),
 .UNSPECIFIED., .F., .F.,
 ( 4, 2, 2, 2, 4 ),
 ( 0.000000000000000000, 0.0001954311564186863865, 0.0003908623128373727731, 0.0005862934692560591325, 0.0007817246256747455461 ),
 .UNSPECIFIED. ) ;
#45224=CARTESIAN_POINT ( 'NONE',  ( 2.307692307692186251, -12.51329471203414379, 31.30864560766407578 ) ) ;
#45226=ORIENTED_EDGE ( 'NONE', *, *, #27274, .T. ) ;
#45227=CARTESIAN_POINT ( 'NONE',  ( 18.25005431163831204, -6.567000820036036579, 34.66262288849541306 ) ) ;
#45228=CARTESIAN_POINT ( 'NONE',  ( -10.61538461538461320, -4.786620604624113540, 33.94971097300155094 ) ) ;
#45229=CARTESIAN_POINT ( 'NONE',  ( -2.557669038634660552, -2.564618984488975961, 30.55390908950641915 ) ) ;
#45230=LINE ( 'NONE', #65943, #70245 ) ;
#45231=FACE_OUTER_BOUND ( 'NONE', #74526, .T. ) ;
#45233=CARTESIAN_POINT ( 'NONE',  ( -0.2115384615384473255, -2.249999999999998668, 29.81603969181031033 ) ) ;
#45234=CARTESIAN_POINT ( 'NONE',  ( 5.010839665967194989, -12.37446782046654192, 30.86335684631486487 ) ) ;
#45235=CARTESIAN_POINT ( 'NONE',  ( -15.45425417449318317, -12.44517049084099725, 30.48991314939691932 ) ) ;
#45236=CARTESIAN_POINT ( 'NONE',  ( -3.230769230769229949, -11.33034616979429110, 35.88435417666054406 ) ) ;
#45237=CARTESIAN_POINT ( 'NONE',  ( 3.295963212552587507, -2.506253911140448043, 29.99999999999988631 ) ) ;
#45238=CYLINDRICAL_SURFACE ( 'NONE', #20479, 0.2500000000000008882 ) ;
#45240=ORIENTED_EDGE ( 'NONE', *, *, #48592, .T. ) ;
#45242=CARTESIAN_POINT ( 'NONE',  ( -12.71156169883143150, -8.432397168068783699, 34.66272746175022945 ) ) ;
#45243=ORIENTED_EDGE ( 'NONE', *, *, #65789, .T. ) ;
#45244=ADVANCED_FACE ( 'NONE', ( #6422 ), #80309, .F. ) ;
#45245=VERTEX_POINT ( 'NONE', #33001 ) ;
#45246=CARTESIAN_POINT ( 'NONE',  ( -16.85391023282967637, -4.026326845037968560, 33.68677907613345468 ) ) ;
#45247=ORIENTED_EDGE ( 'NONE', *, *, #27210, .T. ) ;
#45248=CARTESIAN_POINT ( 'NONE',  ( -5.934744860487159102, -10.33852847137154107, 34.16647553114620450 ) ) ;
#45250=CARTESIAN_POINT ( 'NONE',  ( -13.38461538461550759, -5.941354392335915335, 34.76329471203413846 ) ) ;
#45251=LINE ( 'NONE', #73641, #46767 ) ;
#45252=CARTESIAN_POINT ( 'NONE',  ( 1.634615384615386580, -7.500000000000001776, 35.04278698407183867 ) ) ;
#45253=CARTESIAN_POINT ( 'NONE',  ( -6.223484924564333554, -2.612411019501189813, 31.66733052389439962 ) ) ;
#45254=VECTOR ( 'NONE', #73839, 1000.000000000000227 ) ;
#45255=CARTESIAN_POINT ( 'NONE',  ( -10.39237177129121825, -3.395485233115139057, 33.02377354290275946 ) ) ;
#45256=CARTESIAN_POINT ( 'NONE',  ( 0.5276057948885363169, -5.471508081941601098, 34.59228464037088457 ) ) ;
#45257=CARTESIAN_POINT ( 'NONE',  ( 5.777073782483853392, -4.186968288167446595, 33.49512374952580274 ) ) ;
#45259=CARTESIAN_POINT ( 'NONE',  ( 1.607626736228235265, -3.105924265160262099, 32.13625925475356127 ) ) ;
#45260=CARTESIAN_POINT ( 'NONE',  ( -14.98082371242109012, -2.587454068350147018, 30.68340429815432202 ) ) ;
#45261=LINE ( 'NONE', #67765, #37793 ) ;
#45262=ORIENTED_EDGE ( 'NONE', *, *, #23874, .T. ) ;
#45263=ORIENTED_EDGE ( 'NONE', *, *, #42156, .T. ) ;
#45264=B_SPLINE_CURVE_WITH_KNOTS ( 'NONE', 3,
 ( #65171, #57090, #58405, #79142, #77804, #72373 ),
 .UNSPECIFIED., .F., .F.,
 ( 4, 2, 4 ),
 ( 0.0003909569690057790748, 0.0005862646681846021271, 0.0007815723673634251793 ),
 .UNSPECIFIED. ) ;
#45265=CARTESIAN_POINT ( 'NONE',  ( -11.53846153846165912, -6.026961402154118019, 34.52809138561165270 ) ) ;
#45267=CARTESIAN_POINT ( 'NONE',  ( 16.15384615384603251, -12.51329471203414379, 31.30864560766407578 ) ) ;
#45268=CARTESIAN_POINT ( 'NONE',  ( 6.250000000000000888, -2.249999999999998668, 29.75000000000000355 ) ) ;
#45269=CARTESIAN_POINT ( 'NONE',  ( -15.23076923076892264, -2.506253911140614576, 30.00000000000323297 ) ) ;
#45270=CYLINDRICAL_SURFACE ( 'NONE', #71635, 0.2499999999999986955 ) ;
#45271=EDGE_CURVE ( 'NONE', #73086, #40861, #26245, .T. ) ;
#45273=ORIENTED_EDGE ( 'NONE', *, *, #16168, .T. ) ;
#45274=CARTESIAN_POINT ( 'NONE',  ( 17.07692307692307665, -13.87047571288749737, 32.06866353760679544 ) ) ;
#45276=ORIENTED_EDGE ( 'NONE', *, *, #74804, .F. ) ;
#45278=VECTOR ( 'NONE', #88801, 1000.000000000000000 ) ;
#45280=CARTESIAN_POINT ( 'NONE',  ( -14.17690186672535901, -2.845873456487965747, 32.17976146951972538 ) ) ;
#45281=CARTESIAN_POINT ( 'NONE',  ( 11.60371667797437567, -2.379036618887895305, 30.90682066428158592 ) ) ;
#45282=CARTESIAN_POINT ( 'NONE',  ( 13.31853300525525086, -5.471508081941602875, 34.59228464037088457 ) ) ;
#45283=EDGE_CURVE ( 'NONE', #38452, #63694, #38636, .T. ) ;
#45284=ORIENTED_EDGE ( 'NONE', *, *, #79116, .F. ) ;
#45287=CARTESIAN_POINT ( 'NONE',  ( 1.384615384615265343, -11.48612834414049644, 32.76840700105863391 ) ) ;
#45289=B_SPLINE_CURVE_WITH_KNOTS ( 'NONE', 3,
 ( #12431, #61493, #53859, #75459, #5671, #68261, #81346, #19628, #54290, #13317 ),
 .UNSPECIFIED., .F., .F.,
 ( 4, 2, 2, 2, 4 ),
 ( 0.000000000000000000, 0.0001954339857564072033, 0.0003908679715128144066, 0.0005863019572692215828, 0.0007817359430256288133 ),
 .UNSPECIFIED. ) ;
#45290=B_SPLINE_CURVE_WITH_KNOTS ( 'NONE', 3,
 ( #55319, #42704, #27412, #76034, #76930, #69286, #75166, #13891, #15233, #1710 ),
 .UNSPECIFIED., .F., .F.,
 ( 4, 2, 2, 2, 4 ),
 ( 0.000000000000000000, 0.0001954339857564125972, 0.0003908679715128181471, 0.0005863019572692237513, 0.0007817359430256293554 ),
 .UNSPECIFIED. ) ;
#45291=CARTESIAN_POINT ( 'NONE',  ( -15.23076923076922995, -12.78798330534102767, 29.49999999999997868 ) ) ;
#45292=CARTESIAN_POINT ( 'NONE',  ( -15.00798968950081758, -3.236590943229499029, 32.36255958852954251 ) ) ;
#45293=ADVANCED_FACE ( 'NONE', ( #60466, #40211, #46065, #87983, #81195, #38875, #60020, #74427, #11851, #87524, #86631, #25799, #12729, #67674, #47388, #5981, #33448, #74882, #7749, #33879, #27571, #82963, #54585, #68552, #55043, #14950, #34321, #28013, #21695, #55481, #35210, #83861, #22146, #41530, #21245, #61336, #55921, #61785, #49167, #88853, #47837, #68994, #62235, #48720, #49616, #82532, #14052, #63117, #7304, #83412, #99, #42426, #20810, #76648, #82082, #62670, #6848, #1427, #69884, #42866, #76191, #20377, #27127, #69445, #8191, #48276, #988, #28460, #14494, #75747, #35667, #34765, #28919, #56375, #546, #41983, #77090, #15395, #70332, #75320, #13612, #41089, #57699, #15839, #43736, #71203, #16272, #36549, #36972, #43305, #50915, #9505, #63999, #2298, #50048, #23025, #78405, #57258, #36112, #85180, #29794, #84750, #44161, #64438, #50487, #16706, #9952, #2737, #77529, #37416, #30232, #64885, #77970, #23460, #71645, #8640, #63564, #1869, #29353, #56807, #84307, #22582, #70778, #9082, #30683, #17629, #38784, #72111, #23041, #58147, #64903, #10423, #29811, #86085, #17168, #84764, #38334, #43755, #66241, #57273, #2754, #37433, #9968, #30249, #51365, #31574, #85638, #50506, #72557, #3210, #23475, #71219, #65791, #24360, #77985, #85199, #44624, #9523, #23916, #78869, #50933, #16288, #65357, #36988, #64454, #57717, #78423, #31120, #16722, #37891, #44178, #71665, #3646, #58591, #51823, #11305, #79324, #18070, #45080, #10867, #4091, #59040, #86540, #24813, #52284, #79773, #45531, #73006, #87888, #73905, #75237, #26598, #81998, #53624, #26155, #46422, #53169, #13524, #12201, #5888, #33361, #46864, #86995, #5446, #39686, #74347, #4548, #60823, #81111, #59489, #13085, #18514, #41004, #32024, #66697, #25266, #52726, #12645, #67146, #27043, #40130, #80217, #47305, #19840, #45972, #73463, #47754, #60377, #80672, #11756, #19397, #39236, #5000, #67590, #74796, #87431, #88327, #54056, #81554, #32914, #40570, #25714, #68036, #32462, #6339, #61252, #33796, #88767, #20290, #59932, #18957, #54506, #28824, #48630, #29269, #1336, #35122, #36024, #84218, #62585, #34236, #896, #56282, #76107, #56722, #83771, #28362, #63476, #22495, #42341, #7219, #49957, #49078, #69795, #15749, #76560, #83324, #70240, #1778, #6762, #35576, #68465, #63020, #55835, #61699, #77005, #82445, #77438, #18, #41443, #27486, #54956, #21606, #21163, #20723, #14868, #68908, #75663, #48190, #8104, #14410, #22058, #34688, #49530, #62153, #15304, #13966, #42781, #460, #69363, #8548, #27927, #55395, #82882, #7663, #41894, #85528, #43211, #10310, #30572, #8992, #85089, #37777, #36888, #72446, #44518, #50827, #23369, #16181, #64790, #44966, #24250, #43646, #3541, #2211, #72004, #77875, #44075, #31011, #52171, #23804, #63912, #36458, #78763, #51715, #64350, #17063, #65243, #51256, #78312, #58476, #2647, #10755, #85972, #16612, #71556, #71114, #3096, #38223, #9861, #29706, #37325, #79217, #58043, #3981, #17516, #65682, #31467, #9424, #58933, #86439, #24710, #79660, #70686, #57166, #84654, #22934, #50395, #30139, #57606, #87779, #25603, #19294, #46763, #66596, #6230, #5779, #11653, #53058, #32807, #87327, #80103, #33695, #18849, #61150, #18404, #59826, #54398, #4898, #80566, #12104, #46315, #40466, #60267, #45863, #33255, #45415, #31923, #88663, #73803, #32362, #26941, #67040, #38669, #72893, #53507, #88222, #39129, #81004, #74238, #26052, #39581, #5335, #12537, #40022, #17962, #67484, #74688, #60715, #26495, #11199, #66132, #52620, #53959, #81450, #19735, #67925, #47196, #12980, #4436, #59384, #86888, #25153, #73347, #63369, #76898, #62475, #27818, #21049, #76002, #70131, #13857, #62046, #21951, #55286, #42235, #82332, #62914, #20615, #69688, #40898, #6658, #35914, #48520, #68806, #1676, #41789, #13417, #47650, #28255, #1228, #75556, #55726, #83215, #789, #34579, #76456, #7996, #7104, #48080, #28710, #82776, #29165, #41338, #353, #81893, #14303, #69251, #7554, #89102, #35015, #21497, #48977, #20184, #35463, #14755, #56177, #83669, #49424, #15200, #8441, #34130, #75132, #42671, #68360, #61598, #27382, #54848, #29598, #16077, #84108, #59612, #45656, #59166, #38464, #9329, #52402, #50283, #87113, #86673, #64242, #25389, #65917, #79892, #73594, #66821, #2113, #51956, #18194, #36788, #18644, #73133, #24487, #52851, #11888, #31709, #84549, #39363, #4227, #24939, #5120, #11433, #43540, #46106, #38916, #77772, #2546, #72684, #30036, #66375, #4680, #32154, #57496, #80347, #71018, #56621, #22389, #84985, #79453, #57056, #17752, #49852, #77333, #22826, #45203, #15639, #10992, #43107, #70580, #8884, #36352, #63815, #6454, #60505, #75783, #13209, #33913, #69033, #40689, #47422, #34353, #33482, #67710, #74915, #32585, #14089, #40245, #61373, #88886, #81230, #20842, #20407, #26276, #6015, #68152, #12760, #5564, #48310, #60942, #41561, #33038, #60054, #88016, #25839, #53294, #27159, #74463, #55073, #54619, #46549, #82569, #26717, #61824, #53744, #88446, #67269, #19515, #68587, #74028, #87560, #82114, #134, #46978, #80797, #27601, #47873, #75354, #54176, #81672, #19080, #12323, #39801, #13643, #19954, #41123, #6885, #76225, #55513, #579, #8674, #14532, #1466, #84780, #28494, #76682, #36581, #69917, #56840, #7778, #77563, #35242, #84337, #82997, #36148, #42016, #8226, #22611, #16306, #49646, #28046, #35701, #42901, #15874, #1019, #70366, #63599, #77121, #49205, #1902, #55955, #64032, #29391, #14983, #42455, #69475, #28954, #9117, #63151, #62264, #50079, #56408 ), #21281, .T. ) ;
#45294=FACE_OUTER_BOUND ( 'NONE', #87186, .T. ) ;
#45295=CYLINDRICAL_SURFACE ( 'NONE', #50910, 0.2499999999999995559 ) ;
#45296=ORIENTED_EDGE ( 'NONE', *, *, #29626, .F. ) ;
#45297=ADVANCED_FACE ( 'NONE', ( #43773 ), #48755, .F. ) ;
#45298=VERTEX_POINT ( 'NONE', #43336 ) ;
#45300=VECTOR ( 'NONE', #74734, 1000.000000000000227 ) ;
#45301=ORIENTED_EDGE ( 'NONE', *, *, #1988, .F. ) ;
#45302=CARTESIAN_POINT ( 'NONE',  ( -13.45069776397551564, -5.471508081941602875, 34.59228464037088457 ) ) ;
#45303=ORIENTED_EDGE ( 'NONE', *, *, #40439, .F. ) ;
#45304=DIRECTION ( 'NONE',  ( 0.000000000000000000, 0.6427876096865368094, 0.7660444431189802339 ) ) ;
#45305=CARTESIAN_POINT ( 'NONE',  ( 12.68431813051652846, -8.540255544307065350, 34.89611431652622286 ) ) ;
#45307=ORIENTED_EDGE ( 'NONE', *, *, #16938, .F. ) ;
#45308=EDGE_CURVE ( 'NONE', #60674, #21879, #2331, .T. ) ;
#45309=CARTESIAN_POINT ( 'NONE',  ( -14.53061926659915315, -12.38737895849757820, 31.66785238281580206 ) ) ;
#45310=EDGE_LOOP ( 'NONE', ( #16742, #10449 ) ) ;
#45311=CARTESIAN_POINT ( 'NONE',  ( -13.63463860883684120, -11.56360843649121684, 33.07473185843129926 ) ) ;
#45312=CARTESIAN_POINT ( 'NONE',  ( 14.37375964104238513, -12.34228464037088813, 31.77849191805839268 ) ) ;
#45313=FACE_BOUND ( 'NONE', #78950, .T. ) ;
#45314=DIRECTION ( 'NONE',  ( -0.000000000000000000, 0.5000000000000011102, -0.8660254037844380415 ) ) ;
#45315=CARTESIAN_POINT ( 'NONE',  ( -15.16557524898587594, -2.506253911140448487, 29.99999999999988631 ) ) ;
#45316=EDGE_CURVE ( 'NONE', #14607, #28677, #7341, .T. ) ;
#45317=CARTESIAN_POINT ( 'NONE',  ( -1.450697763975518306, -3.322132147404559976, 32.92929555188719348 ) ) ;
#45318=CYLINDRICAL_SURFACE ( 'NONE', #47737, 0.2500000000000002220 ) ;
#45320=CARTESIAN_POINT ( 'NONE',  ( -11.53846153846153655, -8.164416787775445883, 34.95778746994557906 ) ) ;
#45321=ADVANCED_FACE ( 'NONE', ( #34796 ), #23062, .F. ) ;
#45323=VERTEX_POINT ( 'NONE', #10882 ) ;
#45324=B_SPLINE_CURVE_WITH_KNOTS ( 'NONE', 3,
 ( #72322, #58354, #79087, #24132, #39007, #18732, #72765, #32240, #39453, #46196 ),
 .UNSPECIFIED., .F., .F.,
 ( 4, 2, 2, 2, 4 ),
 ( 0.0007817246256747450040, 0.0009771112852218881168, 0.001172497944769031230, 0.001367884604316174342, 0.001563271263863317455 ),
 .UNSPECIFIED. ) ;
#45325=CARTESIAN_POINT ( 'NONE',  ( 6.700150705560774966, -5.667676309546437530, 34.40238873228292249 ) ) ;
#45326=CARTESIAN_POINT ( 'NONE',  ( -11.53846153846153655, -10.05456864172156806, 36.03766855953608683 ) ) ;
#45327=FACE_OUTER_BOUND ( 'NONE', #18949, .T. ) ;
#45328=CARTESIAN_POINT ( 'NONE',  ( 13.38461538461526423, -4.320704448113951379, 33.92786785259630022 ) ) ;
#45330=EDGE_CURVE ( 'NONE', #19105, #273, #56232, .T. ) ;
#45331=FACE_BOUND ( 'NONE', #77829, .T. ) ;
#45332=CARTESIAN_POINT ( 'NONE',  ( 12.21156171748986985, -10.06842814019191401, 34.32929386961144758 ) ) ;
#45333=CARTESIAN_POINT ( 'NONE',  ( 4.376858997939548246, -12.64618726649961289, 30.78989965857442712 ) ) ;
#45334=DIRECTION ( 'NONE',  ( -0.000000000000000000, 0.9848077530122086864, -0.1736481776669273891 ) ) ;
#45335=CARTESIAN_POINT ( 'NONE',  ( -11.60378555126584388, -7.749976730030849303, 34.74374725381503737 ) ) ;
#45336=CARTESIAN_POINT ( 'NONE',  ( 14.30769230769218581, -11.06231777344772027, 33.60647404775119895 ) ) ;
#45337=CARTESIAN_POINT ( 'NONE',  ( 16.15384615384615330, -10.51840700105979565, 33.73612834413961536 ) ) ;
#45338=CARTESIAN_POINT ( 'NONE',  ( -8.546219417617921366, -3.587049720035815348, 32.86302985866382897 ) ) ;
#45340=ORIENTED_EDGE ( 'NONE', *, *, #58006, .T. ) ;
#45341=DIRECTION ( 'NONE',  ( -0.000000000000000000, 1.000000000000000000, 3.491481338843133355E-15 ) ) ;
#45342=EDGE_CURVE ( 'NONE', #58859, #60261, #73466, .T. ) ;
#45343=EDGE_CURVE ( 'NONE', #40578, #2477, #23494, .T. ) ;
#45344=CARTESIAN_POINT ( 'NONE',  ( 16.15384615384615330, -9.905515769479276145, 34.41647553114623292 ) ) ;
#45347=VECTOR ( 'NONE', #40992, 1000.000000000000114 ) ;
#45348=CARTESIAN_POINT ( 'NONE',  ( 3.296024802045255164, -6.879047030191282275, 34.71129190930002295 ) ) ;
#45349=CARTESIAN_POINT ( 'NONE',  ( -11.76194646302587010, -4.225889041578353655, 33.85425143139329407 ) ) ;
#45351=CARTESIAN_POINT ( 'NONE',  ( -15.23076923076935252, -12.70778746994576025, 30.41441678777401236 ) ) ;
#45352=CARTESIAN_POINT ( 'NONE',  ( -2.084679463598912097, -6.460100341425561332, 34.89618726649961644 ) ) ;
#45354=CARTESIAN_POINT ( 'NONE',  ( -6.923076923076922462, -12.62096338111211580, 30.90682066428153263 ) ) ;
#45355=CARTESIAN_POINT ( 'NONE',  ( 14.43848411551709709, -5.582136614379148654, 34.36778462344220486 ) ) ;
#45357=CARTESIAN_POINT ( 'NONE',  ( -18.00000000000000000, -10.05012543904494748, 36.02546096051201374 ) ) ;
#45358=CARTESIAN_POINT ( 'NONE',  ( 7.976944287120795174, -9.084667340241226796, 34.75534355489798344 ) ) ;
#45359=EDGE_LOOP ( 'NONE', ( #56138, #39460, #74986, #49599 ) ) ;
#45360=CARTESIAN_POINT ( 'NONE',  ( 15.16549923021291058, -11.67786785259540849, 32.92929555188721480 ) ) ;
#45361=CARTESIAN_POINT ( 'NONE',  ( -1.607481647678483005, -2.251424796025575770, 29.88072029997477586 ) ) ;
#45363=CARTESIAN_POINT ( 'NONE',  ( -10.68146699474474914, -2.486705287966279432, 31.30864560766542937 ) ) ;
#45364=CARTESIAN_POINT ( 'NONE',  ( -5.207614543590636913, -2.541943142973490666, 30.39792223712631980 ) ) ;
#45365=VERTEX_POINT ( 'NONE', #31136 ) ;
#45367=CARTESIAN_POINT ( 'NONE',  ( 9.692307692307570832, -12.70778746994576025, 30.41441678777401236 ) ) ;
#45369=ORIENTED_EDGE ( 'NONE', *, *, #11817, .T. ) ;
#45370=CARTESIAN_POINT ( 'NONE',  ( -9.692307692307691624, -11.16473453929635440, 33.15142922261926373 ) ) ;
#45371=DIRECTION ( 'NONE',  ( 0.000000000000000000, 0.4999999999999985567, 0.8660254037844395958 ) ) ;
#45372=CARTESIAN_POINT ( 'NONE',  ( -8.703162418228330921, -2.538708090699994813, 30.37095296980875503 ) ) ;
#45373=EDGE_CURVE ( 'NONE', #15767, #77091, #70271, .T. ) ;
#45374=VECTOR ( 'NONE', #49484, 1000.000000000000114 ) ;
#45375=DIRECTION ( 'NONE',  ( -0.000000000000000000, 1.000000000000000000, -0.000000000000000000 ) ) ;
#45376=ORIENTED_EDGE ( 'NONE', *, *, #3907, .T. ) ;
#45377=CARTESIAN_POINT ( 'NONE',  ( 2.557637826040450868, -12.22109172314383052, 31.39792113162168263 ) ) ;
#45380=ORIENTED_EDGE ( 'NONE', *, *, #9087, .F. ) ;
#45382=EDGE_CURVE ( 'NONE', #32057, #73835, #36915, .T. ) ;
#45386=CARTESIAN_POINT ( 'NONE',  ( -18.22292621751613950, -3.586966769969697211, 32.86292498521068950 ) ) ;
#45387=CARTESIAN_POINT ( 'NONE',  ( -4.153846153846152411, -1.242168528481310874, 33.36296068462461051 ) ) ;
#45388=CARTESIAN_POINT ( 'NONE',  ( -9.442253272394237840, -12.65882529074907126, 30.72640787790839312 ) ) ;
#45389=B_SPLINE_CURVE_WITH_KNOTS ( 'NONE', 3,
 ( #46320, #46768, #39586, #67930, #86891, #5339, #26499, #52174, #53061, #53962 ),
 .UNSPECIFIED., .F., .F.,
 ( 4, 2, 2, 2, 4 ),
 ( 0.0007817359430256324996, 0.0009771253907249993591, 0.001172514838424366110, 0.001367904286123732861, 0.001563293733823099829 ),
 .UNSPECIFIED. ) ;
#45390=EDGE_CURVE ( 'NONE', #42964, #19767, #16498, .T. ) ;
#45391=LINE ( 'NONE', #65654, #60722 ) ;
#45392=VECTOR ( 'NONE', #23034, 1000.000000000000227 ) ;
#45393=ORIENTED_EDGE ( 'NONE', *, *, #71929, .F. ) ;
#45394=ORIENTED_EDGE ( 'NONE', *, *, #42869, .F. ) ;
#45395=CARTESIAN_POINT ( 'NONE',  ( 11.53846153846141576, -11.67786785259630911, 32.92929555188603530 ) ) ;
#45396=ORIENTED_EDGE ( 'NONE', *, *, #42719, .F. ) ;
#45398=CARTESIAN_POINT ( 'NONE',  ( 15.16549878480845770, -3.300289026998414865, 32.46337939537583139 ) ) ;
#45399=CARTESIAN_POINT ( 'NONE',  ( -8.703975197954745724, -12.46129190930001052, 30.37095296980870174 ) ) ;
#45400=CARTESIAN_POINT ( 'NONE',  ( -1.384615384615506484, -12.70778746994576025, 30.41441678777401236 ) ) ;
#45401=EDGE_LOOP ( 'NONE', ( #877, #58801 ) ) ;
#45402=EDGE_CURVE ( 'NONE', #87727, #60602, #78872, .T. ) ;
#45404=ADVANCED_FACE ( 'NONE', ( #46439 ), #73483, .F. ) ;
#45405=VERTEX_POINT ( 'NONE', #61268 ) ;
#45407=ORIENTED_EDGE ( 'NONE', *, *, #30658, .T. ) ;
#45408=CARTESIAN_POINT ( 'NONE',  ( 17.99999999999987566, -12.16647553114689728, 32.15551576947799362 ) ) ;
#45410=VERTEX_POINT ( 'NONE', #53640 ) ;
#45411=CYLINDRICAL_SURFACE ( 'NONE', #70506, 0.2500000000000009437 ) ;
#45412=CARTESIAN_POINT ( 'NONE',  ( -6.923076923076922462, -7.500000000000001776, 35.04278698407183867 ) ) ;
#45413=CARTESIAN_POINT ( 'NONE',  ( 0.4615384615384611755, -13.95598074871891292, 31.83374038241031911 ) ) ;
#45414=B_SPLINE_CURVE_WITH_KNOTS ( 'NONE', 3,
 ( #53717, #86641, #10960, #39336, #32121, #10518 ),
 .UNSPECIFIED., .F., .F.,
 ( 4, 2, 4 ),
 ( 0.000000000000000000, 0.0001954784845028921395, 0.0003909569690057842790 ),
 .UNSPECIFIED. ) ;
#45415=FACE_BOUND ( 'NONE', #88252, .T. ) ;
#45417=CARTESIAN_POINT ( 'NONE',  ( 11.47237812750566022, -8.120952969808774569, 34.71129190930000163 ) ) ;
#45418=CARTESIAN_POINT ( 'NONE',  ( -8.096130577096198877, -12.17611988154120972, 31.52148481390971213 ) ) ;
#45419=CARTESIAN_POINT ( 'NONE',  ( 3.480714640147274608, -3.520799739797214389, 33.17531984108286025 ) ) ;
#45420=CARTESIAN_POINT ( 'NONE',  ( 14.53047197667037160, -3.020022701398814569, 32.48759521482552515 ) ) ;
#45422=CARTESIAN_POINT ( 'NONE',  ( 8.638540166120458608, -9.084618155246140248, 34.75535874321725771 ) ) ;
#45423=CARTESIAN_POINT ( 'NONE',  ( -16.15384615384627409, -8.613356846316285953, 34.62446782046622218 ) ) ;
#45426=CARTESIAN_POINT ( 'NONE',  ( 12.68431813051652846, -3.563462043263030399, 33.22394488606062879 ) ) ;
#45427=ORIENTED_EDGE ( 'NONE', *, *, #18474, .T. ) ;
#45429=AXIS2_PLACEMENT_3D ( 'NONE', #61886, #20471, #13709 ) ;
#45430=CARTESIAN_POINT ( 'NONE',  ( -11.53846153846153655, -12.62096338111211580, 30.90682066428153263 ) ) ;
#45431=CARTESIAN_POINT ( 'NONE',  ( 1.515140822849032176, -5.915461855592777596, 34.75538340440931506 ) ) ;
#45432=CARTESIAN_POINT ( 'NONE',  ( -16.82697766754503377, -12.68172785388650681, 30.59649109432439573 ) ) ;
#45433=CARTESIAN_POINT ( 'NONE',  ( 2.438217745925953750, -2.372941743896878286, 30.88044141588254377 ) ) ;
#45434=DIRECTION ( 'NONE',  ( -0.000000000000000000, 0.1736481776669307198, -0.9848077530122080203 ) ) ;
#45435=ORIENTED_EDGE ( 'NONE', *, *, #43717, .F. ) ;
#45436=CARTESIAN_POINT ( 'NONE',  ( 8.639082799499073317, -12.70455904226513866, 30.44083106164009322 ) ) ;
#45440=CARTESIAN_POINT ( 'NONE',  ( 9.692307692307695177, -1.509761064869970415, 31.06009739812519044 ) ) ;
#45441=CARTESIAN_POINT ( 'NONE',  ( 0.3954560821783247304, -12.62096338111211580, 30.90682066428152197 ) ) ;
#45442=CARTESIAN_POINT ( 'NONE',  ( 7.780883400193070898, -6.026961402152685388, 34.52809138561120506 ) ) ;
#45443=CARTESIAN_POINT ( 'NONE',  ( 10.68145296638705410, -4.098570777380720287, 33.41473453929635440 ) ) ;
#45444=LINE ( 'NONE', #53085, #76543 ) ;
#45446=ORIENTED_EDGE ( 'NONE', *, *, #54589, .T. ) ;
#45448=VERTEX_POINT ( 'NONE', #88345 ) ;
#45450=CARTESIAN_POINT ( 'NONE',  ( 14.17754433796061342, -12.50552854090298638, 31.33409797877408920 ) ) ;
#45452=CARTESIAN_POINT ( 'NONE',  ( -18.22287868242863951, -7.630691491037286056, 34.74850469731152458 ) ) ;
#45453=CARTESIAN_POINT ( 'NONE',  ( -14.30769230769230660, -12.78798330534103123, 29.99999999999997868 ) ) ;
#45454=CARTESIAN_POINT ( 'NONE',  ( 14.30769230769231015, -2.721908614388771852, 31.22303859784724978 ) ) ;
#45455=CYLINDRICAL_SURFACE ( 'NONE', #80229, 0.2499999999999995559 ) ;
#45457=FACE_OUTER_BOUND ( 'NONE', #72981, .T. ) ;
#45458=CARTESIAN_POINT ( 'NONE',  ( -13.60810032833933469, -8.496056993536548418, 34.65000542017679663 ) ) ;
#45459=EDGE_CURVE ( 'NONE', #74166, #19286, #32477, .T. ) ;
#45460=CARTESIAN_POINT ( 'NONE',  ( -8.992157728137618378, -12.64616026154729411, 30.79003144601914244 ) ) ;
#45461=CARTESIAN_POINT ( 'NONE',  ( 12.23805353697412990, -11.60425143139329940, 33.02411095842164457 ) ) ;
#45462=CARTESIAN_POINT ( 'NONE',  ( -39.05038313613820122, -2.499999999999999556, 29.75000000000000355 ) ) ;
#45463=CYLINDRICAL_SURFACE ( 'NONE', #27111, 0.2500000000000004996 ) ;
#45464=CARTESIAN_POINT ( 'NONE',  ( 2.057669070399342992, -3.202444869320336451, 32.30641848906366675 ) ) ;
#45465=DIRECTION ( 'NONE',  ( -0.000000000000000000, 0.9396926207859093161, -0.3420201433256663259 ) ) ;
#45466=VECTOR ( 'NONE', #159, 1000.000000000000000 ) ;
#45467=DIRECTION ( 'NONE',  ( 0.000000000000000000, 0.000000000000000000, 1.000000000000000000 ) ) ;
#45468=B_SPLINE_CURVE_WITH_KNOTS ( 'NONE', 3,
 ( #68269, #7463, #63278, #84020, #257, #48879, #27719, #13324, #89008, #54749 ),
 .UNSPECIFIED., .F., .F.,
 ( 4, 2, 2, 2, 4 ),
 ( 0.000000000000000000, 0.0001954311584214072652, 0.0003908623168428145304, 0.0005862934752642217414, 0.0007817246336856290608 ),
 .UNSPECIFIED. ) ;
#45469=B_SPLINE_CURVE_WITH_KNOTS ( 'NONE', 3,
 ( #8993, #56724, #70687, #63914, #22935, #2648, #32808, #52172, #60268, #58477 ),
 .UNSPECIFIED., .F., .F.,
 ( 4, 2, 2, 2, 4 ),
 ( 0.0007817246256747504250, 0.0009771112852218954894, 0.001172497944769040554, 0.001367884604316185401, 0.001563271263863330466 ),
 .UNSPECIFIED. ) ;
#45470=CARTESIAN_POINT ( 'NONE',  ( -3.100243529005668019, -11.46989282347013095, 32.79007818306219946 ) ) ;
#45471=CARTESIAN_POINT ( 'NONE',  ( -17.01166793741023042, -3.083524468853783951, 32.58852847137153930 ) ) ;
#45472=EDGE_CURVE ( 'NONE', #51215, #80969, #88486, .T. ) ;
#45473=VERTEX_POINT ( 'NONE', #82461 ) ;
#45475=CARTESIAN_POINT ( 'NONE',  ( 8.992010310499177095, -11.89424750095246175, 32.13594075562310337 ) ) ;
#45476=CARTESIAN_POINT ( 'NONE',  ( -4.403869378067610363, -5.765609946408404518, 34.70566812827425451 ) ) ;
#45478=CARTESIAN_POINT ( 'NONE',  ( -17.07692307692307665, -5.471508081941601098, 34.59228464037088457 ) ) ;
#45479=CARTESIAN_POINT ( 'NONE',  ( 8.546303810323914618, -10.01117774369187252, 34.36070679894347535 ) ) ;
#45480=EDGE_CURVE ( 'NONE', #19270, #43177, #35758, .T. ) ;
#45481=CARTESIAN_POINT ( 'NONE',  ( -0.2115929431903192937, -2.587454068350147907, 30.68340429815432202 ) ) ;
#45482=ORIENTED_EDGE ( 'NONE', *, *, #64115, .F. ) ;
#45484=CARTESIAN_POINT ( 'NONE',  ( -1.319360245102545681, -12.51329471203373700, 31.30864560766537963 ) ) ;
#45485=VECTOR ( 'NONE', #8447, 1000.000000000000000 ) ;
#45487=CARTESIAN_POINT ( 'NONE',  ( 6.792386319966616348, -6.369640206132550553, 34.87707690430378449 ) ) ;
#45489=CYLINDRICAL_SURFACE ( 'NONE', #69387, 0.2500000000000002220 ) ;
#45491=CARTESIAN_POINT ( 'NONE',  ( -9.561781990544133691, -2.882268652242222284, 31.66798894389554064 ) ) ;
#45492=CARTESIAN_POINT ( 'NONE',  ( -0.2115930521604184322, -6.653508905675590945, 34.93172785388651391 ) ) ;
#45493=ORIENTED_EDGE ( 'NONE', *, *, #50969, .F. ) ;
#45494=CYLINDRICAL_SURFACE ( 'NONE', #27833, 0.2499999999999998890 ) ;
#45495=VERTEX_POINT ( 'NONE', #25729 ) ;
#45496=CARTESIAN_POINT ( 'NONE',  ( 11.28848480751918437, -3.627789207965226748, 32.91389620160131102 ) ) ;
#45498=ORIENTED_EDGE ( 'NONE', *, *, #67301, .T. ) ;
#45499=CARTESIAN_POINT ( 'NONE',  ( 2.084207383127978375, -9.417330523894424488, 34.63758898049880486 ) ) ;
#45500=CARTESIAN_POINT ( 'NONE',  ( -7.846153846153844924, -5.180354513474913603, 36.12317359536750416 ) ) ;
#45501=AXIS2_PLACEMENT_3D ( 'NONE', #62428, #61549, #1181 ) ;
#45502=ORIENTED_EDGE ( 'NONE', *, *, #68228, .F. ) ;
#45503=DIRECTION ( 'NONE',  ( 0.000000000000000000, 0.4999999999999960032, -0.8660254037844410391 ) ) ;
#45504=CARTESIAN_POINT ( 'NONE',  ( 9.822833130541340552, -10.31582465632705237, 34.18122507451815295 ) ) ;
#45505=CARTESIAN_POINT ( 'NONE',  ( 12.68431800280687050, -5.114059244376869984, 34.14424750095245287 ) ) ;
#45506=B_SPLINE_CURVE_WITH_KNOTS ( 'NONE', 3,
 ( #79232, #3557, #24266, #31025, #11668, #58946, #30584, #17076, #79674, #86452 ),
 .UNSPECIFIED., .F., .F.,
 ( 4, 2, 2, 2, 4 ),
 ( 0.0007817359430256319575, 0.0009771253907249984917, 0.001172514838424365026, 0.001367904286123731343, 0.001563293733823097878 ),
 .UNSPECIFIED. ) ;
#45507=AXIS2_PLACEMENT_3D ( 'NONE', #32440, #40101, #59905 ) ;
#45508=EDGE_CURVE ( 'NONE', #88972, #76747, #66911, .T. ) ;
#45509=CARTESIAN_POINT ( 'NONE',  ( -4.153846153846152411, -13.78497067705608181, 32.30358669280327177 ) ) ;
#45510=CARTESIAN_POINT ( 'NONE',  ( -7.846153846153844924, -12.62096338111211580, 30.90682066428153263 ) ) ;
#45511=B_SPLINE_CURVE_WITH_KNOTS ( 'NONE', 3,
 ( #6870, #33020, #75340, #26700, #41109, #20829 ),
 .UNSPECIFIED., .F., .F.,
 ( 4, 2, 4 ),
 ( 0.000000000000000000, 0.0001954784845028921395, 0.0003909569690057842790 ),
 .UNSPECIFIED. ) ;
#45512=B_SPLINE_CURVE_WITH_KNOTS ( 'NONE', 3,
 ( #52987, #46248, #39505, #26424, #25971, #54323, #18332, #45795, #53436, #73276 ),
 .UNSPECIFIED., .F., .F.,
 ( 4, 2, 2, 2, 4 ),
 ( 0.000000000000000000, 0.0001954339857564098054, 0.0003908679715128196108, 0.0005863019572692293891, 0.0007817359430256392216 ),
 .UNSPECIFIED. ) ;
#45514=VERTEX_POINT ( 'NONE', #55852 ) ;
#45515=ADVANCED_FACE ( 'NONE', ( #42358 ), #28841, .F. ) ;
#45516=AXIS2_PLACEMENT_3D ( 'NONE', #10685, #64277, #79141 ) ;
#45518=CARTESIAN_POINT ( 'NONE',  ( -7.846153846153844924, -11.11383981884818262, 36.00935417666054406 ) ) ;
#45519=EDGE_LOOP ( 'NONE', ( #38081, #65773, #73503, #82976 ) ) ;
#45520=DIRECTION ( 'NONE',  ( -0.000000000000000000, 0.7660444431189791237, -0.6427876096865379196 ) ) ;
#45521=FACE_OUTER_BOUND ( 'NONE', #45359, .T. ) ;
#45522=ORIENTED_EDGE ( 'NONE', *, *, #70965, .T. ) ;
#45523=EDGE_CURVE ( 'NONE', #31425, #7198, #34691, .T. ) ;
#45524=EDGE_CURVE ( 'NONE', #57246, #23981, #20646, .T. ) ;
#45525=EDGE_LOOP ( 'NONE', ( #58362, #35876, #79755, #80416 ) ) ;
#45526=CARTESIAN_POINT ( 'NONE',  ( 16.94677586748485965, -10.19110544564092002, 33.96427741523702792 ) ) ;
#45527=ORIENTED_EDGE ( 'NONE', *, *, #52412, .T. ) ;
#45528=CARTESIAN_POINT ( 'NONE',  ( -18.00000000000000000, -9.058645607665452459, 34.76329471203371924 ) ) ;
#45529=CARTESIAN_POINT ( 'NONE',  ( -13.38461538461550759, -5.941354392335915335, 34.76329471203413846 ) ) ;
#45530=CARTESIAN_POINT ( 'NONE',  ( -16.15384615384627409, -11.06231777344772027, 33.60647404775119895 ) ) ;
#45531=FACE_BOUND ( 'NONE', #8456, .T. ) ;
#45532=CARTESIAN_POINT ( 'NONE',  ( -0.4615384615384611200, -7.500000000000001776, 35.04278698407183867 ) ) ;
#45533=CARTESIAN_POINT ( 'NONE',  ( 12.46153846153846168, -8.973038597847269315, 34.52809138561121927 ) ) ;
#45534=DIRECTION ( 'NONE',  ( 0.000000000000000000, 0.9396926207859126468, -0.3420201433256571111 ) ) ;
#45535=DIRECTION ( 'NONE',  ( -0.000000000000000000, -0.3420201433256694901, -0.9396926207859082059 ) ) ;
#45536=CYLINDRICAL_SURFACE ( 'NONE', #56716, 0.2499999999999986955 ) ;
#45537=CARTESIAN_POINT ( 'NONE',  ( -16.15384615384627409, -3.083524468854526912, 32.58852847137268327 ) ) ;
#45538=VERTEX_POINT ( 'NONE', #68922 ) ;
#45539=CARTESIAN_POINT ( 'NONE',  ( -2.057637996053991447, -9.148310452688873440, 34.47095581063188519 ) ) ;
#45540=ORIENTED_EDGE ( 'NONE', *, *, #26335, .T. ) ;
#45541=ORIENTED_EDGE ( 'NONE', *, *, #29681, .F. ) ;
#45542=CARTESIAN_POINT ( 'NONE',  ( 10.68064018666064108, -12.46129190930001052, 30.37095296980870174 ) ) ;
#45543=CARTESIAN_POINT ( 'NONE',  ( 10.83839596699746721, -5.667800583137506010, 34.40243808032445827 ) ) ;
#45544=B_SPLINE_CURVE_WITH_KNOTS ( 'NONE', 3,
 ( #65844, #38841, #26207, #12250, #67203, #51879, #79376, #59094, #5503, #86593 ),
 .UNSPECIFIED., .F., .F.,
 ( 4, 2, 2, 2, 4 ),
 ( 0.0007817246256747472808, 0.0009771112852218905021, 0.001172497944769033832, 0.001367884604316177161, 0.001563271263863320274 ),
 .UNSPECIFIED. ) ;
#45545=CARTESIAN_POINT ( 'NONE',  ( 2.980792486720639456, -3.436278759898155233, 33.07459398097509506 ) ) ;
#45548=CARTESIAN_POINT ( 'NONE',  ( 1.515405825582337718, -3.957578996910242619, 33.62503395064540257 ) ) ;
#45550=DIRECTION ( 'NONE',  ( -0.000000000000000000, 0.1736481776669307198, -0.9848077530122080203 ) ) ;
#45551=CARTESIAN_POINT ( 'NONE',  ( -5.749999999999999112, -2.249999999999998668, 29.75000000000000355 ) ) ;
#45552=CARTESIAN_POINT ( 'NONE',  ( -1.634638621908348632, -3.711651800289232028, 33.01384336483936011 ) ) ;
#45553=CARTESIAN_POINT ( 'NONE',  ( -4.088590582570129861, -3.835265460703683349, 33.15142922261929925 ) ) ;
#45554=ORIENTED_EDGE ( 'NONE', *, *, #26591, .T. ) ;
#45555=VERTEX_POINT ( 'NONE', #476 ) ;
#45556=EDGE_LOOP ( 'NONE', ( #42001, #50282, #56718, #62192 ) ) ;
#45557=VECTOR ( 'NONE', #64198, 1000.000000000000000 ) ;
#45558=CARTESIAN_POINT ( 'NONE',  ( -17.75000000000000711, -2.249999999999999112, 29.81889780837710902 ) ) ;
#45559=CARTESIAN_POINT ( 'NONE',  ( 5.076923076923075762, -2.833524468853757305, 32.15551576947925838 ) ) ;
#45560=ADVANCED_FACE ( 'NONE', ( #49095 ), #48649, .F. ) ;
#45561=ORIENTED_EDGE ( 'NONE', *, *, #15690, .F. ) ;
#45562=CARTESIAN_POINT ( 'NONE',  ( -3.230769230769229949, -1.790695186598648903, 34.54067556320373455 ) ) ;
#45563=CARTESIAN_POINT ( 'NONE',  ( 6.130525438233644486, -11.66157788607254275, 32.95092075102925833 ) ) ;
#45564=CARTESIAN_POINT ( 'NONE',  ( -8.703975197954740395, -6.879047030191282275, 34.71129190930002295 ) ) ;
#45565=CARTESIAN_POINT ( 'NONE',  ( -1.384615384615506484, -4.320704448113951379, 33.92786785259630022 ) ) ;
#45567=CARTESIAN_POINT ( 'NONE',  ( -0.6844646790546086157, -11.24512374952581872, 33.06303171183252942 ) ) ;
#45568=ORIENTED_EDGE ( 'NONE', *, *, #54665, .T. ) ;
#45569=ADVANCED_FACE ( 'NONE', ( #34705 ), #7680, .F. ) ;
#45570=CARTESIAN_POINT ( 'NONE',  ( 0.2115617305961068062, -9.943427161483782584, 34.11278801902876978 ) ) ;
#45571=ORIENTED_EDGE ( 'NONE', *, *, #23441, .F. ) ;
#45572=CARTESIAN_POINT ( 'NONE',  ( -8.703975197954747500, -10.21337939537593620, 33.94971097300152252 ) ) ;
#45573=CARTESIAN_POINT ( 'NONE',  ( 4.023154687178596589, -6.413092428213692742, 34.63065189839063152 ) ) ;
#45574=CYLINDRICAL_SURFACE ( 'NONE', #45814, 0.2499999999999997502 ) ;
#45575=CARTESIAN_POINT ( 'NONE',  ( -10.74553258511630993, -3.625366637846544116, 33.29286588640298561 ) ) ;
#45576=DIRECTION ( 'NONE',  ( -0.000000000000000000, 0.9848077530122086864, -0.1736481776669273891 ) ) ;
#45579=EDGE_CURVE ( 'NONE', #24114, #2558, #72323, .T. ) ;
#45581=VERTEX_POINT ( 'NONE', #70258 ) ;
#45582=CARTESIAN_POINT ( 'NONE',  ( 5.011653076366755499, -12.16647553114622049, 32.15551576947930812 ) ) ;
#45583=CARTESIAN_POINT ( 'NONE',  ( -9.469296340694842939, -8.239487800360276282, 34.69522927552633718 ) ) ;
#45584=CARTESIAN_POINT ( 'NONE',  ( -0.3307466537136757867, -4.809403383903225304, 33.96459661697924304 ) ) ;
#45585=VERTEX_POINT ( 'NONE', #8565 ) ;
#45586=ORIENTED_EDGE ( 'NONE', *, *, #12433, .T. ) ;
#45587=CARTESIAN_POINT ( 'NONE',  ( 9.692307692307695177, -3.322132147404559976, 32.92929555188717927 ) ) ;
#45590=DIRECTION ( 'NONE',  ( 0.000000000000000000, 0.000000000000000000, -1.000000000000000000 ) ) ;
#45591=EDGE_CURVE ( 'NONE', #81768, #85253, #29284, .T. ) ;
#45592=CARTESIAN_POINT ( 'NONE',  ( 17.77651507543566822, -12.11044203135681840, 32.26167407432752299 ) ) ;
#45593=CARTESIAN_POINT ( 'NONE',  ( 5.749976762707035505, -8.432397168068783699, 34.66272746175022945 ) ) ;
#45594=EDGE_LOOP ( 'NONE', ( #85240, #39722 ) ) ;
#45597=CARTESIAN_POINT ( 'NONE',  ( -2.084912766423897779, -10.11255958852955850, 34.01340905677048454 ) ) ;
#45598=CARTESIAN_POINT ( 'NONE',  ( 9.468822767743361624, -2.612411019501189369, 31.66733052389439962 ) ) ;
#45599=ORIENTED_EDGE ( 'NONE', *, *, #52245, .F. ) ;
#45600=CARTESIAN_POINT ( 'NONE',  ( -7.715362038329059757, -3.530189275343204702, 32.79018710029569661 ) ) ;
#45602=ADVANCED_FACE ( 'NONE', ( #49977 ), #30589, .F. ) ;
#45604=DIRECTION ( 'NONE',  ( -0.000000000000000000, -0.3420201433256694901, -0.9396926207859082059 ) ) ;
#45606=CARTESIAN_POINT ( 'NONE',  ( -5.076923076923075762, -13.37000171582298513, 34.34916445242398453 ) ) ;
#45607=DIRECTION ( 'NONE',  ( 0.000000000000000000, 0.3420201433256641055, -0.9396926207859100932 ) ) ;
#45608=ORIENTED_EDGE ( 'NONE', *, *, #33376, .F. ) ;
#45609=ADVANCED_FACE ( 'NONE', ( #72913 ), #78332, .F. ) ;
#45610=VECTOR ( 'NONE', #10113, 1000.000000000000227 ) ;
#45611=CARTESIAN_POINT ( 'NONE',  ( -17.32692307692307665, -7.500000000000001776, 35.04278698407183867 ) ) ;
#45612=CARTESIAN_POINT ( 'NONE',  ( 13.63456079399343146, -9.357781135181031829, 34.66075350412533851 ) ) ;
#45613=CARTESIAN_POINT ( 'NONE',  ( -1.384615384615383471, -13.20930481340135110, 34.54067556320372745 ) ) ;
#45614=CARTESIAN_POINT ( 'NONE',  ( -6.223484924564328225, -5.827078755546623690, 34.72654668319379567 ) ) ;
#45615=CARTESIAN_POINT ( 'NONE',  ( -2.177166869458664333, -11.04252011169590020, 33.62494198852677130 ) ) ;
#45617=VERTEX_POINT ( 'NONE', #17082 ) ;
#45619=VERTEX_POINT ( 'NONE', #58061 ) ;
#45620=CARTESIAN_POINT ( 'NONE',  ( 8.639083559792549494, -12.45813303252208648, 30.39737893381572675 ) ) ;
#45621=B_SPLINE_CURVE_WITH_KNOTS ( 'NONE', 3,
 ( #57862, #30831, #24517, #24076, #51985, #79481, #9674, #51523, #44782, #3807 ),
 .UNSPECIFIED., .F., .F.,
 ( 4, 2, 2, 2, 4 ),
 ( 0.000000000000000000, 0.0001954339857564125972, 0.0003908679715128181471, 0.0005863019572692237513, 0.0007817359430256293554 ),
 .UNSPECIFIED. ) ;
#45622=FACE_OUTER_BOUND ( 'NONE', #75659, .T. ) ;
#45623=DIRECTION ( 'NONE',  ( 0.000000000000000000, 0.4999999999999960032, -0.8660254037844410391 ) ) ;
#45624=DIRECTION ( 'NONE',  ( 0.000000000000000000, 0.6427876096865368094, 0.7660444431189802339 ) ) ;
#45625=CARTESIAN_POINT ( 'NONE',  ( -9.692307692307691624, -6.343179335718451384, 34.87096338111211935 ) ) ;
#45626=CARTESIAN_POINT ( 'NONE',  ( 9.469381474791545017, -8.239355502252617924, 34.69524867566427417 ) ) ;
#45627=ADVANCED_FACE ( 'NONE', ( #44536 ), #3560, .F. ) ;
#45628=VERTEX_POINT ( 'NONE', #43663 ) ;
#45629=ORIENTED_EDGE ( 'NONE', *, *, #46126, .F. ) ;
#45630=EDGE_LOOP ( 'NONE', ( #55689, #64999, #7247, #24843, #32043, #64819 ) ) ;
#45631=B_SPLINE_CURVE_WITH_KNOTS ( 'NONE', 3,
 ( #31305, #36293, #2051, #2484, #77709, #65524, #36726, #37609, #58770, #86269 ),
 .UNSPECIFIED., .F., .F.,
 ( 4, 2, 2, 2, 4 ),
 ( 0.0007817359430256294638, 0.0009771253907249952391, 0.001172514838424361123, 0.001367904286123726790, 0.001563293733823092673 ),
 .UNSPECIFIED. ) ;
#45633=EDGE_CURVE ( 'NONE', #3517, #77110, #81923, .T. ) ;
#45634=ORIENTED_EDGE ( 'NONE', *, *, #42408, .T. ) ;
#45635=VERTEX_POINT ( 'NONE', #24729 ) ;
#45636=CARTESIAN_POINT ( 'NONE',  ( 12.46153846153833911, -11.94971097300221174, 32.03036669348237098 ) ) ;
#45637=DIRECTION ( 'NONE',  ( -0.000000000000000000, -0.1736481776669307198, -0.9848077530122080203 ) ) ;
#45638=EDGE_CURVE ( 'NONE', #75555, #74750, #58279, .T. ) ;
#45639=CARTESIAN_POINT ( 'NONE',  ( -10.36533019547116119, -4.818054556918156983, 34.26375889529406749 ) ) ;
#45640=EDGE_CURVE ( 'NONE', #54013, #82892, #27201, .T. ) ;
#45641=CARTESIAN_POINT ( 'NONE',  ( -7.173053654019276415, -3.137211980971221781, 32.19342716148376837 ) ) ;
#45642=CARTESIAN_POINT ( 'NONE',  ( 13.16168916709923664, -8.239355502252617924, 34.69524867566427417 ) ) ;
#45643=CARTESIAN_POINT ( 'NONE',  ( -6.000000000000121680, -3.083524468854526912, 32.58852847137268327 ) ) ;
#45644=CARTESIAN_POINT ( 'NONE',  ( -0.4615384615385826339, -11.94971097300221174, 32.03036669348237098 ) ) ;
#45645=CARTESIAN_POINT ( 'NONE',  ( 16.82692307692307665, -2.249999999999998668, 29.75000000000000355 ) ) ;
#45646=LINE ( 'NONE', #18182, #64820 ) ;
#45647=EDGE_LOOP ( 'NONE', ( #12770, #57941 ) ) ;
#45648=VERTEX_POINT ( 'NONE', #52190 ) ;
#45649=VERTEX_POINT ( 'NONE', #72466 ) ;
#45650=CARTESIAN_POINT ( 'NONE',  ( 11.60371667797437212, -2.657715359629132301, 31.77849191805844242 ) ) ;
#45651=ORIENTED_EDGE ( 'NONE', *, *, #36861, .F. ) ;
#45652=CARTESIAN_POINT ( 'NONE',  ( 7.846153846153725020, -3.300289026999228881, 32.46337939537708905 ) ) ;
#45653=CARTESIAN_POINT ( 'NONE',  ( 18.13004505591977278, -2.254550872974305342, 29.97347326024528158 ) ) ;
#45655=CARTESIAN_POINT ( 'NONE',  ( 4.376625695114562120, -2.600157965045225339, 30.74683119005207743 ) ) ;
#45656=FACE_BOUND ( 'NONE', #25210, .T. ) ;
#45657=EDGE_LOOP ( 'NONE', ( #81753, #62782, #65367, #51904 ) ) ;
#45658=VERTEX_POINT ( 'NONE', #44092 ) ;
#45659=CARTESIAN_POINT ( 'NONE',  ( -17.32694630114453105, -11.56360843649121861, 33.07473185843129926 ) ) ;
#45660=VECTOR ( 'NONE', #83313, 1000.000000000000114 ) ;
#45661=VERTEX_POINT ( 'NONE', #10329 ) ;
#45662=FACE_BOUND ( 'NONE', #82199, .T. ) ;
#45663=CYLINDRICAL_SURFACE ( 'NONE', #72026, 0.2499999999999998890 ) ;
#45664=CARTESIAN_POINT ( 'NONE',  ( -16.15384615384615330, -2.486705287966279876, 31.30864560766543647 ) ) ;
#45665=VERTEX_POINT ( 'NONE', #37796 ) ;
#45666=CARTESIAN_POINT ( 'NONE',  ( -1.318548051265308274, -5.471508081941601098, 34.59228464037088457 ) ) ;
#45667=LINE ( 'NONE', #46560, #54746 ) ;
#45668=CARTESIAN_POINT ( 'NONE',  ( 6.000000000000001776, -1.215029322943914858, 32.30358669280327177 ) ) ;
#45669=EDGE_LOOP ( 'NONE', ( #68975, #6071 ) ) ;
#45670=LINE ( 'NONE', #16866, #85965 ) ;
#45673=VERTEX_POINT ( 'NONE', #44986 ) ;
#45674=CARTESIAN_POINT ( 'NONE',  ( -2.373775718648186039, -11.16473453929635440, 33.15142922261925662 ) ) ;
#45675=CARTESIAN_POINT ( 'NONE',  ( 7.053602624840488389, -10.88167719472716399, 33.43325721877153711 ) ) ;
#45676=B_SPLINE_CURVE_WITH_KNOTS ( 'NONE', 3,
 ( #22791, #57912, #16047, #84956, #23681, #63340, #51132, #43516, #85394, #71418 ),
 .UNSPECIFIED., .F., .F.,
 ( 4, 2, 2, 2, 4 ),
 ( 0.0007817246256747452209, 0.0009771112852218887673, 0.001172497944769032531, 0.001367884604316176294, 0.001563271263863319840 ),
 .UNSPECIFIED. ) ;
#45677=ORIENTED_EDGE ( 'NONE', *, *, #81732, .F. ) ;
#45678=CARTESIAN_POINT ( 'NONE',  ( 2.307692307692186251, -11.67786785259630911, 32.92929555188603530 ) ) ;
#45679=FACE_OUTER_BOUND ( 'NONE', #40996, .T. ) ;
#45680=CARTESIAN_POINT ( 'NONE',  ( -16.02332045208259359, -8.586989748646450593, 34.63063291749215011 ) ) ;
#45681=CARTESIAN_POINT ( 'NONE',  ( 15.10062126103753855, -12.70455904226513866, 30.44083106164009322 ) ) ;
#45682=CARTESIAN_POINT ( 'NONE',  ( 5.076923076923075762, -12.37446782046654192, 30.86335684631486131 ) ) ;
#45683=B_SPLINE_CURVE_WITH_KNOTS ( 'NONE', 3,
 ( #67287, #81692, #597, #55532, #40263, #67728, #68606, #75804, #27621, #54196 ),
 .UNSPECIFIED., .F., .F.,
 ( 4, 2, 2, 2, 4 ),
 ( 0.0007817246256747485819, 0.0009771112852218918031, 0.001172497944769034916, 0.001367884604316178029, 0.001563271263863321358 ),
 .UNSPECIFIED. ) ;
#45685=CARTESIAN_POINT ( 'NONE',  ( 2.307692307692309264, -12.29105614889573062, 35.45975837776705220 ) ) ;
#45686=CARTESIAN_POINT ( 'NONE',  ( -1.384615384615506484, -8.656820664282941280, 34.87096338111179961 ) ) ;
#45687=CARTESIAN_POINT ( 'NONE',  ( -3.480792468062195333, -2.587272538249755449, 30.68239716806877837 ) ) ;
#45688=CARTESIAN_POINT ( 'NONE',  ( -15.16551409125639083, -2.657715359629131857, 31.77849191805844242 ) ) ;
#45689=CARTESIAN_POINT ( 'NONE',  ( -8.519230769230768274, -2.249999999999998668, 29.75000000000000355 ) ) ;
#45691=ORIENTED_EDGE ( 'NONE', *, *, #50911, .T. ) ;
#45692=CARTESIAN_POINT ( 'NONE',  ( 17.77651505627605033, -4.386631170607603991, 33.66268669641500111 ) ) ;
#45693=VERTEX_POINT ( 'NONE', #31028 ) ;
#45695=ORIENTED_EDGE ( 'NONE', *, *, #52253, .T. ) ;
#45696=CARTESIAN_POINT ( 'NONE',  ( -12.71153846153846168, -2.499999999999998668, 29.75000000000000355 ) ) ;
#45697=VERTEX_POINT ( 'NONE', #10773 ) ;
#45698=CARTESIAN_POINT ( 'NONE',  ( -15.09997742294444478, -5.582136614379148654, 34.36778462344220486 ) ) ;
#45701=CARTESIAN_POINT ( 'NONE',  ( -18.06608237936013239, -11.91647553114624358, 32.58852847137148245 ) ) ;
#45702=DIRECTION ( 'NONE',  ( -0.000000000000000000, -0.8660254037844399289, -0.4999999999999980016 ) ) ;
#45703=CARTESIAN_POINT ( 'NONE',  ( 7.846153846153723244, -11.06231777344772027, 33.60647404775119895 ) ) ;
#45705=CARTESIAN_POINT ( 'NONE',  ( -8.519285250882628446, -5.057305518903948638, 34.11320923018887896 ) ) ;
#45707=CARTESIAN_POINT ( 'NONE',  ( -24.00000000000000000, -5.499999999999981348, 27.75000000000000000 ) ) ;
#45709=CARTESIAN_POINT ( 'NONE',  ( 5.326977496836527770, -2.920487667080175154, 32.31805714834170828 ) ) ;
#45710=CARTESIAN_POINT ( 'NONE',  ( -16.15384615384615330, -2.538708090699994813, 30.37095296980875503 ) ) ;
#45711=AXIS2_PLACEMENT_3D ( 'NONE', #5284, #5725, #88173 ) ;
#45712=CARTESIAN_POINT ( 'NONE',  ( 6.923076923076924238, -11.91647553114624181, 32.58852847137148245 ) ) ;
#45713=ADVANCED_FACE ( 'NONE', ( #38243 ), #31486, .F. ) ;
#45714=B_SPLINE_CURVE_WITH_KNOTS ( 'NONE', 3,
 ( #48158, #14835, #54926, #20259, #60792, #68006, #20695, #28332, #13934, #27015 ),
 .UNSPECIFIED., .F., .F.,
 ( 4, 2, 2, 2, 4 ),
 ( 0.000000000000000000, 0.0001954311564186876063, 0.0003908623128373752125, 0.0005862934692560628188, 0.0007817246256747504250 ),
 .UNSPECIFIED. ) ;
#45716=ORIENTED_EDGE ( 'NONE', *, *, #48862, .F. ) ;
#45717=CARTESIAN_POINT ( 'NONE',  ( -8.835314180186648159, -12.37446782046654192, 30.86335684631486487 ) ) ;
#45718=CYLINDRICAL_SURFACE ( 'NONE', #4295, 0.2500000000000004996 ) ;
#45719=CARTESIAN_POINT ( 'NONE',  ( -2.557669051740897537, -2.318417181685854533, 30.59732222474233865 ) ) ;
#45720=FACE_OUTER_BOUND ( 'NONE', #2626, .T. ) ;
#45721=B_SPLINE_CURVE_WITH_KNOTS ( 'NONE', 3,
 ( #36370, #76911, #57959, #44426, #8459, #15216, #57072, #42688, #49870, #78678 ),
 .UNSPECIFIED., .F., .F.,
 ( 4, 2, 2, 2, 4 ),
 ( 0.0007817359430256399806, 0.0009771253907250089001, 0.001172514838424378036, 0.001367904286123746956, 0.001563293733823115875 ),
 .UNSPECIFIED. ) ;
#45722=DIRECTION ( 'NONE',  ( 0.000000000000000000, 0.9848077530122072432, -0.1736481776669354937 ) ) ;
#45723=CARTESIAN_POINT ( 'NONE',  ( -9.822998295418001291, -6.369640206132551441, 34.87707690430378449 ) ) ;
#45724=B_SPLINE_CURVE_WITH_KNOTS ( 'NONE', 3,
 ( #76848, #57002, #84496, #22772, #69634, #64192, #83618, #2496, #21895, #29987 ),
 .UNSPECIFIED., .F., .F.,
 ( 4, 2, 2, 2, 4 ),
 ( 0.0007817246256747451124, 0.0009771112852218881168, 0.001172497944769031230, 0.001367884604316174126, 0.001563271263863317238 ),
 .UNSPECIFIED. ) ;
#45725=VECTOR ( 'NONE', #30819, 1000.000000000000114 ) ;
#45726=EDGE_CURVE ( 'NONE', #72078, #78012, #61470, .T. ) ;
#45728=CARTESIAN_POINT ( 'NONE',  ( -6.700297381808513641, -10.11255958852956027, 34.01340905677048454 ) ) ;
#45729=VERTEX_POINT ( 'NONE', #19751 ) ;
#45730=AXIS2_PLACEMENT_3D ( 'NONE', #76563, #76109, #28827 ) ;
#45731=ORIENTED_EDGE ( 'NONE', *, *, #5592, .F. ) ;
#45732=CARTESIAN_POINT ( 'NONE',  ( 0.5267936010512997980, -12.51329471203373700, 31.30864560766537963 ) ) ;
#45734=CARTESIAN_POINT ( 'NONE',  ( 9.915319043920545639, -12.15243808032445827, 31.58219941686247978 ) ) ;
#45735=DIRECTION ( 'NONE',  ( 0.000000000000000000, 0.000000000000000000, 1.000000000000000000 ) ) ;
#45738=VERTEX_POINT ( 'NONE', #73364 ) ;
#45739=EDGE_CURVE ( 'NONE', #65392, #42328, #36752, .T. ) ;
#45740=EDGE_CURVE ( 'NONE', #78212, #78525, #8850, .T. ) ;
#45741=VERTEX_POINT ( 'NONE', #26066 ) ;
#45742=CARTESIAN_POINT ( 'NONE',  ( -7.173100147298381302, -12.07920672191015221, 32.31858351112116168 ) ) ;
#45743=B_SPLINE_CURVE_WITH_KNOTS ( 'NONE', 3,
 ( #29232, #49495, #28783, #36852, #64754, #16145, #35983, #85491, #84181, #36424 ),
 .UNSPECIFIED., .F., .F.,
 ( 4, 2, 2, 2, 4 ),
 ( 0.0007817359430256315238, 0.0009771253907249980580, 0.001172514838424364592, 0.001367904286123731127, 0.001563293733823097661 ),
 .UNSPECIFIED. ) ;
#45745=CARTESIAN_POINT ( 'NONE',  ( 4.219913487196228274, -3.322132147404559976, 32.92929555188717927 ) ) ;
#45747=EDGE_CURVE ( 'NONE', #68539, #9053, #86227, .T. ) ;
#45748=VECTOR ( 'NONE', #17321, 1000.000000000000114 ) ;
#45749=CARTESIAN_POINT ( 'NONE',  ( -4.219170166650461518, -7.749976730030849303, 34.74374725381503737 ) ) ;
#45750=CARTESIAN_POINT ( 'NONE',  ( 5.869852790561782108, -12.45813303252208648, 30.39737893381572675 ) ) ;
#45751=EDGE_LOOP ( 'NONE', ( #62022, #56141 ) ) ;
#45752=EDGE_CURVE ( 'NONE', #57312, #70118, #22878, .T. ) ;
#45753=EDGE_LOOP ( 'NONE', ( #1896, #60335, #3611, #70117 ) ) ;
#45754=CARTESIAN_POINT ( 'NONE',  ( 11.78846153846154010, -2.499999999999998668, 29.75000000000000355 ) ) ;
#45756=CARTESIAN_POINT ( 'NONE',  ( 15.23076923076923173, -5.557115091759785130, 34.35708131394839171 ) ) ;
#45757=ORIENTED_EDGE ( 'NONE', *, *, #75798, .T. ) ;
#45758=LINE ( 'NONE', #4781, #23455 ) ;
#45759=CARTESIAN_POINT ( 'NONE',  ( -2.307692307692428724, -4.320704448113951379, 33.92786785259630022 ) ) ;
#45760=CARTESIAN_POINT ( 'NONE',  ( -3.230769230769229949, -9.780366693483667717, 34.19971097300155094 ) ) ;
#45761=ORIENTED_EDGE ( 'NONE', *, *, #59037, .F. ) ;
#45762=AXIS2_PLACEMENT_3D ( 'NONE', #48925, #83620, #76850 ) ;
#45763=CARTESIAN_POINT ( 'NONE',  ( 10.74617505635156789, -2.295524264805589354, 30.44142389570982488 ) ) ;
#45764=VERTEX_POINT ( 'NONE', #66613 ) ;
#45767=CARTESIAN_POINT ( 'NONE',  ( 7.622668921589514923, -4.225889041578354544, 33.85425143139329407 ) ) ;
#45768=CARTESIAN_POINT ( 'NONE',  ( -6.857008572074484221, -12.37446782046654192, 30.86335684631486842 ) ) ;
#45769=CYLINDRICAL_SURFACE ( 'NONE', #22783, 0.2499999999999995559 ) ;
#45771=ORIENTED_EDGE ( 'NONE', *, *, #64704, .T. ) ;
#45772=CARTESIAN_POINT ( 'NONE',  ( 0.4615384615384611200, -2.292212530054420494, 30.41441678777542634 ) ) ;
#45773=CARTESIAN_POINT ( 'NONE',  ( 11.31559527539844190, -2.251424796025574881, 29.88072029997477230 ) ) ;
#45774=CYLINDRICAL_SURFACE ( 'NONE', #645, 0.2500000000000002220 ) ;
#45775=ORIENTED_EDGE ( 'NONE', *, *, #86211, .T. ) ;
#45777=CARTESIAN_POINT ( 'NONE',  ( -6.066083410955878108, -10.51840700105979387, 33.73612834413961536 ) ) ;
#45779=CARTESIAN_POINT ( 'NONE',  ( 10.55011416942383917, -11.94971097300153140, 32.03036669348370680 ) ) ;
#45780=FACE_BOUND ( 'NONE', #40220, .T. ) ;
#45781=CARTESIAN_POINT ( 'NONE',  ( 12.33139125210024112, -3.285722584762969856, 32.44110544564090759 ) ) ;
#45782=CARTESIAN_POINT ( 'NONE',  ( -1.384615384615383471, -8.120952969808772792, 34.71129190930000163 ) ) ;
#45783=CARTESIAN_POINT ( 'NONE',  ( -9.626240358957616650, -11.91647553114624358, 32.58852847137148245 ) ) ;
#45784=CARTESIAN_POINT ( 'NONE',  ( -1.134669866267241423, -12.22109172314383052, 31.39792113162168263 ) ) ;
#45785=CARTESIAN_POINT ( 'NONE',  ( 14.05771556364371833, -10.82459398097509329, 33.81372124010185587 ) ) ;
#45786=CARTESIAN_POINT ( 'NONE',  ( -3.930833309752758797, -10.77377354290276301, 33.85451476688484718 ) ) ;
#45787=CARTESIAN_POINT ( 'NONE',  ( 13.13459216039392707, -2.588893531581426988, 31.60682220781847818 ) ) ;
#45788=AXIS2_PLACEMENT_3D ( 'NONE', #56844, #84340, #84783 ) ;
#45790=CARTESIAN_POINT ( 'NONE',  ( -8.638705067467205012, -6.001044277235009439, 34.52024696741798948 ) ) ;
#45792=CARTESIAN_POINT ( 'NONE',  ( 0.2380535178145125608, -6.760086850603068243, 34.69517049084099369 ) ) ;
#45795=CARTESIAN_POINT ( 'NONE',  ( -2.437839517130528044, -11.93770438780619259, 32.05411857736982029 ) ) ;
#45796=CARTESIAN_POINT ( 'NONE',  ( -17.01166793741023042, -2.379036618887895305, 30.90682066428158592 ) ) ;
#45797=CARTESIAN_POINT ( 'NONE',  ( 6.130525438233648039, -3.625058011473227815, 33.29252011169590020 ) ) ;
#45799=EDGE_CURVE ( 'NONE', #60707, #58077, #6673, .T. ) ;
#45800=CARTESIAN_POINT ( 'NONE',  ( -9.692307692307814193, -3.643525952248795718, 33.31231777344771672 ) ) ;
#45801=CYLINDRICAL_SURFACE ( 'NONE', #40331, 0.2499999999999997502 ) ;
#45802=CARTESIAN_POINT ( 'NONE',  ( -12.46153846153846168, -9.058645607665452459, 34.76329471203371924 ) ) ;
#45803=CARTESIAN_POINT ( 'NONE',  ( 5.076923076923075762, -9.058645607665452459, 34.76329471203371924 ) ) ;
#45804=CARTESIAN_POINT ( 'NONE',  ( 14.43821800945587519, -6.001044277235009439, 34.52024696741798948 ) ) ;
#45806=CARTESIAN_POINT ( 'NONE',  ( -2.057692307692291500, -2.249999999999999112, 29.81603969181031033 ) ) ;
#45807=CARTESIAN_POINT ( 'NONE',  ( -11.40766973063675493, -10.54018710029568595, 33.71981072465678864 ) ) ;
#45808=ORIENTED_EDGE ( 'NONE', *, *, #26817, .F. ) ;
#45809=CARTESIAN_POINT ( 'NONE',  ( 17.20771488474786182, -2.729792928343269587, 31.24908615093345077 ) ) ;
#45810=CARTESIAN_POINT ( 'NONE',  ( 8.769230769230768274, -11.16473453929635440, 33.15142922261926373 ) ) ;
#45813=CARTESIAN_POINT ( 'NONE',  ( 0.4615384615384611200, -3.513871655860378418, 32.76840700105978499 ) ) ;
#45814=AXIS2_PLACEMENT_3D ( 'NONE', #10910, #3254, #11349 ) ;
#45815=CARTESIAN_POINT ( 'NONE',  ( 17.20771488474786537, -11.71459661697925903, 32.44059661609676937 ) ) ;
#45816=ORIENTED_EDGE ( 'NONE', *, *, #16777, .F. ) ;
#45817=CARTESIAN_POINT ( 'NONE',  ( -3.230769230769229949, -1.117168528481311540, 33.14645433367849847 ) ) ;
#45818=LINE ( 'NONE', #73300, #87711 ) ;
#45819=CARTESIAN_POINT ( 'NONE',  ( -1.384615384615506484, -3.083524468854526912, 32.58852847137268327 ) ) ;
#45820=ORIENTED_EDGE ( 'NONE', *, *, #79541, .F. ) ;
#45821=CARTESIAN_POINT ( 'NONE',  ( -11.53846153846123102, -2.506253911140614576, 30.00000000000323297 ) ) ;
#45822=CARTESIAN_POINT ( 'NONE',  ( 12.59233026936325039, -12.38066358083363738, 30.83685684665853444 ) ) ;
#45824=DIRECTION ( 'NONE',  ( -0.000000000000000000, -0.1736481776669307198, -0.9848077530122080203 ) ) ;
#45825=DIRECTION ( 'NONE',  ( -0.000000000000000000, -0.6427876096865404731, -0.7660444431189771253 ) ) ;
#45826=EDGE_LOOP ( 'NONE', ( #88189, #15525 ) ) ;
#45827=CARTESIAN_POINT ( 'NONE',  ( 2.372947878968333590, -12.27809138561124591, 31.22303859784720359 ) ) ;
#45828=DIRECTION ( 'NONE',  ( -0.000000000000000000, 0.9396926207859092051, -0.3420201433256662704 ) ) ;
#45829=LINE ( 'NONE', #31436, #34100 ) ;
#45832=ORIENTED_EDGE ( 'NONE', *, *, #71929, .T. ) ;
#45833=VERTEX_POINT ( 'NONE', #49869 ) ;
#45834=ADVANCED_FACE ( 'NONE', ( #13872 ), #803, .F. ) ;
#45835=CARTESIAN_POINT ( 'NONE',  ( -9.692307692307691624, -6.435427911321262684, 35.78748833219616898 ) ) ;
#45836=CARTESIAN_POINT ( 'NONE',  ( -3.230769230769229949, -2.833524468853757305, 32.15551576947925838 ) ) ;
#45837=CARTESIAN_POINT ( 'NONE',  ( -12.46153846153846168, -3.513871655860378418, 32.76840700105978499 ) ) ;
#45838=B_SPLINE_CURVE_WITH_KNOTS ( 'NONE', 3,
 ( #2858, #22265, #56049, #43425, #85303, #83984, #37537, #49731, #23585, #63687 ),
 .UNSPECIFIED., .F., .F.,
 ( 4, 2, 2, 2, 4 ),
 ( 0.000000000000000000, 0.0001954311564186868473, 0.0003908623128373736946, 0.0005862934692560605419, 0.0007817246256747473893 ),
 .UNSPECIFIED. ) ;
#45842=ORIENTED_EDGE ( 'NONE', *, *, #59827, .F. ) ;
#45843=CARTESIAN_POINT ( 'NONE',  ( 11.60371667797437567, -11.67786785259547777, 32.92929555188713664 ) ) ;
#45844=EDGE_CURVE ( 'NONE', #51826, #71762, #14270, .T. ) ;
#45846=CARTESIAN_POINT ( 'NONE',  ( -5.326946301144536378, -2.588893531581426544, 31.60682220781847818 ) ) ;
#45848=CARTESIAN_POINT ( 'NONE',  ( -3.480745974817821775, -4.818429247618089661, 34.26397095200675125 ) ) ;
#45849=ADVANCED_FACE ( 'NONE', ( #69704 ), #34593, .F. ) ;
#45850=EDGE_CURVE ( 'NONE', #67493, #28342, #7123, .T. ) ;
#45851=FACE_OUTER_BOUND ( 'NONE', #12186, .T. ) ;
#45852=CARTESIAN_POINT ( 'NONE',  ( 13.45068271796546178, -9.905515769479276145, 34.41647553114623292 ) ) ;
#45853=ORIENTED_EDGE ( 'NONE', *, *, #12099, .F. ) ;
#45854=ORIENTED_EDGE ( 'NONE', *, *, #58953, .F. ) ;
#45855=EDGE_LOOP ( 'NONE', ( #39984, #11788 ) ) ;
#45856=CARTESIAN_POINT ( 'NONE',  ( 15.16549878480846125, -2.625532179533445198, 30.86335684631481513 ) ) ;
#45857=EDGE_LOOP ( 'NONE', ( #83413, #13921, #48465, #74883 ) ) ;
#45858=CARTESIAN_POINT ( 'NONE',  ( 2.177001704582003594, -2.494641256782728966, 31.33461815524612959 ) ) ;
#45859=CARTESIAN_POINT ( 'NONE',  ( -0.2387587925603958106, -4.989023458446561143, 34.36081565061822118 ) ) ;
#45860=CARTESIAN_POINT ( 'NONE',  ( -9.019254006523732770, -10.76384336483936011, 33.53834819971076087 ) ) ;
#45861=CARTESIAN_POINT ( 'NONE',  ( 10.61538461538461675, -12.09954503811598769, 35.62045528018868623 ) ) ;
#45862=CARTESIAN_POINT ( 'NONE',  ( -2.057637996053991891, -11.28795663066794219, 33.01431243580653785 ) ) ;
#45863=FACE_BOUND ( 'NONE', #59007, .T. ) ;
#45864=CARTESIAN_POINT ( 'NONE',  ( 15.23076923076923173, -5.557115091759785130, 34.35708131394839171 ) ) ;
#45865=CARTESIAN_POINT ( 'NONE',  ( 17.07692307692307665, -12.09954503811598769, 35.62045528018868623 ) ) ;
#45866=CARTESIAN_POINT ( 'NONE',  ( -7.976301055592070810, -12.27039167877662251, 31.24851455888617835 ) ) ;
#45867=CARTESIAN_POINT ( 'NONE',  ( 16.21991348719623005, -3.937682226553329556, 33.60647404775216529 ) ) ;
#45868=CARTESIAN_POINT ( 'NONE',  ( -5.207614543590636913, -3.062553014421049546, 32.05460306192773601 ) ) ;
#45869=AXIS2_PLACEMENT_3D ( 'NONE', #55147, #82645, #34877 ) ;
#45870=LINE ( 'NONE', #88669, #23670 ) ;
#45872=ORIENTED_EDGE ( 'NONE', *, *, #819, .T. ) ;
#45873=CARTESIAN_POINT ( 'NONE',  ( 11.28848480751918437, -3.137211980971221781, 32.19342716148376837 ) ) ;
#45874=CARTESIAN_POINT ( 'NONE',  ( -7.846153846153844924, -6.435427911321262684, 35.78748833219616898 ) ) ;
#45875=ORIENTED_EDGE ( 'NONE', *, *, #7511, .T. ) ;
#45876=ORIENTED_EDGE ( 'NONE', *, *, #6509, .T. ) ;
#45878=CARTESIAN_POINT ( 'NONE',  ( 5.999999999999880096, -6.879047030192662504, 34.71129190930017927 ) ) ;
#45879=CYLINDRICAL_SURFACE ( 'NONE', #40531, 0.2500000000000008882 ) ;
#45880=VECTOR ( 'NONE', #82818, 1000.000000000000114 ) ;
#45881=CARTESIAN_POINT ( 'NONE',  ( 16.28463796167094202, -2.541949514083464479, 30.39797389878540557 ) ) ;
#45882=CARTESIAN_POINT ( 'NONE',  ( -13.38461538461538325, -4.661471528628507777, 34.16647553114623292 ) ) ;
#45883=CARTESIAN_POINT ( 'NONE',  ( 12.39545608217832218, -10.67929555188718460, 33.92786785259543336 ) ) ;
#45884=ORIENTED_EDGE ( 'NONE', *, *, #5857, .T. ) ;
#45887=CARTESIAN_POINT ( 'NONE',  ( 18.13079044096695469, -2.494656445102014342, 31.33466734024120015 ) ) ;
#45888=FACE_OUTER_BOUND ( 'NONE', #9995, .T. ) ;
#45889=CARTESIAN_POINT ( 'NONE',  ( 15.23076923076911093, -12.27809138561165270, 31.22303859784587132 ) ) ;
#45890=CARTESIAN_POINT ( 'NONE',  ( 17.07692307692307665, -6.386643153685126251, 34.62446782046654192 ) ) ;
#45891=CARTESIAN_POINT ( 'NONE',  ( 0.6845513056318550671, -4.762714258010882773, 34.23016756924214832 ) ) ;
#45892=CARTESIAN_POINT ( 'NONE',  ( 2.438482748659258625, -5.496552790871119143, 34.60292014791297532 ) ) ;
#45894=ORIENTED_EDGE ( 'NONE', *, *, #77281, .T. ) ;
#45896=CARTESIAN_POINT ( 'NONE',  ( 5.142178648199100977, -6.879047030191282275, 34.71129190930002295 ) ) ;
#45897=DIRECTION ( 'NONE',  ( -0.000000000000000000, -0.1736481776669307198, -0.9848077530122080203 ) ) ;
#45899=CARTESIAN_POINT ( 'NONE',  ( -14.08468095607945969, -6.503523203565941380, 34.64991518177335195 ) ) ;
#45900=CARTESIAN_POINT ( 'NONE',  ( 1.384615384615386802, -13.20930481340135110, 34.54067556320372745 ) ) ;
#45902=EDGE_CURVE ( 'NONE', #43445, #85648, #63709, .T. ) ;
#45904=DIRECTION ( 'NONE',  ( -0.000000000000000000, 0.5000000000000011102, -0.8660254037844381525 ) ) ;
#45905=CARTESIAN_POINT ( 'NONE',  ( 1.450683735617824599, -4.786620604624113540, 33.94971097300155805 ) ) ;
#45906=CARTESIAN_POINT ( 'NONE',  ( -8.769230769230892619, -12.70778746994576025, 30.41441678777401236 ) ) ;
#45907=CARTESIAN_POINT ( 'NONE',  ( 12.46153846153833911, -11.67786785259630911, 32.92929555188603530 ) ) ;
#45908=LINE ( 'NONE', #39176, #10920 ) ;
#45909=CARTESIAN_POINT ( 'NONE',  ( 13.44987052412822059, -2.657715359629132301, 31.77849191805844242 ) ) ;
#45910=CYLINDRICAL_SURFACE ( 'NONE', #19327, 0.2499999999999986955 ) ;
#45911=CARTESIAN_POINT ( 'NONE',  ( 6.989144256427000990, -2.292212530054420494, 30.41441678777542990 ) ) ;
#45912=CARTESIAN_POINT ( 'NONE',  ( -6.249976730942353065, -9.943427161483782584, 34.11278801902876978 ) ) ;
#45913=CARTESIAN_POINT ( 'NONE',  ( 23.00000000000000000, -5.499999999999981348, 27.25000000000000000 ) ) ;
#45914=VERTEX_POINT ( 'NONE', #55298 ) ;
#45915=VECTOR ( 'NONE', #17777, 1000.000000000000114 ) ;
#45916=CARTESIAN_POINT ( 'NONE',  ( 8.992010438208831502, -4.989023458446560255, 34.36081565061822118 ) ) ;
#45917=CARTESIAN_POINT ( 'NONE',  ( 20.99999999999999645, -10.75000000000000000, 29.75000000000000355 ) ) ;
#45918=CARTESIAN_POINT ( 'NONE',  ( -4.153846153846274980, -5.941354392335915335, 34.76329471203413846 ) ) ;
#45920=EDGE_CURVE ( 'NONE', #58039, #73779, #35029, .T. ) ;
#45922=CARTESIAN_POINT ( 'NONE',  ( 14.30769230769218581, -5.094484230521993062, 34.41647553114689373 ) ) ;
#45923=CARTESIAN_POINT ( 'NONE',  ( -0.2385271099256127125, -2.554770724473667709, 30.48948780036025852 ) ) ;
#45926=CARTESIAN_POINT ( 'NONE',  ( 3.361294669002875324, -8.630441415882550871, 34.87705825610312615 ) ) ;
#45927=EDGE_CURVE ( 'NONE', #43633, #28226, #15399, .T. ) ;
#45928=ORIENTED_EDGE ( 'NONE', *, *, #89077, .F. ) ;
#45929=CARTESIAN_POINT ( 'NONE',  ( -7.146003881983769901, -11.43668979543635089, 33.22377378376089752 ) ) ;
#45930=ORIENTED_EDGE ( 'NONE', *, *, #23986, .T. ) ;
#45931=CARTESIAN_POINT ( 'NONE',  ( 3.230769230769108269, -5.094484230521993062, 34.41647553114689373 ) ) ;
#45932=CARTESIAN_POINT ( 'NONE',  ( -1.384615384615383471, -11.91647553114624181, 32.58852847137148245 ) ) ;
#45933=CARTESIAN_POINT ( 'NONE',  ( -1.634592115557738312, -4.236021600441998380, 33.53823185664189310 ) ) ;
#45934=EDGE_CURVE ( 'NONE', #63430, #27372, #85882, .T. ) ;
#45935=ORIENTED_EDGE ( 'NONE', *, *, #81970, .T. ) ;
#45936=CARTESIAN_POINT ( 'NONE',  ( 6.923076923076924238, -13.53365097954675988, 30.81389545987213552 ) ) ;
#45937=VERTEX_POINT ( 'NONE', #65151 ) ;
#45938=CARTESIAN_POINT ( 'NONE',  ( -5.777220331021931443, -2.353885683473779800, 30.79025554430704759 ) ) ;
#45941=VECTOR ( 'NONE', #1003, 999.9999999999998863 ) ;
#45942=CARTESIAN_POINT ( 'NONE',  ( 2.084765348785458272, -9.172386477786396597, 34.72672124145550043 ) ) ;
#45943=CARTESIAN_POINT ( 'NONE',  ( 0.5276068125408986953, -11.16473453929635440, 33.15142922261926373 ) ) ;
#45944=CARTESIAN_POINT ( 'NONE',  ( -10.36533030374629938, -6.567000820036036579, 34.66262288849541306 ) ) ;
#45945=CARTESIAN_POINT ( 'NONE',  ( -39.05038313613820122, -2.499999999999999556, 29.75000000000000355 ) ) ;
#45946=CARTESIAN_POINT ( 'NONE',  ( 7.053867364043876265, -8.191423895709842640, 34.95447573519442130 ) ) ;
#45950=LINE ( 'NONE', #24340, #39136 ) ;
#45951=B_SPLINE_CURVE_WITH_KNOTS ( 'NONE', 3,
 ( #87617, #18255, #58333, #85829, #25002, #18707, #25899, #52471, #79955, #24107 ),
 .UNSPECIFIED., .F., .F.,
 ( 4, 2, 2, 2, 4 ),
 ( 0.000000000000000000, 0.0001954311564186865492, 0.0003908623128373730983, 0.0005862934692560596746, 0.0007817246256747461966 ),
 .UNSPECIFIED. ) ;
#45952=EDGE_CURVE ( 'NONE', #73958, #44944, #84165, .T. ) ;
#45954=ORIENTED_EDGE ( 'NONE', *, *, #66564, .F. ) ;
#45955=ORIENTED_EDGE ( 'NONE', *, *, #57448, .F. ) ;
#45957=ORIENTED_EDGE ( 'NONE', *, *, #83055, .F. ) ;
#45958=EDGE_CURVE ( 'NONE', #37534, #68628, #57958, .T. ) ;
#45959=EDGE_CURVE ( 'NONE', #70825, #58033, #62588, .T. ) ;
#45960=CARTESIAN_POINT ( 'NONE',  ( 10.48469314871705826, -4.809359713505814149, 33.96456829005828837 ) ) ;
#45961=CARTESIAN_POINT ( 'NONE',  ( 1.515407192440170636, -2.729792928343270031, 31.24908615093345432 ) ) ;
#45962=ORIENTED_EDGE ( 'NONE', *, *, #57618, .F. ) ;
#45963=CARTESIAN_POINT ( 'NONE',  ( -14.08491276642389423, -4.387253974876679230, 33.66317474335728832 ) ) ;
#45964=ORIENTED_EDGE ( 'NONE', *, *, #85260, .T. ) ;
#45965=CARTESIAN_POINT ( 'NONE',  ( 0.4615384615387678746, -2.506253911140615021, 30.00000000000323297 ) ) ;
#45966=ORIENTED_EDGE ( 'NONE', *, *, #51582, .F. ) ;
#45967=DIRECTION ( 'NONE',  ( -0.000000000000000000, 0.1736481776669307198, -0.9848077530122080203 ) ) ;
#45968=CARTESIAN_POINT ( 'NONE',  ( -7.976845312821407852, -2.541943142973491554, 30.39792223712631980 ) ) ;
#45971=CARTESIAN_POINT ( 'NONE',  ( -14.30769230769242739, -11.94971097300221174, 32.03036669348237098 ) ) ;
#45972=FACE_BOUND ( 'NONE', #76779, .T. ) ;
#45973=CARTESIAN_POINT ( 'NONE',  ( 17.14217821643591932, -6.835583212224605631, 34.95778746994559327 ) ) ;
#45975=DIRECTION ( 'NONE',  ( -0.000000000000000000, -0.3420201433256694901, -0.9396926207859082059 ) ) ;
#45976=CYLINDRICAL_SURFACE ( 'NONE', #14371, 0.2499999999999986955 ) ;
#45977=EDGE_CURVE ( 'NONE', #13581, #56689, #6765, .T. ) ;
#45978=CARTESIAN_POINT ( 'NONE',  ( 10.48477425576008848, -7.722926236386453702, 34.74524107206102030 ) ) ;
#45979=CARTESIAN_POINT ( 'NONE',  ( 17.32697738856138869, -9.148310452688871663, 34.47095581063188519 ) ) ;
#45981=CYLINDRICAL_SURFACE ( 'NONE', #37392, 0.2500000000000012212 ) ;
#45982=ORIENTED_EDGE ( 'NONE', *, *, #8433, .F. ) ;
#45983=ORIENTED_EDGE ( 'NONE', *, *, #61951, .F. ) ;
#45984=CARTESIAN_POINT ( 'NONE',  ( 5.934729999443680626, -12.16647553114622049, 32.15551576947930812 ) ) ;
#45985=DIRECTION ( 'NONE',  ( 0.000000000000000000, 0.8660254037844377084, -0.5000000000000015543 ) ) ;
#45986=B_SPLINE_CURVE_WITH_KNOTS ( 'NONE', 3,
 ( #26965, #81474, #75157, #34154, #27843, #41361, #68827, #55308, #7577, #16428 ),
 .UNSPECIFIED., .F., .F.,
 ( 4, 2, 2, 2, 4 ),
 ( 0.000000000000000000, 0.0001954339857564079623, 0.0003908679715128159245, 0.0005863019572692238597, 0.0007817359430256318490 ),
 .UNSPECIFIED. ) ;
#45987=CARTESIAN_POINT ( 'NONE',  ( -17.07692307692319744, -3.643525952248796163, 33.31231777344771672 ) ) ;
#45988=CARTESIAN_POINT ( 'NONE',  ( -3.903791842207837259, -4.235687564193446164, 33.53795663066793509 ) ) ;
#45990=CARTESIAN_POINT ( 'NONE',  ( -2.241623956689868358, -2.721908614388771852, 31.22303859784725333 ) ) ;
#45991=EDGE_LOOP ( 'NONE', ( #33562, #62833, #41406, #85993 ) ) ;
#45992=EDGE_CURVE ( 'NONE', #43517, #59172, #24945, .T. ) ;
#45993=CARTESIAN_POINT ( 'NONE',  ( 13.38461538461538680, -9.819645486525091727, 36.12317359536749706 ) ) ;
#45994=CARTESIAN_POINT ( 'NONE',  ( -4.853911725310227077, -2.554770724473668153, 30.48948780036025852 ) ) ;
#45995=CARTESIAN_POINT ( 'NONE',  ( -14.43838377435986864, -8.147922237126337563, 34.70805685702651999 ) ) ;
#45996=AXIS2_PLACEMENT_3D ( 'NONE', #68573, #69017, #28033 ) ;
#45997=CARTESIAN_POINT ( 'NONE',  ( 13.13459214732242408, -12.43535235679832596, 30.55408501211184813 ) ) ;
#45999=EDGE_CURVE ( 'NONE', #56065, #44047, #17462, .T. ) ;
#46000=ORIENTED_EDGE ( 'NONE', *, *, #70440, .T. ) ;
#46004=EDGE_CURVE ( 'NONE', #765, #79986, #77605, .T. ) ;
#46006=CARTESIAN_POINT ( 'NONE',  ( -13.13456107297706588, -10.66356715214248396, 33.62249196103329751 ) ) ;
#46007=VERTEX_POINT ( 'NONE', #38583 ) ;
#46008=CARTESIAN_POINT ( 'NONE',  ( -16.02305434602136103, -4.809403383903226192, 33.96459661697924304 ) ) ;
#46009=CARTESIAN_POINT ( 'NONE',  ( -5.326946314216042921, -2.823816976329319495, 31.52131813110795733 ) ) ;
#46010=CARTESIAN_POINT ( 'NONE',  ( -7.846153846153844924, -11.69971097300155272, 32.46337939537588113 ) ) ;
#46013=AXIS2_PLACEMENT_3D ( 'NONE', #17637, #30692, #42559 ) ;
#46014=EDGE_CURVE ( 'NONE', #40406, #53195, #41074, .T. ) ;
#46015=DIRECTION ( 'NONE',  ( 0.000000000000000000, 1.000000000000000000, 0.000000000000000000 ) ) ;
#46016=ORIENTED_EDGE ( 'NONE', *, *, #45726, .F. ) ;
#46017=AXIS2_PLACEMENT_3D ( 'NONE', #58783, #86285, #25001 ) ;
#46021=LINE ( 'NONE', #32958, #24017 ) ;
#46022=B_SPLINE_CURVE_WITH_KNOTS ( 'NONE', 3,
 ( #21220, #954, #63533, #70300, #36944, #84277, #84720, #63084, #69858, #49585 ),
 .UNSPECIFIED., .F., .F.,
 ( 4, 2, 2, 2, 4 ),
 ( 0.0007817246256747442451, 0.0009771112852218868158, 0.001172497944769029278, 0.001367884604316171740, 0.001563271263863314203 ),
 .UNSPECIFIED. ) ;
#46023=CARTESIAN_POINT ( 'NONE',  ( -13.63463862190834952, -5.056417327199099532, 34.11270091957321426 ) ) ;
#46025=CARTESIAN_POINT ( 'NONE',  ( 13.13459216039392707, -4.175268141568685643, 33.81360843649122216 ) ) ;
#46026=EDGE_CURVE ( 'NONE', #30760, #15316, #4804, .T. ) ;
#46027=CARTESIAN_POINT ( 'NONE',  ( 9.468822748583747284, -6.760086850603066466, 34.69517049084099369 ) ) ;
#46029=EDGE_LOOP ( 'NONE', ( #27683, #17244, #85942, #17793 ) ) ;
#46030=CARTESIAN_POINT ( 'NONE',  ( -3.480792468062196221, -3.202444869320336451, 32.30641848906366675 ) ) ;
#46031=CARTESIAN_POINT ( 'NONE',  ( 5.076923076923075762, -1.790695186598648903, 34.54067556320373455 ) ) ;
#46034=EDGE_LOOP ( 'NONE', ( #63335, #27242, #84282, #44169 ) ) ;
#46035=CARTESIAN_POINT ( 'NONE',  ( -11.53846153846153655, -10.51840700105979565, 33.73612834413961536 ) ) ;
#46036=CARTESIAN_POINT ( 'NONE',  ( 12.71148387091650278, -4.176053281294518804, 33.81426240980091791 ) ) ;
#46038=CARTESIAN_POINT ( 'NONE',  ( -4.153846153846273204, -8.613356846316285953, 34.62446782046622218 ) ) ;
#46040=DIRECTION ( 'NONE',  ( 0.000000000000000000, 0.6427876096865368094, 0.7660444431189802339 ) ) ;
#46043=CARTESIAN_POINT ( 'NONE',  ( -16.37677311275299985, -6.459968553980840689, 34.89616026154728701 ) ) ;
#46044=CARTESIAN_POINT ( 'NONE',  ( -2.177166605928744669, -10.19071101563364401, 33.96452234770658407 ) ) ;
#46045=CARTESIAN_POINT ( 'NONE',  ( 3.903869409797562806, -8.347322224742351082, 34.93158281831414769 ) ) ;
#46046=B_SPLINE_CURVE_WITH_KNOTS ( 'NONE', 3,
 ( #72339, #38116, #3877, #54729, #5664, #13310, #82220, #81781, #27266, #61049 ),
 .UNSPECIFIED., .F., .F.,
 ( 4, 2, 2, 2, 4 ),
 ( 0.0007817246256747455461, 0.0009771112852218885505, 0.001172497944769031446, 0.001367884604316174559, 0.001563271263863317455 ),
 .UNSPECIFIED. ) ;
#46047=AXIS2_PLACEMENT_3D ( 'NONE', #29639, #42273, #14797 ) ;
#46048=VERTEX_POINT ( 'NONE', #53414 ) ;
#46049=CARTESIAN_POINT ( 'NONE',  ( 12.46153846153833911, -3.835265460704628371, 33.15142922262033665 ) ) ;
#46050=B_SPLINE_CURVE_WITH_KNOTS ( 'NONE', 3,
 ( #9910, #85577, #79267, #18457, #45912, #37372, #38719, #73396, #66180, #44123 ),
 .UNSPECIFIED., .F., .F.,
 ( 4, 2, 2, 2, 4 ),
 ( 0.000000000000000000, 0.0001954339857564091278, 0.0003908679715128182556, 0.0005863019572692274375, 0.0007817359430256365111 ),
 .UNSPECIFIED. ) ;
#46051=VERTEX_POINT ( 'NONE', #25511 ) ;
#46052=B_SPLINE_CURVE_WITH_KNOTS ( 'NONE', 3,
 ( #27314, #48016, #1617, #40833, #56115, #75493, #76381, #55223, #54776, #34068 ),
 .UNSPECIFIED., .F., .F.,
 ( 4, 2, 2, 2, 4 ),
 ( 0.000000000000000000, 0.0001954339857564080978, 0.0003908679715128161956, 0.0005863019572692242934, 0.0007817359430256323911 ),
 .UNSPECIFIED. ) ;
#46053=CARTESIAN_POINT ( 'NONE',  ( -0.3310127597748995232, -2.882268652242222728, 31.66798894389554064 ) ) ;
#46054=CARTESIAN_POINT ( 'NONE',  ( 16.15384615384646949, -2.255955759149395501, 30.00000000000324363 ) ) ;
#46055=CARTESIAN_POINT ( 'NONE',  ( 6.000000000000001776, -11.91647553114624181, 32.58852847137148245 ) ) ;
#46056=ORIENTED_EDGE ( 'NONE', *, *, #55918, .T. ) ;
#46057=B_SPLINE_CURVE_WITH_KNOTS ( 'NONE', 3,
 ( #24215, #36421, #50354, #58895, #77837, #63877, #2175, #51672, #29663, #16141 ),
 .UNSPECIFIED., .F., .F.,
 ( 4, 2, 2, 2, 4 ),
 ( 0.0007817359430256288133, 0.0009771253907249948054, 0.001172514838424360689, 0.001367904286123726573, 0.001563293733823092457 ),
 .UNSPECIFIED. ) ;
#46058=CARTESIAN_POINT ( 'NONE',  ( -8.769230769230768274, -10.67929555188718282, 33.92786785259544047 ) ) ;
#46059=CARTESIAN_POINT ( 'NONE',  ( 13.38461538461538680, -9.058645607665452459, 34.76329471203371924 ) ) ;
#46060=CARTESIAN_POINT ( 'NONE',  ( -9.757578138268465651, -2.625532179533444754, 30.86335684631481513 ) ) ;
#46061=CARTESIAN_POINT ( 'NONE',  ( 8.519230769230768274, -7.500000000000001776, 34.75000000000000000 ) ) ;
#46062=CARTESIAN_POINT ( 'NONE',  ( -5.011667937410237528, -11.06231777344671130, 33.60647404775212976 ) ) ;
#46063=ORIENTED_EDGE ( 'NONE', *, *, #48215, .F. ) ;
#46064=VECTOR ( 'NONE', #36359, 1000.000000000000227 ) ;
#46065=FACE_BOUND ( 'NONE', #50547, .T. ) ;
#46066=ORIENTED_EDGE ( 'NONE', *, *, #48301, .T. ) ;
#46067=CARTESIAN_POINT ( 'NONE',  ( -14.98071481085577972, -6.523592122091592671, 34.90882529074906415 ) ) ;
#46068=B_SPLINE_CURVE_WITH_KNOTS ( 'NONE', 3,
 ( #6518, #27665, #14598, #13708, #640, #68215, #33977, #54241, #54684, #61441 ),
 .UNSPECIFIED., .F., .F.,
 ( 4, 2, 2, 2, 4 ),
 ( 0.0007817246256747454377, 0.0009771112852218883336, 0.001172497944769031446, 0.001367884604316174342, 0.001563271263863317238 ),
 .UNSPECIFIED. ) ;
#46069=CARTESIAN_POINT ( 'NONE',  ( -12.23875879256039489, -3.020022701398813236, 32.48759521482552515 ) ) ;
#46070=EDGE_CURVE ( 'NONE', #27377, #5535, #80916, .T. ) ;
#46071=VECTOR ( 'NONE', #24372, 1000.000000000000114 ) ;
#46073=CARTESIAN_POINT ( 'NONE',  ( 12.46153846153833911, -5.094484230521993062, 34.41647553114689373 ) ) ;
#46074=EDGE_CURVE ( 'NONE', #26040, #6052, #66038, .T. ) ;
#46075=DIRECTION ( 'NONE',  ( 0.000000000000000000, 0.1736481776669267785, -0.9848077530122087975 ) ) ;
#46077=CARTESIAN_POINT ( 'NONE',  ( 12.46153846153846168, -9.780366693483667717, 34.19971097300155094 ) ) ;
#46078=VECTOR ( 'NONE', #31307, 1000.000000000000000 ) ;
#46079=AXIS2_PLACEMENT_3D ( 'NONE', #22504, #16190, #85983 ) ;
#46080=ORIENTED_EDGE ( 'NONE', *, *, #49818, .F. ) ;
#46085=ORIENTED_EDGE ( 'NONE', *, *, #81406, .F. ) ;
#46087=CARTESIAN_POINT ( 'NONE',  ( 2.057669070399344768, -5.056417327199099532, 34.11270091957320716 ) ) ;
#46088=CARTESIAN_POINT ( 'NONE',  ( -11.66915300512909859, -8.999036380462717588, 34.52022231692819076 ) ) ;
#46092=CARTESIAN_POINT ( 'NONE',  ( 13.38461538461526601, -8.613356846316285953, 34.62446782046622218 ) ) ;
#46093=CARTESIAN_POINT ( 'NONE',  ( -6.130690603110308778, -2.845849958028613624, 32.17971566917920967 ) ) ;
#46095=CARTESIAN_POINT ( 'NONE',  ( -3.903900635498011251, -10.76462480002816235, 33.53768742498949962 ) ) ;
#46096=CARTESIAN_POINT ( 'NONE',  ( 0.3313912521002406741, -3.285722584762970744, 32.44110544564090759 ) ) ;
#46098=ORIENTED_EDGE ( 'NONE', *, *, #68543, .T. ) ;
#46099=VERTEX_POINT ( 'NONE', #26401 ) ;
#46100=CARTESIAN_POINT ( 'NONE',  ( -11.66860874789975888, -12.45813303252208648, 30.39737893381572675 ) ) ;
#46101=ORIENTED_EDGE ( 'NONE', *, *, #57479, .F. ) ;
#46102=DIRECTION ( 'NONE',  ( -0.000000000000000000, -0.9396926207859092051, -0.3420201433256662704 ) ) ;
#46103=CARTESIAN_POINT ( 'NONE',  ( 18.25000000000000000, -2.249999999999998668, 29.75000000000000355 ) ) ;
#46104=CARTESIAN_POINT ( 'NONE',  ( 16.40384615384759215, -7.500000000000155431, 34.75000000000007105 ) ) ;
#46105=CARTESIAN_POINT ( 'NONE',  ( 6.989145274079363368, -2.538708090699994813, 30.37095296980875503 ) ) ;
#46106=FACE_BOUND ( 'NONE', #62998, .T. ) ;
#46107=VERTEX_POINT ( 'NONE', #74589 ) ;
#46109=VERTEX_POINT ( 'NONE', #59738 ) ;
#46110=DIRECTION ( 'NONE',  ( 0.000000000000000000, 0.9396926207859126468, 0.3420201433256571111 ) ) ;
#46111=ADVANCED_FACE ( 'NONE', ( #67384 ), #33602, .F. ) ;
#46112=ORIENTED_EDGE ( 'NONE', *, *, #80734, .T. ) ;
#46113=FACE_BOUND ( 'NONE', #20602, .T. ) ;
#46115=CARTESIAN_POINT ( 'NONE',  ( -13.38461538461538325, -1.129524287112498415, 32.06866353760679544 ) ) ;
#46116=ORIENTED_EDGE ( 'NONE', *, *, #64839, .F. ) ;
#46117=CARTESIAN_POINT ( 'NONE',  ( -1.254089946381738763, -5.915461855592777596, 34.75538340440931506 ) ) ;
#46118=CARTESIAN_POINT ( 'NONE',  ( -6.792551484843277976, -2.372941743896878286, 30.88044141588254377 ) ) ;
#46119=CARTESIAN_POINT ( 'NONE',  ( 2.057715563643718326, -11.47974371597207899, 33.17467449705390692 ) ) ;
#46121=CARTESIAN_POINT ( 'NONE',  ( 14.24242230713598900, -11.67786785259540849, 32.92929555188721480 ) ) ;
#46122=CARTESIAN_POINT ( 'NONE',  ( 3.100622021331007172, -12.27039167877662251, 31.24851455888617835 ) ) ;
#46123=CARTESIAN_POINT ( 'NONE',  ( -9.469528151039279251, -2.600157965045224451, 30.74683119005207743 ) ) ;
#46124=ORIENTED_EDGE ( 'NONE', *, *, #15039, .F. ) ;
#46125=B_SPLINE_CURVE_WITH_KNOTS ( 'NONE', 3,
 ( #58596, #85641, #86090, #82002, #39691, #6768, #34693, #81117, #13092, #12649 ),
 .UNSPECIFIED., .F., .F.,
 ( 4, 2, 2, 2, 4 ),
 ( 0.0007817359430256319575, 0.0009771253907249984917, 0.001172514838424365026, 0.001367904286123731343, 0.001563293733823097878 ),
 .UNSPECIFIED. ) ;
#46126=EDGE_CURVE ( 'NONE', #65351, #40455, #80011, .T. ) ;
#46127=FACE_OUTER_BOUND ( 'NONE', #69121, .T. ) ;
#46128=CARTESIAN_POINT ( 'NONE',  ( -16.94613126909828793, -11.71459661697925903, 32.44059661609676937 ) ) ;
#46129=EDGE_LOOP ( 'NONE', ( #61029, #68749 ) ) ;
#46130=LINE ( 'NONE', #33510, #50179 ) ;
#46131=DIRECTION ( 'NONE',  ( 0.000000000000000000, 0.7660444431189822323, -0.6427876096865344779 ) ) ;
#46132=CARTESIAN_POINT ( 'NONE',  ( -14.37377468705243899, -2.486705287966279432, 31.30864560766542937 ) ) ;
#46133=CARTESIAN_POINT ( 'NONE',  ( 16.08857615328984281, -11.06231777344662959, 33.60647404775220082 ) ) ;
#46135=DIRECTION ( 'NONE',  ( -0.000000000000000000, 0.6427876096865404731, -0.7660444431189771253 ) ) ;
#46138=EDGE_CURVE ( 'NONE', #43687, #46293, #6128, .T. ) ;
#46139=ADVANCED_FACE ( 'NONE', ( #54299 ), #40367, .F. ) ;
#46141=CARTESIAN_POINT ( 'NONE',  ( -3.453695448285378333, -2.554751324335734264, 30.48935550225260727 ) ) ;
#46142=DIRECTION ( 'NONE',  ( -0.000000000000000000, -0.7660444431189791237, -0.6427876096865379196 ) ) ;
#46144=EDGE_LOOP ( 'NONE', ( #44730, #22290 ) ) ;
#46145=FACE_OUTER_BOUND ( 'NONE', #55392, .T. ) ;
#46148=AXIS2_PLACEMENT_3D ( 'NONE', #11903, #39381, #46565 ) ;
#46150=CYLINDRICAL_SURFACE ( 'NONE', #42759, 0.2499999999999994726 ) ;
#46151=ORIENTED_EDGE ( 'NONE', *, *, #74618, .T. ) ;
#46152=DIRECTION ( 'NONE',  ( 1.000000000000000000, 0.000000000000000000, 0.000000000000000000 ) ) ;
#46154=CARTESIAN_POINT ( 'NONE',  ( -17.86947429823643674, -6.001044277235007662, 34.52024696741798948 ) ) ;
#46156=CARTESIAN_POINT ( 'NONE',  ( 5.749976762707035505, -11.37209801155882971, 32.91403422569032955 ) ) ;
#46157=CARTESIAN_POINT ( 'NONE',  ( -7.846153846153965716, -6.026961402154118019, 34.52809138561165270 ) ) ;
#46158=CARTESIAN_POINT ( 'NONE',  ( 8.769230769230768274, -10.67929555188718282, 33.92786785259544047 ) ) ;
#46159=VECTOR ( 'NONE', #22851, 999.9999999999998863 ) ;
#46160=CARTESIAN_POINT ( 'NONE',  ( -8.769230769230768274, -12.48256725967547354, 35.29906147534542527 ) ) ;
#46161=CARTESIAN_POINT ( 'NONE',  ( 2.307692307692309264, -13.63283147151868846, 33.57946703557072254 ) ) ;
#46162=CARTESIAN_POINT ( 'NONE',  ( 0.4615384615384611200, -2.486705287966279876, 31.30864560766543647 ) ) ;
#46165=EDGE_CURVE ( 'NONE', #17652, #14701, #52950, .T. ) ;
#46166=CARTESIAN_POINT ( 'NONE',  ( -6.989159302437059296, -4.661471528628507777, 34.16647553114621871 ) ) ;
#46167=CARTESIAN_POINT ( 'NONE',  ( -16.15384615384584777, -2.506253911140615021, 30.00000000000323297 ) ) ;
#46168=DIRECTION ( 'NONE',  ( -0.000000000000000000, 0.9848077530122086864, -0.1736481776669273891 ) ) ;
#46169=EDGE_CURVE ( 'NONE', #32375, #87025, #40077, .T. ) ;
#46170=ORIENTED_EDGE ( 'NONE', *, *, #50214, .F. ) ;
#46171=ORIENTED_EDGE ( 'NONE', *, *, #46860, .F. ) ;
#46172=CARTESIAN_POINT ( 'NONE',  ( 3.230769230769231726, -10.67929555188718282, 33.92786785259544047 ) ) ;
#46173=CARTESIAN_POINT ( 'NONE',  ( 10.61538461538461675, -4.786620604624113540, 33.94971097300155094 ) ) ;
#46174=CARTESIAN_POINT ( 'NONE',  ( -2.372962308248625085, -2.379036618887870880, 30.90682066428147934 ) ) ;
#46175=CARTESIAN_POINT ( 'NONE',  ( 15.48076923077065103, -7.500000000000154543, 35.00000000000007105 ) ) ;
#46176=CARTESIAN_POINT ( 'NONE',  ( 14.05771556364371655, -3.436278759898153901, 33.07459398097509506 ) ) ;
#46177=CYLINDRICAL_SURFACE ( 'NONE', #74346, 0.2499999999999986955 ) ;
#46178=AXIS2_PLACEMENT_3D ( 'NONE', #62982, #85055, #8509 ) ;
#46179=VERTEX_POINT ( 'NONE', #69159 ) ;
#46180=CARTESIAN_POINT ( 'NONE',  ( -6.923076923076922462, -9.780366693483667717, 34.19971097300155094 ) ) ;
#46181=ORIENTED_EDGE ( 'NONE', *, *, #53042, .T. ) ;
#46182=AXIS2_PLACEMENT_3D ( 'NONE', #66516, #4818, #74159 ) ;
#46183=ORIENTED_EDGE ( 'NONE', *, *, #11494, .F. ) ;
#46184=EDGE_CURVE ( 'NONE', #26559, #64833, #57270, .T. ) ;
#46185=LINE ( 'NONE', #53374, #435 ) ;
#46186=CARTESIAN_POINT ( 'NONE',  ( -5.076923076923199218, -11.06231777344772027, 33.60647404775119895 ) ) ;
#46187=CARTESIAN_POINT ( 'NONE',  ( 9.942253210655836781, -12.22109172314383052, 31.39792113162168263 ) ) ;
#46188=CARTESIAN_POINT ( 'NONE',  ( -0.4615384615385840772, -2.379036618888197285, 30.90682066428292885 ) ) ;
#46189=CARTESIAN_POINT ( 'NONE',  ( 5.777073782483853392, -2.758268499246657957, 31.33685645148948140 ) ) ;
#46191=B_SPLINE_CURVE_WITH_KNOTS ( 'NONE', 3,
 ( #13384, #6195, #67893, #68332, #6630, #60239, #12505, #61124, #26469, #32771 ),
 .UNSPECIFIED., .F., .F.,
 ( 4, 2, 2, 2, 4 ),
 ( 0.000000000000000000, 0.0001954339857564078809, 0.0003908679715128157619, 0.0005863019572692236428, 0.0007817359430256315238 ),
 .UNSPECIFIED. ) ;
#46192=ORIENTED_EDGE ( 'NONE', *, *, #12099, .T. ) ;
#46193=EDGE_LOOP ( 'NONE', ( #2356, #55619, #52929, #20018 ) ) ;
#46194=CARTESIAN_POINT ( 'NONE',  ( 17.32697749683652688, -10.06805714834173138, 34.32951233291982618 ) ) ;
#46195=LINE ( 'NONE', #17837, #53140 ) ;
#46196=CARTESIAN_POINT ( 'NONE',  ( 8.769230769230768274, -5.471508081941601098, 34.59228464037088457 ) ) ;
#46197=VECTOR ( 'NONE', #49085, 1000.000000000000227 ) ;
#46198=CARTESIAN_POINT ( 'NONE',  ( 1.253923917947825206, -3.530157926970578508, 32.79014554554150607 ) ) ;
#46199=CYLINDRICAL_SURFACE ( 'NONE', #49525, 0.2500000000000012212 ) ;
#46201=ORIENTED_EDGE ( 'NONE', *, *, #42651, .T. ) ;
#46203=EDGE_CURVE ( 'NONE', #8388, #12765, #45468, .T. ) ;
#46204=CARTESIAN_POINT ( 'NONE',  ( -5.933931648997560870, -3.050289026998446840, 32.03036669348366416 ) ) ;
#46205=ORIENTED_EDGE ( 'NONE', *, *, #19278, .F. ) ;
#46206=CARTESIAN_POINT ( 'NONE',  ( -9.757577692864012775, -10.33852847137145048, 34.16647553114627556 ) ) ;
#46207=CARTESIAN_POINT ( 'NONE',  ( -11.53846153846153655, -3.322132147404559976, 32.92929555188717927 ) ) ;
#46209=ORIENTED_EDGE ( 'NONE', *, *, #925, .T. ) ;
#46210=DIRECTION ( 'NONE',  ( -0.000000000000000000, -0.000000000000000000, -1.000000000000000000 ) ) ;
#46211=VERTEX_POINT ( 'NONE', #40806 ) ;
#46212=CARTESIAN_POINT ( 'NONE',  ( -8.835313148590904220, -4.661471528628507777, 34.16647553114621871 ) ) ;
#46213=DIRECTION ( 'NONE',  ( -0.000000000000000000, -0.5000000000000009992, -0.8660254037844380415 ) ) ;
#46214=CARTESIAN_POINT ( 'NONE',  ( 7.846153846153723244, -4.320704448113951379, 33.92786785259630022 ) ) ;
#46215=CARTESIAN_POINT ( 'NONE',  ( -6.792285115252136407, -12.38066358083363738, 30.83685684665853444 ) ) ;
#46217=B_SPLINE_CURVE_WITH_KNOTS ( 'NONE', 3,
 ( #23424, #4497, #51769, #65738, #43700, #78369, #36939, #2701, #23858, #9917 ),
 .UNSPECIFIED., .F., .F.,
 ( 4, 2, 2, 2, 4 ),
 ( 0.000000000000000000, 0.0001954339857564071491, 0.0003908679715128142982, 0.0005863019572692214744, 0.0007817359430256285964 ),
 .UNSPECIFIED. ) ;
#46219=EDGE_LOOP ( 'NONE', ( #43992, #3570, #74823, #85078 ) ) ;
#46220=EDGE_CURVE ( 'NONE', #81809, #35903, #51818, .T. ) ;
#46221=CARTESIAN_POINT ( 'NONE',  ( 6.856993512121043466, -8.120952969808774569, 34.71129190930000163 ) ) ;
#46222=CARTESIAN_POINT ( 'NONE',  ( -9.019207513279360100, -4.075325502946081535, 33.72974371597206300 ) ) ;
#46223=EDGE_CURVE ( 'NONE', #76945, #25666, #33673, .T. ) ;
#46224=DIRECTION ( 'NONE',  ( 1.000000000000000000, 0.000000000000000000, 0.000000000000000000 ) ) ;
#46225=ORIENTED_EDGE ( 'NONE', *, *, #76943, .F. ) ;
#46226=VECTOR ( 'NONE', #5863, 1000.000000000000000 ) ;
#46227=DIRECTION ( 'NONE',  ( 1.000000000000000000, 0.000000000000000000, 0.000000000000000000 ) ) ;
#46230=CARTESIAN_POINT ( 'NONE',  ( 8.834485908743602067, -10.33852847137154107, 34.16647553114620450 ) ) ;
#46231=FACE_BOUND ( 'NONE', #57591, .T. ) ;
#46232=CARTESIAN_POINT ( 'NONE',  ( 13.38461538461526423, -12.16647553114689728, 32.15551576947799362 ) ) ;
#46233=CARTESIAN_POINT ( 'NONE',  ( 16.15384615384615330, -8.164416787775445883, 34.95778746994557906 ) ) ;
#46234=ADVANCED_FACE ( 'NONE', ( #2456 ), #71809, .F. ) ;
#46235=CARTESIAN_POINT ( 'NONE',  ( -9.442253272394237840, -12.01375889529407281, 32.43194544308182969 ) ) ;
#46236=CARTESIAN_POINT ( 'NONE',  ( 18.13052570176356326, -11.46989282347013095, 32.79007818306219946 ) ) ;
#46237=CARTESIAN_POINT ( 'NONE',  ( 18.00000000000000000, -11.16473453929635440, 33.15142922261926373 ) ) ;
#46238=CARTESIAN_POINT ( 'NONE',  ( -4.153846153846152411, -10.67929555188718282, 33.92786785259544047 ) ) ;
#46239=VECTOR ( 'NONE', #86031, 1000.000000000000227 ) ;
#46240=CARTESIAN_POINT ( 'NONE',  ( -8.769230769230768274, -3.513871655860378418, 32.76840700105978499 ) ) ;
#46242=ORIENTED_EDGE ( 'NONE', *, *, #4871, .T. ) ;
#46243=CARTESIAN_POINT ( 'NONE',  ( -8.546219417617917813, -5.667800583137506010, 34.40243808032445827 ) ) ;
#46244=ORIENTED_EDGE ( 'NONE', *, *, #18792, .T. ) ;
#46245=CARTESIAN_POINT ( 'NONE',  ( 1.161749962411747772, -2.501496062324912284, 29.88072118266895671 ) ) ;
#46246=CARTESIAN_POINT ( 'NONE',  ( 16.15384615384615330, -12.62096338111211580, 30.90682066428153263 ) ) ;
#46247=DIRECTION ( 'NONE',  ( 0.000000000000000000, 0.8660254037844377084, -0.5000000000000015543 ) ) ;
#46248=CARTESIAN_POINT ( 'NONE',  ( -2.373775718648187816, -11.69971097300155272, 32.46337939537587403 ) ) ;
#46249=CARTESIAN_POINT ( 'NONE',  ( 3.480714749117373774, -6.696923467548660192, 34.68552623307873972 ) ) ;
#46250=CARTESIAN_POINT ( 'NONE',  ( -11.78843828251013015, -4.075325502946081535, 33.72974371597206300 ) ) ;
#46252=CARTESIAN_POINT ( 'NONE',  ( 15.00784227186238162, -11.98009711892699514, 32.48740034544076138 ) ) ;
#46253=CARTESIAN_POINT ( 'NONE',  ( 6.923076923076924238, -8.810774026931790459, 35.74407628777942847 ) ) ;
#46255=CARTESIAN_POINT ( 'NONE',  ( 5.142990410273152513, -12.62096338111211757, 30.90682066428152908 ) ) ;
#46256=CARTESIAN_POINT ( 'NONE',  ( 14.55763782604045176, -5.852078868378309373, 34.47109172314383585 ) ) ;
#46257=CARTESIAN_POINT ( 'NONE',  ( 9.692307692307570832, -3.643525952248795718, 33.31231777344771672 ) ) ;
#46259=EDGE_CURVE ( 'NONE', #29065, #43002, #57406, .T. ) ;
#46260=CARTESIAN_POINT ( 'NONE',  ( 3.296935837360872146, -7.250054591869667497, 34.99404684341514127 ) ) ;
#46261=CARTESIAN_POINT ( 'NONE',  ( 7.976679284387489410, -9.503571793651731880, 34.60286762892837942 ) ) ;
#46262=VERTEX_POINT ( 'NONE', #24069 ) ;
#46263=B_SPLINE_CURVE_WITH_KNOTS ( 'NONE', 3,
 ( #31950, #4007, #46345, #25184, #10783, #85999, #66622, #85553, #78787, #52649 ),
 .UNSPECIFIED., .F., .F.,
 ( 4, 2, 2, 2, 4 ),
 ( 0.0007817246256747469556, 0.0009771112852218892010, 0.001172497944769031230, 0.001367884604316173258, 0.001563271263863315504 ),
 .UNSPECIFIED. ) ;
#46264=CARTESIAN_POINT ( 'NONE',  ( 16.40379156322419973, -4.932303261841487263, 34.32971442181322885 ) ) ;
#46265=CARTESIAN_POINT ( 'NONE',  ( 15.29683656411930848, -10.67929555188718282, 33.92786785259544757 ) ) ;
#46267=B_SPLINE_CURVE_WITH_KNOTS ( 'NONE', 3,
 ( #69724, #49457, #28748, #8475, #63402, #29199, #56652, #44012, #22422, #23300 ),
 .UNSPECIFIED., .F., .F.,
 ( 4, 2, 2, 2, 4 ),
 ( 0.0007817246256747474977, 0.0009771112852218911526, 0.001172497944769034699, 0.001367884604316178462, 0.001563271263863322009 ),
 .UNSPECIFIED. ) ;
#46268=CARTESIAN_POINT ( 'NONE',  ( 6.250054311638314708, -4.235687564193446164, 33.53795663066793509 ) ) ;
#46269=CARTESIAN_POINT ( 'NONE',  ( -8.899921372341079717, -3.338472653186243644, 32.95098750199972670 ) ) ;
#46270=ORIENTED_EDGE ( 'NONE', *, *, #31041, .T. ) ;
#46271=DIRECTION ( 'NONE',  ( -0.000000000000000000, 1.000000000000000000, 3.491481338843133355E-15 ) ) ;
#46273=CARTESIAN_POINT ( 'NONE',  ( 7.846153846153846700, -2.486705287966279876, 31.30864560766543647 ) ) ;
#46274=ORIENTED_EDGE ( 'NONE', *, *, #15660, .F. ) ;
#46275=CARTESIAN_POINT ( 'NONE',  ( -13.63463860883683942, -10.18141759479407327, 34.26406193332782379 ) ) ;
#46276=DIRECTION ( 'NONE',  ( -0.000000000000000000, 0.5000000000000011102, -0.8660254037844381525 ) ) ;
#46277=CARTESIAN_POINT ( 'NONE',  ( -14.98082382139119062, -12.07971442181322175, 32.31769673815850297 ) ) ;
#46278=AXIS2_PLACEMENT_3D ( 'NONE', #32853, #74739, #61197 ) ;
#46279=CARTESIAN_POINT ( 'NONE',  ( -15.90384615384608757, -7.434744860731433924, 35.00000000000000711 ) ) ;
#46281=CARTESIAN_POINT ( 'NONE',  ( -4.153846153846152411, -3.322132147404559976, 32.92929555188717927 ) ) ;
#46282=CARTESIAN_POINT ( 'NONE',  ( -12.68502338610279523, -2.612411019501189369, 31.66733052389439962 ) ) ;
#46283=CARTESIAN_POINT ( 'NONE',  ( 8.519254025182176449, -3.436278759898153901, 33.07459398097509506 ) ) ;
#46284=VERTEX_POINT ( 'NONE', #64154 ) ;
#46285=VERTEX_POINT ( 'NONE', #23185 ) ;
#46286=VERTEX_POINT ( 'NONE', #37133 ) ;
#46287=CARTESIAN_POINT ( 'NONE',  ( 0.2380535178145121722, -8.496056993536548418, 34.65000542017679663 ) ) ;
#46288=CARTESIAN_POINT ( 'NONE',  ( -2.057746789344163663, -5.852078868378310261, 34.47109172314383585 ) ) ;
#46289=CARTESIAN_POINT ( 'NONE',  ( 2.438484115517096651, -5.582136614379148654, 34.36778462344220486 ) ) ;
#46290=CARTESIAN_POINT ( 'NONE',  ( -10.61538461538473577, -6.835583212225970762, 34.95778746994575670 ) ) ;
#46292=B_SPLINE_CURVE_WITH_KNOTS ( 'NONE', 3,
 ( #8046, #88709, #26989, #6706, #54447, #69304 ),
 .UNSPECIFIED., .F., .F.,
 ( 4, 2, 4 ),
 ( 0.000000000000000000, 0.0001954784845028902421, 0.0003909569690057804843 ),
 .UNSPECIFIED. ) ;
#46293=VERTEX_POINT ( 'NONE', #63719 ) ;
#46294=ORIENTED_EDGE ( 'NONE', *, *, #81193, .F. ) ;
#46295=ORIENTED_EDGE ( 'NONE', *, *, #52203, .F. ) ;
#46297=ORIENTED_EDGE ( 'NONE', *, *, #75421, .T. ) ;
#46298=FACE_OUTER_BOUND ( 'NONE', #24915, .T. ) ;
#46299=VECTOR ( 'NONE', #66878, 1000.000000000000000 ) ;
#46300=CARTESIAN_POINT ( 'NONE',  ( 11.28846153846153832, -7.500000000000001776, 35.04278698407183867 ) ) ;
#46301=CARTESIAN_POINT ( 'NONE',  ( -12.39547011053602610, -12.10708131394839882, 31.69288490824020954 ) ) ;
#46302=CARTESIAN_POINT ( 'NONE',  ( -15.23076923076935074, -9.442884908241554243, 34.35708131394783038 ) ) ;
#46303=VERTEX_POINT ( 'NONE', #50647 ) ;
#46304=EDGE_LOOP ( 'NONE', ( #36850, #45568, #61729, #41685 ) ) ;
#46305=ORIENTED_EDGE ( 'NONE', *, *, #77736, .F. ) ;
#46306=CARTESIAN_POINT ( 'NONE',  ( -10.74607521849492464, -10.70098750199973203, 33.91152734681376302 ) ) ;
#46307=FACE_OUTER_BOUND ( 'NONE', #25689, .T. ) ;
#46308=ORIENTED_EDGE ( 'NONE', *, *, #2186, .T. ) ;
#46310=CARTESIAN_POINT ( 'NONE',  ( -0.3310130233048168558, -5.070358843744209310, 34.40418822224088302 ) ) ;
#46311=CARTESIAN_POINT ( 'NONE',  ( -11.40793610022789650, -4.299079248970732792, 33.91157788607253565 ) ) ;
#46313=CARTESIAN_POINT ( 'NONE',  ( -1.450698795571263799, -8.120952969808774569, 34.71129190930000163 ) ) ;
#46314=DIRECTION ( 'NONE',  ( -0.000000000000000000, -0.6427876096865404731, -0.7660444431189770143 ) ) ;
#46315=FACE_BOUND ( 'NONE', #28161, .T. ) ;
#46316=CARTESIAN_POINT ( 'NONE',  ( -5.207071046654770718, -10.31621877034669588, 34.18098118002070152 ) ) ;
#46317=CARTESIAN_POINT ( 'NONE',  ( -12.68502340526241312, -9.331801661448606566, 34.40259984581193464 ) ) ;
#46318=AXIS2_PLACEMENT_3D ( 'NONE', #3567, #86464, #31036 ) ;
#46319=EDGE_CURVE ( 'NONE', #4757, #3, #70487, .T. ) ;
#46320=CARTESIAN_POINT ( 'NONE',  ( 11.53846153846141753, -12.46129190930018460, 30.37095296980731973 ) ) ;
#46321=CARTESIAN_POINT ( 'NONE',  ( -7.173076923076921574, -7.500000000000001776, 34.75000000000000000 ) ) ;
#46322=CYLINDRICAL_SURFACE ( 'NONE', #13089, 0.2500000000000004996 ) ;
#46323=VECTOR ( 'NONE', #63113, 1000.000000000000000 ) ;
#46324=CARTESIAN_POINT ( 'NONE',  ( -3.930883019579477278, -7.369474539155830506, 34.99858011523957657 ) ) ;
#46325=DIRECTION ( 'NONE',  ( 0.000000000000000000, 0.1736481776669267785, -0.9848077530122087975 ) ) ;
#46326=ORIENTED_EDGE ( 'NONE', *, *, #45015, .T. ) ;
#46327=CARTESIAN_POINT ( 'NONE',  ( -15.00775638667583500, -11.43677907613344757, 33.22367315496202167 ) ) ;
#46328=ADVANCED_FACE ( 'NONE', ( #10566 ), #10115, .F. ) ;
#46330=ORIENTED_EDGE ( 'NONE', *, *, #34606, .T. ) ;
#46332=AXIS2_PLACEMENT_3D ( 'NONE', #69320, #41852, #8947 ) ;
#46335=LINE ( 'NONE', #66151, #51902 ) ;
#46336=VERTEX_POINT ( 'NONE', #58295 ) ;
#46337=CYLINDRICAL_SURFACE ( 'NONE', #18374, 0.2499999999999995559 ) ;
#46338=CARTESIAN_POINT ( 'NONE',  ( -7.173053654019277303, -9.943427161483782584, 34.11278801902876978 ) ) ;
#46339=DIRECTION ( 'NONE',  ( 0.000000000000000000, 0.000000000000000000, 1.000000000000000000 ) ) ;
#46340=CARTESIAN_POINT ( 'NONE',  ( -9.757578138268465651, -4.481592998940162609, 33.73612834413957984 ) ) ;
#46341=CARTESIAN_POINT ( 'NONE',  ( 18.00000000000000000, -11.11383981884818262, 36.00935417666054406 ) ) ;
#46343=FACE_OUTER_BOUND ( 'NONE', #20934, .T. ) ;
#46345=CARTESIAN_POINT ( 'NONE',  ( -16.94639763868943660, -2.647132371071621471, 31.75357179365173010 ) ) ;
#46349=CARTESIAN_POINT ( 'NONE',  ( -15.23076923076935252, -6.835583212225970762, 34.95778746994575670 ) ) ;
#46350=CARTESIAN_POINT ( 'NONE',  ( 7.053602624840490165, -12.27024696741798770, 31.24895572276497546 ) ) ;
#46351=DIRECTION ( 'NONE',  ( -0.000000000000000000, 0.8660254037844399289, -0.4999999999999980016 ) ) ;
#46352=DIRECTION ( 'NONE',  ( -0.000000000000000000, -0.6427876096865404731, -0.7660444431189771253 ) ) ;
#46353=DIRECTION ( 'NONE',  ( -0.000000000000000000, -0.9848077530122085754, -0.1736481776669273613 ) ) ;
#46355=B_SPLINE_CURVE_WITH_KNOTS ( 'NONE', 3,
 ( #88424, #26696, #49070, #87093, #54154, #55829, #25367, #81651, #19934, #47400 ),
 .UNSPECIFIED., .F., .F.,
 ( 4, 2, 2, 2, 4 ),
 ( 0.000000000000000000, 0.0001954339857564070678, 0.0003908679715128141356, 0.0005863019572692211492, 0.0007817359430256282712 ),
 .UNSPECIFIED. ) ;
#46356=CARTESIAN_POINT ( 'NONE',  ( -7.780085495151406683, -8.120952969808772792, 34.71129190929999453 ) ) ;
#46357=DIRECTION ( 'NONE',  ( 0.000000000000000000, 0.1736481776669275834, 0.9848077530122086864 ) ) ;
#46358=DIRECTION ( 'NONE',  ( -0.000000000000000000, 0.9848077530122085754, -0.1736481776669273613 ) ) ;
#46359=DIRECTION ( 'NONE',  ( -0.000000000000000000, -0.7660444431189791237, -0.6427876096865379196 ) ) ;
#46363=CARTESIAN_POINT ( 'NONE',  ( -12.68502338610279523, -8.539481045369596401, 34.89627647299170832 ) ) ;
#46364=CARTESIAN_POINT ( 'NONE',  ( 6.923076923076800782, -2.379036618888197729, 30.90682066428292885 ) ) ;
#46366=CARTESIAN_POINT ( 'NONE',  ( -3.230769230769229949, -8.120952969808772792, 34.71129190930000163 ) ) ;
#46368=ADVANCED_FACE ( 'NONE', ( #16429 ), #43896, .F. ) ;
#46369=AXIS2_PLACEMENT_3D ( 'NONE', #11269, #33326, #73422 ) ;
#46370=ORIENTED_EDGE ( 'NONE', *, *, #87530, .T. ) ;
#46371=LINE ( 'NONE', #67980, #74391 ) ;
#46372=CARTESIAN_POINT ( 'NONE',  ( -17.07692307692307665, -6.343179335718451384, 34.87096338111211935 ) ) ;
#46373=LINE ( 'NONE', #73856, #41943 ) ;
#46375=EDGE_CURVE ( 'NONE', #27377, #64638, #32545, .T. ) ;
#46376=EDGE_CURVE ( 'NONE', #36288, #8676, #22799, .T. ) ;
#46377=FACE_OUTER_BOUND ( 'NONE', #14064, .T. ) ;
#46378=SURFACE_STYLE_USAGE ( .BOTH. , #20673 ) ;
#46379=EDGE_CURVE ( 'NONE', #68002, #16148, #25047, .T. ) ;
#46380=CARTESIAN_POINT ( 'NONE',  ( 5.299702745901139878, -4.226511098958374291, 33.85474049983370293 ) ) ;
#46381=ORIENTED_EDGE ( 'NONE', *, *, #14522, .F. ) ;
#46383=CARTESIAN_POINT ( 'NONE',  ( -4.403846153846151523, -2.249999999999998668, 29.75000000000000355 ) ) ;
#46384=ORIENTED_EDGE ( 'NONE', *, *, #54889, .F. ) ;
#46385=CARTESIAN_POINT ( 'NONE',  ( 18.24994551834813805, -9.272278438253401589, 34.42582936511637826 ) ) ;
#46387=CARTESIAN_POINT ( 'NONE',  ( 17.07692307692307665, -6.681629849574314051, 35.83090037661290239 ) ) ;
#46388=CARTESIAN_POINT ( 'NONE',  ( -1.607542343522231576, -11.98009711892699691, 32.48740034544075428 ) ) ;
#46389=CYLINDRICAL_SURFACE ( 'NONE', #25484, 0.2500000000000012212 ) ;
#46390=ORIENTED_EDGE ( 'NONE', *, *, #68663, .T. ) ;
#46391=VERTEX_POINT ( 'NONE', #25412 ) ;
#46393=AXIS2_PLACEMENT_3D ( 'NONE', #75755, #14059, #76198 ) ;
#46394=CARTESIAN_POINT ( 'NONE',  ( 7.846153846153846700, -3.513871655860378418, 32.76840700105978499 ) ) ;
#46395=CARTESIAN_POINT ( 'NONE',  ( -0.3307466537136757312, -10.54018710029568595, 33.71981072465678864 ) ) ;
#46396=B_SPLINE_CURVE_WITH_KNOTS ( 'NONE', 3,
 ( #49458, #15234, #42705, #62079, #1711, #37254, #16111, #64278, #9363, #78698 ),
 .UNSPECIFIED., .F., .F.,
 ( 4, 2, 2, 2, 4 ),
 ( 0.0007817359430256294638, 0.0009771253907249948054, 0.001172514838424360255, 0.001367904286123725489, 0.001563293733823090939 ),
 .UNSPECIFIED. ) ;
#46397=CYLINDRICAL_SURFACE ( 'NONE', #72926, 0.2499999999999998890 ) ;
#46398=FACE_OUTER_BOUND ( 'NONE', #4780, .T. ) ;
#46400=CARTESIAN_POINT ( 'NONE',  ( -3.007756386675836779, -4.762714258010882773, 34.23016756924214832 ) ) ;
#46401=CARTESIAN_POINT ( 'NONE',  ( -1.134560964701931463, -10.82426656108011720, 33.81400080652039009 ) ) ;
#46402=VECTOR ( 'NONE', #77726, 1000.000000000000227 ) ;
#46403=CARTESIAN_POINT ( 'NONE',  ( -12.52762187249433978, -6.386643153685125363, 34.62446782046654903 ) ) ;
#46404=EDGE_CURVE ( 'NONE', #70678, #33320, #46130, .T. ) ;
#46405=ORIENTED_EDGE ( 'NONE', *, *, #56978, .F. ) ;
#46406=ORIENTED_EDGE ( 'NONE', *, *, #83055, .T. ) ;
#46407=ORIENTED_EDGE ( 'NONE', *, *, #31649, .F. ) ;
#46408=CARTESIAN_POINT ( 'NONE',  ( -3.931066484868086075, -8.540255544307065350, 34.89611431652622286 ) ) ;
#46409=ORIENTED_EDGE ( 'NONE', *, *, #66910, .F. ) ;
#46410=B_SPLINE_CURVE_WITH_KNOTS ( 'NONE', 3,
 ( #59319, #11133, #86826, #80041, #18339, #4831, #37713, #32301, #17452, #73745 ),
 .UNSPECIFIED., .F., .F.,
 ( 4, 2, 2, 2, 4 ),
 ( 0.000000000000000000, 0.0001954311564186866034, 0.0003908623128373732067, 0.0005862934692560597830, 0.0007817246256747464135 ),
 .UNSPECIFIED. ) ;
#46411=CARTESIAN_POINT ( 'NONE',  ( -11.53846153846153655, -1.790695186598648903, 34.54067556320373455 ) ) ;
#46412=CARTESIAN_POINT ( 'NONE',  ( -4.153846153846273204, -11.94971097300221174, 32.03036669348237098 ) ) ;
#46414=CARTESIAN_POINT ( 'NONE',  ( -14.08468095607945614, -4.187068189119699468, 33.49521262558774026 ) ) ;
#46415=EDGE_CURVE ( 'NONE', #22316, #85987, #86328, .T. ) ;
#46417=CARTESIAN_POINT ( 'NONE',  ( 11.66925334628632349, -2.541949514083464479, 30.39797389878540557 ) ) ;
#46418=VERTEX_POINT ( 'NONE', #45678 ) ;
#46420=CARTESIAN_POINT ( 'NONE',  ( -9.019207500173124004, -4.943428324936578910, 34.04746400365624481 ) ) ;
#46421=CARTESIAN_POINT ( 'NONE',  ( -9.758061120621023932, -7.249945578846652694, 34.99404164642496795 ) ) ;
#46422=FACE_BOUND ( 'NONE', #58252, .T. ) ;
#46423=CARTESIAN_POINT ( 'NONE',  ( 17.20771351789002424, -6.369690395747422684, 34.87708834333098196 ) ) ;
#46424=CYLINDRICAL_SURFACE ( 'NONE', #39965, 0.2499999999999995559 ) ;
#46425=ADVANCED_FACE ( 'NONE', ( #4704 ), #31730, .F. ) ;
#46427=CARTESIAN_POINT ( 'NONE',  ( -3.296039676730006640, -4.481592998940161721, 33.73612834413957984 ) ) ;
#46428=DIRECTION ( 'NONE',  ( -0.000000000000000000, -0.6427876096865404731, -0.7660444431189771253 ) ) ;
#46429=LINE ( 'NONE', #73913, #37565 ) ;
#46430=EDGE_LOOP ( 'NONE', ( #41771, #46725 ) ) ;
#46431=CARTESIAN_POINT ( 'NONE',  ( -10.39237326377176451, -4.187068189119699468, 33.49521262558774026 ) ) ;
#46432=EDGE_CURVE ( 'NONE', #72869, #36033, #27125, .T. ) ;
#46434=ORIENTED_EDGE ( 'NONE', *, *, #31478, .T. ) ;
#46435=CARTESIAN_POINT ( 'NONE',  ( -7.146003881983773454, -4.026226216239095379, 33.68668979543632958 ) ) ;
#46436=FACE_OUTER_BOUND ( 'NONE', #87723, .T. ) ;
#46437=CARTESIAN_POINT ( 'NONE',  ( 3.164686851409096224, -3.322132147404559976, 32.92929555188719348 ) ) ;
#46438=CARTESIAN_POINT ( 'NONE',  ( -14.43838291080261449, -11.93127051446799847, 32.56575433478202797 ) ) ;
#46439=FACE_OUTER_BOUND ( 'NONE', #49133, .T. ) ;
#46440=CARTESIAN_POINT ( 'NONE',  ( -13.25382357679060341, -2.729792928343269587, 31.24908615093345077 ) ) ;
#46441=ORIENTED_EDGE ( 'NONE', *, *, #77311, .F. ) ;
#46442=CARTESIAN_POINT ( 'NONE',  ( -8.769230769230768274, -3.886160181151819604, 36.00935417666054406 ) ) ;
#46443=CARTESIAN_POINT ( 'NONE',  ( 0.6843180028068690524, -10.11255958852955672, 34.01340905677048454 ) ) ;
#46445=EDGE_CURVE ( 'NONE', #9159, #67881, #41181, .T. ) ;
#46446=CARTESIAN_POINT ( 'NONE',  ( -3.480745974817820887, -12.65889640711025521, 30.72598325615533454 ) ) ;
#46447=ORIENTED_EDGE ( 'NONE', *, *, #84629, .F. ) ;
#46448=ORIENTED_EDGE ( 'NONE', *, *, #48643, .F. ) ;
#46449=VECTOR ( 'NONE', #8343, 1000.000000000000000 ) ;
#46451=ADVANCED_FACE ( 'NONE', ( #52428 ), #19106, .F. ) ;
#46453=CARTESIAN_POINT ( 'NONE',  ( 10.48523664565292002, -4.299443229763728169, 33.91186481527756058 ) ) ;
#46454=CARTESIAN_POINT ( 'NONE',  ( -13.16160403300253634, -10.61302985866383963, 33.66295027996417843 ) ) ;
#46456=EDGE_CURVE ( 'NONE', #34857, #33744, #29368, .T. ) ;
#46457=DIRECTION ( 'NONE',  ( 0.000000000000000000, 0.6427876096865373645, -0.7660444431189797898 ) ) ;
#46458=DIRECTION ( 'NONE',  ( 0.000000000000000000, 0.000000000000000000, 1.000000000000000000 ) ) ;
#46459=CARTESIAN_POINT ( 'NONE',  ( 3.453548899747296730, -5.827830569534416583, 34.72679350104403539 ) ) ;
#46460=CARTESIAN_POINT ( 'NONE',  ( -16.94639737515950983, -12.27024696741798770, 31.24895572276497546 ) ) ;
#46461=AXIS2_PLACEMENT_3D ( 'NONE', #11736, #18932, #81088 ) ;
#46462=B_SPLINE_CURVE_WITH_KNOTS ( 'NONE', 3,
 ( #48875, #28159, #7459, #35363, #76347, #14655, #8345, #56079, #7898, #56524 ),
 .UNSPECIFIED., .F., .F.,
 ( 4, 2, 2, 2, 4 ),
 ( 0.0007817359430256304396, 0.0009771253907249967570, 0.001172514838424363291, 0.001367904286123729609, 0.001563293733823095926 ),
 .UNSPECIFIED. ) ;
#46463=B_SPLINE_CURVE_WITH_KNOTS ( 'NONE', 3,
 ( #17536, #1797, #57626, #64809, #43664, #51732, #2229, #29285, #56742, #44537 ),
 .UNSPECIFIED., .F., .F.,
 ( 4, 2, 2, 2, 4 ),
 ( 0.0007817359430256393300, 0.0009771253907250075990, 0.001172514838424376085, 0.001367904286123744571, 0.001563293733823112840 ),
 .UNSPECIFIED. ) ;
#46465=ORIENTED_EDGE ( 'NONE', *, *, #8671, .F. ) ;
#46466=CARTESIAN_POINT ( 'NONE',  ( 0.3308469948709013009, -9.804603061927743113, 34.18744698557895845 ) ) ;
#46467=EDGE_LOOP ( 'NONE', ( #70190, #11972, #59205, #68649 ) ) ;
#46468=CARTESIAN_POINT ( 'NONE',  ( -5.999999999999998224, -3.513871655860378418, 32.76840700105978499 ) ) ;
#46469=FACE_OUTER_BOUND ( 'NONE', #26998, .T. ) ;
#46470=CARTESIAN_POINT ( 'NONE',  ( -7.846153846153965716, -6.879047030192662504, 34.71129190930017927 ) ) ;
#46471=B_SPLINE_CURVE_WITH_KNOTS ( 'NONE', 3,
 ( #63980, #76628, #50032, #70310, #50896, #22127, #21678, #14933, #50466, #43286 ),
 .UNSPECIFIED., .F., .F.,
 ( 4, 2, 2, 2, 4 ),
 ( 0.0007817246256747451124, 0.0009771112852218881168, 0.001172497944769031230, 0.001367884604316174126, 0.001563271263863317238 ),
 .UNSPECIFIED. ) ;
#46472=B_SPLINE_CURVE_WITH_KNOTS ( 'NONE', 3,
 ( #38217, #80999, #12100, #66127, #18399, #32802, #72886, #60263, #11648, #80097 ),
 .UNSPECIFIED., .F., .F.,
 ( 4, 2, 2, 2, 4 ),
 ( 0.000000000000000000, 0.0001954339857564063360, 0.0003908679715128126719, 0.0005863019572692189808, 0.0007817359430256253438 ),
 .UNSPECIFIED. ) ;
#46474=CARTESIAN_POINT ( 'NONE',  ( 18.00000000000000000, -2.499999999999998668, 29.75000000000001421 ) ) ;
#46475=EDGE_CURVE ( 'NONE', #42820, #84034, #73397, .T. ) ;
#46476=CARTESIAN_POINT ( 'NONE',  ( 11.53846153846153832, -9.819645486525091727, 36.12317359536749706 ) ) ;
#46477=CARTESIAN_POINT ( 'NONE',  ( -2.372962308248625529, -3.083524468853724443, 32.58852847137143272 ) ) ;
#46480=CARTESIAN_POINT ( 'NONE',  ( 15.10007776410167324, -8.147922237126337563, 34.70805685702651999 ) ) ;
#46481=CARTESIAN_POINT ( 'NONE',  ( -9.561781990544128362, -8.586989748646452369, 34.63063291749215011 ) ) ;
#46482=CARTESIAN_POINT ( 'NONE',  ( -13.38461538461538325, -8.120952969808772792, 34.71129190930000163 ) ) ;
#46483=EDGE_CURVE ( 'NONE', #78412, #54915, #70205, .T. ) ;
#46485=CARTESIAN_POINT ( 'NONE',  ( 8.068933515131909928, -12.11081565061823717, 32.26097654155341843 ) ) ;
#46486=CARTESIAN_POINT ( 'NONE',  ( 11.53846153846141576, -12.70778746994576025, 30.41441678777401236 ) ) ;
#46487=CARTESIAN_POINT ( 'NONE',  ( 13.25446817517716447, -3.817052484675422797, 33.13202310037935661 ) ) ;
#46488=CARTESIAN_POINT ( 'NONE',  ( -10.74553258511630993, -2.373036134822904319, 30.88089517874952250 ) ) ;
#46492=ORIENTED_EDGE ( 'NONE', *, *, #55778, .T. ) ;
#46493=DIRECTION ( 'NONE',  ( -0.000000000000000000, 0.9848077530122086864, -0.1736481776669273891 ) ) ;
#46494=DIRECTION ( 'NONE',  ( 0.000000000000000000, 0.9396926207859126468, -0.3420201433256571111 ) ) ;
#46495=CARTESIAN_POINT ( 'NONE',  ( -2.177166869458661225, -5.915461855592777596, 34.75538340440931506 ) ) ;
#46496=ORIENTED_EDGE ( 'NONE', *, *, #50471, .F. ) ;
#46497=CARTESIAN_POINT ( 'NONE',  ( 13.51514108637895006, -6.852161475712352789, 34.70806712695775786 ) ) ;
#46498=VERTEX_POINT ( 'NONE', #69834 ) ;
#46499=CYLINDRICAL_SURFACE ( 'NONE', #62984, 0.2499999999999986955 ) ;
#46500=DIRECTION ( 'NONE',  ( 0.000000000000000000, 0.6427876096865373645, -0.7660444431189797898 ) ) ;
#46503=LINE ( 'NONE', #26673, #10225 ) ;
#46504=CARTESIAN_POINT ( 'NONE',  ( -14.37294223946638994, -2.255955759149247619, 30.00000000000013856 ) ) ;
#46505=LINE ( 'NONE', #32106, #76794 ) ;
#46506=CARTESIAN_POINT ( 'NONE',  ( 8.546352086802123438, -7.630691491037285168, 34.74850469731152458 ) ) ;
#46507=CYLINDRICAL_SURFACE ( 'NONE', #85735, 0.2499999999999986955 ) ;
#46508=B_SPLINE_CURVE_WITH_KNOTS ( 'NONE', 3,
 ( #71452, #37674, #57943, #71900, #44411, #86334, #85424, #70582, #71020, #37224 ),
 .UNSPECIFIED., .F., .F.,
 ( 4, 2, 2, 2, 4 ),
 ( 0.000000000000000000, 0.0001954311564186879857, 0.0003908623128373759715, 0.0005862934692560640114, 0.0007817246256747519429 ),
 .UNSPECIFIED. ) ;
#46510=CIRCLE ( 'NONE', #74034, 0.2500000000000002220 ) ;
#46511=ORIENTED_EDGE ( 'NONE', *, *, #33885, .T. ) ;
#46512=CARTESIAN_POINT ( 'NONE',  ( -3.903900744468109973, -12.45601412856602863, 31.48342859153981621 ) ) ;
#46513=VERTEX_POINT ( 'NONE', #42817 ) ;
#46514=CARTESIAN_POINT ( 'NONE',  ( -15.16470189741915675, -6.343179335718452272, 34.87096338111212646 ) ) ;
#46515=EDGE_CURVE ( 'NONE', #75445, #41883, #82017, .T. ) ;
#46516=AXIS2_PLACEMENT_3D ( 'NONE', #10490, #72175, #65857 ) ;
#46517=CYLINDRICAL_SURFACE ( 'NONE', #24911, 0.2499999999999998890 ) ;
#46518=EDGE_CURVE ( 'NONE', #27949, #15069, #8586, .T. ) ;
#46520=CARTESIAN_POINT ( 'NONE',  ( -16.15384615384627409, -11.48612834414049644, 32.76840700105863391 ) ) ;
#46521=CARTESIAN_POINT ( 'NONE',  ( 5.999999999999880096, -9.442884908241554243, 34.35708131394783038 ) ) ;
#46522=CYLINDRICAL_SURFACE ( 'NONE', #78081, 0.2499999999999986955 ) ;
#46524=DIRECTION ( 'NONE',  ( -0.000000000000000000, -0.000000000000000000, -1.000000000000000000 ) ) ;
#46525=B_SPLINE_CURVE_WITH_KNOTS ( 'NONE', 3,
 ( #37139, #84025, #22305, #64160, #9673, #16434, #36271, #78131, #2462, #49769 ),
 .UNSPECIFIED., .F., .F.,
 ( 4, 2, 2, 2, 4 ),
 ( 0.0007817246256747530271, 0.0009771112852218978746, 0.001172497944769042939, 0.001367884604316188003, 0.001563271263863332851 ),
 .UNSPECIFIED. ) ;
#46526=ORIENTED_EDGE ( 'NONE', *, *, #64727, .F. ) ;
#46527=EDGE_CURVE ( 'NONE', #43756, #37230, #26742, .T. ) ;
#46529=VERTEX_POINT ( 'NONE', #63061 ) ;
#46530=ORIENTED_EDGE ( 'NONE', *, *, #81563, .T. ) ;
#46531=CARTESIAN_POINT ( 'NONE',  ( 2.177000841024750333, -4.809359713505814149, 33.96456829005828837 ) ) ;
#46532=CARTESIAN_POINT ( 'NONE',  ( 11.28843831424008393, -9.356822207818506598, 34.66110646841856635 ) ) ;
#46533=CARTESIAN_POINT ( 'NONE',  ( 15.16468581981335184, -4.786620604624113540, 33.94971097300155805 ) ) ;
#46534=CARTESIAN_POINT ( 'NONE',  ( 4.087762742890272527, -3.050289026998445951, 32.03036669348365706 ) ) ;
#46535=CARTESIAN_POINT ( 'NONE',  ( 20.74999999999999645, -2.499999999999999556, 29.75000000000000355 ) ) ;
#46536=FACE_OUTER_BOUND ( 'NONE', #14392, .T. ) ;
#46540=EDGE_CURVE ( 'NONE', #17613, #54993, #40716, .T. ) ;
#46541=ORIENTED_EDGE ( 'NONE', *, *, #28575, .T. ) ;
#46542=EDGE_LOOP ( 'NONE', ( #66272, #69825, #27160, #74587 ) ) ;
#46543=CARTESIAN_POINT ( 'NONE',  ( -11.76138775597768138, -12.39988816332205701, 30.74660775122750778 ) ) ;
#46544=VERTEX_POINT ( 'NONE', #28863 ) ;
#46545=DIRECTION ( 'NONE',  ( 0.000000000000000000, 0.000000000000000000, 1.000000000000000000 ) ) ;
#46546=FACE_OUTER_BOUND ( 'NONE', #88420, .T. ) ;
#46547=CARTESIAN_POINT ( 'NONE',  ( 11.28846153846153832, -7.500000000000001776, 35.00000000000000000 ) ) ;
#46548=CARTESIAN_POINT ( 'NONE',  ( -10.86536134632696715, -3.627789207965226748, 32.91389620160131102 ) ) ;
#46549=FACE_BOUND ( 'NONE', #43714, .T. ) ;
#46550=ORIENTED_EDGE ( 'NONE', *, *, #73424, .T. ) ;
#46551=ORIENTED_EDGE ( 'NONE', *, *, #43740, .F. ) ;
#46553=VERTEX_POINT ( 'NONE', #77476 ) ;
#46554=FACE_BOUND ( 'NONE', #62615, .T. ) ;
#46555=B_SPLINE_CURVE_WITH_KNOTS ( 'NONE', 3,
 ( #76389, #83156, #56565, #49366, #83612, #84055, #22335, #41727, #55229, #82718 ),
 .UNSPECIFIED., .F., .F.,
 ( 4, 2, 2, 2, 4 ),
 ( 0.000000000000000000, 0.0001954311564186861155, 0.0003908623128373722310, 0.0005862934692560583735, 0.0007817246256747444619 ),
 .UNSPECIFIED. ) ;
#46556=DIRECTION ( 'NONE',  ( 0.000000000000000000, 0.9848077530122072432, -0.1736481776669354937 ) ) ;
#46557=CARTESIAN_POINT ( 'NONE',  ( 14.98074600654777733, -6.652501968072648708, 34.93155406624980941 ) ) ;
#46559=DIRECTION ( 'NONE',  ( -0.000000000000000000, 0.1736481776669307198, -0.9848077530122080203 ) ) ;
#46560=CARTESIAN_POINT ( 'NONE',  ( -3.480769230769229061, -7.500000000000001776, 35.04278698407183867 ) ) ;
#46562=VERTEX_POINT ( 'NONE', #61399 ) ;
#46563=CARTESIAN_POINT ( 'NONE',  ( 14.37375964104238335, -3.322132147404559976, 32.92929555188717927 ) ) ;
#46564=CARTESIAN_POINT ( 'NONE',  ( -18.06608341095587633, -4.786620604624111763, 33.94971097300155805 ) ) ;
#46565=DIRECTION ( 'NONE',  ( 0.000000000000000000, 0.8660254037844377084, 0.5000000000000015543 ) ) ;
#46567=CARTESIAN_POINT ( 'NONE',  ( 2.530471976670372491, -12.47679350104403007, 31.42216943046555855 ) ) ;
#46568=CARTESIAN_POINT ( 'NONE',  ( -15.36091644020745051, -4.460286881179644780, 33.72017969459903242 ) ) ;
#46569=EDGE_LOOP ( 'NONE', ( #25995, #82944, #79296, #53656 ) ) ;
#46570=DIRECTION ( 'NONE',  ( -0.000000000000000000, 0.9396926207859093161, -0.3420201433256663259 ) ) ;
#46571=CARTESIAN_POINT ( 'NONE',  ( -4.403822884788509029, -2.564618984488975961, 30.55390908950641915 ) ) ;
#46572=CARTESIAN_POINT ( 'NONE',  ( -0.2115384615384615641, -7.500000000000001776, 35.04278698407183867 ) ) ;
#46573=CARTESIAN_POINT ( 'NONE',  ( 13.38461538461526601, -12.46129190930018460, 30.37095296980731973 ) ) ;
#46574=CARTESIAN_POINT ( 'NONE',  ( -10.55012904410858532, -2.625532179533470512, 30.86335684631491105 ) ) ;
#46575=CARTESIAN_POINT ( 'NONE',  ( 6.673100192134570285, -9.148715823498378086, 34.47080413974185120 ) ) ;
#46576=CARTESIAN_POINT ( 'NONE',  ( 0.7115928814519140166, -11.47946981652013498, 33.17500667209846910 ) ) ;
#46578=CARTESIAN_POINT ( 'NONE',  ( 9.758375025657770152, -4.661471528628508665, 34.16647553114624003 ) ) ;
#46579=EDGE_CURVE ( 'NONE', #5299, #20780, #4638, .T. ) ;
#46580=CARTESIAN_POINT ( 'NONE',  ( 10.74591005361826035, -9.503571793651731880, 34.60286762892837942 ) ) ;
#46581=CARTESIAN_POINT ( 'NONE',  ( -12.21159294319032185, -11.37275283266504111, 32.91324779482534524 ) ) ;
#46583=ORIENTED_EDGE ( 'NONE', *, *, #34004, .T. ) ;
#46584=B_SPLINE_CURVE_WITH_KNOTS ( 'NONE', 3,
 ( #46364, #52220, #45017, #79712, #86938, #86484, #52667, #66639, #45911, #10805 ),
 .UNSPECIFIED., .F., .F.,
 ( 4, 2, 2, 2, 4 ),
 ( 0.0007817246256747516176, 0.0009771112852218965736, 0.001172497944769041421, 0.001367884604316186269, 0.001563271263863331333 ),
 .UNSPECIFIED. ) ;
#46585=VECTOR ( 'NONE', #45828, 1000.000000000000114 ) ;
#46586=DIRECTION ( 'NONE',  ( -0.000000000000000000, -0.000000000000000000, -1.000000000000000000 ) ) ;
#46587=EDGE_LOOP ( 'NONE', ( #48599, #49592, #2675, #46205 ) ) ;
#46588=EDGE_CURVE ( 'NONE', #39037, #71584, #15786, .T. ) ;
#46589=AXIS2_PLACEMENT_3D ( 'NONE', #24254, #36462, #85532 ) ;
#46590=ORIENTED_EDGE ( 'NONE', *, *, #16152, .T. ) ;
#46591=CARTESIAN_POINT ( 'NONE',  ( -2.307692307692427391, -12.46129190930018460, 30.37095296980731973 ) ) ;
#46592=EDGE_CURVE ( 'NONE', #88144, #62981, #28231, .T. ) ;
#46594=DIRECTION ( 'NONE',  ( -0.000000000000000000, 0.7660444431189791237, -0.6427876096865379196 ) ) ;
#46596=CARTESIAN_POINT ( 'NONE',  ( 13.63456090296353018, -2.824170634883621744, 31.52227843825338738 ) ) ;
#46597=CARTESIAN_POINT ( 'NONE',  ( 10.61538461538449418, -2.657715359629662544, 31.77849191805970364 ) ) ;
#46598=CARTESIAN_POINT ( 'NONE',  ( 3.230769230769231726, -11.69971097300155272, 32.46337939537588113 ) ) ;
#46599=CARTESIAN_POINT ( 'NONE',  ( -10.39260494640654642, -3.563462043263030399, 33.22394488606062879 ) ) ;
#46600=CARTESIAN_POINT ( 'NONE',  ( -15.36091720050093024, -5.070767119584671079, 34.40440758774516183 ) ) ;
#46601=CARTESIAN_POINT ( 'NONE',  ( 2.307692307692309264, -11.16473453929635440, 33.15142922261926373 ) ) ;
#46602=ADVANCED_FACE ( 'NONE', ( #73386 ), #4018, .F. ) ;
#46603=B_SPLINE_CURVE_WITH_KNOTS ( 'NONE', 3,
 ( #77609, #56883, #49690, #64079, #37048, #17230, #36196, #10028, #57775, #23106 ),
 .UNSPECIFIED., .F., .F.,
 ( 4, 2, 2, 2, 4 ),
 ( 0.000000000000000000, 0.0001954339857564090465, 0.0003908679715128180929, 0.0005863019572692271123, 0.0007817359430256361858 ),
 .UNSPECIFIED. ) ;
#46605=LINE ( 'NONE', #74083, #46299 ) ;
#46606=CARTESIAN_POINT ( 'NONE',  ( -4.153846153846152411, -11.91647553114624181, 32.58852847137148245 ) ) ;
#46607=ADVANCED_FACE ( 'NONE', ( #38264 ), #72039, .F. ) ;
#46611=CARTESIAN_POINT ( 'NONE',  ( -11.28840722682322273, -5.728107161865378494, 34.42597550085002922 ) ) ;
#46612=CARTESIAN_POINT ( 'NONE',  ( -17.14300648787895298, -8.120952969808774569, 34.71129190930000163 ) ) ;
#46613=DIRECTION ( 'NONE',  ( 0.000000000000000000, 0.3420201433256610524, 0.9396926207859113145 ) ) ;
#46614=CARTESIAN_POINT ( 'NONE',  ( -7.173100147298380413, -5.765609946408404518, 34.70566812827425451 ) ) ;
#46615=CARTESIAN_POINT ( 'NONE',  ( -7.596153846153844924, -7.500000000000001776, 35.04278698407183867 ) ) ;
#46616=CARTESIAN_POINT ( 'NONE',  ( -4.826977667545031991, -2.986452184633680673, 32.43230066228895225 ) ) ;
#46617=ORIENTED_EDGE ( 'NONE', *, *, #12940, .F. ) ;
#46618=CARTESIAN_POINT ( 'NONE',  ( 1.253923917947828315, -4.809359713505814149, 33.96456829005828837 ) ) ;
#46620=EDGE_CURVE ( 'NONE', #36760, #82738, #44330, .T. ) ;
#46621=ORIENTED_EDGE ( 'NONE', *, *, #63148, .F. ) ;
#46622=CARTESIAN_POINT ( 'NONE',  ( -8.769230769230768274, -4.661471528628507777, 34.16647553114623292 ) ) ;
#46623=CARTESIAN_POINT ( 'NONE',  ( -14.05763788777885281, -6.523592122091592671, 34.90882529074906415 ) ) ;
#46624=ADVANCED_FACE ( 'NONE', ( #86474 ), #85564, .F. ) ;
#46625=CARTESIAN_POINT ( 'NONE',  ( -9.561781990544126586, -6.852161475712352789, 34.70806712695775786 ) ) ;
#46626=CARTESIAN_POINT ( 'NONE',  ( -4.153846153846152411, -9.905515769479276145, 34.41647553114623292 ) ) ;
#46627=CARTESIAN_POINT ( 'NONE',  ( -13.38461538461538325, -2.486705287966279876, 31.30864560766543647 ) ) ;
#46628=B_SPLINE_CURVE_WITH_KNOTS ( 'NONE', 3,
 ( #46974, #67704, #6011, #1015, #13204, #33477, #20403, #14084, #28488, #48751 ),
 .UNSPECIFIED., .F., .F.,
 ( 4, 2, 2, 2, 4 ),
 ( 0.0007817246256747461966, 0.0009771112852218892010, 0.001172497944769032314, 0.001367884604316175427, 0.001563271263863318323 ),
 .UNSPECIFIED. ) ;
#46629=ORIENTED_EDGE ( 'NONE', *, *, #41341, .T. ) ;
#46630=ADVANCED_FACE ( 'NONE', ( #58515 ), #45455, .F. ) ;
#46632=B_SPLINE_CURVE_WITH_KNOTS ( 'NONE', 3,
 ( #10757, #78765, #17065, #72006, #37779, #10313, #65684, #3983, #31469, #86441 ),
 .UNSPECIFIED., .F., .F.,
 ( 4, 2, 2, 2, 4 ),
 ( 0.0007817359527651101701, 0.0009771254036996489256, 0.001172514854634187790, 0.001367904305568726653, 0.001563293756503265517 ),
 .UNSPECIFIED. ) ;
#46633=ORIENTED_EDGE ( 'NONE', *, *, #73529, .F. ) ;
#46634=EDGE_CURVE ( 'NONE', #7438, #9134, #3505, .T. ) ;
#46635=CARTESIAN_POINT ( 'NONE',  ( -16.15384615384615330, -2.708943851104267164, 35.45975837776705220 ) ) ;
#46636=CARTESIAN_POINT ( 'NONE',  ( -0.3310130233048168558, -10.31582465632705237, 34.18122507451815295 ) ) ;
#46637=CARTESIAN_POINT ( 'NONE',  ( 16.37685899793955357, -5.582272713120730145, 34.63742843783360570 ) ) ;
#46639=CARTESIAN_POINT ( 'NONE',  ( -16.28453675695646652, -2.295517848115768089, 30.44137282052136939 ) ) ;
#46640=CARTESIAN_POINT ( 'NONE',  ( 4.153846153846154188, -1.509761064869970415, 31.06009739812519044 ) ) ;
#46641=DIRECTION ( 'NONE',  ( 0.000000000000000000, 0.3420201433256641055, -0.9396926207859100932 ) ) ;
#46643=ADVANCED_FACE ( 'NONE', ( #31047 ), #80144, .F. ) ;
#46644=ORIENTED_EDGE ( 'NONE', *, *, #24872, .T. ) ;
#46645=CARTESIAN_POINT ( 'NONE',  ( -10.54931626438217585, -11.69971097300155272, 32.46337939537588113 ) ) ;
#46647=EDGE_CURVE ( 'NONE', #82252, #33999, #67976, .T. ) ;
#46648=DIRECTION ( 'NONE',  ( -0.000000000000000000, 0.3420201433256694346, -0.9396926207859080948 ) ) ;
#46649=CARTESIAN_POINT ( 'NONE',  ( -2.084912638714238486, -4.226511098958374291, 33.85474049983370293 ) ) ;
#46650=EDGE_CURVE ( 'NONE', #73234, #41543, #3132, .T. ) ;
#46652=EDGE_LOOP ( 'NONE', ( #20108, #46981, #85506, #89099 ) ) ;
#46653=CARTESIAN_POINT ( 'NONE',  ( 8.069166690247241647, -4.026326845037962343, 33.68677907613344047 ) ) ;
#46654=ORIENTED_EDGE ( 'NONE', *, *, #45799, .F. ) ;
#46655=EDGE_CURVE ( 'NONE', #71986, #37663, #47527, .T. ) ;
#46656=CARTESIAN_POINT ( 'NONE',  ( 2.242421861731533017, -6.879047030191174805, 34.71129190930000163 ) ) ;
#46657=CARTESIAN_POINT ( 'NONE',  ( 0.3313904918067637762, -11.66186481527757124, 32.95055677023625407 ) ) ;
#46658=CARTESIAN_POINT ( 'NONE',  ( -12.39547011053602432, -12.37446782046654192, 30.86335684631486842 ) ) ;
#46659=B_SPLINE_CURVE_WITH_KNOTS ( 'NONE', 3,
 ( #43946, #57460, #17823, #30870, #65545, #58340, #85835, #59239, #78180, #3847 ),
 .UNSPECIFIED., .F., .F.,
 ( 4, 2, 2, 2, 4 ),
 ( 0.0007817359430256366195, 0.0009771253907250045632, 0.001172514838424372615, 0.001367904286123740668, 0.001563293733823108503 ),
 .UNSPECIFIED. ) ;
#46660=CARTESIAN_POINT ( 'NONE',  ( -5.010854725920638408, -12.10708131394839882, 31.69288490824020954 ) ) ;
#46663=CARTESIAN_POINT ( 'NONE',  ( -11.28840711854808632, -8.346898887586323923, 34.93166121998716278 ) ) ;
#46664=DIRECTION ( 'NONE',  ( 0.000000000000000000, 0.1736481776669275834, 0.9848077530122086864 ) ) ;
#46666=AXIS2_PLACEMENT_3D ( 'NONE', #9441, #53411, #66497 ) ;
#46667=CARTESIAN_POINT ( 'NONE',  ( -18.00000000000012079, -12.70778746994576025, 30.41441678777401236 ) ) ;
#46668=CARTESIAN_POINT ( 'NONE',  ( 14.43848274865925774, -9.929761469519743144, 34.40412654351204225 ) ) ;
#46669=CARTESIAN_POINT ( 'NONE',  ( -10.61538461538461320, -2.292212530054420494, 30.41441678777542634 ) ) ;
#46670=CARTESIAN_POINT ( 'NONE',  ( 0.4615384615384611200, -2.708943851104267164, 35.45975837776705220 ) ) ;
#46671=DIRECTION ( 'NONE',  ( -0.000000000000000000, 0.1736481776669307198, -0.9848077530122080203 ) ) ;
#46672=FACE_BOUND ( 'NONE', #16321, .T. ) ;
#46673=DIRECTION ( 'NONE',  ( -0.000000000000000000, 0.8660254037844397068, -0.4999999999999978906 ) ) ;
#46674=CARTESIAN_POINT ( 'NONE',  ( 16.15384615384615330, -6.681629849574314051, 35.83090037661290239 ) ) ;
#46675=CARTESIAN_POINT ( 'NONE',  ( 9.822352855142472805, -2.504778602574659896, 29.97347330155780654 ) ) ;
#46676=CARTESIAN_POINT ( 'NONE',  ( -18.22292695890684655, -2.308479472611653094, 30.53278059502174457 ) ) ;
#46677=CARTESIAN_POINT ( 'NONE',  ( -2.307692307692428724, -12.51329471203414379, 31.30864560766407578 ) ) ;
#46678=CARTESIAN_POINT ( 'NONE',  ( 8.900021210197715860, -12.62708834333097663, 30.88030960425257021 ) ) ;
#46681=CARTESIAN_POINT ( 'NONE',  ( 10.61538461538461675, -11.91647553114624181, 32.58852847137148245 ) ) ;
#46682=ORIENTED_EDGE ( 'NONE', *, *, #33774, .F. ) ;
#46683=CARTESIAN_POINT ( 'NONE',  ( -18.06608237936013239, -3.322132147404557312, 32.92929555188717217 ) ) ;
#46685=CARTESIAN_POINT ( 'NONE',  ( 7.596177115211490971, -9.148715823498378086, 34.47080413974185120 ) ) ;
#46686=LINE ( 'NONE', #6149, #84805 ) ;
#46688=VERTEX_POINT ( 'NONE', #88698 ) ;
#46689=CARTESIAN_POINT ( 'NONE',  ( 3.453548772037639214, -6.760870238392817200, 34.69528174975672385 ) ) ;
#46690=DIRECTION ( 'NONE',  ( -1.000000000000000000, 0.000000000000000000, 0.000000000000000000 ) ) ;
#46692=CARTESIAN_POINT ( 'NONE',  ( -12.21153846153846168, -2.499999999999998668, 29.75000000000000355 ) ) ;
#46696=CARTESIAN_POINT ( 'NONE',  ( -7.146003140593069070, -4.186968288167446595, 33.49512374952580274 ) ) ;
#46697=DIRECTION ( 'NONE',  ( 0.000000000000000000, 0.9396926207859126468, 0.3420201433256571111 ) ) ;
#46698=EDGE_CURVE ( 'NONE', #36558, #16973, #63654, .T. ) ;
#46700=AXIS2_PLACEMENT_3D ( 'NONE', #4443, #40472, #47656 ) ;
#46701=CARTESIAN_POINT ( 'NONE',  ( 5.142178216435913107, -2.657715359629131857, 31.77849191805844242 ) ) ;
#46702=CARTESIAN_POINT ( 'NONE',  ( -11.53846153846153655, -10.51840700105979565, 33.73612834413961536 ) ) ;
#46703=ORIENTED_EDGE ( 'NONE', *, *, #2310, .T. ) ;
#46704=ADVANCED_FACE ( 'NONE', ( #26979 ), #20219, .F. ) ;
#46705=CARTESIAN_POINT ( 'NONE',  ( 16.15384615384603251, -5.094484230521993062, 34.41647553114689373 ) ) ;
#46706=DIRECTION ( 'NONE',  ( 0.000000000000000000, 0.4999999999999960032, -0.8660254037844410391 ) ) ;
#46709=CARTESIAN_POINT ( 'NONE',  ( -10.74553258511631704, -2.647304123082328875, 31.75400227202885972 ) ) ;
#46710=LINE ( 'NONE', #6612, #16730 ) ;
#46711=VERTEX_POINT ( 'NONE', #40934 ) ;
#46713=CARTESIAN_POINT ( 'NONE',  ( 9.468822767743363400, -12.69144148231606017, 30.53333754910549303 ) ) ;
#46714=CARTESIAN_POINT ( 'NONE',  ( 5.076923076922953193, -12.51329471203414379, 31.30864560766407578 ) ) ;
#46715=ORIENTED_EDGE ( 'NONE', *, *, #59685, .F. ) ;
#46716=CARTESIAN_POINT ( 'NONE',  ( -8.096130577096200653, -8.303909089506435137, 34.68538101551103381 ) ) ;
#46717=CARTESIAN_POINT ( 'NONE',  ( -3.164700879766791708, -3.513871655860379306, 32.76840700105978499 ) ) ;
#46718=CARTESIAN_POINT ( 'NONE',  ( 2.057715576749954423, -12.41269422305637171, 30.68257228309993323 ) ) ;
#46719=CARTESIAN_POINT ( 'NONE',  ( 11.76147289007438701, -9.086983370893049639, 34.49168942202179267 ) ) ;
#46720=ADVANCED_FACE ( 'NONE', ( #39170 ), #74726, .F. ) ;
#46721=ORIENTED_EDGE ( 'NONE', *, *, #65950, .F. ) ;
#46722=CARTESIAN_POINT ( 'NONE',  ( 2.307692307692186251, -6.835583212225970762, 34.95778746994575670 ) ) ;
#46723=CARTESIAN_POINT ( 'NONE',  ( -15.48079245499068612, -11.56360843649121684, 33.07473185843129926 ) ) ;
#46724=CARTESIAN_POINT ( 'NONE',  ( -13.25408994638174143, -8.630441415882550871, 34.87705825610312615 ) ) ;
#46725=ORIENTED_EDGE ( 'NONE', *, *, #53694, .T. ) ;
#46726=ORIENTED_EDGE ( 'NONE', *, *, #70965, .F. ) ;
#46727=EDGE_CURVE ( 'NONE', #26582, #41513, #30315, .T. ) ;
#46728=B_SPLINE_CURVE_WITH_KNOTS ( 'NONE', 3,
 ( #69738, #55331, #83714, #35513, #21997, #50333, #42280, #43588, #49471, #69303 ),
 .UNSPECIFIED., .F., .F.,
 ( 4, 2, 2, 2, 4 ),
 ( 0.000000000000000000, 0.0001954311584214072381, 0.0003908623168428144762, 0.0005862934752642217414, 0.0007817246336856289524 ),
 .UNSPECIFIED. ) ;
#46729=ORIENTED_EDGE ( 'NONE', *, *, #66799, .T. ) ;
#46730=CARTESIAN_POINT ( 'NONE',  ( 24.00000000000000000, -5.499999999999981348, 27.75000000000000000 ) ) ;
#46731=CARTESIAN_POINT ( 'NONE',  ( -6.857821351800898135, -4.481592998940251427, 33.73612834413965089 ) ) ;
#46732=ADVANCED_FACE ( 'NONE', ( #54434 ), #11692, .F. ) ;
#46734=AXIS2_PLACEMENT_3D ( 'NONE', #78924, #79829, #18125 ) ;
#46735=CARTESIAN_POINT ( 'NONE',  ( -18.25000000000001066, -7.431102191622666275, 35.00000000000000711 ) ) ;
#46736=ORIENTED_EDGE ( 'NONE', *, *, #57441, .F. ) ;
#46737=ORIENTED_EDGE ( 'NONE', *, *, #50912, .T. ) ;
#46738=EDGE_CURVE ( 'NONE', #42538, #71827, #59864, .T. ) ;
#46739=ORIENTED_EDGE ( 'NONE', *, *, #71759, .T. ) ;
#46740=CARTESIAN_POINT ( 'NONE',  ( -6.989159302437059296, -2.486705287966279432, 31.30864560766542937 ) ) ;
#46741=ORIENTED_EDGE ( 'NONE', *, *, #22430, .F. ) ;
#46742=CARTESIAN_POINT ( 'NONE',  ( -6.923076923076922462, -3.937682226553329556, 33.60647404775216529 ) ) ;
#46743=CARTESIAN_POINT ( 'NONE',  ( -3.296851610129365451, -4.661471528628506888, 34.16647553114621871 ) ) ;
#46744=CYLINDRICAL_SURFACE ( 'NONE', #52231, 0.2500000000000012212 ) ;
#46745=CARTESIAN_POINT ( 'NONE',  ( 16.15384615384615330, -5.180354513474913603, 36.12317359536750416 ) ) ;
#46746=ORIENTED_EDGE ( 'NONE', *, *, #50911, .F. ) ;
#46747=ADVANCED_FACE ( 'NONE', ( #46799 ), #47683, .F. ) ;
#46748=ORIENTED_EDGE ( 'NONE', *, *, #436, .T. ) ;
#46750=CARTESIAN_POINT ( 'NONE',  ( 10.61538461538461675, -10.51840700105979565, 33.73612834413961536 ) ) ;
#46751=CARTESIAN_POINT ( 'NONE',  ( -10.61538461538461320, -2.486705287966279876, 31.30864560766543647 ) ) ;
#46752=VERTEX_POINT ( 'NONE', #25641 ) ;
#46753=CARTESIAN_POINT ( 'NONE',  ( 2.057669083470849980, -2.588893531581426544, 31.60682220781847818 ) ) ;
#46754=EDGE_CURVE ( 'NONE', #66607, #42352, #33518, .T. ) ;
#46755=ADVANCED_FACE ( 'NONE', ( #61186 ), #26085, .F. ) ;
#46756=AXIS2_PLACEMENT_3D ( 'NONE', #5911, #47778, #12668 ) ;
#46757=CARTESIAN_POINT ( 'NONE',  ( -13.51476259405360381, -6.852621066184266141, 34.70813303252209181 ) ) ;
#46758=ORIENTED_EDGE ( 'NONE', *, *, #16946, .T. ) ;
#46759=FACE_OUTER_BOUND ( 'NONE', #87463, .T. ) ;
#46760=B_SPLINE_CURVE_WITH_KNOTS ( 'NONE', 3,
 ( #35867, #40852, #7510, #15151, #63326, #34967, #68318, #82287, #14707, #1638 ),
 .UNSPECIFIED., .F., .F.,
 ( 4, 2, 2, 2, 4 ),
 ( 0.000000000000000000, 0.0001954311564186862510, 0.0003908623128373725020, 0.0005862934692560588072, 0.0007817246256747450040 ),
 .UNSPECIFIED. ) ;
#46761=CARTESIAN_POINT ( 'NONE',  ( -3.903900635498011251, -5.057305518903949526, 34.11320923018887896 ) ) ;
#46762=LINE ( 'NONE', #89101, #72741 ) ;
#46763=FACE_BOUND ( 'NONE', #83575, .T. ) ;
#46764=CARTESIAN_POINT ( 'NONE',  ( -18.00000000000000000, -8.120952969808772792, 34.71129190930000163 ) ) ;
#46765=DIRECTION ( 'NONE',  ( -0.000000000000000000, 0.3420201433256694901, -0.9396926207859082059 ) ) ;
#46766=B_SPLINE_CURVE_WITH_KNOTS ( 'NONE', 3,
 ( #65620, #58417, #64733, #43586, #51651, #22434, #49899, #9372, #50770, #36831 ),
 .UNSPECIFIED., .F., .F.,
 ( 4, 2, 2, 2, 4 ),
 ( 0.000000000000000000, 0.0001954339857564053873, 0.0003908679715128107746, 0.0005863019572692161618, 0.0007817359430256215491 ),
 .UNSPECIFIED. ) ;
#46767=VECTOR ( 'NONE', #6933, 999.9999999999998863 ) ;
#46768=CARTESIAN_POINT ( 'NONE',  ( 11.60371710973756443, -12.46129190930001052, 30.37095296980870174 ) ) ;
#46769=CARTESIAN_POINT ( 'NONE',  ( 11.53846153846153832, -6.681629849574314051, 35.83090037661290239 ) ) ;
#46770=FACE_OUTER_BOUND ( 'NONE', #49501, .T. ) ;
#46771=DIRECTION ( 'NONE',  ( -0.000000000000000000, -0.9848077530122086864, -0.1736481776669273613 ) ) ;
#46772=CARTESIAN_POINT ( 'NONE',  ( -0.4615384615384611200, -3.513871655860378418, 32.76840700105978499 ) ) ;
#46773=ORIENTED_EDGE ( 'NONE', *, *, #59019, .F. ) ;
#46775=AXIS2_PLACEMENT_3D ( 'NONE', #59369, #23790, #24237 ) ;
#46776=CARTESIAN_POINT ( 'NONE',  ( -6.923076923077044142, -10.90142922262034020, 33.41473453929536674 ) ) ;
#46777=ORIENTED_EDGE ( 'NONE', *, *, #24673, .T. ) ;
#46778=ORIENTED_EDGE ( 'NONE', *, *, #28620, .T. ) ;
#46779=CARTESIAN_POINT ( 'NONE',  ( -6.857821351800898135, -5.219633306516380244, 34.19971097300157936 ) ) ;
#46780=CARTESIAN_POINT ( 'NONE',  ( -13.44988538517170440, -5.094484230520674117, 34.41647553114621161 ) ) ;
#46781=CARTESIAN_POINT ( 'NONE',  ( -15.48076923076923173, -7.433931650972299465, 34.75000000000000711 ) ) ;
#46783=CARTESIAN_POINT ( 'NONE',  ( 14.43821800945587341, -9.417988943895561960, 34.36773134775777550 ) ) ;
#46785=FACE_BOUND ( 'NONE', #17205, .T. ) ;
#46786=CARTESIAN_POINT ( 'NONE',  ( -15.45425417449318317, -5.912607949931405926, 34.49155766932282319 ) ) ;
#46788=LINE ( 'NONE', #40920, #33004 ) ;
#46789=LINE ( 'NONE', #26966, #55372 ) ;
#46791=CARTESIAN_POINT ( 'NONE',  ( 2.057669083470850424, -10.92453946501458439, 33.72985991061850086 ) ) ;
#46793=ORIENTED_EDGE ( 'NONE', *, *, #64593, .F. ) ;
#46794=ORIENTED_EDGE ( 'NONE', *, *, #11265, .T. ) ;
#46795=CARTESIAN_POINT ( 'NONE',  ( 2.307692307692187583, -12.27809138561165270, 31.22303859784587132 ) ) ;
#46796=CARTESIAN_POINT ( 'NONE',  ( -17.74994558008654622, -3.435999193479609470, 33.07426656108012253 ) ) ;
#46797=DIRECTION ( 'NONE',  ( -0.000000000000000000, -0.9396926207859093161, -0.3420201433256663259 ) ) ;
#46799=FACE_OUTER_BOUND ( 'NONE', #38539, .T. ) ;
#46801=CARTESIAN_POINT ( 'NONE',  ( -1.384615384615383471, -3.937682226553329556, 33.60647404775216529 ) ) ;
#46802=FACE_OUTER_BOUND ( 'NONE', #44796, .T. ) ;
#46803=AXIS2_PLACEMENT_3D ( 'NONE', #31963, #79706, #12581 ) ;
#46804=DIRECTION ( 'NONE',  ( -0.000000000000000000, -0.9396926207859092051, -0.3420201433256662704 ) ) ;
#46805=CARTESIAN_POINT ( 'NONE',  ( 13.38461538461538680, -9.905515769479276145, 34.41647553114623292 ) ) ;
#46806=CARTESIAN_POINT ( 'NONE',  ( -9.757578138268467427, -11.48612834413959582, 32.76840700105983473 ) ) ;
#46807=CARTESIAN_POINT ( 'NONE',  ( 13.38461538461538680, -2.486705287966279876, 31.30864560766543647 ) ) ;
#46808=CARTESIAN_POINT ( 'NONE',  ( 7.145856592054990131, -3.563462043263029955, 33.22394488606062879 ) ) ;
#46809=CARTESIAN_POINT ( 'NONE',  ( -13.38461538461538325, -9.780366693483667717, 34.19971097300155094 ) ) ;
#46810=CARTESIAN_POINT ( 'NONE',  ( 2.531118706607095703, -7.630147987733843173, 34.99859428049665411 ) ) ;
#46811=CARTESIAN_POINT ( 'NONE',  ( 7.846153846153846700, -2.249999999999998668, 29.75000000000001776 ) ) ;
#46812=ORIENTED_EDGE ( 'NONE', *, *, #75606, .T. ) ;
#46813=DIRECTION ( 'NONE',  ( 0.000000000000000000, 0.000000000000000000, 1.000000000000000000 ) ) ;
#46814=CARTESIAN_POINT ( 'NONE',  ( -3.480792468062194889, -3.711651800289232916, 33.01384336483936011 ) ) ;
#46816=CYLINDRICAL_SURFACE ( 'NONE', #53297, 0.2499999999999998890 ) ;
#46817=CYLINDRICAL_SURFACE ( 'NONE', #85271, 0.2499999999999986955 ) ;
#46818=CARTESIAN_POINT ( 'NONE',  ( 7.846153846153846700, -1.466349020453238561, 30.81389545987213907 ) ) ;
#46819=CARTESIAN_POINT ( 'NONE',  ( 0.2115384615384616196, -2.249999999999998668, 29.75000000000000355 ) ) ;
#46820=ORIENTED_EDGE ( 'NONE', *, *, #8742, .F. ) ;
#46822=CARTESIAN_POINT ( 'NONE',  ( 3.480823650682684178, -8.346898887586323923, 34.93166121998716278 ) ) ;
#46824=CARTESIAN_POINT ( 'NONE',  ( 8.519254038288414321, -8.303909089506435137, 34.68538101551103381 ) ) ;
#46825=CARTESIAN_POINT ( 'NONE',  ( -17.93393164899755732, -3.513871655860376642, 32.76840700105978499 ) ) ;
#46827=CARTESIAN_POINT ( 'NONE',  ( 3.164686851409094892, -4.661471528628506888, 34.16647553114621871 ) ) ;
#46828=CARTESIAN_POINT ( 'NONE',  ( -15.23076923076935252, -3.083524468854526912, 32.58852847137268327 ) ) ;
#46830=DIRECTION ( 'NONE',  ( -0.000000000000000000, -0.3420201433256694901, -0.9396926207859082059 ) ) ;
#46831=ORIENTED_EDGE ( 'NONE', *, *, #40853, .F. ) ;
#46832=VERTEX_POINT ( 'NONE', #67520 ) ;
#46834=ORIENTED_EDGE ( 'NONE', *, *, #69, .F. ) ;
#46836=DIRECTION ( 'NONE',  ( 1.000000000000000000, 0.000000000000000000, 0.000000000000000000 ) ) ;
#46837=CARTESIAN_POINT ( 'NONE',  ( -7.846153846153844924, -11.11383981884818262, 36.00935417666054406 ) ) ;
#46838=CARTESIAN_POINT ( 'NONE',  ( -15.29685161012936589, -2.292212530054419606, 30.41441678777542634 ) ) ;
#46839=B_SPLINE_CURVE_WITH_KNOTS ( 'NONE', 3,
 ( #72106, #16716, #44172, #17160, #29805, #17623, #71657, #9961, #85629, #57266 ),
 .UNSPECIFIED., .F., .F.,
 ( 4, 2, 2, 2, 4 ),
 ( 0.000000000000000000, 0.0001954339857564097783, 0.0003908679715128195566, 0.0005863019572692293891, 0.0007817359430256391132 ),
 .UNSPECIFIED. ) ;
#46840=CYLINDRICAL_SURFACE ( 'NONE', #63453, 0.2499999999999998890 ) ;
#46841=CARTESIAN_POINT ( 'NONE',  ( -3.230769230769352962, -5.094484230521993062, 34.41647553114689373 ) ) ;
#46842=CARTESIAN_POINT ( 'NONE',  ( 11.40777007179398339, -11.71456829005830080, 32.44064028649416542 ) ) ;
#46843=CARTESIAN_POINT ( 'NONE',  ( -12.71151519248081740, -6.567427716900048118, 34.66269422305636283 ) ) ;
#46844=B_SPLINE_CURVE_WITH_KNOTS ( 'NONE', 3,
 ( #23320, #50778, #16567, #44031, #71504, #9811, #64742, #73296, #32748, #31872 ),
 .UNSPECIFIED., .F., .F.,
 ( 4, 2, 2, 2, 4 ),
 ( 0.0007817246256747461966, 0.0009771112852218892010, 0.001172497944769032314, 0.001367884604316175427, 0.001563271263863318323 ),
 .UNSPECIFIED. ) ;
#46845=EDGE_LOOP ( 'NONE', ( #32815, #36603 ) ) ;
#46846=EDGE_LOOP ( 'NONE', ( #66795, #3109 ) ) ;
#46847=EDGE_CURVE ( 'NONE', #57639, #35434, #61410, .T. ) ;
#46848=ORIENTED_EDGE ( 'NONE', *, *, #8916, .T. ) ;
#46849=CARTESIAN_POINT ( 'NONE',  ( 18.22301284409339672, -9.172514111537580561, 34.72667873470787470 ) ) ;
#46850=VERTEX_POINT ( 'NONE', #69289 ) ;
#46851=LINE ( 'NONE', #41431, #39207 ) ;
#46852=CARTESIAN_POINT ( 'NONE',  ( 9.469381474791545017, -4.887634598454295265, 34.01352882383564946 ) ) ;
#46853=ORIENTED_EDGE ( 'NONE', *, *, #60668, .T. ) ;
#46855=VECTOR ( 'NONE', #52113, 1000.000000000000227 ) ;
#46856=VERTEX_POINT ( 'NONE', #36389 ) ;
#46857=FACE_OUTER_BOUND ( 'NONE', #6423, .T. ) ;
#46858=ORIENTED_EDGE ( 'NONE', *, *, #37745, .T. ) ;
#46859=CARTESIAN_POINT ( 'NONE',  ( 9.757563263583717728, -8.613356846314928816, 34.62446782046653482 ) ) ;
#46860=EDGE_CURVE ( 'NONE', #67070, #314, #29202, .T. ) ;
#46861=EDGE_CURVE ( 'NONE', #67515, #48597, #4460, .T. ) ;
#46862=CARTESIAN_POINT ( 'NONE',  ( 1.607394925883795400, -6.760870238392817200, 34.69528174975672385 ) ) ;
#46863=CARTESIAN_POINT ( 'NONE',  ( -4.403822897894745125, -6.524016743844655686, 34.90889640711025521 ) ) ;
#46864=FACE_BOUND ( 'NONE', #5033, .T. ) ;
#46865=FACE_OUTER_BOUND ( 'NONE', #25427, .T. ) ;
#46866=CARTESIAN_POINT ( 'NONE',  ( 16.08857615328984281, -3.643525952247789856, 33.31231777344662959 ) ) ;
#46867=CARTESIAN_POINT ( 'NONE',  ( -1.634592128663975075, -2.318417181685854533, 30.59732222474233865 ) ) ;
#46868=EDGE_CURVE ( 'NONE', #78733, #66835, #19462, .T. ) ;
#46869=CARTESIAN_POINT ( 'NONE',  ( 10.36536139116316058, -10.18141759479407327, 34.26406193332782379 ) ) ;
#46870=CARTESIAN_POINT ( 'NONE',  ( 10.68053039471658394, -7.750023238201979581, 34.74374492549440419 ) ) ;
#46871=CARTESIAN_POINT ( 'NONE',  ( 10.54930223602447903, -10.67929555188718460, 33.92786785259543336 ) ) ;
#46873=EDGE_LOOP ( 'NONE', ( #23140, #9769 ) ) ;
#46875=CARTESIAN_POINT ( 'NONE',  ( 2.057669070399343880, -10.76384336483936011, 33.53834819971076087 ) ) ;
#46876=CARTESIAN_POINT ( 'NONE',  ( 2.373760658694746173, -10.51840700105979565, 33.73612834413962247 ) ) ;
#46877=DIRECTION ( 'NONE',  ( -0.000000000000000000, -0.000000000000000000, -1.000000000000000000 ) ) ;
#46878=CARTESIAN_POINT ( 'NONE',  ( -14.30769230769242917, -12.16647553114689728, 32.15551576947799362 ) ) ;
#46879=CARTESIAN_POINT ( 'NONE',  ( 17.01165263096229907, -8.613356846314824011, 34.62446782046655613 ) ) ;
#46880=CARTESIAN_POINT ( 'NONE',  ( 1.515140822849031732, -4.299079248970732792, 33.91157788607253565 ) ) ;
#46883=DIRECTION ( 'NONE',  ( -0.000000000000000000, -0.7660444431189791237, -0.6427876096865379196 ) ) ;
#46884=CARTESIAN_POINT ( 'NONE',  ( 0.4615384615383396616, -10.21337939537710326, 33.94971097300076224 ) ) ;
#46885=CARTESIAN_POINT ( 'NONE',  ( 17.01084069756293715, -3.937682226553330445, 33.60647404775217240 ) ) ;
#46887=ORIENTED_EDGE ( 'NONE', *, *, #1439, .T. ) ;
#46888=ORIENTED_EDGE ( 'NONE', *, *, #40624, .T. ) ;
#46890=EDGE_LOOP ( 'NONE', ( #79331, #74385 ) ) ;
#46891=CARTESIAN_POINT ( 'NONE',  ( 10.55011461482829738, -4.320704448112771878, 33.92786785259540494 ) ) ;
#46893=CARTESIAN_POINT ( 'NONE',  ( -15.90390063549801347, -5.057305518903949526, 34.11320923018887896 ) ) ;
#46894=CARTESIAN_POINT ( 'NONE',  ( -6.222926958906846551, -9.172386477786396597, 34.72672124145550043 ) ) ;
#46895=CARTESIAN_POINT ( 'NONE',  ( -6.249999999999997335, -7.500000000000001776, 34.75000000000000000 ) ) ;
#46897=CARTESIAN_POINT ( 'NONE',  ( -0.7115616988314271696, -11.37209801155882971, 32.91403422569032955 ) ) ;
#46898=ORIENTED_EDGE ( 'NONE', *, *, #85376, .T. ) ;
#46899=CARTESIAN_POINT ( 'NONE',  ( -0.2114840416250080568, -12.01375889529407637, 32.43194544308182969 ) ) ;
#46901=CARTESIAN_POINT ( 'NONE',  ( -5.300408001487407539, -2.353723527008295680, 30.78948104536958752 ) ) ;
#46902=CARTESIAN_POINT ( 'NONE',  ( -2.980823821391188844, -2.589246495874657938, 31.60778113518102828 ) ) ;
#46903=CARTESIAN_POINT ( 'NONE',  ( -11.78848476268299628, -10.92453946501458795, 33.72985991061850086 ) ) ;
#46904=CARTESIAN_POINT ( 'NONE',  ( 8.769230769230768274, -11.91647553114624181, 32.58852847137148245 ) ) ;
#46905=CARTESIAN_POINT ( 'NONE',  ( 13.31853300525525086, -3.937682226553330445, 33.60647404775217240 ) ) ;
#46906=LINE ( 'NONE', #74392, #50680 ) ;
#46907=CARTESIAN_POINT ( 'NONE',  ( -0.5268084620947811603, -2.657715359629089225, 31.77849191805834295 ) ) ;
#46909=ORIENTED_EDGE ( 'NONE', *, *, #12352, .T. ) ;
#46910=DIRECTION ( 'NONE',  ( -0.000000000000000000, 0.9396926207859092051, -0.3420201433256662704 ) ) ;
#46911=CARTESIAN_POINT ( 'NONE',  ( -9.469528151039281028, -8.496831190052096971, 34.64984203495476578 ) ) ;
#46912=ORIENTED_EDGE ( 'NONE', *, *, #70339, .T. ) ;
#46913=ORIENTED_EDGE ( 'NONE', *, *, #51303, .T. ) ;
#46914=CARTESIAN_POINT ( 'NONE',  ( -12.46153846153846168, -11.35647404775217417, 33.31231777344666511 ) ) ;
#46915=CARTESIAN_POINT ( 'NONE',  ( 3.007903808565593362, -2.501496062324912284, 29.88072118266895671 ) ) ;
#46916=EDGE_CURVE ( 'NONE', #79454, #78447, #21085, .T. ) ;
#46917=VECTOR ( 'NONE', #42186, 1000.000000000000114 ) ;
#46918=CARTESIAN_POINT ( 'NONE',  ( -6.923076923077044142, -6.026961402154118908, 34.52809138561165270 ) ) ;
#46919=CARTESIAN_POINT ( 'NONE',  ( -5.011729095139719092, -2.506253911140448487, 29.99999999999988631 ) ) ;
#46920=CARTESIAN_POINT ( 'NONE',  ( -2.307692307692305711, -3.050289026998446396, 32.03036669348365706 ) ) ;
#46921=ORIENTED_EDGE ( 'NONE', *, *, #32870, .T. ) ;
#46922=CARTESIAN_POINT ( 'NONE',  ( 5.776515056276052995, -3.754499324213721234, 33.06261337010820256 ) ) ;
#46923=B_SPLINE_CURVE_WITH_KNOTS ( 'NONE', 3,
 ( #29765, #69419, #68970, #41505, #50024, #8164, #48691, #42838, #1398, #83834 ),
 .UNSPECIFIED., .F., .F.,
 ( 4, 2, 2, 2, 4 ),
 ( 0.0007817359430256338006, 0.0009771253907250062980, 0.001172514838424371531, 0.001367904286123736981, 0.001563293733823102431 ),
 .UNSPECIFIED. ) ;
#46925=CARTESIAN_POINT ( 'NONE',  ( -2.176901866725356793, -5.496552790871119143, 34.60292014791297532 ) ) ;
#46926=ORIENTED_EDGE ( 'NONE', *, *, #81052, .F. ) ;
#46927=DIRECTION ( 'NONE',  ( -0.000000000000000000, 0.6427876096865404731, -0.7660444431189770143 ) ) ;
#46928=EDGE_CURVE ( 'NONE', #82406, #75693, #70020, .T. ) ;
#46929=VERTEX_POINT ( 'NONE', #34615 ) ;
#46930=CARTESIAN_POINT ( 'NONE',  ( 13.45068373561782593, -3.513871655860379306, 32.76840700105978499 ) ) ;
#46931=CARTESIAN_POINT ( 'NONE',  ( -6.000000000000121680, -12.16647553114689728, 32.15551576947799362 ) ) ;
#46932=EDGE_LOOP ( 'NONE', ( #70385, #72035 ) ) ;
#46933=EDGE_CURVE ( 'NONE', #28537, #32578, #74343, .T. ) ;
#46935=CARTESIAN_POINT ( 'NONE',  ( 13.38461538461526423, -9.528491918059723176, 34.59228464037033035 ) ) ;
#46936=CARTESIAN_POINT ( 'NONE',  ( -13.38461538461550759, -3.083524468854526912, 32.58852847137268327 ) ) ;
#46937=CARTESIAN_POINT ( 'NONE',  ( -8.069080805060693251, -4.762599654559228846, 34.23009711892697737 ) ) ;
#46938=CARTESIAN_POINT ( 'NONE',  ( -2.307692307692305711, -10.67929555188718282, 33.92786785259544047 ) ) ;
#46940=EDGE_CURVE ( 'NONE', #72513, #73958, #51454, .T. ) ;
#46941=DIRECTION ( 'NONE',  ( -0.000000000000000000, -0.7660444431189791237, -0.6427876096865379196 ) ) ;
#46942=EDGE_LOOP ( 'NONE', ( #26173, #68426 ) ) ;
#46943=DIRECTION ( 'NONE',  ( -0.000000000000000000, 0.3420201433256694901, -0.9396926207859082059 ) ) ;
#46945=EDGE_CURVE ( 'NONE', #47170, #46688, #60290, .T. ) ;
#46946=CARTESIAN_POINT ( 'NONE',  ( 6.130791807824788719, -8.999086150933472084, 34.52020707165672064 ) ) ;
#46947=AXIS2_PLACEMENT_3D ( 'NONE', #32984, #20362, #69426 ) ;
#46948=CARTESIAN_POINT ( 'NONE',  ( 2.980792486720641232, -11.47974371597207899, 33.17467449705390692 ) ) ;
#46949=CARTESIAN_POINT ( 'NONE',  ( 14.30769230769218581, -8.656820664282941280, 34.87096338111179961 ) ) ;
#46950=ORIENTED_EDGE ( 'NONE', *, *, #53054, .F. ) ;
#46951=B_SPLINE_CURVE_WITH_KNOTS ( 'NONE', 3,
 ( #79873, #52833, #46088, #11410, #10971, #38897, #17278, #11869, #66355, #39346 ),
 .UNSPECIFIED., .F., .F.,
 ( 4, 2, 2, 2, 4 ),
 ( 0.000000000000000000, 0.0001954339857564073659, 0.0003908679715128147319, 0.0005863019572692221250, 0.0007817359430256294638 ),
 .UNSPECIFIED. ) ;
#46952=EDGE_LOOP ( 'NONE', ( #59613, #13125 ) ) ;
#46954=EDGE_LOOP ( 'NONE', ( #36749, #76190 ) ) ;
#46955=EDGE_CURVE ( 'NONE', #37924, #67105, #77528, .T. ) ;
#46956=CARTESIAN_POINT ( 'NONE',  ( 2.177545098254087819, -5.195881422630167279, 34.18770438780618548 ) ) ;
#46957=CARTESIAN_POINT ( 'NONE',  ( 4.153846153846030731, -10.33852847137269571, 34.16647553114546554 ) ) ;
#46959=CARTESIAN_POINT ( 'NONE',  ( -2.057692307692370104, -7.565270445406050648, 34.75000000000000000 ) ) ;
#46960=CARTESIAN_POINT ( 'NONE',  ( 6.130525701763567703, -12.27024696741798770, 31.24895572276497546 ) ) ;
#46961=CARTESIAN_POINT ( 'NONE',  ( 17.86985279056177944, -10.19110544564092002, 33.96427741523702792 ) ) ;
#46963=VECTOR ( 'NONE', #16574, 1000.000000000000227 ) ;
#46964=CARTESIAN_POINT ( 'NONE',  ( -5.326899807865431491, -8.303909089506435137, 34.68538101551103381 ) ) ;
#46966=CARTESIAN_POINT ( 'NONE',  ( -2.084912766423895558, -3.755027918224367767, 33.06320215134714857 ) ) ;
#46967=CARTESIAN_POINT ( 'NONE',  ( -8.638705330997126453, -3.068774925481847493, 32.56582465632704526 ) ) ;
#46971=ORIENTED_EDGE ( 'NONE', *, *, #83157, .T. ) ;
#46972=CARTESIAN_POINT ( 'NONE',  ( -13.44988538517170440, -12.51329471203370325, 31.30864560766548976 ) ) ;
#46973=EDGE_LOOP ( 'NONE', ( #87293, #62061, #44248, #54539 ) ) ;
#46974=CARTESIAN_POINT ( 'NONE',  ( -3.230769230769352962, -10.33852847137269571, 34.16647553114546554 ) ) ;
#46975=CARTESIAN_POINT ( 'NONE',  ( -9.758390071667825794, -3.937682226553330445, 33.60647404775217240 ) ) ;
#46977=FACE_OUTER_BOUND ( 'NONE', #83660, .T. ) ;
#46978=FACE_BOUND ( 'NONE', #42125, .T. ) ;
#46979=ORIENTED_EDGE ( 'NONE', *, *, #57670, .T. ) ;
#46981=ORIENTED_EDGE ( 'NONE', *, *, #44723, .T. ) ;
#46982=CARTESIAN_POINT ( 'NONE',  ( -8.545854828532586822, -2.501478030877323455, 29.88021232661721172 ) ) ;
#46983=ORIENTED_EDGE ( 'NONE', *, *, #5301, .T. ) ;
#46984=FACE_BOUND ( 'NONE', #6973, .T. ) ;
#46986=B_SPLINE_CURVE_WITH_KNOTS ( 'NONE', 3,
 ( #69585, #48418, #14648, #15537, #7000, #62810, #42131, #88998, #22288, #246 ),
 .UNSPECIFIED., .F., .F.,
 ( 4, 2, 2, 2, 4 ),
 ( 0.000000000000000000, 0.0001954311564186875792, 0.0003908623128373751583, 0.0005862934692560627103, 0.0007817246256747503166 ),
 .UNSPECIFIED. ) ;
#46987=CARTESIAN_POINT ( 'NONE',  ( 17.99999999999987566, -5.219633306517616589, 34.19971097300220464 ) ) ;
#46989=CARTESIAN_POINT ( 'NONE',  ( 3.230769230769231726, -1.422936976036506707, 30.56769352161908415 ) ) ;
#46990=CARTESIAN_POINT ( 'NONE',  ( 12.46153846153846168, -11.11383981884818262, 36.00935417666054406 ) ) ;
#46991=CARTESIAN_POINT ( 'NONE',  ( 3.230769230769231726, -11.91647553114624181, 32.58852847137148245 ) ) ;
#46992=ORIENTED_EDGE ( 'NONE', *, *, #70292, .T. ) ;
#46993=CARTESIAN_POINT ( 'NONE',  ( 6.699591979352975457, -10.11188796281391511, 34.01382737946119050 ) ) ;
#46994=CARTESIAN_POINT ( 'NONE',  ( 14.08476534878546360, -11.43668979543634734, 33.22377378376089752 ) ) ;
#46995=CARTESIAN_POINT ( 'NONE',  ( 12.46153846153833911, -6.879047030192662504, 34.71129190930017927 ) ) ;
#46996=CARTESIAN_POINT ( 'NONE',  ( 5.076923076923075762, -6.386643153685126251, 34.62446782046654192 ) ) ;
#46998=CARTESIAN_POINT ( 'NONE',  ( 2.307692307692309264, -12.34228464037088635, 31.77849191805839268 ) ) ;
#46999=CARTESIAN_POINT ( 'NONE',  ( -16.15384615384627409, -10.33852847137269571, 34.16647553114546554 ) ) ;
#47000=ORIENTED_EDGE ( 'NONE', *, *, #45127, .F. ) ;
#47001=CARTESIAN_POINT ( 'NONE',  ( 17.99999999999987566, -6.879047030192662504, 34.71129190930017927 ) ) ;
#47002=CARTESIAN_POINT ( 'NONE',  ( 9.942307692307759126, -7.434744860731433924, 35.00000000000000711 ) ) ;
#47003=DIRECTION ( 'NONE',  ( -0.000000000000000000, -0.000000000000000000, -1.000000000000000000 ) ) ;
#47004=CARTESIAN_POINT ( 'NONE',  ( 16.15384615384615330, -11.91647553114624181, 32.58852847137148245 ) ) ;
#47005=CARTESIAN_POINT ( 'NONE',  ( 0.4615384615384611200, -2.486705287966279876, 31.30864560766543647 ) ) ;
#47006=ADVANCED_FACE ( 'NONE', ( #50325 ), #64280, .F. ) ;
#47007=VECTOR ( 'NONE', #37404, 999.9999999999998863 ) ;
#47008=DIRECTION ( 'NONE',  ( 0.000000000000000000, 0.9848077530122072432, -0.1736481776669354937 ) ) ;
#47009=CARTESIAN_POINT ( 'NONE',  ( 0.5923289025054125911, -11.37503395064541678, 33.29242100308974983 ) ) ;
#47011=CARTESIAN_POINT ( 'NONE',  ( -6.792551221313360088, -2.882268652242224505, 31.66798894389554064 ) ) ;
#47013=ORIENTED_EDGE ( 'NONE', *, *, #84625, .T. ) ;
#47015=CARTESIAN_POINT ( 'NONE',  ( 17.75002326905764960, -4.236021600441997492, 33.53823185664189310 ) ) ;
#47016=ORIENTED_EDGE ( 'NONE', *, *, #34524, .T. ) ;
#47017=EDGE_CURVE ( 'NONE', #43624, #46336, #57104, .T. ) ;
#47018=EDGE_LOOP ( 'NONE', ( #34652, #8111, #21469, #65819 ) ) ;
#47019=CARTESIAN_POINT ( 'NONE',  ( -3.230769230769229949, -13.57706302396349152, 30.56769352161908060 ) ) ;
#47020=VECTOR ( 'NONE', #3946, 1000.000000000000227 ) ;
#47021=VERTEX_POINT ( 'NONE', #78247 ) ;
#47022=CARTESIAN_POINT ( 'NONE',  ( 1.607628228708781304, -11.98016756924215009, 32.48728574198911190 ) ) ;
#47024=CARTESIAN_POINT ( 'NONE',  ( 13.60739492588379917, -2.847695495035523550, 31.58253572463339154 ) ) ;
#47025=CARTESIAN_POINT ( 'NONE',  ( -18.00000000000012079, -12.16647553114689906, 32.15551576947799362 ) ) ;
#47027=EDGE_CURVE ( 'NONE', #59987, #74290, #73222, .T. ) ;
#47028=CARTESIAN_POINT ( 'NONE',  ( -5.076923076923075762, -3.322132147404559976, 32.92929555188717927 ) ) ;
#47029=CARTESIAN_POINT ( 'NONE',  ( -15.48079245499068612, -4.931416488878822335, 34.32920672191015399 ) ) ;
#47030=CYLINDRICAL_SURFACE ( 'NONE', #78483, 0.2500000000000002220 ) ;
#47032=FACE_OUTER_BOUND ( 'NONE', #67622, .T. ) ;
#47033=CARTESIAN_POINT ( 'NONE',  ( -14.43825289943422696, -2.504760397472875155, 29.97295953869789997 ) ) ;
#47034=LINE ( 'NONE', #39421, #65105 ) ;
#47036=EDGE_LOOP ( 'NONE', ( #2201, #35195, #71358, #12272 ) ) ;
#47037=ORIENTED_EDGE ( 'NONE', *, *, #64573, .F. ) ;
#47038=CIRCLE ( 'NONE', #85872, 0.2500000000000002220 ) ;
#47039=CARTESIAN_POINT ( 'NONE',  ( 6.857806477116147548, -2.625532179533445198, 30.86335684631481513 ) ) ;
#47040=CARTESIAN_POINT ( 'NONE',  ( 5.076923076923075762, -8.973038597847269315, 34.52809138561121927 ) ) ;
#47042=CARTESIAN_POINT ( 'NONE',  ( -6.923076923076922462, -5.471508081941601098, 34.59228464037088457 ) ) ;
#47043=EDGE_CURVE ( 'NONE', #67813, #36002, #166, .T. ) ;
#47045=CARTESIAN_POINT ( 'NONE',  ( -16.21992956480203318, -8.973038597847269315, 34.52809138561120506 ) ) ;
#47046=CARTESIAN_POINT ( 'NONE',  ( 17.07692307692295586, -3.643525952248796163, 33.31231777344771672 ) ) ;
#47047=AXIS2_PLACEMENT_3D ( 'NONE', #29110, #7501, #48466 ) ;
#47048=ORIENTED_EDGE ( 'NONE', *, *, #50110, .T. ) ;
#47049=CARTESIAN_POINT ( 'NONE',  ( -6.792285115252133743, -9.804649428959608670, 34.18742332936588468 ) ) ;
#47050=EDGE_LOOP ( 'NONE', ( #27258, #86645 ) ) ;
#47051=B_SPLINE_CURVE_WITH_KNOTS ( 'NONE', 3,
 ( #33047, #82128, #41575, #47434, #55527, #47884 ),
 .UNSPECIFIED., .F., .F.,
 ( 4, 2, 4 ),
 ( 4.220987180333913380E-17, 0.0001954756301637125201, 0.0003909512603273828648 ),
 .UNSPECIFIED. ) ;
#47052=ORIENTED_EDGE ( 'NONE', *, *, #61418, .T. ) ;
#47053=CARTESIAN_POINT ( 'NONE',  ( 16.37662582282421653, -9.418065098278011860, 34.63729479722530158 ) ) ;
#47054=CARTESIAN_POINT ( 'NONE',  ( -14.30769230769230660, -6.343179335718451384, 34.87096338111211935 ) ) ;
#47055=CARTESIAN_POINT ( 'NONE',  ( -7.053686578281003428, -7.722926974430166069, 34.99546784045485737 ) ) ;
#47056=CARTESIAN_POINT ( 'NONE',  ( 6.065255139512838234, -8.656820664281605460, 34.87096338111211224 ) ) ;
#47058=VERTEX_POINT ( 'NONE', #5705 ) ;
#47059=EDGE_LOOP ( 'NONE', ( #32098, #82511, #86896, #57892 ) ) ;
#47062=ORIENTED_EDGE ( 'NONE', *, *, #33358, .F. ) ;
#47063=EDGE_CURVE ( 'NONE', #33682, #29234, #80741, .T. ) ;
#47064=CARTESIAN_POINT ( 'NONE',  ( 5.869852790561782108, -2.619462340734462380, 30.83744416345203021 ) ) ;
#47065=CARTESIAN_POINT ( 'NONE',  ( 0.4615384615384611200, -7.500000000000001776, 35.04278698407183867 ) ) ;
#47066=VECTOR ( 'NONE', #75865, 999.9999999999998863 ) ;
#47067=CARTESIAN_POINT ( 'NONE',  ( 16.21991348719623360, -5.471508081941601098, 34.59228464037088457 ) ) ;
#47068=EDGE_CURVE ( 'NONE', #70411, #2304, #52796, .T. ) ;
#47069=CARTESIAN_POINT ( 'NONE',  ( -15.36091644020745051, -11.47017969459904130, 32.78971311882034456 ) ) ;
#47070=CARTESIAN_POINT ( 'NONE',  ( 17.99999999999987566, -5.219633306517616589, 34.19971097300220464 ) ) ;
#47071=EDGE_CURVE ( 'NONE', #44439, #74721, #7660, .T. ) ;
#47072=CARTESIAN_POINT ( 'NONE',  ( 14.08420736396836226, -12.44517049084099725, 30.48991314939691932 ) ) ;
#47073=AXIS2_PLACEMENT_3D ( 'NONE', #22664, #64084, #6165 ) ;
#47075=VERTEX_POINT ( 'NONE', #39063 ) ;
#47076=ORIENTED_EDGE ( 'NONE', *, *, #42470, .F. ) ;
#47077=FACE_OUTER_BOUND ( 'NONE', #30085, .T. ) ;
#47078=ORIENTED_EDGE ( 'NONE', *, *, #66693, .T. ) ;
#47079=DIRECTION ( 'NONE',  ( -0.000000000000000000, 0.5000000000000011102, -0.8660254037844381525 ) ) ;
#47080=CARTESIAN_POINT ( 'NONE',  ( 6.792600214960459404, -7.276988635370452485, 34.74523720219453793 ) ) ;
#47081=B_SPLINE_CURVE_WITH_KNOTS ( 'NONE', 3,
 ( #43233, #70710, #61719, #36, #54979, #20744, #62608, #62173, #27951, #918 ),
 .UNSPECIFIED., .F., .F.,
 ( 4, 2, 2, 2, 4 ),
 ( 0.0007817359430256262112, 0.0009771253907249911191, 0.001172514838424356136, 0.001367904286123721152, 0.001563293733823086168 ),
 .UNSPECIFIED. ) ;
#47083=ORIENTED_EDGE ( 'NONE', *, *, #78507, .T. ) ;
#47084=EDGE_CURVE ( 'NONE', #13666, #80199, #88153, .T. ) ;
#47085=CARTESIAN_POINT ( 'NONE',  ( 8.096099255531889582, -4.176053281294515251, 33.81426240980091791 ) ) ;
#47086=EDGE_LOOP ( 'NONE', ( #50662, #34320 ) ) ;
#47087=CARTESIAN_POINT ( 'NONE',  ( -16.15384615384615330, -9.780366693483667717, 34.19971097300155094 ) ) ;
#47088=FACE_BOUND ( 'NONE', #13213, .T. ) ;
#47090=CARTESIAN_POINT ( 'NONE',  ( -17.07692307692307665, -11.11383981884818262, 36.00935417666054406 ) ) ;
#47092=EDGE_CURVE ( 'NONE', #34883, #32683, #16950, .T. ) ;
#47093=DIRECTION ( 'NONE',  ( 0.000000000000000000, 0.4999999999999960032, -0.8660254037844410391 ) ) ;
#47094=DIRECTION ( 'NONE',  ( -0.000000000000000000, -0.8660254037844397068, -0.4999999999999978906 ) ) ;
#47095=CARTESIAN_POINT ( 'NONE',  ( -13.38461538461538325, -1.242168528481310874, 33.36296068462461051 ) ) ;
#47096=VERTEX_POINT ( 'NONE', #6152 ) ;
#47097=DIRECTION ( 'NONE',  ( -0.000000000000000000, 0.9396926207859093161, -0.3420201433256663259 ) ) ;
#47098=CARTESIAN_POINT ( 'NONE',  ( 1.607626736228236375, -8.239487800360276282, 34.69522927552633718 ) ) ;
#47100=CARTESIAN_POINT ( 'NONE',  ( -2.176901866725356349, -9.084667340241226796, 34.75534355489798344 ) ) ;
#47101=LINE ( 'NONE', #39930, #37173 ) ;
#47102=EDGE_CURVE ( 'NONE', #40306, #73925, #33625, .T. ) ;
#47103=FACE_BOUND ( 'NONE', #79800, .T. ) ;
#47104=CARTESIAN_POINT ( 'NONE',  ( 10.61538461538461675, -3.322132147404559976, 32.92929555188717927 ) ) ;
#47105=DIRECTION ( 'NONE',  ( 0.000000000000000000, 0.3420201433256610524, 0.9396926207859113145 ) ) ;
#47106=CIRCLE ( 'NONE', #87395, 0.2500000000000002220 ) ;
#47107=DIRECTION ( 'NONE',  ( 1.000000000000000000, 0.000000000000000000, 0.000000000000000000 ) ) ;
#47109=CYLINDRICAL_SURFACE ( 'NONE', #36307, 0.2500000000000008882 ) ;
#47110=CARTESIAN_POINT ( 'NONE',  ( -8.703162418228330921, -3.513871655860379306, 32.76840700105978499 ) ) ;
#47112=VERTEX_POINT ( 'NONE', #39507 ) ;
#47113=EDGE_CURVE ( 'NONE', #54572, #82999, #85031, .T. ) ;
#47114=CARTESIAN_POINT ( 'NONE',  ( -8.769230769230768274, -5.557115091759785130, 34.35708131394839171 ) ) ;
#47115=ORIENTED_EDGE ( 'NONE', *, *, #26185, .F. ) ;
#47116=CARTESIAN_POINT ( 'NONE',  ( -18.22348492456433178, -3.562934362175797176, 33.22335522853831691 ) ) ;
#47117=ORIENTED_EDGE ( 'NONE', *, *, #15723, .T. ) ;
#47118=CARTESIAN_POINT ( 'NONE',  ( 16.28437159207980045, -12.70449254468099198, 30.44128974285582956 ) ) ;
#47119=CARTESIAN_POINT ( 'NONE',  ( -13.60748164767848323, -2.251424796025575770, 29.88072029997477230 ) ) ;
#47120=CARTESIAN_POINT ( 'NONE',  ( -5.076923076923199218, -9.528491918059723176, 34.59228464037033035 ) ) ;
#47121=VERTEX_POINT ( 'NONE', #10079 ) ;
#47122=CARTESIAN_POINT ( 'NONE',  ( 17.01084069756293715, -12.62096338111211580, 30.90682066428152908 ) ) ;
#47123=CARTESIAN_POINT ( 'NONE',  ( 18.25000000000141753, -7.500000000000154543, 35.00000000000007105 ) ) ;
#47125=FACE_OUTER_BOUND ( 'NONE', #33988, .T. ) ;
#47126=FACE_OUTER_BOUND ( 'NONE', #45519, .T. ) ;
#47128=B_SPLINE_CURVE_WITH_KNOTS ( 'NONE', 3,
 ( #23898, #78851, #44610, #10851, #10408, #58573, #65337, #31102, #72541, #38321 ),
 .UNSPECIFIED., .F., .F.,
 ( 4, 2, 2, 2, 4 ),
 ( 0.000000000000000000, 0.0001954311564186864678, 0.0003908623128373729357, 0.0005862934692560594577, 0.0007817246256747458714 ),
 .UNSPECIFIED. ) ;
#47129=CARTESIAN_POINT ( 'NONE',  ( -12.39547112818838492, -9.058645607665452459, 34.76329471203371924 ) ) ;
#47130=DIRECTION ( 'NONE',  ( -0.000000000000000000, -0.9396926207859093161, -0.3420201433256663259 ) ) ;
#47131=CARTESIAN_POINT ( 'NONE',  ( 2.438484115517092654, -2.729792928343269587, 31.24908615093345077 ) ) ;
#47132=CARTESIAN_POINT ( 'NONE',  ( -11.31568199719312773, -10.11255958852956027, 34.01340905677048454 ) ) ;
#47134=AXIS2_PLACEMENT_3D ( 'NONE', #74481, #34372, #11901 ) ;
#47135=CARTESIAN_POINT ( 'NONE',  ( 5.076923076922953193, -2.657715359629662988, 31.77849191805970364 ) ) ;
#47136=ADVANCED_FACE ( 'NONE', ( #85748 ), #10530, .F. ) ;
#47137=CARTESIAN_POINT ( 'NONE',  ( -8.899378738962470337, -3.069018819979302926, 32.56621877034667278 ) ) ;
#47138=VERTEX_POINT ( 'NONE', #30353 ) ;
#47139=CYLINDRICAL_SURFACE ( 'NONE', #18261, 0.2499999999999973355 ) ;
#47140=DIRECTION ( 'NONE',  ( 0.000000000000000000, 0.8660254037844377084, 0.5000000000000015543 ) ) ;
#47142=FACE_OUTER_BOUND ( 'NONE', #50926, .T. ) ;
#47143=CARTESIAN_POINT ( 'NONE',  ( -16.28399412357785536, -11.04286588640298561, 33.62463336215343901 ) ) ;
#47144=ORIENTED_EDGE ( 'NONE', *, *, #31098, .F. ) ;
#47145=DIRECTION ( 'NONE',  ( -0.000000000000000000, 0.1736481776669307198, -0.9848077530122080203 ) ) ;
#47146=CARTESIAN_POINT ( 'NONE',  ( 2.980745993476266786, -3.711651800289232916, 33.01384336483936011 ) ) ;
#47147=CARTESIAN_POINT ( 'NONE',  ( 5.076923076923075762, -9.819645486525091727, 36.12317359536749706 ) ) ;
#47148=VERTEX_POINT ( 'NONE', #51480 ) ;
#47149=CARTESIAN_POINT ( 'NONE',  ( 12.52760681254089725, -12.37446782046654192, 30.86335684631486842 ) ) ;
#47150=CIRCLE ( 'NONE', #67282, 0.2500000000000002220 ) ;
#47151=EDGE_CURVE ( 'NONE', #86521, #86086, #76408, .T. ) ;
#47152=CARTESIAN_POINT ( 'NONE',  ( -15.10024379253559168, -12.15418822224088835, 32.17964115625579069 ) ) ;
#47153=CARTESIAN_POINT ( 'NONE',  ( 14.30769230769262279, -2.255955759149395501, 30.00000000000324363 ) ) ;
#47154=EDGE_CURVE ( 'NONE', #15980, #79283, #48483, .T. ) ;
#47155=ORIENTED_EDGE ( 'NONE', *, *, #70006, .F. ) ;
#47156=CARTESIAN_POINT ( 'NONE',  ( 3.007284306204897728, -2.612411019501189813, 31.66733052389439962 ) ) ;
#47157=CARTESIAN_POINT ( 'NONE',  ( 6.857806477116148436, -5.219633306516282545, 34.19971097300152252 ) ) ;
#47158=CARTESIAN_POINT ( 'NONE',  ( 1.318533005255250412, -2.833524468853757305, 32.15551576947924417 ) ) ;
#47160=EDGE_LOOP ( 'NONE', ( #23616, #77426 ) ) ;
#47162=ORIENTED_EDGE ( 'NONE', *, *, #3762, .T. ) ;
#47164=CARTESIAN_POINT ( 'NONE',  ( 5.076923076923075762, -12.10708131394839349, 31.69288490824020244 ) ) ;
#47165=CARTESIAN_POINT ( 'NONE',  ( -2.084680956079456582, -5.667800583137508674, 34.40243808032445827 ) ) ;
#47166=DIRECTION ( 'NONE',  ( -0.000000000000000000, -0.000000000000000000, -1.000000000000000000 ) ) ;
#47167=CARTESIAN_POINT ( 'NONE',  ( 4.153846153846154188, -9.905515769479276145, 34.41647553114623292 ) ) ;
#47168=AXIS2_PLACEMENT_3D ( 'NONE', #33462, #26699, #118 ) ;
#47169=CARTESIAN_POINT ( 'NONE',  ( -2.307692307692305711, -1.215029322943914858, 32.30358669280327177 ) ) ;
#47170=VERTEX_POINT ( 'NONE', #30789 ) ;
#47171=EDGE_LOOP ( 'NONE', ( #13343, #17122 ) ) ;
#47173=CARTESIAN_POINT ( 'NONE',  ( -3.007393290071045833, -2.501478030877322567, 29.88021232661720816 ) ) ;
#47174=VERTEX_POINT ( 'NONE', #51039 ) ;
#47176=CARTESIAN_POINT ( 'NONE',  ( -10.68070862818892230, -7.749976730030849303, 34.74374725381503737 ) ) ;
#47177=EDGE_CURVE ( 'NONE', #17613, #42225, #78634, .T. ) ;
#47179=CARTESIAN_POINT ( 'NONE',  ( -15.00798968950081758, -9.332535724633409302, 34.40230450496446934 ) ) ;
#47180=ADVANCED_FACE ( 'NONE', ( #44283 ), #71771, .F. ) ;
#47181=EDGE_LOOP ( 'NONE', ( #60258, #28012 ) ) ;
#47182=ORIENTED_EDGE ( 'NONE', *, *, #46169, .T. ) ;
#47184=CARTESIAN_POINT ( 'NONE',  ( -10.83831157429145975, -10.77366814457252175, 33.85459836347579454 ) ) ;
#47185=CARTESIAN_POINT ( 'NONE',  ( 11.53846153846153832, -6.435427911321262684, 35.78748833219616898 ) ) ;
#47186=ORIENTED_EDGE ( 'NONE', *, *, #35542, .F. ) ;
#47187=EDGE_CURVE ( 'NONE', #33472, #58556, #14197, .T. ) ;
#47188=FACE_OUTER_BOUND ( 'NONE', #7448, .T. ) ;
#47189=CARTESIAN_POINT ( 'NONE',  ( -18.00000000000000000, -13.83693561022309915, 32.05645593858272235 ) ) ;
#47190=EDGE_LOOP ( 'NONE', ( #31803, #25120 ) ) ;
#47191=CARTESIAN_POINT ( 'NONE',  ( 16.15384615384603251, -11.67786785259630911, 32.92929555188603530 ) ) ;
#47192=CARTESIAN_POINT ( 'NONE',  ( -3.931066612577743147, -5.114059244376869984, 34.14424750095245287 ) ) ;
#47193=ADVANCED_FACE ( 'NONE', ( #81655 ), #75339, .F. ) ;
#47194=CARTESIAN_POINT ( 'NONE',  ( 0.3313904918067657190, -9.504002272028875709, 34.60269587691767867 ) ) ;
#47196=FACE_BOUND ( 'NONE', #68805, .T. ) ;
#47197=B_SPLINE_CURVE_WITH_KNOTS ( 'NONE', 3,
 ( #69958, #10369, #49250, #78815, #64849, #58098, #8271, #31523, #38281, #86489 ),
 .UNSPECIFIED., .F., .F.,
 ( 4, 2, 2, 2, 4 ),
 ( 0.0007817246256747481482, 0.0009771112852218909357, 0.001172497944769033832, 0.001367884604316176728, 0.001563271263863319407 ),
 .UNSPECIFIED. ) ;
#47198=CARTESIAN_POINT ( 'NONE',  ( 10.68145296638705410, -9.780366693483667717, 34.19971097300155805 ) ) ;
#47199=DIRECTION ( 'NONE',  ( -0.000000000000000000, 1.000000000000000000, -0.000000000000000000 ) ) ;
#47200=CARTESIAN_POINT ( 'NONE',  ( 15.23076923076923173, -3.050289026998446396, 32.03036669348365706 ) ) ;
#47201=CARTESIAN_POINT ( 'NONE',  ( 9.562160482869472844, -3.285722584762969856, 32.44110544564090759 ) ) ;
#47202=DIRECTION ( 'NONE',  ( 0.000000000000000000, -6.938893903907222067E-15, 1.000000000000000000 ) ) ;
#47203=ADVANCED_FACE ( 'NONE', ( #82098 ), #81214, .F. ) ;
#47204=CARTESIAN_POINT ( 'NONE',  ( 0.3962680155776854285, -12.27809138561121394, 31.22303859784730307 ) ) ;
#47205=CARTESIAN_POINT ( 'NONE',  ( 12.68431813051652313, -3.020022701398814569, 32.48759521482552515 ) ) ;
#47206=ORIENTED_EDGE ( 'NONE', *, *, #10684, .F. ) ;
#47207=VECTOR ( 'NONE', #10728, 1000.000000000000227 ) ;
#47208=CARTESIAN_POINT ( 'NONE',  ( -15.23076923076922995, -11.35647404775217417, 33.31231777344666511 ) ) ;
#47210=ORIENTED_EDGE ( 'NONE', *, *, #11258, .F. ) ;
#47211=CARTESIAN_POINT ( 'NONE',  ( -15.23076923076922995, -1.466349020453238561, 30.81389545987213907 ) ) ;
#47212=EDGE_CURVE ( 'NONE', #48528, #26836, #51655, .T. ) ;
#47213=CARTESIAN_POINT ( 'NONE',  ( -15.36091644020745051, -2.619462340734462380, 30.83744416345203021 ) ) ;
#47214=CARTESIAN_POINT ( 'NONE',  ( 9.626224281351811740, -2.721908614388770964, 31.22303859784723912 ) ) ;
#47215=ORIENTED_EDGE ( 'NONE', *, *, #88857, .F. ) ;
#47216=CARTESIAN_POINT ( 'NONE',  ( -9.692307692307814193, -9.528491918059723176, 34.59228464037033035 ) ) ;
#47217=DIRECTION ( 'NONE',  ( -0.000000000000000000, 0.9396926207859092051, -0.3420201433256662704 ) ) ;
#47218=FACE_BOUND ( 'NONE', #20345, .T. ) ;
#47219=CARTESIAN_POINT ( 'NONE',  ( -14.55771553191376633, -4.175268141568685643, 33.81360843649122216 ) ) ;
#47220=CARTESIAN_POINT ( 'NONE',  ( -10.61538461538461320, -13.20930481340135110, 34.54067556320372745 ) ) ;
#47221=CARTESIAN_POINT ( 'NONE',  ( -13.38461538461550759, -5.094484230521993062, 34.41647553114689373 ) ) ;
#47222=CARTESIAN_POINT ( 'NONE',  ( -5.207614543590635137, -8.999036380462719364, 34.52022231692819076 ) ) ;
#47224=CARTESIAN_POINT ( 'NONE',  ( 2.307692307692309264, -10.67929555188718282, 33.92786785259544047 ) ) ;
#47226=ORIENTED_EDGE ( 'NONE', *, *, #26002, .F. ) ;
#47227=EDGE_CURVE ( 'NONE', #8709, #68144, #66852, .T. ) ;
#47230=EDGE_CURVE ( 'NONE', #43122, #37045, #5549, .T. ) ;
#47231=CARTESIAN_POINT ( 'NONE',  ( 16.40390046548447245, -6.567000820036036579, 34.66262288849541306 ) ) ;
#47232=CARTESIAN_POINT ( 'NONE',  ( -2.307692307692305711, -7.500000000000001776, 35.04278698407183867 ) ) ;
#47233=CARTESIAN_POINT ( 'NONE',  ( -0.7115384615384606759, -7.500000000000001776, 34.75000000000000000 ) ) ;
#47234=CARTESIAN_POINT ( 'NONE',  ( 5.299935921016471596, -3.395485233115139057, 33.02377354290275946 ) ) ;
#47236=CARTESIAN_POINT ( 'NONE',  ( -8.834500769787091201, -10.33852847137145048, 34.16647553114627556 ) ) ;
#47237=CARTESIAN_POINT ( 'NONE',  ( 1.384615384615386802, -9.905515769479276145, 34.41647553114623292 ) ) ;
#47238=AXIS2_PLACEMENT_3D ( 'NONE', #53928, #53480, #81862 ) ;
#47239=CARTESIAN_POINT ( 'NONE',  ( 7.716005876422150855, -5.915902021225892149, 34.75552854090298638 ) ) ;
#47241=CARTESIAN_POINT ( 'NONE',  ( 9.757563263583719504, -2.892918686051625166, 31.69288490824026638 ) ) ;
#47242=VECTOR ( 'NONE', #67080, 1000.000000000000000 ) ;
#47243=CARTESIAN_POINT ( 'NONE',  ( 8.703147358274886614, -12.10708131394839349, 31.69288490824020244 ) ) ;
#47244=B_SPLINE_CURVE_WITH_KNOTS ( 'NONE', 3,
 ( #56888, #56456, #31073, #15920, #42068, #35296, #83943, #70864, #24314, #9166 ),
 .UNSPECIFIED., .F., .F.,
 ( 4, 2, 2, 2, 4 ),
 ( 0.0007817246256747474977, 0.0009771112852218911526, 0.001172497944769034699, 0.001367884604316178462, 0.001563271263863322009 ),
 .UNSPECIFIED. ) ;
#47245=CARTESIAN_POINT ( 'NONE',  ( -0.2385256174450664235, -4.026326845037961455, 33.68677907613344047 ) ) ;
#47246=CARTESIAN_POINT ( 'NONE',  ( -8.638705330997126453, -11.66157788607254098, 32.95092075102925833 ) ) ;
#47247=EDGE_CURVE ( 'NONE', #77897, #18500, #6439, .T. ) ;
#47249=CARTESIAN_POINT ( 'NONE',  ( -3.480745974817820887, -12.41104346484419452, 31.60698883733904196 ) ) ;
#47250=ORIENTED_EDGE ( 'NONE', *, *, #47625, .T. ) ;
#47251=CARTESIAN_POINT ( 'NONE',  ( -4.283993363284374745, -5.195881422630167279, 34.18770438780618548 ) ) ;
#47252=CARTESIAN_POINT ( 'NONE',  ( -3.230769230769229949, -3.513871655860378418, 32.76840700105978499 ) ) ;
#47254=CARTESIAN_POINT ( 'NONE',  ( -0.2115930521604175163, -10.92531984108285670, 33.72920026020278073 ) ) ;
#47255=CARTESIAN_POINT ( 'NONE',  ( 6.000000000000001776, -9.819645486525091727, 36.12317359536749706 ) ) ;
#47256=CARTESIAN_POINT ( 'NONE',  ( 10.36536137809165403, -5.851115903089112003, 34.47074536777953568 ) ) ;
#47257=CARTESIAN_POINT ( 'NONE',  ( 10.36538461538461675, -7.500000000000001776, 35.00000000000000000 ) ) ;
#47258=ORIENTED_EDGE ( 'NONE', *, *, #18171, .T. ) ;
#47260=CARTESIAN_POINT ( 'NONE',  ( 3.453782074862625784, -8.282913670948747864, 34.94150082978203642 ) ) ;
#47261=EDGE_CURVE ( 'NONE', #47404, #37079, #62522, .T. ) ;
#47262=ORIENTED_EDGE ( 'NONE', *, *, #37356, .F. ) ;
#47263=CARTESIAN_POINT ( 'NONE',  ( 11.60371667797437567, -9.528491918058460186, 34.59228464037086326 ) ) ;
#47264=CARTESIAN_POINT ( 'NONE',  ( 0.3962680155776857061, -2.892918686051582533, 31.69288490824015270 ) ) ;
#47265=VERTEX_POINT ( 'NONE', #27143 ) ;
#47266=CARTESIAN_POINT ( 'NONE',  ( 0.4615384615384611200, -4.945431358278436385, 36.03766855953609394 ) ) ;
#47267=EDGE_CURVE ( 'NONE', #14607, #53071, #1274, .T. ) ;
#47268=ADVANCED_FACE ( 'NONE', ( #34337 ), #20392, .F. ) ;
#47269=LINE ( 'NONE', #40965, #24975 ) ;
#47270=CARTESIAN_POINT ( 'NONE',  ( -8.069080063669991532, -3.586966769969701208, 32.86292498521069660 ) ) ;
#47271=ORIENTED_EDGE ( 'NONE', *, *, #88402, .T. ) ;
#47274=EDGE_CURVE ( 'NONE', #78089, #8848, #25841, .T. ) ;
#47276=CARTESIAN_POINT ( 'NONE',  ( 7.596130621932389637, -9.356822207818508375, 34.66110646841856635 ) ) ;
#47278=CARTESIAN_POINT ( 'NONE',  ( 18.13052543823364360, -10.31582465632704704, 34.18122507451815295 ) ) ;
#47279=CARTESIAN_POINT ( 'NONE',  ( -15.48079245499068612, -2.341070481393819236, 30.72580821765574299 ) ) ;
#47280=CARTESIAN_POINT ( 'NONE',  ( -0.4615384615385826339, -12.27809138561165270, 31.22303859784587132 ) ) ;
#47281=CARTESIAN_POINT ( 'NONE',  ( -3.007989561791163613, -4.989023458446561143, 34.36081565061822118 ) ) ;
#47282=CARTESIAN_POINT ( 'NONE',  ( 13.44987095589141113, -3.300289026998473041, 32.46337939537591666 ) ) ;
#47283=LINE ( 'NONE', #81534, #82339 ) ;
#47285=ORIENTED_EDGE ( 'NONE', *, *, #85819, .T. ) ;
#47286=CARTESIAN_POINT ( 'NONE',  ( -2.307692307692305711, -12.09954503811598769, 35.62045528018868623 ) ) ;
#47287=VERTEX_POINT ( 'NONE', #76209 ) ;
#47288=EDGE_CURVE ( 'NONE', #10737, #10260, #82797, .T. ) ;
#47289=AXIS2_PLACEMENT_3D ( 'NONE', #23523, #78466, #44222 ) ;
#47290=LINE ( 'NONE', #75222, #59367 ) ;
#47291=CARTESIAN_POINT ( 'NONE',  ( 11.78851585009985392, -12.17597550085003810, 31.52189283813460463 ) ) ;
#47292=EDGE_LOOP ( 'NONE', ( #10744, #2388, #74298, #58710 ) ) ;
#47293=CARTESIAN_POINT ( 'NONE',  ( -12.23875879256039489, -11.60474049983371003, 33.02348890104160262 ) ) ;
#47294=B_SPLINE_CURVE_WITH_KNOTS ( 'NONE', 3,
 ( #60706, #81440, #74679, #37213, #36776, #69678, #14746, #21939, #50718, #779 ),
 .UNSPECIFIED., .F., .F.,
 ( 4, 2, 2, 2, 4 ),
 ( 0.000000000000000000, 0.0001954339857564126514, 0.0003908679715128183098, 0.0005863019572692239681, 0.0007817359430256294638 ),
 .UNSPECIFIED. ) ;
#47295=VECTOR ( 'NONE', #51693, 1000.000000000000000 ) ;
#47296=ORIENTED_EDGE ( 'NONE', *, *, #73825, .T. ) ;
#47297=CARTESIAN_POINT ( 'NONE',  ( 17.01165263096229907, -10.21337939537584383, 33.94971097300158647 ) ) ;
#47298=ORIENTED_EDGE ( 'NONE', *, *, #5196, .F. ) ;
#47300=CARTESIAN_POINT ( 'NONE',  ( -18.00000000000012079, -9.528491918059723176, 34.59228464037033035 ) ) ;
#47301=VERTEX_POINT ( 'NONE', #83877 ) ;
#47302=AXIS2_PLACEMENT_3D ( 'NONE', #84899, #8795, #29949 ) ;
#47303=CARTESIAN_POINT ( 'NONE',  ( -12.21148404162501144, -10.06805714834173493, 34.32951233291982618 ) ) ;
#47304=CARTESIAN_POINT ( 'NONE',  ( 10.83816415665302380, -5.114059244376869984, 34.14424750095245287 ) ) ;
#47305=FACE_BOUND ( 'NONE', #21911, .T. ) ;
#47306=DIRECTION ( 'NONE',  ( 0.000000000000000000, 0.3420201433256641055, -0.9396926207859100932 ) ) ;
#47308=CARTESIAN_POINT ( 'NONE',  ( -1.634638608836841644, -2.341070481393820124, 30.72580821765574299 ) ) ;
#47309=CARTESIAN_POINT ( 'NONE',  ( 1.384615384615264011, -12.51329471203414379, 31.30864560766407578 ) ) ;
#47310=DIRECTION ( 'NONE',  ( -0.000000000000000000, 0.7660444431189791237, -0.6427876096865379196 ) ) ;
#47312=CARTESIAN_POINT ( 'NONE',  ( -10.36533030374629760, -4.235687564193447052, 33.53795663066793509 ) ) ;
#47314=ORIENTED_EDGE ( 'NONE', *, *, #73658, .T. ) ;
#47315=CARTESIAN_POINT ( 'NONE',  ( -5.299850035829923200, -11.98009711892699691, 32.48740034544075428 ) ) ;
#47316=CARTESIAN_POINT ( 'NONE',  ( -18.00000000000000000, -9.905515769479279697, 34.41647553114623292 ) ) ;
#47317=EDGE_CURVE ( 'NONE', #30720, #61793, #9716, .T. ) ;
#47318=CARTESIAN_POINT ( 'NONE',  ( -4.088701373126520267, -7.750023224968867197, 34.99404313364389907 ) ) ;
#47319=CARTESIAN_POINT ( 'NONE',  ( 3.480714749117372886, -10.76462480002816235, 33.53768742498949962 ) ) ;
#47320=CARTESIAN_POINT ( 'NONE',  ( 8.834375549950401307, -7.750023224968867197, 34.99404313364389907 ) ) ;
#47321=CARTESIAN_POINT ( 'NONE',  ( -13.38461538461538325, -2.721908614388771852, 31.22303859784724978 ) ) ;
#47323=CARTESIAN_POINT ( 'NONE',  ( -5.999999999999998224, -1.790695186598648903, 34.54067556320373455 ) ) ;
#47324=CARTESIAN_POINT ( 'NONE',  ( -4.854143535654667829, -2.600157965045225339, 30.74683119005207743 ) ) ;
#47325=CARTESIAN_POINT ( 'NONE',  ( -14.30769230769242917, -12.51329471203414379, 31.30864560766407578 ) ) ;
#47327=ORIENTED_EDGE ( 'NONE', *, *, #31684, .F. ) ;
#47328=B_SPLINE_CURVE_WITH_KNOTS ( 'NONE', 3,
 ( #24026, #15181, #44737, #44281, #3759, #72215 ),
 .UNSPECIFIED., .F., .F.,
 ( 4, 2, 4 ),
 ( 0.000000000000000000, 0.0001954784845028914619, 0.0003909569690057829237 ),
 .UNSPECIFIED. ) ;
#47329=AXIS2_PLACEMENT_3D ( 'NONE', #22737, #70935, #30829 ) ;
#47330=VERTEX_POINT ( 'NONE', #82551 ) ;
#47331=B_SPLINE_CURVE_WITH_KNOTS ( 'NONE', 3,
 ( #6956, #61890, #34427, #1087, #77627, #48821, #76296, #202, #34864, #83517 ),
 .UNSPECIFIED., .F., .F.,
 ( 4, 2, 2, 2, 4 ),
 ( 0.0007817246256747463051, 0.0009771112852218896347, 0.001172497944769033181, 0.001367884604316176728, 0.001563271263863320057 ),
 .UNSPECIFIED. ) ;
#47332=ORIENTED_EDGE ( 'NONE', *, *, #9846, .F. ) ;
#47333=DIRECTION ( 'NONE',  ( 0.000000000000000000, 0.3420201433256641055, -0.9396926207859100932 ) ) ;
#47334=EDGE_CURVE ( 'NONE', #19302, #22650, #50553, .T. ) ;
#47335=ORIENTED_EDGE ( 'NONE', *, *, #36300, .F. ) ;
#47336=CYLINDRICAL_SURFACE ( 'NONE', #9359, 0.2500000000000002220 ) ;
#47337=CARTESIAN_POINT ( 'NONE',  ( 4.153846153846154188, -2.499999999999998668, 29.75000000000001421 ) ) ;
#47338=DIRECTION ( 'NONE',  ( 0.000000000000000000, 0.1736481776669267785, -0.9848077530122087975 ) ) ;
#47339=B_SPLINE_CURVE_WITH_KNOTS ( 'NONE', 3,
 ( #49591, #42405, #35188, #69864, #68973, #28894, #27987, #21675, #56351, #76622 ),
 .UNSPECIFIED., .F., .F.,
 ( 4, 2, 2, 2, 4 ),
 ( 0.000000000000000000, 0.0001954339857564053873, 0.0003908679715128107746, 0.0005863019572692161618, 0.0007817359430256215491 ),
 .UNSPECIFIED. ) ;
#47340=CARTESIAN_POINT ( 'NONE',  ( 9.692307692307572609, -8.613356846316285953, 34.62446782046622218 ) ) ;
#47342=VERTEX_POINT ( 'NONE', #14072 ) ;
#47343=CARTESIAN_POINT ( 'NONE',  ( 3.230769230769546141, -2.255955759149395501, 30.00000000000324363 ) ) ;
#47344=CARTESIAN_POINT ( 'NONE',  ( -4.153846153846152411, -6.386643153685126251, 34.62446782046654192 ) ) ;
#47345=EDGE_LOOP ( 'NONE', ( #60728, #34370 ) ) ;
#47346=DIRECTION ( 'NONE',  ( 0.000000000000000000, 0.9396926207859126468, 0.3420201433256571111 ) ) ;
#47347=CARTESIAN_POINT ( 'NONE',  ( 8.992010438208829726, -12.47679350104403007, 31.42216943046555855 ) ) ;
#47348=CARTESIAN_POINT ( 'NONE',  ( -11.66860950819323861, -11.04286588640298561, 33.62463336215343901 ) ) ;
#47349=CARTESIAN_POINT ( 'NONE',  ( -2.530619266599154038, -12.64616026154729411, 30.79003144601913533 ) ) ;
#47350=CARTESIAN_POINT ( 'NONE',  ( -8.638705330997124676, -8.630441415882550871, 34.87705825610312615 ) ) ;
#47351=ADVANCED_FACE ( 'NONE', ( #41546 ), #14968, .F. ) ;
#47352=CYLINDRICAL_SURFACE ( 'NONE', #55013, 0.2499999999999995559 ) ;
#47353=DIRECTION ( 'NONE',  ( -0.000000000000000000, 0.9396926207859093161, -0.3420201433256663259 ) ) ;
#47355=ORIENTED_EDGE ( 'NONE', *, *, #75205, .T. ) ;
#47357=CARTESIAN_POINT ( 'NONE',  ( -14.17690186672535901, -3.338503747796866872, 32.95102852606553512 ) ) ;
#47358=AXIS2_PLACEMENT_3D ( 'NONE', #25502, #4338, #33916 ) ;
#47360=ORIENTED_EDGE ( 'NONE', *, *, #82321, .T. ) ;
#47361=DIRECTION ( 'NONE',  ( 0.000000000000000000, 0.8660254037844377084, -0.5000000000000015543 ) ) ;
#47362=CARTESIAN_POINT ( 'NONE',  ( -2.980823712421087901, -5.852078868378310261, 34.47109172314383585 ) ) ;
#47364=CARTESIAN_POINT ( 'NONE',  ( -7.173100160369890510, -5.851115903089112003, 34.47074536777953568 ) ) ;
#47365=CARTESIAN_POINT ( 'NONE',  ( -2.307692307692305711, -8.318370150425687726, 35.83090037661290239 ) ) ;
#47367=CARTESIAN_POINT ( 'NONE',  ( 17.99999999999987566, -2.657715359629662544, 31.77849191805970364 ) ) ;
#47368=EDGE_LOOP ( 'NONE', ( #55334, #25896 ) ) ;
#47369=FACE_OUTER_BOUND ( 'NONE', #86864, .T. ) ;
#47370=EDGE_CURVE ( 'NONE', #71718, #25852, #42441, .T. ) ;
#47372=CARTESIAN_POINT ( 'NONE',  ( 9.692307692307695177, -6.189225973068211317, 35.74407628777942847 ) ) ;
#47373=CARTESIAN_POINT ( 'NONE',  ( 5.207713517890025123, -12.35292014791297710, 31.75344720912887198 ) ) ;
#47374=B_SPLINE_CURVE_WITH_KNOTS ( 'NONE', 3,
 ( #55861, #8130, #49104, #35599, #84243, #8572, #83799, #45892, #24738, #79242 ),
 .UNSPECIFIED., .F., .F.,
 ( 4, 2, 2, 2, 4 ),
 ( 0.0007817246256747458714, 0.0009771112852218889842, 0.001172497944769032097, 0.001367884604316175210, 0.001563271263863318323 ),
 .UNSPECIFIED. ) ;
#47377=EDGE_LOOP ( 'NONE', ( #41818, #69674, #65586, #78027 ) ) ;
#47378=CARTESIAN_POINT ( 'NONE',  ( 12.59206389977210527, -12.50538340440932394, 31.33453814440721885 ) ) ;
#47380=CARTESIAN_POINT ( 'NONE',  ( 11.53846153846141576, -6.835583212225970762, 34.95778746994575670 ) ) ;
#47382=DIRECTION ( 'NONE',  ( -0.000000000000000000, 1.000000000000000000, -0.000000000000000000 ) ) ;
#47383=CARTESIAN_POINT ( 'NONE',  ( -16.15384615384615330, -11.35647404775217417, 33.31231777344666511 ) ) ;
#47385=LINE ( 'NONE', #541, #6218 ) ;
#47386=LINE ( 'NONE', #21242, #78519 ) ;
#47387=VERTEX_POINT ( 'NONE', #50065 ) ;
#47388=FACE_BOUND ( 'NONE', #60008, .T. ) ;
#47389=VERTEX_POINT ( 'NONE', #82979 ) ;
#47390=DIRECTION ( 'NONE',  ( -0.000000000000000000, 1.000000000000000000, 3.491481338843133355E-15 ) ) ;
#47391=AXIS2_PLACEMENT_3D ( 'NONE', #57755, #23516, #84359 ) ;
#47392=CARTESIAN_POINT ( 'NONE',  ( -0.4615384615385826339, -8.613356846316285953, 34.62446782046622218 ) ) ;
#47393=CARTESIAN_POINT ( 'NONE',  ( 5.010839665967194101, -11.69971097300155272, 32.46337939537587403 ) ) ;
#47394=CARTESIAN_POINT ( 'NONE',  ( 3.164686851409094892, -11.35647404775217595, 33.31231777344666511 ) ) ;
#47395=CARTESIAN_POINT ( 'NONE',  ( 14.37294744720514572, -8.656820664281605460, 34.87096338111211224 ) ) ;
#47397=ORIENTED_EDGE ( 'NONE', *, *, #41064, .F. ) ;
#47398=EDGE_LOOP ( 'NONE', ( #34058, #54608, #34085, #1643 ) ) ;
#47400=CARTESIAN_POINT ( 'NONE',  ( -4.153846153846273204, -6.026961402154118908, 34.52809138561165270 ) ) ;
#47401=CARTESIAN_POINT ( 'NONE',  ( -17.07692307692307665, -9.905515769479276145, 34.41647553114623292 ) ) ;
#47402=CARTESIAN_POINT ( 'NONE',  ( 8.769230769230768274, -4.661471528628507777, 34.16647553114623292 ) ) ;
#47403=CARTESIAN_POINT ( 'NONE',  ( 4.153846153846032507, -3.300289026999228881, 32.46337939537708905 ) ) ;
#47404=VERTEX_POINT ( 'NONE', #55056 ) ;
#47405=CARTESIAN_POINT ( 'NONE',  ( 17.75002326905764960, -9.943427161483782584, 34.11278801902876978 ) ) ;
#47406=VECTOR ( 'NONE', #84964, 1000.000000000000227 ) ;
#47407=CARTESIAN_POINT ( 'NONE',  ( 16.15384615384615330, -1.117168528481311540, 33.14645433367849847 ) ) ;
#47408=CARTESIAN_POINT ( 'NONE',  ( -18.00000000104979492, -12.75000000000000355, 29.50000000010276935 ) ) ;
#47409=CARTESIAN_POINT ( 'NONE',  ( -4.826868657009622865, -11.47946981652013498, 33.17500667209846910 ) ) ;
#47410=ORIENTED_EDGE ( 'NONE', *, *, #13423, .T. ) ;
#47411=VERTEX_POINT ( 'NONE', #7323 ) ;
#47413=ORIENTED_EDGE ( 'NONE', *, *, #48351, .F. ) ;
#47414=CARTESIAN_POINT ( 'NONE',  ( -11.60454494941741999, -12.37446782046654192, 30.86335684631486487 ) ) ;
#47415=FACE_OUTER_BOUND ( 'NONE', #27128, .T. ) ;
#47416=CARTESIAN_POINT ( 'NONE',  ( -8.096177083446809419, -4.335965774309649134, 33.62209801155881905 ) ) ;
#47417=ADVANCED_FACE ( 'NONE', ( #34782 ), #62248, .F. ) ;
#47418=AXIS2_PLACEMENT_3D ( 'NONE', #43831, #69976, #50138 ) ;
#47421=CARTESIAN_POINT ( 'NONE',  ( 17.07692307692307665, -1.215029322943914858, 32.30358669280327177 ) ) ;
#47422=FACE_BOUND ( 'NONE', #40250, .T. ) ;
#47423=ORIENTED_EDGE ( 'NONE', *, *, #71947, .F. ) ;
#47424=CARTESIAN_POINT ( 'NONE',  ( 17.01165263096229907, -6.879047030191174805, 34.71129190930000163 ) ) ;
#47425=CARTESIAN_POINT ( 'NONE',  ( -3.453696189676079165, -3.395401636524185474, 33.02366814457250399 ) ) ;
#47426=ORIENTED_EDGE ( 'NONE', *, *, #14039, .F. ) ;
#47427=CARTESIAN_POINT ( 'NONE',  ( -11.53846153846165912, -12.46129190930018460, 30.37095296980731973 ) ) ;
#47428=ORIENTED_EDGE ( 'NONE', *, *, #84200, .T. ) ;
#47429=FACE_BOUND ( 'NONE', #48670, .T. ) ;
#47430=CARTESIAN_POINT ( 'NONE',  ( 7.715462379486289990, -11.71456829005830080, 32.44064028649416542 ) ) ;
#47431=EDGE_CURVE ( 'NONE', #57842, #44468, #63471, .T. ) ;
#47432=CARTESIAN_POINT ( 'NONE',  ( -39.05038313613820122, -2.249999999999998668, 29.75000000000000355 ) ) ;
#47434=CARTESIAN_POINT ( 'NONE',  ( -7.976713759767205758, -2.254533558242300284, 29.97296025877828285 ) ) ;
#47436=DIRECTION ( 'NONE',  ( -0.000000000000000000, 0.6427876096865404731, -0.7660444431189770143 ) ) ;
#47438=EDGE_CURVE ( 'NONE', #2406, #58364, #70983, .T. ) ;
#47439=CARTESIAN_POINT ( 'NONE',  ( 6.923076923076924238, -5.557115091759785130, 34.35708131394839171 ) ) ;
#47440=FACE_OUTER_BOUND ( 'NONE', #13151, .T. ) ;
#47441=CARTESIAN_POINT ( 'NONE',  ( 12.59206416330202494, -6.852161475712352789, 34.70806712695775786 ) ) ;
#47442=CARTESIAN_POINT ( 'NONE',  ( -17.74994558008654622, -12.65882529074907126, 30.72640787790838601 ) ) ;
#47443=ORIENTED_EDGE ( 'NONE', *, *, #74661, .F. ) ;
#47444=CARTESIAN_POINT ( 'NONE',  ( 16.15384615384603251, -10.90142922262034020, 33.41473453929536674 ) ) ;
#47446=ORIENTED_EDGE ( 'NONE', *, *, #55113, .T. ) ;
#47447=CARTESIAN_POINT ( 'NONE',  ( -8.519176457592454454, -10.66356715214248396, 33.62249196103329751 ) ) ;
#47448=CARTESIAN_POINT ( 'NONE',  ( -4.219929564802034072, -2.538708090699994813, 30.37095296980875148 ) ) ;
#47449=CARTESIAN_POINT ( 'NONE',  ( -13.38461538461538325, -13.87047571288749737, 32.06866353760679544 ) ) ;
#47450=CARTESIAN_POINT ( 'NONE',  ( -11.78843826940389583, -8.303909089506435137, 34.68538101551103381 ) ) ;
#47451=CYLINDRICAL_SURFACE ( 'NONE', #15716, 0.2500000000000012212 ) ;
#47452=CARTESIAN_POINT ( 'NONE',  ( -13.13456096470193302, -3.435999193479609914, 33.07426656108010832 ) ) ;
#47453=CARTESIAN_POINT ( 'NONE',  ( 6.222779541268410597, -11.89424750095246175, 32.13594075562311758 ) ) ;
#47455=EDGE_CURVE ( 'NONE', #17031, #56000, #67794, .T. ) ;
#47456=LINE ( 'NONE', #13243, #79509 ) ;
#47457=AXIS2_PLACEMENT_3D ( 'NONE', #22971, #9901, #56323 ) ;
#47459=VERTEX_POINT ( 'NONE', #6309 ) ;
#47460=CARTESIAN_POINT ( 'NONE',  ( -18.00000000000000000, -8.973038597847269315, 34.52809138561121927 ) ) ;
#47461=ORIENTED_EDGE ( 'NONE', *, *, #12170, .T. ) ;
#47462=ORIENTED_EDGE ( 'NONE', *, *, #75227, .T. ) ;
#47463=CARTESIAN_POINT ( 'NONE',  ( -16.15384615384615330, -13.53365097954675988, 30.81389545987213552 ) ) ;
#47465=DIRECTION ( 'NONE',  ( -1.000000000000000000, 0.000000000000000000, 0.000000000000000000 ) ) ;
#47468=B_SPLINE_CURVE_WITH_KNOTS ( 'NONE', 3,
 ( #54122, #81615, #19899, #46043, #73528, #66761, #13590, #62649, #75300, #83393 ),
 .UNSPECIFIED., .F., .F.,
 ( 4, 2, 2, 2, 4 ),
 ( 0.000000000000000000, 0.0001954311564186870371, 0.0003908623128373740741, 0.0005862934692560610840, 0.0007817246256747481482 ),
 .UNSPECIFIED. ) ;
#47469=DIRECTION ( 'NONE',  ( 0.000000000000000000, 0.3420201433256641055, -0.9396926207859100932 ) ) ;
#47470=CARTESIAN_POINT ( 'NONE',  ( -2.241623956689868358, -6.386643153685127139, 34.62446782046654192 ) ) ;
#47471=DIRECTION ( 'NONE',  ( 0.000000000000000000, 0.7660444431189807890, 0.6427876096865361433 ) ) ;
#47472=CARTESIAN_POINT ( 'NONE',  ( 9.915320536401090123, -12.38742843783360748, 31.66772728687926985 ) ) ;
#47473=LINE ( 'NONE', #39853, #9437 ) ;
#47475=CARTESIAN_POINT ( 'NONE',  ( 10.83839745947800992, -12.38742843783360748, 31.66772728687926985 ) ) ;
#47476=DIRECTION ( 'NONE',  ( -0.000000000000000000, -0.9848077530122086864, -0.1736481776669273613 ) ) ;
#47477=ADVANCED_FACE ( 'NONE', ( #46398 ), #68439, .F. ) ;
#47478=VECTOR ( 'NONE', #80712, 1000.000000000000114 ) ;
#47479=EDGE_CURVE ( 'NONE', #7007, #21466, #73877, .T. ) ;
#47480=CARTESIAN_POINT ( 'NONE',  ( -5.999999999999998224, -11.16473453929635440, 33.15142922261926373 ) ) ;
#47482=CIRCLE ( 'NONE', #20164, 0.2500000000000002220 ) ;
#47483=ORIENTED_EDGE ( 'NONE', *, *, #77836, .T. ) ;
#47484=EDGE_LOOP ( 'NONE', ( #17537, #62577 ) ) ;
#47485=EDGE_CURVE ( 'NONE', #14918, #28285, #14034, .T. ) ;
#47486=CARTESIAN_POINT ( 'NONE',  ( 6.699591979352976345, -2.599994579823202923, 30.74605699353653776 ) ) ;
#47487=CARTESIAN_POINT ( 'NONE',  ( 5.326868595271216478, -9.272278438253401589, 34.42582936511637826 ) ) ;
#47488=DIRECTION ( 'NONE',  ( -0.000000000000000000, 0.8660254037844397068, -0.4999999999999978906 ) ) ;
#47489=CARTESIAN_POINT ( 'NONE',  ( -10.61538461538461320, -13.95598074871891292, 31.83374038241031911 ) ) ;
#47490=EDGE_CURVE ( 'NONE', #72105, #8333, #26962, .T. ) ;
#47492=CARTESIAN_POINT ( 'NONE',  ( 8.639083559792549494, -4.460286881179643004, 33.72017969459903242 ) ) ;
#47494=CARTESIAN_POINT ( 'NONE',  ( -6.223484943723948781, -8.496056993536548418, 34.65000542017679663 ) ) ;
#47496=VERTEX_POINT ( 'NONE', #35994 ) ;
#47497=CARTESIAN_POINT ( 'NONE',  ( 1.134638653673031738, -4.943428324936578910, 34.04746400365624481 ) ) ;
#47498=EDGE_LOOP ( 'NONE', ( #32532, #59945 ) ) ;
#47499=ORIENTED_EDGE ( 'NONE', *, *, #74852, .F. ) ;
#47500=CARTESIAN_POINT ( 'NONE',  ( 17.86930853333243618, -3.062553014421049991, 32.05460306192773601 ) ) ;
#47501=CARTESIAN_POINT ( 'NONE',  ( 15.23076923076910916, -3.643525952248795718, 33.31231777344771672 ) ) ;
#47502=CARTESIAN_POINT ( 'NONE',  ( -0.3954701105360232671, -6.386643153685128027, 34.62446782046654903 ) ) ;
#47504=FACE_OUTER_BOUND ( 'NONE', #5160, .T. ) ;
#47505=ORIENTED_EDGE ( 'NONE', *, *, #73101, .T. ) ;
#47506=VERTEX_POINT ( 'NONE', #56693 ) ;
#47507=EDGE_CURVE ( 'NONE', #89050, #65380, #41960, .T. ) ;
#47508=ORIENTED_EDGE ( 'NONE', *, *, #58811, .F. ) ;
#47509=ORIENTED_EDGE ( 'NONE', *, *, #41639, .F. ) ;
#47510=CARTESIAN_POINT ( 'NONE',  ( -6.250023224221455287, -4.931416488878822335, 34.32920672191015399 ) ) ;
#47511=CARTESIAN_POINT ( 'NONE',  ( -2.438382910802615378, -9.929715669179220328, 34.40415004197138416 ) ) ;
#47513=CARTESIAN_POINT ( 'NONE',  ( 14.08420738312797660, -2.612411019501189369, 31.66733052389439962 ) ) ;
#47514=CARTESIAN_POINT ( 'NONE',  ( 11.53846153846141753, -6.879047030192662504, 34.71129190930017927 ) ) ;
#47515=CARTESIAN_POINT ( 'NONE',  ( 17.93472955403921887, -5.219633306516282545, 34.19971097300152252 ) ) ;
#47516=DIRECTION ( 'NONE',  ( 0.000000000000000000, 0.6427876096865368094, 0.7660444431189802339 ) ) ;
#47517=ORIENTED_EDGE ( 'NONE', *, *, #86108, .F. ) ;
#47518=ORIENTED_EDGE ( 'NONE', *, *, #12795, .T. ) ;
#47520=ORIENTED_EDGE ( 'NONE', *, *, #42900, .F. ) ;
#47521=CARTESIAN_POINT ( 'NONE',  ( 11.53846153846141753, -9.442884908241554243, 34.35708131394783038 ) ) ;
#47522=EDGE_LOOP ( 'NONE', ( #38702, #60680, #82921, #17140 ) ) ;
#47523=CARTESIAN_POINT ( 'NONE',  ( 10.61538461538449596, -12.46129190930018460, 30.37095296980731973 ) ) ;
#47524=CARTESIAN_POINT ( 'NONE',  ( 7.146039826638408421, -7.369474270740069777, 34.74850911626239736 ) ) ;
#47526=ORIENTED_EDGE ( 'NONE', *, *, #2412, .T. ) ;
#47527=B_SPLINE_CURVE_WITH_KNOTS ( 'NONE', 3,
 ( #23406, #78350, #51292, #17099, #73840, #82369, #61633, #60307, #19332, #80600 ),
 .UNSPECIFIED., .F., .F.,
 ( 4, 2, 2, 2, 4 ),
 ( 0.0007817359430256293554, 0.0009771253907249941549, 0.001172514838424358954, 0.001367904286123723537, 0.001563293733823095276 ),
 .UNSPECIFIED. ) ;
#47529=ORIENTED_EDGE ( 'NONE', *, *, #771, .F. ) ;
#47530=CARTESIAN_POINT ( 'NONE',  ( 7.911409417429874580, -12.27809138561124414, 31.22303859784719648 ) ) ;
#47531=B_SPLINE_CURVE_WITH_KNOTS ( 'NONE', 3,
 ( #41476, #68940, #34717, #7698, #62183, #35156, #41926, #490, #27960, #62618 ),
 .UNSPECIFIED., .F., .F.,
 ( 4, 2, 2, 2, 4 ),
 ( 0.0007817246256747453293, 0.0009771112852218889842, 0.001172497944769032531, 0.001367884604316176294, 0.001563271263863319840 ),
 .UNSPECIFIED. ) ;
#47532=FACE_BOUND ( 'NONE', #73413, .T. ) ;
#47536=ADVANCED_FACE ( 'NONE', ( #63449 ), #42752, .F. ) ;
#47538=ORIENTED_EDGE ( 'NONE', *, *, #22145, .F. ) ;
#47539=CARTESIAN_POINT ( 'NONE',  ( 8.519254025182180001, -12.01397095200674059, 32.43157075238190146 ) ) ;
#47540=CARTESIAN_POINT ( 'NONE',  ( 6.923076923076924238, -11.91647553114624181, 32.58852847137148245 ) ) ;
#47542=CARTESIAN_POINT ( 'NONE',  ( -16.94639763868943660, -12.70449254468099198, 30.44128974285582956 ) ) ;
#47543=VECTOR ( 'NONE', #5270, 1000.000000000000227 ) ;
#47544=CARTESIAN_POINT ( 'NONE',  ( 0.5267940328144856688, -12.46129190930001052, 30.37095296980870174 ) ) ;
#47547=CARTESIAN_POINT ( 'NONE',  ( 16.22001529480881388, -7.250054483168842268, 34.74374881642865631 ) ) ;
#47548=CYLINDRICAL_SURFACE ( 'NONE', #74215, 0.2499999999999994726 ) ;
#47549=DIRECTION ( 'NONE',  ( -0.000000000000000000, 0.8660254037844397068, -0.4999999999999978906 ) ) ;
#47550=DIRECTION ( 'NONE',  ( 0.000000000000000000, 0.6427876096865373645, -0.7660444431189797898 ) ) ;
#47551=CARTESIAN_POINT ( 'NONE',  ( 9.019285189144222059, -10.06805714834173493, 34.32951233291982618 ) ) ;
#47552=FACE_BOUND ( 'NONE', #7748, .T. ) ;
#47554=CARTESIAN_POINT ( 'NONE',  ( -17.07692307692307665, -10.67929555188718282, 33.92786785259544047 ) ) ;
#47555=EDGE_CURVE ( 'NONE', #38257, #80199, #31254, .T. ) ;
#47556=CARTESIAN_POINT ( 'NONE',  ( 2.177544337960614307, -10.31621877034669588, 34.18098118002070152 ) ) ;
#47557=DIRECTION ( 'NONE',  ( -0.000000000000000000, 0.9396926207859093161, -0.3420201433256663259 ) ) ;
#47558=CARTESIAN_POINT ( 'NONE',  ( 17.99999999999987566, -11.48612834414049644, 32.76840700105863391 ) ) ;
#47559=CARTESIAN_POINT ( 'NONE',  ( -5.143005456283213483, -12.34228464037088280, 31.77849191805838558 ) ) ;
#47561=ORIENTED_EDGE ( 'NONE', *, *, #2281, .F. ) ;
#47563=EDGE_LOOP ( 'NONE', ( #76483, #39294, #87995, #16162 ) ) ;
#47564=EDGE_CURVE ( 'NONE', #46418, #6445, #43066, .T. ) ;
#47566=ORIENTED_EDGE ( 'NONE', *, *, #70539, .F. ) ;
#47567=CARTESIAN_POINT ( 'NONE',  ( -4.087777802843715058, -12.10708131394839882, 31.69288490824020954 ) ) ;
#47568=CARTESIAN_POINT ( 'NONE',  ( 14.24242230713598900, -4.320704448112771878, 33.92786785259540494 ) ) ;
#47569=EDGE_CURVE ( 'NONE', #52382, #73792, #30134, .T. ) ;
#47570=CARTESIAN_POINT ( 'NONE',  ( -4.946397638689432164, -9.503571793651733657, 34.60286762892837942 ) ) ;
#47571=VERTEX_POINT ( 'NONE', #76531 ) ;
#47574=B_SPLINE_CURVE_WITH_KNOTS ( 'NONE', 3,
 ( #51730, #79234, #78330, #29720, #49975, #37795, #9440, #51273, #2663, #16631 ),
 .UNSPECIFIED., .F., .F.,
 ( 4, 2, 2, 2, 4 ),
 ( 0.000000000000000000, 0.0001954311564186865763, 0.0003908623128373731525, 0.0005862934692560596746, 0.0007817246256747463051 ),
 .UNSPECIFIED. ) ;
#47575=CARTESIAN_POINT ( 'NONE',  ( -13.38461538461538325, -1.242168528481310874, 33.36296068462461051 ) ) ;
#47576=B_SPLINE_CURVE_WITH_KNOTS ( 'NONE', 3,
 ( #7230, #21175, #82456, #54516, #20304, #48202, #75674, #6776, #6354, #28 ),
 .UNSPECIFIED., .F., .F.,
 ( 4, 2, 2, 2, 4 ),
 ( 0.0007817359430256359690, 0.0009771253907250036959, 0.001172514838424371314, 0.001367904286123738933, 0.001563293733823106768 ),
 .UNSPECIFIED. ) ;
#47577=CARTESIAN_POINT ( 'NONE',  ( -6.989159302437058408, -12.62096338111211580, 30.90682066428152197 ) ) ;
#47578=CARTESIAN_POINT ( 'NONE',  ( 7.846153846153725020, -11.94971097300221174, 32.03036669348237098 ) ) ;
#47579=CARTESIAN_POINT ( 'NONE',  ( 1.134638640566794754, -4.818429247618089661, 34.26397095200675125 ) ) ;
#47580=DIRECTION ( 'NONE',  ( 0.000000000000000000, 0.4999999999999960032, -0.8660254037844410391 ) ) ;
#47581=DIRECTION ( 'NONE',  ( -0.000000000000000000, -0.8660254037844399289, -0.4999999999999980016 ) ) ;
#47582=B_SPLINE_CURVE_WITH_KNOTS ( 'NONE', 3,
 ( #26920, #75115, #20162, #13396, #47176, #12958, #43964, #56157, #70110, #43086 ),
 .UNSPECIFIED., .F., .F.,
 ( 4, 2, 2, 2, 4 ),
 ( 0.000000000000000000, 0.0001954339881912776238, 0.0003908679763825552477, 0.0005863019645738329257, 0.0007817359527651104954 ),
 .UNSPECIFIED. ) ;
#47584=B_SPLINE_CURVE_WITH_KNOTS ( 'NONE', 3,
 ( #16607, #36018, #44068, #71550, #63469, #16176, #77432, #9856, #37319, #51250 ),
 .UNSPECIFIED., .F., .F.,
 ( 4, 2, 2, 2, 4 ),
 ( 0.0007817359430256371616, 0.0009771253907250049969, 0.001172514838424373049, 0.001367904286123741101, 0.001563293733823108937 ),
 .UNSPECIFIED. ) ;
#47585=CARTESIAN_POINT ( 'NONE',  ( 9.626983679503386071, -7.749976730030849303, 34.74374725381503737 ) ) ;
#47587=ORIENTED_EDGE ( 'NONE', *, *, #2941, .F. ) ;
#47588=AXIS2_PLACEMENT_3D ( 'NONE', #68593, #83456, #19957 ) ;
#47591=AXIS2_PLACEMENT_3D ( 'NONE', #6287, #34187, #61207 ) ;
#47592=EDGE_CURVE ( 'NONE', #84519, #87581, #78737, .T. ) ;
#47593=CARTESIAN_POINT ( 'NONE',  ( 2.057669083470851756, -4.931416488878823223, 34.32920672191015399 ) ) ;
#47594=CARTESIAN_POINT ( 'NONE',  ( 5.326868486301119532, -6.653508905675592722, 34.93172785388651391 ) ) ;
#47595=ORIENTED_EDGE ( 'NONE', *, *, #4314, .T. ) ;
#47596=CARTESIAN_POINT ( 'NONE',  ( -7.846153846153844924, -8.318370150425687726, 35.83090037661290239 ) ) ;
#47598=CARTESIAN_POINT ( 'NONE',  ( 16.15384615384615330, -4.786620604624113540, 33.94971097300155094 ) ) ;
#47599=ORIENTED_EDGE ( 'NONE', *, *, #79069, .T. ) ;
#47600=CARTESIAN_POINT ( 'NONE',  ( -2.057692307690886846, -7.500000000000154543, 35.00000000000007105 ) ) ;
#47601=ADVANCED_FACE ( 'NONE', ( #4408 ), #17487, .F. ) ;
#47602=CARTESIAN_POINT ( 'NONE',  ( -15.09997878980228059, -11.93129842949671726, 32.56571108434900452 ) ) ;
#47603=CARTESIAN_POINT ( 'NONE',  ( 9.626224281351815293, -11.16473453929635440, 33.15142922261925662 ) ) ;
#47604=CARTESIAN_POINT ( 'NONE',  ( 4.853438133199127869, -4.386631170607603991, 33.66268669641500111 ) ) ;
#47605=CARTESIAN_POINT ( 'NONE',  ( -13.63463862190834952, -11.86270091957321249, 32.19358267280087915 ) ) ;
#47606=AXIS2_PLACEMENT_3D ( 'NONE', #78233, #73260, #4356 ) ;
#47608=ORIENTED_EDGE ( 'NONE', *, *, #20923, .F. ) ;
#47609=EDGE_LOOP ( 'NONE', ( #77303, #76180 ) ) ;
#47610=EDGE_CURVE ( 'NONE', #16729, #71888, #75975, .T. ) ;
#47611=ORIENTED_EDGE ( 'NONE', *, *, #1175, .T. ) ;
#47613=AXIS2_PLACEMENT_3D ( 'NONE', #69963, #69521, #6934 ) ;
#47615=CARTESIAN_POINT ( 'NONE',  ( 5.299702618191482806, -12.24180327182771855, 31.33663988360758168 ) ) ;
#47617=EDGE_CURVE ( 'NONE', #84921, #78012, #38193, .T. ) ;
#47618=CARTESIAN_POINT ( 'NONE',  ( 9.758376043310132530, -4.786620604624113540, 33.94971097300155805 ) ) ;
#47621=CARTESIAN_POINT ( 'NONE',  ( -2.373775718648186484, -5.557115091759785130, 34.35708131394839171 ) ) ;
#47622=CARTESIAN_POINT ( 'NONE',  ( 16.15384615384603251, -5.219633306517616589, 34.19971097300220464 ) ) ;
#47623=VERTEX_POINT ( 'NONE', #10729 ) ;
#47624=B_SPLINE_CURVE_WITH_KNOTS ( 'NONE', 3,
 ( #45102, #31140, #44197, #58612, #3230, #24380, #18093, #73030, #72579, #10886 ),
 .UNSPECIFIED., .F., .F.,
 ( 4, 2, 2, 2, 4 ),
 ( 0.000000000000000000, 0.0001954311564186871184, 0.0003908623128373742367, 0.0005862934692560614093, 0.0007817246256747484735 ),
 .UNSPECIFIED. ) ;
#47625=EDGE_CURVE ( 'NONE', #79882, #36678, #38766, .T. ) ;
#47626=ORIENTED_EDGE ( 'NONE', *, *, #61916, .F. ) ;
#47627=EDGE_LOOP ( 'NONE', ( #58230, #21936, #77341, #47298 ) ) ;
#47629=VERTEX_POINT ( 'NONE', #51683 ) ;
#47630=CARTESIAN_POINT ( 'NONE',  ( -1.515305987725693582, -2.845849958028613624, 32.17971566917920967 ) ) ;
#47633=EDGE_CURVE ( 'NONE', #34772, #58985, #36446, .T. ) ;
#47634=VECTOR ( 'NONE', #83271, 1000.000000000000227 ) ;
#47636=FACE_OUTER_BOUND ( 'NONE', #31992, .T. ) ;
#47637=EDGE_LOOP ( 'NONE', ( #30209, #35786 ) ) ;
#47638=VERTEX_POINT ( 'NONE', #9834 ) ;
#47639=EDGE_CURVE ( 'NONE', #71802, #62031, #37553, .T. ) ;
#47640=EDGE_LOOP ( 'NONE', ( #77295, #61385, #23409, #54387 ) ) ;
#47642=DIRECTION ( 'NONE',  ( 0.000000000000000000, 0.8660254037844377084, 0.5000000000000015543 ) ) ;
#47643=ORIENTED_EDGE ( 'NONE', *, *, #58443, .F. ) ;
#47644=CARTESIAN_POINT ( 'NONE',  ( -2.307692307692305711, -8.120952969808772792, 34.71129190930000163 ) ) ;
#47645=AXIS2_PLACEMENT_3D ( 'NONE', #50246, #48933, #28672 ) ;
#47646=DIRECTION ( 'NONE',  ( -0.000000000000000000, -0.6427876096865404731, -0.7660444431189771253 ) ) ;
#47647=ORIENTED_EDGE ( 'NONE', *, *, #40617, .F. ) ;
#47648=CARTESIAN_POINT ( 'NONE',  ( 16.21991450484859953, -3.513871655860379306, 32.76840700105978499 ) ) ;
#47649=CARTESIAN_POINT ( 'NONE',  ( 0.2115617174898694053, -9.234221910056348293, 34.70572697212741531 ) ) ;
#47650=FACE_BOUND ( 'NONE', #38310, .T. ) ;
#47651=DIRECTION ( 'NONE',  ( 0.000000000000000000, 0.7660444431189822323, -0.6427876096865344779 ) ) ;
#47652=CARTESIAN_POINT ( 'NONE',  ( -6.130690603110307002, -12.35290016733513951, 31.75349464988449455 ) ) ;
#47653=LINE ( 'NONE', #75137, #20728 ) ;
#47654=CARTESIAN_POINT ( 'NONE',  ( -18.00000000000000711, -12.74702886152665471, 29.99985851721553587 ) ) ;
#47655=CARTESIAN_POINT ( 'NONE',  ( 5.076923076923075762, -3.050289026998446396, 32.03036669348365706 ) ) ;
#47656=DIRECTION ( 'NONE',  ( 0.000000000000000000, 0.1736481776669275834, 0.9848077530122086864 ) ) ;
#47657=CYLINDRICAL_SURFACE ( 'NONE', #33287, 0.2500000000000008882 ) ;
#47658=EDGE_LOOP ( 'NONE', ( #28139, #33974, #65394, #68529 ) ) ;
#47659=CARTESIAN_POINT ( 'NONE',  ( 14.30769230769231015, -4.098570777380720287, 33.41473453929634729 ) ) ;
#47660=CARTESIAN_POINT ( 'NONE',  ( 13.63461538461682210, -7.500000000000155431, 34.75000000000007105 ) ) ;
#47661=EDGE_CURVE ( 'NONE', #46929, #21962, #8538, .T. ) ;
#47662=ORIENTED_EDGE ( 'NONE', *, *, #1489, .F. ) ;
#47663=CARTESIAN_POINT ( 'NONE',  ( 15.93036122928182330, -2.353723527008297012, 30.78948104536958752 ) ) ;
#47664=CARTESIAN_POINT ( 'NONE',  ( -4.284536756956462966, -3.338472653186242756, 32.95098750199972670 ) ) ;
#47665=ORIENTED_EDGE ( 'NONE', *, *, #50424, .T. ) ;
#47666=CARTESIAN_POINT ( 'NONE',  ( 18.00000000000000000, -3.886160181151819604, 36.00935417666054406 ) ) ;
#47667=CARTESIAN_POINT ( 'NONE',  ( -15.23076923076935252, -12.70778746994576025, 30.41441678777401236 ) ) ;
#47668=FACE_BOUND ( 'NONE', #47484, .T. ) ;
#47669=CARTESIAN_POINT ( 'NONE',  ( -15.23076923076922995, -5.557115091759785130, 34.35708131394839171 ) ) ;
#47671=CARTESIAN_POINT ( 'NONE',  ( 8.096208157792162297, -9.148310452688876993, 34.47095581063188519 ) ) ;
#47672=VECTOR ( 'NONE', #18119, 1000.000000000000000 ) ;
#47674=CARTESIAN_POINT ( 'NONE',  ( -10.36543920600657209, -11.56426240980093745, 33.07394671870546432 ) ) ;
#47676=ORIENTED_EDGE ( 'NONE', *, *, #79009, .F. ) ;
#47677=VECTOR ( 'NONE', #32032, 1000.000000000000000 ) ;
#47678=ORIENTED_EDGE ( 'NONE', *, *, #32237, .F. ) ;
#47681=CARTESIAN_POINT ( 'NONE',  ( 7.173076923076985523, -7.434744860731433924, 35.00000000000000711 ) ) ;
#47683=CYLINDRICAL_SURFACE ( 'NONE', #41404, 0.2499999999999994726 ) ;
#47685=VECTOR ( 'NONE', #61796, 1000.000000000000114 ) ;
#47686=CARTESIAN_POINT ( 'NONE',  ( -12.52762084089859407, -3.937682226553330445, 33.60647404775217240 ) ) ;
#47687=CYLINDRICAL_SURFACE ( 'NONE', #35963, 0.2499999999999986955 ) ;
#47688=CARTESIAN_POINT ( 'NONE',  ( -11.53846153846153655, -13.49023893513002648, 31.06009739812518688 ) ) ;
#47689=CARTESIAN_POINT ( 'NONE',  ( 10.68145194873469173, -3.322132147404559976, 32.92929555188717927 ) ) ;
#47690=DIRECTION ( 'NONE',  ( -0.000000000000000000, -0.9396926207859092051, -0.3420201433256662704 ) ) ;
#47691=CARTESIAN_POINT ( 'NONE',  ( 13.31934493865461278, -4.481592998940162609, 33.73612834413957984 ) ) ;
#47692=CARTESIAN_POINT ( 'NONE',  ( 5.934729554039226862, -12.27809138561121394, 31.22303859784730307 ) ) ;
#47693=CARTESIAN_POINT ( 'NONE',  ( -3.230769230769229949, -2.292212530054420494, 30.41441678777542634 ) ) ;
#47694=ADVANCED_FACE ( 'NONE', ( #4869 ), #71978, .F. ) ;
#47695=CARTESIAN_POINT ( 'NONE',  ( 3.007284287045282944, -2.599994579823203367, 30.74605699353653776 ) ) ;
#47696=ORIENTED_EDGE ( 'NONE', *, *, #54665, .F. ) ;
#47697=CARTESIAN_POINT ( 'NONE',  ( -4.826868765284763718, -11.79725096376909299, 32.30694842903960762 ) ) ;
#47698=CYLINDRICAL_SURFACE ( 'NONE', #41714, 0.2499999999999986955 ) ;
#47701=CARTESIAN_POINT ( 'NONE',  ( -0.2387587925603968930, -10.97394488606064122, 33.68653795673694873 ) ) ;
#47702=PRESENTATION_STYLE_ASSIGNMENT (( #46378 ) ) ;
#47703=FACE_OUTER_BOUND ( 'NONE', #54315, .T. ) ;
#47704=CARTESIAN_POINT ( 'NONE',  ( -14.30769230769230660, -12.10708131394839349, 31.69288490824020244 ) ) ;
#47705=ORIENTED_EDGE ( 'NONE', *, *, #44311, .F. ) ;
#47707=CARTESIAN_POINT ( 'NONE',  ( -14.53117723225663660, -5.827078755546623690, 34.72654668319379567 ) ) ;
#47708=EDGE_CURVE ( 'NONE', #52031, #55252, #46191, .T. ) ;
#47709=VERTEX_POINT ( 'NONE', #26019 ) ;
#47710=CARTESIAN_POINT ( 'NONE',  ( -8.769230769230768274, -10.51840700105979565, 33.73612834413961536 ) ) ;
#47711=LINE ( 'NONE', #75196, #87490 ) ;
#47712=ADVANCED_FACE ( 'NONE', ( #67010 ), #54813, .F. ) ;
#47714=AXIS2_PLACEMENT_3D ( 'NONE', #6554, #46648, #74568 ) ;
#47715=CARTESIAN_POINT ( 'NONE',  ( 7.623227628637700093, -4.186968288167446595, 33.49512374952580274 ) ) ;
#47716=B_SPLINE_CURVE_WITH_KNOTS ( 'NONE', 3,
 ( #1089, #69982, #64106, #1975, #57799, #50594, #64538, #8297, #36216, #83968 ),
 .UNSPECIFIED., .F., .F.,
 ( 4, 2, 2, 2, 4 ),
 ( 0.0007817359430256332585, 0.0009771253907250054306, 0.001172514838424370664, 0.001367904286123735897, 0.001563293733823100913 ),
 .UNSPECIFIED. ) ;
#47717=CARTESIAN_POINT ( 'NONE',  ( 2.438482748659258625, -8.191423895709840863, 34.95447573519442130 ) ) ;
#47718=CARTESIAN_POINT ( 'NONE',  ( 12.46153846153846168, -1.129524287112498415, 32.06866353760679544 ) ) ;
#47721=VERTEX_POINT ( 'NONE', #18822 ) ;
#47722=ADVANCED_FACE ( 'NONE', ( #39990 ), #87745, .F. ) ;
#47723=CARTESIAN_POINT ( 'NONE',  ( 6.130525438233644486, -12.15418822224088657, 32.17964115625579069 ) ) ;
#47724=ORIENTED_EDGE ( 'NONE', *, *, #24772, .T. ) ;
#47725=CARTESIAN_POINT ( 'NONE',  ( -17.74994558008654622, -4.818054556918155207, 34.26375889529406749 ) ) ;
#47726=CARTESIAN_POINT ( 'NONE',  ( 9.692307692307570832, -3.083524468854526912, 32.58852847137268327 ) ) ;
#47727=CARTESIAN_POINT ( 'NONE',  ( -10.83886955910856109, -2.599994579823203367, 30.74605699353653776 ) ) ;
#47728=CARTESIAN_POINT ( 'NONE',  ( -9.822999158975251888, -4.809359713505814149, 33.96456829005828837 ) ) ;
#47729=DIRECTION ( 'NONE',  ( 0.000000000000000000, 0.4999999999999985567, 0.8660254037844395958 ) ) ;
#47730=CARTESIAN_POINT ( 'NONE',  ( 1.254467414883690068, -2.373036134822905208, 30.88089517874951540 ) ) ;
#47731=CARTESIAN_POINT ( 'NONE',  ( -12.46153846153846168, -6.386643153685126251, 34.62446782046654192 ) ) ;
#47732=ORIENTED_EDGE ( 'NONE', *, *, #59918, .T. ) ;
#47733=ORIENTED_EDGE ( 'NONE', *, *, #75188, .F. ) ;
#47734=CARTESIAN_POINT ( 'NONE',  ( -17.32694631421604115, -10.05641848906368097, 34.04755513067966177 ) ) ;
#47735=VERTEX_POINT ( 'NONE', #89071 ) ;
#47736=EDGE_CURVE ( 'NONE', #38569, #45581, #54799, .T. ) ;
#47737=AXIS2_PLACEMENT_3D ( 'NONE', #64698, #2997, #57950 ) ;
#47738=AXIS2_PLACEMENT_3D ( 'NONE', #67677, #87527, #5984 ) ;
#47739=CARTESIAN_POINT ( 'NONE',  ( -13.51509056969110745, -7.276987145209185215, 34.99546412871779211 ) ) ;
#47740=CARTESIAN_POINT ( 'NONE',  ( 8.769230769230645706, -12.16647553114689728, 32.15551576947799362 ) ) ;
#47741=EDGE_LOOP ( 'NONE', ( #25553, #56296 ) ) ;
#47742=CARTESIAN_POINT ( 'NONE',  ( 14.55774672760575861, -12.01375889529407281, 32.43194544308182969 ) ) ;
#47743=AXIS2_PLACEMENT_3D ( 'NONE', #84491, #22766, #8383 ) ;
#47744=B_SPLINE_CURVE_WITH_KNOTS ( 'NONE', 3,
 ( #8773, #2007, #85761, #77217, #9218, #15528, #42994, #43439, #56942, #51492 ),
 .UNSPECIFIED., .F., .F.,
 ( 4, 2, 2, 2, 4 ),
 ( 0.0007817359430256318490, 0.0009771253907249984917, 0.001172514838424365026, 0.001367904286123731560, 0.001563293733823098311 ),
 .UNSPECIFIED. ) ;
#47745=EDGE_CURVE ( 'NONE', #32791, #69549, #27832, .T. ) ;
#47746=VERTEX_POINT ( 'NONE', #87295 ) ;
#47747=CARTESIAN_POINT ( 'NONE',  ( -12.21153846153846168, -2.499999999999998668, 29.75000000000000355 ) ) ;
#47748=ORIENTED_EDGE ( 'NONE', *, *, #65064, .T. ) ;
#47750=ORIENTED_EDGE ( 'NONE', *, *, #7835, .T. ) ;
#47752=CARTESIAN_POINT ( 'NONE',  ( -16.37677237136229991, -6.503392248772476236, 34.64988816332204635 ) ) ;
#47753=CARTESIAN_POINT ( 'NONE',  ( 16.94623161025552704, -2.729777683071817229, 31.24903638046269450 ) ) ;
#47754=FACE_BOUND ( 'NONE', #56444, .T. ) ;
#47755=CARTESIAN_POINT ( 'NONE',  ( 2.307692307692186251, -2.379036618888197285, 30.90682066428292885 ) ) ;
#47756=CARTESIAN_POINT ( 'NONE',  ( 18.00000000000000000, -2.708943851104267164, 35.45975837776705220 ) ) ;
#47757=CARTESIAN_POINT ( 'NONE',  ( -15.90379173393269951, -4.818054556918155207, 34.26375889529406749 ) ) ;
#47759=CARTESIAN_POINT ( 'NONE',  ( -5.076923076923199218, -4.320704448113951379, 33.92786785259630022 ) ) ;
#47760=CARTESIAN_POINT ( 'NONE',  ( -12.46153846153846168, -13.37000171582298513, 34.34916445242398453 ) ) ;
#47761=DIRECTION ( 'NONE',  ( -0.000000000000000000, 0.9396926207859092051, -0.3420201433256662704 ) ) ;
#47762=VERTEX_POINT ( 'NONE', #81417 ) ;
#47764=VERTEX_POINT ( 'NONE', #74657 ) ;
#47765=CARTESIAN_POINT ( 'NONE',  ( 2.241608896736429823, -10.51840700105979387, 33.73612834413961536 ) ) ;
#47766=CARTESIAN_POINT ( 'NONE',  ( -18.00000000000012079, -10.33852847137269926, 34.16647553114546554 ) ) ;
#47767=VECTOR ( 'NONE', #61386, 999.9999999999998863 ) ;
#47768=CARTESIAN_POINT ( 'NONE',  ( 7.173131234715237170, -6.567000820036038355, 34.66262288849541306 ) ) ;
#47769=LINE ( 'NONE', #34252, #22120 ) ;
#47770=EDGE_CURVE ( 'NONE', #84339, #77971, #60049, .T. ) ;
#47771=CARTESIAN_POINT ( 'NONE',  ( -17.14219307747939069, -12.51329471203370325, 31.30864560766548976 ) ) ;
#47772=DIRECTION ( 'NONE',  ( 0.000000000000000000, 1.000000000000000000, 0.000000000000000000 ) ) ;
#47773=EDGE_CURVE ( 'NONE', #49979, #52323, #23515, .T. ) ;
#47774=VERTEX_POINT ( 'NONE', #56143 ) ;
#47775=CARTESIAN_POINT ( 'NONE',  ( -11.60454494941741999, -12.10708131394839349, 31.69288490824020244 ) ) ;
#47776=CARTESIAN_POINT ( 'NONE',  ( 11.28846153846153832, -7.566083408709835645, 34.74999999999999289 ) ) ;
#47777=CARTESIAN_POINT ( 'NONE',  ( -3.230769230769352962, -11.67786785259630911, 32.92929555188603530 ) ) ;
#47778=DIRECTION ( 'NONE',  ( 0.000000000000000000, 1.000000000000000000, 0.000000000000000000 ) ) ;
#47779=AXIS2_PLACEMENT_3D ( 'NONE', #10719, #65642, #66092 ) ;
#47780=ORIENTED_EDGE ( 'NONE', *, *, #51996, .T. ) ;
#47781=EDGE_CURVE ( 'NONE', #64679, #26488, #17259, .T. ) ;
#47782=VERTEX_POINT ( 'NONE', #29564 ) ;
#47783=ORIENTED_EDGE ( 'NONE', *, *, #76428, .T. ) ;
#47784=LINE ( 'NONE', #74375, #70793 ) ;
#47785=B_SPLINE_CURVE_WITH_KNOTS ( 'NONE', 3,
 ( #73897, #66235, #66690, #81546, #40123, #19833, #60816, #46417, #81992, #67583 ),
 .UNSPECIFIED., .F., .F.,
 ( 4, 2, 2, 2, 4 ),
 ( 0.0007817359430256390048, 0.0009771253907250078159, 0.001172514838424376735, 0.001367904286123745655, 0.001563293733823114574 ),
 .UNSPECIFIED. ) ;
#47786=VERTEX_POINT ( 'NONE', #84078 ) ;
#47787=CARTESIAN_POINT ( 'NONE',  ( -15.93083480223330817, -4.887748414852789658, 34.01359900205216746 ) ) ;
#47788=CARTESIAN_POINT ( 'NONE',  ( 5.076923076923075762, -12.09954503811598769, 35.62045528018868623 ) ) ;
#47789=CARTESIAN_POINT ( 'NONE',  ( -5.300408020647025431, -4.386631170607603991, 33.66268669641500111 ) ) ;
#47790=CARTESIAN_POINT ( 'NONE',  ( -2.084680956079457470, -4.887748414852789658, 34.01359900205216746 ) ) ;
#47791=CARTESIAN_POINT ( 'NONE',  ( -11.53846153846153655, -6.386643153685126251, 34.62446782046654192 ) ) ;
#47792=EDGE_LOOP ( 'NONE', ( #84208, #88679 ) ) ;
#47793=FACE_OUTER_BOUND ( 'NONE', #84582, .T. ) ;
#47794=CARTESIAN_POINT ( 'NONE',  ( -16.15384615384615330, -11.69971097300155272, 32.46337939537588113 ) ) ;
#47795=VERTEX_POINT ( 'NONE', #70096 ) ;
#47796=CYLINDRICAL_SURFACE ( 'NONE', #23850, 0.2500000000000004996 ) ;
#47797=CARTESIAN_POINT ( 'NONE',  ( -3.230769230769229949, -2.486705287966279876, 31.30864560766543647 ) ) ;
#47798=CARTESIAN_POINT ( 'NONE',  ( 4.153846153846154188, -4.102666532097928531, 36.13435417666054406 ) ) ;
#47799=CARTESIAN_POINT ( 'NONE',  ( -16.28445580905022894, -7.722926974430166069, 34.99546784045485737 ) ) ;
#47800=CARTESIAN_POINT ( 'NONE',  ( -12.68446467905461006, -2.758268499246657068, 31.33685645148948140 ) ) ;
#47801=CARTESIAN_POINT ( 'NONE',  ( 17.20697068317875988, -7.723484964179501588, 34.74522123443823318 ) ) ;
#47802=CARTESIAN_POINT ( 'NONE',  ( -0.5916856709766811218, -12.45813303252208648, 30.39737893381572675 ) ) ;
#47804=EDGE_LOOP ( 'NONE', ( #47360, #79993 ) ) ;
#47806=CARTESIAN_POINT ( 'NONE',  ( -14.05763788777885637, -3.435999193479609914, 33.07426656108010832 ) ) ;
#47809=CARTESIAN_POINT ( 'NONE',  ( 9.915320536401090123, -10.77377354290276124, 33.85451476688484718 ) ) ;
#47810=CARTESIAN_POINT ( 'NONE',  ( -13.25408968285182354, -8.586989748646452369, 34.63063291749215011 ) ) ;
#47811=ORIENTED_EDGE ( 'NONE', *, *, #10281, .F. ) ;
#47812=CARTESIAN_POINT ( 'NONE',  ( -12.46153846153858247, -11.94971097300221174, 32.03036669348237098 ) ) ;
#47814=AXIS2_PLACEMENT_3D ( 'NONE', #16036, #70978, #83171 ) ;
#47815=CARTESIAN_POINT ( 'NONE',  ( 2.438217745925951085, -11.04252011169590020, 33.62494198852677130 ) ) ;
#47816=DIRECTION ( 'NONE',  ( -0.000000000000000000, 0.1736481776669307198, -0.9848077530122080203 ) ) ;
#47817=EDGE_CURVE ( 'NONE', #10982, #2406, #14272, .T. ) ;
#47818=CARTESIAN_POINT ( 'NONE',  ( -14.53061926659915315, -2.889293201056495786, 32.26117774369186009 ) ) ;
#47819=ORIENTED_EDGE ( 'NONE', *, *, #13702, .F. ) ;
#47820=CARTESIAN_POINT ( 'NONE',  ( -15.23076923076922995, -2.721908614388771852, 31.22303859784724978 ) ) ;
#47822=DIRECTION ( 'NONE',  ( -0.000000000000000000, -0.1736481776669307198, -0.9848077530122080203 ) ) ;
#47823=EDGE_LOOP ( 'NONE', ( #87737, #55265 ) ) ;
#47824=EDGE_CURVE ( 'NONE', #45139, #14506, #34980, .T. ) ;
#47825=CYLINDRICAL_SURFACE ( 'NONE', #55684, 0.2499999999999973355 ) ;
#47826=ORIENTED_EDGE ( 'NONE', *, *, #39525, .F. ) ;
#47827=CARTESIAN_POINT ( 'NONE',  ( -2.557715544985271983, -12.22074536777954989, 31.39888409691088356 ) ) ;
#47828=CARTESIAN_POINT ( 'NONE',  ( 11.47237915910140771, -2.486705287966279432, 31.30864560766542937 ) ) ;
#47829=ORIENTED_EDGE ( 'NONE', *, *, #65431, .F. ) ;
#47830=CARTESIAN_POINT ( 'NONE',  ( -17.93393266664992325, -9.905515769479281474, 34.41647553114623292 ) ) ;
#47831=FACE_OUTER_BOUND ( 'NONE', #3211, .T. ) ;
#47832=CARTESIAN_POINT ( 'NONE',  ( 13.16168916709923664, -6.503392248772476236, 34.64988816332204635 ) ) ;
#47833=EDGE_CURVE ( 'NONE', #3657, #66348, #63337, .T. ) ;
#47834=CARTESIAN_POINT ( 'NONE',  ( 7.053602361310568725, -12.50538340440932217, 31.33453814440721885 ) ) ;
#47835=CARTESIAN_POINT ( 'NONE',  ( -0.6850233861027926752, -11.60425143139329940, 33.02411095842164457 ) ) ;
#47836=EDGE_LOOP ( 'NONE', ( #69230, #55725, #9852, #50375 ) ) ;
#47837=FACE_BOUND ( 'NONE', #42642, .T. ) ;
#47838=EDGE_LOOP ( 'NONE', ( #72646, #47115 ) ) ;
#47839=DIRECTION ( 'NONE',  ( -0.000000000000000000, 0.7660444431189791237, -0.6427876096865379196 ) ) ;
#47840=CARTESIAN_POINT ( 'NONE',  ( 18.06525513951284267, -6.835583212224605631, 34.95778746994559327 ) ) ;
#47842=CARTESIAN_POINT ( 'NONE',  ( -17.07692307692319744, -6.026961402154118908, 34.52809138561165270 ) ) ;
#47843=CARTESIAN_POINT ( 'NONE',  ( -6.130691466667561151, -12.11776431015576172, 31.66791131148498906 ) ) ;
#47844=ORIENTED_EDGE ( 'NONE', *, *, #35388, .F. ) ;
#47845=EDGE_LOOP ( 'NONE', ( #2240, #68683 ) ) ;
#47846=VERTEX_POINT ( 'NONE', #15163 ) ;
#47847=CARTESIAN_POINT ( 'NONE',  ( -0.4615384615385826339, -3.300289026999228881, 32.46337939537708905 ) ) ;
#47849=ADVANCED_FACE ( 'NONE', ( #7521 ), #44720, .F. ) ;
#47851=CARTESIAN_POINT ( 'NONE',  ( -17.14219307747939425, -10.33852847137145048, 34.16647553114627556 ) ) ;
#47852=CARTESIAN_POINT ( 'NONE',  ( -9.442307692307627676, -7.434744429011176159, 34.75000000000000711 ) ) ;
#47853=CARTESIAN_POINT ( 'NONE',  ( 4.946232473812767871, -11.37499894934982514, 33.29245874905763003 ) ) ;
#47855=CARTESIAN_POINT ( 'NONE',  ( 11.47237812750565666, -2.538708090699994813, 30.37095296980875148 ) ) ;
#47856=AXIS2_PLACEMENT_3D ( 'NONE', #56706, #76546, #8532 ) ;
#47859=CARTESIAN_POINT ( 'NONE',  ( -4.946397375159513388, -4.459921816937789885, 33.71989282347011851 ) ) ;
#47860=CARTESIAN_POINT ( 'NONE',  ( -5.076923076923075762, -3.513871655860378418, 32.76840700105978499 ) ) ;
#47861=VERTEX_POINT ( 'NONE', #63779 ) ;
#47862=VERTEX_POINT ( 'NONE', #56587 ) ;
#47863=EDGE_CURVE ( 'NONE', #57873, #5535, #17146, .T. ) ;
#47864=VECTOR ( 'NONE', #35550, 1000.000000000000114 ) ;
#47865=ORIENTED_EDGE ( 'NONE', *, *, #61928, .F. ) ;
#47866=DIRECTION ( 'NONE',  ( 0.000000000000000000, 0.9848077530122072432, 0.1736481776669354937 ) ) ;
#47867=CARTESIAN_POINT ( 'NONE',  ( 1.384615384615265343, -6.026961402154118908, 34.52809138561165270 ) ) ;
#47868=CARTESIAN_POINT ( 'NONE',  ( -5.777220458731585850, -3.755027918224367767, 33.06320215134714857 ) ) ;
#47869=B_SPLINE_CURVE_WITH_KNOTS ( 'NONE', 3,
 ( #59424, #1938, #86931, #15463, #70849, #15905, #4020, #22211, #86011, #63186 ),
 .UNSPECIFIED., .F., .F.,
 ( 4, 2, 2, 2, 4 ),
 ( 0.000000000000000000, 0.0001954311564186865221, 0.0003908623128373730441, 0.0005862934692560595662, 0.0007817246256747460882 ),
 .UNSPECIFIED. ) ;
#47871=CARTESIAN_POINT ( 'NONE',  ( -15.45425415533356173, -10.23692288466677880, 34.23039457007281072 ) ) ;
#47873=FACE_BOUND ( 'NONE', #57839, .T. ) ;
#47874=DIRECTION ( 'NONE',  ( -0.000000000000000000, 1.000000000000000000, 3.491481338843133355E-15 ) ) ;
#47875=VERTEX_POINT ( 'NONE', #81197 ) ;
#47876=CARTESIAN_POINT ( 'NONE',  ( 8.096208266067295156, -2.318338780012835443, 30.59689888758630261 ) ) ;
#47878=CARTESIAN_POINT ( 'NONE',  ( 2.980792499826877329, -10.66389620160130036, 33.62221079203477103 ) ) ;
#47880=CARTESIAN_POINT ( 'NONE',  ( -4.826868765284762830, -6.567000820036038355, 34.66262288849541306 ) ) ;
#47881=ORIENTED_EDGE ( 'NONE', *, *, #67683, .F. ) ;
#47882=FACE_BOUND ( 'NONE', #47823, .T. ) ;
#47883=CARTESIAN_POINT ( 'NONE',  ( 9.692307692307695177, -5.557115091759785130, 34.35708131394839171 ) ) ;
#47884=CARTESIAN_POINT ( 'NONE',  ( -7.846153846153530509, -2.255955759149395501, 30.00000000000324363 ) ) ;
#47885=CARTESIAN_POINT ( 'NONE',  ( -12.59168643127015486, -12.15440758774515473, 32.17923288041532004 ) ) ;
#47886=EDGE_LOOP ( 'NONE', ( #79457, #82825, #65025, #74488 ) ) ;
#47887=CARTESIAN_POINT ( 'NONE',  ( 6.857806477116147548, -6.026961402152685388, 34.52809138561120506 ) ) ;
#47888=CARTESIAN_POINT ( 'NONE',  ( -7.780086512803768173, -8.164416787775445883, 34.95778746994558617 ) ) ;
#47889=DIRECTION ( 'NONE',  ( -0.000000000000000000, -0.9848077530122086864, -0.1736481776669273613 ) ) ;
#47891=ORIENTED_EDGE ( 'NONE', *, *, #86622, .T. ) ;
#47892=CARTESIAN_POINT ( 'NONE',  ( 13.38461538461526601, -6.026961402154118019, 34.52809138561165270 ) ) ;
#47893=AXIS2_PLACEMENT_3D ( 'NONE', #17240, #84837, #70872 ) ;
#47894=CARTESIAN_POINT ( 'NONE',  ( -15.48079246806219267, -4.335965774309649134, 33.62209801155881905 ) ) ;
#47895=CARTESIAN_POINT ( 'NONE',  ( 4.403900573759607084, -2.920487667080175154, 32.31805714834170828 ) ) ;
#47896=AXIS2_PLACEMENT_3D ( 'NONE', #58365, #66922, #51596 ) ;
#47897=EDGE_LOOP ( 'NONE', ( #71351, #43178, #33457, #15894 ) ) ;
#47898=CARTESIAN_POINT ( 'NONE',  ( 16.08776377448601735, -3.937682226553330445, 33.60647404775217240 ) ) ;
#47899=CARTESIAN_POINT ( 'NONE',  ( 5.076923076923075762, -11.91647553114624181, 32.58852847137148245 ) ) ;
#47901=CARTESIAN_POINT ( 'NONE',  ( -2.307692307692427391, -4.481592998941358097, 33.73612834414048933 ) ) ;
#47902=CARTESIAN_POINT ( 'NONE',  ( -13.38461538461550759, -3.643525952248795718, 33.31231777344771672 ) ) ;
#47904=CARTESIAN_POINT ( 'NONE',  ( -16.85414353565466072, -8.496831190052089866, 34.64984203495476578 ) ) ;
#47905=CARTESIAN_POINT ( 'NONE',  ( 16.15384615384615330, -13.75783147151868846, 33.36296068462461051 ) ) ;
#47907=ORIENTED_EDGE ( 'NONE', *, *, #63770, .T. ) ;
#47908=DIRECTION ( 'NONE',  ( 0.000000000000000000, 0.6427876096865368094, 0.7660444431189802339 ) ) ;
#47909=VERTEX_POINT ( 'NONE', #31212 ) ;
#47910=VERTEX_POINT ( 'NONE', #66340 ) ;
#47911=CARTESIAN_POINT ( 'NONE',  ( -22.75000000000000000, -7.500000000000000000, 29.75000000000000355 ) ) ;
#47912=ORIENTED_EDGE ( 'NONE', *, *, #28238, .T. ) ;
#47913=LINE ( 'NONE', #6930, #11018 ) ;
#47916=CARTESIAN_POINT ( 'NONE',  ( -7.976844449264153702, -8.191372820521381826, 34.95448215188424967 ) ) ;
#47917=CARTESIAN_POINT ( 'NONE',  ( 5.999999999999880096, -3.300289026999228881, 32.46337939537708905 ) ) ;
#47918=B_SPLINE_CURVE_WITH_KNOTS ( 'NONE', 3,
 ( #65240, #17060, #11649, #58930, #72443, #52617, #80100, #66593, #44963, #24247 ),
 .UNSPECIFIED., .F., .F.,
 ( 4, 2, 2, 2, 4 ),
 ( 0.000000000000000000, 0.0001954339857564078267, 0.0003908679715128156535, 0.0005863019572692235344, 0.0007817359430256313069 ),
 .UNSPECIFIED. ) ;
#47919=CARTESIAN_POINT ( 'NONE',  ( -7.053767526187232129, -9.084618155246140248, 34.75535874321725771 ) ) ;
#47920=CARTESIAN_POINT ( 'NONE',  ( 9.942362112221147186, -12.41089969410671223, 31.60739465890703670 ) ) ;
#47921=CARTESIAN_POINT ( 'NONE',  ( 2.438218009455871194, -11.46989282347013095, 32.79007818306219946 ) ) ;
#47922=B_SPLINE_CURVE_WITH_KNOTS ( 'NONE', 3,
 ( #34759, #61329, #62229, #6417, #538, #55473, #48714, #977, #28449, #63109 ),
 .UNSPECIFIED., .F., .F.,
 ( 4, 2, 2, 2, 4 ),
 ( 0.000000000000000000, 0.0001954339857564074473, 0.0003908679715128148945, 0.0005863019572692223418, 0.0007817359430256297891 ),
 .UNSPECIFIED. ) ;
#47923=CARTESIAN_POINT ( 'NONE',  ( 6.699591998512590685, -12.47654668319379567, 31.42292124445336654 ) ) ;
#47924=B_SPLINE_CURVE_WITH_KNOTS ( 'NONE', 3,
 ( #10108, #56080, #15990, #78561, #42576, #36699, #23182, #29944, #9239, #16426 ),
 .UNSPECIFIED., .F., .F.,
 ( 4, 2, 2, 2, 4 ),
 ( 0.0007817246256747455461, 0.0009771112852218885505, 0.001172497944769031446, 0.001367884604316174559, 0.001563271263863317455 ),
 .UNSPECIFIED. ) ;
#47925=CARTESIAN_POINT ( 'NONE',  ( -0.6850234052624093462, -2.599994579823202923, 30.74605699353653776 ) ) ;
#47926=CARTESIAN_POINT ( 'NONE',  ( 15.00728430620490350, -9.417330523894424488, 34.63758898049880486 ) ) ;
#47927=CYLINDRICAL_SURFACE ( 'NONE', #60814, 0.2499999999999986955 ) ;
#47928=AXIS2_PLACEMENT_3D ( 'NONE', #85433, #36365, #1688 ) ;
#47929=VERTEX_POINT ( 'NONE', #4642 ) ;
#47930=EDGE_LOOP ( 'NONE', ( #81036, #62120, #48409, #76133, #28233, #44045 ) ) ;
#47931=CARTESIAN_POINT ( 'NONE',  ( 12.68455130563185662, -2.523321265292115534, 31.42251411153756990 ) ) ;
#47932=FACE_OUTER_BOUND ( 'NONE', #36122, .T. ) ;
#47933=LINE ( 'NONE', #88077, #26801 ) ;
#47934=CARTESIAN_POINT ( 'NONE',  ( 5.749976762707036393, -5.851115903089112003, 34.47074536777953568 ) ) ;
#47935=DIRECTION ( 'NONE',  ( -0.000000000000000000, 0.5000000000000011102, -0.8660254037844381525 ) ) ;
#47936=FACE_OUTER_BOUND ( 'NONE', #51678, .T. ) ;
#47937=CARTESIAN_POINT ( 'NONE',  ( -2.438382910802613157, -8.191372820521381826, 34.95448215188423546 ) ) ;
#47938=ORIENTED_EDGE ( 'NONE', *, *, #8344, .T. ) ;
#47939=CARTESIAN_POINT ( 'NONE',  ( -14.37377468705243899, -12.62096338111211580, 30.90682066428152908 ) ) ;
#47940=EDGE_LOOP ( 'NONE', ( #10323, #50457, #18703, #21834 ) ) ;
#47941=CARTESIAN_POINT ( 'NONE',  ( -8.769230769230892619, -5.094484230521993062, 34.41647553114689373 ) ) ;
#47942=EDGE_CURVE ( 'NONE', #17127, #1706, #20355, .T. ) ;
#47943=CARTESIAN_POINT ( 'NONE',  ( 15.29602437028207085, -3.643525952247864463, 33.31231777344670064 ) ) ;
#47944=CARTESIAN_POINT ( 'NONE',  ( -6.673076923076987299, -7.565270000091922853, 34.99999999999999289 ) ) ;
#47946=CARTESIAN_POINT ( 'NONE',  ( -15.29685264172511161, -3.050289026998445951, 32.03036669348365706 ) ) ;
#47947=B_SPLINE_CURVE_WITH_KNOTS ( 'NONE', 3,
 ( #65764, #78392, #32001, #72980, #80188, #64874, #66215, #10838, #37407, #59467 ),
 .UNSPECIFIED., .F., .F.,
 ( 4, 2, 2, 2, 4 ),
 ( 0.0007817359430256327164, 0.0009771253907249993591, 0.001172514838424366110, 0.001367904286123732861, 0.001563293733823099396 ),
 .UNSPECIFIED. ) ;
#47948=CARTESIAN_POINT ( 'NONE',  ( -13.44988538517170618, -2.657715359629089225, 31.77849191805832874 ) ) ;
#47949=EDGE_LOOP ( 'NONE', ( #8545, #37428, #57696, #70995 ) ) ;
#47950=VECTOR ( 'NONE', #88217, 1000.000000000000114 ) ;
#47951=AXIS2_PLACEMENT_3D ( 'NONE', #15064, #82646, #88526 ) ;
#47952=ORIENTED_EDGE ( 'NONE', *, *, #65637, .F. ) ;
#47953=ORIENTED_EDGE ( 'NONE', *, *, #40772, .F. ) ;
#47954=VERTEX_POINT ( 'NONE', #65448 ) ;
#47956=CARTESIAN_POINT ( 'NONE',  ( 17.14299041027315695, -9.905515769479276145, 34.41647553114623292 ) ) ;
#47957=CARTESIAN_POINT ( 'NONE',  ( 7.846153846153846700, -3.513871655860378418, 32.76840700105978499 ) ) ;
#47958=CARTESIAN_POINT ( 'NONE',  ( 4.376858997939548246, -11.98016756924215009, 32.48728574198911190 ) ) ;
#47959=CARTESIAN_POINT ( 'NONE',  ( 14.17708265248822386, -7.722926974430166069, 34.99546784045485737 ) ) ;
#47961=CARTESIAN_POINT ( 'NONE',  ( -9.692307692307691624, -11.91647553114624181, 32.58852847137148245 ) ) ;
#47962=ORIENTED_EDGE ( 'NONE', *, *, #54184, .T. ) ;
#47963=ORIENTED_EDGE ( 'NONE', *, *, #54929, .T. ) ;
#47964=VERTEX_POINT ( 'NONE', #19482 ) ;
#47965=CARTESIAN_POINT ( 'NONE',  ( -9.692307692307691624, -1.044019251281081972, 31.83374038241031911 ) ) ;
#47966=ORIENTED_EDGE ( 'NONE', *, *, #15736, .F. ) ;
#47967=CARTESIAN_POINT ( 'NONE',  ( 9.626225312947561008, -8.164416787775445883, 34.95778746994557906 ) ) ;
#47971=EDGE_LOOP ( 'NONE', ( #62531, #31570 ) ) ;
#47973=ORIENTED_EDGE ( 'NONE', *, *, #69326, .F. ) ;
#47974=CARTESIAN_POINT ( 'NONE',  ( 7.976679547917411739, -12.27024696741798948, 31.24895572276498257 ) ) ;
#47975=EDGE_CURVE ( 'NONE', #47786, #17409, #61165, .T. ) ;
#47976=FACE_BOUND ( 'NONE', #72069, .T. ) ;
#47977=CARTESIAN_POINT ( 'NONE',  ( 17.07692307692307665, -8.564572088678739092, 35.78748833219616898 ) ) ;
#47979=EDGE_CURVE ( 'NONE', #26836, #48528, #72986, .T. ) ;
#47980=CARTESIAN_POINT ( 'NONE',  ( 1.384615384615264011, -2.379036618888197285, 30.90682066428292885 ) ) ;
#47981=ORIENTED_EDGE ( 'NONE', *, *, #35752, .F. ) ;
#47982=CARTESIAN_POINT ( 'NONE',  ( 8.639082799499076870, -12.15440758774515473, 32.17923288041532004 ) ) ;
#47983=CARTESIAN_POINT ( 'NONE',  ( 6.700149964170075023, -11.98009711892699691, 32.48740034544075428 ) ) ;
#47984=CARTESIAN_POINT ( 'NONE',  ( -13.13461538461394973, -7.500000000000155431, 34.75000000000007105 ) ) ;
#47985=CARTESIAN_POINT ( 'NONE',  ( -3.361459833879538728, -9.084618155246140248, 34.75535874321725771 ) ) ;
#47986=ORIENTED_EDGE ( 'NONE', *, *, #36274, .F. ) ;
#47987=CARTESIAN_POINT ( 'NONE',  ( -12.46153846153858424, -2.379036618888197729, 30.90682066428292885 ) ) ;
#47988=CARTESIAN_POINT ( 'NONE',  ( 1.384615384615264011, -4.320704448113951379, 33.92786785259630022 ) ) ;
#47989=CARTESIAN_POINT ( 'NONE',  ( -16.40384615384615330, -2.249999999999998668, 29.75000000000000355 ) ) ;
#47990=CARTESIAN_POINT ( 'NONE',  ( -2.557669038634660108, -10.66389620160130036, 33.62221079203477103 ) ) ;
#47991=CARTESIAN_POINT ( 'NONE',  ( -0.3314908552827783850, -7.723484964179500700, 34.74522123443823318 ) ) ;
#47992=FACE_BOUND ( 'NONE', #10331, .T. ) ;
#47993=CARTESIAN_POINT ( 'NONE',  ( 1.134615384615387246, -7.500000000000001776, 35.00000000000000000 ) ) ;
#47994=CARTESIAN_POINT ( 'NONE',  ( 11.47319109250076430, -12.46129190929999986, 30.37095296980880832 ) ) ;
#47995=CARTESIAN_POINT ( 'NONE',  ( -14.55771553191376277, -3.520140089381495585, 33.17453946501458262 ) ) ;
#47996=CARTESIAN_POINT ( 'NONE',  ( -5.999999999999998224, -8.564572088678739092, 35.78748833219616898 ) ) ;
#47997=CARTESIAN_POINT ( 'NONE',  ( -2.084679463598911653, -8.282913670948747864, 34.94150082978203642 ) ) ;
#47998=CARTESIAN_POINT ( 'NONE',  ( -5.207071046654774271, -12.50552854090298993, 31.33409797877408920 ) ) ;
#48000=ORIENTED_EDGE ( 'NONE', *, *, #6361, .F. ) ;
#48001=B_SPLINE_CURVE_WITH_KNOTS ( 'NONE', 3,
 ( #66626, #45896, #11688, #13890, #70165, #75585, #43141, #8474, #7140, #21983 ),
 .UNSPECIFIED., .F., .F.,
 ( 4, 2, 2, 2, 4 ),
 ( 0.0007817359430256308733, 0.0009771253907249971907, 0.001172514838424363725, 0.001367904286123730259, 0.001563293733823096577 ),
 .UNSPECIFIED. ) ;
#48002=CARTESIAN_POINT ( 'NONE',  ( 12.71148397988660328, -2.587454068350148351, 30.68340429815432202 ) ) ;
#48003=EDGE_LOOP ( 'NONE', ( #7484, #44397, #38049, #52841 ) ) ;
#48004=B_SPLINE_CURVE_WITH_KNOTS ( 'NONE', 3,
 ( #34912, #62376, #689, #28157, #55625, #83115, #21407, #48873, #42136, #7895 ),
 .UNSPECIFIED., .F., .F.,
 ( 4, 2, 2, 2, 4 ),
 ( 0.0007817246256747520513, 0.0009771112852218959231, 0.001172497944769039903, 0.001367884604316183883, 0.001563271263863327864 ),
 .UNSPECIFIED. ) ;
#48005=CARTESIAN_POINT ( 'NONE',  ( -13.31854805126531005, -9.058645607665452459, 34.76329471203371924 ) ) ;
#48006=VERTEX_POINT ( 'NONE', #51921 ) ;
#48007=CARTESIAN_POINT ( 'NONE',  ( -12.46153846153846168, -8.564572088678739092, 35.78748833219616898 ) ) ;
#48008=CARTESIAN_POINT ( 'NONE',  ( 14.30769230769218581, -4.320704448113951379, 33.92786785259630022 ) ) ;
#48009=CYLINDRICAL_SURFACE ( 'NONE', #38062, 0.2500000000000012212 ) ;
#48011=CARTESIAN_POINT ( 'NONE',  ( 18.00000000000000000, -5.471508081941601098, 34.59228464037088457 ) ) ;
#48013=DIRECTION ( 'NONE',  ( 0.000000000000000000, 0.7660444431189822323, -0.6427876096865344779 ) ) ;
#48015=VECTOR ( 'NONE', #52849, 1000.000000000000227 ) ;
#48016=CARTESIAN_POINT ( 'NONE',  ( 17.01083966596719677, -12.37446782046654192, 30.86335684631486487 ) ) ;
#48018=CARTESIAN_POINT ( 'NONE',  ( 2.307692307692187583, -2.892918686052166066, 31.69288490824153470 ) ) ;
#48019=LINE ( 'NONE', #14690, #8028 ) ;
#48021=EDGE_CURVE ( 'NONE', #65186, #54833, #25353, .T. ) ;
#48022=CARTESIAN_POINT ( 'NONE',  ( 11.53846153846153832, -1.509761064869970415, 31.06009739812519044 ) ) ;
#48023=CARTESIAN_POINT ( 'NONE',  ( -4.153846153846274980, -3.083524468854526912, 32.58852847137268327 ) ) ;
#48024=VERTEX_POINT ( 'NONE', #17717 ) ;
#48027=CARTESIAN_POINT ( 'NONE',  ( 2.177001704582000485, -4.684245665217971144, 34.18127051446801090 ) ) ;
#48030=CARTESIAN_POINT ( 'NONE',  ( -17.74994568836168085, -2.779044189368095275, 31.39831045268884324 ) ) ;
#48031=CARTESIAN_POINT ( 'NONE',  ( -14.55766903863466055, -11.28823185664190376, 33.01397839955799896 ) ) ;
#48032=DIRECTION ( 'NONE',  ( -0.000000000000000000, -0.6427876096865404731, -0.7660444431189771253 ) ) ;
#48033=VERTEX_POINT ( 'NONE', #31670 ) ;
#48034=CARTESIAN_POINT ( 'NONE',  ( 6.673076923076925127, -2.499999999999998668, 29.75000000000000355 ) ) ;
#48035=CARTESIAN_POINT ( 'NONE',  ( -15.16551409125639083, -12.16647553114626490, 32.15551576947920864 ) ) ;
#48036=EDGE_CURVE ( 'NONE', #31874, #69663, #77289, .T. ) ;
#48037=CARTESIAN_POINT ( 'NONE',  ( 15.93091993633000136, -9.086856451489516928, 34.49173150075333183 ) ) ;
#48038=CARTESIAN_POINT ( 'NONE',  ( 3.100078627658925612, -2.494641256782728966, 31.33461815524612959 ) ) ;
#48042=ORIENTED_EDGE ( 'NONE', *, *, #53224, .T. ) ;
#48043=ORIENTED_EDGE ( 'NONE', *, *, #47633, .F. ) ;
#48044=AXIS2_PLACEMENT_3D ( 'NONE', #10758, #60719, #66136 ) ;
#48045=EDGE_CURVE ( 'NONE', #36328, #43306, #64338, .T. ) ;
#48046=DIRECTION ( 'NONE',  ( 0.000000000000000000, 1.000000000000000000, 0.000000000000000000 ) ) ;
#48047=CARTESIAN_POINT ( 'NONE',  ( 0.2380535178145129771, -2.599994579823202923, 30.74605699353653776 ) ) ;
#48048=EDGE_CURVE ( 'NONE', #62255, #64011, #82965, .T. ) ;
#48051=CARTESIAN_POINT ( 'NONE',  ( 5.076923076923075762, -5.557115091759785130, 34.35708131394839171 ) ) ;
#48053=ORIENTED_EDGE ( 'NONE', *, *, #20665, .F. ) ;
#48054=EDGE_CURVE ( 'NONE', #27738, #221, #48722, .T. ) ;
#48055=ORIENTED_EDGE ( 'NONE', *, *, #85615, .F. ) ;
#48056=CARTESIAN_POINT ( 'NONE',  ( -18.00000000000000000, -13.02631839243208667, 34.71348354719103924 ) ) ;
#48057=ORIENTED_EDGE ( 'NONE', *, *, #7616, .F. ) ;
#48060=EDGE_CURVE ( 'NONE', #64638, #57873, #21247, .T. ) ;
#48063=ADVANCED_FACE ( 'NONE', ( #68554 ), #101, .F. ) ;
#48064=ORIENTED_EDGE ( 'NONE', *, *, #73926, .F. ) ;
#48065=VERTEX_POINT ( 'NONE', #76193 ) ;
#48066=B_SPLINE_CURVE_WITH_KNOTS ( 'NONE', 3,
 ( #22692, #23137, #84857, #42534, #77638, #43418, #70890, #2411, #50604, #29906 ),
 .UNSPECIFIED., .F., .F.,
 ( 4, 2, 2, 2, 4 ),
 ( 0.000000000000000000, 0.0001954311564186861697, 0.0003908623128373723394, 0.0005862934692560584820, 0.0007817246256747446788 ),
 .UNSPECIFIED. ) ;
#48067=CIRCLE ( 'NONE', #46666, 2.000000000000001776 ) ;
#48068=EDGE_LOOP ( 'NONE', ( #2840, #881 ) ) ;
#48070=CARTESIAN_POINT ( 'NONE',  ( 7.846153846153846700, -2.538708090699994813, 30.37095296980875503 ) ) ;
#48071=ORIENTED_EDGE ( 'NONE', *, *, #43070, .T. ) ;
#48072=CARTESIAN_POINT ( 'NONE',  ( 6.923076923076802558, -6.879047030192662504, 34.71129190930017927 ) ) ;
#48073=B_SPLINE_CURVE_WITH_KNOTS ( 'NONE', 3,
 ( #64407, #77938, #69416, #15363, #28426, #43273, #14923, #36081, #55892, #28887 ),
 .UNSPECIFIED., .F., .F.,
 ( 4, 2, 2, 2, 4 ),
 ( 0.0007817246256747459798, 0.0009771112852218887673, 0.001172497944769031663, 0.001367884604316174559, 0.001563271263863317455 ),
 .UNSPECIFIED. ) ;
#48074=LINE ( 'NONE', #783, #47950 ) ;
#48075=EDGE_CURVE ( 'NONE', #65429, #79653, #75322, .T. ) ;
#48076=VERTEX_POINT ( 'NONE', #67676 ) ;
#48079=VERTEX_POINT ( 'NONE', #13614 ) ;
#48080=FACE_BOUND ( 'NONE', #39469, .T. ) ;
#48081=CARTESIAN_POINT ( 'NONE',  ( 10.74617642320940369, -9.804649428959608670, 34.18742332936588468 ) ) ;
#48083=CARTESIAN_POINT ( 'NONE',  ( -0.4615384615384611200, -11.35647404775217417, 33.31231777344666511 ) ) ;
#48084=CARTESIAN_POINT ( 'NONE',  ( 9.626224281351813516, -3.050289026998445951, 32.03036669348365706 ) ) ;
#48085=CARTESIAN_POINT ( 'NONE',  ( -0.5276218724943415594, -12.10708131394839349, 31.69288490824020244 ) ) ;
#48087=CARTESIAN_POINT ( 'NONE',  ( -3.007756386675835447, -3.395485233115138168, 33.02377354290276656 ) ) ;
#48088=CARTESIAN_POINT ( 'NONE',  ( -3.931066484868087851, -11.60474049983371003, 33.02348890104160262 ) ) ;
#48089=ORIENTED_EDGE ( 'NONE', *, *, #24855, .F. ) ;
#48090=EDGE_CURVE ( 'NONE', #31586, #71975, #50057, .T. ) ;
#48091=CARTESIAN_POINT ( 'NONE',  ( -8.069638770718176701, -6.716662450894489211, 34.94144148231605840 ) ) ;
#48093=VERTEX_POINT ( 'NONE', #20812 ) ;
#48094=DIRECTION ( 'NONE',  ( 0.000000000000000000, 0.8660254037844377084, 0.5000000000000015543 ) ) ;
#48095=LINE ( 'NONE', #62490, #83566 ) ;
#48096=VERTEX_POINT ( 'NONE', #40213 ) ;
#48097=CYLINDRICAL_SURFACE ( 'NONE', #44252, 0.2500000000000009437 ) ;
#48098=CARTESIAN_POINT ( 'NONE',  ( -4.219116154402471786, -2.379036618887870436, 30.90682066428147934 ) ) ;
#48100=FACE_BOUND ( 'NONE', #43480, .T. ) ;
#48101=CARTESIAN_POINT ( 'NONE',  ( -14.55766905174089665, -4.075325502946081535, 33.72974371597206300 ) ) ;
#48102=CARTESIAN_POINT ( 'NONE',  ( 15.45378058238208219, -12.15243808032445827, 31.58219941686247978 ) ) ;
#48103=CARTESIAN_POINT ( 'NONE',  ( 2.177001704582002262, -6.369640206132550553, 34.87707690430378449 ) ) ;
#48104=CARTESIAN_POINT ( 'NONE',  ( -2.307692307692305711, -3.669653830205710676, 35.88435417666054406 ) ) ;
#48106=CARTESIAN_POINT ( 'NONE',  ( -8.638705067467203236, -12.27024696741798948, 31.24895572276497546 ) ) ;
#48109=VERTEX_POINT ( 'NONE', #48278 ) ;
#48111=ORIENTED_EDGE ( 'NONE', *, *, #65566, .F. ) ;
#48112=VECTOR ( 'NONE', #37938, 999.9999999999998863 ) ;
#48113=B_SPLINE_CURVE_WITH_KNOTS ( 'NONE', 3,
 ( #79165, #57998, #43598, #44921, #59332, #72397, #86389, #17912, #86840, #52569 ),
 .UNSPECIFIED., .F., .F.,
 ( 4, 2, 2, 2, 4 ),
 ( 0.0007817246256747473893, 0.0009771112852218900684, 0.001172497944769032747, 0.001367884604316175427, 0.001563271263863318106 ),
 .UNSPECIFIED. ) ;
#48114=CARTESIAN_POINT ( 'NONE',  ( 15.90386940979756858, -9.234221910056350069, 34.70572697212741531 ) ) ;
#48115=CARTESIAN_POINT ( 'NONE',  ( -15.36145983387953962, -5.496505350115501010, 34.60290016733514307 ) ) ;
#48116=CARTESIAN_POINT ( 'NONE',  ( 14.30769230769218581, -9.528491918059723176, 34.59228464037033035 ) ) ;
#48117=CARTESIAN_POINT ( 'NONE',  ( 6.700150705560775855, -12.15238873228292071, 31.58232369045353849 ) ) ;
#48118=CARTESIAN_POINT ( 'NONE',  ( 5.142178216435913107, -3.643525952247864463, 33.31231777344670064 ) ) ;
#48120=CARTESIAN_POINT ( 'NONE',  ( -7.846153846153965716, -2.625532179533778709, 30.86335684631627174 ) ) ;
#48121=CARTESIAN_POINT ( 'NONE',  ( -6.130147969731693181, -8.630895178749536711, 34.87696386517710323 ) ) ;
#48122=CARTESIAN_POINT ( 'NONE',  ( 9.692307692307695177, -10.67929555188718282, 33.92786785259544047 ) ) ;
#48124=CARTESIAN_POINT ( 'NONE',  ( -15.23076923076935074, -11.48612834414049644, 32.76840700105863391 ) ) ;
#48125=CARTESIAN_POINT ( 'NONE',  ( 16.21910172512217585, -5.219633306516380244, 34.19971097300157936 ) ) ;
#48126=CARTESIAN_POINT ( 'NONE',  ( 5.749976762707035505, -12.22074536777954989, 31.39888409691088356 ) ) ;
#48127=EDGE_CURVE ( 'NONE', #18188, #5178, #55923, .T. ) ;
#48128=CARTESIAN_POINT ( 'NONE',  ( -3.360916440207451839, -8.587444163452046197, 34.63053765926554206 ) ) ;
#48129=CARTESIAN_POINT ( 'NONE',  ( 12.59206416330202494, -2.882268652242222284, 31.66798894389554064 ) ) ;
#48131=EDGE_CURVE ( 'NONE', #67886, #18976, #75749, .T. ) ;
#48132=CARTESIAN_POINT ( 'NONE',  ( 2.084207383127978375, -3.562934362175799841, 33.22335522853832401 ) ) ;
#48133=EDGE_CURVE ( 'NONE', #47148, #24566, #41532, .T. ) ;
#48137=CARTESIAN_POINT ( 'NONE',  ( -9.822998295417999515, -10.70098750199973203, 33.91152734681376302 ) ) ;
#48138=CARTESIAN_POINT ( 'NONE',  ( 15.23076923076923173, -13.87047571288749737, 32.06866353760679544 ) ) ;
#48139=DIRECTION ( 'NONE',  ( 0.000000000000000000, 0.8660254037844377084, -0.5000000000000015543 ) ) ;
#48140=CARTESIAN_POINT ( 'NONE',  ( -1.134561072977068985, -4.235687564193446164, 33.53795663066793509 ) ) ;
#48141=ORIENTED_EDGE ( 'NONE', *, *, #40597, .F. ) ;
#48143=CARTESIAN_POINT ( 'NONE',  ( -9.561782254074046250, -5.915461855592780260, 34.75538340440931506 ) ) ;
#48144=ORIENTED_EDGE ( 'NONE', *, *, #27521, .T. ) ;
#48145=CARTESIAN_POINT ( 'NONE',  ( -16.08777780284371417, -9.780366693483667717, 34.19971097300155805 ) ) ;
#48146=EDGE_CURVE ( 'NONE', #64222, #76630, #88855, .T. ) ;
#48147=VECTOR ( 'NONE', #18569, 1000.000000000000000 ) ;
#48148=CARTESIAN_POINT ( 'NONE',  ( 7.911299625485813891, -7.750023238201979581, 34.74374492549440419 ) ) ;
#48150=CARTESIAN_POINT ( 'NONE',  ( -7.846153846153844924, -6.343179335718451384, 34.87096338111211935 ) ) ;
#48151=CARTESIAN_POINT ( 'NONE',  ( -15.48076923076922995, -7.433932668274256805, 35.00000000000000711 ) ) ;
#48152=CARTESIAN_POINT ( 'NONE',  ( -14.98082371242109012, -12.43552623307873972, 30.55307653245132826 ) ) ;
#48153=ORIENTED_EDGE ( 'NONE', *, *, #66914, .F. ) ;
#48154=VERTEX_POINT ( 'NONE', #74884 ) ;
#48155=LINE ( 'NONE', #32101, #44133 ) ;
#48156=B_SPLINE_CURVE_WITH_KNOTS ( 'NONE', 3,
 ( #22768, #77718, #16026, #61002, #74085, #5176, #38975, #38521, #11045, #60557 ),
 .UNSPECIFIED., .F., .F.,
 ( 4, 2, 2, 2, 4 ),
 ( 0.000000000000000000, 0.0001954339857564076099, 0.0003908679715128152198, 0.0005863019572692228839, 0.0007817359430256304396 ),
 .UNSPECIFIED. ) ;
#48157=VERTEX_POINT ( 'NONE', #6424 ) ;
#48158=CARTESIAN_POINT ( 'NONE',  ( -7.846153846153844924, -2.292212530054420494, 30.41441678777542634 ) ) ;
#48159=CARTESIAN_POINT ( 'NONE',  ( 5.326868486301119532, -4.932303261841489039, 34.32971442181322885 ) ) ;
#48160=CARTESIAN_POINT ( 'NONE',  ( -10.74553182482283198, -2.619462340734462380, 30.83744416345203021 ) ) ;
#48163=EDGE_CURVE ( 'NONE', #40118, #85711, #28975, .T. ) ;
#48164=CARTESIAN_POINT ( 'NONE',  ( 1.384615384615386802, -2.292212530054420494, 30.41441678777542634 ) ) ;
#48166=ORIENTED_EDGE ( 'NONE', *, *, #3444, .F. ) ;
#48167=ORIENTED_EDGE ( 'NONE', *, *, #16817, .T. ) ;
#48168=LINE ( 'NONE', #47286, #64513 ) ;
#48169=VERTEX_POINT ( 'NONE', #50050 ) ;
#48170=CARTESIAN_POINT ( 'NONE',  ( 7.716005876422147303, -2.647304123082328875, 31.75400227202885972 ) ) ;
#48171=VECTOR ( 'NONE', #35061, 1000.000000000000000 ) ;
#48172=ORIENTED_EDGE ( 'NONE', *, *, #17347, .T. ) ;
#48173=B_SPLINE_CURVE_WITH_KNOTS ( 'NONE', 3,
 ( #10764, #36897, #3106, #57176, #72013, #77448, #49968, #10321, #31477, #37786 ),
 .UNSPECIFIED., .F., .F.,
 ( 4, 2, 2, 2, 4 ),
 ( 0.0007817359430256390048, 0.0009771253907250075990, 0.001172514838424376085, 0.001367904286123744571, 0.001563293733823113056 ),
 .UNSPECIFIED. ) ;
#48174=DIRECTION ( 'NONE',  ( -0.000000000000000000, -0.7660444431189791237, -0.6427876096865379196 ) ) ;
#48175=CARTESIAN_POINT ( 'NONE',  ( 12.59233026936324684, -3.062576670634119758, 32.05464942895959979 ) ) ;
#48176=CIRCLE ( 'NONE', #38153, 0.2500000000000002220 ) ;
#48177=ORIENTED_EDGE ( 'NONE', *, *, #34021, .F. ) ;
#48178=CARTESIAN_POINT ( 'NONE',  ( 7.846153846153846700, -8.120952969808772792, 34.71129190930000163 ) ) ;
#48179=B_SPLINE_CURVE_WITH_KNOTS ( 'NONE', 3,
 ( #78663, #84989, #16966, #24156, #3442, #71023, #30475, #65582, #30909, #23272 ),
 .UNSPECIFIED., .F., .F.,
 ( 4, 2, 2, 2, 4 ),
 ( 0.000000000000000000, 0.0001954311564186879857, 0.0003908623128373759715, 0.0005862934692560640114, 0.0007817246256747519429 ),
 .UNSPECIFIED. ) ;
#48180=ORIENTED_EDGE ( 'NONE', *, *, #19530, .F. ) ;
#48182=B_SPLINE_CURVE_WITH_KNOTS ( 'NONE', 3,
 ( #30044, #44871, #72349, #24158, #64697, #86340, #2996, #57063, #30478, #77779 ),
 .UNSPECIFIED., .F., .F.,
 ( 4, 2, 2, 2, 4 ),
 ( 0.000000000000000000, 0.0001954311564186881213, 0.0003908623128373762425, 0.0005862934692560643367, 0.0007817246256747524850 ),
 .UNSPECIFIED. ) ;
#48184=CARTESIAN_POINT ( 'NONE',  ( -12.59222906464877134, -3.338472653186243644, 32.95098750199972670 ) ) ;
#48186=ORIENTED_EDGE ( 'NONE', *, *, #83418, .F. ) ;
#48187=EDGE_CURVE ( 'NONE', #19974, #61584, #45055, .T. ) ;
#48188=CARTESIAN_POINT ( 'NONE',  ( -16.40382288478850725, -6.567427716900048118, 34.66269422305636283 ) ) ;
#48189=CARTESIAN_POINT ( 'NONE',  ( 12.46153846153833911, -2.379036618888197729, 30.90682066428292885 ) ) ;
#48190=FACE_BOUND ( 'NONE', #73898, .T. ) ;
#48191=LINE ( 'NONE', #20292, #49928 ) ;
#48192=CARTESIAN_POINT ( 'NONE',  ( -17.74994568836169151, -12.17597550085003633, 31.52189283813461884 ) ) ;
#48193=EDGE_CURVE ( 'NONE', #35118, #49988, #16038, .T. ) ;
#48194=CARTESIAN_POINT ( 'NONE',  ( 4.376625695114563008, -12.44528174975671853, 30.48912976160716681 ) ) ;
#48195=CARTESIAN_POINT ( 'NONE',  ( 1.254467414883688070, -12.50552854090298993, 31.33409797877408920 ) ) ;
#48196=CARTESIAN_POINT ( 'NONE',  ( -17.20761368003338632, -8.191372820521381826, 34.95448215188424967 ) ) ;
#48197=CARTESIAN_POINT ( 'NONE',  ( -7.846153846153844924, -9.058645607665452459, 34.76329471203371924 ) ) ;
#48198=EDGE_CURVE ( 'NONE', #42793, #25852, #34377, .T. ) ;
#48199=CARTESIAN_POINT ( 'NONE',  ( 10.48523740594639619, -10.19110544564092002, 33.96427741523702792 ) ) ;
#48200=EDGE_LOOP ( 'NONE', ( #75388, #38127, #4244, #86294 ) ) ;
#48201=VERTEX_POINT ( 'NONE', #84309 ) ;
#48202=CARTESIAN_POINT ( 'NONE',  ( -16.82686876528476105, -9.943054286541403997, 34.11300777759954883 ) ) ;
#48203=CARTESIAN_POINT ( 'NONE',  ( -3.480792454990687013, -5.765609946408404518, 34.70566812827425451 ) ) ;
#48205=CARTESIAN_POINT ( 'NONE',  ( -9.469294848214296678, -12.38742843783360748, 31.66772728687926985 ) ) ;
#48206=LINE ( 'NONE', #43228, #13503 ) ;
#48207=CARTESIAN_POINT ( 'NONE',  ( 15.48071474911737333, -3.712312575010499494, 33.01462480002815170 ) ) ;
#48208=CARTESIAN_POINT ( 'NONE',  ( -7.846153846153844924, -8.810774026931790459, 35.74407628777942847 ) ) ;
#48210=CARTESIAN_POINT ( 'NONE',  ( 2.307692307692187583, -9.442884908241554243, 34.35708131394783038 ) ) ;
#48211=DIRECTION ( 'NONE',  ( -0.000000000000000000, 0.6427876096865404731, -0.7660444431189771253 ) ) ;
#48212=CARTESIAN_POINT ( 'NONE',  ( -9.019254006523736322, -12.22074536777954989, 31.39888409691088356 ) ) ;
#48214=ORIENTED_EDGE ( 'NONE', *, *, #72290, .T. ) ;
#48215=EDGE_CURVE ( 'NONE', #82729, #39385, #36551, .T. ) ;
#48216=ORIENTED_EDGE ( 'NONE', *, *, #20027, .T. ) ;
#48217=ORIENTED_EDGE ( 'NONE', *, *, #69265, .T. ) ;
#48218=DIRECTION ( 'NONE',  ( -0.000000000000000000, 0.9848077530122085754, -0.1736481776669273613 ) ) ;
#48220=EDGE_LOOP ( 'NONE', ( #45716, #5868, #23555, #28607 ) ) ;
#48221=CARTESIAN_POINT ( 'NONE',  ( -9.915233909823838232, -12.39988816332205701, 30.74660775122750778 ) ) ;
#48222=CARTESIAN_POINT ( 'NONE',  ( -17.32689980786543060, -3.137211980971222225, 32.19342716148376837 ) ) ;
#48223=CARTESIAN_POINT ( 'NONE',  ( -5.076923076923075762, -4.098570777380720287, 33.41473453929634729 ) ) ;
#48225=CARTESIAN_POINT ( 'NONE',  ( -11.31568199719312773, -6.760870238392817200, 34.69528174975672385 ) ) ;
#48226=ORIENTED_EDGE ( 'NONE', *, *, #67985, .F. ) ;
#48228=FACE_OUTER_BOUND ( 'NONE', #59990, .T. ) ;
#48229=EDGE_LOOP ( 'NONE', ( #33975, #42894, #66222, #49848 ) ) ;
#48231=FACE_OUTER_BOUND ( 'NONE', #38176, .T. ) ;
#48232=CARTESIAN_POINT ( 'NONE',  ( 3.230769230769231726, -10.05456864172156806, 36.03766855953608683 ) ) ;
#48234=EDGE_CURVE ( 'NONE', #44313, #75481, #87055, .T. ) ;
#48236=VECTOR ( 'NONE', #88351, 999.9999999999998863 ) ;
#48237=CARTESIAN_POINT ( 'NONE',  ( 17.14206885625503674, -7.750023238201980469, 34.74374492549440419 ) ) ;
#48238=CARTESIAN_POINT ( 'NONE',  ( 12.52760681254089725, -11.16473453929635440, 33.15142922261926373 ) ) ;
#48240=ORIENTED_EDGE ( 'NONE', *, *, #13081, .T. ) ;
#48241=EDGE_CURVE ( 'NONE', #14268, #61355, #50480, .T. ) ;
#48242=CARTESIAN_POINT ( 'NONE',  ( 13.38461538461538680, -13.53365097954675988, 30.81389545987213552 ) ) ;
#48243=CARTESIAN_POINT ( 'NONE',  ( 0.5276068125408990284, -3.050289026998446840, 32.03036669348366416 ) ) ;
#48244=FACE_OUTER_BOUND ( 'NONE', #18659, .T. ) ;
#48247=LINE ( 'NONE', #53680, #36907 ) ;
#48248=DIRECTION ( 'NONE',  ( -0.000000000000000000, -0.9396926207859093161, -0.3420201433256663259 ) ) ;
#48249=B_SPLINE_CURVE_WITH_KNOTS ( 'NONE', 3,
 ( #41669, #27261, #61923, #236, #33585, #33131, #48410, #13304, #6991, #34462 ),
 .UNSPECIFIED., .F., .F.,
 ( 4, 2, 2, 2, 4 ),
 ( 0.0007817246256747485819, 0.0009771112852218918031, 0.001172497944769034916, 0.001367884604316178029, 0.001563271263863321358 ),
 .UNSPECIFIED. ) ;
#48250=B_SPLINE_CURVE_WITH_KNOTS ( 'NONE', 3,
 ( #17744, #45197, #4673, #32146, #72675, #51047, #65910, #38909, #4220, #52396 ),
 .UNSPECIFIED., .F., .F.,
 ( 4, 2, 2, 2, 4 ),
 ( 0.000000000000000000, 0.0001954311564186863594, 0.0003908623128373727188, 0.0005862934692560590241, 0.0007817246256747454377 ),
 .UNSPECIFIED. ) ;
#48251=CARTESIAN_POINT ( 'NONE',  ( -8.992157728137614825, -10.77366814457252175, 33.85459836347579454 ) ) ;
#48252=ADVANCED_FACE ( 'NONE', ( #79757 ), #51348, .F. ) ;
#48253=CYLINDRICAL_SURFACE ( 'NONE', #81687, 0.2500000000000008882 ) ;
#48254=CARTESIAN_POINT ( 'NONE',  ( -17.07692307692307665, -2.292212530054420494, 30.41441678777542634 ) ) ;
#48255=ORIENTED_EDGE ( 'NONE', *, *, #69309, .T. ) ;
#48256=LINE ( 'NONE', #56353, #20390 ) ;
#48257=EDGE_CURVE ( 'NONE', #14427, #30672, #14928, .T. ) ;
#48258=CYLINDRICAL_SURFACE ( 'NONE', #42656, 0.2499999999999986955 ) ;
#48259=CARTESIAN_POINT ( 'NONE',  ( -15.23076923076922995, -3.886160181151819604, 36.00935417666054406 ) ) ;
#48260=ORIENTED_EDGE ( 'NONE', *, *, #76997, .F. ) ;
#48261=FACE_OUTER_BOUND ( 'NONE', #31866, .T. ) ;
#48262=EDGE_LOOP ( 'NONE', ( #53286, #16491 ) ) ;
#48264=CARTESIAN_POINT ( 'NONE',  ( 11.53846153846153832, -6.343179335718451384, 34.87096338111211935 ) ) ;
#48266=ORIENTED_EDGE ( 'NONE', *, *, #6475, .T. ) ;
#48268=DIRECTION ( 'NONE',  ( -0.000000000000000000, -0.000000000000000000, -1.000000000000000000 ) ) ;
#48269=ADVANCED_FACE ( 'NONE', ( #31562 ), #72098, .F. ) ;
#48270=CARTESIAN_POINT ( 'NONE',  ( -1.384615384615505151, -10.21337939537710326, 33.94971097300076224 ) ) ;
#48271=AXIS2_PLACEMENT_3D ( 'NONE', #65971, #32637, #51105 ) ;
#48272=EDGE_CURVE ( 'NONE', #61398, #10299, #50300, .T. ) ;
#48273=CARTESIAN_POINT ( 'NONE',  ( 7.145856592054990131, -12.47679350104403007, 31.42216943046555855 ) ) ;
#48275=ORIENTED_EDGE ( 'NONE', *, *, #54939, .T. ) ;
#48276=FACE_BOUND ( 'NONE', #81613, .T. ) ;
#48278=CARTESIAN_POINT ( 'NONE',  ( 9.692307692307695177, -9.905515769479276145, 34.41647553114623292 ) ) ;
#48279=B_SPLINE_CURVE_WITH_KNOTS ( 'NONE', 3,
 ( #85527, #58475, #73802, #23803, #39580, #45862, #12103, #4897, #51255, #24249 ),
 .UNSPECIFIED., .F., .F.,
 ( 4, 2, 2, 2, 4 ),
 ( 0.0007817359430256262112, 0.0009771253907249911191, 0.001172514838424356136, 0.001367904286123721152, 0.001563293733823086168 ),
 .UNSPECIFIED. ) ;
#48280=B_SPLINE_CURVE_WITH_KNOTS ( 'NONE', 3,
 ( #69435, #70321, #41081, #14942, #42420, #69877, #8184, #28912, #56365, #68546 ),
 .UNSPECIFIED., .F., .F.,
 ( 4, 2, 2, 2, 4 ),
 ( 0.000000000000000000, 0.0001954339857564098054, 0.0003908679715128196108, 0.0005863019572692293891, 0.0007817359430256392216 ),
 .UNSPECIFIED. ) ;
#48281=B_SPLINE_CURVE_WITH_KNOTS ( 'NONE', 3,
 ( #17574, #71609, #78816, #45475, #72502, #10812, #16670, #64850, #11255, #17117 ),
 .UNSPECIFIED., .F., .F.,
 ( 4, 2, 2, 2, 4 ),
 ( 0.0007817359430256388964, 0.0009771253907250073822, 0.001172514838424375868, 0.001367904286123744571, 0.001563293733823113056 ),
 .UNSPECIFIED. ) ;
#48282=CARTESIAN_POINT ( 'NONE',  ( 18.00000000000000000, -6.343179335718451384, 34.87096338111211935 ) ) ;
#48283=CARTESIAN_POINT ( 'NONE',  ( 8.835299120233207404, -3.513871655860379306, 32.76840700105978499 ) ) ;
#48284=CYLINDRICAL_SURFACE ( 'NONE', #20858, 0.2499999999999979738 ) ;
#48285=VERTEX_POINT ( 'NONE', #52710 ) ;
#48286=ORIENTED_EDGE ( 'NONE', *, *, #6509, .F. ) ;
#48287=EDGE_LOOP ( 'NONE', ( #33392, #58289 ) ) ;
#48288=CARTESIAN_POINT ( 'NONE',  ( 13.44976116394735222, -7.750023238201979581, 34.74374492549440419 ) ) ;
#48289=ORIENTED_EDGE ( 'NONE', *, *, #51590, .T. ) ;
#48290=AXIS2_PLACEMENT_3D ( 'NONE', #5441, #81104, #60371 ) ;
#48291=CARTESIAN_POINT ( 'NONE',  ( -17.32694630114453105, -10.18141759479407327, 34.26406193332782379 ) ) ;
#48292=CARTESIAN_POINT ( 'NONE',  ( 1.607394925883796732, -3.755027918224367767, 33.06320215134714857 ) ) ;
#48293=B_SPLINE_CURVE_WITH_KNOTS ( 'NONE', 3,
 ( #45144, #32085, #86604, #85259, #44689, #17233, #79388, #80280, #78485, #65854 ),
 .UNSPECIFIED., .F., .F.,
 ( 4, 2, 2, 2, 4 ),
 ( 0.000000000000000000, 0.0001954339857564078809, 0.0003908679715128157619, 0.0005863019572692236428, 0.0007817359430256315238 ),
 .UNSPECIFIED. ) ;
#48294=CARTESIAN_POINT ( 'NONE',  ( -18.25002323729296450, -11.37209801155882261, 32.91403422569033665 ) ) ;
#48295=CARTESIAN_POINT ( 'NONE',  ( 3.296836564119306701, -9.058645607665452459, 34.76329471203371924 ) ) ;
#48297=CARTESIAN_POINT ( 'NONE',  ( -4.284406067459515022, -2.254533558242299396, 29.97296025877828285 ) ) ;
#48298=CARTESIAN_POINT ( 'NONE',  ( 14.53047184896071542, -6.760870238392817200, 34.69528174975672385 ) ) ;
#48299=CARTESIAN_POINT ( 'NONE',  ( -5.010855743572999010, -11.35647404775217595, 33.31231777344667222 ) ) ;
#48300=ORIENTED_EDGE ( 'NONE', *, *, #6786, .T. ) ;
#48301=EDGE_CURVE ( 'NONE', #41851, #5737, #80656, .T. ) ;
#48302=VERTEX_POINT ( 'NONE', #18499 ) ;
#48303=EDGE_LOOP ( 'NONE', ( #1105, #9158 ) ) ;
#48304=DIRECTION ( 'NONE',  ( -0.000000000000000000, 0.3420201433256694901, -0.9396926207859082059 ) ) ;
#48306=CARTESIAN_POINT ( 'NONE',  ( 17.07692307692307665, -1.367168528481310208, 33.57946703557072254 ) ) ;
#48308=CARTESIAN_POINT ( 'NONE',  ( 8.769230769230768274, -5.180354513474913603, 36.12317359536750416 ) ) ;
#48309=CARTESIAN_POINT ( 'NONE',  ( -15.48079245499068435, -10.18141759479407327, 34.26406193332782379 ) ) ;
#48310=FACE_BOUND ( 'NONE', #71537, .T. ) ;
#48312=ORIENTED_EDGE ( 'NONE', *, *, #47592, .T. ) ;
#48313=DIRECTION ( 'NONE',  ( -0.000000000000000000, -0.7660444431189791237, -0.6427876096865379196 ) ) ;
#48314=CARTESIAN_POINT ( 'NONE',  ( -0.3310127597748971362, -9.417988943895561960, 34.36773134775778260 ) ) ;
#48315=CARTESIAN_POINT ( 'NONE',  ( -12.46153846153858424, -4.320704448113951379, 33.92786785259630022 ) ) ;
#48316=CARTESIAN_POINT ( 'NONE',  ( -3.454254155333560394, -3.562934362175799841, 33.22335522853832401 ) ) ;
#48318=EDGE_CURVE ( 'NONE', #16798, #22156, #82563, .T. ) ;
#48319=CARTESIAN_POINT ( 'NONE',  ( -18.24997673094235751, -8.303909089506435137, 34.68538101551103381 ) ) ;
#48321=FACE_BOUND ( 'NONE', #84290, .T. ) ;
#48322=CARTESIAN_POINT ( 'NONE',  ( -17.07692307692319744, -6.835583212225970762, 34.95778746994575670 ) ) ;
#48326=EDGE_LOOP ( 'NONE', ( #42904, #63803, #84721, #58720 ) ) ;
#48327=CARTESIAN_POINT ( 'NONE',  ( -12.71151519248081740, -9.943427161483782584, 34.11278801902876978 ) ) ;
#48328=CARTESIAN_POINT ( 'NONE',  ( -17.77722033102192967, -4.226511098958373402, 33.85474049983370293 ) ) ;
#48329=LINE ( 'NONE', #12338, #43768 ) ;
#48330=CARTESIAN_POINT ( 'NONE',  ( -4.854143407945009869, -5.827830569534416583, 34.72679350104403539 ) ) ;
#48331=ORIENTED_EDGE ( 'NONE', *, *, #38503, .F. ) ;
#48332=EDGE_CURVE ( 'NONE', #18497, #47795, #47128, .T. ) ;
#48333=CARTESIAN_POINT ( 'NONE',  ( -12.33101275977489841, -3.285477652293413264, 32.44071101563363158 ) ) ;
#48334=CARTESIAN_POINT ( 'NONE',  ( 4.087763774486017354, -9.905515769479276145, 34.41647553114623292 ) ) ;
#48335=CARTESIAN_POINT ( 'NONE',  ( -8.769230769230768274, -3.513871655860378418, 32.76840700105978499 ) ) ;
#48336=ORIENTED_EDGE ( 'NONE', *, *, #23867, .T. ) ;
#48337=LINE ( 'NONE', #34825, #28167 ) ;
#48339=CARTESIAN_POINT ( 'NONE',  ( -4.853911725310227077, -8.239487800360276282, 34.69522927552633718 ) ) ;
#48340=CARTESIAN_POINT ( 'NONE',  ( 14.24242186173153435, -9.442884908240170461, 34.35708131394840592 ) ) ;
#48341=DIRECTION ( 'NONE',  ( 1.000000000000000000, 0.000000000000000000, 0.000000000000000000 ) ) ;
#48342=CARTESIAN_POINT ( 'NONE',  ( -7.976301055592065481, -10.88202310037935661, 33.43294751532457099 ) ) ;
#48343=DIRECTION ( 'NONE',  ( -0.000000000000000000, 0.7660444431189791237, -0.6427876096865379196 ) ) ;
#48344=CARTESIAN_POINT ( 'NONE',  ( 14.05766907039934210, -3.711651800289232028, 33.01384336483936011 ) ) ;
#48346=ORIENTED_EDGE ( 'NONE', *, *, #10835, .T. ) ;
#48348=CARTESIAN_POINT ( 'NONE',  ( -17.77722045873158763, -9.332535724633405749, 34.40230450496446224 ) ) ;
#48349=ORIENTED_EDGE ( 'NONE', *, *, #66802, .T. ) ;
#48350=ORIENTED_EDGE ( 'NONE', *, *, #65921, .T. ) ;
#48351=EDGE_CURVE ( 'NONE', #3309, #29230, #48168, .T. ) ;
#48352=CARTESIAN_POINT ( 'NONE',  ( -8.519176349317314489, -6.523592122091592671, 34.90882529074906415 ) ) ;
#48353=ORIENTED_EDGE ( 'NONE', *, *, #33429, .F. ) ;
#48354=FACE_OUTER_BOUND ( 'NONE', #84772, .T. ) ;
#48356=CARTESIAN_POINT ( 'NONE',  ( 14.55774661933062042, -11.28795663066794575, 33.01431243580653785 ) ) ;
#48357=DIRECTION ( 'NONE',  ( 0.000000000000000000, -6.938893903907222067E-15, 1.000000000000000000 ) ) ;
#48358=CARTESIAN_POINT ( 'NONE',  ( 6.130791807824786943, -3.062576670634119758, 32.05464942895959979 ) ) ;
#48359=CARTESIAN_POINT ( 'NONE',  ( 1.254467414883686960, -2.647304123082328875, 31.75400227202885262 ) ) ;
#48360=LINE ( 'NONE', #75839, #17209 ) ;
#48361=CARTESIAN_POINT ( 'NONE',  ( 2.438484115517096207, -11.18335022499818621, 33.13157742990016885 ) ) ;
#48362=B_SPLINE_CURVE_WITH_KNOTS ( 'NONE', 3,
 ( #64797, #72452, #44081, #23810, #79667, #23376, #71123, #2217, #3550, #17969 ),
 .UNSPECIFIED., .F., .F.,
 ( 4, 2, 2, 2, 4 ),
 ( 0.000000000000000000, 0.0001954339857564080707, 0.0003908679715128161414, 0.0005863019572692241849, 0.0007817359430256322827 ),
 .UNSPECIFIED. ) ;
#48365=CARTESIAN_POINT ( 'NONE',  ( -1.384615384615383471, -6.435427911321262684, 35.78748833219616898 ) ) ;
#48366=CARTESIAN_POINT ( 'NONE',  ( -2.177166869458665222, -3.068774925481847493, 32.56582465632704526 ) ) ;
#48367=EDGE_CURVE ( 'NONE', #63956, #16211, #49199, .T. ) ;
#48368=CARTESIAN_POINT ( 'NONE',  ( 18.00000000000000000, -13.87047571288749737, 32.06866353760679544 ) ) ;
#48369=CARTESIAN_POINT ( 'NONE',  ( -7.846153846153844924, -8.120952969808772792, 34.71129190930000163 ) ) ;
#48370=ORIENTED_EDGE ( 'NONE', *, *, #5734, .F. ) ;
#48371=ORIENTED_EDGE ( 'NONE', *, *, #671, .F. ) ;
#48372=CARTESIAN_POINT ( 'NONE',  ( 3.230769230769231726, -6.435427911321262684, 35.78748833219616898 ) ) ;
#48374=CARTESIAN_POINT ( 'NONE',  ( -6.923076923077045919, -12.16647553114689728, 32.15551576947799362 ) ) ;
#48375=CARTESIAN_POINT ( 'NONE',  ( 9.758375025657770152, -11.91647553114624358, 32.58852847137148245 ) ) ;
#48376=VECTOR ( 'NONE', #7504, 1000.000000000000000 ) ;
#48377=CARTESIAN_POINT ( 'NONE',  ( 12.23805351781451201, -9.331801661448606566, 34.40259984581193464 ) ) ;
#48379=CARTESIAN_POINT ( 'NONE',  ( -6.130147209438218781, -8.587444163452046197, 34.63053765926554206 ) ) ;
#48381=ADVANCED_FACE ( 'NONE', ( #55376 ), #13508, .F. ) ;
#48382=EDGE_CURVE ( 'NONE', #74290, #59987, #31001, .T. ) ;
#48383=EDGE_LOOP ( 'NONE', ( #10848, #49273 ) ) ;
#48384=CARTESIAN_POINT ( 'NONE',  ( 0.7115927731767752729, -5.728107161865378494, 34.42597550085002922 ) ) ;
#48385=ORIENTED_EDGE ( 'NONE', *, *, #84014, .T. ) ;
#48386=EDGE_CURVE ( 'NONE', #14886, #28072, #29912, .T. ) ;
#48387=CARTESIAN_POINT ( 'NONE',  ( 10.68145296638705410, -8.120952969808772792, 34.71129190929999453 ) ) ;
#48388=CARTESIAN_POINT ( 'NONE',  ( -18.12834546407006542, -12.74539338292710511, 29.97517285561845668 ) ) ;
#48389=VECTOR ( 'NONE', #77941, 1000.000000000000000 ) ;
#48390=CARTESIAN_POINT ( 'NONE',  ( -6.673076923075503153, -7.500000000000154543, 35.00000000000007105 ) ) ;
#48391=DIRECTION ( 'NONE',  ( -0.000000000000000000, -0.9396926207859093161, -0.3420201433256663259 ) ) ;
#48392=DIRECTION ( 'NONE',  ( -0.000000000000000000, -0.000000000000000000, -1.000000000000000000 ) ) ;
#48393=AXIS2_PLACEMENT_3D ( 'NONE', #17883, #4361, #79586 ) ;
#48394=ORIENTED_EDGE ( 'NONE', *, *, #55386, .T. ) ;
#48395=ORIENTED_EDGE ( 'NONE', *, *, #73930, .T. ) ;
#48396=EDGE_LOOP ( 'NONE', ( #20031, #36956 ) ) ;
#48397=VERTEX_POINT ( 'NONE', #60362 ) ;
#48398=AXIS2_PLACEMENT_3D ( 'NONE', #79492, #4722, #18234 ) ;
#48399=CARTESIAN_POINT ( 'NONE',  ( -6.000000000000119904, -11.48612834414049644, 32.76840700105863391 ) ) ;
#48400=CARTESIAN_POINT ( 'NONE',  ( 5.011652630962299959, -10.90142922261923886, 33.41473453929638993 ) ) ;
#48401=CARTESIAN_POINT ( 'NONE',  ( 15.90384615384613021, -2.249999999999998668, 29.81609741502487054 ) ) ;
#48403=CARTESIAN_POINT ( 'NONE',  ( 8.096153846155266010, -7.500000000000154543, 35.00000000000007105 ) ) ;
#48404=CARTESIAN_POINT ( 'NONE',  ( 14.30769230769218758, -12.46129190930018460, 30.37095296980731973 ) ) ;
#48405=ORIENTED_EDGE ( 'NONE', *, *, #46540, .F. ) ;
#48407=ORIENTED_EDGE ( 'NONE', *, *, #13585, .F. ) ;
#48408=CYLINDRICAL_SURFACE ( 'NONE', #83314, 0.2499999999999986955 ) ;
#48409=ORIENTED_EDGE ( 'NONE', *, *, #65091, .T. ) ;
#48410=CARTESIAN_POINT ( 'NONE',  ( 17.29993592101647337, -10.77377354290276301, 33.85451476688484718 ) ) ;
#48411=CARTESIAN_POINT ( 'NONE',  ( -5.076923076923197442, -11.48612834414049644, 32.76840700105863391 ) ) ;
#48413=EDGE_LOOP ( 'NONE', ( #23398, #22361 ) ) ;
#48414=ORIENTED_EDGE ( 'NONE', *, *, #4410, .F. ) ;
#48415=DIRECTION ( 'NONE',  ( 0.000000000000000000, 0.8660254037844377084, -0.5000000000000015543 ) ) ;
#48417=FACE_BOUND ( 'NONE', #22792, .T. ) ;
#48418=CARTESIAN_POINT ( 'NONE',  ( 5.010840697562940704, -4.661471528628507777, 34.16647553114621871 ) ) ;
#48419=FACE_OUTER_BOUND ( 'NONE', #40246, .T. ) ;
#48420=VERTEX_POINT ( 'NONE', #82423 ) ;
#48423=DIRECTION ( 'NONE',  ( -0.000000000000000000, -0.1736481776669307198, -0.9848077530122080203 ) ) ;
#48424=CARTESIAN_POINT ( 'NONE',  ( 16.37662582282421653, -6.717445702608400460, 34.94155399931962336 ) ) ;
#48425=CARTESIAN_POINT ( 'NONE',  ( -3.480745974817822219, -9.234221910056348293, 34.70572697212741531 ) ) ;
#48426=ORIENTED_EDGE ( 'NONE', *, *, #79555, .F. ) ;
#48427=CARTESIAN_POINT ( 'NONE',  ( 11.76147289007438523, -3.105924265160262543, 32.13625925475356127 ) ) ;
#48428=CARTESIAN_POINT ( 'NONE',  ( -2.980769230769230393, -7.500000000000001776, 35.04278698407183867 ) ) ;
#48429=CARTESIAN_POINT ( 'NONE',  ( -3.931066484868084299, -2.353885683473779800, 30.79025554430704759 ) ) ;
#48430=CARTESIAN_POINT ( 'NONE',  ( -2.530618525208451874, -10.61292498521070549, 33.66303323003028680 ) ) ;
#48432=FACE_BOUND ( 'NONE', #25562, .T. ) ;
#48433=CARTESIAN_POINT ( 'NONE',  ( 13.31853197365950514, -11.69971097300155272, 32.46337939537587403 ) ) ;
#48434=CARTESIAN_POINT ( 'NONE',  ( -17.30040800148741553, -10.97335522853832579, 33.68706563782419749 ) ) ;
#48436=CARTESIAN_POINT ( 'NONE',  ( -8.519176457592456231, -11.79725096376909299, 32.30694842903960762 ) ) ;
#48437=CARTESIAN_POINT ( 'NONE',  ( 15.29683758177167086, -9.780366693483667717, 34.19971097300155805 ) ) ;
#48438=CYLINDRICAL_SURFACE ( 'NONE', #28998, 0.2500000000000009437 ) ;
#48440=VERTEX_POINT ( 'NONE', #41426 ) ;
#48441=B_SPLINE_CURVE_WITH_KNOTS ( 'NONE', 3,
 ( #70880, #43400, #72191, #59121, #10504, #78068, #30762, #57794, #9187, #15936 ),
 .UNSPECIFIED., .F., .F.,
 ( 4, 2, 2, 2, 4 ),
 ( 0.000000000000000000, 0.0001954311564186867389, 0.0003908623128373734778, 0.0005862934692560602167, 0.0007817246256747469556 ),
 .UNSPECIFIED. ) ;
#48443=EDGE_LOOP ( 'NONE', ( #41763, #43786, #52572, #72855 ) ) ;
#48444=EDGE_CURVE ( 'NONE', #50622, #21128, #6314, .T. ) ;
#48445=FACE_OUTER_BOUND ( 'NONE', #32438, .T. ) ;
#48446=VECTOR ( 'NONE', #20691, 1000.000000000000000 ) ;
#48448=DIRECTION ( 'NONE',  ( -0.000000000000000000, 0.1736481776669307198, -0.9848077530122080203 ) ) ;
#48449=CARTESIAN_POINT ( 'NONE',  ( -8.096177083446809419, -10.05641848906368097, 34.04755513067966177 ) ) ;
#48450=EDGE_LOOP ( 'NONE', ( #83938, #76247 ) ) ;
#48451=CARTESIAN_POINT ( 'NONE',  ( 17.75000000000000355, -7.433932668274255917, 35.00000000000000711 ) ) ;
#48453=CARTESIAN_POINT ( 'NONE',  ( -10.54931728203453822, -12.62096338111211757, 30.90682066428152908 ) ) ;
#48454=DIRECTION ( 'NONE',  ( 0.000000000000000000, 0.9396926207859126468, 0.3420201433256571111 ) ) ;
#48456=CARTESIAN_POINT ( 'NONE',  ( 12.39626801557768587, -2.892918686051582533, 31.69288490824015980 ) ) ;
#48458=CARTESIAN_POINT ( 'NONE',  ( -0.4615384615385826339, -4.481592998941358097, 33.73612834414048933 ) ) ;
#48461=CARTESIAN_POINT ( 'NONE',  ( -10.36533030374629938, -2.779044189368095275, 31.39831045268885745 ) ) ;
#48462=CYLINDRICAL_SURFACE ( 'NONE', #54947, 0.2500000000000002220 ) ;
#48463=EDGE_CURVE ( 'NONE', #32867, #314, #66444, .T. ) ;
#48465=ORIENTED_EDGE ( 'NONE', *, *, #82065, .F. ) ;
#48466=DIRECTION ( 'NONE',  ( 0.000000000000000000, 0.000000000000000000, 1.000000000000000000 ) ) ;
#48468=CARTESIAN_POINT ( 'NONE',  ( -17.86947429823644029, -12.45806712695776319, 30.39783852428763566 ) ) ;
#48469=LINE ( 'NONE', #69635, #25431 ) ;
#48470=VERTEX_POINT ( 'NONE', #71095 ) ;
#48471=CARTESIAN_POINT ( 'NONE',  ( -17.86920819217520773, -2.729792928343270919, 31.24908615093346498 ) ) ;
#48472=CARTESIAN_POINT ( 'NONE',  ( -16.94613263595612906, -9.084667340241228572, 34.75534355489798344 ) ) ;
#48473=CARTESIAN_POINT ( 'NONE',  ( 3.903822929624696236, -9.356822207818506598, 34.66110646841856635 ) ) ;
#48474=ORIENTED_EDGE ( 'NONE', *, *, #58443, .T. ) ;
#48475=DIRECTION ( 'NONE',  ( -0.000000000000000000, 0.9848077530122086864, -0.1736481776669273891 ) ) ;
#48476=CARTESIAN_POINT ( 'NONE',  ( -1.607541602131529856, -10.61292498521070549, 33.66303323003028680 ) ) ;
#48477=DIRECTION ( 'NONE',  ( -0.000000000000000000, -0.5000000000000009992, -0.8660254037844380415 ) ) ;
#48478=CARTESIAN_POINT ( 'NONE',  ( -17.01085472592064463, -2.721908614388772740, 31.22303859784725333 ) ) ;
#48479=DIRECTION ( 'NONE',  ( -0.000000000000000000, 0.9396926207859092051, -0.3420201433256662704 ) ) ;
#48480=VECTOR ( 'NONE', #1076, 1000.000000000000227 ) ;
#48481=ADVANCED_FACE ( 'NONE', ( #36438 ), #30117, .F. ) ;
#48482=EDGE_CURVE ( 'NONE', #33581, #70917, #31482, .T. ) ;
#48483=B_SPLINE_CURVE_WITH_KNOTS ( 'NONE', 3,
 ( #2861, #72217, #31236, #72665, #24473, #52387, #4662, #37099, #65468, #64559 ),
 .UNSPECIFIED., .F., .F.,
 ( 4, 2, 2, 2, 4 ),
 ( 0.000000000000000000, 0.0001954311564186876605, 0.0003908623128373753209, 0.0005862934692560629272, 0.0007817246256747506419 ),
 .UNSPECIFIED. ) ;
#48484=B_SPLINE_CURVE_WITH_KNOTS ( 'NONE', 3,
 ( #64139, #36251, #63706, #56948, #2012, #682, #48866, #84443, #2442, #29934 ),
 .UNSPECIFIED., .F., .F.,
 ( 4, 2, 2, 2, 4 ),
 ( 0.000000000000000000, 0.0001954311584214072923, 0.0003908623168428145846, 0.0005862934752642218498, 0.0007817246336856291692 ),
 .UNSPECIFIED. ) ;
#48485=EDGE_LOOP ( 'NONE', ( #59847, #26027 ) ) ;
#48488=EDGE_LOOP ( 'NONE', ( #69329, #79138, #14, #8088 ) ) ;
#48490=LINE ( 'NONE', #6629, #5505 ) ;
#48493=CARTESIAN_POINT ( 'NONE',  ( 2.241608896736428047, -5.557115091759785130, 34.35708131394839171 ) ) ;
#48494=CARTESIAN_POINT ( 'NONE',  ( -7.976301815885546098, -11.04286588640298561, 33.62463336215343901 ) ) ;
#48495=ORIENTED_EDGE ( 'NONE', *, *, #33364, .F. ) ;
#48496=CARTESIAN_POINT ( 'NONE',  ( 17.07692307692295586, -11.67786785259630911, 32.92929555188603530 ) ) ;
#48497=EDGE_LOOP ( 'NONE', ( #7641, #64378, #87577, #49123 ) ) ;
#48498=EDGE_LOOP ( 'NONE', ( #65831, #17728, #74020, #60493 ) ) ;
#48499=VERTEX_POINT ( 'NONE', #83303 ) ;
#48501=EDGE_LOOP ( 'NONE', ( #33032, #43090 ) ) ;
#48502=CARTESIAN_POINT ( 'NONE',  ( 4.153846153846154188, -5.557115091759785130, 34.35708131394839171 ) ) ;
#48503=CARTESIAN_POINT ( 'NONE',  ( 6.000000000000001776, -12.62096338111211580, 30.90682066428153263 ) ) ;
#48505=DIRECTION ( 'NONE',  ( -0.000000000000000000, -0.3420201433256694901, -0.9396926207859082059 ) ) ;
#48506=CARTESIAN_POINT ( 'NONE',  ( 14.55769230769237232, -7.434744860731433924, 35.00000000000000711 ) ) ;
#48508=ORIENTED_EDGE ( 'NONE', *, *, #28483, .T. ) ;
#48509=ORIENTED_EDGE ( 'NONE', *, *, #34747, .F. ) ;
#48510=CARTESIAN_POINT ( 'NONE',  ( -14.55769230769230660, -7.500000000000001776, 34.75000000000000000 ) ) ;
#48511=DIRECTION ( 'NONE',  ( -0.000000000000000000, -0.9848077530122085754, -0.1736481776669273613 ) ) ;
#48512=VERTEX_POINT ( 'NONE', #64331 ) ;
#48513=CARTESIAN_POINT ( 'NONE',  ( -11.31568186948346977, -12.69155399931963046, 30.53255429739157734 ) ) ;
#48514=DIRECTION ( 'NONE',  ( -0.000000000000000000, 0.1736481776669307198, -0.9848077530122080203 ) ) ;
#48515=ORIENTED_EDGE ( 'NONE', *, *, #54439, .F. ) ;
#48516=AXIS2_PLACEMENT_3D ( 'NONE', #57116, #411, #49911 ) ;
#48517=CARTESIAN_POINT ( 'NONE',  ( -17.93393164899756087, -2.538708090699994813, 30.37095296980875858 ) ) ;
#48518=CARTESIAN_POINT ( 'NONE',  ( 0.3962684609821413573, -9.528491918058357157, 34.59228464037090589 ) ) ;
#48520=FACE_BOUND ( 'NONE', #63053, .T. ) ;
#48521=CARTESIAN_POINT ( 'NONE',  ( -15.48079245499068612, -8.475808217655753651, 34.90892951860618609 ) ) ;
#48522=CARTESIAN_POINT ( 'NONE',  ( -18.06527000055631405, -12.51329471203370325, 31.30864560766548976 ) ) ;
#48523=CARTESIAN_POINT ( 'NONE',  ( 10.61538461538461675, -6.435427911321262684, 35.78748833219616898 ) ) ;
#48524=CARTESIAN_POINT ( 'NONE',  ( 16.15384615384615330, -9.780366693483667717, 34.19971097300155094 ) ) ;
#48525=CARTESIAN_POINT ( 'NONE',  ( -0.7115151924808156281, -12.17611988154120972, 31.52148481390971213 ) ) ;
#48526=CARTESIAN_POINT ( 'NONE',  ( 1.384615384615386802, -12.37446782046654192, 30.86335684631486131 ) ) ;
#48527=CARTESIAN_POINT ( 'NONE',  ( 14.53070515178570332, -2.308499170217967134, 30.53291367094873721 ) ) ;
#48528=VERTEX_POINT ( 'NONE', #21589 ) ;
#48531=VERTEX_POINT ( 'NONE', #70664 ) ;
#48532=ADVANCED_FACE ( 'NONE', ( #49058 ), #50809, .F. ) ;
#48533=CARTESIAN_POINT ( 'NONE',  ( 14.05766907039934210, -10.05641848906368097, 34.04755513067966177 ) ) ;
#48534=CARTESIAN_POINT ( 'NONE',  ( -3.230769230769229949, -11.69971097300155272, 32.46337939537588113 ) ) ;
#48535=ORIENTED_EDGE ( 'NONE', *, *, #33341, .F. ) ;
#48536=CARTESIAN_POINT ( 'NONE',  ( -9.822998295418001291, -9.084618155246140248, 34.75535874321725771 ) ) ;
#48538=FACE_BOUND ( 'NONE', #56100, .T. ) ;
#48539=CARTESIAN_POINT ( 'NONE',  ( -1.450697763975519194, -6.343179335718451384, 34.87096338111212646 ) ) ;
#48540=CARTESIAN_POINT ( 'NONE',  ( 3.903869409797563250, -12.41104346484419452, 31.60698883733904196 ) ) ;
#48541=CARTESIAN_POINT ( 'NONE',  ( -13.63463860883683942, -2.341070481393819236, 30.72580821765574299 ) ) ;
#48542=CARTESIAN_POINT ( 'NONE',  ( 12.33084785842815911, -12.35290016733513951, 31.75349464988449455 ) ) ;
#48544=DIRECTION ( 'NONE',  ( -0.000000000000000000, 0.5000000000000009992, -0.8660254037844380415 ) ) ;
#48545=CARTESIAN_POINT ( 'NONE',  ( 0.4615384615384611200, -9.058645607665452459, 34.76329471203371924 ) ) ;
#48546=VECTOR ( 'NONE', #62048, 999.9999999999998863 ) ;
#48549=VERTEX_POINT ( 'NONE', #14848 ) ;
#48550=EDGE_CURVE ( 'NONE', #62397, #7759, #8377, .T. ) ;
#48551=CARTESIAN_POINT ( 'NONE',  ( -9.915792616872025178, -2.353723527008296568, 30.78948104536958752 ) ) ;
#48554=DIRECTION ( 'NONE',  ( 0.000000000000000000, 0.9848077530122072432, 0.1736481776669354937 ) ) ;
#48555=CARTESIAN_POINT ( 'NONE',  ( -1.634592115557737424, -3.137211980971221781, 32.19342716148376837 ) ) ;
#48556=EDGE_CURVE ( 'NONE', #8808, #51516, #69623, .T. ) ;
#48557=CARTESIAN_POINT ( 'NONE',  ( -13.16183571563731824, -2.612705202774698421, 31.66806509827799943 ) ) ;
#48559=DIRECTION ( 'NONE',  ( 0.000000000000000000, -1.000000000000000000, -8.673617379884033500E-16 ) ) ;
#48560=DIRECTION ( 'NONE',  ( 0.000000000000000000, 0.9848077530122072432, -0.1736481776669354937 ) ) ;
#48561=CARTESIAN_POINT ( 'NONE',  ( 9.561617089197390840, -10.70098750199973203, 33.91152734681376302 ) ) ;
#48562=CARTESIAN_POINT ( 'NONE',  ( -4.854143407945009869, -2.353885683473779800, 30.79025554430704759 ) ) ;
#48563=CARTESIAN_POINT ( 'NONE',  ( -1.634615384615383027, -7.500000000000001776, 35.00000000000000000 ) ) ;
#48564=CARTESIAN_POINT ( 'NONE',  ( -4.854143407945009869, -6.717445702608402236, 34.94155399931962336 ) ) ;
#48565=B_SPLINE_CURVE_WITH_KNOTS ( 'NONE', 3,
 ( #36043, #56305, #29288, #77025, #77462, #63043, #41915, #77898, #70708, #43666 ),
 .UNSPECIFIED., .F., .F.,
 ( 4, 2, 2, 2, 4 ),
 ( 0.000000000000000000, 0.0001954339857564069594, 0.0003908679715128139187, 0.0005863019572692209323, 0.0007817359430256278375 ),
 .UNSPECIFIED. ) ;
#48567=CARTESIAN_POINT ( 'NONE',  ( -14.30769230769242739, -3.300289026999228881, 32.46337939537708905 ) ) ;
#48568=EDGE_CURVE ( 'NONE', #77057, #10775, #33103, .T. ) ;
#48570=EDGE_LOOP ( 'NONE', ( #23917, #49829 ) ) ;
#48571=CARTESIAN_POINT ( 'NONE',  ( -0.3954701105360229341, -3.513871655860379306, 32.76840700105978499 ) ) ;
#48572=CARTESIAN_POINT ( 'NONE',  ( 0.5267940328144855577, -2.625532179533470512, 30.86335684631491105 ) ) ;
#48574=EDGE_CURVE ( 'NONE', #75011, #7293, #22038, .T. ) ;
#48577=DIRECTION ( 'NONE',  ( -0.000000000000000000, 0.8660254037844397068, -0.4999999999999978906 ) ) ;
#48578=EDGE_LOOP ( 'NONE', ( #15930, #64836, #45263, #7888, #83766, #36652 ) ) ;
#48579=CARTESIAN_POINT ( 'NONE',  ( -16.40384615384615685, -2.499999999999999556, 29.81609845454691765 ) ) ;
#48580=CARTESIAN_POINT ( 'NONE',  ( -14.43838377435986864, -12.11776431015576172, 31.66791131148498906 ) ) ;
#48581=ORIENTED_EDGE ( 'NONE', *, *, #68557, .T. ) ;
#48582=CARTESIAN_POINT ( 'NONE',  ( 9.823098133274644539, -12.62708834333097663, 30.88030960425257021 ) ) ;
#48583=LINE ( 'NONE', #29226, #19594 ) ;
#48584=B_SPLINE_CURVE_WITH_KNOTS ( 'NONE', 3,
 ( #68746, #61982, #83155, #82717, #20990, #48461, #76388, #21447, #16023, #30421 ),
 .UNSPECIFIED., .F., .F.,
 ( 4, 2, 2, 2, 4 ),
 ( 0.0007817359430256293554, 0.0009771253907249941549, 0.001172514838424358954, 0.001367904286123723537, 0.001563293733823095276 ),
 .UNSPECIFIED. ) ;
#48585=ORIENTED_EDGE ( 'NONE', *, *, #28539, .F. ) ;
#48586=DIRECTION ( 'NONE',  ( -0.000000000000000000, -0.8660254037844397068, -0.4999999999999978906 ) ) ;
#48587=VECTOR ( 'NONE', #39617, 1000.000000000000227 ) ;
#48588=CARTESIAN_POINT ( 'NONE',  ( 8.096153846153782752, -7.565270445406050648, 34.75000000000000000 ) ) ;
#48590=CARTESIAN_POINT ( 'NONE',  ( -10.83831157429146508, -4.026226216239094491, 33.68668979543634379 ) ) ;
#48592=EDGE_CURVE ( 'NONE', #34081, #23012, #67438, .T. ) ;
#48593=VECTOR ( 'NONE', #57449, 1000.000000000000227 ) ;
#48594=CARTESIAN_POINT ( 'NONE',  ( 12.71148387091650278, -12.07971442181322352, 32.31769673815850297 ) ) ;
#48596=EDGE_CURVE ( 'NONE', #45649, #46211, #38531, .T. ) ;
#48597=VERTEX_POINT ( 'NONE', #9842 ) ;
#48598=CARTESIAN_POINT ( 'NONE',  ( -6.700064078983528404, -8.282913670948747864, 34.94150082978203642 ) ) ;
#48599=ORIENTED_EDGE ( 'NONE', *, *, #73154, .F. ) ;
#48600=CARTESIAN_POINT ( 'NONE',  ( -5.999999999999998224, -13.53365097954675988, 30.81389545987213552 ) ) ;
#48602=CARTESIAN_POINT ( 'NONE',  ( -5.326899820971668476, -9.234221910056348293, 34.70572697212741531 ) ) ;
#48603=CARTESIAN_POINT ( 'NONE',  ( -14.43838377435986864, -3.062553014421049546, 32.05460306192773601 ) ) ;
#48604=EDGE_CURVE ( 'NONE', #70832, #34382, #23786, .T. ) ;
#48605=CARTESIAN_POINT ( 'NONE',  ( -9.758391103263569732, -4.786620604624113540, 33.94971097300155805 ) ) ;
#48606=CYLINDRICAL_SURFACE ( 'NONE', #11954, 0.2499999999999973355 ) ;
#48607=LINE ( 'NONE', #8080, #6410 ) ;
#48608=CARTESIAN_POINT ( 'NONE',  ( 15.45414517146741140, -2.501478030877322567, 29.88021232661721172 ) ) ;
#48610=EDGE_LOOP ( 'NONE', ( #75453, #88039, #50352, #64529 ) ) ;
#48611=ORIENTED_EDGE ( 'NONE', *, *, #19707, .T. ) ;
#48612=DIRECTION ( 'NONE',  ( 0.000000000000000000, -6.938893903907222067E-15, 1.000000000000000000 ) ) ;
#48614=B_SPLINE_CURVE_WITH_KNOTS ( 'NONE', 3,
 ( #81204, #20382, #47843, #28466, #33454, #88417, #61792, #69001, #75326, #27133 ),
 .UNSPECIFIED., .F., .F.,
 ( 4, 2, 2, 2, 4 ),
 ( 0.000000000000000000, 0.0001954339857564081520, 0.0003908679715128163040, 0.0005863019572692244018, 0.0007817359430256326080 ),
 .UNSPECIFIED. ) ;
#48615=AXIS2_PLACEMENT_3D ( 'NONE', #9759, #84552, #50727 ) ;
#48616=CARTESIAN_POINT ( 'NONE',  ( 7.780883845597526438, -2.657715359629088780, 31.77849191805832874 ) ) ;
#48618=VECTOR ( 'NONE', #22347, 1000.000000000000114 ) ;
#48619=CYLINDRICAL_SURFACE ( 'NONE', #49282, 0.2500000000000009437 ) ;
#48620=CARTESIAN_POINT ( 'NONE',  ( 5.326868595271218254, -3.712312575010499494, 33.01462480002815170 ) ) ;
#48622=CARTESIAN_POINT ( 'NONE',  ( -24.00000000000000000, -9.499999999999982236, 27.74999999999999645 ) ) ;
#48623=EDGE_LOOP ( 'NONE', ( #25323, #86093, #36339, #60704 ) ) ;
#48624=ORIENTED_EDGE ( 'NONE', *, *, #77315, .T. ) ;
#48626=EDGE_CURVE ( 'NONE', #21723, #83108, #41718, .T. ) ;
#48627=ORIENTED_EDGE ( 'NONE', *, *, #20165, .F. ) ;
#48628=CYLINDRICAL_SURFACE ( 'NONE', #87759, 0.2500000000000009437 ) ;
#48629=CARTESIAN_POINT ( 'NONE',  ( 17.01165263096230262, -2.892918686051582533, 31.69288490824015980 ) ) ;
#48630=FACE_BOUND ( 'NONE', #78973, .T. ) ;
#48631=FACE_OUTER_BOUND ( 'NONE', #26902, .T. ) ;
#48632=DIRECTION ( 'NONE',  ( 0.000000000000000000, 0.4999999999999960032, -0.8660254037844410391 ) ) ;
#48633=CARTESIAN_POINT ( 'NONE',  ( 9.692307692307695177, -2.292212530054420494, 30.41441678777542634 ) ) ;
#48634=CARTESIAN_POINT ( 'NONE',  ( 3.296836564119306701, -4.661471528628508665, 34.16647553114624003 ) ) ;
#48635=AXIS2_PLACEMENT_3D ( 'NONE', #22302, #70041, #77242 ) ;
#48636=CARTESIAN_POINT ( 'NONE',  ( 5.326977388561387805, -10.66356715214248396, 33.62249196103329751 ) ) ;
#48637=CARTESIAN_POINT ( 'NONE',  ( 15.93036121012220541, -4.386631170607603991, 33.66268669641500111 ) ) ;
#48638=EDGE_LOOP ( 'NONE', ( #20543, #32560 ) ) ;
#48639=CYLINDRICAL_SURFACE ( 'NONE', #84974, 0.2500000000000008882 ) ;
#48640=EDGE_LOOP ( 'NONE', ( #2880, #25929, #70874, #12260 ) ) ;
#48641=EDGE_CURVE ( 'NONE', #58240, #22124, #57811, .T. ) ;
#48642=ORIENTED_EDGE ( 'NONE', *, *, #87179, .T. ) ;
#48643=EDGE_CURVE ( 'NONE', #31900, #75897, #86875, .T. ) ;
#48644=VECTOR ( 'NONE', #10511, 999.9999999999998863 ) ;
#48645=CARTESIAN_POINT ( 'NONE',  ( 2.307692307692309264, -2.833524468853757305, 32.15551576947925838 ) ) ;
#48647=DIRECTION ( 'NONE',  ( -0.000000000000000000, -0.8660254037844397068, -0.4999999999999978906 ) ) ;
#48648=DIRECTION ( 'NONE',  ( -0.000000000000000000, 0.9396926207859092051, -0.3420201433256662704 ) ) ;
#48649=CYLINDRICAL_SURFACE ( 'NONE', #2734, 0.2499999999999986955 ) ;
#48650=FACE_OUTER_BOUND ( 'NONE', #76126, .T. ) ;
#48651=ORIENTED_EDGE ( 'NONE', *, *, #14055, .T. ) ;
#48652=CARTESIAN_POINT ( 'NONE',  ( -5.076923076923199218, -5.941354392335915335, 34.76329471203413846 ) ) ;
#48653=CARTESIAN_POINT ( 'NONE',  ( -6.249976730942353065, -6.567427716900047230, 34.66269422305636283 ) ) ;
#48654=CARTESIAN_POINT ( 'NONE',  ( 17.07692307692307665, -3.937682226553329556, 33.60647404775216529 ) ) ;
#48655=CARTESIAN_POINT ( 'NONE',  ( 15.29602437028207085, -12.51329471203373345, 31.30864560766537963 ) ) ;
#48656=ORIENTED_EDGE ( 'NONE', *, *, #23028, .T. ) ;
#48657=B_SPLINE_CURVE_WITH_KNOTS ( 'NONE', 3,
 ( #32370, #3551, #59836, #51265, #44974, #17525, #4444, #85536, #86446, #64798 ),
 .UNSPECIFIED., .F., .F.,
 ( 4, 2, 2, 2, 4 ),
 ( 0.0007817246256747515092, 0.0009771112852218961399, 0.001172497944769040771, 0.001367884604316185401, 0.001563271263863330032 ),
 .UNSPECIFIED. ) ;
#48659=B_SPLINE_CURVE_WITH_KNOTS ( 'NONE', 3,
 ( #72724, #80393, #87603, #25881, #86719, #5165, #4727, #17799, #32202, #40293 ),
 .UNSPECIFIED., .F., .F.,
 ( 4, 2, 2, 2, 4 ),
 ( 0.000000000000000000, 0.0001954311564186882568, 0.0003908623128373765136, 0.0005862934692560647703, 0.0007817246256747530271 ),
 .UNSPECIFIED. ) ;
#48660=ORIENTED_EDGE ( 'NONE', *, *, #12414, .T. ) ;
#48661=EDGE_CURVE ( 'NONE', #32595, #13908, #1989, .T. ) ;
#48662=CARTESIAN_POINT ( 'NONE',  ( -6.988347369037697376, -8.613356846314824011, 34.62446782046655613 ) ) ;
#48663=VERTEX_POINT ( 'NONE', #3520 ) ;
#48664=CYLINDRICAL_SURFACE ( 'NONE', #71408, 0.2499999999999994726 ) ;
#48665=CARTESIAN_POINT ( 'NONE',  ( 15.48082365068267841, -4.074993327901527351, 33.72946981652012255 ) ) ;
#48666=CARTESIAN_POINT ( 'NONE',  ( 14.08476534878545827, -10.01117774369187252, 34.36070679894347535 ) ) ;
#48667=EDGE_CURVE ( 'NONE', #58521, #42680, #58456, .T. ) ;
#48668=CARTESIAN_POINT ( 'NONE',  ( 6.923076923076924238, -9.780366693483667717, 34.19971097300155094 ) ) ;
#48669=CARTESIAN_POINT ( 'NONE',  ( 12.23861224402231151, -9.886141570436013382, 34.14413921362392301 ) ) ;
#48670=EDGE_LOOP ( 'NONE', ( #28834, #47182 ) ) ;
#48671=CARTESIAN_POINT ( 'NONE',  ( 4.284637961670941131, -4.118422570099827595, 33.43335022499816489 ) ) ;
#48672=DIRECTION ( 'NONE',  ( 0.000000000000000000, 0.000000000000000000, 1.000000000000000000 ) ) ;
#48673=VERTEX_POINT ( 'NONE', #65659 ) ;
#48674=CARTESIAN_POINT ( 'NONE',  ( -3.480769230769229061, -2.499999999999998668, 29.75000000000000355 ) ) ;
#48675=CARTESIAN_POINT ( 'NONE',  ( -8.519230769230832223, -7.565270000091922853, 34.99999999999999289 ) ) ;
#48676=CARTESIAN_POINT ( 'NONE',  ( 16.94623161025551639, -3.530157926970578508, 32.79014554554150607 ) ) ;
#48677=CARTESIAN_POINT ( 'NONE',  ( 4.153846153846154188, -6.189225973068211317, 35.74407628777942847 ) ) ;
#48678=CARTESIAN_POINT ( 'NONE',  ( -12.59168567097668223, -2.882441371585227508, 31.66841991370172238 ) ) ;
#48680=ADVANCED_FACE ( 'NONE', ( #86421 ), #6204, .F. ) ;
#48681=DIRECTION ( 'NONE',  ( -0.000000000000000000, -0.7660444431189791237, -0.6427876096865379196 ) ) ;
#48683=ORIENTED_EDGE ( 'NONE', *, *, #48351, .T. ) ;
#48684=AXIS2_PLACEMENT_3D ( 'NONE', #54753, #35370, #82239 ) ;
#48685=CARTESIAN_POINT ( 'NONE',  ( -1.318547033612945896, -11.16473453929635440, 33.15142922261926373 ) ) ;
#48686=CARTESIAN_POINT ( 'NONE',  ( -14.24162497434223340, -3.322132147404559976, 32.92929555188717927 ) ) ;
#48687=CYLINDRICAL_SURFACE ( 'NONE', #57603, 0.2499999999999995559 ) ;
#48688=CARTESIAN_POINT ( 'NONE',  ( 9.561617089197383734, -6.369640206132551441, 34.87707690430378449 ) ) ;
#48689=VERTEX_POINT ( 'NONE', #13836 ) ;
#48690=CARTESIAN_POINT ( 'NONE',  ( 0.2380535369741295093, -4.225889041578353655, 33.85425143139329407 ) ) ;
#48691=CARTESIAN_POINT ( 'NONE',  ( -15.93083480223330817, -12.15243808032446005, 31.58219941686247978 ) ) ;
#48692=B_SPLINE_CURVE_WITH_KNOTS ( 'NONE', 3,
 ( #5011, #31587, #80687, #46435, #52296, #38349, #4104, #79786, #12214, #86553 ),
 .UNSPECIFIED., .F., .F.,
 ( 4, 2, 2, 2, 4 ),
 ( 0.000000000000000000, 0.0001954311564186868473, 0.0003908623128373736946, 0.0005862934692560605419, 0.0007817246256747473893 ),
 .UNSPECIFIED. ) ;
#48693=CARTESIAN_POINT ( 'NONE',  ( -0.5916864312701589634, -12.70455904226513866, 30.44083106164009322 ) ) ;
#48694=CARTESIAN_POINT ( 'NONE',  ( -0.6850233861027944515, -10.97335522853832579, 33.68706563782419749 ) ) ;
#48695=B_SPLINE_CURVE_WITH_KNOTS ( 'NONE', 3,
 ( #68450, #880, #28345, #41429, #80768, #69779, #8087, #48170, #48616, #76984 ),
 .UNSPECIFIED., .F., .F.,
 ( 4, 2, 2, 2, 4 ),
 ( 0.000000000000000000, 0.0001954311564186862239, 0.0003908623128373724478, 0.0005862934692560586988, 0.0007817246256747448956 ),
 .UNSPECIFIED. ) ;
#48696=ORIENTED_EDGE ( 'NONE', *, *, #64020, .F. ) ;
#48697=B_SPLINE_CURVE_WITH_KNOTS ( 'NONE', 3,
 ( #52123, #71505, #45364, #9813, #37277, #38621, #44467, #25552, #67869, #53909 ),
 .UNSPECIFIED., .F., .F.,
 ( 4, 2, 2, 2, 4 ),
 ( 0.000000000000000000, 0.0001954339857564099951, 0.0003908679715128199903, 0.0005863019572692300396, 0.0007817359430256399806 ),
 .UNSPECIFIED. ) ;
#48698=B_SPLINE_CURVE_WITH_KNOTS ( 'NONE', 3,
 ( #26084, #77368, #42706, #70170, #76036, #84587, #41823, #15677, #35050, #21986 ),
 .UNSPECIFIED., .F., .F.,
 ( 4, 2, 2, 2, 4 ),
 ( 0.0007817359430256251270, 0.0009771253907249900349, 0.001172514838424354834, 0.001367904286123719851, 0.001563293733823084650 ),
 .UNSPECIFIED. ) ;
#48699=CARTESIAN_POINT ( 'NONE',  ( 17.07692307692295586, -3.300289026999228437, 32.46337939537709616 ) ) ;
#48700=EDGE_CURVE ( 'NONE', #7957, #4203, #77116, .T. ) ;
#48702=CARTESIAN_POINT ( 'NONE',  ( 18.13052543823364360, -12.50538340440932394, 31.33453814440721885 ) ) ;
#48703=ORIENTED_EDGE ( 'NONE', *, *, #44715, .F. ) ;
#48704=CYLINDRICAL_SURFACE ( 'NONE', #72916, 0.2500000000000009437 ) ;
#48706=ORIENTED_EDGE ( 'NONE', *, *, #53449, .T. ) ;
#48707=VECTOR ( 'NONE', #65730, 1000.000000000000227 ) ;
#48708=FACE_OUTER_BOUND ( 'NONE', #66320, .T. ) ;
#48709=CARTESIAN_POINT ( 'NONE',  ( 5.076923076923075762, -5.471508081941601098, 34.59228464037088457 ) ) ;
#48710=EDGE_LOOP ( 'NONE', ( #42919, #46913, #16200, #26668 ) ) ;
#48711=ADVANCED_FACE ( 'NONE', ( #34109 ), #81869, .F. ) ;
#48712=CARTESIAN_POINT ( 'NONE',  ( -39.05038313613820122, -2.249999999999998668, 29.75000000000000355 ) ) ;
#48713=CARTESIAN_POINT ( 'NONE',  ( 4.284636594813103549, -9.084667340241226796, 34.75534355489798344 ) ) ;
#48714=CARTESIAN_POINT ( 'NONE',  ( -11.76194648218548622, -6.760086850603066466, 34.69517049084099369 ) ) ;
#48715=AXIS2_PLACEMENT_3D ( 'NONE', #76540, #84197, #70221 ) ;
#48717=CARTESIAN_POINT ( 'NONE',  ( 11.40777093535123399, -12.35290016733513951, 31.75349464988449455 ) ) ;
#48720=FACE_BOUND ( 'NONE', #81537, .T. ) ;
#48721=EDGE_LOOP ( 'NONE', ( #82650, #68562 ) ) ;
#48722=LINE ( 'NONE', #27573, #41456 ) ;
#48723=EDGE_CURVE ( 'NONE', #52054, #15626, #67460, .T. ) ;
#48724=B_SPLINE_CURVE_WITH_KNOTS ( 'NONE', 3,
 ( #75860, #2842, #65446, #58241, #10509, #37078, #45169, #71751, #9192, #16376 ),
 .UNSPECIFIED., .F., .F.,
 ( 4, 2, 2, 2, 4 ),
 ( 0.000000000000000000, 0.0001954339857564079623, 0.0003908679715128159245, 0.0005863019572692238597, 0.0007817359430256318490 ),
 .UNSPECIFIED. ) ;
#48725=CARTESIAN_POINT ( 'NONE',  ( -14.05763788777885281, -11.47946981652013498, 33.17500667209847620 ) ) ;
#48726=EDGE_CURVE ( 'NONE', #18197, #22884, #63240, .T. ) ;
#48728=CARTESIAN_POINT ( 'NONE',  ( 16.82694634598072625, -2.564618984488975517, 30.55390908950641915 ) ) ;
#48729=ORIENTED_EDGE ( 'NONE', *, *, #76538, .F. ) ;
#48730=VERTEX_POINT ( 'NONE', #27354 ) ;
#48731=ORIENTED_EDGE ( 'NONE', *, *, #81780, .T. ) ;
#48732=B_SPLINE_CURVE_WITH_KNOTS ( 'NONE', 3,
 ( #53404, #67374, #88120, #56411, #62707, #7781, #70370, #22184, #35246, #70818 ),
 .UNSPECIFIED., .F., .F.,
 ( 4, 2, 2, 2, 4 ),
 ( 0.0007817246256747469556, 0.0009771112852218896347, 0.001172497944769032531, 0.001367884604316175427, 0.001563271263863318106 ),
 .UNSPECIFIED. ) ;
#48733=CARTESIAN_POINT ( 'NONE',  ( -3.230769230769352962, -11.67786785259630911, 32.92929555188603530 ) ) ;
#48734=ORIENTED_EDGE ( 'NONE', *, *, #54167, .F. ) ;
#48735=EDGE_CURVE ( 'NONE', #44386, #4983, #35327, .T. ) ;
#48736=CARTESIAN_POINT ( 'NONE',  ( -6.250023237292964495, -12.43535235679832596, 30.55408501211184813 ) ) ;
#48738=CARTESIAN_POINT ( 'NONE',  ( -13.38461538461550759, -8.656820664282941280, 34.87096338111179961 ) ) ;
#48739=ADVANCED_FACE ( 'NONE', ( #34557 ), #33231, .F. ) ;
#48740=CARTESIAN_POINT ( 'NONE',  ( 13.63466980452883881, -11.47946981652013498, 33.17500667209847620 ) ) ;
#48741=CARTESIAN_POINT ( 'NONE',  ( 16.15384615384615330, -2.292212530054420494, 30.41441678777542634 ) ) ;
#48742=EDGE_CURVE ( 'NONE', #26012, #83335, #21026, .T. ) ;
#48744=CARTESIAN_POINT ( 'NONE',  ( 3.930919194939305861, -2.523278758544489797, 31.42238647778637528 ) ) ;
#48745=CARTESIAN_POINT ( 'NONE',  ( 17.07692307692295586, -2.625532179533778709, 30.86335684631627174 ) ) ;
#48746=ORIENTED_EDGE ( 'NONE', *, *, #78057, .F. ) ;
#48747=EDGE_LOOP ( 'NONE', ( #69614, #26569, #28003, #49097 ) ) ;
#48748=VERTEX_POINT ( 'NONE', #60692 ) ;
#48750=EDGE_CURVE ( 'NONE', #17603, #10737, #73784, .T. ) ;
#48751=CARTESIAN_POINT ( 'NONE',  ( -3.230769230769229949, -9.905515769479276145, 34.41647553114623292 ) ) ;
#48753=DIRECTION ( 'NONE',  ( 0.000000000000000000, 0.6427876096865373645, -0.7660444431189797898 ) ) ;
#48754=CARTESIAN_POINT ( 'NONE',  ( 12.52679360105129724, -12.70778746994558439, 30.41441678777536595 ) ) ;
#48755=CYLINDRICAL_SURFACE ( 'NONE', #44329, 0.2499999999999994726 ) ;
#48756=DIRECTION ( 'NONE',  ( 0.000000000000000000, 0.9396926207859126468, -0.3420201433256571111 ) ) ;
#48758=CARTESIAN_POINT ( 'NONE',  ( -5.076923076923075762, -13.78497067705608181, 32.30358669280327177 ) ) ;
#48760=CARTESIAN_POINT ( 'NONE',  ( -1.384615384615383471, -2.721908614388771852, 31.22303859784724978 ) ) ;
#48761=CARTESIAN_POINT ( 'NONE',  ( 3.296024370282069071, -11.67786785259547777, 32.92929555188713664 ) ) ;
#48762=ORIENTED_EDGE ( 'NONE', *, *, #32713, .T. ) ;
#48763=CARTESIAN_POINT ( 'NONE',  ( 18.06606835100243913, -12.37446782046654192, 30.86335684631486842 ) ) ;
#48764=ORIENTED_EDGE ( 'NONE', *, *, #33667, .T. ) ;
#48765=FACE_BOUND ( 'NONE', #11876, .T. ) ;
#48766=CARTESIAN_POINT ( 'NONE',  ( -17.20761368003338987, -3.957541250942358424, 33.62499894934981626 ) ) ;
#48767=AXIS2_PLACEMENT_3D ( 'NONE', #20482, #7418, #74544 ) ;
#48768=CARTESIAN_POINT ( 'NONE',  ( 16.82694634598072625, -11.79746400365624659, 32.30657167506340954 ) ) ;
#48769=DIRECTION ( 'NONE',  ( -0.000000000000000000, 1.000000000000000000, -0.000000000000000000 ) ) ;
#48771=CARTESIAN_POINT ( 'NONE',  ( -12.68446467905460828, -9.886141570436013382, 34.14413921362392301 ) ) ;
#48772=CARTESIAN_POINT ( 'NONE',  ( 4.826923076923076650, -7.500000000000001776, 34.75000000000000000 ) ) ;
#48773=CARTESIAN_POINT ( 'NONE',  ( -16.15384615384627409, -12.46129190930018460, 30.37095296980731973 ) ) ;
#48774=EDGE_CURVE ( 'NONE', #59465, #46553, #81437, .T. ) ;
#48777=VECTOR ( 'NONE', #57487, 1000.000000000000227 ) ;
#48778=CARTESIAN_POINT ( 'NONE',  ( -4.853910232829682592, -4.762714258010880997, 34.23016756924214832 ) ) ;
#48779=ORIENTED_EDGE ( 'NONE', *, *, #48932, .F. ) ;
#48780=AXIS2_PLACEMENT_3D ( 'NONE', #87162, #24990, #58323 ) ;
#48781=CARTESIAN_POINT ( 'NONE',  ( 16.40384615384622080, -7.434744860731433924, 35.00000000000000711 ) ) ;
#48782=ORIENTED_EDGE ( 'NONE', *, *, #28763, .F. ) ;
#48783=CARTESIAN_POINT ( 'NONE',  ( 9.442330961365341224, -3.627789207965226748, 32.91389620160131102 ) ) ;
#48784=CARTESIAN_POINT ( 'NONE',  ( -4.284537620513710010, -2.729777683071817229, 31.24903638046268739 ) ) ;
#48785=CARTESIAN_POINT ( 'NONE',  ( -3.480769230769229061, -7.500000000000001776, 35.00000000000000000 ) ) ;
#48786=CARTESIAN_POINT ( 'NONE',  ( -17.75000000000000000, -2.499999999999999556, 29.75000000000000355 ) ) ;
#48787=CARTESIAN_POINT ( 'NONE',  ( -13.16183571563731824, -3.563462043263030399, 33.22394488606062879 ) ) ;
#48788=CARTESIAN_POINT ( 'NONE',  ( 13.63456090296352841, -5.852078868378309373, 34.47109172314383585 ) ) ;
#48789=LINE ( 'NONE', #33517, #48955 ) ;
#48790=FACE_OUTER_BOUND ( 'NONE', #47940, .T. ) ;
#48794=VERTEX_POINT ( 'NONE', #28690 ) ;
#48795=VERTEX_POINT ( 'NONE', #63788 ) ;
#48796=CARTESIAN_POINT ( 'NONE',  ( 3.165498784808455923, -5.219633306516282545, 34.19971097300152252 ) ) ;
#48797=EDGE_LOOP ( 'NONE', ( #82541, #60479 ) ) ;
#48798=CARTESIAN_POINT ( 'NONE',  ( 14.30769230769218758, -8.613356846316285953, 34.62446782046622218 ) ) ;
#48800=CARTESIAN_POINT ( 'NONE',  ( -11.47239420511146513, -9.905515769479276145, 34.41647553114623292 ) ) ;
#48801=CARTESIAN_POINT ( 'NONE',  ( -16.02332045208259359, -6.001044277235011215, 34.52024696741798948 ) ) ;
#48802=CARTESIAN_POINT ( 'NONE',  ( -11.60373198442231413, -11.48612834413959582, 32.76840700105983473 ) ) ;
#48803=CARTESIAN_POINT ( 'NONE',  ( 11.53846153846153832, -1.422936976036506707, 30.56769352161908415 ) ) ;
#48804=CARTESIAN_POINT ( 'NONE',  ( 12.33084699487090674, -10.54014554554150607, 33.71984207302941883 ) ) ;
#48807=CARTESIAN_POINT ( 'NONE',  ( 6.923076923076924238, -9.905515769479276145, 34.41647553114623292 ) ) ;
#48808=CARTESIAN_POINT ( 'NONE',  ( 17.75002326905764605, -11.79746400365624659, 32.30657167506340954 ) ) ;
#48809=CARTESIAN_POINT ( 'NONE',  ( 5.299702745901138989, -10.97394488606064122, 33.68653795673694873 ) ) ;
#48811=CARTESIAN_POINT ( 'NONE',  ( -9.822455662039390134, -11.66186481527757302, 32.95055677023626117 ) ) ;
#48812=B_SPLINE_CURVE_WITH_KNOTS ( 'NONE', 3,
 ( #32282, #18322, #23727, #10236, #25521, #72808, #3461, #44888, #11116, #66047 ),
 .UNSPECIFIED., .F., .F.,
 ( 4, 2, 2, 2, 4 ),
 ( 0.000000000000000000, 0.0001954339857564076099, 0.0003908679715128152198, 0.0005863019572692228839, 0.0007817359430256304396 ),
 .UNSPECIFIED. ) ;
#48814=ORIENTED_EDGE ( 'NONE', *, *, #27945, .F. ) ;
#48815=ORIENTED_EDGE ( 'NONE', *, *, #56091, .T. ) ;
#48816=CARTESIAN_POINT ( 'NONE',  ( -18.06608237936013239, -2.486705287966280320, 31.30864560766542937 ) ) ;
#48817=CARTESIAN_POINT ( 'NONE',  ( -14.30769230769230660, -1.629998284177014645, 34.34916445242399163 ) ) ;
#48818=LINE ( 'NONE', #6952, #23892 ) ;
#48820=EDGE_CURVE ( 'NONE', #43614, #14333, #36765, .T. ) ;
#48821=CARTESIAN_POINT ( 'NONE',  ( 9.942362112221147186, -11.47946981652013498, 33.17500667209847620 ) ) ;
#48823=EDGE_CURVE ( 'NONE', #11766, #83962, #766, .T. ) ;
#48824=LINE ( 'NONE', #61448, #62372 ) ;
#48825=B_SPLINE_CURVE_WITH_KNOTS ( 'NONE', 3,
 ( #48403, #75883, #21380, #56933, #34890, #14181, #63691, #1998, #41660, #29480 ),
 .UNSPECIFIED., .F., .F.,
 ( 4, 2, 2, 2, 4 ),
 ( 0.0007817246336856291692, 0.0009771112958940103739, 0.001172497958102391470, 0.001367884620310772566, 0.001563271282519153879 ),
 .UNSPECIFIED. ) ;
#48826=VERTEX_POINT ( 'NONE', #28234 ) ;
#48827=B_SPLINE_CURVE_WITH_KNOTS ( 'NONE', 3,
 ( #4849, #87281, #66549, #4396, #31880, #80514, #25559, #81844, #46717, #59337 ),
 .UNSPECIFIED., .F., .F.,
 ( 4, 2, 2, 2, 4 ),
 ( 0.0007817359430256372700, 0.0009771253907250054306, 0.001172514838424373700, 0.001367904286123741969, 0.001563293733823110021 ),
 .UNSPECIFIED. ) ;
#48828=CARTESIAN_POINT ( 'NONE',  ( -13.44988583057615905, -10.21337939537584383, 33.94971097300158647 ) ) ;
#48829=ORIENTED_EDGE ( 'NONE', *, *, #44859, .T. ) ;
#48830=EDGE_CURVE ( 'NONE', #84649, #45729, #39665, .T. ) ;
#48831=LINE ( 'NONE', #76305, #20419 ) ;
#48832=CARTESIAN_POINT ( 'NONE',  ( 15.45354889974729318, -3.563462043263030399, 33.22394488606062879 ) ) ;
#48833=CARTESIAN_POINT ( 'NONE',  ( 11.60452988946397745, -10.51840700105979565, 33.73612834413962247 ) ) ;
#48834=CARTESIAN_POINT ( 'NONE',  ( 3.100621261037537213, -8.630895178749536711, 34.87696386517710323 ) ) ;
#48835=CARTESIAN_POINT ( 'NONE',  ( -3.007342831854442622, -7.630147987733843173, 34.99859428049665411 ) ) ;
#48837=AXIS2_PLACEMENT_3D ( 'NONE', #42118, #62795, #69571 ) ;
#48838=VERTEX_POINT ( 'NONE', #77308 ) ;
#48839=VECTOR ( 'NONE', #5726, 1000.000000000000114 ) ;
#48840=ORIENTED_EDGE ( 'NONE', *, *, #31373, .F. ) ;
#48841=ORIENTED_EDGE ( 'NONE', *, *, #57622, .T. ) ;
#48842=EDGE_LOOP ( 'NONE', ( #39340, #23518, #8451, #5956 ) ) ;
#48843=DIRECTION ( 'NONE',  ( -0.000000000000000000, -0.7660444431189791237, -0.6427876096865379196 ) ) ;
#48844=CARTESIAN_POINT ( 'NONE',  ( 4.946775867484856093, -10.88202310037935661, 33.43294751532457099 ) ) ;
#48845=EDGE_CURVE ( 'NONE', #37408, #66547, #3085, .T. ) ;
#48847=CARTESIAN_POINT ( 'NONE',  ( 16.82694633287448838, -10.06842814019191401, 34.32929386961144758 ) ) ;
#48849=DIRECTION ( 'NONE',  ( -0.000000000000000000, -0.3420201433256694901, -0.9396926207859082059 ) ) ;
#48850=ORIENTED_EDGE ( 'NONE', *, *, #11291, .T. ) ;
#48852=EDGE_LOOP ( 'NONE', ( #87047, #43690, #71898, #72718 ) ) ;
#48853=CARTESIAN_POINT ( 'NONE',  ( 4.284636594813105326, -3.957578996910242619, 33.62503395064540257 ) ) ;
#48854=EDGE_CURVE ( 'NONE', #87106, #63890, #13793, .T. ) ;
#48855=VERTEX_POINT ( 'NONE', #43082 ) ;
#48857=CARTESIAN_POINT ( 'NONE',  ( -10.39260494640654819, -6.717445702608402236, 34.94155399931962336 ) ) ;
#48858=CYLINDRICAL_SURFACE ( 'NONE', #17269, 0.2499999999999994726 ) ;
#48859=B_SPLINE_CURVE_WITH_KNOTS ( 'NONE', 3,
 ( #40707, #26735, #7360, #5580, #81249, #19535, #34815, #34373, #19972, #61392 ),
 .UNSPECIFIED., .F., .F.,
 ( 4, 2, 2, 2, 4 ),
 ( 0.000000000000000000, 0.0001954339857564080707, 0.0003908679715128161414, 0.0005863019572692241849, 0.0007817359430256322827 ),
 .UNSPECIFIED. ) ;
#48861=ORIENTED_EDGE ( 'NONE', *, *, #1243, .T. ) ;
#48862=EDGE_CURVE ( 'NONE', #74896, #19448, #22801, .T. ) ;
#48863=ADVANCED_FACE ( 'NONE', ( #64223 ), #2521, .F. ) ;
#48866=CARTESIAN_POINT ( 'NONE',  ( 5.206970512173528576, -7.723484941389743952, 34.99544897038808955 ) ) ;
#48867=ORIENTED_EDGE ( 'NONE', *, *, #81144, .F. ) ;
#48868=FACE_BOUND ( 'NONE', #23168, .T. ) ;
#48869=CARTESIAN_POINT ( 'NONE',  ( 3.296024370282069071, -2.657715359629131857, 31.77849191805844242 ) ) ;
#48872=CARTESIAN_POINT ( 'NONE',  ( 0.5276057948885366500, -8.164416787775445883, 34.95778746994558617 ) ) ;
#48873=CARTESIAN_POINT ( 'NONE',  ( -16.02305571287920571, -12.62708834333097663, 30.88030960425256310 ) ) ;
#48874=DIRECTION ( 'NONE',  ( 1.000000000000000000, 0.000000000000000000, 0.000000000000000000 ) ) ;
#48875=CARTESIAN_POINT ( 'NONE',  ( 0.4615384615383396616, -6.879047030192662504, 34.71129190930017927 ) ) ;
#48876=CYLINDRICAL_SURFACE ( 'NONE', #13561, 0.2500000000000004996 ) ;
#48878=ORIENTED_EDGE ( 'NONE', *, *, #26903, .T. ) ;
#48879=CARTESIAN_POINT ( 'NONE',  ( -0.3963936808188295857, -7.750023224968865421, 34.99404313364389907 ) ) ;
#48880=CARTESIAN_POINT ( 'NONE',  ( 1.384615384615386802, -3.937682226553329556, 33.60647404775216529 ) ) ;
#48881=CARTESIAN_POINT ( 'NONE',  ( -6.223484943723947893, -5.912607949931405038, 34.49155766932282319 ) ) ;
#48882=CYLINDRICAL_SURFACE ( 'NONE', #48635, 0.2500000000000009437 ) ;
#48883=EDGE_CURVE ( 'NONE', #64502, #86296, #6634, .T. ) ;
#48885=EDGE_CURVE ( 'NONE', #81622, #47387, #44259, .T. ) ;
#48886=FACE_BOUND ( 'NONE', #67804, .T. ) ;
#48887=CARTESIAN_POINT ( 'NONE',  ( 17.29993442853592711, -3.587049720035815348, 32.86302985866382897 ) ) ;
#48888=CARTESIAN_POINT ( 'NONE',  ( 7.846153846153846700, -13.63283147151868846, 33.57946703557072254 ) ) ;
#48889=CARTESIAN_POINT ( 'NONE',  ( 5.076923076922953193, -9.528491918059723176, 34.59228464037033035 ) ) ;
#48890=CARTESIAN_POINT ( 'NONE',  ( 3.480769230769167333, -7.565270445406050648, 34.75000000000000000 ) ) ;
#48891=CARTESIAN_POINT ( 'NONE',  ( -18.06608237936013239, -2.833524468853756861, 32.15551576947925838 ) ) ;
#48892=CARTESIAN_POINT ( 'NONE',  ( -5.326899820971668476, -12.41104346484419452, 31.60698883733904196 ) ) ;
#48894=EDGE_CURVE ( 'NONE', #44944, #24055, #10947, .T. ) ;
#48895=EDGE_LOOP ( 'NONE', ( #86138, #8758 ) ) ;
#48897=EDGE_LOOP ( 'NONE', ( #31452, #31445, #27661, #62989 ) ) ;
#48898=AXIS2_PLACEMENT_3D ( 'NONE', #36376, #87682, #18767 ) ;
#48899=CARTESIAN_POINT ( 'NONE',  ( -15.16551365949320562, -4.481592998940250538, 33.73612834413965089 ) ) ;
#48900=VERTEX_POINT ( 'NONE', #38097 ) ;
#48902=CARTESIAN_POINT ( 'NONE',  ( -16.15384615384627409, -12.16647553114689728, 32.15551576947799362 ) ) ;
#48904=CARTESIAN_POINT ( 'NONE',  ( -15.48074596171158390, -4.943428324936578910, 34.04746400365624481 ) ) ;
#48906=B_SPLINE_CURVE_WITH_KNOTS ( 'NONE', 3,
 ( #64947, #59085, #79817, #37936, #52325, #3253, #45125, #18116, #65399, #9569 ),
 .UNSPECIFIED., .F., .F.,
 ( 4, 2, 2, 2, 4 ),
 ( 0.000000000000000000, 0.0001954311564186860613, 0.0003908623128373721225, 0.0005862934692560581567, 0.0007817246256747442451 ),
 .UNSPECIFIED. ) ;
#48908=CARTESIAN_POINT ( 'NONE',  ( -10.61538461538461320, -12.62096338111211580, 30.90682066428153263 ) ) ;
#48909=CARTESIAN_POINT ( 'NONE',  ( -5.207614543590635137, -4.809359713505814149, 33.96456829005828837 ) ) ;
#48911=CARTESIAN_POINT ( 'NONE',  ( -17.74999999976641973, -2.249999999999989786, 29.74999979494859303 ) ) ;
#48912=DIRECTION ( 'NONE',  ( -0.000000000000000000, 0.5000000000000011102, -0.8660254037844380415 ) ) ;
#48913=CARTESIAN_POINT ( 'NONE',  ( -5.076923076923075762, -4.945431358278436385, 36.03766855953609394 ) ) ;
#48914=FACE_OUTER_BOUND ( 'NONE', #44703, .T. ) ;
#48916=CARTESIAN_POINT ( 'NONE',  ( 11.53846153846141576, -5.941354392335915335, 34.76329471203413846 ) ) ;
#48918=VERTEX_POINT ( 'NONE', #18277 ) ;
#48919=CARTESIAN_POINT ( 'NONE',  ( 2.307692307692309264, -9.584722331328613620, 36.20867863119891439 ) ) ;
#48921=EDGE_CURVE ( 'NONE', #15863, #88652, #75399, .T. ) ;
#48922=LINE ( 'NONE', #42618, #40407 ) ;
#48923=CARTESIAN_POINT ( 'NONE',  ( -9.469296340694842939, -11.24521262558773493, 33.06293181088029343 ) ) ;
#48924=ORIENTED_EDGE ( 'NONE', *, *, #36555, .T. ) ;
#48925=CARTESIAN_POINT ( 'NONE',  ( 18.00000000000000000, -13.53365097954675988, 30.81389545987213552 ) ) ;
#48927=CARTESIAN_POINT ( 'NONE',  ( 2.242421861731534349, -2.892918686051582533, 31.69288490824015270 ) ) ;
#48928=VERTEX_POINT ( 'NONE', #11075 ) ;
#48929=CARTESIAN_POINT ( 'NONE',  ( -5.326946314216043810, -5.851115903089112003, 34.47074536777953568 ) ) ;
#48931=CYLINDRICAL_SURFACE ( 'NONE', #8321, 0.2499999999999994726 ) ;
#48932=EDGE_CURVE ( 'NONE', #74896, #78895, #23840, .T. ) ;
#48933=DIRECTION ( 'NONE',  ( -0.000000000000000000, 0.6427876096865404731, -0.7660444431189770143 ) ) ;
#48934=CARTESIAN_POINT ( 'NONE',  ( -15.23076923076922995, -13.20930481340135110, 34.54067556320372745 ) ) ;
#48935=ORIENTED_EDGE ( 'NONE', *, *, #13976, .T. ) ;
#48936=DIRECTION ( 'NONE',  ( 0.000000000000000000, 0.9848077530122072432, -0.1736481776669354937 ) ) ;
#48939=FACE_OUTER_BOUND ( 'NONE', #30169, .T. ) ;
#48940=CARTESIAN_POINT ( 'NONE',  ( -4.153846153846152411, -5.415277668671390821, 36.20867863119892149 ) ) ;
#48945=CARTESIAN_POINT ( 'NONE',  ( 17.14299041027315695, -11.35647404775217595, 33.31231777344667222 ) ) ;
#48946=ORIENTED_EDGE ( 'NONE', *, *, #57199, .F. ) ;
#48947=ORIENTED_EDGE ( 'NONE', *, *, #20852, .T. ) ;
#48948=VECTOR ( 'NONE', #77825, 1000.000000000000000 ) ;
#48949=EDGE_LOOP ( 'NONE', ( #40969, #87992, #71336, #26819 ) ) ;
#48950=CARTESIAN_POINT ( 'NONE',  ( -15.45425417449318140, -12.24155766932282496, 31.33739205006857986 ) ) ;
#48951=ORIENTED_EDGE ( 'NONE', *, *, #8682, .T. ) ;
#48952=CARTESIAN_POINT ( 'NONE',  ( -0.6844646790546093928, -4.887634598454295265, 34.01352882383564946 ) ) ;
#48953=B_SPLINE_CURVE_WITH_KNOTS ( 'NONE', 3,
 ( #20973, #15566, #274, #27740, #61518, #49350 ),
 .UNSPECIFIED., .F., .F.,
 ( 4, 2, 4 ),
 ( 0.0003909569690057822190, 0.0005862646681846078733, 0.0007815723673634334193 ),
 .UNSPECIFIED. ) ;
#48954=CARTESIAN_POINT ( 'NONE',  ( 15.23076923076923173, -2.499999999999998668, 29.75000000000001421 ) ) ;
#48955=VECTOR ( 'NONE', #48343, 1000.000000000000227 ) ;
#48956=VECTOR ( 'NONE', #63600, 1000.000000000000114 ) ;
#48957=CARTESIAN_POINT ( 'NONE',  ( -9.757578138268467427, -8.613356846314824011, 34.62446782046655613 ) ) ;
#48958=EDGE_CURVE ( 'NONE', #86398, #42183, #68844, .T. ) ;
#48959=CARTESIAN_POINT ( 'NONE',  ( 2.307692307692309264, -10.89733346790207413, 36.13435417666054406 ) ) ;
#48960=ORIENTED_EDGE ( 'NONE', *, *, #49208, .T. ) ;
#48961=EDGE_CURVE ( 'NONE', #61992, #52419, #59701, .T. ) ;
#48962=VECTOR ( 'NONE', #37263, 1000.000000000000000 ) ;
#48963=VERTEX_POINT ( 'NONE', #9736 ) ;
#48964=VECTOR ( 'NONE', #75907, 1000.000000000000000 ) ;
#48966=CARTESIAN_POINT ( 'NONE',  ( -6.857009589726848375, -2.833524468853757750, 32.15551576947925838 ) ) ;
#48967=CARTESIAN_POINT ( 'NONE',  ( 1.384615384615386802, -8.120952969808772792, 34.71129190930000163 ) ) ;
#48968=ORIENTED_EDGE ( 'NONE', *, *, #37975, .F. ) ;
#48971=CARTESIAN_POINT ( 'NONE',  ( -14.30769230769242739, -2.625532179533778709, 30.86335684631627174 ) ) ;
#48972=ORIENTED_EDGE ( 'NONE', *, *, #60439, .T. ) ;
#48973=EDGE_CURVE ( 'NONE', #63168, #18413, #56082, .T. ) ;
#48975=CARTESIAN_POINT ( 'NONE',  ( 9.692307692307695177, -8.164416787775445883, 34.95778746994557906 ) ) ;
#48976=EDGE_LOOP ( 'NONE', ( #24491, #18142 ) ) ;
#48977=FACE_BOUND ( 'NONE', #54065, .T. ) ;
#48978=CARTESIAN_POINT ( 'NONE',  ( -11.76194646302586655, -11.60425143139329940, 33.02411095842164457 ) ) ;
#48979=CARTESIAN_POINT ( 'NONE',  ( 8.769230769230768274, -1.790695186598648903, 34.54067556320373455 ) ) ;
#48981=CARTESIAN_POINT ( 'NONE',  ( 8.096208266067295156, -10.82426656108012075, 33.81400080652039009 ) ) ;
#48982=DIRECTION ( 'NONE',  ( 0.000000000000000000, 0.7660444431189807890, 0.6427876096865361433 ) ) ;
#48983=CARTESIAN_POINT ( 'NONE',  ( -3.164701897419155419, -3.322132147404559976, 32.92929555188717927 ) ) ;
#48984=CARTESIAN_POINT ( 'NONE',  ( 18.22277954126840527, -2.847695495035524882, 31.58253572463339154 ) ) ;
#48985=ORIENTED_EDGE ( 'NONE', *, *, #78684, .F. ) ;
#48986=CARTESIAN_POINT ( 'NONE',  ( -7.976301815885541657, -6.809168938359901446, 34.95455904226513866 ) ) ;
#48987=CARTESIAN_POINT ( 'NONE',  ( 5.076923076923075762, -9.780366693483667717, 34.19971097300155094 ) ) ;
#48988=ORIENTED_EDGE ( 'NONE', *, *, #1561, .F. ) ;
#48989=CARTESIAN_POINT ( 'NONE',  ( 8.769230769230768274, -11.11383981884818262, 36.00935417666054406 ) ) ;
#48990=CARTESIAN_POINT ( 'NONE',  ( -4.219928533206287469, -3.322132147404559976, 32.92929555188719348 ) ) ;
#48991=ORIENTED_EDGE ( 'NONE', *, *, #74577, .T. ) ;
#48992=CARTESIAN_POINT ( 'NONE',  ( 11.47319153790521717, -10.33852847137145048, 34.16647553114627556 ) ) ;
#48993=ADVANCED_FACE ( 'NONE', ( #87642 ), #27248, .F. ) ;
#48994=CARTESIAN_POINT ( 'NONE',  ( 4.376625695114559456, -10.11255958852955672, 34.01340905677048454 ) ) ;
#48995=FACE_BOUND ( 'NONE', #1201, .T. ) ;
#48996=CARTESIAN_POINT ( 'NONE',  ( -1.384615384615383471, -6.343179335718451384, 34.87096338111211935 ) ) ;
#48997=CARTESIAN_POINT ( 'NONE',  ( -17.01085472592063397, -12.37446782046654192, 30.86335684631486842 ) ) ;
#48998=CARTESIAN_POINT ( 'NONE',  ( 3.296024802045254720, -8.613356846314928816, 34.62446782046653482 ) ) ;
#48999=B_SPLINE_CURVE_WITH_KNOTS ( 'NONE', 3,
 ( #11264, #22995, #10378, #51321, #38737, #38293, #71179, #9482, #36947, #64410 ),
 .UNSPECIFIED., .F., .F.,
 ( 4, 2, 2, 2, 4 ),
 ( 0.000000000000000000, 0.0001954339857564073388, 0.0003908679715128146777, 0.0005863019572692220165, 0.0007817359430256293554 ),
 .UNSPECIFIED. ) ;
#49000=CARTESIAN_POINT ( 'NONE',  ( 12.23805353697412812, -12.47654668319379567, 31.42292124445336654 ) ) ;
#49001=DIRECTION ( 'NONE',  ( 0.000000000000000000, 0.1736481776669267785, -0.9848077530122087975 ) ) ;
#49002=CARTESIAN_POINT ( 'NONE',  ( -12.68502340526241312, -4.386631170607603991, 33.66268669641500111 ) ) ;
#49003=VECTOR ( 'NONE', #79488, 999.9999999999998863 ) ;
#49004=CYLINDRICAL_SURFACE ( 'NONE', #53345, 0.2500000000000004996 ) ;
#49006=EDGE_LOOP ( 'NONE', ( #69807, #80276, #25390, #6827 ) ) ;
#49007=ORIENTED_EDGE ( 'NONE', *, *, #35770, .T. ) ;
#49008=CARTESIAN_POINT ( 'NONE',  ( -9.822455662039388358, -2.373036134822904319, 30.88089517874952250 ) ) ;
#49009=CARTESIAN_POINT ( 'NONE',  ( 14.43821774592595197, -12.70449254468099198, 30.44128974285582956 ) ) ;
#49010=CARTESIAN_POINT ( 'NONE',  ( 7.146040057343598484, -7.369474539155828730, 34.99858011523957657 ) ) ;
#49011=DIRECTION ( 'NONE',  ( -0.000000000000000000, -0.9396926207859093161, -0.3420201433256663259 ) ) ;
#49012=CARTESIAN_POINT ( 'NONE',  ( -13.38461538461538325, -2.486705287966279876, 31.30864560766543647 ) ) ;
#49014=CARTESIAN_POINT ( 'NONE',  ( -17.07692307692307665, -9.819645486525091727, 36.12317359536749706 ) ) ;
#49015=CARTESIAN_POINT ( 'NONE',  ( 4.088576153289833037, -12.16647553114622049, 32.15551576947930812 ) ) ;
#49016=CARTESIAN_POINT ( 'NONE',  ( 6.249945409378045547, -4.176053281294514363, 33.81426240980091791 ) ) ;
#49017=CARTESIAN_POINT ( 'NONE',  ( -18.00000000000000000, -2.724637637897661335, 35.44105525097462106 ) ) ;
#49019=CARTESIAN_POINT ( 'NONE',  ( 16.40379167219429490, -5.057305518903949526, 34.11320923018887896 ) ) ;
#49020=FACE_OUTER_BOUND ( 'NONE', #76431, .T. ) ;
#49021=CARTESIAN_POINT ( 'NONE',  ( 12.68455130563185662, -2.308499170217967134, 30.53291367094873721 ) ) ;
#49022=AXIS2_PLACEMENT_3D ( 'NONE', #61172, #33278, #46339 ) ;
#49023=DIRECTION ( 'NONE',  ( -0.000000000000000000, 0.9848077530122086864, -0.1736481776669273891 ) ) ;
#49024=ORIENTED_EDGE ( 'NONE', *, *, #66033, .F. ) ;
#49028=VECTOR ( 'NONE', #85546, 1000.000000000000114 ) ;
#49029=CARTESIAN_POINT ( 'NONE',  ( 4.153846153846154188, -4.661471528628507777, 34.16647553114623292 ) ) ;
#49030=LINE ( 'NONE', #70635, #64870 ) ;
#49031=VERTEX_POINT ( 'NONE', #25919 ) ;
#49032=CARTESIAN_POINT ( 'NONE',  ( -7.053224892808621860, -3.069018819979302926, 32.56621877034667278 ) ) ;
#49033=CARTESIAN_POINT ( 'NONE',  ( -3.230769230769229949, -1.422936976036506707, 30.56769352161908415 ) ) ;
#49036=CARTESIAN_POINT ( 'NONE',  ( -9.692307692307691624, -5.471508081941601098, 34.59228464037088457 ) ) ;
#49037=ORIENTED_EDGE ( 'NONE', *, *, #5391, .T. ) ;
#49038=CARTESIAN_POINT ( 'NONE',  ( 14.30769230769231015, -1.790695186598648903, 34.54067556320373455 ) ) ;
#49039=CARTESIAN_POINT ( 'NONE',  ( 10.74617505635156789, -10.70102852606553157, 33.91149625220312913 ) ) ;
#49042=CARTESIAN_POINT ( 'NONE',  ( -11.66860950819323861, -12.50552854090298993, 31.33409797877408920 ) ) ;
#49043=CARTESIAN_POINT ( 'NONE',  ( 9.758375025657768376, -6.343179335718452272, 34.87096338111212646 ) ) ;
#49046=CARTESIAN_POINT ( 'NONE',  ( 15.45354877203763877, -10.81320215134717344, 33.49497208177562868 ) ) ;
#49048=CYLINDRICAL_SURFACE ( 'NONE', #28554, 0.2500000000000009437 ) ;
#49049=CARTESIAN_POINT ( 'NONE',  ( 12.71159277317677549, -9.148310452688876993, 34.47095581063188519 ) ) ;
#49050=CARTESIAN_POINT ( 'NONE',  ( 13.60739505359345181, -3.563462043263030399, 33.22394488606062879 ) ) ;
#49051=CARTESIAN_POINT ( 'NONE',  ( -2.438383774359865974, -5.582088688514999397, 34.36776431015576350 ) ) ;
#49052=CARTESIAN_POINT ( 'NONE',  ( -4.376772371362299019, -6.503392248772476236, 34.64988816332204635 ) ) ;
#49054=CARTESIAN_POINT ( 'NONE',  ( -39.05038313613820122, -2.249999999999998668, 29.75000000000000355 ) ) ;
#49055=AXIS2_PLACEMENT_3D ( 'NONE', #19370, #32442, #45503 ) ;
#49057=ORIENTED_EDGE ( 'NONE', *, *, #74403, .T. ) ;
#49058=FACE_OUTER_BOUND ( 'NONE', #55426, .T. ) ;
#49059=ORIENTED_EDGE ( 'NONE', *, *, #64272, .T. ) ;
#49060=LINE ( 'NONE', #15287, #68120 ) ;
#49062=ORIENTED_EDGE ( 'NONE', *, *, #47261, .F. ) ;
#49063=B_SPLINE_CURVE_WITH_KNOTS ( 'NONE', 3,
 ( #15442, #8686, #36162, #63611, #22624, #15886, #43349, #81472, #54419, #81915 ),
 .UNSPECIFIED., .F., .F.,
 ( 4, 2, 2, 2, 4 ),
 ( 0.0007817359430256315238, 0.0009771253907249980580, 0.001172514838424364592, 0.001367904286123731127, 0.001563293733823097661 ),
 .UNSPECIFIED. ) ;
#49064=FACE_OUTER_BOUND ( 'NONE', #72658, .T. ) ;
#49065=CARTESIAN_POINT ( 'NONE',  ( 6.673100179028331524, -9.234221910056348293, 34.70572697212741531 ) ) ;
#49066=ADVANCED_FACE ( 'NONE', ( #75437 ), #52931, .F. ) ;
#49067=ORIENTED_EDGE ( 'NONE', *, *, #87837, .T. ) ;
#49068=CARTESIAN_POINT ( 'NONE',  ( 10.61538461538461675, -2.499999999999998668, 29.75000000000001421 ) ) ;
#49069=VERTEX_POINT ( 'NONE', #66907 ) ;
#49070=CARTESIAN_POINT ( 'NONE',  ( -4.284537620513712675, -5.582088688514999397, 34.36776431015576350 ) ) ;
#49071=ORIENTED_EDGE ( 'NONE', *, *, #8344, .F. ) ;
#49072=CARTESIAN_POINT ( 'NONE',  ( -12.46153846153846168, -12.29105614889573062, 35.45975837776705220 ) ) ;
#49073=VERTEX_POINT ( 'NONE', #80883 ) ;
#49074=AXIS2_PLACEMENT_3D ( 'NONE', #68718, #41692, #2030 ) ;
#49075=ADVANCED_FACE ( 'NONE', ( #40329 ), #68674, .F. ) ;
#49076=CARTESIAN_POINT ( 'NONE',  ( 15.29683758177167086, -3.050289026998446840, 32.03036669348366416 ) ) ;
#49077=CARTESIAN_POINT ( 'NONE',  ( -8.899921372341074388, -11.93127051446799847, 32.56575433478202797 ) ) ;
#49078=FACE_BOUND ( 'NONE', #43190, .T. ) ;
#49079=DIRECTION ( 'NONE',  ( -0.000000000000000000, 0.8660254037844399289, -0.4999999999999980016 ) ) ;
#49080=CARTESIAN_POINT ( 'NONE',  ( -17.77722045873158407, -12.24180327182771855, 31.33663988360758168 ) ) ;
#49081=CIRCLE ( 'NONE', #21773, 0.2500000000000002220 ) ;
#49082=CARTESIAN_POINT ( 'NONE',  ( 15.36155967173618286, -2.494656445102012565, 31.33466734024120015 ) ) ;
#49084=CARTESIAN_POINT ( 'NONE',  ( -17.29985003582992320, -8.282780595021769443, 34.94152052738834158 ) ) ;
#49085=DIRECTION ( 'NONE',  ( -0.000000000000000000, -0.7660444431189791237, -0.6427876096865379196 ) ) ;
#49086=ORIENTED_EDGE ( 'NONE', *, *, #34256, .T. ) ;
#49088=ORIENTED_EDGE ( 'NONE', *, *, #83394, .T. ) ;
#49089=VERTEX_POINT ( 'NONE', #82201 ) ;
#49090=VECTOR ( 'NONE', #85468, 1000.000000000000227 ) ;
#49091=DIRECTION ( 'NONE',  ( -0.000000000000000000, 0.8660254037844399289, -0.4999999999999980016 ) ) ;
#49092=CARTESIAN_POINT ( 'NONE',  ( 2.307692307692186251, -11.06231777344772027, 33.60647404775119895 ) ) ;
#49093=CARTESIAN_POINT ( 'NONE',  ( -12.68502340526241134, -2.599994579823203367, 30.74605699353653776 ) ) ;
#49094=DIRECTION ( 'NONE',  ( -0.000000000000000000, -0.3420201433256694346, -0.9396926207859080948 ) ) ;
#49095=FACE_OUTER_BOUND ( 'NONE', #83288, .T. ) ;
#49096=LINE ( 'NONE', #48208, #56234 ) ;
#49097=ORIENTED_EDGE ( 'NONE', *, *, #6766, .F. ) ;
#49098=EDGE_CURVE ( 'NONE', #24353, #51788, #6100, .T. ) ;
#49099=CARTESIAN_POINT ( 'NONE',  ( 1.384615384615386802, -9.584722331328613620, 36.20867863119891439 ) ) ;
#49100=CARTESIAN_POINT ( 'NONE',  ( -6.066083410955878996, -6.386643153685125363, 34.62446782046654903 ) ) ;
#49102=EDGE_CURVE ( 'NONE', #59690, #16656, #74278, .T. ) ;
#49103=CARTESIAN_POINT ( 'NONE',  ( -15.23076923076922995, -13.95598074871891292, 31.83374038241031911 ) ) ;
#49104=CARTESIAN_POINT ( 'NONE',  ( 2.438217745925954194, -5.915461855592777596, 34.75538340440931506 ) ) ;
#49105=ORIENTED_EDGE ( 'NONE', *, *, #11258, .T. ) ;
#49106=B_SPLINE_CURVE_WITH_KNOTS ( 'NONE', 3,
 ( #86506, #79736, #24782, #52249, #24165, #8897, #36368, #37233, #44424, #85436 ),
 .UNSPECIFIED., .F., .F.,
 ( 4, 2, 2, 2, 4 ),
 ( 0.000000000000000000, 0.0001954311564186862239, 0.0003908623128373724478, 0.0005862934692560586988, 0.0007817246256747448956 ),
 .UNSPECIFIED. ) ;
#49107=CARTESIAN_POINT ( 'NONE',  ( -4.826923076921656452, -7.500000000000154543, 35.00000000000007105 ) ) ;
#49108=VERTEX_POINT ( 'NONE', #11974 ) ;
#49109=EDGE_CURVE ( 'NONE', #45585, #30008, #12077, .T. ) ;
#49110=VERTEX_POINT ( 'NONE', #60137 ) ;
#49111=EDGE_CURVE ( 'NONE', #33529, #55035, #63572, .T. ) ;
#49112=DIRECTION ( 'NONE',  ( -0.000000000000000000, 0.1736481776669307198, -0.9848077530122080203 ) ) ;
#49113=ORIENTED_EDGE ( 'NONE', *, *, #655, .T. ) ;
#49114=FACE_OUTER_BOUND ( 'NONE', #41129, .T. ) ;
#49115=CARTESIAN_POINT ( 'NONE',  ( -17.30040802064702987, -3.236172620538810385, 32.36188796281389557 ) ) ;
#49116=CARTESIAN_POINT ( 'NONE',  ( 14.05771556364371655, -10.06842814019191401, 34.32929386961144758 ) ) ;
#49117=CARTESIAN_POINT ( 'NONE',  ( 2.307692307692309264, -9.905515769479276145, 34.41647553114623292 ) ) ;
#49118=CARTESIAN_POINT ( 'NONE',  ( -16.82697755857493505, -12.22109172314383052, 31.39792113162168263 ) ) ;
#49119=CARTESIAN_POINT ( 'NONE',  ( 8.769230769230768274, -6.386643153685126251, 34.62446782046654192 ) ) ;
#49120=EDGE_LOOP ( 'NONE', ( #76665, #88749 ) ) ;
#49121=CYLINDRICAL_SURFACE ( 'NONE', #84673, 0.2499999999999998890 ) ;
#49122=FACE_OUTER_BOUND ( 'NONE', #41271, .T. ) ;
#49123=ORIENTED_EDGE ( 'NONE', *, *, #58218, .F. ) ;
#49124=CARTESIAN_POINT ( 'NONE',  ( -3.480769230769241052, -2.499999999999999556, 29.81609845454692120 ) ) ;
#49126=CARTESIAN_POINT ( 'NONE',  ( 17.32686859527121825, -11.37275283266504111, 32.91324779482534524 ) ) ;
#49127=CARTESIAN_POINT ( 'NONE',  ( -3.230769230769351186, -5.219633306517616589, 34.19971097300220464 ) ) ;
#49128=CARTESIAN_POINT ( 'NONE',  ( -17.93393266664992325, -10.67929555188718282, 33.92786785259543336 ) ) ;
#49129=DIRECTION ( 'NONE',  ( -0.000000000000000000, 0.6427876096865404731, -0.7660444431189770143 ) ) ;
#49130=CARTESIAN_POINT ( 'NONE',  ( 18.00000000000000000, -1.367168528481310208, 33.57946703557072254 ) ) ;
#49131=AXIS2_PLACEMENT_3D ( 'NONE', #36618, #57325, #16775 ) ;
#49133=EDGE_LOOP ( 'NONE', ( #38347, #38925, #4185, #65517 ) ) ;
#49134=CARTESIAN_POINT ( 'NONE',  ( -15.36091720050093024, -6.809168938359901446, 34.95455904226513866 ) ) ;
#49135=CARTESIAN_POINT ( 'NONE',  ( 1.253924781505078689, -9.084618155246140248, 34.75535874321725771 ) ) ;
#49136=B_SPLINE_CURVE_WITH_KNOTS ( 'NONE', 3,
 ( #26730, #19529, #83012, #69049, #75367, #54190, #82582, #34368, #7356, #76239 ),
 .UNSPECIFIED., .F., .F.,
 ( 4, 2, 2, 2, 4 ),
 ( 0.000000000000000000, 0.0001954311564186867389, 0.0003908623128373734778, 0.0005862934692560602167, 0.0007817246256747469556 ),
 .UNSPECIFIED. ) ;
#49137=CARTESIAN_POINT ( 'NONE',  ( 7.911409417429874580, -2.625532179533470512, 30.86335684631491105 ) ) ;
#49138=CARTESIAN_POINT ( 'NONE',  ( 13.38461538461538680, -2.499999999999998668, 29.50000000000001066 ) ) ;
#49139=VERTEX_POINT ( 'NONE', #88102 ) ;
#49141=CARTESIAN_POINT ( 'NONE',  ( 1.384615384615386802, -9.780366693483667717, 34.19971097300155094 ) ) ;
#49142=CARTESIAN_POINT ( 'NONE',  ( -0.5268084620947806052, -12.70778746994557551, 30.41441678777548319 ) ) ;
#49143=CARTESIAN_POINT ( 'NONE',  ( 2.980769230769232170, -7.500000000000001776, 35.04278698407183867 ) ) ;
#49144=ORIENTED_EDGE ( 'NONE', *, *, #62026, .T. ) ;
#49145=EDGE_CURVE ( 'NONE', #34884, #78839, #19563, .T. ) ;
#49146=CARTESIAN_POINT ( 'NONE',  ( 6.066068351002440906, -5.557115091759786019, 34.35708131394839882 ) ) ;
#49147=DIRECTION ( 'NONE',  ( -0.000000000000000000, 1.000000000000000000, -0.000000000000000000 ) ) ;
#49148=CARTESIAN_POINT ( 'NONE',  ( 4.153846153846032507, -2.625532179533778709, 30.86335684631627174 ) ) ;
#49149=ORIENTED_EDGE ( 'NONE', *, *, #73577, .T. ) ;
#49150=CARTESIAN_POINT ( 'NONE',  ( -13.16183571563731647, -3.020022701398813236, 32.48759521482552515 ) ) ;
#49151=VECTOR ( 'NONE', #20077, 1000.000000000000114 ) ;
#49152=EDGE_LOOP ( 'NONE', ( #69005, #7856 ) ) ;
#49153=CARTESIAN_POINT ( 'NONE',  ( -16.37733109757010652, -5.912607949931405038, 34.49155766932282319 ) ) ;
#49154=DIRECTION ( 'NONE',  ( -0.000000000000000000, -0.5000000000000009992, -0.8660254037844380415 ) ) ;
#49155=ORIENTED_EDGE ( 'NONE', *, *, #67473, .F. ) ;
#49156=CARTESIAN_POINT ( 'NONE',  ( 10.86533002476265786, -11.56426240980093745, 33.07394671870546432 ) ) ;
#49157=DIRECTION ( 'NONE',  ( -1.000000000000000000, 0.000000000000000000, 0.000000000000000000 ) ) ;
#49158=CARTESIAN_POINT ( 'NONE',  ( 0.3954550505825801254, -4.098570777380720287, 33.41473453929635440 ) ) ;
#49159=VECTOR ( 'NONE', #89165, 1000.000000000000227 ) ;
#49160=EDGE_CURVE ( 'NONE', #7198, #31425, #54967, .T. ) ;
#49161=CARTESIAN_POINT ( 'NONE',  ( 17.07692307692307665, -10.51840700105979565, 33.73612834413961536 ) ) ;
#49162=CARTESIAN_POINT ( 'NONE',  ( -18.06608341095587278, -4.098570777380720287, 33.41473453929634019 ) ) ;
#49163=B_SPLINE_CURVE_WITH_KNOTS ( 'NONE', 3,
 ( #56090, #68276, #68719, #27289, #264, #61954, #82242, #61071, #75473, #1147 ),
 .UNSPECIFIED., .F., .F.,
 ( 4, 2, 2, 2, 4 ),
 ( 0.000000000000000000, 0.0001954311564186887718, 0.0003908623128373775435, 0.0005862934692560662882, 0.0007817246256747550871 ),
 .UNSPECIFIED. ) ;
#49164=B_SPLINE_CURVE_WITH_KNOTS ( 'NONE', 3,
 ( #19486, #47394, #21252, #27575, #46948, #6857, #54592, #82970, #13616, #26689 ),
 .UNSPECIFIED., .F., .F.,
 ( 4, 2, 2, 2, 4 ),
 ( 0.000000000000000000, 0.0001954311564186869557, 0.0003908623128373739115, 0.0005862934692560608672, 0.0007817246256747478229 ),
 .UNSPECIFIED. ) ;
#49165=EDGE_LOOP ( 'NONE', ( #21587, #17560, #56832, #24355 ) ) ;
#49166=ORIENTED_EDGE ( 'NONE', *, *, #66406, .F. ) ;
#49167=FACE_BOUND ( 'NONE', #50136, .T. ) ;
#49168=EDGE_LOOP ( 'NONE', ( #62842, #7655, #34347, #21098 ) ) ;
#49169=CARTESIAN_POINT ( 'NONE',  ( 8.519207531937803779, -3.711651800289232028, 33.01384336483936011 ) ) ;
#49170=EDGE_CURVE ( 'NONE', #88377, #41347, #62351, .T. ) ;
#49171=FACE_OUTER_BOUND ( 'NONE', #33202, .T. ) ;
#49172=CARTESIAN_POINT ( 'NONE',  ( 6.222779668978062340, -3.020022701398814569, 32.48759521482552515 ) ) ;
#49173=CARTESIAN_POINT ( 'NONE',  ( 5.076923076922954969, -4.481592998941358097, 33.73612834414048933 ) ) ;
#49174=EDGE_CURVE ( 'NONE', #2875, #53698, #61910, .T. ) ;
#49176=EDGE_LOOP ( 'NONE', ( #71256, #48946 ) ) ;
#49177=EDGE_LOOP ( 'NONE', ( #46550, #43079, #86776, #41207 ) ) ;
#49178=B_SPLINE_CURVE_WITH_KNOTS ( 'NONE', 3,
 ( #85907, #10692, #44450, #51646, #25539, #85462, #45352, #79148, #18337, #17449 ),
 .UNSPECIFIED., .F., .F.,
 ( 4, 2, 2, 2, 4 ),
 ( 0.0007817246256747469556, 0.0009771112852218902852, 0.001172497944769033615, 0.001367884604316176728, 0.001563271263863320057 ),
 .UNSPECIFIED. ) ;
#49180=CARTESIAN_POINT ( 'NONE',  ( -0.3310127597748959705, -3.285477652293412820, 32.44071101563363158 ) ) ;
#49181=ORIENTED_EDGE ( 'NONE', *, *, #88466, .T. ) ;
#49182=EDGE_CURVE ( 'NONE', #38219, #36959, #69562, .T. ) ;
#49183=CARTESIAN_POINT ( 'NONE',  ( -13.38461538461538325, -1.790695186598648903, 34.54067556320373455 ) ) ;
#49184=CARTESIAN_POINT ( 'NONE',  ( -6.673076923076923350, -2.249999999999998668, 29.75000000000000355 ) ) ;
#49185=CARTESIAN_POINT ( 'NONE',  ( -18.22292695890684655, -6.459968553980840689, 34.89616026154728701 ) ) ;
#49187=CARTESIAN_POINT ( 'NONE',  ( 13.13459214732242408, -10.76384336483936011, 33.53834819971076087 ) ) ;
#49188=EDGE_CURVE ( 'NONE', #18436, #44265, #34548, .T. ) ;
#49190=DIRECTION ( 'NONE',  ( -0.000000000000000000, 1.000000000000000000, 3.491481338843133355E-15 ) ) ;
#49191=CARTESIAN_POINT ( 'NONE',  ( -11.76194648218548444, -3.236172620538810385, 32.36188796281390267 ) ) ;
#49193=ADVANCED_FACE ( 'NONE', ( #21820 ), #35332, .F. ) ;
#49194=B_SPLINE_CURVE_WITH_KNOTS ( 'NONE', 3,
 ( #80344, #4676, #10989, #58270, #65020, #65480, #78544, #16848, #59163, #17748 ),
 .UNSPECIFIED., .F., .F.,
 ( 4, 2, 2, 2, 4 ),
 ( 0.0007817246256747524850, 0.0009771112852218967904, 0.001172497944769040987, 0.001367884604316185184, 0.001563271263863329381 ),
 .UNSPECIFIED. ) ;
#49195=ORIENTED_EDGE ( 'NONE', *, *, #39995, .T. ) ;
#49196=B_SPLINE_CURVE_WITH_KNOTS ( 'NONE', 3,
 ( #23259, #77326, #43098, #43534, #70574, #78208, #8877, #71443, #36346, #22819 ),
 .UNSPECIFIED., .F., .F.,
 ( 4, 2, 2, 2, 4 ),
 ( 0.000000000000000000, 0.0001954339857564093175, 0.0003908679715128186350, 0.0005863019572692279796, 0.0007817359430256372700 ),
 .UNSPECIFIED. ) ;
#49197=ORIENTED_EDGE ( 'NONE', *, *, #13721, .F. ) ;
#49198=CARTESIAN_POINT ( 'NONE',  ( 4.087763774486018242, -2.833524468853757305, 32.15551576947924417 ) ) ;
#49199=B_SPLINE_CURVE_WITH_KNOTS ( 'NONE', 3,
 ( #21143, #33782, #75642, #74331, #41876, #47734, #33345, #27025, #20270, #87870 ),
 .UNSPECIFIED., .F., .F.,
 ( 4, 2, 2, 2, 4 ),
 ( 0.000000000000000000, 0.0001954339857564089923, 0.0003908679715128179845, 0.0005863019572692270039, 0.0007817359430256359690 ),
 .UNSPECIFIED. ) ;
#49201=CARTESIAN_POINT ( 'NONE',  ( 12.46153846153833911, -6.879047030192662504, 34.71129190930017927 ) ) ;
#49202=CARTESIAN_POINT ( 'NONE',  ( 10.86543892702292879, -6.567000820036036579, 34.66262288849541306 ) ) ;
#49203=CARTESIAN_POINT ( 'NONE',  ( 11.40831356872984514, -2.373036134822904319, 30.88089517874952250 ) ) ;
#49204=CARTESIAN_POINT ( 'NONE',  ( -6.923076923076922462, -3.513871655860378418, 32.76840700105978499 ) ) ;
#49205=FACE_BOUND ( 'NONE', #58462, .T. ) ;
#49206=CARTESIAN_POINT ( 'NONE',  ( -0.4615384615384611200, -5.180354513474913603, 36.12317359536750416 ) ) ;
#49207=ORIENTED_EDGE ( 'NONE', *, *, #43182, .F. ) ;
#49208=EDGE_CURVE ( 'NONE', #64959, #81167, #5528, .T. ) ;
#49209=CARTESIAN_POINT ( 'NONE',  ( 17.32697738856138869, -10.66356715214248574, 33.62249196103329751 ) ) ;
#49211=DIRECTION ( 'NONE',  ( -0.000000000000000000, 0.8660254037844397068, -0.4999999999999978906 ) ) ;
#49213=ORIENTED_EDGE ( 'NONE', *, *, #82110, .T. ) ;
#49214=CARTESIAN_POINT ( 'NONE',  ( 6.066067333350078528, -10.67929555188718282, 33.92786785259544757 ) ) ;
#49216=FACE_BOUND ( 'NONE', #66339, .T. ) ;
#49217=CYLINDRICAL_SURFACE ( 'NONE', #84962, 0.2499999999999998890 ) ;
#49218=AXIS2_PLACEMENT_3D ( 'NONE', #56645, #22414, #25075 ) ;
#49220=EDGE_CURVE ( 'NONE', #88554, #64611, #37735, .T. ) ;
#49221=DIRECTION ( 'NONE',  ( -0.000000000000000000, 0.9396926207859093161, -0.3420201433256663259 ) ) ;
#49222=CARTESIAN_POINT ( 'NONE',  ( 14.24160889673642671, -11.69971097300155272, 32.46337939537587403 ) ) ;
#49223=ADVANCED_FACE ( 'NONE', ( #56926 ), #43424, .F. ) ;
#49224=ORIENTED_EDGE ( 'NONE', *, *, #39432, .F. ) ;
#49225=CARTESIAN_POINT ( 'NONE',  ( -14.30769230769230660, -12.37446782046654192, 30.86335684631486131 ) ) ;
#49226=CARTESIAN_POINT ( 'NONE',  ( -3.230769230769229949, -2.292212530054420494, 30.41441678777542634 ) ) ;
#49227=CARTESIAN_POINT ( 'NONE',  ( -14.98082382139118884, -10.18230066228895758, 34.26354781536631577 ) ) ;
#49229=ORIENTED_EDGE ( 'NONE', *, *, #8313, .T. ) ;
#49231=FACE_OUTER_BOUND ( 'NONE', #56382, .T. ) ;
#49233=CARTESIAN_POINT ( 'NONE',  ( 5.999999999999878320, -5.941354392335915335, 34.76329471203413846 ) ) ;
#49235=CARTESIAN_POINT ( 'NONE',  ( 9.468822748583743731, -3.754499324213721234, 33.06261337010820256 ) ) ;
#49236=CYLINDRICAL_SURFACE ( 'NONE', #12524, 0.2500000000000009437 ) ;
#49237=CARTESIAN_POINT ( 'NONE',  ( 13.16168916709923487, -9.086856451489515152, 34.49173150075333183 ) ) ;
#49238=CARTESIAN_POINT ( 'NONE',  ( -10.48485891362104994, -2.619367082507849442, 30.83698974864643461 ) ) ;
#49239=CARTESIAN_POINT ( 'NONE',  ( -4.023320452082590037, -12.45806712695776319, 30.39783852428763922 ) ) ;
#49240=CARTESIAN_POINT ( 'NONE',  ( -8.069080063669987979, -10.61292498521070549, 33.66303323003028680 ) ) ;
#49241=CARTESIAN_POINT ( 'NONE',  ( 8.519254025182180001, -4.075325502946081535, 33.72974371597206300 ) ) ;
#49243=B_SPLINE_CURVE_WITH_KNOTS ( 'NONE', 3,
 ( #33700, #34136, #62480, #795, #82338, #7111, #28260, #40903, #56183, #27387 ),
 .UNSPECIFIED., .F., .F.,
 ( 4, 2, 2, 2, 4 ),
 ( 0.000000000000000000, 0.0001954339857564091278, 0.0003908679715128182556, 0.0005863019572692274375, 0.0007817359430256365111 ),
 .UNSPECIFIED. ) ;
#49245=EDGE_LOOP ( 'NONE', ( #10456, #43201, #88541, #39753 ) ) ;
#49247=EDGE_LOOP ( 'NONE', ( #15510, #33128, #34146, #62581 ) ) ;
#49248=EDGE_CURVE ( 'NONE', #89050, #42119, #50614, .T. ) ;
#49249=ORIENTED_EDGE ( 'NONE', *, *, #77235, .T. ) ;
#49250=CARTESIAN_POINT ( 'NONE',  ( -16.02332071561251325, -6.808710257144159783, 34.95449254468098843 ) ) ;
#49253=B_SPLINE_CURVE_WITH_KNOTS ( 'NONE', 3,
 ( #88304, #19815, #47278, #40102, #32885, #53143, #26574, #54030, #61671, #80647 ),
 .UNSPECIFIED., .F., .F.,
 ( 4, 2, 2, 2, 4 ),
 ( 0.0007817246256747470640, 0.0009771112852218898515, 0.001172497944769032747, 0.001367884604316175643, 0.001563271263863318539 ),
 .UNSPECIFIED. ) ;
#49254=CARTESIAN_POINT ( 'NONE',  ( -2.057746789344163663, -6.696923467548660192, 34.68552623307873972 ) ) ;
#49255=CARTESIAN_POINT ( 'NONE',  ( -6.923076923076922462, -9.058645607665452459, 34.76329471203371924 ) ) ;
#49256=CARTESIAN_POINT ( 'NONE',  ( 10.68145194873469173, -6.343179335718452272, 34.87096338111212646 ) ) ;
#49257=CARTESIAN_POINT ( 'NONE',  ( 1.384615384615386802, -1.790695186598648903, 34.54067556320373455 ) ) ;
#49258=DIRECTION ( 'NONE',  ( -0.000000000000000000, -0.000000000000000000, 1.000000000000000000 ) ) ;
#49259=DIRECTION ( 'NONE',  ( -0.000000000000000000, -0.1736481776669307198, -0.9848077530122080203 ) ) ;
#49260=EDGE_CURVE ( 'NONE', #48900, #58457, #3426, .T. ) ;
#49261=CARTESIAN_POINT ( 'NONE',  ( 6.792386319966614572, -9.929715669179216775, 34.40415004197138416 ) ) ;
#49262=CARTESIAN_POINT ( 'NONE',  ( 1.384615384615386802, -5.180354513474913603, 36.12317359536750416 ) ) ;
#49263=DIRECTION ( 'NONE',  ( 1.000000000000000000, 0.000000000000000000, 0.000000000000000000 ) ) ;
#49264=CARTESIAN_POINT ( 'NONE',  ( 13.38461538461538680, -2.249999999999998668, 29.50000000000001421 ) ) ;
#49266=EDGE_CURVE ( 'NONE', #8131, #68101, #45183, .T. ) ;
#49267=ORIENTED_EDGE ( 'NONE', *, *, #7407, .F. ) ;
#49269=CARTESIAN_POINT ( 'NONE',  ( 3.165499230212911019, -11.06231777344662781, 33.60647404775220082 ) ) ;
#49272=CARTESIAN_POINT ( 'NONE',  ( 0.4615384615384611200, -9.905515769479276145, 34.41647553114623292 ) ) ;
#49273=ORIENTED_EDGE ( 'NONE', *, *, #87534, .F. ) ;
#49274=CARTESIAN_POINT ( 'NONE',  ( -15.93106648486808119, -8.540255544307068902, 34.89611431652622286 ) ) ;
#49275=CARTESIAN_POINT ( 'NONE',  ( 4.153846153846154188, -13.20930481340135110, 34.54067556320372745 ) ) ;
#49277=CARTESIAN_POINT ( 'NONE',  ( 9.019176287578908102, -4.336752205174649433, 33.62275283266504289 ) ) ;
#49278=VERTEX_POINT ( 'NONE', #37094 ) ;
#49279=CARTESIAN_POINT ( 'NONE',  ( -13.60810032833933469, -10.11188796281391511, 34.01382737946119050 ) ) ;
#49282=AXIS2_PLACEMENT_3D ( 'NONE', #67577, #41881, #74334 ) ;
#49283=CARTESIAN_POINT ( 'NONE',  ( -2.307692307692305711, -13.78497067705608181, 32.30358669280327177 ) ) ;
#49284=CARTESIAN_POINT ( 'NONE',  ( 12.39626801557768587, -8.613356846314824011, 34.62446782046655613 ) ) ;
#49285=CARTESIAN_POINT ( 'NONE',  ( 3.164686851409094448, -8.164416787775445883, 34.95778746994557906 ) ) ;
#49286=CARTESIAN_POINT ( 'NONE',  ( -18.00000000000000000, -12.34228464037088635, 31.77849191805839268 ) ) ;
#49287=ADVANCED_FACE ( 'NONE', ( #30784 ), #52383, .F. ) ;
#49288=EDGE_LOOP ( 'NONE', ( #72692, #66298, #85645, #75013 ) ) ;
#49289=EDGE_CURVE ( 'NONE', #25149, #67006, #30239, .T. ) ;
#49290=EDGE_LOOP ( 'NONE', ( #36719, #47907, #55504, #56611 ) ) ;
#49291=EDGE_LOOP ( 'NONE', ( #40493, #73768 ) ) ;
#49292=ORIENTED_EDGE ( 'NONE', *, *, #46483, .F. ) ;
#49293=CARTESIAN_POINT ( 'NONE',  ( -6.130691466667556710, -11.18331474514187995, 33.13161551792790505 ) ) ;
#49294=CARTESIAN_POINT ( 'NONE',  ( 13.38461538461538680, -9.780366693483667717, 34.19971097300155094 ) ) ;
#49295=CARTESIAN_POINT ( 'NONE',  ( 17.20771488474786892, -4.118422570099827595, 33.43335022499816489 ) ) ;
#49296=CARTESIAN_POINT ( 'NONE',  ( 11.31553532094538994, -12.15238873228292071, 31.58232369045353849 ) ) ;
#49297=B_SPLINE_CURVE_WITH_KNOTS ( 'NONE', 3,
 ( #37442, #51374, #3656, #31129, #38346, #65800, #4100, #66252, #32922, #54513 ),
 .UNSPECIFIED., .F., .F.,
 ( 4, 2, 2, 2, 4 ),
 ( 0.000000000000000000, 0.0001954339857564077183, 0.0003908679715128154366, 0.0005863019572692231007, 0.0007817359430256308733 ),
 .UNSPECIFIED. ) ;
#49298=CARTESIAN_POINT ( 'NONE',  ( -10.36538461538319389, -7.500000000000154543, 35.00000000000007105 ) ) ;
#49300=EDGE_LOOP ( 'NONE', ( #45561, #86074, #23378, #73485 ) ) ;
#49301=VERTEX_POINT ( 'NONE', #24919 ) ;
#49302=ORIENTED_EDGE ( 'NONE', *, *, #37463, .F. ) ;
#49303=CARTESIAN_POINT ( 'NONE',  ( 12.71159277317677549, -8.303483539816731707, 34.68545999027711702 ) ) ;
#49304=ORIENTED_EDGE ( 'NONE', *, *, #69002, .T. ) ;
#49305=CIRCLE ( 'NONE', #85315, 0.2500000000000002220 ) ;
#49306=CARTESIAN_POINT ( 'NONE',  ( -16.85414353565466072, -9.332535724633405749, 34.40230450496446224 ) ) ;
#49307=CARTESIAN_POINT ( 'NONE',  ( -5.076923076923199218, -12.70778746994576025, 30.41441678777401236 ) ) ;
#49309=AXIS2_PLACEMENT_3D ( 'NONE', #78653, #17852, #45304 ) ;
#49310=B_SPLINE_CURVE_WITH_KNOTS ( 'NONE', 3,
 ( #43939, #9709, #1637, #37178, #64641, #63765, #56574, #84064, #29552, #86738 ),
 .UNSPECIFIED., .F., .F.,
 ( 4, 2, 2, 2, 4 ),
 ( 0.000000000000000000, 0.0001954339857564063089, 0.0003908679715128126177, 0.0005863019572692189808, 0.0007817359430256252354 ),
 .UNSPECIFIED. ) ;
#49311=CARTESIAN_POINT ( 'NONE',  ( -10.83831083290076158, -11.76352882383564769, 32.36236540154569497 ) ) ;
#49312=EDGE_LOOP ( 'NONE', ( #33658, #82190 ) ) ;
#49313=EDGE_CURVE ( 'NONE', #30501, #48096, #79872, .T. ) ;
#49315=ORIENTED_EDGE ( 'NONE', *, *, #73936, .T. ) ;
#49316=DIRECTION ( 'NONE',  ( 0.000000000000000000, -6.938893903907222067E-15, 1.000000000000000000 ) ) ;
#49317=VERTEX_POINT ( 'NONE', #23146 ) ;
#49318=EDGE_CURVE ( 'NONE', #86922, #72884, #73322, .T. ) ;
#49319=FACE_BOUND ( 'NONE', #7120, .T. ) ;
#49320=CARTESIAN_POINT ( 'NONE',  ( -2.084679463598912097, -4.762714258010882773, 34.23016756924214832 ) ) ;
#49322=ORIENTED_EDGE ( 'NONE', *, *, #15954, .F. ) ;
#49323=CARTESIAN_POINT ( 'NONE',  ( -39.05038313613820122, -2.249999999999998668, 29.75000000000000355 ) ) ;
#49324=CARTESIAN_POINT ( 'NONE',  ( 11.28848479441294650, -6.524016743844655686, 34.90889640711025521 ) ) ;
#49325=EDGE_CURVE ( 'NONE', #9234, #82350, #36773, .T. ) ;
#49326=CARTESIAN_POINT ( 'NONE',  ( 10.55011416942384272, -2.892918686051582533, 31.69288490824015980 ) ) ;
#49327=CARTESIAN_POINT ( 'NONE',  ( -15.36146069743678844, -6.413092428213692742, 34.63065189839063152 ) ) ;
#49328=CARTESIAN_POINT ( 'NONE',  ( -4.153846153846274980, -5.094484230521993062, 34.41647553114689373 ) ) ;
#49329=EDGE_LOOP ( 'NONE', ( #69853, #68781, #45482, #45928 ) ) ;
#49330=EDGE_CURVE ( 'NONE', #86499, #22286, #39994, .T. ) ;
#49331=CARTESIAN_POINT ( 'NONE',  ( -11.53846153846166089, -12.51329471203414379, 31.30864560766407578 ) ) ;
#49332=LINE ( 'NONE', #35824, #38276 ) ;
#49333=DIRECTION ( 'NONE',  ( 0.000000000000000000, 0.6427876096865373645, -0.7660444431189797898 ) ) ;
#49334=CARTESIAN_POINT ( 'NONE',  ( 15.90382292962469890, -10.92453946501459328, 33.72985991061849376 ) ) ;
#49335=FACE_OUTER_BOUND ( 'NONE', #69041, .T. ) ;
#49336=FACE_BOUND ( 'NONE', #28049, .T. ) ;
#49337=B_SPLINE_CURVE_WITH_KNOTS ( 'NONE', 3,
 ( #19820, #54934, #34665, #7195, #75216, #20267, #54482, #32890, #74325, #80651 ),
 .UNSPECIFIED., .F., .F.,
 ( 4, 2, 2, 2, 4 ),
 ( 0.000000000000000000, 0.0001954339857564083688, 0.0003908679715128167377, 0.0005863019572692250523, 0.0007817359430256334753 ),
 .UNSPECIFIED. ) ;
#49338=CYLINDRICAL_SURFACE ( 'NONE', #10258, 0.2499999999999986955 ) ;
#49340=CARTESIAN_POINT ( 'NONE',  ( 5.207448515156721136, -9.503571793651733657, 34.60286762892837942 ) ) ;
#49342=CARTESIAN_POINT ( 'NONE',  ( -5.999999999999998224, -4.786620604624113540, 33.94971097300155094 ) ) ;
#49343=EDGE_CURVE ( 'NONE', #23595, #37993, #66065, .T. ) ;
#49346=ORIENTED_EDGE ( 'NONE', *, *, #59911, .F. ) ;
#49348=CARTESIAN_POINT ( 'NONE',  ( 12.59233026936324684, -2.541949514083464479, 30.39797389878540557 ) ) ;
#49349=ORIENTED_EDGE ( 'NONE', *, *, #69220, .T. ) ;
#49350=CARTESIAN_POINT ( 'NONE',  ( 0.7115384615384606759, -2.499999999999998668, 29.75000000000000355 ) ) ;
#49351=EDGE_CURVE ( 'NONE', #53313, #19610, #76514, .T. ) ;
#49352=VERTEX_POINT ( 'NONE', #4657 ) ;
#49353=CARTESIAN_POINT ( 'NONE',  ( 2.307692307692186251, -12.51329471203414379, 31.30864560766407578 ) ) ;
#49354=CARTESIAN_POINT ( 'NONE',  ( -15.93106648486808119, -12.11081565061823717, 32.26097654155341843 ) ) ;
#49356=CARTESIAN_POINT ( 'NONE',  ( -1.384615384615383471, -13.37000171582298513, 34.34916445242398453 ) ) ;
#49358=CARTESIAN_POINT ( 'NONE',  ( 12.46153846153846168, -4.661471528628507777, 34.16647553114623292 ) ) ;
#49359=CARTESIAN_POINT ( 'NONE',  ( -10.61538461538473577, -12.70778746994576025, 30.41441678777401236 ) ) ;
#49360=CARTESIAN_POINT ( 'NONE',  ( 16.08857615328984281, -8.656820664281497102, 34.87096338111211935 ) ) ;
#49361=CARTESIAN_POINT ( 'NONE',  ( 12.33139125210024112, -2.882441371585227508, 31.66841991370172238 ) ) ;
#49362=CARTESIAN_POINT ( 'NONE',  ( 14.98076923076923173, -7.500000000000001776, 34.75000000000000000 ) ) ;
#49366=CARTESIAN_POINT ( 'NONE',  ( -6.222926958906846551, -3.395401636524186362, 33.02366814457250399 ) ) ;
#49367=CARTESIAN_POINT ( 'NONE',  ( 8.900022577055556994, -9.804649428959608670, 34.18742332936588468 ) ) ;
#49370=CARTESIAN_POINT ( 'NONE',  ( 6.250000000000000888, -2.249999999999998668, 29.75000000000000355 ) ) ;
#49371=ORIENTED_EDGE ( 'NONE', *, *, #2822, .T. ) ;
#49372=CARTESIAN_POINT ( 'NONE',  ( 9.692307692307570832, -2.657715359629662544, 31.77849191805970364 ) ) ;
#49373=FACE_OUTER_BOUND ( 'NONE', #5426, .T. ) ;
#49374=CARTESIAN_POINT ( 'NONE',  ( -11.53846153846153655, -1.790695186598648903, 34.54067556320373455 ) ) ;
#49375=CARTESIAN_POINT ( 'NONE',  ( 10.61538461538461675, -2.249999999999998668, 29.50000000000001421 ) ) ;
#49376=B_SPLINE_CURVE_WITH_KNOTS ( 'NONE', 3,
 ( #88845, #55910, #91, #21686, #49156, #22137, #69876, #83852, #42419, #70320 ),
 .UNSPECIFIED., .F., .F.,
 ( 4, 2, 2, 2, 4 ),
 ( 0.0007817246256747463051, 0.0009771112852218896347, 0.001172497944769033181, 0.001367884604316176728, 0.001563271263863320057 ),
 .UNSPECIFIED. ) ;
#49377=B_SPLINE_CURVE_WITH_KNOTS ( 'NONE', 3,
 ( #28354, #82440, #48184, #41887, #42334, #75233, #68901, #69359, #76998, #15299 ),
 .UNSPECIFIED., .F., .F.,
 ( 4, 2, 2, 2, 4 ),
 ( 0.000000000000000000, 0.0001954311564186858715, 0.0003908623128373717431, 0.0005862934692560576146, 0.0007817246256747434861 ),
 .UNSPECIFIED. ) ;
#49378=CARTESIAN_POINT ( 'NONE',  ( -3.230769230769351186, -5.219633306517616589, 34.19971097300220464 ) ) ;
#49379=CARTESIAN_POINT ( 'NONE',  ( 7.053602361310567836, -12.15418822224088657, 32.17964115625579069 ) ) ;
#49381=VECTOR ( 'NONE', #84543, 1000.000000000000227 ) ;
#49382=CARTESIAN_POINT ( 'NONE',  ( 8.546304551714625219, -10.61292498521070549, 33.66303323003028680 ) ) ;
#49383=DIRECTION ( 'NONE',  ( -0.000000000000000000, -0.5000000000000009992, -0.8660254037844380415 ) ) ;
#49384=EDGE_CURVE ( 'NONE', #85420, #14506, #46355, .T. ) ;
#49386=VERTEX_POINT ( 'NONE', #40668 ) ;
#49388=CARTESIAN_POINT ( 'NONE',  ( 5.299702618191484582, -11.89424750095246175, 32.13594075562311758 ) ) ;
#49389=DIRECTION ( 'NONE',  ( -0.000000000000000000, -0.3420201433256694346, -0.9396926207859080948 ) ) ;
#49390=CARTESIAN_POINT ( 'NONE',  ( -8.992715693795103604, -2.353723527008296568, 30.78948104536958752 ) ) ;
#49393=EDGE_CURVE ( 'NONE', #27552, #88462, #51752, .T. ) ;
#49394=ORIENTED_EDGE ( 'NONE', *, *, #28483, .F. ) ;
#49395=EDGE_CURVE ( 'NONE', #61816, #4310, #78564, .T. ) ;
#49396=CARTESIAN_POINT ( 'NONE',  ( -18.22282669247899989, -7.369208160676171460, 34.74850200257122879 ) ) ;
#49397=EDGE_LOOP ( 'NONE', ( #36363, #63244 ) ) ;
#49398=ADVANCED_FACE ( 'NONE', ( #23360 ), #9853, .F. ) ;
#49399=ORIENTED_EDGE ( 'NONE', *, *, #72574, .F. ) ;
#49401=ORIENTED_EDGE ( 'NONE', *, *, #24604, .F. ) ;
#49402=CARTESIAN_POINT ( 'NONE',  ( 8.519254025182178225, -12.41104346484419452, 31.60698883733904196 ) ) ;
#49403=VERTEX_POINT ( 'NONE', #63010 ) ;
#49404=CARTESIAN_POINT ( 'NONE',  ( -4.854143407945007205, -12.47679350104403007, 31.42216943046555855 ) ) ;
#49405=CARTESIAN_POINT ( 'NONE',  ( -16.21911659980693443, -4.481592998940161721, 33.73612834413957984 ) ) ;
#49406=CIRCLE ( 'NONE', #58015, 0.2500000000000002220 ) ;
#49407=B_SPLINE_CURVE_WITH_KNOTS ( 'NONE', 3,
 ( #86490, #24764, #72954, #66187, #39186, #81059, #5832, #59883, #26551, #80163 ),
 .UNSPECIFIED., .F., .F.,
 ( 4, 2, 2, 2, 4 ),
 ( 0.0007817246256747514008, 0.0009771112852218952725, 0.001172497944769039036, 0.001367884604316182799, 0.001563271263863326779 ),
 .UNSPECIFIED. ) ;
#49408=LINE ( 'NONE', #2526, #36430 ) ;
#49409=CARTESIAN_POINT ( 'NONE',  ( 14.05769230769230838, -7.500000000000001776, 35.00000000000000000 ) ) ;
#49410=ORIENTED_EDGE ( 'NONE', *, *, #11166, .F. ) ;
#49411=B_SPLINE_CURVE_WITH_KNOTS ( 'NONE', 3,
 ( #71283, #11369, #3271, #23540, #86153, #78934, #16354, #31187, #50997, #10031 ),
 .UNSPECIFIED., .F., .F.,
 ( 4, 2, 2, 2, 4 ),
 ( 0.0007817246256747450040, 0.0009771112852218872494, 0.001172497944769029278, 0.001367884604316171523, 0.001563271263863313769 ),
 .UNSPECIFIED. ) ;
#49412=ORIENTED_EDGE ( 'NONE', *, *, #54590, .F. ) ;
#49413=ORIENTED_EDGE ( 'NONE', *, *, #5592, .T. ) ;
#49414=CARTESIAN_POINT ( 'NONE',  ( -9.561515884482904681, -5.582136614379148654, 34.36778462344220486 ) ) ;
#49415=CARTESIAN_POINT ( 'NONE',  ( 11.78851595837499566, -5.642605341092957971, 34.66089969410670335 ) ) ;
#49416=VERTEX_POINT ( 'NONE', #70677 ) ;
#49417=CARTESIAN_POINT ( 'NONE',  ( -4.153846153846152411, -2.499999999999998668, 29.50000000000001066 ) ) ;
#49419=CARTESIAN_POINT ( 'NONE',  ( 7.173131234715236282, -11.79725096376909299, 32.30694842903960762 ) ) ;
#49420=EDGE_LOOP ( 'NONE', ( #87216, #70055, #79912, #31683 ) ) ;
#49421=LINE ( 'NONE', #15635, #78198 ) ;
#49422=CARTESIAN_POINT ( 'NONE',  ( -15.23076923076935252, -12.51329471203414379, 31.30864560766407578 ) ) ;
#49423=EDGE_LOOP ( 'NONE', ( #40166, #776, #22962, #10723 ) ) ;
#49424=FACE_BOUND ( 'NONE', #58574, .T. ) ;
#49425=CARTESIAN_POINT ( 'NONE',  ( 15.45378207486262667, -11.43677907613344757, 33.22367315496202167 ) ) ;
#49426=CARTESIAN_POINT ( 'NONE',  ( -13.38461538461538325, -10.05456864172156806, 36.03766855953608683 ) ) ;
#49427=FACE_OUTER_BOUND ( 'NONE', #12606, .T. ) ;
#49428=FACE_OUTER_BOUND ( 'NONE', #78954, .T. ) ;
#49429=CARTESIAN_POINT ( 'NONE',  ( -0.6844646790546066173, -12.15238873228291538, 31.58232369045354915 ) ) ;
#49430=CARTESIAN_POINT ( 'NONE',  ( -12.46153846153846168, -13.87047571288749737, 32.06866353760679544 ) ) ;
#49431=DIRECTION ( 'NONE',  ( 1.000000000000000000, 0.000000000000000000, 0.000000000000000000 ) ) ;
#49432=ORIENTED_EDGE ( 'NONE', *, *, #67646, .T. ) ;
#49433=CARTESIAN_POINT ( 'NONE',  ( 14.55763782604045176, -12.43552623307873972, 30.55307653245132826 ) ) ;
#49434=CARTESIAN_POINT ( 'NONE',  ( -16.85391023282967993, -6.460100341425561332, 34.89618726649961644 ) ) ;
#49435=ORIENTED_EDGE ( 'NONE', *, *, #54053, .T. ) ;
#49436=AXIS2_PLACEMENT_3D ( 'NONE', #11774, #87909, #68480 ) ;
#49439=DIRECTION ( 'NONE',  ( -0.000000000000000000, -0.000000000000000000, -1.000000000000000000 ) ) ;
#49440=CARTESIAN_POINT ( 'NONE',  ( -7.846153846153844924, -10.67929555188718282, 33.92786785259544047 ) ) ;
#49441=VERTEX_POINT ( 'NONE', #64781 ) ;
#49442=CARTESIAN_POINT ( 'NONE',  ( -0.3307466537136760643, -12.38066358083363738, 30.83685684665853444 ) ) ;
#49443=DIRECTION ( 'NONE',  ( 0.000000000000000000, 0.9396926207859126468, -0.3420201433256571111 ) ) ;
#49444=FACE_BOUND ( 'NONE', #78192, .T. ) ;
#49445=CARTESIAN_POINT ( 'NONE',  ( 8.769230769230768274, -8.120952969808772792, 34.71129190930000163 ) ) ;
#49446=CARTESIAN_POINT ( 'NONE',  ( -3.903900635498011251, -8.433404298154334455, 34.66254593164985920 ) ) ;
#49447=CARTESIAN_POINT ( 'NONE',  ( -16.02305434602136458, -2.541949514083464479, 30.39797389878540557 ) ) ;
#49448=DIRECTION ( 'NONE',  ( -0.000000000000000000, -0.9848077530122085754, -0.1736481776669273613 ) ) ;
#49449=CYLINDRICAL_SURFACE ( 'NONE', #49218, 0.2499999999999997502 ) ;
#49450=EDGE_CURVE ( 'NONE', #54935, #82557, #67897, .T. ) ;
#49451=CARTESIAN_POINT ( 'NONE',  ( -17.77722045873158763, -5.114059244376869984, 34.14424750095245287 ) ) ;
#49454=B_SPLINE_CURVE_WITH_KNOTS ( 'NONE', 3,
 ( #69741, #84161, #35066, #76946, #13909, #22000, #15250, #76503, #28307, #83267 ),
 .UNSPECIFIED., .F., .F.,
 ( 4, 2, 2, 2, 4 ),
 ( 0.000000000000000000, 0.0001954311564186866034, 0.0003908623128373732067, 0.0005862934692560597830, 0.0007817246256747464135 ),
 .UNSPECIFIED. ) ;
#49456=CARTESIAN_POINT ( 'NONE',  ( -9.561515884482904681, -11.71459661697925903, 32.44059661609676937 ) ) ;
#49457=CARTESIAN_POINT ( 'NONE',  ( -12.39628332202562433, -6.835583212224610072, 34.95778746994559327 ) ) ;
#49458=CARTESIAN_POINT ( 'NONE',  ( -9.692307692307812417, -9.442884908241554243, 34.35708131394783038 ) ) ;
#49459=CARTESIAN_POINT ( 'NONE',  ( 8.638670855617402111, -2.254533558242300284, 29.97296025877827930 ) ) ;
#49460=CARTESIAN_POINT ( 'NONE',  ( -17.01085472592063752, -6.386643153685127139, 34.62446782046654192 ) ) ;
#49462=CARTESIAN_POINT ( 'NONE',  ( 6.923076923076800782, -2.379036618888197729, 30.90682066428292885 ) ) ;
#49463=CARTESIAN_POINT ( 'NONE',  ( -39.05038313613820122, -2.249999999999998668, 29.75000000000000355 ) ) ;
#49464=EDGE_CURVE ( 'NONE', #8676, #36288, #79702, .T. ) ;
#49465=FACE_OUTER_BOUND ( 'NONE', #71214, .T. ) ;
#49467=CARTESIAN_POINT ( 'NONE',  ( 5.326923076923075762, -2.499999999999998668, 29.75000000000000355 ) ) ;
#49468=DIRECTION ( 'NONE',  ( -0.000000000000000000, 0.3420201433256694901, -0.9396926207859082059 ) ) ;
#49469=CARTESIAN_POINT ( 'NONE',  ( -5.011667505647052323, -2.892918686051625166, 31.69288490824025928 ) ) ;
#49470=AXIS2_PLACEMENT_3D ( 'NONE', #37399, #85596, #23873 ) ;
#49471=CARTESIAN_POINT ( 'NONE',  ( 10.86538461538455458, -7.565270000091922853, 34.99999999999999289 ) ) ;
#49472=CARTESIAN_POINT ( 'NONE',  ( 3.165498784808455479, -2.625532179533444754, 30.86335684631481513 ) ) ;
#49473=ORIENTED_EDGE ( 'NONE', *, *, #37081, .F. ) ;
#49474=CARTESIAN_POINT ( 'NONE',  ( -14.43838377435986686, -3.530157926970578952, 32.79014554554150607 ) ) ;
#49475=CYLINDRICAL_SURFACE ( 'NONE', #61815, 0.2500000000000008882 ) ;
#49477=EDGE_CURVE ( 'NONE', #1316, #20998, #16192, .T. ) ;
#49478=VECTOR ( 'NONE', #68116, 999.9999999999998863 ) ;
#49480=CARTESIAN_POINT ( 'NONE',  ( 0.4615384615384611200, -3.322132147404559976, 32.92929555188717927 ) ) ;
#49481=CARTESIAN_POINT ( 'NONE',  ( 16.15384615384615330, -4.102666532097928531, 36.13435417666054406 ) ) ;
#49483=LINE ( 'NONE', #69747, #21211 ) ;
#49484=DIRECTION ( 'NONE',  ( -0.000000000000000000, 0.9848077530122085754, -0.1736481776669273613 ) ) ;
#49485=ORIENTED_EDGE ( 'NONE', *, *, #39541, .T. ) ;
#49486=CARTESIAN_POINT ( 'NONE',  ( 2.307692307692623679, -2.255955759149395501, 30.00000000000324363 ) ) ;
#49487=ADVANCED_FACE ( 'NONE', ( #77866 ), #14861, .F. ) ;
#49488=CARTESIAN_POINT ( 'NONE',  ( -2.372962308248626417, -11.06231777344662781, 33.60647404775220082 ) ) ;
#49489=VERTEX_POINT ( 'NONE', #30564 ) ;
#49490=CARTESIAN_POINT ( 'NONE',  ( -13.38461538461538325, -3.513871655860378418, 32.76840700105978499 ) ) ;
#49491=CARTESIAN_POINT ( 'NONE',  ( 10.68063975489745410, -11.06231777344671130, 33.60647404775212976 ) ) ;
#49492=EDGE_LOOP ( 'NONE', ( #44528, #39290, #79856, #11707 ) ) ;
#49493=B_SPLINE_CURVE_WITH_KNOTS ( 'NONE', 3,
 ( #67099, #81506, #39191, #19794, #45481, #80170, #45923, #24769, #52234, #79724 ),
 .UNSPECIFIED., .F., .F.,
 ( 4, 2, 2, 2, 4 ),
 ( 0.0007817359430256401974, 0.0009771253907250091169, 0.001172514838424378036, 0.001367904286123747173, 0.001563293733823116092 ),
 .UNSPECIFIED. ) ;
#49495=CARTESIAN_POINT ( 'NONE',  ( -16.08859058257013075, -3.300289026998475261, 32.46337939537591666 ) ) ;
#49496=EDGE_CURVE ( 'NONE', #48689, #18273, #16173, .T. ) ;
#49498=ORIENTED_EDGE ( 'NONE', *, *, #74428, .F. ) ;
#49499=ORIENTED_EDGE ( 'NONE', *, *, #44686, .T. ) ;
#49500=CARTESIAN_POINT ( 'NONE',  ( 6.250054311638314708, -6.567000820036038355, 34.66262288849541306 ) ) ;
#49501=EDGE_LOOP ( 'NONE', ( #49851, #82985, #53371, #45527, #13856, #49249 ) ) ;
#49502=CARTESIAN_POINT ( 'NONE',  ( -1.253823576790598748, -2.541949514083463590, 30.39797389878540557 ) ) ;
#49503=CARTESIAN_POINT ( 'NONE',  ( 2.438482748659261290, -11.37503395064541678, 33.29242100308974983 ) ) ;
#49504=CARTESIAN_POINT ( 'NONE',  ( -7.596153846153780087, -7.434744429011175271, 34.75000000000000000 ) ) ;
#49505=EDGE_CURVE ( 'NONE', #59888, #10587, #8718, .T. ) ;
#49506=AXIS2_PLACEMENT_3D ( 'NONE', #27962, #22531, #57203 ) ;
#49510=EDGE_LOOP ( 'NONE', ( #74049, #80930, #20834, #23332 ) ) ;
#49511=ORIENTED_EDGE ( 'NONE', *, *, #36260, .F. ) ;
#49512=DIRECTION ( 'NONE',  ( -0.000000000000000000, -0.8660254037844397068, -0.4999999999999978906 ) ) ;
#49514=EDGE_CURVE ( 'NONE', #63322, #11864, #22575, .T. ) ;
#49515=DIRECTION ( 'NONE',  ( -0.000000000000000000, 0.7660444431189791237, -0.6427876096865379196 ) ) ;
#49516=ORIENTED_EDGE ( 'NONE', *, *, #28396, .F. ) ;
#49517=CARTESIAN_POINT ( 'NONE',  ( 14.30769230769231015, -9.584722331328613620, 36.20867863119891439 ) ) ;
#49519=VERTEX_POINT ( 'NONE', #59375 ) ;
#49520=CARTESIAN_POINT ( 'NONE',  ( -12.23875892027004753, -5.913360116392397892, 34.49180327182771322 ) ) ;
#49522=CARTESIAN_POINT ( 'NONE',  ( -8.546219417617919589, -8.239487800360276282, 34.69522927552633718 ) ) ;
#49524=CARTESIAN_POINT ( 'NONE',  ( -10.86538461538461320, -7.500000000000001776, 34.75000000000000000 ) ) ;
#49525=AXIS2_PLACEMENT_3D ( 'NONE', #27255, #53390, #46641 ) ;
#49526=CARTESIAN_POINT ( 'NONE',  ( -5.326946314216043810, -10.05641848906368097, 34.04755513067966177 ) ) ;
#49527=VERTEX_POINT ( 'NONE', #80093 ) ;
#49528=DIRECTION ( 'NONE',  ( 0.000000000000000000, 1.000000000000000000, 0.000000000000000000 ) ) ;
#49529=DIRECTION ( 'NONE',  ( -0.000000000000000000, 0.9396926207859093161, -0.3420201433256663259 ) ) ;
#49530=FACE_BOUND ( 'NONE', #7549, .T. ) ;
#49531=VECTOR ( 'NONE', #81089, 1000.000000000000000 ) ;
#49532=CARTESIAN_POINT ( 'NONE',  ( -11.53846153846165912, -2.625532179533778709, 30.86335684631627174 ) ) ;
#49533=CARTESIAN_POINT ( 'NONE',  ( -11.76194646302587010, -6.716662450894489211, 34.94144148231605840 ) ) ;
#49535=CARTESIAN_POINT ( 'NONE',  ( 9.562159722575998444, -11.66186481527757302, 32.95055677023626117 ) ) ;
#49537=CARTESIAN_POINT ( 'NONE',  ( -3.164700879766792152, -3.050289026998446840, 32.03036669348366416 ) ) ;
#49538=CYLINDRICAL_SURFACE ( 'NONE', #11685, 0.2499999999999994726 ) ;
#49540=CARTESIAN_POINT ( 'NONE',  ( -7.846153846153965716, -6.026961402154118019, 34.52809138561165270 ) ) ;
#49541=ORIENTED_EDGE ( 'NONE', *, *, #47154, .F. ) ;
#49542=VERTEX_POINT ( 'NONE', #51246 ) ;
#49543=CARTESIAN_POINT ( 'NONE',  ( 14.43848411551709177, -3.530189275343204702, 32.79018710029569661 ) ) ;
#49544=CARTESIAN_POINT ( 'NONE',  ( 16.21991450484859953, -12.10708131394839882, 31.69288490824020954 ) ) ;
#49545=CARTESIAN_POINT ( 'NONE',  ( -9.442362282929648742, -12.45601412856602686, 31.48342859153981621 ) ) ;
#49546=CARTESIAN_POINT ( 'NONE',  ( -8.769230769230890843, -2.892918686052166066, 31.69288490824153470 ) ) ;
#49547=CARTESIAN_POINT ( 'NONE',  ( -12.21148404162500611, -2.544122305571458575, 31.48381861865057729 ) ) ;
#49548=CARTESIAN_POINT ( 'NONE',  ( 9.822833394071260216, -2.619367082507849442, 30.83698974864643461 ) ) ;
#49550=CARTESIAN_POINT ( 'NONE',  ( -6.923076923077045919, -3.643525952248796163, 33.31231777344771672 ) ) ;
#49551=CARTESIAN_POINT ( 'NONE',  ( 1.449870955891411350, -12.27809138561124591, 31.22303859784720359 ) ) ;
#49553=CARTESIAN_POINT ( 'NONE',  ( 18.00000000000000000, -2.499999999999998668, 29.50000000000001066 ) ) ;
#49555=EDGE_LOOP ( 'NONE', ( #35652, #43277 ) ) ;
#49556=CARTESIAN_POINT ( 'NONE',  ( 3.007284306204902613, -12.11044203135681840, 32.26167407432752299 ) ) ;
#49557=VERTEX_POINT ( 'NONE', #39574 ) ;
#49558=ORIENTED_EDGE ( 'NONE', *, *, #18951, .F. ) ;
#49559=CARTESIAN_POINT ( 'NONE',  ( -7.173053654019277303, -8.303909089506435137, 34.68538101551103381 ) ) ;
#49560=ORIENTED_EDGE ( 'NONE', *, *, #17347, .F. ) ;
#49561=CARTESIAN_POINT ( 'NONE',  ( -1.318547033612945674, -8.120952969808772792, 34.71129190929999453 ) ) ;
#49562=CARTESIAN_POINT ( 'NONE',  ( -17.29984929443921970, -3.105860786376062332, 32.13614157043599562 ) ) ;
#49563=FACE_OUTER_BOUND ( 'NONE', #54806, .T. ) ;
#49564=CARTESIAN_POINT ( 'NONE',  ( -8.638438961405983108, -10.54018710029568595, 33.71981072465678864 ) ) ;
#49565=CARTESIAN_POINT ( 'NONE',  ( -16.15384615384615330, -8.164416787775445883, 34.95778746994557906 ) ) ;
#49566=CARTESIAN_POINT ( 'NONE',  ( 0.6843181305165270123, -9.418065098278011860, 34.63729479722530158 ) ) ;
#49568=EDGE_LOOP ( 'NONE', ( #53036, #70551, #51028, #73047 ) ) ;
#49569=CARTESIAN_POINT ( 'NONE',  ( 3.903846153846155076, -7.566083408709834757, 34.74999999999999289 ) ) ;
#49570=CARTESIAN_POINT ( 'NONE',  ( 17.77713373693690002, -2.251424796025574881, 29.88072029997477941 ) ) ;
#49573=DIRECTION ( 'NONE',  ( -0.000000000000000000, -0.6427876096865404731, -0.7660444431189770143 ) ) ;
#49574=DIRECTION ( 'NONE',  ( 0.000000000000000000, -6.938893903907222067E-15, 1.000000000000000000 ) ) ;
#49575=CARTESIAN_POINT ( 'NONE',  ( 5.076923076922954969, -11.48612834414049644, 32.76840700105863391 ) ) ;
#49576=LINE ( 'NONE', #20339, #31794 ) ;
#49579=VERTEX_POINT ( 'NONE', #4426 ) ;
#49580=B_SPLINE_CURVE_WITH_KNOTS ( 'NONE', 3,
 ( #43745, #71207, #63571, #9511, #15403, #3197, #1875, #36978, #69889, #2741 ),
 .UNSPECIFIED., .F., .F.,
 ( 4, 2, 2, 2, 4 ),
 ( 0.0007817359430256294638, 0.0009771253907249948054, 0.001172514838424360255, 0.001367904286123725489, 0.001563293733823090939 ),
 .UNSPECIFIED. ) ;
#49581=CARTESIAN_POINT ( 'NONE',  ( -3.230769230769352962, -6.835583212225970762, 34.95778746994575670 ) ) ;
#49582=CARTESIAN_POINT ( 'NONE',  ( 4.376625822824220080, -10.97394488606064122, 33.68653795673696294 ) ) ;
#49584=CARTESIAN_POINT ( 'NONE',  ( 0.3954550505825799589, -3.513871655860377086, 32.76840700105978499 ) ) ;
#49585=CARTESIAN_POINT ( 'NONE',  ( -7.846153846153844924, -2.833524468853757305, 32.15551576947925838 ) ) ;
#49587=CARTESIAN_POINT ( 'NONE',  ( 0.2115152373170042510, -4.175268141568690083, 33.81360843649122927 ) ) ;
#49588=CARTESIAN_POINT ( 'NONE',  ( -3.296039676730006196, -10.90142922261923886, 33.41473453929638993 ) ) ;
#49589=ORIENTED_EDGE ( 'NONE', *, *, #48641, .T. ) ;
#49590=CARTESIAN_POINT ( 'NONE',  ( -0.4615384615385840772, -12.70778746994576025, 30.41441678777401236 ) ) ;
#49591=CARTESIAN_POINT ( 'NONE',  ( -4.153846153846152411, -10.51840700105979565, 33.73612834413961536 ) ) ;
#49592=ORIENTED_EDGE ( 'NONE', *, *, #63735, .T. ) ;
#49593=CARTESIAN_POINT ( 'NONE',  ( 14.37376065869475106, -12.10708131394839704, 31.69288490824020954 ) ) ;
#49594=CYLINDRICAL_SURFACE ( 'NONE', #76790, 0.2499999999999995559 ) ;
#49595=AXIS2_PLACEMENT_3D ( 'NONE', #6890, #74465, #27606 ) ;
#49597=CARTESIAN_POINT ( 'NONE',  ( -11.28846153846011902, -7.500000000000154543, 35.00000000000007105 ) ) ;
#49598=CARTESIAN_POINT ( 'NONE',  ( 7.846153846153846700, -3.050289026998446396, 32.03036669348365706 ) ) ;
#49599=ORIENTED_EDGE ( 'NONE', *, *, #40484, .F. ) ;
#49600=CARTESIAN_POINT ( 'NONE',  ( -2.438382910802613601, -11.93127051446800024, 32.56575433478200665 ) ) ;
#49601=VECTOR ( 'NONE', #75666, 1000.000000000000000 ) ;
#49602=ORIENTED_EDGE ( 'NONE', *, *, #7616, .T. ) ;
#49603=CARTESIAN_POINT ( 'NONE',  ( -6.793031760242145722, -2.504778602574660340, 29.97347330155780298 ) ) ;
#49604=CARTESIAN_POINT ( 'NONE',  ( 0.5267936010512989098, -10.33852847137154107, 34.16647553114620450 ) ) ;
#49605=EDGE_LOOP ( 'NONE', ( #59709, #37419 ) ) ;
#49606=CARTESIAN_POINT ( 'NONE',  ( 16.15384615384615330, -1.790695186598648903, 34.54067556320373455 ) ) ;
#49607=DIRECTION ( 'NONE',  ( 0.000000000000000000, 0.8660254037844377084, -0.5000000000000015543 ) ) ;
#49608=LINE ( 'NONE', #7743, #49478 ) ;
#49609=DIRECTION ( 'NONE',  ( 0.000000000000000000, 0.7660444431189807890, 0.6427876096865361433 ) ) ;
#49610=CYLINDRICAL_SURFACE ( 'NONE', #22467, 0.2500000000000008882 ) ;
#49611=EDGE_CURVE ( 'NONE', #20058, #51973, #59101, .T. ) ;
#49612=ADVANCED_FACE ( 'NONE', ( #86878 ), #11189, .F. ) ;
#49613=ORIENTED_EDGE ( 'NONE', *, *, #57453, .T. ) ;
#49614=ORIENTED_EDGE ( 'NONE', *, *, #80852, .T. ) ;
#49615=B_SPLINE_CURVE_WITH_KNOTS ( 'NONE', 3,
 ( #87563, #34361, #54625, #33488, #39805, #47880, #80351, #18648, #67272, #81235 ),
 .UNSPECIFIED., .F., .F.,
 ( 4, 2, 2, 2, 4 ),
 ( 0.0007817359430256308733, 0.0009771253907249971907, 0.001172514838424363725, 0.001367904286123730259, 0.001563293733823096577 ),
 .UNSPECIFIED. ) ;
#49616=FACE_BOUND ( 'NONE', #23758, .T. ) ;
#49617=ORIENTED_EDGE ( 'NONE', *, *, #11877, .F. ) ;
#49618=CARTESIAN_POINT ( 'NONE',  ( -4.826923076923076650, -2.249999999999998668, 29.75000000000000355 ) ) ;
#49619=CARTESIAN_POINT ( 'NONE',  ( 4.219914504848593317, -11.69971097300155272, 32.46337939537588113 ) ) ;
#49620=CARTESIAN_POINT ( 'NONE',  ( -18.00000000000000000, -1.270656007487078965, 33.34651343095210052 ) ) ;
#49621=LINE ( 'NONE', #42432, #36676 ) ;
#49622=EDGE_CURVE ( 'NONE', #61355, #14268, #31182, .T. ) ;
#49623=ORIENTED_EDGE ( 'NONE', *, *, #79759, .T. ) ;
#49624=VECTOR ( 'NONE', #43795, 1000.000000000000227 ) ;
#49625=ORIENTED_EDGE ( 'NONE', *, *, #88355, .T. ) ;
#49627=CARTESIAN_POINT ( 'NONE',  ( -10.68146699474474914, -8.164416787775445883, 34.95778746994557906 ) ) ;
#49629=CARTESIAN_POINT ( 'NONE',  ( 13.25446817517716980, -2.882441371585227508, 31.66841991370172238 ) ) ;
#49630=CARTESIAN_POINT ( 'NONE',  ( 16.82694633287448838, -3.436278759898155677, 33.07459398097509506 ) ) ;
#49631=CARTESIAN_POINT ( 'NONE',  ( -18.13069146666755671, -11.18331474514187640, 33.13161551792790505 ) ) ;
#49632=ORIENTED_EDGE ( 'NONE', *, *, #56002, .F. ) ;
#49633=CARTESIAN_POINT ( 'NONE',  ( -5.300408020647025431, -10.81261337010820256, 33.49550067578627477 ) ) ;
#49634=DIRECTION ( 'NONE',  ( 0.000000000000000000, 0.9848077530122072432, 0.1736481776669354937 ) ) ;
#49635=CARTESIAN_POINT ( 'NONE',  ( 3.903869409797563250, -2.544273027872574922, 31.48422191005632342 ) ) ;
#49636=CARTESIAN_POINT ( 'NONE',  ( 10.61538461538461675, -12.62096338111211580, 30.90682066428153263 ) ) ;
#49637=ORIENTED_EDGE ( 'NONE', *, *, #16892, .T. ) ;
#49638=VERTEX_POINT ( 'NONE', #66120 ) ;
#49639=ORIENTED_EDGE ( 'NONE', *, *, #25481, .T. ) ;
#49640=CARTESIAN_POINT ( 'NONE',  ( 13.38461538461538680, -2.499999999999998668, 29.75000000000001421 ) ) ;
#49642=CARTESIAN_POINT ( 'NONE',  ( 1.384615384615386802, -11.35647404775217417, 33.31231777344666511 ) ) ;
#49643=B_SPLINE_CURVE_WITH_KNOTS ( 'NONE', 3,
 ( #65901, #44738, #4208, #31693, #45641, #52386, #11413, #38900, #66358, #4661 ),
 .UNSPECIFIED., .F., .F.,
 ( 4, 2, 2, 2, 4 ),
 ( 0.000000000000000000, 0.0001954339857564080165, 0.0003908679715128160329, 0.0005863019572692240765, 0.0007817359430256320659 ),
 .UNSPECIFIED. ) ;
#49644=DIRECTION ( 'NONE',  ( -0.000000000000000000, 0.8660254037844399289, -0.4999999999999980016 ) ) ;
#49645=DIRECTION ( 'NONE',  ( -0.000000000000000000, 1.000000000000000000, 3.491481338843133355E-15 ) ) ;
#49646=FACE_BOUND ( 'NONE', #28125, .T. ) ;
#49647=CARTESIAN_POINT ( 'NONE',  ( 7.911409417429871027, -11.48612834413965977, 32.76840700105972815 ) ) ;
#49648=VERTEX_POINT ( 'NONE', #79208 ) ;
#49650=CARTESIAN_POINT ( 'NONE',  ( -2.980823712421087901, -2.587454068350147907, 30.68340429815432202 ) ) ;
#49651=CARTESIAN_POINT ( 'NONE',  ( -0.3307466537136744544, -8.999086150933472084, 34.52020707165672064 ) ) ;
#49652=CARTESIAN_POINT ( 'NONE',  ( -17.07692307692307665, -11.69971097300155272, 32.46337939537588113 ) ) ;
#49655=CARTESIAN_POINT ( 'NONE',  ( 4.826899852701617810, -12.68155406624981119, 30.59749803192733708 ) ) ;
#49656=ORIENTED_EDGE ( 'NONE', *, *, #82826, .F. ) ;
#49657=FACE_BOUND ( 'NONE', #78463, .T. ) ;
#49658=CARTESIAN_POINT ( 'NONE',  ( -17.29985003582992320, -4.026226216239093603, 33.68668979543632958 ) ) ;
#49659=FACE_OUTER_BOUND ( 'NONE', #48610, .T. ) ;
#49660=CARTESIAN_POINT ( 'NONE',  ( 12.39545505058258001, -12.10708131394839349, 31.69288490824020244 ) ) ;
#49661=ORIENTED_EDGE ( 'NONE', *, *, #60237, .F. ) ;
#49663=CARTESIAN_POINT ( 'NONE',  ( -12.46153846153858247, -10.21337939537710326, 33.94971097300076224 ) ) ;
#49664=CARTESIAN_POINT ( 'NONE',  ( 15.36155967173618286, -2.295524264805589354, 30.44142389570982488 ) ) ;
#49665=CARTESIAN_POINT ( 'NONE',  ( -14.98071481085577972, -10.06805714834173493, 34.32951233291982618 ) ) ;
#49666=CARTESIAN_POINT ( 'NONE',  ( -16.15384615384627409, -2.625532179533778709, 30.86335684631627174 ) ) ;
#49667=ORIENTED_EDGE ( 'NONE', *, *, #70658, .T. ) ;
#49668=EDGE_CURVE ( 'NONE', #80366, #71586, #68841, .T. ) ;
#49669=CARTESIAN_POINT ( 'NONE',  ( -7.623374304885436104, -10.81320215134717344, 33.49497208177562868 ) ) ;
#49671=DIRECTION ( 'NONE',  ( -0.000000000000000000, 0.7660444431189791237, -0.6427876096865379196 ) ) ;
#49673=CARTESIAN_POINT ( 'NONE',  ( 3.453548772037639658, -2.600157965045225783, 30.74683119005207743 ) ) ;
#49674=CARTESIAN_POINT ( 'NONE',  ( -6.700065571464072889, -11.76359900205217457, 32.36225158514719880 ) ) ;
#49675=CARTESIAN_POINT ( 'NONE',  ( 13.31853197365950514, -8.973038597847271092, 34.52809138561120506 ) ) ;
#49676=CARTESIAN_POINT ( 'NONE',  ( 12.46153846153833911, -4.481592998941358097, 33.73612834414048933 ) ) ;
#49677=CARTESIAN_POINT ( 'NONE',  ( -3.165514091256391715, -4.320704448112861584, 33.92786785259548310 ) ) ;
#49679=CARTESIAN_POINT ( 'NONE',  ( 12.52668424087042531, -7.750023238201979581, 34.74374492549440419 ) ) ;
#49681=VERTEX_POINT ( 'NONE', #18840 ) ;
#49682=CARTESIAN_POINT ( 'NONE',  ( -15.09997742294444478, -3.530189275343204702, 32.79018710029569661 ) ) ;
#49683=CARTESIAN_POINT ( 'NONE',  ( -9.561517251340740486, -11.37503395064541678, 33.29242100308974273 ) ) ;
#49684=ORIENTED_EDGE ( 'NONE', *, *, #2527, .T. ) ;
#49685=ADVANCED_FACE ( 'NONE', ( #46307 ), #67916, .F. ) ;
#49686=EDGE_LOOP ( 'NONE', ( #8610, #75978, #3780, #17940 ) ) ;
#49687=ORIENTED_EDGE ( 'NONE', *, *, #16040, .F. ) ;
#49688=LINE ( 'NONE', #56001, #62755 ) ;
#49689=ADVANCED_FACE ( 'NONE', ( #27371 ), #54837, .F. ) ;
#49690=CARTESIAN_POINT ( 'NONE',  ( 3.100077764101672795, -9.804603061927743113, 34.18744698557895845 ) ) ;
#49691=VECTOR ( 'NONE', #20555, 1000.000000000000114 ) ;
#49692=CARTESIAN_POINT ( 'NONE',  ( -2.307692307692305711, -1.509761064869970415, 31.06009739812519044 ) ) ;
#49693=DIRECTION ( 'NONE',  ( -0.000000000000000000, -0.9848077530122086864, -0.1736481776669273613 ) ) ;
#49694=CARTESIAN_POINT ( 'NONE',  ( -16.40386939113911779, -3.202444869320336895, 32.30641848906366675 ) ) ;
#49695=CARTESIAN_POINT ( 'NONE',  ( 7.145856464345329506, -11.41317474335729187, 32.86274602512330034 ) ) ;
#49696=CARTESIAN_POINT ( 'NONE',  ( 13.44980837291003795, -2.255955759149235629, 29.99999999999988987 ) ) ;
#49697=B_SPLINE_CURVE_WITH_KNOTS ( 'NONE', 3,
 ( #16095, #79127, #66041, #23287, #24622, #37689, #50307, #78231, #78683, #17428 ),
 .UNSPECIFIED., .F., .F.,
 ( 4, 2, 2, 2, 4 ),
 ( 0.000000000000000000, 0.0001954339857564078809, 0.0003908679715128157619, 0.0005863019572692236428, 0.0007817359430256315238 ),
 .UNSPECIFIED. ) ;
#49698=CARTESIAN_POINT ( 'NONE',  ( 16.15384615384615330, -11.33034616979429110, 35.88435417666054406 ) ) ;
#49699=CARTESIAN_POINT ( 'NONE',  ( 11.28848480751918437, -10.66389620160130036, 33.62221079203477103 ) ) ;
#49701=CARTESIAN_POINT ( 'NONE',  ( 2.177545098254086486, -3.817052484675422797, 33.13202310037935661 ) ) ;
#49703=EDGE_CURVE ( 'NONE', #14282, #35719, #34121, .T. ) ;
#49705=ORIENTED_EDGE ( 'NONE', *, *, #8303, .F. ) ;
#49706=CARTESIAN_POINT ( 'NONE',  ( 17.07692307692295586, -11.06231777344772027, 33.60647404775119895 ) ) ;
#49707=CARTESIAN_POINT ( 'NONE',  ( 3.296024370282069071, -11.06231777344671130, 33.60647404775212976 ) ) ;
#49708=CARTESIAN_POINT ( 'NONE',  ( 13.38461538461526601, -12.27809138561165270, 31.22303859784587132 ) ) ;
#49709=VERTEX_POINT ( 'NONE', #19285 ) ;
#49711=CARTESIAN_POINT ( 'NONE',  ( -12.71153846153846345, -7.433931650972299465, 34.75000000000000711 ) ) ;
#49712=CARTESIAN_POINT ( 'NONE',  ( -8.835313148590904220, -9.058645607665454236, 34.76329471203372634 ) ) ;
#49713=VECTOR ( 'NONE', #11569, 1000.000000000000114 ) ;
#49714=EDGE_CURVE ( 'NONE', #86676, #46211, #40457, .T. ) ;
#49715=ORIENTED_EDGE ( 'NONE', *, *, #38194, .F. ) ;
#49716=CARTESIAN_POINT ( 'NONE',  ( 16.15384615384603251, -2.892918686052165622, 31.69288490824153470 ) ) ;
#49717=ADVANCED_FACE ( 'NONE', ( #68796 ), #26487, .F. ) ;
#49718=ORIENTED_EDGE ( 'NONE', *, *, #76773, .F. ) ;
#49719=CARTESIAN_POINT ( 'NONE',  ( 16.28463659481310444, -9.084667340241228572, 34.75534355489798344 ) ) ;
#49720=FACE_OUTER_BOUND ( 'NONE', #6239, .T. ) ;
#49721=ADVANCED_FACE ( 'NONE', ( #88654 ), #5771, .F. ) ;
#49722=CARTESIAN_POINT ( 'NONE',  ( 17.07692307692307665, -1.129524287112498415, 32.06866353760679544 ) ) ;
#49725=CYLINDRICAL_SURFACE ( 'NONE', #10544, 0.2500000000000008882 ) ;
#49726=CARTESIAN_POINT ( 'NONE',  ( 13.38461538461538680, -1.466349020453238561, 30.81389545987213907 ) ) ;
#49727=EDGE_LOOP ( 'NONE', ( #72226, #14291 ) ) ;
#49728=VERTEX_POINT ( 'NONE', #53948 ) ;
#49730=CARTESIAN_POINT ( 'NONE',  ( -10.68146699474474914, -12.34228464037088280, 31.77849191805838558 ) ) ;
#49731=CARTESIAN_POINT ( 'NONE',  ( 16.02369818411445834, -5.915902021225892149, 34.75552854090298638 ) ) ;
#49732=CARTESIAN_POINT ( 'NONE',  ( 0.4615384615384611200, -6.343179335718451384, 34.87096338111211935 ) ) ;
#49733=B_SPLINE_CURVE_WITH_KNOTS ( 'NONE', 3,
 ( #30856, #58327, #65532, #85822, #24100, #3833, #31315, #58777, #24547, #25890 ),
 .UNSPECIFIED., .F., .F.,
 ( 4, 2, 2, 2, 4 ),
 ( 0.000000000000000000, 0.0001954311564186858715, 0.0003908623128373717431, 0.0005862934692560576146, 0.0007817246256747434861 ),
 .UNSPECIFIED. ) ;
#49734=CARTESIAN_POINT ( 'NONE',  ( 11.28843830116857383, -12.22074536777954989, 31.39888409691088356 ) ) ;
#49735=CARTESIAN_POINT ( 'NONE',  ( 4.219914504848592429, -6.386643153685127139, 34.62446782046654192 ) ) ;
#49736=CARTESIAN_POINT ( 'NONE',  ( 14.37376065869474751, -9.780366693483667717, 34.19971097300155805 ) ) ;
#49738=VERTEX_POINT ( 'NONE', #48070 ) ;
#49739=VECTOR ( 'NONE', #21002, 1000.000000000000000 ) ;
#49740=ORIENTED_EDGE ( 'NONE', *, *, #56562, .T. ) ;
#49741=CARTESIAN_POINT ( 'NONE',  ( 3.903822916553188360, -2.823816976329321271, 31.52131813110797154 ) ) ;
#49742=VERTEX_POINT ( 'NONE', #34571 ) ;
#49743=CARTESIAN_POINT ( 'NONE',  ( -9.692307692307691624, -8.973038597847269315, 34.52809138561121927 ) ) ;
#49744=CARTESIAN_POINT ( 'NONE',  ( -8.638438961405981331, -11.18335022499818621, 33.13157742990016885 ) ) ;
#49745=EDGE_CURVE ( 'NONE', #18725, #52344, #35006, .T. ) ;
#49747=ORIENTED_EDGE ( 'NONE', *, *, #74571, .F. ) ;
#49749=CARTESIAN_POINT ( 'NONE',  ( 13.60799132531357003, -2.501478030877322567, 29.88021232661721172 ) ) ;
#49750=VERTEX_POINT ( 'NONE', #68353 ) ;
#49751=FACE_BOUND ( 'NONE', #1756, .T. ) ;
#49752=CARTESIAN_POINT ( 'NONE',  ( -5.933932666649923249, -2.833524468853757750, 32.15551576947925838 ) ) ;
#49753=EDGE_CURVE ( 'NONE', #62900, #29059, #10768, .T. ) ;
#49754=CARTESIAN_POINT ( 'NONE',  ( -8.769230769230892619, -12.16647553114689728, 32.15551576947799362 ) ) ;
#49755=ORIENTED_EDGE ( 'NONE', *, *, #6301, .F. ) ;
#49756=CARTESIAN_POINT ( 'NONE',  ( -14.98082371242109012, -5.057305518903948638, 34.11320923018887896 ) ) ;
#49757=CARTESIAN_POINT ( 'NONE',  ( 11.53846153846141576, -6.835583212225970762, 34.95778746994575670 ) ) ;
#49759=CARTESIAN_POINT ( 'NONE',  ( -15.23076923076922995, -6.386643153685126251, 34.62446782046654192 ) ) ;
#49760=CARTESIAN_POINT ( 'NONE',  ( 4.284637961670939355, -3.062576670634119758, 32.05464942895959979 ) ) ;
#49761=EDGE_LOOP ( 'NONE', ( #10405, #26913 ) ) ;
#49762=EDGE_CURVE ( 'NONE', #12856, #22911, #7094, .T. ) ;
#49763=CARTESIAN_POINT ( 'NONE',  ( -7.146561866800870355, -11.41268669641500466, 32.86336882939237825 ) ) ;
#49764=CARTESIAN_POINT ( 'NONE',  ( -8.096177070375304652, -12.07920672191015221, 32.31858351112116168 ) ) ;
#49765=LINE ( 'NONE', #22301, #35546 ) ;
#49767=CARTESIAN_POINT ( 'NONE',  ( -14.98071491913091791, -11.79725096376909299, 32.30694842903960762 ) ) ;
#49768=AXIS2_PLACEMENT_3D ( 'NONE', #39040, #80466, #44881 ) ;
#49769=CARTESIAN_POINT ( 'NONE',  ( -13.38461538461538325, -12.34228464037088635, 31.77849191805839268 ) ) ;
#49770=DIRECTION ( 'NONE',  ( 0.000000000000000000, 0.9396926207859126468, -0.3420201433256571111 ) ) ;
#49771=CARTESIAN_POINT ( 'NONE',  ( 11.76124107972994359, -4.387253974876679230, 33.66317474335728832 ) ) ;
#49772=CARTESIAN_POINT ( 'NONE',  ( 5.142178216435913107, -9.528491918058460186, 34.59228464037085615 ) ) ;
#49773=CARTESIAN_POINT ( 'NONE',  ( -11.47320596718551755, -11.48612834413965977, 32.76840700105972815 ) ) ;
#49775=CARTESIAN_POINT ( 'NONE',  ( 6.000000000000001776, -1.629998284177014645, 34.34916445242399163 ) ) ;
#49776=B_SPLINE_CURVE_WITH_KNOTS ( 'NONE', 3,
 ( #70357, #77551, #64023, #35692, #77992, #55945, #2321, #71225, #8662, #2759 ),
 .UNSPECIFIED., .F., .F.,
 ( 4, 2, 2, 2, 4 ),
 ( 0.0007817246256747473893, 0.0009771112852218909357, 0.001172497944769034482, 0.001367884604316178246, 0.001563271263863321792 ),
 .UNSPECIFIED. ) ;
#49780=ORIENTED_EDGE ( 'NONE', *, *, #79416, .F. ) ;
#49781=CARTESIAN_POINT ( 'NONE',  ( 6.000000000000001776, -4.102666532097928531, 36.13435417666054406 ) ) ;
#49782=ADVANCED_FACE ( 'NONE', ( #74230 ), #33243, .F. ) ;
#49783=ORIENTED_EDGE ( 'NONE', *, *, #46847, .F. ) ;
#49784=CARTESIAN_POINT ( 'NONE',  ( -3.930834802233303282, -11.24521262558773671, 33.06293181088029343 ) ) ;
#49785=LINE ( 'NONE', #1609, #7192 ) ;
#49788=CARTESIAN_POINT ( 'NONE',  ( -18.22348494372394967, -12.44517049084099725, 30.48991314939691932 ) ) ;
#49790=CARTESIAN_POINT ( 'NONE',  ( -17.77698715590660328, -9.172514111537580561, 34.72667873470787470 ) ) ;
#49791=EDGE_CURVE ( 'NONE', #58385, #46391, #47294, .T. ) ;
#49792=CYLINDRICAL_SURFACE ( 'NONE', #70505, 0.2499999999999998890 ) ;
#49793=CARTESIAN_POINT ( 'NONE',  ( 7.053868730901711182, -8.999086150933472084, 34.52020707165672064 ) ) ;
#49794=CARTESIAN_POINT ( 'NONE',  ( 7.912222197156284054, -11.69971097300155272, 32.46337939537588113 ) ) ;
#49795=DIRECTION ( 'NONE',  ( -0.000000000000000000, -0.3420201433256694901, -0.9396926207859082059 ) ) ;
#49796=CARTESIAN_POINT ( 'NONE',  ( 5.011652630962299959, -8.613356846314824011, 34.62446782046655613 ) ) ;
#49799=LINE ( 'NONE', #20991, #63559 ) ;
#49800=LINE ( 'NONE', #48919, #53613 ) ;
#49802=CARTESIAN_POINT ( 'NONE',  ( -14.08491276642389245, -10.81320215134717344, 33.49497208177562868 ) ) ;
#49803=EDGE_LOOP ( 'NONE', ( #42351, #70665 ) ) ;
#49806=CARTESIAN_POINT ( 'NONE',  ( 16.15384615384615330, -12.10708131394839349, 31.69288490824020244 ) ) ;
#49807=CARTESIAN_POINT ( 'NONE',  ( 1.318531973659505807, -12.37446782046654192, 30.86335684631486487 ) ) ;
#49809=CARTESIAN_POINT ( 'NONE',  ( 13.60762673622823549, -2.554770724473668153, 30.48948780036025852 ) ) ;
#49810=B_SPLINE_CURVE_WITH_KNOTS ( 'NONE', 3,
 ( #48645, #34700, #12656, #27497, #27941, #74359, #88779, #40142, #82894, #87904 ),
 .UNSPECIFIED., .F., .F.,
 ( 4, 2, 2, 2, 4 ),
 ( 0.000000000000000000, 0.0001954311564186861697, 0.0003908623128373723394, 0.0005862934692560584820, 0.0007817246256747446788 ),
 .UNSPECIFIED. ) ;
#49812=CARTESIAN_POINT ( 'NONE',  ( 2.057669070399343436, -12.22074536777954989, 31.39888409691088356 ) ) ;
#49814=B_SPLINE_CURVE_WITH_KNOTS ( 'NONE', 3,
 ( #59311, #44445, #4371, #37255, #23738, #65610, #71485, #86817, #72374, #30507 ),
 .UNSPECIFIED., .F., .F.,
 ( 4, 2, 2, 2, 4 ),
 ( 0.000000000000000000, 0.0001954339857564054144, 0.0003908679715128108288, 0.0005863019572692162703, 0.0007817359430256216575 ),
 .UNSPECIFIED. ) ;
#49815=EDGE_CURVE ( 'NONE', #79032, #32391, #64511, .T. ) ;
#49816=ORIENTED_EDGE ( 'NONE', *, *, #72427, .T. ) ;
#49817=EDGE_LOOP ( 'NONE', ( #15404, #22569, #38929, #36034 ) ) ;
#49818=EDGE_CURVE ( 'NONE', #50723, #66717, #11905, .T. ) ;
#49820=LINE ( 'NONE', #55690, #38409 ) ;
#49821=CARTESIAN_POINT ( 'NONE',  ( -10.61538461538461320, -12.48256725967547354, 35.29906147534542527 ) ) ;
#49822=DIRECTION ( 'NONE',  ( -0.000000000000000000, 0.3420201433256694901, -0.9396926207859082059 ) ) ;
#49823=ADVANCED_FACE ( 'NONE', ( #2102 ), #29153, .F. ) ;
#49824=CARTESIAN_POINT ( 'NONE',  ( -9.692307692307377209, -2.255955759149395501, 30.00000000000324363 ) ) ;
#49825=DIRECTION ( 'NONE',  ( -0.000000000000000000, -0.000000000000000000, -1.000000000000000000 ) ) ;
#49826=ORIENTED_EDGE ( 'NONE', *, *, #72075, .F. ) ;
#49827=CARTESIAN_POINT ( 'NONE',  ( -17.20761454359064047, -4.118384482072086072, 33.43331474514187107 ) ) ;
#49828=EDGE_LOOP ( 'NONE', ( #83935, #63681 ) ) ;
#49829=ORIENTED_EDGE ( 'NONE', *, *, #29449, .F. ) ;
#49830=CARTESIAN_POINT ( 'NONE',  ( 4.219913487196230939, -12.34228464037088813, 31.77849191805839268 ) ) ;
#49831=ORIENTED_EDGE ( 'NONE', *, *, #11173, .F. ) ;
#49832=CARTESIAN_POINT ( 'NONE',  ( 8.769230769230768274, -2.721908614388771852, 31.22303859784724978 ) ) ;
#49833=EDGE_CURVE ( 'NONE', #65922, #75150, #53844, .T. ) ;
#49835=EDGE_CURVE ( 'NONE', #85483, #61122, #35453, .T. ) ;
#49836=CARTESIAN_POINT ( 'NONE',  ( -9.942330929600657896, -8.432397168068783699, 34.66272746175022945 ) ) ;
#49837=FACE_OUTER_BOUND ( 'NONE', #32761, .T. ) ;
#49838=ORIENTED_EDGE ( 'NONE', *, *, #46515, .T. ) ;
#49839=VERTEX_POINT ( 'NONE', #56610 ) ;
#49840=EDGE_LOOP ( 'NONE', ( #20623, #71248, #72454, #25671 ) ) ;
#49841=CARTESIAN_POINT ( 'NONE',  ( -2.057637887778853703, -3.435999193479609470, 33.07426656108011542 ) ) ;
#49842=CARTESIAN_POINT ( 'NONE',  ( -14.08491263871423982, -2.353885683473779800, 30.79025554430704403 ) ) ;
#49843=ORIENTED_EDGE ( 'NONE', *, *, #23010, .F. ) ;
#49844=CARTESIAN_POINT ( 'NONE',  ( -6.923076923077044142, -12.46129190930018460, 30.37095296980731973 ) ) ;
#49845=CARTESIAN_POINT ( 'NONE',  ( -11.53846153846153655, -13.95598074871891292, 31.83374038241031911 ) ) ;
#49846=EDGE_CURVE ( 'NONE', #44756, #53910, #51573, .T. ) ;
#49847=CARTESIAN_POINT ( 'NONE',  ( 6.923076923076802558, -11.94971097300221174, 32.03036669348237098 ) ) ;
#49848=ORIENTED_EDGE ( 'NONE', *, *, #19045, .F. ) ;
#49849=DIRECTION ( 'NONE',  ( -0.000000000000000000, 0.7660444431189791237, -0.6427876096865379196 ) ) ;
#49850=CARTESIAN_POINT ( 'NONE',  ( -15.10024379253558635, -12.50538340440932394, 31.33453814440721885 ) ) ;
#49851=ORIENTED_EDGE ( 'NONE', *, *, #53227, .F. ) ;
#49852=FACE_BOUND ( 'NONE', #75390, .T. ) ;
#49854=CARTESIAN_POINT ( 'NONE',  ( 4.153846153846154188, -4.661471528628507777, 34.16647553114623292 ) ) ;
#49856=CARTESIAN_POINT ( 'NONE',  ( -1.384615384615383471, -7.500000000000001776, 35.04278698407183867 ) ) ;
#49857=CARTESIAN_POINT ( 'NONE',  ( 7.976679284387491187, -11.04252011169590020, 33.62494198852677130 ) ) ;
#49859=AXIS2_PLACEMENT_3D ( 'NONE', #10942, #75204, #18593 ) ;
#49860=CARTESIAN_POINT ( 'NONE',  ( -1.161602540521988969, -8.282913670948747864, 34.94150082978203642 ) ) ;
#49861=CARTESIAN_POINT ( 'NONE',  ( -15.93106661257773560, -9.332535724633405749, 34.40230450496446224 ) ) ;
#49862=ORIENTED_EDGE ( 'NONE', *, *, #79821, .F. ) ;
#49863=FACE_OUTER_BOUND ( 'NONE', #19621, .T. ) ;
#49864=CARTESIAN_POINT ( 'NONE',  ( -16.85414340794500276, -6.717445702608400460, 34.94155399931962336 ) ) ;
#49865=VERTEX_POINT ( 'NONE', #16067 ) ;
#49868=CARTESIAN_POINT ( 'NONE',  ( -16.15384615384627409, -12.70778746994576025, 30.41441678777401236 ) ) ;
#49869=CARTESIAN_POINT ( 'NONE',  ( -16.15384615384615330, -9.058645607665452459, 34.76329471203371924 ) ) ;
#49870=CARTESIAN_POINT ( 'NONE',  ( -4.087777802843712394, -2.538708090699994813, 30.37095296980875503 ) ) ;
#49872=CARTESIAN_POINT ( 'NONE',  ( 17.99999999999987566, -6.026961402154118908, 34.52809138561165270 ) ) ;
#49874=FACE_BOUND ( 'NONE', #79893, .T. ) ;
#49875=EDGE_CURVE ( 'NONE', #31330, #53433, #69962, .T. ) ;
#49876=FACE_OUTER_BOUND ( 'NONE', #44828, .T. ) ;
#49879=DIRECTION ( 'NONE',  ( -0.000000000000000000, -0.1736481776669307198, -0.9848077530122080203 ) ) ;
#49880=CARTESIAN_POINT ( 'NONE',  ( -6.792551484843280640, -11.04252011169590020, 33.62494198852677130 ) ) ;
#49881=CARTESIAN_POINT ( 'NONE',  ( -15.10024352900566846, -6.852161475712352789, 34.70806712695775786 ) ) ;
#49882=LINE ( 'NONE', #76481, #39016 ) ;
#49884=ORIENTED_EDGE ( 'NONE', *, *, #46004, .T. ) ;
#49885=VERTEX_POINT ( 'NONE', #2982 ) ;
#49886=CARTESIAN_POINT ( 'NONE',  ( -9.692307692307814193, -2.379036618888197729, 30.90682066428292885 ) ) ;
#49887=CARTESIAN_POINT ( 'NONE',  ( -0.4615384615385826339, -10.90142922262034020, 33.41473453929536674 ) ) ;
#49888=CARTESIAN_POINT ( 'NONE',  ( 2.307692307692309264, -2.249999999999998668, 29.50000000000001421 ) ) ;
#49889=CARTESIAN_POINT ( 'NONE',  ( -1.634638621908350187, -3.202444869320336451, 32.30641848906366675 ) ) ;
#49890=CARTESIAN_POINT ( 'NONE',  ( -3.930833309752755245, -2.889357225399416418, 32.26129605718031002 ) ) ;
#49892=EDGE_CURVE ( 'NONE', #67170, #62464, #78651, .T. ) ;
#49893=CARTESIAN_POINT ( 'NONE',  ( 4.220015294808810324, -7.250054483168843156, 34.74374881642865631 ) ) ;
#49894=CARTESIAN_POINT ( 'NONE',  ( -6.000000000000119904, -12.46129190930018460, 30.37095296980731973 ) ) ;
#49895=EDGE_CURVE ( 'NONE', #34931, #21233, #65638, .T. ) ;
#49896=DIRECTION ( 'NONE',  ( 0.000000000000000000, 0.6427876096865368094, 0.7660444431189802339 ) ) ;
#49897=CARTESIAN_POINT ( 'NONE',  ( -1.515306851282942624, -12.38065189839062263, 30.83690757178629482 ) ) ;
#49898=CARTESIAN_POINT ( 'NONE',  ( -3.296039231325550212, -4.320704448112771878, 33.92786785259540494 ) ) ;
#49899=CARTESIAN_POINT ( 'NONE',  ( 3.930361210122205406, -10.81261337010820256, 33.49550067578627477 ) ) ;
#49900=CYLINDRICAL_SURFACE ( 'NONE', #33296, 0.2500000000000004996 ) ;
#49901=CARTESIAN_POINT ( 'NONE',  ( 14.24242186173153435, -6.879047030191174805, 34.71129190930000163 ) ) ;
#49902=VERTEX_POINT ( 'NONE', #86320 ) ;
#49903=DIRECTION ( 'NONE',  ( -0.000000000000000000, -0.1736481776669307198, -0.9848077530122080203 ) ) ;
#49904=CARTESIAN_POINT ( 'NONE',  ( 0.7114839798866029463, -2.587454068350147462, 30.68340429815432202 ) ) ;
#49905=CIRCLE ( 'NONE', #5300, 0.2500000000000002220 ) ;
#49907=B_SPLINE_CURVE_WITH_KNOTS ( 'NONE', 3,
 ( #41542, #49627, #77099, #15409, #42879, #69006, #7316, #34777, #2308, #2749 ),
 .UNSPECIFIED., .F., .F.,
 ( 4, 2, 2, 2, 4 ),
 ( 0.000000000000000000, 0.0001954311564186871184, 0.0003908623128373742367, 0.0005862934692560614093, 0.0007817246256747484735 ),
 .UNSPECIFIED. ) ;
#49908=CARTESIAN_POINT ( 'NONE',  ( -2.372962308248625973, -5.094484230520674117, 34.41647553114621161 ) ) ;
#49909=CARTESIAN_POINT ( 'NONE',  ( -15.90379173393269596, -2.544122305571458575, 31.48381861865057729 ) ) ;
#49910=ORIENTED_EDGE ( 'NONE', *, *, #40594, .T. ) ;
#49911=DIRECTION ( 'NONE',  ( 0.000000000000000000, -6.938893903907222067E-15, 1.000000000000000000 ) ) ;
#49914=CARTESIAN_POINT ( 'NONE',  ( 9.692307692307570832, -12.70778746994576025, 30.41441678777401236 ) ) ;
#49915=CARTESIAN_POINT ( 'NONE',  ( 12.52679360105129547, -5.941354392334607049, 34.76329471203374055 ) ) ;
#49917=CARTESIAN_POINT ( 'NONE',  ( -5.076923076923075762, -11.16473453929635440, 33.15142922261926373 ) ) ;
#49918=CARTESIAN_POINT ( 'NONE',  ( -13.44988583057615905, -3.300289026998414865, 32.46337939537583139 ) ) ;
#49919=ORIENTED_EDGE ( 'NONE', *, *, #62359, .T. ) ;
#49920=CARTESIAN_POINT ( 'NONE',  ( -11.53846153846153655, -4.098570777380720287, 33.41473453929634729 ) ) ;
#49921=CARTESIAN_POINT ( 'NONE',  ( 15.23076923076923173, -13.37000171582298513, 34.34916445242398453 ) ) ;
#49922=CARTESIAN_POINT ( 'NONE',  ( -3.230769230769352962, -12.16647553114689728, 32.15551576947799362 ) ) ;
#49923=ORIENTED_EDGE ( 'NONE', *, *, #62521, .T. ) ;
#49924=EDGE_LOOP ( 'NONE', ( #50575, #43780 ) ) ;
#49925=B_SPLINE_CURVE_WITH_KNOTS ( 'NONE', 3,
 ( #11351, #46905, #12243, #25314, #24859, #46025, #74846, #4597, #40614, #67638 ),
 .UNSPECIFIED., .F., .F.,
 ( 4, 2, 2, 2, 4 ),
 ( 0.000000000000000000, 0.0001954311564186866034, 0.0003908623128373732067, 0.0005862934692560597830, 0.0007817246256747464135 ),
 .UNSPECIFIED. ) ;
#49927=ORIENTED_EDGE ( 'NONE', *, *, #35056, .F. ) ;
#49928=VECTOR ( 'NONE', #75238, 1000.000000000000114 ) ;
#49929=CARTESIAN_POINT ( 'NONE',  ( 12.59233026936325217, -8.999086150933475636, 34.52020707165672775 ) ) ;
#49931=EDGE_CURVE ( 'NONE', #39557, #49527, #29135, .T. ) ;
#49932=CARTESIAN_POINT ( 'NONE',  ( 15.23076923076910916, -12.16647553114689728, 32.15551576947799362 ) ) ;
#49933=EDGE_CURVE ( 'NONE', #45473, #80310, #63407, .T. ) ;
#49934=FACE_OUTER_BOUND ( 'NONE', #33624, .T. ) ;
#49935=B_SPLINE_CURVE_WITH_KNOTS ( 'NONE', 3,
 ( #9367, #72378, #65177, #85461, #79147, #36825, #51195, #64282, #24643, #50764 ),
 .UNSPECIFIED., .F., .F.,
 ( 4, 2, 2, 2, 4 ),
 ( 0.000000000000000000, 0.0001954311564186860613, 0.0003908623128373721225, 0.0005862934692560581567, 0.0007817246256747442451 ),
 .UNSPECIFIED. ) ;
#49936=ORIENTED_EDGE ( 'NONE', *, *, #995, .F. ) ;
#49937=B_SPLINE_CURVE_WITH_KNOTS ( 'NONE', 3,
 ( #79171, #17472, #44926, #71511, #72402, #10714, #3052, #71078, #9820, #65636 ),
 .UNSPECIFIED., .F., .F.,
 ( 4, 2, 2, 2, 4 ),
 ( 0.000000000000000000, 0.0001954311584214072381, 0.0003908623168428144762, 0.0005862934752642217414, 0.0007817246336856289524 ),
 .UNSPECIFIED. ) ;
#49938=EDGE_LOOP ( 'NONE', ( #75125, #66128 ) ) ;
#49939=CARTESIAN_POINT ( 'NONE',  ( 4.284371592079798674, -8.630441415882550871, 34.87705825610312615 ) ) ;
#49940=ORIENTED_EDGE ( 'NONE', *, *, #46445, .F. ) ;
#49941=EDGE_CURVE ( 'NONE', #5224, #54359, #55912, .T. ) ;
#49942=CARTESIAN_POINT ( 'NONE',  ( 16.21910129335899597, -8.656820664281605460, 34.87096338111211224 ) ) ;
#49943=ORIENTED_EDGE ( 'NONE', *, *, #3674, .T. ) ;
#49944=CARTESIAN_POINT ( 'NONE',  ( -16.15384615384627409, -5.094484230521993062, 34.41647553114689373 ) ) ;
#49945=CARTESIAN_POINT ( 'NONE',  ( -8.769230769230768274, -12.62096338111211580, 30.90682066428153263 ) ) ;
#49946=ORIENTED_EDGE ( 'NONE', *, *, #8764, .F. ) ;
#49947=ORIENTED_EDGE ( 'NONE', *, *, #75162, .F. ) ;
#49948=CARTESIAN_POINT ( 'NONE',  ( 9.822833130541342328, -8.630441415882550871, 34.87705825610312615 ) ) ;
#49949=ORIENTED_EDGE ( 'NONE', *, *, #76216, .F. ) ;
#49950=CYLINDRICAL_SURFACE ( 'NONE', #25831, 0.2500000000000004996 ) ;
#49952=CARTESIAN_POINT ( 'NONE',  ( 14.17754433796061164, -5.915902021225889484, 34.75552854090298638 ) ) ;
#49953=EDGE_LOOP ( 'NONE', ( #78434, #56042, #11747, #70233 ) ) ;
#49954=CARTESIAN_POINT ( 'NONE',  ( 15.93091993633000847, -12.39988816332205701, 30.74660775122750778 ) ) ;
#49955=CARTESIAN_POINT ( 'NONE',  ( -4.403846153846174616, -2.249999999999999112, 29.81609741502488120 ) ) ;
#49956=CARTESIAN_POINT ( 'NONE',  ( 14.30769230769231015, -6.189225973068211317, 35.74407628777942847 ) ) ;
#49957=FACE_BOUND ( 'NONE', #30556, .T. ) ;
#49958=ADVANCED_FACE ( 'NONE', ( #59713 ), #73689, .F. ) ;
#49959=CARTESIAN_POINT ( 'NONE',  ( -9.692307692307691624, -3.937682226553329556, 33.60647404775216529 ) ) ;
#49960=DIRECTION ( 'NONE',  ( -0.000000000000000000, -0.6427876096865404731, -0.7660444431189770143 ) ) ;
#49961=CARTESIAN_POINT ( 'NONE',  ( -15.23076923076935074, -10.90142922262034020, 33.41473453929536674 ) ) ;
#49962=CARTESIAN_POINT ( 'NONE',  ( 12.21151523731700550, -3.520140089381495585, 33.17453946501458262 ) ) ;
#49963=CARTESIAN_POINT ( 'NONE',  ( -5.776988648387150427, -2.758310577978207778, 31.33698337089303010 ) ) ;
#49965=DIRECTION ( 'NONE',  ( 0.000000000000000000, 0.9848077530122072432, 0.1736481776669354937 ) ) ;
#49966=ORIENTED_EDGE ( 'NONE', *, *, #35336, .T. ) ;
#49968=CARTESIAN_POINT ( 'NONE',  ( -5.776988648387149539, -11.76359900205217457, 32.36225158514719880 ) ) ;
#49969=EDGE_LOOP ( 'NONE', ( #44418, #39654, #67959, #84184 ) ) ;
#49970=ORIENTED_EDGE ( 'NONE', *, *, #69778, .T. ) ;
#49971=B_SPLINE_CURVE_WITH_KNOTS ( 'NONE', 3,
 ( #77435, #8546, #56719, #84650, #50391, #894, #70683, #8989, #9421, #15746 ),
 .UNSPECIFIED., .F., .F.,
 ( 4, 2, 2, 2, 4 ),
 ( 0.000000000000000000, 0.0001954311564186876334, 0.0003908623128373752667, 0.0005862934692560629272, 0.0007817246256747505334 ),
 .UNSPECIFIED. ) ;
#49972=CARTESIAN_POINT ( 'NONE',  ( 7.846153846153725020, -6.879047030192662504, 34.71129190930017927 ) ) ;
#49973=CARTESIAN_POINT ( 'NONE',  ( 11.53846153846153832, -13.87047571288749737, 32.06866353760679544 ) ) ;
#49974=EDGE_CURVE ( 'NONE', #82483, #66781, #3266, .T. ) ;
#49975=CARTESIAN_POINT ( 'NONE',  ( 13.13463864056679853, -11.47974371597207899, 33.17467449705390692 ) ) ;
#49976=CARTESIAN_POINT ( 'NONE',  ( -13.38461538461538325, -2.486705287966279876, 31.30864560766543647 ) ) ;
#49977=FACE_OUTER_BOUND ( 'NONE', #79725, .T. ) ;
#49978=CARTESIAN_POINT ( 'NONE',  ( -2.531177232256638376, -11.60425143139329940, 33.02411095842164457 ) ) ;
#49979=VERTEX_POINT ( 'NONE', #19613 ) ;
#49980=CARTESIAN_POINT ( 'NONE',  ( -1.384615384615383471, -12.34228464037088635, 31.77849191805839268 ) ) ;
#49981=ADVANCED_FACE ( 'NONE', ( #47077 ), #53845, .F. ) ;
#49982=ADVANCED_FACE ( 'NONE', ( #68686 ), #20937, .F. ) ;
#49983=CARTESIAN_POINT ( 'NONE',  ( -6.923076923076922462, -13.95598074871891292, 31.83374038241031911 ) ) ;
#49984=DIRECTION ( 'NONE',  ( -0.000000000000000000, -0.3420201433256694901, -0.9396926207859082059 ) ) ;
#49985=CARTESIAN_POINT ( 'NONE',  ( -11.53846153846123102, -2.506253911140614576, 30.00000000000323297 ) ) ;
#49988=VERTEX_POINT ( 'NONE', #39462 ) ;
#49989=ORIENTED_EDGE ( 'NONE', *, *, #54439, .T. ) ;
#49990=AXIS2_PLACEMENT_3D ( 'NONE', #22285, #8780, #15091 ) ;
#49991=DIRECTION ( 'NONE',  ( 0.000000000000000000, 0.9848077530122072432, 0.1736481776669354937 ) ) ;
#49992=ORIENTED_EDGE ( 'NONE', *, *, #86135, .F. ) ;
#49993=DIRECTION ( 'NONE',  ( 0.000000000000000000, 0.3420201433256610524, 0.9396926207859113145 ) ) ;
#49994=CARTESIAN_POINT ( 'NONE',  ( -1.253824943648434331, -9.929761469519744921, 34.40412654351204225 ) ) ;
#49995=CARTESIAN_POINT ( 'NONE',  ( 3.230769230769110045, -9.442884908241554243, 34.35708131394783038 ) ) ;
#49998=EDGE_CURVE ( 'NONE', #4532, #66010, #75890, .T. ) ;
#49999=CARTESIAN_POINT ( 'NONE',  ( 0.6845513056318561773, -9.172514111537584114, 34.72667873470787470 ) ) ;
#50000=ORIENTED_EDGE ( 'NONE', *, *, #63165, .F. ) ;
#50001=AXIS2_PLACEMENT_3D ( 'NONE', #12902, #40393, #19661 ) ;
#50002=LINE ( 'NONE', #15791, #47242 ) ;
#50003=CARTESIAN_POINT ( 'NONE',  ( -2.307692307692428724, -12.70778746994576025, 30.41441678777401236 ) ) ;
#50004=ORIENTED_EDGE ( 'NONE', *, *, #21032, .F. ) ;
#50005=CARTESIAN_POINT ( 'NONE',  ( -15.23076923076922995, -5.415277668671390821, 36.20867863119892149 ) ) ;
#50006=CYLINDRICAL_SURFACE ( 'NONE', #83245, 0.2500000000000002220 ) ;
#50007=EDGE_CURVE ( 'NONE', #41676, #1947, #67807, .T. ) ;
#50008=EDGE_CURVE ( 'NONE', #24402, #50148, #35504, .T. ) ;
#50009=CARTESIAN_POINT ( 'NONE',  ( -17.93474442872397390, -11.94971097300157936, 32.03036669348361443 ) ) ;
#50010=CARTESIAN_POINT ( 'NONE',  ( 0.5276068125408994725, -2.721908614388772740, 31.22303859784725333 ) ) ;
#50012=FACE_OUTER_BOUND ( 'NONE', #14351, .T. ) ;
#50013=CARTESIAN_POINT ( 'NONE',  ( -7.846153846153965716, -12.46129190930018460, 30.37095296980731973 ) ) ;
#50015=VERTEX_POINT ( 'NONE', #234 ) ;
#50016=ADVANCED_FACE ( 'NONE', ( #33129 ), #48408, .F. ) ;
#50017=CARTESIAN_POINT ( 'NONE',  ( -16.85391172531022619, -10.61302985866384141, 33.66295027996417843 ) ) ;
#50018=CARTESIAN_POINT ( 'NONE',  ( -17.30040800148741553, -4.988325925672468131, 34.36044203135681130 ) ) ;
#50020=CARTESIAN_POINT ( 'NONE',  ( 0.2380535369741308138, -5.827078755546623690, 34.72654668319379567 ) ) ;
#50021=CARTESIAN_POINT ( 'NONE',  ( -18.00000000000000000, -5.419720871348011393, 36.19647103217484130 ) ) ;
#50022=ORIENTED_EDGE ( 'NONE', *, *, #28818, .F. ) ;
#50023=CARTESIAN_POINT ( 'NONE',  ( 0.2115617174898685449, -4.075325502946085976, 33.72974371597207721 ) ) ;
#50024=CARTESIAN_POINT ( 'NONE',  ( -15.90390063549801347, -12.22109172314383052, 31.39792113162168263 ) ) ;
#50025=B_SPLINE_CURVE_WITH_KNOTS ( 'NONE', 3,
 ( #74387, #33406, #501, #27971, #21654, #14911, #76604, #34280, #48675, #77483 ),
 .UNSPECIFIED., .F., .F.,
 ( 4, 2, 2, 2, 4 ),
 ( 0.000000000000000000, 0.0001954311584214072923, 0.0003908623168428145846, 0.0005862934752642218498, 0.0007817246336856291692 ),
 .UNSPECIFIED. ) ;
#50026=ORIENTED_EDGE ( 'NONE', *, *, #65965, .T. ) ;
#50027=CARTESIAN_POINT ( 'NONE',  ( 9.942307692309114486, -7.500000000000154543, 35.00000000000007105 ) ) ;
#50028=EDGE_LOOP ( 'NONE', ( #33572, #11616, #80122, #5913 ) ) ;
#50029=AXIS2_PLACEMENT_3D ( 'NONE', #78560, #18660, #37574 ) ;
#50031=CARTESIAN_POINT ( 'NONE',  ( 3.930919936330005360, -3.586966769969700763, 32.86292498521069660 ) ) ;
#50032=CARTESIAN_POINT ( 'NONE',  ( -8.638705330997124676, -5.915461855592780260, 34.75538340440931506 ) ) ;
#50034=ORIENTED_EDGE ( 'NONE', *, *, #19555, .T. ) ;
#50035=CARTESIAN_POINT ( 'NONE',  ( -6.792551484843277976, -6.808710257144159783, 34.95449254468098843 ) ) ;
#50036=EDGE_CURVE ( 'NONE', #763, #73158, #45223, .T. ) ;
#50037=ORIENTED_EDGE ( 'NONE', *, *, #42602, .F. ) ;
#50039=FACE_OUTER_BOUND ( 'NONE', #67555, .T. ) ;
#50040=ORIENTED_EDGE ( 'NONE', *, *, #63416, .F. ) ;
#50041=CARTESIAN_POINT ( 'NONE',  ( 11.66925197942848769, -12.62708834333097663, 30.88030960425257021 ) ) ;
#50042=CARTESIAN_POINT ( 'NONE',  ( 10.86533013373275836, -3.202959910592335646, 32.30730279482227019 ) ) ;
#50043=DIRECTION ( 'NONE',  ( 0.000000000000000000, 0.8660254037844377084, -0.5000000000000015543 ) ) ;
#50044=CARTESIAN_POINT ( 'NONE',  ( 13.60762822870878352, -11.98016756924215009, 32.48728574198911190 ) ) ;
#50045=DIRECTION ( 'NONE',  ( 1.000000000000000000, 0.000000000000000000, 0.000000000000000000 ) ) ;
#50046=VERTEX_POINT ( 'NONE', #6988 ) ;
#50047=EDGE_LOOP ( 'NONE', ( #36757, #76674 ) ) ;
#50048=FACE_BOUND ( 'NONE', #87952, .T. ) ;
#50050=CARTESIAN_POINT ( 'NONE',  ( 12.21153846153846168, -2.249999999999998668, 29.75000000000000355 ) ) ;
#50051=B_SPLINE_CURVE_WITH_KNOTS ( 'NONE', 3,
 ( #23493, #72126, #66261, #79789, #44642, #58608, #72573, #52742, #38353, #65806 ),
 .UNSPECIFIED., .F., .F.,
 ( 4, 2, 2, 2, 4 ),
 ( 0.0007817359430256332585, 0.0009771253907250054306, 0.001172514838424370664, 0.001367904286123735897, 0.001563293733823100913 ),
 .UNSPECIFIED. ) ;
#50052=AXIS2_PLACEMENT_3D ( 'NONE', #44671, #24407, #18117 ) ;
#50053=CARTESIAN_POINT ( 'NONE',  ( -14.17690186672535901, -11.37503395064541678, 33.29242100308974273 ) ) ;
#50054=CARTESIAN_POINT ( 'NONE',  ( -2.307692307692427391, -2.625532179533779154, 30.86335684631627174 ) ) ;
#50056=ORIENTED_EDGE ( 'NONE', *, *, #20911, .F. ) ;
#50057=CIRCLE ( 'NONE', #38560, 0.2500000000000002220 ) ;
#50058=EDGE_CURVE ( 'NONE', #36412, #47496, #88178, .T. ) ;
#50059=ORIENTED_EDGE ( 'NONE', *, *, #60487, .F. ) ;
#50060=ORIENTED_EDGE ( 'NONE', *, *, #18813, .T. ) ;
#50061=CARTESIAN_POINT ( 'NONE',  ( 15.90386942290380290, -9.943427161483782584, 34.11278801902876978 ) ) ;
#50062=VECTOR ( 'NONE', #77722, 1000.000000000000000 ) ;
#50063=CARTESIAN_POINT ( 'NONE',  ( -2.307692307692305711, -1.129524287112498415, 32.06866353760679544 ) ) ;
#50065=CARTESIAN_POINT ( 'NONE',  ( 1.384615384615265343, -11.48612834414049644, 32.76840700105863391 ) ) ;
#50066=ORIENTED_EDGE ( 'NONE', *, *, #42475, .T. ) ;
#50067=CARTESIAN_POINT ( 'NONE',  ( 13.25446817517716980, -10.88202310037935661, 33.43294751532457099 ) ) ;
#50068=CARTESIAN_POINT ( 'NONE',  ( 0.4615384615384611200, -11.69971097300155272, 32.46337939537588113 ) ) ;
#50071=VERTEX_POINT ( 'NONE', #26378 ) ;
#50072=EDGE_CURVE ( 'NONE', #3390, #17581, #67731, .T. ) ;
#50074=ORIENTED_EDGE ( 'NONE', *, *, #72300, .F. ) ;
#50075=CARTESIAN_POINT ( 'NONE',  ( -7.976301055592065481, -6.852621066184266141, 34.70813303252209181 ) ) ;
#50076=CARTESIAN_POINT ( 'NONE',  ( 10.83839596699746721, -6.503523203565941380, 34.64991518177335195 ) ) ;
#50077=DIRECTION ( 'NONE',  ( -0.000000000000000000, -0.3420201433256694901, -0.9396926207859082059 ) ) ;
#50078=CARTESIAN_POINT ( 'NONE',  ( -3.296039676730005308, -11.48612834413959582, 32.76840700105983473 ) ) ;
#50079=FACE_BOUND ( 'NONE', #17496, .T. ) ;
#50080=CARTESIAN_POINT ( 'NONE',  ( -11.66860950819323328, -2.373036134822904319, 30.88089517874952250 ) ) ;
#50081=ORIENTED_EDGE ( 'NONE', *, *, #5439, .T. ) ;
#50082=CARTESIAN_POINT ( 'NONE',  ( 17.20771488474786892, -10.54018710029568595, 33.71981072465678864 ) ) ;
#50083=EDGE_CURVE ( 'NONE', #35424, #49441, #57023, .T. ) ;
#50084=CARTESIAN_POINT ( 'NONE',  ( -0.4615384615385826339, -9.442884908241554243, 34.35708131394783038 ) ) ;
#50085=DIRECTION ( 'NONE',  ( -0.000000000000000000, 0.7660444431189791237, -0.6427876096865379196 ) ) ;
#50086=CYLINDRICAL_SURFACE ( 'NONE', #87039, 0.2499999999999973355 ) ;
#50087=VERTEX_POINT ( 'NONE', #2004 ) ;
#50088=CARTESIAN_POINT ( 'NONE',  ( 2.372947878968334035, -11.94971097300157403, 32.03036669348361443 ) ) ;
#50089=AXIS2_PLACEMENT_3D ( 'NONE', #47323, #46883, #26618 ) ;
#50091=FACE_BOUND ( 'NONE', #41101, .T. ) ;
#50092=CYLINDRICAL_SURFACE ( 'NONE', #70625, 0.2500000000000009437 ) ;
#50093=DIRECTION ( 'NONE',  ( -0.000000000000000000, -0.000000000000000000, -1.000000000000000000 ) ) ;
#50094=CARTESIAN_POINT ( 'NONE',  ( -3.007989689500820685, -8.496831190052096971, 34.64984203495476578 ) ) ;
#50095=ORIENTED_EDGE ( 'NONE', *, *, #49313, .F. ) ;
#50096=CARTESIAN_POINT ( 'NONE',  ( 5.326977388561388693, -3.136992222400443175, 32.19305428654138979 ) ) ;
#50097=CARTESIAN_POINT ( 'NONE',  ( -14.37296275365308418, -4.481592998940162609, 33.73612834413957984 ) ) ;
#50099=CARTESIAN_POINT ( 'NONE',  ( 6.130525701763568591, -3.816742781228458448, 33.13167719472716044 ) ) ;
#50101=CARTESIAN_POINT ( 'NONE',  ( -7.780898274877821486, -10.90142922261932057, 33.41473453929631887 ) ) ;
#50102=ORIENTED_EDGE ( 'NONE', *, *, #10966, .T. ) ;
#50103=FACE_OUTER_BOUND ( 'NONE', #13514, .T. ) ;
#50104=ORIENTED_EDGE ( 'NONE', *, *, #53622, .F. ) ;
#50105=DIRECTION ( 'NONE',  ( -0.000000000000000000, 0.3420201433256694346, -0.9396926207859080948 ) ) ;
#50106=FACE_OUTER_BOUND ( 'NONE', #19722, .T. ) ;
#50107=FACE_OUTER_BOUND ( 'NONE', #46569, .T. ) ;
#50108=B_SPLINE_CURVE_WITH_KNOTS ( 'NONE', 3,
 ( #13242, #19989, #69067, #88480, #75819, #13678, #68622, #28081, #82149, #74952 ),
 .UNSPECIFIED., .F., .F.,
 ( 4, 2, 2, 2, 4 ),
 ( 0.000000000000000000, 0.0001954311564186869286, 0.0003908623128373738573, 0.0005862934692560607588, 0.0007817246256747477145 ),
 .UNSPECIFIED. ) ;
#50110=EDGE_CURVE ( 'NONE', #52382, #820, #1562, .T. ) ;
#50111=CYLINDRICAL_SURFACE ( 'NONE', #20796, 0.2499999999999997502 ) ;
#50112=FACE_OUTER_BOUND ( 'NONE', #29141, .T. ) ;
#50113=CARTESIAN_POINT ( 'NONE',  ( 18.00000000000000000, -11.11383981884818262, 36.00935417666054406 ) ) ;
#50114=LINE ( 'NONE', #15906, #19064 ) ;
#50116=EDGE_LOOP ( 'NONE', ( #6006, #61477 ) ) ;
#50117=CARTESIAN_POINT ( 'NONE',  ( 2.307692307692309264, -8.318370150425687726, 35.83090037661290239 ) ) ;
#50118=DIRECTION ( 'NONE',  ( -0.000000000000000000, 0.3420201433256694901, -0.9396926207859082059 ) ) ;
#50119=EDGE_LOOP ( 'NONE', ( #75245, #32156 ) ) ;
#50120=AXIS2_PLACEMENT_3D ( 'NONE', #61194, #73847, #12145 ) ;
#50121=VERTEX_POINT ( 'NONE', #29050 ) ;
#50122=ORIENTED_EDGE ( 'NONE', *, *, #28751, .T. ) ;
#50123=CYLINDRICAL_SURFACE ( 'NONE', #74287, 0.2500000000000002220 ) ;
#50124=CARTESIAN_POINT ( 'NONE',  ( 4.153846153846154188, -12.29105614889573062, 35.45975837776705220 ) ) ;
#50127=CARTESIAN_POINT ( 'NONE',  ( 8.769230769230645706, -11.67786785259630911, 32.92929555188603530 ) ) ;
#50128=CARTESIAN_POINT ( 'NONE',  ( 8.703960323269992472, -11.48612834413959582, 32.76840700105983473 ) ) ;
#50129=CARTESIAN_POINT ( 'NONE',  ( 7.173022441425066731, -11.37275283266503756, 32.91324779482534524 ) ) ;
#50130=AXIS2_PLACEMENT_3D ( 'NONE', #9354, #64715, #71475 ) ;
#50131=CARTESIAN_POINT ( 'NONE',  ( -4.153846153846273204, -3.835265460704628371, 33.15142922262033665 ) ) ;
#50132=CARTESIAN_POINT ( 'NONE',  ( 3.164685819813350065, -6.386643153685125363, 34.62446782046654903 ) ) ;
#50133=CARTESIAN_POINT ( 'NONE',  ( -1.449885830576159496, -6.879047030191174805, 34.71129190930000163 ) ) ;
#50134=CARTESIAN_POINT ( 'NONE',  ( 12.46153846153833911, -11.94971097300221174, 32.03036669348237098 ) ) ;
#50135=DIRECTION ( 'NONE',  ( -0.000000000000000000, -0.6427876096865404731, -0.7660444431189770143 ) ) ;
#50136=EDGE_LOOP ( 'NONE', ( #28819, #15803 ) ) ;
#50137=CARTESIAN_POINT ( 'NONE',  ( 0.5923302693632481741, -8.999086150933472084, 34.52020707165672064 ) ) ;
#50138=DIRECTION ( 'NONE',  ( 0.000000000000000000, 0.4999999999999985567, 0.8660254037844395958 ) ) ;
#50139=DIRECTION ( 'NONE',  ( -0.000000000000000000, -0.6427876096865404731, -0.7660444431189771253 ) ) ;
#50140=FACE_OUTER_BOUND ( 'NONE', #75997, .T. ) ;
#50141=ORIENTED_EDGE ( 'NONE', *, *, #62570, .T. ) ;
#50142=CARTESIAN_POINT ( 'NONE',  ( -14.30769230769230660, -9.905515769479276145, 34.41647553114623292 ) ) ;
#50143=CARTESIAN_POINT ( 'NONE',  ( 9.626225312947559232, -2.833524468853757305, 32.15551576947924417 ) ) ;
#50144=B_SPLINE_CURVE_WITH_KNOTS ( 'NONE', 3,
 ( #19605, #12848, #13295, #61467, #21375, #6542, #34003, #48844, #48400, #75878 ),
 .UNSPECIFIED., .F., .F.,
 ( 4, 2, 2, 2, 4 ),
 ( 0.000000000000000000, 0.0001954339857564053873, 0.0003908679715128107746, 0.0005863019572692161618, 0.0007817359430256215491 ),
 .UNSPECIFIED. ) ;
#50145=CARTESIAN_POINT ( 'NONE',  ( -8.769230769230768274, -9.058645607665452459, 34.76329471203371924 ) ) ;
#50146=ORIENTED_EDGE ( 'NONE', *, *, #11981, .F. ) ;
#50147=CARTESIAN_POINT ( 'NONE',  ( 7.716005876422150855, -11.66186481527757302, 32.95055677023626117 ) ) ;
#50148=VERTEX_POINT ( 'NONE', #64130 ) ;
#50149=FACE_OUTER_BOUND ( 'NONE', #71654, .T. ) ;
#50150=CARTESIAN_POINT ( 'NONE',  ( 8.769230769230768274, -9.058645607665452459, 34.76329471203371924 ) ) ;
#50151=CARTESIAN_POINT ( 'NONE',  ( 12.46153846153833911, -8.613356846316285953, 34.62446782046622218 ) ) ;
#50152=CARTESIAN_POINT ( 'NONE',  ( 1.161130460051055913, -8.539481045369598178, 34.89627647299170832 ) ) ;
#50153=CARTESIAN_POINT ( 'NONE',  ( -17.75005459062195712, -12.45601412856602686, 31.48342859153981621 ) ) ;
#50154=ORIENTED_EDGE ( 'NONE', *, *, #35378, .T. ) ;
#50155=EDGE_CURVE ( 'NONE', #78633, #35413, #78399, .T. ) ;
#50157=ORIENTED_EDGE ( 'NONE', *, *, #12170, .F. ) ;
#50158=CARTESIAN_POINT ( 'NONE',  ( -17.07692307692319744, -10.90142922262034020, 33.41473453929536674 ) ) ;
#50159=CARTESIAN_POINT ( 'NONE',  ( -17.07692307692319744, -3.835265460704628815, 33.15142922262033665 ) ) ;
#50160=CARTESIAN_POINT ( 'NONE',  ( -4.153846153846152411, -12.34228464037088635, 31.77849191805839268 ) ) ;
#50162=EDGE_CURVE ( 'NONE', #10616, #43687, #3083, .T. ) ;
#50163=B_SPLINE_CURVE_WITH_KNOTS ( 'NONE', 3,
 ( #12430, #5669, #8783, #82676, #83110, #76340, #36255, #61932, #49752, #62371 ),
 .UNSPECIFIED., .F., .F.,
 ( 4, 2, 2, 2, 4 ),
 ( 0.0007817246256747447872, 0.0009771112852218874663, 0.001172497944769030362, 0.001367884604316173258, 0.001563271263863315937 ),
 .UNSPECIFIED. ) ;
#50165=CARTESIAN_POINT ( 'NONE',  ( 11.53846153846153832, -2.499999999999998668, 29.50000000000001066 ) ) ;
#50167=ORIENTED_EDGE ( 'NONE', *, *, #21347, .T. ) ;
#50169=B_SPLINE_CURVE_WITH_KNOTS ( 'NONE', 3,
 ( #22134, #36961, #973, #63104, #14939, #9495, #56796, #22571, #50474, #77959 ),
 .UNSPECIFIED., .F., .F.,
 ( 4, 2, 2, 2, 4 ),
 ( 0.0007817359527651090859, 0.0009771254036996478414, 0.001172514854634186705, 0.001367904305568725569, 0.001563293756503264433 ),
 .UNSPECIFIED. ) ;
#50171=ORIENTED_EDGE ( 'NONE', *, *, #8010, .T. ) ;
#50172=CARTESIAN_POINT ( 'NONE',  ( 4.088575707885378385, -2.892918686051582089, 31.69288490824015270 ) ) ;
#50173=EDGE_LOOP ( 'NONE', ( #34019, #30347 ) ) ;
#50174=FACE_OUTER_BOUND ( 'NONE', #19119, .T. ) ;
#50175=CARTESIAN_POINT ( 'NONE',  ( -8.546451227962361230, -11.41317474335729543, 32.86274602512330034 ) ) ;
#50176=AXIS2_PLACEMENT_3D ( 'NONE', #21091, #75173, #69734 ) ;
#50178=EDGE_LOOP ( 'NONE', ( #69150, #78536 ) ) ;
#50179=VECTOR ( 'NONE', #67735, 1000.000000000000227 ) ;
#50180=EDGE_CURVE ( 'NONE', #58342, #17484, #14186, .T. ) ;
#50181=EDGE_LOOP ( 'NONE', ( #416, #61572, #39681, #14275, #40651, #41187 ) ) ;
#50182=CARTESIAN_POINT ( 'NONE',  ( 13.60762822870878352, -10.77377354290276124, 33.85451476688484718 ) ) ;
#50183=EDGE_LOOP ( 'NONE', ( #4786, #66678, #30275, #30844 ) ) ;
#50184=FACE_BOUND ( 'NONE', #50925, .T. ) ;
#50185=CARTESIAN_POINT ( 'NONE',  ( 13.38461538461538680, -12.34228464037088635, 31.77849191805839268 ) ) ;
#50186=CARTESIAN_POINT ( 'NONE',  ( 11.53846153846153832, -12.37446782046654192, 30.86335684631486131 ) ) ;
#50187=ORIENTED_EDGE ( 'NONE', *, *, #17366, .T. ) ;
#50188=CARTESIAN_POINT ( 'NONE',  ( 16.28437185560971656, -11.46989282347013095, 32.79007818306219946 ) ) ;
#50190=FACE_OUTER_BOUND ( 'NONE', #35316, .T. ) ;
#50191=CARTESIAN_POINT ( 'NONE',  ( -11.76138775597768671, -5.667676309546437530, 34.40238873228292249 ) ) ;
#50192=CARTESIAN_POINT ( 'NONE',  ( -13.16160403300253634, -11.76359900205217457, 32.36225158514719880 ) ) ;
#50193=CARTESIAN_POINT ( 'NONE',  ( -6.988347369037698265, -11.48612834413959582, 32.76840700105983473 ) ) ;
#50194=CARTESIAN_POINT ( 'NONE',  ( -7.596208327805704208, -6.696923467548660192, 34.68552623307873972 ) ) ;
#50196=CARTESIAN_POINT ( 'NONE',  ( -0.5268084620947812713, -5.094484230520674117, 34.41647553114621161 ) ) ;
#50197=CARTESIAN_POINT ( 'NONE',  ( -18.00000000000000000, -6.386643153685127139, 34.62446782046654192 ) ) ;
#50198=ADVANCED_FACE ( 'NONE', ( #55610 ), #14633, .F. ) ;
#50199=CARTESIAN_POINT ( 'NONE',  ( 8.068933515131908152, -3.020022701398814569, 32.48759521482552515 ) ) ;
#50200=CARTESIAN_POINT ( 'NONE',  ( 13.38461538461526601, -11.94971097300221174, 32.03036669348237098 ) ) ;
#50201=CARTESIAN_POINT ( 'NONE',  ( 6.988332494352947677, -3.300289026998475705, 32.46337939537591666 ) ) ;
#50202=LINE ( 'NONE', #2905, #59804 ) ;
#50203=CARTESIAN_POINT ( 'NONE',  ( -3.454254155333563503, -3.019605429927184836, 32.48692288466676814 ) ) ;
#50205=EDGE_CURVE ( 'NONE', #59796, #18998, #35928, .T. ) ;
#50206=CARTESIAN_POINT ( 'NONE',  ( -2.438382910802614933, -5.496505350115500121, 34.60290016733514307 ) ) ;
#50207=VECTOR ( 'NONE', #64926, 1000.000000000000000 ) ;
#50209=B_SPLINE_CURVE_WITH_KNOTS ( 'NONE', 3,
 ( #13155, #69427, #7734, #35193, #40636, #76629, #75302, #13594, #41071, #3170 ),
 .UNSPECIFIED., .F., .F.,
 ( 4, 2, 2, 2, 4 ),
 ( 0.0007817246336856291692, 0.0009771112958940105907, 0.001172497958102391904, 0.001367884620310773434, 0.001563271282519154747 ),
 .UNSPECIFIED. ) ;
#50210=ORIENTED_EDGE ( 'NONE', *, *, #35607, .F. ) ;
#50212=EDGE_LOOP ( 'NONE', ( #58157, #82083 ) ) ;
#50213=CARTESIAN_POINT ( 'NONE',  ( -2.307692307692428724, -3.083524468854526912, 32.58852847137268327 ) ) ;
#50214=EDGE_CURVE ( 'NONE', #87648, #13360, #45053, .T. ) ;
#50216=ADVANCED_FACE ( 'NONE', ( #11426 ), #38007, .F. ) ;
#50217=CARTESIAN_POINT ( 'NONE',  ( -13.13466997523734037, -2.341251567377310217, 30.72681386836322659 ) ) ;
#50218=ORIENTED_EDGE ( 'NONE', *, *, #15597, .F. ) ;
#50219=DIRECTION ( 'NONE',  ( -0.000000000000000000, 0.7660444431189791237, -0.6427876096865379196 ) ) ;
#50221=CARTESIAN_POINT ( 'NONE',  ( 17.20771488474786892, -8.147973898785416225, 34.70805048591653730 ) ) ;
#50222=CARTESIAN_POINT ( 'NONE',  ( 7.146089767170319185, -10.01129605718032778, 34.36064277460058491 ) ) ;
#50223=CARTESIAN_POINT ( 'NONE',  ( 17.75002325595141173, -2.318417181685854978, 30.59732222474233865 ) ) ;
#50224=CARTESIAN_POINT ( 'NONE',  ( -16.21992853320628925, -9.905515769479276145, 34.41647553114623292 ) ) ;
#50225=CARTESIAN_POINT ( 'NONE',  ( 6.923076923076924238, -7.500000000000001776, 35.04278698407183867 ) ) ;
#50228=CARTESIAN_POINT ( 'NONE',  ( 17.99999999999987566, -11.67786785259630911, 32.92929555188603530 ) ) ;
#50229=CARTESIAN_POINT ( 'NONE',  ( -2.242437168179468365, -12.16647553114626490, 32.15551576947920864 ) ) ;
#50230=CARTESIAN_POINT ( 'NONE',  ( 10.55011461482829560, -5.941354392334499579, 34.76329471203369792 ) ) ;
#50232=B_SPLINE_CURVE_WITH_KNOTS ( 'NONE', 3,
 ( #33370, #19848, #25276, #12210, #53179, #52735 ),
 .UNSPECIFIED., .F., .F.,
 ( 4, 2, 4 ),
 ( 0.0003909512603273899664, 0.0005862562993132173919, 0.0007815613382990448717 ),
 .UNSPECIFIED. ) ;
#50233=AXIS2_PLACEMENT_3D ( 'NONE', #65812, #4112, #24832 ) ;
#50236=ORIENTED_EDGE ( 'NONE', *, *, #20773, .F. ) ;
#50237=CARTESIAN_POINT ( 'NONE',  ( 17.20771488474786892, -12.11778462344220841, 31.66786338562085135 ) ) ;
#50238=CARTESIAN_POINT ( 'NONE',  ( 11.53846153846153832, -5.557115091759785130, 34.35708131394839171 ) ) ;
#50239=CARTESIAN_POINT ( 'NONE',  ( 1.319345384059066983, -5.941354392334500467, 34.76329471203369792 ) ) ;
#50241=VECTOR ( 'NONE', #25533, 999.9999999999998863 ) ;
#50242=CARTESIAN_POINT ( 'NONE',  ( 3.230769230769231726, -12.48256725967547354, 35.29906147534542527 ) ) ;
#50244=CARTESIAN_POINT ( 'NONE',  ( 7.846153846153723244, -3.083524468854526912, 32.58852847137268327 ) ) ;
#50246=CARTESIAN_POINT ( 'NONE',  ( -17.07692307692307665, -12.29105614889573062, 35.45975837776705220 ) ) ;
#50247=EDGE_CURVE ( 'NONE', #87443, #43614, #1041, .T. ) ;
#50248=EDGE_LOOP ( 'NONE', ( #12800, #14754, #71895, #50442 ) ) ;
#50251=CARTESIAN_POINT ( 'NONE',  ( -6.700064078983529292, -5.582272713120727481, 34.63742843783360570 ) ) ;
#50252=CARTESIAN_POINT ( 'NONE',  ( -6.700297381808511865, -4.387253974876676565, 33.66317474335728832 ) ) ;
#50253=CARTESIAN_POINT ( 'NONE',  ( 16.28463796167093847, -2.729792928343269587, 31.24908615093345077 ) ) ;
#50254=CARTESIAN_POINT ( 'NONE',  ( -13.13466986626724342, -9.272278438253398036, 34.42582936511637115 ) ) ;
#50255=CARTESIAN_POINT ( 'NONE',  ( 17.86985203026830504, -9.504002272028873932, 34.60269587691767867 ) ) ;
#50257=ORIENTED_EDGE ( 'NONE', *, *, #44201, .F. ) ;
#50258=CYLINDRICAL_SURFACE ( 'NONE', #80873, 0.2499999999999979738 ) ;
#50259=ORIENTED_EDGE ( 'NONE', *, *, #10967, .T. ) ;
#50260=EDGE_LOOP ( 'NONE', ( #71267, #2866, #25364, #6446 ) ) ;
#50261=CARTESIAN_POINT ( 'NONE',  ( -4.153846153846152411, -13.88283147151868846, 33.14645433367849847 ) ) ;
#50263=FACE_OUTER_BOUND ( 'NONE', #34503, .T. ) ;
#50265=CARTESIAN_POINT ( 'NONE',  ( 6.000000000000001776, -5.180354513474913603, 36.12317359536750416 ) ) ;
#50266=CARTESIAN_POINT ( 'NONE',  ( -11.53846153846153655, -13.63283147151868846, 33.57946703557072254 ) ) ;
#50267=ORIENTED_EDGE ( 'NONE', *, *, #14290, .F. ) ;
#50268=EDGE_CURVE ( 'NONE', #88017, #87879, #48250, .T. ) ;
#50269=EDGE_LOOP ( 'NONE', ( #54277, #11296, #1414, #143 ) ) ;
#50271=EDGE_LOOP ( 'NONE', ( #69774, #62744, #38407, #71202 ) ) ;
#50272=CARTESIAN_POINT ( 'NONE',  ( 11.76147438255493327, -5.582272713120729257, 34.63742843783360570 ) ) ;
#50274=CARTESIAN_POINT ( 'NONE',  ( -6.923076923076922462, -12.37446782046654192, 30.86335684631486131 ) ) ;
#50275=DIRECTION ( 'NONE',  ( -0.000000000000000000, 0.7660444431189791237, -0.6427876096865379196 ) ) ;
#50279=ADVANCED_FACE ( 'NONE', ( #30796 ), #79886, .F. ) ;
#50280=CARTESIAN_POINT ( 'NONE',  ( 15.10062202133100939, -10.88202310037935661, 33.43294751532457099 ) ) ;
#50281=CARTESIAN_POINT ( 'NONE',  ( -14.30769230769242917, -8.656820664282941280, 34.87096338111179961 ) ) ;
#50282=ORIENTED_EDGE ( 'NONE', *, *, #66365, .T. ) ;
#50283=FACE_BOUND ( 'NONE', #83439, .T. ) ;
#50284=DIRECTION ( 'NONE',  ( 0.000000000000000000, 0.000000000000000000, -1.000000000000000000 ) ) ;
#50285=CARTESIAN_POINT ( 'NONE',  ( 10.83839596699746721, -9.086983370893049639, 34.49168942202179267 ) ) ;
#50286=CARTESIAN_POINT ( 'NONE',  ( -15.23076923076922995, -2.833524468853757305, 32.15551576947925838 ) ) ;
#50287=CARTESIAN_POINT ( 'NONE',  ( 4.153846153846154188, -11.69971097300155272, 32.46337939537588113 ) ) ;
#50289=CARTESIAN_POINT ( 'NONE',  ( 4.826946345980720920, -3.137211980971221781, 32.19342716148376837 ) ) ;
#50290=VECTOR ( 'NONE', #36244, 1000.000000000000227 ) ;
#50291=EDGE_CURVE ( 'NONE', #37623, #23768, #82731, .T. ) ;
#50292=CYLINDRICAL_SURFACE ( 'NONE', #33779, 0.2499999999999998890 ) ;
#50294=ORIENTED_EDGE ( 'NONE', *, *, #81563, .F. ) ;
#50295=DIRECTION ( 'NONE',  ( -0.000000000000000000, 0.9848077530122085754, -0.1736481776669273613 ) ) ;
#50297=B_SPLINE_CURVE_WITH_KNOTS ( 'NONE', 3,
 ( #63596, #77558, #15869, #2328, #51379, #73023, #37448, #24825, #3660, #32038 ),
 .UNSPECIFIED., .F., .F.,
 ( 4, 2, 2, 2, 4 ),
 ( 0.0007817246256747484735, 0.0009771112852218928873, 0.001172497944769037084, 0.001367884604316181498, 0.001563271263863325912 ),
 .UNSPECIFIED. ) ;
#50298=VECTOR ( 'NONE', #41497, 1000.000000000000000 ) ;
#50299=EDGE_LOOP ( 'NONE', ( #15348, #7305, #7719, #42864 ) ) ;
#50300=B_SPLINE_CURVE_WITH_KNOTS ( 'NONE', 3,
 ( #87413, #53153, #59477, #11289, #11743, #39219, #66226, #25248, #85619, #65775 ),
 .UNSPECIFIED., .F., .F.,
 ( 4, 2, 2, 2, 4 ),
 ( 0.0007817359430256372700, 0.0009771253907250054306, 0.001172514838424373700, 0.001367904286123741969, 0.001563293733823110021 ),
 .UNSPECIFIED. ) ;
#50302=CARTESIAN_POINT ( 'NONE',  ( -12.39547112818838670, -3.322132147404559976, 32.92929555188717927 ) ) ;
#50303=CARTESIAN_POINT ( 'NONE',  ( 10.55011416942384272, -6.879047030191174805, 34.71129190930000163 ) ) ;
#50304=CARTESIAN_POINT ( 'NONE',  ( -15.23076923076935252, -5.941354392335915335, 34.76329471203413846 ) ) ;
#50305=CARTESIAN_POINT ( 'NONE',  ( -5.999999999999998224, -12.78798330534102767, 29.49999999999997868 ) ) ;
#50307=CARTESIAN_POINT ( 'NONE',  ( 12.23805351781451201, -4.386631170607603991, 33.66268669641500111 ) ) ;
#50308=ADVANCED_FACE ( 'NONE', ( #10086 ), #65017, .F. ) ;
#50309=FACE_BOUND ( 'NONE', #12252, .T. ) ;
#50310=DIRECTION ( 'NONE',  ( -0.000000000000000000, 0.1736481776669307198, -0.9848077530122080203 ) ) ;
#50311=DIRECTION ( 'NONE',  ( -0.000000000000000000, 0.3420201433256694901, -0.9396926207859082059 ) ) ;
#50313=CARTESIAN_POINT ( 'NONE',  ( -6.673131513698879580, -10.92531984108285670, 33.72920026020278073 ) ) ;
#50314=CARTESIAN_POINT ( 'NONE',  ( -15.00775787915638126, -6.503523203565941380, 34.64991518177335195 ) ) ;
#50315=FACE_OUTER_BOUND ( 'NONE', #76741, .T. ) ;
#50317=ORIENTED_EDGE ( 'NONE', *, *, #81766, .T. ) ;
#50318=EDGE_CURVE ( 'NONE', #66274, #42667, #54170, .T. ) ;
#50320=DIRECTION ( 'NONE',  ( 0.000000000000000000, 0.9396926207859126468, -0.3420201433256571111 ) ) ;
#50321=EDGE_CURVE ( 'NONE', #4390, #76768, #84804, .T. ) ;
#50322=CARTESIAN_POINT ( 'NONE',  ( -14.43783951713053249, -6.852621066184266141, 34.70813303252209181 ) ) ;
#50324=CARTESIAN_POINT ( 'NONE',  ( 8.546364506167671848, -2.251424796025575326, 29.88072029997477586 ) ) ;
#50325=FACE_OUTER_BOUND ( 'NONE', #53954, .T. ) ;
#50327=CARTESIAN_POINT ( 'NONE',  ( -1.161652250348709003, -7.369474539155830506, 34.99858011523957657 ) ) ;
#50328=CARTESIAN_POINT ( 'NONE',  ( 18.22277954126840172, -3.236590943229497697, 32.36255958852954251 ) ) ;
#50329=CARTESIAN_POINT ( 'NONE',  ( 3.480823650682684178, -4.074993327901525575, 33.72946981652012255 ) ) ;
#50330=CARTESIAN_POINT ( 'NONE',  ( 10.36536139116316235, -6.652501968072648708, 34.93155406624980941 ) ) ;
#50331=CARTESIAN_POINT ( 'NONE',  ( 2.531067793464728766, -2.251407671071270489, 29.88021292934942252 ) ) ;
#50333=CARTESIAN_POINT ( 'NONE',  ( 10.68052939610424623, -7.750023224968867197, 34.99404313364389907 ) ) ;
#50334=CARTESIAN_POINT ( 'NONE',  ( 7.846153846153846700, -6.386643153685126251, 34.62446782046654192 ) ) ;
#50335=EDGE_CURVE ( 'NONE', #84739, #28583, #75348, .T. ) ;
#50336=ORIENTED_EDGE ( 'NONE', *, *, #46379, .T. ) ;
#50337=VECTOR ( 'NONE', #11242, 999.9999999999998863 ) ;
#50338=CYLINDRICAL_SURFACE ( 'NONE', #39873, 0.2499999999999994726 ) ;
#50339=CARTESIAN_POINT ( 'NONE',  ( -17.32689980786543060, -2.779195860258148798, 31.39871582349836743 ) ) ;
#50341=B_SPLINE_CURVE_WITH_KNOTS ( 'NONE', 3,
 ( #20805, #13609, #47834, #48273, #75742, #67671, #26237, #87979, #5530, #61331 ),
 .UNSPECIFIED., .F., .F.,
 ( 4, 2, 2, 2, 4 ),
 ( 0.0007817246256747519429, 0.0009771112852218970073, 0.001172497944769042288, 0.001367884604316187353, 0.001563271263863332417 ),
 .UNSPECIFIED. ) ;
#50342=CARTESIAN_POINT ( 'NONE',  ( 6.700149964170072359, -4.762599654559228846, 34.23009711892697737 ) ) ;
#50343=CARTESIAN_POINT ( 'NONE',  ( 17.07692307692307665, -11.35647404775217417, 33.31231777344666511 ) ) ;
#50344=ORIENTED_EDGE ( 'NONE', *, *, #20575, .T. ) ;
#50345=EDGE_CURVE ( 'NONE', #14556, #76544, #16035, .T. ) ;
#50346=CARTESIAN_POINT ( 'NONE',  ( -6.923076923076922462, -2.833524468853757305, 32.15551576947925838 ) ) ;
#50347=LINE ( 'NONE', #17019, #888 ) ;
#50348=ORIENTED_EDGE ( 'NONE', *, *, #2114, .T. ) ;
#50349=CARTESIAN_POINT ( 'NONE',  ( 11.53846153846141576, -5.094484230521993062, 34.41647553114689373 ) ) ;
#50350=CARTESIAN_POINT ( 'NONE',  ( 4.153846153846154188, -8.120952969808772792, 34.71129190930000163 ) ) ;
#50351=B_SPLINE_CURVE_WITH_KNOTS ( 'NONE', 3,
 ( #8063, #61659, #35533, #21567, #35081, #1293, #62980, #15263, #28780, #62111 ),
 .UNSPECIFIED., .F., .F.,
 ( 4, 2, 2, 2, 4 ),
 ( 0.000000000000000000, 0.0001954311564186864949, 0.0003908623128373729899, 0.0005862934692560594577, 0.0007817246256747459798 ),
 .UNSPECIFIED. ) ;
#50352=ORIENTED_EDGE ( 'NONE', *, *, #88185, .T. ) ;
#50353=CARTESIAN_POINT ( 'NONE',  ( -13.38461538461550582, -2.625532179533778709, 30.86335684631627174 ) ) ;
#50354=CARTESIAN_POINT ( 'NONE',  ( 8.899756470994333313, -5.195472089885680766, 34.18748526763464923 ) ) ;
#50355=VERTEX_POINT ( 'NONE', #81665 ) ;
#50356=FACE_OUTER_BOUND ( 'NONE', #18556, .T. ) ;
#50359=VECTOR ( 'NONE', #84889, 1000.000000000000000 ) ;
#50360=CARTESIAN_POINT ( 'NONE',  ( 15.16468685140909400, -9.905515769479276145, 34.41647553114623292 ) ) ;
#50361=ORIENTED_EDGE ( 'NONE', *, *, #12922, .F. ) ;
#50362=ORIENTED_EDGE ( 'NONE', *, *, #57103, .T. ) ;
#50363=ADVANCED_FACE ( 'NONE', ( #20402 ), #61818, .F. ) ;
#50364=ORIENTED_EDGE ( 'NONE', *, *, #84756, .T. ) ;
#50365=AXIS2_PLACEMENT_3D ( 'NONE', #74616, #4375, #86821 ) ;
#50367=EDGE_CURVE ( 'NONE', #22025, #54188, #25771, .T. ) ;
#50368=CARTESIAN_POINT ( 'NONE',  ( -18.24997673094235751, -3.627789207965225415, 32.91389620160128970 ) ) ;
#50369=CARTESIAN_POINT ( 'NONE',  ( -5.749945580086545327, -5.642605341092957083, 34.66089969410670335 ) ) ;
#50370=DIRECTION ( 'NONE',  ( -0.000000000000000000, 0.9848077530122086864, -0.1736481776669273891 ) ) ;
#50371=AXIS2_PLACEMENT_3D ( 'NONE', #65915, #29930, #78545 ) ;
#50372=EDGE_CURVE ( 'NONE', #65236, #74312, #12752, .T. ) ;
#50374=CARTESIAN_POINT ( 'NONE',  ( -2.307692307692305711, -9.905515769479276145, 34.41647553114623292 ) ) ;
#50375=ORIENTED_EDGE ( 'NONE', *, *, #76740, .F. ) ;
#50376=VERTEX_POINT ( 'NONE', #60047 ) ;
#50377=CARTESIAN_POINT ( 'NONE',  ( 4.403900573759605308, -8.346898887586323923, 34.93166121998716278 ) ) ;
#50378=EDGE_LOOP ( 'NONE', ( #32434, #69444, #5096, #51589 ) ) ;
#50379=B_SPLINE_CURVE_WITH_KNOTS ( 'NONE', 3,
 ( #77691, #29518, #70498, #55202, #84468, #82696, #69607, #55641, #70942, #7913 ),
 .UNSPECIFIED., .F., .F.,
 ( 4, 2, 2, 2, 4 ),
 ( 0.000000000000000000, 0.0001954339857564053873, 0.0003908679715128107746, 0.0005863019572692161618, 0.0007817359430256215491 ),
 .UNSPECIFIED. ) ;
#50380=CARTESIAN_POINT ( 'NONE',  ( 16.37662582282421653, -8.540255544307068902, 34.89611431652622286 ) ) ;
#50381=CYLINDRICAL_SURFACE ( 'NONE', #82474, 0.2500000000000012212 ) ;
#50382=CARTESIAN_POINT ( 'NONE',  ( 6.792928953345229282, -9.504002272028875709, 34.60269587691767867 ) ) ;
#50384=EDGE_CURVE ( 'NONE', #5929, #15629, #8536, .T. ) ;
#50385=VERTEX_POINT ( 'NONE', #26710 ) ;
#50386=CARTESIAN_POINT ( 'NONE',  ( 9.942253101685738059, -8.476813868363244353, 34.90874843262270133 ) ) ;
#50387=EDGE_LOOP ( 'NONE', ( #5401, #40417 ) ) ;
#50390=ORIENTED_EDGE ( 'NONE', *, *, #80136, .T. ) ;
#50391=CARTESIAN_POINT ( 'NONE',  ( 14.98079248672064345, -2.318417181685855422, 30.59732222474233865 ) ) ;
#50392=VECTOR ( 'NONE', #87705, 1000.000000000000227 ) ;
#50393=CARTESIAN_POINT ( 'NONE',  ( -6.923076923077044142, -12.27809138561165270, 31.22303859784587132 ) ) ;
#50394=DIRECTION ( 'NONE',  ( 0.000000000000000000, 0.1736481776669275834, 0.9848077530122086864 ) ) ;
#50395=FACE_BOUND ( 'NONE', #8137, .T. ) ;
#50396=CARTESIAN_POINT ( 'NONE',  ( 7.976679284387494739, -12.50538340440932394, 31.33453814440721885 ) ) ;
#50397=CARTESIAN_POINT ( 'NONE',  ( 11.40777007179398161, -8.147922237126337563, 34.70805685702651999 ) ) ;
#50398=CARTESIAN_POINT ( 'NONE',  ( 13.16168842570853670, -12.64616026154729411, 30.79003144601914244 ) ) ;
#50399=CARTESIAN_POINT ( 'NONE',  ( -16.82697766754503377, -12.45601412856602686, 31.48342859153981621 ) ) ;
#50400=CARTESIAN_POINT ( 'NONE',  ( 6.792385456409367528, -11.71456829005830080, 32.44064028649416542 ) ) ;
#50402=CYLINDRICAL_SURFACE ( 'NONE', #77822, 0.2499999999999995559 ) ;
#50403=ORIENTED_EDGE ( 'NONE', *, *, #7080, .T. ) ;
#50404=CARTESIAN_POINT ( 'NONE',  ( 10.39245839786847014, -10.61292498521070549, 33.66303323003028680 ) ) ;
#50405=EDGE_LOOP ( 'NONE', ( #66141, #32016, #65934, #50845 ) ) ;
#50406=VERTEX_POINT ( 'NONE', #19509 ) ;
#50407=CARTESIAN_POINT ( 'NONE',  ( 7.715462379486289990, -6.413092428213692742, 34.63065189839063152 ) ) ;
#50408=CARTESIAN_POINT ( 'NONE',  ( 10.86543903529806876, -12.01375889529407281, 32.43194544308182969 ) ) ;
#50409=CARTESIAN_POINT ( 'NONE',  ( 11.28848479441294650, -8.347322224742351082, 34.93158281831414769 ) ) ;
#50410=LINE ( 'NONE', #87231, #71091 ) ;
#50411=DIRECTION ( 'NONE',  ( 0.000000000000000000, 0.6427876096865373645, -0.7660444431189797898 ) ) ;
#50412=CARTESIAN_POINT ( 'NONE',  ( 1.161130440891438242, -11.89387501736622710, 32.13663884655806413 ) ) ;
#50413=EDGE_LOOP ( 'NONE', ( #25745, #88010, #66146, #49498 ) ) ;
#50414=LINE ( 'NONE', #27950, #54397 ) ;
#50415=ADVANCED_FACE ( 'NONE', ( #8668 ), #35237, .F. ) ;
#50416=CARTESIAN_POINT ( 'NONE',  ( 0.3308478584281529522, -12.62707690430377383, 30.88035979386743435 ) ) ;
#50417=CARTESIAN_POINT ( 'NONE',  ( -12.68502338610279345, -11.60425143139329940, 33.02411095842164457 ) ) ;
#50418=AXIS2_PLACEMENT_3D ( 'NONE', #1247, #71038, #62496 ) ;
#50420=DIRECTION ( 'NONE',  ( -0.000000000000000000, 0.9848077530122085754, -0.1736481776669273613 ) ) ;
#50421=VECTOR ( 'NONE', #9052, 1000.000000000000114 ) ;
#50424=EDGE_CURVE ( 'NONE', #18739, #33177, #4217, .T. ) ;
#50425=AXIS2_PLACEMENT_3D ( 'NONE', #86720, #45702, #87159 ) ;
#50427=ORIENTED_EDGE ( 'NONE', *, *, #19710, .T. ) ;
#50428=CARTESIAN_POINT ( 'NONE',  ( -7.846153846153844924, -11.91647553114624181, 32.58852847137148245 ) ) ;
#50429=EDGE_CURVE ( 'NONE', #83191, #17226, #27830, .T. ) ;
#50430=ORIENTED_EDGE ( 'NONE', *, *, #24615, .T. ) ;
#50436=AXIS2_PLACEMENT_3D ( 'NONE', #64800, #4908, #32372 ) ;
#50437=DIRECTION ( 'NONE',  ( -0.000000000000000000, 0.6427876096865404731, -0.7660444431189770143 ) ) ;
#50438=ORIENTED_EDGE ( 'NONE', *, *, #23238, .T. ) ;
#50440=CARTESIAN_POINT ( 'NONE',  ( -12.46153846153846168, -10.51840700105979565, 33.73612834413961536 ) ) ;
#50441=CARTESIAN_POINT ( 'NONE',  ( -2.242436736416281384, -10.90142922261932057, 33.41473453929631887 ) ) ;
#50442=ORIENTED_EDGE ( 'NONE', *, *, #58212, .F. ) ;
#50443=CARTESIAN_POINT ( 'NONE',  ( -13.45069879557126136, -11.16473453929635440, 33.15142922261925662 ) ) ;
#50444=CARTESIAN_POINT ( 'NONE',  ( -12.23875892027004397, -3.755027918224367323, 33.06320215134714857 ) ) ;
#50445=CARTESIAN_POINT ( 'NONE',  ( -17.93393164899756087, -11.69971097300155449, 32.46337939537587403 ) ) ;
#50447=CARTESIAN_POINT ( 'NONE',  ( 10.61538461538461675, -1.466349020453238561, 30.81389545987213907 ) ) ;
#50449=EDGE_CURVE ( 'NONE', #62741, #34985, #57979, .T. ) ;
#50451=ORIENTED_EDGE ( 'NONE', *, *, #72418, .F. ) ;
#50453=CARTESIAN_POINT ( 'NONE',  ( 4.403791563224197070, -10.92531984108285670, 33.72920026020278073 ) ) ;
#50455=CARTESIAN_POINT ( 'NONE',  ( -3.296039676730006196, -9.442884908240170461, 34.35708131394840592 ) ) ;
#50456=CARTESIAN_POINT ( 'NONE',  ( -4.153846153846274980, -3.643525952248796163, 33.31231777344771672 ) ) ;
#50457=ORIENTED_EDGE ( 'NONE', *, *, #9836, .T. ) ;
#50458=CARTESIAN_POINT ( 'NONE',  ( 0.2386115026316108223, -4.026226216239096267, 33.68668979543633668 ) ) ;
#50459=CARTESIAN_POINT ( 'NONE',  ( -10.61538461538461320, -13.78497067705608181, 32.30358669280327177 ) ) ;
#50460=ORIENTED_EDGE ( 'NONE', *, *, #21421, .F. ) ;
#50461=CARTESIAN_POINT ( 'NONE',  ( -9.692307692307691624, -13.53365097954675988, 30.81389545987213552 ) ) ;
#50462=ORIENTED_EDGE ( 'NONE', *, *, #13938, .F. ) ;
#50463=VECTOR ( 'NONE', #32875, 1000.000000000000000 ) ;
#50464=LINE ( 'NONE', #37396, #26179 ) ;
#50465=CARTESIAN_POINT ( 'NONE',  ( 4.153846153846154188, -3.513871655860378418, 32.76840700105978499 ) ) ;
#50466=CARTESIAN_POINT ( 'NONE',  ( -8.703163435880695076, -5.471508081941601098, 34.59228464037088457 ) ) ;
#50467=CARTESIAN_POINT ( 'NONE',  ( 16.15384615384615330, -2.292212530054420494, 30.41441678777542634 ) ) ;
#50468=VECTOR ( 'NONE', #10705, 1000.000000000000114 ) ;
#50470=CARTESIAN_POINT ( 'NONE',  ( 7.846153846153846700, -4.098570777380720287, 33.41473453929634729 ) ) ;
#50471=EDGE_CURVE ( 'NONE', #26348, #16935, #28947, .T. ) ;
#50472=VERTEX_POINT ( 'NONE', #82990 ) ;
#50473=CARTESIAN_POINT ( 'NONE',  ( -14.30769230769230660, -12.09954503811598769, 35.62045528018868623 ) ) ;
#50474=CARTESIAN_POINT ( 'NONE',  ( -4.403846153846152411, -7.433931650972300353, 34.75000000000000711 ) ) ;
#50475=VERTEX_POINT ( 'NONE', #22175 ) ;
#50476=CARTESIAN_POINT ( 'NONE',  ( 8.703148389870632329, -4.661471528628507777, 34.16647553114621871 ) ) ;
#50477=CARTESIAN_POINT ( 'NONE',  ( -12.59222992820602371, -5.582088688514999397, 34.36776431015576350 ) ) ;
#50478=CARTESIAN_POINT ( 'NONE',  ( -11.78843826940389050, -2.779195860258146578, 31.39871582349836032 ) ) ;
#50479=EDGE_CURVE ( 'NONE', #80774, #148, #8615, .T. ) ;
#50480=B_SPLINE_CURVE_WITH_KNOTS ( 'NONE', 3,
 ( #30666, #21697, #77092, #15397, #42868, #8642, #36114, #45064, #73447, #4073 ),
 .UNSPECIFIED., .F., .F.,
 ( 4, 2, 2, 2, 4 ),
 ( 0.0007817359430256390048, 0.0009771253907250078159, 0.001172514838424376735, 0.001367904286123745655, 0.001563293733823114574 ),
 .UNSPECIFIED. ) ;
#50481=CARTESIAN_POINT ( 'NONE',  ( 9.692307692307695177, -12.29105614889573062, 35.45975837776705220 ) ) ;
#50482=CARTESIAN_POINT ( 'NONE',  ( 13.38461538461538680, -13.53365097954675988, 30.81389545987213552 ) ) ;
#50483=VERTEX_POINT ( 'NONE', #14082 ) ;
#50484=ORIENTED_EDGE ( 'NONE', *, *, #72442, .F. ) ;
#50485=ADVANCED_FACE ( 'NONE', ( #69027 ), #7335, .F. ) ;
#50486=AXIS2_PLACEMENT_3D ( 'NONE', #22542, #77486, #63960 ) ;
#50487=FACE_BOUND ( 'NONE', #77345, .T. ) ;
#50489=CARTESIAN_POINT ( 'NONE',  ( -4.946878021003303871, -2.254550872974306674, 29.97347326024527447 ) ) ;
#50490=VECTOR ( 'NONE', #66390, 1000.000000000000227 ) ;
#50491=CARTESIAN_POINT ( 'NONE',  ( 17.86930939688969033, -5.496505350115500121, 34.60290016733514307 ) ) ;
#50492=CARTESIAN_POINT ( 'NONE',  ( 0.6843181305165274564, -12.69155399931963046, 30.53255429739158444 ) ) ;
#50494=AXIS2_PLACEMENT_3D ( 'NONE', #9356, #38145, #24632 ) ;
#50495=ORIENTED_EDGE ( 'NONE', *, *, #5948, .F. ) ;
#50496=ORIENTED_EDGE ( 'NONE', *, *, #1210, .T. ) ;
#50497=CARTESIAN_POINT ( 'NONE',  ( 15.23076923076911093, -9.442884908241554243, 34.35708131394783038 ) ) ;
#50499=CARTESIAN_POINT ( 'NONE',  ( -10.54931626438217585, -8.973038597847271092, 34.52809138561121216 ) ) ;
#50500=EDGE_CURVE ( 'NONE', #84435, #71169, #33269, .T. ) ;
#50501=EDGE_CURVE ( 'NONE', #88089, #77626, #5884, .T. ) ;
#50502=LINE ( 'NONE', #77102, #8607 ) ;
#50503=B_SPLINE_CURVE_WITH_KNOTS ( 'NONE', 3,
 ( #59488, #12200, #32023, #32913, #4999, #51822, #86539, #11304, #38782, #73904 ),
 .UNSPECIFIED., .F., .F.,
 ( 4, 2, 2, 2, 4 ),
 ( 0.0007817246256747447872, 0.0009771112852218876831, 0.001172497944769030579, 0.001367884604316173475, 0.001563271263863316371 ),
 .UNSPECIFIED. ) ;
#50504=CARTESIAN_POINT ( 'NONE',  ( -2.307692307692428724, -12.51329471203414379, 31.30864560766407578 ) ) ;
#50505=EDGE_CURVE ( 'NONE', #68329, #69454, #68030, .T. ) ;
#50506=FACE_BOUND ( 'NONE', #40054, .T. ) ;
#50507=EDGE_LOOP ( 'NONE', ( #9748, #44946 ) ) ;
#50508=CYLINDRICAL_SURFACE ( 'NONE', #34219, 0.2500000000000009437 ) ;
#50509=B_SPLINE_CURVE_WITH_KNOTS ( 'NONE', 3,
 ( #49581, #43269, #70743, #57223, #22987, #82933, #75714, #14019, #7270, #34736 ),
 .UNSPECIFIED., .F., .F.,
 ( 4, 2, 2, 2, 4 ),
 ( 0.0007817246256747469556, 0.0009771112852218902852, 0.001172497944769033615, 0.001367884604316176728, 0.001563271263863320057 ),
 .UNSPECIFIED. ) ;
#50510=CYLINDRICAL_SURFACE ( 'NONE', #41898, 0.2499999999999979738 ) ;
#50511=CARTESIAN_POINT ( 'NONE',  ( -14.53061852520845498, -9.086856451489515152, 34.49173150075333183 ) ) ;
#50512=CARTESIAN_POINT ( 'NONE',  ( 10.61538461538461675, -3.886160181151819604, 36.00935417666054406 ) ) ;
#50516=CARTESIAN_POINT ( 'NONE',  ( -7.846153846153965716, -6.879047030192662504, 34.71129190930017927 ) ) ;
#50518=CARTESIAN_POINT ( 'NONE',  ( 16.15384615384615330, -5.557115091759785130, 34.35708131394839171 ) ) ;
#50519=CARTESIAN_POINT ( 'NONE',  ( -3.296852641725110278, -11.16473453929635440, 33.15142922261925662 ) ) ;
#50520=CARTESIAN_POINT ( 'NONE',  ( -9.692307692307691624, -3.886160181151819604, 36.00935417666054406 ) ) ;
#50521=CARTESIAN_POINT ( 'NONE',  ( 14.17754433796061164, -3.069018819979302926, 32.56621877034667278 ) ) ;
#50523=CARTESIAN_POINT ( 'NONE',  ( 11.53846153846141576, -5.094484230521993062, 34.41647553114689373 ) ) ;
#50524=LINE ( 'NONE', #16744, #67560 ) ;
#50525=CARTESIAN_POINT ( 'NONE',  ( -4.153846153846152411, -1.951392089020283160, 34.73218667398347748 ) ) ;
#50526=CYLINDRICAL_SURFACE ( 'NONE', #58254, 0.2499999999999979738 ) ;
#50527=AXIS2_PLACEMENT_3D ( 'NONE', #87594, #54215, #24976 ) ;
#50528=ORIENTED_EDGE ( 'NONE', *, *, #82274, .T. ) ;
#50529=FACE_OUTER_BOUND ( 'NONE', #71735, .T. ) ;
#50530=B_SPLINE_CURVE_WITH_KNOTS ( 'NONE', 3,
 ( #44238, #4155, #10030, #3269, #23978, #59550, #86152, #52790, #79836, #30741 ),
 .UNSPECIFIED., .F., .F.,
 ( 4, 2, 2, 2, 4 ),
 ( 0.000000000000000000, 0.0001954311564186860071, 0.0003908623128373720141, 0.0005862934692560580483, 0.0007817246256747440282 ),
 .UNSPECIFIED. ) ;
#50531=EDGE_LOOP ( 'NONE', ( #21754, #72400 ) ) ;
#50532=FACE_BOUND ( 'NONE', #23102, .T. ) ;
#50533=EDGE_CURVE ( 'NONE', #60787, #82557, #26595, .T. ) ;
#50534=FACE_OUTER_BOUND ( 'NONE', #47018, .T. ) ;
#50535=CARTESIAN_POINT ( 'NONE',  ( 18.13052543823364360, -12.70449254468099198, 30.44128974285582956 ) ) ;
#50536=CARTESIAN_POINT ( 'NONE',  ( -11.47239318745909742, -11.69971097300155272, 32.46337939537588113 ) ) ;
#50538=DIRECTION ( 'NONE',  ( -0.000000000000000000, -0.9396926207859092051, -0.3420201433256662704 ) ) ;
#50539=CARTESIAN_POINT ( 'NONE',  ( -10.61538461538461320, -6.386643153685126251, 34.62446782046654192 ) ) ;
#50540=CARTESIAN_POINT ( 'NONE',  ( -11.53846153846153655, -4.661471528628507777, 34.16647553114623292 ) ) ;
#50543=DIRECTION ( 'NONE',  ( -0.000000000000000000, -0.9396926207859093161, -0.3420201433256663259 ) ) ;
#50544=ORIENTED_EDGE ( 'NONE', *, *, #15567, .T. ) ;
#50545=EDGE_CURVE ( 'NONE', #43177, #52380, #7121, .T. ) ;
#50546=CARTESIAN_POINT ( 'NONE',  ( 13.51514082284903040, -8.630441415882550871, 34.87705825610312615 ) ) ;
#50547=EDGE_LOOP ( 'NONE', ( #35343, #44758 ) ) ;
#50548=CARTESIAN_POINT ( 'NONE',  ( 7.716006636715626144, -10.88202310037936194, 33.43294751532457099 ) ) ;
#50549=CARTESIAN_POINT ( 'NONE',  ( -17.07692307692307665, -2.708943851104267164, 35.45975837776705220 ) ) ;
#50550=FACE_OUTER_BOUND ( 'NONE', #57003, .T. ) ;
#50551=CARTESIAN_POINT ( 'NONE',  ( -12.71156168575991963, -10.92453946501458795, 33.72985991061850086 ) ) ;
#50552=CARTESIAN_POINT ( 'NONE',  ( -6.923076923076922462, -9.819645486525091727, 36.12317359536749706 ) ) ;
#50553=B_SPLINE_CURVE_WITH_KNOTS ( 'NONE', 3,
 ( #75766, #77104, #35227, #28476, #55939, #15413, #63583, #76664, #28030, #1885 ),
 .UNSPECIFIED., .F., .F.,
 ( 4, 2, 2, 2, 4 ),
 ( 0.000000000000000000, 0.0001954311564186888531, 0.0003908623128373777062, 0.0005862934692560666135, 0.0007817246256747554124 ),
 .UNSPECIFIED. ) ;
#50554=B_SPLINE_CURVE_WITH_KNOTS ( 'NONE', 3,
 ( #42581, #29511, #63281, #57409, #78129, #36269, #50650, #1591, #43460, #37136 ),
 .UNSPECIFIED., .F., .F.,
 ( 4, 2, 2, 2, 4 ),
 ( 0.0007817246256747505334, 0.0009771112852218954894, 0.001172497944769040554, 0.001367884604316185618, 0.001563271263863330682 ),
 .UNSPECIFIED. ) ;
#50555=CARTESIAN_POINT ( 'NONE',  ( -9.915792616872019849, -12.11044203135681840, 32.26167407432752299 ) ) ;
#50556=B_SPLINE_CURVE_WITH_KNOTS ( 'NONE', 3,
 ( #59298, #58852, #3015, #18323, #45785, #86358, #79585, #44434, #17882, #45336 ),
 .UNSPECIFIED., .F., .F.,
 ( 4, 2, 2, 2, 4 ),
 ( 0.000000000000000000, 0.0001954311564186862781, 0.0003908623128373725562, 0.0005862934692560588072, 0.0007817246256747451124 ),
 .UNSPECIFIED. ) ;
#50559=ORIENTED_EDGE ( 'NONE', *, *, #74213, .F. ) ;
#50560=B_SPLINE_CURVE_WITH_KNOTS ( 'NONE', 3,
 ( #19221, #31851, #25532, #59309, #87251, #4821, #81373, #25969, #74163, #19657 ),
 .UNSPECIFIED., .F., .F.,
 ( 4, 2, 2, 2, 4 ),
 ( 0.000000000000000000, 0.0001954311564186879044, 0.0003908623128373758088, 0.0005862934692560636861, 0.0007817246256747516176 ),
 .UNSPECIFIED. ) ;
#50561=CARTESIAN_POINT ( 'NONE',  ( -0.5268089074992370335, -6.026961402152685388, 34.52809138561120506 ) ) ;
#50562=DIRECTION ( 'NONE',  ( -0.000000000000000000, -0.9848077530122086864, -0.1736481776669273613 ) ) ;
#50563=ORIENTED_EDGE ( 'NONE', *, *, #16052, .T. ) ;
#50564=ORIENTED_EDGE ( 'NONE', *, *, #19101, .F. ) ;
#50565=ORIENTED_EDGE ( 'NONE', *, *, #61274, .F. ) ;
#50566=CARTESIAN_POINT ( 'NONE',  ( -10.74553182482283198, -11.47017969459904130, 32.78971311882034456 ) ) ;
#50567=DIRECTION ( 'NONE',  ( 1.000000000000000000, -0.000000000000000000, -0.000000000000000000 ) ) ;
#50568=CARTESIAN_POINT ( 'NONE',  ( -5.999999999999998224, -12.62096338111211580, 30.90682066428153263 ) ) ;
#50569=AXIS2_PLACEMENT_3D ( 'NONE', #77815, #1272, #56225 ) ;
#50570=DIRECTION ( 'NONE',  ( -0.000000000000000000, -0.9848077530122085754, -0.1736481776669273613 ) ) ;
#50571=DIRECTION ( 'NONE',  ( -0.000000000000000000, 0.9848077530122086864, -0.1736481776669273891 ) ) ;
#50572=EDGE_CURVE ( 'NONE', #45405, #81436, #66237, .T. ) ;
#50573=LINE ( 'NONE', #40631, #54271 ) ;
#50574=DIRECTION ( 'NONE',  ( -0.000000000000000000, -0.5000000000000009992, -0.8660254037844380415 ) ) ;
#50575=ORIENTED_EDGE ( 'NONE', *, *, #5336, .T. ) ;
#50576=CARTESIAN_POINT ( 'NONE',  ( -0.4615384615384611200, -13.95598074871891292, 31.83374038241031911 ) ) ;
#50577=CARTESIAN_POINT ( 'NONE',  ( -1.634592115557738090, -6.567427716900047230, 34.66269422305636283 ) ) ;
#50578=CARTESIAN_POINT ( 'NONE',  ( -18.00000000000000000, -12.62096338111211580, 30.90682066428153263 ) ) ;
#50579=CARTESIAN_POINT ( 'NONE',  ( 8.096099364501990081, -2.824170634883622633, 31.52227843825338738 ) ) ;
#50580=ORIENTED_EDGE ( 'NONE', *, *, #46184, .T. ) ;
#50581=LINE ( 'NONE', #2829, #65702 ) ;
#50582=EDGE_CURVE ( 'NONE', #18632, #34976, #23514, .T. ) ;
#50584=CARTESIAN_POINT ( 'NONE',  ( 8.992243613324166773, -2.889357225399416418, 32.26129605718031002 ) ) ;
#50585=CARTESIAN_POINT ( 'NONE',  ( 3.230769230769108269, -11.06231777344772027, 33.60647404775119895 ) ) ;
#50586=CARTESIAN_POINT ( 'NONE',  ( 1.384615384615264011, -11.67786785259630911, 32.92929555188603530 ) ) ;
#50588=EDGE_CURVE ( 'NONE', #61992, #70675, #13955, .T. ) ;
#50589=DIRECTION ( 'NONE',  ( 0.000000000000000000, 0.4999999999999985567, 0.8660254037844395958 ) ) ;
#50590=B_SPLINE_CURVE_WITH_KNOTS ( 'NONE', 3,
 ( #371, #47214, #75570, #1241, #68377, #54865, #7570, #8012, #28732, #74708 ),
 .UNSPECIFIED., .F., .F.,
 ( 4, 2, 2, 2, 4 ),
 ( 0.000000000000000000, 0.0001954339857564073659, 0.0003908679715128147319, 0.0005863019572692221250, 0.0007817359430256294638 ),
 .UNSPECIFIED. ) ;
#50591=CARTESIAN_POINT ( 'NONE',  ( -12.52729526405276772, -7.249945686854186278, 34.74374336980224598 ) ) ;
#50592=B_SPLINE_CURVE_WITH_KNOTS ( 'NONE', 3,
 ( #20397, #11874, #87548, #88003, #61811, #66810, #53731, #34342, #39351, #13198 ),
 .UNSPECIFIED., .F., .F.,
 ( 4, 2, 2, 2, 4 ),
 ( 0.000000000000000000, 0.0001954339857564098054, 0.0003908679715128196108, 0.0005863019572692293891, 0.0007817359430256392216 ),
 .UNSPECIFIED. ) ;
#50593=AXIS2_PLACEMENT_3D ( 'NONE', #2764, #45096, #10879 ) ;
#50594=CARTESIAN_POINT ( 'NONE',  ( -2.980714919130916574, -12.17597550085003455, 31.52189283813461884 ) ) ;
#50595=B_SPLINE_CURVE_WITH_KNOTS ( 'NONE', 3,
 ( #87367, #60312, #87821, #72941, #10801, #38270 ),
 .UNSPECIFIED., .F., .F.,
 ( 4, 2, 4 ),
 ( 0.0003909569690057415072, 0.0005862646681845472664, 0.0007815723673633529715 ),
 .UNSPECIFIED. ) ;
#50597=ORIENTED_EDGE ( 'NONE', *, *, #66981, .T. ) ;
#50598=CARTESIAN_POINT ( 'NONE',  ( -10.61538461538430589, -2.506253911140614576, 30.00000000000323297 ) ) ;
#50599=EDGE_CURVE ( 'NONE', #83223, #22047, #37548, .T. ) ;
#50600=ORIENTED_EDGE ( 'NONE', *, *, #37251, .T. ) ;
#50601=AXIS2_PLACEMENT_3D ( 'NONE', #74518, #5173, #80400 ) ;
#50602=DIRECTION ( 'NONE',  ( -0.000000000000000000, 0.3420201433256694346, -0.9396926207859080948 ) ) ;
#50604=CARTESIAN_POINT ( 'NONE',  ( -7.911423846710166075, -2.657715359629089225, 31.77849191805832874 ) ) ;
#50605=CARTESIAN_POINT ( 'NONE',  ( -14.30769230769230660, -9.780366693483667717, 34.19971097300155094 ) ) ;
#50606=CARTESIAN_POINT ( 'NONE',  ( 18.24994540937804643, -8.476813868363244353, 34.90874843262270133 ) ) ;
#50607=EDGE_CURVE ( 'NONE', #38805, #57991, #25262, .T. ) ;
#50610=ADVANCED_FACE ( 'NONE', ( #34684 ), #63012, .F. ) ;
#50611=VERTEX_POINT ( 'NONE', #54500 ) ;
#50613=EDGE_LOOP ( 'NONE', ( #27826, #57637, #87693, #47226 ) ) ;
#50614=LINE ( 'NONE', #58699, #35870 ) ;
#50615=DIRECTION ( 'NONE',  ( -0.000000000000000000, -0.000000000000000000, -1.000000000000000000 ) ) ;
#50616=CARTESIAN_POINT ( 'NONE',  ( 17.29970261819148902, -4.387253974876675677, 33.66317474335728832 ) ) ;
#50617=AXIS2_PLACEMENT_3D ( 'NONE', #16206, #21632, #36485 ) ;
#50618=CARTESIAN_POINT ( 'NONE',  ( 0.3962684609821411907, -12.51329471203370325, 31.30864560766548976 ) ) ;
#50619=CARTESIAN_POINT ( 'NONE',  ( -4.153846153846152411, -12.78798330534102945, 29.74999999999997868 ) ) ;
#50620=CARTESIAN_POINT ( 'NONE',  ( 5.076923076923075762, -9.780366693483667717, 34.19971097300155094 ) ) ;
#50622=VERTEX_POINT ( 'NONE', #7658 ) ;
#50623=AXIS2_PLACEMENT_3D ( 'NONE', #23216, #2935, #52014 ) ;
#50626=ORIENTED_EDGE ( 'NONE', *, *, #56622, .T. ) ;
#50627=CARTESIAN_POINT ( 'NONE',  ( 0.5276068125408990284, -8.120952969808772792, 34.71129190929999453 ) ) ;
#50628=CARTESIAN_POINT ( 'NONE',  ( -8.519285250882626670, -11.37275283266504111, 32.91324779482534524 ) ) ;
#50629=B_SPLINE_CURVE_WITH_KNOTS ( 'NONE', 3,
 ( #27032, #87421, #67580, #20278, #66688, #47742, #80663, #19831, #75226, #33787 ),
 .UNSPECIFIED., .F., .F.,
 ( 4, 2, 2, 2, 4 ),
 ( 0.0007817246256747448956, 0.0009771112852218876831, 0.001172497944769030579, 0.001367884604316173475, 0.001563271263863316371 ),
 .UNSPECIFIED. ) ;
#50630=CARTESIAN_POINT ( 'NONE',  ( -1.384615384615383471, -4.661471528628507777, 34.16647553114623292 ) ) ;
#50632=ORIENTED_EDGE ( 'NONE', *, *, #25470, .T. ) ;
#50634=CARTESIAN_POINT ( 'NONE',  ( -17.93474486048716088, -3.083524468853784839, 32.58852847137153930 ) ) ;
#50635=ORIENTED_EDGE ( 'NONE', *, *, #59028, .T. ) ;
#50636=FACE_BOUND ( 'NONE', #37459, .T. ) ;
#50637=CARTESIAN_POINT ( 'NONE',  ( 15.00728428704528561, -10.11188796281391511, 34.01382737946119050 ) ) ;
#50638=DIRECTION ( 'NONE',  ( 0.000000000000000000, 0.9396926207859126468, 0.3420201433256571111 ) ) ;
#50640=CARTESIAN_POINT ( 'NONE',  ( -15.23076923076922995, -4.786620604624113540, 33.94971097300155094 ) ) ;
#50641=DIRECTION ( 'NONE',  ( -0.000000000000000000, 0.8660254037844399289, -0.4999999999999980016 ) ) ;
#50642=CARTESIAN_POINT ( 'NONE',  ( 12.21153846153846168, -7.500000000000001776, 34.75000000000000000 ) ) ;
#50644=CARTESIAN_POINT ( 'NONE',  ( -2.307692307692305711, -8.164416787775445883, 34.95778746994557906 ) ) ;
#50645=CYLINDRICAL_SURFACE ( 'NONE', #44485, 0.2500000000000009437 ) ;
#50646=AXIS2_PLACEMENT_3D ( 'NONE', #76238, #49221, #1479 ) ;
#50647=CARTESIAN_POINT ( 'NONE',  ( 12.46153846153846168, -5.471508081941601098, 34.59228464037088457 ) ) ;
#50648=CARTESIAN_POINT ( 'NONE',  ( 2.177001704582001818, -11.93127051446800024, 32.56575433478200665 ) ) ;
#50650=CARTESIAN_POINT ( 'NONE',  ( 13.60762822870878352, -2.308499170217967134, 30.53291367094873721 ) ) ;
#50651=CARTESIAN_POINT ( 'NONE',  ( -12.46153846153846168, -2.499999999999998668, 29.75000000000001421 ) ) ;
#50652=CARTESIAN_POINT ( 'NONE',  ( 8.834485908743602067, -4.320704448112861584, 33.92786785259548310 ) ) ;
#50653=CARTESIAN_POINT ( 'NONE',  ( -13.38461538461550759, -4.320704448113951379, 33.92786785259630022 ) ) ;
#50654=CARTESIAN_POINT ( 'NONE',  ( 11.60452988946397745, -4.098570777380720287, 33.41473453929635440 ) ) ;
#50655=CYLINDRICAL_SURFACE ( 'NONE', #74148, 0.2499999999999995559 ) ;
#50656=CARTESIAN_POINT ( 'NONE',  ( 4.023698184114459231, -5.915902021225892149, 34.75552854090298638 ) ) ;
#50657=DIRECTION ( 'NONE',  ( -0.000000000000000000, 1.000000000000000000, 3.491481338843133355E-15 ) ) ;
#50658=DIRECTION ( 'NONE',  ( -0.000000000000000000, 1.000000000000000000, 3.491481338843133355E-15 ) ) ;
#50662=ORIENTED_EDGE ( 'NONE', *, *, #29147, .T. ) ;
#50663=CARTESIAN_POINT ( 'NONE',  ( -9.915792636031639518, -5.912607949931405926, 34.49155766932282319 ) ) ;
#50664=VERTEX_POINT ( 'NONE', #6332 ) ;
#50665=CARTESIAN_POINT ( 'NONE',  ( -3.903791842207838148, -11.28795663066794219, 33.01431243580653785 ) ) ;
#50666=VERTEX_POINT ( 'NONE', #54952 ) ;
#50669=CARTESIAN_POINT ( 'NONE',  ( -18.00000000000000000, -9.058645607665452459, 34.76329471203371924 ) ) ;
#50670=DIRECTION ( 'NONE',  ( -0.000000000000000000, 1.000000000000000000, -0.000000000000000000 ) ) ;
#50671=CARTESIAN_POINT ( 'NONE',  ( -5.299850035829926753, -2.889293201056495786, 32.26117774369186009 ) ) ;
#50672=FACE_OUTER_BOUND ( 'NONE', #10102, .T. ) ;
#50673=CARTESIAN_POINT ( 'NONE',  ( 14.98076923076922817, -7.566083408709835645, 34.74999999999999289 ) ) ;
#50674=CARTESIAN_POINT ( 'NONE',  ( -14.24243716817946925, -5.094484230520773593, 34.41647553114626845 ) ) ;
#50676=CARTESIAN_POINT ( 'NONE',  ( 18.13052543823364360, -11.66157788607254275, 32.95092075102925833 ) ) ;
#50677=CARTESIAN_POINT ( 'NONE',  ( -15.16551365949320740, -2.625532179533470512, 30.86335684631491105 ) ) ;
#50678=CARTESIAN_POINT ( 'NONE',  ( 10.36536139116315880, -5.765609946408404518, 34.70566812827425451 ) ) ;
#50680=VECTOR ( 'NONE', #54104, 1000.000000000000114 ) ;
#50682=CARTESIAN_POINT ( 'NONE',  ( -14.17690049986752143, -10.54018710029568595, 33.71981072465678864 ) ) ;
#50684=ORIENTED_EDGE ( 'NONE', *, *, #3994, .F. ) ;
#50685=CARTESIAN_POINT ( 'NONE',  ( 14.37376065869474751, -4.786620604624113540, 33.94971097300155805 ) ) ;
#50686=CARTESIAN_POINT ( 'NONE',  ( -11.40793583669797506, -8.586989748646452369, 34.63063291749215011 ) ) ;
#50687=CARTESIAN_POINT ( 'NONE',  ( 1.161130440891438687, -12.44517049084099725, 30.48991314939691932 ) ) ;
#50688=CARTESIAN_POINT ( 'NONE',  ( 1.634615384615386580, -2.499999999999998668, 29.75000000000000355 ) ) ;
#50690=VECTOR ( 'NONE', #22243, 1000.000000000000227 ) ;
#50691=CARTESIAN_POINT ( 'NONE',  ( 9.627037246346917598, -11.48612834413959582, 32.76840700105983473 ) ) ;
#50692=ADVANCED_FACE ( 'NONE', ( #76554 ), #22051, .F. ) ;
#50694=DIRECTION ( 'NONE',  ( 0.000000000000000000, 0.3420201433256610524, 0.9396926207859113145 ) ) ;
#50695=EDGE_LOOP ( 'NONE', ( #76089, #68433, #69706, #60521 ) ) ;
#50697=CARTESIAN_POINT ( 'NONE',  ( 14.98079249982687777, -6.567427716900048118, 34.66269422305636283 ) ) ;
#50698=CARTESIAN_POINT ( 'NONE',  ( -11.53846153846153655, -11.35647404775217417, 33.31231777344666511 ) ) ;
#50699=DIRECTION ( 'NONE',  ( -0.000000000000000000, -0.9396926207859092051, -0.3420201433256662704 ) ) ;
#50700=CARTESIAN_POINT ( 'NONE',  ( 1.450683735617825709, -11.69971097300155272, 32.46337939537588113 ) ) ;
#50701=LINE ( 'NONE', #70548, #32312 ) ;
#50702=ORIENTED_EDGE ( 'NONE', *, *, #63653, .T. ) ;
#50703=CYLINDRICAL_SURFACE ( 'NONE', #63675, 0.2499999999999986955 ) ;
#50704=VECTOR ( 'NONE', #39288, 1000.000000000000000 ) ;
#50707=ORIENTED_EDGE ( 'NONE', *, *, #41608, .F. ) ;
#50708=CARTESIAN_POINT ( 'NONE',  ( -6.989159302437059296, -11.91647553114624181, 32.58852847137148245 ) ) ;
#50710=DIRECTION ( 'NONE',  ( -0.000000000000000000, 1.000000000000000000, 3.491481338843133355E-15 ) ) ;
#50711=EDGE_CURVE ( 'NONE', #33924, #25611, #19228, .T. ) ;
#50712=CARTESIAN_POINT ( 'NONE',  ( -11.53846153846153655, -8.164416787775445883, 34.95778746994557906 ) ) ;
#50713=DIRECTION ( 'NONE',  ( -0.000000000000000000, 1.000000000000000000, -0.000000000000000000 ) ) ;
#50714=ORIENTED_EDGE ( 'NONE', *, *, #65991, .T. ) ;
#50718=CARTESIAN_POINT ( 'NONE',  ( -2.372962753653081514, -2.892918686051582533, 31.69288490824015270 ) ) ;
#50720=CARTESIAN_POINT ( 'NONE',  ( 1.450683735617824599, -8.973038597847269315, 34.52809138561122637 ) ) ;
#50721=CARTESIAN_POINT ( 'NONE',  ( 10.61538461538461675, -3.050289026998446396, 32.03036669348365706 ) ) ;
#50722=CARTESIAN_POINT ( 'NONE',  ( -0.4615384615384611200, -9.058645607665452459, 34.76329471203371924 ) ) ;
#50723=VERTEX_POINT ( 'NONE', #41439 ) ;
#50724=DIRECTION ( 'NONE',  ( 0.000000000000000000, 0.6427876096865373645, -0.7660444431189797898 ) ) ;
#50726=CARTESIAN_POINT ( 'NONE',  ( 17.07692307692307665, -2.538708090699994813, 30.37095296980875503 ) ) ;
#50727=DIRECTION ( 'NONE',  ( 0.000000000000000000, 0.9396926207859126468, 0.3420201433256571111 ) ) ;
#50729=CARTESIAN_POINT ( 'NONE',  ( -17.86947456176635640, -2.647132371071621026, 31.75357179365173010 ) ) ;
#50730=CARTESIAN_POINT ( 'NONE',  ( 0.4615384615384611200, -11.35647404775217417, 33.31231777344666511 ) ) ;
#50731=CARTESIAN_POINT ( 'NONE',  ( 4.153846153846030731, -5.941354392335915335, 34.76329471203413846 ) ) ;
#50732=VECTOR ( 'NONE', #8766, 1000.000000000000227 ) ;
#50733=CARTESIAN_POINT ( 'NONE',  ( 16.15384615384603251, -2.625532179533778709, 30.86335684631627174 ) ) ;
#50734=CARTESIAN_POINT ( 'NONE',  ( -0.4615384615385840772, -12.70778746994576025, 30.41441678777401236 ) ) ;
#50735=EDGE_LOOP ( 'NONE', ( #471, #10180, #38622, #32091 ) ) ;
#50736=LINE ( 'NONE', #64252, #71981 ) ;
#50738=ORIENTED_EDGE ( 'NONE', *, *, #44442, .F. ) ;
#50739=VECTOR ( 'NONE', #31334, 1000.000000000000227 ) ;
#50740=B_SPLINE_CURVE_WITH_KNOTS ( 'NONE', 3,
 ( #61498, #59403, #27277, #48424, #86454, #82231, #17980, #41244, #86904, #52638 ),
 .UNSPECIFIED., .F., .F.,
 ( 4, 2, 2, 2, 4 ),
 ( 0.0007817246256747486903, 0.0009771112852218918031, 0.001172497944769034699, 0.001367884604316177595, 0.001563271263863320708 ),
 .UNSPECIFIED. ) ;
#50741=B_SPLINE_CURVE_WITH_KNOTS ( 'NONE', 3,
 ( #31937, #65695, #23817, #64803, #80117, #10325, #85988, #31483, #9874, #45878 ),
 .UNSPECIFIED., .F., .F.,
 ( 4, 2, 2, 2, 4 ),
 ( 0.000000000000000000, 0.0001954339857564077183, 0.0003908679715128154366, 0.0005863019572692231007, 0.0007817359430256308733 ),
 .UNSPECIFIED. ) ;
#50742=DIRECTION ( 'NONE',  ( -0.000000000000000000, -0.5000000000000009992, -0.8660254037844380415 ) ) ;
#50743=CARTESIAN_POINT ( 'NONE',  ( 15.23076923076923173, -4.098570777380720287, 33.41473453929634729 ) ) ;
#50744=CARTESIAN_POINT ( 'NONE',  ( 3.361607648781993696, -7.277220443632450575, 34.74524770363009196 ) ) ;
#50745=LINE ( 'NONE', #50305, #10190 ) ;
#50746=CARTESIAN_POINT ( 'NONE',  ( -0.4615384615384611200, -12.37446782046654192, 30.86335684631486131 ) ) ;
#50747=CARTESIAN_POINT ( 'NONE',  ( -8.096153846153844924, -7.500000000000001776, 35.00000000000000000 ) ) ;
#50748=FACE_BOUND ( 'NONE', #87968, .T. ) ;
#50749=CARTESIAN_POINT ( 'NONE',  ( 13.13463864056679675, -2.318417181685855422, 30.59732222474233865 ) ) ;
#50750=DIRECTION ( 'NONE',  ( 0.000000000000000000, -6.938893903907222067E-15, 1.000000000000000000 ) ) ;
#50751=CARTESIAN_POINT ( 'NONE',  ( -6.792551221313359200, -10.88167719472716399, 33.43325721877153711 ) ) ;
#50752=CARTESIAN_POINT ( 'NONE',  ( -4.946397638689432164, -10.31582465632705237, 34.18122507451815295 ) ) ;
#50753=CARTESIAN_POINT ( 'NONE',  ( -14.05769230769237055, -7.565270000091922853, 34.99999999999999289 ) ) ;
#50756=ORIENTED_EDGE ( 'NONE', *, *, #42757, .F. ) ;
#50757=CARTESIAN_POINT ( 'NONE',  ( 15.93036122928182330, -9.417330523894424488, 34.63758898049880486 ) ) ;
#50758=CARTESIAN_POINT ( 'NONE',  ( -14.30769230769230660, -6.386643153685126251, 34.62446782046654192 ) ) ;
#50759=DIRECTION ( 'NONE',  ( -0.000000000000000000, 0.9848077530122086864, -0.1736481776669273891 ) ) ;
#50760=CARTESIAN_POINT ( 'NONE',  ( -10.74607521849492464, -11.37499894934982692, 33.29245874905763003 ) ) ;
#50761=CARTESIAN_POINT ( 'NONE',  ( 7.846153846153725020, -5.219633306517616589, 34.19971097300220464 ) ) ;
#50763=EDGE_CURVE ( 'NONE', #32348, #18061, #49377, .T. ) ;
#50764=CARTESIAN_POINT ( 'NONE',  ( -2.307692307692428724, -3.643525952248796163, 33.31231777344771672 ) ) ;
#50767=CARTESIAN_POINT ( 'NONE',  ( 11.76188793737632743, -7.630147987733840509, 34.99859428049665411 ) ) ;
#50769=CARTESIAN_POINT ( 'NONE',  ( 14.30769230769231015, -9.819645486525091727, 36.12317359536749706 ) ) ;
#50770=CARTESIAN_POINT ( 'NONE',  ( 4.088575707885377497, -10.90142922261923886, 33.41473453929638993 ) ) ;
#50771=CARTESIAN_POINT ( 'NONE',  ( -18.06527044596077047, -2.892918686051583421, 31.69288490824015270 ) ) ;
#50773=EDGE_LOOP ( 'NONE', ( #83013, #62242, #19858, #66036 ) ) ;
#50774=CARTESIAN_POINT ( 'NONE',  ( 17.32697749683652688, -12.65882529074907126, 30.72640787790838601 ) ) ;
#50775=CARTESIAN_POINT ( 'NONE',  ( -6.000000000000121680, -2.657715359629662988, 31.77849191805970364 ) ) ;
#50777=EDGE_CURVE ( 'NONE', #63664, #29143, #6757, .T. ) ;
#50778=CARTESIAN_POINT ( 'NONE',  ( 6.988332062589762472, -11.06231777344671130, 33.60647404775212976 ) ) ;
#50779=CARTESIAN_POINT ( 'NONE',  ( 3.453548772037640546, -11.89424750095246175, 32.13594075562311758 ) ) ;
#50780=ORIENTED_EDGE ( 'NONE', *, *, #77427, .F. ) ;
#50782=CARTESIAN_POINT ( 'NONE',  ( -0.4615384615384611200, -3.513871655860378418, 32.76840700105978499 ) ) ;
#50784=CARTESIAN_POINT ( 'NONE',  ( -3.903846153846152855, -2.249999999999998668, 29.75000000000000355 ) ) ;
#50785=CARTESIAN_POINT ( 'NONE',  ( 23.00000000000000000, -9.499999999999982236, 27.25000000000000000 ) ) ;
#50786=ADVANCED_FACE ( 'NONE', ( #13517 ), #55831, .F. ) ;
#50788=FACE_OUTER_BOUND ( 'NONE', #77098, .T. ) ;
#50789=ORIENTED_EDGE ( 'NONE', *, *, #35536, .T. ) ;
#50790=CARTESIAN_POINT ( 'NONE',  ( -13.38461538461538325, -12.09954503811598769, 35.62045528018868623 ) ) ;
#50791=CARTESIAN_POINT ( 'NONE',  ( 5.326923076923075762, -2.249999999999998668, 29.75000000000000355 ) ) ;
#50792=AXIS2_PLACEMENT_3D ( 'NONE', #71761, #38435, #86642 ) ;
#50793=CARTESIAN_POINT ( 'NONE',  ( -1.253823576790597194, -5.582136614379148654, 34.36778462344220486 ) ) ;
#50794=EDGE_CURVE ( 'NONE', #20449, #45365, #71856, .T. ) ;
#50796=ORIENTED_EDGE ( 'NONE', *, *, #20634, .T. ) ;
#50797=AXIS2_PLACEMENT_3D ( 'NONE', #23541, #50574, #50998 ) ;
#50798=EDGE_LOOP ( 'NONE', ( #46295, #84521 ) ) ;
#50799=ADVANCED_FACE ( 'NONE', ( #78304 ), #23362, .F. ) ;
#50800=CARTESIAN_POINT ( 'NONE',  ( 3.296836564119307589, -2.292212530054420494, 30.41441678777542990 ) ) ;
#50801=CARTESIAN_POINT ( 'NONE',  ( 9.823098133274648092, -3.957578996910242619, 33.62503395064540257 ) ) ;
#50802=B_SPLINE_CURVE_WITH_KNOTS ( 'NONE', 3,
 ( #8829, #15583, #22334, #36301, #69630, #63315, #1625, #41285, #20558, #48916 ),
 .UNSPECIFIED., .F., .F.,
 ( 4, 2, 2, 2, 4 ),
 ( 0.000000000000000000, 0.0001954311564186862510, 0.0003908623128373725020, 0.0005862934692560588072, 0.0007817246256747450040 ),
 .UNSPECIFIED. ) ;
#50804=B_SPLINE_CURVE_WITH_KNOTS ( 'NONE', 3,
 ( #38672, #52623, #67487, #4902, #80107, #33258, #18408, #11657, #39133, #66599 ),
 .UNSPECIFIED., .F., .F.,
 ( 4, 2, 2, 2, 4 ),
 ( 0.000000000000000000, 0.0001954339857564078267, 0.0003908679715128156535, 0.0005863019572692235344, 0.0007817359430256313069 ),
 .UNSPECIFIED. ) ;
#50807=ORIENTED_EDGE ( 'NONE', *, *, #60133, .F. ) ;
#50809=CYLINDRICAL_SURFACE ( 'NONE', #48715, 0.2499999999999973355 ) ;
#50810=EDGE_CURVE ( 'NONE', #29819, #61584, #58468, .T. ) ;
#50812=CARTESIAN_POINT ( 'NONE',  ( 9.692307692307572609, -12.46129190930018460, 30.37095296980731973 ) ) ;
#50814=EDGE_CURVE ( 'NONE', #45215, #6722, #71548, .T. ) ;
#50815=CARTESIAN_POINT ( 'NONE',  ( 7.623226887246997485, -11.98009711892699691, 32.48740034544075428 ) ) ;
#50816=CARTESIAN_POINT ( 'NONE',  ( -9.019230769230768274, -7.500000000000001776, 34.75000000000000000 ) ) ;
#50817=ORIENTED_EDGE ( 'NONE', *, *, #12454, .F. ) ;
#50819=CARTESIAN_POINT ( 'NONE',  ( -6.792285115252135519, -11.18335022499818621, 33.13157742990016885 ) ) ;
#50820=VERTEX_POINT ( 'NONE', #51249 ) ;
#50821=DIRECTION ( 'NONE',  ( -0.000000000000000000, -0.9848077530122085754, -0.1736481776669273613 ) ) ;
#50822=FACE_OUTER_BOUND ( 'NONE', #51286, .T. ) ;
#50823=EDGE_LOOP ( 'NONE', ( #59273, #9257, #69883, #48703 ) ) ;
#50824=CARTESIAN_POINT ( 'NONE',  ( 12.71159288145191368, -6.523592122091592671, 34.90882529074906415 ) ) ;
#50825=CARTESIAN_POINT ( 'NONE',  ( 15.29683758177166908, -8.973038597847271092, 34.52809138561121216 ) ) ;
#50826=CARTESIAN_POINT ( 'NONE',  ( 10.86533013373275836, -3.712312575010499494, 33.01462480002815170 ) ) ;
#50827=FACE_BOUND ( 'NONE', #48287, .T. ) ;
#50828=CARTESIAN_POINT ( 'NONE',  ( -9.442253272394237840, -4.074993327901527351, 33.72946981652012255 ) ) ;
#50829=CARTESIAN_POINT ( 'NONE',  ( 7.846153846153846700, -1.129524287112498415, 32.06866353760679544 ) ) ;
#50830=CARTESIAN_POINT ( 'NONE',  ( 13.38461538461526423, -12.70778746994576025, 30.41441678777401236 ) ) ;
#50831=CARTESIAN_POINT ( 'NONE',  ( 16.82689985270161870, -9.356822207818511927, 34.66110646841856635 ) ) ;
#50832=DIRECTION ( 'NONE',  ( -0.000000000000000000, -0.9848077530122086864, -0.1736481776669273613 ) ) ;
#50833=CARTESIAN_POINT ( 'NONE',  ( -11.40766973063675493, -3.062576670634119758, 32.05464942895959979 ) ) ;
#50835=ORIENTED_EDGE ( 'NONE', *, *, #16413, .T. ) ;
#50836=DIRECTION ( 'NONE',  ( 0.000000000000000000, 0.3420201433256641055, -0.9396926207859100932 ) ) ;
#50837=EDGE_LOOP ( 'NONE', ( #76789, #66001, #27430, #51006 ) ) ;
#50838=ORIENTED_EDGE ( 'NONE', *, *, #36863, .T. ) ;
#50839=CARTESIAN_POINT ( 'NONE',  ( 9.469441429244595199, -2.251424796025574881, 29.88072029997477230 ) ) ;
#50840=CARTESIAN_POINT ( 'NONE',  ( 1.134638653673032183, -10.66389620160130036, 33.62221079203477103 ) ) ;
#50841=CARTESIAN_POINT ( 'NONE',  ( -6.700297381808513641, -6.760870238392817200, 34.69528174975672385 ) ) ;
#50842=CARTESIAN_POINT ( 'NONE',  ( -14.30769230769242739, -2.892918686052166066, 31.69288490824153470 ) ) ;
#50843=CARTESIAN_POINT ( 'NONE',  ( 1.134638653673032405, -6.567427716900047230, 34.66269422305636283 ) ) ;
#50844=CARTESIAN_POINT ( 'NONE',  ( -2.307692307692428724, -11.67786785259630911, 32.92929555188603530 ) ) ;
#50845=ORIENTED_EDGE ( 'NONE', *, *, #67814, .F. ) ;
#50846=ADVANCED_FACE ( 'NONE', ( #64342 ), #9855, .F. ) ;
#50847=CARTESIAN_POINT ( 'NONE',  ( 18.13052543823364360, -2.647132371071621471, 31.75357179365173010 ) ) ;
#50849=CARTESIAN_POINT ( 'NONE',  ( 15.10062126103753322, -11.04286588640298561, 33.62463336215343901 ) ) ;
#50851=DIRECTION ( 'NONE',  ( -0.000000000000000000, 0.5000000000000011102, -0.8660254037844380415 ) ) ;
#50852=CARTESIAN_POINT ( 'NONE',  ( 15.23076923076923173, -2.708943851104267164, 35.45975837776705220 ) ) ;
#50853=ADVANCED_FACE ( 'NONE', ( #77868 ), #49950, .F. ) ;
#50856=ORIENTED_EDGE ( 'NONE', *, *, #36667, .T. ) ;
#50857=EDGE_CURVE ( 'NONE', #76807, #77663, #79360, .T. ) ;
#50858=AXIS2_PLACEMENT_3D ( 'NONE', #62335, #40757, #81301 ) ;
#50859=CARTESIAN_POINT ( 'NONE',  ( -7.846153846153967493, -11.67786785259630911, 32.92929555188603530 ) ) ;
#50860=EDGE_LOOP ( 'NONE', ( #37357, #11060, #56549, #47953 ) ) ;
#50861=CARTESIAN_POINT ( 'NONE',  ( 12.46153846153846168, -7.500000000000001776, 35.04278698407183867 ) ) ;
#50862=CARTESIAN_POINT ( 'NONE',  ( -12.21148414990014963, -9.943054286541403997, 34.11300777759954883 ) ) ;
#50863=CARTESIAN_POINT ( 'NONE',  ( -16.15384615384615330, -2.721908614388771852, 31.22303859784724978 ) ) ;
#50864=CARTESIAN_POINT ( 'NONE',  ( -1.384615384615383471, -6.435427911321262684, 35.78748833219616898 ) ) ;
#50866=EDGE_CURVE ( 'NONE', #19392, #52736, #56713, .T. ) ;
#50867=CYLINDRICAL_SURFACE ( 'NONE', #16, 0.2499999999999995559 ) ;
#50868=EDGE_LOOP ( 'NONE', ( #10266, #79262 ) ) ;
#50869=LINE ( 'NONE', #57649, #37197 ) ;
#50870=CARTESIAN_POINT ( 'NONE',  ( -1.254089682851819987, -9.417988943895561960, 34.36773134775778260 ) ) ;
#50871=VERTEX_POINT ( 'NONE', #10304 ) ;
#50872=CARTESIAN_POINT ( 'NONE',  ( 3.007842271862382066, -12.38737895849757820, 31.66785238281580206 ) ) ;
#50873=CARTESIAN_POINT ( 'NONE',  ( 6.923076923076924238, -13.20930481340135110, 34.54067556320372745 ) ) ;
#50874=CARTESIAN_POINT ( 'NONE',  ( -3.480792468062195333, -5.056417327199099532, 34.11270091957320716 ) ) ;
#50876=DIRECTION ( 'NONE',  ( -0.000000000000000000, -0.5000000000000009992, -0.8660254037844380415 ) ) ;
#50877=CARTESIAN_POINT ( 'NONE',  ( 7.596177102105254875, -3.436278759898155677, 33.07459398097509506 ) ) ;
#50878=CYLINDRICAL_SURFACE ( 'NONE', #57110, 0.2499999999999995559 ) ;
#50880=ORIENTED_EDGE ( 'NONE', *, *, #45579, .F. ) ;
#50881=CARTESIAN_POINT ( 'NONE',  ( -17.07692307692307665, -9.780366693483667717, 34.19971097300155094 ) ) ;
#50882=DIRECTION ( 'NONE',  ( -0.000000000000000000, 1.000000000000000000, -0.000000000000000000 ) ) ;
#50883=CARTESIAN_POINT ( 'NONE',  ( -1.253824943648432555, -3.338503747796865984, 32.95102852606552801 ) ) ;
#50885=LINE ( 'NONE', #78373, #87873 ) ;
#50886=CARTESIAN_POINT ( 'NONE',  ( 14.08476534878545827, -4.762599654559228846, 34.23009711892697737 ) ) ;
#50887=EDGE_LOOP ( 'NONE', ( #60537, #8663, #59753, #81663 ) ) ;
#50889=CARTESIAN_POINT ( 'NONE',  ( -1.254089946381742759, -12.50538340440932394, 31.33453814440721885 ) ) ;
#50890=EDGE_CURVE ( 'NONE', #87401, #63245, #18110, .T. ) ;
#50891=ORIENTED_EDGE ( 'NONE', *, *, #73596, .F. ) ;
#50892=CARTESIAN_POINT ( 'NONE',  ( 6.856994543716787405, -6.343179335718451384, 34.87096338111212646 ) ) ;
#50893=ORIENTED_EDGE ( 'NONE', *, *, #82548, .F. ) ;
#50894=CARTESIAN_POINT ( 'NONE',  ( 14.55763782604044998, -12.22109172314383052, 31.39792113162168263 ) ) ;
#50895=CARTESIAN_POINT ( 'NONE',  ( 3.007284306204900837, -4.225889041578354544, 33.85425143139329407 ) ) ;
#50896=CARTESIAN_POINT ( 'NONE',  ( -8.519285359852727169, -5.766571408460171355, 34.70601412856602508 ) ) ;
#50897=CARTESIAN_POINT ( 'NONE',  ( -12.33101302330481808, -11.04252011169590020, 33.62494198852677130 ) ) ;
#50898=ORIENTED_EDGE ( 'NONE', *, *, #84404, .T. ) ;
#50899=CARTESIAN_POINT ( 'NONE',  ( -13.13456096470193302, -2.920487667080175598, 32.31805714834170828 ) ) ;
#50900=ORIENTED_EDGE ( 'NONE', *, *, #24997, .T. ) ;
#50901=DIRECTION ( 'NONE',  ( 1.000000000000000000, 0.000000000000000000, 0.000000000000000000 ) ) ;
#50902=LINE ( 'NONE', #57686, #87259 ) ;
#50903=VERTEX_POINT ( 'NONE', #43204 ) ;
#50904=CARTESIAN_POINT ( 'NONE',  ( 8.703960768674447124, -5.094484230520674117, 34.41647553114621161 ) ) ;
#50905=CARTESIAN_POINT ( 'NONE',  ( -14.30769230769230660, -10.51840700105979565, 33.73612834413961536 ) ) ;
#50906=CARTESIAN_POINT ( 'NONE',  ( -11.60454391782167427, -2.833524468853757305, 32.15551576947924417 ) ) ;
#50907=CARTESIAN_POINT ( 'NONE',  ( 8.769230769230768274, -13.87047571288749737, 32.06866353760679544 ) ) ;
#50908=CARTESIAN_POINT ( 'NONE',  ( -18.22348494372394967, -4.386631170607604879, 33.66268669641500111 ) ) ;
#50909=B_SPLINE_CURVE_WITH_KNOTS ( 'NONE', 3,
 ( #82884, #34690, #35126, #42344, #41896, #41445, #56284, #83773, #68910, #15751 ),
 .UNSPECIFIED., .F., .F.,
 ( 4, 2, 2, 2, 4 ),
 ( 0.0007817359430256326080, 0.0009771253907250047801, 0.001172514838424369796, 0.001367904286123735030, 0.001563293733823100046 ),
 .UNSPECIFIED. ) ;
#50910=AXIS2_PLACEMENT_3D ( 'NONE', #4319, #31802, #5210 ) ;
#50911=EDGE_CURVE ( 'NONE', #44484, #78555, #70752, .T. ) ;
#50912=EDGE_CURVE ( 'NONE', #24183, #73834, #40603, .T. ) ;
#50914=ORIENTED_EDGE ( 'NONE', *, *, #78938, .T. ) ;
#50915=FACE_BOUND ( 'NONE', #32599, .T. ) ;
#50916=ORIENTED_EDGE ( 'NONE', *, *, #14671, .T. ) ;
#50918=VECTOR ( 'NONE', #54481, 1000.000000000000227 ) ;
#50919=ADVANCED_FACE ( 'NONE', ( #32355 ), #18397, .F. ) ;
#50920=AXIS2_PLACEMENT_3D ( 'NONE', #49856, #9760, #35917 ) ;
#50922=CARTESIAN_POINT ( 'NONE',  ( 17.75002325595141173, -5.643011162660950042, 34.66104346484419096 ) ) ;
#50923=CYLINDRICAL_SURFACE ( 'NONE', #55384, 0.2499999999999994726 ) ;
#50924=ORIENTED_EDGE ( 'NONE', *, *, #45271, .T. ) ;
#50925=EDGE_LOOP ( 'NONE', ( #49602, #5027 ) ) ;
#50926=EDGE_LOOP ( 'NONE', ( #27040, #5009, #76541, #8301 ) ) ;
#50927=CARTESIAN_POINT ( 'NONE',  ( 3.296024802045255164, -5.219633306516380244, 34.19971097300157936 ) ) ;
#50928=ORIENTED_EDGE ( 'NONE', *, *, #18080, .F. ) ;
#50929=CARTESIAN_POINT ( 'NONE',  ( 16.02369894440793630, -10.19110544564092002, 33.96427741523702792 ) ) ;
#50930=CARTESIAN_POINT ( 'NONE',  ( -4.826868765284761942, -4.943051570960391494, 34.04725096376909477 ) ) ;
#50931=EDGE_CURVE ( 'NONE', #6445, #12293, #24703, .T. ) ;
#50932=CARTESIAN_POINT ( 'NONE',  ( -12.33149340561869067, -2.254550872974305342, 29.97347326024527092 ) ) ;
#50933=FACE_BOUND ( 'NONE', #64319, .T. ) ;
#50935=CARTESIAN_POINT ( 'NONE',  ( 13.13459216039392707, -10.92453946501458795, 33.72985991061850086 ) ) ;
#50936=CARTESIAN_POINT ( 'NONE',  ( 4.946775107191381693, -3.625366637846544560, 33.29286588640298561 ) ) ;
#50937=EDGE_CURVE ( 'NONE', #53938, #87198, #81442, .T. ) ;
#50938=CARTESIAN_POINT ( 'NONE',  ( 8.900022577055551665, -3.062576670634119758, 32.05464942895959979 ) ) ;
#50939=CARTESIAN_POINT ( 'NONE',  ( 11.53846153846153832, -8.120952969808772792, 34.71129190930000163 ) ) ;
#50940=VERTEX_POINT ( 'NONE', #12097 ) ;
#50942=CARTESIAN_POINT ( 'NONE',  ( 9.442330961365341224, -2.564618984488975517, 30.55390908950641915 ) ) ;
#50944=ORIENTED_EDGE ( 'NONE', *, *, #82677, .T. ) ;
#50945=LINE ( 'NONE', #9113, #28854 ) ;
#50946=CARTESIAN_POINT ( 'NONE',  ( 5.869308533332441513, -3.062553014421049546, 32.05460306192773601 ) ) ;
#50949=CARTESIAN_POINT ( 'NONE',  ( 17.32692307692314415, -7.434744429011175271, 34.75000000000000711 ) ) ;
#50950=CARTESIAN_POINT ( 'NONE',  ( -11.53846153846153655, -2.292212530054420494, 30.41441678777542634 ) ) ;
#50951=VERTEX_POINT ( 'NONE', #44960 ) ;
#50952=EDGE_CURVE ( 'NONE', #31437, #6751, #33098, .T. ) ;
#50954=CARTESIAN_POINT ( 'NONE',  ( 17.93472999944368240, -3.643525952247789856, 33.31231777344662959 ) ) ;
#50955=CARTESIAN_POINT ( 'NONE',  ( 4.284637961670941131, -8.999086150933472084, 34.52020707165672064 ) ) ;
#50956=CARTESIAN_POINT ( 'NONE',  ( 5.300350038784647388, -7.630147231320743018, 34.74852402298682819 ) ) ;
#50958=EDGE_CURVE ( 'NONE', #57723, #75758, #872, .T. ) ;
#50959=ORIENTED_EDGE ( 'NONE', *, *, #24027, .T. ) ;
#50960=FACE_BOUND ( 'NONE', #15422, .T. ) ;
#50961=CARTESIAN_POINT ( 'NONE',  ( 7.846153846153725020, -2.892918686052165622, 31.69288490824153470 ) ) ;
#50962=CARTESIAN_POINT ( 'NONE',  ( -3.007757879156381264, -8.239487800360276282, 34.69522927552633718 ) ) ;
#50963=ORIENTED_EDGE ( 'NONE', *, *, #74087, .T. ) ;
#50964=LINE ( 'NONE', #78454, #3546 ) ;
#50965=LINE ( 'NONE', #9559, #84568 ) ;
#50966=CARTESIAN_POINT ( 'NONE',  ( 15.90382291655318880, -8.432397168068783699, 34.66272746175022945 ) ) ;
#50967=CARTESIAN_POINT ( 'NONE',  ( 4.153846153846154188, -5.471508081941601098, 34.59228464037088457 ) ) ;
#50968=EDGE_LOOP ( 'NONE', ( #26821, #64052 ) ) ;
#50969=EDGE_CURVE ( 'NONE', #32456, #85159, #28799, .T. ) ;
#50970=CYLINDRICAL_SURFACE ( 'NONE', #8575, 0.2499999999999973355 ) ;
#50971=ORIENTED_EDGE ( 'NONE', *, *, #3824, .T. ) ;
#50972=LINE ( 'NONE', #22636, #49624 ) ;
#50973=ORIENTED_EDGE ( 'NONE', *, *, #46928, .T. ) ;
#50974=CARTESIAN_POINT ( 'NONE',  ( 11.60452988946397923, -6.386643153685127139, 34.62446782046654192 ) ) ;
#50975=CARTESIAN_POINT ( 'NONE',  ( 15.16468581981334651, -2.721908614388770964, 31.22303859784723912 ) ) ;
#50976=DIRECTION ( 'NONE',  ( 0.000000000000000000, 1.000000000000000000, 0.000000000000000000 ) ) ;
#50977=CYLINDRICAL_SURFACE ( 'NONE', #86983, 0.2499999999999998890 ) ;
#50978=DIRECTION ( 'NONE',  ( -0.000000000000000000, 1.000000000000000000, 3.491481338843133355E-15 ) ) ;
#50979=AXIS2_PLACEMENT_3D ( 'NONE', #12110, #33701, #61157 ) ;
#50980=EDGE_CURVE ( 'NONE', #42554, #17692, #41713, .T. ) ;
#50981=DIRECTION ( 'NONE',  ( -0.000000000000000000, 0.6427876096865404731, -0.7660444431189771253 ) ) ;
#50983=EDGE_LOOP ( 'NONE', ( #36679, #86017 ) ) ;
#50985=DIRECTION ( 'NONE',  ( -0.000000000000000000, -0.8660254037844399289, -0.4999999999999980016 ) ) ;
#50986=CARTESIAN_POINT ( 'NONE',  ( 6.000000000000001776, -8.164416787775445883, 34.95778746994557906 ) ) ;
#50987=VECTOR ( 'NONE', #13240, 1000.000000000000227 ) ;
#50988=VERTEX_POINT ( 'NONE', #61589 ) ;
#50989=ORIENTED_EDGE ( 'NONE', *, *, #43948, .T. ) ;
#50990=CARTESIAN_POINT ( 'NONE',  ( 16.85399685940693004, -4.887634598454295265, 34.01352882383564946 ) ) ;
#50992=ADVANCED_FACE ( 'NONE', ( #47188 ), #74681, .F. ) ;
#50993=CARTESIAN_POINT ( 'NONE',  ( -17.29984929443921970, -9.086856451489516928, 34.49173150075333183 ) ) ;
#50994=CARTESIAN_POINT ( 'NONE',  ( 5.076923076923075762, -2.249999999999998668, 29.50000000000001421 ) ) ;
#50995=CARTESIAN_POINT ( 'NONE',  ( 8.769230769230768274, -11.35647404775217417, 33.31231777344666511 ) ) ;
#50996=EDGE_CURVE ( 'NONE', #45323, #14249, #27374, .T. ) ;
#50997=CARTESIAN_POINT ( 'NONE',  ( 16.21991348719623360, -3.322132147404559532, 32.92929555188717927 ) ) ;
#50998=DIRECTION ( 'NONE',  ( 0.000000000000000000, 0.8660254037844377084, -0.5000000000000015543 ) ) ;
#50999=EDGE_LOOP ( 'NONE', ( #59096, #74908, #65955, #76157 ) ) ;
#51000=CARTESIAN_POINT ( 'NONE',  ( -11.53846153846153655, -2.708943851104267164, 35.45975837776705220 ) ) ;
#51002=CARTESIAN_POINT ( 'NONE',  ( -9.019253993452229778, -11.56360843649121684, 33.07473185843129926 ) ) ;
#51004=EDGE_LOOP ( 'NONE', ( #51093, #72307 ) ) ;
#51005=CARTESIAN_POINT ( 'NONE',  ( -17.07692307692276046, -2.255955759149395501, 30.00000000000324363 ) ) ;
#51006=ORIENTED_EDGE ( 'NONE', *, *, #60998, .F. ) ;
#51007=CARTESIAN_POINT ( 'NONE',  ( 0.4615384615384611200, -8.973038597847269315, 34.52809138561121927 ) ) ;
#51008=DIRECTION ( 'NONE',  ( 0.000000000000000000, 0.000000000000000000, 1.000000000000000000 ) ) ;
#51009=CARTESIAN_POINT ( 'NONE',  ( -15.23076923076922995, -1.509761064869970415, 31.06009739812519044 ) ) ;
#51010=CYLINDRICAL_SURFACE ( 'NONE', #32647, 0.2499999999999994726 ) ;
#51012=DIRECTION ( 'NONE',  ( -0.000000000000000000, 0.8660254037844399289, -0.4999999999999980016 ) ) ;
#51013=CARTESIAN_POINT ( 'NONE',  ( -10.48459280755982981, -10.54018710029568595, 33.71981072465678864 ) ) ;
#51014=CARTESIAN_POINT ( 'NONE',  ( -10.83886953994894853, -12.69144148231606017, 30.53333754910549303 ) ) ;
#51016=CARTESIAN_POINT ( 'NONE',  ( -9.469528023329624844, -3.563462043263030399, 33.22394488606062879 ) ) ;
#51017=ORIENTED_EDGE ( 'NONE', *, *, #17283, .F. ) ;
#51018=CARTESIAN_POINT ( 'NONE',  ( 12.46153846153833911, -10.90142922262034020, 33.41473453929536674 ) ) ;
#51019=ORIENTED_EDGE ( 'NONE', *, *, #80713, .F. ) ;
#51020=DIRECTION ( 'NONE',  ( 0.000000000000000000, 0.000000000000000000, 1.000000000000000000 ) ) ;
#51022=LINE ( 'NONE', #16379, #36976 ) ;
#51023=CARTESIAN_POINT ( 'NONE',  ( -6.222926217516146608, -2.554751324335733820, 30.48935550225260727 ) ) ;
#51024=EDGE_CURVE ( 'NONE', #39385, #3, #58919, .T. ) ;
#51025=CARTESIAN_POINT ( 'NONE',  ( -14.17716660592874689, -10.19071101563364756, 33.96452234770658407 ) ) ;
#51026=CYLINDRICAL_SURFACE ( 'NONE', #50792, 0.2500000000000004996 ) ;
#51027=ORIENTED_EDGE ( 'NONE', *, *, #58070, .F. ) ;
#51028=ORIENTED_EDGE ( 'NONE', *, *, #16955, .T. ) ;
#51029=EDGE_CURVE ( 'NONE', #49865, #20268, #57809, .T. ) ;
#51030=B_SPLINE_CURVE_WITH_KNOTS ( 'NONE', 3,
 ( #3475, #10691, #50327, #2152, #57536, #38157, #65615, #71489, #57980, #16999 ),
 .UNSPECIFIED., .F., .F.,
 ( 4, 2, 2, 2, 4 ),
 ( 0.0007817246336856293861, 0.0009771112958940105907, 0.001172497958102391904, 0.001367884620310773217, 0.001563271282519154530 ),
 .UNSPECIFIED. ) ;
#51032=ORIENTED_EDGE ( 'NONE', *, *, #59573, .F. ) ;
#51036=EDGE_CURVE ( 'NONE', #27164, #7165, #14296, .T. ) ;
#51037=CARTESIAN_POINT ( 'NONE',  ( 14.43853063817906524, -7.277220318596961057, 34.99547417642776992 ) ) ;
#51038=CARTESIAN_POINT ( 'NONE',  ( -4.284536756956459413, -12.35290016733513951, 31.75349464988449455 ) ) ;
#51039=CARTESIAN_POINT ( 'NONE',  ( 17.99999999999987566, -9.442884908241554243, 34.35708131394783038 ) ) ;
#51041=CARTESIAN_POINT ( 'NONE',  ( -17.86947429823644029, -10.19071101563364579, 33.96452234770658407 ) ) ;
#51044=ORIENTED_EDGE ( 'NONE', *, *, #9067, .F. ) ;
#51045=EDGE_LOOP ( 'NONE', ( #59815, #929 ) ) ;
#51046=EDGE_CURVE ( 'NONE', #2381, #84018, #78223, .T. ) ;
#51047=CARTESIAN_POINT ( 'NONE',  ( 0.2115152373170022249, -12.07920672191015221, 32.31858351112116168 ) ) ;
#51048=ORIENTED_EDGE ( 'NONE', *, *, #75012, .F. ) ;
#51049=DIRECTION ( 'NONE',  ( -0.000000000000000000, -0.6427876096865404731, -0.7660444431189771253 ) ) ;
#51050=CARTESIAN_POINT ( 'NONE',  ( -16.15384615384627409, -10.21337939537710326, 33.94971097300076224 ) ) ;
#51051=CARTESIAN_POINT ( 'NONE',  ( -1.384615384615069056, -2.255955759149395501, 30.00000000000324363 ) ) ;
#51052=DIRECTION ( 'NONE',  ( 0.000000000000000000, 0.6427876096865368094, 0.7660444431189802339 ) ) ;
#51053=ORIENTED_EDGE ( 'NONE', *, *, #42763, .F. ) ;
#51055=CARTESIAN_POINT ( 'NONE',  ( -17.07692307692307665, -11.35647404775217417, 33.31231777344666511 ) ) ;
#51056=EDGE_CURVE ( 'NONE', #28593, #49579, #12680, .T. ) ;
#51057=VERTEX_POINT ( 'NONE', #40893 ) ;
#51058=FACE_BOUND ( 'NONE', #87091, .T. ) ;
#51060=CARTESIAN_POINT ( 'NONE',  ( 16.02315468717859659, -6.413092428213692742, 34.63065189839063152 ) ) ;
#51061=ORIENTED_EDGE ( 'NONE', *, *, #48568, .F. ) ;
#51063=EDGE_CURVE ( 'NONE', #84960, #25936, #21273, .T. ) ;
#51064=CARTESIAN_POINT ( 'NONE',  ( 5.011653076366756387, -8.656820664281497102, 34.87096338111211935 ) ) ;
#51065=FACE_OUTER_BOUND ( 'NONE', #20047, .T. ) ;
#51066=ORIENTED_EDGE ( 'NONE', *, *, #19049, .F. ) ;
#51067=CYLINDRICAL_SURFACE ( 'NONE', #50029, 0.2500000000000008882 ) ;
#51068=CARTESIAN_POINT ( 'NONE',  ( 4.219101725122177626, -3.300289026998475705, 32.46337939537591666 ) ) ;
#51070=B_SPLINE_CURVE_WITH_KNOTS ( 'NONE', 3,
 ( #55454, #40187, #82939, #46485, #60436, #87953, #26212, #60880, #29764, #2707 ),
 .UNSPECIFIED., .F., .F.,
 ( 4, 2, 2, 2, 4 ),
 ( 0.0007817246256747446788, 0.0009771112852218874663, 0.001172497944769030362, 0.001367884604316173258, 0.001563271263863315937 ),
 .UNSPECIFIED. ) ;
#51071=B_SPLINE_CURVE_WITH_KNOTS ( 'NONE', 3,
 ( #47401, #82096, #81212, #20825, #20389, #48291, #40669, #61800, #47851, #33894 ),
 .UNSPECIFIED., .F., .F.,
 ( 4, 2, 2, 2, 4 ),
 ( 0.000000000000000000, 0.0001954311564186867660, 0.0003908623128373735320, 0.0005862934692560603251, 0.0007817246256747470640 ),
 .UNSPECIFIED. ) ;
#51072=VECTOR ( 'NONE', #14455, 1000.000000000000114 ) ;
#51076=CARTESIAN_POINT ( 'NONE',  ( -7.846153846153967493, -12.16647553114689728, 32.15551576947799362 ) ) ;
#51077=DIRECTION ( 'NONE',  ( 0.000000000000000000, 8.673617379884033500E-16, -1.000000000000000000 ) ) ;
#51078=CARTESIAN_POINT ( 'NONE',  ( -8.769230769230768274, -8.973038597847269315, 34.52809138561121927 ) ) ;
#51079=CARTESIAN_POINT ( 'NONE',  ( 9.627037691751372250, -12.51329471203370325, 31.30864560766548976 ) ) ;
#51080=CARTESIAN_POINT ( 'NONE',  ( 7.912221179503922563, -2.833524468853757750, 32.15551576947925838 ) ) ;
#51081=CARTESIAN_POINT ( 'NONE',  ( 4.853438133199127869, -12.44517049084099725, 30.48991314939691932 ) ) ;
#51082=CARTESIAN_POINT ( 'NONE',  ( 1.384615384615386802, -8.318370150425687726, 35.83090037661290239 ) ) ;
#51083=ADVANCED_FACE ( 'NONE', ( #29156 ), #44403, .F. ) ;
#51084=CARTESIAN_POINT ( 'NONE',  ( 8.519230769230770051, -2.499999999999999556, 29.81609845454691765 ) ) ;
#51085=CARTESIAN_POINT ( 'NONE',  ( 12.33092880633437716, -7.722926974430166069, 34.99546784045485737 ) ) ;
#51086=CARTESIAN_POINT ( 'NONE',  ( -8.704037780936115354, -2.255955759149235629, 29.99999999999988987 ) ) ;
#51087=CARTESIAN_POINT ( 'NONE',  ( -2.530619266599154038, -5.582147617184174848, 34.63737895849758530 ) ) ;
#51091=ORIENTED_EDGE ( 'NONE', *, *, #10622, .T. ) ;
#51093=ORIENTED_EDGE ( 'NONE', *, *, #48198, .T. ) ;
#51094=CARTESIAN_POINT ( 'NONE',  ( 17.74997676270703550, -12.22074536777955345, 31.39888409691088356 ) ) ;
#51095=EDGE_LOOP ( 'NONE', ( #21648, #52698, #30675, #42803 ) ) ;
#51096=CARTESIAN_POINT ( 'NONE',  ( 5.869309396889695662, -10.70098750199973203, 33.91152734681376302 ) ) ;
#51098=DIRECTION ( 'NONE',  ( -0.000000000000000000, -0.9848077530122086864, -0.1736481776669273613 ) ) ;
#51099=EDGE_CURVE ( 'NONE', #82533, #10196, #30463, .T. ) ;
#51100=CARTESIAN_POINT ( 'NONE',  ( -5.076923076923197442, -2.892918686052165622, 31.69288490824153470 ) ) ;
#51102=CARTESIAN_POINT ( 'NONE',  ( -14.53117723225664015, -10.97335522853832579, 33.68706563782419749 ) ) ;
#51103=CARTESIAN_POINT ( 'NONE',  ( -17.74999999976641973, -2.249999999999989786, 29.74999979494859303 ) ) ;
#51104=CARTESIAN_POINT ( 'NONE',  ( -11.53846153846153655, -9.819645486525091727, 36.12317359536749706 ) ) ;
#51105=DIRECTION ( 'NONE',  ( -1.000000000000000000, 0.000000000000000000, 0.000000000000000000 ) ) ;
#51108=EDGE_CURVE ( 'NONE', #87066, #33781, #65310, .T. ) ;
#51110=LINE ( 'NONE', #24099, #10365 ) ;
#51112=CARTESIAN_POINT ( 'NONE',  ( 16.15384615384615330, -11.11383981884818262, 36.00935417666054406 ) ) ;
#51115=ORIENTED_EDGE ( 'NONE', *, *, #56336, .F. ) ;
#51117=CARTESIAN_POINT ( 'NONE',  ( -11.53846153846165912, -8.613356846316285953, 34.62446782046622218 ) ) ;
#51118=CARTESIAN_POINT ( 'NONE',  ( -3.230769230769229949, -13.53365097954675988, 30.81389545987213552 ) ) ;
#51119=CARTESIAN_POINT ( 'NONE',  ( 18.00000000000000000, -10.51840700105979565, 33.73612834413961536 ) ) ;
#51121=CARTESIAN_POINT ( 'NONE',  ( 4.023155550735844521, -3.338472653186242756, 32.95098750199972670 ) ) ;
#51122=CARTESIAN_POINT ( 'NONE',  ( 2.084766090176160436, -12.15238873228292071, 31.58232369045353849 ) ) ;
#51123=EDGE_LOOP ( 'NONE', ( #49718, #63470, #67633, #43782 ) ) ;
#51124=CARTESIAN_POINT ( 'NONE',  ( -14.30769230769230660, -1.242168528481310874, 33.36296068462461051 ) ) ;
#51125=ORIENTED_EDGE ( 'NONE', *, *, #87665, .F. ) ;
#51126=VERTEX_POINT ( 'NONE', #15191 ) ;
#51127=LINE ( 'NONE', #79527, #50739 ) ;
#51128=CARTESIAN_POINT ( 'NONE',  ( 5.142991427925514891, -11.69971097300155272, 32.46337939537588113 ) ) ;
#51129=VECTOR ( 'NONE', #10468, 999.9999999999998863 ) ;
#51130=DIRECTION ( 'NONE',  ( 0.000000000000000000, 0.6427876096865368094, 0.7660444431189802339 ) ) ;
#51131=CARTESIAN_POINT ( 'NONE',  ( -13.25382357679059453, -8.999086150933475636, 34.52020707165672775 ) ) ;
#51132=CARTESIAN_POINT ( 'NONE',  ( 10.83839745947800992, -10.01129605718032600, 34.36064277460058491 ) ) ;
#51135=CARTESIAN_POINT ( 'NONE',  ( -6.857008572074484221, -5.557115091759786019, 34.35708131394839882 ) ) ;
#51136=VERTEX_POINT ( 'NONE', #8431 ) ;
#51137=VERTEX_POINT ( 'NONE', #50721 ) ;
#51138=CARTESIAN_POINT ( 'NONE',  ( -3.931066484868086963, -12.11081565061823717, 32.26097654155341843 ) ) ;
#51139=CYLINDRICAL_SURFACE ( 'NONE', #21505, 0.2499999999999994726 ) ;
#51141=LINE ( 'NONE', #48622, #38469 ) ;
#51142=CARTESIAN_POINT ( 'NONE',  ( -11.60454391782167249, -8.164416787775445883, 34.95778746994557906 ) ) ;
#51143=CARTESIAN_POINT ( 'NONE',  ( 17.77707378248385339, -8.239355502252617924, 34.69524867566427417 ) ) ;
#51144=EDGE_LOOP ( 'NONE', ( #80292, #41837 ) ) ;
#51145=ORIENTED_EDGE ( 'NONE', *, *, #34535, .T. ) ;
#51148=ADVANCED_FACE ( 'NONE', ( #35905 ), #63805, .F. ) ;
#51149=CARTESIAN_POINT ( 'NONE',  ( -12.59222992820602194, -11.18331474514187995, 33.13161551792790505 ) ) ;
#51151=CARTESIAN_POINT ( 'NONE',  ( -7.053768389744481837, -12.38065189839062263, 30.83690757178629482 ) ) ;
#51152=CARTESIAN_POINT ( 'NONE',  ( 6.066068351002440906, -12.37446782046654192, 30.86335684631486842 ) ) ;
#51153=AXIS2_PLACEMENT_3D ( 'NONE', #17669, #37477, #3691 ) ;
#51154=DIRECTION ( 'NONE',  ( -0.000000000000000000, -0.1736481776669307198, -0.9848077530122080203 ) ) ;
#51155=ORIENTED_EDGE ( 'NONE', *, *, #2408, .T. ) ;
#51156=CARTESIAN_POINT ( 'NONE',  ( 10.61538461538461675, -2.292212530054420494, 30.41441678777542634 ) ) ;
#51157=VERTEX_POINT ( 'NONE', #57490 ) ;
#51158=CARTESIAN_POINT ( 'NONE',  ( -8.899921372341079717, -4.684245665217972032, 34.18127051446801090 ) ) ;
#51159=CYLINDRICAL_SURFACE ( 'NONE', #48615, 0.2499999999999986955 ) ;
#51160=FACE_OUTER_BOUND ( 'NONE', #3654, .T. ) ;
#51161=CARTESIAN_POINT ( 'NONE',  ( 1.384615384615386802, -2.486705287966279876, 31.30864560766543647 ) ) ;
#51162=CARTESIAN_POINT ( 'NONE',  ( -10.83831157429146330, -5.582147617184174848, 34.63737895849758530 ) ) ;
#51164=CARTESIAN_POINT ( 'NONE',  ( -0.2385256174450664512, -12.64618726649961289, 30.78989965857442712 ) ) ;
#51165=ORIENTED_EDGE ( 'NONE', *, *, #3219, .T. ) ;
#51167=DIRECTION ( 'NONE',  ( 0.000000000000000000, 0.9848077530122072432, -0.1736481776669354937 ) ) ;
#51168=AXIS2_PLACEMENT_3D ( 'NONE', #26238, #40209, #33876 ) ;
#51169=CARTESIAN_POINT ( 'NONE',  ( -6.250023224221458840, -11.56360843649121861, 33.07473185843129926 ) ) ;
#51171=CARTESIAN_POINT ( 'NONE',  ( 7.173131234715239835, -2.779044189368096163, 31.39831045268886456 ) ) ;
#51172=CARTESIAN_POINT ( 'NONE',  ( 15.48071474911737333, -4.336752205174649433, 33.62275283266504289 ) ) ;
#51173=CARTESIAN_POINT ( 'NONE',  ( -15.93106661257773560, -10.81320215134717166, 33.49497208177562868 ) ) ;
#51174=CARTESIAN_POINT ( 'NONE',  ( -7.715628407920204879, -11.04252011169590020, 33.62494198852677130 ) ) ;
#51175=CARTESIAN_POINT ( 'NONE',  ( 8.096099255531889582, -6.653508905675592722, 34.93172785388651391 ) ) ;
#51176=CARTESIAN_POINT ( 'NONE',  ( -17.07692307692307665, -13.75783147151868846, 33.36296068462461051 ) ) ;
#51177=FACE_BOUND ( 'NONE', #54066, .T. ) ;
#51178=CARTESIAN_POINT ( 'NONE',  ( 12.23805353697412990, -10.23692288466677880, 34.23039457007281072 ) ) ;
#51179=DIRECTION ( 'NONE',  ( 0.000000000000000000, 0.9848077530122072432, -0.1736481776669354937 ) ) ;
#51182=CARTESIAN_POINT ( 'NONE',  ( -11.28846153846160050, -7.565270445406050648, 34.75000000000000000 ) ) ;
#51183=FACE_OUTER_BOUND ( 'NONE', #20378, .T. ) ;
#51184=DIRECTION ( 'NONE',  ( -0.000000000000000000, 0.7660444431189791237, -0.6427876096865379196 ) ) ;
#51185=CARTESIAN_POINT ( 'NONE',  ( 8.992010310499177095, -10.81320215134717344, 33.49497208177562868 ) ) ;
#51187=EDGE_LOOP ( 'NONE', ( #62020, #11006, #51891, #136 ) ) ;
#51188=CARTESIAN_POINT ( 'NONE',  ( -4.377331097570100304, -11.89387501736622710, 32.13663884655806413 ) ) ;
#51189=CARTESIAN_POINT ( 'NONE',  ( -14.53061852520844965, -6.503392248772476236, 34.64988816332204635 ) ) ;
#51190=FACE_OUTER_BOUND ( 'NONE', #32382, .T. ) ;
#51191=CARTESIAN_POINT ( 'NONE',  ( -10.86540783960607293, -11.56360843649121684, 33.07473185843129926 ) ) ;
#51192=DIRECTION ( 'NONE',  ( 0.000000000000000000, 0.000000000000000000, 1.000000000000000000 ) ) ;
#51193=CARTESIAN_POINT ( 'NONE',  ( -4.153846153846152411, -1.367168528481310208, 33.57946703557072254 ) ) ;
#51195=CARTESIAN_POINT ( 'NONE',  ( -2.531177232256636600, -3.562934362175799841, 33.22335522853832401 ) ) ;
#51196=CARTESIAN_POINT ( 'NONE',  ( -14.53061926659915315, -11.43668979543635089, 33.22377378376089752 ) ) ;
#51197=DIRECTION ( 'NONE',  ( -0.000000000000000000, -0.9848077530122085754, -0.1736481776669273613 ) ) ;
#51199=CARTESIAN_POINT ( 'NONE',  ( 5.076923076923383071, -2.506253911140614576, 30.00000000000323297 ) ) ;
#51200=CARTESIAN_POINT ( 'NONE',  ( 12.39626846098214230, -12.70778746994557551, 30.41441678777548319 ) ) ;
#51201=EDGE_CURVE ( 'NONE', #17652, #5312, #9321, .T. ) ;
#51202=EDGE_CURVE ( 'NONE', #5871, #48512, #49196, .T. ) ;
#51206=CARTESIAN_POINT ( 'NONE',  ( -17.07692307692307665, -13.49023893513002648, 31.06009739812518688 ) ) ;
#51207=CARTESIAN_POINT ( 'NONE',  ( -1.634615384615383027, -2.249999999999998668, 29.75000000000000355 ) ) ;
#51209=CARTESIAN_POINT ( 'NONE',  ( -2.307692307692428724, -5.094484230521993062, 34.41647553114689373 ) ) ;
#51210=CARTESIAN_POINT ( 'NONE',  ( 13.38461538461538680, -6.189225973068211317, 35.74407628777942847 ) ) ;
#51211=ORIENTED_EDGE ( 'NONE', *, *, #64002, .F. ) ;
#51212=CARTESIAN_POINT ( 'NONE',  ( -16.15384615384627409, -4.320704448113951379, 33.92786785259630022 ) ) ;
#51213=CARTESIAN_POINT ( 'NONE',  ( 9.692307692307572609, -11.48612834414049644, 32.76840700105863391 ) ) ;
#51215=VERTEX_POINT ( 'NONE', #36779 ) ;
#51216=CARTESIAN_POINT ( 'NONE',  ( 6.923076923076924238, -3.050289026998446396, 32.03036669348365706 ) ) ;
#51217=LINE ( 'NONE', #78271, #25374 ) ;
#51218=CARTESIAN_POINT ( 'NONE',  ( -4.946397375159511611, -9.417988943895561960, 34.36773134775778260 ) ) ;
#51219=CARTESIAN_POINT ( 'NONE',  ( -14.30769230769242739, -11.48612834414049644, 32.76840700105863391 ) ) ;
#51220=ORIENTED_EDGE ( 'NONE', *, *, #21370, .T. ) ;
#51221=CARTESIAN_POINT ( 'NONE',  ( -11.76194648218548622, -4.386631170607604879, 33.66268669641500111 ) ) ;
#51222=CARTESIAN_POINT ( 'NONE',  ( -11.66902145207490094, -2.254533558242300284, 29.97296025877828285 ) ) ;
#51223=VECTOR ( 'NONE', #76603, 1000.000000000000000 ) ;
#51224=CARTESIAN_POINT ( 'NONE',  ( -1.134669866267241867, -5.852078868378310261, 34.47109172314383585 ) ) ;
#51225=ORIENTED_EDGE ( 'NONE', *, *, #28144, .F. ) ;
#51226=ORIENTED_EDGE ( 'NONE', *, *, #40652, .F. ) ;
#51227=ORIENTED_EDGE ( 'NONE', *, *, #24010, .F. ) ;
#51228=CYLINDRICAL_SURFACE ( 'NONE', #44287, 0.2500000000000004996 ) ;
#51229=CARTESIAN_POINT ( 'NONE',  ( 6.065255139512838234, -2.379036618887895305, 30.90682066428159303 ) ) ;
#51230=B_SPLINE_CURVE_WITH_KNOTS ( 'NONE', 3,
 ( #33926, #28062, #19091, #35716, #71246, #35258, #2782, #63166, #36594, #69930 ),
 .UNSPECIFIED., .F., .F.,
 ( 4, 2, 2, 2, 4 ),
 ( 0.000000000000000000, 0.0001954311564186865221, 0.0003908623128373730441, 0.0005862934692560595662, 0.0007817246256747460882 ),
 .UNSPECIFIED. ) ;
#51231=AXIS2_PLACEMENT_3D ( 'NONE', #53457, #11601, #80959 ) ;
#51232=CYLINDRICAL_SURFACE ( 'NONE', #17907, 0.2500000000000009437 ) ;
#51233=CARTESIAN_POINT ( 'NONE',  ( -10.36543909703647159, -3.202959910592335646, 32.30730279482227019 ) ) ;
#51234=ORIENTED_EDGE ( 'NONE', *, *, #13208, .T. ) ;
#51235=ORIENTED_EDGE ( 'NONE', *, *, #73696, .T. ) ;
#51236=CARTESIAN_POINT ( 'NONE',  ( 11.66898697669518192, -11.66157788607254098, 32.95092075102925833 ) ) ;
#51238=DIRECTION ( 'NONE',  ( -0.000000000000000000, 0.1736481776669307198, -0.9848077530122080203 ) ) ;
#51240=DIRECTION ( 'NONE',  ( -0.000000000000000000, 0.3420201433256694901, -0.9396926207859082059 ) ) ;
#51241=CARTESIAN_POINT ( 'NONE',  ( -4.153846153846152411, -10.89733346790207413, 36.13435417666054406 ) ) ;
#51243=ORIENTED_EDGE ( 'NONE', *, *, #6537, .T. ) ;
#51245=VERTEX_POINT ( 'NONE', #9750 ) ;
#51246=CARTESIAN_POINT ( 'NONE',  ( -16.15384615384627409, -2.657715359629662988, 31.77849191805970364 ) ) ;
#51247=ORIENTED_EDGE ( 'NONE', *, *, #11183, .F. ) ;
#51248=EDGE_CURVE ( 'NONE', #44876, #622, #37217, .T. ) ;
#51249=CARTESIAN_POINT ( 'NONE',  ( -7.846153846153965716, -2.892918686052166066, 31.69288490824153470 ) ) ;
#51250=CARTESIAN_POINT ( 'NONE',  ( -16.15384615384615330, -3.513871655860378418, 32.76840700105978499 ) ) ;
#51251=ORIENTED_EDGE ( 'NONE', *, *, #46165, .T. ) ;
#51252=VECTOR ( 'NONE', #71048, 1000.000000000000114 ) ;
#51253=CARTESIAN_POINT ( 'NONE',  ( 12.59232890250540926, -6.369690395747422684, 34.87708834333098196 ) ) ;
#51254=DIRECTION ( 'NONE',  ( 0.000000000000000000, 0.3420201433256641055, -0.9396926207859100932 ) ) ;
#51255=CARTESIAN_POINT ( 'NONE',  ( -2.241623956689868358, -11.16473453929635440, 33.15142922261926373 ) ) ;
#51256=FACE_BOUND ( 'NONE', #52140, .T. ) ;
#51258=CARTESIAN_POINT ( 'NONE',  ( 4.088576153289833925, -2.379036618887870436, 30.90682066428147934 ) ) ;
#51259=EDGE_CURVE ( 'NONE', #44052, #44046, #4046, .T. ) ;
#51260=CARTESIAN_POINT ( 'NONE',  ( -15.10024352900566846, -10.88167719472716399, 33.43325721877153711 ) ) ;
#51261=CARTESIAN_POINT ( 'NONE',  ( 9.692307692307695177, -12.62096338111211580, 30.90682066428153263 ) ) ;
#51262=CARTESIAN_POINT ( 'NONE',  ( 6.673100192134569397, -11.79746400365624659, 32.30657167506340954 ) ) ;
#51263=B_SPLINE_CURVE_WITH_KNOTS ( 'NONE', 3,
 ( #1129, #83564, #42567, #21402, #75458, #15094 ),
 .UNSPECIFIED., .F., .F.,
 ( 4, 2, 4 ),
 ( 0.0003909569690057822732, 0.0005862646681846077649, 0.0007815723673634333108 ),
 .UNSPECIFIED. ) ;
#51264=CARTESIAN_POINT ( 'NONE',  ( 8.639082799499075094, -9.504002272028875709, 34.60269587691767867 ) ) ;
#51265=CARTESIAN_POINT ( 'NONE',  ( 1.607395053593452028, -2.353885683473779356, 30.79025554430704759 ) ) ;
#51266=EDGE_LOOP ( 'NONE', ( #62943, #17332, #11442, #63693 ) ) ;
#51267=CARTESIAN_POINT ( 'NONE',  ( -16.02305571287920216, -3.338503747796866872, 32.95102852606552801 ) ) ;
#51268=EDGE_CURVE ( 'NONE', #33434, #82159, #56695, .T. ) ;
#51269=EDGE_LOOP ( 'NONE', ( #49862, #84644, #29584, #47829 ) ) ;
#51270=EDGE_LOOP ( 'NONE', ( #15777, #17084 ) ) ;
#51271=DIRECTION ( 'NONE',  ( -0.000000000000000000, 0.8660254037844397068, -0.4999999999999978906 ) ) ;
#51272=CARTESIAN_POINT ( 'NONE',  ( 10.68145194873469173, -12.62096338111211757, 30.90682066428152908 ) ) ;
#51273=CARTESIAN_POINT ( 'NONE',  ( 13.25446741488368829, -11.66186481527757302, 32.95055677023626117 ) ) ;
#51274=CARTESIAN_POINT ( 'NONE',  ( 2.557637717070352590, -2.341251567377310217, 30.72681386836322659 ) ) ;
#51275=CARTESIAN_POINT ( 'NONE',  ( -2.557669051740896649, -11.47974371597207899, 33.17467449705390692 ) ) ;
#51277=FACE_OUTER_BOUND ( 'NONE', #83100, .T. ) ;
#51278=CARTESIAN_POINT ( 'NONE',  ( 6.699591979352973681, -3.754499324213721234, 33.06261337010820256 ) ) ;
#51279=CARTESIAN_POINT ( 'NONE',  ( -1.384615384615506484, -10.33852847137269571, 34.16647553114546554 ) ) ;
#51281=CARTESIAN_POINT ( 'NONE',  ( 10.68064018666064285, -4.481592998940250538, 33.73612834413965089 ) ) ;
#51282=CARTESIAN_POINT ( 'NONE',  ( -15.00775638667583678, -10.77377354290276124, 33.85451476688484718 ) ) ;
#51283=AXIS2_PLACEMENT_3D ( 'NONE', #45835, #80977, #33221 ) ;
#51285=ORIENTED_EDGE ( 'NONE', *, *, #24713, .T. ) ;
#51286=EDGE_LOOP ( 'NONE', ( #7771, #71738, #69242, #39844 ) ) ;
#51287=CARTESIAN_POINT ( 'NONE',  ( -7.911423846710166075, -11.67786785259540849, 32.92929555188721480 ) ) ;
#51288=ORIENTED_EDGE ( 'NONE', *, *, #38218, .T. ) ;
#51289=CARTESIAN_POINT ( 'NONE',  ( 17.32686848630112308, -4.176053281294515251, 33.81426240980091791 ) ) ;
#51290=CARTESIAN_POINT ( 'NONE',  ( 9.823099500132483897, -9.804649428959608670, 34.18742332936588468 ) ) ;
#51291=CARTESIAN_POINT ( 'NONE',  ( -16.28399336328437386, -5.195881422630167279, 34.18770438780618548 ) ) ;
#51292=CARTESIAN_POINT ( 'NONE',  ( -15.10024352900566669, -2.882268652242222284, 31.66798894389554064 ) ) ;
#51294=FACE_OUTER_BOUND ( 'NONE', #33588, .T. ) ;
#51295=ORIENTED_EDGE ( 'NONE', *, *, #10809, .T. ) ;
#51297=CARTESIAN_POINT ( 'NONE',  ( 4.153846153846154188, -13.95598074871891292, 31.83374038241031911 ) ) ;
#51298=ORIENTED_EDGE ( 'NONE', *, *, #72083, .T. ) ;
#51299=CARTESIAN_POINT ( 'NONE',  ( -13.63463862190834952, -11.37209801155882971, 32.91403422569032955 ) ) ;
#51300=CARTESIAN_POINT ( 'NONE',  ( 3.296837581771669523, -2.721908614388771852, 31.22303859784725333 ) ) ;
#51301=CARTESIAN_POINT ( 'NONE',  ( -3.453595923248235167, -7.369208160676173236, 34.74850200257122879 ) ) ;
#51302=CARTESIAN_POINT ( 'NONE',  ( 0.5267940328144850026, -2.892918686051626498, 31.69288490824025928 ) ) ;
#51303=EDGE_CURVE ( 'NONE', #6050, #34465, #20170, .T. ) ;
#51304=DIRECTION ( 'NONE',  ( -0.000000000000000000, 0.1736481776669307198, -0.9848077530122080203 ) ) ;
#51305=DIRECTION ( 'NONE',  ( -0.000000000000000000, 0.1736481776669307198, -0.9848077530122080203 ) ) ;
#51306=CARTESIAN_POINT ( 'NONE',  ( -11.28851612908349722, -2.986452184633680229, 32.43230066228895225 ) ) ;
#51307=EDGE_CURVE ( 'NONE', #39142, #43722, #17067, .T. ) ;
#51311=CARTESIAN_POINT ( 'NONE',  ( -15.23076923076922995, -13.63283147151868846, 33.57946703557072254 ) ) ;
#51312=CARTESIAN_POINT ( 'NONE',  ( 4.219913487196229163, -10.67929555188718282, 33.92786785259544757 ) ) ;
#51314=EDGE_CURVE ( 'NONE', #74101, #40454, #33195, .T. ) ;
#51315=CARTESIAN_POINT ( 'NONE',  ( 0.3313912521002385092, -3.817052484675422797, 33.13202310037935661 ) ) ;
#51317=CARTESIAN_POINT ( 'NONE',  ( 14.30769230769231015, -4.661471528628507777, 34.16647553114623292 ) ) ;
#51319=VERTEX_POINT ( 'NONE', #18741 ) ;
#51321=CARTESIAN_POINT ( 'NONE',  ( 3.007843013253082898, -9.086856451489515152, 34.49173150075333183 ) ) ;
#51322=VERTEX_POINT ( 'NONE', #46207 ) ;
#51325=ORIENTED_EDGE ( 'NONE', *, *, #41655, .F. ) ;
#51326=CARTESIAN_POINT ( 'NONE',  ( 14.43848411551709532, -12.11778462344221019, 31.66786338562085135 ) ) ;
#51327=LINE ( 'NONE', #25228, #88324 ) ;
#51328=CIRCLE ( 'NONE', #71473, 0.2500000000000002220 ) ;
#51329=CARTESIAN_POINT ( 'NONE',  ( -1.514762594053604028, -4.460286881179644780, 33.72017969459903242 ) ) ;
#51330=ORIENTED_EDGE ( 'NONE', *, *, #32693, .T. ) ;
#51331=DIRECTION ( 'NONE',  ( -0.000000000000000000, -0.1736481776669307198, -0.9848077530122080203 ) ) ;
#51332=ORIENTED_EDGE ( 'NONE', *, *, #19585, .F. ) ;
#51333=DIRECTION ( 'NONE',  ( 0.000000000000000000, 0.6427876096865368094, 0.7660444431189802339 ) ) ;
#51334=ORIENTED_EDGE ( 'NONE', *, *, #28878, .T. ) ;
#51335=CARTESIAN_POINT ( 'NONE',  ( -17.93393266664992680, -11.91647553114624358, 32.58852847137147535 ) ) ;
#51336=FACE_OUTER_BOUND ( 'NONE', #41139, .T. ) ;
#51339=CARTESIAN_POINT ( 'NONE',  ( 4.153846153846154188, -8.318370150425687726, 35.83090037661290239 ) ) ;
#51340=DIRECTION ( 'NONE',  ( 1.000000000000000000, 0.000000000000000000, 0.000000000000000000 ) ) ;
#51341=CARTESIAN_POINT ( 'NONE',  ( 4.826946345980720920, -9.148715823498378086, 34.47080413974185120 ) ) ;
#51342=CARTESIAN_POINT ( 'NONE',  ( -16.21992853320628925, -2.833524468853757305, 32.15551576947924417 ) ) ;
#51343=EDGE_CURVE ( 'NONE', #54183, #66607, #74124, .T. ) ;
#51344=VECTOR ( 'NONE', #20840, 1000.000000000000000 ) ;
#51345=EDGE_LOOP ( 'NONE', ( #80717, #84917, #15913, #15730 ) ) ;
#51346=ORIENTED_EDGE ( 'NONE', *, *, #84019, .F. ) ;
#51347=ORIENTED_EDGE ( 'NONE', *, *, #38078, .T. ) ;
#51348=CYLINDRICAL_SURFACE ( 'NONE', #15682, 0.2499999999999994726 ) ;
#51349=ORIENTED_EDGE ( 'NONE', *, *, #18294, .F. ) ;
#51350=AXIS2_PLACEMENT_3D ( 'NONE', #19170, #69127, #7433 ) ;
#51351=VECTOR ( 'NONE', #2159, 999.9999999999998863 ) ;
#51352=LINE ( 'NONE', #24348, #26262 ) ;
#51354=ORIENTED_EDGE ( 'NONE', *, *, #25004, .F. ) ;
#51355=ADVANCED_FACE ( 'NONE', ( #79098 ), #67367, .F. ) ;
#51356=ORIENTED_EDGE ( 'NONE', *, *, #78057, .T. ) ;
#51359=CARTESIAN_POINT ( 'NONE',  ( -11.53846153846153655, -9.780366693483667717, 34.19971097300155094 ) ) ;
#51360=ORIENTED_EDGE ( 'NONE', *, *, #57103, .F. ) ;
#51362=B_SPLINE_CURVE_WITH_KNOTS ( 'NONE', 3,
 ( #61676, #68017, #6316, #53149, #60357, #12625, #68882, #18934, #27021, #26579 ),
 .UNSPECIFIED., .F., .F.,
 ( 4, 2, 2, 2, 4 ),
 ( 0.0007817246256747524850, 0.0009771112852218974409, 0.001172497944769042288, 0.001367884604316187136, 0.001563271263863332200 ),
 .UNSPECIFIED. ) ;
#51363=CARTESIAN_POINT ( 'NONE',  ( 4.088576153289834814, -12.70778746994557551, 30.41441678777548319 ) ) ;
#51364=CARTESIAN_POINT ( 'NONE',  ( 12.33084699487089964, -2.541943142973491554, 30.39792223712631980 ) ) ;
#51365=FACE_BOUND ( 'NONE', #70200, .T. ) ;
#51366=ORIENTED_EDGE ( 'NONE', *, *, #51389, .F. ) ;
#51367=CARTESIAN_POINT ( 'NONE',  ( 12.59233026936325039, -5.582136614379148654, 34.36778462344220486 ) ) ;
#51368=ADVANCED_FACE ( 'NONE', ( #72776 ), #82669, .F. ) ;
#51369=CARTESIAN_POINT ( 'NONE',  ( 5.011653076366756387, -3.643525952247789412, 33.31231777344662959 ) ) ;
#51370=AXIS2_PLACEMENT_3D ( 'NONE', #26599, #20726, #54058 ) ;
#51372=CARTESIAN_POINT ( 'NONE',  ( 7.846153846153725020, -10.90142922262034020, 33.41473453929536674 ) ) ;
#51373=ORIENTED_EDGE ( 'NONE', *, *, #68142, .T. ) ;
#51374=CARTESIAN_POINT ( 'NONE',  ( -6.989160334032802346, -6.386643153685125363, 34.62446782046654903 ) ) ;
#51377=VERTEX_POINT ( 'NONE', #54724 ) ;
#51378=CARTESIAN_POINT ( 'NONE',  ( 5.750023255951410839, -12.01397095200673881, 32.43157075238190146 ) ) ;
#51379=CARTESIAN_POINT ( 'NONE',  ( -9.442362282929646966, -8.476813868363244353, 34.90874843262270133 ) ) ;
#51380=CARTESIAN_POINT ( 'NONE',  ( 8.769230769230768274, -13.49023893513002648, 31.06009739812518688 ) ) ;
#51382=DIRECTION ( 'NONE',  ( -0.000000000000000000, -0.5000000000000009992, -0.8660254037844380415 ) ) ;
#51383=CARTESIAN_POINT ( 'NONE',  ( -15.29603923132555110, -3.643525952247789412, 33.31231777344662959 ) ) ;
#51384=ORIENTED_EDGE ( 'NONE', *, *, #55704, .F. ) ;
#51385=CARTESIAN_POINT ( 'NONE',  ( 6.923076923076800782, -2.657715359629662988, 31.77849191805970364 ) ) ;
#51386=AXIS2_PLACEMENT_3D ( 'NONE', #65418, #20241, #72619 ) ;
#51387=CARTESIAN_POINT ( 'NONE',  ( 17.77707304109314279, -3.395401636524186362, 33.02366814457250399 ) ) ;
#51388=FACE_OUTER_BOUND ( 'NONE', #53708, .T. ) ;
#51389=EDGE_CURVE ( 'NONE', #74826, #41702, #51, .T. ) ;
#51390=CARTESIAN_POINT ( 'NONE',  ( 13.31853197365950514, -12.37446782046654192, 30.86335684631486487 ) ) ;
#51392=ORIENTED_EDGE ( 'NONE', *, *, #3824, .F. ) ;
#51393=FACE_BOUND ( 'NONE', #69937, .T. ) ;
#51394=ORIENTED_EDGE ( 'NONE', *, *, #38503, .T. ) ;
#51395=FACE_OUTER_BOUND ( 'NONE', #26353, .T. ) ;
#51396=CARTESIAN_POINT ( 'NONE',  ( -7.846153846153844924, -4.786620604624113540, 33.94971097300155094 ) ) ;
#51397=ORIENTED_EDGE ( 'NONE', *, *, #66406, .T. ) ;
#51398=EDGE_CURVE ( 'NONE', #1771, #77592, #54610, .T. ) ;
#51399=CARTESIAN_POINT ( 'NONE',  ( -3.296852641725109834, -12.37446782046654192, 30.86335684631486487 ) ) ;
#51400=CARTESIAN_POINT ( 'NONE',  ( -5.076923076923075762, -10.89733346790207413, 36.13435417666054406 ) ) ;
#51401=DIRECTION ( 'NONE',  ( 0.000000000000000000, 0.6427876096865368094, 0.7660444431189802339 ) ) ;
#51403=VERTEX_POINT ( 'NONE', #34463 ) ;
#51404=CARTESIAN_POINT ( 'NONE',  ( 7.173076923076923350, -2.249999999999998668, 29.75000000000000355 ) ) ;
#51405=EDGE_LOOP ( 'NONE', ( #13931, #81180, #27817, #77190 ) ) ;
#51406=CARTESIAN_POINT ( 'NONE',  ( 16.94677586748485965, -10.88202310037936194, 33.43294751532457099 ) ) ;
#51408=CARTESIAN_POINT ( 'NONE',  ( 11.53846153846153832, -6.386643153685126251, 34.62446782046654192 ) ) ;
#51409=CARTESIAN_POINT ( 'NONE',  ( 4.088575707885377497, -6.879047030191174805, 34.71129190930000163 ) ) ;
#51411=AXIS2_PLACEMENT_3D ( 'NONE', #18422, #7005, #73363 ) ;
#51412=CARTESIAN_POINT ( 'NONE',  ( 10.55011461482829738, -12.51329471203370325, 31.30864560766548976 ) ) ;
#51414=EDGE_CURVE ( 'NONE', #68029, #42856, #83617, .T. ) ;
#51415=CARTESIAN_POINT ( 'NONE',  ( 5.299934428535925335, -12.39991518177334129, 30.74647679643404530 ) ) ;
#51418=AXIS2_PLACEMENT_3D ( 'NONE', #56725, #899, #48632 ) ;
#51419=CARTESIAN_POINT ( 'NONE',  ( 17.07692307692307665, -2.833524468853757305, 32.15551576947925838 ) ) ;
#51420=CARTESIAN_POINT ( 'NONE',  ( -15.16551365949320029, -3.835265460703683349, 33.15142922261929925 ) ) ;
#51421=CYLINDRICAL_SURFACE ( 'NONE', #62540, 0.2500000000000009437 ) ;
#51422=ADVANCED_FACE ( 'NONE', ( #88113 ), #48858, .F. ) ;
#51424=EDGE_CURVE ( 'NONE', #78537, #75330, #1916, .T. ) ;
#51425=ORIENTED_EDGE ( 'NONE', *, *, #88361, .T. ) ;
#51426=CARTESIAN_POINT ( 'NONE',  ( -15.23076923076922995, -13.53365097954675988, 30.81389545987213552 ) ) ;
#51427=CARTESIAN_POINT ( 'NONE',  ( 7.780071466793711643, -6.343179335718451384, 34.87096338111212646 ) ) ;
#51428=LINE ( 'NONE', #22223, #40431 ) ;
#51430=CARTESIAN_POINT ( 'NONE',  ( 16.08857615328984281, -10.33852847137145048, 34.16647553114627556 ) ) ;
#51431=CARTESIAN_POINT ( 'NONE',  ( -6.923076923076922462, -6.435427911321262684, 35.78748833219616898 ) ) ;
#51432=CARTESIAN_POINT ( 'NONE',  ( -14.98082382139119062, -8.476813868363244353, 34.90874843262270133 ) ) ;
#51433=VERTEX_POINT ( 'NONE', #75451 ) ;
#51434=CARTESIAN_POINT ( 'NONE',  ( -9.692307692307812417, -12.27809138561165270, 31.22303859784587132 ) ) ;
#51435=CARTESIAN_POINT ( 'NONE',  ( -17.30040802064703342, -12.24155766932282496, 31.33739205006857986 ) ) ;
#51436=CARTESIAN_POINT ( 'NONE',  ( -6.222878682428645725, -7.630691491037286056, 34.74850469731152458 ) ) ;
#51437=ADVANCED_FACE ( 'NONE', ( #19616 ), #41670, .F. ) ;
#51439=B_SPLINE_CURVE_WITH_KNOTS ( 'NONE', 3,
 ( #33694, #40897, #75999, #88221, #68359, #68803, #69249, #34577, #7102, #27816 ),
 .UNSPECIFIED., .F., .F.,
 ( 4, 2, 2, 2, 4 ),
 ( 0.0007817246256747459798, 0.0009771112852218896347, 0.001172497944769033398, 0.001367884604316177161, 0.001563271263863320708 ),
 .UNSPECIFIED. ) ;
#51440=ORIENTED_EDGE ( 'NONE', *, *, #44800, .T. ) ;
#51441=CARTESIAN_POINT ( 'NONE',  ( 13.63456090296352841, -6.696923467548660192, 34.68552623307873972 ) ) ;
#51442=B_SPLINE_CURVE_WITH_KNOTS ( 'NONE', 3,
 ( #69550, #36654, #20915, #1541, #56033, #22690, #42972, #56914, #48387, #70445 ),
 .UNSPECIFIED., .F., .F.,
 ( 4, 2, 2, 2, 4 ),
 ( 0.0007817359430256318490, 0.0009771253907249984917, 0.001172514838424365026, 0.001367904286123731560, 0.001563293733823098311 ),
 .UNSPECIFIED. ) ;
#51443=EDGE_LOOP ( 'NONE', ( #19380, #70843, #50344, #47062 ) ) ;
#51444=VECTOR ( 'NONE', #42251, 1000.000000000000227 ) ;
#51445=CARTESIAN_POINT ( 'NONE',  ( 0.5267940328144851136, -9.442884908240271713, 34.35708131394835618 ) ) ;
#51446=CARTESIAN_POINT ( 'NONE',  ( 2.307692307692309264, -7.500000000000001776, 35.04278698407183867 ) ) ;
#51447=ADVANCED_FACE ( 'NONE', ( #27702 ), #88989, .F. ) ;
#51448=CARTESIAN_POINT ( 'NONE',  ( 6.923076923076924238, -1.466349020453238561, 30.81389545987213907 ) ) ;
#51449=ORIENTED_EDGE ( 'NONE', *, *, #35378, .F. ) ;
#51450=B_SPLINE_CURVE_WITH_KNOTS ( 'NONE', 3,
 ( #35980, #41405, #22015, #70199, #76066, #48148, #14365, #76962, #48588, #68866 ),
 .UNSPECIFIED., .F., .F.,
 ( 4, 2, 2, 2, 4 ),
 ( 0.000000000000000000, 0.0001954339881912759433, 0.0003908679763825518867, 0.0005863019645738304321, 0.0007817359527651089775 ),
 .UNSPECIFIED. ) ;
#51451=CARTESIAN_POINT ( 'NONE',  ( -1.634638608836841867, -12.68155406624981119, 30.59749803192733708 ) ) ;
#51452=CARTESIAN_POINT ( 'NONE',  ( -5.999999999999998224, -4.786620604624113540, 33.94971097300155094 ) ) ;
#51454=CIRCLE ( 'NONE', #25577, 0.2500000000000002220 ) ;
#51455=DIRECTION ( 'NONE',  ( 0.000000000000000000, 0.3420201433256641055, -0.9396926207859100932 ) ) ;
#51456=CARTESIAN_POINT ( 'NONE',  ( 3.230769230769231726, -2.833524468853757305, 32.15551576947925838 ) ) ;
#51457=EDGE_CURVE ( 'NONE', #71885, #71376, #87949, .T. ) ;
#51459=ORIENTED_EDGE ( 'NONE', *, *, #51926, .F. ) ;
#51460=CARTESIAN_POINT ( 'NONE',  ( 16.21991348719623360, -9.905515769479276145, 34.41647553114623292 ) ) ;
#51461=VERTEX_POINT ( 'NONE', #3217 ) ;
#51462=ADVANCED_FACE ( 'NONE', ( #64911 ), #8329, .F. ) ;
#51463=CARTESIAN_POINT ( 'NONE',  ( 4.946231610255514610, -12.11776431015576172, 31.66791131148498906 ) ) ;
#51465=CARTESIAN_POINT ( 'NONE',  ( -16.40382288478850725, -11.28823185664190376, 33.01397839955799896 ) ) ;
#51467=CARTESIAN_POINT ( 'NONE',  ( -14.08491276642389423, -11.89424750095246175, 32.13594075562311758 ) ) ;
#51468=CARTESIAN_POINT ( 'NONE',  ( 12.59233026936325039, -9.804649428959608670, 34.18742332936588468 ) ) ;
#51469=VERTEX_POINT ( 'NONE', #17178 ) ;
#51471=ORIENTED_EDGE ( 'NONE', *, *, #78853, .T. ) ;
#51473=ORIENTED_EDGE ( 'NONE', *, *, #28009, .T. ) ;
#51474=ORIENTED_EDGE ( 'NONE', *, *, #46445, .T. ) ;
#51475=B_SPLINE_CURVE_WITH_KNOTS ( 'NONE', 3,
 ( #77151, #49675, #34827, #49237, #606, #69503, #28077, #64066, #69945, #15457 ),
 .UNSPECIFIED., .F., .F.,
 ( 4, 2, 2, 2, 4 ),
 ( 0.000000000000000000, 0.0001954339857564073659, 0.0003908679715128147319, 0.0005863019572692221250, 0.0007817359430256294638 ),
 .UNSPECIFIED. ) ;
#51477=CARTESIAN_POINT ( 'NONE',  ( -2.177166605928740672, -3.285477652293413264, 32.44071101563363158 ) ) ;
#51478=DIRECTION ( 'NONE',  ( 0.000000000000000000, 0.6427876096865368094, 0.7660444431189802339 ) ) ;
#51479=LINE ( 'NONE', #38445, #82530 ) ;
#51480=CARTESIAN_POINT ( 'NONE',  ( -4.153846153846274980, -9.528491918059723176, 34.59228464037033035 ) ) ;
#51481=CARTESIAN_POINT ( 'NONE',  ( -12.71156168575991785, -12.45566812827425451, 31.48439005359158926 ) ) ;
#51482=CARTESIAN_POINT ( 'NONE',  ( 5.749976762707035505, -11.86270091957321249, 32.19358267280087915 ) ) ;
#51483=CARTESIAN_POINT ( 'NONE',  ( -4.153846153846152411, -10.51840700105979565, 33.73612834413961536 ) ) ;
#51484=CARTESIAN_POINT ( 'NONE',  ( 8.096208266067298709, -4.818054556918156983, 34.26375889529406749 ) ) ;
#51487=EDGE_CURVE ( 'NONE', #84770, #37942, #86813, .T. ) ;
#51488=ORIENTED_EDGE ( 'NONE', *, *, #17043, .F. ) ;
#51489=ORIENTED_EDGE ( 'NONE', *, *, #25820, .F. ) ;
#51490=CARTESIAN_POINT ( 'NONE',  ( 6.066067333350078528, -12.34228464037088813, 31.77849191805839268 ) ) ;
#51491=ORIENTED_EDGE ( 'NONE', *, *, #79140, .T. ) ;
#51492=CARTESIAN_POINT ( 'NONE',  ( 8.769230769230768274, -8.120952969808772792, 34.71129190930000163 ) ) ;
#51493=CARTESIAN_POINT ( 'NONE',  ( 8.769230769230768274, -5.471508081941601098, 34.59228464037088457 ) ) ;
#51494=CARTESIAN_POINT ( 'NONE',  ( 1.634560793993429462, -4.932303261841489039, 34.32971442181322885 ) ) ;
#51495=CARTESIAN_POINT ( 'NONE',  ( -11.40767109749459074, -9.084667340241226796, 34.75534355489798344 ) ) ;
#51496=ORIENTED_EDGE ( 'NONE', *, *, #38635, .T. ) ;
#51497=ORIENTED_EDGE ( 'NONE', *, *, #49313, .T. ) ;
#51498=CARTESIAN_POINT ( 'NONE',  ( -2.242498325908949486, -2.506253911140448043, 29.99999999999988631 ) ) ;
#51500=FACE_BOUND ( 'NONE', #36052, .T. ) ;
#51501=CARTESIAN_POINT ( 'NONE',  ( 13.45068271796546178, -12.34228464037088813, 31.77849191805839268 ) ) ;
#51502=AXIS2_PLACEMENT_3D ( 'NONE', #5680, #6131, #47550 ) ;
#51503=FACE_OUTER_BOUND ( 'NONE', #15083, .T. ) ;
#51504=ORIENTED_EDGE ( 'NONE', *, *, #49477, .T. ) ;
#51505=CARTESIAN_POINT ( 'NONE',  ( 14.24160889673642671, -2.721908614388770964, 31.22303859784723912 ) ) ;
#51506=CARTESIAN_POINT ( 'NONE',  ( 8.546402671595890510, -7.369209533119137845, 34.99857337881830688 ) ) ;
#51507=CARTESIAN_POINT ( 'NONE',  ( -2.307692307692305711, -2.708943851104267164, 35.45975837776705220 ) ) ;
#51508=ORIENTED_EDGE ( 'NONE', *, *, #55368, .T. ) ;
#51509=CARTESIAN_POINT ( 'NONE',  ( -11.66860950819323328, -5.070767119584671079, 34.40440758774516183 ) ) ;
#51510=CARTESIAN_POINT ( 'NONE',  ( 6.989144256427000990, -5.471508081941601098, 34.59228464037088457 ) ) ;
#51511=EDGE_LOOP ( 'NONE', ( #63333, #49113, #7542, #7425, #53923 ) ) ;
#51512=B_SPLINE_CURVE_WITH_KNOTS ( 'NONE', 3,
 ( #55839, #56289, #22499, #57170, #69800, #49962, #35129, #55399, #8108, #29710 ),
 .UNSPECIFIED., .F., .F.,
 ( 4, 2, 2, 2, 4 ),
 ( 0.000000000000000000, 0.0001954311564186858715, 0.0003908623128373717431, 0.0005862934692560576146, 0.0007817246256747434861 ),
 .UNSPECIFIED. ) ;
#51513=AXIS2_PLACEMENT_3D ( 'NONE', #34767, #88411, #81638 ) ;
#51514=CARTESIAN_POINT ( 'NONE',  ( 6.066166606591640864, -7.250054591869668386, 34.99404684341514127 ) ) ;
#51515=DIRECTION ( 'NONE',  ( 0.000000000000000000, 0.7660444431189807890, 0.6427876096865361433 ) ) ;
#51516=VERTEX_POINT ( 'NONE', #44186 ) ;
#51517=CARTESIAN_POINT ( 'NONE',  ( -0.4615384615384611200, -8.318370150425687726, 35.83090037661290239 ) ) ;
#51518=CARTESIAN_POINT ( 'NONE',  ( -12.39628289026243380, -2.625532179533470512, 30.86335684631491105 ) ) ;
#51519=DIRECTION ( 'NONE',  ( 0.000000000000000000, 1.000000000000000000, 8.673617379884033500E-16 ) ) ;
#51520=CARTESIAN_POINT ( 'NONE',  ( -10.55012904410859242, -6.026961402152789304, 34.52809138561124769 ) ) ;
#51521=CARTESIAN_POINT ( 'NONE',  ( -8.769230769230768274, -12.78798330534102945, 29.74999999999997868 ) ) ;
#51522=FACE_BOUND ( 'NONE', #75479, .T. ) ;
#51523=CARTESIAN_POINT ( 'NONE',  ( -1.514762594053602029, -2.882441371585227952, 31.66841991370172948 ) ) ;
#51525=AXIS2_PLACEMENT_3D ( 'NONE', #60905, #52368, #11392 ) ;
#51526=DIRECTION ( 'NONE',  ( -0.000000000000000000, 0.1736481776669307198, -0.9848077530122080203 ) ) ;
#51527=DIRECTION ( 'NONE',  ( -0.000000000000000000, 0.7660444431189791237, -0.6427876096865379196 ) ) ;
#51528=CARTESIAN_POINT ( 'NONE',  ( 9.019285080869085647, -2.779044189368095719, 31.39831045268885745 ) ) ;
#51530=ORIENTED_EDGE ( 'NONE', *, *, #65218, .T. ) ;
#51531=LINE ( 'NONE', #9683, #30350 ) ;
#51532=ORIENTED_EDGE ( 'NONE', *, *, #48163, .F. ) ;
#51533=EDGE_CURVE ( 'NONE', #49416, #19438, #24821, .T. ) ;
#51535=CARTESIAN_POINT ( 'NONE',  ( 16.15384615384603251, -11.48612834414049644, 32.76840700105863391 ) ) ;
#51538=CARTESIAN_POINT ( 'NONE',  ( -39.05038313613820122, -2.249999999999998668, 29.75000000000000355 ) ) ;
#51540=CARTESIAN_POINT ( 'NONE',  ( -13.16160254052198830, -5.582272713120729257, 34.63742843783360570 ) ) ;
#51541=CARTESIAN_POINT ( 'NONE',  ( -9.822455662039388358, -12.70455904226513866, 30.44083106164009322 ) ) ;
#51543=CARTESIAN_POINT ( 'NONE',  ( -14.37296230824862953, -11.06231777344662781, 33.60647404775220082 ) ) ;
#51544=CARTESIAN_POINT ( 'NONE',  ( 14.30769230769231015, -6.386643153685126251, 34.62446782046654192 ) ) ;
#51545=CARTESIAN_POINT ( 'NONE',  ( -12.46153846153846168, -13.04860791097971706, 34.73218667398347037 ) ) ;
#51546=DIRECTION ( 'NONE',  ( 1.000000000000000000, -0.000000000000000000, -0.000000000000000000 ) ) ;
#51547=EDGE_CURVE ( 'NONE', #51792, #30710, #7354, .T. ) ;
#51549=CARTESIAN_POINT ( 'NONE',  ( 17.07692307692307665, -5.557115091759785130, 34.35708131394839171 ) ) ;
#51550=CARTESIAN_POINT ( 'NONE',  ( 14.37376065869474751, -10.51840700105979565, 33.73612834413962247 ) ) ;
#51551=ADVANCED_FACE ( 'NONE', ( #63260 ), #56063, .F. ) ;
#51552=DIRECTION ( 'NONE',  ( -0.000000000000000000, 0.5000000000000011102, -0.8660254037844381525 ) ) ;
#51553=AXIS2_PLACEMENT_3D ( 'NONE', #51176, #30922, #17875 ) ;
#51554=EDGE_LOOP ( 'NONE', ( #3346, #5545 ) ) ;
#51555=CARTESIAN_POINT ( 'NONE',  ( -13.44988538517170440, -6.835583212224499938, 34.95778746994557906 ) ) ;
#51556=CARTESIAN_POINT ( 'NONE',  ( 11.53846153846141753, -3.835265460704628371, 33.15142922262033665 ) ) ;
#51557=CARTESIAN_POINT ( 'NONE',  ( -2.307692307692305711, -2.292212530054420494, 30.41441678777542634 ) ) ;
#51558=CARTESIAN_POINT ( 'NONE',  ( 1.634615384615389688, -2.499999999999999556, 29.81604066197450109 ) ) ;
#51559=CARTESIAN_POINT ( 'NONE',  ( 15.36160764878199458, -7.277220443632450575, 34.74524770363009196 ) ) ;
#51560=CARTESIAN_POINT ( 'NONE',  ( -2.980714810855777497, -5.642605341092957083, 34.66089969410670335 ) ) ;
#51561=B_SPLINE_CURVE_WITH_KNOTS ( 'NONE', 3,
 ( #56413, #77126, #17190, #10888, #60397, #45552, #51849, #31142, #31597, #38808 ),
 .UNSPECIFIED., .F., .F.,
 ( 4, 2, 2, 2, 4 ),
 ( 0.000000000000000000, 0.0001954339857564092904, 0.0003908679715128185808, 0.0005863019572692278712, 0.0007817359430256371616 ),
 .UNSPECIFIED. ) ;
#51562=ORIENTED_EDGE ( 'NONE', *, *, #62800, .T. ) ;
#51563=DIRECTION ( 'NONE',  ( 0.000000000000000000, 0.6427876096865373645, -0.7660444431189797898 ) ) ;
#51564=ORIENTED_EDGE ( 'NONE', *, *, #86161, .F. ) ;
#51566=ORIENTED_EDGE ( 'NONE', *, *, #7791, .T. ) ;
#51568=AXIS2_PLACEMENT_3D ( 'NONE', #59086, #59534, #87036 ) ;
#51569=CARTESIAN_POINT ( 'NONE',  ( 3.361561038594018225, -5.582136614379148654, 34.36778462344220486 ) ) ;
#51570=CARTESIAN_POINT ( 'NONE',  ( -9.442362173959550020, -6.696923467548660192, 34.68552623307873972 ) ) ;
#51572=CARTESIAN_POINT ( 'NONE',  ( 5.869308533332444178, -2.729777683071817229, 31.24903638046268739 ) ) ;
#51573=B_SPLINE_CURVE_WITH_KNOTS ( 'NONE', 3,
 ( #42224, #56167, #30026, #22816, #64232, #7985, #1217, #9318, #43094, #28701 ),
 .UNSPECIFIED., .F., .F.,
 ( 4, 2, 2, 2, 4 ),
 ( 0.0007817359430256257775, 0.0009771253907249911191, 0.001172514838424356352, 0.001367904286123721586, 0.001563293733823086819 ),
 .UNSPECIFIED. ) ;
#51574=AXIS2_PLACEMENT_3D ( 'NONE', #74666, #53937, #329 ) ;
#51575=EDGE_LOOP ( 'NONE', ( #18857, #56691 ) ) ;
#51576=EDGE_CURVE ( 'NONE', #43597, #25676, #49297, .T. ) ;
#51578=ORIENTED_EDGE ( 'NONE', *, *, #41605, .F. ) ;
#51579=ORIENTED_EDGE ( 'NONE', *, *, #63537, .T. ) ;
#51580=EDGE_CURVE ( 'NONE', #51322, #10219, #40699, .T. ) ;
#51582=EDGE_CURVE ( 'NONE', #76630, #39878, #50232, .T. ) ;
#51583=CARTESIAN_POINT ( 'NONE',  ( 1.318531973659506251, -11.16473453929635440, 33.15142922261925662 ) ) ;
#51584=CARTESIAN_POINT ( 'NONE',  ( 15.23076923076910916, -4.320704448113951379, 33.92786785259630022 ) ) ;
#51585=FACE_OUTER_BOUND ( 'NONE', #68326, .T. ) ;
#51586=CARTESIAN_POINT ( 'NONE',  ( -14.98071491913091791, -3.136992222400443175, 32.19305428654138979 ) ) ;
#51587=CARTESIAN_POINT ( 'NONE',  ( -11.60373153901785948, -8.656820664281498878, 34.87096338111211935 ) ) ;
#51588=CARTESIAN_POINT ( 'NONE',  ( -16.15384615384627409, -2.892918686052165622, 31.69288490824153470 ) ) ;
#51589=ORIENTED_EDGE ( 'NONE', *, *, #29503, .F. ) ;
#51590=EDGE_CURVE ( 'NONE', #75299, #68166, #24568, .T. ) ;
#51591=ORIENTED_EDGE ( 'NONE', *, *, #38429, .T. ) ;
#51593=VERTEX_POINT ( 'NONE', #20300 ) ;
#51594=CARTESIAN_POINT ( 'NONE',  ( -10.61538461538473399, -11.94971097300221174, 32.03036669348237098 ) ) ;
#51595=ORIENTED_EDGE ( 'NONE', *, *, #54730, .T. ) ;
#51596=DIRECTION ( 'NONE',  ( -1.000000000000000000, 0.000000000000000000, 0.000000000000000000 ) ) ;
#51598=ADVANCED_FACE ( 'NONE', ( #26606 ), #45981, .F. ) ;
#51599=ADVANCED_FACE ( 'NONE', ( #73018 ), #5897, .F. ) ;
#51601=ORIENTED_EDGE ( 'NONE', *, *, #74131, .F. ) ;
#51602=DIRECTION ( 'NONE',  ( -0.000000000000000000, 1.000000000000000000, 3.491481338843133355E-15 ) ) ;
#51603=B_SPLINE_CURVE_WITH_KNOTS ( 'NONE', 3,
 ( #75542, #54832, #67469, #34565, #33237, #60701, #18835, #88208, #33681, #62028 ),
 .UNSPECIFIED., .F., .F.,
 ( 4, 2, 2, 2, 4 ),
 ( 0.0007817359430256303312, 0.0009771253907249965402, 0.001172514838424362641, 0.001367904286123728958, 0.001563293733823095059 ),
 .UNSPECIFIED. ) ;
#51604=AXIS2_PLACEMENT_3D ( 'NONE', #38490, #60529, #32612 ) ;
#51605=EDGE_LOOP ( 'NONE', ( #80340, #44998, #82261, #55183 ) ) ;
#51606=ADVANCED_FACE ( 'NONE', ( #88775 ), #32034, .F. ) ;
#51607=CARTESIAN_POINT ( 'NONE',  ( -2.307692307692305711, -12.10708131394839349, 31.69288490824020244 ) ) ;
#51608=DIRECTION ( 'NONE',  ( -0.000000000000000000, 0.6427876096865404731, -0.7660444431189771253 ) ) ;
#51609=B_SPLINE_CURVE_WITH_KNOTS ( 'NONE', 3,
 ( #72637, #10946, #4180, #58231, #30327, #44258, #5527, #6416, #66331, #53701 ),
 .UNSPECIFIED., .F., .F.,
 ( 4, 2, 2, 2, 4 ),
 ( 0.000000000000000000, 0.0001954339857564091278, 0.0003908679715128182556, 0.0005863019572692274375, 0.0007817359430256365111 ),
 .UNSPECIFIED. ) ;
#51610=CARTESIAN_POINT ( 'NONE',  ( -15.23076923076935252, -3.083524468854526912, 32.58852847137268327 ) ) ;
#51611=CARTESIAN_POINT ( 'NONE',  ( 10.74622303339737606, -7.277220443632450575, 34.74524770363009196 ) ) ;
#51612=CARTESIAN_POINT ( 'NONE',  ( -6.792285115252136407, -2.541949514083464479, 30.39797389878540557 ) ) ;
#51613=CARTESIAN_POINT ( 'NONE',  ( 8.639083559792549494, -6.001485441113819874, 34.52039167877662607 ) ) ;
#51614=CARTESIAN_POINT ( 'NONE',  ( -3.361459833879537840, -8.191372820521381826, 34.95448215188423546 ) ) ;
#51616=CARTESIAN_POINT ( 'NONE',  ( -10.74553182482283198, -10.19110544564092002, 33.96427741523702792 ) ) ;
#51617=CARTESIAN_POINT ( 'NONE',  ( -8.899378738962466784, -4.299443229763728169, 33.91186481527756058 ) ) ;
#51618=ORIENTED_EDGE ( 'NONE', *, *, #56395, .F. ) ;
#51619=CARTESIAN_POINT ( 'NONE',  ( -7.846153846153844924, -4.102666532097928531, 36.13435417666054406 ) ) ;
#51620=CARTESIAN_POINT ( 'NONE',  ( 15.36129493253279676, -4.459921816937791661, 33.71989282347011851 ) ) ;
#51621=CARTESIAN_POINT ( 'NONE',  ( 10.39189969082028675, -8.539481045369596401, 34.89627647299170832 ) ) ;
#51622=DIRECTION ( 'NONE',  ( -0.000000000000000000, 0.1736481776669307198, -0.9848077530122080203 ) ) ;
#51623=CARTESIAN_POINT ( 'NONE',  ( 7.716006636715626144, -8.587444163452046197, 34.63053765926554206 ) ) ;
#51624=FACE_BOUND ( 'NONE', #56736, .T. ) ;
#51625=CARTESIAN_POINT ( 'NONE',  ( 5.207713517890025123, -5.496552790871117367, 34.60292014791297532 ) ) ;
#51626=DIRECTION ( 'NONE',  ( 0.000000000000000000, 0.000000000000000000, 1.000000000000000000 ) ) ;
#51628=DIRECTION ( 'NONE',  ( -0.000000000000000000, 0.9396926207859093161, -0.3420201433256663259 ) ) ;
#51629=CARTESIAN_POINT ( 'NONE',  ( 0.7114838709165041131, -2.986452184633680229, 32.43230066228895225 ) ) ;
#51630=CYLINDRICAL_SURFACE ( 'NONE', #64256, 0.2499999999999997502 ) ;
#51635=VECTOR ( 'NONE', #13987, 1000.000000000000000 ) ;
#51636=AXIS2_PLACEMENT_3D ( 'NONE', #78083, #63677, #15062 ) ;
#51638=CARTESIAN_POINT ( 'NONE',  ( -13.38461538461506883, -2.255955759149395501, 30.00000000000324363 ) ) ;
#51639=DIRECTION ( 'NONE',  ( 0.000000000000000000, 0.1736481776669275834, 0.9848077530122086864 ) ) ;
#51641=CARTESIAN_POINT ( 'NONE',  ( -4.219116154402472674, -5.094484230520674117, 34.41647553114621161 ) ) ;
#51642=CARTESIAN_POINT ( 'NONE',  ( -9.627052121031661969, -4.481592998940250538, 33.73612834413965089 ) ) ;
#51644=EDGE_CURVE ( 'NONE', #58712, #3792, #65411, .T. ) ;
#51645=CYLINDRICAL_SURFACE ( 'NONE', #87835, 0.2499999999999986955 ) ;
#51646=CARTESIAN_POINT ( 'NONE',  ( -2.084912638714239375, -6.717445702608402236, 34.94155399931962336 ) ) ;
#51647=AXIS2_PLACEMENT_3D ( 'NONE', #41776, #67476, #47642 ) ;
#51648=CARTESIAN_POINT ( 'NONE',  ( 3.230769230769231726, -3.937682226553329556, 33.60647404775216529 ) ) ;
#51649=DIRECTION ( 'NONE',  ( -0.000000000000000000, -0.000000000000000000, -1.000000000000000000 ) ) ;
#51650=CARTESIAN_POINT ( 'NONE',  ( 8.545745825506822158, -10.11188796281391511, 34.01382737946119050 ) ) ;
#51651=CARTESIAN_POINT ( 'NONE',  ( 3.903869422903799347, -10.66389620160130036, 33.62221079203477103 ) ) ;
#51652=ADVANCED_FACE ( 'NONE', ( #27050 ), #82005, .F. ) ;
#51654=LINE ( 'NONE', #45357, #34760 ) ;
#51655=B_SPLINE_CURVE_WITH_KNOTS ( 'NONE', 3,
 ( #25821, #73579, #47853, #13627, #74447, #53278, #11871, #61354, #60488, #74901 ),
 .UNSPECIFIED., .F., .F.,
 ( 4, 2, 2, 2, 4 ),
 ( 0.000000000000000000, 0.0001954311564186868744, 0.0003908623128373737488, 0.0005862934692560606504, 0.0007817246256747474977 ),
 .UNSPECIFIED. ) ;
#51657=ORIENTED_EDGE ( 'NONE', *, *, #51590, .F. ) ;
#51658=EDGE_CURVE ( 'NONE', #15864, #51461, #39695, .T. ) ;
#51659=CARTESIAN_POINT ( 'NONE',  ( -6.923076923076922462, -3.886160181151819604, 36.00935417666054406 ) ) ;
#51662=CARTESIAN_POINT ( 'NONE',  ( -10.74553258511630993, -10.31621877034669588, 34.18098118002070152 ) ) ;
#51663=CARTESIAN_POINT ( 'NONE',  ( 3.230769230769231726, -11.69971097300155272, 32.46337939537588113 ) ) ;
#51664=ORIENTED_EDGE ( 'NONE', *, *, #81102, .F. ) ;
#51665=CARTESIAN_POINT ( 'NONE',  ( 14.30769230769261569, -2.506253911140615021, 30.00000000000323297 ) ) ;
#51666=DIRECTION ( 'NONE',  ( -0.000000000000000000, 0.7660444431189791237, -0.6427876096865379196 ) ) ;
#51669=CARTESIAN_POINT ( 'NONE',  ( -12.46153846153858424, -9.528491918059723176, 34.59228464037033035 ) ) ;
#51670=DIRECTION ( 'NONE',  ( 0.000000000000000000, 0.9396926207859126468, 0.3420201433256571111 ) ) ;
#51671=CARTESIAN_POINT ( 'NONE',  ( 14.30769230769218758, -4.481592998941358097, 33.73612834414048933 ) ) ;
#51672=CARTESIAN_POINT ( 'NONE',  ( 8.900022577055556994, -4.809403383903225304, 33.96459661697924304 ) ) ;
#51673=EDGE_CURVE ( 'NONE', #13144, #72929, #4146, .T. ) ;
#51675=CARTESIAN_POINT ( 'NONE',  ( 2.307692307692187583, -12.27809138561165270, 31.22303859784587132 ) ) ;
#51676=CARTESIAN_POINT ( 'NONE',  ( -11.78846153846154543, -2.249999999999999556, 29.81609741502489541 ) ) ;
#51677=CARTESIAN_POINT ( 'NONE',  ( -10.61538461538461320, -7.500000000000001776, 35.04278698407183867 ) ) ;
#51678=EDGE_LOOP ( 'NONE', ( #56153, #75801, #56842, #8648 ) ) ;
#51679=ORIENTED_EDGE ( 'NONE', *, *, #86075, .T. ) ;
#51680=AXIS2_PLACEMENT_3D ( 'NONE', #41147, #15895, #70392 ) ;
#51681=EDGE_LOOP ( 'NONE', ( #42570, #55373, #15296, #17769 ) ) ;
#51682=CYLINDRICAL_SURFACE ( 'NONE', #24185, 0.2499999999999995559 ) ;
#51683=CARTESIAN_POINT ( 'NONE',  ( 10.61538461538461675, -11.35647404775217417, 33.31231777344666511 ) ) ;
#51684=EDGE_CURVE ( 'NONE', #82908, #69788, #8558, .T. ) ;
#51685=EDGE_CURVE ( 'NONE', #42060, #45555, #76090, .T. ) ;
#51686=CARTESIAN_POINT ( 'NONE',  ( 13.16168916709923664, -11.24512374952581872, 33.06303171183252942 ) ) ;
#51687=CARTESIAN_POINT ( 'NONE',  ( -0.4615384615384611200, -9.819645486525091727, 36.12317359536749706 ) ) ;
#51688=B_SPLINE_CURVE_WITH_KNOTS ( 'NONE', 3,
 ( #34651, #62119, #6728, #68000, #7178, #88296, #26568, #12167, #54024, #39652 ),
 .UNSPECIFIED., .F., .F.,
 ( 4, 2, 2, 2, 4 ),
 ( 0.000000000000000000, 0.0001954311564186877960, 0.0003908623128373755920, 0.0005862934692560633609, 0.0007817246256747511840 ),
 .UNSPECIFIED. ) ;
#51689=B_SPLINE_CURVE_WITH_KNOTS ( 'NONE', 3,
 ( #78253, #76940, #1720, #42715, #63857, #70177, #2156, #29643, #49898, #78707 ),
 .UNSPECIFIED., .F., .F.,
 ( 4, 2, 2, 2, 4 ),
 ( 0.000000000000000000, 0.0001954311564186868202, 0.0003908623128373736404, 0.0005862934692560604335, 0.0007817246256747472808 ),
 .UNSPECIFIED. ) ;
#51690=EDGE_LOOP ( 'NONE', ( #66842, #12698 ) ) ;
#51691=EDGE_CURVE ( 'NONE', #69353, #60920, #34134, .T. ) ;
#51692=EDGE_LOOP ( 'NONE', ( #34269, #16602 ) ) ;
#51693=DIRECTION ( 'NONE',  ( -0.000000000000000000, -0.1736481776669307198, -0.9848077530122080203 ) ) ;
#51694=ORIENTED_EDGE ( 'NONE', *, *, #583, .F. ) ;
#51695=CARTESIAN_POINT ( 'NONE',  ( 7.596153846153846700, -7.500000000000001776, 34.75000000000000000 ) ) ;
#51696=CARTESIAN_POINT ( 'NONE',  ( 16.21991348719623360, -8.164416787775445883, 34.95778746994558617 ) ) ;
#51697=VECTOR ( 'NONE', #32563, 999.9999999999998863 ) ;
#51698=CARTESIAN_POINT ( 'NONE',  ( -8.519176457592452678, -12.41262288849542017, 30.68299917996395010 ) ) ;
#51699=DIRECTION ( 'NONE',  ( -0.000000000000000000, 0.5000000000000011102, -0.8660254037844380415 ) ) ;
#51700=ORIENTED_EDGE ( 'NONE', *, *, #23884, .F. ) ;
#51701=AXIS2_PLACEMENT_3D ( 'NONE', #71484, #50759, #51639 ) ;
#51702=ORIENTED_EDGE ( 'NONE', *, *, #70344, .T. ) ;
#51704=ORIENTED_EDGE ( 'NONE', *, *, #26826, .F. ) ;
#51706=EDGE_LOOP ( 'NONE', ( #40315, #66681 ) ) ;
#51708=CARTESIAN_POINT ( 'NONE',  ( -5.749945688361683516, -8.303483539816728154, 34.68545999027711702 ) ) ;
#51709=ADVANCED_FACE ( 'NONE', ( #62594 ), #8112, .F. ) ;
#51710=CARTESIAN_POINT ( 'NONE',  ( -13.63463862190834952, -6.695914987888146541, 34.68535235679833306 ) ) ;
#51711=ORIENTED_EDGE ( 'NONE', *, *, #81891, .T. ) ;
#51713=CARTESIAN_POINT ( 'NONE',  ( 17.07692307692295586, -4.320704448113951379, 33.92786785259630022 ) ) ;
#51714=CARTESIAN_POINT ( 'NONE',  ( -5.934744860487159102, -3.643525952247864463, 33.31231777344670064 ) ) ;
#51715=FACE_BOUND ( 'NONE', #19945, .T. ) ;
#51717=CARTESIAN_POINT ( 'NONE',  ( -4.284537620513714451, -12.11776431015576172, 31.66791131148498906 ) ) ;
#51718=CARTESIAN_POINT ( 'NONE',  ( 8.519254038288416098, -2.564618984488975517, 30.55390908950641915 ) ) ;
#51720=CARTESIAN_POINT ( 'NONE',  ( 9.823099500132480344, -3.062576670634119758, 32.05464942895959979 ) ) ;
#51721=CARTESIAN_POINT ( 'NONE',  ( 17.99999999999987566, -6.835583212225970762, 34.95778746994575670 ) ) ;
#51723=ORIENTED_EDGE ( 'NONE', *, *, #61421, .T. ) ;
#51724=CARTESIAN_POINT ( 'NONE',  ( 14.53111926955388000, -7.630147231320743018, 34.74852402298682819 ) ) ;
#51725=CARTESIAN_POINT ( 'NONE',  ( -13.31854805126531005, -3.937682226553329556, 33.60647404775216529 ) ) ;
#51726=ORIENTED_EDGE ( 'NONE', *, *, #35977, .T. ) ;
#51727=VERTEX_POINT ( 'NONE', #49540 ) ;
#51728=DIRECTION ( 'NONE',  ( 1.000000000000000000, 0.000000000000000000, 0.000000000000000000 ) ) ;
#51729=CARTESIAN_POINT ( 'NONE',  ( 15.23076923076923173, -2.833524468853757305, 32.15551576947925838 ) ) ;
#51730=CARTESIAN_POINT ( 'NONE',  ( 13.38461538461538680, -11.35647404775217417, 33.31231777344666511 ) ) ;
#51731=CARTESIAN_POINT ( 'NONE',  ( -8.769230769230768274, -12.29105614889573062, 35.45975837776705220 ) ) ;
#51732=CARTESIAN_POINT ( 'NONE',  ( -0.2114841499001479108, -11.79725096376909654, 32.30694842903960762 ) ) ;
#51733=ORIENTED_EDGE ( 'NONE', *, *, #45747, .T. ) ;
#51734=CARTESIAN_POINT ( 'NONE',  ( 17.07692307692307665, -1.790695186598648903, 34.54067556320373455 ) ) ;
#51735=FACE_OUTER_BOUND ( 'NONE', #80703, .T. ) ;
#51736=CARTESIAN_POINT ( 'NONE',  ( 7.623227628637697428, -5.667676309546437530, 34.40238873228292249 ) ) ;
#51737=CARTESIAN_POINT ( 'NONE',  ( -12.46153846153846168, -11.16473453929635440, 33.15142922261926373 ) ) ;
#51739=AXIS2_PLACEMENT_3D ( 'NONE', #59972, #32062, #73502 ) ;
#51741=ORIENTED_EDGE ( 'NONE', *, *, #6851, .T. ) ;
#51742=ORIENTED_EDGE ( 'NONE', *, *, #15951, .F. ) ;
#51745=ORIENTED_EDGE ( 'NONE', *, *, #11989, .F. ) ;
#51747=CARTESIAN_POINT ( 'NONE',  ( 17.93472999944367530, -11.67786785259541027, 32.92929555188721480 ) ) ;
#51748=B_SPLINE_CURVE_WITH_KNOTS ( 'NONE', 3,
 ( #24879, #26223, #60889, #10932, #59555, #74409, #66314, #18137, #32525, #80740 ),
 .UNSPECIFIED., .F., .F.,
 ( 4, 2, 2, 2, 4 ),
 ( 0.000000000000000000, 0.0001954339857564054144, 0.0003908679715128108288, 0.0005863019572692162703, 0.0007817359430256216575 ),
 .UNSPECIFIED. ) ;
#51749=CARTESIAN_POINT ( 'NONE',  ( 12.46153846153846168, -13.87047571288749737, 32.06866353760679544 ) ) ;
#51750=CARTESIAN_POINT ( 'NONE',  ( 17.14308968351471663, -7.250054591869668386, 34.99404684341514127 ) ) ;
#51752=B_SPLINE_CURVE_WITH_KNOTS ( 'NONE', 3,
 ( #69357, #66800, #7654, #52832, #39783, #890, #62578, #83316, #11409, #80327 ),
 .UNSPECIFIED., .F., .F.,
 ( 4, 2, 2, 2, 4 ),
 ( 0.000000000000000000, 0.0001954339857564092904, 0.0003908679715128185808, 0.0005863019572692278712, 0.0007817359430256371616 ),
 .UNSPECIFIED. ) ;
#51753=FACE_OUTER_BOUND ( 'NONE', #72735, .T. ) ;
#51754=LINE ( 'NONE', #73389, #28766 ) ;
#51756=DIRECTION ( 'NONE',  ( 0.000000000000000000, 0.4999999999999985567, 0.8660254037844395958 ) ) ;
#51757=LINE ( 'NONE', #60758, #43894 ) ;
#51758=ORIENTED_EDGE ( 'NONE', *, *, #71630, .T. ) ;
#51759=FACE_OUTER_BOUND ( 'NONE', #12901, .T. ) ;
#51760=CARTESIAN_POINT ( 'NONE',  ( -9.942284423250045577, -12.17611988154120972, 31.52148481390971213 ) ) ;
#51761=DIRECTION ( 'NONE',  ( 0.000000000000000000, 0.6427876096865368094, 0.7660444431189802339 ) ) ;
#51763=CARTESIAN_POINT ( 'NONE',  ( -0.3310127597748993566, -11.46989282347013095, 32.79007818306219946 ) ) ;
#51764=CARTESIAN_POINT ( 'NONE',  ( -4.376772371362300795, -9.086856451489516928, 34.49173150075333183 ) ) ;
#51767=ORIENTED_EDGE ( 'NONE', *, *, #19496, .F. ) ;
#51768=CARTESIAN_POINT ( 'NONE',  ( 11.76147289007438701, -11.76359900205217635, 32.36225158514719880 ) ) ;
#51769=CARTESIAN_POINT ( 'NONE',  ( 1.253923917947827205, -5.582088688514999397, 34.36776431015576350 ) ) ;
#51770=CARTESIAN_POINT ( 'NONE',  ( 14.30769230769231015, -1.951392089020283160, 34.73218667398347748 ) ) ;
#51772=AXIS2_PLACEMENT_3D ( 'NONE', #57383, #71785, #70469 ) ;
#51773=CARTESIAN_POINT ( 'NONE',  ( 0.4615384615383382183, -5.941354392335915335, 34.76329471203413846 ) ) ;
#51775=CARTESIAN_POINT ( 'NONE',  ( -14.30769230769242739, -10.90142922262034020, 33.41473453929536674 ) ) ;
#51778=CARTESIAN_POINT ( 'NONE',  ( -1.161602540521989635, -12.38742843783360748, 31.66772728687926985 ) ) ;
#51779=VECTOR ( 'NONE', #53566, 1000.000000000000227 ) ;
#51780=ORIENTED_EDGE ( 'NONE', *, *, #21717, .F. ) ;
#51781=CYLINDRICAL_SURFACE ( 'NONE', #84584, 0.2500000000000008882 ) ;
#51783=CARTESIAN_POINT ( 'NONE',  ( -13.13461538461396394, -7.500000000000154543, 35.00000000000007105 ) ) ;
#51784=CARTESIAN_POINT ( 'NONE',  ( 3.230769230769110045, -10.21337939537710326, 33.94971097300076224 ) ) ;
#51785=CARTESIAN_POINT ( 'NONE',  ( -0.3954711281883860896, -6.343179335718452272, 34.87096338111212646 ) ) ;
#51786=EDGE_LOOP ( 'NONE', ( #35107, #77527, #45396, #70718 ) ) ;
#51787=CARTESIAN_POINT ( 'NONE',  ( -0.5267883933125464546, -2.255955759149247619, 30.00000000000013856 ) ) ;
#51788=VERTEX_POINT ( 'NONE', #28374 ) ;
#51789=LINE ( 'NONE', #31544, #47007 ) ;
#51790=B_SPLINE_CURVE_WITH_KNOTS ( 'NONE', 3,
 ( #37310, #39116, #64778, #30559, #58031, #40451, #53943, #61136, #39568, #87762 ),
 .UNSPECIFIED., .F., .F.,
 ( 4, 2, 2, 2, 4 ),
 ( 0.000000000000000000, 0.0001954311564186872268, 0.0003908623128373744536, 0.0005862934692560616261, 0.0007817246256747489071 ),
 .UNSPECIFIED. ) ;
#51791=EDGE_CURVE ( 'NONE', #19576, #11048, #28905, .T. ) ;
#51792=VERTEX_POINT ( 'NONE', #41452 ) ;
#51793=DIRECTION ( 'NONE',  ( -0.000000000000000000, -0.7660444431189791237, -0.6427876096865379196 ) ) ;
#51794=CARTESIAN_POINT ( 'NONE',  ( 10.61538461538449596, -4.481592998941358097, 33.73612834414048933 ) ) ;
#51795=B_SPLINE_CURVE_WITH_KNOTS ( 'NONE', 3,
 ( #31503, #17998, #85124, #84692, #25191, #38706, #66167, #31956, #67074, #61184 ),
 .UNSPECIFIED., .F., .F.,
 ( 4, 2, 2, 2, 4 ),
 ( 0.0007817359430256390048, 0.0009771253907250078159, 0.001172514838424376735, 0.001367904286123745655, 0.001563293733823114574 ),
 .UNSPECIFIED. ) ;
#51796=ORIENTED_EDGE ( 'NONE', *, *, #81305, .F. ) ;
#51798=LINE ( 'NONE', #72089, #24618 ) ;
#51799=DIRECTION ( 'NONE',  ( 0.000000000000000000, 0.6427876096865373645, -0.7660444431189797898 ) ) ;
#51800=CARTESIAN_POINT ( 'NONE',  ( -3.230769230769229949, -6.189225973068211317, 35.74407628777942847 ) ) ;
#51801=CYLINDRICAL_SURFACE ( 'NONE', #59307, 0.2499999999999973355 ) ;
#51802=CYLINDRICAL_SURFACE ( 'NONE', #57987, 0.2499999999999993616 ) ;
#51804=VERTEX_POINT ( 'NONE', #68915 ) ;
#51805=EDGE_CURVE ( 'NONE', #63541, #17157, #42350, .T. ) ;
#51806=EDGE_LOOP ( 'NONE', ( #29781, #12417, #61696, #65569 ) ) ;
#51807=CARTESIAN_POINT ( 'NONE',  ( -3.903791733932699515, -8.346898887586323923, 34.93166121998716278 ) ) ;
#51808=EDGE_LOOP ( 'NONE', ( #24614, #2286, #84, #77845, #6862, #85928 ) ) ;
#51809=DIRECTION ( 'NONE',  ( -0.000000000000000000, -0.9848077530122086864, -0.1736481776669273613 ) ) ;
#51810=CARTESIAN_POINT ( 'NONE',  ( -10.61538461538461320, -8.973038597847269315, 34.52809138561121927 ) ) ;
#51811=ORIENTED_EDGE ( 'NONE', *, *, #82535, .F. ) ;
#51812=ORIENTED_EDGE ( 'NONE', *, *, #80536, .F. ) ;
#51814=CARTESIAN_POINT ( 'NONE',  ( 16.94677586748485965, -4.460286881179643004, 33.72017969459903242 ) ) ;
#51815=EDGE_LOOP ( 'NONE', ( #78618, #56772, #64719, #39354 ) ) ;
#51816=CARTESIAN_POINT ( 'NONE',  ( 2.372947878968333146, -4.481592998940250538, 33.73612834413965089 ) ) ;
#51817=ADVANCED_FACE ( 'NONE', ( #15314 ), #7227, .F. ) ;
#51818=B_SPLINE_CURVE_WITH_KNOTS ( 'NONE', 3,
 ( #34037, #34918, #1588, #68710, #47547, #75913, #21854, #27281, #20522, #696 ),
 .UNSPECIFIED., .F., .F.,
 ( 4, 2, 2, 2, 4 ),
 ( 0.0007817359527651133143, 0.0009771254036996530456, 0.001172514854634192777, 0.001367904305568732291, 0.001563293756503272023 ),
 .UNSPECIFIED. ) ;
#51819=B_SPLINE_CURVE_WITH_KNOTS ( 'NONE', 3,
 ( #71899, #72341, #24153, #18747, #31821, #45311, #25498, #80453, #73700, #52069 ),
 .UNSPECIFIED., .F., .F.,
 ( 4, 2, 2, 2, 4 ),
 ( 0.000000000000000000, 0.0001954311564186865763, 0.0003908623128373731525, 0.0005862934692560596746, 0.0007817246256747463051 ),
 .UNSPECIFIED. ) ;
#51821=CARTESIAN_POINT ( 'NONE',  ( 17.07692307692307665, -11.16473453929635440, 33.15142922261926373 ) ) ;
#51822=CARTESIAN_POINT ( 'NONE',  ( -11.28840711854808632, -12.01375889529407281, 32.43194544308182969 ) ) ;
#51823=FACE_BOUND ( 'NONE', #45826, .T. ) ;
#51824=B_SPLINE_CURVE_WITH_KNOTS ( 'NONE', 3,
 ( #30281, #84799, #23080, #3682, #86121, #85229, #79806, #23509, #79356, #9558 ),
 .UNSPECIFIED., .F., .F.,
 ( 4, 2, 2, 2, 4 ),
 ( 0.000000000000000000, 0.0001954311564186872268, 0.0003908623128373744536, 0.0005862934692560616261, 0.0007817246256747489071 ),
 .UNSPECIFIED. ) ;
#51825=EDGE_CURVE ( 'NONE', #27494, #85233, #29277, .T. ) ;
#51826=VERTEX_POINT ( 'NONE', #27936 ) ;
#51828=CARTESIAN_POINT ( 'NONE',  ( 12.52679403281448423, -6.026961402152789304, 34.52809138561124769 ) ) ;
#51829=AXIS2_PLACEMENT_3D ( 'NONE', #41908, #53636, #81124 ) ;
#51830=ADVANCED_FACE ( 'NONE', ( #82891 ), #48639, .F. ) ;
#51831=CARTESIAN_POINT ( 'NONE',  ( 7.846153846153846700, -11.11383981884818262, 36.00935417666054406 ) ) ;
#51832=DIRECTION ( 'NONE',  ( -0.000000000000000000, 0.9848077530122085754, -0.1736481776669273613 ) ) ;
#51833=CYLINDRICAL_SURFACE ( 'NONE', #53387, 0.2500000000000004996 ) ;
#51835=CARTESIAN_POINT ( 'NONE',  ( -17.30040802064702987, -12.44517049084099725, 30.48991314939691932 ) ) ;
#51836=ORIENTED_EDGE ( 'NONE', *, *, #42077, .T. ) ;
#51838=EDGE_LOOP ( 'NONE', ( #58176, #79926, #18140, #45930, #8949, #85664 ) ) ;
#51839=VECTOR ( 'NONE', #14206, 1000.000000000000000 ) ;
#51840=CARTESIAN_POINT ( 'NONE',  ( 5.869852030268307708, -12.15440758774515473, 32.17923288041532004 ) ) ;
#51841=LINE ( 'NONE', #43770, #3071 ) ;
#51842=DIRECTION ( 'NONE',  ( -0.000000000000000000, -0.7660444431189791237, -0.6427876096865379196 ) ) ;
#51843=CARTESIAN_POINT ( 'NONE',  ( -13.60754234352223335, -2.889293201056495786, 32.26117774369186009 ) ) ;
#51844=CARTESIAN_POINT ( 'NONE',  ( 1.515141086378947621, -10.19071101563364756, 33.96452234770658407 ) ) ;
#51845=CARTESIAN_POINT ( 'NONE',  ( 14.05766908347085220, -2.985938066672154445, 32.43141759479405550 ) ) ;
#51846=VERTEX_POINT ( 'NONE', #16622 ) ;
#51847=CARTESIAN_POINT ( 'NONE',  ( 6.923076923076924238, -2.486705287966279876, 31.30864560766543647 ) ) ;
#51848=CARTESIAN_POINT ( 'NONE',  ( -0.3954711281883869778, -3.322132147404560865, 32.92929555188719348 ) ) ;
#51849=CARTESIAN_POINT ( 'NONE',  ( -1.608100328339333807, -3.754499324213721234, 33.06261337010820256 ) ) ;
#51850=DIRECTION ( 'NONE',  ( 0.000000000000000000, 0.7660444431189822323, -0.6427876096865344779 ) ) ;
#51851=ORIENTED_EDGE ( 'NONE', *, *, #34392, .F. ) ;
#51852=ORIENTED_EDGE ( 'NONE', *, *, #19517, .F. ) ;
#51853=FACE_BOUND ( 'NONE', #59015, .T. ) ;
#51856=CARTESIAN_POINT ( 'NONE',  ( -13.38461538461550759, -2.379036618888197729, 30.90682066428292885 ) ) ;
#51857=CARTESIAN_POINT ( 'NONE',  ( -14.30769230769242739, -11.48612834414049644, 32.76840700105863391 ) ) ;
#51858=ORIENTED_EDGE ( 'NONE', *, *, #32932, .F. ) ;
#51859=DIRECTION ( 'NONE',  ( 0.000000000000000000, 0.000000000000000000, 1.000000000000000000 ) ) ;
#51860=CARTESIAN_POINT ( 'NONE',  ( 6.673053685783957967, -10.76384336483936011, 33.53834819971076087 ) ) ;
#51861=CARTESIAN_POINT ( 'NONE',  ( -8.703162418228330921, -6.386643153685127139, 34.62446782046654192 ) ) ;
#51862=FACE_OUTER_BOUND ( 'NONE', #11497, .T. ) ;
#51863=B_SPLINE_CURVE_WITH_KNOTS ( 'NONE', 3,
 ( #23011, #17596, #18483, #30648, #64869, #80184 ),
 .UNSPECIFIED., .F., .F.,
 ( 4, 2, 4 ),
 ( 4.220987180333913997E-17, 0.0001954756301637137399, 0.0003909512603273853043 ),
 .UNSPECIFIED. ) ;
#51864=LINE ( 'NONE', #4131, #41747 ) ;
#51865=EDGE_LOOP ( 'NONE', ( #67114, #39987, #49656, #56255, #30341, #3666, #36950, #81606, #25947, #62467, #34987, #81507, #27506, #56263, #14061, #73962, #19803, #40786, #58174, #15089, #39018, #53288, #64582, #9169, #58350, #27166, #54527, #53757, #37844, #4843, #53634, #43200, #45219, #32644, #2743, #74226, #24139, #10746, #75928, #52779, #64883, #41164, #56923, #9261, #7331, #47538, #71693, #2431, #86682, #7092, #25014, #58739, #57951, #45820, #33286, #42924, #53652, #352, #60233, #14787, #36490, #15617, #7854, #26226, #15079, #77960, #29562, #79206, #23347, #52179, #74778, #48535, #10642, #23402, #78860, #68288, #53135, #18679, #26266, #25751, #8397, #76325, #18385, #24334, #37344, #20569, #88182, #74956, #39435, #27995, #33127, #70652, #66164, #33788, #60012, #12988, #444, #8398, #63515, #49412, #85143, #34989, #56681, #45081, #55899, #82105, #80727, #74651, #43834, #12362, #54966, #73073, #87080, #45983, #42158, #24564, #9517, #43539, #27185, #20366, #87982, #87662, #52596, #54371 ) ) ;
#51866=CARTESIAN_POINT ( 'NONE',  ( 23.00000000000000000, -5.499999999999982236, 27.75000000000000000 ) ) ;
#51867=VERTEX_POINT ( 'NONE', #38235 ) ;
#51868=DIRECTION ( 'NONE',  ( -0.000000000000000000, 0.5000000000000011102, -0.8660254037844380415 ) ) ;
#51869=CARTESIAN_POINT ( 'NONE',  ( 15.00784227186237807, -4.762599654559228846, 34.23009711892697737 ) ) ;
#51870=CARTESIAN_POINT ( 'NONE',  ( -3.230769230769229949, -8.564572088678739092, 35.78748833219616898 ) ) ;
#51871=EDGE_CURVE ( 'NONE', #30893, #59397, #68600, .T. ) ;
#51872=CARTESIAN_POINT ( 'NONE',  ( -10.83831157429146330, -3.395401636524185474, 33.02366814457250399 ) ) ;
#51873=DIRECTION ( 'NONE',  ( 0.000000000000000000, -6.938893903907222067E-15, 1.000000000000000000 ) ) ;
#51874=CARTESIAN_POINT ( 'NONE',  ( 12.23861150263161335, -5.582147617184174848, 34.63737895849758530 ) ) ;
#51877=ORIENTED_EDGE ( 'NONE', *, *, #61408, .F. ) ;
#51878=LINE ( 'NONE', #18123, #37312 ) ;
#51879=CARTESIAN_POINT ( 'NONE',  ( 2.557746727605761272, -4.074993327901525575, 33.72946981652012255 ) ) ;
#51881=VERTEX_POINT ( 'NONE', #31021 ) ;
#51882=ORIENTED_EDGE ( 'NONE', *, *, #61888, .T. ) ;
#51883=CARTESIAN_POINT ( 'NONE',  ( -5.999999999999998224, -12.62096338111211580, 30.90682066428153263 ) ) ;
#51884=CARTESIAN_POINT ( 'NONE',  ( -14.08467946359890988, -2.523321265292115534, 31.42251411153756990 ) ) ;
#51885=CYLINDRICAL_SURFACE ( 'NONE', #41841, 0.2500000000000009437 ) ;
#51886=ADVANCED_FACE ( 'NONE', ( #70696 ), #17527, .F. ) ;
#51887=DIRECTION ( 'NONE',  ( -0.000000000000000000, -0.9848077530122085754, -0.1736481776669273613 ) ) ;
#51888=DIRECTION ( 'NONE',  ( 1.000000000000000000, 0.000000000000000000, 0.000000000000000000 ) ) ;
#51890=CARTESIAN_POINT ( 'NONE',  ( 5.869852790561781219, -8.587444163452046197, 34.63053765926554206 ) ) ;
#51891=ORIENTED_EDGE ( 'NONE', *, *, #20514, .F. ) ;
#51892=DIRECTION ( 'NONE',  ( -0.000000000000000000, -0.3420201433256694346, -0.9396926207859080948 ) ) ;
#51893=CARTESIAN_POINT ( 'NONE',  ( -17.14300648787895653, -12.10708131394839349, 31.69288490824020244 ) ) ;
#51894=VECTOR ( 'NONE', #72241, 1000.000000000000000 ) ;
#51895=CARTESIAN_POINT ( 'NONE',  ( -3.230769230769229949, -9.058645607665452459, 34.76329471203371924 ) ) ;
#51897=CARTESIAN_POINT ( 'NONE',  ( 17.07692307692307665, -8.973038597847269315, 34.52809138561121927 ) ) ;
#51899=CARTESIAN_POINT ( 'NONE',  ( 13.60762673622823726, -6.503523203565941380, 34.64991518177335195 ) ) ;
#51902=VECTOR ( 'NONE', #33273, 999.9999999999998863 ) ;
#51903=ADVANCED_FACE ( 'NONE', ( #22943 ), #17073, .F. ) ;
#51904=ORIENTED_EDGE ( 'NONE', *, *, #49505, .F. ) ;
#51905=CARTESIAN_POINT ( 'NONE',  ( 12.46153846153846168, -9.058645607665452459, 34.76329471203371924 ) ) ;
#51906=CARTESIAN_POINT ( 'NONE',  ( 10.48523664565292179, -3.625366637846545892, 33.29286588640298561 ) ) ;
#51907=CARTESIAN_POINT ( 'NONE',  ( 17.74997677577853850, -10.18141759479407327, 34.26406193332782379 ) ) ;
#51908=ORIENTED_EDGE ( 'NONE', *, *, #28640, .T. ) ;
#51909=EDGE_CURVE ( 'NONE', #17639, #8057, #48173, .T. ) ;
#51910=CARTESIAN_POINT ( 'NONE',  ( -11.53846153846153655, -2.292212530054420494, 30.41441678777542634 ) ) ;
#51911=CARTESIAN_POINT ( 'NONE',  ( 12.59206389977210705, -11.04252011169590020, 33.62494198852677130 ) ) ;
#51912=CARTESIAN_POINT ( 'NONE',  ( -39.05038313613820122, -2.499999999999999556, 29.75000000000000355 ) ) ;
#51914=DIRECTION ( 'NONE',  ( -0.000000000000000000, -0.9396926207859093161, -0.3420201433256663259 ) ) ;
#51915=CARTESIAN_POINT ( 'NONE',  ( -2.980714919130914797, -12.41262288849542017, 30.68299917996395010 ) ) ;
#51916=B_SPLINE_CURVE_WITH_KNOTS ( 'NONE', 3,
 ( #71685, #38357, #11325, #38806, #66718, #66266, #4570, #87014, #25286, #52748 ),
 .UNSPECIFIED., .F., .F.,
 ( 4, 2, 2, 2, 4 ),
 ( 0.000000000000000000, 0.0001954339857564074202, 0.0003908679715128148403, 0.0005863019572692222334, 0.0007817359430256296806 ),
 .UNSPECIFIED. ) ;
#51918=EDGE_CURVE ( 'NONE', #18937, #5324, #13725, .T. ) ;
#51919=CARTESIAN_POINT ( 'NONE',  ( 16.37685899793954292, -10.01129605718032423, 34.36064277460058491 ) ) ;
#51920=ORIENTED_EDGE ( 'NONE', *, *, #3481, .T. ) ;
#51921=CARTESIAN_POINT ( 'NONE',  ( -11.53846153846153655, -3.937682226553329556, 33.60647404775216529 ) ) ;
#51922=CARTESIAN_POINT ( 'NONE',  ( -10.36538461538460965, -2.499999999999999556, 29.81604066197449754 ) ) ;
#51923=ADVANCED_FACE ( 'NONE', ( #9871 ), #58485, .F. ) ;
#51924=CARTESIAN_POINT ( 'NONE',  ( -0.4615384615385840772, -2.657715359629662544, 31.77849191805970364 ) ) ;
#51925=CARTESIAN_POINT ( 'NONE',  ( 9.757562831820530747, -2.657715359629132301, 31.77849191805844242 ) ) ;
#51926=EDGE_CURVE ( 'NONE', #57710, #5662, #81540, .T. ) ;
#51927=DIRECTION ( 'NONE',  ( -0.000000000000000000, -0.8660254037844397068, -0.4999999999999978906 ) ) ;
#51928=CARTESIAN_POINT ( 'NONE',  ( 15.23076923076923173, -11.69971097300155272, 32.46337939537588113 ) ) ;
#51930=ORIENTED_EDGE ( 'NONE', *, *, #79510, .F. ) ;
#51931=ORIENTED_EDGE ( 'NONE', *, *, #27866, .T. ) ;
#51932=ORIENTED_EDGE ( 'NONE', *, *, #75105, .F. ) ;
#51933=ORIENTED_EDGE ( 'NONE', *, *, #71141, .F. ) ;
#51934=ADVANCED_FACE ( 'NONE', ( #37334 ), #23380, .F. ) ;
#51935=CARTESIAN_POINT ( 'NONE',  ( -12.68440472460156521, -2.251424796025575326, 29.88072029997477586 ) ) ;
#51937=AXIS2_PLACEMENT_3D ( 'NONE', #61304, #54553, #13578 ) ;
#51938=CARTESIAN_POINT ( 'NONE',  ( -10.54931728203453822, -4.661471528628508665, 34.16647553114624003 ) ) ;
#51939=CARTESIAN_POINT ( 'NONE',  ( -5.869208192175213945, -4.809403383903225304, 33.96459661697924304 ) ) ;
#51940=CARTESIAN_POINT ( 'NONE',  ( -13.38461538461538325, -3.322132147404559976, 32.92929555188717927 ) ) ;
#51941=CARTESIAN_POINT ( 'NONE',  ( -12.71151520558705350, -12.41104346484419452, 31.60698883733904196 ) ) ;
#51942=EDGE_CURVE ( 'NONE', #20277, #12856, #32078, .T. ) ;
#51943=LINE ( 'NONE', #23591, #66701 ) ;
#51944=EDGE_CURVE ( 'NONE', #56137, #43657, #58860, .T. ) ;
#51945=CARTESIAN_POINT ( 'NONE',  ( 17.07692307692339284, -2.255955759149395501, 30.00000000000324363 ) ) ;
#51948=ORIENTED_EDGE ( 'NONE', *, *, #29946, .F. ) ;
#51949=ORIENTED_EDGE ( 'NONE', *, *, #61708, .T. ) ;
#51950=CARTESIAN_POINT ( 'NONE',  ( 0.2380535369741276219, -3.019605429927184836, 32.48692288466676814 ) ) ;
#51951=VERTEX_POINT ( 'NONE', #53518 ) ;
#51952=CARTESIAN_POINT ( 'NONE',  ( 7.716006636715626144, -3.285722584762969856, 32.44110544564090759 ) ) ;
#51953=DIRECTION ( 'NONE',  ( -0.000000000000000000, -0.1736481776669307198, -0.9848077530122080203 ) ) ;
#51954=CARTESIAN_POINT ( 'NONE',  ( -1.254570328695612247, -2.254550872974306674, 29.97347326024527447 ) ) ;
#51955=LINE ( 'NONE', #17751, #72435 ) ;
#51956=FACE_BOUND ( 'NONE', #44634, .T. ) ;
#51957=EDGE_LOOP ( 'NONE', ( #69043, #63573 ) ) ;
#51958=AXIS2_PLACEMENT_3D ( 'NONE', #45685, #4710, #12792 ) ;
#51959=ORIENTED_EDGE ( 'NONE', *, *, #68209, .F. ) ;
#51961=ORIENTED_EDGE ( 'NONE', *, *, #42519, .T. ) ;
#51962=FACE_BOUND ( 'NONE', #62931, .T. ) ;
#51963=CARTESIAN_POINT ( 'NONE',  ( 13.63456079399342791, -12.45601412856602686, 31.48342859153981621 ) ) ;
#51964=AXIS2_PLACEMENT_3D ( 'NONE', #5006, #24819, #66250 ) ;
#51965=DIRECTION ( 'NONE',  ( 0.000000000000000000, 0.8660254037844377084, -0.5000000000000015543 ) ) ;
#51966=ORIENTED_EDGE ( 'NONE', *, *, #60778, .T. ) ;
#51967=CARTESIAN_POINT ( 'NONE',  ( 14.30769230769218758, -2.892918686052165622, 31.69288490824153470 ) ) ;
#51969=CYLINDRICAL_SURFACE ( 'NONE', #40745, 0.2500000000000009437 ) ;
#51970=ORIENTED_EDGE ( 'NONE', *, *, #88306, .T. ) ;
#51971=CARTESIAN_POINT ( 'NONE',  ( 12.46153846153833911, -5.219633306517616589, 34.19971097300220464 ) ) ;
#51972=CARTESIAN_POINT ( 'NONE',  ( 16.15384615384603251, -11.94971097300221174, 32.03036669348237098 ) ) ;
#51973=VERTEX_POINT ( 'NONE', #24722 ) ;
#51975=CARTESIAN_POINT ( 'NONE',  ( 5.750000000000003553, -7.433932668274256805, 35.00000000000000711 ) ) ;
#51978=DIRECTION ( 'NONE',  ( -0.000000000000000000, -0.000000000000000000, -1.000000000000000000 ) ) ;
#51979=CARTESIAN_POINT ( 'NONE',  ( 13.25392391794783009, -2.541943142973491554, 30.39792223712631980 ) ) ;
#51980=DIRECTION ( 'NONE',  ( -0.000000000000000000, -0.6427876096865404731, -0.7660444431189770143 ) ) ;
#51981=CARTESIAN_POINT ( 'NONE',  ( 15.23076923076923173, -12.62096338111211580, 30.90682066428153263 ) ) ;
#51982=CARTESIAN_POINT ( 'NONE',  ( 9.626225312947559232, -12.34228464037088280, 31.77849191805838558 ) ) ;
#51984=CARTESIAN_POINT ( 'NONE',  ( -16.15384615384615330, -12.09954503811598769, 35.62045528018868623 ) ) ;
#51985=CARTESIAN_POINT ( 'NONE',  ( -1.634592115557736092, -2.779195860258146134, 31.39871582349836032 ) ) ;
#51986=CARTESIAN_POINT ( 'NONE',  ( -0.4615384615384611200, -11.69971097300155272, 32.46337939537588113 ) ) ;
#51987=CARTESIAN_POINT ( 'NONE',  ( -0.4615384615385840772, -8.656820664282941280, 34.87096338111179961 ) ) ;
#51988=CARTESIAN_POINT ( 'NONE',  ( -5.076923076923197442, -9.442884908241554243, 34.35708131394783038 ) ) ;
#51989=CARTESIAN_POINT ( 'NONE',  ( -10.74553182482283198, -8.587444163452046197, 34.63053765926554206 ) ) ;
#51990=EDGE_CURVE ( 'NONE', #10982, #25678, #20274, .T. ) ;
#51992=VERTEX_POINT ( 'NONE', #26505 ) ;
#51994=CARTESIAN_POINT ( 'NONE',  ( 0.4615384615383396616, -12.46129190930018460, 30.37095296980731973 ) ) ;
#51995=ORIENTED_EDGE ( 'NONE', *, *, #44715, .T. ) ;
#51996=EDGE_CURVE ( 'NONE', #39467, #8676, #33266, .T. ) ;
#51997=ORIENTED_EDGE ( 'NONE', *, *, #3523, .F. ) ;
#51998=CARTESIAN_POINT ( 'NONE',  ( -2.057746789344164107, -12.43552623307873972, 30.55307653245132826 ) ) ;
#51999=ORIENTED_EDGE ( 'NONE', *, *, #69804, .F. ) ;
#52000=CARTESIAN_POINT ( 'NONE',  ( -15.16551365949320740, -6.026961402152789304, 34.52809138561124769 ) ) ;
#52002=CARTESIAN_POINT ( 'NONE',  ( 2.980792486720640344, -2.318417181685854533, 30.59732222474233865 ) ) ;
#52003=CARTESIAN_POINT ( 'NONE',  ( 5.777073782483853392, -11.24512374952581872, 33.06303171183252942 ) ) ;
#52005=CARTESIAN_POINT ( 'NONE',  ( -12.46153846153858424, -4.320704448113951379, 33.92786785259630022 ) ) ;
#52006=EDGE_CURVE ( 'NONE', #64208, #38006, #27762, .T. ) ;
#52007=CARTESIAN_POINT ( 'NONE',  ( -10.36533019547116474, -3.435999193479609914, 33.07426656108010832 ) ) ;
#52009=FACE_OUTER_BOUND ( 'NONE', #47059, .T. ) ;
#52012=B_SPLINE_CURVE_WITH_KNOTS ( 'NONE', 3,
 ( #23567, #21802, #84403, #51016, #71748, #57357, #78510, #70439, #29896, #16809 ),
 .UNSPECIFIED., .F., .F.,
 ( 4, 2, 2, 2, 4 ),
 ( 0.0007817246256747434861, 0.0009771112852218859484, 0.001172497944769028411, 0.001367884604316171090, 0.001563271263863313552 ),
 .UNSPECIFIED. ) ;
#52014=DIRECTION ( 'NONE',  ( 0.000000000000000000, 0.1736481776669275834, 0.9848077530122086864 ) ) ;
#52015=B_SPLINE_CURVE_WITH_KNOTS ( 'NONE', 3,
 ( #70209, #62550, #35989, #63444, #863, #14832, #48598, #41413, #7181, #14375 ),
 .UNSPECIFIED., .F., .F.,
 ( 4, 2, 2, 2, 4 ),
 ( 0.0007817246256747491240, 0.0009771112852218931041, 0.001172497944769036867, 0.001367884604316180631, 0.001563271263863324611 ),
 .UNSPECIFIED. ) ;
#52016=VECTOR ( 'NONE', #42177, 1000.000000000000000 ) ;
#52017=CARTESIAN_POINT ( 'NONE',  ( 14.30769230769231015, -13.37000171582298513, 34.34916445242398453 ) ) ;
#52018=B_SPLINE_CURVE_WITH_KNOTS ( 'NONE', 3,
 ( #81456, #4904, #53964, #18854, #67932, #32368, #60721, #4442, #31928, #87332 ),
 .UNSPECIFIED., .F., .F.,
 ( 4, 2, 2, 2, 4 ),
 ( 0.000000000000000000, 0.0001954311564186865492, 0.0003908623128373730983, 0.0005862934692560596746, 0.0007817246256747461966 ),
 .UNSPECIFIED. ) ;
#52019=EDGE_LOOP ( 'NONE', ( #27804, #4222 ) ) ;
#52020=EDGE_LOOP ( 'NONE', ( #78280, #1607, #19466, #85208 ) ) ;
#52021=DIRECTION ( 'NONE',  ( 0.000000000000000000, 0.000000000000000000, 1.000000000000000000 ) ) ;
#52022=LINE ( 'NONE', #38073, #84862 ) ;
#52024=CARTESIAN_POINT ( 'NONE',  ( -15.93106661257773915, -12.44528174975671853, 30.48912976160715615 ) ) ;
#52025=EDGE_CURVE ( 'NONE', #64833, #26559, #80419, .T. ) ;
#52026=CARTESIAN_POINT ( 'NONE',  ( 17.14217821643591932, -12.51329471203373345, 31.30864560766537963 ) ) ;
#52027=PLANE ( 'NONE',  #32758 ) ;
#52028=EDGE_CURVE ( 'NONE', #8235, #18795, #15210, .T. ) ;
#52029=EDGE_LOOP ( 'NONE', ( #24814, #79930 ) ) ;
#52030=CARTESIAN_POINT ( 'NONE',  ( -10.83826413212219641, -7.630690623152299956, 34.99857592706774057 ) ) ;
#52031=VERTEX_POINT ( 'NONE', #47659 ) ;
#52033=CARTESIAN_POINT ( 'NONE',  ( -5.869474298236436738, -6.001044277235011215, 34.52024696741798948 ) ) ;
#52034=AXIS2_PLACEMENT_3D ( 'NONE', #29787, #8187, #62666 ) ;
#52035=FACE_OUTER_BOUND ( 'NONE', #21274, .T. ) ;
#52036=CARTESIAN_POINT ( 'NONE',  ( -10.61538461538461320, -4.102666532097928531, 36.13435417666054406 ) ) ;
#52037=CARTESIAN_POINT ( 'NONE',  ( 1.254467414883689846, -11.66186481527757479, 32.95055677023626117 ) ) ;
#52038=CARTESIAN_POINT ( 'NONE',  ( -2.176900499867520100, -11.71459661697925903, 32.44059661609676937 ) ) ;
#52039=AXIS2_PLACEMENT_3D ( 'NONE', #3720, #85266, #1958 ) ;
#52040=VERTEX_POINT ( 'NONE', #20624 ) ;
#52041=ORIENTED_EDGE ( 'NONE', *, *, #10683, .F. ) ;
#52042=B_SPLINE_CURVE_WITH_KNOTS ( 'NONE', 3,
 ( #30574, #85974, #31013, #52173, #22936, #84657, #65245, #79219, #11201, #44077 ),
 .UNSPECIFIED., .F., .F.,
 ( 4, 2, 2, 2, 4 ),
 ( 0.0007817359430256317406, 0.0009771253907249982749, 0.001172514838424365026, 0.001367904286123731560, 0.001563293733823098094 ),
 .UNSPECIFIED. ) ;
#52044=EDGE_CURVE ( 'NONE', #34465, #6050, #35257, .T. ) ;
#52045=EDGE_CURVE ( 'NONE', #77968, #79258, #14853, .T. ) ;
#52046=CARTESIAN_POINT ( 'NONE',  ( -3.930833309752757909, -11.98016756924215009, 32.48728574198911190 ) ) ;
#52047=CARTESIAN_POINT ( 'NONE',  ( 15.23076923076911093, -11.48612834414049644, 32.76840700105863391 ) ) ;
#52049=EDGE_CURVE ( 'NONE', #5606, #51992, #30934, .T. ) ;
#52050=CARTESIAN_POINT ( 'NONE',  ( -8.703163435880695076, -9.905515769479276145, 34.41647553114623292 ) ) ;
#52051=CARTESIAN_POINT ( 'NONE',  ( 11.53846153846153832, -10.67929555188718282, 33.92786785259544047 ) ) ;
#52052=EDGE_CURVE ( 'NONE', #79032, #75182, #54859, .T. ) ;
#52053=CARTESIAN_POINT ( 'NONE',  ( 6.000000000000001776, -12.37446782046654192, 30.86335684631486131 ) ) ;
#52054=VERTEX_POINT ( 'NONE', #88672 ) ;
#52055=EDGE_LOOP ( 'NONE', ( #54039, #3531 ) ) ;
#52057=VERTEX_POINT ( 'NONE', #41800 ) ;
#52058=CARTESIAN_POINT ( 'NONE',  ( 2.438218009455871638, -12.45806712695776319, 30.39783852428763922 ) ) ;
#52059=ORIENTED_EDGE ( 'NONE', *, *, #33145, .T. ) ;
#52060=ADVANCED_FACE ( 'NONE', ( #34140 ), #40907, .F. ) ;
#52061=CARTESIAN_POINT ( 'NONE',  ( 1.134638653673032849, -9.943427161483782584, 34.11278801902876978 ) ) ;
#52063=AXIS2_PLACEMENT_3D ( 'NONE', #56316, #77034, #84248 ) ;
#52065=ORIENTED_EDGE ( 'NONE', *, *, #39642, .F. ) ;
#52067=DIRECTION ( 'NONE',  ( 0.000000000000000000, 0.1736481776669267785, -0.9848077530122087975 ) ) ;
#52068=VERTEX_POINT ( 'NONE', #61608 ) ;
#52069=CARTESIAN_POINT ( 'NONE',  ( -13.38461538461550759, -11.67786785259630911, 32.92929555188603530 ) ) ;
#52071=FACE_BOUND ( 'NONE', #69372, .T. ) ;
#52072=CARTESIAN_POINT ( 'NONE',  ( 5.750000000000002665, -7.500000000000001776, 34.75000000000000000 ) ) ;
#52074=DIRECTION ( 'NONE',  ( -0.000000000000000000, 0.3420201433256694346, -0.9396926207859080948 ) ) ;
#52075=CYLINDRICAL_SURFACE ( 'NONE', #33348, 0.2500000000000002220 ) ;
#52076=ORIENTED_EDGE ( 'NONE', *, *, #87224, .F. ) ;
#52077=ADVANCED_FACE ( 'NONE', ( #76012 ), #75565, .F. ) ;
#52078=CARTESIAN_POINT ( 'NONE',  ( 11.47319153790521717, -11.67786785259540849, 32.92929555188721480 ) ) ;
#52079=CARTESIAN_POINT ( 'NONE',  ( 8.899756470994335089, -6.852161475712352789, 34.70806712695775786 ) ) ;
#52082=CARTESIAN_POINT ( 'NONE',  ( -18.00000000000000000, -12.62096338111211580, 30.90682066428153263 ) ) ;
#52084=CARTESIAN_POINT ( 'NONE',  ( 14.30769230769218581, -10.33852847137269571, 34.16647553114546554 ) ) ;
#52085=B_SPLINE_CURVE_WITH_KNOTS ( 'NONE', 3,
 ( #67746, #59648, #60538, #6051, #39838, #60981, #80835, #88484, #39402, #52885 ),
 .UNSPECIFIED., .F., .F.,
 ( 4, 2, 2, 2, 4 ),
 ( 0.000000000000000000, 0.0001954311564186871184, 0.0003908623128373742367, 0.0005862934692560614093, 0.0007817246256747484735 ),
 .UNSPECIFIED. ) ;
#52086=DIRECTION ( 'NONE',  ( 0.000000000000000000, 0.1736481776669267785, -0.9848077530122087975 ) ) ;
#52088=EDGE_CURVE ( 'NONE', #59241, #24770, #71613, .T. ) ;
#52089=FACE_BOUND ( 'NONE', #971, .T. ) ;
#52090=CARTESIAN_POINT ( 'NONE',  ( 13.16113044089143891, -12.24155766932282496, 31.33739205006857986 ) ) ;
#52091=CARTESIAN_POINT ( 'NONE',  ( 4.403900573759605308, -12.65882529074907126, 30.72640787790839312 ) ) ;
#52093=CARTESIAN_POINT ( 'NONE',  ( 18.06606835100243913, -11.16473453929635440, 33.15142922261926373 ) ) ;
#52094=CARTESIAN_POINT ( 'NONE',  ( 9.915087233576098669, -4.387253974876679230, 33.66317474335728832 ) ) ;
#52095=LINE ( 'NONE', #10678, #75723 ) ;
#52096=DIRECTION ( 'NONE',  ( -0.000000000000000000, 0.3420201433256694346, -0.9396926207859080948 ) ) ;
#52098=EDGE_CURVE ( 'NONE', #5312, #11434, #78167, .T. ) ;
#52100=CIRCLE ( 'NONE', #83755, 0.2500000000000002220 ) ;
#52101=CARTESIAN_POINT ( 'NONE',  ( 12.46153846153846168, -2.708943851104267164, 35.45975837776705220 ) ) ;
#52102=CARTESIAN_POINT ( 'NONE',  ( -14.98076923076929567, -7.565270445406050648, 34.75000000000000000 ) ) ;
#52104=CARTESIAN_POINT ( 'NONE',  ( 6.000000000000001776, -12.10708131394839349, 31.69288490824020244 ) ) ;
#52106=CARTESIAN_POINT ( 'NONE',  ( 5.326977496836529546, -12.01375889529407281, 32.43194544308182969 ) ) ;
#52108=CARTESIAN_POINT ( 'NONE',  ( -15.48079245499068612, -12.68155406624981119, 30.59749803192733708 ) ) ;
#52110=EDGE_CURVE ( 'NONE', #84431, #51157, #40539, .T. ) ;
#52112=CARTESIAN_POINT ( 'NONE',  ( 5.207448515156722912, -12.70449254468099198, 30.44128974285582956 ) ) ;
#52113=DIRECTION ( 'NONE',  ( -0.000000000000000000, 0.7660444431189791237, -0.6427876096865379196 ) ) ;
#52114=DIRECTION ( 'NONE',  ( -0.000000000000000000, 0.8660254037844399289, -0.4999999999999980016 ) ) ;
#52115=DIRECTION ( 'NONE',  ( 0.000000000000000000, 0.000000000000000000, 1.000000000000000000 ) ) ;
#52116=EDGE_CURVE ( 'NONE', #33268, #74563, #50736, .T. ) ;
#52117=CARTESIAN_POINT ( 'NONE',  ( -1.319360245102545681, -12.16647553114626490, 32.15551576947920864 ) ) ;
#52118=ORIENTED_EDGE ( 'NONE', *, *, #46698, .T. ) ;
#52119=CARTESIAN_POINT ( 'NONE',  ( 17.07692307692295586, -12.70778746994576025, 30.41441678777401236 ) ) ;
#52120=DIRECTION ( 'NONE',  ( 0.000000000000000000, 0.3420201433256610524, 0.9396926207859113145 ) ) ;
#52122=CARTESIAN_POINT ( 'NONE',  ( 2.241608896736428047, -4.098570777380720287, 33.41473453929634729 ) ) ;
#52123=CARTESIAN_POINT ( 'NONE',  ( -5.076923076923075762, -2.538708090699994813, 30.37095296980875503 ) ) ;
#52124=ORIENTED_EDGE ( 'NONE', *, *, #87743, .T. ) ;
#52125=CARTESIAN_POINT ( 'NONE',  ( -6.673022503163469565, -10.06805714834173848, 34.32951233291982618 ) ) ;
#52128=VERTEX_POINT ( 'NONE', #37231 ) ;
#52129=CYLINDRICAL_SURFACE ( 'NONE', #21157, 0.2500000000000009437 ) ;
#52130=CYLINDRICAL_SURFACE ( 'NONE', #42621, 0.2500000000000009437 ) ;
#52132=LINE ( 'NONE', #3054, #30562 ) ;
#52134=EDGE_CURVE ( 'NONE', #373, #60933, #67328, .T. ) ;
#52135=VERTEX_POINT ( 'NONE', #84117 ) ;
#52137=DIRECTION ( 'NONE',  ( 0.000000000000000000, 0.9396926207859126468, 0.3420201433256571111 ) ) ;
#52138=CARTESIAN_POINT ( 'NONE',  ( -12.71156168575992318, -2.588893531581426988, 31.60682220781847818 ) ) ;
#52140=EDGE_LOOP ( 'NONE', ( #24404, #56067 ) ) ;
#52141=ORIENTED_EDGE ( 'NONE', *, *, #8657, .T. ) ;
#52142=ORIENTED_EDGE ( 'NONE', *, *, #67104, .T. ) ;
#52143=CARTESIAN_POINT ( 'NONE',  ( 3.480714640147274608, -2.341251567377310217, 30.72681386836322659 ) ) ;
#52145=CARTESIAN_POINT ( 'NONE',  ( -7.846153846153844924, -2.538708090699994813, 30.37095296980875503 ) ) ;
#52146=CARTESIAN_POINT ( 'NONE',  ( -17.20707028636129721, -6.852621066184266141, 34.70813303252209181 ) ) ;
#52147=ORIENTED_EDGE ( 'NONE', *, *, #50572, .T. ) ;
#52148=EDGE_LOOP ( 'NONE', ( #69927, #85071, #67850, #60217, #17585, #65519 ) ) ;
#52149=CARTESIAN_POINT ( 'NONE',  ( 4.219913487196229163, -5.471508081941601098, 34.59228464037088457 ) ) ;
#52151=CARTESIAN_POINT ( 'NONE',  ( -5.076923076923199218, -2.657715359629662988, 31.77849191805970364 ) ) ;
#52154=CARTESIAN_POINT ( 'NONE',  ( 2.557746619330623528, -3.627508038966689163, 32.91356715214248396 ) ) ;
#52155=CARTESIAN_POINT ( 'NONE',  ( 13.51540582558233794, -9.929761469519743144, 34.40412654351204225 ) ) ;
#52156=ADVANCED_FACE ( 'NONE', ( #23712 ), #22398, .F. ) ;
#52157=ORIENTED_EDGE ( 'NONE', *, *, #22436, .F. ) ;
#52158=AXIS2_PLACEMENT_3D ( 'NONE', #4630, #53250, #19910 ) ;
#52159=ORIENTED_EDGE ( 'NONE', *, *, #38982, .T. ) ;
#52160=ORIENTED_EDGE ( 'NONE', *, *, #81885, .T. ) ;
#52161=CARTESIAN_POINT ( 'NONE',  ( 5.076923076923075762, -4.786620604624113540, 33.94971097300155094 ) ) ;
#52162=VERTEX_POINT ( 'NONE', #44419 ) ;
#52163=ADVANCED_FACE ( 'NONE', ( #49863 ), #15650, .F. ) ;
#52164=CARTESIAN_POINT ( 'NONE',  ( 18.13052543823364360, -12.15418822224088657, 32.17964115625579069 ) ) ;
#52165=CARTESIAN_POINT ( 'NONE',  ( -0.2114840416250083899, -4.818054556918156983, 34.26375889529406749 ) ) ;
#52166=ORIENTED_EDGE ( 'NONE', *, *, #41106, .F. ) ;
#52167=CARTESIAN_POINT ( 'NONE',  ( -8.992715712954719720, -10.81261337010820256, 33.49550067578627477 ) ) ;
#52168=FACE_OUTER_BOUND ( 'NONE', #29401, .T. ) ;
#52169=ADVANCED_FACE ( 'NONE', ( #63825 ), #3449, .F. ) ;
#52170=CARTESIAN_POINT ( 'NONE',  ( -16.82692307692164135, -7.500000000000155431, 34.75000000000007105 ) ) ;
#52171=FACE_BOUND ( 'NONE', #60917, .T. ) ;
#52172=CARTESIAN_POINT ( 'NONE',  ( -8.638440328263820689, -2.295524264805589354, 30.44142389570982488 ) ) ;
#52173=CARTESIAN_POINT ( 'NONE',  ( 2.530471848960717640, -8.496831190052096971, 34.64984203495476578 ) ) ;
#52174=CARTESIAN_POINT ( 'NONE',  ( 11.66925334628632882, -12.38066358083363738, 30.83685684665853444 ) ) ;
#52175=DIRECTION ( 'NONE',  ( 0.000000000000000000, 0.8660254037844377084, -0.5000000000000015543 ) ) ;
#52176=CARTESIAN_POINT ( 'NONE',  ( -8.519176349317314489, -12.01375889529407281, 32.43194544308182969 ) ) ;
#52177=CARTESIAN_POINT ( 'NONE',  ( 13.38461538461538680, -4.098570777380720287, 33.41473453929634729 ) ) ;
#52178=CARTESIAN_POINT ( 'NONE',  ( 5.076923076923075762, -2.538708090699994813, 30.37095296980875503 ) ) ;
#52179=ORIENTED_EDGE ( 'NONE', *, *, #18714, .F. ) ;
#52180=CARTESIAN_POINT ( 'NONE',  ( -15.00798956179116317, -11.60474049983371003, 33.02348890104160262 ) ) ;
#52181=CARTESIAN_POINT ( 'NONE',  ( -7.715362038329061534, -2.541949514083464479, 30.39797389878540557 ) ) ;
#52182=EDGE_LOOP ( 'NONE', ( #9754, #10322 ) ) ;
#52184=CARTESIAN_POINT ( 'NONE',  ( -11.66915214157184444, -12.62707690430377383, 30.88035979386743435 ) ) ;
#52185=CARTESIAN_POINT ( 'NONE',  ( 10.68145194873469173, -11.91647553114624358, 32.58852847137148245 ) ) ;
#52186=EDGE_CURVE ( 'NONE', #6380, #15876, #84560, .T. ) ;
#52187=VECTOR ( 'NONE', #17810, 1000.000000000000227 ) ;
#52189=CARTESIAN_POINT ( 'NONE',  ( 16.15384615384603251, -2.625532179533778709, 30.86335684631627174 ) ) ;
#52190=CARTESIAN_POINT ( 'NONE',  ( 10.61538461538449418, -3.083524468854526912, 32.58852847137268327 ) ) ;
#52191=CARTESIAN_POINT ( 'NONE',  ( -15.45359592324823517, -7.369208160676171460, 34.74850200257122879 ) ) ;
#52193=CARTESIAN_POINT ( 'NONE',  ( 8.703148389870632329, -12.62096338111211580, 30.90682066428152908 ) ) ;
#52194=CARTESIAN_POINT ( 'NONE',  ( 18.13079044096696180, -3.957578996910245284, 33.62503395064540257 ) ) ;
#52195=CARTESIAN_POINT ( 'NONE',  ( 11.78851595837499211, -2.920487667080175598, 32.31805714834170828 ) ) ;
#52196=CARTESIAN_POINT ( 'NONE',  ( 0.2380535369741288987, -12.69144148231606017, 30.53333754910549303 ) ) ;
#52197=CARTESIAN_POINT ( 'NONE',  ( 17.14299142792551578, -6.386643153685127139, 34.62446782046654192 ) ) ;
#52198=CARTESIAN_POINT ( 'NONE',  ( 17.99999999999987566, -6.879047030192662504, 34.71129190930017927 ) ) ;
#52199=( NAMED_UNIT ( * ) PLANE_ANGLE_UNIT ( ) SI_UNIT ( $, .RADIAN. ) );
#52200=CARTESIAN_POINT ( 'NONE',  ( -15.10024379253558635, -11.04252011169590020, 33.62494198852677130 ) ) ;
#52203=EDGE_CURVE ( 'NONE', #22124, #58240, #84554, .T. ) ;
#52204=ORIENTED_EDGE ( 'NONE', *, *, #10835, .F. ) ;
#52205=CARTESIAN_POINT ( 'NONE',  ( -14.37296230824862775, -5.094484230520674117, 34.41647553114621161 ) ) ;
#52207=CARTESIAN_POINT ( 'NONE',  ( -17.74999999999856115, -7.500000000000155431, 34.75000000000007105 ) ) ;
#52208=CARTESIAN_POINT ( 'NONE',  ( -12.39547011053602432, -9.780366693483667717, 34.19971097300155805 ) ) ;
#52209=CARTESIAN_POINT ( 'NONE',  ( 14.43821800945586986, -2.882268652242222284, 31.66798894389554064 ) ) ;
#52210=CARTESIAN_POINT ( 'NONE',  ( 17.01116964860974079, -7.249945578846654470, 34.99404164642496795 ) ) ;
#52212=CARTESIAN_POINT ( 'NONE',  ( -6.923076923077045919, -3.083524468854526912, 32.58852847137268327 ) ) ;
#52214=CARTESIAN_POINT ( 'NONE',  ( -13.31844624365272800, -7.250054483168843156, 34.74374881642865631 ) ) ;
#52215=CARTESIAN_POINT ( 'NONE',  ( 5.776515075435672664, -10.23692288466677880, 34.23039457007281072 ) ) ;
#52216=CARTESIAN_POINT ( 'NONE',  ( 2.980746006547774218, -12.45566812827425096, 31.48439005359158926 ) ) ;
#52217=B_SPLINE_CURVE_WITH_KNOTS ( 'NONE', 3,
 ( #21240, #54580, #41976, #82077, #22139, #33873, #8185, #68988, #93, #68547 ),
 .UNSPECIFIED., .F., .F.,
 ( 4, 2, 2, 2, 4 ),
 ( 0.000000000000000000, 0.0001954339857564075557, 0.0003908679715128151114, 0.0005863019572692226671, 0.0007817359430256302227 ),
 .UNSPECIFIED. ) ;
#52218=CARTESIAN_POINT ( 'NONE',  ( 14.05766907039934210, -12.22074536777954989, 31.39888409691088356 ) ) ;
#52219=DIRECTION ( 'NONE',  ( -0.000000000000000000, -0.3420201433256694901, -0.9396926207859080948 ) ) ;
#52220=CARTESIAN_POINT ( 'NONE',  ( 6.988332062589762472, -2.379036618887895305, 30.90682066428159303 ) ) ;
#52221=CARTESIAN_POINT ( 'NONE',  ( -0.3954701105360237667, -11.16473453929635440, 33.15142922261926373 ) ) ;
#52222=EDGE_CURVE ( 'NONE', #87108, #42300, #65226, .T. ) ;
#52223=CARTESIAN_POINT ( 'NONE',  ( -3.007757879156381708, -11.24521262558773671, 33.06293181088029343 ) ) ;
#52224=CARTESIAN_POINT ( 'NONE',  ( -7.715362038329059757, -12.38066358083363738, 30.83685684665853444 ) ) ;
#52225=ORIENTED_EDGE ( 'NONE', *, *, #17477, .F. ) ;
#52226=CYLINDRICAL_SURFACE ( 'NONE', #34127, 0.2500000000000002220 ) ;
#52227=CARTESIAN_POINT ( 'NONE',  ( -13.13466997523734037, -10.18230066228895758, 34.26354781536631577 ) ) ;
#52230=AXIS2_PLACEMENT_3D ( 'NONE', #42367, #63051, #33928 ) ;
#52231=AXIS2_PLACEMENT_3D ( 'NONE', #74223, #12519, #67468 ) ;
#52232=CARTESIAN_POINT ( 'NONE',  ( -18.13056059174191148, -2.504760397472873379, 29.97295953869786800 ) ) ;
#52233=CARTESIAN_POINT ( 'NONE',  ( 11.53846153846153832, -11.69971097300155272, 32.46337939537588113 ) ) ;
#52234=CARTESIAN_POINT ( 'NONE',  ( -0.3954701105360219349, -2.538708090699994813, 30.37095296980875503 ) ) ;
#52235=ORIENTED_EDGE ( 'NONE', *, *, #43114, .F. ) ;
#52239=AXIS2_PLACEMENT_3D ( 'NONE', #16378, #38430, #10059 ) ;
#52240=ORIENTED_EDGE ( 'NONE', *, *, #73615, .F. ) ;
#52241=CARTESIAN_POINT ( 'NONE',  ( -4.377331078410483300, -8.539481045369598178, 34.89627647299170832 ) ) ;
#52242=ORIENTED_EDGE ( 'NONE', *, *, #64148, .F. ) ;
#52243=CARTESIAN_POINT ( 'NONE',  ( 3.007284306204899504, -4.988325925672468131, 34.36044203135681130 ) ) ;
#52244=ADVANCED_FACE ( 'NONE', ( #11102 ), #4343, .F. ) ;
#52245=EDGE_CURVE ( 'NONE', #8848, #75979, #66034, .T. ) ;
#52246=CARTESIAN_POINT ( 'NONE',  ( -1.384615384615506484, -12.16647553114689728, 32.15551576947799362 ) ) ;
#52248=ORIENTED_EDGE ( 'NONE', *, *, #34838, .T. ) ;
#52249=CARTESIAN_POINT ( 'NONE',  ( 11.31553457955469000, -11.98009711892699514, 32.48740034544076138 ) ) ;
#52250=ORIENTED_EDGE ( 'NONE', *, *, #86412, .T. ) ;
#52251=CYLINDRICAL_SURFACE ( 'NONE', #61462, 0.2499999999999997502 ) ;
#52252=EDGE_CURVE ( 'NONE', #69985, #78986, #31906, .T. ) ;
#52253=EDGE_CURVE ( 'NONE', #19260, #46007, #12434, .T. ) ;
#52254=ORIENTED_EDGE ( 'NONE', *, *, #10857, .T. ) ;
#52255=DIRECTION ( 'NONE',  ( -0.000000000000000000, -0.6427876096865404731, -0.7660444431189771253 ) ) ;
#52256=CYLINDRICAL_SURFACE ( 'NONE', #88740, 0.2499999999999986955 ) ;
#52257=ORIENTED_EDGE ( 'NONE', *, *, #76324, .T. ) ;
#52258=B_SPLINE_CURVE_WITH_KNOTS ( 'NONE', 3,
 ( #69605, #35831, #7911, #89016, #63287, #47995, #75474, #13772, #29084, #56538 ),
 .UNSPECIFIED., .F., .F.,
 ( 4, 2, 2, 2, 4 ),
 ( 0.000000000000000000, 0.0001954311564186858715, 0.0003908623128373717431, 0.0005862934692560576146, 0.0007817246256747434861 ),
 .UNSPECIFIED. ) ;
#52259=B_SPLINE_CURVE_WITH_KNOTS ( 'NONE', 3,
 ( #5523, #64426, #29780, #56362, #36101, #57248, #35201, #8181, #42855, #70318 ),
 .UNSPECIFIED., .F., .F.,
 ( 4, 2, 2, 2, 4 ),
 ( 0.000000000000000000, 0.0001954339881912772715, 0.0003908679763825545429, 0.0005863019645738318415, 0.0007817359527651090859 ),
 .UNSPECIFIED. ) ;
#52260=CARTESIAN_POINT ( 'NONE',  ( 10.61538461538461675, -12.78798330534102945, 29.74999999999997868 ) ) ;
#52261=DIRECTION ( 'NONE',  ( -0.000000000000000000, 1.000000000000000000, 3.491481338843133355E-15 ) ) ;
#52262=CARTESIAN_POINT ( 'NONE',  ( 11.53846153846141753, -11.94971097300221174, 32.03036669348237098 ) ) ;
#52267=ORIENTED_EDGE ( 'NONE', *, *, #6305, .T. ) ;
#52268=ORIENTED_EDGE ( 'NONE', *, *, #9713, .F. ) ;
#52269=ORIENTED_EDGE ( 'NONE', *, *, #27663, .T. ) ;
#52270=CARTESIAN_POINT ( 'NONE',  ( 3.230769230769231726, -12.62096338111211580, 30.90682066428153263 ) ) ;
#52271=ORIENTED_EDGE ( 'NONE', *, *, #10358, .F. ) ;
#52272=DIRECTION ( 'NONE',  ( 0.000000000000000000, 0.6427876096865373645, -0.7660444431189797898 ) ) ;
#52273=CARTESIAN_POINT ( 'NONE',  ( 1.515141086378948732, -2.882268652242222728, 31.66798894389554064 ) ) ;
#52274=ORIENTED_EDGE ( 'NONE', *, *, #10849, .F. ) ;
#52275=ORIENTED_EDGE ( 'NONE', *, *, #47479, .T. ) ;
#52276=CARTESIAN_POINT ( 'NONE',  ( 3.296837581771669523, -4.786620604624113540, 33.94971097300155805 ) ) ;
#52277=ORIENTED_EDGE ( 'NONE', *, *, #86764, .T. ) ;
#52278=CARTESIAN_POINT ( 'NONE',  ( -12.71153846153846168, -7.566082377512564960, 35.00000000000000711 ) ) ;
#52279=AXIS2_PLACEMENT_3D ( 'NONE', #33234, #67021, #66111 ) ;
#52280=B_SPLINE_CURVE_WITH_KNOTS ( 'NONE', 3,
 ( #53714, #47840, #27131, #34325, #82537, #33884, #60472, #20813, #68999, #48282 ),
 .UNSPECIFIED., .F., .F.,
 ( 4, 2, 2, 2, 4 ),
 ( 0.0007817246256747486903, 0.0009771112852218918031, 0.001172497944769034699, 0.001367884604316177595, 0.001563271263863320708 ),
 .UNSPECIFIED. ) ;
#52282=B_SPLINE_CURVE_WITH_KNOTS ( 'NONE', 3,
 ( #46991, #21634, #15333, #70268, #74931, #8576, #49556, #33049, #26288, #53756 ),
 .UNSPECIFIED., .F., .F.,
 ( 4, 2, 2, 2, 4 ),
 ( 0.000000000000000000, 0.0001954311564186862781, 0.0003908623128373725562, 0.0005862934692560588072, 0.0007817246256747451124 ),
 .UNSPECIFIED. ) ;
#52283=CARTESIAN_POINT ( 'NONE',  ( 0.4615384615383396616, -5.219633306517616589, 34.19971097300220464 ) ) ;
#52284=FACE_BOUND ( 'NONE', #58518, .T. ) ;
#52286=CARTESIAN_POINT ( 'NONE',  ( -6.065270445960775803, -6.026961402152685388, 34.52809138561120506 ) ) ;
#52287=FACE_OUTER_BOUND ( 'NONE', #15009, .T. ) ;
#52288=VECTOR ( 'NONE', #31921, 1000.000000000000000 ) ;
#52289=CARTESIAN_POINT ( 'NONE',  ( -0.4615384615384611200, -1.422936976036506707, 30.56769352161908415 ) ) ;
#52290=CARTESIAN_POINT ( 'NONE',  ( 2.177544337960613863, -8.630895178749536711, 34.87696386517710323 ) ) ;
#52291=LINE ( 'NONE', #30690, #47677 ) ;
#52292=VERTEX_POINT ( 'NONE', #45772 ) ;
#52293=CARTESIAN_POINT ( 'NONE',  ( -17.29984929443922681, -12.39988816332205701, 30.74660775122750778 ) ) ;
#52295=EDGE_LOOP ( 'NONE', ( #41674, #32006 ) ) ;
#52296=CARTESIAN_POINT ( 'NONE',  ( -7.173053667125515176, -4.075325502946086864, 33.72974371597207721 ) ) ;
#52297=CARTESIAN_POINT ( 'NONE',  ( 10.68064018666063930, -6.026961402152789304, 34.52809138561124769 ) ) ;
#52298=CYLINDRICAL_SURFACE ( 'NONE', #67267, 0.2499999999999995559 ) ;
#52301=CARTESIAN_POINT ( 'NONE',  ( 1.607628228708781748, -4.026326845037962343, 33.68677907613344047 ) ) ;
#52302=VERTEX_POINT ( 'NONE', #11552 ) ;
#52304=CARTESIAN_POINT ( 'NONE',  ( 3.164686851409095336, -9.058645607665454236, 34.76329471203372634 ) ) ;
#52305=CARTESIAN_POINT ( 'NONE',  ( 2.530705151785704210, -12.64618726649961289, 30.78989965857442712 ) ) ;
#52306=CARTESIAN_POINT ( 'NONE',  ( -4.153846153846273204, -3.835265460704628371, 33.15142922262033665 ) ) ;
#52307=ORIENTED_EDGE ( 'NONE', *, *, #3092, .F. ) ;
#52308=VERTEX_POINT ( 'NONE', #32697 ) ;
#52309=ADVANCED_FACE ( 'NONE', ( #67380 ), #87671, .F. ) ;
#52312=FACE_OUTER_BOUND ( 'NONE', #23845, .T. ) ;
#52313=CARTESIAN_POINT ( 'NONE',  ( -1.318548051265307386, -2.292212530054420494, 30.41441678777542990 ) ) ;
#52314=VERTEX_POINT ( 'NONE', #88125 ) ;
#52315=DIRECTION ( 'NONE',  ( -0.000000000000000000, 1.000000000000000000, -0.000000000000000000 ) ) ;
#52316=CARTESIAN_POINT ( 'NONE',  ( 6.066067333350078528, -11.35647404775217595, 33.31231777344667222 ) ) ;
#52317=CARTESIAN_POINT ( 'NONE',  ( -7.846153846153965716, -11.94971097300221174, 32.03036669348237098 ) ) ;
#52318=CARTESIAN_POINT ( 'NONE',  ( 4.284636594813103549, -6.369690395747422684, 34.87708834333098196 ) ) ;
#52319=CARTESIAN_POINT ( 'NONE',  ( -7.596153846153844924, -2.499999999999998668, 29.75000000000000355 ) ) ;
#52320=AXIS2_PLACEMENT_3D ( 'NONE', #68921, #2227, #42799 ) ;
#52321=ORIENTED_EDGE ( 'NONE', *, *, #75688, .F. ) ;
#52322=CARTESIAN_POINT ( 'NONE',  ( -7.715628144390285215, -10.19071101563364756, 33.96452234770658407 ) ) ;
#52323=VERTEX_POINT ( 'NONE', #26396 ) ;
#52324=CARTESIAN_POINT ( 'NONE',  ( -7.623142494540994463, -9.086983370893049639, 34.49168942202179267 ) ) ;
#52325=CARTESIAN_POINT ( 'NONE',  ( -12.71151520558705528, -2.920706130388546651, 32.31842814019191223 ) ) ;
#52326=CARTESIAN_POINT ( 'NONE',  ( -2.307692307692305711, -1.951392089020283160, 34.73218667398347748 ) ) ;
#52328=CARTESIAN_POINT ( 'NONE',  ( -5.999999999999998224, -13.75783147151868846, 33.36296068462461051 ) ) ;
#52329=EDGE_CURVE ( 'NONE', #28930, #10260, #53861, .T. ) ;
#52330=CARTESIAN_POINT ( 'NONE',  ( 6.249945518348143381, -2.824170634883622188, 31.52227843825338738 ) ) ;
#52333=CARTESIAN_POINT ( 'NONE',  ( -3.361460697436790657, -3.062553014421049991, 32.05460306192774311 ) ) ;
#52334=CARTESIAN_POINT ( 'NONE',  ( 8.096153846155266010, -7.500000000000154543, 35.00000000000007105 ) ) ;
#52335=DIRECTION ( 'NONE',  ( -0.000000000000000000, 0.3420201433256694346, -0.9396926207859080948 ) ) ;
#52336=ORIENTED_EDGE ( 'NONE', *, *, #24694, .T. ) ;
#52337=ORIENTED_EDGE ( 'NONE', *, *, #82879, .T. ) ;
#52338=CARTESIAN_POINT ( 'NONE',  ( -8.769230769230892619, -5.941354392335915335, 34.76329471203413846 ) ) ;
#52339=CARTESIAN_POINT ( 'NONE',  ( -7.780898706641007578, -5.941354392334607049, 34.76329471203374055 ) ) ;
#52340=CARTESIAN_POINT ( 'NONE',  ( 13.38461538461538680, -3.513871655860378418, 32.76840700105978499 ) ) ;
#52343=CARTESIAN_POINT ( 'NONE',  ( 5.750023269057646935, -8.303909089506435137, 34.68538101551103381 ) ) ;
#52344=VERTEX_POINT ( 'NONE', #54741 ) ;
#52345=DIRECTION ( 'NONE',  ( 0.000000000000000000, -6.938893903907222067E-15, 1.000000000000000000 ) ) ;
#52346=ADVANCED_FACE ( 'NONE', ( #33598 ), #83570, .F. ) ;
#52348=VECTOR ( 'NONE', #30018, 1000.000000000000227 ) ;
#52349=CARTESIAN_POINT ( 'NONE',  ( 7.173022332454967120, -6.653508905675592722, 34.93172785388651391 ) ) ;
#52350=CARTESIAN_POINT ( 'NONE',  ( 3.903822929624696236, -8.475808217655753651, 34.90892951860618609 ) ) ;
#52352=CARTESIAN_POINT ( 'NONE',  ( 12.59206416330202671, -3.816742781228458448, 33.13167719472716044 ) ) ;
#52354=AXIS2_PLACEMENT_3D ( 'NONE', #76901, #15204, #83218 ) ;
#52356=EDGE_CURVE ( 'NONE', #327, #25620, #41681, .T. ) ;
#52357=CARTESIAN_POINT ( 'NONE',  ( 9.692307692307695177, -6.435427911321262684, 35.78748833219616898 ) ) ;
#52358=FACE_OUTER_BOUND ( 'NONE', #11742, .T. ) ;
#52360=VERTEX_POINT ( 'NONE', #55184 ) ;
#52361=EDGE_CURVE ( 'NONE', #74826, #31771, #82680, .T. ) ;
#52362=LINE ( 'NONE', #45611, #41872 ) ;
#52364=FACE_OUTER_BOUND ( 'NONE', #44146, .T. ) ;
#52365=CARTESIAN_POINT ( 'NONE',  ( -6.250023224221455287, -5.765609946408404518, 34.70566812827425451 ) ) ;
#52366=CARTESIAN_POINT ( 'NONE',  ( -2.307692307692428724, -11.06231777344772027, 33.60647404775119895 ) ) ;
#52367=ORIENTED_EDGE ( 'NONE', *, *, #10777, .F. ) ;
#52368=DIRECTION ( 'NONE',  ( -0.000000000000000000, 1.000000000000000000, 3.491481338843133355E-15 ) ) ;
#52369=ORIENTED_EDGE ( 'NONE', *, *, #70270, .T. ) ;
#52371=CARTESIAN_POINT ( 'NONE',  ( -10.48533945254983557, -2.504778602574660340, 29.97347330155780654 ) ) ;
#52373=CARTESIAN_POINT ( 'NONE',  ( 7.623226887246994821, -12.38737895849757820, 31.66785238281580206 ) ) ;
#52374=DIRECTION ( 'NONE',  ( -0.000000000000000000, -0.7660444431189791237, -0.6427876096865379196 ) ) ;
#52375=CARTESIAN_POINT ( 'NONE',  ( 12.46153846153833911, -10.21337939537710326, 33.94971097300076224 ) ) ;
#52376=ORIENTED_EDGE ( 'NONE', *, *, #45480, .T. ) ;
#52377=B_SPLINE_CURVE_WITH_KNOTS ( 'NONE', 3,
 ( #33111, #41202, #33993, #75866, #215, #60576, #53822, #12837, #67786, #33565 ),
 .UNSPECIFIED., .F., .F.,
 ( 4, 2, 2, 2, 4 ),
 ( 0.000000000000000000, 0.0001954339857564072033, 0.0003908679715128144066, 0.0005863019572692215828, 0.0007817359430256288133 ),
 .UNSPECIFIED. ) ;
#52379=EDGE_LOOP ( 'NONE', ( #3605, #61717 ) ) ;
#52380=VERTEX_POINT ( 'NONE', #20079 ) ;
#52381=EDGE_LOOP ( 'NONE', ( #75246, #54193, #76265, #54112 ) ) ;
#52382=VERTEX_POINT ( 'NONE', #34475 ) ;
#52383=CYLINDRICAL_SURFACE ( 'NONE', #44451, 0.2499999999999973355 ) ;
#52384=DIRECTION ( 'NONE',  ( 0.000000000000000000, 0.4999999999999960032, -0.8660254037844410391 ) ) ;
#52385=CARTESIAN_POINT ( 'NONE',  ( 14.98074599347626368, -5.056417327199099532, 34.11270091957321426 ) ) ;
#52386=CARTESIAN_POINT ( 'NONE',  ( -7.173100160369890510, -3.202444869320336451, 32.30641848906366675 ) ) ;
#52387=CARTESIAN_POINT ( 'NONE',  ( 7.596130621932389637, -12.68155406624981119, 30.59749803192733708 ) ) ;
#52389=CYLINDRICAL_SURFACE ( 'NONE', #10515, 0.2499999999999994726 ) ;
#52390=CARTESIAN_POINT ( 'NONE',  ( -17.74994568836168440, -6.567000820036036579, 34.66262288849541306 ) ) ;
#52391=DIRECTION ( 'NONE',  ( -0.000000000000000000, -0.3420201433256694346, -0.9396926207859080948 ) ) ;
#52392=ORIENTED_EDGE ( 'NONE', *, *, #76293, .T. ) ;
#52394=EDGE_CURVE ( 'NONE', #82761, #19526, #60928, .T. ) ;
#52395=EDGE_LOOP ( 'NONE', ( #4971, #43056, #87384, #27071 ) ) ;
#52396=CARTESIAN_POINT ( 'NONE',  ( 0.4615384615383382183, -12.16647553114689728, 32.15551576947799362 ) ) ;
#52397=VERTEX_POINT ( 'NONE', #75461 ) ;
#52398=CARTESIAN_POINT ( 'NONE',  ( 7.623227628637696540, -3.105860786376062332, 32.13614157043599562 ) ) ;
#52399=CARTESIAN_POINT ( 'NONE',  ( -16.28399336328437386, -10.19110544564092002, 33.96427741523702792 ) ) ;
#52400=CARTESIAN_POINT ( 'NONE',  ( -1.515305987725692471, -4.684245665217972032, 34.18127051446801090 ) ) ;
#52401=CARTESIAN_POINT ( 'NONE',  ( -1.384615384615383471, -2.517432740324522911, 35.29906147534542527 ) ) ;
#52402=FACE_BOUND ( 'NONE', #10868, .T. ) ;
#52403=ORIENTED_EDGE ( 'NONE', *, *, #29640, .F. ) ;
#52404=AXIS2_PLACEMENT_3D ( 'NONE', #86547, #85203, #71671 ) ;
#52405=B_SPLINE_CURVE_WITH_KNOTS ( 'NONE', 3,
 ( #52366, #79855, #45615, #73093, #38873, #4636, #34319, #27122, #26678, #46938 ),
 .UNSPECIFIED., .F., .F.,
 ( 4, 2, 2, 2, 4 ),
 ( 0.0007817246256747459798, 0.0009771112852218887673, 0.001172497944769031663, 0.001367884604316174559, 0.001563271263863317455 ),
 .UNSPECIFIED. ) ;
#52406=ORIENTED_EDGE ( 'NONE', *, *, #16955, .F. ) ;
#52407=CARTESIAN_POINT ( 'NONE',  ( -2.557669038634660552, -12.41269422305637171, 30.68257228309993323 ) ) ;
#52408=AXIS2_PLACEMENT_3D ( 'NONE', #75214, #19819, #55367 ) ;
#52410=FACE_BOUND ( 'NONE', #29884, .T. ) ;
#52411=CARTESIAN_POINT ( 'NONE',  ( 9.692307692307695177, -2.538708090699994813, 30.37095296980875503 ) ) ;
#52412=EDGE_CURVE ( 'NONE', #85101, #53248, #13319, .T. ) ;
#52413=B_SPLINE_CURVE_WITH_KNOTS ( 'NONE', 3,
 ( #36413, #48579, #63870, #84609, #35074, #62532 ),
 .UNSPECIFIED., .F., .F.,
 ( 4, 2, 4 ),
 ( 0.000000000000000000, 0.0001954784845028914076, 0.0003909569690057828153 ),
 .UNSPECIFIED. ) ;
#52414=CARTESIAN_POINT ( 'NONE',  ( 15.23076923076923173, -6.343179335718451384, 34.87096338111211935 ) ) ;
#52416=CARTESIAN_POINT ( 'NONE',  ( 2.057715576749954423, -8.303909089506435137, 34.68538101551103381 ) ) ;
#52417=CARTESIAN_POINT ( 'NONE',  ( -6.857009589726846599, -2.292212530054420494, 30.41441678777542990 ) ) ;
#52418=DIRECTION ( 'NONE',  ( -0.000000000000000000, -0.6427876096865404731, -0.7660444431189770143 ) ) ;
#52419=VERTEX_POINT ( 'NONE', #67824 ) ;
#52420=B_SPLINE_CURVE_WITH_KNOTS ( 'NONE', 3,
 ( #29239, #76530, #56692, #69766, #84187, #868, #70656, #68877, #14382, #20696 ),
 .UNSPECIFIED., .F., .F.,
 ( 4, 2, 2, 2, 4 ),
 ( 0.000000000000000000, 0.0001954311564186879044, 0.0003908623128373758088, 0.0005862934692560636861, 0.0007817246256747516176 ),
 .UNSPECIFIED. ) ;
#52421=EDGE_CURVE ( 'NONE', #53195, #40406, #5105, .T. ) ;
#52422=CARTESIAN_POINT ( 'NONE',  ( 18.22342639891478910, -7.630147987733843173, 34.99859428049665411 ) ) ;
#52423=CARTESIAN_POINT ( 'NONE',  ( -18.00000000000000000, -8.973038597847269315, 34.52809138561121927 ) ) ;
#52424=VERTEX_POINT ( 'NONE', #74584 ) ;
#52425=CARTESIAN_POINT ( 'NONE',  ( -2.372962753653081069, -11.48612834413959582, 32.76840700105983473 ) ) ;
#52426=LINE ( 'NONE', #17316, #71433 ) ;
#52427=ORIENTED_EDGE ( 'NONE', *, *, #84375, .T. ) ;
#52428=FACE_OUTER_BOUND ( 'NONE', #85879, .T. ) ;
#52429=DIRECTION ( 'NONE',  ( -0.000000000000000000, -0.6427876096865404731, -0.7660444431189770143 ) ) ;
#52430=DIRECTION ( 'NONE',  ( 0.000000000000000000, 0.7660444431189822323, -0.6427876096865344779 ) ) ;
#52431=DIRECTION ( 'NONE',  ( -0.000000000000000000, 0.9848077530122086864, -0.1736481776669273891 ) ) ;
#52432=DIRECTION ( 'NONE',  ( 0.000000000000000000, 0.3420201433256641055, -0.9396926207859100932 ) ) ;
#52433=CARTESIAN_POINT ( 'NONE',  ( -20.99999999999999645, -4.249999999999998224, 29.75000000000000355 ) ) ;
#52434=CARTESIAN_POINT ( 'NONE',  ( -13.63459212866397507, -4.075325502946081535, 33.72974371597206300 ) ) ;
#52435=CYLINDRICAL_SURFACE ( 'NONE', #18702, 0.2499999999999995559 ) ;
#52437=CARTESIAN_POINT ( 'NONE',  ( 8.992242120843618736, -12.15243808032445827, 31.58219941686247978 ) ) ;
#52438=CARTESIAN_POINT ( 'NONE',  ( -9.692307692307691624, -13.04860791097971706, 34.73218667398347037 ) ) ;
#52439=CARTESIAN_POINT ( 'NONE',  ( 12.39545608217832395, -4.661471528628507777, 34.16647553114621871 ) ) ;
#52441=ORIENTED_EDGE ( 'NONE', *, *, #49762, .T. ) ;
#52442=CARTESIAN_POINT ( 'NONE',  ( -9.692307692307691624, -8.164416787775445883, 34.95778746994557906 ) ) ;
#52443=ORIENTED_EDGE ( 'NONE', *, *, #80319, .F. ) ;
#52444=EDGE_CURVE ( 'NONE', #20922, #88377, #48004, .T. ) ;
#52445=ORIENTED_EDGE ( 'NONE', *, *, #77944, .F. ) ;
#52446=CARTESIAN_POINT ( 'NONE',  ( 13.13461538461538680, -2.249999999999998668, 29.75000000000000355 ) ) ;
#52447=ORIENTED_EDGE ( 'NONE', *, *, #43858, .T. ) ;
#52448=DIRECTION ( 'NONE',  ( 1.000000000000000000, 0.000000000000000000, 0.000000000000000000 ) ) ;
#52450=CARTESIAN_POINT ( 'NONE',  ( -17.77722045873159473, -5.913360116392396115, 34.49180327182771322 ) ) ;
#52451=CARTESIAN_POINT ( 'NONE',  ( -8.769230769230890843, -3.300289026999228881, 32.46337939537708905 ) ) ;
#52452=CARTESIAN_POINT ( 'NONE',  ( -7.623374304885435215, -5.913360116392397892, 34.49180327182771322 ) ) ;
#52453=FACE_OUTER_BOUND ( 'NONE', #52967, .T. ) ;
#52454=VECTOR ( 'NONE', #13346, 1000.000000000000000 ) ;
#52455=CARTESIAN_POINT ( 'NONE',  ( -5.207613680033387205, -3.338472653186242756, 32.95098750199972670 ) ) ;
#52459=CARTESIAN_POINT ( 'NONE',  ( 17.32697749683652688, -2.318338780012835443, 30.59689888758630616 ) ) ;
#52460=CARTESIAN_POINT ( 'NONE',  ( -14.55769230769230660, -2.499999999999998668, 29.75000000000000355 ) ) ;
#52461=ADVANCED_FACE ( 'NONE', ( #62815 ), #56077, .F. ) ;
#52462=B_SPLINE_CURVE_WITH_KNOTS ( 'NONE', 3,
 ( #13253, #19561, #75397, #5609, #61426, #48356, #82162, #27647, #180, #33532 ),
 .UNSPECIFIED., .F., .F.,
 ( 4, 2, 2, 2, 4 ),
 ( 0.0007817359430256253438, 0.0009771253907249898181, 0.001172514838424354401, 0.001367904286123718983, 0.001563293733823083566 ),
 .UNSPECIFIED. ) ;
#52464=B_SPLINE_CURVE_WITH_KNOTS ( 'NONE', 3,
 ( #88126, #33149, #33599, #74138, #89003, #53862, #26397, #61058, #54294, #34913 ),
 .UNSPECIFIED., .F., .F.,
 ( 4, 2, 2, 2, 4 ),
 ( 0.0007817359430256392216, 0.0009771253907250080327, 0.001172514838424376952, 0.001367904286123745872, 0.001563293733823114791 ),
 .UNSPECIFIED. ) ;
#52465=CARTESIAN_POINT ( 'NONE',  ( 5.999999999999878320, -3.643525952248796163, 33.31231777344771672 ) ) ;
#52466=ORIENTED_EDGE ( 'NONE', *, *, #45638, .F. ) ;
#52468=EDGE_CURVE ( 'NONE', #84116, #6052, #60477, .T. ) ;
#52469=CARTESIAN_POINT ( 'NONE',  ( 14.24160992833217421, -8.164416787775445883, 34.95778746994557906 ) ) ;
#52470=CARTESIAN_POINT ( 'NONE',  ( 7.846153846153725020, -11.48612834414049644, 32.76840700105863391 ) ) ;
#52471=CARTESIAN_POINT ( 'NONE',  ( 1.254467414883688292, -11.04286588640298561, 33.62463336215343901 ) ) ;
#52472=CARTESIAN_POINT ( 'NONE',  ( -6.923076923077045919, -5.941354392335915335, 34.76329471203413846 ) ) ;
#52473=EDGE_CURVE ( 'NONE', #39792, #21373, #2845, .T. ) ;
#52474=CARTESIAN_POINT ( 'NONE',  ( 8.519254038288416098, -11.79746400365624659, 32.30657167506340954 ) ) ;
#52475=DIRECTION ( 'NONE',  ( 0.000000000000000000, 0.9396926207859126468, 0.3420201433256571111 ) ) ;
#52476=AXIS2_PLACEMENT_3D ( 'NONE', #62270, #52074, #55079 ) ;
#52477=ORIENTED_EDGE ( 'NONE', *, *, #68083, .F. ) ;
#52478=CARTESIAN_POINT ( 'NONE',  ( 17.93472955403921887, -12.46129190929999986, 30.37095296980880832 ) ) ;
#52480=ORIENTED_EDGE ( 'NONE', *, *, #83880, .F. ) ;
#52481=CYLINDRICAL_SURFACE ( 'NONE', #30637, 0.2500000000000004996 ) ;
#52482=AXIS2_PLACEMENT_3D ( 'NONE', #70722, #61730, #70276 ) ;
#52483=CARTESIAN_POINT ( 'NONE',  ( 6.130838418012763746, -7.277220443632450575, 34.74524770363009196 ) ) ;
#52484=LINE ( 'NONE', #58797, #27169 ) ;
#52485=CIRCLE ( 'NONE', #63990, 0.2500000000000002220 ) ;
#52486=CARTESIAN_POINT ( 'NONE',  ( 11.53846153846153832, -2.292212530054420494, 30.41441678777542634 ) ) ;
#52487=CARTESIAN_POINT ( 'NONE',  ( -5.326946301144532825, -8.475808217655753651, 34.90892951860618609 ) ) ;
#52488=ORIENTED_EDGE ( 'NONE', *, *, #50214, .T. ) ;
#52489=ORIENTED_EDGE ( 'NONE', *, *, #72683, .T. ) ;
#52490=EDGE_CURVE ( 'NONE', #7165, #3616, #82499, .T. ) ;
#52491=EDGE_LOOP ( 'NONE', ( #16717, #65567, #89083, #31007 ) ) ;
#52492=CARTESIAN_POINT ( 'NONE',  ( -6.923076923076922462, -11.91647553114624181, 32.58852847137148245 ) ) ;
#52493=CARTESIAN_POINT ( 'NONE',  ( -5.076923076923197442, -4.481592998941358097, 33.73612834414048933 ) ) ;
#52494=LINE ( 'NONE', #79542, #10627 ) ;
#52496=DIRECTION ( 'NONE',  ( -0.000000000000000000, -0.5000000000000009992, -0.8660254037844380415 ) ) ;
#52497=CARTESIAN_POINT ( 'NONE',  ( 5.750023269057646935, -12.41269422305637171, 30.68257228309993323 ) ) ;
#52499=EDGE_CURVE ( 'NONE', #43224, #5405, #15807, .T. ) ;
#52500=EDGE_LOOP ( 'NONE', ( #36467, #79616 ) ) ;
#52502=ADVANCED_FACE ( 'NONE', ( #9659 ), #36696, .F. ) ;
#52504=ORIENTED_EDGE ( 'NONE', *, *, #65666, .F. ) ;
#52505=CARTESIAN_POINT ( 'NONE',  ( -12.71156169883142617, -11.37209801155882971, 32.91403422569032955 ) ) ;
#52506=ORIENTED_EDGE ( 'NONE', *, *, #15521, .T. ) ;
#52507=CARTESIAN_POINT ( 'NONE',  ( -10.36533019547115941, -4.074993327901527351, 33.72946981652012255 ) ) ;
#52508=CARTESIAN_POINT ( 'NONE',  ( 7.846153846154153122, -2.506253911140614576, 30.00000000000323297 ) ) ;
#52510=ORIENTED_EDGE ( 'NONE', *, *, #56076, .T. ) ;
#52511=CARTESIAN_POINT ( 'NONE',  ( -14.37296230824862775, -12.51329471203370325, 31.30864560766548976 ) ) ;
#52512=ORIENTED_EDGE ( 'NONE', *, *, #63030, .T. ) ;
#52514=CARTESIAN_POINT ( 'NONE',  ( 0.4615384615384611200, -11.35647404775217417, 33.31231777344666511 ) ) ;
#52515=CARTESIAN_POINT ( 'NONE',  ( 7.716005876422150855, -4.299443229763728169, 33.91186481527756058 ) ) ;
#52516=CARTESIAN_POINT ( 'NONE',  ( -6.700297381808513641, -12.44528174975671853, 30.48912976160716681 ) ) ;
#52517=DIRECTION ( 'NONE',  ( -0.000000000000000000, 0.9848077530122085754, -0.1736481776669273613 ) ) ;
#52518=EDGE_CURVE ( 'NONE', #22873, #1344, #65033, .T. ) ;
#52519=CARTESIAN_POINT ( 'NONE',  ( -2.980823712421088345, -6.696923467548660192, 34.68552623307873972 ) ) ;
#52520=DIRECTION ( 'NONE',  ( -0.000000000000000000, 0.9396926207859093161, -0.3420201433256663259 ) ) ;
#52521=ORIENTED_EDGE ( 'NONE', *, *, #8186, .T. ) ;
#52522=DIRECTION ( 'NONE',  ( -0.000000000000000000, 0.7660444431189791237, -0.6427876096865379196 ) ) ;
#52523=CARTESIAN_POINT ( 'NONE',  ( 11.28846153846153832, -2.249999999999998668, 29.75000000000000355 ) ) ;
#52524=EDGE_CURVE ( 'NONE', #71802, #7759, #36261, .T. ) ;
#52525=CARTESIAN_POINT ( 'NONE',  ( 14.55774672760576394, -4.074993327901527351, 33.72946981652012255 ) ) ;
#52528=CARTESIAN_POINT ( 'NONE',  ( -14.98082382139119062, -5.766571408460171355, 34.70601412856602508 ) ) ;
#52530=CARTESIAN_POINT ( 'NONE',  ( -9.692307692307812417, -2.625532179533778709, 30.86335684631627174 ) ) ;
#52531=CIRCLE ( 'NONE', #9403, 0.2500000000000002220 ) ;
#52532=FACE_BOUND ( 'NONE', #38741, .T. ) ;
#52533=CARTESIAN_POINT ( 'NONE',  ( 12.21156173059610772, -3.137211980971221781, 32.19342716148376837 ) ) ;
#52535=EDGE_CURVE ( 'NONE', #85190, #88762, #20100, .T. ) ;
#52536=CARTESIAN_POINT ( 'NONE',  ( -15.10024379253558635, -5.070358843744210198, 34.40418822224088302 ) ) ;
#52537=CARTESIAN_POINT ( 'NONE',  ( 18.13079180782478872, -11.18335022499818621, 33.13157742990016885 ) ) ;
#52538=CARTESIAN_POINT ( 'NONE',  ( -11.47320639894870276, -11.06231777344671130, 33.60647404775212976 ) ) ;
#52540=CARTESIAN_POINT ( 'NONE',  ( 6.000000000000001776, -4.661471528628507777, 34.16647553114623292 ) ) ;
#52542=CARTESIAN_POINT ( 'NONE',  ( 10.61538461538449418, -12.16647553114689728, 32.15551576947799362 ) ) ;
#52544=CARTESIAN_POINT ( 'NONE',  ( -9.692307692307691624, -1.129524287112498415, 32.06866353760679544 ) ) ;
#52545=CARTESIAN_POINT ( 'NONE',  ( -15.16562345143726631, -7.750023238201979581, 34.74374492549440419 ) ) ;
#52546=CARTESIAN_POINT ( 'NONE',  ( -3.230769230769229949, -3.050289026998446396, 32.03036669348365706 ) ) ;
#52548=AXIS2_PLACEMENT_3D ( 'NONE', #63911, #22932, #50394 ) ;
#52549=CARTESIAN_POINT ( 'NONE',  ( 16.94623247381277054, -12.62707690430377383, 30.88035979386743435 ) ) ;
#52550=CARTESIAN_POINT ( 'NONE',  ( 1.384615384615386802, -11.91647553114624181, 32.58852847137148245 ) ) ;
#52552=CARTESIAN_POINT ( 'NONE',  ( 14.30769230769218758, -10.90142922262034020, 33.41473453929536674 ) ) ;
#52553=LINE ( 'NONE', #80038, #28822 ) ;
#52554=DIRECTION ( 'NONE',  ( 0.000000000000000000, 1.000000000000000000, 0.000000000000000000 ) ) ;
#52555=CARTESIAN_POINT ( 'NONE',  ( -0.5922290646487686772, -8.191372820521381826, 34.95448215188423546 ) ) ;
#52556=CARTESIAN_POINT ( 'NONE',  ( 14.53070365930516239, -5.667800583137506010, 34.40243808032445827 ) ) ;
#52557=CARTESIAN_POINT ( 'NONE',  ( -8.899377978668987055, -9.418419913701741919, 34.36755862841477693 ) ) ;
#52558=CARTESIAN_POINT ( 'NONE',  ( -18.25002323729295739, -2.823816976329321271, 31.52131813110797154 ) ) ;
#52561=ORIENTED_EDGE ( 'NONE', *, *, #18382, .F. ) ;
#52562=CARTESIAN_POINT ( 'NONE',  ( 2.307692307692309264, -10.67929555188718282, 33.92786785259544047 ) ) ;
#52563=CARTESIAN_POINT ( 'NONE',  ( -11.53846153846153655, -8.810774026931790459, 35.74407628777942847 ) ) ;
#52565=ADVANCED_FACE ( 'NONE', ( #70483 ), #4238, .F. ) ;
#52566=CARTESIAN_POINT ( 'NONE',  ( 6.000000000000001776, -4.098570777380720287, 33.41473453929634729 ) ) ;
#52567=CARTESIAN_POINT ( 'NONE',  ( 3.296837581771670411, -11.69971097300155272, 32.46337939537588113 ) ) ;
#52568=EDGE_LOOP ( 'NONE', ( #12718, #16970 ) ) ;
#52569=CARTESIAN_POINT ( 'NONE',  ( -18.00000000000000000, -6.343179335718452272, 34.87096338111211935 ) ) ;
#52571=CARTESIAN_POINT ( 'NONE',  ( 8.834485908743600291, -2.657715359629132301, 31.77849191805844242 ) ) ;
#52572=ORIENTED_EDGE ( 'NONE', *, *, #28502, .T. ) ;
#52573=CARTESIAN_POINT ( 'NONE',  ( 11.78851595837499211, -4.818054556918156983, 34.26375889529406749 ) ) ;
#52574=CARTESIAN_POINT ( 'NONE',  ( -15.23076923076922995, -5.180354513474913603, 36.12317359536750416 ) ) ;
#52575=EDGE_CURVE ( 'NONE', #77667, #10170, #45667, .T. ) ;
#52576=CARTESIAN_POINT ( 'NONE',  ( -4.946131269098287930, -8.999086150933472084, 34.52020707165672064 ) ) ;
#52577=VECTOR ( 'NONE', #79943, 1000.000000000000227 ) ;
#52578=CARTESIAN_POINT ( 'NONE',  ( -11.66915214157184444, -2.494641256782728966, 31.33461815524612959 ) ) ;
#52579=ORIENTED_EDGE ( 'NONE', *, *, #69279, .F. ) ;
#52580=DIRECTION ( 'NONE',  ( -0.000000000000000000, 0.7660444431189791237, -0.6427876096865379196 ) ) ;
#52581=CARTESIAN_POINT ( 'NONE',  ( -12.59168643127016374, -2.647304123082328875, 31.75400227202885972 ) ) ;
#52583=VERTEX_POINT ( 'NONE', #86684 ) ;
#52584=VERTEX_POINT ( 'NONE', #86232 ) ;
#52586=B_SPLINE_CURVE_WITH_KNOTS ( 'NONE', 3,
 ( #43210, #2210, #22057, #64348, #69794, #29705, #2646, #63475, #8103, #28823 ),
 .UNSPECIFIED., .F., .F.,
 ( 4, 2, 2, 2, 4 ),
 ( 0.000000000000000000, 0.0001954311564186880399, 0.0003908623128373760799, 0.0005862934692560641198, 0.0007817246256747521597 ),
 .UNSPECIFIED. ) ;
#52587=ORIENTED_EDGE ( 'NONE', *, *, #2804, .T. ) ;
#52589=CARTESIAN_POINT ( 'NONE',  ( -8.519285250882628446, -3.202959910592335646, 32.30730279482227019 ) ) ;
#52591=B_SPLINE_CURVE_WITH_KNOTS ( 'NONE', 3,
 ( #14264, #34534, #69207, #48037, #76856, #27336, #68320, #54798, #34088, #61552 ),
 .UNSPECIFIED., .F., .F.,
 ( 4, 2, 2, 2, 4 ),
 ( 0.000000000000000000, 0.0001954339857564073388, 0.0003908679715128146777, 0.0005863019572692220165, 0.0007817359430256293554 ),
 .UNSPECIFIED. ) ;
#52592=FACE_OUTER_BOUND ( 'NONE', #6360, .T. ) ;
#52593=CARTESIAN_POINT ( 'NONE',  ( 4.826923076923076650, -7.500000000000001776, 34.75000000000000000 ) ) ;
#52594=EDGE_CURVE ( 'NONE', #80969, #51215, #81370, .T. ) ;
#52595=VECTOR ( 'NONE', #49439, 1000.000000000000000 ) ;
#52596=ORIENTED_EDGE ( 'NONE', *, *, #5988, .F. ) ;
#52597=VERTEX_POINT ( 'NONE', #12334 ) ;
#52598=CARTESIAN_POINT ( 'NONE',  ( 11.53846153846153832, -11.35647404775217417, 33.31231777344666511 ) ) ;
#52602=CARTESIAN_POINT ( 'NONE',  ( 18.00000000000000000, -2.486705287966279876, 31.30864560766543647 ) ) ;
#52603=CARTESIAN_POINT ( 'NONE',  ( 1.607394925883795844, -10.81320215134717344, 33.49497208177562868 ) ) ;
#52604=DIRECTION ( 'NONE',  ( 1.000000000000000000, 0.000000000000000000, 0.000000000000000000 ) ) ;
#52605=AXIS2_PLACEMENT_3D ( 'NONE', #1224, #35912, #21495 ) ;
#52606=ORIENTED_EDGE ( 'NONE', *, *, #5301, .F. ) ;
#52608=EDGE_CURVE ( 'NONE', #65351, #79454, #53431, .T. ) ;
#52609=ORIENTED_EDGE ( 'NONE', *, *, #82508, .T. ) ;
#52611=EDGE_LOOP ( 'NONE', ( #70556, #82949, #49322, #4403 ) ) ;
#52612=DIRECTION ( 'NONE',  ( -0.000000000000000000, 0.7660444431189791237, -0.6427876096865379196 ) ) ;
#52614=ORIENTED_EDGE ( 'NONE', *, *, #46647, .F. ) ;
#52616=B_SPLINE_CURVE_WITH_KNOTS ( 'NONE', 3,
 ( #74710, #20201, #34148, #83232, #26959, #68379, #82794, #55744, #48992, #33275 ),
 .UNSPECIFIED., .F., .F.,
 ( 4, 2, 2, 2, 4 ),
 ( 0.000000000000000000, 0.0001954311564186863052, 0.0003908623128373726104, 0.0005862934692560589156, 0.0007817246256747452209 ),
 .UNSPECIFIED. ) ;
#52617=CARTESIAN_POINT ( 'NONE',  ( -13.63463862190834952, -4.335965774309648246, 33.62209801155881905 ) ) ;
#52618=CARTESIAN_POINT ( 'NONE',  ( 15.23076923076923173, -4.102666532097928531, 36.13435417666054406 ) ) ;
#52619=CARTESIAN_POINT ( 'NONE',  ( -5.999999999999998224, -13.57706302396349152, 30.56769352161908060 ) ) ;
#52620=FACE_BOUND ( 'NONE', #10537, .T. ) ;
#52621=CARTESIAN_POINT ( 'NONE',  ( -5.299850035829926753, -10.01117774369187252, 34.36070679894347535 ) ) ;
#52622=CARTESIAN_POINT ( 'NONE',  ( 16.15384615384615330, -10.67929555188718282, 33.92786785259544047 ) ) ;
#52623=CARTESIAN_POINT ( 'NONE',  ( -8.835314180186648159, -4.098570777380719399, 33.41473453929634729 ) ) ;
#52624=CARTESIAN_POINT ( 'NONE',  ( 3.296836564119306257, -3.322132147404559976, 32.92929555188717927 ) ) ;
#52625=CARTESIAN_POINT ( 'NONE',  ( 14.53070515178570865, -2.889357225399416418, 32.26129605718031002 ) ) ;
#52627=LINE ( 'NONE', #67935, #38080 ) ;
#52628=DIRECTION ( 'NONE',  ( -0.000000000000000000, 1.000000000000000000, -0.000000000000000000 ) ) ;
#52629=ORIENTED_EDGE ( 'NONE', *, *, #4537, .T. ) ;
#52630=CARTESIAN_POINT ( 'NONE',  ( -16.08767701288349627, -7.250054483168842268, 34.74374881642865631 ) ) ;
#52631=CARTESIAN_POINT ( 'NONE',  ( 12.46153846153833911, -3.643525952248795718, 33.31231777344771672 ) ) ;
#52632=VERTEX_POINT ( 'NONE', #72246 ) ;
#52633=EDGE_CURVE ( 'NONE', #87267, #23252, #16911, .T. ) ;
#52634=ORIENTED_EDGE ( 'NONE', *, *, #19522, .F. ) ;
#52635=CIRCLE ( 'NONE', #64128, 0.2500000000000002220 ) ;
#52637=CARTESIAN_POINT ( 'NONE',  ( -17.29984929443922681, -11.24512374952581872, 33.06303171183252942 ) ) ;
#52638=CARTESIAN_POINT ( 'NONE',  ( 16.15384615384615330, -6.343179335718451384, 34.87096338111211935 ) ) ;
#52639=CARTESIAN_POINT ( 'NONE',  ( 16.02315468717859304, -3.530157926970578508, 32.79014554554150607 ) ) ;
#52640=CARTESIAN_POINT ( 'NONE',  ( 13.38461538461538680, -11.33034616979429110, 35.88435417666054406 ) ) ;
#52642=LINE ( 'NONE', #79681, #70188 ) ;
#52643=CARTESIAN_POINT ( 'NONE',  ( 4.376625822824220080, -4.989023458446560255, 34.36081565061822118 ) ) ;
#52644=CARTESIAN_POINT ( 'NONE',  ( 2.307692307692309264, -1.509761064869970415, 31.06009739812519044 ) ) ;
#52645=LINE ( 'NONE', #80129, #44501 ) ;
#52647=CARTESIAN_POINT ( 'NONE',  ( 2.530703659305157949, -4.887748414852789658, 34.01359900205216746 ) ) ;
#52649=CARTESIAN_POINT ( 'NONE',  ( -17.07692307692307665, -2.486705287966279876, 31.30864560766543647 ) ) ;
#52651=VERTEX_POINT ( 'NONE', #5131 ) ;
#52652=ORIENTED_EDGE ( 'NONE', *, *, #17418, .T. ) ;
#52653=DIRECTION ( 'NONE',  ( 0.000000000000000000, 1.000000000000000000, 0.000000000000000000 ) ) ;
#52654=CARTESIAN_POINT ( 'NONE',  ( -4.377331097570100304, -12.44517049084099725, 30.48991314939691932 ) ) ;
#52656=DIRECTION ( 'NONE',  ( -0.000000000000000000, -0.9396926207859093161, -0.3420201433256663259 ) ) ;
#52657=DIRECTION ( 'NONE',  ( 0.000000000000000000, 0.9848077530122072432, -0.1736481776669354937 ) ) ;
#52659=B_SPLINE_CURVE_WITH_KNOTS ( 'NONE', 3,
 ( #53526, #45883, #39600, #80581, #4915, #79679, #32381, #18865, #81467, #31941 ),
 .UNSPECIFIED., .F., .F.,
 ( 4, 2, 2, 2, 4 ),
 ( 0.000000000000000000, 0.0001954311564186862781, 0.0003908623128373725562, 0.0005862934692560588072, 0.0007817246256747451124 ),
 .UNSPECIFIED. ) ;
#52660=CARTESIAN_POINT ( 'NONE',  ( -1.634638608836840534, -4.175268141568689195, 33.81360843649122216 ) ) ;
#52661=CARTESIAN_POINT ( 'NONE',  ( -13.63459211555773720, -8.303909089506435137, 34.68538101551103381 ) ) ;
#52662=LINE ( 'NONE', #11697, #57385 ) ;
#52663=CARTESIAN_POINT ( 'NONE',  ( -6.250000000000018652, -2.249999999999999112, 29.81609741502488120 ) ) ;
#52664=CARTESIAN_POINT ( 'NONE',  ( 6.923076923076924238, -10.51840700105979565, 33.73612834413961536 ) ) ;
#52665=CARTESIAN_POINT ( 'NONE',  ( 15.10062126103753855, -12.50552854090298638, 31.33409797877408920 ) ) ;
#52666=CARTESIAN_POINT ( 'NONE',  ( 2.241608896736428491, -3.050289026998445951, 32.03036669348365706 ) ) ;
#52667=CARTESIAN_POINT ( 'NONE',  ( 7.146089767170317408, -2.308499170217967134, 30.53291367094873721 ) ) ;
#52668=AXIS2_PLACEMENT_3D ( 'NONE', #86130, #24405, #73050 ) ;
#52669=CARTESIAN_POINT ( 'NONE',  ( -5.934744860487160878, -5.094484230520773593, 34.41647553114626845 ) ) ;
#52670=CARTESIAN_POINT ( 'NONE',  ( -4.219929564802033184, -8.973038597847269315, 34.52809138561120506 ) ) ;
#52671=CARTESIAN_POINT ( 'NONE',  ( -15.48074596171158390, -9.943427161483782584, 34.11278801902876978 ) ) ;
#52673=CARTESIAN_POINT ( 'NONE',  ( 1.384615384615264011, -10.33852847137269571, 34.16647553114546554 ) ) ;
#52674=FACE_OUTER_BOUND ( 'NONE', #86833, .T. ) ;
#52675=CARTESIAN_POINT ( 'NONE',  ( -4.283994123577847368, -5.915902021225892149, 34.75552854090298638 ) ) ;
#52678=CARTESIAN_POINT ( 'NONE',  ( 4.153846153846154188, -9.780366693483667717, 34.19971097300155094 ) ) ;
#52680=DIRECTION ( 'NONE',  ( 1.000000000000000000, 0.000000000000000000, 0.000000000000000000 ) ) ;
#52681=ORIENTED_EDGE ( 'NONE', *, *, #15670, .F. ) ;
#52683=CARTESIAN_POINT ( 'NONE',  ( 3.230769230769108269, -8.656820664282941280, 34.87096338111179961 ) ) ;
#52686=ORIENTED_EDGE ( 'NONE', *, *, #22456, .F. ) ;
#52687=CARTESIAN_POINT ( 'NONE',  ( 17.99999999999987566, -9.442884908241554243, 34.35708131394783038 ) ) ;
#52689=EDGE_LOOP ( 'NONE', ( #46736, #84874, #69589, #75112 ) ) ;
#52690=CARTESIAN_POINT ( 'NONE',  ( -7.596208436775802930, -6.653508905675592722, 34.93172785388651391 ) ) ;
#52691=CARTESIAN_POINT ( 'NONE',  ( 13.16168916709923664, -9.886141570436013382, 34.14413921362392301 ) ) ;
#52693=ORIENTED_EDGE ( 'NONE', *, *, #27313, .T. ) ;
#52694=CARTESIAN_POINT ( 'NONE',  ( -10.54931626438217585, -12.37446782046654192, 30.86335684631486842 ) ) ;
#52695=EDGE_LOOP ( 'NONE', ( #3076, #38626, #33324, #71805 ) ) ;
#52696=EDGE_CURVE ( 'NONE', #70675, #41861, #13223, .T. ) ;
#52697=CARTESIAN_POINT ( 'NONE',  ( -18.00000000000000000, -12.37446782046654192, 30.86335684631486131 ) ) ;
#52698=ORIENTED_EDGE ( 'NONE', *, *, #52222, .T. ) ;
#52699=CARTESIAN_POINT ( 'NONE',  ( -0.7115151924808151840, -3.137211980971221781, 32.19342716148376837 ) ) ;
#52700=CARTESIAN_POINT ( 'NONE',  ( 0.4615384615384611200, -13.75783147151868846, 33.36296068462461051 ) ) ;
#52701=CARTESIAN_POINT ( 'NONE',  ( 9.626224281351815293, -8.973038597847271092, 34.52809138561120506 ) ) ;
#52702=DIRECTION ( 'NONE',  ( 0.000000000000000000, 0.7660444431189807890, 0.6427876096865361433 ) ) ;
#52703=CARTESIAN_POINT ( 'NONE',  ( 14.30769230769231015, -2.249999999999998668, 29.75000000000001776 ) ) ;
#52705=LINE ( 'NONE', #44602, #14700 ) ;
#52706=B_SPLINE_CURVE_WITH_KNOTS ( 'NONE', 3,
 ( #65047, #51982, #37585, #29512, #3357, #79479, #36705, #38041, #51079, #36270 ),
 .UNSPECIFIED., .F., .F.,
 ( 4, 2, 2, 2, 4 ),
 ( 0.000000000000000000, 0.0001954311564186881213, 0.0003908623128373762425, 0.0005862934692560643367, 0.0007817246256747524850 ),
 .UNSPECIFIED. ) ;
#52707=ORIENTED_EDGE ( 'NONE', *, *, #69652, .F. ) ;
#52708=ORIENTED_EDGE ( 'NONE', *, *, #45934, .T. ) ;
#52709=ORIENTED_EDGE ( 'NONE', *, *, #71444, .T. ) ;
#52710=CARTESIAN_POINT ( 'NONE',  ( 17.75000000000000000, -7.500000000000001776, 35.00000000000000000 ) ) ;
#52711=ORIENTED_EDGE ( 'NONE', *, *, #63555, .T. ) ;
#52713=CYLINDRICAL_SURFACE ( 'NONE', #80933, 0.2499999999999998890 ) ;
#52714=CARTESIAN_POINT ( 'NONE',  ( 9.692307692307570832, -5.941354392335915335, 34.76329471203413846 ) ) ;
#52715=ORIENTED_EDGE ( 'NONE', *, *, #38520, .F. ) ;
#52716=CARTESIAN_POINT ( 'NONE',  ( -0.7115384615384606759, -7.500000000000001776, 35.00000000000000000 ) ) ;
#52717=EDGE_CURVE ( 'NONE', #42856, #68029, #23271, .T. ) ;
#52718=ORIENTED_EDGE ( 'NONE', *, *, #39369, .T. ) ;
#52719=CARTESIAN_POINT ( 'NONE',  ( -10.83886955910856464, -3.236172620538810385, 32.36188796281390267 ) ) ;
#52722=EDGE_CURVE ( 'NONE', #30240, #23926, #62015, .T. ) ;
#52723=EDGE_CURVE ( 'NONE', #33268, #49750, #49136, .T. ) ;
#52724=CARTESIAN_POINT ( 'NONE',  ( 3.930361229281821966, -12.69144148231606017, 30.53333754910549303 ) ) ;
#52725=CYLINDRICAL_SURFACE ( 'NONE', #58335, 0.2499999999999995559 ) ;
#52726=FACE_BOUND ( 'NONE', #46846, .T. ) ;
#52728=CARTESIAN_POINT ( 'NONE',  ( 2.307692307692309264, -2.538708090699994813, 30.37095296980875503 ) ) ;
#52730=CARTESIAN_POINT ( 'NONE',  ( -14.05774678934416499, -5.852078868378309373, 34.47109172314383585 ) ) ;
#52731=CARTESIAN_POINT ( 'NONE',  ( -6.000000000000119904, -5.219633306517616589, 34.19971097300220464 ) ) ;
#52733=ORIENTED_EDGE ( 'NONE', *, *, #88331, .F. ) ;
#52734=AXIS2_PLACEMENT_3D ( 'NONE', #11375, #17697, #78943 ) ;
#52735=CARTESIAN_POINT ( 'NONE',  ( 1.634615384615386580, -2.249999999999998668, 29.75000000000000355 ) ) ;
#52736=VERTEX_POINT ( 'NONE', #20856 ) ;
#52738=ORIENTED_EDGE ( 'NONE', *, *, #20807, .T. ) ;
#52739=CARTESIAN_POINT ( 'NONE',  ( 10.68145296638705233, -12.37446782046654192, 30.86335684631486842 ) ) ;
#52741=CARTESIAN_POINT ( 'NONE',  ( -12.46153846153846168, -13.75783147151868846, 33.36296068462461051 ) ) ;
#52742=CARTESIAN_POINT ( 'NONE',  ( -2.176900499867519212, -12.11778462344221019, 31.66786338562085135 ) ) ;
#52743=EDGE_CURVE ( 'NONE', #62464, #75687, #41853, .T. ) ;
#52744=CARTESIAN_POINT ( 'NONE',  ( 17.01116627440877238, -7.249945686854186278, 34.74374336980224598 ) ) ;
#52745=CARTESIAN_POINT ( 'NONE',  ( -2.057637996053991003, -2.779044189368095719, 31.39831045268885745 ) ) ;
#52747=EDGE_LOOP ( 'NONE', ( #45074, #19007 ) ) ;
#52748=CARTESIAN_POINT ( 'NONE',  ( 17.07692307692295586, -6.026961402154118908, 34.52809138561165270 ) ) ;
#52749=CARTESIAN_POINT ( 'NONE',  ( 15.23076923076910916, -4.320704448113951379, 33.92786785259630022 ) ) ;
#52750=CARTESIAN_POINT ( 'NONE',  ( 10.39189969082028497, -3.019605429927184392, 32.48692288466676814 ) ) ;
#52751=CARTESIAN_POINT ( 'NONE',  ( 10.86543892702293057, -11.79725096376909654, 32.30694842903959341 ) ) ;
#52753=ADVANCED_FACE ( 'NONE', ( #34811 ), #27616, .F. ) ;
#52754=ORIENTED_EDGE ( 'NONE', *, *, #44412, .T. ) ;
#52756=VERTEX_POINT ( 'NONE', #74930 ) ;
#52757=CARTESIAN_POINT ( 'NONE',  ( -0.4615384615384611200, -4.098570777380720287, 33.41473453929634729 ) ) ;
#52758=CARTESIAN_POINT ( 'NONE',  ( 4.853996118016225658, -2.889293201056495786, 32.26117774369186009 ) ) ;
#52759=ORIENTED_EDGE ( 'NONE', *, *, #47151, .F. ) ;
#52761=DIRECTION ( 'NONE',  ( 0.000000000000000000, 0.8660254037844377084, 0.5000000000000015543 ) ) ;
#52762=CARTESIAN_POINT ( 'NONE',  ( 16.02315468717859659, -8.147922237126337563, 34.70805685702651999 ) ) ;
#52763=B_SPLINE_CURVE_WITH_KNOTS ( 'NONE', 3,
 ( #19784, #45471, #60318, #13027, #26099, #40513, #72950, #80159, #11705, #40078 ),
 .UNSPECIFIED., .F., .F.,
 ( 4, 2, 2, 2, 4 ),
 ( 0.0007817246256747554124, 0.0009771112852218991757, 0.001172497944769043156, 0.001367884604316187136, 0.001563271263863330899 ),
 .UNSPECIFIED. ) ;
#52764=CARTESIAN_POINT ( 'NONE',  ( 1.450682717965461999, -6.343179335718451384, 34.87096338111212646 ) ) ;
#52765=CIRCLE ( 'NONE', #13942, 0.2500000000000002220 ) ;
#52766=CARTESIAN_POINT ( 'NONE',  ( -13.38461538461538325, -12.78798330534103123, 29.99999999999997868 ) ) ;
#52767=ORIENTED_EDGE ( 'NONE', *, *, #61774, .T. ) ;
#52768=CARTESIAN_POINT ( 'NONE',  ( 0.2380535178145120334, -10.11188796281391511, 34.01382737946119050 ) ) ;
#52769=ORIENTED_EDGE ( 'NONE', *, *, #48075, .F. ) ;
#52770=CARTESIAN_POINT ( 'NONE',  ( 15.36156103859402045, -8.147973898785416225, 34.70805048591653730 ) ) ;
#52771=CARTESIAN_POINT ( 'NONE',  ( -3.165514091256391715, -2.657715359629131857, 31.77849191805844242 ) ) ;
#52772=CARTESIAN_POINT ( 'NONE',  ( -7.780898706641008467, -3.643525952247865352, 33.31231777344670064 ) ) ;
#52773=CARTESIAN_POINT ( 'NONE',  ( 10.36536139116315525, -12.45566812827425451, 31.48439005359158926 ) ) ;
#52774=DIRECTION ( 'NONE',  ( 0.000000000000000000, 0.4999999999999985567, 0.8660254037844395958 ) ) ;
#52775=AXIS2_PLACEMENT_3D ( 'NONE', #47911, #1061, #61861 ) ;
#52776=DIRECTION ( 'NONE',  ( 1.000000000000000000, 0.000000000000000000, 0.000000000000000000 ) ) ;
#52777=FACE_OUTER_BOUND ( 'NONE', #35391, .T. ) ;
#52779=ORIENTED_EDGE ( 'NONE', *, *, #10287, .F. ) ;
#52780=DIRECTION ( 'NONE',  ( -0.000000000000000000, -0.6427876096865404731, -0.7660444431189771253 ) ) ;
#52781=B_SPLINE_CURVE_WITH_KNOTS ( 'NONE', 3,
 ( #49362, #50673, #36729, #30418, #1618, #43046, #42173, #14688, #84932, #22330 ),
 .UNSPECIFIED., .F., .F.,
 ( 4, 2, 2, 2, 4 ),
 ( 0.000000000000000000, 0.0001954339881912775425, 0.0003908679763825550850, 0.0005863019645738326005, 0.0007817359527651101701 ),
 .UNSPECIFIED. ) ;
#52782=FACE_OUTER_BOUND ( 'NONE', #5544, .T. ) ;
#52783=CARTESIAN_POINT ( 'NONE',  ( -0.2385271099256122407, -4.887748414852793211, 34.01359900205216746 ) ) ;
#52785=EDGE_LOOP ( 'NONE', ( #88084, #75933, #15280, #31086 ) ) ;
#52786=ORIENTED_EDGE ( 'NONE', *, *, #30504, .F. ) ;
#52787=CARTESIAN_POINT ( 'NONE',  ( -11.78843826940389583, -10.66389620160130036, 33.62221079203477103 ) ) ;
#52788=CARTESIAN_POINT ( 'NONE',  ( 11.31497661389720832, -4.988325925672468131, 34.36044203135681130 ) ) ;
#52790=CARTESIAN_POINT ( 'NONE',  ( 13.25446741488369007, -3.069018819979302926, 32.56621877034667278 ) ) ;
#52792=CARTESIAN_POINT ( 'NONE',  ( 5.934729554039225974, -8.613356846314824011, 34.62446782046655613 ) ) ;
#52793=ORIENTED_EDGE ( 'NONE', *, *, #30119, .F. ) ;
#52794=AXIS2_PLACEMENT_3D ( 'NONE', #27558, #7736, #67662 ) ;
#52795=LINE ( 'NONE', #72624, #54922 ) ;
#52796=B_SPLINE_CURVE_WITH_KNOTS ( 'NONE', 3,
 ( #60640, #47122, #52549, #25535, #74612, #53438, #59759, #61087, #80034, #80486 ),
 .UNSPECIFIED., .F., .F.,
 ( 4, 2, 2, 2, 4 ),
 ( 0.000000000000000000, 0.0001954311564186879857, 0.0003908623128373759715, 0.0005862934692560640114, 0.0007817246256747519429 ),
 .UNSPECIFIED. ) ;
#52797=FACE_OUTER_BOUND ( 'NONE', #52395, .T. ) ;
#52798=CARTESIAN_POINT ( 'NONE',  ( 4.023155550735846298, -8.191372820521381826, 34.95448215188423546 ) ) ;
#52799=ORIENTED_EDGE ( 'NONE', *, *, #13391, .T. ) ;
#52800=CARTESIAN_POINT ( 'NONE',  ( 16.08857615328983925, -12.51329471203370325, 31.30864560766548976 ) ) ;
#52801=ORIENTED_EDGE ( 'NONE', *, *, #88970, .T. ) ;
#52803=CARTESIAN_POINT ( 'NONE',  ( -0.4615384615384611200, -12.34228464037088635, 31.77849191805839268 ) ) ;
#52804=CARTESIAN_POINT ( 'NONE',  ( 6.222779668978065004, -12.11081565061823717, 32.26097654155341843 ) ) ;
#52805=ORIENTED_EDGE ( 'NONE', *, *, #10671, .T. ) ;
#52806=CARTESIAN_POINT ( 'NONE',  ( 0.7114839798866027243, -4.336752205174647656, 33.62275283266504289 ) ) ;
#52807=FACE_OUTER_BOUND ( 'NONE', #69687, .T. ) ;
#52808=CARTESIAN_POINT ( 'NONE',  ( -9.758391103263571509, -2.538708090699994813, 30.37095296980875148 ) ) ;
#52810=DIRECTION ( 'NONE',  ( -0.000000000000000000, -0.5000000000000009992, -0.8660254037844380415 ) ) ;
#52811=CARTESIAN_POINT ( 'NONE',  ( 3.480823650682684622, -2.920487667080175154, 32.31805714834170828 ) ) ;
#52812=ORIENTED_EDGE ( 'NONE', *, *, #57239, .F. ) ;
#52813=FACE_OUTER_BOUND ( 'NONE', #66411, .T. ) ;
#52815=CARTESIAN_POINT ( 'NONE',  ( 8.519254038288414321, -12.41269422305637171, 30.68257228309993323 ) ) ;
#52816=DIRECTION ( 'NONE',  ( -0.000000000000000000, -0.7660444431189791237, -0.6427876096865379196 ) ) ;
#52817=CARTESIAN_POINT ( 'NONE',  ( -11.53846153846153655, -5.557115091759785130, 34.35708131394839171 ) ) ;
#52820=EDGE_CURVE ( 'NONE', #2196, #25833, #54631, .T. ) ;
#52821=CARTESIAN_POINT ( 'NONE',  ( 6.923076923076924238, -2.833524468853757305, 32.15551576947925838 ) ) ;
#52823=CARTESIAN_POINT ( 'NONE',  ( 15.16468581981335007, -11.69971097300155272, 32.46337939537587403 ) ) ;
#52824=ADVANCED_FACE ( 'NONE', ( #21297 ), #74476, .F. ) ;
#52825=ORIENTED_EDGE ( 'NONE', *, *, #72543, .F. ) ;
#52826=ORIENTED_EDGE ( 'NONE', *, *, #72516, .F. ) ;
#52828=B_SPLINE_CURVE_WITH_KNOTS ( 'NONE', 3,
 ( #24323, #79290, #11271, #17592, #3168, #23875, #45040, #72520, #53132, #4053 ),
 .UNSPECIFIED., .F., .F.,
 ( 4, 2, 2, 2, 4 ),
 ( 0.000000000000000000, 0.0001954311564186871726, 0.0003908623128373743452, 0.0005862934692560615177, 0.0007817246256747486903 ),
 .UNSPECIFIED. ) ;
#52829=ORIENTED_EDGE ( 'NONE', *, *, #38163, .F. ) ;
#52830=VERTEX_POINT ( 'NONE', #26287 ) ;
#52831=EDGE_CURVE ( 'NONE', #41914, #49557, #41138, .T. ) ;
#52832=CARTESIAN_POINT ( 'NONE',  ( -16.37677237136229991, -3.586966769969702540, 32.86292498521069660 ) ) ;
#52833=CARTESIAN_POINT ( 'NONE',  ( -11.60454494941741999, -8.973038597847271092, 34.52809138561120506 ) ) ;
#52834=CARTESIAN_POINT ( 'NONE',  ( -17.07692307692307665, -13.04860791097971706, 34.73218667398347037 ) ) ;
#52835=CARTESIAN_POINT ( 'NONE',  ( -5.749945688361683516, -4.943051570960391494, 34.04725096376909477 ) ) ;
#52836=CARTESIAN_POINT ( 'NONE',  ( -13.38461538461538325, -5.557115091759785130, 34.35708131394839171 ) ) ;
#52837=CARTESIAN_POINT ( 'NONE',  ( -6.222926958906846551, -2.889293201056495786, 32.26117774369186009 ) ) ;
#52838=CARTESIAN_POINT ( 'NONE',  ( -0.5268089074992379217, -11.94971097300153140, 32.03036669348370680 ) ) ;
#52839=CARTESIAN_POINT ( 'NONE',  ( -4.023054346021365468, -10.54018710029568595, 33.71981072465678864 ) ) ;
#52840=CARTESIAN_POINT ( 'NONE',  ( 0.2386122440223125696, -3.105860786376062332, 32.13614157043599562 ) ) ;
#52841=ORIENTED_EDGE ( 'NONE', *, *, #38853, .F. ) ;
#52843=VERTEX_POINT ( 'NONE', #63167 ) ;
#52844=CARTESIAN_POINT ( 'NONE',  ( -1.450698795571263577, -11.16473453929635440, 33.15142922261925662 ) ) ;
#52846=DIRECTION ( 'NONE',  ( -0.000000000000000000, -0.9848077530122085754, -0.1736481776669273613 ) ) ;
#52848=CARTESIAN_POINT ( 'NONE',  ( 11.53846153846141753, -3.835265460704628371, 33.15142922262033665 ) ) ;
#52849=DIRECTION ( 'NONE',  ( -0.000000000000000000, -0.6427876096865404731, -0.7660444431189771253 ) ) ;
#52851=FACE_BOUND ( 'NONE', #45207, .T. ) ;
#52852=ORIENTED_EDGE ( 'NONE', *, *, #77415, .F. ) ;
#52853=VERTEX_POINT ( 'NONE', #42472 ) ;
#52854=CARTESIAN_POINT ( 'NONE',  ( 4.946232473812767871, -2.295517848115769421, 30.44137282052136939 ) ) ;
#52855=VERTEX_POINT ( 'NONE', #29838 ) ;
#52856=FACE_BOUND ( 'NONE', #13917, .T. ) ;
#52857=CARTESIAN_POINT ( 'NONE',  ( 7.623227628637698317, -11.76352882383564769, 32.36236540154569497 ) ) ;
#52858=DIRECTION ( 'NONE',  ( -0.000000000000000000, -0.000000000000000000, -1.000000000000000000 ) ) ;
#52859=EDGE_LOOP ( 'NONE', ( #45070, #73674 ) ) ;
#52862=AXIS2_PLACEMENT_3D ( 'NONE', #83715, #89149, #69739 ) ;
#52863=FACE_OUTER_BOUND ( 'NONE', #8647, .T. ) ;
#52864=ORIENTED_EDGE ( 'NONE', *, *, #85186, .F. ) ;
#52865=CARTESIAN_POINT ( 'NONE',  ( -6.923076923077044142, -2.892918686052165622, 31.69288490824153470 ) ) ;
#52866=CARTESIAN_POINT ( 'NONE',  ( -2.980769230767794653, -7.500000000000155431, 34.75000000000007105 ) ) ;
#52867=CARTESIAN_POINT ( 'NONE',  ( -0.4615384615384611200, -8.564572088678739092, 35.78748833219616898 ) ) ;
#52868=ORIENTED_EDGE ( 'NONE', *, *, #35494, .F. ) ;
#52869=CARTESIAN_POINT ( 'NONE',  ( -4.153846153846152411, -12.10708131394839349, 31.69288490824020244 ) ) ;
#52870=CARTESIAN_POINT ( 'NONE',  ( -16.82697755857493149, -11.86320923018887541, 32.19269448109604781 ) ) ;
#52871=ORIENTED_EDGE ( 'NONE', *, *, #76937, .F. ) ;
#52872=CARTESIAN_POINT ( 'NONE',  ( 0.2380535178145126440, -9.331801661448606566, 34.40259984581193464 ) ) ;
#52873=CARTESIAN_POINT ( 'NONE',  ( -12.46153846153846168, -2.538708090699994813, 30.37095296980875503 ) ) ;
#52874=DIRECTION ( 'NONE',  ( -0.000000000000000000, -0.7660444431189791237, -0.6427876096865379196 ) ) ;
#52875=B_SPLINE_CURVE_WITH_KNOTS ( 'NONE', 3,
 ( #11564, #74594, #4807, #33606, #53871, #32707, #26847, #25514, #80468, #52971 ),
 .UNSPECIFIED., .F., .F.,
 ( 4, 2, 2, 2, 4 ),
 ( 0.0007817359430256320659, 0.0009771253907249989254, 0.001172514838424365676, 0.001367904286123732428, 0.001563293733823099179 ),
 .UNSPECIFIED. ) ;
#52876=CARTESIAN_POINT ( 'NONE',  ( 15.16468685140909400, -12.62096338111211580, 30.90682066428152908 ) ) ;
#52877=CARTESIAN_POINT ( 'NONE',  ( -3.230769230769229949, -6.435427911321262684, 35.78748833219616898 ) ) ;
#52878=DIRECTION ( 'NONE',  ( -0.000000000000000000, 0.6427876096865404731, -0.7660444431189771253 ) ) ;
#52881=CARTESIAN_POINT ( 'NONE',  ( 8.769230769230768274, -12.10708131394839349, 31.69288490824020244 ) ) ;
#52882=CARTESIAN_POINT ( 'NONE',  ( 11.53846153846153832, -11.91647553114624181, 32.58852847137148245 ) ) ;
#52884=VERTEX_POINT ( 'NONE', #69931 ) ;
#52885=CARTESIAN_POINT ( 'NONE',  ( 5.076923076922953193, -6.835583212225970762, 34.95778746994575670 ) ) ;
#52886=ORIENTED_EDGE ( 'NONE', *, *, #62398, .F. ) ;
#52888=DIRECTION ( 'NONE',  ( 0.000000000000000000, 0.1736481776669275834, 0.9848077530122086864 ) ) ;
#52889=VERTEX_POINT ( 'NONE', #9133 ) ;
#52890=CARTESIAN_POINT ( 'NONE',  ( 17.75000000000000000, -7.500000000000001776, 34.75000000000000000 ) ) ;
#52893=CARTESIAN_POINT ( 'NONE',  ( -18.06527000055631760, -12.16647553114622049, 32.15551576947930812 ) ) ;
#52894=CARTESIAN_POINT ( 'NONE',  ( -2.980823712421088789, -9.272278438253398036, 34.42582936511637826 ) ) ;
#52896=VECTOR ( 'NONE', #28752, 999.9999999999998863 ) ;
#52897=CARTESIAN_POINT ( 'NONE',  ( -5.207071046654769830, -3.625366637846544560, 33.29286588640298561 ) ) ;
#52898=CARTESIAN_POINT ( 'NONE',  ( -7.846153846153844924, -2.721908614388771852, 31.22303859784724978 ) ) ;
#52899=LINE ( 'NONE', #80398, #52577 ) ;
#52901=CARTESIAN_POINT ( 'NONE',  ( 5.299702745901138101, -3.020022701398814569, 32.48759521482552515 ) ) ;
#52902=CARTESIAN_POINT ( 'NONE',  ( -4.284536756956460302, -11.93127051446800024, 32.56575433478200665 ) ) ;
#52903=AXIS2_PLACEMENT_3D ( 'NONE', #88399, #54128, #17703 ) ;
#52905=EDGE_LOOP ( 'NONE', ( #21205, #16723, #5756, #69360 ) ) ;
#52906=VERTEX_POINT ( 'NONE', #15444 ) ;
#52907=CARTESIAN_POINT ( 'NONE',  ( -8.899377978668987055, -12.45813303252208648, 30.39737893381572675 ) ) ;
#52908=CARTESIAN_POINT ( 'NONE',  ( -14.08468095607945791, -8.239487800360276282, 34.69522927552633718 ) ) ;
#52909=CARTESIAN_POINT ( 'NONE',  ( -2.437840277424001556, -2.373036134822904319, 30.88089517874952250 ) ) ;
#52910=CYLINDRICAL_SURFACE ( 'NONE', #64248, 0.2499999999999973355 ) ;
#52911=CARTESIAN_POINT ( 'NONE',  ( 8.545745825506822158, -4.386631170607603991, 33.66268669641500111 ) ) ;
#52912=FACE_OUTER_BOUND ( 'NONE', #7236, .T. ) ;
#52913=AXIS2_PLACEMENT_3D ( 'NONE', #53658, #32495, #52761 ) ;
#52914=EDGE_LOOP ( 'NONE', ( #88776, #53971 ) ) ;
#52915=CARTESIAN_POINT ( 'NONE',  ( 1.134592147322421862, -5.056417327199099532, 34.11270091957321426 ) ) ;
#52916=ORIENTED_EDGE ( 'NONE', *, *, #23547, .F. ) ;
#52918=EDGE_LOOP ( 'NONE', ( #42980, #28643 ) ) ;
#52919=CARTESIAN_POINT ( 'NONE',  ( -9.627052552794857831, -3.083524468853784839, 32.58852847137153930 ) ) ;
#52920=EDGE_CURVE ( 'NONE', #67556, #56376, #73703, .T. ) ;
#52922=CARTESIAN_POINT ( 'NONE',  ( -4.219928533206288357, -12.62096338111211580, 30.90682066428152197 ) ) ;
#52923=VECTOR ( 'NONE', #21462, 1000.000000000000000 ) ;
#52924=EDGE_CURVE ( 'NONE', #47721, #31669, #83464, .T. ) ;
#52925=CARTESIAN_POINT ( 'NONE',  ( 1.161688425708537808, -11.43668979543635089, 33.22377378376089752 ) ) ;
#52926=CARTESIAN_POINT ( 'NONE',  ( 13.38461538461526423, -5.941354392335915335, 34.76329471203413846 ) ) ;
#52927=ORIENTED_EDGE ( 'NONE', *, *, #57838, .T. ) ;
#52928=EDGE_LOOP ( 'NONE', ( #58014, #36219 ) ) ;
#52929=ORIENTED_EDGE ( 'NONE', *, *, #39422, .T. ) ;
#52930=EDGE_CURVE ( 'NONE', #32624, #82469, #636, .T. ) ;
#52931=CYLINDRICAL_SURFACE ( 'NONE', #35800, 0.2500000000000004996 ) ;
#52932=CARTESIAN_POINT ( 'NONE',  ( -0.4615384615385840772, -10.33852847137269571, 34.16647553114546554 ) ) ;
#52933=CARTESIAN_POINT ( 'NONE',  ( 4.403791563224197070, -3.520799739797213501, 33.17531984108286025 ) ) ;
#52934=B_SPLINE_CURVE_WITH_KNOTS ( 'NONE', 3,
 ( #69400, #88807, #82919, #27524, #68076, #28869 ),
 .UNSPECIFIED., .F., .F.,
 ( 4, 2, 4 ),
 ( 0.000000000000000000, 0.0001954784845028902692, 0.0003909569690057805385 ),
 .UNSPECIFIED. ) ;
#52935=CARTESIAN_POINT ( 'NONE',  ( 1.134592147322421862, -3.711651800289232028, 33.01384336483936011 ) ) ;
#52936=VECTOR ( 'NONE', #70490, 1000.000000000000114 ) ;
#52937=LINE ( 'NONE', #16944, #82599 ) ;
#52938=ORIENTED_EDGE ( 'NONE', *, *, #67392, .T. ) ;
#52939=ORIENTED_EDGE ( 'NONE', *, *, #55342, .F. ) ;
#52940=CARTESIAN_POINT ( 'NONE',  ( 4.853438152358744873, -10.23692288466677880, 34.23039457007281072 ) ) ;
#52943=ORIENTED_EDGE ( 'NONE', *, *, #3609, .T. ) ;
#52944=CARTESIAN_POINT ( 'NONE',  ( -12.46153846153858424, -11.67786785259630911, 32.92929555188603530 ) ) ;
#52945=CARTESIAN_POINT ( 'NONE',  ( 8.069529786852024600, -2.501478030877322567, 29.88021232661721172 ) ) ;
#52947=EDGE_CURVE ( 'NONE', #54362, #88546, #81200, .T. ) ;
#52948=EDGE_LOOP ( 'NONE', ( #27268, #48240, #5533, #6491 ) ) ;
#52949=VECTOR ( 'NONE', #36651, 999.9999999999998863 ) ;
#52950=B_SPLINE_CURVE_WITH_KNOTS ( 'NONE', 3,
 ( #49331, #82686, #42141, #70038, #7902, #83576, #76808, #75037, #20955, #14660 ),
 .UNSPECIFIED., .F., .F.,
 ( 4, 2, 2, 2, 4 ),
 ( 0.0007817246256747530271, 0.0009771112852218978746, 0.001172497944769042939, 0.001367884604316188003, 0.001563271263863332851 ),
 .UNSPECIFIED. ) ;
#52951=EDGE_CURVE ( 'NONE', #31266, #85917, #32862, .T. ) ;
#52952=CARTESIAN_POINT ( 'NONE',  ( -9.692307692307691624, -12.78798330534103123, 29.99999999999997868 ) ) ;
#52953=ORIENTED_EDGE ( 'NONE', *, *, #238, .F. ) ;
#52954=CARTESIAN_POINT ( 'NONE',  ( 2.438484115517096207, -8.999086150933472084, 34.52020707165672064 ) ) ;
#52956=B_SPLINE_CURVE_WITH_KNOTS ( 'NONE', 3,
 ( #27208, #82163, #47916, #626, #83046, #21332, #14578, #7826, #35291, #62748 ),
 .UNSPECIFIED., .F., .F.,
 ( 4, 2, 2, 2, 4 ),
 ( 0.000000000000000000, 0.0001954311564186871184, 0.0003908623128373742367, 0.0005862934692560614093, 0.0007817246256747484735 ),
 .UNSPECIFIED. ) ;
#52957=FACE_BOUND ( 'NONE', #18482, .T. ) ;
#52959=CARTESIAN_POINT ( 'NONE',  ( 10.61538461538461675, -10.67929555188718282, 33.92786785259544047 ) ) ;
#52960=EDGE_CURVE ( 'NONE', #27628, #49317, #57572, .T. ) ;
#52961=DIRECTION ( 'NONE',  ( -0.000000000000000000, -0.000000000000000000, -1.000000000000000000 ) ) ;
#52963=EDGE_CURVE ( 'NONE', #46553, #59465, #28558, .T. ) ;
#52964=DIRECTION ( 'NONE',  ( -0.000000000000000000, -0.8660254037844399289, -0.4999999999999980016 ) ) ;
#52965=CARTESIAN_POINT ( 'NONE',  ( 15.16549878480846125, -4.481592998940162609, 33.73612834413957984 ) ) ;
#52966=CARTESIAN_POINT ( 'NONE',  ( 9.692307692307695177, -9.819645486525091727, 36.12317359536749706 ) ) ;
#52967=EDGE_LOOP ( 'NONE', ( #42551, #76718, #21080, #23325 ) ) ;
#52968=CARTESIAN_POINT ( 'NONE',  ( -18.06527000055631405, -12.70778746994557551, 30.41441678777548319 ) ) ;
#52969=CYLINDRICAL_SURFACE ( 'NONE', #88639, 0.2499999999999994726 ) ;
#52970=CARTESIAN_POINT ( 'NONE',  ( 14.55769230769231015, -2.249999999999998668, 29.75000000000000355 ) ) ;
#52971=CARTESIAN_POINT ( 'NONE',  ( 7.846153846153846700, -3.050289026998446396, 32.03036669348365706 ) ) ;
#52972=FACE_BOUND ( 'NONE', #76704, .T. ) ;
#52973=CARTESIAN_POINT ( 'NONE',  ( 1.514662819865838062, -7.723484941389743952, 34.99544897038808955 ) ) ;
#52974=CARTESIAN_POINT ( 'NONE',  ( -15.23076923076922995, -11.16473453929635440, 33.15142922261926373 ) ) ;
#52975=CARTESIAN_POINT ( 'NONE',  ( -39.05038313613820122, -2.249999999999998668, 29.75000000000000355 ) ) ;
#52976=CARTESIAN_POINT ( 'NONE',  ( -17.77698864838715309, -11.24521262558773493, 33.06293181088030053 ) ) ;
#52977=FACE_OUTER_BOUND ( 'NONE', #44083, .T. ) ;
#52978=FACE_OUTER_BOUND ( 'NONE', #57812, .T. ) ;
#52979=CARTESIAN_POINT ( 'NONE',  ( 17.99999999999987566, -4.320704448113951379, 33.92786785259630022 ) ) ;
#52982=CARTESIAN_POINT ( 'NONE',  ( 10.36540787133602848, -12.01397095200674059, 32.43157075238190146 ) ) ;
#52983=EDGE_LOOP ( 'NONE', ( #77854, #13080, #26973, #33027, #31051, #50914 ) ) ;
#52984=CARTESIAN_POINT ( 'NONE',  ( 0.2386122440223136798, -6.503392248772476236, 34.64988816332204635 ) ) ;
#52985=CARTESIAN_POINT ( 'NONE',  ( -4.153846153846273204, -12.27809138561165270, 31.22303859784587132 ) ) ;
#52987=CARTESIAN_POINT ( 'NONE',  ( -2.307692307692305711, -11.69971097300155272, 32.46337939537588113 ) ) ;
#52988=CARTESIAN_POINT ( 'NONE',  ( -10.39260494640654819, -12.11081565061824250, 32.26097654155340422 ) ) ;
#52989=CARTESIAN_POINT ( 'NONE',  ( -12.68446542044531178, -6.459968553980841577, 34.89616026154728701 ) ) ;
#52991=CARTESIAN_POINT ( 'NONE',  ( 2.307692307692187583, -11.94971097300221174, 32.03036669348237098 ) ) ;
#52992=CARTESIAN_POINT ( 'NONE',  ( 8.638540166120462160, -2.494641256782728966, 31.33461815524612959 ) ) ;
#52993=CARTESIAN_POINT ( 'NONE',  ( -12.23852561744506851, -9.172514111537584114, 34.72667873470787470 ) ) ;
#52994=CARTESIAN_POINT ( 'NONE',  ( 5.076923076922953193, -9.528491918059723176, 34.59228464037033035 ) ) ;
#52995=DIRECTION ( 'NONE',  ( -0.000000000000000000, -0.3420201433256694346, -0.9396926207859080948 ) ) ;
#52996=CARTESIAN_POINT ( 'NONE',  ( -11.53846153846153655, -9.780366693483667717, 34.19971097300155094 ) ) ;
#52997=B_SPLINE_CURVE_WITH_KNOTS ( 'NONE', 3,
 ( #36460, #21165, #63915, #29271, #63478, #63022, #49533, #20727, #62155, #2213 ),
 .UNSPECIFIED., .F., .F.,
 ( 4, 2, 2, 2, 4 ),
 ( 0.000000000000000000, 0.0001954311564186868744, 0.0003908623128373737488, 0.0005862934692560606504, 0.0007817246256747474977 ),
 .UNSPECIFIED. ) ;
#52998=EDGE_CURVE ( 'NONE', #72857, #798, #38818, .T. ) ;
#52999=CARTESIAN_POINT ( 'NONE',  ( 9.942307692307631228, -7.565270445406050648, 34.75000000000000000 ) ) ;
#53000=CARTESIAN_POINT ( 'NONE',  ( -11.31568199719312773, -10.81320215134717344, 33.49497208177562868 ) ) ;
#53001=VERTEX_POINT ( 'NONE', #32491 ) ;
#53002=DIRECTION ( 'NONE',  ( 0.000000000000000000, 0.8660254037844377084, 0.5000000000000015543 ) ) ;
#53003=CYLINDRICAL_SURFACE ( 'NONE', #22997, 0.2500000000000004996 ) ;
#53005=CARTESIAN_POINT ( 'NONE',  ( 6.065255571276025215, -4.481592998940251427, 33.73612834413965089 ) ) ;
#53006=CARTESIAN_POINT ( 'NONE',  ( 17.07692307692307665, -4.945431358278436385, 36.03766855953609394 ) ) ;
#53007=ORIENTED_EDGE ( 'NONE', *, *, #48921, .T. ) ;
#53008=CARTESIAN_POINT ( 'NONE',  ( 2.307692307692309264, -6.386643153685126251, 34.62446782046654192 ) ) ;
#53010=CARTESIAN_POINT ( 'NONE',  ( 7.912221179503920787, -2.486705287966279876, 31.30864560766543647 ) ) ;
#53012=CARTESIAN_POINT ( 'NONE',  ( -9.822998295417999515, -11.37499894934982692, 33.29245874905763003 ) ) ;
#53013=CARTESIAN_POINT ( 'NONE',  ( 4.023698944407932743, -8.587444163452046197, 34.63053765926554206 ) ) ;
#53014=CARTESIAN_POINT ( 'NONE',  ( -17.20739826199879730, -7.276987145209182550, 34.99546412871779211 ) ) ;
#53015=EDGE_CURVE ( 'NONE', #327, #85237, #84392, .T. ) ;
#53016=CARTESIAN_POINT ( 'NONE',  ( -39.05038313613820122, -2.249999999999998668, 29.75000000000000355 ) ) ;
#53017=ORIENTED_EDGE ( 'NONE', *, *, #30527, .F. ) ;
#53018=AXIS2_PLACEMENT_3D ( 'NONE', #53559, #45465, #59432 ) ;
#53019=DIRECTION ( 'NONE',  ( 0.000000000000000000, 0.7660444431189807890, 0.6427876096865361433 ) ) ;
#53022=CARTESIAN_POINT ( 'NONE',  ( 8.545745844666440050, -3.562934362175799841, 33.22335522853832401 ) ) ;
#53023=ORIENTED_EDGE ( 'NONE', *, *, #7468, .T. ) ;
#53024=ORIENTED_EDGE ( 'NONE', *, *, #84053, .T. ) ;
#53025=VERTEX_POINT ( 'NONE', #4123 ) ;
#53026=EDGE_CURVE ( 'NONE', #45061, #63264, #37153, .T. ) ;
#53027=CARTESIAN_POINT ( 'NONE',  ( -16.28453675695646652, -3.338472653186243200, 32.95098750199972670 ) ) ;
#53029=EDGE_CURVE ( 'NONE', #36439, #62255, #85496, .T. ) ;
#53030=CARTESIAN_POINT ( 'NONE',  ( -9.442362282929646966, -12.68172785388650681, 30.59649109432439218 ) ) ;
#53031=CARTESIAN_POINT ( 'NONE',  ( -17.01085472592063752, -4.786620604624113540, 33.94971097300155805 ) ) ;
#53032=ORIENTED_EDGE ( 'NONE', *, *, #15459, .T. ) ;
#53033=B_SPLINE_CURVE_WITH_KNOTS ( 'NONE', 3,
 ( #12106, #39583, #87781, #42673, #70133, #56624, #8444, #89104, #48522, #35916 ),
 .UNSPECIFIED., .F., .F.,
 ( 4, 2, 2, 2, 4 ),
 ( 0.000000000000000000, 0.0001954311564186883110, 0.0003908623128373766220, 0.0005862934692560648788, 0.0007817246256747532440 ),
 .UNSPECIFIED. ) ;
#53035=EDGE_CURVE ( 'NONE', #7863, #1158, #44627, .T. ) ;
#53036=ORIENTED_EDGE ( 'NONE', *, *, #21023, .F. ) ;
#53037=CARTESIAN_POINT ( 'NONE',  ( 15.23076923076923173, -4.786620604624113540, 33.94971097300155094 ) ) ;
#53038=ORIENTED_EDGE ( 'NONE', *, *, #37201, .T. ) ;
#53039=CARTESIAN_POINT ( 'NONE',  ( -16.37733107841048863, -12.47654668319379567, 31.42292124445336654 ) ) ;
#53040=AXIS2_PLACEMENT_3D ( 'NONE', #50651, #24515, #78130 ) ;
#53041=CARTESIAN_POINT ( 'NONE',  ( 15.23076923076923173, -3.050289026998446396, 32.03036669348365706 ) ) ;
#53042=EDGE_CURVE ( 'NONE', #60227, #28663, #44655, .T. ) ;
#53043=LINE ( 'NONE', #58916, #72347 ) ;
#53044=CARTESIAN_POINT ( 'NONE',  ( 13.63466980452883526, -10.06805714834173493, 34.32951233291982618 ) ) ;
#53046=VERTEX_POINT ( 'NONE', #51857 ) ;
#53047=ORIENTED_EDGE ( 'NONE', *, *, #34481, .T. ) ;
#53048=ORIENTED_EDGE ( 'NONE', *, *, #38115, .T. ) ;
#53049=CARTESIAN_POINT ( 'NONE',  ( -10.68065461594093435, -11.06231777344662781, 33.60647404775220082 ) ) ;
#53050=CARTESIAN_POINT ( 'NONE',  ( 8.899756470994335089, -2.619367082507849442, 30.83698974864643461 ) ) ;
#53051=ORIENTED_EDGE ( 'NONE', *, *, #11760, .F. ) ;
#53052=CARTESIAN_POINT ( 'NONE',  ( 16.82694633287449193, -5.643011162660950042, 34.66104346484419096 ) ) ;
#53054=EDGE_CURVE ( 'NONE', #879, #80092, #79354, .T. ) ;
#53055=CARTESIAN_POINT ( 'NONE',  ( 13.63461538461538680, -2.499999999999998668, 29.75000000000000355 ) ) ;
#53056=FACE_OUTER_BOUND ( 'NONE', #13622, .T. ) ;
#53057=CARTESIAN_POINT ( 'NONE',  ( 9.019176287578909879, -5.852078868378309373, 34.47109172314383585 ) ) ;
#53058=FACE_BOUND ( 'NONE', #87926, .T. ) ;
#53059=LINE ( 'NONE', #38670, #87381 ) ;
#53060=DIRECTION ( 'NONE',  ( -0.000000000000000000, 0.6427876096865404731, -0.7660444431189771253 ) ) ;
#53061=CARTESIAN_POINT ( 'NONE',  ( 11.60452988946397923, -12.37446782046654192, 30.86335684631486842 ) ) ;
#53063=FACE_OUTER_BOUND ( 'NONE', #80071, .T. ) ;
#53064=VECTOR ( 'NONE', #17943, 1000.000000000000114 ) ;
#53065=FACE_OUTER_BOUND ( 'NONE', #54911, .T. ) ;
#53066=CARTESIAN_POINT ( 'NONE',  ( 7.173076923076926015, -2.499999999999999112, 29.81604066197450109 ) ) ;
#53067=ORIENTED_EDGE ( 'NONE', *, *, #2973, .T. ) ;
#53069=DIRECTION ( 'NONE',  ( -0.000000000000000000, 0.7660444431189791237, -0.6427876096865379196 ) ) ;
#53070=CARTESIAN_POINT ( 'NONE',  ( -13.25408994638174143, -4.299079248970732792, 33.91157788607253565 ) ) ;
#53071=VERTEX_POINT ( 'NONE', #35942 ) ;
#53072=ORIENTED_EDGE ( 'NONE', *, *, #7656, .T. ) ;
#53075=CARTESIAN_POINT ( 'NONE',  ( 16.08857570788537572, -3.835265460703609186, 33.15142922261924241 ) ) ;
#53077=ORIENTED_EDGE ( 'NONE', *, *, #71798, .F. ) ;
#53079=CARTESIAN_POINT ( 'NONE',  ( -1.384615384615505151, -11.94971097300221174, 32.03036669348237098 ) ) ;
#53080=DIRECTION ( 'NONE',  ( -0.000000000000000000, -0.000000000000000000, -1.000000000000000000 ) ) ;
#53081=CARTESIAN_POINT ( 'NONE',  ( -1.384615384615506484, -12.51329471203414379, 31.30864560766407578 ) ) ;
#53082=CARTESIAN_POINT ( 'NONE',  ( 11.53846153846153832, -2.708943851104267164, 35.45975837776705220 ) ) ;
#53085=CARTESIAN_POINT ( 'NONE',  ( 7.846153846153846700, -6.681629849574314051, 35.83090037661290239 ) ) ;
#53086=EDGE_CURVE ( 'NONE', #10442, #61210, #21530, .T. ) ;
#53087=B_SPLINE_CURVE_WITH_KNOTS ( 'NONE', 3,
 ( #66182, #23419, #78364, #45019, #37826, #79268, #86024, #31518, #4493, #58983 ),
 .UNSPECIFIED., .F., .F.,
 ( 4, 2, 2, 2, 4 ),
 ( 0.000000000000000000, 0.0001954311564186871184, 0.0003908623128373742367, 0.0005862934692560614093, 0.0007817246256747484735 ),
 .UNSPECIFIED. ) ;
#53089=EDGE_LOOP ( 'NONE', ( #39712, #60593 ) ) ;
#53090=B_SPLINE_CURVE_WITH_KNOTS ( 'NONE', 3,
 ( #55933, #42437, #63126, #1441, #28931, #48288, #75761, #56387, #14066, #83872 ),
 .UNSPECIFIED., .F., .F.,
 ( 4, 2, 2, 2, 4 ),
 ( 0.000000000000000000, 0.0001954339881912775425, 0.0003908679763825550850, 0.0005863019645738326005, 0.0007817359527651101701 ),
 .UNSPECIFIED. ) ;
#53091=ORIENTED_EDGE ( 'NONE', *, *, #51063, .F. ) ;
#53092=CARTESIAN_POINT ( 'NONE',  ( 5.011653076366754611, -11.06231777344662781, 33.60647404775220082 ) ) ;
#53093=EDGE_CURVE ( 'NONE', #24465, #10994, #40353, .T. ) ;
#53094=CARTESIAN_POINT ( 'NONE',  ( 7.146088274689775588, -12.15243808032446005, 31.58219941686247978 ) ) ;
#53095=FACE_OUTER_BOUND ( 'NONE', #3774, .T. ) ;
#53097=CARTESIAN_POINT ( 'NONE',  ( -3.480745961711583902, -5.728515186090277211, 34.42611988154120439 ) ) ;
#53099=CYLINDRICAL_SURFACE ( 'NONE', #54678, 0.2499999999999994726 ) ;
#53100=CYLINDRICAL_SURFACE ( 'NONE', #74794, 0.2500000000000012212 ) ;
#53101=CARTESIAN_POINT ( 'NONE',  ( -13.60744207709438847, -7.369208160676171460, 34.74850200257122879 ) ) ;
#53102=CARTESIAN_POINT ( 'NONE',  ( -12.46153846153846168, -1.951392089020283160, 34.73218667398347748 ) ) ;
#53104=CARTESIAN_POINT ( 'NONE',  ( 13.45068271796546178, -2.486705287966280320, 31.30864560766543647 ) ) ;
#53105=CARTESIAN_POINT ( 'NONE',  ( -18.00000000000012079, -12.16647553114689906, 32.15551576947799362 ) ) ;
#53107=CARTESIAN_POINT ( 'NONE',  ( 7.912221179503920787, -8.164416787775445883, 34.95778746994558617 ) ) ;
#53108=CARTESIAN_POINT ( 'NONE',  ( -6.700297254098854793, -3.563462043263029955, 33.22394488606062879 ) ) ;
#53109=CARTESIAN_POINT ( 'NONE',  ( -15.45369544828537656, -9.886141570436013382, 34.14413921362392301 ) ) ;
#53110=ORIENTED_EDGE ( 'NONE', *, *, #41889, .F. ) ;
#53112=CARTESIAN_POINT ( 'NONE',  ( 8.900021210197715860, -4.684288915650983043, 34.18129842949671371 ) ) ;
#53113=EDGE_CURVE ( 'NONE', #3961, #75689, #1252, .T. ) ;
#53114=DIRECTION ( 'NONE',  ( 0.000000000000000000, 0.9396926207859126468, -0.3420201433256571111 ) ) ;
#53115=CARTESIAN_POINT ( 'NONE',  ( 5.869852030268300602, -2.647304123082328875, 31.75400227202885262 ) ) ;
#53117=B_SPLINE_CURVE_WITH_KNOTS ( 'NONE', 3,
 ( #71263, #36610, #45129, #57319, #84817, #24409, #79371, #72603, #23093, #78034 ),
 .UNSPECIFIED., .F., .F.,
 ( 4, 2, 2, 2, 4 ),
 ( 0.000000000000000000, 0.0001954339857564073659, 0.0003908679715128147319, 0.0005863019572692221250, 0.0007817359430256294638 ),
 .UNSPECIFIED. ) ;
#53118=ADVANCED_FACE ( 'NONE', ( #35491 ), #49004, .F. ) ;
#53119=CARTESIAN_POINT ( 'NONE',  ( -20.74999999999999645, -7.500000000000000000, 32.75000000000000000 ) ) ;
#53120=CARTESIAN_POINT ( 'NONE',  ( -17.75005448165186195, -10.76462480002816235, 33.53768742498949962 ) ) ;
#53122=ORIENTED_EDGE ( 'NONE', *, *, #16286, .T. ) ;
#53125=VERTEX_POINT ( 'NONE', #55753 ) ;
#53127=CARTESIAN_POINT ( 'NONE',  ( -7.146561847641254239, -11.60425143139329940, 33.02411095842164457 ) ) ;
#53128=ORIENTED_EDGE ( 'NONE', *, *, #41473, .T. ) ;
#53129=CARTESIAN_POINT ( 'NONE',  ( 6.000000000000001776, -13.53365097954675988, 30.81389545987213552 ) ) ;
#53130=CARTESIAN_POINT ( 'NONE',  ( -7.623374304885435215, -11.89424750095246175, 32.13594075562311758 ) ) ;
#53131=B_SPLINE_CURVE_WITH_KNOTS ( 'NONE', 3,
 ( #18807, #38628, #39974, #86845, #12930, #53915, #33649, #45822, #47149, #67435 ),
 .UNSPECIFIED., .F., .F.,
 ( 4, 2, 2, 2, 4 ),
 ( 0.0007817359430256324996, 0.0009771253907249993591, 0.001172514838424366110, 0.001367904286123732861, 0.001563293733823099829 ),
 .UNSPECIFIED. ) ;
#53132=CARTESIAN_POINT ( 'NONE',  ( 17.01165307636676260, -6.835583212224500826, 34.95778746994557906 ) ) ;
#53133=ORIENTED_EDGE ( 'NONE', *, *, #51942, .F. ) ;
#53134=CARTESIAN_POINT ( 'NONE',  ( 0.3962684609821410797, -5.094484230520674117, 34.41647553114621161 ) ) ;
#53135=ORIENTED_EDGE ( 'NONE', *, *, #14678, .T. ) ;
#53136=B_SPLINE_CURVE_WITH_KNOTS ( 'NONE', 3,
 ( #44523, #43217, #72009, #72451, #57612, #31016, #85978, #51720, #79223, #17522 ),
 .UNSPECIFIED., .F., .F.,
 ( 4, 2, 2, 2, 4 ),
 ( 0.0007817359430256322827, 0.0009771253907249989254, 0.001172514838424365676, 0.001367904286123732428, 0.001563293733823099179 ),
 .UNSPECIFIED. ) ;
#53137=B_SPLINE_CURVE_WITH_KNOTS ( 'NONE', 3,
 ( #62736, #67740, #6045, #75382, #33515, #61852, #60972, #81704, #88478, #26747 ),
 .UNSPECIFIED., .F., .F.,
 ( 4, 2, 2, 2, 4 ),
 ( 0.000000000000000000, 0.0001954311564186862510, 0.0003908623128373725020, 0.0005862934692560588072, 0.0007817246256747450040 ),
 .UNSPECIFIED. ) ;
#53138=VERTEX_POINT ( 'NONE', #48545 ) ;
#53140=VECTOR ( 'NONE', #12409, 1000.000000000000000 ) ;
#53141=CARTESIAN_POINT ( 'NONE',  ( -0.4615384615384611200, -3.050289026998446396, 32.03036669348365706 ) ) ;
#53142=CARTESIAN_POINT ( 'NONE',  ( -20.99999999999999645, -4.249999999999999112, 29.75000000000000355 ) ) ;
#53143=CARTESIAN_POINT ( 'NONE',  ( 18.25005441991345734, -10.06805714834173138, 34.32951233291982618 ) ) ;
#53144=CARTESIAN_POINT ( 'NONE',  ( 8.096153846155266010, -7.500000000000154543, 35.00000000000007105 ) ) ;
#53145=CARTESIAN_POINT ( 'NONE',  ( -2.980714810855777497, -4.818054556918156983, 34.26375889529406749 ) ) ;
#53146=EDGE_CURVE ( 'NONE', #48673, #13156, #49882, .T. ) ;
#53147=CARTESIAN_POINT ( 'NONE',  ( -8.769230769230768274, -6.189225973068211317, 35.74407628777942847 ) ) ;
#53148=VECTOR ( 'NONE', #17508, 1000.000000000000000 ) ;
#53149=CARTESIAN_POINT ( 'NONE',  ( -0.2387587925603944505, -12.47679350104403007, 31.42216943046555855 ) ) ;
#53151=ORIENTED_EDGE ( 'NONE', *, *, #64839, .T. ) ;
#53152=ORIENTED_EDGE ( 'NONE', *, *, #75722, .F. ) ;
#53153=CARTESIAN_POINT ( 'NONE',  ( 3.296024802045255608, -3.835265460703683349, 33.15142922261929925 ) ) ;
#53154=ORIENTED_EDGE ( 'NONE', *, *, #11568, .T. ) ;
#53155=CARTESIAN_POINT ( 'NONE',  ( -14.08467946359890988, -10.77377354290276124, 33.85451476688484718 ) ) ;
#53156=CARTESIAN_POINT ( 'NONE',  ( -10.83886955910856464, -9.331801661448606566, 34.40259984581193464 ) ) ;
#53157=ORIENTED_EDGE ( 'NONE', *, *, #73893, .T. ) ;
#53159=B_SPLINE_CURVE_WITH_KNOTS ( 'NONE', 3,
 ( #1524, #23118, #71292, #85270, #77620, #76736, #9599, #15041, #29008, #56464 ),
 .UNSPECIFIED., .F., .F.,
 ( 4, 2, 2, 2, 4 ),
 ( 0.000000000000000000, 0.0001954311564186876876, 0.0003908623128373753751, 0.0005862934692560630356, 0.0007817246256747507503 ),
 .UNSPECIFIED. ) ;
#53160=VERTEX_POINT ( 'NONE', #816 ) ;
#53161=CARTESIAN_POINT ( 'NONE',  ( 17.07692307692307665, -9.780366693483667717, 34.19971097300155094 ) ) ;
#53162=ORIENTED_EDGE ( 'NONE', *, *, #11411, .T. ) ;
#53163=CARTESIAN_POINT ( 'NONE',  ( -18.22292695890684655, -9.172386477786394821, 34.72672124145550043 ) ) ;
#53164=B_SPLINE_CURVE_WITH_KNOTS ( 'NONE', 3,
 ( #54636, #20861, #6472, #61840, #82135, #62283, #33932, #21301, #13664, #48773 ),
 .UNSPECIFIED., .F., .F.,
 ( 4, 2, 2, 2, 4 ),
 ( 0.000000000000000000, 0.0001954339857564082062, 0.0003908679715128164124, 0.0005863019572692246186, 0.0007817359430256328248 ),
 .UNSPECIFIED. ) ;
#53166=DIRECTION ( 'NONE',  ( -0.000000000000000000, -0.7660444431189791237, -0.6427876096865379196 ) ) ;
#53168=CARTESIAN_POINT ( 'NONE',  ( 4.153846153846468603, -2.255955759149395501, 30.00000000000324363 ) ) ;
#53169=FACE_BOUND ( 'NONE', #66916, .T. ) ;
#53170=CARTESIAN_POINT ( 'NONE',  ( 17.07692307692295586, -6.835583212225970762, 34.95778746994575670 ) ) ;
#53171=CARTESIAN_POINT ( 'NONE',  ( 2.307692307692309264, -1.242168528481310874, 33.36296068462461051 ) ) ;
#53172=EDGE_CURVE ( 'NONE', #21818, #43106, #88715, .T. ) ;
#53173=CARTESIAN_POINT ( 'NONE',  ( 5.934749009838759193, -2.506253911140460477, 30.00000000000013856 ) ) ;
#53174=LINE ( 'NONE', #54961, #22982 ) ;
#53176=CARTESIAN_POINT ( 'NONE',  ( 17.32686859527121825, -9.272278438253401589, 34.42582936511637826 ) ) ;
#53178=EDGE_CURVE ( 'NONE', #38632, #8057, #75581, .T. ) ;
#53179=CARTESIAN_POINT ( 'NONE',  ( 1.634615384615401013, -2.249999999999999112, 29.81603969181031033 ) ) ;
#53180=ORIENTED_EDGE ( 'NONE', *, *, #60582, .F. ) ;
#53181=ORIENTED_EDGE ( 'NONE', *, *, #22774, .T. ) ;
#53182=CARTESIAN_POINT ( 'NONE',  ( -0.4615384615384611200, -8.973038597847269315, 34.52809138561121927 ) ) ;
#53183=CARTESIAN_POINT ( 'NONE',  ( -3.230769230769229949, -4.661471528628507777, 34.16647553114623292 ) ) ;
#53185=CARTESIAN_POINT ( 'NONE',  ( -4.023798718595700485, -7.723484941389743952, 34.99544897038808955 ) ) ;
#53186=CARTESIAN_POINT ( 'NONE',  ( -9.692307692307691624, -8.318370150425687726, 35.83090037661290239 ) ) ;
#53188=CARTESIAN_POINT ( 'NONE',  ( -18.00000000000000000, -10.67929555188718282, 33.92786785259543336 ) ) ;
#53189=EDGE_LOOP ( 'NONE', ( #46979, #69122 ) ) ;
#53190=CARTESIAN_POINT ( 'NONE',  ( 2.242421861731533017, -9.442884908240170461, 34.35708131394840592 ) ) ;
#53191=CARTESIAN_POINT ( 'NONE',  ( 11.40785117883701183, -7.722926236386453702, 34.74524107206102030 ) ) ;
#53192=CARTESIAN_POINT ( 'NONE',  ( -14.53061852520844965, -8.239355502252617924, 34.69524867566427417 ) ) ;
#53193=AXIS2_PLACEMENT_3D ( 'NONE', #72594, #10902, #2790 ) ;
#53194=CYLINDRICAL_SURFACE ( 'NONE', #6524, 0.2500000000000008882 ) ;
#53195=VERTEX_POINT ( 'NONE', #34607 ) ;
#53196=ADVANCED_FACE ( 'NONE', ( #383 ), #2138, .F. ) ;
#53197=ORIENTED_EDGE ( 'NONE', *, *, #40379, .T. ) ;
#53198=B_SPLINE_CURVE_WITH_KNOTS ( 'NONE', 3,
 ( #7291, #533, #28001, #7738, #20367, #47827, #8180, #19906, #35200, #75308 ),
 .UNSPECIFIED., .F., .F.,
 ( 4, 2, 2, 2, 4 ),
 ( 0.000000000000000000, 0.0001954339857564083146, 0.0003908679715128166293, 0.0005863019572692249439, 0.0007817359430256332585 ),
 .UNSPECIFIED. ) ;
#53199=AXIS2_PLACEMENT_3D ( 'NONE', #24625, #72805, #60623 ) ;
#53201=AXIS2_PLACEMENT_3D ( 'NONE', #56061, #81889, #32803 ) ;
#53202=ORIENTED_EDGE ( 'NONE', *, *, #62389, .T. ) ;
#53203=CARTESIAN_POINT ( 'NONE',  ( 0.6843180028068704956, -10.81320215134717344, 33.49497208177562868 ) ) ;
#53204=CARTESIAN_POINT ( 'NONE',  ( -7.846153846153965716, -5.219633306517616589, 34.19971097300220464 ) ) ;
#53205=ORIENTED_EDGE ( 'NONE', *, *, #70142, .T. ) ;
#53206=DIRECTION ( 'NONE',  ( -0.000000000000000000, -0.6427876096865404731, -0.7660444431189770143 ) ) ;
#53207=CARTESIAN_POINT ( 'NONE',  ( -5.076923076923075762, -2.721908614388771852, 31.22303859784724978 ) ) ;
#53208=DIRECTION ( 'NONE',  ( -0.000000000000000000, 0.3420201433256694346, -0.9396926207859080948 ) ) ;
#53211=CARTESIAN_POINT ( 'NONE',  ( -0.6850234052624084580, -11.41268669641500466, 32.86336882939237825 ) ) ;
#53212=ORIENTED_EDGE ( 'NONE', *, *, #3737, .F. ) ;
#53214=CARTESIAN_POINT ( 'NONE',  ( -7.623374304885437880, -10.11255958852956027, 34.01340905677048454 ) ) ;
#53215=ORIENTED_EDGE ( 'NONE', *, *, #68904, .F. ) ;
#53216=CARTESIAN_POINT ( 'NONE',  ( 4.153846153846032507, -3.300289026999228881, 32.46337939537708905 ) ) ;
#53217=CYLINDRICAL_SURFACE ( 'NONE', #57069, 0.2499999999999973355 ) ;
#53218=DIRECTION ( 'NONE',  ( -0.000000000000000000, -0.9848077530122086864, -0.1736481776669273613 ) ) ;
#53220=CARTESIAN_POINT ( 'NONE',  ( -4.087778820496076548, -4.661471528628508665, 34.16647553114624003 ) ) ;
#53221=LINE ( 'NONE', #19005, #62231 ) ;
#53223=ORIENTED_EDGE ( 'NONE', *, *, #15846, .F. ) ;
#53224=EDGE_CURVE ( 'NONE', #10043, #328, #77989, .T. ) ;
#53225=CARTESIAN_POINT ( 'NONE',  ( 15.23076923076911093, -8.613356846316285953, 34.62446782046622218 ) ) ;
#53226=CARTESIAN_POINT ( 'NONE',  ( -9.692307692307812417, -8.613356846316285953, 34.62446782046622218 ) ) ;
#53227=EDGE_CURVE ( 'NONE', #59485, #49728, #57527, .T. ) ;
#53228=ORIENTED_EDGE ( 'NONE', *, *, #28972, .F. ) ;
#53229=EDGE_LOOP ( 'NONE', ( #13163, #16222 ) ) ;
#53230=CARTESIAN_POINT ( 'NONE',  ( 9.915087361285758405, -3.563462043263030399, 33.22394488606062879 ) ) ;
#53231=CARTESIAN_POINT ( 'NONE',  ( -12.52762187249433978, -3.050289026998445951, 32.03036669348365706 ) ) ;
#53232=CARTESIAN_POINT ( 'NONE',  ( 13.31853197365950514, -3.513871655860377086, 32.76840700105978499 ) ) ;
#53233=CARTESIAN_POINT ( 'NONE',  ( -7.173053654019277303, -5.728515186090277211, 34.42611988154120439 ) ) ;
#53234=ADVANCED_FACE ( 'NONE', ( #36381 ), #72368, .F. ) ;
#53235=CARTESIAN_POINT ( 'NONE',  ( 7.145856464345329506, -5.913360116392398780, 34.49180327182771322 ) ) ;
#53236=DIRECTION ( 'NONE',  ( -0.000000000000000000, -0.1736481776669307198, -0.9848077530122080203 ) ) ;
#53237=ORIENTED_EDGE ( 'NONE', *, *, #27023, .T. ) ;
#53238=CARTESIAN_POINT ( 'NONE',  ( 5.869308533332440625, -3.530157926970578508, 32.79014554554150607 ) ) ;
#53239=EDGE_CURVE ( 'NONE', #6052, #76630, #41471, .T. ) ;
#53240=DIRECTION ( 'NONE',  ( -0.000000000000000000, 0.8660254037844397068, -0.4999999999999978906 ) ) ;
#53241=DIRECTION ( 'NONE',  ( 0.000000000000000000, 0.6427876096865368094, 0.7660444431189802339 ) ) ;
#53242=EDGE_LOOP ( 'NONE', ( #38318, #51091 ) ) ;
#53243=CARTESIAN_POINT ( 'NONE',  ( 13.38461538461526601, -6.879047030192662504, 34.71129190930017927 ) ) ;
#53244=ORIENTED_EDGE ( 'NONE', *, *, #57901, .F. ) ;
#53245=FACE_OUTER_BOUND ( 'NONE', #83668, .T. ) ;
#53247=CARTESIAN_POINT ( 'NONE',  ( -13.44993830010755609, -7.749976743299138882, 34.99404534957040624 ) ) ;
#53248=VERTEX_POINT ( 'NONE', #10240 ) ;
#53250=DIRECTION ( 'NONE',  ( -0.000000000000000000, 0.3420201433256694346, -0.9396926207859080948 ) ) ;
#53252=CARTESIAN_POINT ( 'NONE',  ( -8.769230769230768274, -2.517432740324522911, 35.29906147534542527 ) ) ;
#53253=CARTESIAN_POINT ( 'NONE',  ( -6.000000000000121680, -5.941354392335915335, 34.76329471203413846 ) ) ;
#53254=CARTESIAN_POINT ( 'NONE',  ( -4.946397638689432164, -8.630441415882550871, 34.87705825610312615 ) ) ;
#53255=ADVANCED_FACE ( 'NONE', ( #50315 ), #84578, .F. ) ;
#53256=EDGE_CURVE ( 'NONE', #11627, #6016, #16104, .T. ) ;
#53257=VERTEX_POINT ( 'NONE', #77799 ) ;
#53259=CARTESIAN_POINT ( 'NONE',  ( -5.076923076923075762, -6.343179335718451384, 34.87096338111211935 ) ) ;
#53260=ORIENTED_EDGE ( 'NONE', *, *, #75188, .T. ) ;
#53261=CARTESIAN_POINT ( 'NONE',  ( -14.98082382139119062, -6.653508905675592722, 34.93172785388651391 ) ) ;
#53262=ADVANCED_FACE ( 'NONE', ( #65603 ), #57969, .F. ) ;
#53263=CARTESIAN_POINT ( 'NONE',  ( -10.55012947587177941, -10.33852847137154107, 34.16647553114620450 ) ) ;
#53264=CARTESIAN_POINT ( 'NONE',  ( -14.30769230769242917, -10.33852847137269571, 34.16647553114546554 ) ) ;
#53265=LINE ( 'NONE', #5985, #32971 ) ;
#53266=CARTESIAN_POINT ( 'NONE',  ( 11.53846153846141576, -11.67786785259630911, 32.92929555188603530 ) ) ;
#53267=CARTESIAN_POINT ( 'NONE',  ( -0.4615384615384611200, -13.78497067705608181, 32.30358669280327177 ) ) ;
#53268=DIRECTION ( 'NONE',  ( 0.000000000000000000, 0.3420201433256641055, -0.9396926207859100932 ) ) ;
#53269=VECTOR ( 'NONE', #32206, 1000.000000000000000 ) ;
#53270=AXIS2_PLACEMENT_3D ( 'NONE', #6123, #50641, #29067 ) ;
#53271=ORIENTED_EDGE ( 'NONE', *, *, #995, .T. ) ;
#53272=ORIENTED_EDGE ( 'NONE', *, *, #24010, .T. ) ;
#53273=VERTEX_POINT ( 'NONE', #9785 ) ;
#53274=EDGE_LOOP ( 'NONE', ( #32424, #4836, #13289, #24207 ) ) ;
#53275=CARTESIAN_POINT ( 'NONE',  ( 2.307692307692309264, -4.786620604624113540, 33.94971097300155094 ) ) ;
#53276=CARTESIAN_POINT ( 'NONE',  ( -3.230769230769352962, -6.835583212225970762, 34.95778746994575670 ) ) ;
#53277=DIRECTION ( 'NONE',  ( -0.000000000000000000, 1.000000000000000000, -0.000000000000000000 ) ) ;
#53278=CARTESIAN_POINT ( 'NONE',  ( 4.826899852701616034, -11.56360843649121861, 33.07473185843129926 ) ) ;
#53281=CARTESIAN_POINT ( 'NONE',  ( -0.7115151924808161832, -11.79746400365624659, 32.30657167506340954 ) ) ;
#53282=CARTESIAN_POINT ( 'NONE',  ( -5.011667505647053211, -4.481592998940251427, 33.73612834413965089 ) ) ;
#53283=DIRECTION ( 'NONE',  ( -0.000000000000000000, 0.6427876096865404731, -0.7660444431189771253 ) ) ;
#53284=EDGE_LOOP ( 'NONE', ( #10300, #2010, #73421, #55271, #47962, #26588 ) ) ;
#53286=ORIENTED_EDGE ( 'NONE', *, *, #54246, .T. ) ;
#53287=CARTESIAN_POINT ( 'NONE',  ( -13.60810030917971858, -12.47654668319379567, 31.42292124445336654 ) ) ;
#53288=ORIENTED_EDGE ( 'NONE', *, *, #20116, .F. ) ;
#53289=DIRECTION ( 'NONE',  ( -0.000000000000000000, 0.9396926207859093161, -0.3420201433256663259 ) ) ;
#53290=LINE ( 'NONE', #576, #10289 ) ;
#53291=EDGE_CURVE ( 'NONE', #60920, #60370, #85896, .T. ) ;
#53293=CARTESIAN_POINT ( 'NONE',  ( -8.992157728137618378, -6.459968553980841577, 34.89616026154728701 ) ) ;
#53294=FACE_BOUND ( 'NONE', #10993, .T. ) ;
#53295=ORIENTED_EDGE ( 'NONE', *, *, #48054, .F. ) ;
#53296=B_SPLINE_CURVE_WITH_KNOTS ( 'NONE', 3,
 ( #16499, #10193, #64671, #57925, #85409, #71882, #80439, #66913, #13738, #81765 ),
 .UNSPECIFIED., .F., .F.,
 ( 4, 2, 2, 2, 4 ),
 ( 0.0007817359430256315238, 0.0009771253907249980580, 0.001172514838424364592, 0.001367904286123731127, 0.001563293733823097661 ),
 .UNSPECIFIED. ) ;
#53297=AXIS2_PLACEMENT_3D ( 'NONE', #66193, #39636, #40083 ) ;
#53298=ORIENTED_EDGE ( 'NONE', *, *, #68061, .T. ) ;
#53300=CARTESIAN_POINT ( 'NONE',  ( 5.076923076923075762, -12.78798330534102767, 29.49999999999997868 ) ) ;
#53302=FACE_BOUND ( 'NONE', #34916, .T. ) ;
#53303=CARTESIAN_POINT ( 'NONE',  ( -10.74553258511631348, -3.069018819979302926, 32.56621877034667278 ) ) ;
#53304=CARTESIAN_POINT ( 'NONE',  ( 15.10007862765892206, -6.369640206132551441, 34.87707690430378449 ) ) ;
#53305=ORIENTED_EDGE ( 'NONE', *, *, #11488, .T. ) ;
#53306=CARTESIAN_POINT ( 'NONE',  ( -2.307692307692305711, -1.466349020453238561, 30.81389545987213907 ) ) ;
#53307=CARTESIAN_POINT ( 'NONE',  ( -1.634592128663975297, -8.347322224742351082, 34.93158281831414769 ) ) ;
#53310=CARTESIAN_POINT ( 'NONE',  ( -7.846153846153844924, -8.164416787775445883, 34.95778746994557906 ) ) ;
#53312=CARTESIAN_POINT ( 'NONE',  ( 2.307692307692309264, -2.833524468853757305, 32.15551576947925838 ) ) ;
#53313=VERTEX_POINT ( 'NONE', #37245 ) ;
#53315=CARTESIAN_POINT ( 'NONE',  ( -2.531177251416253604, -11.41268669641500466, 32.86336882939237825 ) ) ;
#53316=CARTESIAN_POINT ( 'NONE',  ( -16.08777882049607655, -9.905515769479276145, 34.41647553114623292 ) ) ;
#53317=ORIENTED_EDGE ( 'NONE', *, *, #47863, .T. ) ;
#53318=CARTESIAN_POINT ( 'NONE',  ( 3.453548899747296730, -6.717445702608402236, 34.94155399931962336 ) ) ;
#53319=LINE ( 'NONE', #71810, #3738 ) ;
#53320=CARTESIAN_POINT ( 'NONE',  ( 5.869308533332443290, -8.999036380462719364, 34.52022231692819076 ) ) ;
#53321=CARTESIAN_POINT ( 'NONE',  ( -5.010854725920638408, -8.120952969808772792, 34.71129190929999453 ) ) ;
#53322=CARTESIAN_POINT ( 'NONE',  ( 8.769230769230645706, -4.320704448113951379, 33.92786785259630022 ) ) ;
#53323=CARTESIAN_POINT ( 'NONE',  ( -1.384615384615383471, -13.49023893513002648, 31.06009739812518688 ) ) ;
#53325=CARTESIAN_POINT ( 'NONE',  ( 9.942253101685738059, -4.932303261841489928, 34.32971442181322885 ) ) ;
#53326=AXIS2_PLACEMENT_3D ( 'NONE', #43563, #50310, #16097 ) ;
#53327=CARTESIAN_POINT ( 'NONE',  ( 10.86533002476265963, -9.357781135181031829, 34.66075350412533851 ) ) ;
#53330=VERTEX_POINT ( 'NONE', #17884 ) ;
#53331=EDGE_CURVE ( 'NONE', #87991, #52162, #25525, .T. ) ;
#53332=CARTESIAN_POINT ( 'NONE',  ( -12.59168567097668401, -8.587444163452046197, 34.63053765926554206 ) ) ;
#53333=EDGE_LOOP ( 'NONE', ( #9524, #9160, #66814, #39022 ) ) ;
#53334=VECTOR ( 'NONE', #43093, 1000.000000000000000 ) ;
#53335=VECTOR ( 'NONE', #80121, 1000.000000000000114 ) ;
#53336=ORIENTED_EDGE ( 'NONE', *, *, #58150, .F. ) ;
#53337=EDGE_CURVE ( 'NONE', #73147, #26379, #54382, .T. ) ;
#53338=CARTESIAN_POINT ( 'NONE',  ( -3.007989561791163613, -9.418065098278011860, 34.63729479722530158 ) ) ;
#53339=ORIENTED_EDGE ( 'NONE', *, *, #214, .F. ) ;
#53340=LINE ( 'NONE', #19123, #71423 ) ;
#53342=CARTESIAN_POINT ( 'NONE',  ( -17.93474442872397390, -6.026961402152790193, 34.52809138561124769 ) ) ;
#53343=CARTESIAN_POINT ( 'NONE',  ( 10.83839745947800992, -2.523321265292115534, 31.42251411153756990 ) ) ;
#53344=CARTESIAN_POINT ( 'NONE',  ( -0.3954701105360234892, -5.557115091759786019, 34.35708131394839882 ) ) ;
#53345=AXIS2_PLACEMENT_3D ( 'NONE', #56646, #84140, #62501 ) ;
#53346=B_SPLINE_CURVE_WITH_KNOTS ( 'NONE', 3,
 ( #30785, #87542, #51477, #19060, #80328, #72213, #4659, #87094, #44735, #59148 ),
 .UNSPECIFIED., .F., .F.,
 ( 4, 2, 2, 2, 4 ),
 ( 0.0007817359430256327164, 0.0009771253907249993591, 0.001172514838424366110, 0.001367904286123732861, 0.001563293733823099396 ),
 .UNSPECIFIED. ) ;
#53348=CARTESIAN_POINT ( 'NONE',  ( -15.29603923132555110, -5.094484230520674117, 34.41647553114621161 ) ) ;
#53349=CARTESIAN_POINT ( 'NONE',  ( 13.38461538461526601, -9.442884908241554243, 34.35708131394783038 ) ) ;
#53352=B_SPLINE_CURVE_WITH_KNOTS ( 'NONE', 3,
 ( #64211, #29563, #2511, #44378, #71866, #57463, #37638, #78184, #65099, #77737 ),
 .UNSPECIFIED., .F., .F.,
 ( 4, 2, 2, 2, 4 ),
 ( 0.000000000000000000, 0.0001954311564186879315, 0.0003908623128373758630, 0.0005862934692560637946, 0.0007817246256747517261 ),
 .UNSPECIFIED. ) ;
#53353=B_SPLINE_CURVE_WITH_KNOTS ( 'NONE', 3,
 ( #27058, #54519, #82012, #31, #47319, #54973, #5467, #66714, #67605, #20307 ),
 .UNSPECIFIED., .F., .F.,
 ( 4, 2, 2, 2, 4 ),
 ( 0.0007817359430256219828, 0.0009771253907249863487, 0.001172514838424350498, 0.001367904286123714647, 0.001563293733823079013 ),
 .UNSPECIFIED. ) ;
#53354=CARTESIAN_POINT ( 'NONE',  ( 17.32686848630112308, -2.341251567377310217, 30.72681386836322659 ) ) ;
#53355=CARTESIAN_POINT ( 'NONE',  ( -10.55019162708995850, -2.255955759149236073, 29.99999999999988987 ) ) ;
#53356=EDGE_CURVE ( 'NONE', #44478, #27810, #33973, .T. ) ;
#53357=CARTESIAN_POINT ( 'NONE',  ( 11.53846153846153832, -3.050289026998446396, 32.03036669348365706 ) ) ;
#53358=ORIENTED_EDGE ( 'NONE', *, *, #56925, .T. ) ;
#53359=EDGE_LOOP ( 'NONE', ( #58139, #51397, #3220, #86647, #7313, #66881 ) ) ;
#53360=CARTESIAN_POINT ( 'NONE',  ( 14.17754433796061875, -8.630895178749533159, 34.87696386517710323 ) ) ;
#53362=CARTESIAN_POINT ( 'NONE',  ( 9.692307692307695177, -10.89733346790207413, 36.13435417666054406 ) ) ;
#53363=CARTESIAN_POINT ( 'NONE',  ( -7.173053667125516952, -5.643011162660950042, 34.66104346484419096 ) ) ;
#53364=DIRECTION ( 'NONE',  ( -0.000000000000000000, 1.000000000000000000, 3.491481338843133355E-15 ) ) ;
#53365=EDGE_CURVE ( 'NONE', #56098, #39942, #80476, .T. ) ;
#53366=CARTESIAN_POINT ( 'NONE',  ( -16.37733109757010652, -9.331801661448606566, 34.40259984581193464 ) ) ;
#53367=EDGE_CURVE ( 'NONE', #26351, #17177, #60629, .T. ) ;
#53368=ADVANCED_FACE ( 'NONE', ( #66050 ), #32717, .F. ) ;
#53369=EDGE_LOOP ( 'NONE', ( #55934, #64339, #56864, #83545 ) ) ;
#53371=ORIENTED_EDGE ( 'NONE', *, *, #83385, .F. ) ;
#53372=VECTOR ( 'NONE', #4388, 1000.000000000000114 ) ;
#53374=CARTESIAN_POINT ( 'NONE',  ( 5.076923076923075762, -12.78798330534103123, 29.99999999999997868 ) ) ;
#53375=B_SPLINE_CURVE_WITH_KNOTS ( 'NONE', 3,
 ( #37564, #78553, #84447, #43883, #51963, #58280, #43447, #24053, #51501, #50185 ),
 .UNSPECIFIED., .F., .F.,
 ( 4, 2, 2, 2, 4 ),
 ( 0.0007817246256747524850, 0.0009771112852218972241, 0.001172497944769042072, 0.001367884604316186702, 0.001563271263863331550 ),
 .UNSPECIFIED. ) ;
#53376=CARTESIAN_POINT ( 'NONE',  ( 5.750000000000002665, -7.500000000000001776, 34.75000000000000000 ) ) ;
#53379=LINE ( 'NONE', #68234, #53835 ) ;
#53380=VERTEX_POINT ( 'NONE', #52979 ) ;
#53382=EDGE_LOOP ( 'NONE', ( #76568, #7650, #63177, #62534 ) ) ;
#53384=CARTESIAN_POINT ( 'NONE',  ( 5.933916589044118339, -2.538708090699994813, 30.37095296980875148 ) ) ;
#53385=CARTESIAN_POINT ( 'NONE',  ( 10.48469401227430886, -11.37499894934982692, 33.29245874905763003 ) ) ;
#53386=CARTESIAN_POINT ( 'NONE',  ( 4.376858997939549134, -3.395485233115139057, 33.02377354290275946 ) ) ;
#53387=AXIS2_PLACEMENT_3D ( 'NONE', #37897, #25720, #24367 ) ;
#53388=CARTESIAN_POINT ( 'NONE',  ( -8.546451100252701494, -10.23759521482555357, 34.22997729860117033 ) ) ;
#53390=DIRECTION ( 'NONE',  ( -0.000000000000000000, -0.9396926207859093161, -0.3420201433256663259 ) ) ;
#53392=ORIENTED_EDGE ( 'NONE', *, *, #44665, .F. ) ;
#53394=CARTESIAN_POINT ( 'NONE',  ( -3.454254155333563503, -2.612411019501189813, 31.66733052389439962 ) ) ;
#53395=EDGE_LOOP ( 'NONE', ( #12191, #8836 ) ) ;
#53396=CARTESIAN_POINT ( 'NONE',  ( 10.36536137809165403, -12.43535235679832596, 30.55408501211184813 ) ) ;
#53397=CARTESIAN_POINT ( 'NONE',  ( 8.096153846153848477, -2.499999999999999112, 29.81604066197449754 ) ) ;
#53400=CARTESIAN_POINT ( 'NONE',  ( -1.384615384615506484, -11.67786785259630911, 32.92929555188603530 ) ) ;
#53402=B_SPLINE_CURVE_WITH_KNOTS ( 'NONE', 3,
 ( #63830, #35929, #84564, #65150, #22839, #16526, #9771, #1691, #64705, #49868 ),
 .UNSPECIFIED., .F., .F.,
 ( 4, 2, 2, 2, 4 ),
 ( 0.000000000000000000, 0.0001954311564186880128, 0.0003908623128373760257, 0.0005862934692560640114, 0.0007817246256747520513 ),
 .UNSPECIFIED. ) ;
#53404=CARTESIAN_POINT ( 'NONE',  ( 17.07692307692295586, -12.16647553114689728, 32.15551576947799362 ) ) ;
#53405=FACE_BOUND ( 'NONE', #1426, .T. ) ;
#53406=CARTESIAN_POINT ( 'NONE',  ( -4.853911725310226188, -12.15243808032446005, 31.58219941686247978 ) ) ;
#53407=CARTESIAN_POINT ( 'NONE',  ( 1.134615384615387246, -7.500000000000001776, 35.04278698407183867 ) ) ;
#53408=ORIENTED_EDGE ( 'NONE', *, *, #83874, .F. ) ;
#53409=DIRECTION ( 'NONE',  ( -0.000000000000000000, 0.9396926207859093161, -0.3420201433256663259 ) ) ;
#53410=CARTESIAN_POINT ( 'NONE',  ( 8.835299120233207404, -6.386643153685127139, 34.62446782046654192 ) ) ;
#53411=DIRECTION ( 'NONE',  ( -0.000000000000000000, 0.000000000000000000, 1.000000000000000000 ) ) ;
#53412=ORIENTED_EDGE ( 'NONE', *, *, #29659, .T. ) ;
#53414=CARTESIAN_POINT ( 'NONE',  ( -0.4615384615381544209, -2.506253911140615021, 30.00000000000323297 ) ) ;
#53415=CARTESIAN_POINT ( 'NONE',  ( 14.43821774592595553, -10.31582465632705237, 34.18122507451815295 ) ) ;
#53416=CARTESIAN_POINT ( 'NONE',  ( -4.153846153846152411, -2.292212530054420494, 30.41441678777542634 ) ) ;
#53417=CARTESIAN_POINT ( 'NONE',  ( -16.40386937806761125, -12.07920672191015221, 32.31858351112116168 ) ) ;
#53419=FACE_BOUND ( 'NONE', #43519, .T. ) ;
#53420=CARTESIAN_POINT ( 'NONE',  ( 13.16113046005105858, -12.11044203135681840, 32.26167407432752299 ) ) ;
#53421=CARTESIAN_POINT ( 'NONE',  ( 8.769230769230645706, -2.657715359629662544, 31.77849191805970364 ) ) ;
#53422=CARTESIAN_POINT ( 'NONE',  ( 2.242422307135988557, -10.33852847137145048, 34.16647553114627556 ) ) ;
#53423=CYLINDRICAL_SURFACE ( 'NONE', #54443, 0.2500000000000008882 ) ;
#53424=CARTESIAN_POINT ( 'NONE',  ( 15.29602480204525250, -10.21337939537593620, 33.94971097300152252 ) ) ;
#53425=CARTESIAN_POINT ( 'NONE',  ( 6.065255139512838234, -5.094484230520773593, 34.41647553114626845 ) ) ;
#53427=ORIENTED_EDGE ( 'NONE', *, *, #44095, .F. ) ;
#53428=CARTESIAN_POINT ( 'NONE',  ( -7.173053654019277303, -9.148715823498378086, 34.47080413974185120 ) ) ;
#53429=ORIENTED_EDGE ( 'NONE', *, *, #61243, .T. ) ;
#53431=B_SPLINE_CURVE_WITH_KNOTS ( 'NONE', 3,
 ( #18205, #38028, #46118, #67281, #73606, #87571, #80359, #65492, #52417, #3790 ),
 .UNSPECIFIED., .F., .F.,
 ( 4, 2, 2, 2, 4 ),
 ( 0.0007817246256747516176, 0.0009771112852218965736, 0.001172497944769041421, 0.001367884604316186269, 0.001563271263863331333 ),
 .UNSPECIFIED. ) ;
#53432=CARTESIAN_POINT ( 'NONE',  ( 0.4615384615383396616, -6.879047030192662504, 34.71129190930017927 ) ) ;
#53433=VERTEX_POINT ( 'NONE', #18772 ) ;
#53434=CARTESIAN_POINT ( 'NONE',  ( 7.976944287120795174, -9.929761469519743144, 34.40412654351204225 ) ) ;
#53435=LINE ( 'NONE', #60195, #86288 ) ;
#53436=CARTESIAN_POINT ( 'NONE',  ( -2.372962753653081958, -11.94971097300153140, 32.03036669348370680 ) ) ;
#53438=CARTESIAN_POINT ( 'NONE',  ( 16.82689985270161515, -12.68155406624981119, 30.59749803192733708 ) ) ;
#53439=CARTESIAN_POINT ( 'NONE',  ( 1.161688425708538697, -11.98009711892699691, 32.48740034544075428 ) ) ;
#53441=CARTESIAN_POINT ( 'NONE',  ( 14.05766907039934210, -10.76384336483936011, 33.53834819971076087 ) ) ;
#53442=CARTESIAN_POINT ( 'NONE',  ( -12.46153846153858247, -12.27809138561165270, 31.22303859784587132 ) ) ;
#53443=CARTESIAN_POINT ( 'NONE',  ( -12.33074802057151409, -9.084667340241226796, 34.75534355489798344 ) ) ;
#53444=CARTESIAN_POINT ( 'NONE',  ( -14.30769230769242917, -6.835583212225970762, 34.95778746994575670 ) ) ;
#53445=CARTESIAN_POINT ( 'NONE',  ( 7.173131234715237170, -4.235687564193446164, 33.53795663066793509 ) ) ;
#53446=CARTESIAN_POINT ( 'NONE',  ( -11.53846153846165912, -10.21337939537710326, 33.94971097300076224 ) ) ;
#53448=CARTESIAN_POINT ( 'NONE',  ( 14.08476609017615644, -5.667676309546437530, 34.40238873228292249 ) ) ;
#53449=EDGE_CURVE ( 'NONE', #5201, #64026, #29673, .T. ) ;
#53450=CARTESIAN_POINT ( 'NONE',  ( -1.254089946381740761, -12.15418822224088657, 32.17964115625579069 ) ) ;
#53451=ORIENTED_EDGE ( 'NONE', *, *, #13894, .T. ) ;
#53452=DIRECTION ( 'NONE',  ( -0.000000000000000000, 0.6427876096865404731, -0.7660444431189770143 ) ) ;
#53453=CARTESIAN_POINT ( 'NONE',  ( 15.45378207486262667, -10.77377354290276124, 33.85451476688484718 ) ) ;
#53455=VECTOR ( 'NONE', #64250, 1000.000000000000000 ) ;
#53456=CARTESIAN_POINT ( 'NONE',  ( 2.057669070399344324, -4.335965774309649134, 33.62209801155881905 ) ) ;
#53457=CARTESIAN_POINT ( 'NONE',  ( -13.38461538461538325, -3.886160181151819604, 36.00935417666054406 ) ) ;
#53458=VERTEX_POINT ( 'NONE', #67396 ) ;
#53459=CYLINDRICAL_SURFACE ( 'NONE', #83073, 0.2500000000000009437 ) ;
#53460=CARTESIAN_POINT ( 'NONE',  ( -12.39628332202562433, -12.70778746994558439, 30.41441678777536595 ) ) ;
#53461=CARTESIAN_POINT ( 'NONE',  ( 11.60365452675619302, -2.255955759149235629, 29.99999999999988987 ) ) ;
#53462=EDGE_LOOP ( 'NONE', ( #67185, #81989 ) ) ;
#53463=CARTESIAN_POINT ( 'NONE',  ( -13.13466986626724164, -11.37275283266504111, 32.91324779482534524 ) ) ;
#53464=CARTESIAN_POINT ( 'NONE',  ( -2.557692307692305267, -7.500000000000001776, 35.00000000000000000 ) ) ;
#53466=AXIS2_PLACEMENT_3D ( 'NONE', #32305, #66980, #5275 ) ;
#53467=CARTESIAN_POINT ( 'NONE',  ( -16.40384615384615330, -7.500000000000001776, 35.00000000000000000 ) ) ;
#53468=VERTEX_POINT ( 'NONE', #88583 ) ;
#53469=B_SPLINE_CURVE_WITH_KNOTS ( 'NONE', 3,
 ( #22847, #10674, #71039, #71920, #65598, #31384, #16535, #79130, #37692, #17431 ),
 .UNSPECIFIED., .F., .F.,
 ( 4, 2, 2, 2, 4 ),
 ( 0.0007817246336856291692, 0.0009771112958940105907, 0.001172497958102391904, 0.001367884620310773434, 0.001563271282519154747 ),
 .UNSPECIFIED. ) ;
#53470=LINE ( 'NONE', #10277, #34666 ) ;
#53471=CARTESIAN_POINT ( 'NONE',  ( 6.923076923076802558, -5.219633306517616589, 34.19971097300220464 ) ) ;
#53472=EDGE_CURVE ( 'NONE', #87090, #70251, #22004, .T. ) ;
#53473=EDGE_CURVE ( 'NONE', #59229, #58032, #70335, .T. ) ;
#53474=CARTESIAN_POINT ( 'NONE',  ( 8.638540166120458608, -3.338472653186243644, 32.95098750199972670 ) ) ;
#53475=EDGE_LOOP ( 'NONE', ( #14909, #53162 ) ) ;
#53476=EDGE_LOOP ( 'NONE', ( #80834, #36775, #76590, #28635 ) ) ;
#53477=ORIENTED_EDGE ( 'NONE', *, *, #35459, .F. ) ;
#53478=EDGE_CURVE ( 'NONE', #15316, #485, #12266, .T. ) ;
#53479=CARTESIAN_POINT ( 'NONE',  ( 0.4615384615383396616, -8.613356846316285953, 34.62446782046622218 ) ) ;
#53480=DIRECTION ( 'NONE',  ( -0.000000000000000000, -0.8660254037844399289, -0.4999999999999980016 ) ) ;
#53481=CARTESIAN_POINT ( 'NONE',  ( 2.307692307692187583, -6.026961402154118908, 34.52809138561165270 ) ) ;
#53482=CARTESIAN_POINT ( 'NONE',  ( -17.77703709643851226, -7.369474270740072441, 34.74850911626239736 ) ) ;
#53484=ORIENTED_EDGE ( 'NONE', *, *, #13554, .T. ) ;
#53485=VERTEX_POINT ( 'NONE', #75477 ) ;
#53486=ORIENTED_EDGE ( 'NONE', *, *, #38296, .T. ) ;
#53487=CARTESIAN_POINT ( 'NONE',  ( -8.096177083446809419, -5.056417327199099532, 34.11270091957321426 ) ) ;
#53489=DIRECTION ( 'NONE',  ( 0.000000000000000000, 0.9848077530122072432, 0.1736481776669354937 ) ) ;
#53490=VECTOR ( 'NONE', #71730, 1000.000000000000114 ) ;
#53491=DIRECTION ( 'NONE',  ( -0.000000000000000000, -0.000000000000000000, -1.000000000000000000 ) ) ;
#53493=DIRECTION ( 'NONE',  ( -0.000000000000000000, -0.3420201433256694346, -0.9396926207859080948 ) ) ;
#53494=B_SPLINE_CURVE_WITH_KNOTS ( 'NONE', 3,
 ( #59055, #52297, #79787, #66259, #18083, #25280, #45543, #11318, #16302, #6355 ),
 .UNSPECIFIED., .F., .F.,
 ( 4, 2, 2, 2, 4 ),
 ( 0.0007817359430256297891, 0.0009771253907249958896, 0.001172514838424362207, 0.001367904286123728524, 0.001563293733823094625 ),
 .UNSPECIFIED. ) ;
#53495=ORIENTED_EDGE ( 'NONE', *, *, #53093, .F. ) ;
#53496=EDGE_LOOP ( 'NONE', ( #40862, #1218, #48762, #57122 ) ) ;
#53498=CARTESIAN_POINT ( 'NONE',  ( -4.826923076921640465, -7.500000000000155431, 34.75000000000007105 ) ) ;
#53499=CARTESIAN_POINT ( 'NONE',  ( -10.36533019547115764, -2.544122305571458575, 31.48381861865057729 ) ) ;
#53500=EDGE_LOOP ( 'NONE', ( #35232, #46406 ) ) ;
#53501=CARTESIAN_POINT ( 'NONE',  ( 2.057715563643719658, -2.544273027872574922, 31.48422191005632342 ) ) ;
#53503=ORIENTED_EDGE ( 'NONE', *, *, #8303, .T. ) ;
#53504=CARTESIAN_POINT ( 'NONE',  ( -16.85391172531022619, -9.086983370893049639, 34.49168942202179267 ) ) ;
#53505=CARTESIAN_POINT ( 'NONE',  ( 16.37685750545900376, -3.587049720035815348, 32.86302985866382897 ) ) ;
#53507=FACE_BOUND ( 'NONE', #24160, .T. ) ;
#53508=CARTESIAN_POINT ( 'NONE',  ( -17.77698864838715309, -8.239487800360276282, 34.69522927552633718 ) ) ;
#53509=CARTESIAN_POINT ( 'NONE',  ( -12.71156169883143150, -9.271318131107980420, 34.42618302367067429 ) ) ;
#53511=CARTESIAN_POINT ( 'NONE',  ( -10.61538461538473577, -11.06231777344772027, 33.60647404775119895 ) ) ;
#53513=CARTESIAN_POINT ( 'NONE',  ( -5.076923076923075762, -1.242168528481310874, 33.36296068462461051 ) ) ;
#53514=VECTOR ( 'NONE', #83189, 1000.000000000000114 ) ;
#53516=CARTESIAN_POINT ( 'NONE',  ( -11.53846153846153655, -11.11383981884818262, 36.00935417666054406 ) ) ;
#53518=CARTESIAN_POINT ( 'NONE',  ( 16.15384615384646949, -2.255955759149395501, 30.00000000000324363 ) ) ;
#53519=CARTESIAN_POINT ( 'NONE',  ( -13.60810030917971503, -9.417330523894424488, 34.63758898049880486 ) ) ;
#53520=VERTEX_POINT ( 'NONE', #83591 ) ;
#53521=ORIENTED_EDGE ( 'NONE', *, *, #23249, .F. ) ;
#53524=CARTESIAN_POINT ( 'NONE',  ( 0.6843181305165264572, -8.540255544307065350, 34.89611431652622286 ) ) ;
#53525=CARTESIAN_POINT ( 'NONE',  ( 16.15384615384603251, -2.379036618888197729, 30.90682066428292885 ) ) ;
#53526=CARTESIAN_POINT ( 'NONE',  ( 12.46153846153846168, -10.67929555188718282, 33.92786785259544047 ) ) ;
#53527=EDGE_LOOP ( 'NONE', ( #75191, #42647 ) ) ;
#53529=CYLINDRICAL_SURFACE ( 'NONE', #21362, 0.2500000000000002220 ) ;
#53530=FACE_BOUND ( 'NONE', #66364, .T. ) ;
#53531=CARTESIAN_POINT ( 'NONE',  ( -10.61538461538461320, -4.661471528628507777, 34.16647553114623292 ) ) ;
#53532=CARTESIAN_POINT ( 'NONE',  ( 5.869852030268306819, -6.809168938359898782, 34.95455904226513866 ) ) ;
#53533=CARTESIAN_POINT ( 'NONE',  ( -8.769230769230890843, -6.879047030192662504, 34.71129190930017927 ) ) ;
#53534=CARTESIAN_POINT ( 'NONE',  ( 0.4615384615383382183, -5.094484230521993062, 34.41647553114689373 ) ) ;
#53535=FILL_AREA_STYLE_COLOUR ( '', #87850 ) ;
#53536=CYLINDRICAL_SURFACE ( 'NONE', #1760, 0.2499999999999994726 ) ;
#53537=B_SPLINE_CURVE_WITH_KNOTS ( 'NONE', 3,
 ( #81192, #74424, #12726, #19915, #82527, #67672, #27569, #5976, #41085, #33445 ),
 .UNSPECIFIED., .F., .F.,
 ( 4, 2, 2, 2, 4 ),
 ( 0.000000000000000000, 0.0001954311564186865492, 0.0003908623128373730983, 0.0005862934692560596746, 0.0007817246256747461966 ),
 .UNSPECIFIED. ) ;
#53540=ORIENTED_EDGE ( 'NONE', *, *, #14187, .F. ) ;
#53541=ADVANCED_FACE ( 'NONE', ( #56096 ), #42591, .F. ) ;
#53542=B_SPLINE_CURVE_WITH_KNOTS ( 'NONE', 3,
 ( #21440, #56559, #14687, #83607, #42609, #84049, #22329, #35396, #13353, #70070 ),
 .UNSPECIFIED., .F., .F.,
 ( 4, 2, 2, 2, 4 ),
 ( 0.000000000000000000, 0.0001954339857564080707, 0.0003908679715128161414, 0.0005863019572692241849, 0.0007817359430256322827 ),
 .UNSPECIFIED. ) ;
#53543=CARTESIAN_POINT ( 'NONE',  ( -12.21148404162501144, -5.642605341092957971, 34.66089969410670335 ) ) ;
#53544=DIRECTION ( 'NONE',  ( -0.000000000000000000, -0.5000000000000009992, -0.8660254037844380415 ) ) ;
#53546=CYLINDRICAL_SURFACE ( 'NONE', #81282, 0.2499999999999973355 ) ;
#53547=B_SPLINE_CURVE_WITH_KNOTS ( 'NONE', 3,
 ( #31777, #32654, #59235, #73660, #46616, #11955, #25006, #79959, #26345, #53810 ),
 .UNSPECIFIED., .F., .F.,
 ( 4, 2, 2, 2, 4 ),
 ( 0.0007817246256747447872, 0.0009771112852218874663, 0.001172497944769030362, 0.001367884604316173258, 0.001563271263863315937 ),
 .UNSPECIFIED. ) ;
#53548=ADVANCED_FACE ( 'NONE', ( #8361 ), #48438, .F. ) ;
#53549=DIRECTION ( 'NONE',  ( -0.000000000000000000, 0.5000000000000011102, -0.8660254037844381525 ) ) ;
#53551=CARTESIAN_POINT ( 'NONE',  ( -7.623142494540996239, -8.239487800360276282, 34.69522927552633718 ) ) ;
#53552=CARTESIAN_POINT ( 'NONE',  ( 1.634669696253701732, -4.943051570960395047, 34.04725096376909477 ) ) ;
#53553=DIRECTION ( 'NONE',  ( -0.000000000000000000, -0.9396926207859092051, -0.3420201433256662704 ) ) ;
#53554=CARTESIAN_POINT ( 'NONE',  ( 12.21151523731700372, -11.56360843649121861, 33.07473185843129926 ) ) ;
#53555=CARTESIAN_POINT ( 'NONE',  ( -9.942284423250047354, -11.28823185664190376, 33.01397839955799896 ) ) ;
#53556=CARTESIAN_POINT ( 'NONE',  ( 13.63466980452884236, -2.544122305571458575, 31.48381861865057729 ) ) ;
#53558=CARTESIAN_POINT ( 'NONE',  ( 6.923076923076800782, -3.643525952248796163, 33.31231777344771672 ) ) ;
#53559=CARTESIAN_POINT ( 'NONE',  ( 9.692307692307695177, -13.87047571288749737, 32.06866353760679544 ) ) ;
#53560=CARTESIAN_POINT ( 'NONE',  ( -6.673131513698879580, -3.520799739797213501, 33.17531984108286025 ) ) ;
#53561=EDGE_CURVE ( 'NONE', #88595, #71008, #709, .T. ) ;
#53562=CARTESIAN_POINT ( 'NONE',  ( -15.36091644020745051, -8.587444163452046197, 34.63053765926554206 ) ) ;
#53564=EDGE_LOOP ( 'NONE', ( #36099, #72459 ) ) ;
#53566=DIRECTION ( 'NONE',  ( -0.000000000000000000, -0.8660254037844397068, -0.4999999999999978906 ) ) ;
#53568=EDGE_CURVE ( 'NONE', #11900, #30370, #57394, .T. ) ;
#53569=CARTESIAN_POINT ( 'NONE',  ( 13.45068373561782593, -4.786620604624113540, 33.94971097300155805 ) ) ;
#53570=FACE_OUTER_BOUND ( 'NONE', #23551, .T. ) ;
#53571=CYLINDRICAL_SURFACE ( 'NONE', #28414, 0.2500000000000012212 ) ;
#53572=CARTESIAN_POINT ( 'NONE',  ( 5.207713517890028676, -3.957578996910242619, 33.62503395064540257 ) ) ;
#53575=CARTESIAN_POINT ( 'NONE',  ( 7.846153846153846700, -11.16473453929635440, 33.15142922261926373 ) ) ;
#53576=ORIENTED_EDGE ( 'NONE', *, *, #11331, .F. ) ;
#53578=CARTESIAN_POINT ( 'NONE',  ( 18.06525557127602610, -9.442884908240273489, 34.35708131394835618 ) ) ;
#53579=VERTEX_POINT ( 'NONE', #61513 ) ;
#53580=FACE_OUTER_BOUND ( 'NONE', #33029, .T. ) ;
#53581=CARTESIAN_POINT ( 'NONE',  ( -7.596208327805705096, -11.86320923018887719, 32.19269448109603360 ) ) ;
#53582=EDGE_CURVE ( 'NONE', #24932, #24126, #34907, .T. ) ;
#53583=CARTESIAN_POINT ( 'NONE',  ( 3.230769230769231726, -5.180354513474913603, 36.12317359536750416 ) ) ;
#53584=ORIENTED_EDGE ( 'NONE', *, *, #13046, .F. ) ;
#53585=EDGE_CURVE ( 'NONE', #15450, #7242, #68724, .T. ) ;
#53586=B_SPLINE_CURVE_WITH_KNOTS ( 'NONE', 3,
 ( #21212, #55884, #68512, #27534, #76608, #34732, #62199, #83371, #14463, #14915 ),
 .UNSPECIFIED., .F., .F.,
 ( 4, 2, 2, 2, 4 ),
 ( 0.000000000000000000, 0.0001954339857564091007, 0.0003908679715128182013, 0.0005863019572692273291, 0.0007817359430256364027 ),
 .UNSPECIFIED. ) ;
#53587=ORIENTED_EDGE ( 'NONE', *, *, #60848, .T. ) ;
#53588=B_SPLINE_CURVE_WITH_KNOTS ( 'NONE', 3,
 ( #25782, #80743, #46495, #73974, #53691, #81179, #19464, #46925, #74412, #62651 ),
 .UNSPECIFIED., .F., .F.,
 ( 4, 2, 2, 2, 4 ),
 ( 0.0007817246256747458714, 0.0009771112852218889842, 0.001172497944769032097, 0.001367884604316175210, 0.001563271263863318323 ),
 .UNSPECIFIED. ) ;
#53589=VECTOR ( 'NONE', #1940, 1000.000000000000114 ) ;
#53591=AXIS2_PLACEMENT_3D ( 'NONE', #31564, #66229, #78855 ) ;
#53593=CARTESIAN_POINT ( 'NONE',  ( 6.923076923076924238, -11.35647404775217417, 33.31231777344666511 ) ) ;
#53594=EDGE_CURVE ( 'NONE', #69885, #63787, #70051, .T. ) ;
#53596=CARTESIAN_POINT ( 'NONE',  ( -10.61538461538461320, -2.538708090699994813, 30.37095296980875503 ) ) ;
#53597=EDGE_CURVE ( 'NONE', #88692, #19422, #30399, .T. ) ;
#53598=CARTESIAN_POINT ( 'NONE',  ( -9.692307692307691624, -9.058645607665452459, 34.76329471203371924 ) ) ;
#53599=CARTESIAN_POINT ( 'NONE',  ( 14.30769230769218758, -11.94971097300221174, 32.03036669348237098 ) ) ;
#53600=CARTESIAN_POINT ( 'NONE',  ( 12.59233026936325039, -4.809403383903225304, 33.96459661697924304 ) ) ;
#53601=AXIS2_PLACEMENT_3D ( 'NONE', #33872, #27117, #87974 ) ;
#53602=CARTESIAN_POINT ( 'NONE',  ( 15.90386940979756858, -12.65889640711025521, 30.72598325615533454 ) ) ;
#53604=ORIENTED_EDGE ( 'NONE', *, *, #84883, .T. ) ;
#53606=CARTESIAN_POINT ( 'NONE',  ( 18.13052543823364360, -9.503571793651730104, 34.60286762892837942 ) ) ;
#53607=VERTEX_POINT ( 'NONE', #84032 ) ;
#53608=CARTESIAN_POINT ( 'NONE',  ( -8.546217925137375104, -10.77377354290276124, 33.85451476688484718 ) ) ;
#53609=CARTESIAN_POINT ( 'NONE',  ( 6.000000000000001776, -9.905515769479276145, 34.41647553114623292 ) ) ;
#53611=CARTESIAN_POINT ( 'NONE',  ( -14.17690049986751433, -4.118422570099831148, 33.43335022499816489 ) ) ;
#53612=B_SPLINE_CURVE_WITH_KNOTS ( 'NONE', 3,
 ( #8553, #79665, #44971, #58048, #57611, #78767, #18409, #37329, #45867, #11203 ),
 .UNSPECIFIED., .F., .F.,
 ( 4, 2, 2, 2, 4 ),
 ( 0.0007817246256747476061, 0.0009771112852218896347, 0.001172497944769031880, 0.001367884604316173909, 0.001563271263863315937 ),
 .UNSPECIFIED. ) ;
#53613=VECTOR ( 'NONE', #13361, 999.9999999999998863 ) ;
#53614=EDGE_LOOP ( 'NONE', ( #43637, #32214 ) ) ;
#53615=LINE ( 'NONE', #4995, #56908 ) ;
#53618=B_SPLINE_CURVE_WITH_KNOTS ( 'NONE', 3,
 ( #74636, #19684, #743, #13812, #54347, #48473, #68759, #302, #28207, #21458 ),
 .UNSPECIFIED., .F., .F.,
 ( 4, 2, 2, 2, 4 ),
 ( 0.000000000000000000, 0.0001954311564186868202, 0.0003908623128373736404, 0.0005862934692560604335, 0.0007817246256747472808 ),
 .UNSPECIFIED. ) ;
#53619=CARTESIAN_POINT ( 'NONE',  ( -18.13014796973170206, -9.504002272028873932, 34.60269587691767867 ) ) ;
#53620=EDGE_CURVE ( 'NONE', #10201, #33117, #39239, .T. ) ;
#53621=CARTESIAN_POINT ( 'NONE',  ( -4.377331078410484189, -4.225889041578354544, 33.85425143139329407 ) ) ;
#53622=EDGE_CURVE ( 'NONE', #57810, #86321, #44465, .T. ) ;
#53623=CARTESIAN_POINT ( 'NONE',  ( -16.02305571287920571, -10.70102852606553157, 33.91149625220312913 ) ) ;
#53624=FACE_BOUND ( 'NONE', #87809, .T. ) ;
#53625=DIRECTION ( 'NONE',  ( 0.000000000000000000, 1.000000000000000000, 0.000000000000000000 ) ) ;
#53626=CARTESIAN_POINT ( 'NONE',  ( 1.634615384616805889, -7.500000000000154543, 35.00000000000007105 ) ) ;
#53627=EDGE_CURVE ( 'NONE', #44944, #54584, #37593, .T. ) ;
#53628=DIRECTION ( 'NONE',  ( -0.000000000000000000, 0.6427876096865404731, -0.7660444431189771253 ) ) ;
#53629=CARTESIAN_POINT ( 'NONE',  ( 3.480714640147273720, -4.932303261841488151, 34.32971442181322885 ) ) ;
#53630=CARTESIAN_POINT ( 'NONE',  ( -17.07692307692319744, -2.379036618888197285, 30.90682066428292885 ) ) ;
#53631=DIRECTION ( 'NONE',  ( -0.000000000000000000, -0.8660254037844397068, -0.4999999999999978906 ) ) ;
#53632=CARTESIAN_POINT ( 'NONE',  ( -11.78848476268299628, -3.520140089381495585, 33.17453946501458262 ) ) ;
#53633=EDGE_LOOP ( 'NONE', ( #62743, #3234, #21455, #51811 ) ) ;
#53634=ORIENTED_EDGE ( 'NONE', *, *, #57046, .F. ) ;
#53635=EDGE_CURVE ( 'NONE', #10850, #73234, #73538, .T. ) ;
#53636=DIRECTION ( 'NONE',  ( -0.000000000000000000, 0.5000000000000011102, -0.8660254037844381525 ) ) ;
#53637=CARTESIAN_POINT ( 'NONE',  ( 15.23076923076923173, -3.886160181151819604, 36.00935417666054406 ) ) ;
#53638=CARTESIAN_POINT ( 'NONE',  ( 15.36129466900288065, -8.630441415882550871, 34.87705825610312615 ) ) ;
#53640=CARTESIAN_POINT ( 'NONE',  ( -3.230769230769229949, -2.499999999999998668, 29.50000000000001066 ) ) ;
#53643=CARTESIAN_POINT ( 'NONE',  ( -5.299850035829923200, -5.582147617184174848, 34.63737895849758530 ) ) ;
#53644=B_SPLINE_CURVE_WITH_KNOTS ( 'NONE', 3,
 ( #61127, #34104, #81865, #61569, #87299, #88637, #32775, #12509, #13831, #47622 ),
 .UNSPECIFIED., .F., .F.,
 ( 4, 2, 2, 2, 4 ),
 ( 0.000000000000000000, 0.0001954339857564071491, 0.0003908679715128142982, 0.0005863019572692214744, 0.0007817359430256285964 ),
 .UNSPECIFIED. ) ;
#53646=CARTESIAN_POINT ( 'NONE',  ( -6.923076923076922462, -12.29105614889573062, 35.45975837776705220 ) ) ;
#53647=CARTESIAN_POINT ( 'NONE',  ( -7.173053667125516064, -6.524016743844655686, 34.90889640711025521 ) ) ;
#53648=ORIENTED_EDGE ( 'NONE', *, *, #58686, .T. ) ;
#53649=ORIENTED_EDGE ( 'NONE', *, *, #20266, .T. ) ;
#53650=VECTOR ( 'NONE', #29942, 1000.000000000000114 ) ;
#53652=ORIENTED_EDGE ( 'NONE', *, *, #65091, .F. ) ;
#53653=AXIS2_PLACEMENT_3D ( 'NONE', #72223, #31239, #65470 ) ;
#53654=CARTESIAN_POINT ( 'NONE',  ( 0.2115384615384615641, -7.500000000000001776, 34.75000000000000000 ) ) ;
#53655=CARTESIAN_POINT ( 'NONE',  ( -14.17716686945866122, -5.915461855592780260, 34.75538340440931506 ) ) ;
#53656=ORIENTED_EDGE ( 'NONE', *, *, #79636, .F. ) ;
#53658=CARTESIAN_POINT ( 'NONE',  ( 2.307692307692309264, -11.11383981884818262, 36.00935417666054406 ) ) ;
#53660=ADVANCED_FACE ( 'NONE', ( #77692 ), #29960, .F. ) ;
#53661=CARTESIAN_POINT ( 'NONE',  ( 1.449870524128224814, -6.835583212224609184, 34.95778746994559327 ) ) ;
#53663=CARTESIAN_POINT ( 'NONE',  ( -0.4615384615384611200, -11.16473453929635440, 33.15142922261926373 ) ) ;
#53665=CARTESIAN_POINT ( 'NONE',  ( -0.3310130233048185211, -12.15418822224088657, 32.17964115625579069 ) ) ;
#53666=VERTEX_POINT ( 'NONE', #16004 ) ;
#53667=LINE ( 'NONE', #12239, #21022 ) ;
#53668=CARTESIAN_POINT ( 'NONE',  ( 16.02328556210422761, -2.504760397472873823, 29.97295953869789997 ) ) ;
#53669=CARTESIAN_POINT ( 'NONE',  ( 1.254005024990858308, -7.722926236386453702, 34.74524107206102030 ) ) ;
#53670=CARTESIAN_POINT ( 'NONE',  ( 8.899756207464411872, -12.15418822224088657, 32.17964115625579069 ) ) ;
#53671=FACE_OUTER_BOUND ( 'NONE', #53274, .T. ) ;
#53672=CARTESIAN_POINT ( 'NONE',  ( -5.076923076923199218, -11.06231777344772027, 33.60647404775119895 ) ) ;
#53673=CARTESIAN_POINT ( 'NONE',  ( -14.30769230769230660, -12.37446782046654192, 30.86335684631486131 ) ) ;
#53676=CARTESIAN_POINT ( 'NONE',  ( 15.16549878480845770, -8.613356846314824011, 34.62446782046655613 ) ) ;
#53677=CARTESIAN_POINT ( 'NONE',  ( 7.780830930661671196, -7.749976743299137993, 34.99404534957040624 ) ) ;
#53678=CARTESIAN_POINT ( 'NONE',  ( 20.74999999999999645, -12.50000000000000000, 27.25000000000000000 ) ) ;
#53679=VERTEX_POINT ( 'NONE', #9254 ) ;
#53680=CARTESIAN_POINT ( 'NONE',  ( -2.307692307692305711, -2.900454961884010974, 35.62045528018868623 ) ) ;
#53682=CARTESIAN_POINT ( 'NONE',  ( -8.769230769230892619, -11.06231777344772027, 33.60647404775119895 ) ) ;
#53684=CARTESIAN_POINT ( 'NONE',  ( 6.923076923076800782, -9.528491918059723176, 34.59228464037033035 ) ) ;
#53686=EDGE_LOOP ( 'NONE', ( #22810, #12419 ) ) ;
#53687=CARTESIAN_POINT ( 'NONE',  ( 2.307692307692309264, -11.69971097300155272, 32.46337939537588113 ) ) ;
#53688=EDGE_CURVE ( 'NONE', #62981, #53520, #78139, .T. ) ;
#53691=CARTESIAN_POINT ( 'NONE',  ( -2.057746898314263717, -5.766571408460171355, 34.70601412856602508 ) ) ;
#53692=EDGE_LOOP ( 'NONE', ( #33760, #76871, #85738, #37849 ) ) ;
#53693=DIRECTION ( 'NONE',  ( 0.000000000000000000, 0.7660444431189807890, 0.6427876096865361433 ) ) ;
#53694=EDGE_CURVE ( 'NONE', #81733, #21693, #85326, .T. ) ;
#53696=DIRECTION ( 'NONE',  ( -0.000000000000000000, -0.1736481776669307198, -0.9848077530122080203 ) ) ;
#53697=CARTESIAN_POINT ( 'NONE',  ( 11.78851595837499211, -6.523592122091592671, 34.90882529074906415 ) ) ;
#53698=VERTEX_POINT ( 'NONE', #75332 ) ;
#53700=CARTESIAN_POINT ( 'NONE',  ( 12.33139125210023934, -3.817052484675422797, 33.13202310037935661 ) ) ;
#53701=CARTESIAN_POINT ( 'NONE',  ( 5.999999999999880096, -10.21337939537710326, 33.94971097300076224 ) ) ;
#53702=LINE ( 'NONE', #25346, #81112 ) ;
#53703=CARTESIAN_POINT ( 'NONE',  ( 11.28848479441294828, -12.41104346484419452, 31.60698883733904196 ) ) ;
#53706=ORIENTED_EDGE ( 'NONE', *, *, #24046, .T. ) ;
#53707=DIRECTION ( 'NONE',  ( 0.000000000000000000, 0.6427876096865373645, -0.7660444431189797898 ) ) ;
#53708=EDGE_LOOP ( 'NONE', ( #54629, #28564, #64774, #36622 ) ) ;
#53709=CARTESIAN_POINT ( 'NONE',  ( -2.557669051740895760, -2.544273027872574922, 31.48422191005632342 ) ) ;
#53710=ADVANCED_FACE ( 'NONE', ( #36125 ), #999, .F. ) ;
#53711=B_SPLINE_CURVE_WITH_KNOTS ( 'NONE', 3,
 ( #79301, #65767, #30656, #29344, #50042, #77519, #44153, #10842, #36965, #9498 ),
 .UNSPECIFIED., .F., .F.,
 ( 4, 2, 2, 2, 4 ),
 ( 0.0007817359430256322827, 0.0009771253907249989254, 0.001172514838424365676, 0.001367904286123732428, 0.001563293733823099179 ),
 .UNSPECIFIED. ) ;
#53712=AXIS2_PLACEMENT_3D ( 'NONE', #57780, #49259, #15035 ) ;
#53713=CARTESIAN_POINT ( 'NONE',  ( -10.61538461538461320, -9.905515769479276145, 34.41647553114623292 ) ) ;
#53714=CARTESIAN_POINT ( 'NONE',  ( 17.99999999999987566, -6.835583212225970762, 34.95778746994575670 ) ) ;
#53715=EDGE_CURVE ( 'NONE', #3961, #3690, #17701, .T. ) ;
#53716=DIRECTION ( 'NONE',  ( -0.000000000000000000, 0.3420201433256694901, -0.9396926207859082059 ) ) ;
#53717=CARTESIAN_POINT ( 'NONE',  ( 4.826923076923076650, -2.499999999999998668, 29.75000000000000355 ) ) ;
#53718=B_SPLINE_CURVE_WITH_KNOTS ( 'NONE', 3,
 ( #52687, #53578, #81513, #86957, #46385, #81073, #4962, #5848, #25223, #19802 ),
 .UNSPECIFIED., .F., .F.,
 ( 4, 2, 2, 2, 4 ),
 ( 0.0007817359430256293554, 0.0009771253907249952391, 0.001172514838424361123, 0.001367904286123726790, 0.001563293733823092673 ),
 .UNSPECIFIED. ) ;
#53719=ORIENTED_EDGE ( 'NONE', *, *, #26280, .T. ) ;
#53720=ORIENTED_EDGE ( 'NONE', *, *, #85554, .F. ) ;
#53721=VERTEX_POINT ( 'NONE', #22157 ) ;
#53722=ORIENTED_EDGE ( 'NONE', *, *, #82859, .T. ) ;
#53723=EDGE_CURVE ( 'NONE', #60966, #13706, #68564, .T. ) ;
#53724=CARTESIAN_POINT ( 'NONE',  ( -5.299850035829926753, -4.026226216239095379, 33.68668979543632958 ) ) ;
#53725=CARTESIAN_POINT ( 'NONE',  ( 16.21910129335899597, -11.06231777344670952, 33.60647404775212266 ) ) ;
#53726=DIRECTION ( 'NONE',  ( 0.000000000000000000, 0.000000000000000000, 1.000000000000000000 ) ) ;
#53727=EDGE_CURVE ( 'NONE', #35101, #22351, #82975, .T. ) ;
#53728=CARTESIAN_POINT ( 'NONE',  ( -8.096130590202436750, -3.436278759898153901, 33.07459398097509506 ) ) ;
#53729=CARTESIAN_POINT ( 'NONE',  ( 11.53846153846153832, -2.538708090699994813, 30.37095296980875503 ) ) ;
#53730=DIRECTION ( 'NONE',  ( 0.000000000000000000, 0.000000000000000000, 1.000000000000000000 ) ) ;
#53731=CARTESIAN_POINT ( 'NONE',  ( 17.77651505627605033, -2.599994579823202923, 30.74605699353653776 ) ) ;
#53732=CARTESIAN_POINT ( 'NONE',  ( -8.703975629717932705, -3.083524468853784839, 32.58852847137153930 ) ) ;
#53733=ORIENTED_EDGE ( 'NONE', *, *, #65204, .T. ) ;
#53735=EDGE_LOOP ( 'NONE', ( #7228, #82865, #43854, #24370 ) ) ;
#53736=CARTESIAN_POINT ( 'NONE',  ( 2.242421861731532573, -2.625532179533444754, 30.86335684631481513 ) ) ;
#53738=ORIENTED_EDGE ( 'NONE', *, *, #62673, .F. ) ;
#53739=AXIS2_PLACEMENT_3D ( 'NONE', #69032, #54618, #12759 ) ;
#53741=CARTESIAN_POINT ( 'NONE',  ( 11.28846153846153832, -2.499999999999998668, 29.75000000000000355 ) ) ;
#53742=CARTESIAN_POINT ( 'NONE',  ( 5.326923076923075762, -2.499999999999998668, 29.75000000000000355 ) ) ;
#53743=CARTESIAN_POINT ( 'NONE',  ( -9.942330929600657896, -6.695914987888146541, 34.68535235679833306 ) ) ;
#53744=FACE_BOUND ( 'NONE', #67212, .T. ) ;
#53745=ORIENTED_EDGE ( 'NONE', *, *, #22304, .F. ) ;
#53746=ADVANCED_FACE ( 'NONE', ( #113 ), #28471, .F. ) ;
#53747=ORIENTED_EDGE ( 'NONE', *, *, #36512, .T. ) ;
#53748=CARTESIAN_POINT ( 'NONE',  ( 5.999999999999878320, -11.06231777344772027, 33.60647404775119895 ) ) ;
#53749=ORIENTED_EDGE ( 'NONE', *, *, #57440, .F. ) ;
#53750=FACE_BOUND ( 'NONE', #46890, .T. ) ;
#53751=CARTESIAN_POINT ( 'NONE',  ( -10.61538461538473577, -3.083524468854526912, 32.58852847137268327 ) ) ;
#53753=ORIENTED_EDGE ( 'NONE', *, *, #63704, .T. ) ;
#53754=LINE ( 'NONE', #6897, #37666 ) ;
#53755=CARTESIAN_POINT ( 'NONE',  ( -12.71151520558704995, -12.01397095200674059, 32.43157075238190146 ) ) ;
#53756=CARTESIAN_POINT ( 'NONE',  ( 3.230769230769108269, -12.16647553114689728, 32.15551576947799362 ) ) ;
#53757=ORIENTED_EDGE ( 'NONE', *, *, #40548, .F. ) ;
#53758=CARTESIAN_POINT ( 'NONE',  ( 6.792929713638703682, -6.001485441113818986, 34.52039167877662607 ) ) ;
#53760=CARTESIAN_POINT ( 'NONE',  ( -3.296852641725110278, -2.721908614388772296, 31.22303859784724622 ) ) ;
#53761=EDGE_CURVE ( 'NONE', #79237, #41543, #53090, .T. ) ;
#53762=CARTESIAN_POINT ( 'NONE',  ( -9.561781990544128362, -2.619367082507849442, 30.83698974864643461 ) ) ;
#53763=ORIENTED_EDGE ( 'NONE', *, *, #47084, .F. ) ;
#53764=EDGE_CURVE ( 'NONE', #72978, #77307, #49907, .T. ) ;
#53766=DIRECTION ( 'NONE',  ( -0.000000000000000000, 0.6427876096865404731, -0.7660444431189771253 ) ) ;
#53767=EDGE_LOOP ( 'NONE', ( #24045, #8413 ) ) ;
#53768=CARTESIAN_POINT ( 'NONE',  ( 3.296024370282069071, -6.835583212224609184, 34.95778746994559327 ) ) ;
#53769=DIRECTION ( 'NONE',  ( -0.000000000000000000, 0.6427876096865404731, -0.7660444431189771253 ) ) ;
#53770=CARTESIAN_POINT ( 'NONE',  ( -8.096130590202434973, -12.41104346484419452, 31.60698883733904196 ) ) ;
#53771=LINE ( 'NONE', #74492, #17014 ) ;
#53772=CARTESIAN_POINT ( 'NONE',  ( -6.792238592590160273, -7.277220318596959281, 34.99547417642776992 ) ) ;
#53773=DIRECTION ( 'NONE',  ( -0.000000000000000000, -0.1736481776669307198, -0.9848077530122080203 ) ) ;
#53776=CARTESIAN_POINT ( 'NONE',  ( 8.546303810323914618, -2.889293201056495786, 32.26117774369186009 ) ) ;
#53777=CARTESIAN_POINT ( 'NONE',  ( -15.90390063549800992, -11.86320923018887541, 32.19269448109604781 ) ) ;
#53778=CARTESIAN_POINT ( 'NONE',  ( -6.673131404728782634, -2.824170634883622188, 31.52227843825338738 ) ) ;
#53780=EDGE_LOOP ( 'NONE', ( #907, #6926 ) ) ;
#53781=AXIS2_PLACEMENT_3D ( 'NONE', #1186, #49383, #9609 ) ;
#53782=DIRECTION ( 'NONE',  ( -0.000000000000000000, -0.6427876096865404731, -0.7660444431189771253 ) ) ;
#53783=EDGE_LOOP ( 'NONE', ( #40155, #36926, #8425, #76822 ) ) ;
#53784=ORIENTED_EDGE ( 'NONE', *, *, #77400, .F. ) ;
#53785=CARTESIAN_POINT ( 'NONE',  ( -7.596208436775802930, -2.589246495874658383, 31.60778113518102828 ) ) ;
#53787=CARTESIAN_POINT ( 'NONE',  ( -5.300408001487407539, -11.60425143139329940, 33.02411095842164457 ) ) ;
#53789=CARTESIAN_POINT ( 'NONE',  ( -14.24243716817946925, -3.083524468853784839, 32.58852847137153930 ) ) ;
#53790=CARTESIAN_POINT ( 'NONE',  ( 10.83816428436267465, -2.612705202774698421, 31.66806509827799943 ) ) ;
#53791=CARTESIAN_POINT ( 'NONE',  ( 9.915320536401090123, -9.172514111537584114, 34.72667873470787470 ) ) ;
#53793=CARTESIAN_POINT ( 'NONE',  ( -2.307692307692305711, -3.322132147404559976, 32.92929555188717927 ) ) ;
#53795=B_SPLINE_CURVE_WITH_KNOTS ( 'NONE', 3,
 ( #58743, #78567, #30823, #72254, #10564, #32606, #31728, #24067, #37579, #58293 ),
 .UNSPECIFIED., .F., .F.,
 ( 4, 2, 2, 2, 4 ),
 ( 0.0007817246256747460882, 0.0009771112852218900684, 0.001172497944769033832, 0.001367884604316177595, 0.001563271263863321575 ),
 .UNSPECIFIED. ) ;
#53796=CARTESIAN_POINT ( 'NONE',  ( -1.384615384615383471, -8.973038597847269315, 34.52809138561121927 ) ) ;
#53797=B_SPLINE_CURVE_WITH_KNOTS ( 'NONE', 3,
 ( #80626, #18908, #33316, #26558, #39639, #18469 ),
 .UNSPECIFIED., .F., .F.,
 ( 4, 2, 4 ),
 ( 0.000000000000000000, 0.2500000631573452425, 0.5000001263146904851 ),
 .UNSPECIFIED. ) ;
#53798=CARTESIAN_POINT ( 'NONE',  ( 5.142990410273151625, -2.833524468853757750, 32.15551576947925838 ) ) ;
#53799=CARTESIAN_POINT ( 'NONE',  ( -13.25408968285182176, -6.852161475712352789, 34.70806712695775786 ) ) ;
#53800=FACE_OUTER_BOUND ( 'NONE', #60507, .T. ) ;
#53802=ORIENTED_EDGE ( 'NONE', *, *, #83868, .F. ) ;
#53803=EDGE_LOOP ( 'NONE', ( #87810, #43329 ) ) ;
#53804=CARTESIAN_POINT ( 'NONE',  ( 6.792929713638703682, -2.619462340734462380, 30.83744416345203021 ) ) ;
#53805=CARTESIAN_POINT ( 'NONE',  ( -16.15384615384615330, -12.78798330534102945, 29.74999999999997868 ) ) ;
#53806=DIRECTION ( 'NONE',  ( -0.000000000000000000, -0.1736481776669307198, -0.9848077530122080203 ) ) ;
#53807=CARTESIAN_POINT ( 'NONE',  ( -6.065270445960774914, -3.835265460703609186, 33.15142922261924241 ) ) ;
#53809=DIRECTION ( 'NONE',  ( -0.000000000000000000, -0.000000000000000000, -1.000000000000000000 ) ) ;
#53810=CARTESIAN_POINT ( 'NONE',  ( -5.076923076923075762, -2.833524468853757305, 32.15551576947925838 ) ) ;
#53811=VECTOR ( 'NONE', #67382, 1000.000000000000000 ) ;
#53812=ADVANCED_FACE ( 'NONE', ( #36983 ), #9094, .F. ) ;
#53813=CARTESIAN_POINT ( 'NONE',  ( -2.530619266599154038, -8.282780595021769443, 34.94152052738834868 ) ) ;
#53814=ORIENTED_EDGE ( 'NONE', *, *, #12302, .T. ) ;
#53815=CARTESIAN_POINT ( 'NONE',  ( -4.946397375159514276, -12.45806712695776319, 30.39783852428763922 ) ) ;
#53816=EDGE_LOOP ( 'NONE', ( #45011, #80666, #39769, #4819 ) ) ;
#53817=EDGE_CURVE ( 'NONE', #84095, #54976, #66006, .T. ) ;
#53818=ORIENTED_EDGE ( 'NONE', *, *, #50205, .F. ) ;
#53819=FACE_OUTER_BOUND ( 'NONE', #74336, .T. ) ;
#53820=CARTESIAN_POINT ( 'NONE',  ( 3.930361210122205406, -2.599994579823202923, 30.74605699353653776 ) ) ;
#53821=ADVANCED_FACE ( 'NONE', ( #72552 ), #16718, .F. ) ;
#53822=CARTESIAN_POINT ( 'NONE',  ( 14.08420736396836226, -5.113361153441934093, 34.14387501736622710 ) ) ;
#53823=CARTESIAN_POINT ( 'NONE',  ( 1.134638640566795642, -11.47974371597208076, 33.17467449705390692 ) ) ;
#53824=CARTESIAN_POINT ( 'NONE',  ( -13.60810030917972036, -2.612411019501189369, 31.66733052389439962 ) ) ;
#53826=EDGE_CURVE ( 'NONE', #5010, #28697, #59650, .T. ) ;
#53827=ORIENTED_EDGE ( 'NONE', *, *, #53597, .T. ) ;
#53829=EDGE_LOOP ( 'NONE', ( #65758, #23697, #75618, #45541 ) ) ;
#53830=AXIS2_PLACEMENT_3D ( 'NONE', #6873, #60491, #82102 ) ;
#53831=DIRECTION ( 'NONE',  ( 0.000000000000000000, 0.4999999999999960032, -0.8660254037844410391 ) ) ;
#53832=CARTESIAN_POINT ( 'NONE',  ( 6.923076923076924238, -3.886160181151819604, 36.00935417666054406 ) ) ;
#53833=EDGE_CURVE ( 'NONE', #60125, #79174, #41305, .T. ) ;
#53835=VECTOR ( 'NONE', #60578, 1000.000000000000000 ) ;
#53836=VECTOR ( 'NONE', #72495, 1000.000000000000114 ) ;
#53837=CARTESIAN_POINT ( 'NONE',  ( 16.40390046548447245, -9.943054286541403997, 34.11300777759954883 ) ) ;
#53839=EDGE_CURVE ( 'NONE', #19138, #65478, #87596, .T. ) ;
#53840=CARTESIAN_POINT ( 'NONE',  ( -15.45369618967607828, -2.523278758544489797, 31.42238647778637528 ) ) ;
#53842=B_SPLINE_CURVE_WITH_KNOTS ( 'NONE', 3,
 ( #55900, #35644, #69424, #69866, #14478, #8171, #7282, #82512, #27991, #88833 ),
 .UNSPECIFIED., .F., .F.,
 ( 4, 2, 2, 2, 4 ),
 ( 0.0007817359430256294638, 0.0009771253907249948054, 0.001172514838424360255, 0.001367904286123725489, 0.001563293733823090939 ),
 .UNSPECIFIED. ) ;
#53843=VERTEX_POINT ( 'NONE', #77980 ) ;
#53844=B_SPLINE_CURVE_WITH_KNOTS ( 'NONE', 3,
 ( #48967, #15628, #28245, #76442, #63802, #77761, #84538, #36343, #43531, #29588 ),
 .UNSPECIFIED., .F., .F.,
 ( 4, 2, 2, 2, 4 ),
 ( 0.000000000000000000, 0.0001954339857564079623, 0.0003908679715128159245, 0.0005863019572692238597, 0.0007817359430256318490 ),
 .UNSPECIFIED. ) ;
#53845=CYLINDRICAL_SURFACE ( 'NONE', #80425, 0.2499999999999997502 ) ;
#53847=CYLINDRICAL_SURFACE ( 'NONE', #14605, 0.2500000000000008882 ) ;
#53848=CARTESIAN_POINT ( 'NONE',  ( -4.853911725310227077, -11.24521262558773671, 33.06293181088029343 ) ) ;
#53850=EDGE_LOOP ( 'NONE', ( #40771, #50944, #65693, #19712 ) ) ;
#53851=EDGE_CURVE ( 'NONE', #68800, #45914, #75751, .T. ) ;
#53852=ADVANCED_FACE ( 'NONE', ( #26546 ), #61644, .F. ) ;
#53853=CARTESIAN_POINT ( 'NONE',  ( 7.976679284387491187, -4.299079248970732792, 33.91157788607253565 ) ) ;
#53854=EDGE_LOOP ( 'NONE', ( #15357, #14230, #52801, #84833 ) ) ;
#53856=CARTESIAN_POINT ( 'NONE',  ( 16.15384615384615330, -3.669653830205710676, 35.88435417666054406 ) ) ;
#53858=CARTESIAN_POINT ( 'NONE',  ( -6.989160334032800570, -3.513871655860377086, 32.76840700105978499 ) ) ;
#53859=CARTESIAN_POINT ( 'NONE',  ( 8.638539302563209787, -4.809359713505814149, 33.96456829005828837 ) ) ;
#53860=ORIENTED_EDGE ( 'NONE', *, *, #4362, .F. ) ;
#53861=LINE ( 'NONE', #81348, #80633 ) ;
#53862=CARTESIAN_POINT ( 'NONE',  ( -14.05763799605399278, -2.564540009722895419, 30.55348353981670684 ) ) ;
#53864=EDGE_CURVE ( 'NONE', #43306, #12236, #67975, .T. ) ;
#53865=EDGE_LOOP ( 'NONE', ( #3202, #34841, #2912, #33644 ) ) ;
#53867=CARTESIAN_POINT ( 'NONE',  ( 0.4615384615383396616, -2.892918686052166066, 31.69288490824153470 ) ) ;
#53868=CARTESIAN_POINT ( 'NONE',  ( -12.59168567097668934, -12.27039167877662251, 31.24851455888617835 ) ) ;
#53869=DIRECTION ( 'NONE',  ( -0.000000000000000000, 0.9848077530122085754, -0.1736481776669273613 ) ) ;
#53870=EDGE_CURVE ( 'NONE', #7171, #53, #2677, .T. ) ;
#53871=CARTESIAN_POINT ( 'NONE',  ( 8.096099364501988305, -3.202959910592335202, 32.30730279482227019 ) ) ;
#53872=EDGE_CURVE ( 'NONE', #49709, #34790, #16565, .T. ) ;
#53873=FACE_BOUND ( 'NONE', #61004, .T. ) ;
#53874=CARTESIAN_POINT ( 'NONE',  ( 13.25446741488369540, -12.15440758774515473, 32.17923288041532004 ) ) ;
#53875=CARTESIAN_POINT ( 'NONE',  ( 4.284636594813103549, -12.62708834333097663, 30.88030960425257021 ) ) ;
#53876=CARTESIAN_POINT ( 'NONE',  ( 2.057669083470851756, -10.18141759479407327, 34.26406193332782379 ) ) ;
#53877=CARTESIAN_POINT ( 'NONE',  ( -8.769230769230890843, -11.94971097300221174, 32.03036669348237098 ) ) ;
#53878=CARTESIAN_POINT ( 'NONE',  ( 17.93391658904412012, -11.16473453929635440, 33.15142922261925662 ) ) ;
#53879=CARTESIAN_POINT ( 'NONE',  ( -9.692307692307691624, -5.415277668671390821, 36.20867863119892149 ) ) ;
#53881=ADVANCED_FACE ( 'NONE', ( #67530 ), #82379, .F. ) ;
#53882=VERTEX_POINT ( 'NONE', #13024 ) ;
#53883=CARTESIAN_POINT ( 'NONE',  ( -12.39537185494681992, -7.250054591869670162, 34.99404684341514127 ) ) ;
#53885=CARTESIAN_POINT ( 'NONE',  ( -18.13069060311030611, -3.338472653186240091, 32.95098750199971960 ) ) ;
#53886=VERTEX_POINT ( 'NONE', #47693 ) ;
#53887=FACE_OUTER_BOUND ( 'NONE', #7842, .T. ) ;
#53888=DIRECTION ( 'NONE',  ( -0.000000000000000000, -0.5000000000000009992, -0.8660254037844380415 ) ) ;
#53889=CARTESIAN_POINT ( 'NONE',  ( 14.98076923076923173, -2.499999999999998668, 29.75000000000000355 ) ) ;
#53891=CARTESIAN_POINT ( 'NONE',  ( -14.30769230769230660, -1.367168528481310208, 33.57946703557072254 ) ) ;
#53892=CARTESIAN_POINT ( 'NONE',  ( -11.78848476268299628, -4.175268141568685643, 33.81360843649122216 ) ) ;
#53894=CARTESIAN_POINT ( 'NONE',  ( 2.057715576749954423, -11.79746400365624659, 32.30657167506340954 ) ) ;
#53895=CARTESIAN_POINT ( 'NONE',  ( -2.980769230769230393, -2.249999999999998668, 29.75000000000000355 ) ) ;
#53896=CARTESIAN_POINT ( 'NONE',  ( 3.230769230769231726, -2.499999999999998668, 29.75000000000001421 ) ) ;
#53897=CARTESIAN_POINT ( 'NONE',  ( 10.48469401227430886, -2.494641256782728966, 31.33461815524612959 ) ) ;
#53898=CARTESIAN_POINT ( 'NONE',  ( -0.3310127597748976913, -4.459921816937789885, 33.71989282347011851 ) ) ;
#53899=CARTESIAN_POINT ( 'NONE',  ( 9.469380733400843297, -3.395401636524185474, 33.02366814457250399 ) ) ;
#53901=CARTESIAN_POINT ( 'NONE',  ( -4.283994123577850921, -3.069018819979302926, 32.56621877034667278 ) ) ;
#53903=VERTEX_POINT ( 'NONE', #40075 ) ;
#53905=FACE_OUTER_BOUND ( 'NONE', #1540, .T. ) ;
#53908=CARTESIAN_POINT ( 'NONE',  ( 2.242422307135989890, -5.094484230520674117, 34.41647553114621161 ) ) ;
#53909=CARTESIAN_POINT ( 'NONE',  ( -5.076923076923197442, -2.625532179533778709, 30.86335684631627174 ) ) ;
#53910=VERTEX_POINT ( 'NONE', #88270 ) ;
#53911=CARTESIAN_POINT ( 'NONE',  ( 14.30769230769231015, -9.780366693483667717, 34.19971097300155094 ) ) ;
#53912=CARTESIAN_POINT ( 'NONE',  ( -16.85391023282967993, -9.172514111537580561, 34.72667873470787470 ) ) ;
#53913=CARTESIAN_POINT ( 'NONE',  ( -17.14267987943738802, -7.249945686854186278, 34.74374336980224598 ) ) ;
#53915=CARTESIAN_POINT ( 'NONE',  ( 12.71159277317677905, -12.41262288849542017, 30.68299917996395010 ) ) ;
#53916=DIRECTION ( 'NONE',  ( -0.000000000000000000, 0.1736481776669307198, -0.9848077530122080203 ) ) ;
#53917=CARTESIAN_POINT ( 'NONE',  ( -12.52762084089859407, -4.661471528628507777, 34.16647553114621871 ) ) ;
#53919=CARTESIAN_POINT ( 'NONE',  ( 2.980792486720641676, -2.544273027872574922, 31.48422191005632342 ) ) ;
#53920=CARTESIAN_POINT ( 'NONE',  ( 15.23076923076910916, -12.70778746994576025, 30.41441678777401236 ) ) ;
#53921=B_SPLINE_CURVE_WITH_KNOTS ( 'NONE', 3,
 ( #7786, #52193, #60286, #29833, #57295, #17985, #31943, #45436, #87798, #84789 ),
 .UNSPECIFIED., .F., .F.,
 ( 4, 2, 2, 2, 4 ),
 ( 0.000000000000000000, 0.0001954311564186876876, 0.0003908623128373753751, 0.0005862934692560630356, 0.0007817246256747507503 ),
 .UNSPECIFIED. ) ;
#53922=DIRECTION ( 'NONE',  ( -0.000000000000000000, -0.9848077530122086864, -0.1736481776669273613 ) ) ;
#53923=ORIENTED_EDGE ( 'NONE', *, *, #26142, .T. ) ;
#53924=ORIENTED_EDGE ( 'NONE', *, *, #21387, .T. ) ;
#53925=ORIENTED_EDGE ( 'NONE', *, *, #54569, .T. ) ;
#53926=ORIENTED_EDGE ( 'NONE', *, *, #14215, .T. ) ;
#53927=CARTESIAN_POINT ( 'NONE',  ( 12.59206389977210705, -10.31582465632705237, 34.18122507451815295 ) ) ;
#53928=CARTESIAN_POINT ( 'NONE',  ( 8.769230769230768274, -1.242168528481310874, 33.36296068462461051 ) ) ;
#53929=CARTESIAN_POINT ( 'NONE',  ( -11.40793610022789650, -3.625058011473228703, 33.29252011169590020 ) ) ;
#53930=DIRECTION ( 'NONE',  ( 0.000000000000000000, 1.000000000000000000, 0.000000000000000000 ) ) ;
#53932=EDGE_CURVE ( 'NONE', #82469, #32624, #78948, .T. ) ;
#53933=CARTESIAN_POINT ( 'NONE',  ( 5.299702618191482806, -5.913360116392398780, 34.49180327182771322 ) ) ;
#53935=ORIENTED_EDGE ( 'NONE', *, *, #58792, .F. ) ;
#53937=DIRECTION ( 'NONE',  ( -0.000000000000000000, -0.3420201433256694901, -0.9396926207859082059 ) ) ;
#53938=VERTEX_POINT ( 'NONE', #12148 ) ;
#53940=CARTESIAN_POINT ( 'NONE',  ( 14.98074599347626368, -3.202444869320336451, 32.30641848906366675 ) ) ;
#53941=CARTESIAN_POINT ( 'NONE',  ( 5.749976775778542937, -4.175268141568689195, 33.81360843649122216 ) ) ;
#53943=CARTESIAN_POINT ( 'NONE',  ( 15.93036122928182330, -11.60425143139329940, 33.02411095842164457 ) ) ;
#53944=ORIENTED_EDGE ( 'NONE', *, *, #68429, .T. ) ;
#53946=ORIENTED_EDGE ( 'NONE', *, *, #33136, .T. ) ;
#53947=CARTESIAN_POINT ( 'NONE',  ( -9.627052121031667298, -6.026961402152789304, 34.52809138561124769 ) ) ;
#53948=CARTESIAN_POINT ( 'NONE',  ( 11.53846153846153832, -2.249999999999998668, 29.50000000000001421 ) ) ;
#53949=EDGE_LOOP ( 'NONE', ( #81434, #19459 ) ) ;
#53950=CARTESIAN_POINT ( 'NONE',  ( -5.999999999999998224, -5.180354513474913603, 36.12317359536750416 ) ) ;
#53951=B_SPLINE_CURVE_WITH_KNOTS ( 'NONE', 3,
 ( #17210, #2355, #50546, #23519, #64490, #72150, #78462, #17667, #36174, #78028 ),
 .UNSPECIFIED., .F., .F.,
 ( 4, 2, 2, 2, 4 ),
 ( 0.0007817246256747483650, 0.0009771112852218926705, 0.001172497944769037084, 0.001367884604316181498, 0.001563271263863325695 ),
 .UNSPECIFIED. ) ;
#53952=VECTOR ( 'NONE', #74820, 1000.000000000000000 ) ;
#53953=CARTESIAN_POINT ( 'NONE',  ( -0.4615384615385840772, -6.835583212225970762, 34.95778746994575670 ) ) ;
#53954=EDGE_LOOP ( 'NONE', ( #3402, #65364, #13380, #53540 ) ) ;
#53956=CARTESIAN_POINT ( 'NONE',  ( 18.00000000000000000, -13.37000171582298513, 34.34916445242398453 ) ) ;
#53957=CARTESIAN_POINT ( 'NONE',  ( -17.07692307692307665, -12.78798330534102945, 29.74999999999997868 ) ) ;
#53959=FACE_BOUND ( 'NONE', #4929, .T. ) ;
#53962=CARTESIAN_POINT ( 'NONE',  ( 11.53846153846153832, -12.37446782046654192, 30.86335684631486131 ) ) ;
#53963=CARTESIAN_POINT ( 'NONE',  ( 0.2380535369741297591, -6.716662450894490100, 34.94144148231605840 ) ) ;
#53964=CARTESIAN_POINT ( 'NONE',  ( 6.792386319966619013, -10.70098750199973203, 33.91152734681376302 ) ) ;
#53966=CARTESIAN_POINT ( 'NONE',  ( -0.5268089074992371446, -3.835265460703609186, 33.15142922261924241 ) ) ;
#53968=CARTESIAN_POINT ( 'NONE',  ( -14.98082382139119062, -11.56426240980093745, 33.07394671870546432 ) ) ;
#53969=AXIS2_PLACEMENT_3D ( 'NONE', #46745, #75118, #89089 ) ;
#53970=CARTESIAN_POINT ( 'NONE',  ( 0.3308478584281538404, -10.70098750199973203, 33.91152734681376302 ) ) ;
#53971=ORIENTED_EDGE ( 'NONE', *, *, #64272, .F. ) ;
#53972=EDGE_LOOP ( 'NONE', ( #46703, #69790 ) ) ;
#53973=CARTESIAN_POINT ( 'NONE',  ( 0.4615384615384611200, -8.164416787775445883, 34.95778746994557906 ) ) ;
#53974=CARTESIAN_POINT ( 'NONE',  ( -13.60754234352223335, -4.762599654559228846, 34.23009711892697737 ) ) ;
#53975=CARTESIAN_POINT ( 'NONE',  ( -11.78843828251013015, -10.06842814019191401, 34.32929386961144758 ) ) ;
#53976=ORIENTED_EDGE ( 'NONE', *, *, #87891, .F. ) ;
#53977=LINE ( 'NONE', #81469, #11167 ) ;
#53978=ADVANCED_FACE ( 'NONE', ( #33305 ), #49900, .F. ) ;
#53979=EDGE_CURVE ( 'NONE', #80426, #62209, #28366, .T. ) ;
#53980=CARTESIAN_POINT ( 'NONE',  ( 6.700149964170072359, -8.282780595021769443, 34.94152052738834868 ) ) ;
#53981=FACE_BOUND ( 'NONE', #53767, .T. ) ;
#53984=CARTESIAN_POINT ( 'NONE',  ( 7.846153846153846700, -8.973038597847269315, 34.52809138561121927 ) ) ;
#53985=CARTESIAN_POINT ( 'NONE',  ( 2.373760658694747061, -4.786620604624113540, 33.94971097300155805 ) ) ;
#53987=CARTESIAN_POINT ( 'NONE',  ( 0.3308469948709015784, -5.582088688514999397, 34.36776431015576350 ) ) ;
#53989=VERTEX_POINT ( 'NONE', #62959 ) ;
#53990=ORIENTED_EDGE ( 'NONE', *, *, #81263, .T. ) ;
#53991=CARTESIAN_POINT ( 'NONE',  ( 0.4615384615384611755, -12.48256725967547354, 35.29906147534542527 ) ) ;
#53992=CARTESIAN_POINT ( 'NONE',  ( 16.15384615384603251, -6.879047030192662504, 34.71129190930017927 ) ) ;
#53993=CARTESIAN_POINT ( 'NONE',  ( 13.38461538461538680, -1.129524287112498415, 32.06866353760679544 ) ) ;
#53994=DIRECTION ( 'NONE',  ( -0.000000000000000000, 0.1736481776669307198, -0.9848077530122080203 ) ) ;
#53995=CARTESIAN_POINT ( 'NONE',  ( -7.622778360381425422, -2.251407671071268712, 29.88021292934942252 ) ) ;
#53997=LINE ( 'NONE', #40505, #23045 ) ;
#53998=CARTESIAN_POINT ( 'NONE',  ( -6.223484924564328225, -8.539481045369598178, 34.89627647299170832 ) ) ;
#53999=CARTESIAN_POINT ( 'NONE',  ( -4.946132635956127288, -2.295524264805589354, 30.44142389570982488 ) ) ;
#54000=CARTESIAN_POINT ( 'NONE',  ( 10.74591005361826390, -3.625058011473228703, 33.29252011169590020 ) ) ;
#54001=CARTESIAN_POINT ( 'NONE',  ( -6.000000000000119904, -2.892918686052165622, 31.69288490824153470 ) ) ;
#54002=CARTESIAN_POINT ( 'NONE',  ( 15.16468685140909400, -12.34228464037088280, 31.77849191805838558 ) ) ;
#54003=CARTESIAN_POINT ( 'NONE',  ( -0.3307480205715105370, -3.957578996910242619, 33.62503395064540257 ) ) ;
#54004=CARTESIAN_POINT ( 'NONE',  ( -8.638440328263817136, -11.37503395064541678, 33.29242100308974273 ) ) ;
#54005=CARTESIAN_POINT ( 'NONE',  ( -7.780085495151406683, -12.37446782046654192, 30.86335684631486842 ) ) ;
#54006=EDGE_LOOP ( 'NONE', ( #28617, #303, #72468, #77906 ) ) ;
#54007=CARTESIAN_POINT ( 'NONE',  ( -4.946131269098290595, -11.71459661697925903, 32.44059661609676937 ) ) ;
#54008=CARTESIAN_POINT ( 'NONE',  ( 5.076923076923075762, -6.189225973068211317, 35.74407628777942847 ) ) ;
#54010=CARTESIAN_POINT ( 'NONE',  ( -9.692307692307691624, -10.67929555188718282, 33.92786785259544047 ) ) ;
#54011=DIRECTION ( 'NONE',  ( 0.000000000000000000, 0.1736481776669267785, -0.9848077530122087975 ) ) ;
#54012=CARTESIAN_POINT ( 'NONE',  ( 6.923076923076924238, -2.708943851104267164, 35.45975837776705220 ) ) ;
#54013=VERTEX_POINT ( 'NONE', #76942 ) ;
#54016=B_SPLINE_CURVE_WITH_KNOTS ( 'NONE', 3,
 ( #10120, #5594, #31284, #4709, #33063, #81260, #66849, #60530, #79919, #39391 ),
 .UNSPECIFIED., .F., .F.,
 ( 4, 2, 2, 2, 4 ),
 ( 0.0007817246256747514008, 0.0009771112852218952725, 0.001172497944769039036, 0.001367884604316182799, 0.001563271263863326779 ),
 .UNSPECIFIED. ) ;
#54017=ORIENTED_EDGE ( 'NONE', *, *, #87906, .F. ) ;
#54018=CARTESIAN_POINT ( 'NONE',  ( -16.02332045208259359, -10.19071101563364401, 33.96452234770658407 ) ) ;
#54019=CARTESIAN_POINT ( 'NONE',  ( -17.75005448165186195, -3.712312575010499494, 33.01462480002815880 ) ) ;
#54020=ORIENTED_EDGE ( 'NONE', *, *, #16201, .T. ) ;
#54021=DIRECTION ( 'NONE',  ( -0.000000000000000000, -0.7660444431189791237, -0.6427876096865379196 ) ) ;
#54022=CARTESIAN_POINT ( 'NONE',  ( -15.36124441584495237, -7.276987145209185215, 34.99546412871779211 ) ) ;
#54023=AXIS2_PLACEMENT_3D ( 'NONE', #34491, #61955, #16001 ) ;
#54024=CARTESIAN_POINT ( 'NONE',  ( 2.242422307135989890, -12.70778746994557551, 30.41441678777548319 ) ) ;
#54026=EDGE_LOOP ( 'NONE', ( #51226, #43033, #61237, #50451 ) ) ;
#54027=ORIENTED_EDGE ( 'NONE', *, *, #28027, .F. ) ;
#54028=CARTESIAN_POINT ( 'NONE',  ( -18.00000000000000000, -4.661471528628506000, 34.16647553114623292 ) ) ;
#54029=CYLINDRICAL_SURFACE ( 'NONE', #72823, 0.2499999999999994726 ) ;
#54030=CARTESIAN_POINT ( 'NONE',  ( 18.13079044096694759, -9.929761469519743144, 34.40412654351204225 ) ) ;
#54031=CARTESIAN_POINT ( 'NONE',  ( -17.20707028636129721, -6.001485441113818986, 34.52039167877662607 ) ) ;
#54032=DIRECTION ( 'NONE',  ( 0.000000000000000000, 0.7660444431189807890, 0.6427876096865361433 ) ) ;
#54033=CARTESIAN_POINT ( 'NONE',  ( 9.942253101685738059, -10.18230066228895758, 34.26354781536631577 ) ) ;
#54034=CARTESIAN_POINT ( 'NONE',  ( 1.384615384615264011, -2.379036618888197285, 30.90682066428292885 ) ) ;
#54035=ADVANCED_FACE ( 'NONE', ( #14349 ), #84599, .F. ) ;
#54036=CARTESIAN_POINT ( 'NONE',  ( 16.02369818411445479, -12.70455904226513866, 30.44083106164009322 ) ) ;
#54037=EDGE_CURVE ( 'NONE', #17526, #4994, #36403, .T. ) ;
#54039=ORIENTED_EDGE ( 'NONE', *, *, #78853, .F. ) ;
#54041=ORIENTED_EDGE ( 'NONE', *, *, #32699, .T. ) ;
#54042=EDGE_CURVE ( 'NONE', #56376, #67556, #58505, .T. ) ;
#54045=CARTESIAN_POINT ( 'NONE',  ( 12.52760681254089903, -3.050289026998446840, 32.03036669348366416 ) ) ;
#54046=ADVANCED_FACE ( 'NONE', ( #28762 ), #15247, .F. ) ;
#54047=ORIENTED_EDGE ( 'NONE', *, *, #35494, .T. ) ;
#54048=CARTESIAN_POINT ( 'NONE',  ( -12.39547112818838670, -11.35647404775217595, 33.31231777344666511 ) ) ;
#54049=ORIENTED_EDGE ( 'NONE', *, *, #48643, .T. ) ;
#54050=CARTESIAN_POINT ( 'NONE',  ( 0.2115384615384616196, -2.499999999999998668, 29.75000000000000355 ) ) ;
#54051=ORIENTED_EDGE ( 'NONE', *, *, #87230, .F. ) ;
#54052=DIRECTION ( 'NONE',  ( -0.000000000000000000, 1.000000000000000000, -0.000000000000000000 ) ) ;
#54053=EDGE_CURVE ( 'NONE', #45298, #38438, #22869, .T. ) ;
#54054=CARTESIAN_POINT ( 'NONE',  ( -12.33101302330481985, -10.31582465632705237, 34.18122507451815295 ) ) ;
#54055=CARTESIAN_POINT ( 'NONE',  ( -8.992156986746914882, -2.758268499246657068, 31.33685645148948140 ) ) ;
#54056=FACE_BOUND ( 'NONE', #62133, .T. ) ;
#54057=B_SPLINE_CURVE_WITH_KNOTS ( 'NONE', 3,
 ( #3810, #19877, #3362, #31290, #86252, #47343 ),
 .UNSPECIFIED., .F., .F.,
 ( 4, 2, 4 ),
 ( 4.220987180333913997E-17, 0.0001954756301637161793, 0.0003909512603273901832 ),
 .UNSPECIFIED. ) ;
#54058=DIRECTION ( 'NONE',  ( 0.000000000000000000, 0.7660444431189822323, -0.6427876096865344779 ) ) ;
#54059=CARTESIAN_POINT ( 'NONE',  ( 1.634615384615449862, -7.434744860731434812, 35.00000000000000711 ) ) ;
#54062=CARTESIAN_POINT ( 'NONE',  ( 10.55006060258030942, -7.749976730030849303, 34.74374725381503737 ) ) ;
#54063=CARTESIAN_POINT ( 'NONE',  ( 16.15384615384615330, -4.098570777380720287, 33.41473453929634729 ) ) ;
#54064=CARTESIAN_POINT ( 'NONE',  ( -13.13461538461538325, -2.499999999999999556, 29.81604066197449754 ) ) ;
#54065=EDGE_LOOP ( 'NONE', ( #44292, #6260 ) ) ;
#54066=EDGE_LOOP ( 'NONE', ( #28888, #37490 ) ) ;
#54067=CARTESIAN_POINT ( 'NONE',  ( -5.076923076923075762, -11.91647553114624181, 32.58852847137148245 ) ) ;
#54069=DIRECTION ( 'NONE',  ( -0.000000000000000000, 0.3420201433256694901, -0.9396926207859082059 ) ) ;
#54070=CARTESIAN_POINT ( 'NONE',  ( 14.30769230769218581, -11.06231777344772027, 33.60647404775119895 ) ) ;
#54071=CARTESIAN_POINT ( 'NONE',  ( 16.94677586748485965, -8.587444163452046197, 34.63053765926554206 ) ) ;
#54072=CARTESIAN_POINT ( 'NONE',  ( -12.23852710992561121, -4.187068189119699468, 33.49521262558774026 ) ) ;
#54073=ORIENTED_EDGE ( 'NONE', *, *, #64333, .F. ) ;
#54075=EDGE_CURVE ( 'NONE', #70832, #88089, #46728, .T. ) ;
#54076=CARTESIAN_POINT ( 'NONE',  ( -6.000000000000121680, -8.656820664282941280, 34.87096338111179961 ) ) ;
#54077=CARTESIAN_POINT ( 'NONE',  ( 11.28846153846153832, -7.500000000000001776, 34.75000000000000000 ) ) ;
#54078=CARTESIAN_POINT ( 'NONE',  ( -8.899377978668994160, -12.27039167877662251, 31.24851455888617835 ) ) ;
#54080=DIRECTION ( 'NONE',  ( -0.000000000000000000, -0.3420201433256694901, -0.9396926207859082059 ) ) ;
#54081=VERTEX_POINT ( 'NONE', #82823 ) ;
#54082=B_SPLINE_CURVE_WITH_KNOTS ( 'NONE', 3,
 ( #54063, #13972, #81560, #27049, #60830, #19847, #48637, #54512, #5454, #34695 ),
 .UNSPECIFIED., .F., .F.,
 ( 4, 2, 2, 2, 4 ),
 ( 0.000000000000000000, 0.0001954339857564078538, 0.0003908679715128157077, 0.0005863019572692235344, 0.0007817359430256314154 ),
 .UNSPECIFIED. ) ;
#54083=ORIENTED_EDGE ( 'NONE', *, *, #2057, .F. ) ;
#54084=ORIENTED_EDGE ( 'NONE', *, *, #37512, .F. ) ;
#54085=EDGE_CURVE ( 'NONE', #80199, #38257, #15471, .T. ) ;
#54086=CYLINDRICAL_SURFACE ( 'NONE', #80898, 0.2500000000000012212 ) ;
#54087=ADVANCED_FACE ( 'NONE', ( #30952 ), #85030, .F. ) ;
#54088=ORIENTED_EDGE ( 'NONE', *, *, #45591, .T. ) ;
#54089=VECTOR ( 'NONE', #10650, 1000.000000000000000 ) ;
#54090=FACE_OUTER_BOUND ( 'NONE', #80939, .T. ) ;
#54091=CARTESIAN_POINT ( 'NONE',  ( 14.55763771707034948, -5.766571408460171355, 34.70601412856602508 ) ) ;
#54092=CARTESIAN_POINT ( 'NONE',  ( 16.15384615384603251, -8.613356846316285953, 34.62446782046622218 ) ) ;
#54093=CARTESIAN_POINT ( 'NONE',  ( 8.769230769230768274, -3.322132147404559976, 32.92929555188717927 ) ) ;
#54094=CARTESIAN_POINT ( 'NONE',  ( -5.999999999999998224, -9.819645486525091727, 36.12317359536749706 ) ) ;
#54095=ORIENTED_EDGE ( 'NONE', *, *, #67646, .F. ) ;
#54096=CARTESIAN_POINT ( 'NONE',  ( 12.68496486045324900, -7.630147987733840509, 34.99859428049665411 ) ) ;
#54097=CARTESIAN_POINT ( 'NONE',  ( -2.307692307692428724, -3.643525952248796163, 33.31231777344771672 ) ) ;
#54098=ORIENTED_EDGE ( 'NONE', *, *, #56596, .T. ) ;
#54099=FACE_OUTER_BOUND ( 'NONE', #77184, .T. ) ;
#54100=DIRECTION ( 'NONE',  ( 0.000000000000000000, 0.6427876096865368094, 0.7660444431189802339 ) ) ;
#54101=CARTESIAN_POINT ( 'NONE',  ( 16.15384615384603251, -3.835265460704628815, 33.15142922262033665 ) ) ;
#54102=CARTESIAN_POINT ( 'NONE',  ( -2.307692307692305711, -12.62096338111211580, 30.90682066428153263 ) ) ;
#54103=CARTESIAN_POINT ( 'NONE',  ( 2.557637717070350813, -2.589246495874657938, 31.60778113518102828 ) ) ;
#54104=DIRECTION ( 'NONE',  ( -0.000000000000000000, -0.9396926207859092051, -0.3420201433256662704 ) ) ;
#54105=FACE_OUTER_BOUND ( 'NONE', #70294, .T. ) ;
#54107=ORIENTED_EDGE ( 'NONE', *, *, #65796, .F. ) ;
#54109=CARTESIAN_POINT ( 'NONE',  ( -1.134669975237340589, -3.520799739797214389, 33.17531984108286025 ) ) ;
#54110=AXIS2_PLACEMENT_3D ( 'NONE', #87493, #40188, #73964 ) ;
#54111=ORIENTED_EDGE ( 'NONE', *, *, #49496, .T. ) ;
#54112=ORIENTED_EDGE ( 'NONE', *, *, #5926, .F. ) ;
#54113=CARTESIAN_POINT ( 'NONE',  ( -12.59168567097668401, -11.93770438780619259, 32.05411857736982029 ) ) ;
#54114=DIRECTION ( 'NONE',  ( -0.000000000000000000, -0.7660444431189791237, -0.6427876096865379196 ) ) ;
#54115=B_SPLINE_CURVE_WITH_KNOTS ( 'NONE', 3,
 ( #42898, #62700, #22179, #76223, #69031, #1464, #28952, #42014, #55071, #1017 ),
 .UNSPECIFIED., .F., .F.,
 ( 4, 2, 2, 2, 4 ),
 ( 0.0007817246256747463051, 0.0009771112852218887673, 0.001172497944769031446, 0.001367884604316173909, 0.001563271263863316371 ),
 .UNSPECIFIED. ) ;
#54116=VECTOR ( 'NONE', #57007, 1000.000000000000000 ) ;
#54117=DIRECTION ( 'NONE',  ( 0.000000000000000000, 0.9848077530122072432, 0.1736481776669354937 ) ) ;
#54118=CARTESIAN_POINT ( 'NONE',  ( -4.153846153846152411, -11.69971097300155272, 32.46337939537588113 ) ) ;
#54119=CARTESIAN_POINT ( 'NONE',  ( 17.77651507543566822, -2.612411019501191589, 31.66733052389440672 ) ) ;
#54121=ADVANCED_FACE ( 'NONE', ( #44025 ), #25096, .F. ) ;
#54122=CARTESIAN_POINT ( 'NONE',  ( -16.15384615384615330, -6.343179335718451384, 34.87096338111211935 ) ) ;
#54123=CARTESIAN_POINT ( 'NONE',  ( -14.53061852520845321, -2.758268499246657068, 31.33685645148948140 ) ) ;
#54124=CARTESIAN_POINT ( 'NONE',  ( -16.15384615384627409, -2.379036618888197285, 30.90682066428292885 ) ) ;
#54126=CARTESIAN_POINT ( 'NONE',  ( -16.94613263595612906, -11.93129842949672437, 32.56571108434900452 ) ) ;
#54127=ORIENTED_EDGE ( 'NONE', *, *, #27013, .F. ) ;
#54128=DIRECTION ( 'NONE',  ( -0.000000000000000000, -0.8660254037844399289, -0.4999999999999980016 ) ) ;
#54129=CARTESIAN_POINT ( 'NONE',  ( 11.53846153846153832, -2.486705287966279876, 31.30864560766543647 ) ) ;
#54130=VERTEX_POINT ( 'NONE', #44911 ) ;
#54131=CARTESIAN_POINT ( 'NONE',  ( 0.4615384615384611200, -2.249999999999998668, 29.75000000000001776 ) ) ;
#54132=CARTESIAN_POINT ( 'NONE',  ( -6.065270000556318486, -2.379036618887870436, 30.90682066428147934 ) ) ;
#54133=CARTESIAN_POINT ( 'NONE',  ( 12.46153846153846168, -13.95598074871891292, 31.83374038241031911 ) ) ;
#54134=EDGE_CURVE ( 'NONE', #69108, #88101, #3922, .T. ) ;
#54135=DIRECTION ( 'NONE',  ( -0.000000000000000000, 0.3420201433256694901, -0.9396926207859082059 ) ) ;
#54136=DIRECTION ( 'NONE',  ( -0.000000000000000000, -0.8660254037844397068, -0.4999999999999978906 ) ) ;
#54137=AXIS2_PLACEMENT_3D ( 'NONE', #70954, #37159, #56988 ) ;
#54138=ORIENTED_EDGE ( 'NONE', *, *, #39214, .F. ) ;
#54139=DIRECTION ( 'NONE',  ( 0.000000000000000000, 0.3420201433256610524, 0.9396926207859113145 ) ) ;
#54142=FACE_OUTER_BOUND ( 'NONE', #17398, .T. ) ;
#54143=B_SPLINE_CURVE_WITH_KNOTS ( 'NONE', 3,
 ( #30769, #85728, #84406, #78076, #43844, #30334, #51919, #24008, #51460, #84852 ),
 .UNSPECIFIED., .F., .F.,
 ( 4, 2, 2, 2, 4 ),
 ( 0.0007817246256747470640, 0.0009771112852218898515, 0.001172497944769032747, 0.001367884604316175643, 0.001563271263863318539 ),
 .UNSPECIFIED. ) ;
#54144=EDGE_CURVE ( 'NONE', #71169, #40972, #51654, .T. ) ;
#54145=CARTESIAN_POINT ( 'NONE',  ( -18.24997674404859183, -10.82459398097509862, 33.81372124010183455 ) ) ;
#54146=AXIS2_PLACEMENT_3D ( 'NONE', #11828, #39307, #19025 ) ;
#54147=CYLINDRICAL_SURFACE ( 'NONE', #57891, 0.2500000000000004996 ) ;
#54148=CARTESIAN_POINT ( 'NONE',  ( 16.94623161025552349, -2.541943142973489334, 30.39792223712631980 ) ) ;
#54149=EDGE_CURVE ( 'NONE', #24050, #40179, #70163, .T. ) ;
#54150=ORIENTED_EDGE ( 'NONE', *, *, #60176, .F. ) ;
#54151=ORIENTED_EDGE ( 'NONE', *, *, #13821, .T. ) ;
#54152=ORIENTED_EDGE ( 'NONE', *, *, #60809, .T. ) ;
#54154=CARTESIAN_POINT ( 'NONE',  ( -4.403822884788507253, -5.728515186090277211, 34.42611988154120439 ) ) ;
#54156=CARTESIAN_POINT ( 'NONE',  ( 16.40390057375961064, -10.82426656108011720, 33.81400080652039009 ) ) ;
#54158=CARTESIAN_POINT ( 'NONE',  ( -7.976844449264153702, -3.338472653186243644, 32.95098750199972670 ) ) ;
#54159=ORIENTED_EDGE ( 'NONE', *, *, #5266, .T. ) ;
#54160=CYLINDRICAL_SURFACE ( 'NONE', #31259, 0.2499999999999995559 ) ;
#54161=EDGE_CURVE ( 'NONE', #38632, #72796, #72393, .T. ) ;
#54162=CIRCLE ( 'NONE', #72874, 0.2500000000000002220 ) ;
#54164=CARTESIAN_POINT ( 'NONE',  ( -2.241623956689867914, -3.513871655860379306, 32.76840700105978499 ) ) ;
#54165=CARTESIAN_POINT ( 'NONE',  ( -5.011667937410240192, -11.67786785259547777, 32.92929555188713664 ) ) ;
#54166=ORIENTED_EDGE ( 'NONE', *, *, #54814, .T. ) ;
#54167=EDGE_CURVE ( 'NONE', #69237, #85805, #24649, .T. ) ;
#54168=ORIENTED_EDGE ( 'NONE', *, *, #32820, .F. ) ;
#54170=LINE ( 'NONE', #5113, #33030 ) ;
#54171=ORIENTED_EDGE ( 'NONE', *, *, #26653, .F. ) ;
#54172=CARTESIAN_POINT ( 'NONE',  ( -4.153846153846152411, -3.886160181151819604, 36.00935417666054406 ) ) ;
#54175=CARTESIAN_POINT ( 'NONE',  ( 16.15384615384615330, -6.435427911321262684, 35.78748833219616898 ) ) ;
#54176=FACE_BOUND ( 'NONE', #12082, .T. ) ;
#54177=ORIENTED_EDGE ( 'NONE', *, *, #63895, .F. ) ;
#54178=ADVANCED_FACE ( 'NONE', ( #3482 ), #3035, .T. ) ;
#54179=CARTESIAN_POINT ( 'NONE',  ( 17.01083966596719677, -6.386643153685125363, 34.62446782046654903 ) ) ;
#54180=DIRECTION ( 'NONE',  ( -0.000000000000000000, 0.5000000000000011102, -0.8660254037844381525 ) ) ;
#54181=ORIENTED_EDGE ( 'NONE', *, *, #70562, .T. ) ;
#54182=CARTESIAN_POINT ( 'NONE',  ( -10.61538461538461320, -2.249999999999998668, 29.50000000000001421 ) ) ;
#54183=VERTEX_POINT ( 'NONE', #38613 ) ;
#54184=EDGE_CURVE ( 'NONE', #66121, #36550, #68108, .T. ) ;
#54185=FACE_BOUND ( 'NONE', #28944, .T. ) ;
#54187=CARTESIAN_POINT ( 'NONE',  ( 18.25005431163831204, -4.943051570960395047, 34.04725096376909477 ) ) ;
#54188=VERTEX_POINT ( 'NONE', #30518 ) ;
#54189=CARTESIAN_POINT ( 'NONE',  ( -12.23875892027004753, -8.496831190052096971, 34.64984203495476578 ) ) ;
#54190=CARTESIAN_POINT ( 'NONE',  ( 16.82689985270161870, -12.07920672191015221, 32.31858351112116168 ) ) ;
#54191=EDGE_CURVE ( 'NONE', #88099, #72117, #57989, .T. ) ;
#54192=CARTESIAN_POINT ( 'NONE',  ( 1.134592147322420752, -3.202444869320336451, 32.30641848906366675 ) ) ;
#54193=ORIENTED_EDGE ( 'NONE', *, *, #74155, .T. ) ;
#54194=DIRECTION ( 'NONE',  ( -0.000000000000000000, 0.6427876096865404731, -0.7660444431189770143 ) ) ;
#54195=CARTESIAN_POINT ( 'NONE',  ( 14.43848274865926129, -3.338503747796866872, 32.95102852606553512 ) ) ;
#54196=CARTESIAN_POINT ( 'NONE',  ( 18.00000000000000000, -10.67929555188718282, 33.92786785259544047 ) ) ;
#54197=CARTESIAN_POINT ( 'NONE',  ( -9.692307692307812417, -2.625532179533778709, 30.86335684631627174 ) ) ;
#54198=ORIENTED_EDGE ( 'NONE', *, *, #78241, .T. ) ;
#54199=CARTESIAN_POINT ( 'NONE',  ( -1.384615384615383471, -5.557115091759785130, 34.35708131394839171 ) ) ;
#54201=EDGE_LOOP ( 'NONE', ( #46629, #68349, #50462, #31341 ) ) ;
#54203=CARTESIAN_POINT ( 'NONE',  ( 15.93091919493929964, -4.026226216239093603, 33.68668979543632958 ) ) ;
#54204=CARTESIAN_POINT ( 'NONE',  ( -7.976301815885545210, -12.50552854090298993, 31.33409797877408920 ) ) ;
#54205=CARTESIAN_POINT ( 'NONE',  ( 13.45068373561782415, -12.37446782046654192, 30.86335684631486842 ) ) ;
#54206=CARTESIAN_POINT ( 'NONE',  ( 0.3308478584281552837, -2.494641256782729410, 31.33461815524612248 ) ) ;
#54209=CARTESIAN_POINT ( 'NONE',  ( -5.076923076923197442, -10.21337939537710326, 33.94971097300076224 ) ) ;
#54211=CYLINDRICAL_SURFACE ( 'NONE', #33464, 0.2500000000000009437 ) ;
#54214=ORIENTED_EDGE ( 'NONE', *, *, #8557, .F. ) ;
#54215=DIRECTION ( 'NONE',  ( -0.000000000000000000, -0.9396926207859093161, -0.3420201433256663259 ) ) ;
#54216=ORIENTED_EDGE ( 'NONE', *, *, #36048, .F. ) ;
#54217=EDGE_CURVE ( 'NONE', #27545, #38500, #43375, .T. ) ;
#54218=ORIENTED_EDGE ( 'NONE', *, *, #87179, .F. ) ;
#54219=CARTESIAN_POINT ( 'NONE',  ( 2.307692307692309264, -3.669653830205710676, 35.88435417666054406 ) ) ;
#54220=VECTOR ( 'NONE', #53766, 1000.000000000000227 ) ;
#54221=ORIENTED_EDGE ( 'NONE', *, *, #25976, .T. ) ;
#54222=CARTESIAN_POINT ( 'NONE',  ( -4.153846153846274980, -2.657715359629662988, 31.77849191805970364 ) ) ;
#54224=CARTESIAN_POINT ( 'NONE',  ( 13.63466969625370417, -2.779044189368095719, 31.39831045268885745 ) ) ;
#54225=DIRECTION ( 'NONE',  ( -0.000000000000000000, 0.3420201433256694901, -0.9396926207859082059 ) ) ;
#54226=CARTESIAN_POINT ( 'NONE',  ( -2.177166605928742893, -6.852161475712352789, 34.70806712695775786 ) ) ;
#54227=CARTESIAN_POINT ( 'NONE',  ( -11.53846153846165912, -11.48612834414049644, 32.76840700105863391 ) ) ;
#54228=CARTESIAN_POINT ( 'NONE',  ( -13.63463862190834952, -2.587272538249755893, 30.68239716806877837 ) ) ;
#54229=LINE ( 'NONE', #6506, #15241 ) ;
#54231=EDGE_CURVE ( 'NONE', #10613, #36751, #88606, .T. ) ;
#54232=CARTESIAN_POINT ( 'NONE',  ( 5.142178216435912219, -3.083524468853784839, 32.58852847137153930 ) ) ;
#54233=CARTESIAN_POINT ( 'NONE',  ( -14.53055772989594807, -2.501496062324912284, 29.88072118266895671 ) ) ;
#54234=CARTESIAN_POINT ( 'NONE',  ( 5.750023255951411727, -11.47974371597207899, 33.17467449705390692 ) ) ;
#54235=EDGE_CURVE ( 'NONE', #34985, #62741, #62655, .T. ) ;
#54236=EDGE_CURVE ( 'NONE', #79333, #19438, #83091, .T. ) ;
#54237=VERTEX_POINT ( 'NONE', #40404 ) ;
#54238=ORIENTED_EDGE ( 'NONE', *, *, #4871, .F. ) ;
#54239=AXIS2_PLACEMENT_3D ( 'NONE', #26944, #20186, #47651 ) ;
#54240=CARTESIAN_POINT ( 'NONE',  ( -8.992156986746914882, -12.39988816332205701, 30.74660775122750778 ) ) ;
#54241=CARTESIAN_POINT ( 'NONE',  ( 0.5923289025054093715, -11.93129842949671726, 32.56571108434900452 ) ) ;
#54244=CARTESIAN_POINT ( 'NONE',  ( 5.999999999999880096, -5.219633306517616589, 34.19971097300220464 ) ) ;
#54245=CARTESIAN_POINT ( 'NONE',  ( -13.60754234352223158, -10.77366814457252175, 33.85459836347579454 ) ) ;
#54246=EDGE_CURVE ( 'NONE', #75680, #42058, #65846, .T. ) ;
#54248=VERTEX_POINT ( 'NONE', #67419 ) ;
#54249=CARTESIAN_POINT ( 'NONE',  ( 3.007842271862381622, -6.459968553980839800, 34.89616026154728701 ) ) ;
#54250=VERTEX_POINT ( 'NONE', #18791 ) ;
#54251=B_SPLINE_CURVE_WITH_KNOTS ( 'NONE', 3,
 ( #25313, #65401, #39284, #86133, #31166, #52773, #59981, #72155, #51412, #80263 ),
 .UNSPECIFIED., .F., .F.,
 ( 4, 2, 2, 2, 4 ),
 ( 0.000000000000000000, 0.0001954311564186881213, 0.0003908623128373762425, 0.0005862934692560643367, 0.0007817246256747524850 ),
 .UNSPECIFIED. ) ;
#54252=ORIENTED_EDGE ( 'NONE', *, *, #6213, .T. ) ;
#54253=CARTESIAN_POINT ( 'NONE',  ( 15.23076923076923173, -4.098570777380720287, 33.41473453929634729 ) ) ;
#54254=CARTESIAN_POINT ( 'NONE',  ( 5.076923076922953193, -5.094484230521993062, 34.41647553114689373 ) ) ;
#54255=CARTESIAN_POINT ( 'NONE',  ( -0.2114841499001470504, -6.567000820036036579, 34.66262288849542728 ) ) ;
#54257=DIRECTION ( 'NONE',  ( -0.000000000000000000, -0.1736481776669307198, -0.9848077530122080203 ) ) ;
#54258=EDGE_CURVE ( 'NONE', #32578, #28537, #56285, .T. ) ;
#54259=ORIENTED_EDGE ( 'NONE', *, *, #42062, .T. ) ;
#54261=VECTOR ( 'NONE', #86967, 1000.000000000000000 ) ;
#54262=ORIENTED_EDGE ( 'NONE', *, *, #56121, .T. ) ;
#54264=DIRECTION ( 'NONE',  ( -0.000000000000000000, -0.8660254037844399289, -0.4999999999999980016 ) ) ;
#54265=CYLINDRICAL_SURFACE ( 'NONE', #31606, 0.2500000000000008882 ) ;
#54267=CARTESIAN_POINT ( 'NONE',  ( 15.93097989078305687, -2.251424796025574881, 29.88072029997477230 ) ) ;
#54268=CARTESIAN_POINT ( 'NONE',  ( 2.057669070399343880, -11.37209801155882971, 32.91403422569032955 ) ) ;
#54269=CARTESIAN_POINT ( 'NONE',  ( -15.00775638667583678, -9.172514111537584114, 34.72667873470787470 ) ) ;
#54270=CARTESIAN_POINT ( 'NONE',  ( 12.23861150263161157, -2.889293201056495786, 32.26117774369186009 ) ) ;
#54271=VECTOR ( 'NONE', #61314, 1000.000000000000227 ) ;
#54273=ORIENTED_EDGE ( 'NONE', *, *, #85686, .T. ) ;
#54274=B_SPLINE_CURVE_WITH_KNOTS ( 'NONE', 3,
 ( #68905, #67143, #60374, #46862, #87886, #15, #5885, #27484, #33359, #40128 ),
 .UNSPECIFIED., .F., .F.,
 ( 4, 2, 2, 2, 4 ),
 ( 0.0007817359430256307648, 0.0009771253907249971907, 0.001172514838424363508, 0.001367904286123729826, 0.001563293733823096143 ),
 .UNSPECIFIED. ) ;
#54275=ORIENTED_EDGE ( 'NONE', *, *, #47102, .T. ) ;
#54276=DIRECTION ( 'NONE',  ( -0.000000000000000000, 0.6427876096865404731, -0.7660444431189771253 ) ) ;
#54277=ORIENTED_EDGE ( 'NONE', *, *, #43278, .F. ) ;
#54278=CARTESIAN_POINT ( 'NONE',  ( -9.915792636031639518, -5.113361153441934093, 34.14387501736622710 ) ) ;
#54279=CARTESIAN_POINT ( 'NONE',  ( 6.700250230597919909, -7.369208160676172348, 34.74850200257122879 ) ) ;
#54281=ORIENTED_EDGE ( 'NONE', *, *, #23734, .F. ) ;
#54282=ADVANCED_FACE ( 'NONE', ( #59769 ), #11591, .F. ) ;
#54283=CARTESIAN_POINT ( 'NONE',  ( -1.134560964701931240, -11.47946981652013498, 33.17500667209846910 ) ) ;
#54284=ORIENTED_EDGE ( 'NONE', *, *, #44096, .F. ) ;
#54285=CARTESIAN_POINT ( 'NONE',  ( 2.084207363968360927, -6.760086850603068243, 34.69517049084099369 ) ) ;
#54287=FACE_BOUND ( 'NONE', #1904, .T. ) ;
#54288=DIRECTION ( 'NONE',  ( -0.000000000000000000, 0.6427876096865404731, -0.7660444431189770143 ) ) ;
#54290=CARTESIAN_POINT ( 'NONE',  ( 8.703960323269994248, -5.219633306516282545, 34.19971097300152962 ) ) ;
#54291=ORIENTED_EDGE ( 'NONE', *, *, #80951, .T. ) ;
#54292=CARTESIAN_POINT ( 'NONE',  ( -5.749999999999999112, -7.500000000000001776, 35.04278698407183867 ) ) ;
#54293=EDGE_CURVE ( 'NONE', #70654, #61347, #42264, .T. ) ;
#54294=CARTESIAN_POINT ( 'NONE',  ( -14.24162395668986747, -2.538708090699994813, 30.37095296980875503 ) ) ;
#54296=CARTESIAN_POINT ( 'NONE',  ( -3.296039231325549768, -9.528491918058357157, 34.59228464037090589 ) ) ;
#54297=ORIENTED_EDGE ( 'NONE', *, *, #21189, .F. ) ;
#54298=ADVANCED_FACE ( 'NONE', ( #56999 ), #48462, .F. ) ;
#54299=FACE_OUTER_BOUND ( 'NONE', #2761, .T. ) ;
#54301=CARTESIAN_POINT ( 'NONE',  ( 1.254467414883690290, -4.299443229763728169, 33.91186481527756058 ) ) ;
#54302=CARTESIAN_POINT ( 'NONE',  ( 4.376625822824220080, -11.60474049983371003, 33.02348890104160262 ) ) ;
#54303=DIRECTION ( 'NONE',  ( -0.000000000000000000, 1.000000000000000000, -0.000000000000000000 ) ) ;
#54304=CARTESIAN_POINT ( 'NONE',  ( 10.54930120442873154, -11.69971097300155272, 32.46337939537587403 ) ) ;
#54305=FACE_BOUND ( 'NONE', #28472, .T. ) ;
#54306=CARTESIAN_POINT ( 'NONE',  ( 13.13463864056679853, -12.01397095200674059, 32.43157075238190146 ) ) ;
#54307=CARTESIAN_POINT ( 'NONE',  ( 8.769230769230768274, -3.886160181151819604, 36.00935417666054406 ) ) ;
#54309=FACE_OUTER_BOUND ( 'NONE', #3321, .T. ) ;
#54310=CYLINDRICAL_SURFACE ( 'NONE', #58744, 0.2499999999999995559 ) ;
#54311=CARTESIAN_POINT ( 'NONE',  ( -0.7115384615384606759, -2.249999999999998668, 29.75000000000000355 ) ) ;
#54312=EDGE_CURVE ( 'NONE', #38219, #37130, #46555, .T. ) ;
#54313=DIRECTION ( 'NONE',  ( -0.000000000000000000, 0.9848077530122086864, -0.1736481776669273891 ) ) ;
#54315=EDGE_LOOP ( 'NONE', ( #49747, #28344, #6440, #22718 ) ) ;
#54316=CARTESIAN_POINT ( 'NONE',  ( -6.988347369037697376, -9.442884908240170461, 34.35708131394840592 ) ) ;
#54317=VERTEX_POINT ( 'NONE', #76845 ) ;
#54318=CARTESIAN_POINT ( 'NONE',  ( 0.4615384615384611200, -6.386643153685126251, 34.62446782046654192 ) ) ;
#54319=ORIENTED_EDGE ( 'NONE', *, *, #449, .F. ) ;
#54320=B_SPLINE_CURVE_WITH_KNOTS ( 'NONE', 3,
 ( #13077, #68028, #6330, #33789, #11298, #61246, #73455, #88758, #59484, #86990 ),
 .UNSPECIFIED., .F., .F.,
 ( 4, 2, 2, 2, 4 ),
 ( 0.0007817246256747484735, 0.0009771112852218915863, 0.001172497944769034916, 0.001367884604316178029, 0.001563271263863321141 ),
 .UNSPECIFIED. ) ;
#54321=DIRECTION ( 'NONE',  ( -0.000000000000000000, -0.5000000000000009992, -0.8660254037844380415 ) ) ;
#54322=FACE_OUTER_BOUND ( 'NONE', #18527, .T. ) ;
#54323=CARTESIAN_POINT ( 'NONE',  ( -2.557715544985270206, -11.86270091957321249, 32.19358267280087915 ) ) ;
#54324=ORIENTED_EDGE ( 'NONE', *, *, #66755, .T. ) ;
#54325=CARTESIAN_POINT ( 'NONE',  ( 3.480823542407545101, -6.567000820036038355, 34.66262288849541306 ) ) ;
#54328=CARTESIAN_POINT ( 'NONE',  ( 2.241608896736427159, -11.69971097300155272, 32.46337939537587403 ) ) ;
#54329=CARTESIAN_POINT ( 'NONE',  ( -6.988346923633240948, -12.70778746994557551, 30.41441678777548319 ) ) ;
#54331=CARTESIAN_POINT ( 'NONE',  ( 4.153846153846032507, -11.94971097300221174, 32.03036669348237098 ) ) ;
#54332=CARTESIAN_POINT ( 'NONE',  ( -1.253824943648433665, -6.369690395747424461, 34.87708834333098196 ) ) ;
#54333=DIRECTION ( 'NONE',  ( 0.000000000000000000, 0.7660444431189807890, 0.6427876096865361433 ) ) ;
#54335=VECTOR ( 'NONE', #55428, 1000.000000000000114 ) ;
#54336=CARTESIAN_POINT ( 'NONE',  ( 3.007941133134353073, -7.369209533119137845, 34.99857337881830688 ) ) ;
#54337=ORIENTED_EDGE ( 'NONE', *, *, #21446, .F. ) ;
#54338=CARTESIAN_POINT ( 'NONE',  ( 17.07692307692307665, -12.62096338111211580, 30.90682066428153263 ) ) ;
#54339=AXIS2_PLACEMENT_3D ( 'NONE', #61254, #74799, #5002 ) ;
#54341=EDGE_CURVE ( 'NONE', #63622, #55385, #49799, .T. ) ;
#54342=LINE ( 'NONE', #26445, #38991 ) ;
#54344=EDGE_LOOP ( 'NONE', ( #42482, #35132, #37919, #80994 ) ) ;
#54345=DIRECTION ( 'NONE',  ( -0.000000000000000000, 0.6427876096865404731, -0.7660444431189771253 ) ) ;
#54346=CARTESIAN_POINT ( 'NONE',  ( 3.100622021331009392, -3.817052484675422797, 33.13202310037935661 ) ) ;
#54347=CARTESIAN_POINT ( 'NONE',  ( 3.903869409797563250, -9.234221910056348293, 34.70572697212741531 ) ) ;
#54348=ORIENTED_EDGE ( 'NONE', *, *, #8895, .T. ) ;
#54349=DIRECTION ( 'NONE',  ( -0.000000000000000000, -0.3420201433256694901, -0.9396926207859082059 ) ) ;
#54350=VECTOR ( 'NONE', #40529, 1000.000000000000227 ) ;
#54351=CARTESIAN_POINT ( 'NONE',  ( 2.177000841024750333, -12.38065189839062263, 30.83690757178629482 ) ) ;
#54352=CARTESIAN_POINT ( 'NONE',  ( 7.173022332454966232, -12.07971442181322352, 32.31769673815850297 ) ) ;
#54354=VERTEX_POINT ( 'NONE', #69191 ) ;
#54355=CARTESIAN_POINT ( 'NONE',  ( 2.177544337960612975, -4.299443229763728169, 33.91186481527756058 ) ) ;
#54356=CARTESIAN_POINT ( 'NONE',  ( -18.13014720943822766, -12.27039167877662251, 31.24851455888617480 ) ) ;
#54357=ADVANCED_FACE ( 'NONE', ( #21891 ), #15142, .F. ) ;
#54358=CARTESIAN_POINT ( 'NONE',  ( 1.161130460051053470, -3.019605429927184836, 32.48692288466676814 ) ) ;
#54359=VERTEX_POINT ( 'NONE', #34955 ) ;
#54360=B_SPLINE_CURVE_WITH_KNOTS ( 'NONE', 3,
 ( #87735, #13819, #40424, #88184, #67443, #41302, #14266, #54801, #47157, #53471 ),
 .UNSPECIFIED., .F., .F.,
 ( 4, 2, 2, 2, 4 ),
 ( 0.000000000000000000, 0.0001954339857564070678, 0.0003908679715128141356, 0.0005863019572692211492, 0.0007817359430256282712 ),
 .UNSPECIFIED. ) ;
#54361=VERTEX_POINT ( 'NONE', #68747 ) ;
#54362=VERTEX_POINT ( 'NONE', #1172 ) ;
#54363=ORIENTED_EDGE ( 'NONE', *, *, #84122, .F. ) ;
#54364=AXIS2_PLACEMENT_3D ( 'NONE', #55987, #70846, #70400 ) ;
#54365=CARTESIAN_POINT ( 'NONE',  ( -5.999999999999998224, -13.20930481340135110, 34.54067556320372745 ) ) ;
#54366=CARTESIAN_POINT ( 'NONE',  ( -2.242436736416282272, -6.026961402152789304, 34.52809138561124769 ) ) ;
#54367=CARTESIAN_POINT ( 'NONE',  ( -13.38461538461538325, -12.10708131394839349, 31.69288490824020244 ) ) ;
#54368=DIRECTION ( 'NONE',  ( -0.000000000000000000, 0.8660254037844399289, -0.4999999999999980016 ) ) ;
#54369=ADVANCED_FACE ( 'NONE', ( #29544 ), #77274, .F. ) ;
#54370=DIRECTION ( 'NONE',  ( -0.000000000000000000, 0.9396926207859093161, -0.3420201433256663259 ) ) ;
#54371=ORIENTED_EDGE ( 'NONE', *, *, #10333, .F. ) ;
#54372=EDGE_CURVE ( 'NONE', #35493, #75936, #86602, .T. ) ;
#54373=ADVANCED_FACE ( 'NONE', ( #43050 ), #15584, .F. ) ;
#54374=EDGE_LOOP ( 'NONE', ( #271, #70543, #716, #15520 ) ) ;
#54376=ORIENTED_EDGE ( 'NONE', *, *, #44311, .T. ) ;
#54377=CARTESIAN_POINT ( 'NONE',  ( -6.923076923076922462, -1.466349020453238561, 30.81389545987213907 ) ) ;
#54378=ORIENTED_EDGE ( 'NONE', *, *, #52960, .T. ) ;
#54379=CARTESIAN_POINT ( 'NONE',  ( -1.450697763975519861, -2.833524468853757305, 32.15551576947924417 ) ) ;
#54380=EDGE_CURVE ( 'NONE', #3164, #70275, #35856, .T. ) ;
#54381=CARTESIAN_POINT ( 'NONE',  ( 15.23076923076911093, -5.219633306517616589, 34.19971097300220464 ) ) ;
#54382=B_SPLINE_CURVE_WITH_KNOTS ( 'NONE', 3,
 ( #33613, #12889, #11573, #59750, #31845, #86807, #45338, #19649, #47110, #46240 ),
 .UNSPECIFIED., .F., .F.,
 ( 4, 2, 2, 2, 4 ),
 ( 0.0007817359430256369448, 0.0009771253907250049969, 0.001172514838424373049, 0.001367904286123741101, 0.001563293733823109153 ),
 .UNSPECIFIED. ) ;
#54383=CARTESIAN_POINT ( 'NONE',  ( 5.776515075435670887, -4.225889041578354544, 33.85425143139329407 ) ) ;
#54384=DIRECTION ( 'NONE',  ( -0.000000000000000000, 0.5000000000000011102, -0.8660254037844380415 ) ) ;
#54386=EDGE_LOOP ( 'NONE', ( #21058, #88732, #2181, #25592 ) ) ;
#54387=ORIENTED_EDGE ( 'NONE', *, *, #78285, .F. ) ;
#54388=CARTESIAN_POINT ( 'NONE',  ( 14.30769230769218581, -11.06231777344772027, 33.60647404775119895 ) ) ;
#54391=CARTESIAN_POINT ( 'NONE',  ( -2.057637996053990559, -8.303483539816728154, 34.68545999027711702 ) ) ;
#54392=CARTESIAN_POINT ( 'NONE',  ( -17.30040800148741198, -3.562934362175799841, 33.22335522853832401 ) ) ;
#54393=VERTEX_POINT ( 'NONE', #69631 ) ;
#54394=CARTESIAN_POINT ( 'NONE',  ( 16.15384615384603251, -8.613356846316285953, 34.62446782046622218 ) ) ;
#54395=CARTESIAN_POINT ( 'NONE',  ( -17.93474442872397390, -2.625532179533469623, 30.86335684631491105 ) ) ;
#54396=DIRECTION ( 'NONE',  ( -0.000000000000000000, -0.7660444431189791237, -0.6427876096865379196 ) ) ;
#54397=VECTOR ( 'NONE', #14429, 1000.000000000000227 ) ;
#54398=FACE_BOUND ( 'NONE', #72022, .T. ) ;
#54399=CYLINDRICAL_SURFACE ( 'NONE', #54239, 0.2499999999999979738 ) ;
#54400=CARTESIAN_POINT ( 'NONE',  ( -1.134561072977070317, -11.79725096376909654, 32.30694842903960762 ) ) ;
#54401=EDGE_CURVE ( 'NONE', #78771, #17034, #14334, .T. ) ;
#54402=CARTESIAN_POINT ( 'NONE',  ( -12.46153846153846168, -1.509761064869970415, 31.06009739812519044 ) ) ;
#54403=CYLINDRICAL_SURFACE ( 'NONE', #5827, 0.2500000000000008882 ) ;
#54405=CARTESIAN_POINT ( 'NONE',  ( 0.2386122440223155117, -12.15238873228291538, 31.58232369045354915 ) ) ;
#54406=CARTESIAN_POINT ( 'NONE',  ( 12.59206389977210350, -3.068774925481848825, 32.56582465632704526 ) ) ;
#54407=ORIENTED_EDGE ( 'NONE', *, *, #19183, .F. ) ;
#54408=CARTESIAN_POINT ( 'NONE',  ( -18.06608341095587278, -10.51840700105979387, 33.73612834413961536 ) ) ;
#54409=CARTESIAN_POINT ( 'NONE',  ( 0.4615384615383382183, -11.06231777344772027, 33.60647404775119895 ) ) ;
#54410=ORIENTED_EDGE ( 'NONE', *, *, #69579, .F. ) ;
#54411=ADVANCED_FACE ( 'NONE', ( #57887 ), #36735, .F. ) ;
#54414=ORIENTED_EDGE ( 'NONE', *, *, #70782, .F. ) ;
#54415=CARTESIAN_POINT ( 'NONE',  ( -16.02332045208259359, -11.46989282347013095, 32.79007818306219946 ) ) ;
#54416=CARTESIAN_POINT ( 'NONE',  ( -4.377331078410483300, -9.417330523894424488, 34.63758898049880486 ) ) ;
#54417=B_SPLINE_CURVE_WITH_KNOTS ( 'NONE', 3,
 ( #79982, #57480, #16943, #18281, #45749, #73228, #44394, #39010, #66469, #78199 ),
 .UNSPECIFIED., .F., .F.,
 ( 4, 2, 2, 2, 4 ),
 ( 0.000000000000000000, 0.0001954339881912772715, 0.0003908679763825545429, 0.0005863019645738318415, 0.0007817359527651090859 ),
 .UNSPECIFIED. ) ;
#54418=FACE_BOUND ( 'NONE', #3019, .T. ) ;
#54419=CARTESIAN_POINT ( 'NONE',  ( -17.01085472592063752, -4.098570777380720287, 33.41473453929635440 ) ) ;
#54420=FACE_OUTER_BOUND ( 'NONE', #82200, .T. ) ;
#54421=CARTESIAN_POINT ( 'NONE',  ( -13.63459212866397685, -2.318417181685855422, 30.59732222474233865 ) ) ;
#54422=DIRECTION ( 'NONE',  ( 0.000000000000000000, 0.9396926207859126468, 0.3420201433256571111 ) ) ;
#54424=CARTESIAN_POINT ( 'NONE',  ( 0.2115617305961066674, -5.728515186090277211, 34.42611988154120439 ) ) ;
#54425=ADVANCED_FACE ( 'NONE', ( #65976 ), #86730, .F. ) ;
#54427=ORIENTED_EDGE ( 'NONE', *, *, #1808, .T. ) ;
#54428=ORIENTED_EDGE ( 'NONE', *, *, #72781, .F. ) ;
#54430=CARTESIAN_POINT ( 'NONE',  ( -9.758390071667825794, -2.486705287966279432, 31.30864560766542937 ) ) ;
#54431=CARTESIAN_POINT ( 'NONE',  ( 16.28437185560972011, -6.852161475712351013, 34.70806712695775786 ) ) ;
#54432=DIRECTION ( 'NONE',  ( -0.000000000000000000, 0.9396926207859092051, -0.3420201433256662704 ) ) ;
#54433=CARTESIAN_POINT ( 'NONE',  ( 10.74591005361825680, -3.068774925481848825, 32.56582465632704526 ) ) ;
#54434=FACE_OUTER_BOUND ( 'NONE', #7454, .T. ) ;
#54437=CARTESIAN_POINT ( 'NONE',  ( -6.000000000000121680, -8.656820664282941280, 34.87096338111179961 ) ) ;
#54438=VECTOR ( 'NONE', #69447, 999.9999999999998863 ) ;
#54439=EDGE_CURVE ( 'NONE', #68982, #69859, #33641, .T. ) ;
#54440=CARTESIAN_POINT ( 'NONE',  ( 17.93472999944368240, -4.320704448112772766, 33.92786785259540494 ) ) ;
#54441=CARTESIAN_POINT ( 'NONE',  ( -1.449938300107559641, -7.749976743299137993, 34.99404534957040624 ) ) ;
#54442=CARTESIAN_POINT ( 'NONE',  ( 9.915319043920542086, -2.758310577978208666, 31.33698337089302299 ) ) ;
#54443=AXIS2_PLACEMENT_3D ( 'NONE', #41696, #47557, #75047 ) ;
#54444=DIRECTION ( 'NONE',  ( 0.000000000000000000, 1.000000000000000000, 0.000000000000000000 ) ) ;
#54445=CARTESIAN_POINT ( 'NONE',  ( -13.38461538461538325, -1.117168528481311540, 33.14645433367849847 ) ) ;
#54446=CARTESIAN_POINT ( 'NONE',  ( 2.557692307693728129, -7.500000000000154543, 35.00000000000007105 ) ) ;
#54447=CARTESIAN_POINT ( 'NONE',  ( -12.52678945169970604, -2.506253911140460922, 30.00000000000013856 ) ) ;
#54448=ORIENTED_EDGE ( 'NONE', *, *, #64523, .F. ) ;
#54449=CARTESIAN_POINT ( 'NONE',  ( 1.384615384615265343, -2.625532179533778709, 30.86335684631627174 ) ) ;
#54450=CARTESIAN_POINT ( 'NONE',  ( -17.20761368003338276, -6.369640206132551441, 34.87707690430378449 ) ) ;
#54453=CARTESIAN_POINT ( 'NONE',  ( -17.77722045873158763, -10.81320215134717344, 33.49497208177562868 ) ) ;
#54454=CARTESIAN_POINT ( 'NONE',  ( -11.40793610022789828, -5.070358843744210198, 34.40418822224088302 ) ) ;
#54456=EDGE_LOOP ( 'NONE', ( #51125, #25764 ) ) ;
#54459=CARTESIAN_POINT ( 'NONE',  ( 17.86985279056177944, -3.817052484675422797, 33.13202310037935661 ) ) ;
#54460=B_SPLINE_CURVE_WITH_KNOTS ( 'NONE', 3,
 ( #11003, #18204, #46117, #25849, #60065, #79007, #10103, #85775, #45666, #24056 ),
 .UNSPECIFIED., .F., .F.,
 ( 4, 2, 2, 2, 4 ),
 ( 0.0007817246256747465219, 0.0009771112852218898515, 0.001172497944769033181, 0.001367884604316176294, 0.001563271263863319624 ),
 .UNSPECIFIED. ) ;
#54461=ORIENTED_EDGE ( 'NONE', *, *, #4207, .F. ) ;
#54462=CARTESIAN_POINT ( 'NONE',  ( -16.15384615384615330, -9.780366693483667717, 34.19971097300155094 ) ) ;
#54463=CARTESIAN_POINT ( 'NONE',  ( -6.989159302437058408, -11.35647404775217595, 33.31231777344666511 ) ) ;
#54465=CARTESIAN_POINT ( 'NONE',  ( 7.780883400193072674, -4.481592998940162609, 33.73612834413957984 ) ) ;
#54466=B_SPLINE_CURVE_WITH_KNOTS ( 'NONE', 3,
 ( #49847, #16071, #36783, #62907, #9322, #49419, #2540, #70124, #21946, #71013 ),
 .UNSPECIFIED., .F., .F.,
 ( 4, 2, 2, 2, 4 ),
 ( 0.0007817359430256390048, 0.0009771253907250075990, 0.001172514838424376085, 0.001367904286123744571, 0.001563293733823113056 ),
 .UNSPECIFIED. ) ;
#54467=CARTESIAN_POINT ( 'NONE',  ( -15.00780609650255570, -7.369474539155828730, 34.99858011523957657 ) ) ;
#54469=DIRECTION ( 'NONE',  ( 0.000000000000000000, 0.3420201433256641055, -0.9396926207859100932 ) ) ;
#54470=EDGE_CURVE ( 'NONE', #78525, #78212, #25013, .T. ) ;
#54471=ORIENTED_EDGE ( 'NONE', *, *, #18602, .F. ) ;
#54473=CARTESIAN_POINT ( 'NONE',  ( -6.923076923076922462, -12.78798330534102945, 29.74999999999997868 ) ) ;
#54474=AXIS2_PLACEMENT_3D ( 'NONE', #72918, #64370, #71576 ) ;
#54475=ORIENTED_EDGE ( 'NONE', *, *, #28904, .T. ) ;
#54476=CARTESIAN_POINT ( 'NONE',  ( -18.00000000000012079, -5.094484230521992174, 34.41647553114689373 ) ) ;
#54477=DIRECTION ( 'NONE',  ( 0.000000000000000000, 0.3420201433256610524, 0.9396926207859113145 ) ) ;
#54478=CARTESIAN_POINT ( 'NONE',  ( 9.561617089197383734, -9.084618155246140248, 34.75535874321725771 ) ) ;
#54479=CARTESIAN_POINT ( 'NONE',  ( -2.307692307692305711, -5.557115091759785130, 34.35708131394839171 ) ) ;
#54480=CARTESIAN_POINT ( 'NONE',  ( -0.3310130233048163562, -5.915461855592777596, 34.75538340440931506 ) ) ;
#54481=DIRECTION ( 'NONE',  ( -0.000000000000000000, -0.8660254037844397068, -0.4999999999999978906 ) ) ;
#54482=CARTESIAN_POINT ( 'NONE',  ( 10.39189967166066708, -12.24155766932282496, 31.33739205006857986 ) ) ;
#54483=EDGE_CURVE ( 'NONE', #3281, #19723, #59224, .T. ) ;
#54486=CARTESIAN_POINT ( 'NONE',  ( 6.923076923076924238, -12.62096338111211580, 30.90682066428153263 ) ) ;
#54487=ORIENTED_EDGE ( 'NONE', *, *, #86603, .T. ) ;
#54488=CIRCLE ( 'NONE', #47289, 3.249999999999999556 ) ;
#54489=CARTESIAN_POINT ( 'NONE',  ( -13.63461538461538325, -7.500000000000001776, 35.00000000000000000 ) ) ;
#54490=CARTESIAN_POINT ( 'NONE',  ( 12.46153846153846168, -3.050289026998446396, 32.03036669348365706 ) ) ;
#54491=B_SPLINE_CURVE_WITH_KNOTS ( 'NONE', 3,
 ( #32770, #25573, #53027, #62011, #317, #62878, #56586, #75525, #28221, #1191 ),
 .UNSPECIFIED., .F., .F.,
 ( 4, 2, 2, 2, 4 ),
 ( 0.000000000000000000, 0.0001954311564186863052, 0.0003908623128373726104, 0.0005862934692560589156, 0.0007817246256747452209 ),
 .UNSPECIFIED. ) ;
#54492=ORIENTED_EDGE ( 'NONE', *, *, #8617, .T. ) ;
#54493=B_SPLINE_CURVE_WITH_KNOTS ( 'NONE', 3,
 ( #66326, #16801, #58672, #44705, #37970, #3728, #79847, #51906, #18592, #66771 ),
 .UNSPECIFIED., .F., .F.,
 ( 4, 2, 2, 2, 4 ),
 ( 0.000000000000000000, 0.0001954311564186858715, 0.0003908623128373717431, 0.0005862934692560576146, 0.0007817246256747434861 ),
 .UNSPECIFIED. ) ;
#54495=AXIS2_PLACEMENT_3D ( 'NONE', #77418, #55816, #42761 ) ;
#54496=ORIENTED_EDGE ( 'NONE', *, *, #26707, .F. ) ;
#54497=CARTESIAN_POINT ( 'NONE',  ( -10.61538461538473399, -3.300289026999228881, 32.46337939537708905 ) ) ;
#54498=ORIENTED_EDGE ( 'NONE', *, *, #35016, .T. ) ;
#54500=CARTESIAN_POINT ( 'NONE',  ( 1.384615384615386802, -2.833524468853757305, 32.15551576947925838 ) ) ;
#54501=B_SPLINE_CURVE_WITH_KNOTS ( 'NONE', 3,
 ( #80395, #73185, #11483, #18692, #68966, #34292, #32634, #60104, #61752, #21219 ),
 .UNSPECIFIED., .F., .F.,
 ( 4, 2, 2, 2, 4 ),
 ( 0.0007817246256747440282, 0.0009771112852218863821, 0.001172497944769028844, 0.001367884604316171307, 0.001563271263863313769 ),
 .UNSPECIFIED. ) ;
#54502=EDGE_LOOP ( 'NONE', ( #10640, #17822, #27396, #81187 ) ) ;
#54503=VECTOR ( 'NONE', #60616, 1000.000000000000000 ) ;
#54504=CARTESIAN_POINT ( 'NONE',  ( -4.376773112753002515, -4.026226216239095379, 33.68668979543632958 ) ) ;
#54506=FACE_BOUND ( 'NONE', #1318, .T. ) ;
#54507=CARTESIAN_POINT ( 'NONE',  ( -14.55771553191376633, -9.356822207818506598, 34.66110646841856635 ) ) ;
#54508=DIRECTION ( 'NONE',  ( 0.000000000000000000, 0.4999999999999960032, -0.8660254037844410391 ) ) ;
#54509=CARTESIAN_POINT ( 'NONE',  ( 13.38461538461538680, -4.661471528628507777, 34.16647553114623292 ) ) ;
#54510=CARTESIAN_POINT ( 'NONE',  ( -3.296852641725110722, -4.098570777380720287, 33.41473453929634729 ) ) ;
#54511=DIRECTION ( 'NONE',  ( -0.000000000000000000, 0.6427876096865404731, -0.7660444431189770143 ) ) ;
#54512=CARTESIAN_POINT ( 'NONE',  ( 16.02369894440793630, -4.460286881179643004, 33.72017969459903242 ) ) ;
#54513=CARTESIAN_POINT ( 'NONE',  ( -6.923076923077044142, -6.879047030192662504, 34.71129190930017927 ) ) ;
#54514=VERTEX_POINT ( 'NONE', #10601 ) ;
#54516=CARTESIAN_POINT ( 'NONE',  ( -16.85414353565466428, -10.11255958852955672, 34.01340905677048454 ) ) ;
#54517=CARTESIAN_POINT ( 'NONE',  ( -18.22348492456433178, -10.23692288466677525, 34.23039457007281072 ) ) ;
#54518=CARTESIAN_POINT ( 'NONE',  ( -4.376725670583738292, -7.630690623152302621, 34.99857592706774057 ) ) ;
#54519=CARTESIAN_POINT ( 'NONE',  ( 3.296024802045254720, -10.90142922261932057, 33.41473453929631887 ) ) ;
#54520=CARTESIAN_POINT ( 'NONE',  ( 16.82694634598072625, -8.303909089506435137, 34.68538101551103381 ) ) ;
#54521=CARTESIAN_POINT ( 'NONE',  ( 13.45068373561782415, -11.16473453929635440, 33.15142922261926373 ) ) ;
#54522=VERTEX_POINT ( 'NONE', #16466 ) ;
#54523=CARTESIAN_POINT ( 'NONE',  ( -11.53846153846165912, -12.27809138561165270, 31.22303859784587132 ) ) ;
#54525=CARTESIAN_POINT ( 'NONE',  ( 16.85343815235874487, -4.225889041578354544, 33.85425143139329407 ) ) ;
#54526=CARTESIAN_POINT ( 'NONE',  ( -16.15384615384615330, -3.937682226553329556, 33.60647404775216529 ) ) ;
#54527=ORIENTED_EDGE ( 'NONE', *, *, #47092, .F. ) ;
#54528=AXIS2_PLACEMENT_3D ( 'NONE', #66847, #87586, #19985 ) ;
#54529=B_SPLINE_CURVE_WITH_KNOTS ( 'NONE', 3,
 ( #47439, #86348, #40705, #45325, #58840, #19970, #74934, #53758, #47887, #68604 ),
 .UNSPECIFIED., .F., .F.,
 ( 4, 2, 2, 2, 4 ),
 ( 0.000000000000000000, 0.0001954339857564070678, 0.0003908679715128141356, 0.0005863019572692211492, 0.0007817359430256282712 ),
 .UNSPECIFIED. ) ;
#54530=ORIENTED_EDGE ( 'NONE', *, *, #4182, .T. ) ;
#54531=VERTEX_POINT ( 'NONE', #43932 ) ;
#54532=CARTESIAN_POINT ( 'NONE',  ( -6.923076923076922462, -13.20930481340135110, 34.54067556320372745 ) ) ;
#54534=CARTESIAN_POINT ( 'NONE',  ( -16.08859058257012720, -5.219633306516380244, 34.19971097300157936 ) ) ;
#54535=CARTESIAN_POINT ( 'NONE',  ( -6.066082379360133281, -9.058645607665454236, 34.76329471203372634 ) ) ;
#54536=CARTESIAN_POINT ( 'NONE',  ( 5.076923076923075762, -6.386643153685126251, 34.62446782046654192 ) ) ;
#54537=CARTESIAN_POINT ( 'NONE',  ( 8.769230769230645706, -3.643525952248795718, 33.31231777344771672 ) ) ;
#54538=CARTESIAN_POINT ( 'NONE',  ( 14.53070365930516061, -4.187068189119697692, 33.49521262558774026 ) ) ;
#54539=ORIENTED_EDGE ( 'NONE', *, *, #72295, .F. ) ;
#54541=CARTESIAN_POINT ( 'NONE',  ( -13.25382357679059453, -4.118422570099831148, 33.43335022499816489 ) ) ;
#54543=CARTESIAN_POINT ( 'NONE',  ( -5.299850035829923200, -2.308479472611653094, 30.53278059502174457 ) ) ;
#54544=CARTESIAN_POINT ( 'NONE',  ( -3.164701897419155419, -2.486705287966280320, 31.30864560766543647 ) ) ;
#54545=CARTESIAN_POINT ( 'NONE',  ( -13.45069879557126136, -4.786620604624113540, 33.94971097300155805 ) ) ;
#54546=CARTESIAN_POINT ( 'NONE',  ( 11.78840694783958298, -10.18230066228895758, 34.26354781536631577 ) ) ;
#54547=DIRECTION ( 'NONE',  ( -0.000000000000000000, -0.5000000000000009992, -0.8660254037844380415 ) ) ;
#54549=CARTESIAN_POINT ( 'NONE',  ( 12.46153846153833911, -11.48612834414049644, 32.76840700105863391 ) ) ;
#54551=VERTEX_POINT ( 'NONE', #78602 ) ;
#54553=DIRECTION ( 'NONE',  ( -0.000000000000000000, -0.9396926207859093161, -0.3420201433256663259 ) ) ;
#54557=DIRECTION ( 'NONE',  ( -0.000000000000000000, 0.8660254037844399289, -0.4999999999999980016 ) ) ;
#54559=VERTEX_POINT ( 'NONE', #72733 ) ;
#54560=CARTESIAN_POINT ( 'NONE',  ( -12.68502340526241312, -11.89387501736622710, 32.13663884655806413 ) ) ;
#54561=CARTESIAN_POINT ( 'NONE',  ( -5.326946314216043810, -6.695914987888143877, 34.68535235679833306 ) ) ;
#54563=CARTESIAN_POINT ( 'NONE',  ( -10.61538461538473577, -2.379036618888197729, 30.90682066428292885 ) ) ;
#54564=CARTESIAN_POINT ( 'NONE',  ( -4.826923076923073985, -2.499999999999999112, 29.81604066197450109 ) ) ;
#54567=ORIENTED_EDGE ( 'NONE', *, *, #48556, .F. ) ;
#54568=CARTESIAN_POINT ( 'NONE',  ( 6.223011351612852238, -5.667800583137508674, 34.40243808032445827 ) ) ;
#54569=EDGE_CURVE ( 'NONE', #65380, #89050, #49733, .T. ) ;
#54570=DIRECTION ( 'NONE',  ( 0.000000000000000000, 0.9396926207859126468, -0.3420201433256571111 ) ) ;
#54571=CARTESIAN_POINT ( 'NONE',  ( -14.30769230769230660, -6.189225973068211317, 35.74407628777942847 ) ) ;
#54572=VERTEX_POINT ( 'NONE', #45710 ) ;
#54574=ORIENTED_EDGE ( 'NONE', *, *, #78457, .F. ) ;
#54575=CARTESIAN_POINT ( 'NONE',  ( -16.15384615384627409, -6.026961402154118908, 34.52809138561165270 ) ) ;
#54576=LINE ( 'NONE', #82073, #61312 ) ;
#54578=CARTESIAN_POINT ( 'NONE',  ( -11.53846153846153655, -12.34228464037088635, 31.77849191805839268 ) ) ;
#54579=FACE_OUTER_BOUND ( 'NONE', #29812, .T. ) ;
#54580=CARTESIAN_POINT ( 'NONE',  ( 1.318531973659505807, -4.098570777380720287, 33.41473453929634729 ) ) ;
#54581=CARTESIAN_POINT ( 'NONE',  ( -7.976844449264155479, -4.684245665217972032, 34.18127051446801090 ) ) ;
#54582=DIRECTION ( 'NONE',  ( 0.000000000000000000, 0.9848077530122072432, 0.1736481776669354937 ) ) ;
#54584=VERTEX_POINT ( 'NONE', #81289 ) ;
#54585=FACE_BOUND ( 'NONE', #37562, .T. ) ;
#54586=VERTEX_POINT ( 'NONE', #46167 ) ;
#54587=CARTESIAN_POINT ( 'NONE',  ( -8.992157728137618378, -12.38737895849757820, 31.66785238281580206 ) ) ;
#54589=EDGE_CURVE ( 'NONE', #1870, #7785, #11491, .T. ) ;
#54590=EDGE_CURVE ( 'NONE', #13908, #74567, #26147, .T. ) ;
#54591=CARTESIAN_POINT ( 'NONE',  ( 18.13079180782478161, -12.11778462344220841, 31.66786338562085135 ) ) ;
#54592=CARTESIAN_POINT ( 'NONE',  ( 3.007284306204899504, -11.60425143139329940, 33.02411095842164457 ) ) ;
#54593=CARTESIAN_POINT ( 'NONE',  ( -11.31568199719312773, -2.600157965045224451, 30.74683119005207743 ) ) ;
#54594=ORIENTED_EDGE ( 'NONE', *, *, #33487, .T. ) ;
#54595=VERTEX_POINT ( 'NONE', #18248 ) ;
#54596=ORIENTED_EDGE ( 'NONE', *, *, #70633, .T. ) ;
#54597=B_SPLINE_CURVE_WITH_KNOTS ( 'NONE', 3,
 ( #40711, #83020, #33938, #68173, #21753, #21305, #48778, #76246, #42039, #27181 ),
 .UNSPECIFIED., .F., .F.,
 ( 4, 2, 2, 2, 4 ),
 ( 0.0007817246256747503166, 0.0009771112852218946220, 0.001172497944769039036, 0.001367884604316183233, 0.001563271263863327647 ),
 .UNSPECIFIED. ) ;
#54598=ORIENTED_EDGE ( 'NONE', *, *, #10938, .F. ) ;
#54599=CARTESIAN_POINT ( 'NONE',  ( -4.826977558574935934, -5.057305518903949526, 34.11320923018887896 ) ) ;
#54600=CARTESIAN_POINT ( 'NONE',  ( 6.673076923076925127, -7.500000000000001776, 35.00000000000000000 ) ) ;
#54601=CARTESIAN_POINT ( 'NONE',  ( -7.911423846710166075, -3.643525952247789412, 33.31231777344662959 ) ) ;
#54602=CARTESIAN_POINT ( 'NONE',  ( 11.28843830116857383, -2.587272538249754117, 30.68239716806877837 ) ) ;
#54603=AXIS2_PLACEMENT_3D ( 'NONE', #86651, #24920, #52384 ) ;
#54606=CYLINDRICAL_SURFACE ( 'NONE', #53830, 0.2499999999999973355 ) ;
#54607=CARTESIAN_POINT ( 'NONE',  ( 11.28848480751918437, -9.943427161483782584, 34.11278801902876978 ) ) ;
#54608=ORIENTED_EDGE ( 'NONE', *, *, #26817, .T. ) ;
#54609=EDGE_LOOP ( 'NONE', ( #51449, #61180, #6184, #23842 ) ) ;
#54610=B_SPLINE_CURVE_WITH_KNOTS ( 'NONE', 3,
 ( #13305, #55171, #47524, #33132, #69136, #12860, #47080, #54279, #21393, #60598 ),
 .UNSPECIFIED., .F., .F.,
 ( 4, 2, 2, 2, 4 ),
 ( 0.0007817359527651090859, 0.0009771254036996478414, 0.001172514854634186489, 0.001367904305568725136, 0.001563293756503263783 ),
 .UNSPECIFIED. ) ;
#54612=ORIENTED_EDGE ( 'NONE', *, *, #16558, .T. ) ;
#54613=DIRECTION ( 'NONE',  ( -0.000000000000000000, -0.9396926207859092051, -0.3420201433256662704 ) ) ;
#54614=CARTESIAN_POINT ( 'NONE',  ( 1.384615384615386802, -5.557115091759785130, 34.35708131394839171 ) ) ;
#54615=CARTESIAN_POINT ( 'NONE',  ( -7.715363405186893786, -9.084667340241226796, 34.75534355489798344 ) ) ;
#54616=EDGE_CURVE ( 'NONE', #49089, #69788, #40200, .T. ) ;
#54617=CARTESIAN_POINT ( 'NONE',  ( -0.2114840416250090560, -2.318338780012835443, 30.59689888758630261 ) ) ;
#54618=DIRECTION ( 'NONE',  ( -0.000000000000000000, -0.6427876096865404731, -0.7660444431189770143 ) ) ;
#54619=FACE_BOUND ( 'NONE', #73595, .T. ) ;
#54621=FACE_OUTER_BOUND ( 'NONE', #55259, .T. ) ;
#54622=CARTESIAN_POINT ( 'NONE',  ( 16.94623161025552704, -6.413092428213692742, 34.63065189839063152 ) ) ;
#54623=CARTESIAN_POINT ( 'NONE',  ( 3.230769230769231726, -10.51840700105979565, 33.73612834413961536 ) ) ;
#54624=VERTEX_POINT ( 'NONE', #66432 ) ;
#54625=CARTESIAN_POINT ( 'NONE',  ( -4.946397375159514276, -6.852161475712352789, 34.70806712695775786 ) ) ;
#54626=EDGE_LOOP ( 'NONE', ( #38889, #12635 ) ) ;
#54627=FACE_BOUND ( 'NONE', #35655, .T. ) ;
#54628=CARTESIAN_POINT ( 'NONE',  ( -16.08865217206279752, -2.506253911140448043, 29.99999999999988631 ) ) ;
#54629=ORIENTED_EDGE ( 'NONE', *, *, #21772, .F. ) ;
#54630=CARTESIAN_POINT ( 'NONE',  ( -22.75000000000000000, -4.499999999999999112, 29.75000000000000355 ) ) ;
#54631=LINE ( 'NONE', #593, #54817 ) ;
#54632=CARTESIAN_POINT ( 'NONE',  ( -0.4615384615384611200, -2.292212530054420494, 30.41441678777542634 ) ) ;
#54633=ORIENTED_EDGE ( 'NONE', *, *, #8506, .F. ) ;
#54634=CARTESIAN_POINT ( 'NONE',  ( 6.857806477116148436, -10.21337939537584383, 33.94971097300158647 ) ) ;
#54635=CARTESIAN_POINT ( 'NONE',  ( 14.05766908347085220, -11.56360843649121861, 33.07473185843129926 ) ) ;
#54636=CARTESIAN_POINT ( 'NONE',  ( -16.15384615384615330, -12.37446782046654192, 30.86335684631486131 ) ) ;
#54637=CARTESIAN_POINT ( 'NONE',  ( -8.096177083446812972, -2.823816976329319051, 31.52131813110795733 ) ) ;
#54638=EDGE_LOOP ( 'NONE', ( #51733, #43092, #86125, #29308 ) ) ;
#54639=EDGE_CURVE ( 'NONE', #39942, #69003, #39078, .T. ) ;
#54640=LINE ( 'NONE', #82138, #61788 ) ;
#54641=CARTESIAN_POINT ( 'NONE',  ( -15.36146069743678844, -4.118384482072085184, 33.43331474514187107 ) ) ;
#54642=CARTESIAN_POINT ( 'NONE',  ( -3.230769230769351186, -12.27809138561165270, 31.22303859784587132 ) ) ;
#54643=ORIENTED_EDGE ( 'NONE', *, *, #32527, .F. ) ;
#54644=CARTESIAN_POINT ( 'NONE',  ( 2.557637717070353034, -10.18230066228895758, 34.26354781536631577 ) ) ;
#54645=CARTESIAN_POINT ( 'NONE',  ( -4.283993363284372080, -2.619462340734462380, 30.83744416345203021 ) ) ;
#54646=CARTESIAN_POINT ( 'NONE',  ( 5.777073782483852504, -9.086856451489516928, 34.49173150075333183 ) ) ;
#54647=DIRECTION ( 'NONE',  ( 0.000000000000000000, 0.000000000000000000, 1.000000000000000000 ) ) ;
#54648=LINE ( 'NONE', #41154, #67464 ) ;
#54649=CARTESIAN_POINT ( 'NONE',  ( 9.942362003946010773, -9.148310452688876993, 34.47095581063188519 ) ) ;
#54650=CARTESIAN_POINT ( 'NONE',  ( -7.976845312821404299, -10.54014554554150607, 33.71984207302941883 ) ) ;
#54651=FACE_OUTER_BOUND ( 'NONE', #88800, .T. ) ;
#54652=CARTESIAN_POINT ( 'NONE',  ( -6.792285115252139072, -2.729792928343270919, 31.24908615093345077 ) ) ;
#54653=AXIS2_PLACEMENT_3D ( 'NONE', #45007, #59868, #46357 ) ;
#54657=ORIENTED_EDGE ( 'NONE', *, *, #21772, .T. ) ;
#54659=EDGE_LOOP ( 'NONE', ( #20647, #70742 ) ) ;
#54660=CARTESIAN_POINT ( 'NONE',  ( 3.007843013253082898, -4.887634598454295265, 34.01352882383564946 ) ) ;
#54661=VERTEX_POINT ( 'NONE', #33540 ) ;
#54662=CARTESIAN_POINT ( 'NONE',  ( 14.05771557674995442, -8.303909089506435137, 34.68538101551103381 ) ) ;
#54664=CARTESIAN_POINT ( 'NONE',  ( 17.74997677577854205, -4.931416488878822335, 34.32920672191015399 ) ) ;
#54665=EDGE_CURVE ( 'NONE', #3680, #16511, #24052, .T. ) ;
#54666=DIRECTION ( 'NONE',  ( -0.000000000000000000, 0.1736481776669307198, -0.9848077530122080203 ) ) ;
#54667=CARTESIAN_POINT ( 'NONE',  ( 6.000000000000001776, -11.11383981884818262, 36.00935417666054406 ) ) ;
#54668=CARTESIAN_POINT ( 'NONE',  ( -7.173100147298381302, -9.356822207818506598, 34.66110646841856635 ) ) ;
#54669=DIRECTION ( 'NONE',  ( 0.000000000000000000, 0.6427876096865373645, -0.7660444431189797898 ) ) ;
#54672=CARTESIAN_POINT ( 'NONE',  ( 10.36540788444226102, -2.564618984488975517, 30.55390908950641915 ) ) ;
#54673=CARTESIAN_POINT ( 'NONE',  ( 17.77707378248385339, -11.76352882383564769, 32.36236540154569497 ) ) ;
#54674=AXIS2_PLACEMENT_3D ( 'NONE', #21167, #1783, #69367 ) ;
#54675=EDGE_CURVE ( 'NONE', #6751, #57920, #84221, .T. ) ;
#54676=CARTESIAN_POINT ( 'NONE',  ( 5.777073041093150785, -11.43668979543635089, 33.22377378376089752 ) ) ;
#54677=B_SPLINE_CURVE_WITH_KNOTS ( 'NONE', 3,
 ( #49806, #10161, #43058, #42623, #83621, #65085, #36742, #64196, #56130, #1636 ),
 .UNSPECIFIED., .F., .F.,
 ( 4, 2, 2, 2, 4 ),
 ( 0.000000000000000000, 0.0001954339857564084773, 0.0003908679715128169545, 0.0005863019572692254860, 0.0007817359430256339090 ),
 .UNSPECIFIED. ) ;
#54678=AXIS2_PLACEMENT_3D ( 'NONE', #33734, #45904, #61188 ) ;
#54679=AXIS2_PLACEMENT_3D ( 'NONE', #10752, #38220, #37774 ) ;
#54680=EDGE_CURVE ( 'NONE', #78895, #74896, #18652, .T. ) ;
#54681=ORIENTED_EDGE ( 'NONE', *, *, #78903, .T. ) ;
#54683=CARTESIAN_POINT ( 'NONE',  ( -18.00000000000000000, -2.486705287966279876, 31.30864560766543647 ) ) ;
#54684=CARTESIAN_POINT ( 'NONE',  ( 0.5276057948885367610, -11.91647553114624358, 32.58852847137148245 ) ) ;
#54685=LINE ( 'NONE', #6519, #19599 ) ;
#54686=CARTESIAN_POINT ( 'NONE',  ( 9.822833130541338775, -12.15418822224088657, 32.17964115625579069 ) ) ;
#54687=EDGE_CURVE ( 'NONE', #27674, #20836, #6068, .T. ) ;
#54688=VECTOR ( 'NONE', #81394, 1000.000000000000114 ) ;
#54689=CARTESIAN_POINT ( 'NONE',  ( 8.546304551714619890, -4.186968288167450147, 33.49512374952580274 ) ) ;
#54690=AXIS2_PLACEMENT_3D ( 'NONE', #6555, #68690, #20504 ) ;
#54691=CARTESIAN_POINT ( 'NONE',  ( -9.692307692307814193, -11.06231777344772027, 33.60647404775119895 ) ) ;
#54694=EDGE_CURVE ( 'NONE', #74098, #58055, #7959, .T. ) ;
#54695=VERTEX_POINT ( 'NONE', #41620 ) ;
#54696=CARTESIAN_POINT ( 'NONE',  ( 1.319344938654611665, -5.219633306516282545, 34.19971097300152962 ) ) ;
#54697=ORIENTED_EDGE ( 'NONE', *, *, #11480, .T. ) ;
#54698=B_SPLINE_CURVE_WITH_KNOTS ( 'NONE', 3,
 ( #60655, #59772, #66076, #19675, #12048, #25099, #74627, #6167, #32744, #12481 ),
 .UNSPECIFIED., .F., .F.,
 ( 4, 2, 2, 2, 4 ),
 ( 0.000000000000000000, 0.0001954311584214072923, 0.0003908623168428145846, 0.0005862934752642218498, 0.0007817246336856291692 ),
 .UNSPECIFIED. ) ;
#54699=CARTESIAN_POINT ( 'NONE',  ( 17.77707378248384629, -3.105860786376062332, 32.13614157043599562 ) ) ;
#54700=CARTESIAN_POINT ( 'NONE',  ( -18.06870381900337108, -12.74406763069169202, 29.99950897402481687 ) ) ;
#54701=EDGE_CURVE ( 'NONE', #59987, #24082, #1074, .T. ) ;
#54702=CARTESIAN_POINT ( 'NONE',  ( -6.793029487826470536, -7.723484941389743952, 34.99544897038808955 ) ) ;
#54703=ADVANCED_FACE ( 'NONE', ( #76733 ), #21787, .F. ) ;
#54704=CARTESIAN_POINT ( 'NONE',  ( 3.165499230212911908, -8.656820664281497102, 34.87096338111211935 ) ) ;
#54705=CARTESIAN_POINT ( 'NONE',  ( -13.45069776397551742, -2.486705287966279432, 31.30864560766542937 ) ) ;
#54706=ORIENTED_EDGE ( 'NONE', *, *, #82743, .F. ) ;
#54707=EDGE_LOOP ( 'NONE', ( #72832, #81412, #63345, #59271 ) ) ;
#54708=ORIENTED_EDGE ( 'NONE', *, *, #18880, .F. ) ;
#54710=CARTESIAN_POINT ( 'NONE',  ( 17.29993592101647337, -10.01129605718032423, 34.36064277460058491 ) ) ;
#54711=CARTESIAN_POINT ( 'NONE',  ( -2.372962308248626417, -10.33852847137145048, 34.16647553114627556 ) ) ;
#54713=CARTESIAN_POINT ( 'NONE',  ( 16.15384615384615330, -5.471508081941601098, 34.59228464037088457 ) ) ;
#54714=CARTESIAN_POINT ( 'NONE',  ( 14.05769230769230838, -7.500000000000001776, 35.00000000000000000 ) ) ;
#54715=CARTESIAN_POINT ( 'NONE',  ( 18.00000000000000000, -2.833524468853757305, 32.15551576947925838 ) ) ;
#54716=DIRECTION ( 'NONE',  ( -0.000000000000000000, 0.8660254037844397068, -0.4999999999999978906 ) ) ;
#54717=VERTEX_POINT ( 'NONE', #69088 ) ;
#54719=B_SPLINE_CURVE_WITH_KNOTS ( 'NONE', 3,
 ( #65795, #38339, #73013, #71670, #52730, #78428, #86999, #25271, #30688, #11309 ),
 .UNSPECIFIED., .F., .F.,
 ( 4, 2, 2, 2, 4 ),
 ( 0.0007817359430256297891, 0.0009771253907249961065, 0.001172514838424362424, 0.001367904286123728741, 0.001563293733823095059 ),
 .UNSPECIFIED. ) ;
#54720=ORIENTED_EDGE ( 'NONE', *, *, #88799, .F. ) ;
#54721=CARTESIAN_POINT ( 'NONE',  ( 11.47319109250076430, -9.442884908240170461, 34.35708131394840592 ) ) ;
#54722=ORIENTED_EDGE ( 'NONE', *, *, #5164, .F. ) ;
#54723=DIRECTION ( 'NONE',  ( 0.000000000000000000, 0.1736481776669267785, -0.9848077530122087975 ) ) ;
#54724=CARTESIAN_POINT ( 'NONE',  ( -17.07692307692277112, -2.506253911140615021, 30.00000000000323297 ) ) ;
#54725=EDGE_CURVE ( 'NONE', #30706, #79011, #79740, .T. ) ;
#54727=ORIENTED_EDGE ( 'NONE', *, *, #65014, .T. ) ;
#54728=VECTOR ( 'NONE', #72471, 999.9999999999998863 ) ;
#54729=CARTESIAN_POINT ( 'NONE',  ( -1.161835715637319133, -2.612705202774697533, 31.66806509827799943 ) ) ;
#54730=EDGE_CURVE ( 'NONE', #84238, #51881, #63610, .T. ) ;
#54732=EDGE_CURVE ( 'NONE', #71085, #30670, #25964, .T. ) ;
#54733=CARTESIAN_POINT ( 'NONE',  ( 2.241608896736428047, -6.386643153685125363, 34.62446782046654903 ) ) ;
#54734=FACE_BOUND ( 'NONE', #71832, .T. ) ;
#54735=CARTESIAN_POINT ( 'NONE',  ( -2.057746898314263273, -4.932303261841488151, 34.32971442181322885 ) ) ;
#54736=VECTOR ( 'NONE', #29152, 1000.000000000000000 ) ;
#54737=AXIS2_PLACEMENT_3D ( 'NONE', #2224, #16628, #36900 ) ;
#54738=EDGE_CURVE ( 'NONE', #20850, #82752, #59303, .T. ) ;
#54740=ORIENTED_EDGE ( 'NONE', *, *, #69907, .T. ) ;
#54741=CARTESIAN_POINT ( 'NONE',  ( -10.86538461538461320, -2.499999999999998668, 29.75000000000000355 ) ) ;
#54743=CARTESIAN_POINT ( 'NONE',  ( -0.4615384615381544209, -2.506253911140615021, 30.00000000000323297 ) ) ;
#54744=CARTESIAN_POINT ( 'NONE',  ( 15.36155967173618286, -6.369690395747422684, 34.87708834333098196 ) ) ;
#54745=ORIENTED_EDGE ( 'NONE', *, *, #26377, .T. ) ;
#54746=VECTOR ( 'NONE', #31269, 1000.000000000000000 ) ;
#54747=EDGE_CURVE ( 'NONE', #86296, #54717, #82625, .T. ) ;
#54749=CARTESIAN_POINT ( 'NONE',  ( -0.2115384615370421995, -7.500000000000154543, 35.00000000000007105 ) ) ;
#54750=CARTESIAN_POINT ( 'NONE',  ( 1.318533005255251744, -3.937682226553329556, 33.60647404775217240 ) ) ;
#54751=CARTESIAN_POINT ( 'NONE',  ( 18.00000000000000000, -12.48256725967547354, 35.29906147534542527 ) ) ;
#54752=DIRECTION ( 'NONE',  ( 0.000000000000000000, 0.4999999999999960032, -0.8660254037844410391 ) ) ;
#54753=CARTESIAN_POINT ( 'NONE',  ( -20.99999999999999645, -4.249999999999998224, 27.25000000000000000 ) ) ;
#54754=FACE_BOUND ( 'NONE', #56186, .T. ) ;
#54755=CARTESIAN_POINT ( 'NONE',  ( 13.16168842570853492, -11.98009711892699514, 32.48740034544076138 ) ) ;
#54756=CARTESIAN_POINT ( 'NONE',  ( -17.20761368003338632, -10.70098750199973203, 33.91152734681376302 ) ) ;
#54757=CARTESIAN_POINT ( 'NONE',  ( -7.053224132515145683, -12.27039167877662251, 31.24851455888617835 ) ) ;
#54758=CARTESIAN_POINT ( 'NONE',  ( 2.980769230769232170, -7.500000000000001776, 34.75000000000000000 ) ) ;
#54759=CARTESIAN_POINT ( 'NONE',  ( 15.36129493253279499, -10.19071101563364756, 33.96452234770658407 ) ) ;
#54760=CARTESIAN_POINT ( 'NONE',  ( -8.096130590202436750, -4.075325502946081535, 33.72974371597206300 ) ) ;
#54762=ORIENTED_EDGE ( 'NONE', *, *, #32693, .F. ) ;
#54763=CARTESIAN_POINT ( 'NONE',  ( -8.703061628268114802, -7.250054483168843156, 34.74374881642865631 ) ) ;
#54764=ORIENTED_EDGE ( 'NONE', *, *, #18584, .T. ) ;
#54765=DIRECTION ( 'NONE',  ( -0.000000000000000000, 1.000000000000000000, 3.491481338843133355E-15 ) ) ;
#54766=ORIENTED_EDGE ( 'NONE', *, *, #47592, .F. ) ;
#54767=CYLINDRICAL_SURFACE ( 'NONE', #8173, 0.2499999999999995559 ) ;
#54768=CARTESIAN_POINT ( 'NONE',  ( -16.15384615384615330, -11.91647553114624181, 32.58852847137148245 ) ) ;
#54770=ORIENTED_EDGE ( 'NONE', *, *, #50588, .F. ) ;
#54771=CARTESIAN_POINT ( 'NONE',  ( -15.36091644020745051, -5.195881422630166391, 34.18770438780619259 ) ) ;
#54774=CARTESIAN_POINT ( 'NONE',  ( -15.48079245499068435, -9.356822207818506598, 34.66110646841856635 ) ) ;
#54776=CARTESIAN_POINT ( 'NONE',  ( 17.01165263096229907, -12.46129190929999986, 30.37095296980880832 ) ) ;
#54777=LINE ( 'NONE', #69186, #7064 ) ;
#54778=CARTESIAN_POINT ( 'NONE',  ( -0.3307466537136745655, -4.118422570099827595, 33.43335022499816489 ) ) ;
#54779=DIRECTION ( 'NONE',  ( -0.000000000000000000, 0.6427876096865404731, -0.7660444431189770143 ) ) ;
#54780=B_SPLINE_CURVE_WITH_KNOTS ( 'NONE', 3,
 ( #72473, #31034, #80130, #31947, #72921, #4005, #17088, #10781, #44541, #51279 ),
 .UNSPECIFIED., .F., .F.,
 ( 4, 2, 2, 2, 4 ),
 ( 0.000000000000000000, 0.0001954311564186864407, 0.0003908623128373728815, 0.0005862934692560593493, 0.0007817246256747457630 ),
 .UNSPECIFIED. ) ;
#54782=CARTESIAN_POINT ( 'NONE',  ( -16.15384615384615330, -1.422936976036506707, 30.56769352161908415 ) ) ;
#54783=CARTESIAN_POINT ( 'NONE',  ( -4.284536756956462078, -2.845849958028613624, 32.17971566917920967 ) ) ;
#54785=VECTOR ( 'NONE', #82387, 1000.000000000000227 ) ;
#54786=CARTESIAN_POINT ( 'NONE',  ( 9.442307692307693401, -7.500000000000001776, 35.04278698407183867 ) ) ;
#54788=CARTESIAN_POINT ( 'NONE',  ( -17.75005448165186195, -12.43552623307873972, 30.55307653245132826 ) ) ;
#54789=CARTESIAN_POINT ( 'NONE',  ( 17.32686859527121825, -11.86320923018887541, 32.19269448109604781 ) ) ;
#54791=CARTESIAN_POINT ( 'NONE',  ( 1.607395053593451806, -8.540255544307065350, 34.89611431652622286 ) ) ;
#54793=CARTESIAN_POINT ( 'NONE',  ( -5.076923076923197442, -6.026961402154118908, 34.52809138561165270 ) ) ;
#54794=ORIENTED_EDGE ( 'NONE', *, *, #27771, .T. ) ;
#54795=DIRECTION ( 'NONE',  ( -0.000000000000000000, -0.9396926207859092051, -0.3420201433256662704 ) ) ;
#54796=B_SPLINE_CURVE_WITH_KNOTS ( 'NONE', 3,
 ( #12498, #88625, #75966, #67883, #19691, #34089, #82292, #7515, #81408, #34971 ),
 .UNSPECIFIED., .F., .F.,
 ( 4, 2, 2, 2, 4 ),
 ( 0.0007817246256747446788, 0.0009771112852218874663, 0.001172497944769030145, 0.001367884604316172825, 0.001563271263863315720 ),
 .UNSPECIFIED. ) ;
#54797=CARTESIAN_POINT ( 'NONE',  ( 5.299886211189750895, -7.369474539155828730, 34.99858011523957657 ) ) ;
#54798=CARTESIAN_POINT ( 'NONE',  ( 16.02369894440793630, -9.418419913701741919, 34.36755862841477693 ) ) ;
#54799=B_SPLINE_CURVE_WITH_KNOTS ( 'NONE', 3,
 ( #27347, #67451, #26906, #82300, #20148, #20581, #48047, #59798, #88633, #75526 ),
 .UNSPECIFIED., .F., .F.,
 ( 4, 2, 2, 2, 4 ),
 ( 0.000000000000000000, 0.0001954339857564099680, 0.0003908679715128199361, 0.0005863019572692299312, 0.0007817359430256398721 ),
 .UNSPECIFIED. ) ;
#54800=CARTESIAN_POINT ( 'NONE',  ( 2.057715563643716994, -4.075325502946086864, 33.72974371597207721 ) ) ;
#54801=CARTESIAN_POINT ( 'NONE',  ( 6.792929713638702793, -5.195881422630167279, 34.18770438780618548 ) ) ;
#54802=EDGE_CURVE ( 'NONE', #38366, #18924, #35713, .T. ) ;
#54803=EDGE_CURVE ( 'NONE', #6878, #36243, #19016, .T. ) ;
#54805=ORIENTED_EDGE ( 'NONE', *, *, #16887, .F. ) ;
#54806=EDGE_LOOP ( 'NONE', ( #28150, #71984, #65494, #56410 ) ) ;
#54807=ORIENTED_EDGE ( 'NONE', *, *, #82435, .F. ) ;
#54808=ADVANCED_FACE ( 'NONE', ( #71731 ), #37058, .F. ) ;
#54809=ORIENTED_EDGE ( 'NONE', *, *, #76660, .F. ) ;
#54811=AXIS2_PLACEMENT_3D ( 'NONE', #86456, #67058, #24730 ) ;
#54812=CARTESIAN_POINT ( 'NONE',  ( -13.44988583057615728, -3.835265460703609186, 33.15142922261924241 ) ) ;
#54813=CYLINDRICAL_SURFACE ( 'NONE', #47238, 0.2500000000000004996 ) ;
#54814=EDGE_CURVE ( 'NONE', #20693, #1437, #15286, .T. ) ;
#54815=CARTESIAN_POINT ( 'NONE',  ( 2.307692307692309264, -5.557115091759785130, 34.35708131394839171 ) ) ;
#54816=CARTESIAN_POINT ( 'NONE',  ( -16.94687564167263005, -7.723484941389743952, 34.99544897038808955 ) ) ;
#54817=VECTOR ( 'NONE', #28063, 999.9999999999998863 ) ;
#54818=EDGE_CURVE ( 'NONE', #11535, #20749, #72218, .T. ) ;
#54819=CARTESIAN_POINT ( 'NONE',  ( -16.94613126909829148, -4.809403383903226192, 33.96459661697924304 ) ) ;
#54820=ORIENTED_EDGE ( 'NONE', *, *, #4194, .T. ) ;
#54822=VERTEX_POINT ( 'NONE', #71287 ) ;
#54823=CARTESIAN_POINT ( 'NONE',  ( -7.146003881983769901, -2.523278758544489797, 31.42238647778637528 ) ) ;
#54824=EDGE_LOOP ( 'NONE', ( #16258, #40889, #47410, #42262 ) ) ;
#54827=B_SPLINE_CURVE_WITH_KNOTS ( 'NONE', 3,
 ( #63107, #20372, #82076, #6842, #7297, #55911, #62662, #48713, #83406, #1419 ),
 .UNSPECIFIED., .F., .F.,
 ( 4, 2, 2, 2, 4 ),
 ( 0.0007817246256747472808, 0.0009771112852218907189, 0.001172497944769034265, 0.001367884604316177595, 0.001563271263863321141 ),
 .UNSPECIFIED. ) ;
#54828=DIRECTION ( 'NONE',  ( 0.000000000000000000, 0.7660444431189807890, 0.6427876096865361433 ) ) ;
#54829=B_SPLINE_CURVE_WITH_KNOTS ( 'NONE', 3,
 ( #8049, #35518, #1278, #7161, #21554, #28768, #406, #22440, #15693, #55776 ),
 .UNSPECIFIED., .F., .F.,
 ( 4, 2, 2, 2, 4 ),
 ( 0.000000000000000000, 0.0001954311564186873623, 0.0003908623128373747246, 0.0005862934692560620598, 0.0007817246256747494492 ),
 .UNSPECIFIED. ) ;
#54830=EDGE_CURVE ( 'NONE', #57014, #43002, #27093, .T. ) ;
#54832=CARTESIAN_POINT ( 'NONE',  ( -5.934744428723973897, -4.481592998940251427, 33.73612834413965089 ) ) ;
#54833=VERTEX_POINT ( 'NONE', #2384 ) ;
#54835=EDGE_LOOP ( 'NONE', ( #49410, #73545, #24238, #316 ) ) ;
#54836=CARTESIAN_POINT ( 'NONE',  ( 14.37375964104238513, -10.67929555188718282, 33.92786785259544757 ) ) ;
#54837=CYLINDRICAL_SURFACE ( 'NONE', #58872, 0.2500000000000009437 ) ;
#54839=CARTESIAN_POINT ( 'NONE',  ( -11.40767109749459074, -12.62708834333097663, 30.88030960425257021 ) ) ;
#54842=CARTESIAN_POINT ( 'NONE',  ( -0.6850233861027926752, -6.716662450894490100, 34.94144148231605840 ) ) ;
#54844=AXIS2_PLACEMENT_3D ( 'NONE', #84372, #29862, #42938 ) ;
#54847=ORIENTED_EDGE ( 'NONE', *, *, #76555, .F. ) ;
#54848=FACE_BOUND ( 'NONE', #72046, .T. ) ;
#54849=EDGE_CURVE ( 'NONE', #38767, #39886, #16791, .T. ) ;
#54850=B_SPLINE_CURVE_WITH_KNOTS ( 'NONE', 3,
 ( #88384, #81172, #13147, #19895, #53233, #47364, #39299, #80736, #19456, #46918 ),
 .UNSPECIFIED., .F., .F.,
 ( 4, 2, 2, 2, 4 ),
 ( 0.000000000000000000, 0.0001954339857564070678, 0.0003908679715128141356, 0.0005863019572692211492, 0.0007817359430256282712 ),
 .UNSPECIFIED. ) ;
#54851=LINE ( 'NONE', #12981, #42750 ) ;
#54852=CARTESIAN_POINT ( 'NONE',  ( 16.15384615384615330, -2.486705287966279876, 31.30864560766543647 ) ) ;
#54853=CARTESIAN_POINT ( 'NONE',  ( 12.46153846153833911, -6.835583212225970762, 34.95778746994575670 ) ) ;
#54854=CARTESIAN_POINT ( 'NONE',  ( -17.75000000000000711, -12.75000000000000178, 29.81919447696817116 ) ) ;
#54855=CARTESIAN_POINT ( 'NONE',  ( 18.22277954126840172, -4.387253974876675677, 33.66317474335728832 ) ) ;
#54856=CARTESIAN_POINT ( 'NONE',  ( -4.153846153846273204, -2.892918686052165622, 31.69288490824153470 ) ) ;
#54857=LINE ( 'NONE', #82341, #1646 ) ;
#54858=EDGE_LOOP ( 'NONE', ( #74891, #59591, #80090, #11446 ) ) ;
#54859=LINE ( 'NONE', #364, #44637 ) ;
#54860=CARTESIAN_POINT ( 'NONE',  ( -7.911404836315086619, -2.506253911140460922, 30.00000000000013856 ) ) ;
#54861=EDGE_LOOP ( 'NONE', ( #56023, #25307, #82747, #73677 ) ) ;
#54862=EDGE_CURVE ( 'NONE', #48928, #18617, #78606, .T. ) ;
#54865=CARTESIAN_POINT ( 'NONE',  ( 9.442284455014727129, -2.823816976329317274, 31.52131813110795733 ) ) ;
#54866=ORIENTED_EDGE ( 'NONE', *, *, #25633, .T. ) ;
#54867=DIRECTION ( 'NONE',  ( -0.000000000000000000, -0.5000000000000009992, -0.8660254037844380415 ) ) ;
#54868=CARTESIAN_POINT ( 'NONE',  ( -7.053768389744483613, -9.804603061927743113, 34.18744698557895845 ) ) ;
#54869=FACE_BOUND ( 'NONE', #61464, .T. ) ;
#54871=DIRECTION ( 'NONE',  ( 1.000000000000000000, 0.000000000000000000, 0.000000000000000000 ) ) ;
#54872=CARTESIAN_POINT ( 'NONE',  ( 3.930361229281820190, -12.47654668319379567, 31.42292124445336654 ) ) ;
#54874=CARTESIAN_POINT ( 'NONE',  ( 9.692307692307695177, -6.435427911321262684, 35.78748833219616898 ) ) ;
#54876=LINE ( 'NONE', #6687, #31996 ) ;
#54877=B_SPLINE_CURVE_WITH_KNOTS ( 'NONE', 3,
 ( #60743, #26526, #40491, #67955, #33721, #89129, #20641, #15226, #50753, #1251 ),
 .UNSPECIFIED., .F., .F.,
 ( 4, 2, 2, 2, 4 ),
 ( 0.000000000000000000, 0.0001954311584214072923, 0.0003908623168428145846, 0.0005862934752642218498, 0.0007817246336856291692 ),
 .UNSPECIFIED. ) ;
#54879=ORIENTED_EDGE ( 'NONE', *, *, #50500, .T. ) ;
#54880=B_SPLINE_CURVE_WITH_KNOTS ( 'NONE', 3,
 ( #39060, #79591, #47118, #74608, #80483, #40389, #67847, #18330, #17888, #46246 ),
 .UNSPECIFIED., .F., .F.,
 ( 4, 2, 2, 2, 4 ),
 ( 0.0007817246256747519429, 0.0009771112852218959231, 0.001172497944769039686, 0.001367884604316183667, 0.001563271263863327647 ),
 .UNSPECIFIED. ) ;
#54881=AXIS2_PLACEMENT_3D ( 'NONE', #75029, #67378, #25942 ) ;
#54882=ORIENTED_EDGE ( 'NONE', *, *, #14503, .T. ) ;
#54883=LINE ( 'NONE', #67516, #76574 ) ;
#54885=CARTESIAN_POINT ( 'NONE',  ( 14.37375964104238513, -9.058645607665452459, 34.76329471203371924 ) ) ;
#54886=CARTESIAN_POINT ( 'NONE',  ( 10.83839745947801347, -2.889357225399416418, 32.26129605718031002 ) ) ;
#54887=CARTESIAN_POINT ( 'NONE',  ( 5.207448515156721136, -3.625058011473227815, 33.29252011169590020 ) ) ;
#54889=EDGE_CURVE ( 'NONE', #10626, #1790, #42093, .T. ) ;
#54890=CARTESIAN_POINT ( 'NONE',  ( 14.30769230769231015, -5.471508081941601098, 34.59228464037088457 ) ) ;
#54891=CARTESIAN_POINT ( 'NONE',  ( 5.933917620639865831, -2.833524468853757305, 32.15551576947924417 ) ) ;
#54892=EDGE_CURVE ( 'NONE', #85253, #73759, #71098, .T. ) ;
#54893=CARTESIAN_POINT ( 'NONE',  ( 6.130525438233648039, -4.299079248970732792, 33.91157788607253565 ) ) ;
#54894=CARTESIAN_POINT ( 'NONE',  ( -4.853910232829682592, -2.308499170217967134, 30.53291367094873721 ) ) ;
#54895=DIRECTION ( 'NONE',  ( -0.000000000000000000, -0.8660254037844397068, -0.4999999999999978906 ) ) ;
#54896=CARTESIAN_POINT ( 'NONE',  ( 18.22301135161285046, -9.886259254753566594, 34.14407573483972413 ) ) ;
#54897=CARTESIAN_POINT ( 'NONE',  ( 5.777073782483852504, -12.15238873228292071, 31.58232369045353849 ) ) ;
#54898=CARTESIAN_POINT ( 'NONE',  ( -6.673022503163469565, -3.435999193479609914, 33.07426656108010832 ) ) ;
#54899=DIRECTION ( 'NONE',  ( 0.000000000000000000, 0.1736481776669275834, 0.9848077530122086864 ) ) ;
#54900=ORIENTED_EDGE ( 'NONE', *, *, #62979, .T. ) ;
#54901=CARTESIAN_POINT ( 'NONE',  ( 3.930919936330005360, -4.887634598454295265, 34.01352882383564946 ) ) ;
#54902=CARTESIAN_POINT ( 'NONE',  ( 0.5923302693632462868, -2.541949514083464479, 30.39797389878540557 ) ) ;
#54905=FACE_OUTER_BOUND ( 'NONE', #50887, .T. ) ;
#54906=CYLINDRICAL_SURFACE ( 'NONE', #51386, 0.2499999999999994726 ) ;
#54910=CARTESIAN_POINT ( 'NONE',  ( 16.94677510719138169, -2.647304123082329763, 31.75400227202886683 ) ) ;
#54911=EDGE_LOOP ( 'NONE', ( #85414, #25135, #84803, #7260 ) ) ;
#54912=CARTESIAN_POINT ( 'NONE',  ( 6.000000000000001776, -13.49023893513002648, 31.06009739812518688 ) ) ;
#54914=B_SPLINE_CURVE_WITH_KNOTS ( 'NONE', 3,
 ( #5553, #6443, #33901, #46966, #60042, #75343, #41112, #26264, #54164, #33024 ),
 .UNSPECIFIED., .F., .F.,
 ( 4, 2, 2, 2, 4 ),
 ( 0.0007817359430256372700, 0.0009771253907250054306, 0.001172514838424373700, 0.001367904286123741969, 0.001563293733823110021 ),
 .UNSPECIFIED. ) ;
#54915=VERTEX_POINT ( 'NONE', #47710 ) ;
#54917=B_SPLINE_CURVE_WITH_KNOTS ( 'NONE', 3,
 ( #19258, #40426, #46724, #74202, #39983, #68325, #67885, #67445, #75092, #13377 ),
 .UNSPECIFIED., .F., .F.,
 ( 4, 2, 2, 2, 4 ),
 ( 0.0007817246256747484735, 0.0009771112852218928873, 0.001172497944769037084, 0.001367884604316181498, 0.001563271263863325912 ),
 .UNSPECIFIED. ) ;
#54918=CARTESIAN_POINT ( 'NONE',  ( 14.24242186173153435, -2.625532179533445198, 30.86335684631481513 ) ) ;
#54919=DIRECTION ( 'NONE',  ( -0.000000000000000000, 0.6427876096865404731, -0.7660444431189771253 ) ) ;
#54920=CARTESIAN_POINT ( 'NONE',  ( -15.16551365949320562, -12.46129190930001052, 30.37095296980870174 ) ) ;
#54921=EDGE_LOOP ( 'NONE', ( #39366, #86302, #10847, #22881 ) ) ;
#54922=VECTOR ( 'NONE', #33428, 1000.000000000000000 ) ;
#54923=EDGE_LOOP ( 'NONE', ( #69370, #77838, #4405, #9019 ) ) ;
#54924=DIRECTION ( 'NONE',  ( -0.000000000000000000, 1.000000000000000000, 3.491481338843133355E-15 ) ) ;
#54925=ORIENTED_EDGE ( 'NONE', *, *, #15921, .T. ) ;
#54926=CARTESIAN_POINT ( 'NONE',  ( -7.976844449264155479, -2.295517848115769421, 30.44137282052137294 ) ) ;
#54927=CARTESIAN_POINT ( 'NONE',  ( 12.46153846153846168, -8.973038597847269315, 34.52809138561121927 ) ) ;
#54928=CARTESIAN_POINT ( 'NONE',  ( -17.32689980786543060, -5.728515186090277211, 34.42611988154120439 ) ) ;
#54929=EDGE_CURVE ( 'NONE', #68374, #3616, #86609, .T. ) ;
#54930=CARTESIAN_POINT ( 'NONE',  ( -2.307692307692427391, -6.026961402154118908, 34.52809138561165270 ) ) ;
#54931=CYLINDRICAL_SURFACE ( 'NONE', #33473, 0.2500000000000009437 ) ;
#54932=CARTESIAN_POINT ( 'NONE',  ( 1.319345384059066983, -2.379036618887870880, 30.90682066428147579 ) ) ;
#54934=CARTESIAN_POINT ( 'NONE',  ( 10.54930120442873687, -12.10708131394839349, 31.69288490824020244 ) ) ;
#54935=VERTEX_POINT ( 'NONE', #31647 ) ;
#54936=VERTEX_POINT ( 'NONE', #33757 ) ;
#54937=CARTESIAN_POINT ( 'NONE',  ( -0.3310127597748961925, -12.27024696741798770, 31.24895572276497546 ) ) ;
#54938=ORIENTED_EDGE ( 'NONE', *, *, #36108, .F. ) ;
#54939=EDGE_CURVE ( 'NONE', #84958, #33781, #59109, .T. ) ;
#54942=AXIS2_PLACEMENT_3D ( 'NONE', #64843, #86485, #45467 ) ;
#54943=CARTESIAN_POINT ( 'NONE',  ( 10.48482470177125059, -2.254533558242299396, 29.97296025877828285 ) ) ;
#54944=CARTESIAN_POINT ( 'NONE',  ( 11.53846153846153832, -12.10708131394839349, 31.69288490824020244 ) ) ;
#54945=ORIENTED_EDGE ( 'NONE', *, *, #83067, .T. ) ;
#54946=CARTESIAN_POINT ( 'NONE',  ( -12.33101275977489841, -6.001044277235009439, 34.52024696741798948 ) ) ;
#54947=AXIS2_PLACEMENT_3D ( 'NONE', #291, #75951, #28195 ) ;
#54948=ADVANCED_FACE ( 'NONE', ( #67994 ), #67547, .F. ) ;
#54949=ORIENTED_EDGE ( 'NONE', *, *, #1303, .T. ) ;
#54951=VERTEX_POINT ( 'NONE', #5846 ) ;
#54952=CARTESIAN_POINT ( 'NONE',  ( 7.846153846153846700, -9.780366693483667717, 34.19971097300155094 ) ) ;
#54953=ORIENTED_EDGE ( 'NONE', *, *, #63224, .F. ) ;
#54954=CARTESIAN_POINT ( 'NONE',  ( -8.835314180186648159, -4.786620604624113540, 33.94971097300155805 ) ) ;
#54956=FACE_BOUND ( 'NONE', #35572, .T. ) ;
#54957=EDGE_CURVE ( 'NONE', #87554, #76215, #67928, .T. ) ;
#54959=CARTESIAN_POINT ( 'NONE',  ( 15.90382292962469890, -3.520140089381496473, 33.17453946501458262 ) ) ;
#54960=CARTESIAN_POINT ( 'NONE',  ( -16.15384615384615330, -4.661471528628507777, 34.16647553114623292 ) ) ;
#54961=CARTESIAN_POINT ( 'NONE',  ( 17.07692307692307665, -13.95598074871891292, 31.83374038241031911 ) ) ;
#54964=ADVANCED_FACE ( 'NONE', ( #75616 ), #83729, .T. ) ;
#54965=CARTESIAN_POINT ( 'NONE',  ( -14.30769230769242739, -3.835265460704628371, 33.15142922262033665 ) ) ;
#54966=ORIENTED_EDGE ( 'NONE', *, *, #87400, .F. ) ;
#54967=B_SPLINE_CURVE_WITH_KNOTS ( 'NONE', 3,
 ( #76316, #49730, #84423, #14623, #42543, #7428, #63246, #27687, #223, #29037 ),
 .UNSPECIFIED., .F., .F.,
 ( 4, 2, 2, 2, 4 ),
 ( 0.000000000000000000, 0.0001954311564186882568, 0.0003908623128373765136, 0.0005862934692560647703, 0.0007817246256747530271 ),
 .UNSPECIFIED. ) ;
#54968=EDGE_LOOP ( 'NONE', ( #39802, #16679, #20565, #69973, #72526, #9936, #9436, #46778 ) ) ;
#54969=CARTESIAN_POINT ( 'NONE',  ( 17.07692307692307665, -12.48256725967547354, 35.29906147534542527 ) ) ;
#54970=CARTESIAN_POINT ( 'NONE',  ( 8.069165197766697162, -9.886259254753566594, 34.14407573483972413 ) ) ;
#54971=AXIS2_PLACEMENT_3D ( 'NONE', #86470, #80138, #18439 ) ;
#54972=CARTESIAN_POINT ( 'NONE',  ( -12.46153846153858247, -2.625532179533778709, 30.86335684631627174 ) ) ;
#54973=CARTESIAN_POINT ( 'NONE',  ( 3.480823542407545546, -10.66356715214248396, 33.62249196103329751 ) ) ;
#54974=CARTESIAN_POINT ( 'NONE',  ( -17.30040800148741553, -12.47654668319379567, 31.42292124445336654 ) ) ;
#54975=CARTESIAN_POINT ( 'NONE',  ( 9.757563263583721280, -2.625532179533470512, 30.86335684631491105 ) ) ;
#54976=VERTEX_POINT ( 'NONE', #30097 ) ;
#54977=CARTESIAN_POINT ( 'NONE',  ( -5.750054590621955342, -8.476813868363244353, 34.90874843262270133 ) ) ;
#54978=EDGE_CURVE ( 'NONE', #32754, #4121, #2342, .T. ) ;
#54979=CARTESIAN_POINT ( 'NONE',  ( 3.480714749117373330, -11.37275283266503756, 32.91324779482534524 ) ) ;
#54980=CARTESIAN_POINT ( 'NONE',  ( -14.24162497434223162, -12.34228464037088813, 31.77849191805839268 ) ) ;
#54981=CARTESIAN_POINT ( 'NONE',  ( 3.230769230769231726, -3.050289026998446396, 32.03036669348365706 ) ) ;
#54982=ORIENTED_EDGE ( 'NONE', *, *, #81443, .T. ) ;
#54983=ORIENTED_EDGE ( 'NONE', *, *, #83582, .F. ) ;
#54984=ORIENTED_EDGE ( 'NONE', *, *, #35536, .F. ) ;
#54985=DIRECTION ( 'NONE',  ( -0.000000000000000000, 0.7660444431189791237, -0.6427876096865379196 ) ) ;
#54986=VERTEX_POINT ( 'NONE', #76516 ) ;
#54987=CARTESIAN_POINT ( 'NONE',  ( -9.822454901745912181, -12.45813303252208648, 30.39737893381572675 ) ) ;
#54988=CARTESIAN_POINT ( 'NONE',  ( -12.23875892027004930, -6.760870238392817200, 34.69528174975672385 ) ) ;
#54989=CARTESIAN_POINT ( 'NONE',  ( 5.076923076922954969, -6.879047030192662504, 34.71129190930017927 ) ) ;
#54990=CARTESIAN_POINT ( 'NONE',  ( -16.94613126909829148, -12.11778462344220841, 31.66786338562085135 ) ) ;
#54991=ADVANCED_FACE ( 'NONE', ( #85051 ), #15705, .F. ) ;
#54992=CARTESIAN_POINT ( 'NONE',  ( 9.915087233576102221, -5.913360116392397892, 34.49180327182771322 ) ) ;
#54993=VERTEX_POINT ( 'NONE', #49490 ) ;
#54995=CARTESIAN_POINT ( 'NONE',  ( -0.5916864312701560769, -5.915902021225892149, 34.75552854090298638 ) ) ;
#54996=ORIENTED_EDGE ( 'NONE', *, *, #22345, .F. ) ;
#54997=CARTESIAN_POINT ( 'NONE',  ( -5.143005456283213483, -2.292212530054419606, 30.41441678777542634 ) ) ;
#54998=DIRECTION ( 'NONE',  ( 0.000000000000000000, -6.938893903907222067E-15, 1.000000000000000000 ) ) ;
#54999=CARTESIAN_POINT ( 'NONE',  ( -11.53846153846153655, -10.67929555188718282, 33.92786785259544047 ) ) ;
#55001=EDGE_CURVE ( 'NONE', #77704, #56543, #4605, .T. ) ;
#55002=CARTESIAN_POINT ( 'NONE',  ( 9.692307692307695177, -10.51840700105979565, 33.73612834413961536 ) ) ;
#55003=CARTESIAN_POINT ( 'NONE',  ( -12.71156169883142795, -2.823816976329319051, 31.52131813110795733 ) ) ;
#55004=CARTESIAN_POINT ( 'NONE',  ( 17.30035003878465005, -7.630147231320743018, 34.74852402298682819 ) ) ;
#55005=CARTESIAN_POINT ( 'NONE',  ( 12.71159277317677549, -11.28795663066794575, 33.01431243580653785 ) ) ;
#55007=EDGE_CURVE ( 'NONE', #72869, #25632, #14823, .T. ) ;
#55008=ORIENTED_EDGE ( 'NONE', *, *, #56649, .T. ) ;
#55009=B_SPLINE_CURVE_WITH_KNOTS ( 'NONE', 3,
 ( #17156, #37878, #31107, #65782, #24349, #4077, #41882, #40557, #61685, #53609 ),
 .UNSPECIFIED., .F., .F.,
 ( 4, 2, 2, 2, 4 ),
 ( 0.0007817246256747460882, 0.0009771112852218892010, 0.001172497944769032314, 0.001367884604316175210, 0.001563271263863318323 ),
 .UNSPECIFIED. ) ;
#55010=ADVANCED_FACE ( 'NONE', ( #9387 ), #8505, .F. ) ;
#55011=CARTESIAN_POINT ( 'NONE',  ( -15.23076923076935252, -12.16647553114689728, 32.15551576947799362 ) ) ;
#55012=CARTESIAN_POINT ( 'NONE',  ( 1.319345384059066761, -9.528491918058357157, 34.59228464037090589 ) ) ;
#55013=AXIS2_PLACEMENT_3D ( 'NONE', #32072, #80265, #87481 ) ;
#55014=AXIS2_PLACEMENT_3D ( 'NONE', #69340, #21586, #63452 ) ;
#55015=B_SPLINE_CURVE_WITH_KNOTS ( 'NONE', 3,
 ( #2242, #57202, #3130, #86472, #64383, #58968, #71588, #24287, #22967, #9458 ),
 .UNSPECIFIED., .F., .F.,
 ( 4, 2, 2, 2, 4 ),
 ( 0.0007817359430256296806, 0.0009771253907249958896, 0.001172514838424361990, 0.001367904286123728091, 0.001563293733823094408 ),
 .UNSPECIFIED. ) ;
#55016=CARTESIAN_POINT ( 'NONE',  ( 9.757562831820530747, -11.06231777344671130, 33.60647404775212976 ) ) ;
#55017=CARTESIAN_POINT ( 'NONE',  ( 6.923076923076800782, -3.643525952248796163, 33.31231777344771672 ) ) ;
#55018=EDGE_LOOP ( 'NONE', ( #27454, #67717 ) ) ;
#55019=FACE_OUTER_BOUND ( 'NONE', #73872, .T. ) ;
#55020=CARTESIAN_POINT ( 'NONE',  ( -5.999999999999998224, -5.471508081941601098, 34.59228464037088457 ) ) ;
#55023=CARTESIAN_POINT ( 'NONE',  ( -0.7115152055870523906, -10.82459398097509684, 33.81372124010185587 ) ) ;
#55024=LINE ( 'NONE', #82510, #22086 ) ;
#55025=ORIENTED_EDGE ( 'NONE', *, *, #83264, .T. ) ;
#55026=CARTESIAN_POINT ( 'NONE',  ( 6.249945518348143381, -5.852078868378311149, 34.47109172314383585 ) ) ;
#55027=CARTESIAN_POINT ( 'NONE',  ( -14.37296275365308418, -2.892918686051582977, 31.69288490824015980 ) ) ;
#55028=FACE_OUTER_BOUND ( 'NONE', #34835, .T. ) ;
#55029=ORIENTED_EDGE ( 'NONE', *, *, #30398, .F. ) ;
#55030=CYLINDRICAL_SURFACE ( 'NONE', #52794, 0.2499999999999986955 ) ;
#55031=ORIENTED_EDGE ( 'NONE', *, *, #43754, .F. ) ;
#55032=CARTESIAN_POINT ( 'NONE',  ( 12.46153846153846168, -12.34228464037088635, 31.77849191805839268 ) ) ;
#55034=CARTESIAN_POINT ( 'NONE',  ( 11.76147438255493327, -6.460100341425560444, 34.89618726649961644 ) ) ;
#55035=VERTEX_POINT ( 'NONE', #29228 ) ;
#55037=DIRECTION ( 'NONE',  ( 0.000000000000000000, 0.9396926207859126468, -0.3420201433256571111 ) ) ;
#55038=CARTESIAN_POINT ( 'NONE',  ( -10.74553182482283198, -6.001485441113819874, 34.52039167877662607 ) ) ;
#55039=VECTOR ( 'NONE', #5256, 1000.000000000000000 ) ;
#55040=CARTESIAN_POINT ( 'NONE',  ( -8.069638770718176701, -4.988325925672468131, 34.36044203135681130 ) ) ;
#55041=FACE_OUTER_BOUND ( 'NONE', #85386, .T. ) ;
#55042=ORIENTED_EDGE ( 'NONE', *, *, #8416, .T. ) ;
#55043=FACE_BOUND ( 'NONE', #56295, .T. ) ;
#55044=ORIENTED_EDGE ( 'NONE', *, *, #83558, .T. ) ;
#55045=CARTESIAN_POINT ( 'NONE',  ( -8.992715693795103604, -12.47654668319379567, 31.42292124445336654 ) ) ;
#55047=CARTESIAN_POINT ( 'NONE',  ( 6.130525438233648039, -5.915461855592777596, 34.75538340440931506 ) ) ;
#55048=CARTESIAN_POINT ( 'NONE',  ( 16.85399685940693004, -2.554751324335733376, 30.48935550225260727 ) ) ;
#55051=ORIENTED_EDGE ( 'NONE', *, *, #37624, .T. ) ;
#55052=CARTESIAN_POINT ( 'NONE',  ( -2.980823821391187511, -11.56426240980093567, 33.07394671870546432 ) ) ;
#55053=ORIENTED_EDGE ( 'NONE', *, *, #74196, .F. ) ;
#55055=CARTESIAN_POINT ( 'NONE',  ( -9.469344788746207442, -7.369474270740069777, 34.74850911626239736 ) ) ;
#55056=CARTESIAN_POINT ( 'NONE',  ( 4.153846153846154188, -3.050289026998446396, 32.03036669348365706 ) ) ;
#55057=VECTOR ( 'NONE', #48423, 1000.000000000000000 ) ;
#55058=DIRECTION ( 'NONE',  ( -0.000000000000000000, -0.1736481776669307198, -0.9848077530122080203 ) ) ;
#55059=EDGE_CURVE ( 'NONE', #59461, #33924, #84176, .T. ) ;
#55063=DIRECTION ( 'NONE',  ( 0.000000000000000000, 0.9396926207859126468, 0.3420201433256571111 ) ) ;
#55064=ORIENTED_EDGE ( 'NONE', *, *, #76972, .F. ) ;
#55065=ORIENTED_EDGE ( 'NONE', *, *, #54161, .F. ) ;
#55067=CARTESIAN_POINT ( 'NONE',  ( 3.230769230769231726, -9.584722331328613620, 36.20867863119891439 ) ) ;
#55068=LINE ( 'NONE', #61819, #12960 ) ;
#55069=CARTESIAN_POINT ( 'NONE',  ( -7.846153846153965716, -4.481592998941358097, 33.73612834414048933 ) ) ;
#55070=B_SPLINE_CURVE_WITH_KNOTS ( 'NONE', 3,
 ( #43205, #80561, #46310, #45859, #4429, #52165, #87321, #85966, #86882, #67035 ),
 .UNSPECIFIED., .F., .F.,
 ( 4, 2, 2, 2, 4 ),
 ( 0.0007817246256747502082, 0.0009771112852218941883, 0.001172497944769038385, 0.001367884604316182365, 0.001563271263863326346 ),
 .UNSPECIFIED. ) ;
#55071=CARTESIAN_POINT ( 'NONE',  ( -17.93393266664992680, -5.471508081941600210, 34.59228464037088457 ) ) ;
#55072=CARTESIAN_POINT ( 'NONE',  ( -15.29685161012936589, -9.905515769479276145, 34.41647553114623292 ) ) ;
#55073=FACE_BOUND ( 'NONE', #17851, .T. ) ;
#55074=CARTESIAN_POINT ( 'NONE',  ( 16.28463796167094202, -3.062576670634119758, 32.05464942895959979 ) ) ;
#55075=ORIENTED_EDGE ( 'NONE', *, *, #1489, .T. ) ;
#55076=EDGE_CURVE ( 'NONE', #75330, #78537, #20708, .T. ) ;
#55077=CARTESIAN_POINT ( 'NONE',  ( -18.00000000000012079, -5.219633306517615701, 34.19971097300220464 ) ) ;
#55078=CARTESIAN_POINT ( 'NONE',  ( 16.85343813319912698, -6.760086850603066466, 34.69517049084099369 ) ) ;
#55079=DIRECTION ( 'NONE',  ( 0.000000000000000000, 0.9396926207859126468, 0.3420201433256571111 ) ) ;
#55080=ORIENTED_EDGE ( 'NONE', *, *, #4309, .F. ) ;
#55081=CARTESIAN_POINT ( 'NONE',  ( -18.13069146666755671, -8.147922237126337563, 34.70805685702651999 ) ) ;
#55082=ORIENTED_EDGE ( 'NONE', *, *, #64848, .F. ) ;
#55083=FACE_BOUND ( 'NONE', #39217, .T. ) ;
#55085=CARTESIAN_POINT ( 'NONE',  ( -4.153846153846152411, -13.04860791097971706, 34.73218667398347037 ) ) ;
#55087=VERTEX_POINT ( 'NONE', #71079 ) ;
#55089=CARTESIAN_POINT ( 'NONE',  ( -17.07692307692307665, -9.905515769479276145, 34.41647553114623292 ) ) ;
#55090=CARTESIAN_POINT ( 'NONE',  ( -1.384615384615505151, -3.835265460704628371, 33.15142922262033665 ) ) ;
#55091=DIRECTION ( 'NONE',  ( -0.000000000000000000, -0.1736481776669307198, -0.9848077530122080203 ) ) ;
#55092=ORIENTED_EDGE ( 'NONE', *, *, #85795, .F. ) ;
#55093=CARTESIAN_POINT ( 'NONE',  ( 16.21991450484859243, -10.51840700105979565, 33.73612834413962247 ) ) ;
#55094=CIRCLE ( 'NONE', #59401, 0.2500000000000002220 ) ;
#55095=CARTESIAN_POINT ( 'NONE',  ( 5.076923076923075762, -1.117168528481311540, 33.14645433367849847 ) ) ;
#55096=CARTESIAN_POINT ( 'NONE',  ( -12.46153846153846168, -9.905515769479276145, 34.41647553114623292 ) ) ;
#55097=AXIS2_PLACEMENT_3D ( 'NONE', #71640, #5746, #37413 ) ;
#55098=ORIENTED_EDGE ( 'NONE', *, *, #82653, .T. ) ;
#55099=CARTESIAN_POINT ( 'NONE',  ( 6.000000000000001776, -2.292212530054420494, 30.41441678777542634 ) ) ;
#55100=CARTESIAN_POINT ( 'NONE',  ( 5.999999999999880096, -9.442884908241554243, 34.35708131394783038 ) ) ;
#55101=CARTESIAN_POINT ( 'NONE',  ( 16.21910129335899597, -12.16647553114626490, 32.15551576947920864 ) ) ;
#55102=FACE_OUTER_BOUND ( 'NONE', #60921, .T. ) ;
#55103=EDGE_CURVE ( 'NONE', #32391, #51245, #28779, .T. ) ;
#55105=DIRECTION ( 'NONE',  ( -0.000000000000000000, 0.9848077530122085754, -0.1736481776669273613 ) ) ;
#55106=CARTESIAN_POINT ( 'NONE',  ( 3.230769230769231726, -12.37446782046654192, 30.86335684631486131 ) ) ;
#55107=CARTESIAN_POINT ( 'NONE',  ( -2.530557729895944963, -2.501496062324912284, 29.88072118266895671 ) ) ;
#55108=CARTESIAN_POINT ( 'NONE',  ( 7.912222197156284054, -4.098570777380720287, 33.41473453929635440 ) ) ;
#55111=CARTESIAN_POINT ( 'NONE',  ( -17.77698864838715309, -9.086983370893047862, 34.49168942202179267 ) ) ;
#55112=VERTEX_POINT ( 'NONE', #39089 ) ;
#55113=EDGE_CURVE ( 'NONE', #60496, #10987, #44039, .T. ) ;
#55114=ORIENTED_EDGE ( 'NONE', *, *, #78644, .T. ) ;
#55115=CARTESIAN_POINT ( 'NONE',  ( -11.40767109749459074, -2.295524264805589354, 30.44142389570982488 ) ) ;
#55116=EDGE_LOOP ( 'NONE', ( #60987, #46777, #39520, #35251 ) ) ;
#55117=CARTESIAN_POINT ( 'NONE',  ( -4.284536756956458525, -2.494641256782728966, 31.33461815524612959 ) ) ;
#55119=CARTESIAN_POINT ( 'NONE',  ( 12.21153846153846168, -7.500000000000001776, 35.00000000000000000 ) ) ;
#55120=CARTESIAN_POINT ( 'NONE',  ( -12.46153846153846168, -12.78798330534102945, 29.74999999999997868 ) ) ;
#55121=CARTESIAN_POINT ( 'NONE',  ( -15.90379184220783948, -5.728107161865375829, 34.42597550085002922 ) ) ;
#55122=CARTESIAN_POINT ( 'NONE',  ( 22.75000000000000000, -10.50000000000000000, 29.75000000000000355 ) ) ;
#55124=FACE_OUTER_BOUND ( 'NONE', #61691, .T. ) ;
#55125=CARTESIAN_POINT ( 'NONE',  ( 6.857806922520603976, -12.51329471203370325, 31.30864560766548976 ) ) ;
#55127=CARTESIAN_POINT ( 'NONE',  ( -17.07692307692307665, -10.67929555188718282, 33.92786785259544047 ) ) ;
#55128=CARTESIAN_POINT ( 'NONE',  ( -2.307692307692305711, -5.180354513474913603, 36.12317359536750416 ) ) ;
#55131=VECTOR ( 'NONE', #51240, 999.9999999999998863 ) ;
#55132=ORIENTED_EDGE ( 'NONE', *, *, #1837, .T. ) ;
#55134=CARTESIAN_POINT ( 'NONE',  ( -15.23076923076922995, -6.681629849574314051, 35.83090037661290239 ) ) ;
#55135=DIRECTION ( 'NONE',  ( -0.000000000000000000, 1.000000000000000000, 3.491481338843133355E-15 ) ) ;
#55136=CARTESIAN_POINT ( 'NONE',  ( -6.923076923076922462, -13.20930481340135110, 34.54067556320372745 ) ) ;
#55137=CARTESIAN_POINT ( 'NONE',  ( 5.777073782483852504, -5.667676309546437530, 34.40238873228292249 ) ) ;
#55138=B_SPLINE_CURVE_WITH_KNOTS ( 'NONE', 3,
 ( #3386, #70966, #85821, #3832, #31766, #16905, #45259, #79050, #4278, #78161 ),
 .UNSPECIFIED., .F., .F.,
 ( 4, 2, 2, 2, 4 ),
 ( 0.0007817359430256324996, 0.0009771253907249991422, 0.001172514838424365676, 0.001367904286123732428, 0.001563293733823098962 ),
 .UNSPECIFIED. ) ;
#55139=CARTESIAN_POINT ( 'NONE',  ( 12.39545505058258001, -8.973038597847271092, 34.52809138561120506 ) ) ;
#55141=CARTESIAN_POINT ( 'NONE',  ( 14.30769230769218758, -9.442884908241554243, 34.35708131394783038 ) ) ;
#55142=ORIENTED_EDGE ( 'NONE', *, *, #73192, .F. ) ;
#55143=CARTESIAN_POINT ( 'NONE',  ( 18.25005441991345378, -3.435999193479609026, 33.07426656108011542 ) ) ;
#55145=CARTESIAN_POINT ( 'NONE',  ( -18.00000000000012079, -4.481592998941359873, 33.73612834414048933 ) ) ;
#55146=DIRECTION ( 'NONE',  ( 0.000000000000000000, 0.1736481776669267785, -0.9848077530122087975 ) ) ;
#55147=CARTESIAN_POINT ( 'NONE',  ( 17.07692307692307665, -2.249999999999998668, 29.75000000000001776 ) ) ;
#55148=DIRECTION ( 'NONE',  ( 0.000000000000000000, 0.3420201433256641055, -0.9396926207859100932 ) ) ;
#55149=CARTESIAN_POINT ( 'NONE',  ( -5.999999999999998224, -7.500000000000001776, 35.04278698407183867 ) ) ;
#55150=ADVANCED_FACE ( 'NONE', ( #71512 ), #17919, .F. ) ;
#55151=VERTEX_POINT ( 'NONE', #44927 ) ;
#55152=VECTOR ( 'NONE', #348, 1000.000000000000114 ) ;
#55153=VECTOR ( 'NONE', #8754, 1000.000000000000227 ) ;
#55154=ORIENTED_EDGE ( 'NONE', *, *, #81780, .F. ) ;
#55155=VERTEX_POINT ( 'NONE', #78273 ) ;
#55157=CARTESIAN_POINT ( 'NONE',  ( 13.31934493865461278, -3.300289026998414865, 32.46337939537583139 ) ) ;
#55158=CARTESIAN_POINT ( 'NONE',  ( -15.93106648486808119, -9.418065098278011860, 34.63729479722530158 ) ) ;
#55159=CARTESIAN_POINT ( 'NONE',  ( 14.24160992833217243, -2.486705287966279432, 31.30864560766542937 ) ) ;
#55160=CARTESIAN_POINT ( 'NONE',  ( 16.21991450484859953, -9.780366693483667717, 34.19971097300155805 ) ) ;
#55162=CARTESIAN_POINT ( 'NONE',  ( 17.86985203026830504, -3.069018819979304702, 32.56621877034667278 ) ) ;
#55163=CARTESIAN_POINT ( 'NONE',  ( 14.17700084102475344, -12.38065189839062263, 30.83690757178629482 ) ) ;
#55164=ORIENTED_EDGE ( 'NONE', *, *, #20701, .T. ) ;
#55165=EDGE_CURVE ( 'NONE', #7875, #73152, #14165, .T. ) ;
#55167=EDGE_LOOP ( 'NONE', ( #25362, #46112 ) ) ;
#55168=CARTESIAN_POINT ( 'NONE',  ( 11.28843830116857383, -9.271318131107980420, 34.42618302367067429 ) ) ;
#55169=VERTEX_POINT ( 'NONE', #87283 ) ;
#55170=CARTESIAN_POINT ( 'NONE',  ( 9.468822767743363400, -8.539481045369596401, 34.89627647299170832 ) ) ;
#55171=CARTESIAN_POINT ( 'NONE',  ( 7.173076923076986411, -7.434744429011176159, 34.75000000000000711 ) ) ;
#55173=ORIENTED_EDGE ( 'NONE', *, *, #9339, .T. ) ;
#55175=EDGE_CURVE ( 'NONE', #84371, #77885, #52132, .T. ) ;
#55178=VECTOR ( 'NONE', #2615, 1000.000000000000114 ) ;
#55179=FACE_BOUND ( 'NONE', #38764, .T. ) ;
#55180=CARTESIAN_POINT ( 'NONE',  ( -2.176901866725357237, -4.684288915650983043, 34.18129842949671371 ) ) ;
#55181=EDGE_CURVE ( 'NONE', #14974, #37386, #31428, .T. ) ;
#55183=ORIENTED_EDGE ( 'NONE', *, *, #1623, .F. ) ;
#55184=CARTESIAN_POINT ( 'NONE',  ( -3.230769230769229949, -10.67929555188718282, 33.92786785259544047 ) ) ;
#55185=CARTESIAN_POINT ( 'NONE',  ( -5.076923076923199218, -9.528491918059723176, 34.59228464037033035 ) ) ;
#55186=FACE_OUTER_BOUND ( 'NONE', #59022, .T. ) ;
#55187=DIRECTION ( 'NONE',  ( -0.000000000000000000, 1.000000000000000000, 3.491481338843133355E-15 ) ) ;
#55188=ORIENTED_EDGE ( 'NONE', *, *, #55970, .F. ) ;
#55189=B_SPLINE_CURVE_WITH_KNOTS ( 'NONE', 3,
 ( #20887, #35747, #15029, #27209, #82164, #34405 ),
 .UNSPECIFIED., .F., .F.,
 ( 4, 2, 4 ),
 ( 4.220987180333913997E-17, 0.0001954756301637145801, 0.0003909512603273869848 ),
 .UNSPECIFIED. ) ;
#55190=CARTESIAN_POINT ( 'NONE',  ( 6.222779541268409709, -8.496831190052096971, 34.64984203495476578 ) ) ;
#55191=CARTESIAN_POINT ( 'NONE',  ( 1.319345384059067428, -4.320704448112771878, 33.92786785259540494 ) ) ;
#55192=CARTESIAN_POINT ( 'NONE',  ( -12.52680890749923748, -12.27809138561121394, 31.22303859784730307 ) ) ;
#55193=CARTESIAN_POINT ( 'NONE',  ( -39.05038313613820122, -2.249999999999998668, 29.75000000000000355 ) ) ;
#55194=DIRECTION ( 'NONE',  ( -0.000000000000000000, 1.000000000000000000, 3.491481338843133355E-15 ) ) ;
#55195=EDGE_CURVE ( 'NONE', #86900, #54833, #22771, .T. ) ;
#55196=FACE_BOUND ( 'NONE', #7461, .T. ) ;
#55197=CARTESIAN_POINT ( 'NONE',  ( 2.307692307692309264, -11.33034616979429110, 35.88435417666054406 ) ) ;
#55198=CARTESIAN_POINT ( 'NONE',  ( 11.40777007179398339, -12.38065189839062263, 30.83690757178629482 ) ) ;
#55199=B_SPLINE_CURVE_WITH_KNOTS ( 'NONE', 3,
 ( #5448, #38336, #66242, #3648, #73907, #87889, #87432, #32026, #86996, #67147 ),
 .UNSPECIFIED., .F., .F.,
 ( 4, 2, 2, 2, 4 ),
 ( 0.000000000000000000, 0.0001954339881912774070, 0.0003908679763825548140, 0.0005863019645738322752, 0.0007817359527651096280 ),
 .UNSPECIFIED. ) ;
#55200=CARTESIAN_POINT ( 'NONE',  ( 5.142178216435913107, -2.379036618887895305, 30.90682066428159303 ) ) ;
#55201=CARTESIAN_POINT ( 'NONE',  ( 3.165445217964922175, -7.749976730030849303, 34.74374725381503737 ) ) ;
#55202=CARTESIAN_POINT ( 'NONE',  ( 5.777073782483853392, -10.61292498521070549, 33.66303323003028680 ) ) ;
#55203=EDGE_CURVE ( 'NONE', #51403, #30568, #37736, .T. ) ;
#55204=CARTESIAN_POINT ( 'NONE',  ( -7.976301815885541657, -4.299443229763728169, 33.91186481527756058 ) ) ;
#55205=B_SPLINE_CURVE_WITH_KNOTS ( 'NONE', 3,
 ( #38229, #65687, #3986, #56730, #84224, #22500, #49963, #77443, #11659, #40028 ),
 .UNSPECIFIED., .F., .F.,
 ( 4, 2, 2, 2, 4 ),
 ( 0.0007817359430256294638, 0.0009771253907249974075, 0.001172514838424365460, 0.001367904286123733295, 0.001563293733823094191 ),
 .UNSPECIFIED. ) ;
#55207=ORIENTED_EDGE ( 'NONE', *, *, #75433, .T. ) ;
#55208=LINE ( 'NONE', #15121, #10239 ) ;
#55209=ORIENTED_EDGE ( 'NONE', *, *, #81722, .T. ) ;
#55210=CARTESIAN_POINT ( 'NONE',  ( -13.16183571563731647, -10.97394488606064122, 33.68653795673694873 ) ) ;
#55211=ADVANCED_FACE ( 'NONE', ( #38629 ), #66088, .F. ) ;
#55212=ORIENTED_EDGE ( 'NONE', *, *, #29358, .F. ) ;
#55213=ADVANCED_FACE ( 'NONE', ( #25113 ), #44476, .F. ) ;
#55214=CARTESIAN_POINT ( 'NONE',  ( -11.31568186948346977, -6.717445702608402236, 34.94155399931962336 ) ) ;
#55215=CARTESIAN_POINT ( 'NONE',  ( -18.00000000000012079, -2.625532179533778709, 30.86335684631627174 ) ) ;
#55216=CARTESIAN_POINT ( 'NONE',  ( -9.469294848214294902, -11.43677907613344757, 33.22367315496202167 ) ) ;
#55217=ORIENTED_EDGE ( 'NONE', *, *, #49464, .T. ) ;
#55220=CARTESIAN_POINT ( 'NONE',  ( -10.55012947587177941, -12.70778746994558439, 30.41441678777536595 ) ) ;
#55221=CARTESIAN_POINT ( 'NONE',  ( -12.46153846153846168, -9.819645486525091727, 36.12317359536749706 ) ) ;
#55223=CARTESIAN_POINT ( 'NONE',  ( 16.94677586748485965, -12.45813303252208648, 30.39737893381572675 ) ) ;
#55224=CARTESIAN_POINT ( 'NONE',  ( 10.39189969082028497, -2.612411019501189369, 31.66733052389439962 ) ) ;
#55225=CARTESIAN_POINT ( 'NONE',  ( 2.372947878968334035, -2.892918686051626498, 31.69288490824026638 ) ) ;
#55226=CARTESIAN_POINT ( 'NONE',  ( -5.869474298236434961, -10.88167719472716399, 33.43325721877153711 ) ) ;
#55228=LINE ( 'NONE', #84054, #67839 ) ;
#55229=CARTESIAN_POINT ( 'NONE',  ( -6.065270000556318486, -3.643525952247789412, 33.31231777344662959 ) ) ;
#55230=EDGE_LOOP ( 'NONE', ( #8073, #72414, #29352, #53976 ) ) ;
#55233=DIRECTION ( 'NONE',  ( -0.000000000000000000, 0.5000000000000011102, -0.8660254037844380415 ) ) ;
#55234=CARTESIAN_POINT ( 'NONE',  ( -8.899378738962465007, -3.625366637846544116, 33.29286588640298561 ) ) ;
#55236=CARTESIAN_POINT ( 'NONE',  ( 7.053124529332606585, -7.723484964179500700, 34.74522123443823318 ) ) ;
#55237=CARTESIAN_POINT ( 'NONE',  ( -0.3954701105360226010, -9.780366693483669494, 34.19971097300155805 ) ) ;
#55238=LINE ( 'NONE', #7947, #49739 ) ;
#55240=CARTESIAN_POINT ( 'NONE',  ( -5.143006487878955646, -5.557115091759785130, 34.35708131394839171 ) ) ;
#55241=CARTESIAN_POINT ( 'NONE',  ( 13.60739492588379385, -2.600157965045224895, 30.74683119005207743 ) ) ;
#55242=B_SPLINE_CURVE_WITH_KNOTS ( 'NONE', 3,
 ( #68537, #5962, #20365, #81181, #55464, #6409, #75734, #54126, #33433, #14038 ),
 .UNSPECIFIED., .F., .F.,
 ( 4, 2, 2, 2, 4 ),
 ( 0.0007817246256747470640, 0.0009771112852218898515, 0.001172497944769032531, 0.001367884604316175427, 0.001563271263863318106 ),
 .UNSPECIFIED. ) ;
#55243=CARTESIAN_POINT ( 'NONE',  ( -10.61538461538473577, -9.528491918059723176, 34.59228464037033035 ) ) ;
#55244=CARTESIAN_POINT ( 'NONE',  ( -16.85414353565466783, -2.847695495035524438, 31.58253572463339154 ) ) ;
#55245=B_SPLINE_CURVE_WITH_KNOTS ( 'NONE', 3,
 ( #9970, #24816, #37894, #79776, #59493, #23918, #65360, #37435, #79327, #66243 ),
 .UNSPECIFIED., .F., .F.,
 ( 4, 2, 2, 2, 4 ),
 ( 0.0007817359430256294638, 0.0009771253907249950223, 0.001172514838424360472, 0.001367904286123725922, 0.001563293733823091372 ),
 .UNSPECIFIED. ) ;
#55246=ADVANCED_FACE ( 'NONE', ( #18363 ), #10273, .F. ) ;
#55247=CARTESIAN_POINT ( 'NONE',  ( -13.63459211555773720, -11.79746400365624659, 32.30657167506340954 ) ) ;
#55248=AXIS2_PLACEMENT_3D ( 'NONE', #13298, #80890, #19173 ) ;
#55249=ORIENTED_EDGE ( 'NONE', *, *, #83558, .F. ) ;
#55250=ORIENTED_EDGE ( 'NONE', *, *, #46634, .T. ) ;
#55252=VERTEX_POINT ( 'NONE', #51671 ) ;
#55253=CARTESIAN_POINT ( 'NONE',  ( 11.53846153846153832, -2.708943851104267164, 35.45975837776705220 ) ) ;
#55254=DIRECTION ( 'NONE',  ( -0.000000000000000000, -0.3420201433256694346, -0.9396926207859080948 ) ) ;
#55255=CARTESIAN_POINT ( 'NONE',  ( -7.846153846153844924, -12.78798330534103123, 29.99999999999997868 ) ) ;
#55256=FACE_OUTER_BOUND ( 'NONE', #65863, .T. ) ;
#55257=EDGE_CURVE ( 'NONE', #48006, #60933, #17474, .T. ) ;
#55258=EDGE_CURVE ( 'NONE', #41455, #13933, #36815, .T. ) ;
#55259=EDGE_LOOP ( 'NONE', ( #76303, #55948, #73241, #68685, #70800, #87901 ) ) ;
#55260=CARTESIAN_POINT ( 'NONE',  ( -17.07692307692307665, -4.098570777380720287, 33.41473453929634729 ) ) ;
#55261=EDGE_LOOP ( 'NONE', ( #5742, #82391 ) ) ;
#55263=ORIENTED_EDGE ( 'NONE', *, *, #77950, .T. ) ;
#55264=CARTESIAN_POINT ( 'NONE',  ( -3.165575248985873280, -2.506253911140448043, 29.99999999999988631 ) ) ;
#55265=ORIENTED_EDGE ( 'NONE', *, *, #8506, .T. ) ;
#55267=CARTESIAN_POINT ( 'NONE',  ( 5.869309396889694774, -12.62707690430377383, 30.88035979386743435 ) ) ;
#55268=EDGE_CURVE ( 'NONE', #46752, #64747, #41134, .T. ) ;
#55269=CARTESIAN_POINT ( 'NONE',  ( 6.000000000000001776, -1.129524287112498415, 32.06866353760679544 ) ) ;
#55270=CARTESIAN_POINT ( 'NONE',  ( 15.23076923076923173, -8.164416787775445883, 34.95778746994557906 ) ) ;
#55271=ORIENTED_EDGE ( 'NONE', *, *, #43823, .T. ) ;
#55272=EDGE_CURVE ( 'NONE', #65911, #9598, #69045, .T. ) ;
#55274=VECTOR ( 'NONE', #56860, 999.9999999999998863 ) ;
#55276=CARTESIAN_POINT ( 'NONE',  ( 4.153846153846154188, -2.900454961884010974, 35.62045528018868623 ) ) ;
#55277=CARTESIAN_POINT ( 'NONE',  ( 8.769230769230768274, -7.500000000000001776, 35.04278698407183867 ) ) ;
#55279=CARTESIAN_POINT ( 'NONE',  ( 6.856993512121044354, -6.386643153685125363, 34.62446782046654903 ) ) ;
#55280=CARTESIAN_POINT ( 'NONE',  ( -0.7115616857599186273, -6.652501968072646932, 34.93155406624980941 ) ) ;
#55282=ADVANCED_FACE ( 'NONE', ( #66999 ), #5291, .F. ) ;
#55283=CARTESIAN_POINT ( 'NONE',  ( -17.74994568836168440, -2.564540009722896752, 30.55348353981672105 ) ) ;
#55285=ORIENTED_EDGE ( 'NONE', *, *, #55709, .F. ) ;
#55286=FACE_BOUND ( 'NONE', #16398, .T. ) ;
#55287=CARTESIAN_POINT ( 'NONE',  ( 10.68064018666063575, -10.21337939537593620, 33.94971097300152252 ) ) ;
#55288=CARTESIAN_POINT ( 'NONE',  ( 16.08776377448601735, -2.486705287966279432, 31.30864560766543647 ) ) ;
#55289=CARTESIAN_POINT ( 'NONE',  ( 3.480823542407545546, -9.148310452688873440, 34.47095581063188519 ) ) ;
#55290=CARTESIAN_POINT ( 'NONE',  ( 7.846153846153846700, -10.67929555188718282, 33.92786785259544047 ) ) ;
#55291=CARTESIAN_POINT ( 'NONE',  ( -8.769230769230768274, -7.500000000000001776, 35.04278698407183867 ) ) ;
#55292=CYLINDRICAL_SURFACE ( 'NONE', #58195, 0.2499999999999998890 ) ;
#55293=CARTESIAN_POINT ( 'NONE',  ( -4.377331078410485077, -10.97335522853832579, 33.68706563782419749 ) ) ;
#55294=ORIENTED_EDGE ( 'NONE', *, *, #21133, .F. ) ;
#55295=CARTESIAN_POINT ( 'NONE',  ( 14.43848411551709887, -12.38066358083363738, 30.83685684665853444 ) ) ;
#55296=FACE_OUTER_BOUND ( 'NONE', #80700, .T. ) ;
#55298=CARTESIAN_POINT ( 'NONE',  ( 2.557692307693728129, -7.500000000000154543, 35.00000000000007105 ) ) ;
#55299=CARTESIAN_POINT ( 'NONE',  ( -7.846153846153844924, -2.292212530054420494, 30.41441678777542634 ) ) ;
#55301=DIRECTION ( 'NONE',  ( 0.000000000000000000, 0.1736481776669275834, 0.9848077530122086864 ) ) ;
#55302=CARTESIAN_POINT ( 'NONE',  ( 2.373759641042384683, -4.661471528628508665, 34.16647553114624003 ) ) ;
#55304=EDGE_CURVE ( 'NONE', #16656, #33691, #88620, .T. ) ;
#55305=FACE_BOUND ( 'NONE', #77547, .T. ) ;
#55306=CARTESIAN_POINT ( 'NONE',  ( 6.792386319966614572, -3.957541250942359756, 33.62499894934981626 ) ) ;
#55307=CARTESIAN_POINT ( 'NONE',  ( -6.923076923076922462, -1.215029322943914858, 32.30358669280327177 ) ) ;
#55308=CARTESIAN_POINT ( 'NONE',  ( 10.48523740594639619, -8.587444163452046197, 34.63053765926554206 ) ) ;
#55309=DIRECTION ( 'NONE',  ( -0.000000000000000000, -0.5000000000000009992, -0.8660254037844380415 ) ) ;
#55310=CARTESIAN_POINT ( 'NONE',  ( 16.15384615384603251, -10.33852847137269571, 34.16647553114546554 ) ) ;
#55311=CARTESIAN_POINT ( 'NONE',  ( -17.74994568836168440, -4.943051570960393271, 34.04725096376909477 ) ) ;
#55313=ORIENTED_EDGE ( 'NONE', *, *, #3553, .T. ) ;
#55315=EDGE_CURVE ( 'NONE', #20998, #22047, #33205, .T. ) ;
#55316=ORIENTED_EDGE ( 'NONE', *, *, #6293, .T. ) ;
#55317=CARTESIAN_POINT ( 'NONE',  ( -9.822998295418001291, -2.295517848115769421, 30.44137282052137294 ) ) ;
#55318=EDGE_CURVE ( 'NONE', #49527, #39557, #28199, .T. ) ;
#55319=CARTESIAN_POINT ( 'NONE',  ( -0.4615384615384611200, -2.721908614388771852, 31.22303859784724978 ) ) ;
#55320=CARTESIAN_POINT ( 'NONE',  ( 16.15384615384615330, -2.833524468853757305, 32.15551576947925838 ) ) ;
#55321=CARTESIAN_POINT ( 'NONE',  ( 7.846153846153846700, -13.53365097954675988, 30.81389545987213552 ) ) ;
#55322=CARTESIAN_POINT ( 'NONE',  ( 2.980792499826877773, -11.28823185664190376, 33.01397839955799896 ) ) ;
#55324=CARTESIAN_POINT ( 'NONE',  ( 4.403846153847589484, -7.500000000000155431, 34.75000000000007105 ) ) ;
#55325=CYLINDRICAL_SURFACE ( 'NONE', #43157, 0.2499999999999995559 ) ;
#55326=CARTESIAN_POINT ( 'NONE',  ( -5.999999999999998224, -6.681629849574314051, 35.83090037661290239 ) ) ;
#55327=LINE ( 'NONE', #47688, #45880 ) ;
#55329=DIRECTION ( 'NONE',  ( -0.000000000000000000, -0.5000000000000009992, -0.8660254037844380415 ) ) ;
#55330=CARTESIAN_POINT ( 'NONE',  ( -0.3962833220256233302, -4.320704448112861584, 33.92786785259548310 ) ) ;
#55331=CARTESIAN_POINT ( 'NONE',  ( 10.36538461538461675, -7.566082377512564960, 35.00000000000000711 ) ) ;
#55332=CARTESIAN_POINT ( 'NONE',  ( 2.980792499826876440, -2.564618984488975961, 30.55390908950641915 ) ) ;
#55333=EDGE_CURVE ( 'NONE', #34697, #36124, #7789, .T. ) ;
#55334=ORIENTED_EDGE ( 'NONE', *, *, #9022, .T. ) ;
#55335=CARTESIAN_POINT ( 'NONE',  ( 2.177001704582000485, -3.338472653186242756, 32.95098750199972670 ) ) ;
#55337=B_SPLINE_CURVE_WITH_KNOTS ( 'NONE', 3,
 ( #18778, #61081, #46245, #12457, #6146, #39502 ),
 .UNSPECIFIED., .F., .F.,
 ( 4, 2, 4 ),
 ( 2.168404344971008868E-19, 0.0001954784845028926274, 0.0003909569690057850379 ),
 .UNSPECIFIED. ) ;
#55341=VERTEX_POINT ( 'NONE', #62867 ) ;
#55342=EDGE_CURVE ( 'NONE', #65473, #47265, #13054, .T. ) ;
#55344=CARTESIAN_POINT ( 'NONE',  ( -14.53117725141625449, -12.24155766932282496, 31.33739205006857986 ) ) ;
#55345=ORIENTED_EDGE ( 'NONE', *, *, #56315, .F. ) ;
#55346=DIRECTION ( 'NONE',  ( -0.000000000000000000, 0.7660444431189791237, -0.6427876096865379196 ) ) ;
#55347=CARTESIAN_POINT ( 'NONE',  ( 12.46153846153833911, -5.941354392335915335, 34.76329471203413846 ) ) ;
#55348=EDGE_LOOP ( 'NONE', ( #34202, #13404 ) ) ;
#55349=CARTESIAN_POINT ( 'NONE',  ( 3.230769230769231726, -1.117168528481311540, 33.14645433367849847 ) ) ;
#55351=ORIENTED_EDGE ( 'NONE', *, *, #48661, .T. ) ;
#55352=CARTESIAN_POINT ( 'NONE',  ( -7.780086512803769949, -6.343179335718451384, 34.87096338111212646 ) ) ;
#55354=CARTESIAN_POINT ( 'NONE',  ( 8.703960768674447124, -6.835583212224499938, 34.95778746994557906 ) ) ;
#55355=DIRECTION ( 'NONE',  ( -0.000000000000000000, 0.7660444431189791237, -0.6427876096865379196 ) ) ;
#55356=ORIENTED_EDGE ( 'NONE', *, *, #15289, .F. ) ;
#55357=ORIENTED_EDGE ( 'NONE', *, *, #11073, .T. ) ;
#55358=CARTESIAN_POINT ( 'NONE',  ( 15.23076923076911093, -10.90142922262034020, 33.41473453929536674 ) ) ;
#55360=ORIENTED_EDGE ( 'NONE', *, *, #36491, .F. ) ;
#55361=EDGE_CURVE ( 'NONE', #70706, #72614, #19423, .T. ) ;
#55362=CARTESIAN_POINT ( 'NONE',  ( 3.453548899747295398, -12.11081565061823717, 32.26097654155341843 ) ) ;
#55363=CARTESIAN_POINT ( 'NONE',  ( 12.71148397988660150, -9.272278438253398036, 34.42582936511637115 ) ) ;
#55365=CARTESIAN_POINT ( 'NONE',  ( -9.692307692307691624, -4.786620604624113540, 33.94971097300155094 ) ) ;
#55366=CARTESIAN_POINT ( 'NONE',  ( -4.377331097570101193, -6.760086850603068243, 34.69517049084099369 ) ) ;
#55367=DIRECTION ( 'NONE',  ( 0.000000000000000000, 0.8660254037844377084, -0.5000000000000015543 ) ) ;
#55368=EDGE_CURVE ( 'NONE', #2477, #87198, #40971, .T. ) ;
#55369=LINE ( 'NONE', #69772, #77957 ) ;
#55370=B_SPLINE_CURVE_WITH_KNOTS ( 'NONE', 3,
 ( #67966, #81489, #88262, #12140, #67522, #66632, #19775, #5819, #47236, #74730 ),
 .UNSPECIFIED., .F., .F.,
 ( 4, 2, 2, 2, 4 ),
 ( 0.000000000000000000, 0.0001954311564186863323, 0.0003908623128373726646, 0.0005862934692560590241, 0.0007817246256747453293 ),
 .UNSPECIFIED. ) ;
#55371=B_SPLINE_CURVE_WITH_KNOTS ( 'NONE', 3,
 ( #13197, #40677, #6442, #88873, #33900, #15747, #6872, #9859, #16179, #61809 ),
 .UNSPECIFIED., .F., .F.,
 ( 4, 2, 2, 2, 4 ),
 ( 0.000000000000000000, 0.0001954339857564070949, 0.0003908679715128141898, 0.0005863019572692212576, 0.0007817359430256283796 ),
 .UNSPECIFIED. ) ;
#55372=VECTOR ( 'NONE', #20208, 1000.000000000000227 ) ;
#55373=ORIENTED_EDGE ( 'NONE', *, *, #62802, .T. ) ;
#55376=FACE_OUTER_BOUND ( 'NONE', #7046, .T. ) ;
#55377=EDGE_LOOP ( 'NONE', ( #27805, #26317, #5916, #968 ) ) ;
#55378=B_SPLINE_CURVE_WITH_KNOTS ( 'NONE', 3,
 ( #74943, #47002, #74490, #13236, #12787, #68178, #88474, #62292, #26743, #82143 ),
 .UNSPECIFIED., .F., .F.,
 ( 4, 2, 2, 2, 4 ),
 ( 0.0007817246336856289524, 0.0009771112958940101571, 0.001172497958102391253, 0.001367884620310772350, 0.001563271282519153446 ),
 .UNSPECIFIED. ) ;
#55379=CARTESIAN_POINT ( 'NONE',  ( 16.15384615384603251, -6.879047030192662504, 34.71129190930017927 ) ) ;
#55381=ORIENTED_EDGE ( 'NONE', *, *, #11877, .T. ) ;
#55382=CYLINDRICAL_SURFACE ( 'NONE', #16239, 0.2500000000000002220 ) ;
#55383=CARTESIAN_POINT ( 'NONE',  ( 5.207448778686640800, -3.816742781228458448, 33.13167719472716044 ) ) ;
#55384=AXIS2_PLACEMENT_3D ( 'NONE', #22589, #70787, #78410 ) ;
#55385=VERTEX_POINT ( 'NONE', #41740 ) ;
#55386=EDGE_CURVE ( 'NONE', #60358, #39836, #26919, .T. ) ;
#55387=CARTESIAN_POINT ( 'NONE',  ( -9.822868284049613763, -2.504760397472875155, 29.97295953869789997 ) ) ;
#55389=DIRECTION ( 'NONE',  ( -0.000000000000000000, -0.000000000000000000, -1.000000000000000000 ) ) ;
#55390=ORIENTED_EDGE ( 'NONE', *, *, #38859, .F. ) ;
#55391=DIRECTION ( 'NONE',  ( -0.000000000000000000, 0.6427876096865404731, -0.7660444431189770143 ) ) ;
#55392=EDGE_LOOP ( 'NONE', ( #14622, #88710, #7091, #153 ) ) ;
#55393=CARTESIAN_POINT ( 'NONE',  ( -9.019254006523732770, -5.056417327199099532, 34.11270091957321426 ) ) ;
#55394=CARTESIAN_POINT ( 'NONE',  ( -4.283994123577848256, -6.809168938359898782, 34.95455904226513866 ) ) ;
#55395=FACE_BOUND ( 'NONE', #20610, .T. ) ;
#55396=CARTESIAN_POINT ( 'NONE',  ( -17.77662405930182032, -2.501478030877322567, 29.88021232661720461 ) ) ;
#55397=LINE ( 'NONE', #77007, #3980 ) ;
#55398=CARTESIAN_POINT ( 'NONE',  ( 4.219914504848592429, -12.37446782046654192, 30.86335684631486842 ) ) ;
#55399=CARTESIAN_POINT ( 'NONE',  ( 12.33139049180676672, -3.625366637846545892, 33.29286588640298561 ) ) ;
#55400=CARTESIAN_POINT ( 'NONE',  ( 5.326868595271218254, -10.76462480002816235, 33.53768742498949962 ) ) ;
#55401=CARTESIAN_POINT ( 'NONE',  ( -4.403869391139119571, -11.37209801155882971, 32.91403422569032955 ) ) ;
#55402=CARTESIAN_POINT ( 'NONE',  ( 2.307692307692309264, -13.95598074871891292, 31.83374038241031911 ) ) ;
#55404=ORIENTED_EDGE ( 'NONE', *, *, #14671, .F. ) ;
#55406=CARTESIAN_POINT ( 'NONE',  ( 24.00000000000000000, -5.499999999999981348, 27.75000000000000000 ) ) ;
#55407=CARTESIAN_POINT ( 'NONE',  ( 16.37685750545900376, -12.15243808032446005, 31.58219941686247978 ) ) ;
#55408=B_SPLINE_CURVE_WITH_KNOTS ( 'NONE', 3,
 ( #40646, #7298, #20373, #47832, #61777, #34314, #35659, #69436, #75313, #28007 ),
 .UNSPECIFIED., .F., .F.,
 ( 4, 2, 2, 2, 4 ),
 ( 0.000000000000000000, 0.0001954339857564074473, 0.0003908679715128148945, 0.0005863019572692223418, 0.0007817359430256297891 ),
 .UNSPECIFIED. ) ;
#55409=CARTESIAN_POINT ( 'NONE',  ( -11.53846153846165912, -11.94971097300221174, 32.03036669348237098 ) ) ;
#55411=B_SPLINE_CURVE_WITH_KNOTS ( 'NONE', 3,
 ( #9725, #70988, #85839, #58344, #23678, #65549, #50251, #57908, #22787, #10175 ),
 .UNSPECIFIED., .F., .F.,
 ( 4, 2, 2, 2, 4 ),
 ( 0.0007817246256747459798, 0.0009771112852218896347, 0.001172497944769033181, 0.001367884604316176728, 0.001563271263863320491 ),
 .UNSPECIFIED. ) ;
#55412=CARTESIAN_POINT ( 'NONE',  ( 1.515405825582337052, -10.70102852606553157, 33.91149625220312913 ) ) ;
#55413=CARTESIAN_POINT ( 'NONE',  ( -12.23875879256039489, -4.989023458446560255, 34.36081565061822118 ) ) ;
#55414=B_SPLINE_CURVE_WITH_KNOTS ( 'NONE', 3,
 ( #58737, #46564, #18661, #17768, #3348, #73610, #5135, #31725, #38931, #19097 ),
 .UNSPECIFIED., .F., .F.,
 ( 4, 2, 2, 2, 4 ),
 ( 0.000000000000000000, 0.0001954339857564071491, 0.0003908679715128142982, 0.0005863019572692214744, 0.0007817359430256285964 ),
 .UNSPECIFIED. ) ;
#55415=ORIENTED_EDGE ( 'NONE', *, *, #12406, .F. ) ;
#55416=LINE ( 'NONE', #21626, #9786 ) ;
#55417=LINE ( 'NONE', #82902, #51635 ) ;
#55418=CARTESIAN_POINT ( 'NONE',  ( -8.769230769230890843, -12.27809138561165270, 31.22303859784587132 ) ) ;
#55420=ORIENTED_EDGE ( 'NONE', *, *, #81166, .T. ) ;
#55421=ORIENTED_EDGE ( 'NONE', *, *, #6964, .F. ) ;
#55422=EDGE_CURVE ( 'NONE', #23361, #46498, #84502, .T. ) ;
#55423=ORIENTED_EDGE ( 'NONE', *, *, #74142, .T. ) ;
#55424=CARTESIAN_POINT ( 'NONE',  ( -9.469528151039281028, -12.44528174975671853, 30.48912976160716681 ) ) ;
#55425=EDGE_CURVE ( 'NONE', #22884, #45410, #66526, .T. ) ;
#55426=EDGE_LOOP ( 'NONE', ( #43173, #30694, #9870, #77539 ) ) ;
#55427=CARTESIAN_POINT ( 'NONE',  ( -10.61538461538461320, -3.937682226553329556, 33.60647404775216529 ) ) ;
#55428=DIRECTION ( 'NONE',  ( -0.000000000000000000, 0.9396926207859092051, -0.3420201433256662704 ) ) ;
#55431=CARTESIAN_POINT ( 'NONE',  ( 14.43821800945587519, -4.459921816937791661, 33.71989282347011851 ) ) ;
#55432=ORIENTED_EDGE ( 'NONE', *, *, #20083, .T. ) ;
#55434=CARTESIAN_POINT ( 'NONE',  ( 11.53846153846141753, -10.21337939537710326, 33.94971097300076224 ) ) ;
#55435=LINE ( 'NONE', #76145, #81330 ) ;
#55436=ORIENTED_EDGE ( 'NONE', *, *, #78422, .T. ) ;
#55437=CARTESIAN_POINT ( 'NONE',  ( -39.05038313613820122, -2.249999999999998668, 29.75000000000000355 ) ) ;
#55438=CARTESIAN_POINT ( 'NONE',  ( -10.36533030374629938, -3.627508038966690496, 32.91356715214248396 ) ) ;
#55439=CARTESIAN_POINT ( 'NONE',  ( 0.4615384615384611200, -12.78798330534102945, 29.74999999999997868 ) ) ;
#55440=CARTESIAN_POINT ( 'NONE',  ( -18.00000000000000000, -1.145656007487079631, 33.13000708000598848 ) ) ;
#55441=CARTESIAN_POINT ( 'NONE',  ( -9.757577692864010999, -12.51329471203370325, 31.30864560766548976 ) ) ;
#55442=VECTOR ( 'NONE', #3201, 1000.000000000000114 ) ;
#55443=CARTESIAN_POINT ( 'NONE',  ( -3.454254155333563059, -10.97335522853832579, 33.68706563782419749 ) ) ;
#55444=CARTESIAN_POINT ( 'NONE',  ( -3.099930900282468649, -7.277220318596959281, 34.99547417642776992 ) ) ;
#55447=EDGE_LOOP ( 'NONE', ( #75276, #30259, #56363, #40875 ) ) ;
#55448=DIRECTION ( 'NONE',  ( -0.000000000000000000, -0.9848077530122086864, -0.1736481776669273613 ) ) ;
#55450=B_SPLINE_CURVE_WITH_KNOTS ( 'NONE', 3,
 ( #47993, #68275, #25517, #25956, #5684, #81359, #52973, #81801, #33608, #61507 ),
 .UNSPECIFIED., .F., .F.,
 ( 4, 2, 2, 2, 4 ),
 ( 0.000000000000000000, 0.0001954311584214073465, 0.0003908623168428146930, 0.0005862934752642220667, 0.0007817246336856293861 ),
 .UNSPECIFIED. ) ;
#55451=FACE_OUTER_BOUND ( 'NONE', #48003, .T. ) ;
#55452=DIRECTION ( 'NONE',  ( -0.000000000000000000, 0.1736481776669307198, -0.9848077530122080203 ) ) ;
#55453=EDGE_LOOP ( 'NONE', ( #44510, #59771 ) ) ;
#55454=CARTESIAN_POINT ( 'NONE',  ( 7.846153846153723244, -12.16647553114689728, 32.15551576947799362 ) ) ;
#55455=CARTESIAN_POINT ( 'NONE',  ( -3.361460697436787104, -10.54014554554150607, 33.71984207302941883 ) ) ;
#55456=AXIS2_PLACEMENT_3D ( 'NONE', #31010, #46314, #72445 ) ;
#55457=CARTESIAN_POINT ( 'NONE',  ( 14.30769230769262279, -2.255955759149395501, 30.00000000000324363 ) ) ;
#55458=DIRECTION ( 'NONE',  ( -0.000000000000000000, -0.9848077530122085754, -0.1736481776669273613 ) ) ;
#55459=VERTEX_POINT ( 'NONE', #17364 ) ;
#55460=CARTESIAN_POINT ( 'NONE',  ( 6.923076923076802558, -4.481592998941358097, 33.73612834414048933 ) ) ;
#55461=CARTESIAN_POINT ( 'NONE',  ( 17.14299142792551578, -5.557115091759786019, 34.35708131394839882 ) ) ;
#55464=CARTESIAN_POINT ( 'NONE',  ( -16.82697766754503377, -12.07971442181321997, 32.31769673815850297 ) ) ;
#55466=EDGE_LOOP ( 'NONE', ( #77784, #34778 ) ) ;
#55467=CARTESIAN_POINT ( 'NONE',  ( 1.134615384615387468, -7.433931650972300353, 34.75000000000000711 ) ) ;
#55468=CARTESIAN_POINT ( 'NONE',  ( 0.5920638997721054952, -10.31582465632705237, 34.18122507451815295 ) ) ;
#55470=ORIENTED_EDGE ( 'NONE', *, *, #46861, .F. ) ;
#55471=CARTESIAN_POINT ( 'NONE',  ( -18.00000000000000000, -9.905515769479279697, 34.41647553114623292 ) ) ;
#55473=CARTESIAN_POINT ( 'NONE',  ( -11.78848477575450282, -6.695914987888146541, 34.68535235679833306 ) ) ;
#55474=AXIS2_PLACEMENT_3D ( 'NONE', #32866, #13038, #11261 ) ;
#55475=EDGE_CURVE ( 'NONE', #79227, #61132, #29168, .T. ) ;
#55476=CARTESIAN_POINT ( 'NONE',  ( 8.769230769230768274, -1.129524287112498415, 32.06866353760679544 ) ) ;
#55478=EDGE_CURVE ( 'NONE', #65424, #34542, #81811, .T. ) ;
#55479=VERTEX_POINT ( 'NONE', #18257 ) ;
#55480=EDGE_CURVE ( 'NONE', #6648, #4047, #88204, .T. ) ;
#55481=FACE_BOUND ( 'NONE', #55830, .T. ) ;
#55482=VERTEX_POINT ( 'NONE', #85831 ) ;
#55483=CARTESIAN_POINT ( 'NONE',  ( -8.899378738962468560, -12.50552854090298993, 31.33409797877408920 ) ) ;
#55484=CARTESIAN_POINT ( 'NONE',  ( -14.30769230769230660, -11.35647404775217417, 33.31231777344666511 ) ) ;
#55485=FACE_OUTER_BOUND ( 'NONE', #66707, .T. ) ;
#55486=CARTESIAN_POINT ( 'NONE',  ( -11.40766973063675493, -2.541949514083464479, 30.39797389878540557 ) ) ;
#55487=ADVANCED_FACE ( 'NONE', ( #44821 ), #11054, .F. ) ;
#55488=ORIENTED_EDGE ( 'NONE', *, *, #35617, .T. ) ;
#55489=EDGE_LOOP ( 'NONE', ( #73653, #38545, #15697, #9881 ) ) ;
#55490=ORIENTED_EDGE ( 'NONE', *, *, #71289, .T. ) ;
#55491=CARTESIAN_POINT ( 'NONE',  ( -3.230769230769229949, -11.35647404775217417, 33.31231777344666511 ) ) ;
#55493=EDGE_CURVE ( 'NONE', #34480, #84245, #21666, .T. ) ;
#55495=CARTESIAN_POINT ( 'NONE',  ( 15.00784227186237807, -3.395401636524185474, 33.02366814457250399 ) ) ;
#55496=CARTESIAN_POINT ( 'NONE',  ( -11.60454391782167249, -5.471508081941602875, 34.59228464037088457 ) ) ;
#55498=B_SPLINE_CURVE_WITH_KNOTS ( 'NONE', 3,
 ( #69488, #7793, #28966, #56853, #48768, #77579, #70383, #56422, #14997, #42471 ),
 .UNSPECIFIED., .F., .F.,
 ( 4, 2, 2, 2, 4 ),
 ( 0.000000000000000000, 0.0001954339857564096699, 0.0003908679715128193398, 0.0005863019572692289554, 0.0007817359430256386795 ),
 .UNSPECIFIED. ) ;
#55499=DIRECTION ( 'NONE',  ( 0.000000000000000000, -6.938893903907222067E-15, 1.000000000000000000 ) ) ;
#55500=DIRECTION ( 'NONE',  ( -0.000000000000000000, 0.5000000000000011102, -0.8660254037844380415 ) ) ;
#55501=FACE_OUTER_BOUND ( 'NONE', #55799, .T. ) ;
#55502=DIRECTION ( 'NONE',  ( -0.000000000000000000, -0.000000000000000000, -1.000000000000000000 ) ) ;
#55503=CARTESIAN_POINT ( 'NONE',  ( 7.846153846153846700, -4.661471528628507777, 34.16647553114623292 ) ) ;
#55504=ORIENTED_EDGE ( 'NONE', *, *, #30433, .T. ) ;
#55505=AXIS2_PLACEMENT_3D ( 'NONE', #68256, #25935, #12425 ) ;
#55506=VERTEX_POINT ( 'NONE', #45269 ) ;
#55507=ORIENTED_EDGE ( 'NONE', *, *, #74903, .T. ) ;
#55509=DIRECTION ( 'NONE',  ( 0.000000000000000000, 1.000000000000000000, 0.000000000000000000 ) ) ;
#55510=CARTESIAN_POINT ( 'NONE',  ( 10.54930223602447725, -2.292212530054419606, 30.41441678777542634 ) ) ;
#55511=CARTESIAN_POINT ( 'NONE',  ( 11.28843831424008393, -2.341070481393819236, 30.72580821765574299 ) ) ;
#55512=CARTESIAN_POINT ( 'NONE',  ( -3.230769230769229949, -11.16473453929635440, 33.15142922261926373 ) ) ;
#55513=FACE_BOUND ( 'NONE', #41469, .T. ) ;
#55514=CYLINDRICAL_SURFACE ( 'NONE', #40356, 0.2499999999999986955 ) ;
#55515=EDGE_LOOP ( 'NONE', ( #67913, #59142, #35087, #4415 ) ) ;
#55516=CARTESIAN_POINT ( 'NONE',  ( -6.000000000000119904, -10.21337939537710326, 33.94971097300076224 ) ) ;
#55517=LINE ( 'NONE', #28498, #80480 ) ;
#55518=CARTESIAN_POINT ( 'NONE',  ( -1.319359813339360477, -2.892918686051626498, 31.69288490824025928 ) ) ;
#55519=CARTESIAN_POINT ( 'NONE',  ( 6.923076923076800782, -9.528491918059723176, 34.59228464037033035 ) ) ;
#55520=ORIENTED_EDGE ( 'NONE', *, *, #1894, .F. ) ;
#55521=CARTESIAN_POINT ( 'NONE',  ( 18.06525557127602610, -12.46129190930001052, 30.37095296980869819 ) ) ;
#55522=EDGE_LOOP ( 'NONE', ( #63125, #72388 ) ) ;
#55523=FACE_BOUND ( 'NONE', #2977, .T. ) ;
#55524=EDGE_CURVE ( 'NONE', #65891, #34882, #69987, .T. ) ;
#55526=VECTOR ( 'NONE', #76384, 1000.000000000000114 ) ;
#55527=CARTESIAN_POINT ( 'NONE',  ( -7.911403777927930925, -2.255955759149247619, 30.00000000000013856 ) ) ;
#55528=CARTESIAN_POINT ( 'NONE',  ( -12.71156168575991963, -12.07920672191015221, 32.31858351112116168 ) ) ;
#55529=ORIENTED_EDGE ( 'NONE', *, *, #63223, .F. ) ;
#55530=CARTESIAN_POINT ( 'NONE',  ( 11.66925197942848769, -10.70102852606553157, 33.91149625220312913 ) ) ;
#55531=CARTESIAN_POINT ( 'NONE',  ( -14.55766903863466055, -4.236021600441997492, 33.53823185664189310 ) ) ;
#55532=CARTESIAN_POINT ( 'NONE',  ( 18.22277966897806678, -10.97394488606063589, 33.68653795673696294 ) ) ;
#55533=CARTESIAN_POINT ( 'NONE',  ( -4.826868657009623753, -5.642605341092957083, 34.66089969410670335 ) ) ;
#55535=VECTOR ( 'NONE', #2168, 1000.000000000000114 ) ;
#55536=CARTESIAN_POINT ( 'NONE',  ( -12.23852710992561299, -3.105924265160262543, 32.13625925475356127 ) ) ;
#55537=ORIENTED_EDGE ( 'NONE', *, *, #60698, .F. ) ;
#55538=EDGE_CURVE ( 'NONE', #54237, #62563, #25455, .T. ) ;
#55539=CARTESIAN_POINT ( 'NONE',  ( 4.403791563224197070, -2.986452184633681117, 32.43230066228895225 ) ) ;
#55540=ORIENTED_EDGE ( 'NONE', *, *, #48257, .F. ) ;
#55541=CARTESIAN_POINT ( 'NONE',  ( 3.296024802045255164, -2.625532179533470512, 30.86335684631491105 ) ) ;
#55542=CARTESIAN_POINT ( 'NONE',  ( -4.219929564802033184, -2.721908614388772740, 31.22303859784724622 ) ) ;
#55543=CARTESIAN_POINT ( 'NONE',  ( 7.846153846153846700, -9.905515769479276145, 34.41647553114623292 ) ) ;
#55544=CARTESIAN_POINT ( 'NONE',  ( 14.05766907039934210, -9.271318131107980420, 34.42618302367067429 ) ) ;
#55546=CARTESIAN_POINT ( 'NONE',  ( 13.44987095589141290, -6.026961402152789304, 34.52809138561124769 ) ) ;
#55548=CARTESIAN_POINT ( 'NONE',  ( 14.30769230769218758, -3.835265460704628371, 33.15142922262033665 ) ) ;
#55550=ORIENTED_EDGE ( 'NONE', *, *, #78384, .T. ) ;
#55551=FACE_OUTER_BOUND ( 'NONE', #78300, .T. ) ;
#55552=ORIENTED_EDGE ( 'NONE', *, *, #8916, .F. ) ;
#55553=ORIENTED_EDGE ( 'NONE', *, *, #36621, .F. ) ;
#55555=ORIENTED_EDGE ( 'NONE', *, *, #84912, .F. ) ;
#55557=CARTESIAN_POINT ( 'NONE',  ( -11.40793610022789650, -10.31582465632705237, 34.18122507451815295 ) ) ;
#55558=CARTESIAN_POINT ( 'NONE',  ( 3.165498784808455923, -8.613356846314824011, 34.62446782046655613 ) ) ;
#55559=CARTESIAN_POINT ( 'NONE',  ( -0.4615384615384611200, -8.120952969808772792, 34.71129190930000163 ) ) ;
#55560=CARTESIAN_POINT ( 'NONE',  ( 6.249945518348143381, -2.587454068350147462, 30.68340429815432202 ) ) ;
#55561=CARTESIAN_POINT ( 'NONE',  ( -16.37677237136229991, -3.105860786376062332, 32.13614157043599562 ) ) ;
#55562=ADVANCED_FACE ( 'NONE', ( #18710 ), #26343, .F. ) ;
#55563=CARTESIAN_POINT ( 'NONE',  ( 16.02315468717859659, -11.71456829005830080, 32.44064028649416542 ) ) ;
#55564=CARTESIAN_POINT ( 'NONE',  ( -5.999999999999998224, -1.422936976036506707, 30.56769352161908415 ) ) ;
#55565=AXIS2_PLACEMENT_3D ( 'NONE', #74508, #20001, #47465 ) ;
#55566=DIRECTION ( 'NONE',  ( -0.000000000000000000, 0.9848077530122086864, -0.1736481776669273891 ) ) ;
#55567=CARTESIAN_POINT ( 'NONE',  ( 11.31497659473759043, -10.81261337010820256, 33.49550067578627477 ) ) ;
#55568=CARTESIAN_POINT ( 'NONE',  ( 5.999999999999878320, -11.67786785259630911, 32.92929555188603530 ) ) ;
#55569=CARTESIAN_POINT ( 'NONE',  ( -13.60810030917971680, -10.23692288466677880, 34.23039457007281072 ) ) ;
#55570=ORIENTED_EDGE ( 'NONE', *, *, #33829, .T. ) ;
#55572=DIRECTION ( 'NONE',  ( 0.000000000000000000, 0.9848077530122072432, -0.1736481776669354937 ) ) ;
#55573=CARTESIAN_POINT ( 'NONE',  ( 1.607628228708782414, -3.395485233115138168, 33.02377354290276656 ) ) ;
#55575=CARTESIAN_POINT ( 'NONE',  ( 9.692307692307695177, -10.05456864172156806, 36.03766855953608683 ) ) ;
#55576=EDGE_CURVE ( 'NONE', #17484, #68101, #59131, .T. ) ;
#55577=VECTOR ( 'NONE', #36840, 1000.000000000000000 ) ;
#55578=EDGE_CURVE ( 'NONE', #31488, #5024, #39869, .T. ) ;
#55579=DIRECTION ( 'NONE',  ( -0.000000000000000000, -0.7660444431189791237, -0.6427876096865379196 ) ) ;
#55580=DIRECTION ( 'NONE',  ( -0.000000000000000000, -0.1736481776669307198, -0.9848077530122080203 ) ) ;
#55581=B_SPLINE_CURVE_WITH_KNOTS ( 'NONE', 3,
 ( #60641, #44901, #24641, #72376, #10689, #52106, #280, #26868, #41272, #82262 ),
 .UNSPECIFIED., .F., .F.,
 ( 4, 2, 2, 2, 4 ),
 ( 0.0007817246256747446788, 0.0009771112852218879000, 0.001172497944769031013, 0.001367884604316174126, 0.001563271263863317238 ),
 .UNSPECIFIED. ) ;
#55582=B_SPLINE_CURVE_WITH_KNOTS ( 'NONE', 3,
 ( #39334, #47393, #82086, #106, #19485, #551, #13177, #27574, #26246, #34769 ),
 .UNSPECIFIED., .F., .F.,
 ( 4, 2, 2, 2, 4 ),
 ( 0.000000000000000000, 0.0001954339857564097512, 0.0003908679715128195024, 0.0005863019572692292807, 0.0007817359430256390048 ),
 .UNSPECIFIED. ) ;
#55583=CARTESIAN_POINT ( 'NONE',  ( -2.373774687052440768, -8.164416787775445883, 34.95778746994557906 ) ) ;
#55584=EDGE_CURVE ( 'NONE', #1538, #34578, #82183, .T. ) ;
#55585=VERTEX_POINT ( 'NONE', #33551 ) ;
#55586=DIRECTION ( 'NONE',  ( -1.000000000000000000, 0.000000000000000000, 0.000000000000000000 ) ) ;
#55587=ORIENTED_EDGE ( 'NONE', *, *, #10156, .F. ) ;
#55589=CARTESIAN_POINT ( 'NONE',  ( 10.61538461538461675, -9.584722331328613620, 36.20867863119891439 ) ) ;
#55590=AXIS2_PLACEMENT_3D ( 'NONE', #86394, #64307, #2171 ) ;
#55591=CARTESIAN_POINT ( 'NONE',  ( 12.46153846153846168, -8.120952969808772792, 34.71129190930000163 ) ) ;
#55592=DIRECTION ( 'NONE',  ( 0.000000000000000000, 0.3420201433256641055, -0.9396926207859100932 ) ) ;
#55593=CARTESIAN_POINT ( 'NONE',  ( -3.296092146261405897, -7.749976743299137993, 34.99404534957040624 ) ) ;
#55594=CIRCLE ( 'NONE', #6672, 2.000000000000001776 ) ;
#55595=ORIENTED_EDGE ( 'NONE', *, *, #68089, .F. ) ;
#55596=ORIENTED_EDGE ( 'NONE', *, *, #35542, .T. ) ;
#55599=VERTEX_POINT ( 'NONE', #67337 ) ;
#55600=AXIS2_PLACEMENT_3D ( 'NONE', #41821, #82810, #82366 ) ;
#55601=CARTESIAN_POINT ( 'NONE',  ( -6.250023237292964495, -11.37209801155882971, 32.91403422569032955 ) ) ;
#55602=CARTESIAN_POINT ( 'NONE',  ( 8.769230769230645706, -11.06231777344772027, 33.60647404775119895 ) ) ;
#55603=CARTESIAN_POINT ( 'NONE',  ( 4.284636594813102661, -11.93129842949671726, 32.56571108434900452 ) ) ;
#55604=CARTESIAN_POINT ( 'NONE',  ( 14.30769230769218758, -2.625532179533778709, 30.86335684631627174 ) ) ;
#55605=CARTESIAN_POINT ( 'NONE',  ( -7.780086512803769949, -3.937682226553329556, 33.60647404775216529 ) ) ;
#55606=CARTESIAN_POINT ( 'NONE',  ( 14.30769230769231015, -9.780366693483667717, 34.19971097300155094 ) ) ;
#55607=EDGE_LOOP ( 'NONE', ( #35090, #53733, #76828, #28945 ) ) ;
#55608=ORIENTED_EDGE ( 'NONE', *, *, #40521, .T. ) ;
#55609=ORIENTED_EDGE ( 'NONE', *, *, #26580, .T. ) ;
#55610=FACE_OUTER_BOUND ( 'NONE', #72696, .T. ) ;
#55611=ORIENTED_EDGE ( 'NONE', *, *, #21670, .F. ) ;
#55613=CARTESIAN_POINT ( 'NONE',  ( -5.011667505647053211, -11.48612834413965977, 32.76840700105972815 ) ) ;
#55615=ORIENTED_EDGE ( 'NONE', *, *, #85294, .F. ) ;
#55617=FACE_OUTER_BOUND ( 'NONE', #84666, .T. ) ;
#55618=AXIS2_PLACEMENT_3D ( 'NONE', #69543, #55580, #61447 ) ;
#55619=ORIENTED_EDGE ( 'NONE', *, *, #75028, .T. ) ;
#55620=FACE_BOUND ( 'NONE', #46873, .T. ) ;
#55621=DIRECTION ( 'NONE',  ( -0.000000000000000000, 0.1736481776669307198, -0.9848077530122080203 ) ) ;
#55622=CARTESIAN_POINT ( 'NONE',  ( -8.769230769230768274, -3.513871655860378418, 32.76840700105978499 ) ) ;
#55623=VERTEX_POINT ( 'NONE', #20473 ) ;
#55624=CARTESIAN_POINT ( 'NONE',  ( -6.923076923076922462, -4.786620604624113540, 33.94971097300155094 ) ) ;
#55625=CARTESIAN_POINT ( 'NONE',  ( -15.90390074446811042, -12.68172785388650681, 30.59649109432439573 ) ) ;
#55628=CARTESIAN_POINT ( 'NONE',  ( -3.360917200500926239, -9.504002272028875709, 34.60269587691767867 ) ) ;
#55630=CARTESIAN_POINT ( 'NONE',  ( -12.23875879256039489, -2.353885683473779800, 30.79025554430704403 ) ) ;
#55631=CARTESIAN_POINT ( 'NONE',  ( -5.869474561766354626, -4.299079248970732792, 33.91157788607253565 ) ) ;
#55633=CARTESIAN_POINT ( 'NONE',  ( 22.75000000000000000, -4.499999999999999112, 29.75000000000000355 ) ) ;
#55634=DIRECTION ( 'NONE',  ( -0.000000000000000000, -0.1736481776669307198, -0.9848077530122080203 ) ) ;
#55635=FACE_BOUND ( 'NONE', #45669, .T. ) ;
#55636=CARTESIAN_POINT ( 'NONE',  ( -8.769230769230460965, -2.506253911140614576, 30.00000000000323297 ) ) ;
#55637=CARTESIAN_POINT ( 'NONE',  ( -7.846153846153844924, -7.500000000000001776, 35.04278698407183867 ) ) ;
#55638=B_SPLINE_CURVE_WITH_KNOTS ( 'NONE', 3,
 ( #63748, #2482, #44348, #42606, #43041, #6702, #34174, #70514, #56110, #21882 ),
 .UNSPECIFIED., .F., .F.,
 ( 4, 2, 2, 2, 4 ),
 ( 0.0007817246256747484735, 0.0009771112852218920199, 0.001172497944769035783, 0.001367884604316179330, 0.001563271263863322876 ),
 .UNSPECIFIED. ) ;
#55639=DIRECTION ( 'NONE',  ( -0.000000000000000000, -0.6427876096865404731, -0.7660444431189771253 ) ) ;
#55641=CARTESIAN_POINT ( 'NONE',  ( 5.869852790561781219, -10.88202310037935661, 33.43294751532457099 ) ) ;
#55642=CARTESIAN_POINT ( 'NONE',  ( -7.912236225513978205, -3.937682226553330445, 33.60647404775217240 ) ) ;
#55644=B_SPLINE_CURVE_WITH_KNOTS ( 'NONE', 3,
 ( #14036, #75732, #48702, #76177, #6407, #26665, #88392, #5960, #61766, #40197 ),
 .UNSPECIFIED., .F., .F.,
 ( 4, 2, 2, 2, 4 ),
 ( 0.0007817246256747521597, 0.0009771112852218961399, 0.001172497944769040337, 0.001367884604316184534, 0.001563271263863328514 ),
 .UNSPECIFIED. ) ;
#55645=ORIENTED_EDGE ( 'NONE', *, *, #49835, .F. ) ;
#55646=CARTESIAN_POINT ( 'NONE',  ( -6.923076923076922462, -2.900454961884010974, 35.62045528018868623 ) ) ;
#55648=LINE ( 'NONE', #68730, #56458 ) ;
#55649=AXIS2_PLACEMENT_3D ( 'NONE', #15994, #29076, #69599 ) ;
#55650=ORIENTED_EDGE ( 'NONE', *, *, #42973, .T. ) ;
#55651=CARTESIAN_POINT ( 'NONE',  ( -18.00000000000000000, -2.499999999999999556, 29.74999999999998579 ) ) ;
#55652=CARTESIAN_POINT ( 'NONE',  ( -15.90390074446811042, -12.07971442181321997, 32.31769673815850297 ) ) ;
#55656=CARTESIAN_POINT ( 'NONE',  ( -4.088653165551497715, -2.255955759149235629, 29.99999999999988631 ) ) ;
#55657=CARTESIAN_POINT ( 'NONE',  ( -5.076923076923199218, -3.083524468854526912, 32.58852847137268327 ) ) ;
#55658=VECTOR ( 'NONE', #6385, 999.9999999999998863 ) ;
#55659=CARTESIAN_POINT ( 'NONE',  ( 12.39545505058258001, -2.721908614388770964, 31.22303859784723912 ) ) ;
#55661=CARTESIAN_POINT ( 'NONE',  ( 11.53846153846153832, -1.242168528481310874, 33.36296068462461051 ) ) ;
#55662=CARTESIAN_POINT ( 'NONE',  ( 11.78851585009985570, -3.627508038966690496, 32.91356715214248396 ) ) ;
#55664=CARTESIAN_POINT ( 'NONE',  ( -9.758391103263571509, -3.513871655860377086, 32.76840700105978499 ) ) ;
#55665=DIRECTION ( 'NONE',  ( -0.000000000000000000, 0.6427876096865404731, -0.7660444431189771253 ) ) ;
#55667=ORIENTED_EDGE ( 'NONE', *, *, #37207, .T. ) ;
#55670=ADVANCED_FACE ( 'NONE', ( #19583 ), #40754, .F. ) ;
#55671=CARTESIAN_POINT ( 'NONE',  ( -16.15384615384615330, -12.34228464037088635, 31.77849191805839268 ) ) ;
#55672=DIRECTION ( 'NONE',  ( -0.000000000000000000, -0.7660444431189791237, -0.6427876096865379196 ) ) ;
#55673=ORIENTED_EDGE ( 'NONE', *, *, #74521, .T. ) ;
#55675=CARTESIAN_POINT ( 'NONE',  ( 3.230769230769110045, -3.835265460704628371, 33.15142922262033665 ) ) ;
#55676=CARTESIAN_POINT ( 'NONE',  ( 2.177000841024751221, -2.729777683071816785, 31.24903638046268739 ) ) ;
#55677=VERTEX_POINT ( 'NONE', #26785 ) ;
#55678=CARTESIAN_POINT ( 'NONE',  ( -5.076923076923197442, -6.026961402154118908, 34.52809138561165270 ) ) ;
#55680=CARTESIAN_POINT ( 'NONE',  ( -16.15384615384627409, -10.90142922262034020, 33.41473453929536674 ) ) ;
#55681=DIRECTION ( 'NONE',  ( 0.000000000000000000, 0.4999999999999985567, 0.8660254037844395958 ) ) ;
#55682=CARTESIAN_POINT ( 'NONE',  ( 2.307692307692186251, -4.320704448113951379, 33.92786785259630022 ) ) ;
#55683=CYLINDRICAL_SURFACE ( 'NONE', #19262, 0.2500000000000008882 ) ;
#55684=AXIS2_PLACEMENT_3D ( 'NONE', #14482, #46927, #53693 ) ;
#55687=CARTESIAN_POINT ( 'NONE',  ( 4.153846153846154188, -11.11383981884818262, 36.00935417666054406 ) ) ;
#55688=ORIENTED_EDGE ( 'NONE', *, *, #42574, .F. ) ;
#55689=ORIENTED_EDGE ( 'NONE', *, *, #34876, .F. ) ;
#55690=CARTESIAN_POINT ( 'NONE',  ( 5.076923076923075762, -5.415277668671390821, 36.20867863119892149 ) ) ;
#55692=VECTOR ( 'NONE', #42069, 1000.000000000000000 ) ;
#55693=CARTESIAN_POINT ( 'NONE',  ( -2.307692307692305711, -9.819645486525091727, 36.12317359536749706 ) ) ;
#55694=CARTESIAN_POINT ( 'NONE',  ( -17.01177829620344895, -7.750023224968867197, 34.99404313364389907 ) ) ;
#55695=ORIENTED_EDGE ( 'NONE', *, *, #80829, .T. ) ;
#55696=CARTESIAN_POINT ( 'NONE',  ( -18.25000000000000000, -7.433931650972299465, 34.75000000000000711 ) ) ;
#55697=ORIENTED_EDGE ( 'NONE', *, *, #57988, .T. ) ;
#55698=B_SPLINE_CURVE_WITH_KNOTS ( 'NONE', 3,
 ( #54077, #47776, #60396, #53191, #87456, #40588, #81132, #18978, #88789, #68486 ),
 .UNSPECIFIED., .F., .F.,
 ( 4, 2, 2, 2, 4 ),
 ( 0.000000000000000000, 0.0001954339881912775425, 0.0003908679763825550850, 0.0005863019645738326005, 0.0007817359527651101701 ),
 .UNSPECIFIED. ) ;
#55700=B_SPLINE_CURVE_WITH_KNOTS ( 'NONE', 3,
 ( #6198, #46735, #59802, #4872, #74211, #33670, #73778, #5309, #75529, #26911 ),
 .UNSPECIFIED., .F., .F.,
 ( 4, 2, 2, 2, 4 ),
 ( 0.000000000000000000, 0.1250000000000000000, 0.2500000000000000000, 0.3750000000000000000, 0.5000000000000000000 ),
 .UNSPECIFIED. ) ;
#55702=ORIENTED_EDGE ( 'NONE', *, *, #40247, .F. ) ;
#55703=CARTESIAN_POINT ( 'NONE',  ( 4.219101293358989757, -12.51329471203373700, 31.30864560766537963 ) ) ;
#55704=EDGE_CURVE ( 'NONE', #16132, #38188, #74982, .T. ) ;
#55706=CARTESIAN_POINT ( 'NONE',  ( -0.5268089074992365894, -5.219633306516282545, 34.19971097300152962 ) ) ;
#55707=EDGE_CURVE ( 'NONE', #19274, #16174, #61356, .T. ) ;
#55708=FACE_OUTER_BOUND ( 'NONE', #72032, .T. ) ;
#55709=EDGE_CURVE ( 'NONE', #49902, #83302, #33463, .T. ) ;
#55710=CARTESIAN_POINT ( 'NONE',  ( -2.980823712421088789, -4.336752205174647656, 33.62275283266504289 ) ) ;
#55711=CARTESIAN_POINT ( 'NONE',  ( 14.37385891428395013, -7.250054591869670162, 34.99404684341514127 ) ) ;
#55712=EDGE_LOOP ( 'NONE', ( #8872, #24610, #66725, #18114 ) ) ;
#55713=ORIENTED_EDGE ( 'NONE', *, *, #14158, .T. ) ;
#55714=ORIENTED_EDGE ( 'NONE', *, *, #88082, .F. ) ;
#55715=CARTESIAN_POINT ( 'NONE',  ( -6.673131513698878692, -2.986452184633680673, 32.43230066228895225 ) ) ;
#55716=CARTESIAN_POINT ( 'NONE',  ( 11.53846153846141576, -5.941354392335915335, 34.76329471203413846 ) ) ;
#55717=ORIENTED_EDGE ( 'NONE', *, *, #13585, .T. ) ;
#55718=B_SPLINE_CURVE_WITH_KNOTS ( 'NONE', 3,
 ( #61174, #12562, #6682, #33280, #40488, #47671, #60740, #26521, #380, #53984 ),
 .UNSPECIFIED., .F., .F.,
 ( 4, 2, 2, 2, 4 ),
 ( 0.0007817359430256294638, 0.0009771253907249948054, 0.001172514838424360255, 0.001367904286123725489, 0.001563293733823090939 ),
 .UNSPECIFIED. ) ;
#55719=CARTESIAN_POINT ( 'NONE',  ( 9.469381474791543241, -11.76352882383564769, 32.36236540154569497 ) ) ;
#55720=CARTESIAN_POINT ( 'NONE',  ( -17.14300545628320904, -3.322132147404559976, 32.92929555188719348 ) ) ;
#55721=ORIENTED_EDGE ( 'NONE', *, *, #9767, .T. ) ;
#55722=VECTOR ( 'NONE', #44688, 999.9999999999998863 ) ;
#55723=CYLINDRICAL_SURFACE ( 'NONE', #22088, 0.2499999999999986955 ) ;
#55724=FACE_OUTER_BOUND ( 'NONE', #63590, .T. ) ;
#55725=ORIENTED_EDGE ( 'NONE', *, *, #214, .T. ) ;
#55726=FACE_BOUND ( 'NONE', #85939, .T. ) ;
#55727=DIRECTION ( 'NONE',  ( -0.000000000000000000, -0.9848077530122086864, -0.1736481776669273613 ) ) ;
#55729=CYLINDRICAL_SURFACE ( 'NONE', #79694, 0.2499999999999995559 ) ;
#55730=CARTESIAN_POINT ( 'NONE',  ( -6.793029316821241004, -7.723484964179500700, 34.74522123443823318 ) ) ;
#55731=FACE_OUTER_BOUND ( 'NONE', #78381, .T. ) ;
#55732=CARTESIAN_POINT ( 'NONE',  ( -3.007989561791163169, -3.563462043263030399, 33.22394488606062879 ) ) ;
#55733=CARTESIAN_POINT ( 'NONE',  ( -2.437839517130528488, -3.817052484675422797, 33.13202310037935661 ) ) ;
#55734=ORIENTED_EDGE ( 'NONE', *, *, #32741, .F. ) ;
#55735=DIRECTION ( 'NONE',  ( -0.000000000000000000, -0.7660444431189791237, -0.6427876096865379196 ) ) ;
#55736=B_SPLINE_CURVE_WITH_KNOTS ( 'NONE', 3,
 ( #24790, #80191, #67123, #74321, #65766, #60351, #4523, #87862, #12621, #26576 ),
 .UNSPECIFIED., .F., .F.,
 ( 4, 2, 2, 2, 4 ),
 ( 0.000000000000000000, 0.0001954311564186861968, 0.0003908623128373723936, 0.0005862934692560585904, 0.0007817246256747447872 ),
 .UNSPECIFIED. ) ;
#55737=CARTESIAN_POINT ( 'NONE',  ( -8.096153846153846700, -2.499999999999999556, 29.81609845454691765 ) ) ;
#55738=ORIENTED_EDGE ( 'NONE', *, *, #28211, .T. ) ;
#55739=CARTESIAN_POINT ( 'NONE',  ( 14.08476609017615644, -9.886141570436013382, 34.14413921362392301 ) ) ;
#55741=ORIENTED_EDGE ( 'NONE', *, *, #66533, .T. ) ;
#55742=EDGE_CURVE ( 'NONE', #51126, #41438, #68655, .T. ) ;
#55743=VECTOR ( 'NONE', #33035, 1000.000000000000114 ) ;
#55744=CARTESIAN_POINT ( 'NONE',  ( 11.40831356872984514, -10.31621877034669588, 34.18098118002070152 ) ) ;
#55745=CARTESIAN_POINT ( 'NONE',  ( 2.307692307692309264, -4.661471528628507777, 34.16647553114623292 ) ) ;
#55746=FACE_BOUND ( 'NONE', #24981, .T. ) ;
#55747=CARTESIAN_POINT ( 'NONE',  ( -2.307692307692305711, -6.386643153685126251, 34.62446782046654192 ) ) ;
#55748=CARTESIAN_POINT ( 'NONE',  ( -17.07692307692319744, -12.46129190930018460, 30.37095296980731973 ) ) ;
#55749=CARTESIAN_POINT ( 'NONE',  ( -6.923076923077044142, -9.442884908241554243, 34.35708131394783038 ) ) ;
#55752=CARTESIAN_POINT ( 'NONE',  ( -12.46153846153846168, -4.098570777380720287, 33.41473453929634729 ) ) ;
#55753=CARTESIAN_POINT ( 'NONE',  ( 13.38461538461538680, -2.833524468853757305, 32.15551576947925838 ) ) ;
#55755=EDGE_LOOP ( 'NONE', ( #65776, #51966 ) ) ;
#55756=VERTEX_POINT ( 'NONE', #50142 ) ;
#55757=CARTESIAN_POINT ( 'NONE',  ( 5.076923076923075762, -2.538708090699994813, 30.37095296980875503 ) ) ;
#55758=VECTOR ( 'NONE', #43279, 1000.000000000000000 ) ;
#55759=CARTESIAN_POINT ( 'NONE',  ( 14.53070515178570332, -12.64618726649961289, 30.78989965857442712 ) ) ;
#55760=DIRECTION ( 'NONE',  ( 0.000000000000000000, 0.1736481776669267785, -0.9848077530122087975 ) ) ;
#55761=CARTESIAN_POINT ( 'NONE',  ( -1.449885830576160162, -3.300289026998414865, 32.46337939537583139 ) ) ;
#55762=CARTESIAN_POINT ( 'NONE',  ( -3.931066484868087851, -3.020022701398814124, 32.48759521482552515 ) ) ;
#55764=EDGE_CURVE ( 'NONE', #25331, #39262, #47331, .T. ) ;
#55765=CARTESIAN_POINT ( 'NONE',  ( 4.403846153846216360, -7.434744429011176159, 34.75000000000000711 ) ) ;
#55766=DIRECTION ( 'NONE',  ( -0.000000000000000000, 0.6427876096865404731, -0.7660444431189770143 ) ) ;
#55767=CARTESIAN_POINT ( 'NONE',  ( 9.442330948259105128, -10.82459398097509329, 33.81372124010185587 ) ) ;
#55768=DIRECTION ( 'NONE',  ( -0.000000000000000000, -0.9848077530122086864, -0.1736481776669273613 ) ) ;
#55769=CARTESIAN_POINT ( 'NONE',  ( 10.61538461538449418, -3.643525952248795718, 33.31231777344771672 ) ) ;
#55770=CARTESIAN_POINT ( 'NONE',  ( 18.13079180782478872, -9.804649428959608670, 34.18742332936588468 ) ) ;
#55771=CARTESIAN_POINT ( 'NONE',  ( 10.61538461538461675, -11.33034616979429110, 35.88435417666054406 ) ) ;
#55772=CARTESIAN_POINT ( 'NONE',  ( -14.08468095607945969, -3.105924265160262543, 32.13625925475356127 ) ) ;
#55774=EDGE_LOOP ( 'NONE', ( #29834, #72688, #45035, #38392 ) ) ;
#55775=CARTESIAN_POINT ( 'NONE',  ( 3.903822916553188804, -5.056417327199098644, 34.11270091957320716 ) ) ;
#55776=CARTESIAN_POINT ( 'NONE',  ( 7.846153846153723244, -5.094484230521993062, 34.41647553114689373 ) ) ;
#55778=EDGE_CURVE ( 'NONE', #5919, #25778, #10815, .T. ) ;
#55779=B_SPLINE_CURVE_WITH_KNOTS ( 'NONE', 3,
 ( #18338, #59765, #25979, #33183, #81825, #81383, #52993, #53443, #47129, #45802 ),
 .UNSPECIFIED., .F., .F.,
 ( 4, 2, 2, 2, 4 ),
 ( 0.0007817246256747460882, 0.0009771112852218900684, 0.001172497944769033832, 0.001367884604316177595, 0.001563271263863321575 ),
 .UNSPECIFIED. ) ;
#55780=CARTESIAN_POINT ( 'NONE',  ( -5.776987155906605942, -12.38742843783360748, 31.66772728687926985 ) ) ;
#55783=CARTESIAN_POINT ( 'NONE',  ( -12.46153846153846168, -2.538708090699994813, 30.37095296980875503 ) ) ;
#55784=CARTESIAN_POINT ( 'NONE',  ( -6.249999999999997335, -7.500000000000001776, 35.00000000000000000 ) ) ;
#55786=CARTESIAN_POINT ( 'NONE',  ( 9.627056702146452594, -2.506253911140460922, 30.00000000000013856 ) ) ;
#55787=CARTESIAN_POINT ( 'NONE',  ( 9.692307692307695177, -2.486705287966279876, 31.30864560766543647 ) ) ;
#55788=B_SPLINE_CURVE_WITH_KNOTS ( 'NONE', 3,
 ( #27004, #54463, #81960, #45929, #87390, #25670, #53127, #80634, #29229, #83280 ),
 .UNSPECIFIED., .F., .F.,
 ( 4, 2, 2, 2, 4 ),
 ( 0.000000000000000000, 0.0001954311564186868744, 0.0003908623128373737488, 0.0005862934692560606504, 0.0007817246256747474977 ),
 .UNSPECIFIED. ) ;
#55790=ORIENTED_EDGE ( 'NONE', *, *, #13042, .F. ) ;
#55791=CARTESIAN_POINT ( 'NONE',  ( -13.13466986626724164, -2.587454068350147018, 30.68340429815432202 ) ) ;
#55792=VECTOR ( 'NONE', #73738, 1000.000000000000227 ) ;
#55795=CARTESIAN_POINT ( 'NONE',  ( 17.01083966596719677, -11.16473453929635440, 33.15142922261925662 ) ) ;
#55796=CARTESIAN_POINT ( 'NONE',  ( 2.373759641042384683, -8.164416787775445883, 34.95778746994558617 ) ) ;
#55797=CARTESIAN_POINT ( 'NONE',  ( 9.915087361285756629, -6.717445702608402236, 34.94155399931962336 ) ) ;
#55798=EDGE_CURVE ( 'NONE', #15172, #73147, #28112, .T. ) ;
#55799=EDGE_LOOP ( 'NONE', ( #43289, #68768, #64757, #85674 ) ) ;
#55800=VERTEX_POINT ( 'NONE', #62768 ) ;
#55801=CARTESIAN_POINT ( 'NONE',  ( 3.165499230212911908, -3.083524468853724443, 32.58852847137143272 ) ) ;
#55803=EDGE_CURVE ( 'NONE', #8424, #27342, #56024, .T. ) ;
#55804=CARTESIAN_POINT ( 'NONE',  ( 3.230769230769108269, -12.16647553114689728, 32.15551576947799362 ) ) ;
#55805=CARTESIAN_POINT ( 'NONE',  ( 15.23076923076910916, -12.70778746994576025, 30.41441678777401236 ) ) ;
#55806=CARTESIAN_POINT ( 'NONE',  ( -14.53061852520844965, -3.105860786376062332, 32.13614157043599562 ) ) ;
#55809=CARTESIAN_POINT ( 'NONE',  ( 15.16549878480846125, -6.879047030191174805, 34.71129190930000163 ) ) ;
#55810=CARTESIAN_POINT ( 'NONE',  ( 0.5277050681301012069, -7.250054591869666609, 34.99404684341514127 ) ) ;
#55811=DIRECTION ( 'NONE',  ( -0.000000000000000000, 0.9848077530122086864, -0.1736481776669273891 ) ) ;
#55812=CIRCLE ( 'NONE', #42844, 2.999999999999999112 ) ;
#55813=ADVANCED_FACE ( 'NONE', ( #21799 ), #76749, .F. ) ;
#55814=ORIENTED_EDGE ( 'NONE', *, *, #64896, .F. ) ;
#55815=EDGE_LOOP ( 'NONE', ( #56173, #69078, #5112, #48861, #2011, #43879 ) ) ;
#55816=DIRECTION ( 'NONE',  ( 0.000000000000000000, -0.000000000000000000, -1.000000000000000000 ) ) ;
#55817=ORIENTED_EDGE ( 'NONE', *, *, #70968, .F. ) ;
#55818=VECTOR ( 'NONE', #51608, 1000.000000000000227 ) ;
#55819=LINE ( 'NONE', #6748, #37886 ) ;
#55820=ORIENTED_EDGE ( 'NONE', *, *, #38423, .T. ) ;
#55821=EDGE_CURVE ( 'NONE', #26289, #5224, #36214, .T. ) ;
#55823=VECTOR ( 'NONE', #78506, 1000.000000000000000 ) ;
#55824=CARTESIAN_POINT ( 'NONE',  ( 15.45414471654164856, -2.251407671071270489, 29.88021292934942963 ) ) ;
#55825=CARTESIAN_POINT ( 'NONE',  ( -8.069638770718176701, -10.23692288466677880, 34.23039457007281072 ) ) ;
#55826=ORIENTED_EDGE ( 'NONE', *, *, #21906, .T. ) ;
#55827=LINE ( 'NONE', #7651, #6835 ) ;
#55828=ORIENTED_EDGE ( 'NONE', *, *, #37875, .T. ) ;
#55829=CARTESIAN_POINT ( 'NONE',  ( -4.403869391139119571, -5.851115903089112003, 34.47074536777953568 ) ) ;
#55830=EDGE_LOOP ( 'NONE', ( #20154, #30213 ) ) ;
#55831=CYLINDRICAL_SURFACE ( 'NONE', #15815, 0.2499999999999995559 ) ;
#55832=ORIENTED_EDGE ( 'NONE', *, *, #2096, .T. ) ;
#55833=CARTESIAN_POINT ( 'NONE',  ( 0.4615384615384611200, -5.557115091759785130, 34.35708131394839171 ) ) ;
#55834=CARTESIAN_POINT ( 'NONE',  ( -4.219116154402471786, -6.835583212224499938, 34.95778746994557906 ) ) ;
#55835=FACE_BOUND ( 'NONE', #40384, .T. ) ;
#55836=CARTESIAN_POINT ( 'NONE',  ( 5.933917620639864943, -2.292212530054419606, 30.41441678777542634 ) ) ;
#55837=CYLINDRICAL_SURFACE ( 'NONE', #16923, 0.2499999999999994726 ) ;
#55838=CARTESIAN_POINT ( 'NONE',  ( 9.692307692307570832, -11.67786785259630911, 32.92929555188603530 ) ) ;
#55839=CARTESIAN_POINT ( 'NONE',  ( 12.46153846153846168, -3.322132147404559976, 32.92929555188717927 ) ) ;
#55840=CIRCLE ( 'NONE', #22722, 0.2500000000000002220 ) ;
#55841=ADVANCED_FACE ( 'NONE', ( #31661 ), #17250, .F. ) ;
#55843=CARTESIAN_POINT ( 'NONE',  ( -16.37677311275300340, -2.523278758544490685, 31.42238647778638239 ) ) ;
#55844=ORIENTED_EDGE ( 'NONE', *, *, #81015, .T. ) ;
#55845=CARTESIAN_POINT ( 'NONE',  ( 14.53047197667037516, -6.717445702608402236, 34.94155399931962336 ) ) ;
#55846=ORIENTED_EDGE ( 'NONE', *, *, #28146, .T. ) ;
#55848=CARTESIAN_POINT ( 'NONE',  ( 7.596130608860880429, -6.695914987888143877, 34.68535235679833306 ) ) ;
#55850=DIRECTION ( 'NONE',  ( -0.000000000000000000, -0.3420201433256694346, -0.9396926207859080948 ) ) ;
#55851=CARTESIAN_POINT ( 'NONE',  ( -17.01085574357299990, -9.905515769479276145, 34.41647553114623292 ) ) ;
#55852=CARTESIAN_POINT ( 'NONE',  ( 14.30769230769218581, -5.941354392335915335, 34.76329471203413846 ) ) ;
#55853=CARTESIAN_POINT ( 'NONE',  ( 13.63456090296352841, -11.37275283266504111, 32.91324779482534524 ) ) ;
#55854=ORIENTED_EDGE ( 'NONE', *, *, #40277, .F. ) ;
#55855=EDGE_CURVE ( 'NONE', #13051, #83441, #119, .T. ) ;
#55856=CARTESIAN_POINT ( 'NONE',  ( 3.230769230769110045, -3.300289026999228881, 32.46337939537708905 ) ) ;
#55857=AXIS2_PLACEMENT_3D ( 'NONE', #51124, #11061, #17368 ) ;
#55859=CARTESIAN_POINT ( 'NONE',  ( -39.05038313613820122, -2.499999999999999556, 29.75000000000000355 ) ) ;
#55860=CARTESIAN_POINT ( 'NONE',  ( -8.769230769230768274, -2.708943851104267164, 35.45975837776705220 ) ) ;
#55861=CARTESIAN_POINT ( 'NONE',  ( 2.307692307692186251, -5.941354392335915335, 34.76329471203413846 ) ) ;
#55862=ORIENTED_EDGE ( 'NONE', *, *, #16793, .T. ) ;
#55863=EDGE_CURVE ( 'NONE', #31586, #17756, #44708, .T. ) ;
#55864=EDGE_LOOP ( 'NONE', ( #50928, #57160 ) ) ;
#55865=ORIENTED_EDGE ( 'NONE', *, *, #29446, .T. ) ;
#55866=EDGE_CURVE ( 'NONE', #3281, #18498, #48441, .T. ) ;
#55867=CARTESIAN_POINT ( 'NONE',  ( -0.4615384615384611200, -11.33034616979429110, 35.88435417666054406 ) ) ;
#55869=LINE ( 'NONE', #83356, #64205 ) ;
#55870=CARTESIAN_POINT ( 'NONE',  ( 15.48071464014727106, -4.176053281294518804, 33.81426240980091791 ) ) ;
#55871=CYLINDRICAL_SURFACE ( 'NONE', #79729, 0.2499999999999986955 ) ;
#55873=EDGE_CURVE ( 'NONE', #42788, #81338, #7630, .T. ) ;
#55874=CARTESIAN_POINT ( 'NONE',  ( 12.33084699487090319, -9.804603061927743113, 34.18744698557895845 ) ) ;
#55876=CARTESIAN_POINT ( 'NONE',  ( -6.000000000000119904, -3.835265460704628371, 33.15142922262033665 ) ) ;
#55877=DIRECTION ( 'NONE',  ( -0.000000000000000000, 1.000000000000000000, -0.000000000000000000 ) ) ;
#55878=ORIENTED_EDGE ( 'NONE', *, *, #76712, .T. ) ;
#55880=CARTESIAN_POINT ( 'NONE',  ( 3.100622021331011169, -12.45813303252208648, 30.39737893381572675 ) ) ;
#55881=DIRECTION ( 'NONE',  ( -0.000000000000000000, 1.000000000000000000, 3.491481338843133355E-15 ) ) ;
#55882=CARTESIAN_POINT ( 'NONE',  ( 15.23076923076910916, -3.083524468854526912, 32.58852847137268327 ) ) ;
#55883=CARTESIAN_POINT ( 'NONE',  ( -17.77698715590660328, -10.77377354290276301, 33.85451476688484718 ) ) ;
#55884=CARTESIAN_POINT ( 'NONE',  ( 9.626224281351811740, -9.780366693483667717, 34.19971097300155805 ) ) ;
#55885=CARTESIAN_POINT ( 'NONE',  ( 6.923076923076924238, -9.819645486525091727, 36.12317359536749706 ) ) ;
#55887=ORIENTED_EDGE ( 'NONE', *, *, #28009, .F. ) ;
#55888=AXIS2_PLACEMENT_3D ( 'NONE', #35935, #76915, #49443 ) ;
#55889=CARTESIAN_POINT ( 'NONE',  ( -15.29685161012936412, -6.343179335718451384, 34.87096338111212646 ) ) ;
#55890=CARTESIAN_POINT ( 'NONE',  ( -1.254089946381738763, -3.625058011473228259, 33.29252011169590020 ) ) ;
#55891=CARTESIAN_POINT ( 'NONE',  ( 8.992010438208831502, -10.97394488606064122, 33.68653795673694873 ) ) ;
#55892=CARTESIAN_POINT ( 'NONE',  ( -3.164701897419154530, -10.67929555188718282, 33.92786785259544757 ) ) ;
#55893=ORIENTED_EDGE ( 'NONE', *, *, #37251, .F. ) ;
#55894=CARTESIAN_POINT ( 'NONE',  ( 0.3954560821783256741, -3.937682226553328668, 33.60647404775217950 ) ) ;
#55895=CARTESIAN_POINT ( 'NONE',  ( -2.530618525208454983, -3.105860786376062332, 32.13614157043598851 ) ) ;
#55897=CARTESIAN_POINT ( 'NONE',  ( 1.384615384615386802, -8.973038597847269315, 34.52809138561121927 ) ) ;
#55898=CARTESIAN_POINT ( 'NONE',  ( 14.05766907039934210, -3.202444869320336451, 32.30641848906366675 ) ) ;
#55899=ORIENTED_EDGE ( 'NONE', *, *, #15177, .F. ) ;
#55900=CARTESIAN_POINT ( 'NONE',  ( -12.46153846153858247, -9.442884908241554243, 34.35708131394783038 ) ) ;
#55901=CARTESIAN_POINT ( 'NONE',  ( -0.5276208408985970655, -9.905515769479276145, 34.41647553114623292 ) ) ;
#55902=CARTESIAN_POINT ( 'NONE',  ( 5.076923076923075762, -12.34228464037088635, 31.77849191805839268 ) ) ;
#55903=ORIENTED_EDGE ( 'NONE', *, *, #37660, .F. ) ;
#55904=CARTESIAN_POINT ( 'NONE',  ( -13.16160254052199008, -2.889357225399414197, 32.26129605718031002 ) ) ;
#55905=EDGE_LOOP ( 'NONE', ( #40715, #80524, #78411, #59820 ) ) ;
#55906=AXIS2_PLACEMENT_3D ( 'NONE', #86132, #73508, #32959 ) ;
#55908=CARTESIAN_POINT ( 'NONE',  ( 0.4615384615384611755, -13.88283147151868846, 33.14645433367849847 ) ) ;
#55909=ORIENTED_EDGE ( 'NONE', *, *, #52490, .T. ) ;
#55910=CARTESIAN_POINT ( 'NONE',  ( 10.68063975489745410, -11.67786785259547777, 32.92929555188713664 ) ) ;
#55911=CARTESIAN_POINT ( 'NONE',  ( 4.403900573759605308, -9.233818618650603938, 34.70587769442853698 ) ) ;
#55912=B_SPLINE_CURVE_WITH_KNOTS ( 'NONE', 3,
 ( #79988, #72773, #66015, #85415, #38561, #4324, #23696, #3429, #46204, #4779 ),
 .UNSPECIFIED., .F., .F.,
 ( 4, 2, 2, 2, 4 ),
 ( 0.0007817359430256320659, 0.0009771253907249987086, 0.001172514838424365460, 0.001367904286123731994, 0.001563293733823098745 ),
 .UNSPECIFIED. ) ;
#55913=CARTESIAN_POINT ( 'NONE',  ( 0.4615384615384611200, -4.098570777380720287, 33.41473453929634729 ) ) ;
#55915=FACE_OUTER_BOUND ( 'NONE', #8047, .T. ) ;
#55918=EDGE_CURVE ( 'NONE', #30358, #87048, #83760, .T. ) ;
#55919=ORIENTED_EDGE ( 'NONE', *, *, #9216, .T. ) ;
#55920=VERTEX_POINT ( 'NONE', #9608 ) ;
#55921=FACE_BOUND ( 'NONE', #11971, .T. ) ;
#55922=ORIENTED_EDGE ( 'NONE', *, *, #43966, .T. ) ;
#55923=LINE ( 'NONE', #41985, #54438 ) ;
#55925=CARTESIAN_POINT ( 'NONE',  ( 4.376857505459002873, -11.76359900205217457, 32.36225158514719880 ) ) ;
#55926=EDGE_CURVE ( 'NONE', #65002, #82311, #38417, .T. ) ;
#55927=CARTESIAN_POINT ( 'NONE',  ( 6.130790440966954691, -2.845873456487966635, 32.17976146951972538 ) ) ;
#55928=CARTESIAN_POINT ( 'NONE',  ( 5.207448778686639912, -4.459921816937789885, 33.71989282347011851 ) ) ;
#55929=ORIENTED_EDGE ( 'NONE', *, *, #73902, .F. ) ;
#55930=EDGE_LOOP ( 'NONE', ( #73080, #64293, #55080, #21771 ) ) ;
#55931=EDGE_CURVE ( 'NONE', #22606, #40886, #51609, .T. ) ;
#55932=ORIENTED_EDGE ( 'NONE', *, *, #63943, .F. ) ;
#55933=CARTESIAN_POINT ( 'NONE',  ( 13.13461538461538680, -7.500000000000001776, 34.75000000000000000 ) ) ;
#55934=ORIENTED_EDGE ( 'NONE', *, *, #64510, .F. ) ;
#55935=CARTESIAN_POINT ( 'NONE',  ( 10.61538461538461675, -2.292212530054420494, 30.41441678777542634 ) ) ;
#55936=ADVANCED_FACE ( 'NONE', ( #52807 ), #39317, .F. ) ;
#55937=B_SPLINE_CURVE_WITH_KNOTS ( 'NONE', 3,
 ( #11412, #87095, #33018, #60037, #74446, #18622, #80330, #87544, #67693, #25819 ),
 .UNSPECIFIED., .F., .F.,
 ( 4, 2, 2, 2, 4 ),
 ( 0.0007817359430256294638, 0.0009771253907249952391, 0.001172514838424361123, 0.001367904286123727007, 0.001563293733823092890 ),
 .UNSPECIFIED. ) ;
#55938=CARTESIAN_POINT ( 'NONE',  ( 1.515407192440173745, -3.530189275343204702, 32.79018710029569661 ) ) ;
#55939=CARTESIAN_POINT ( 'NONE',  ( -17.32689982097166492, -2.920706130388546651, 32.31842814019191223 ) ) ;
#55940=CARTESIAN_POINT ( 'NONE',  ( 13.25392391794783187, -10.54014554554150607, 33.71984207302941883 ) ) ;
#55941=B_SPLINE_CURVE_WITH_KNOTS ( 'NONE', 3,
 ( #61968, #69616, #20106, #82258, #7486, #7923, #21433, #14234, #47568, #48008 ),
 .UNSPECIFIED., .F., .F.,
 ( 4, 2, 2, 2, 4 ),
 ( 0.000000000000000000, 0.0001954311564186866034, 0.0003908623128373732067, 0.0005862934692560597830, 0.0007817246256747464135 ),
 .UNSPECIFIED. ) ;
#55942=DIRECTION ( 'NONE',  ( 0.000000000000000000, 0.7660444431189822323, -0.6427876096865344779 ) ) ;
#55943=EDGE_CURVE ( 'NONE', #4654, #75693, #11386, .T. ) ;
#55944=CARTESIAN_POINT ( 'NONE',  ( 5.076923076923075762, -10.51840700105979565, 33.73612834413961536 ) ) ;
#55945=CARTESIAN_POINT ( 'NONE',  ( 9.019285189144222059, -6.523592122091592671, 34.90882529074906415 ) ) ;
#55947=B_SPLINE_CURVE_WITH_KNOTS ( 'NONE', 3,
 ( #67421, #59323, #44912, #86832, #25097, #69967, #57337, #56457, #70421, #7831 ),
 .UNSPECIFIED., .F., .F.,
 ( 4, 2, 2, 2, 4 ),
 ( 0.0007817246256747476061, 0.0009771112852218902852, 0.001172497944769033181, 0.001367884604316175860, 0.001563271263863318539 ),
 .UNSPECIFIED. ) ;
#55948=ORIENTED_EDGE ( 'NONE', *, *, #31899, .F. ) ;
#55949=ORIENTED_EDGE ( 'NONE', *, *, #81536, .F. ) ;
#55950=DIRECTION ( 'NONE',  ( 0.000000000000000000, 0.9848077530122072432, -0.1736481776669354937 ) ) ;
#55951=CARTESIAN_POINT ( 'NONE',  ( -1.449885385171703733, -2.657715359629089225, 31.77849191805834295 ) ) ;
#55952=DIRECTION ( 'NONE',  ( -0.000000000000000000, -0.8660254037844397068, -0.4999999999999978906 ) ) ;
#55953=DIRECTION ( 'NONE',  ( 0.000000000000000000, 0.9396926207859126468, -0.3420201433256571111 ) ) ;
#55954=CARTESIAN_POINT ( 'NONE',  ( -8.769230769230892619, -6.835583212225970762, 34.95778746994575670 ) ) ;
#55955=FACE_BOUND ( 'NONE', #30898, .T. ) ;
#55956=CARTESIAN_POINT ( 'NONE',  ( 9.942362003946010773, -3.627508038966690496, 32.91356715214248396 ) ) ;
#55957=ORIENTED_EDGE ( 'NONE', *, *, #48973, .T. ) ;
#55958=CARTESIAN_POINT ( 'NONE',  ( -8.096153846153844924, -7.566082377512565849, 35.00000000000000711 ) ) ;
#55959=CARTESIAN_POINT ( 'NONE',  ( 9.468822767743365176, -12.11044203135681840, 32.26167407432752299 ) ) ;
#55961=CARTESIAN_POINT ( 'NONE',  ( 3.480823650682683734, -11.47946981652013498, 33.17500667209846910 ) ) ;
#55962=EDGE_LOOP ( 'NONE', ( #37405, #4455 ) ) ;
#55963=FACE_OUTER_BOUND ( 'NONE', #55447, .T. ) ;
#55964=ADVANCED_FACE ( 'NONE', ( #32994 ), #74876, .F. ) ;
#55965=VERTEX_POINT ( 'NONE', #38869 ) ;
#55966=FACE_BOUND ( 'NONE', #81770, .T. ) ;
#55967=CARTESIAN_POINT ( 'NONE',  ( -17.07692307692307665, -3.937682226553329556, 33.60647404775216529 ) ) ;
#55968=AXIS2_PLACEMENT_3D ( 'NONE', #35749, #62750, #13695 ) ;
#55970=EDGE_CURVE ( 'NONE', #36014, #54362, #81630, .T. ) ;
#55971=DIRECTION ( 'NONE',  ( 0.000000000000000000, 0.9848077530122072432, -0.1736481776669354937 ) ) ;
#55972=CARTESIAN_POINT ( 'NONE',  ( -7.145903615555926791, -7.369208160676172348, 34.74850200257122879 ) ) ;
#55973=EDGE_LOOP ( 'NONE', ( #2954, #23943, #38456, #12130 ) ) ;
#55974=CARTESIAN_POINT ( 'NONE',  ( -14.43783951713053249, -12.45813303252208648, 30.39737893381572675 ) ) ;
#55975=CARTESIAN_POINT ( 'NONE',  ( 15.36129466900287532, -2.372941743896879174, 30.88044141588253666 ) ) ;
#55976=CARTESIAN_POINT ( 'NONE',  ( -7.173076923076921574, -2.499999999999998668, 29.75000000000000355 ) ) ;
#55978=EDGE_LOOP ( 'NONE', ( #60790, #79349, #36366, #79205 ) ) ;
#55980=EDGE_CURVE ( 'NONE', #3730, #59070, #68697, .T. ) ;
#55981=CARTESIAN_POINT ( 'NONE',  ( 13.25446817517716980, -6.001485441113819874, 34.52039167877662607 ) ) ;
#55982=VERTEX_POINT ( 'NONE', #47383 ) ;
#55983=CARTESIAN_POINT ( 'NONE',  ( 4.284371592079796010, -3.068774925481847493, 32.56582465632704526 ) ) ;
#55985=CARTESIAN_POINT ( 'NONE',  ( 3.480823542407545101, -2.564540009722895419, 30.55348353981670684 ) ) ;
#55986=FACE_OUTER_BOUND ( 'NONE', #5556, .T. ) ;
#55987=CARTESIAN_POINT ( 'NONE',  ( 16.15384615384615330, -11.11383981884818262, 36.00935417666054406 ) ) ;
#55988=CARTESIAN_POINT ( 'NONE',  ( -13.25408968285181821, -3.816742781228458004, 33.13167719472716044 ) ) ;
#55989=LINE ( 'NONE', #610, #25103 ) ;
#55990=CARTESIAN_POINT ( 'NONE',  ( -5.933932666649925025, -6.343179335718452272, 34.87096338111212646 ) ) ;
#55991=CARTESIAN_POINT ( 'NONE',  ( -2.372943297853547850, -2.506253911140460922, 30.00000000000013856 ) ) ;
#55992=EDGE_CURVE ( 'NONE', #76544, #14556, #32189, .T. ) ;
#55993=CARTESIAN_POINT ( 'NONE',  ( 14.08420736396835871, -3.754499324213721234, 33.06261337010820256 ) ) ;
#55995=ORIENTED_EDGE ( 'NONE', *, *, #53026, .F. ) ;
#55996=DIRECTION ( 'NONE',  ( -0.000000000000000000, 0.7660444431189791237, -0.6427876096865379196 ) ) ;
#55997=ORIENTED_EDGE ( 'NONE', *, *, #85498, .F. ) ;
#55998=ORIENTED_EDGE ( 'NONE', *, *, #6928, .F. ) ;
#55999=CARTESIAN_POINT ( 'NONE',  ( 2.980792499826876440, -4.943428324936578910, 34.04746400365624481 ) ) ;
#56000=VERTEX_POINT ( 'NONE', #18148 ) ;
#56001=CARTESIAN_POINT ( 'NONE',  ( -8.769230769230768274, -13.88283147151868846, 33.14645433367849847 ) ) ;
#56002=EDGE_CURVE ( 'NONE', #18112, #20214, #61204, .T. ) ;
#56004=CARTESIAN_POINT ( 'NONE',  ( -2.307692307692427391, -6.879047030192662504, 34.71129190930017927 ) ) ;
#56005=CARTESIAN_POINT ( 'NONE',  ( -7.053224892808618307, -9.504002272028875709, 34.60269587691767867 ) ) ;
#56006=CARTESIAN_POINT ( 'NONE',  ( 6.065255571276025215, -2.625532179533470512, 30.86335684631491105 ) ) ;
#56007=CARTESIAN_POINT ( 'NONE',  ( 8.519254038288414321, -11.28823185664190376, 33.01397839955799896 ) ) ;
#56008=ADVANCED_FACE ( 'NONE', ( #73548 ), #66777, .F. ) ;
#56009=CARTESIAN_POINT ( 'NONE',  ( 16.02369894440793985, -11.93770438780619259, 32.05411857736982029 ) ) ;
#56011=EDGE_CURVE ( 'NONE', #11473, #37767, #60090, .T. ) ;
#56012=CARTESIAN_POINT ( 'NONE',  ( -0.7115151924808164052, -2.564618984488975961, 30.55390908950641915 ) ) ;
#56013=CARTESIAN_POINT ( 'NONE',  ( 17.99999999999987566, -11.94971097300221174, 32.03036669348237098 ) ) ;
#56014=CYLINDRICAL_SURFACE ( 'NONE', #68026, 0.2500000000000008882 ) ;
#56015=AXIS2_PLACEMENT_3D ( 'NONE', #33718, #67509, #5361 ) ;
#56016=CARTESIAN_POINT ( 'NONE',  ( -9.915234651214539952, -3.395401636524185474, 33.02366814457250399 ) ) ;
#56017=ORIENTED_EDGE ( 'NONE', *, *, #16286, .F. ) ;
#56018=ORIENTED_EDGE ( 'NONE', *, *, #55709, .T. ) ;
#56019=CARTESIAN_POINT ( 'NONE',  ( -18.24997674404858827, -2.544273027872574922, 31.48422191005632342 ) ) ;
#56020=CARTESIAN_POINT ( 'NONE',  ( -3.230769230769229949, -11.16473453929635440, 33.15142922261926373 ) ) ;
#56021=CARTESIAN_POINT ( 'NONE',  ( 11.76147289007438701, -9.886259254753566594, 34.14407573483972413 ) ) ;
#56022=CARTESIAN_POINT ( 'NONE',  ( 0.4615384615387756462, -2.255955759149395501, 30.00000000000324363 ) ) ;
#56023=ORIENTED_EDGE ( 'NONE', *, *, #84001, .F. ) ;
#56024=LINE ( 'NONE', #14602, #21904 ) ;
#56025=CARTESIAN_POINT ( 'NONE',  ( -9.692307692307814193, -6.835583212225970762, 34.95778746994575670 ) ) ;
#56026=B_SPLINE_CURVE_WITH_KNOTS ( 'NONE', 3,
 ( #66470, #38102, #73229, #51143, #10194, #65564, #66915, #3423, #31350, #80440 ),
 .UNSPECIFIED., .F., .F.,
 ( 4, 2, 2, 2, 4 ),
 ( 0.000000000000000000, 0.0001954339857564080165, 0.0003908679715128160329, 0.0005863019572692240765, 0.0007817359430256320659 ),
 .UNSPECIFIED. ) ;
#56027=B_SPLINE_CURVE_WITH_KNOTS ( 'NONE', 3,
 ( #5736, #47158, #12067, #33213, #5297, #87736, #54358, #74649, #81855, #80973 ),
 .UNSPECIFIED., .F., .F.,
 ( 4, 2, 2, 2, 4 ),
 ( 0.000000000000000000, 0.0001954311564186862510, 0.0003908623128373725020, 0.0005862934692560588072, 0.0007817246256747450040 ),
 .UNSPECIFIED. ) ;
#56029=VERTEX_POINT ( 'NONE', #61776 ) ;
#56030=CARTESIAN_POINT ( 'NONE',  ( 15.90386942290380290, -2.779195860258148798, 31.39871582349836743 ) ) ;
#56031=ORIENTED_EDGE ( 'NONE', *, *, #14299, .F. ) ;
#56032=CIRCLE ( 'NONE', #67557, 0.2500000000000002220 ) ;
#56033=CARTESIAN_POINT ( 'NONE',  ( 10.86533013373275658, -8.433404298154334455, 34.66254593164985920 ) ) ;
#56034=VECTOR ( 'NONE', #77464, 1000.000000000000114 ) ;
#56037=FACE_OUTER_BOUND ( 'NONE', #51187, .T. ) ;
#56038=CARTESIAN_POINT ( 'NONE',  ( 4.088576153289833925, -6.835583212224499938, 34.95778746994557906 ) ) ;
#56039=CARTESIAN_POINT ( 'NONE',  ( -6.700297254098858346, -2.612705202774697533, 31.66806509827799943 ) ) ;
#56040=AXIS2_PLACEMENT_3D ( 'NONE', #75587, #6693, #34165 ) ;
#56041=AXIS2_PLACEMENT_3D ( 'NONE', #34791, #62259, #28040 ) ;
#56042=ORIENTED_EDGE ( 'NONE', *, *, #56614, .T. ) ;
#56043=EDGE_CURVE ( 'NONE', #33723, #6671, #54827, .T. ) ;
#56044=VECTOR ( 'NONE', #38848, 999.9999999999998863 ) ;
#56045=ORIENTED_EDGE ( 'NONE', *, *, #13293, .F. ) ;
#56046=ORIENTED_EDGE ( 'NONE', *, *, #55272, .T. ) ;
#56047=EDGE_LOOP ( 'NONE', ( #63436, #24224 ) ) ;
#56048=CARTESIAN_POINT ( 'NONE',  ( -17.29984929443921970, -10.61292498521070549, 33.66303323003028680 ) ) ;
#56049=CARTESIAN_POINT ( 'NONE',  ( 16.02315555073584719, -5.496505350115500121, 34.60290016733514307 ) ) ;
#56050=ADVANCED_FACE ( 'NONE', ( #47831 ), #92, .F. ) ;
#56051=CARTESIAN_POINT ( 'NONE',  ( -12.33074802057151409, -12.35292014791297710, 31.75344720912887198 ) ) ;
#56052=CARTESIAN_POINT ( 'NONE',  ( 17.07692307692295586, -10.33852847137269571, 34.16647553114546554 ) ) ;
#56053=CARTESIAN_POINT ( 'NONE',  ( -17.86920819217521483, -4.118422570099828484, 33.43335022499816489 ) ) ;
#56054=LINE ( 'NONE', #64125, #76859 ) ;
#56057=ORIENTED_EDGE ( 'NONE', *, *, #19648, .T. ) ;
#56058=ADVANCED_FACE ( 'NONE', ( #54579 ), #68987, .F. ) ;
#56059=CARTESIAN_POINT ( 'NONE',  ( -3.230769230769351186, -10.90142922262034020, 33.41473453929536674 ) ) ;
#56060=EDGE_LOOP ( 'NONE', ( #75097, #79869 ) ) ;
#56061=CARTESIAN_POINT ( 'NONE',  ( 17.07692307692307665, -1.129524287112498415, 32.06866353760679544 ) ) ;
#56063=CYLINDRICAL_SURFACE ( 'NONE', #14388, 0.2499999999999986955 ) ;
#56065=VERTEX_POINT ( 'NONE', #14488 ) ;
#56066=VECTOR ( 'NONE', #30610, 1000.000000000000000 ) ;
#56067=ORIENTED_EDGE ( 'NONE', *, *, #79701, .F. ) ;
#56068=DIRECTION ( 'NONE',  ( -0.000000000000000000, -0.8660254037844398178, -0.4999999999999980571 ) ) ;
#56070=ORIENTED_EDGE ( 'NONE', *, *, #40173, .F. ) ;
#56071=FACE_BOUND ( 'NONE', #30183, .T. ) ;
#56072=CARTESIAN_POINT ( 'NONE',  ( -2.241624974342230292, -4.661471528628508665, 34.16647553114624003 ) ) ;
#56074=EDGE_LOOP ( 'NONE', ( #69560, #49989, #72628, #6219 ) ) ;
#56075=CARTESIAN_POINT ( 'NONE',  ( 15.45373236503590952, -7.369474539155828730, 34.99858011523957657 ) ) ;
#56076=EDGE_CURVE ( 'NONE', #66717, #50723, #77313, .T. ) ;
#56077=CYLINDRICAL_SURFACE ( 'NONE', #53270, 0.2500000000000009437 ) ;
#56078=CARTESIAN_POINT ( 'NONE',  ( -13.38461538461538325, -4.945431358278436385, 36.03766855953609394 ) ) ;
#56079=CARTESIAN_POINT ( 'NONE',  ( 0.5923302693632480631, -6.413143153341454017, 34.63066358083362672 ) ) ;
#56080=CARTESIAN_POINT ( 'NONE',  ( 1.449870524128223703, -2.657715359629131857, 31.77849191805844242 ) ) ;
#56081=ORIENTED_EDGE ( 'NONE', *, *, #32617, .F. ) ;
#56082=B_SPLINE_CURVE_WITH_KNOTS ( 'NONE', 3,
 ( #85403, #37202, #78636, #16939, #44389, #10185, #88533, #75003, #13294, #67796 ),
 .UNSPECIFIED., .F., .F.,
 ( 4, 2, 2, 2, 4 ),
 ( 0.0007817246256747530271, 0.0009771112852218974409, 0.001172497944769041638, 0.001367884604316185835, 0.001563271263863330249 ),
 .UNSPECIFIED. ) ;
#56083=CARTESIAN_POINT ( 'NONE',  ( 11.66925334628632527, -3.062576670634119758, 32.05464942895959979 ) ) ;
#56084=CARTESIAN_POINT ( 'NONE',  ( -7.780898274877819709, -6.879047030191282275, 34.71129190930002295 ) ) ;
#56085=CARTESIAN_POINT ( 'NONE',  ( -7.846153846153844924, -13.88283147151868846, 33.14645433367849847 ) ) ;
#56086=FACE_OUTER_BOUND ( 'NONE', #76557, .T. ) ;
#56087=DIRECTION ( 'NONE',  ( 0.000000000000000000, 0.000000000000000000, 1.000000000000000000 ) ) ;
#56088=FACE_BOUND ( 'NONE', #17092, .T. ) ;
#56089=CARTESIAN_POINT ( 'NONE',  ( -6.857821783564083340, -12.70778746994558439, 30.41441678777537305 ) ) ;
#56090=CARTESIAN_POINT ( 'NONE',  ( 17.07692307692307665, -2.833524468853757305, 32.15551576947925838 ) ) ;
#56091=EDGE_CURVE ( 'NONE', #73152, #7875, #48280, .T. ) ;
#56093=CARTESIAN_POINT ( 'NONE',  ( 11.76124120743959978, -12.11081565061823717, 32.26097654155341843 ) ) ;
#56094=CARTESIAN_POINT ( 'NONE',  ( 4.087763774486018242, -5.471508081941601986, 34.59228464037088457 ) ) ;
#56096=FACE_OUTER_BOUND ( 'NONE', #42823, .T. ) ;
#56098=VERTEX_POINT ( 'NONE', #34313 ) ;
#56099=CARTESIAN_POINT ( 'NONE',  ( -5.776987155906605942, -10.77377354290276301, 33.85451476688484718 ) ) ;
#56100=EDGE_LOOP ( 'NONE', ( #64061, #10839 ) ) ;
#56102=VECTOR ( 'NONE', #81001, 1000.000000000000227 ) ;
#56103=CARTESIAN_POINT ( 'NONE',  ( -13.13456096470193302, -9.233818618650603938, 34.70587769442853698 ) ) ;
#56104=ORIENTED_EDGE ( 'NONE', *, *, #47274, .T. ) ;
#56105=CARTESIAN_POINT ( 'NONE',  ( -11.47320596718551577, -2.892918686051626498, 31.69288490824026638 ) ) ;
#56106=CARTESIAN_POINT ( 'NONE',  ( -15.90379173393269951, -12.01375889529407992, 32.43194544308182969 ) ) ;
#56107=ORIENTED_EDGE ( 'NONE', *, *, #6200, .T. ) ;
#56108=CYLINDRICAL_SURFACE ( 'NONE', #59929, 0.2499999999999994726 ) ;
#56110=CARTESIAN_POINT ( 'NONE',  ( 6.066067333350075863, -6.343179335718452272, 34.87096338111212646 ) ) ;
#56111=ADVANCED_FACE ( 'NONE', ( #82523 ), #20802, .F. ) ;
#56112=CYLINDRICAL_SURFACE ( 'NONE', #80621, 0.2499999999999979738 ) ;
#56113=DIRECTION ( 'NONE',  ( -0.000000000000000000, -0.000000000000000000, -1.000000000000000000 ) ) ;
#56115=CARTESIAN_POINT ( 'NONE',  ( 16.82694634598072625, -12.41269422305637171, 30.68257228309993323 ) ) ;
#56117=CARTESIAN_POINT ( 'NONE',  ( -14.17716686945866655, -5.070358843744210198, 34.40418822224088302 ) ) ;
#56120=ADVANCED_FACE ( 'NONE', ( #41975 ), #8632, .F. ) ;
#56121=EDGE_CURVE ( 'NONE', #59958, #80080, #77082, .T. ) ;
#56122=CARTESIAN_POINT ( 'NONE',  ( -18.06608237936013950, -11.35647404775217595, 33.31231777344666511 ) ) ;
#56123=DIRECTION ( 'NONE',  ( -0.000000000000000000, -0.6427876096865404731, -0.7660444431189770143 ) ) ;
#56124=CARTESIAN_POINT ( 'NONE',  ( 8.834486340506792601, -10.21337939537593620, 33.94971097300152252 ) ) ;
#56127=CARTESIAN_POINT ( 'NONE',  ( -14.24162395668986747, -10.51840700105979565, 33.73612834413962247 ) ) ;
#56128=ORIENTED_EDGE ( 'NONE', *, *, #53627, .T. ) ;
#56129=CARTESIAN_POINT ( 'NONE',  ( 6.988222702408889653, -7.750023238201980469, 34.74374492549440419 ) ) ;
#56130=CARTESIAN_POINT ( 'NONE',  ( 16.08857570788537927, -12.27809138561121394, 31.22303859784730307 ) ) ;
#56131=CARTESIAN_POINT ( 'NONE',  ( 1.134638653673032183, -12.41269422305637171, 30.68257228309993323 ) ) ;
#56132=CARTESIAN_POINT ( 'NONE',  ( -14.43783951713052893, -11.93770438780619259, 32.05411857736982029 ) ) ;
#56133=CARTESIAN_POINT ( 'NONE',  ( -16.15384615384615330, -10.51840700105979565, 33.73612834413961536 ) ) ;
#56134=FACE_OUTER_BOUND ( 'NONE', #34117, .T. ) ;
#56135=DIRECTION ( 'NONE',  ( 0.000000000000000000, 0.8660254037844377084, -0.5000000000000015543 ) ) ;
#56136=CARTESIAN_POINT ( 'NONE',  ( -10.36543909703647337, -10.76462480002816235, 33.53768742498949962 ) ) ;
#56137=VERTEX_POINT ( 'NONE', #28006 ) ;
#56138=ORIENTED_EDGE ( 'NONE', *, *, #28891, .T. ) ;
#56141=ORIENTED_EDGE ( 'NONE', *, *, #88466, .F. ) ;
#56142=CARTESIAN_POINT ( 'NONE',  ( -13.38461538461538325, -2.708943851104267164, 35.45975837776705220 ) ) ;
#56143=CARTESIAN_POINT ( 'NONE',  ( 1.384615384615386802, -11.35647404775217417, 33.31231777344666511 ) ) ;
#56144=CARTESIAN_POINT ( 'NONE',  ( -15.23076923076922995, -10.67929555188718282, 33.92786785259544047 ) ) ;
#56145=CARTESIAN_POINT ( 'NONE',  ( 3.230769230769231726, -5.471508081941601098, 34.59228464037088457 ) ) ;
#56146=CARTESIAN_POINT ( 'NONE',  ( 13.16168842570853492, -8.282780595021769443, 34.94152052738834868 ) ) ;
#56147=VERTEX_POINT ( 'NONE', #21239 ) ;
#56148=CARTESIAN_POINT ( 'NONE',  ( -17.32689980786543060, -4.236021600441997492, 33.53823185664189310 ) ) ;
#56149=ORIENTED_EDGE ( 'NONE', *, *, #59357, .T. ) ;
#56150=ORIENTED_EDGE ( 'NONE', *, *, #41170, .T. ) ;
#56151=B_SPLINE_CURVE_WITH_KNOTS ( 'NONE', 3,
 ( #42672, #77334, #76458, #16079, #15640, #43541, #35915, #57057, #43108, #29166 ),
 .UNSPECIFIED., .F., .F.,
 ( 4, 2, 2, 2, 4 ),
 ( 0.000000000000000000, 0.0001954339857564072033, 0.0003908679715128144066, 0.0005863019572692215828, 0.0007817359430256288133 ),
 .UNSPECIFIED. ) ;
#56152=VECTOR ( 'NONE', #86336, 1000.000000000000000 ) ;
#56153=ORIENTED_EDGE ( 'NONE', *, *, #32487, .F. ) ;
#56157=CARTESIAN_POINT ( 'NONE',  ( -10.39195765352304512, -7.630147231320743018, 34.74852402298682819 ) ) ;
#56158=VECTOR ( 'NONE', #2332, 1000.000000000000227 ) ;
#56160=CARTESIAN_POINT ( 'NONE',  ( 14.05769230769231015, -7.433932668274256805, 35.00000000000000711 ) ) ;
#56161=ORIENTED_EDGE ( 'NONE', *, *, #75753, .T. ) ;
#56163=ORIENTED_EDGE ( 'NONE', *, *, #22256, .F. ) ;
#56164=AXIS2_PLACEMENT_3D ( 'NONE', #2123, #29608, #57066 ) ;
#56165=ORIENTED_EDGE ( 'NONE', *, *, #86722, .T. ) ;
#56166=CARTESIAN_POINT ( 'NONE',  ( -2.307692307692428724, -3.643525952248796163, 33.31231777344771672 ) ) ;
#56167=CARTESIAN_POINT ( 'NONE',  ( 4.219101725122177626, -11.48612834413965977, 32.76840700105972815 ) ) ;
#56168=ORIENTED_EDGE ( 'NONE', *, *, #16338, .F. ) ;
#56170=LINE ( 'NONE', #84101, #9077 ) ;
#56171=CARTESIAN_POINT ( 'NONE',  ( -2.176900499867520100, -8.147973898785416225, 34.70805048591653730 ) ) ;
#56172=DIRECTION ( 'NONE',  ( -0.000000000000000000, -0.9396926207859092051, -0.3420201433256662704 ) ) ;
#56173=ORIENTED_EDGE ( 'NONE', *, *, #84000, .F. ) ;
#56174=CYLINDRICAL_SURFACE ( 'NONE', #43676, 0.2499999999999979738 ) ;
#56175=CARTESIAN_POINT ( 'NONE',  ( -15.23076923076922995, -12.34228464037088635, 31.77849191805839268 ) ) ;
#56176=VERTEX_POINT ( 'NONE', #38312 ) ;
#56177=FACE_BOUND ( 'NONE', #19837, .T. ) ;
#56178=CARTESIAN_POINT ( 'NONE',  ( -6.249999999999997335, -2.249999999999998668, 29.75000000000000355 ) ) ;
#56179=DIRECTION ( 'NONE',  ( -0.000000000000000000, -0.7660444431189791237, -0.6427876096865379196 ) ) ;
#56180=EDGE_CURVE ( 'NONE', #14452, #28219, #45052, .T. ) ;
#56181=CARTESIAN_POINT ( 'NONE',  ( 3.361294932532796764, -9.417988943895561960, 34.36773134775778260 ) ) ;
#56182=CARTESIAN_POINT ( 'NONE',  ( -17.07692307692307665, -1.215029322943914858, 32.30358669280327177 ) ) ;
#56183=CARTESIAN_POINT ( 'NONE',  ( 5.011652630962299959, -10.21337939537584383, 33.94971097300158647 ) ) ;
#56184=CARTESIAN_POINT ( 'NONE',  ( -3.903900635498011695, -2.824170634883622188, 31.52227843825338738 ) ) ;
#56185=DIRECTION ( 'NONE',  ( 0.000000000000000000, 0.1736481776669267785, -0.9848077530122087975 ) ) ;
#56186=EDGE_LOOP ( 'NONE', ( #25767, #78921 ) ) ;
#56187=CARTESIAN_POINT ( 'NONE',  ( -2.531177232256637488, -4.225889041578354544, 33.85425143139329407 ) ) ;
#56189=ORIENTED_EDGE ( 'NONE', *, *, #66564, .T. ) ;
#56190=B_SPLINE_CURVE_WITH_KNOTS ( 'NONE', 3,
 ( #83340, #7232, #474, #62601, #1794, #1350, #27943, #41459, #41910, #55409 ),
 .UNSPECIFIED., .F., .F.,
 ( 4, 2, 2, 2, 4 ),
 ( 0.000000000000000000, 0.0001954339857564097241, 0.0003908679715128194482, 0.0005863019572692291723, 0.0007817359430256388964 ),
 .UNSPECIFIED. ) ;
#56191=B_SPLINE_CURVE_WITH_KNOTS ( 'NONE', 3,
 ( #56409, #49647, #135, #42456, #69918, #8675, #76683, #15430, #8227, #75784 ),
 .UNSPECIFIED., .F., .F.,
 ( 4, 2, 2, 2, 4 ),
 ( 0.0007817359430256256691, 0.0009771253907249902518, 0.001172514838424355051, 0.001367904286123719851, 0.001563293733823084434 ),
 .UNSPECIFIED. ) ;
#56192=B_SPLINE_CURVE_WITH_KNOTS ( 'NONE', 3,
 ( #74185, #32315, #46269, #39968, #26446, #73758, #76396, #55234, #68755, #297 ),
 .UNSPECIFIED., .F., .F.,
 ( 4, 2, 2, 2, 4 ),
 ( 0.000000000000000000, 0.0001954311564186858715, 0.0003908623128373717431, 0.0005862934692560576146, 0.0007817246256747434861 ),
 .UNSPECIFIED. ) ;
#56194=CARTESIAN_POINT ( 'NONE',  ( -17.32692307692307665, -7.500000000000001776, 35.00000000000000000 ) ) ;
#56195=CARTESIAN_POINT ( 'NONE',  ( 7.596153846153846700, -7.500000000000001776, 35.04278698407183867 ) ) ;
#56196=ORIENTED_EDGE ( 'NONE', *, *, #40660, .T. ) ;
#56197=CARTESIAN_POINT ( 'NONE',  ( -13.13466997523734214, -11.56426240980093745, 33.07394671870546432 ) ) ;
#56199=FACE_BOUND ( 'NONE', #34094, .T. ) ;
#56200=CARTESIAN_POINT ( 'NONE',  ( -1.514763354347079982, -6.809168938359898782, 34.95455904226513866 ) ) ;
#56201=CARTESIAN_POINT ( 'NONE',  ( -3.930834802233302394, -8.239487800360276282, 34.69522927552633718 ) ) ;
#56202=ADVANCED_FACE ( 'NONE', ( #15830 ), #78841, .T. ) ;
#56203=CARTESIAN_POINT ( 'NONE',  ( -15.93106661257774270, -2.600157965045223563, 30.74683119005207033 ) ) ;
#56204=CARTESIAN_POINT ( 'NONE',  ( -5.011667937410237528, -10.33852847137154107, 34.16647553114620450 ) ) ;
#56205=CARTESIAN_POINT ( 'NONE',  ( -17.07692307692276046, -2.255955759149395501, 30.00000000000324363 ) ) ;
#56209=EDGE_LOOP ( 'NONE', ( #56608, #32035, #4142, #86144 ) ) ;
#56210=CARTESIAN_POINT ( 'NONE',  ( -9.469528151039279251, -11.89424750095246175, 32.13594075562311758 ) ) ;
#56211=CARTESIAN_POINT ( 'NONE',  ( -10.54931728203453822, -8.164416787775445883, 34.95778746994558617 ) ) ;
#56212=CARTESIAN_POINT ( 'NONE',  ( 7.173076923078343548, -7.500000000000154543, 35.00000000000007105 ) ) ;
#56213=CARTESIAN_POINT ( 'NONE',  ( -0.5916864312701606288, -3.069018819979302926, 32.56621877034667278 ) ) ;
#56214=CARTESIAN_POINT ( 'NONE',  ( -16.21992956480203318, -12.10708131394839349, 31.69288490824020244 ) ) ;
#56216=CARTESIAN_POINT ( 'NONE',  ( 0.4615384615383382183, -4.320704448113951379, 33.92786785259630022 ) ) ;
#56217=DIRECTION ( 'NONE',  ( 0.000000000000000000, 0.9396926207859126468, -0.3420201433256571111 ) ) ;
#56218=CARTESIAN_POINT ( 'NONE',  ( -17.14300648787895298, -4.786620604624113540, 33.94971097300155805 ) ) ;
#56219=CARTESIAN_POINT ( 'NONE',  ( 18.00000000000000000, -8.164416787775445883, 34.95778746994557906 ) ) ;
#56220=DIRECTION ( 'NONE',  ( -0.000000000000000000, 0.7660444431189791237, -0.6427876096865379196 ) ) ;
#56222=CARTESIAN_POINT ( 'NONE',  ( -5.776987155906604166, -11.43677907613344757, 33.22367315496201456 ) ) ;
#56223=ADVANCED_FACE ( 'NONE', ( #70769 ), #86058, .F. ) ;
#56224=EDGE_CURVE ( 'NONE', #12547, #70275, #39687, .T. ) ;
#56225=DIRECTION ( 'NONE',  ( 0.000000000000000000, 0.9396926207859126468, -0.3420201433256571111 ) ) ;
#56226=AXIS2_PLACEMENT_3D ( 'NONE', #69272, #82798, #21521 ) ;
#56227=CARTESIAN_POINT ( 'NONE',  ( 3.100077764101672351, -2.541943142973489778, 30.39792223712631980 ) ) ;
#56228=ORIENTED_EDGE ( 'NONE', *, *, #28936, .T. ) ;
#56229=CARTESIAN_POINT ( 'NONE',  ( -14.30769230769230660, -3.513871655860378418, 32.76840700105978499 ) ) ;
#56230=CARTESIAN_POINT ( 'NONE',  ( -5.076923076923075762, -3.322132147404559976, 32.92929555188717927 ) ) ;
#56232=B_SPLINE_CURVE_WITH_KNOTS ( 'NONE', 3,
 ( #64920, #71234, #85653, #18533, #17185, #79790, #9539, #72575, #37005, #2767 ),
 .UNSPECIFIED., .F., .F.,
 ( 4, 2, 2, 2, 4 ),
 ( 0.000000000000000000, 0.0001954339857564080978, 0.0003908679715128161956, 0.0005863019572692242934, 0.0007817359430256323911 ),
 .UNSPECIFIED. ) ;
#56233=VECTOR ( 'NONE', #86209, 999.9999999999998863 ) ;
#56234=VECTOR ( 'NONE', #14426, 1000.000000000000000 ) ;
#56235=CARTESIAN_POINT ( 'NONE',  ( 0.6845513056318562883, -3.395485233115138168, 33.02377354290275946 ) ) ;
#56236=CARTESIAN_POINT ( 'NONE',  ( 16.85343815235874132, -11.60425143139329940, 33.02411095842164457 ) ) ;
#56237=ORIENTED_EDGE ( 'NONE', *, *, #23064, .T. ) ;
#56238=CARTESIAN_POINT ( 'NONE',  ( -9.942284436356281674, -5.643011162660950042, 34.66104346484419096 ) ) ;
#56240=VERTEX_POINT ( 'NONE', #56800 ) ;
#56241=CARTESIAN_POINT ( 'NONE',  ( 7.846153846153846700, -3.513871655860378418, 32.76840700105978499 ) ) ;
#56242=CARTESIAN_POINT ( 'NONE',  ( -2.557715531913763662, -10.92453946501458439, 33.72985991061850086 ) ) ;
#56243=ORIENTED_EDGE ( 'NONE', *, *, #47334, .F. ) ;
#56249=CARTESIAN_POINT ( 'NONE',  ( 8.769230769230645706, -2.379036618888197729, 30.90682066428292885 ) ) ;
#56250=CARTESIAN_POINT ( 'NONE',  ( -11.53846153846166089, -12.51329471203414379, 31.30864560766407578 ) ) ;
#56251=CARTESIAN_POINT ( 'NONE',  ( -9.442307692307688072, -2.499999999999999556, 29.81604066197449754 ) ) ;
#56252=ORIENTED_EDGE ( 'NONE', *, *, #24908, .T. ) ;
#56253=EDGE_LOOP ( 'NONE', ( #61537, #11948, #45284, #31131 ) ) ;
#56254=CARTESIAN_POINT ( 'NONE',  ( 6.066068351002440906, -6.386643153685127139, 34.62446782046654192 ) ) ;
#56255=ORIENTED_EDGE ( 'NONE', *, *, #27874, .T. ) ;
#56256=CARTESIAN_POINT ( 'NONE',  ( 5.142990410273151625, -4.661471528628508665, 34.16647553114624003 ) ) ;
#56257=CARTESIAN_POINT ( 'NONE',  ( 13.63466980452883881, -3.435999193479609914, 33.07426656108010832 ) ) ;
#56258=CARTESIAN_POINT ( 'NONE',  ( -4.403822884788506364, -6.567427716900047230, 34.66269422305636283 ) ) ;
#56259=CARTESIAN_POINT ( 'NONE',  ( -4.153846153846152411, -12.62096338111211580, 30.90682066428153263 ) ) ;
#56260=CARTESIAN_POINT ( 'NONE',  ( -17.07692307692307665, -5.180354513474913603, 36.12317359536750416 ) ) ;
#56261=VECTOR ( 'NONE', #35418, 1000.000000000000000 ) ;
#56262=ORIENTED_EDGE ( 'NONE', *, *, #74398, .T. ) ;
#56263=ORIENTED_EDGE ( 'NONE', *, *, #28038, .T. ) ;
#56264=CARTESIAN_POINT ( 'NONE',  ( 9.626224281351811740, -4.098570777380720287, 33.41473453929634729 ) ) ;
#56265=ORIENTED_EDGE ( 'NONE', *, *, #51248, .F. ) ;
#56266=VECTOR ( 'NONE', #44130, 999.9999999999998863 ) ;
#56267=CARTESIAN_POINT ( 'NONE',  ( -9.442307692307691624, -2.499999999999998668, 29.75000000000000355 ) ) ;
#56269=CARTESIAN_POINT ( 'NONE',  ( -17.93474442872397034, -3.300289026998476150, 32.46337939537591666 ) ) ;
#56271=VERTEX_POINT ( 'NONE', #43728 ) ;
#56272=DIRECTION ( 'NONE',  ( 0.000000000000000000, 0.9848077530122072432, -0.1736481776669354937 ) ) ;
#56273=EDGE_CURVE ( 'NONE', #53485, #51137, #53711, .T. ) ;
#56275=CARTESIAN_POINT ( 'NONE',  ( -6.857008572074484221, -11.16473453929635440, 33.15142922261926373 ) ) ;
#56277=DIRECTION ( 'NONE',  ( 0.000000000000000000, 0.9848077530122072432, -0.1736481776669354937 ) ) ;
#56278=ORIENTED_EDGE ( 'NONE', *, *, #62165, .F. ) ;
#56279=CARTESIAN_POINT ( 'NONE',  ( 17.93472955403921887, -10.90142922261923886, 33.41473453929638993 ) ) ;
#56280=DIRECTION ( 'NONE',  ( 0.000000000000000000, 0.3420201433256610524, 0.9396926207859113145 ) ) ;
#56281=B_SPLINE_CURVE_WITH_KNOTS ( 'NONE', 3,
 ( #59715, #72335, #18740, #32684, #52061, #10645, #38110, #60152, #79553, #72775 ),
 .UNSPECIFIED., .F., .F.,
 ( 4, 2, 2, 2, 4 ),
 ( 0.000000000000000000, 0.0001954339857564091549, 0.0003908679715128183098, 0.0005863019572692274375, 0.0007817359430256366195 ),
 .UNSPECIFIED. ) ;
#56282=FACE_BOUND ( 'NONE', #19090, .T. ) ;
#56283=CARTESIAN_POINT ( 'NONE',  ( -11.78843826940389405, -2.564618984488975073, 30.55390908950641915 ) ) ;
#56284=CARTESIAN_POINT ( 'NONE',  ( -6.700065571464072889, -12.15243808032446005, 31.58219941686247978 ) ) ;
#56285=B_SPLINE_CURVE_WITH_KNOTS ( 'NONE', 3,
 ( #27321, #5716, #54783, #33189, #88163, #82273, #39518, #53901, #20559, #48023 ),
 .UNSPECIFIED., .F., .F.,
 ( 4, 2, 2, 2, 4 ),
 ( 0.000000000000000000, 0.0001954311564186861968, 0.0003908623128373723936, 0.0005862934692560585904, 0.0007817246256747447872 ),
 .UNSPECIFIED. ) ;
#56288=CARTESIAN_POINT ( 'NONE',  ( 15.45354889974729318, -2.612705202774698421, 31.66806509827799943 ) ) ;
#56289=CARTESIAN_POINT ( 'NONE',  ( 12.39545608217832395, -3.322132147404559532, 32.92929555188719348 ) ) ;
#56290=CARTESIAN_POINT ( 'NONE',  ( 5.299702618191484582, -10.81320215134717344, 33.49497208177562868 ) ) ;
#56291=CARTESIAN_POINT ( 'NONE',  ( -17.07692307692319744, -5.941354392335915335, 34.76329471203413846 ) ) ;
#56292=EDGE_LOOP ( 'NONE', ( #29428, #53814 ) ) ;
#56293=CARTESIAN_POINT ( 'NONE',  ( 10.55011416942384095, -10.21337939537584383, 33.94971097300158647 ) ) ;
#56294=ADVANCED_FACE ( 'NONE', ( #37864 ), #9942, .F. ) ;
#56295=EDGE_LOOP ( 'NONE', ( #19933, #33274 ) ) ;
#56296=ORIENTED_EDGE ( 'NONE', *, *, #3699, .F. ) ;
#56298=CARTESIAN_POINT ( 'NONE',  ( 14.55774661933062397, -3.627508038966690496, 32.91356715214248396 ) ) ;
#56299=CARTESIAN_POINT ( 'NONE',  ( 7.976945653978634532, -9.804649428959608670, 34.18742332936588468 ) ) ;
#56300=CARTESIAN_POINT ( 'NONE',  ( -18.00000000000000000, -6.436573248120765811, 35.78099280442780383 ) ) ;
#56301=CARTESIAN_POINT ( 'NONE',  ( 7.976679284387491187, -3.625058011473228703, 33.29252011169590020 ) ) ;
#56302=CARTESIAN_POINT ( 'NONE',  ( 1.634560793993430794, -10.92531984108285670, 33.72920026020278073 ) ) ;
#56303=CARTESIAN_POINT ( 'NONE',  ( -12.46153846153846168, -4.661471528628507777, 34.16647553114623292 ) ) ;
#56304=VERTEX_POINT ( 'NONE', #85171 ) ;
#56305=CARTESIAN_POINT ( 'NONE',  ( -18.06608341095587278, -5.557115091759785130, 34.35708131394839171 ) ) ;
#56306=CARTESIAN_POINT ( 'NONE',  ( -17.07692307692307665, -12.09954503811598769, 35.62045528018868623 ) ) ;
#56307=CARTESIAN_POINT ( 'NONE',  ( -12.46153846153858424, -11.67786785259630911, 32.92929555188603530 ) ) ;
#56308=EDGE_CURVE ( 'NONE', #25632, #15004, #17171, .T. ) ;
#56309=CARTESIAN_POINT ( 'NONE',  ( -8.703163435880695076, -2.486705287966280320, 31.30864560766543647 ) ) ;
#56310=CARTESIAN_POINT ( 'NONE',  ( -15.23076923076892264, -2.506253911140614576, 30.00000000000323297 ) ) ;
#56311=ORIENTED_EDGE ( 'NONE', *, *, #4017, .F. ) ;
#56312=CARTESIAN_POINT ( 'NONE',  ( -0.5268084620947809382, -2.379036618887870880, 30.90682066428147579 ) ) ;
#56313=EDGE_LOOP ( 'NONE', ( #53152, #88991, #29969, #87917 ) ) ;
#56314=EDGE_LOOP ( 'NONE', ( #38425, #78590, #59349, #76553 ) ) ;
#56315=EDGE_CURVE ( 'NONE', #10775, #28383, #2730, .T. ) ;
#56316=CARTESIAN_POINT ( 'NONE',  ( 17.07692307692307665, -13.75783147151868846, 33.36296068462461051 ) ) ;
#56317=ORIENTED_EDGE ( 'NONE', *, *, #22671, .T. ) ;
#56318=CARTESIAN_POINT ( 'NONE',  ( -1.134561072977068763, -8.303483539816728154, 34.68545999027711702 ) ) ;
#56319=CARTESIAN_POINT ( 'NONE',  ( -1.384615384615506484, -10.33852847137269571, 34.16647553114546554 ) ) ;
#56320=CARTESIAN_POINT ( 'NONE',  ( 14.17700170458200404, -9.929715669179220328, 34.40415004197138416 ) ) ;
#56321=CARTESIAN_POINT ( 'NONE',  ( -5.076923076923199218, -3.643525952248796163, 33.31231777344771672 ) ) ;
#56323=DIRECTION ( 'NONE',  ( -1.000000000000000000, 0.000000000000000000, 0.000000000000000000 ) ) ;
#56324=EDGE_LOOP ( 'NONE', ( #55404, #27244, #68313, #7243, #58579, #66376 ) ) ;
#56325=CARTESIAN_POINT ( 'NONE',  ( -11.47229493186989657, -7.250054591869670162, 34.99404684341514127 ) ) ;
#56326=CARTESIAN_POINT ( 'NONE',  ( -13.13466986626724342, -4.336752205174649433, 33.62275283266504289 ) ) ;
#56327=ORIENTED_EDGE ( 'NONE', *, *, #81963, .T. ) ;
#56328=DIRECTION ( 'NONE',  ( -0.000000000000000000, -0.8660254037844397068, -0.4999999999999978906 ) ) ;
#56329=CARTESIAN_POINT ( 'NONE',  ( -10.48459280755982981, -3.530189275343204702, 32.79018710029569661 ) ) ;
#56330=CARTESIAN_POINT ( 'NONE',  ( 16.82694634598072270, -3.627789207965226304, 32.91389620160131102 ) ) ;
#56331=CARTESIAN_POINT ( 'NONE',  ( -17.75005448165186195, -11.86320923018887896, 32.19269448109603360 ) ) ;
#56332=CARTESIAN_POINT ( 'NONE',  ( -2.057746898314262385, -2.341251567377310217, 30.72681386836322659 ) ) ;
#56333=ADVANCED_FACE ( 'NONE', ( #17143 ), #44600, .F. ) ;
#56334=CARTESIAN_POINT ( 'NONE',  ( 16.82692307692307665, -7.500000000000001776, 34.75000000000000000 ) ) ;
#56335=LINE ( 'NONE', #9041, #20573 ) ;
#56336=EDGE_CURVE ( 'NONE', #59263, #86041, #34418, .T. ) ;
#56337=AXIS2_PLACEMENT_3D ( 'NONE', #21342, #69087, #14589 ) ;
#56339=EDGE_LOOP ( 'NONE', ( #50236, #16592 ) ) ;
#56340=CARTESIAN_POINT ( 'NONE',  ( -1.134561072977069651, -11.28795663066794219, 33.01431243580653785 ) ) ;
#56341=CARTESIAN_POINT ( 'NONE',  ( -1.449885830576159274, -12.27809138561121394, 31.22303859784730307 ) ) ;
#56343=CARTESIAN_POINT ( 'NONE',  ( 8.069165197766695385, -2.554770724473667709, 30.48948780036025852 ) ) ;
#56345=EDGE_CURVE ( 'NONE', #1161, #48109, #27872, .T. ) ;
#56346=ORIENTED_EDGE ( 'NONE', *, *, #52006, .F. ) ;
#56347=LINE ( 'NONE', #77940, #67213 ) ;
#56348=CARTESIAN_POINT ( 'NONE',  ( 6.000000000000001776, -4.098570777380720287, 33.41473453929634729 ) ) ;
#56349=ORIENTED_EDGE ( 'NONE', *, *, #50582, .F. ) ;
#56351=CARTESIAN_POINT ( 'NONE',  ( -4.219116599806928214, -10.90142922261923886, 33.41473453929638993 ) ) ;
#56352=ORIENTED_EDGE ( 'NONE', *, *, #66072, .F. ) ;
#56353=CARTESIAN_POINT ( 'NONE',  ( -39.05038313613820122, -2.249999999999998668, 29.75000000000000355 ) ) ;
#56354=DIRECTION ( 'NONE',  ( -0.000000000000000000, -0.000000000000000000, -1.000000000000000000 ) ) ;
#56355=CARTESIAN_POINT ( 'NONE',  ( -13.38461538461538325, -10.51840700105979565, 33.73612834413961536 ) ) ;
#56356=CARTESIAN_POINT ( 'NONE',  ( -4.284536756956459413, -11.37499894934982514, 33.29245874905763003 ) ) ;
#56357=EDGE_LOOP ( 'NONE', ( #34331, #45502 ) ) ;
#56358=CARTESIAN_POINT ( 'NONE',  ( -6.857821783564084228, -6.835583212224609184, 34.95778746994559327 ) ) ;
#56359=ORIENTED_EDGE ( 'NONE', *, *, #29881, .T. ) ;
#56361=FACE_OUTER_BOUND ( 'NONE', #79181, .T. ) ;
#56362=CARTESIAN_POINT ( 'NONE',  ( 5.869389640375470840, -7.722926236386453702, 34.74524107206102030 ) ) ;
#56363=ORIENTED_EDGE ( 'NONE', *, *, #72348, .F. ) ;
#56365=CARTESIAN_POINT ( 'NONE',  ( -8.834501215191544077, -2.625532179533444754, 30.86335684631481513 ) ) ;
#56367=B_SPLINE_CURVE_WITH_KNOTS ( 'NONE', 3,
 ( #78724, #10713, #38177, #65635, #3937, #46275, #55569, #14592, #19250, #32321 ),
 .UNSPECIFIED., .F., .F.,
 ( 4, 2, 2, 2, 4 ),
 ( 0.000000000000000000, 0.0001954311564186863323, 0.0003908623128373726646, 0.0005862934692560590241, 0.0007817246256747453293 ),
 .UNSPECIFIED. ) ;
#56368=B_SPLINE_CURVE_WITH_KNOTS ( 'NONE', 3,
 ( #12977, #60264, #7881, #49306, #28599, #14635, #53504, #15084, #1120, #40462 ),
 .UNSPECIFIED., .F., .F.,
 ( 4, 2, 2, 2, 4 ),
 ( 0.0007817359430256293554, 0.0009771253907249950223, 0.001172514838424360906, 0.001367904286123726790, 0.001563293733823092457 ),
 .UNSPECIFIED. ) ;
#56369=CARTESIAN_POINT ( 'NONE',  ( -11.28851612908349722, -5.766571408460171355, 34.70601412856602508 ) ) ;
#56371=B_SPLINE_CURVE_WITH_KNOTS ( 'NONE', 3,
 ( #40333, #67801, #46639, #74116, #12850, #12412, #61037, #26813, #20053, #40779 ),
 .UNSPECIFIED., .F., .F.,
 ( 4, 2, 2, 2, 4 ),
 ( 0.000000000000000000, 0.0001954311564186882026, 0.0003908623128373764051, 0.0005862934692560646619, 0.0007817246256747528103 ),
 .UNSPECIFIED. ) ;
#56372=EDGE_CURVE ( 'NONE', #55677, #22548, #12622, .T. ) ;
#56374=EDGE_LOOP ( 'NONE', ( #54414, #24433 ) ) ;
#56375=FACE_BOUND ( 'NONE', #7671, .T. ) ;
#56376=VERTEX_POINT ( 'NONE', #53599 ) ;
#56377=CARTESIAN_POINT ( 'NONE',  ( 8.519254038288416098, -3.627789207965226748, 32.91389620160131102 ) ) ;
#56378=ADVANCED_FACE ( 'NONE', ( #60352 ), #73438, .F. ) ;
#56379=CARTESIAN_POINT ( 'NONE',  ( -14.17716686945866655, -11.66157788607254098, 32.95092075102925833 ) ) ;
#56380=CARTESIAN_POINT ( 'NONE',  ( 13.38461538461526601, -8.613356846316285953, 34.62446782046622218 ) ) ;
#56381=CARTESIAN_POINT ( 'NONE',  ( -15.23076923076922995, -9.905515769479276145, 34.41647553114623292 ) ) ;
#56382=EDGE_LOOP ( 'NONE', ( #40001, #4236, #9962, #63193 ) ) ;
#56383=ADVANCED_FACE ( 'NONE', ( #19818 ), #40105, .F. ) ;
#56384=ORIENTED_EDGE ( 'NONE', *, *, #40660, .F. ) ;
#56385=ORIENTED_EDGE ( 'NONE', *, *, #35553, .F. ) ;
#56386=AXIS2_PLACEMENT_3D ( 'NONE', #66276, #45112, #73494 ) ;
#56387=CARTESIAN_POINT ( 'NONE',  ( 13.60804234647695843, -7.630147231320743018, 34.74852402298682819 ) ) ;
#56388=VERTEX_POINT ( 'NONE', #32888 ) ;
#56390=AXIS2_PLACEMENT_3D ( 'NONE', #67442, #33210, #60675 ) ;
#56391=CARTESIAN_POINT ( 'NONE',  ( -2.557715531913763662, -12.45566812827425096, 31.48439005359158926 ) ) ;
#56392=CARTESIAN_POINT ( 'NONE',  ( -18.00000000000000000, -11.16473453929635440, 33.15142922261927083 ) ) ;
#56393=ORIENTED_EDGE ( 'NONE', *, *, #20665, .T. ) ;
#56394=CARTESIAN_POINT ( 'NONE',  ( -6.923076923076922462, -10.67929555188718282, 33.92786785259544047 ) ) ;
#56395=EDGE_CURVE ( 'NONE', #73783, #15793, #11757, .T. ) ;
#56396=CARTESIAN_POINT ( 'NONE',  ( -6.222926958906846551, -6.459968553980839800, 34.89616026154728701 ) ) ;
#56397=DIRECTION ( 'NONE',  ( 0.000000000000000000, 0.000000000000000000, 1.000000000000000000 ) ) ;
#56398=CARTESIAN_POINT ( 'NONE',  ( 9.692307692307570832, -11.67786785259630911, 32.92929555188603530 ) ) ;
#56399=ORIENTED_EDGE ( 'NONE', *, *, #31470, .F. ) ;
#56400=EDGE_CURVE ( 'NONE', #41883, #47389, #13061, .T. ) ;
#56401=ORIENTED_EDGE ( 'NONE', *, *, #60568, .T. ) ;
#56402=ORIENTED_EDGE ( 'NONE', *, *, #66459, .T. ) ;
#56403=CARTESIAN_POINT ( 'NONE',  ( 4.023155550735844521, -2.845849958028613624, 32.17971566917920967 ) ) ;
#56404=DIRECTION ( 'NONE',  ( 0.000000000000000000, 0.3420201433256610524, 0.9396926207859113145 ) ) ;
#56405=CARTESIAN_POINT ( 'NONE',  ( 17.07692307692307665, -1.117168528481311540, 33.14645433367849847 ) ) ;
#56406=CARTESIAN_POINT ( 'NONE',  ( 11.31553457955468645, -2.308479472611653094, 30.53278059502174457 ) ) ;
#56407=CARTESIAN_POINT ( 'NONE',  ( -2.242437168179468365, -2.657715359629131857, 31.77849191805844242 ) ) ;
#56408=FACE_BOUND ( 'NONE', #52928, .T. ) ;
#56409=CARTESIAN_POINT ( 'NONE',  ( 7.846153846153725020, -11.48612834414049644, 32.76840700105863391 ) ) ;
#56410=ORIENTED_EDGE ( 'NONE', *, *, #74669, .F. ) ;
#56411=CARTESIAN_POINT ( 'NONE',  ( 17.29970274590113632, -12.11081565061823717, 32.26097654155341843 ) ) ;
#56412=CARTESIAN_POINT ( 'NONE',  ( 8.769230769230768274, -4.786620604624113540, 33.94971097300155094 ) ) ;
#56413=CARTESIAN_POINT ( 'NONE',  ( -1.384615384615383471, -3.513871655860378418, 32.76840700105978499 ) ) ;
#56415=ORIENTED_EDGE ( 'NONE', *, *, #41064, .T. ) ;
#56416=CARTESIAN_POINT ( 'NONE',  ( 2.373760658694747949, -11.69971097300155272, 32.46337939537588113 ) ) ;
#56417=ORIENTED_EDGE ( 'NONE', *, *, #29407, .F. ) ;
#56418=FACE_BOUND ( 'NONE', #19070, .T. ) ;
#56419=CARTESIAN_POINT ( 'NONE',  ( 13.13461538461538680, -2.499999999999998668, 29.75000000000000355 ) ) ;
#56421=AXIS2_PLACEMENT_3D ( 'NONE', #35884, #63343, #22360 ) ;
#56422=CARTESIAN_POINT ( 'NONE',  ( 16.94677586748486320, -11.93770438780619259, 32.05411857736982029 ) ) ;
#56423=CARTESIAN_POINT ( 'NONE',  ( -11.28840722682322273, -11.79725096376909299, 32.30694842903960762 ) ) ;
#56424=VERTEX_POINT ( 'NONE', #67124 ) ;
#56425=CARTESIAN_POINT ( 'NONE',  ( 11.66898697669518192, -11.04252011169590020, 33.62494198852677130 ) ) ;
#56426=CARTESIAN_POINT ( 'NONE',  ( -3.360917200500926239, -2.373036134822904319, 30.88089517874952250 ) ) ;
#56427=CARTESIAN_POINT ( 'NONE',  ( 8.546303810323919947, -8.282780595021769443, 34.94152052738834868 ) ) ;
#56428=CARTESIAN_POINT ( 'NONE',  ( 6.223011351612852238, -3.587049720035815348, 32.86302985866382897 ) ) ;
#56429=ORIENTED_EDGE ( 'NONE', *, *, #34013, .T. ) ;
#56431=CARTESIAN_POINT ( 'NONE',  ( -3.930834802233303282, -6.503523203565942268, 34.64991518177335195 ) ) ;
#56432=EDGE_LOOP ( 'NONE', ( #28843, #13887, #73307, #5925 ) ) ;
#56433=LINE ( 'NONE', #75810, #59778 ) ;
#56434=EDGE_LOOP ( 'NONE', ( #7068, #49740 ) ) ;
#56435=CARTESIAN_POINT ( 'NONE',  ( 11.76124107972994537, -6.760870238392817200, 34.69528174975672385 ) ) ;
#56437=CARTESIAN_POINT ( 'NONE',  ( -5.076923076923075762, -12.10708131394839349, 31.69288490824020244 ) ) ;
#56438=FACE_OUTER_BOUND ( 'NONE', #49329, .T. ) ;
#56439=CARTESIAN_POINT ( 'NONE',  ( -5.749945580086545327, -6.523592122091591783, 34.90882529074906415 ) ) ;
#56440=CARTESIAN_POINT ( 'NONE',  ( 0.3962144487341521248, -7.749976730030849303, 34.74374725381503737 ) ) ;
#56441=EDGE_CURVE ( 'NONE', #88317, #32595, #32003, .T. ) ;
#56444=EDGE_LOOP ( 'NONE', ( #75146, #51048 ) ) ;
#56445=CARTESIAN_POINT ( 'NONE',  ( -15.16470087976679437, -3.513871655860379306, 32.76840700105978499 ) ) ;
#56447=ADVANCED_FACE ( 'NONE', ( #72983 ), #11282, .F. ) ;
#56449=CARTESIAN_POINT ( 'NONE',  ( 11.66925334628632882, -11.71459661697925903, 32.44059661609676937 ) ) ;
#56450=EDGE_CURVE ( 'NONE', #42680, #87653, #73007, .T. ) ;
#56451=EDGE_LOOP ( 'NONE', ( #27332, #39814, #61270, #34228 ) ) ;
#56452=DIRECTION ( 'NONE',  ( -0.000000000000000000, 0.3420201433256694901, -0.9396926207859082059 ) ) ;
#56454=LINE ( 'NONE', #77166, #16907 ) ;
#56455=DIRECTION ( 'NONE',  ( -0.000000000000000000, -0.9848077530122086864, -0.1736481776669273613 ) ) ;
#56456=CARTESIAN_POINT ( 'NONE',  ( -13.31936024510254413, -6.835583212224610072, 34.95778746994559327 ) ) ;
#56457=CARTESIAN_POINT ( 'NONE',  ( 17.20771351789003489, -8.191423895709842640, 34.95447573519442130 ) ) ;
#56458=VECTOR ( 'NONE', #7025, 1000.000000000000227 ) ;
#56459=CARTESIAN_POINT ( 'NONE',  ( 16.15384615384603251, -10.90142922262034020, 33.41473453929536674 ) ) ;
#56460=CARTESIAN_POINT ( 'NONE',  ( -6.923076923076922462, -13.53365097954675988, 30.81389545987213552 ) ) ;
#56461=CARTESIAN_POINT ( 'NONE',  ( 15.10062126103753499, -9.504002272028875709, 34.60269587691767867 ) ) ;
#56462=EDGE_CURVE ( 'NONE', #68993, #55800, #82756, .T. ) ;
#56463=CARTESIAN_POINT ( 'NONE',  ( 7.976679547917408186, -2.882268652242222728, 31.66798894389554064 ) ) ;
#56464=CARTESIAN_POINT ( 'NONE',  ( 7.846153846153723244, -2.379036618888197729, 30.90682066428292885 ) ) ;
#56466=ORIENTED_EDGE ( 'NONE', *, *, #32641, .T. ) ;
#56467=ORIENTED_EDGE ( 'NONE', *, *, #12708, .T. ) ;
#56468=CYLINDRICAL_SURFACE ( 'NONE', #35684, 0.2500000000000009437 ) ;
#56470=CARTESIAN_POINT ( 'NONE',  ( -3.007989689500821129, -2.847695495035523550, 31.58253572463339154 ) ) ;
#56471=ADVANCED_FACE ( 'NONE', ( #61230 ), #6312, .F. ) ;
#56472=LINE ( 'NONE', #85718, #26860 ) ;
#56473=EDGE_LOOP ( 'NONE', ( #57200, #20056 ) ) ;
#56474=DIRECTION ( 'NONE',  ( 0.000000000000000000, 0.6427876096865368094, 0.7660444431189802339 ) ) ;
#56475=CARTESIAN_POINT ( 'NONE',  ( -17.29984929443921970, -3.586966769969702540, 32.86292498521069660 ) ) ;
#56476=CARTESIAN_POINT ( 'NONE',  ( 8.769230769230768274, -4.098570777380720287, 33.41473453929634729 ) ) ;
#56477=EDGE_CURVE ( 'NONE', #38481, #69764, #40979, .T. ) ;
#56478=ORIENTED_EDGE ( 'NONE', *, *, #42638, .T. ) ;
#56479=CARTESIAN_POINT ( 'NONE',  ( 0.7114839798866030574, -5.852078868378310261, 34.47109172314383585 ) ) ;
#56482=CIRCLE ( 'NONE', #86732, 0.2500000000000002220 ) ;
#56483=CARTESIAN_POINT ( 'NONE',  ( 13.16113046005105325, -12.47654668319379567, 31.42292124445336654 ) ) ;
#56484=VECTOR ( 'NONE', #21593, 1000.000000000000227 ) ;
#56485=CARTESIAN_POINT ( 'NONE',  ( -16.94613263595612551, -3.338503747796866872, 32.95102852606552801 ) ) ;
#56486=DIRECTION ( 'NONE',  ( -0.000000000000000000, -0.9396926207859093161, -0.3420201433256663259 ) ) ;
#56487=CARTESIAN_POINT ( 'NONE',  ( 1.161688425708537808, -8.282780595021769443, 34.94152052738834868 ) ) ;
#56488=CARTESIAN_POINT ( 'NONE',  ( -17.93393266664992325, -12.34228464037088813, 31.77849191805839268 ) ) ;
#56489=AXIS2_PLACEMENT_3D ( 'NONE', #28798, #81978, #41419 ) ;
#56490=EDGE_LOOP ( 'NONE', ( #19921, #45147 ) ) ;
#56491=ADVANCED_FACE ( 'NONE', ( #22030 ), #54931, .F. ) ;
#56494=ADVANCED_FACE ( 'NONE', ( #61674 ), #69769, .F. ) ;
#56496=B_SPLINE_CURVE_WITH_KNOTS ( 'NONE', 3,
 ( #34296, #53231, #27547, #68095, #67207, #13146, #40628, #5508, #67650, #32976 ),
 .UNSPECIFIED., .F., .F.,
 ( 4, 2, 2, 2, 4 ),
 ( 0.000000000000000000, 0.0001954339857564080707, 0.0003908679715128161414, 0.0005863019572692241849, 0.0007817359430256322827 ),
 .UNSPECIFIED. ) ;
#56498=CARTESIAN_POINT ( 'NONE',  ( 17.14217864819909920, -4.481592998940251427, 33.73612834413965089 ) ) ;
#56499=CARTESIAN_POINT ( 'NONE',  ( 0.2115617174898697384, -12.41104346484419452, 31.60698883733904196 ) ) ;
#56500=CARTESIAN_POINT ( 'NONE',  ( 17.75002325595140817, -2.920706130388546651, 32.31842814019191223 ) ) ;
#56501=CARTESIAN_POINT ( 'NONE',  ( -7.846153846153844924, -5.180354513474913603, 36.12317359536750416 ) ) ;
#56502=EDGE_LOOP ( 'NONE', ( #2443, #601, #39368, #84757 ) ) ;
#56503=EDGE_CURVE ( 'NONE', #80445, #36228, #23553, .T. ) ;
#56505=ORIENTED_EDGE ( 'NONE', *, *, #77315, .F. ) ;
#56506=CARTESIAN_POINT ( 'NONE',  ( 12.59206416330202671, -8.586989748646452369, 34.63063291749215011 ) ) ;
#56507=VERTEX_POINT ( 'NONE', #21581 ) ;
#56508=ADVANCED_FACE ( 'NONE', ( #7637 ), #48606, .F. ) ;
#56509=CARTESIAN_POINT ( 'NONE',  ( -9.915233909823841785, -9.086856451489515152, 34.49173150075333183 ) ) ;
#56510=CARTESIAN_POINT ( 'NONE',  ( 13.51514082284903218, -4.299079248970732792, 33.91157788607253565 ) ) ;
#56513=ORIENTED_EDGE ( 'NONE', *, *, #13097, .T. ) ;
#56514=VERTEX_POINT ( 'NONE', #6737 ) ;
#56515=DIRECTION ( 'NONE',  ( 0.000000000000000000, 0.4999999999999960032, -0.8660254037844410391 ) ) ;
#56517=FACE_BOUND ( 'NONE', #29657, .T. ) ;
#56518=CARTESIAN_POINT ( 'NONE',  ( 6.857806477116147548, -4.481592998940161721, 33.73612834413957984 ) ) ;
#56519=CARTESIAN_POINT ( 'NONE',  ( -4.153846153846274980, -10.33852847137269571, 34.16647553114546554 ) ) ;
#56520=ORIENTED_EDGE ( 'NONE', *, *, #61279, .F. ) ;
#56521=CARTESIAN_POINT ( 'NONE',  ( 15.10029404569351286, -7.276987145209184327, 34.99546412871779211 ) ) ;
#56522=CARTESIAN_POINT ( 'NONE',  ( 11.47319153790521717, -6.835583212224499938, 34.95778746994557906 ) ) ;
#56523=CARTESIAN_POINT ( 'NONE',  ( 12.46153846153846168, -4.786620604624113540, 33.94971097300155094 ) ) ;
#56524=CARTESIAN_POINT ( 'NONE',  ( 0.4615384615384611200, -6.386643153685126251, 34.62446782046654192 ) ) ;
#56525=CARTESIAN_POINT ( 'NONE',  ( -16.94613126909828793, -2.541949514083464479, 30.39797389878540557 ) ) ;
#56526=ORIENTED_EDGE ( 'NONE', *, *, #48894, .T. ) ;
#56527=B_SPLINE_CURVE_WITH_KNOTS ( 'NONE', 3,
 ( #84612, #22885, #8944, #62975, #55786, #83276 ),
 .UNSPECIFIED., .F., .F.,
 ( 4, 2, 4 ),
 ( 0.000000000000000000, 0.0001954784845028902692, 0.0003909569690057805385 ),
 .UNSPECIFIED. ) ;
#56528=CARTESIAN_POINT ( 'NONE',  ( 11.53846153846153832, -3.050289026998446396, 32.03036669348365706 ) ) ;
#56529=CARTESIAN_POINT ( 'NONE',  ( 3.296024802045255164, -4.481592998940250538, 33.73612834413965089 ) ) ;
#56530=CARTESIAN_POINT ( 'NONE',  ( -8.769230769230460965, -2.506253911140614576, 30.00000000000323297 ) ) ;
#56531=CARTESIAN_POINT ( 'NONE',  ( -0.5922290646487701204, -4.684245665217972032, 34.18127051446801090 ) ) ;
#56532=B_SPLINE_CURVE_WITH_KNOTS ( 'NONE', 3,
 ( #43071, #15603, #3405, #30877, #8852, #24118, #16044, #51569, #79075, #37191 ),
 .UNSPECIFIED., .F., .F.,
 ( 4, 2, 2, 2, 4 ),
 ( 0.0007817359430256283796, 0.0009771253907249941549, 0.001172514838424359822, 0.001367904286123725489, 0.001563293733823091156 ),
 .UNSPECIFIED. ) ;
#56534=B_SPLINE_CURVE_WITH_KNOTS ( 'NONE', 3,
 ( #36903, #64366, #57624, #30588, #85106, #52525, #58060, #16632, #44091, #71572 ),
 .UNSPECIFIED., .F., .F.,
 ( 4, 2, 2, 2, 4 ),
 ( 0.0007817246256747464135, 0.0009771112852218900684, 0.001172497944769033615, 0.001367884604316177161, 0.001563271263863320925 ),
 .UNSPECIFIED. ) ;
#56535=CARTESIAN_POINT ( 'NONE',  ( 7.173076923078343548, -7.500000000000154543, 35.00000000000007105 ) ) ;
#56536=CARTESIAN_POINT ( 'NONE',  ( 17.20744877868664346, -3.816742781228458448, 33.13167719472716044 ) ) ;
#56537=CYLINDRICAL_SURFACE ( 'NONE', #66112, 0.2499999999999973355 ) ;
#56538=CARTESIAN_POINT ( 'NONE',  ( -14.30769230769242917, -3.643525952248795718, 33.31231777344771672 ) ) ;
#56539=CARTESIAN_POINT ( 'NONE',  ( 13.38461538461538680, -9.905515769479276145, 34.41647553114623292 ) ) ;
#56540=CARTESIAN_POINT ( 'NONE',  ( 2.530471976670374712, -6.717445702608402236, 34.94155399931962336 ) ) ;
#56543=VERTEX_POINT ( 'NONE', #8079 ) ;
#56544=AXIS2_PLACEMENT_3D ( 'NONE', #51507, #65930, #79010 ) ;
#56545=CARTESIAN_POINT ( 'NONE',  ( 12.52760681254089903, -2.538708090699994813, 30.37095296980875503 ) ) ;
#56546=ORIENTED_EDGE ( 'NONE', *, *, #39924, .F. ) ;
#56547=EDGE_CURVE ( 'NONE', #5737, #77395, #69468, .T. ) ;
#56548=CARTESIAN_POINT ( 'NONE',  ( -13.13456096470193302, -10.82426656108012075, 33.81400080652039009 ) ) ;
#56549=ORIENTED_EDGE ( 'NONE', *, *, #21139, .F. ) ;
#56550=CARTESIAN_POINT ( 'NONE',  ( 16.15384615384615330, -12.37446782046654192, 30.86335684631486131 ) ) ;
#56551=EDGE_CURVE ( 'NONE', #54237, #47138, #82417, .T. ) ;
#56552=CARTESIAN_POINT ( 'NONE',  ( 4.826946332874485712, -12.01397095200673881, 32.43157075238190146 ) ) ;
#56553=ORIENTED_EDGE ( 'NONE', *, *, #63724, .F. ) ;
#56554=CARTESIAN_POINT ( 'NONE',  ( 5.749976775778544713, -10.92453946501458439, 33.72985991061850086 ) ) ;
#56556=CARTESIAN_POINT ( 'NONE',  ( -5.076923076923075762, -6.435427911321262684, 35.78748833219616898 ) ) ;
#56557=CARTESIAN_POINT ( 'NONE',  ( -3.903846153846138201, -2.249999999999999112, 29.81603969181031033 ) ) ;
#56558=CARTESIAN_POINT ( 'NONE',  ( -14.98076923076781064, -7.500000000000154543, 35.00000000000007105 ) ) ;
#56559=CARTESIAN_POINT ( 'NONE',  ( -5.143006487878956534, -12.37446782046654192, 30.86335684631486487 ) ) ;
#56560=CARTESIAN_POINT ( 'NONE',  ( 11.47237812750565666, -2.721908614388770964, 31.22303859784723912 ) ) ;
#56561=CARTESIAN_POINT ( 'NONE',  ( 4.946231610255517275, -8.147922237126337563, 34.70805685702651999 ) ) ;
#56562=EDGE_CURVE ( 'NONE', #820, #77192, #43962, .T. ) ;
#56564=CARTESIAN_POINT ( 'NONE',  ( -9.692307692307812417, -3.835265460704628371, 33.15142922262033665 ) ) ;
#56565=CARTESIAN_POINT ( 'NONE',  ( -6.130690603110308778, -3.338472653186242756, 32.95098750199972670 ) ) ;
#56566=ADVANCED_FACE ( 'NONE', ( #86297 ), #52481, .F. ) ;
#56569=CARTESIAN_POINT ( 'NONE',  ( 14.30769230769231015, -2.538708090699994813, 30.37095296980875503 ) ) ;
#56570=ORIENTED_EDGE ( 'NONE', *, *, #55175, .F. ) ;
#56572=CYLINDRICAL_SURFACE ( 'NONE', #45762, 0.2500000000000009437 ) ;
#56573=DIRECTION ( 'NONE',  ( -0.000000000000000000, -0.9848077530122085754, -0.1736481776669273613 ) ) ;
#56574=CARTESIAN_POINT ( 'NONE',  ( -8.992715712954716167, -11.41268669641500466, 32.86336882939237825 ) ) ;
#56575=CARTESIAN_POINT ( 'NONE',  ( -7.596153846153909761, -7.565270445406050648, 34.75000000000000000 ) ) ;
#56576=B_SPLINE_CURVE_WITH_KNOTS ( 'NONE', 3,
 ( #48709, #14485, #41971, #36538, #63988, #69432, #7739, #85166, #23883, #24788 ),
 .UNSPECIFIED., .F., .F.,
 ( 4, 2, 2, 2, 4 ),
 ( 0.000000000000000000, 0.0001954311564186864949, 0.0003908623128373729899, 0.0005862934692560594577, 0.0007817246256747459798 ),
 .UNSPECIFIED. ) ;
#56577=CARTESIAN_POINT ( 'NONE',  ( 13.44987095589141468, -2.625532179533470512, 30.86335684631491105 ) ) ;
#56581=CARTESIAN_POINT ( 'NONE',  ( 11.53846153846153832, -8.164416787775445883, 34.95778746994557906 ) ) ;
#56582=ORIENTED_EDGE ( 'NONE', *, *, #24461, .T. ) ;
#56584=EDGE_CURVE ( 'NONE', #25408, #5324, #51127, .T. ) ;
#56585=ORIENTED_EDGE ( 'NONE', *, *, #67497, .T. ) ;
#56586=CARTESIAN_POINT ( 'NONE',  ( -16.37733107841048152, -3.562934362175799841, 33.22335522853832401 ) ) ;
#56587=CARTESIAN_POINT ( 'NONE',  ( -2.307692307691999289, -2.506253911140615021, 30.00000000000323297 ) ) ;
#56588=CARTESIAN_POINT ( 'NONE',  ( -9.019207513279360100, -2.318417181685855422, 30.59732222474233865 ) ) ;
#56589=CARTESIAN_POINT ( 'NONE',  ( 2.177545098254088707, -6.001485441113818986, 34.52039167877662607 ) ) ;
#56590=CARTESIAN_POINT ( 'NONE',  ( 17.74997677577853850, -9.356822207818511927, 34.66110646841856635 ) ) ;
#56591=ORIENTED_EDGE ( 'NONE', *, *, #70116, .T. ) ;
#56592=LINE ( 'NONE', #62447, #53514 ) ;
#56593=VERTEX_POINT ( 'NONE', #16926 ) ;
#56594=ORIENTED_EDGE ( 'NONE', *, *, #76293, .F. ) ;
#56595=B_SPLINE_CURVE_WITH_KNOTS ( 'NONE', 3,
 ( #21250, #42430, #56379, #1433, #79200, #48725, #72426, #50053, #65662, #55484 ),
 .UNSPECIFIED., .F., .F.,
 ( 4, 2, 2, 2, 4 ),
 ( 0.0007817246256747463051, 0.0009771112852218896347, 0.001172497944769032747, 0.001367884604316176077, 0.001563271263863319407 ),
 .UNSPECIFIED. ) ;
#56596=EDGE_CURVE ( 'NONE', #73377, #10767, #69826, .T. ) ;
#56597=EDGE_CURVE ( 'NONE', #17339, #39542, #25803, .T. ) ;
#56598=CARTESIAN_POINT ( 'NONE',  ( 4.376625822824220080, -12.47679350104403007, 31.42216943046555855 ) ) ;
#56599=ORIENTED_EDGE ( 'NONE', *, *, #74571, .T. ) ;
#56600=DIRECTION ( 'NONE',  ( -0.000000000000000000, -0.000000000000000000, -1.000000000000000000 ) ) ;
#56601=B_SPLINE_CURVE_WITH_KNOTS ( 'NONE', 3,
 ( #20180, #19729, #81445, #41782, #89098, #75551, #69683, #12975, #81887, #48971 ),
 .UNSPECIFIED., .F., .F.,
 ( 4, 2, 2, 2, 4 ),
 ( 0.000000000000000000, 0.0001954339857564098054, 0.0003908679715128196108, 0.0005863019572692293891, 0.0007817359430256392216 ),
 .UNSPECIFIED. ) ;
#56603=AXIS2_PLACEMENT_3D ( 'NONE', #5333, #18402, #4434 ) ;
#56604=CARTESIAN_POINT ( 'NONE',  ( -9.692307692307812417, -8.613356846316285953, 34.62446782046622218 ) ) ;
#56606=EDGE_CURVE ( 'NONE', #35354, #25404, #59243, .T. ) ;
#56607=ORIENTED_EDGE ( 'NONE', *, *, #29128, .F. ) ;
#56608=ORIENTED_EDGE ( 'NONE', *, *, #31520, .T. ) ;
#56609=CARTESIAN_POINT ( 'NONE',  ( -9.469296340694841163, -5.667800583137506010, 34.40243808032445827 ) ) ;
#56610=CARTESIAN_POINT ( 'NONE',  ( -0.4615384615384611200, -3.937682226553329556, 33.60647404775216529 ) ) ;
#56611=ORIENTED_EDGE ( 'NONE', *, *, #67558, .F. ) ;
#56612=CARTESIAN_POINT ( 'NONE',  ( 1.607394925883795844, -9.332535724633405749, 34.40230450496446224 ) ) ;
#56614=EDGE_CURVE ( 'NONE', #63009, #29939, #16057, .T. ) ;
#56616=CARTESIAN_POINT ( 'NONE',  ( -3.099977422944443894, -9.804649428959608670, 34.18742332936588468 ) ) ;
#56617=ORIENTED_EDGE ( 'NONE', *, *, #43221, .F. ) ;
#56619=CARTESIAN_POINT ( 'NONE',  ( 15.10007862765892739, -2.494641256782728966, 31.33461815524612959 ) ) ;
#56620=EDGE_LOOP ( 'NONE', ( #42496, #75777 ) ) ;
#56621=FACE_BOUND ( 'NONE', #69192, .T. ) ;
#56622=EDGE_CURVE ( 'NONE', #80708, #33767, #46185, .T. ) ;
#56623=CARTESIAN_POINT ( 'NONE',  ( 13.38461538461538680, -11.16473453929635440, 33.15142922261926373 ) ) ;
#56624=CARTESIAN_POINT ( 'NONE',  ( -18.25002322422145440, -12.45566812827425096, 31.48439005359158926 ) ) ;
#56625=CYLINDRICAL_SURFACE ( 'NONE', #71118, 0.2499999999999997502 ) ;
#56626=LINE ( 'NONE', #35467, #20156 ) ;
#56627=CARTESIAN_POINT ( 'NONE',  ( 15.00790296770613352, -2.251424796025574881, 29.88072029997477586 ) ) ;
#56628=LINE ( 'NONE', #61605, #19377 ) ;
#56629=CARTESIAN_POINT ( 'NONE',  ( 14.37294744720514572, -2.379036618887895305, 30.90682066428158592 ) ) ;
#56631=CARTESIAN_POINT ( 'NONE',  ( -11.31545018684868786, -12.15243808032446005, 31.58219941686247978 ) ) ;
#56632=CARTESIAN_POINT ( 'NONE',  ( -5.999999999999998224, -11.35647404775217417, 33.31231777344666511 ) ) ;
#56633=ORIENTED_EDGE ( 'NONE', *, *, #25983, .F. ) ;
#56634=CARTESIAN_POINT ( 'NONE',  ( 6.923076923076802558, -2.892918686052165622, 31.69288490824153470 ) ) ;
#56635=CARTESIAN_POINT ( 'NONE',  ( -14.30769230769230660, -9.058645607665452459, 34.76329471203371924 ) ) ;
#56637=DIRECTION ( 'NONE',  ( -0.000000000000000000, 1.000000000000000000, 3.491481338843133355E-15 ) ) ;
#56638=DIRECTION ( 'NONE',  ( 0.000000000000000000, 0.4999999999999985567, 0.8660254037844395958 ) ) ;
#56639=CARTESIAN_POINT ( 'NONE',  ( -4.403822897894745125, -2.318417181685854978, 30.59732222474233865 ) ) ;
#56640=FACE_BOUND ( 'NONE', #69443, .T. ) ;
#56641=CYLINDRICAL_SURFACE ( 'NONE', #53326, 0.2499999999999995559 ) ;
#56642=CARTESIAN_POINT ( 'NONE',  ( -7.846153846153844924, -4.661471528628507777, 34.16647553114623292 ) ) ;
#56643=CARTESIAN_POINT ( 'NONE',  ( -14.30769230769230660, -2.486705287966279876, 31.30864560766543647 ) ) ;
#56644=CARTESIAN_POINT ( 'NONE',  ( -7.715628407920204879, -12.70449254468099198, 30.44128974285582956 ) ) ;
#56645=CARTESIAN_POINT ( 'NONE',  ( 6.923076923076924238, -13.20930481340135110, 34.54067556320372745 ) ) ;
#56646=CARTESIAN_POINT ( 'NONE',  ( 8.769230769230768274, -1.242168528481310874, 33.36296068462461051 ) ) ;
#56649=EDGE_CURVE ( 'NONE', #33013, #10290, #78425, .T. ) ;
#56650=VERTEX_POINT ( 'NONE', #88521 ) ;
#56651=CARTESIAN_POINT ( 'NONE',  ( -9.915234651214538175, -2.308479472611653094, 30.53278059502174457 ) ) ;
#56652=CARTESIAN_POINT ( 'NONE',  ( -12.23852561744506673, -6.460100341425560444, 34.89618726649961644 ) ) ;
#56653=FACE_OUTER_BOUND ( 'NONE', #1330, .T. ) ;
#56654=FACE_OUTER_BOUND ( 'NONE', #51786, .T. ) ;
#56655=CARTESIAN_POINT ( 'NONE',  ( -16.94613126909829148, -6.413143153341451352, 34.63066358083362672 ) ) ;
#56657=CARTESIAN_POINT ( 'NONE',  ( 6.792928953345228393, -2.373036134822904319, 30.88089517874952250 ) ) ;
#56658=FACE_OUTER_BOUND ( 'NONE', #27577, .T. ) ;
#56659=CARTESIAN_POINT ( 'NONE',  ( 15.45378058238208219, -11.76359900205217635, 32.36225158514719880 ) ) ;
#56660=CARTESIAN_POINT ( 'NONE',  ( 4.153846153846460609, -2.506253911140614576, 30.00000000000323297 ) ) ;
#56662=CARTESIAN_POINT ( 'NONE',  ( -3.230769230769352962, -2.657715359629662544, 31.77849191805970364 ) ) ;
#56663=B_SPLINE_CURVE_WITH_KNOTS ( 'NONE', 3,
 ( #55748, #34153, #63391, #13440, #35485, #82355, #62936, #21522, #48997, #76476 ),
 .UNSPECIFIED., .F., .F.,
 ( 4, 2, 2, 2, 4 ),
 ( 0.0007817359430256328248, 0.0009771253907249997928, 0.001172514838424366544, 0.001367904286123733295, 0.001563293733823100263 ),
 .UNSPECIFIED. ) ;
#56664=B_SPLINE_CURVE_WITH_KNOTS ( 'NONE', 3,
 ( #38771, #44613, #18942, #11745, #72100, #66685, #53155, #80660, #86070, #37877 ),
 .UNSPECIFIED., .F., .F.,
 ( 4, 2, 2, 2, 4 ),
 ( 0.0007817246256747453293, 0.0009771112852218889842, 0.001172497944769032531, 0.001367884604316176294, 0.001563271263863319840 ),
 .UNSPECIFIED. ) ;
#56665=CARTESIAN_POINT ( 'NONE',  ( 12.71159288145191013, -2.318338780012835443, 30.59689888758630261 ) ) ;
#56666=CARTESIAN_POINT ( 'NONE',  ( 14.17754509825408960, -6.852621066184266141, 34.70813303252209181 ) ) ;
#56667=ORIENTED_EDGE ( 'NONE', *, *, #36048, .T. ) ;
#56668=CARTESIAN_POINT ( 'NONE',  ( -6.923076923076615152, -2.506253911140614576, 30.00000000000323297 ) ) ;
#56669=DIRECTION ( 'NONE',  ( -0.000000000000000000, 0.9396926207859093161, -0.3420201433256663259 ) ) ;
#56672=VECTOR ( 'NONE', #52810, 1000.000000000000000 ) ;
#56673=CARTESIAN_POINT ( 'NONE',  ( 8.992606709928951503, -2.501478030877322567, 29.88021232661721172 ) ) ;
#56675=EDGE_LOOP ( 'NONE', ( #59808, #41337 ) ) ;
#56677=CARTESIAN_POINT ( 'NONE',  ( 1.384615384615386802, -5.415277668671390821, 36.20867863119892149 ) ) ;
#56678=ORIENTED_EDGE ( 'NONE', *, *, #53585, .F. ) ;
#56679=CARTESIAN_POINT ( 'NONE',  ( 9.942253101685738059, -12.68172785388650681, 30.59649109432439218 ) ) ;
#56680=CARTESIAN_POINT ( 'NONE',  ( -4.946131269098288818, -9.804649428959608670, 34.18742332936588468 ) ) ;
#56681=ORIENTED_EDGE ( 'NONE', *, *, #77235, .F. ) ;
#56682=DIRECTION ( 'NONE',  ( 0.000000000000000000, -0.000000000000000000, -1.000000000000000000 ) ) ;
#56684=EDGE_CURVE ( 'NONE', #46285, #55965, #85941, .T. ) ;
#56685=ORIENTED_EDGE ( 'NONE', *, *, #61961, .F. ) ;
#56686=CARTESIAN_POINT ( 'NONE',  ( -13.38461538461538325, -12.78798330534102767, 29.49999999999997868 ) ) ;
#56687=CARTESIAN_POINT ( 'NONE',  ( -1.384615384615383471, -13.57706302396349152, 30.56769352161908060 ) ) ;
#56688=CARTESIAN_POINT ( 'NONE',  ( 12.68455130563185662, -11.98016756924215009, 32.48728574198911190 ) ) ;
#56689=VERTEX_POINT ( 'NONE', #54253 ) ;
#56690=ORIENTED_EDGE ( 'NONE', *, *, #1001, .F. ) ;
#56691=ORIENTED_EDGE ( 'NONE', *, *, #41393, .F. ) ;
#56692=CARTESIAN_POINT ( 'NONE',  ( -7.053767526187231240, -2.295517848115769421, 30.44137282052136939 ) ) ;
#56693=CARTESIAN_POINT ( 'NONE',  ( 17.07692307692295586, -11.94971097300221174, 32.03036669348237098 ) ) ;
#56694=EDGE_CURVE ( 'NONE', #83315, #13183, #37596, .T. ) ;
#56695=B_SPLINE_CURVE_WITH_KNOTS ( 'NONE', 3,
 ( #52508, #80897, #39906, #52945, #53397, #4327 ),
 .UNSPECIFIED., .F., .F.,
 ( 4, 2, 4 ),
 ( 0.0003909569690057824900, 0.0005862646681846072228, 0.0007815723673634320098 ),
 .UNSPECIFIED. ) ;
#56696=LINE ( 'NONE', #57138, #84074 ) ;
#56697=CARTESIAN_POINT ( 'NONE',  ( -17.32694631421604115, -6.695914987888146541, 34.68535235679833306 ) ) ;
#56698=B_SPLINE_CURVE_WITH_KNOTS ( 'NONE', 3,
 ( #79723, #23431, #86494, #72959, #3156, #80168, #85587, #25217, #72064, #57666 ),
 .UNSPECIFIED., .F., .F.,
 ( 4, 2, 2, 2, 4 ),
 ( 0.000000000000000000, 0.0001954311564186878502, 0.0003908623128373757004, 0.0005862934692560635777, 0.0007817246256747514008 ),
 .UNSPECIFIED. ) ;
#56699=VERTEX_POINT ( 'NONE', #55145 ) ;
#56700=EDGE_CURVE ( 'NONE', #79283, #273, #26355, .T. ) ;
#56701=ORIENTED_EDGE ( 'NONE', *, *, #66768, .F. ) ;
#56702=CARTESIAN_POINT ( 'NONE',  ( -1.384615384615383471, -11.11383981884818262, 36.00935417666054406 ) ) ;
#56703=ORIENTED_EDGE ( 'NONE', *, *, #74669, .T. ) ;
#56704=CARTESIAN_POINT ( 'NONE',  ( 17.14217864819909920, -5.219633306516380244, 34.19971097300157936 ) ) ;
#56705=ORIENTED_EDGE ( 'NONE', *, *, #74654, .T. ) ;
#56706=CARTESIAN_POINT ( 'NONE',  ( 3.230769230769231726, -3.886160181151819604, 36.00935417666054406 ) ) ;
#56707=CARTESIAN_POINT ( 'NONE',  ( 6.673053698855465399, -9.356822207818506598, 34.66110646841856635 ) ) ;
#56709=CARTESIAN_POINT ( 'NONE',  ( 8.096099364501986528, -8.433404298154334455, 34.66254593164985920 ) ) ;
#56710=EDGE_LOOP ( 'NONE', ( #55929, #79119, #59837, #67582 ) ) ;
#56711=CARTESIAN_POINT ( 'NONE',  ( -10.54931626438217585, -11.16473453929635440, 33.15142922261926373 ) ) ;
#56712=VERTEX_POINT ( 'NONE', #61454 ) ;
#56713=LINE ( 'NONE', #79210, #14316 ) ;
#56714=EDGE_CURVE ( 'NONE', #54514, #29911, #897, .T. ) ;
#56715=ADVANCED_FACE ( 'NONE', ( #53819 ), #33108, .F. ) ;
#56716=AXIS2_PLACEMENT_3D ( 'NONE', #73014, #44630, #2758 ) ;
#56717=CARTESIAN_POINT ( 'NONE',  ( 14.05771556364371833, -5.643011162660950042, 34.66104346484419096 ) ) ;
#56718=ORIENTED_EDGE ( 'NONE', *, *, #13712, .F. ) ;
#56719=CARTESIAN_POINT ( 'NONE',  ( 15.10007862765892206, -2.295517848115769421, 30.44137282052137294 ) ) ;
#56722=FACE_BOUND ( 'NONE', #23177, .T. ) ;
#56723=VECTOR ( 'NONE', #45054, 1000.000000000000000 ) ;
#56724=CARTESIAN_POINT ( 'NONE',  ( -8.703975629717932705, -2.379036618887895305, 30.90682066428158592 ) ) ;
#56725=CARTESIAN_POINT ( 'NONE',  ( 12.46153846153846168, -1.242168528481310874, 33.36296068462461051 ) ) ;
#56726=AXIS2_PLACEMENT_3D ( 'NONE', #32614, #31735, #73164 ) ;
#56727=CARTESIAN_POINT ( 'NONE',  ( -5.999999999999998224, -9.905515769479276145, 34.41647553114623292 ) ) ;
#56728=B_SPLINE_CURVE_WITH_KNOTS ( 'NONE', 3,
 ( #50346, #29655, #43164, #21560, #70637, #83723, #34637, #49032, #76509, #14816 ),
 .UNSPECIFIED., .F., .F.,
 ( 4, 2, 2, 2, 4 ),
 ( 0.000000000000000000, 0.0001954311564186861968, 0.0003908623128373723936, 0.0005862934692560585904, 0.0007817246256747447872 ),
 .UNSPECIFIED. ) ;
#56730=CARTESIAN_POINT ( 'NONE',  ( -5.777220458731590291, -2.847695495035524882, 31.58253572463339509 ) ) ;
#56731=CARTESIAN_POINT ( 'NONE',  ( -4.853910232829680815, -4.026326845037961455, 33.68677907613344047 ) ) ;
#56732=DIRECTION ( 'NONE',  ( -0.000000000000000000, 0.1736481776669307198, -0.9848077530122080203 ) ) ;
#56733=ORIENTED_EDGE ( 'NONE', *, *, #23340, .T. ) ;
#56734=CARTESIAN_POINT ( 'NONE',  ( -14.08491276642389245, -3.755027918224367323, 33.06320215134714857 ) ) ;
#56735=EDGE_LOOP ( 'NONE', ( #34966, #54745, #29381, #60747 ) ) ;
#56736=EDGE_LOOP ( 'NONE', ( #68503, #86964 ) ) ;
#56737=CARTESIAN_POINT ( 'NONE',  ( 14.53047184896071720, -3.755027918224367767, 33.06320215134714857 ) ) ;
#56740=CARTESIAN_POINT ( 'NONE',  ( 8.096208266067295156, -3.435999193479609914, 33.07426656108010832 ) ) ;
#56741=CARTESIAN_POINT ( 'NONE',  ( 8.769230769230768274, -8.318370150425687726, 35.83090037661290239 ) ) ;
#56742=CARTESIAN_POINT ( 'NONE',  ( -0.3954701105360223234, -11.69971097300155272, 32.46337939537588113 ) ) ;
#56743=ORIENTED_EDGE ( 'NONE', *, *, #33706, .T. ) ;
#56744=CARTESIAN_POINT ( 'NONE',  ( 13.25392391794782654, -4.809359713505814149, 33.96456829005828837 ) ) ;
#56745=CARTESIAN_POINT ( 'NONE',  ( 1.450683735617824599, -12.10708131394839704, 31.69288490824020954 ) ) ;
#56746=DIRECTION ( 'NONE',  ( -0.000000000000000000, 0.9848077530122085754, -0.1736481776669273613 ) ) ;
#56747=CARTESIAN_POINT ( 'NONE',  ( 15.48082365068268018, -12.41089969410671223, 31.60739465890703670 ) ) ;
#56748=CARTESIAN_POINT ( 'NONE',  ( -15.48076923076922995, -2.499999999999999556, 29.81609845454691765 ) ) ;
#56750=VERTEX_POINT ( 'NONE', #6965 ) ;
#56751=ORIENTED_EDGE ( 'NONE', *, *, #19049, .T. ) ;
#56752=CARTESIAN_POINT ( 'NONE',  ( -6.923076923077044142, -8.613356846316285953, 34.62446782046622218 ) ) ;
#56754=CARTESIAN_POINT ( 'NONE',  ( -10.61538461538473577, -2.657715359629662544, 31.77849191805970364 ) ) ;
#56755=CARTESIAN_POINT ( 'NONE',  ( -1.134669975237340367, -10.18230066228895758, 34.26354781536631577 ) ) ;
#56756=DIRECTION ( 'NONE',  ( -0.000000000000000000, -0.1736481776669307198, -0.9848077530122080203 ) ) ;
#56757=CARTESIAN_POINT ( 'NONE',  ( -17.20707104665477516, -12.70455904226513866, 30.44083106164009322 ) ) ;
#56758=CARTESIAN_POINT ( 'NONE',  ( -2.307692307692427391, -5.219633306517616589, 34.19971097300220464 ) ) ;
#56759=CARTESIAN_POINT ( 'NONE',  ( 8.519207531937803779, -6.695914987888146541, 34.68535235679833306 ) ) ;
#56760=VERTEX_POINT ( 'NONE', #61899 ) ;
#56761=CARTESIAN_POINT ( 'NONE',  ( 13.38461538461538680, -2.538708090699994813, 30.37095296980875503 ) ) ;
#56762=CARTESIAN_POINT ( 'NONE',  ( -2.084912766423896446, -10.81320215134717344, 33.49497208177562868 ) ) ;
#56763=ORIENTED_EDGE ( 'NONE', *, *, #38744, .T. ) ;
#56764=CARTESIAN_POINT ( 'NONE',  ( 3.007284287045283389, -12.44517049084099725, 30.48991314939691932 ) ) ;
#56765=CARTESIAN_POINT ( 'NONE',  ( -0.6844654204453112234, -4.026226216239095379, 33.68668979543632958 ) ) ;
#56766=CARTESIAN_POINT ( 'NONE',  ( -3.296852641725110722, -4.786620604624113540, 33.94971097300155805 ) ) ;
#56767=CARTESIAN_POINT ( 'NONE',  ( 0.6843180028068698295, -2.847695495035523106, 31.58253572463339154 ) ) ;
#56768=CARTESIAN_POINT ( 'NONE',  ( 10.61538461538461675, -8.564572088678739092, 35.78748833219616898 ) ) ;
#56769=CARTESIAN_POINT ( 'NONE',  ( 15.23076923076923173, -11.16473453929635440, 33.15142922261926373 ) ) ;
#56770=B_SPLINE_CURVE_WITH_KNOTS ( 'NONE', 3,
 ( #73056, #26647, #11353, #74847, #19885, #13136, #40615, #38837, #66295, #4598 ),
 .UNSPECIFIED., .F., .F.,
 ( 4, 2, 2, 2, 4 ),
 ( 0.0007817359430256392216, 0.0009771253907250078159, 0.001172514838424376302, 0.001367904286123745004, 0.001563293733823113490 ),
 .UNSPECIFIED. ) ;
#56772=ORIENTED_EDGE ( 'NONE', *, *, #32410, .T. ) ;
#56773=DIRECTION ( 'NONE',  ( -0.000000000000000000, 0.9396926207859093161, -0.3420201433256663259 ) ) ;
#56774=CARTESIAN_POINT ( 'NONE',  ( 4.284636594813102661, -10.70102852606553157, 33.91149625220312913 ) ) ;
#56776=CARTESIAN_POINT ( 'NONE',  ( -13.60754160213153163, -12.39988816332205701, 30.74660775122750778 ) ) ;
#56778=ORIENTED_EDGE ( 'NONE', *, *, #21103, .F. ) ;
#56780=CARTESIAN_POINT ( 'NONE',  ( -1.384615384615383471, -9.780366693483667717, 34.19971097300155094 ) ) ;
#56781=ORIENTED_EDGE ( 'NONE', *, *, #8101, .T. ) ;
#56782=CARTESIAN_POINT ( 'NONE',  ( 14.30769230769231015, -3.050289026998446396, 32.03036669348365706 ) ) ;
#56783=EDGE_CURVE ( 'NONE', #32856, #69537, #82606, .T. ) ;
#56785=ORIENTED_EDGE ( 'NONE', *, *, #8064, .F. ) ;
#56786=CARTESIAN_POINT ( 'NONE',  ( 7.053602361310569613, -4.299079248970732792, 33.91157788607253565 ) ) ;
#56787=CARTESIAN_POINT ( 'NONE',  ( -17.07692307692319744, -2.379036618888197285, 30.90682066428292885 ) ) ;
#56788=AXIS2_PLACEMENT_3D ( 'NONE', #80680, #47310, #74802 ) ;
#56789=CARTESIAN_POINT ( 'NONE',  ( -12.71156168575991785, -10.18141759479407327, 34.26406193332782379 ) ) ;
#56790=CARTESIAN_POINT ( 'NONE',  ( -13.31936024510254413, -12.70778746994558439, 30.41441678777536595 ) ) ;
#56792=DIRECTION ( 'NONE',  ( -0.000000000000000000, 0.6427876096865404731, -0.7660444431189771253 ) ) ;
#56794=ORIENTED_EDGE ( 'NONE', *, *, #48774, .T. ) ;
#56795=CARTESIAN_POINT ( 'NONE',  ( 2.557692307692311928, -2.499999999999999556, 29.81604066197450109 ) ) ;
#56796=CARTESIAN_POINT ( 'NONE',  ( -4.284322861962616358, -7.276988635370452485, 34.74523720219453793 ) ) ;
#56798=EDGE_CURVE ( 'NONE', #74166, #85495, #19261, .T. ) ;
#56799=CARTESIAN_POINT ( 'NONE',  ( 11.60452887181161508, -12.62096338111211757, 30.90682066428152908 ) ) ;
#56800=CARTESIAN_POINT ( 'NONE',  ( -17.32692307692307665, -2.499999999999998668, 29.75000000000000355 ) ) ;
#56801=CARTESIAN_POINT ( 'NONE',  ( 5.076923076923075762, -9.905515769479276145, 34.41647553114623292 ) ) ;
#56802=CARTESIAN_POINT ( 'NONE',  ( -11.31568186948346977, -5.827830569534417471, 34.72679350104403539 ) ) ;
#56804=EDGE_LOOP ( 'NONE', ( #1380, #330, #29755, #64436 ) ) ;
#56805=EDGE_LOOP ( 'NONE', ( #13413, #84887 ) ) ;
#56806=EDGE_CURVE ( 'NONE', #34885, #34676, #51442, .T. ) ;
#56807=FACE_BOUND ( 'NONE', #83226, .T. ) ;
#56808=EDGE_LOOP ( 'NONE', ( #16827, #24395 ) ) ;
#56810=CARTESIAN_POINT ( 'NONE',  ( 8.769230769230768274, -8.564572088678739092, 35.78748833219616898 ) ) ;
#56811=FACE_OUTER_BOUND ( 'NONE', #713, .T. ) ;
#56812=CARTESIAN_POINT ( 'NONE',  ( 13.38461538461538680, -12.10708131394839349, 31.69288490824020244 ) ) ;
#56813=ORIENTED_EDGE ( 'NONE', *, *, #87151, .T. ) ;
#56815=VERTEX_POINT ( 'NONE', #1095 ) ;
#56817=CARTESIAN_POINT ( 'NONE',  ( -10.61538461538461320, -8.973038597847269315, 34.52809138561121927 ) ) ;
#56818=ORIENTED_EDGE ( 'NONE', *, *, #13462, .F. ) ;
#56819=EDGE_CURVE ( 'NONE', #49579, #28593, #41748, .T. ) ;
#56820=B_SPLINE_CURVE_WITH_KNOTS ( 'NONE', 3,
 ( #47731, #46403, #68445, #73883, #46843, #12179, #6741, #34212, #40108, #67127 ),
 .UNSPECIFIED., .F., .F.,
 ( 4, 2, 2, 2, 4 ),
 ( 0.000000000000000000, 0.0001954339857564074473, 0.0003908679715128148945, 0.0005863019572692223418, 0.0007817359430256297891 ),
 .UNSPECIFIED. ) ;
#56821=CARTESIAN_POINT ( 'NONE',  ( 18.00000000000000000, -13.87047571288749737, 32.06866353760679544 ) ) ;
#56822=ADVANCED_FACE ( 'NONE', ( #50149 ), #650, .F. ) ;
#56823=CARTESIAN_POINT ( 'NONE',  ( -2.372962308248625529, -12.51329471203370325, 31.30864560766548976 ) ) ;
#56824=DIRECTION ( 'NONE',  ( -0.000000000000000000, -0.7660444431189791237, -0.6427876096865379196 ) ) ;
#56825=VERTEX_POINT ( 'NONE', #15059 ) ;
#56826=CYLINDRICAL_SURFACE ( 'NONE', #88894, 0.2500000000000004996 ) ;
#56828=CARTESIAN_POINT ( 'NONE',  ( 0.7114839798866037235, -11.86320923018887719, 32.19269448109604781 ) ) ;
#56830=CARTESIAN_POINT ( 'NONE',  ( 14.37376065869474751, -6.386643153685127139, 34.62446782046654192 ) ) ;
#56832=ORIENTED_EDGE ( 'NONE', *, *, #47113, .F. ) ;
#56833=ORIENTED_EDGE ( 'NONE', *, *, #41234, .T. ) ;
#56834=ORIENTED_EDGE ( 'NONE', *, *, #45799, .T. ) ;
#56835=CARTESIAN_POINT ( 'NONE',  ( -4.153846153846152411, -9.780366693483667717, 34.19971097300155094 ) ) ;
#56836=FACE_OUTER_BOUND ( 'NONE', #76203, .T. ) ;
#56837=LINE ( 'NONE', #56405, #75036 ) ;
#56838=CARTESIAN_POINT ( 'NONE',  ( -39.05038313613820122, -2.249999999999998668, 29.75000000000000355 ) ) ;
#56839=CARTESIAN_POINT ( 'NONE',  ( -6.857008572074484221, -3.513871655860379306, 32.76840700105978499 ) ) ;
#56840=FACE_BOUND ( 'NONE', #24230, .T. ) ;
#56841=CARTESIAN_POINT ( 'NONE',  ( -11.76138849736838488, -2.308479472611653094, 30.53278059502174457 ) ) ;
#56842=ORIENTED_EDGE ( 'NONE', *, *, #12406, .T. ) ;
#56844=CARTESIAN_POINT ( 'NONE',  ( -15.23076923076922995, -13.53365097954675988, 30.81389545987213552 ) ) ;
#56846=CARTESIAN_POINT ( 'NONE',  ( 4.219914504848592429, -8.973038597847269315, 34.52809138561122637 ) ) ;
#56847=CARTESIAN_POINT ( 'NONE',  ( -11.47320596718551045, -3.835265460703683349, 33.15142922261929925 ) ) ;
#56848=EDGE_LOOP ( 'NONE', ( #52852, #51285, #63698, #86986 ) ) ;
#56850=ORIENTED_EDGE ( 'NONE', *, *, #34339, .F. ) ;
#56851=FACE_BOUND ( 'NONE', #68162, .T. ) ;
#56852=LINE ( 'NONE', #52644, #34626 ) ;
#56853=CARTESIAN_POINT ( 'NONE',  ( 16.85399685940693004, -11.76352882383564769, 32.36236540154569497 ) ) ;
#56854=CARTESIAN_POINT ( 'NONE',  ( -11.53846153846165912, -11.94971097300221174, 32.03036669348237098 ) ) ;
#56855=ORIENTED_EDGE ( 'NONE', *, *, #81824, .F. ) ;
#56856=B_SPLINE_CURVE_WITH_KNOTS ( 'NONE', 3,
 ( #82857, #76533, #40978, #40545, #27462, #83297, #68442, #7636, #68879, #21580 ),
 .UNSPECIFIED., .F., .F.,
 ( 4, 2, 2, 2, 4 ),
 ( 0.0007817246256747474977, 0.0009771112852218909357, 0.001172497944769034482, 0.001367884604316178029, 0.001563271263863321575 ),
 .UNSPECIFIED. ) ;
#56857=VECTOR ( 'NONE', #32013, 1000.000000000000000 ) ;
#56858=CYLINDRICAL_SURFACE ( 'NONE', #3326, 0.2499999999999973355 ) ;
#56859=CARTESIAN_POINT ( 'NONE',  ( 5.326923076923137934, -7.434744429011176159, 34.75000000000000711 ) ) ;
#56860=DIRECTION ( 'NONE',  ( -0.000000000000000000, -0.9848077530122086864, -0.1736481776669273613 ) ) ;
#56861=CARTESIAN_POINT ( 'NONE',  ( -4.946132635956127288, -5.496552790871117367, 34.60292014791297532 ) ) ;
#56862=ORIENTED_EDGE ( 'NONE', *, *, #72584, .T. ) ;
#56863=CARTESIAN_POINT ( 'NONE',  ( -9.942284436356285227, -2.920706130388546651, 32.31842814019191223 ) ) ;
#56864=ORIENTED_EDGE ( 'NONE', *, *, #62429, .T. ) ;
#56865=CARTESIAN_POINT ( 'NONE',  ( 16.85343813319912698, -10.81261337010820256, 33.49550067578627477 ) ) ;
#56867=CARTESIAN_POINT ( 'NONE',  ( 9.692307692307695177, -3.513871655860378418, 32.76840700105978499 ) ) ;
#56868=DIRECTION ( 'NONE',  ( -0.000000000000000000, 0.5000000000000011102, -0.8660254037844381525 ) ) ;
#56869=DIRECTION ( 'NONE',  ( -0.000000000000000000, -0.6427876096865404731, -0.7660444431189771253 ) ) ;
#56870=EDGE_CURVE ( 'NONE', #36685, #83058, #48831, .T. ) ;
#56871=DIRECTION ( 'NONE',  ( 0.000000000000000000, 1.000000000000000000, 0.000000000000000000 ) ) ;
#56872=FACE_OUTER_BOUND ( 'NONE', #68047, .T. ) ;
#56877=CYLINDRICAL_SURFACE ( 'NONE', #54844, 0.2500000000000004996 ) ;
#56878=CARTESIAN_POINT ( 'NONE',  ( -9.442362282929648742, -11.56426240980093745, 33.07394671870546432 ) ) ;
#56879=EDGE_LOOP ( 'NONE', ( #87920, #61686 ) ) ;
#56880=VERTEX_POINT ( 'NONE', #29465 ) ;
#56881=VERTEX_POINT ( 'NONE', #42532 ) ;
#56882=CARTESIAN_POINT ( 'NONE',  ( 16.82694634598072625, -4.943428324936578910, 34.04746400365624481 ) ) ;
#56883=CARTESIAN_POINT ( 'NONE',  ( 3.164685819813350065, -9.780366693483667717, 34.19971097300155805 ) ) ;
#56885=VECTOR ( 'NONE', #40954, 1000.000000000000227 ) ;
#56888=CARTESIAN_POINT ( 'NONE',  ( -13.38461538461550759, -6.835583212225970762, 34.95778746994575670 ) ) ;
#56889=LINE ( 'NONE', #15922, #81627 ) ;
#56890=CARTESIAN_POINT ( 'NONE',  ( 13.63461538461540457, -2.249999999999999112, 29.81603969181030322 ) ) ;
#56892=DIRECTION ( 'NONE',  ( -0.000000000000000000, -0.5000000000000009992, -0.8660254037844380415 ) ) ;
#56893=CARTESIAN_POINT ( 'NONE',  ( 2.084766090176160436, -3.586966769969700763, 32.86292498521069660 ) ) ;
#56896=ORIENTED_EDGE ( 'NONE', *, *, #46647, .T. ) ;
#56897=B_SPLINE_CURVE_WITH_KNOTS ( 'NONE', 3,
 ( #50775, #23318, #23754, #78261, #3927, #57109, #43593, #63865, #17460, #29649 ),
 .UNSPECIFIED., .F., .F.,
 ( 4, 2, 2, 2, 4 ),
 ( 0.0007817246256747457630, 0.0009771112852218887673, 0.001172497944769031880, 0.001367884604316174993, 0.001563271263863318106 ),
 .UNSPECIFIED. ) ;
#56898=CARTESIAN_POINT ( 'NONE',  ( -17.20707104665477516, -2.647304123082328875, 31.75400227202885262 ) ) ;
#56900=CARTESIAN_POINT ( 'NONE',  ( 3.453782074862625340, -10.77377354290276301, 33.85451476688484718 ) ) ;
#56901=DIRECTION ( 'NONE',  ( 0.000000000000000000, 0.9848077530122072432, 0.1736481776669354937 ) ) ;
#56902=ORIENTED_EDGE ( 'NONE', *, *, #9095, .T. ) ;
#56903=B_SPLINE_CURVE_WITH_KNOTS ( 'NONE', 3,
 ( #70087, #47603, #2504, #84503, #22781, #85383, #79065, #8842, #50691, #23668 ),
 .UNSPECIFIED., .F., .F.,
 ( 4, 2, 2, 2, 4 ),
 ( 0.000000000000000000, 0.0001954339857564063360, 0.0003908679715128126719, 0.0005863019572692189808, 0.0007817359430256253438 ),
 .UNSPECIFIED. ) ;
#56904=EDGE_CURVE ( 'NONE', #13379, #76411, #21418, .T. ) ;
#56905=CARTESIAN_POINT ( 'NONE',  ( -5.999999999999998224, -1.367168528481310208, 33.57946703557072254 ) ) ;
#56906=CARTESIAN_POINT ( 'NONE',  ( -12.33070004352569704, -7.277220443632450575, 34.74524770363009196 ) ) ;
#56907=CARTESIAN_POINT ( 'NONE',  ( -8.899378738962465007, -9.504002272028875709, 34.60269587691767867 ) ) ;
#56908=VECTOR ( 'NONE', #32905, 1000.000000000000227 ) ;
#56909=ORIENTED_EDGE ( 'NONE', *, *, #16212, .F. ) ;
#56910=ADVANCED_FACE ( 'NONE', ( #71755 ), #10514, .F. ) ;
#56911=CARTESIAN_POINT ( 'NONE',  ( -13.51530685128294529, -9.804603061927743113, 34.18744698557895845 ) ) ;
#56912=EDGE_LOOP ( 'NONE', ( #8627, #41886, #40461, #10549 ) ) ;
#56913=B_SPLINE_CURVE_WITH_KNOTS ( 'NONE', 3,
 ( #27767, #82284, #19683, #75511, #21457, #47146, #26888, #54346, #40849, #55675 ),
 .UNSPECIFIED., .F., .F.,
 ( 4, 2, 2, 2, 4 ),
 ( 0.000000000000000000, 0.0001954339857564093175, 0.0003908679715128186350, 0.0005863019572692279796, 0.0007817359430256372700 ),
 .UNSPECIFIED. ) ;
#56914=CARTESIAN_POINT ( 'NONE',  ( 10.74617642320940369, -8.147973898785416225, 34.70805048591653730 ) ) ;
#56915=ADVANCED_FACE ( 'NONE', ( #58687 ), #37982, .F. ) ;
#56916=DIRECTION ( 'NONE',  ( -0.000000000000000000, -0.7660444431189791237, -0.6427876096865379196 ) ) ;
#56917=CYLINDRICAL_SURFACE ( 'NONE', #28662, 0.2499999999999997502 ) ;
#56918=EDGE_CURVE ( 'NONE', #61846, #33850, #37421, .T. ) ;
#56920=CARTESIAN_POINT ( 'NONE',  ( -9.692307692307691624, -8.164416787775445883, 34.95778746994557906 ) ) ;
#56921=CARTESIAN_POINT ( 'NONE',  ( 9.692307692307695177, -2.499999999999998668, 29.75000000000001421 ) ) ;
#56922=ORIENTED_EDGE ( 'NONE', *, *, #82986, .F. ) ;
#56923=ORIENTED_EDGE ( 'NONE', *, *, #34856, .F. ) ;
#56924=ORIENTED_EDGE ( 'NONE', *, *, #36461, .F. ) ;
#56925=EDGE_CURVE ( 'NONE', #50406, #59796, #57938, .T. ) ;
#56926=FACE_OUTER_BOUND ( 'NONE', #72197, .T. ) ;
#56927=CARTESIAN_POINT ( 'NONE',  ( 13.63456090296352841, -10.05730279482229683, 34.04704008940765902 ) ) ;
#56928=B_SPLINE_CURVE_WITH_KNOTS ( 'NONE', 3,
 ( #39632, #13029, #33308, #40947, #60766, #6280, #26550, #33745, #26991, #54449 ),
 .UNSPECIFIED., .F., .F.,
 ( 4, 2, 2, 2, 4 ),
 ( 0.000000000000000000, 0.0001954339857564099680, 0.0003908679715128199361, 0.0005863019572692299312, 0.0007817359430256398721 ),
 .UNSPECIFIED. ) ;
#56929=CARTESIAN_POINT ( 'NONE',  ( 17.32697738856138869, -4.235687564193445276, 33.53795663066793509 ) ) ;
#56930=EDGE_CURVE ( 'NONE', #23513, #57142, #57804, .T. ) ;
#56931=CARTESIAN_POINT ( 'NONE',  ( 14.30769230769218581, -2.657715359629662544, 31.77849191805970364 ) ) ;
#56932=VECTOR ( 'NONE', #84827, 1000.000000000000227 ) ;
#56933=CARTESIAN_POINT ( 'NONE',  ( 7.976992176640605337, -7.277220318596961057, 34.99547417642776992 ) ) ;
#56934=ADVANCED_FACE ( 'NONE', ( #45622 ), #45172, .F. ) ;
#56935=CARTESIAN_POINT ( 'NONE',  ( -2.307692307692305711, -12.78798330534102767, 29.49999999999997868 ) ) ;
#56936=ORIENTED_EDGE ( 'NONE', *, *, #10012, .T. ) ;
#56937=ORIENTED_EDGE ( 'NONE', *, *, #56714, .F. ) ;
#56939=VERTEX_POINT ( 'NONE', #72648 ) ;
#56940=CARTESIAN_POINT ( 'NONE',  ( -5.999999999999998224, -5.415277668671390821, 36.20867863119892149 ) ) ;
#56941=ORIENTED_EDGE ( 'NONE', *, *, #79384, .T. ) ;
#56942=CARTESIAN_POINT ( 'NONE',  ( 8.835299120233207404, -8.120952969808772792, 34.71129190929999453 ) ) ;
#56943=CARTESIAN_POINT ( 'NONE',  ( 14.30769230769218581, -5.094484230521993062, 34.41647553114689373 ) ) ;
#56945=ORIENTED_EDGE ( 'NONE', *, *, #20485, .T. ) ;
#56946=ADVANCED_FACE ( 'NONE', ( #10956 ), #71312, .F. ) ;
#56947=EDGE_LOOP ( 'NONE', ( #39923, #53722, #69282, #53077 ) ) ;
#56948=CARTESIAN_POINT ( 'NONE',  ( 4.946313421718993020, -7.722926974430166069, 34.99546784045485737 ) ) ;
#56950=FACE_BOUND ( 'NONE', #78345, .T. ) ;
#56954=ADVANCED_FACE ( 'NONE', ( #4191 ), #78080, .F. ) ;
#56955=DIRECTION ( 'NONE',  ( 1.000000000000000000, 0.000000000000000000, 0.000000000000000000 ) ) ;
#56956=DIRECTION ( 'NONE',  ( -0.000000000000000000, 1.000000000000000000, -0.000000000000000000 ) ) ;
#56957=DIRECTION ( 'NONE',  ( 0.000000000000000000, -0.000000000000000000, 1.000000000000000000 ) ) ;
#56958=CARTESIAN_POINT ( 'NONE',  ( 4.153846153846032507, -11.48612834414049644, 32.76840700105863391 ) ) ;
#56959=CARTESIAN_POINT ( 'NONE',  ( -13.13456107297707121, -11.79725096376909299, 32.30694842903960762 ) ) ;
#56960=B_SPLINE_CURVE_WITH_KNOTS ( 'NONE', 3,
 ( #63482, #1784, #29274, #84225, #22501, #77445, #30578, #50833, #3987, #31474 ),
 .UNSPECIFIED., .F., .F.,
 ( 4, 2, 2, 2, 4 ),
 ( 0.0007817359430256322827, 0.0009771253907249989254, 0.001172514838424365676, 0.001367904286123732428, 0.001563293733823098962 ),
 .UNSPECIFIED. ) ;
#56961=CARTESIAN_POINT ( 'NONE',  ( 6.989144256426998325, -2.486705287966279876, 31.30864560766543647 ) ) ;
#56962=CARTESIAN_POINT ( 'NONE',  ( -7.780085495151407571, -6.386643153685127139, 34.62446782046654192 ) ) ;
#56963=CARTESIAN_POINT ( 'NONE',  ( 16.15384615384615330, -8.973038597847269315, 34.52809138561121927 ) ) ;
#56964=B_SPLINE_CURVE_WITH_KNOTS ( 'NONE', 3,
 ( #16902, #31309, #39416, #5170, #79047, #17350, #18245, #25443, #66427, #3830 ),
 .UNSPECIFIED., .F., .F.,
 ( 4, 2, 2, 2, 4 ),
 ( 0.0007817359430256333669, 0.0009771253907250056474, 0.001172514838424371098, 0.001367904286123736331, 0.001563293733823101781 ),
 .UNSPECIFIED. ) ;
#56965=CARTESIAN_POINT ( 'NONE',  ( 5.933916589044120116, -4.786620604624113540, 33.94971097300155805 ) ) ;
#56966=CARTESIAN_POINT ( 'NONE',  ( -18.06527044596078113, -6.879047030191175693, 34.71129190930000163 ) ) ;
#56967=EDGE_CURVE ( 'NONE', #74567, #58941, #70764, .T. ) ;
#56968=CIRCLE ( 'NONE', #18153, 0.2500000000000002220 ) ;
#56969=CARTESIAN_POINT ( 'NONE',  ( 6.222779541268408821, -10.11255958852956027, 34.01340905677048454 ) ) ;
#56970=CARTESIAN_POINT ( 'NONE',  ( 13.25446817517716802, -11.93770438780619259, 32.05411857736982029 ) ) ;
#56971=CARTESIAN_POINT ( 'NONE',  ( 11.53846153846153832, -4.098570777380720287, 33.41473453929634729 ) ) ;
#56972=CARTESIAN_POINT ( 'NONE',  ( 8.546365347027130355, -2.501496062324912284, 29.88072118266895671 ) ) ;
#56973=DIRECTION ( 'NONE',  ( -0.000000000000000000, 0.7660444431189791237, -0.6427876096865379196 ) ) ;
#56975=CARTESIAN_POINT ( 'NONE',  ( 13.51466281986583873, -7.723484941389743952, 34.99544897038808955 ) ) ;
#56978=EDGE_CURVE ( 'NONE', #3936, #13945, #44268, .T. ) ;
#56980=EDGE_LOOP ( 'NONE', ( #15741, #4637, #49399, #80759 ) ) ;
#56981=EDGE_CURVE ( 'NONE', #46544, #55585, #21321, .T. ) ;
#56982=CARTESIAN_POINT ( 'NONE',  ( -2.557715531913763218, -2.985938066672154445, 32.43141759479405550 ) ) ;
#56983=VERTEX_POINT ( 'NONE', #74885 ) ;
#56984=CARTESIAN_POINT ( 'NONE',  ( 15.93091993633000847, -11.24512374952581872, 33.06303171183252942 ) ) ;
#56985=CARTESIAN_POINT ( 'NONE',  ( 5.010840697562939816, -11.91647553114624181, 32.58852847137148245 ) ) ;
#56986=VECTOR ( 'NONE', #35920, 1000.000000000000000 ) ;
#56987=ORIENTED_EDGE ( 'NONE', *, *, #82044, .T. ) ;
#56988=DIRECTION ( 'NONE',  ( -1.000000000000000000, 0.000000000000000000, 0.000000000000000000 ) ) ;
#56990=CARTESIAN_POINT ( 'NONE',  ( -17.86947456176635640, -9.503571793651730104, 34.60286762892837942 ) ) ;
#56991=CARTESIAN_POINT ( 'NONE',  ( 13.60762822870878530, -2.889357225399416418, 32.26129605718031002 ) ) ;
#56992=CARTESIAN_POINT ( 'NONE',  ( 17.93391762063986050, -2.292212530054419606, 30.41441678777542634 ) ) ;
#56993=ADVANCED_FACE ( 'NONE', ( #5537 ), #46517, .F. ) ;
#56994=CARTESIAN_POINT ( 'NONE',  ( -16.15384615384615330, -9.905515769479276145, 34.41647553114623292 ) ) ;
#56995=FACE_OUTER_BOUND ( 'NONE', #53854, .T. ) ;
#56996=DIRECTION ( 'NONE',  ( 0.000000000000000000, 0.1736481776669267785, -0.9848077530122087975 ) ) ;
#56998=FACE_OUTER_BOUND ( 'NONE', #14631, .T. ) ;
#56999=FACE_OUTER_BOUND ( 'NONE', #28594, .T. ) ;
#57000=DIRECTION ( 'NONE',  ( -1.000000000000000000, -0.000000000000000000, -0.000000000000000000 ) ) ;
#57002=CARTESIAN_POINT ( 'NONE',  ( -10.55012947587177941, -5.941354392334607049, 34.76329471203374055 ) ) ;
#57003=EDGE_LOOP ( 'NONE', ( #2397, #84419, #80744, #82775 ) ) ;
#57005=CARTESIAN_POINT ( 'NONE',  ( 14.30769230769231015, -4.786620604624113540, 33.94971097300155094 ) ) ;
#57006=CARTESIAN_POINT ( 'NONE',  ( 12.21156171748986807, -8.347322224742351082, 34.93158281831414769 ) ) ;
#57007=DIRECTION ( 'NONE',  ( 1.000000000000000000, 0.000000000000000000, 0.000000000000000000 ) ) ;
#57008=CARTESIAN_POINT ( 'NONE',  ( 1.384615384615693667, -2.506253911140615021, 30.00000000000323297 ) ) ;
#57009=ADVANCED_FACE ( 'NONE', ( #54142 ), #39330, .F. ) ;
#57010=CARTESIAN_POINT ( 'NONE',  ( -3.230769230769229949, -4.786620604624113540, 33.94971097300155094 ) ) ;
#57011=VECTOR ( 'NONE', #74316, 1000.000000000000227 ) ;
#57012=CARTESIAN_POINT ( 'NONE',  ( 2.084207363968358706, -12.24155766932282496, 31.33739205006857986 ) ) ;
#57013=CARTESIAN_POINT ( 'NONE',  ( 3.230769230769231726, -3.886160181151819604, 36.00935417666054406 ) ) ;
#57014=VERTEX_POINT ( 'NONE', #47392 ) ;
#57016=ORIENTED_EDGE ( 'NONE', *, *, #49833, .F. ) ;
#57017=VECTOR ( 'NONE', #42728, 1000.000000000000227 ) ;
#57018=CARTESIAN_POINT ( 'NONE',  ( -11.28851612908349722, -11.56426240980093745, 33.07394671870546432 ) ) ;
#57019=CARTESIAN_POINT ( 'NONE',  ( -4.023320452082588261, -3.285477652293412820, 32.44071101563363158 ) ) ;
#57020=FACE_OUTER_BOUND ( 'NONE', #22581, .T. ) ;
#57022=CARTESIAN_POINT ( 'NONE',  ( 18.00000000000000000, -4.786620604624113540, 33.94971097300155094 ) ) ;
#57023=B_SPLINE_CURVE_WITH_KNOTS ( 'NONE', 3,
 ( #56059, #8771, #42555, #35801, #15969, #21388, #8325, #83992, #23158, #63256 ),
 .UNSPECIFIED., .F., .F.,
 ( 4, 2, 2, 2, 4 ),
 ( 0.0007817359430256219828, 0.0009771253907249863487, 0.001172514838424350498, 0.001367904286123714647, 0.001563293733823079013 ),
 .UNSPECIFIED. ) ;
#57024=ORIENTED_EDGE ( 'NONE', *, *, #51926, .T. ) ;
#57025=DIRECTION ( 'NONE',  ( -0.000000000000000000, -0.5000000000000009992, -0.8660254037844380415 ) ) ;
#57026=ORIENTED_EDGE ( 'NONE', *, *, #36522, .F. ) ;
#57030=CARTESIAN_POINT ( 'NONE',  ( 4.284636594813102661, -12.35292014791297710, 31.75344720912887198 ) ) ;
#57032=CARTESIAN_POINT ( 'NONE',  ( 16.15384615384603251, -12.46129190930018460, 30.37095296980731973 ) ) ;
#57033=LINE ( 'NONE', #22806, #30748 ) ;
#57034=ADVANCED_FACE ( 'NONE', ( #81639 ), #32115, .F. ) ;
#57035=CARTESIAN_POINT ( 'NONE',  ( 2.057692307692299938, -2.499999999999999556, 29.81609845454692120 ) ) ;
#57036=EDGE_CURVE ( 'NONE', #83747, #4121, #33005, .T. ) ;
#57037=CARTESIAN_POINT ( 'NONE',  ( -16.15384615384615330, -5.471508081941601098, 34.59228464037088457 ) ) ;
#57039=ORIENTED_EDGE ( 'NONE', *, *, #69892, .F. ) ;
#57040=ORIENTED_EDGE ( 'NONE', *, *, #15651, .F. ) ;
#57043=CARTESIAN_POINT ( 'NONE',  ( -14.37301632049661571, -7.749976730030849303, 34.74374725381503737 ) ) ;
#57044=CARTESIAN_POINT ( 'NONE',  ( -14.24162497434223162, -2.292212530054420494, 30.41441678777542990 ) ) ;
#57045=VERTEX_POINT ( 'NONE', #33451 ) ;
#57046=EDGE_CURVE ( 'NONE', #57920, #76633, #40755, .T. ) ;
#57048=CARTESIAN_POINT ( 'NONE',  ( 6.249945518348142492, -12.43552623307873972, 30.55307653245132826 ) ) ;
#57049=CARTESIAN_POINT ( 'NONE',  ( -0.2385256174450662570, -9.172514111537584114, 34.72667873470787470 ) ) ;
#57050=ORIENTED_EDGE ( 'NONE', *, *, #55798, .T. ) ;
#57051=DIRECTION ( 'NONE',  ( 0.000000000000000000, 0.9396926207859126468, -0.3420201433256571111 ) ) ;
#57054=B_SPLINE_CURVE_WITH_KNOTS ( 'NONE', 3,
 ( #12304, #38444, #11870, #4206, #19498, #45639, #81213, #66804, #51938, #66357 ),
 .UNSPECIFIED., .F., .F.,
 ( 4, 2, 2, 2, 4 ),
 ( 0.0007817246256747484735, 0.0009771112852218922368, 0.001172497944769036217, 0.001367884604316180197, 0.001563271263863323960 ),
 .UNSPECIFIED. ) ;
#57055=ORIENTED_EDGE ( 'NONE', *, *, #35727, .F. ) ;
#57056=FACE_BOUND ( 'NONE', #88172, .T. ) ;
#57057=CARTESIAN_POINT ( 'NONE',  ( 11.40831432902331954, -5.195881422630166391, 34.18770438780619259 ) ) ;
#57058=FACE_OUTER_BOUND ( 'NONE', #64317, .T. ) ;
#57059=CARTESIAN_POINT ( 'NONE',  ( -18.00000000000012079, -2.657715359629662988, 31.77849191805970364 ) ) ;
#57060=CARTESIAN_POINT ( 'NONE',  ( -6.673076923076987299, -7.565270445406050648, 34.75000000000000000 ) ) ;
#57061=CARTESIAN_POINT ( 'NONE',  ( -10.68065461594093435, -5.941354392334499579, 34.76329471203369792 ) ) ;
#57062=AXIS2_PLACEMENT_3D ( 'NONE', #10163, #30864, #58334 ) ;
#57063=CARTESIAN_POINT ( 'NONE',  ( -0.5916864312701598516, -12.50552854090298993, 31.33409797877408920 ) ) ;
#57064=CARTESIAN_POINT ( 'NONE',  ( -16.15384615384627409, -9.442884908241554243, 34.35708131394783038 ) ) ;
#57066=DIRECTION ( 'NONE',  ( 0.000000000000000000, 0.6427876096865373645, -0.7660444431189797898 ) ) ;
#57067=CARTESIAN_POINT ( 'NONE',  ( -16.82686865700962286, -6.523592122091590895, 34.90882529074906415 ) ) ;
#57068=ORIENTED_EDGE ( 'NONE', *, *, #40039, .T. ) ;
#57069=AXIS2_PLACEMENT_3D ( 'NONE', #75278, #19000, #26199 ) ;
#57071=CARTESIAN_POINT ( 'NONE',  ( 10.36540788444226102, -6.567427716900048118, 34.66269422305636283 ) ) ;
#57072=CARTESIAN_POINT ( 'NONE',  ( -3.930834802233304170, -2.554770724473668153, 30.48948780036025852 ) ) ;
#57073=LINE ( 'NONE', #71467, #50490 ) ;
#57074=CARTESIAN_POINT ( 'NONE',  ( -16.15384615384627409, -12.46129190930018460, 30.37095296980731973 ) ) ;
#57075=CARTESIAN_POINT ( 'NONE',  ( -8.899922235898330314, -5.582088688514999397, 34.36776431015576350 ) ) ;
#57076=FACE_BOUND ( 'NONE', #34804, .T. ) ;
#57077=CARTESIAN_POINT ( 'NONE',  ( 6.856994543716788293, -3.937682226553329556, 33.60647404775217240 ) ) ;
#57078=DIRECTION ( 'NONE',  ( -0.000000000000000000, 1.000000000000000000, 3.491481338843133355E-15 ) ) ;
#57080=CARTESIAN_POINT ( 'NONE',  ( -18.22348492456433178, -8.539481045369599954, 34.89627647299170832 ) ) ;
#57081=CARTESIAN_POINT ( 'NONE',  ( 20.99999999999999645, -12.75000000000000178, 29.75000000000000355 ) ) ;
#57082=CARTESIAN_POINT ( 'NONE',  ( -15.23076923076935074, -6.879047030192662504, 34.71129190930017927 ) ) ;
#57085=EDGE_LOOP ( 'NONE', ( #64169, #2043, #2688, #5768 ) ) ;
#57086=EDGE_CURVE ( 'NONE', #19283, #33070, #73977, .T. ) ;
#57087=EDGE_LOOP ( 'NONE', ( #63883, #62040, #59478, #1821 ) ) ;
#57088=CARTESIAN_POINT ( 'NONE',  ( -9.561781990544126586, -11.93748526763465279, 32.05452791011430946 ) ) ;
#57090=CARTESIAN_POINT ( 'NONE',  ( -7.780959864370489143, -2.506253911140448487, 29.99999999999988631 ) ) ;
#57092=CARTESIAN_POINT ( 'NONE',  ( -4.023055712879200385, -2.845873456487966635, 32.17976146951972538 ) ) ;
#57094=CARTESIAN_POINT ( 'NONE',  ( -7.846153846153844924, -9.819645486525091727, 36.12317359536749706 ) ) ;
#57095=CYLINDRICAL_SURFACE ( 'NONE', #84884, 0.2499999999999986955 ) ;
#57096=EDGE_CURVE ( 'NONE', #33571, #25404, #14953, .T. ) ;
#57097=CARTESIAN_POINT ( 'NONE',  ( 3.453782074862627560, -4.026326845037965008, 33.68677907613344047 ) ) ;
#57098=CARTESIAN_POINT ( 'NONE',  ( 17.75000000000000000, -2.499999999999998668, 29.75000000000000355 ) ) ;
#57099=CARTESIAN_POINT ( 'NONE',  ( 2.307692307692187583, -3.835265460704628371, 33.15142922262033665 ) ) ;
#57102=DIRECTION ( 'NONE',  ( 0.000000000000000000, 0.9396926207859126468, -0.3420201433256571111 ) ) ;
#57103=EDGE_CURVE ( 'NONE', #23768, #22173, #3591, .T. ) ;
#57104=B_SPLINE_CURVE_WITH_KNOTS ( 'NONE', 3,
 ( #78700, #58408, #16996, #85457, #66060, #30071, #37706, #23740, #23303, #50761 ),
 .UNSPECIFIED., .F., .F.,
 ( 4, 2, 2, 2, 4 ),
 ( 0.000000000000000000, 0.0001954339857564072033, 0.0003908679715128144066, 0.0005863019572692215828, 0.0007817359430256288133 ),
 .UNSPECIFIED. ) ;
#57105=B_SPLINE_CURVE_WITH_KNOTS ( 'NONE', 3,
 ( #12764, #74467, #33920, #13652, #19084, #6020, #66824, #61380, #68596, #13214 ),
 .UNSPECIFIED., .F., .F.,
 ( 4, 2, 2, 2, 4 ),
 ( 0.0007817246256747473893, 0.0009771112852218900684, 0.001172497944769032747, 0.001367884604316175643, 0.001563271263863318323 ),
 .UNSPECIFIED. ) ;
#57106=DIRECTION ( 'NONE',  ( 0.000000000000000000, 1.000000000000000000, 0.000000000000000000 ) ) ;
#57107=ORIENTED_EDGE ( 'NONE', *, *, #15552, .F. ) ;
#57108=CARTESIAN_POINT ( 'NONE',  ( -8.519230769230768274, -2.499999999999998668, 29.75000000000000355 ) ) ;
#57109=CARTESIAN_POINT ( 'NONE',  ( -5.749945580086543551, -2.544122305571457687, 31.48381861865059150 ) ) ;
#57110=AXIS2_PLACEMENT_3D ( 'NONE', #78365, #42329, #56272 ) ;
#57112=B_SPLINE_CURVE_WITH_KNOTS ( 'NONE', 3,
 ( #72933, #11689, #31955, #81483, #19770, #4931, #59419, #86925, #67517, #13012 ),
 .UNSPECIFIED., .F., .F.,
 ( 4, 2, 2, 2, 4 ),
 ( 0.0007817359527651101701, 0.0009771254036996489256, 0.001172514854634187790, 0.001367904305568726653, 0.001563293756503265517 ),
 .UNSPECIFIED. ) ;
#57113=DIRECTION ( 'NONE',  ( -0.000000000000000000, 0.8660254037844397068, -0.4999999999999978906 ) ) ;
#57115=VERTEX_POINT ( 'NONE', #59878 ) ;
#57116=CARTESIAN_POINT ( 'NONE',  ( 15.23076923076923173, -12.78798330534102945, 29.74999999999997868 ) ) ;
#57117=CARTESIAN_POINT ( 'NONE',  ( 22.75000000000000000, -7.500000000000000000, 29.75000000000000355 ) ) ;
#57118=ORIENTED_EDGE ( 'NONE', *, *, #54293, .T. ) ;
#57119=CARTESIAN_POINT ( 'NONE',  ( 7.173022441425065843, -3.712312575010499494, 33.01462480002815170 ) ) ;
#57120=CARTESIAN_POINT ( 'NONE',  ( -13.38461538461538325, -9.780366693483667717, 34.19971097300155094 ) ) ;
#57121=EDGE_CURVE ( 'NONE', #16656, #59690, #79399, .T. ) ;
#57122=ORIENTED_EDGE ( 'NONE', *, *, #59251, .F. ) ;
#57123=CARTESIAN_POINT ( 'NONE',  ( -5.326899807865431491, -11.28823185664190376, 33.01397839955799896 ) ) ;
#57124=CARTESIAN_POINT ( 'NONE',  ( -17.07692307692319744, -3.300289026999228437, 32.46337939537709616 ) ) ;
#57125=EDGE_LOOP ( 'NONE', ( #39810, #14718, #42198, #69399 ) ) ;
#57126=CARTESIAN_POINT ( 'NONE',  ( -11.66860874789976066, -4.460286881179644780, 33.72017969459903242 ) ) ;
#57127=EDGE_CURVE ( 'NONE', #13990, #44873, #45018, .T. ) ;
#57128=EDGE_CURVE ( 'NONE', #82159, #56176, #79379, .T. ) ;
#57129=DIRECTION ( 'NONE',  ( 0.000000000000000000, 0.000000000000000000, 1.000000000000000000 ) ) ;
#57130=CARTESIAN_POINT ( 'NONE',  ( 12.59206389977210705, -12.15418822224088657, 32.17964115625579069 ) ) ;
#57131=ORIENTED_EDGE ( 'NONE', *, *, #4646, .T. ) ;
#57132=ORIENTED_EDGE ( 'NONE', *, *, #73926, .T. ) ;
#57133=EDGE_CURVE ( 'NONE', #20836, #23257, #6340, .T. ) ;
#57134=VERTEX_POINT ( 'NONE', #72948 ) ;
#57135=AXIS2_PLACEMENT_3D ( 'NONE', #7220, #81555, #13967 ) ;
#57136=CARTESIAN_POINT ( 'NONE',  ( 3.453782074862624896, -2.308499170217967134, 30.53291367094873721 ) ) ;
#57137=CARTESIAN_POINT ( 'NONE',  ( -5.869474561766354626, -5.915461855592777596, 34.75538340440931506 ) ) ;
#57138=CARTESIAN_POINT ( 'NONE',  ( 18.00000000000000000, -5.415277668671390821, 36.20867863119892149 ) ) ;
#57139=B_SPLINE_CURVE_WITH_KNOTS ( 'NONE', 3,
 ( #36952, #84729, #57676, #16252, #23440, #43716, #50895, #78383, #16687, #44142 ),
 .UNSPECIFIED., .F., .F.,
 ( 4, 2, 2, 2, 4 ),
 ( 0.000000000000000000, 0.0001954311564186868202, 0.0003908623128373736404, 0.0005862934692560604335, 0.0007817246256747472808 ),
 .UNSPECIFIED. ) ;
#57140=CARTESIAN_POINT ( 'NONE',  ( 3.007842271862380290, -10.01117774369187252, 34.36070679894347535 ) ) ;
#57141=B_SPLINE_CURVE_WITH_KNOTS ( 'NONE', 3,
 ( #77508, #9489, #1851, #29334, #16688, #56789, #22565, #23007, #77951, #16253 ),
 .UNSPECIFIED., .F., .F.,
 ( 4, 2, 2, 2, 4 ),
 ( 0.000000000000000000, 0.0001954311564186863323, 0.0003908623128373726646, 0.0005862934692560590241, 0.0007817246256747453293 ),
 .UNSPECIFIED. ) ;
#57142=VERTEX_POINT ( 'NONE', #11250 ) ;
#57144=ORIENTED_EDGE ( 'NONE', *, *, #46527, .F. ) ;
#57146=ORIENTED_EDGE ( 'NONE', *, *, #10210, .F. ) ;
#57147=EDGE_CURVE ( 'NONE', #58077, #6775, #46050, .T. ) ;
#57148=CARTESIAN_POINT ( 'NONE',  ( 17.14299142792551578, -4.786620604624113540, 33.94971097300155805 ) ) ;
#57149=ORIENTED_EDGE ( 'NONE', *, *, #2045, .T. ) ;
#57150=CARTESIAN_POINT ( 'NONE',  ( -17.86920819217521483, -3.062576670634121534, 32.05464942895958558 ) ) ;
#57153=ORIENTED_EDGE ( 'NONE', *, *, #76457, .T. ) ;
#57154=CARTESIAN_POINT ( 'NONE',  ( -12.33074665371367651, -4.809403383903225304, 33.96459661697924304 ) ) ;
#57156=ADVANCED_FACE ( 'NONE', ( #3144 ), #39181, .F. ) ;
#57157=CARTESIAN_POINT ( 'NONE',  ( 4.376857505459002873, -4.887748414852789658, 34.01359900205216746 ) ) ;
#57158=AXIS2_PLACEMENT_3D ( 'NONE', #132, #49644, #69473 ) ;
#57159=CARTESIAN_POINT ( 'NONE',  ( -11.53846153846153655, -3.050289026998446396, 32.03036669348365706 ) ) ;
#57160=ORIENTED_EDGE ( 'NONE', *, *, #23330, .F. ) ;
#57161=CARTESIAN_POINT ( 'NONE',  ( 15.48071474911737333, -3.202959910592335646, 32.30730279482227019 ) ) ;
#57163=EDGE_CURVE ( 'NONE', #77307, #9234, #30620, .T. ) ;
#57164=CYLINDRICAL_SURFACE ( 'NONE', #3681, 0.2500000000000008882 ) ;
#57165=AXIS2_PLACEMENT_3D ( 'NONE', #50829, #77877, #17964 ) ;
#57166=FACE_BOUND ( 'NONE', #25219, .T. ) ;
#57167=CARTESIAN_POINT ( 'NONE',  ( 8.069166690247241647, -12.38742843783360748, 31.66772728687926985 ) ) ;
#57168=CARTESIAN_POINT ( 'NONE',  ( -2.307692307692305711, -12.37446782046654192, 30.86335684631486131 ) ) ;
#57169=CARTESIAN_POINT ( 'NONE',  ( 8.703147358274884837, -2.538708090699994813, 30.37095296980875148 ) ) ;
#57170=CARTESIAN_POINT ( 'NONE',  ( 12.23861150263161157, -3.395401636524185474, 33.02366814457250399 ) ) ;
#57171=CARTESIAN_POINT ( 'NONE',  ( 6.856993512121042578, -11.69971097300155272, 32.46337939537587403 ) ) ;
#57172=CARTESIAN_POINT ( 'NONE',  ( 11.28848480751918437, -11.28823185664190376, 33.01397839955799896 ) ) ;
#57173=CARTESIAN_POINT ( 'NONE',  ( -16.21911615440246734, -2.657715359629089669, 31.77849191805834295 ) ) ;
#57174=ORIENTED_EDGE ( 'NONE', *, *, #69548, .F. ) ;
#57176=CARTESIAN_POINT ( 'NONE',  ( -5.777220458731589403, -11.89424750095246175, 32.13594075562311758 ) ) ;
#57178=EDGE_LOOP ( 'NONE', ( #32701, #11834 ) ) ;
#57179=CARTESIAN_POINT ( 'NONE',  ( 14.55763782604045353, -3.712312575010499494, 33.01462480002815170 ) ) ;
#57180=CARTESIAN_POINT ( 'NONE',  ( -5.750054481651856619, -12.22109172314383052, 31.39792113162168263 ) ) ;
#57181=EDGE_CURVE ( 'NONE', #12918, #48531, #78809, .T. ) ;
#57182=B_SPLINE_CURVE_WITH_KNOTS ( 'NONE', 3,
 ( #5908, #87454, #68926, #53643, #33384, #67611, #7237, #59953, #35595, #48652 ),
 .UNSPECIFIED., .F., .F.,
 ( 4, 2, 2, 2, 4 ),
 ( 0.000000000000000000, 0.0001954311564186864949, 0.0003908623128373729899, 0.0005862934692560594577, 0.0007817246256747459798 ),
 .UNSPECIFIED. ) ;
#57183=CARTESIAN_POINT ( 'NONE',  ( -5.934744428723973897, -6.879047030191282275, 34.71129190930002295 ) ) ;
#57184=CARTESIAN_POINT ( 'NONE',  ( 7.846153846153846700, -11.11383981884818262, 36.00935417666054406 ) ) ;
#57185=CARTESIAN_POINT ( 'NONE',  ( 1.449870524128225036, -11.06231777344671130, 33.60647404775212976 ) ) ;
#57186=CARTESIAN_POINT ( 'NONE',  ( -4.087778820496077437, -3.322132147404559976, 32.92929555188717927 ) ) ;
#57187=VERTEX_POINT ( 'NONE', #10362 ) ;
#57188=CARTESIAN_POINT ( 'NONE',  ( 11.28848479441294650, -3.436278759898153901, 33.07459398097509506 ) ) ;
#57189=CARTESIAN_POINT ( 'NONE',  ( 0.3313904918067634431, -12.70455904226513866, 30.44083106164009322 ) ) ;
#57190=CARTESIAN_POINT ( 'NONE',  ( -5.076923076923075762, -13.49023893513002648, 31.06009739812518688 ) ) ;
#57191=CARTESIAN_POINT ( 'NONE',  ( 11.53846153846153832, -12.78798330534102945, 29.74999999999997868 ) ) ;
#57192=CARTESIAN_POINT ( 'NONE',  ( -15.45363465297287142, -2.501496062324912284, 29.88072118266895671 ) ) ;
#57195=EDGE_CURVE ( 'NONE', #34806, #84581, #27568, .T. ) ;
#57196=ORIENTED_EDGE ( 'NONE', *, *, #22945, .F. ) ;
#57197=VECTOR ( 'NONE', #24732, 1000.000000000000114 ) ;
#57198=CARTESIAN_POINT ( 'NONE',  ( -9.692307692307812417, -12.46129190930018460, 30.37095296980731973 ) ) ;
#57199=EDGE_CURVE ( 'NONE', #51136, #33889, #50341, .T. ) ;
#57200=ORIENTED_EDGE ( 'NONE', *, *, #1976, .F. ) ;
#57201=CARTESIAN_POINT ( 'NONE',  ( -6.989160334032804123, -2.538708090699994813, 30.37095296980875148 ) ) ;
#57202=CARTESIAN_POINT ( 'NONE',  ( 18.06525557127601900, -6.026961402152790193, 34.52809138561124769 ) ) ;
#57203=DIRECTION ( 'NONE',  ( 0.000000000000000000, -6.938893903907222067E-15, 1.000000000000000000 ) ) ;
#57204=CARTESIAN_POINT ( 'NONE',  ( 2.438482748659258625, -9.929761469519744921, 34.40412654351204225 ) ) ;
#57208=AXIS2_PLACEMENT_3D ( 'NONE', #45003, #18000, #25193 ) ;
#57209=CYLINDRICAL_SURFACE ( 'NONE', #86080, 0.2500000000000012212 ) ;
#57210=CARTESIAN_POINT ( 'NONE',  ( -2.177166605928742005, -10.88167719472716399, 33.43325721877153711 ) ) ;
#57211=EDGE_LOOP ( 'NONE', ( #81666, #54530, #29549, #40530 ) ) ;
#57212=CARTESIAN_POINT ( 'NONE',  ( -13.51476259405360558, -11.47017969459904130, 32.78971311882034456 ) ) ;
#57213=CARTESIAN_POINT ( 'NONE',  ( -9.692307692307691624, -8.564572088678739092, 35.78748833219616898 ) ) ;
#57214=CARTESIAN_POINT ( 'NONE',  ( 11.40831432902331954, -4.460286881179643004, 33.72017969459903242 ) ) ;
#57216=ADVANCED_FACE ( 'NONE', ( #67232 ), #88406, .F. ) ;
#57217=VECTOR ( 'NONE', #26887, 1000.000000000000114 ) ;
#57218=EDGE_CURVE ( 'NONE', #17825, #26012, #34237, .T. ) ;
#57219=CARTESIAN_POINT ( 'NONE',  ( -3.480769230769229505, -7.433932668274255029, 35.00000000000000711 ) ) ;
#57220=CARTESIAN_POINT ( 'NONE',  ( 15.48082354240754555, -11.28795663066794575, 33.01431243580653785 ) ) ;
#57222=VERTEX_POINT ( 'NONE', #6418 ) ;
#57223=CARTESIAN_POINT ( 'NONE',  ( -3.007989561791163613, -6.717445702608402236, 34.94155399931962336 ) ) ;
#57224=CARTESIAN_POINT ( 'NONE',  ( 4.153846153846154188, -10.67929555188718282, 33.92786785259544047 ) ) ;
#57226=CARTESIAN_POINT ( 'NONE',  ( -16.02305571287920216, -11.37503395064541678, 33.29242100308974983 ) ) ;
#57227=CARTESIAN_POINT ( 'NONE',  ( 2.438217745925951530, -12.15418822224088657, 32.17964115625579069 ) ) ;
#57228=ORIENTED_EDGE ( 'NONE', *, *, #69144, .T. ) ;
#57230=DIRECTION ( 'NONE',  ( -0.000000000000000000, 0.1736481776669307198, -0.9848077530122080203 ) ) ;
#57231=EDGE_CURVE ( 'NONE', #88055, #26451, #61779, .T. ) ;
#57232=ORIENTED_EDGE ( 'NONE', *, *, #23734, .T. ) ;
#57233=DIRECTION ( 'NONE',  ( -0.000000000000000000, -0.9848077530122085754, -0.1736481776669273613 ) ) ;
#57235=VERTEX_POINT ( 'NONE', #81632 ) ;
#57237=CARTESIAN_POINT ( 'NONE',  ( 17.99999999999987566, -6.879047030192662504, 34.71129190930017927 ) ) ;
#57238=EDGE_CURVE ( 'NONE', #22716, #81377, #66465, .T. ) ;
#57239=EDGE_CURVE ( 'NONE', #78895, #2854, #68990, .T. ) ;
#57240=CARTESIAN_POINT ( 'NONE',  ( -17.20761368003338632, -2.295517848115768089, 30.44137282052136939 ) ) ;
#57241=DIRECTION ( 'NONE',  ( -0.000000000000000000, -0.5000000000000009992, -0.8660254037844380415 ) ) ;
#57242=CARTESIAN_POINT ( 'NONE',  ( 13.38461538461538680, -3.322132147404559976, 32.92929555188717927 ) ) ;
#57243=ORIENTED_EDGE ( 'NONE', *, *, #1781, .T. ) ;
#57244=CARTESIAN_POINT ( 'NONE',  ( -0.7115384615384606759, -2.499999999999998668, 29.75000000000000355 ) ) ;
#57246=VERTEX_POINT ( 'NONE', #27121 ) ;
#57247=CARTESIAN_POINT ( 'NONE',  ( -18.00000000000012079, -12.16647553114689906, 32.15551576947799362 ) ) ;
#57248=CARTESIAN_POINT ( 'NONE',  ( 6.065145779331965414, -7.750023238201980469, 34.74374492549440419 ) ) ;
#57249=B_SPLINE_CURVE_WITH_KNOTS ( 'NONE', 3,
 ( #69934, #2348, #55975, #83467, #69053, #42034, #22197, #49664, #36167, #28067 ),
 .UNSPECIFIED., .F., .F.,
 ( 4, 2, 2, 2, 4 ),
 ( 0.0007817246256747505334, 0.0009771112852218954894, 0.001172497944769040554, 0.001367884604316185618, 0.001563271263863330682 ),
 .UNSPECIFIED. ) ;
#57251=LINE ( 'NONE', #70768, #73569 ) ;
#57253=CARTESIAN_POINT ( 'NONE',  ( -11.76194646302586833, -3.019605429927184836, 32.48692288466676814 ) ) ;
#57254=CARTESIAN_POINT ( 'NONE',  ( 13.63456079399342791, -12.07971442181322352, 32.31769673815850297 ) ) ;
#57255=CARTESIAN_POINT ( 'NONE',  ( -3.903900744468109529, -4.176053281294514363, 33.81426240980091791 ) ) ;
#57256=ORIENTED_EDGE ( 'NONE', *, *, #50372, .F. ) ;
#57258=FACE_BOUND ( 'NONE', #60782, .T. ) ;
#57259=ORIENTED_EDGE ( 'NONE', *, *, #61916, .T. ) ;
#57260=CARTESIAN_POINT ( 'NONE',  ( -8.519176457592452678, -4.235687564193447052, 33.53795663066793509 ) ) ;
#57261=VECTOR ( 'NONE', #27284, 1000.000000000000227 ) ;
#57262=CARTESIAN_POINT ( 'NONE',  ( 9.468822748583745508, -12.24155766932282496, 31.33739205006857986 ) ) ;
#57263=CARTESIAN_POINT ( 'NONE',  ( 5.207714884747862705, -4.118422570099827595, 33.43335022499816489 ) ) ;
#57264=ORIENTED_EDGE ( 'NONE', *, *, #49846, .F. ) ;
#57265=VERTEX_POINT ( 'NONE', #13169 ) ;
#57266=CARTESIAN_POINT ( 'NONE',  ( -1.384615384615505151, -11.94971097300221174, 32.03036669348237098 ) ) ;
#57267=ORIENTED_EDGE ( 'NONE', *, *, #55181, .F. ) ;
#57268=CARTESIAN_POINT ( 'NONE',  ( 2.530471848960718528, -4.387253974876676565, 33.66317474335728832 ) ) ;
#57270=B_SPLINE_CURVE_WITH_KNOTS ( 'NONE', 3,
 ( #62381, #6571, #41686, #35823, #13763, #8349, #48427, #56083, #61501, #56528 ),
 .UNSPECIFIED., .F., .F.,
 ( 4, 2, 2, 2, 4 ),
 ( 0.0007817359430256322827, 0.0009771253907249989254, 0.001172514838424365676, 0.001367904286123732428, 0.001563293733823099179 ),
 .UNSPECIFIED. ) ;
#57271=CARTESIAN_POINT ( 'NONE',  ( 3.100077764101674127, -2.729777683071816785, 31.24903638046268739 ) ) ;
#57273=FACE_BOUND ( 'NONE', #7761, .T. ) ;
#57274=ORIENTED_EDGE ( 'NONE', *, *, #38296, .F. ) ;
#57275=CARTESIAN_POINT ( 'NONE',  ( -17.07692307692307665, -13.75783147151868846, 33.36296068462461051 ) ) ;
#57276=CARTESIAN_POINT ( 'NONE',  ( 0.7115927731767742737, -11.79725096376909654, 32.30694842903960762 ) ) ;
#57277=CARTESIAN_POINT ( 'NONE',  ( -17.74999994631756906, -12.75000000000001066, 29.68455032392686732 ) ) ;
#57278=LINE ( 'NONE', #9107, #17463 ) ;
#57283=DIRECTION ( 'NONE',  ( -0.000000000000000000, -0.6427876096865404731, -0.7660444431189770143 ) ) ;
#57284=CARTESIAN_POINT ( 'NONE',  ( 1.515140822849029734, -11.66157788607254275, 32.95092075102925833 ) ) ;
#57285=DIRECTION ( 'NONE',  ( -0.000000000000000000, 0.9848077530122085754, -0.1736481776669273613 ) ) ;
#57286=CARTESIAN_POINT ( 'NONE',  ( 12.71148387091650278, -12.68172785388650681, 30.59649109432439218 ) ) ;
#57287=DIRECTION ( 'NONE',  ( -0.000000000000000000, -0.7660444431189791237, -0.6427876096865379196 ) ) ;
#57288=CYLINDRICAL_SURFACE ( 'NONE', #5835, 0.2500000000000009437 ) ;
#57289=ORIENTED_EDGE ( 'NONE', *, *, #14217, .T. ) ;
#57290=CYLINDRICAL_SURFACE ( 'NONE', #45788, 0.2500000000000009437 ) ;
#57292=CARTESIAN_POINT ( 'NONE',  ( 4.376857505459002873, -9.086983370893049639, 34.49168942202179267 ) ) ;
#57293=FACE_OUTER_BOUND ( 'NONE', #23774, .T. ) ;
#57294=VERTEX_POINT ( 'NONE', #7299 ) ;
#57295=CARTESIAN_POINT ( 'NONE',  ( 8.519254025182178225, -12.65889640711025521, 30.72598325615533454 ) ) ;
#57297=ORIENTED_EDGE ( 'NONE', *, *, #6661, .F. ) ;
#57298=FACE_BOUND ( 'NONE', #70776, .T. ) ;
#57299=CARTESIAN_POINT ( 'NONE',  ( -17.07692307692307665, -1.466349020453238561, 30.81389545987213907 ) ) ;
#57300=ADVANCED_FACE ( 'NONE', ( #82078 ), #19914, .F. ) ;
#57302=CARTESIAN_POINT ( 'NONE',  ( 14.30769230769231015, -11.69971097300155272, 32.46337939537588113 ) ) ;
#57305=CARTESIAN_POINT ( 'NONE',  ( 5.299702618191484582, -3.236590943229499029, 32.36255958852954251 ) ) ;
#57306=DIRECTION ( 'NONE',  ( 0.000000000000000000, 0.1736481776669267785, -0.9848077530122087975 ) ) ;
#57307=CARTESIAN_POINT ( 'NONE',  ( -4.153846153846152411, -12.62096338111211580, 30.90682066428153263 ) ) ;
#57308=CARTESIAN_POINT ( 'NONE',  ( -6.700297381808511865, -3.236590943229499029, 32.36255958852954251 ) ) ;
#57309=ORIENTED_EDGE ( 'NONE', *, *, #55778, .F. ) ;
#57310=B_SPLINE_CURVE_WITH_KNOTS ( 'NONE', 3,
 ( #22130, #22568, #49600, #64421, #83398, #69870, #9935, #16256, #28439, #23445 ),
 .UNSPECIFIED., .F., .F.,
 ( 4, 2, 2, 2, 4 ),
 ( 0.000000000000000000, 0.0001954311564186862781, 0.0003908623128373725562, 0.0005862934692560588072, 0.0007817246256747451124 ),
 .UNSPECIFIED. ) ;
#57311=CARTESIAN_POINT ( 'NONE',  ( -7.780085495151408459, -10.51840700105979565, 33.73612834413962247 ) ) ;
#57312=VERTEX_POINT ( 'NONE', #5975 ) ;
#57314=ORIENTED_EDGE ( 'NONE', *, *, #76813, .T. ) ;
#57315=CARTESIAN_POINT ( 'NONE',  ( 9.692307692307572609, -3.835265460704628371, 33.15142922262033665 ) ) ;
#57316=CARTESIAN_POINT ( 'NONE',  ( 3.903822916553187028, -6.695914987888143877, 34.68535235679833306 ) ) ;
#57317=CARTESIAN_POINT ( 'NONE',  ( 7.780883845597525550, -10.33852847137145048, 34.16647553114627556 ) ) ;
#57318=CARTESIAN_POINT ( 'NONE',  ( -12.21148414990014608, -2.779044189368095275, 31.39831045268885745 ) ) ;
#57319=CARTESIAN_POINT ( 'NONE',  ( -8.069080063669991532, -9.086856451489515152, 34.49173150075333183 ) ) ;
#57321=EDGE_CURVE ( 'NONE', #8388, #43710, #47385, .T. ) ;
#57322=CARTESIAN_POINT ( 'NONE',  ( -4.153846153846152411, -8.810774026931790459, 35.74407628777942847 ) ) ;
#57325=DIRECTION ( 'NONE',  ( -0.000000000000000000, -0.5000000000000009992, -0.8660254037844380415 ) ) ;
#57326=CARTESIAN_POINT ( 'NONE',  ( 5.776515075435672664, -8.539481045369598178, 34.89627647299170832 ) ) ;
#57328=VECTOR ( 'NONE', #85363, 1000.000000000000227 ) ;
#57329=ORIENTED_EDGE ( 'NONE', *, *, #28922, .F. ) ;
#57330=VERTEX_POINT ( 'NONE', #60902 ) ;
#57331=CARTESIAN_POINT ( 'NONE',  ( 3.903869422903798903, -12.17611988154120972, 31.52148481390971213 ) ) ;
#57332=CARTESIAN_POINT ( 'NONE',  ( -6.673076923076923350, -2.499999999999998668, 29.75000000000000355 ) ) ;
#57334=VECTOR ( 'NONE', #20158, 1000.000000000000000 ) ;
#57335=CARTESIAN_POINT ( 'NONE',  ( 0.5915858967889124909, -7.723484941389743952, 34.99544897038808955 ) ) ;
#57336=CARTESIAN_POINT ( 'NONE',  ( -4.946397375159509835, -3.816742781228458448, 33.13167719472716044 ) ) ;
#57337=CARTESIAN_POINT ( 'NONE',  ( 17.29993592101647693, -8.282913670948747864, 34.94150082978203642 ) ) ;
#57338=DIRECTION ( 'NONE',  ( 0.000000000000000000, 0.9848077530122072432, 0.1736481776669354937 ) ) ;
#57339=VERTEX_POINT ( 'NONE', #74878 ) ;
#57340=CARTESIAN_POINT ( 'NONE',  ( 3.100622021331010725, -6.852621066184267029, 34.70813303252209181 ) ) ;
#57342=EDGE_CURVE ( 'NONE', #29327, #20327, #28825, .T. ) ;
#57344=CARTESIAN_POINT ( 'NONE',  ( 12.21151522424549896, -11.86270091957321249, 32.19358267280087915 ) ) ;
#57345=VERTEX_POINT ( 'NONE', #84745 ) ;
#57346=CARTESIAN_POINT ( 'NONE',  ( 3.480769230769230838, -7.500000000000001776, 35.04278698407183867 ) ) ;
#57347=ADVANCED_FACE ( 'NONE', ( #77524 ), #63995, .F. ) ;
#57348=B_SPLINE_CURVE_WITH_KNOTS ( 'NONE', 3,
 ( #42091, #69547, #35317, #8300, #34432, #55143, #36218, #20477, #63226, #27673 ),
 .UNSPECIFIED., .F., .F.,
 ( 4, 2, 2, 2, 4 ),
 ( 0.0007817246256747450040, 0.0009771112852218872494, 0.001172497944769029278, 0.001367884604316171523, 0.001563271263863313769 ),
 .UNSPECIFIED. ) ;
#57349=ORIENTED_EDGE ( 'NONE', *, *, #71969, .T. ) ;
#57351=CARTESIAN_POINT ( 'NONE',  ( -17.86947456176635640, -8.630441415882550871, 34.87705825610312615 ) ) ;
#57353=CARTESIAN_POINT ( 'NONE',  ( 6.065255139512839122, -12.70778746994558439, 30.41441678777537305 ) ) ;
#57354=VERTEX_POINT ( 'NONE', #49161 ) ;
#57355=CARTESIAN_POINT ( 'NONE',  ( -39.05038313613820122, -2.499999999999999556, 29.75000000000000355 ) ) ;
#57356=CARTESIAN_POINT ( 'NONE',  ( -17.32694631421604115, -3.711651800289232916, 33.01384336483936011 ) ) ;
#57357=CARTESIAN_POINT ( 'NONE',  ( -9.442253272394241392, -3.435999193479609914, 33.07426656108010832 ) ) ;
#57358=VERTEX_POINT ( 'NONE', #23456 ) ;
#57359=CARTESIAN_POINT ( 'NONE',  ( 7.780883845597524662, -11.67786785259540849, 32.92929555188721480 ) ) ;
#57360=EDGE_LOOP ( 'NONE', ( #15934, #31687, #54291, #42054 ) ) ;
#57361=VECTOR ( 'NONE', #43020, 1000.000000000000227 ) ;
#57362=CARTESIAN_POINT ( 'NONE',  ( 16.15384615384615330, -9.819645486525091727, 36.12317359536749706 ) ) ;
#57363=CARTESIAN_POINT ( 'NONE',  ( -15.23076923076922995, -9.819645486525091727, 36.12317359536749706 ) ) ;
#57364=CARTESIAN_POINT ( 'NONE',  ( 12.21151522424549896, -8.432397168068783699, 34.66272746175022945 ) ) ;
#57365=CARTESIAN_POINT ( 'NONE',  ( 1.384615384615386802, -8.164416787775445883, 34.95778746994557906 ) ) ;
#57366=DIRECTION ( 'NONE',  ( 0.000000000000000000, 0.9396926207859126468, -0.3420201433256571111 ) ) ;
#57367=ORIENTED_EDGE ( 'NONE', *, *, #53864, .F. ) ;
#57368=ORIENTED_EDGE ( 'NONE', *, *, #36663, .T. ) ;
#57369=ORIENTED_EDGE ( 'NONE', *, *, #77903, .F. ) ;
#57370=CARTESIAN_POINT ( 'NONE',  ( 12.68454981315131214, -11.76359900205217635, 32.36225158514719880 ) ) ;
#57371=DIRECTION ( 'NONE',  ( 0.000000000000000000, 0.8660254037844377084, 0.5000000000000015543 ) ) ;
#57372=CARTESIAN_POINT ( 'NONE',  ( -12.46153846153858424, -12.51329471203414379, 31.30864560766407578 ) ) ;
#57373=CARTESIAN_POINT ( 'NONE',  ( -14.30769230769230660, -2.708943851104267164, 35.45975837776705220 ) ) ;
#57374=CYLINDRICAL_SURFACE ( 'NONE', #53653, 0.2500000000000008882 ) ;
#57375=CARTESIAN_POINT ( 'NONE',  ( 5.326868595271216478, -10.05730279482229683, 34.04704008940765902 ) ) ;
#57376=ORIENTED_EDGE ( 'NONE', *, *, #37848, .F. ) ;
#57377=EDGE_LOOP ( 'NONE', ( #40339, #74605 ) ) ;
#57379=VERTEX_POINT ( 'NONE', #22140 ) ;
#57380=AXIS2_PLACEMENT_3D ( 'NONE', #30897, #85859, #24143 ) ;
#57383=CARTESIAN_POINT ( 'NONE',  ( -11.53846153846153655, -1.129524287112498415, 32.06866353760679544 ) ) ;
#57385=VECTOR ( 'NONE', #53553, 1000.000000000000114 ) ;
#57386=CARTESIAN_POINT ( 'NONE',  ( -1.450697763975519194, -4.661471528628507777, 34.16647553114621871 ) ) ;
#57388=ORIENTED_EDGE ( 'NONE', *, *, #87519, .F. ) ;
#57389=VECTOR ( 'NONE', #12008, 1000.000000000000227 ) ;
#57390=EDGE_LOOP ( 'NONE', ( #29850, #11147, #40565, #8334 ) ) ;
#57391=CARTESIAN_POINT ( 'NONE',  ( -2.373775718648186928, -12.37446782046654192, 30.86335684631486487 ) ) ;
#57393=FACE_BOUND ( 'NONE', #54626, .T. ) ;
#57394=B_SPLINE_CURVE_WITH_KNOTS ( 'NONE', 3,
 ( #61958, #47559, #41260, #21425, #48892, #6585, #40817, #47998, #15117, #13335 ),
 .UNSPECIFIED., .F., .F.,
 ( 4, 2, 2, 2, 4 ),
 ( 0.000000000000000000, 0.0001954311564186879857, 0.0003908623128373759715, 0.0005862934692560640114, 0.0007817246256747519429 ),
 .UNSPECIFIED. ) ;
#57395=CARTESIAN_POINT ( 'NONE',  ( 14.98074599347626368, -10.05641848906368097, 34.04755513067966177 ) ) ;
#57397=CYLINDRICAL_SURFACE ( 'NONE', #31871, 0.2499999999999986955 ) ;
#57398=ORIENTED_EDGE ( 'NONE', *, *, #65395, .T. ) ;
#57399=CARTESIAN_POINT ( 'NONE',  ( -15.23076923076922995, -8.164416787775445883, 34.95778746994557906 ) ) ;
#57400=CARTESIAN_POINT ( 'NONE',  ( 3.230769230769110045, -3.300289026999228881, 32.46337939537708905 ) ) ;
#57401=CARTESIAN_POINT ( 'NONE',  ( -7.846153846153844924, -3.513871655860378418, 32.76840700105978499 ) ) ;
#57402=ADVANCED_FACE ( 'NONE', ( #23020 ), #36106, .F. ) ;
#57403=CARTESIAN_POINT ( 'NONE',  ( 4.087762742890272527, -11.16473453929635440, 33.15142922261925662 ) ) ;
#57404=CARTESIAN_POINT ( 'NONE',  ( -16.94639737515951339, -2.619367082507847222, 30.83698974864643461 ) ) ;
#57405=DIRECTION ( 'NONE',  ( -0.000000000000000000, 0.8660254037844399289, -0.4999999999999980016 ) ) ;
#57406=LINE ( 'NONE', #51517, #15688 ) ;
#57407=CARTESIAN_POINT ( 'NONE',  ( -7.623374304885435215, -6.760870238392817200, 34.69528174975672385 ) ) ;
#57408=CARTESIAN_POINT ( 'NONE',  ( 16.37662569511456567, -9.332535724633405749, 34.40230450496446224 ) ) ;
#57409=CARTESIAN_POINT ( 'NONE',  ( 13.60739505359345181, -2.353885683473779800, 30.79025554430704403 ) ) ;
#57410=CARTESIAN_POINT ( 'NONE',  ( -5.999999999999998224, -11.69971097300155272, 32.46337939537588113 ) ) ;
#57411=CARTESIAN_POINT ( 'NONE',  ( 6.066068351002442682, -9.780366693483667717, 34.19971097300155805 ) ) ;
#57412=CARTESIAN_POINT ( 'NONE',  ( -13.51476335434707821, -4.299443229763728169, 33.91186481527756058 ) ) ;
#57413=CARTESIAN_POINT ( 'NONE',  ( 7.846153846153846700, -1.215029322943914858, 32.30358669280327177 ) ) ;
#57414=ADVANCED_FACE ( 'NONE', ( #21689 ), #77085, .F. ) ;
#57415=LINE ( 'NONE', #84909, #85657 ) ;
#57416=DIRECTION ( 'NONE',  ( 0.000000000000000000, 0.7660444431189807890, 0.6427876096865361433 ) ) ;
#57417=DIRECTION ( 'NONE',  ( 0.000000000000000000, 0.3420201433256610524, 0.9396926207859113145 ) ) ;
#57418=DIRECTION ( 'NONE',  ( -0.000000000000000000, 0.8660254037844399289, -0.4999999999999980016 ) ) ;
#57421=B_SPLINE_CURVE_WITH_KNOTS ( 'NONE', 3,
 ( #4139, #26202, #73054, #12689, #59088, #87038 ),
 .UNSPECIFIED., .F., .F.,
 ( 4, 2, 4 ),
 ( 0.0003909512603273906169, 0.0005862562993132179340, 0.0007815613382990451970 ),
 .UNSPECIFIED. ) ;
#57422=CARTESIAN_POINT ( 'NONE',  ( 0.2115152242454955145, -12.43535235679832596, 30.55408501211184813 ) ) ;
#57423=ORIENTED_EDGE ( 'NONE', *, *, #12352, .F. ) ;
#57424=ADVANCED_FACE ( 'NONE', ( #42862 ), #15390, .F. ) ;
#57425=CARTESIAN_POINT ( 'NONE',  ( -9.915233909823841785, -5.667676309546437530, 34.40238873228292249 ) ) ;
#57426=VERTEX_POINT ( 'NONE', #14491 ) ;
#57427=CARTESIAN_POINT ( 'NONE',  ( 15.90382291655318880, -11.37209801155882793, 32.91403422569033665 ) ) ;
#57428=ORIENTED_EDGE ( 'NONE', *, *, #82177, .T. ) ;
#57429=CARTESIAN_POINT ( 'NONE',  ( -16.15384615384627409, -3.300289026999228437, 32.46337939537709616 ) ) ;
#57431=CARTESIAN_POINT ( 'NONE',  ( -17.77722033102192967, -9.418065098278011860, 34.63729479722530158 ) ) ;
#57432=CARTESIAN_POINT ( 'NONE',  ( -3.164701897419153642, -12.34228464037088813, 31.77849191805839268 ) ) ;
#57433=CARTESIAN_POINT ( 'NONE',  ( 15.90386940979756858, -8.347322224742351082, 34.93158281831414769 ) ) ;
#57435=CARTESIAN_POINT ( 'NONE',  ( -13.63459212866397863, -8.347322224742351082, 34.93158281831414058 ) ) ;
#57436=CARTESIAN_POINT ( 'NONE',  ( 4.853438133199127869, -8.496056993536548418, 34.65000542017679663 ) ) ;
#57438=CARTESIAN_POINT ( 'NONE',  ( 1.161130440891440241, -2.847400154188068022, 31.58180166144859058 ) ) ;
#57439=CARTESIAN_POINT ( 'NONE',  ( -2.057637887778852814, -12.01375889529407637, 32.43194544308182969 ) ) ;
#57440=EDGE_CURVE ( 'NONE', #18050, #17526, #25733, .T. ) ;
#57441=EDGE_CURVE ( 'NONE', #14948, #10893, #36967, .T. ) ;
#57442=CYLINDRICAL_SURFACE ( 'NONE', #450, 0.2500000000000012212 ) ;
#57444=B_SPLINE_CURVE_WITH_KNOTS ( 'NONE', 3,
 ( #70736, #56766, #2254, #9469, #77485, #50874, #1384, #28411, #78360, #49127 ),
 .UNSPECIFIED., .F., .F.,
 ( 4, 2, 2, 2, 4 ),
 ( 0.000000000000000000, 0.0001954339857564070949, 0.0003908679715128141898, 0.0005863019572692212576, 0.0007817359430256283796 ),
 .UNSPECIFIED. ) ;
#57445=VECTOR ( 'NONE', #3883, 1000.000000000000000 ) ;
#57447=ORIENTED_EDGE ( 'NONE', *, *, #46319, .F. ) ;
#57448=EDGE_CURVE ( 'NONE', #20488, #84107, #26680, .T. ) ;
#57449=DIRECTION ( 'NONE',  ( -0.000000000000000000, -0.8660254037844397068, -0.4999999999999978906 ) ) ;
#57450=CARTESIAN_POINT ( 'NONE',  ( -11.47239318745910097, -8.120952969808772792, 34.71129190929999453 ) ) ;
#57451=CARTESIAN_POINT ( 'NONE',  ( -13.38461538461550582, -5.219633306517616589, 34.19971097300220464 ) ) ;
#57452=CARTESIAN_POINT ( 'NONE',  ( 1.449809366398742361, -2.506253911140448043, 29.99999999999988631 ) ) ;
#57453=EDGE_CURVE ( 'NONE', #40861, #9213, #87408, .T. ) ;
#57454=VECTOR ( 'NONE', #12898, 1000.000000000000000 ) ;
#57455=CARTESIAN_POINT ( 'NONE',  ( 15.16501242825492390, -7.249945686854186278, 34.74374336980224598 ) ) ;
#57456=CARTESIAN_POINT ( 'NONE',  ( -14.55769230769230660, -2.249999999999998668, 29.75000000000000355 ) ) ;
#57457=VECTOR ( 'NONE', #15478, 1000.000000000000114 ) ;
#57458=CARTESIAN_POINT ( 'NONE',  ( 8.545745825506822158, -10.81261337010820256, 33.49550067578627477 ) ) ;
#57459=EDGE_LOOP ( 'NONE', ( #19698, #39696 ) ) ;
#57460=CARTESIAN_POINT ( 'NONE',  ( -1.319359813339360032, -10.21337939537593620, 33.94971097300152252 ) ) ;
#57461=ORIENTED_EDGE ( 'NONE', *, *, #61298, .F. ) ;
#57463=CARTESIAN_POINT ( 'NONE',  ( -6.250023224221457063, -12.68155406624981119, 30.59749803192733708 ) ) ;
#57465=CARTESIAN_POINT ( 'NONE',  ( 15.23076923076923173, -8.564572088678739092, 35.78748833219616898 ) ) ;
#57466=DIRECTION ( 'NONE',  ( 0.000000000000000000, -6.938893903907222067E-15, 1.000000000000000000 ) ) ;
#57467=B_SPLINE_CURVE_WITH_KNOTS ( 'NONE', 3,
 ( #78947, #80290, #17242, #38858, #87507, #31196, #18141, #45600, #38408, #80745 ),
 .UNSPECIFIED., .F., .F.,
 ( 4, 2, 2, 2, 4 ),
 ( 0.0007817359430256369448, 0.0009771253907250049969, 0.001172514838424373266, 0.001367904286123741535, 0.001563293733823109587 ),
 .UNSPECIFIED. ) ;
#57468=ORIENTED_EDGE ( 'NONE', *, *, #70274, .T. ) ;
#57469=CARTESIAN_POINT ( 'NONE',  ( -14.08468095607945969, -12.15243808032446005, 31.58219941686247978 ) ) ;
#57470=B_SPLINE_CURVE_WITH_KNOTS ( 'NONE', 3,
 ( #17933, #59354, #24227, #74209, #53030, #45388, #3955, #44941, #80533, #80979 ),
 .UNSPECIFIED., .F., .F.,
 ( 4, 2, 2, 2, 4 ),
 ( 0.0007817246256747507503, 0.0009771112852218957062, 0.001172497944769040771, 0.001367884604316185835, 0.001563271263863330682 ),
 .UNSPECIFIED. ) ;
#57471=ORIENTED_EDGE ( 'NONE', *, *, #35774, .T. ) ;
#57472=B_SPLINE_CURVE_WITH_KNOTS ( 'NONE', 3,
 ( #25032, #58356, #46198, #17390, #60140, #52935, #25480, #86762, #73227, #44393 ),
 .UNSPECIFIED., .F., .F.,
 ( 4, 2, 2, 2, 4 ),
 ( 0.000000000000000000, 0.0001954339857564092904, 0.0003908679715128185808, 0.0005863019572692278712, 0.0007817359430256371616 ),
 .UNSPECIFIED. ) ;
#57473=EDGE_CURVE ( 'NONE', #51319, #48499, #43904, .T. ) ;
#57474=ORIENTED_EDGE ( 'NONE', *, *, #88960, .T. ) ;
#57475=DIRECTION ( 'NONE',  ( 0.000000000000000000, 0.1736481776669267785, -0.9848077530122087975 ) ) ;
#57476=CARTESIAN_POINT ( 'NONE',  ( 14.30769230769231015, -11.11383981884818262, 36.00935417666054406 ) ) ;
#57477=EDGE_CURVE ( 'NONE', #22156, #28775, #45950, .T. ) ;
#57478=CARTESIAN_POINT ( 'NONE',  ( -16.28453762051371712, -4.118384482072086072, 33.43331474514187107 ) ) ;
#57479=EDGE_CURVE ( 'NONE', #43220, #20800, #78016, .T. ) ;
#57480=CARTESIAN_POINT ( 'NONE',  ( -4.403846153846151523, -7.566083408709834757, 34.74999999999999289 ) ) ;
#57481=CARTESIAN_POINT ( 'NONE',  ( 7.846153846153846700, -12.62096338111211580, 30.90682066428153263 ) ) ;
#57482=ORIENTED_EDGE ( 'NONE', *, *, #53035, .T. ) ;
#57483=ORIENTED_EDGE ( 'NONE', *, *, #3655, .T. ) ;
#57485=EDGE_CURVE ( 'NONE', #5035, #55756, #71816, .T. ) ;
#57486=ORIENTED_EDGE ( 'NONE', *, *, #43677, .F. ) ;
#57487=DIRECTION ( 'NONE',  ( -0.000000000000000000, -0.7660444431189791237, -0.6427876096865379196 ) ) ;
#57488=ORIENTED_EDGE ( 'NONE', *, *, #51791, .F. ) ;
#57489=CARTESIAN_POINT ( 'NONE',  ( 1.515141086378950952, -9.417988943895561960, 34.36773134775778260 ) ) ;
#57490=CARTESIAN_POINT ( 'NONE',  ( -10.61538461538473399, -10.21337939537710326, 33.94971097300076224 ) ) ;
#57491=CARTESIAN_POINT ( 'NONE',  ( 2.307692307692186251, -9.528491918059723176, 34.59228464037033035 ) ) ;
#57492=ORIENTED_EDGE ( 'NONE', *, *, #81956, .F. ) ;
#57493=AXIS2_PLACEMENT_3D ( 'NONE', #30253, #69463, #7766 ) ;
#57494=CARTESIAN_POINT ( 'NONE',  ( -15.23076923076935074, -3.835265460704628371, 33.15142922262033665 ) ) ;
#57495=ORIENTED_EDGE ( 'NONE', *, *, #78010, .T. ) ;
#57496=FACE_BOUND ( 'NONE', #59698, .T. ) ;
#57497=CARTESIAN_POINT ( 'NONE',  ( 15.48071464014727283, -11.56426240980093745, 33.07394671870546432 ) ) ;
#57498=CARTESIAN_POINT ( 'NONE',  ( -7.146003140593069958, -2.758268499246657957, 31.33685645148948140 ) ) ;
#57499=CARTESIAN_POINT ( 'NONE',  ( 2.307692307692186251, -12.51329471203414379, 31.30864560766407578 ) ) ;
#57500=B_SPLINE_CURVE_WITH_KNOTS ( 'NONE', 3,
 ( #53141, #18925, #58559, #32000, #52699, #80187, #60347, #73874, #18487, #4060 ),
 .UNSPECIFIED., .F., .F.,
 ( 4, 2, 2, 2, 4 ),
 ( 0.000000000000000000, 0.0001954339857564081249, 0.0003908679715128162498, 0.0005863019572692244018, 0.0007817359430256324996 ),
 .UNSPECIFIED. ) ;
#57501=CARTESIAN_POINT ( 'NONE',  ( -0.3962833220256231637, -11.67786785259547777, 32.92929555188713664 ) ) ;
#57502=VECTOR ( 'NONE', #35374, 1000.000000000000227 ) ;
#57503=CYLINDRICAL_SURFACE ( 'NONE', #71316, 0.2499999999999994726 ) ;
#57505=CARTESIAN_POINT ( 'NONE',  ( 15.93091993633000847, -2.554751324335733376, 30.48935550225260727 ) ) ;
#57506=CARTESIAN_POINT ( 'NONE',  ( 18.13079180782477096, -2.729792928343269587, 31.24908615093345077 ) ) ;
#57508=CARTESIAN_POINT ( 'NONE',  ( -11.40766973063674961, -12.11778462344220841, 31.66786338562085135 ) ) ;
#57509=CARTESIAN_POINT ( 'NONE',  ( 4.946232473812766095, -3.957541250942359756, 33.62499894934981626 ) ) ;
#57510=B_SPLINE_CURVE_WITH_KNOTS ( 'NONE', 3,
 ( #7711, #83819, #941, #63519, #29312, #22102, #56764, #55880, #15349, #84260 ),
 .UNSPECIFIED., .F., .F.,
 ( 4, 2, 2, 2, 4 ),
 ( 0.000000000000000000, 0.0001954339857564082062, 0.0003908679715128164124, 0.0005863019572692246186, 0.0007817359430256328248 ),
 .UNSPECIFIED. ) ;
#57511=ADVANCED_FACE ( 'NONE', ( #71639 ), #51801, .F. ) ;
#57512=VECTOR ( 'NONE', #82049, 1000.000000000000000 ) ;
#57513=ORIENTED_EDGE ( 'NONE', *, *, #83071, .T. ) ;
#57515=CARTESIAN_POINT ( 'NONE',  ( -9.692307692307691624, -3.669653830205710676, 35.88435417666054406 ) ) ;
#57516=CARTESIAN_POINT ( 'NONE',  ( -18.13069060311030967, -12.62707690430377383, 30.88035979386743435 ) ) ;
#57517=DIRECTION ( 'NONE',  ( -0.000000000000000000, 1.000000000000000000, -0.000000000000000000 ) ) ;
#57518=FACE_OUTER_BOUND ( 'NONE', #32226, .T. ) ;
#57519=CARTESIAN_POINT ( 'NONE',  ( 7.911408985666682270, -6.835583212224610072, 34.95778746994559327 ) ) ;
#57520=CARTESIAN_POINT ( 'NONE',  ( -8.992715712954719720, -5.912607949931405926, 34.49155766932282319 ) ) ;
#57521=FACE_BOUND ( 'NONE', #82863, .T. ) ;
#57522=CARTESIAN_POINT ( 'NONE',  ( 9.942307692307695177, -2.499999999999998668, 29.75000000000000355 ) ) ;
#57523=CARTESIAN_POINT ( 'NONE',  ( 1.384615384615386802, -2.538708090699994813, 30.37095296980875503 ) ) ;
#57524=CARTESIAN_POINT ( 'NONE',  ( -18.22292695890684655, -8.282780595021769443, 34.94152052738834158 ) ) ;
#57525=CARTESIAN_POINT ( 'NONE',  ( 5.999999999999880096, -6.879047030192662504, 34.71129190930017927 ) ) ;
#57526=CARTESIAN_POINT ( 'NONE',  ( 7.053602624840485724, -12.45806712695776319, 30.39783852428763922 ) ) ;
#57527=LINE ( 'NONE', #44891, #85052 ) ;
#57530=CARTESIAN_POINT ( 'NONE',  ( -9.692307692307691624, -13.63283147151868846, 33.57946703557072254 ) ) ;
#57531=CARTESIAN_POINT ( 'NONE',  ( -14.37377571864818293, -6.386643153685125363, 34.62446782046654903 ) ) ;
#57532=CARTESIAN_POINT ( 'NONE',  ( 5.999999999999878320, -5.941354392335915335, 34.76329471203413846 ) ) ;
#57533=CARTESIAN_POINT ( 'NONE',  ( 17.07692307692307665, -8.164416787775445883, 34.95778746994557906 ) ) ;
#57534=CARTESIAN_POINT ( 'NONE',  ( 10.61538461538461675, -12.10708131394839349, 31.69288490824020244 ) ) ;
#57536=CARTESIAN_POINT ( 'NONE',  ( -1.318448778023743273, -7.250054591869667497, 34.99404684341514127 ) ) ;
#57537=CARTESIAN_POINT ( 'NONE',  ( 12.46153846153846168, -7.500000000000001776, 35.04278698407183867 ) ) ;
#57538=CARTESIAN_POINT ( 'NONE',  ( -16.85391172531022619, -5.667800583137506898, 34.40243808032445827 ) ) ;
#57539=CARTESIAN_POINT ( 'NONE',  ( 10.39245765647776309, -6.459968553980841577, 34.89616026154728701 ) ) ;
#57540=CARTESIAN_POINT ( 'NONE',  ( 5.142117058706431543, -2.506253911140448487, 29.99999999999988631 ) ) ;
#57542=DIRECTION ( 'NONE',  ( 0.000000000000000000, 0.8660254037844377084, -0.5000000000000015543 ) ) ;
#57544=EDGE_CURVE ( 'NONE', #87399, #26565, #52705, .T. ) ;
#57545=CARTESIAN_POINT ( 'NONE',  ( 7.912222197156284054, -6.386643153685127139, 34.62446782046654192 ) ) ;
#57546=ORIENTED_EDGE ( 'NONE', *, *, #63784, .F. ) ;
#57549=CARTESIAN_POINT ( 'NONE',  ( 6.923076923076924238, -4.786620604624113540, 33.94971097300155094 ) ) ;
#57552=CARTESIAN_POINT ( 'NONE',  ( 9.019230769230775380, -2.499999999999999556, 29.81604066197449754 ) ) ;
#57553=DIRECTION ( 'NONE',  ( 0.000000000000000000, -0.000000000000000000, 1.000000000000000000 ) ) ;
#57554=VERTEX_POINT ( 'NONE', #39215 ) ;
#57555=CARTESIAN_POINT ( 'NONE',  ( 15.23076923076923173, -4.661471528628507777, 34.16647553114623292 ) ) ;
#57556=CARTESIAN_POINT ( 'NONE',  ( 4.153846153846032507, -6.026961402154118908, 34.52809138561165270 ) ) ;
#57557=EDGE_LOOP ( 'NONE', ( #62291, #43077 ) ) ;
#57559=DIRECTION ( 'NONE',  ( 0.000000000000000000, 0.9848077530122072432, -0.1736481776669354937 ) ) ;
#57560=ADVANCED_FACE ( 'NONE', ( #45059 ), #66220, .F. ) ;
#57561=CARTESIAN_POINT ( 'NONE',  ( -5.207070286361296318, -11.47017969459903952, 32.78971311882034456 ) ) ;
#57562=CARTESIAN_POINT ( 'NONE',  ( -13.63459211555773720, -3.137211980971221781, 32.19342716148376837 ) ) ;
#57563=EDGE_CURVE ( 'NONE', #34671, #50071, #52100, .T. ) ;
#57565=CARTESIAN_POINT ( 'NONE',  ( -11.76138775597768138, -4.186968288167451036, 33.49512374952580274 ) ) ;
#57566=CARTESIAN_POINT ( 'NONE',  ( 12.46153846153846168, -6.189225973068211317, 35.74407628777942847 ) ) ;
#57567=VECTOR ( 'NONE', #31368, 999.9999999999998863 ) ;
#57568=CARTESIAN_POINT ( 'NONE',  ( -2.307692307692305711, -1.422936976036506707, 30.56769352161908415 ) ) ;
#57570=ORIENTED_EDGE ( 'NONE', *, *, #16892, .F. ) ;
#57571=EDGE_CURVE ( 'NONE', #57617, #54951, #32005, .T. ) ;
#57572=B_SPLINE_CURVE_WITH_KNOTS ( 'NONE', 3,
 ( #36164, #57748, #16753, #44208, #71695, #9997, #62718, #55972, #83910, #38368 ),
 .UNSPECIFIED., .F., .F.,
 ( 4, 2, 2, 2, 4 ),
 ( 0.0007817359527651090859, 0.0009771254036996478414, 0.001172514854634186489, 0.001367904305568725136, 0.001563293756503263783 ),
 .UNSPECIFIED. ) ;
#57573=ORIENTED_EDGE ( 'NONE', *, *, #80658, .T. ) ;
#57575=VECTOR ( 'NONE', #72016, 1000.000000000000000 ) ;
#57576=CARTESIAN_POINT ( 'NONE',  ( -9.915792636031639518, -10.11188796281391511, 34.01382737946119050 ) ) ;
#57577=DIRECTION ( 'NONE',  ( -0.000000000000000000, -0.7660444431189791237, -0.6427876096865379196 ) ) ;
#57578=ADVANCED_FACE ( 'NONE', ( #59912 ), #37412, .F. ) ;
#57579=DIRECTION ( 'NONE',  ( -0.000000000000000000, -0.3420201433256694346, -0.9396926207859080948 ) ) ;
#57582=ADVANCED_FACE ( 'NONE', ( #20702 ), #61232, .F. ) ;
#57584=ORIENTED_EDGE ( 'NONE', *, *, #75306, .F. ) ;
#57585=CARTESIAN_POINT ( 'NONE',  ( -2.084729173425631465, -7.369474539155830506, 34.99858011523957657 ) ) ;
#57586=EDGE_LOOP ( 'NONE', ( #85119, #82754, #83034, #42660 ) ) ;
#57587=EDGE_CURVE ( 'NONE', #46688, #47170, #49337, .T. ) ;
#57588=CARTESIAN_POINT ( 'NONE',  ( 17.32697738856138869, -4.943051570960395047, 34.04725096376909477 ) ) ;
#57589=DIRECTION ( 'NONE',  ( 0.000000000000000000, 0.3420201433256641055, -0.9396926207859100932 ) ) ;
#57590=CARTESIAN_POINT ( 'NONE',  ( -8.519285359852727169, -12.68172785388650681, 30.59649109432439218 ) ) ;
#57591=EDGE_LOOP ( 'NONE', ( #71102, #20269 ) ) ;
#57592=EDGE_CURVE ( 'NONE', #85237, #67642, #39666, .T. ) ;
#57593=EDGE_LOOP ( 'NONE', ( #85497, #38363, #56149, #62796 ) ) ;
#57594=CARTESIAN_POINT ( 'NONE',  ( 9.915087361285758405, -8.540255544307065350, 34.89611431652622286 ) ) ;
#57595=ORIENTED_EDGE ( 'NONE', *, *, #66872, .F. ) ;
#57598=ORIENTED_EDGE ( 'NONE', *, *, #6917, .F. ) ;
#57599=EDGE_CURVE ( 'NONE', #63565, #69312, #15998, .T. ) ;
#57600=CARTESIAN_POINT ( 'NONE',  ( -8.899922235898326761, -10.54014554554150607, 33.71984207302941883 ) ) ;
#57601=B_SPLINE_CURVE_WITH_KNOTS ( 'NONE', 3,
 ( #65309, #16681, #37388, #45033, #72511, #10822, #16244, #30636, #59449, #78377 ),
 .UNSPECIFIED., .F., .F.,
 ( 4, 2, 2, 2, 4 ),
 ( 0.000000000000000000, 0.0001954311564186866305, 0.0003908623128373732609, 0.0005862934692560598914, 0.0007817246256747465219 ),
 .UNSPECIFIED. ) ;
#57603=AXIS2_PLACEMENT_3D ( 'NONE', #73643, #66871, #41949 ) ;
#57604=CARTESIAN_POINT ( 'NONE',  ( 5.076923076923075762, -11.16473453929635440, 33.15142922261926373 ) ) ;
#57605=CARTESIAN_POINT ( 'NONE',  ( 10.74591031714818357, -3.816742781228458448, 33.13167719472716044 ) ) ;
#57606=FACE_BOUND ( 'NONE', #15007, .T. ) ;
#57608=FACE_OUTER_BOUND ( 'NONE', #6108, .T. ) ;
#57609=B_SPLINE_CURVE_WITH_KNOTS ( 'NONE', 3,
 ( #73287, #40401, #5273, #17899, #88161, #12473, #81386, #4380, #5713, #39515 ),
 .UNSPECIFIED., .F., .F.,
 ( 4, 2, 2, 2, 4 ),
 ( 0.0007817246256747457630, 0.0009771112852218887673, 0.001172497944769031663, 0.001367884604316174559, 0.001563271263863317672 ),
 .UNSPECIFIED. ) ;
#57610=FACE_OUTER_BOUND ( 'NONE', #50260, .T. ) ;
#57611=CARTESIAN_POINT ( 'NONE',  ( 16.40379156322419973, -4.176053281294515251, 33.81426240980091791 ) ) ;
#57612=CARTESIAN_POINT ( 'NONE',  ( 9.942253210655836781, -3.202959910592335646, 32.30730279482227019 ) ) ;
#57613=CARTESIAN_POINT ( 'NONE',  ( 8.519254025182178225, -9.234221910056348293, 34.70572697212741531 ) ) ;
#57614=CARTESIAN_POINT ( 'NONE',  ( 11.53846153846153832, -1.951392089020283160, 34.73218667398347748 ) ) ;
#57616=CARTESIAN_POINT ( 'NONE',  ( 14.24236829488800105, -7.749976730030849303, 34.74374725381503737 ) ) ;
#57617=VERTEX_POINT ( 'NONE', #41421 ) ;
#57618=EDGE_CURVE ( 'NONE', #53071, #64411, #47283, .T. ) ;
#57620=CYLINDRICAL_SURFACE ( 'NONE', #77753, 0.2500000000000009437 ) ;
#57621=CARTESIAN_POINT ( 'NONE',  ( 10.83816428436268176, -12.11081565061823717, 32.26097654155341843 ) ) ;
#57622=EDGE_CURVE ( 'NONE', #64660, #71506, #51362, .T. ) ;
#57623=CARTESIAN_POINT ( 'NONE',  ( 11.53846153846141576, -8.656820664282941280, 34.87096338111179961 ) ) ;
#57624=CARTESIAN_POINT ( 'NONE',  ( 14.43821774592595553, -4.299079248970732792, 33.91157788607253565 ) ) ;
#57625=CARTESIAN_POINT ( 'NONE',  ( 1.253923917947829203, -6.413092428213692742, 34.63065189839063152 ) ) ;
#57626=CARTESIAN_POINT ( 'NONE',  ( -0.3310127597748964146, -11.93748526763465279, 32.05452791011430946 ) ) ;
#57627=ORIENTED_EDGE ( 'NONE', *, *, #84593, .T. ) ;
#57628=DIRECTION ( 'NONE',  ( -0.000000000000000000, 0.9396926207859092051, -0.3420201433256662704 ) ) ;
#57629=CARTESIAN_POINT ( 'NONE',  ( 14.05766908347085042, -12.68155406624981119, 30.59749803192733708 ) ) ;
#57630=CARTESIAN_POINT ( 'NONE',  ( -12.52762084089859584, -11.35647404775217595, 33.31231777344666511 ) ) ;
#57631=DIRECTION ( 'NONE',  ( -0.000000000000000000, 0.7660444431189791237, -0.6427876096865379196 ) ) ;
#57632=CARTESIAN_POINT ( 'NONE',  ( 13.60739505359345536, -5.827830569534417471, 34.72679350104403539 ) ) ;
#57634=ORIENTED_EDGE ( 'NONE', *, *, #38260, .F. ) ;
#57635=AXIS2_PLACEMENT_3D ( 'NONE', #6502, #33962, #62310 ) ;
#57636=VECTOR ( 'NONE', #42479, 1000.000000000000227 ) ;
#57637=ORIENTED_EDGE ( 'NONE', *, *, #30037, .T. ) ;
#57638=DIRECTION ( 'NONE',  ( -0.000000000000000000, 1.000000000000000000, -0.000000000000000000 ) ) ;
#57639=VERTEX_POINT ( 'NONE', #81981 ) ;
#57640=DIRECTION ( 'NONE',  ( 0.000000000000000000, 0.3420201433256641055, -0.9396926207859100932 ) ) ;
#57641=CARTESIAN_POINT ( 'NONE',  ( -13.38461538461538325, -4.102666532097928531, 36.13435417666054406 ) ) ;
#57642=CARTESIAN_POINT ( 'NONE',  ( 4.088576153289833037, -11.06231777344662781, 33.60647404775220082 ) ) ;
#57643=CARTESIAN_POINT ( 'NONE',  ( 5.934750068225916664, -2.255955759149247619, 30.00000000000013856 ) ) ;
#57646=B_SPLINE_CURVE_WITH_KNOTS ( 'NONE', 3,
 ( #33836, #54997, #67634, #54543, #74840, #14008, #46901, #27081, #40610, #73950 ),
 .UNSPECIFIED., .F., .F.,
 ( 4, 2, 2, 2, 4 ),
 ( 0.000000000000000000, 0.0001954311564186879044, 0.0003908623128373758088, 0.0005862934692560636861, 0.0007817246256747516176 ),
 .UNSPECIFIED. ) ;
#57648=ORIENTED_EDGE ( 'NONE', *, *, #88535, .F. ) ;
#57649=CARTESIAN_POINT ( 'NONE',  ( -5.999999999999998224, -2.517432740324522911, 35.29906147534542527 ) ) ;
#57650=CARTESIAN_POINT ( 'NONE',  ( -1.134561072977068763, -9.148310452688873440, 34.47095581063188519 ) ) ;
#57651=ORIENTED_EDGE ( 'NONE', *, *, #55707, .F. ) ;
#57653=CARTESIAN_POINT ( 'NONE',  ( -12.33074665371367651, -3.530189275343204702, 32.79018710029569661 ) ) ;
#57654=B_SPLINE_CURVE_WITH_KNOTS ( 'NONE', 3,
 ( #73214, #67344, #61020, #81310, #65993, #80874, #53820, #86748, #88522, #79966 ),
 .UNSPECIFIED., .F., .F.,
 ( 4, 2, 2, 2, 4 ),
 ( 0.000000000000000000, 0.0001954339857564099951, 0.0003908679715128199903, 0.0005863019572692300396, 0.0007817359430256399806 ),
 .UNSPECIFIED. ) ;
#57655=B_SPLINE_CURVE_WITH_KNOTS ( 'NONE', 3,
 ( #4697, #31274, #59629, #79907, #24506, #24062, #85781, #46122, #4242, #18209 ),
 .UNSPECIFIED., .F., .F.,
 ( 4, 2, 2, 2, 4 ),
 ( 0.000000000000000000, 0.0001954339857564083146, 0.0003908679715128166293, 0.0005863019572692249439, 0.0007817359430256332585 ),
 .UNSPECIFIED. ) ;
#57656=CARTESIAN_POINT ( 'NONE',  ( 11.47237812750565666, -4.098570777380720287, 33.41473453929634729 ) ) ;
#57657=CARTESIAN_POINT ( 'NONE',  ( 6.923076923076924238, -3.322132147404559976, 32.92929555188717927 ) ) ;
#57658=DIRECTION ( 'NONE',  ( 0.000000000000000000, 0.9848077530122072432, -0.1736481776669354937 ) ) ;
#57659=CARTESIAN_POINT ( 'NONE',  ( -11.31568186948346977, -3.020022701398813236, 32.48759521482552515 ) ) ;
#57661=ORIENTED_EDGE ( 'NONE', *, *, #68893, .F. ) ;
#57662=CARTESIAN_POINT ( 'NONE',  ( -13.13456096470193302, -10.06805714834173493, 34.32951233291982618 ) ) ;
#57663=CARTESIAN_POINT ( 'NONE',  ( -13.60810032833933469, -9.331801661448606566, 34.40259984581193464 ) ) ;
#57665=CARTESIAN_POINT ( 'NONE',  ( -16.08859101433331062, -11.67786785259547777, 32.92929555188713664 ) ) ;
#57666=CARTESIAN_POINT ( 'NONE',  ( 16.15384615384603251, -5.094484230521993062, 34.41647553114689373 ) ) ;
#57667=ORIENTED_EDGE ( 'NONE', *, *, #25204, .F. ) ;
#57668=DIRECTION ( 'NONE',  ( 0.000000000000000000, 0.8660254037844377084, -0.5000000000000015543 ) ) ;
#57669=LINE ( 'NONE', #50459, #26797 ) ;
#57670=EDGE_CURVE ( 'NONE', #10085, #66377, #56820, .T. ) ;
#57671=ORIENTED_EDGE ( 'NONE', *, *, #70043, .T. ) ;
#57672=CARTESIAN_POINT ( 'NONE',  ( -12.46153846153846168, -1.466349020453238561, 30.81389545987213907 ) ) ;
#57673=EDGE_CURVE ( 'NONE', #62136, #29682, #33342, .T. ) ;
#57674=ORIENTED_EDGE ( 'NONE', *, *, #14593, .T. ) ;
#57676=CARTESIAN_POINT ( 'NONE',  ( 3.100078627658921615, -3.957541250942359756, 33.62499894934981626 ) ) ;
#57677=CARTESIAN_POINT ( 'NONE',  ( -0.7115152055870533898, -10.06842814019191401, 34.32929386961144758 ) ) ;
#57678=DIRECTION ( 'NONE',  ( -0.000000000000000000, 0.9848077530122086864, -0.1736481776669273891 ) ) ;
#57679=AXIS2_PLACEMENT_3D ( 'NONE', #75077, #41291, #61105 ) ;
#57681=ADVANCED_FACE ( 'NONE', ( #13943 ), #60801, .F. ) ;
#57682=CARTESIAN_POINT ( 'NONE',  ( -13.31854805126531005, -2.833524468853757305, 32.15551576947925838 ) ) ;
#57683=ORIENTED_EDGE ( 'NONE', *, *, #80522, .T. ) ;
#57684=B_SPLINE_CURVE_WITH_KNOTS ( 'NONE', 3,
 ( #27271, #21845, #27709, #43006, #54735, #7452, #49320, #55180, #56072, #34908 ),
 .UNSPECIFIED., .F., .F.,
 ( 4, 2, 2, 2, 4 ),
 ( 0.0007817246256747499913, 0.0009771112852218944052, 0.001172497944769038819, 0.001367884604316183016, 0.001563271263863327430 ),
 .UNSPECIFIED. ) ;
#57685=CYLINDRICAL_SURFACE ( 'NONE', #37075, 0.2499999999999986955 ) ;
#57686=CARTESIAN_POINT ( 'NONE',  ( 6.000000000000001776, -13.57706302396349152, 30.56769352161908060 ) ) ;
#57688=B_SPLINE_CURVE_WITH_KNOTS ( 'NONE', 3,
 ( #79026, #9676, #24078, #23194, #64163, #37590, #65052, #78136, #2032, #17328 ),
 .UNSPECIFIED., .F., .F.,
 ( 4, 2, 2, 2, 4 ),
 ( 0.0007817246256747471724, 0.0009771112852218905021, 0.001172497944769033832, 0.001367884604316177161, 0.001563271263863320491 ),
 .UNSPECIFIED. ) ;
#57690=CARTESIAN_POINT ( 'NONE',  ( -12.52680890749923570, -6.026961402152685388, 34.52809138561120506 ) ) ;
#57692=ADVANCED_FACE ( 'NONE', ( #88310 ), #15724, .F. ) ;
#57693=CARTESIAN_POINT ( 'NONE',  ( 1.161688425708537808, -6.459968553980839800, 34.89616026154728701 ) ) ;
#57695=B_SPLINE_CURVE_WITH_KNOTS ( 'NONE', 3,
 ( #85477, #22005, #35969, #50342, #17013, #43595, #36410, #44466, #35521, #37276 ),
 .UNSPECIFIED., .F., .F.,
 ( 4, 2, 2, 2, 4 ),
 ( 0.000000000000000000, 0.0001954311564186875792, 0.0003908623128373751583, 0.0005862934692560627103, 0.0007817246256747503166 ),
 .UNSPECIFIED. ) ;
#57696=ORIENTED_EDGE ( 'NONE', *, *, #7047, .F. ) ;
#57697=ORIENTED_EDGE ( 'NONE', *, *, #54236, .F. ) ;
#57698=AXIS2_PLACEMENT_3D ( 'NONE', #38492, #16877, #10121 ) ;
#57699=FACE_BOUND ( 'NONE', #14106, .T. ) ;
#57701=CARTESIAN_POINT ( 'NONE',  ( -5.076923076922761346, -2.255955759149395501, 30.00000000000324363 ) ) ;
#57702=EDGE_CURVE ( 'NONE', #25936, #8816, #55369, .T. ) ;
#57704=EDGE_CURVE ( 'NONE', #45635, #66313, #68644, .T. ) ;
#57705=CARTESIAN_POINT ( 'NONE',  ( 13.45068373561782593, -10.51840700105979565, 33.73612834413962247 ) ) ;
#57706=CARTESIAN_POINT ( 'NONE',  ( -10.61538461538473577, -10.33852847137269571, 34.16647553114546554 ) ) ;
#57707=VERTEX_POINT ( 'NONE', #50374 ) ;
#57709=VERTEX_POINT ( 'NONE', #76083 ) ;
#57710=VERTEX_POINT ( 'NONE', #77851 ) ;
#57711=CARTESIAN_POINT ( 'NONE',  ( 3.230769230769110045, -5.219633306517616589, 34.19971097300220464 ) ) ;
#57712=VERTEX_POINT ( 'NONE', #43189 ) ;
#57713=CARTESIAN_POINT ( 'NONE',  ( -4.153846153846152411, -5.180354513474913603, 36.12317359536750416 ) ) ;
#57714=ADVANCED_FACE ( 'NONE', ( #16157 ), #7640, .F. ) ;
#57715=CARTESIAN_POINT ( 'NONE',  ( 3.230769230769110045, -2.892918686052166066, 31.69288490824153470 ) ) ;
#57716=CARTESIAN_POINT ( 'NONE',  ( -2.530619266599154038, -12.38737895849757820, 31.66785238281580206 ) ) ;
#57717=FACE_BOUND ( 'NONE', #55864, .T. ) ;
#57718=ORIENTED_EDGE ( 'NONE', *, *, #47017, .F. ) ;
#57720=CARTESIAN_POINT ( 'NONE',  ( -12.46153846153846168, -2.708943851104267164, 35.45975837776705220 ) ) ;
#57721=CYLINDRICAL_SURFACE ( 'NONE', #52404, 0.2499999999999979738 ) ;
#57722=CARTESIAN_POINT ( 'NONE',  ( 11.66898724022510514, -8.586989748646452369, 34.63063291749215011 ) ) ;
#57723=VERTEX_POINT ( 'NONE', #84633 ) ;
#57724=CARTESIAN_POINT ( 'NONE',  ( -17.32694631421604115, -12.43535235679832596, 30.55408501211184813 ) ) ;
#57726=EDGE_CURVE ( 'NONE', #80807, #27135, #67529, .T. ) ;
#57727=EDGE_LOOP ( 'NONE', ( #27353, #4070 ) ) ;
#57728=CARTESIAN_POINT ( 'NONE',  ( -18.00000000000000711, -2.252971138473345292, 29.99985851721553942 ) ) ;
#57731=CARTESIAN_POINT ( 'NONE',  ( -8.638705330997124676, -12.50538340440932394, 31.33453814440721885 ) ) ;
#57732=CARTESIAN_POINT ( 'NONE',  ( 16.15384615384615330, -5.415277668671390821, 36.20867863119892149 ) ) ;
#57733=ADVANCED_FACE ( 'NONE', ( #49934 ), #70660, .F. ) ;
#57734=CARTESIAN_POINT ( 'NONE',  ( -18.13014796973169851, -5.915902021225892149, 34.75552854090298638 ) ) ;
#57735=DIRECTION ( 'NONE',  ( -0.000000000000000000, 0.6427876096865404731, -0.7660444431189770143 ) ) ;
#57737=EDGE_LOOP ( 'NONE', ( #64486, #13491, #86551, #11253 ) ) ;
#57739=DIRECTION ( 'NONE',  ( -0.000000000000000000, 1.000000000000000000, -0.000000000000000000 ) ) ;
#57740=CARTESIAN_POINT ( 'NONE',  ( -17.32694631421604115, -11.86270091957321071, 32.19358267280088626 ) ) ;
#57741=CARTESIAN_POINT ( 'NONE',  ( 14.30769230769218581, -2.657715359629662544, 31.77849191805970364 ) ) ;
#57743=VERTEX_POINT ( 'NONE', #22032 ) ;
#57746=FACE_BOUND ( 'NONE', #20578, .T. ) ;
#57748=CARTESIAN_POINT ( 'NONE',  ( -6.673076923076859401, -7.434744429011176159, 34.75000000000000711 ) ) ;
#57749=ORIENTED_EDGE ( 'NONE', *, *, #12411, .T. ) ;
#57751=CARTESIAN_POINT ( 'NONE',  ( 5.999999999999878320, -11.67786785259630911, 32.92929555188603530 ) ) ;
#57753=CARTESIAN_POINT ( 'NONE',  ( -6.673022611438607754, -3.136992222400443175, 32.19305428654138979 ) ) ;
#57755=CARTESIAN_POINT ( 'NONE',  ( 8.769230769230768274, -1.790695186598648903, 34.54067556320373455 ) ) ;
#57756=EDGE_LOOP ( 'NONE', ( #68141, #86164 ) ) ;
#57757=DIRECTION ( 'NONE',  ( 0.000000000000000000, 0.000000000000000000, 1.000000000000000000 ) ) ;
#57758=ORIENTED_EDGE ( 'NONE', *, *, #23029, .F. ) ;
#57759=CARTESIAN_POINT ( 'NONE',  ( 15.45378058238208041, -8.239487800360276282, 34.69522927552633718 ) ) ;
#57760=CARTESIAN_POINT ( 'NONE',  ( -4.153846153846273204, -2.892918686052165622, 31.69288490824153470 ) ) ;
#57761=LINE ( 'NONE', #32068, #1256 ) ;
#57762=CYLINDRICAL_SURFACE ( 'NONE', #35198, 0.2499999999999986955 ) ;
#57763=CARTESIAN_POINT ( 'NONE',  ( 13.38461538461538680, -5.557115091759785130, 34.35708131394839171 ) ) ;
#57766=ORIENTED_EDGE ( 'NONE', *, *, #15929, .T. ) ;
#57767=CARTESIAN_POINT ( 'NONE',  ( -0.6850234052624096792, -5.912607949931405926, 34.49155766932282319 ) ) ;
#57769=VERTEX_POINT ( 'NONE', #70218 ) ;
#57771=ORIENTED_EDGE ( 'NONE', *, *, #5196, .T. ) ;
#57772=VERTEX_POINT ( 'NONE', #8966 ) ;
#57773=DIRECTION ( 'NONE',  ( -0.000000000000000000, 0.8660254037844397068, -0.4999999999999978906 ) ) ;
#57774=CARTESIAN_POINT ( 'NONE',  ( 12.68455130563185840, -4.026326845037962343, 33.68677907613344047 ) ) ;
#57775=CARTESIAN_POINT ( 'NONE',  ( 3.165498784808455923, -10.21337939537584383, 33.94971097300158647 ) ) ;
#57777=DIRECTION ( 'NONE',  ( 0.000000000000000000, 0.1736481776669267785, -0.9848077530122087975 ) ) ;
#57778=CARTESIAN_POINT ( 'NONE',  ( -17.07692307692307665, -2.900454961884010974, 35.62045528018868623 ) ) ;
#57779=DIRECTION ( 'NONE',  ( -0.000000000000000000, 0.9396926207859093161, -0.3420201433256663259 ) ) ;
#57780=CARTESIAN_POINT ( 'NONE',  ( 1.384615384615386802, -6.435427911321262684, 35.78748833219616898 ) ) ;
#57781=ORIENTED_EDGE ( 'NONE', *, *, #58854, .F. ) ;
#57782=DIRECTION ( 'NONE',  ( -0.000000000000000000, -0.6427876096865404731, -0.7660444431189770143 ) ) ;
#57783=CARTESIAN_POINT ( 'NONE',  ( -0.2385271099256120464, -8.239487800360278058, 34.69522927552634428 ) ) ;
#57784=CARTESIAN_POINT ( 'NONE',  ( -9.561781990544131915, -11.46989282347013095, 32.79007818306219946 ) ) ;
#57785=CARTESIAN_POINT ( 'NONE',  ( 14.30769230769231015, -8.164416787775445883, 34.95778746994557906 ) ) ;
#57787=CARTESIAN_POINT ( 'NONE',  ( 0.4615384615384611200, -9.905515769479276145, 34.41647553114623292 ) ) ;
#57788=ORIENTED_EDGE ( 'NONE', *, *, #51576, .F. ) ;
#57789=CARTESIAN_POINT ( 'NONE',  ( 0.7115927731767761610, -9.148310452688873440, 34.47095581063188519 ) ) ;
#57790=CARTESIAN_POINT ( 'NONE',  ( -8.769230769230768274, -2.499999999999998668, 29.75000000000001421 ) ) ;
#57792=CARTESIAN_POINT ( 'NONE',  ( 12.59233026936324684, -10.54018710029568595, 33.71981072465678864 ) ) ;
#57794=CARTESIAN_POINT ( 'NONE',  ( -2.437840277424001556, -6.809168938359898782, 34.95455904226513866 ) ) ;
#57795=CARTESIAN_POINT ( 'NONE',  ( -16.15384615384615330, -8.318370150425687726, 35.83090037661290239 ) ) ;
#57796=CARTESIAN_POINT ( 'NONE',  ( -18.00000000104979492, -12.75000000000000355, 29.50000000010276935 ) ) ;
#57797=B_SPLINE_CURVE_WITH_KNOTS ( 'NONE', 3,
 ( #49119, #76598, #42380, #5924, #2246, #56759, #36500, #70281, #8143, #29307 ),
 .UNSPECIFIED., .F., .F.,
 ( 4, 2, 2, 2, 4 ),
 ( 0.000000000000000000, 0.0001954339857564074473, 0.0003908679715128148945, 0.0005863019572692223418, 0.0007817359430256297891 ),
 .UNSPECIFIED. ) ;
#57799=CARTESIAN_POINT ( 'NONE',  ( -2.980823712421088345, -12.22109172314383052, 31.39792113162168263 ) ) ;
#57800=ORIENTED_EDGE ( 'NONE', *, *, #514, .T. ) ;
#57801=CARTESIAN_POINT ( 'NONE',  ( -1.254089682851817988, -3.816742781228458448, 33.13167719472716044 ) ) ;
#57802=ORIENTED_EDGE ( 'NONE', *, *, #41341, .F. ) ;
#57804=LINE ( 'NONE', #31214, #29043 ) ;
#57805=CARTESIAN_POINT ( 'NONE',  ( 7.145856592054986578, -3.020022701398814569, 32.48759521482552515 ) ) ;
#57806=CARTESIAN_POINT ( 'NONE',  ( -1.515305987725692249, -9.084618155246140248, 34.75535874321725771 ) ) ;
#57807=CARTESIAN_POINT ( 'NONE',  ( -14.05774678934416499, -10.05730279482229683, 34.04704008940765902 ) ) ;
#57808=FACE_OUTER_BOUND ( 'NONE', #40430, .T. ) ;
#57809=B_SPLINE_CURVE_WITH_KNOTS ( 'NONE', 3,
 ( #12974, #61143, #89097, #48513, #62906, #88656, #7096, #54839, #41779, #6653 ),
 .UNSPECIFIED., .F., .F.,
 ( 4, 2, 2, 2, 4 ),
 ( 0.0007817246256747507503, 0.0009771112852218957062, 0.001172497944769040771, 0.001367884604316185835, 0.001563271263863330682 ),
 .UNSPECIFIED. ) ;
#57810=VERTEX_POINT ( 'NONE', #42756 ) ;
#57811=B_SPLINE_CURVE_WITH_KNOTS ( 'NONE', 3,
 ( #45395, #45843, #51236, #44947, #59361, #66572, #37304, #4878, #10736, #52598 ),
 .UNSPECIFIED., .F., .F.,
 ( 4, 2, 2, 2, 4 ),
 ( 0.0007817246256747463051, 0.0009771112852218896347, 0.001172497944769033181, 0.001367884604316176728, 0.001563271263863320057 ),
 .UNSPECIFIED. ) ;
#57812=EDGE_LOOP ( 'NONE', ( #55520, #54221, #27682, #52634 ) ) ;
#57816=ADVANCED_FACE ( 'NONE', ( #14390 ), #41870, .F. ) ;
#57817=CARTESIAN_POINT ( 'NONE',  ( -10.54931626438217585, -8.120952969808772792, 34.71129190929999453 ) ) ;
#57819=CARTESIAN_POINT ( 'NONE',  ( -5.299749769402080979, -7.369208160676172348, 34.74850200257122879 ) ) ;
#57820=CARTESIAN_POINT ( 'NONE',  ( -18.00000000000000000, -2.724637637897661335, 35.44105525097462106 ) ) ;
#57821=CARTESIAN_POINT ( 'NONE',  ( -13.16160403300253634, -5.667800583137506010, 34.40243808032445827 ) ) ;
#57823=CARTESIAN_POINT ( 'NONE',  ( -6.130147969731697621, -3.069018819979302926, 32.56621877034667278 ) ) ;
#57824=VECTOR ( 'NONE', #79193, 1000.000000000000000 ) ;
#57825=CARTESIAN_POINT ( 'NONE',  ( 5.999999999999880096, -11.94971097300221174, 32.03036669348237098 ) ) ;
#57826=CARTESIAN_POINT ( 'NONE',  ( -17.77722045873158763, -6.760870238392815423, 34.69528174975672385 ) ) ;
#57827=ORIENTED_EDGE ( 'NONE', *, *, #70420, .F. ) ;
#57829=VECTOR ( 'NONE', #48586, 1000.000000000000227 ) ;
#57830=ORIENTED_EDGE ( 'NONE', *, *, #14227, .F. ) ;
#57831=DIRECTION ( 'NONE',  ( 0.000000000000000000, 0.000000000000000000, 1.000000000000000000 ) ) ;
#57832=EDGE_LOOP ( 'NONE', ( #43303, #38104 ) ) ;
#57833=CARTESIAN_POINT ( 'NONE',  ( 0.7114839798866022802, -8.433404298154336232, 34.66254593164985920 ) ) ;
#57834=DIRECTION ( 'NONE',  ( 0.000000000000000000, 0.9396926207859126468, -0.3420201433256571111 ) ) ;
#57836=EDGE_CURVE ( 'NONE', #35268, #32683, #84192, .T. ) ;
#57838=EDGE_CURVE ( 'NONE', #35434, #57639, #1959, .T. ) ;
#57839=EDGE_LOOP ( 'NONE', ( #70662, #71673 ) ) ;
#57840=ORIENTED_EDGE ( 'NONE', *, *, #43902, .T. ) ;
#57841=CARTESIAN_POINT ( 'NONE',  ( -2.557715544985270650, -12.43535235679832596, 30.55408501211184813 ) ) ;
#57842=VERTEX_POINT ( 'NONE', #86863 ) ;
#57843=FACE_BOUND ( 'NONE', #51957, .T. ) ;
#57845=DIRECTION ( 'NONE',  ( -0.000000000000000000, -0.5000000000000009992, -0.8660254037844380415 ) ) ;
#57846=ORIENTED_EDGE ( 'NONE', *, *, #89142, .F. ) ;
#57847=CARTESIAN_POINT ( 'NONE',  ( -15.23076923076935074, -5.219633306517616589, 34.19971097300220464 ) ) ;
#57848=DIRECTION ( 'NONE',  ( -0.000000000000000000, -0.6427876096865404731, -0.7660444431189771253 ) ) ;
#57849=CARTESIAN_POINT ( 'NONE',  ( 17.99999999999987566, -8.613356846316285953, 34.62446782046622218 ) ) ;
#57850=EDGE_LOOP ( 'NONE', ( #68255, #66689 ) ) ;
#57851=DIRECTION ( 'NONE',  ( -0.000000000000000000, -0.000000000000000000, -1.000000000000000000 ) ) ;
#57852=FACE_OUTER_BOUND ( 'NONE', #82286, .T. ) ;
#57853=ORIENTED_EDGE ( 'NONE', *, *, #84696, .T. ) ;
#57854=CARTESIAN_POINT ( 'NONE',  ( -6.673022611438605978, -9.148310452688871663, 34.47095581063188519 ) ) ;
#57856=CARTESIAN_POINT ( 'NONE',  ( -6.989160334032800570, -11.16473453929635440, 33.15142922261925662 ) ) ;
#57857=DIRECTION ( 'NONE',  ( -0.000000000000000000, 1.000000000000000000, 3.491481338843133355E-15 ) ) ;
#57859=CARTESIAN_POINT ( 'NONE',  ( -10.36533030374629938, -5.728107161865378494, 34.42597550085002922 ) ) ;
#57861=CARTESIAN_POINT ( 'NONE',  ( 8.069166690247241647, -2.889357225399416418, 32.26129605718031002 ) ) ;
#57862=CARTESIAN_POINT ( 'NONE',  ( -1.384615384615383471, -2.721908614388771852, 31.22303859784724978 ) ) ;
#57863=CARTESIAN_POINT ( 'NONE',  ( 7.846153846153846700, -4.661471528628507777, 34.16647553114623292 ) ) ;
#57864=DIRECTION ( 'NONE',  ( -0.000000000000000000, -0.3420201433256694346, -0.9396926207859080948 ) ) ;
#57865=CARTESIAN_POINT ( 'NONE',  ( -15.23076923076935074, -11.94971097300221174, 32.03036669348237098 ) ) ;
#57866=CARTESIAN_POINT ( 'NONE',  ( 5.076923076922953193, -2.657715359629662988, 31.77849191805970364 ) ) ;
#57867=CARTESIAN_POINT ( 'NONE',  ( -5.869474298236438514, -12.45806712695776319, 30.39783852428763922 ) ) ;
#57869=EDGE_LOOP ( 'NONE', ( #35944, #86779, #44508, #3799 ) ) ;
#57871=EDGE_LOOP ( 'NONE', ( #48217, #6372, #27978, #14406 ) ) ;
#57872=CARTESIAN_POINT ( 'NONE',  ( 9.442284455014730682, -6.695914987888146541, 34.68535235679833306 ) ) ;
#57873=VERTEX_POINT ( 'NONE', #72420 ) ;
#57874=CARTESIAN_POINT ( 'NONE',  ( -4.088590582570128973, -11.48612834413965977, 32.76840700105972815 ) ) ;
#57875=ORIENTED_EDGE ( 'NONE', *, *, #78502, .F. ) ;
#57876=CARTESIAN_POINT ( 'NONE',  ( -5.326923076923075762, -7.500000000000001776, 34.75000000000000000 ) ) ;
#57878=CARTESIAN_POINT ( 'NONE',  ( 7.623226887246995709, -8.282780595021769443, 34.94152052738834868 ) ) ;
#57879=CARTESIAN_POINT ( 'NONE',  ( 8.769230769230768274, -3.886160181151819604, 36.00935417666054406 ) ) ;
#57880=CARTESIAN_POINT ( 'NONE',  ( 13.44987052412822059, -3.083524468853784839, 32.58852847137153930 ) ) ;
#57881=LINE ( 'NONE', #71389, #63334 ) ;
#57882=DIRECTION ( 'NONE',  ( 1.000000000000000000, 0.000000000000000000, 0.000000000000000000 ) ) ;
#57883=CARTESIAN_POINT ( 'NONE',  ( 11.31553532094538994, -2.758268499246657068, 31.33685645148948140 ) ) ;
#57884=CARTESIAN_POINT ( 'NONE',  ( 2.307692307692309264, -12.34228464037088635, 31.77849191805839268 ) ) ;
#57886=CARTESIAN_POINT ( 'NONE',  ( -11.47239420511146157, -2.486705287966280320, 31.30864560766543647 ) ) ;
#57887=FACE_OUTER_BOUND ( 'NONE', #17702, .T. ) ;
#57888=CARTESIAN_POINT ( 'NONE',  ( 14.30769230769231015, -3.050289026998446396, 32.03036669348365706 ) ) ;
#57890=VECTOR ( 'NONE', #42492, 1000.000000000000000 ) ;
#57891=AXIS2_PLACEMENT_3D ( 'NONE', #81643, #68559, #34326 ) ;
#57892=ORIENTED_EDGE ( 'NONE', *, *, #26244, .F. ) ;
#57894=CARTESIAN_POINT ( 'NONE',  ( 12.46153846153833911, -8.656820664282941280, 34.87096338111179961 ) ) ;
#57895=CARTESIAN_POINT ( 'NONE',  ( 1.134638640566795420, -5.643011162660950042, 34.66104346484419096 ) ) ;
#57896=LINE ( 'NONE', #79061, #45557 ) ;
#57897=CARTESIAN_POINT ( 'NONE',  ( 15.10029252265276867, -7.276988635370452485, 34.74523720219453793 ) ) ;
#57900=CARTESIAN_POINT ( 'NONE',  ( -3.230769230769352962, -5.941354392335915335, 34.76329471203413846 ) ) ;
#57901=EDGE_CURVE ( 'NONE', #15863, #83740, #4411, .T. ) ;
#57902=ORIENTED_EDGE ( 'NONE', *, *, #52499, .F. ) ;
#57904=ORIENTED_EDGE ( 'NONE', *, *, #76055, .T. ) ;
#57905=ORIENTED_EDGE ( 'NONE', *, *, #59703, .T. ) ;
#57907=EDGE_CURVE ( 'NONE', #1726, #74923, #83644, .T. ) ;
#57908=CARTESIAN_POINT ( 'NONE',  ( -6.792286482109972212, -5.496552790871117367, 34.60292014791297532 ) ) ;
#57909=CARTESIAN_POINT ( 'NONE',  ( -8.899378738962466784, -2.373036134822904319, 30.88089517874952250 ) ) ;
#57910=ADVANCED_FACE ( 'NONE', ( #37301 ), #24228, .F. ) ;
#57912=CARTESIAN_POINT ( 'NONE',  ( 10.68063975489745232, -10.33852847137154107, 34.16647553114620450 ) ) ;
#57913=B_SPLINE_CURVE_WITH_KNOTS ( 'NONE', 3,
 ( #43216, #62590, #2215, #84660, #902, #83775 ),
 .UNSPECIFIED., .F., .F.,
 ( 4, 2, 4 ),
 ( 0.0003909512603273874185, 0.0005862562993132133804, 0.0007815613382990393423 ),
 .UNSPECIFIED. ) ;
#57914=ORIENTED_EDGE ( 'NONE', *, *, #32820, .T. ) ;
#57915=AXIS2_PLACEMENT_3D ( 'NONE', #68535, #33862, #68105 ) ;
#57916=B_SPLINE_CURVE_WITH_KNOTS ( 'NONE', 3,
 ( #52306, #45553, #72133, #79798, #59514, #3672, #2773, #73033, #65378, #11328 ),
 .UNSPECIFIED., .F., .F.,
 ( 4, 2, 2, 2, 4 ),
 ( 0.0007817359430256372700, 0.0009771253907250052138, 0.001172514838424373049, 0.001367904286123741101, 0.001563293733823108937 ),
 .UNSPECIFIED. ) ;
#57917=DIRECTION ( 'NONE',  ( -0.000000000000000000, 0.3420201433256694346, -0.9396926207859080948 ) ) ;
#57918=AXIS2_PLACEMENT_3D ( 'NONE', #31394, #58863, #16109 ) ;
#57919=VERTEX_POINT ( 'NONE', #52593 ) ;
#57920=VERTEX_POINT ( 'NONE', #80078 ) ;
#57922=CARTESIAN_POINT ( 'NONE',  ( -4.153846153846152411, -11.91647553114624181, 32.58852847137148245 ) ) ;
#57923=DIRECTION ( 'NONE',  ( 0.000000000000000000, 0.000000000000000000, 1.000000000000000000 ) ) ;
#57924=CYLINDRICAL_SURFACE ( 'NONE', #6333, 0.2500000000000002220 ) ;
#57925=CARTESIAN_POINT ( 'NONE',  ( -16.85414353565466783, -3.236590943229499473, 32.36255958852954251 ) ) ;
#57926=DIRECTION ( 'NONE',  ( 0.000000000000000000, 0.000000000000000000, 1.000000000000000000 ) ) ;
#57927=ORIENTED_EDGE ( 'NONE', *, *, #36088, .T. ) ;
#57930=VERTEX_POINT ( 'NONE', #78290 ) ;
#57931=CARTESIAN_POINT ( 'NONE',  ( 2.307692307692309264, -12.37446782046654192, 30.86335684631486131 ) ) ;
#57932=ORIENTED_EDGE ( 'NONE', *, *, #85795, .T. ) ;
#57933=CARTESIAN_POINT ( 'NONE',  ( -3.230769230768923084, -2.506253911140615021, 30.00000000000323297 ) ) ;
#57935=CARTESIAN_POINT ( 'NONE',  ( 2.530471976670375600, -9.418065098278011860, 34.63729479722530158 ) ) ;
#57937=ORIENTED_EDGE ( 'NONE', *, *, #24896, .T. ) ;
#57938=B_SPLINE_CURVE_WITH_KNOTS ( 'NONE', 3,
 ( #66342, #24452, #52371, #85730, #51922, #79860 ),
 .UNSPECIFIED., .F., .F.,
 ( 4, 2, 4 ),
 ( 0.0003909569690057804843, 0.0005862646681846042955, 0.0007815723673634281067 ),
 .UNSPECIFIED. ) ;
#57939=EDGE_CURVE ( 'NONE', #23981, #57246, #64314, .T. ) ;
#57940=CARTESIAN_POINT ( 'NONE',  ( -14.30769230769242917, -12.51329471203414379, 31.30864560766407578 ) ) ;
#57941=ORIENTED_EDGE ( 'NONE', *, *, #42620, .F. ) ;
#57942=LINE ( 'NONE', #2991, #21193 ) ;
#57943=CARTESIAN_POINT ( 'NONE',  ( 17.86930939688969033, -12.62707690430377383, 30.88035979386743435 ) ) ;
#57945=CARTESIAN_POINT ( 'NONE',  ( -14.98071481085577972, -2.920487667080175598, 32.31805714834170828 ) ) ;
#57946=CARTESIAN_POINT ( 'NONE',  ( -6.923076923077044142, -12.46129190930018460, 30.37095296980731973 ) ) ;
#57947=CARTESIAN_POINT ( 'NONE',  ( 4.853996859406926490, -3.105860786376062332, 32.13614157043599562 ) ) ;
#57948=EDGE_CURVE ( 'NONE', #40774, #62177, #17491, .T. ) ;
#57949=CARTESIAN_POINT ( 'NONE',  ( 16.02315468717859659, -2.541943142973489334, 30.39792223712631980 ) ) ;
#57950=DIRECTION ( 'NONE',  ( -1.000000000000000000, 0.000000000000000000, 0.000000000000000000 ) ) ;
#57951=ORIENTED_EDGE ( 'NONE', *, *, #70901, .T. ) ;
#57952=EDGE_CURVE ( 'NONE', #64392, #65658, #17936, .T. ) ;
#57953=CARTESIAN_POINT ( 'NONE',  ( -11.40793583669797506, -4.459921816937791661, 33.71989282347011851 ) ) ;
#57954=CARTESIAN_POINT ( 'NONE',  ( 4.946775107191379028, -4.299443229763728169, 33.91186481527756058 ) ) ;
#57955=ORIENTED_EDGE ( 'NONE', *, *, #13821, .F. ) ;
#57957=LINE ( 'NONE', #51619, #70980 ) ;
#57958=LINE ( 'NONE', #45326, #43001 ) ;
#57959=CARTESIAN_POINT ( 'NONE',  ( -4.023320452082591814, -2.619367082507848554, 30.83698974864644171 ) ) ;
#57960=LINE ( 'NONE', #5581, #70632 ) ;
#57961=CARTESIAN_POINT ( 'NONE',  ( -13.38461538461550759, -11.67786785259630911, 32.92929555188603530 ) ) ;
#57962=DIRECTION ( 'NONE',  ( 0.000000000000000000, 0.000000000000000000, -1.000000000000000000 ) ) ;
#57963=FACE_BOUND ( 'NONE', #3263, .T. ) ;
#57964=CARTESIAN_POINT ( 'NONE',  ( 12.46153846153846168, -9.905515769479276145, 34.41647553114623292 ) ) ;
#57965=CARTESIAN_POINT ( 'NONE',  ( 17.75002325595140462, -10.82459398097509862, 33.81372124010183455 ) ) ;
#57966=CARTESIAN_POINT ( 'NONE',  ( -18.13069060311030611, -8.191372820521383602, 34.95448215188424967 ) ) ;
#57967=CARTESIAN_POINT ( 'NONE',  ( -6.923076923077045919, -11.06231777344772027, 33.60647404775119895 ) ) ;
#57968=CARTESIAN_POINT ( 'NONE',  ( 9.942253210655836781, -4.336752205174649433, 33.62275283266504289 ) ) ;
#57969=CYLINDRICAL_SURFACE ( 'NONE', #59123, 0.2499999999999986955 ) ;
#57971=ORIENTED_EDGE ( 'NONE', *, *, #39432, .T. ) ;
#57972=CARTESIAN_POINT ( 'NONE',  ( -4.376772371362298131, -11.76352882383564769, 32.36236540154569497 ) ) ;
#57973=CARTESIAN_POINT ( 'NONE',  ( -4.853911725310228853, -3.105924265160262543, 32.13625925475356127 ) ) ;
#57974=CYLINDRICAL_SURFACE ( 'NONE', #64643, 0.2499999999999994726 ) ;
#57976=CARTESIAN_POINT ( 'NONE',  ( -4.153846153846274980, -5.094484230521993062, 34.41647553114689373 ) ) ;
#57977=CARTESIAN_POINT ( 'NONE',  ( -5.142174067084318345, -2.506253911140460477, 30.00000000000013856 ) ) ;
#57979=B_SPLINE_CURVE_WITH_KNOTS ( 'NONE', 3,
 ( #42449, #21726, #42011, #63593, #41556, #35696, #69470, #1460, #21275, #27595 ),
 .UNSPECIFIED., .F., .F.,
 ( 4, 2, 2, 2, 4 ),
 ( 0.000000000000000000, 0.0001954311584214071026, 0.0003908623168428142051, 0.0005862934752642213077, 0.0007817246336856284103 ),
 .UNSPECIFIED. ) ;
#57980=CARTESIAN_POINT ( 'NONE',  ( -1.634615384615383027, -7.433932668274255029, 35.00000000000000711 ) ) ;
#57981=CARTESIAN_POINT ( 'NONE',  ( -18.00000000000000000, -3.322132147404558200, 32.92929555188717217 ) ) ;
#57982=VECTOR ( 'NONE', #5516, 1000.000000000000114 ) ;
#57983=CARTESIAN_POINT ( 'NONE',  ( -8.069080805060693251, -2.889293201056495786, 32.26117774369186009 ) ) ;
#57984=DIRECTION ( 'NONE',  ( -0.000000000000000000, 0.8660254037844399289, -0.4999999999999980016 ) ) ;
#57985=CARTESIAN_POINT ( 'NONE',  ( -2.307692307692428724, -2.657715359629662544, 31.77849191805970364 ) ) ;
#57986=CARTESIAN_POINT ( 'NONE',  ( 12.39545608217832218, -12.62096338111211580, 30.90682066428152908 ) ) ;
#57987=AXIS2_PLACEMENT_3D ( 'NONE', #79304, #47166, #74659 ) ;
#57988=EDGE_CURVE ( 'NONE', #37091, #43657, #78740, .T. ) ;
#57989=LINE ( 'NONE', #36832, #49090 ) ;
#57990=CARTESIAN_POINT ( 'NONE',  ( 8.769230769230768274, -2.499999999999998668, 29.75000000000001421 ) ) ;
#57991=VERTEX_POINT ( 'NONE', #3516 ) ;
#57992=CARTESIAN_POINT ( 'NONE',  ( 15.00728430620490350, -11.60425143139329940, 33.02411095842164457 ) ) ;
#57993=DIRECTION ( 'NONE',  ( -0.000000000000000000, -0.1736481776669307198, -0.9848077530122080203 ) ) ;
#57995=CARTESIAN_POINT ( 'NONE',  ( -2.437840277424002888, -5.070767119584671967, 34.40440758774516183 ) ) ;
#57996=LINE ( 'NONE', #51210, #55577 ) ;
#57997=EDGE_LOOP ( 'NONE', ( #83421, #83792, #6469, #86607 ) ) ;
#57998=CARTESIAN_POINT ( 'NONE',  ( -17.93474486048716088, -6.835583212224609184, 34.95778746994559327 ) ) ;
#57999=CARTESIAN_POINT ( 'NONE',  ( 1.254468175177165801, -9.418419913701741919, 34.36755862841477693 ) ) ;
#58000=CARTESIAN_POINT ( 'NONE',  ( 3.930361210122205406, -5.912607949931405038, 34.49155766932282319 ) ) ;
#58002=CARTESIAN_POINT ( 'NONE',  ( -14.30769230769230660, -3.050289026998446396, 32.03036669348365706 ) ) ;
#58003=CARTESIAN_POINT ( 'NONE',  ( -2.307692307692428724, -12.70778746994576025, 30.41441678777401236 ) ) ;
#58004=EDGE_CURVE ( 'NONE', #6887, #64930, #44491, .T. ) ;
#58005=CARTESIAN_POINT ( 'NONE',  ( -5.011667505647053211, -9.442884908240271713, 34.35708131394835618 ) ) ;
#58006=EDGE_CURVE ( 'NONE', #58570, #79428, #45391, .T. ) ;
#58008=VERTEX_POINT ( 'NONE', #18825 ) ;
#58010=CARTESIAN_POINT ( 'NONE',  ( -11.53846153846153655, -12.34228464037088635, 31.77849191805839268 ) ) ;
#58012=CARTESIAN_POINT ( 'NONE',  ( 4.088575707885378385, -10.21337939537584383, 33.94971097300158647 ) ) ;
#58013=ORIENTED_EDGE ( 'NONE', *, *, #47212, .F. ) ;
#58014=ORIENTED_EDGE ( 'NONE', *, *, #58070, .T. ) ;
#58015=AXIS2_PLACEMENT_3D ( 'NONE', #70203, #62983, #57129 ) ;
#58016=ORIENTED_EDGE ( 'NONE', *, *, #59028, .F. ) ;
#58017=VECTOR ( 'NONE', #32359, 999.9999999999998863 ) ;
#58018=EDGE_CURVE ( 'NONE', #69663, #46391, #68338, .T. ) ;
#58020=CARTESIAN_POINT ( 'NONE',  ( 6.066067333350078528, -2.292212530054420494, 30.41441678777542990 ) ) ;
#58021=EDGE_CURVE ( 'NONE', #22897, #4699, #40871, .T. ) ;
#58022=DIRECTION ( 'NONE',  ( 0.000000000000000000, 0.1736481776669275834, 0.9848077530122086864 ) ) ;
#58023=DIRECTION ( 'NONE',  ( -0.000000000000000000, 0.3420201433256694346, -0.9396926207859080948 ) ) ;
#58024=ORIENTED_EDGE ( 'NONE', *, *, #66434, .F. ) ;
#58026=ORIENTED_EDGE ( 'NONE', *, *, #58018, .F. ) ;
#58027=CARTESIAN_POINT ( 'NONE',  ( 10.68057760367926790, -2.255955759149235629, 29.99999999999988987 ) ) ;
#58028=EDGE_LOOP ( 'NONE', ( #73814, #1546, #66536, #32665 ) ) ;
#58029=LINE ( 'NONE', #23788, #69721 ) ;
#58030=DIRECTION ( 'NONE',  ( -0.000000000000000000, -0.6427876096865404731, -0.7660444431189770143 ) ) ;
#58031=CARTESIAN_POINT ( 'NONE',  ( 15.90386940979756858, -11.47974371597207899, 33.17467449705390692 ) ) ;
#58032=VERTEX_POINT ( 'NONE', #46290 ) ;
#58033=VERTEX_POINT ( 'NONE', #33226 ) ;
#58034=CARTESIAN_POINT ( 'NONE',  ( -8.703975197954745724, -8.613356846314928816, 34.62446782046653482 ) ) ;
#58035=ORIENTED_EDGE ( 'NONE', *, *, #77740, .F. ) ;
#58037=CARTESIAN_POINT ( 'NONE',  ( 14.05766908347085220, -5.765609946408404518, 34.70566812827425451 ) ) ;
#58038=EDGE_CURVE ( 'NONE', #48024, #60048, #23471, .T. ) ;
#58039=VERTEX_POINT ( 'NONE', #19269 ) ;
#58042=DIRECTION ( 'NONE',  ( -0.000000000000000000, -0.6427876096865404731, -0.7660444431189771253 ) ) ;
#58043=FACE_BOUND ( 'NONE', #41324, .T. ) ;
#58044=CARTESIAN_POINT ( 'NONE',  ( 0.4615384615384611755, -6.681629849574314051, 35.83090037661290239 ) ) ;
#58045=CARTESIAN_POINT ( 'NONE',  ( -4.153846153846152411, -12.10708131394839349, 31.69288490824020244 ) ) ;
#58046=ADVANCED_FACE ( 'NONE', ( #32337 ), #80534, .F. ) ;
#58048=CARTESIAN_POINT ( 'NONE',  ( 16.37662582282421653, -4.226511098958373402, 33.85474049983370293 ) ) ;
#58049=CARTESIAN_POINT ( 'NONE',  ( -15.90379173393269596, -2.920487667080175154, 32.31805714834170828 ) ) ;
#58050=CARTESIAN_POINT ( 'NONE',  ( 11.40831432902331777, -11.47017969459903952, 32.78971311882035167 ) ) ;
#58052=ORIENTED_EDGE ( 'NONE', *, *, #12518, .F. ) ;
#58053=EDGE_CURVE ( 'NONE', #3642, #46562, #6276, .T. ) ;
#58054=CARTESIAN_POINT ( 'NONE',  ( 14.05769230769230838, -7.500000000000001776, 34.75000000000000000 ) ) ;
#58055=VERTEX_POINT ( 'NONE', #6635 ) ;
#58056=ORIENTED_EDGE ( 'NONE', *, *, #88088, .F. ) ;
#58057=CARTESIAN_POINT ( 'NONE',  ( -0.4615384615385826339, -3.300289026999228881, 32.46337939537708905 ) ) ;
#58058=CARTESIAN_POINT ( 'NONE',  ( 10.83816428436268176, -12.69155399931963046, 30.53255429739157734 ) ) ;
#58059=CARTESIAN_POINT ( 'NONE',  ( -4.153846153846274980, -12.70778746994576025, 30.41441678777401236 ) ) ;
#58060=CARTESIAN_POINT ( 'NONE',  ( 14.53070515178570510, -4.026326845037962343, 33.68677907613344047 ) ) ;
#58061=CARTESIAN_POINT ( 'NONE',  ( -11.53846153846165912, -6.026961402154118019, 34.52809138561165270 ) ) ;
#58062=LINE ( 'NONE', #43230, #49028 ) ;
#58063=EDGE_LOOP ( 'NONE', ( #50066, #82213, #62913, #16764 ) ) ;
#58065=AXIS2_PLACEMENT_3D ( 'NONE', #15178, #50710, #42652 ) ;
#58066=CARTESIAN_POINT ( 'NONE',  ( -14.98071491913091791, -9.943054286541403997, 34.11300777759954883 ) ) ;
#58067=FACE_OUTER_BOUND ( 'NONE', #12891, .T. ) ;
#58068=CARTESIAN_POINT ( 'NONE',  ( 0.3954560821783261182, -3.322132147404559976, 32.92929555188719348 ) ) ;
#58070=EDGE_CURVE ( 'NONE', #6072, #40774, #55700, .T. ) ;
#58073=VECTOR ( 'NONE', #37072, 1000.000000000000000 ) ;
#58075=CARTESIAN_POINT ( 'NONE',  ( 15.23076923076923173, -12.09954503811598769, 35.62045528018868623 ) ) ;
#58076=EDGE_CURVE ( 'NONE', #70789, #58120, #53644, .T. ) ;
#58077=VERTEX_POINT ( 'NONE', #60242 ) ;
#58078=CARTESIAN_POINT ( 'NONE',  ( -4.153846153846273204, -4.481592998941358097, 33.73612834414048933 ) ) ;
#58079=CARTESIAN_POINT ( 'NONE',  ( 17.74997677577853850, -11.56360843649121861, 33.07473185843129926 ) ) ;
#58080=CARTESIAN_POINT ( 'NONE',  ( -16.37733109757010652, -5.113361153441931428, 34.14387501736621999 ) ) ;
#58081=CARTESIAN_POINT ( 'NONE',  ( 13.63461538461538680, -7.500000000000001776, 35.04278698407183867 ) ) ;
#58083=CARTESIAN_POINT ( 'NONE',  ( 0.4615384615384611200, -9.058645607665452459, 34.76329471203371924 ) ) ;
#58084=ORIENTED_EDGE ( 'NONE', *, *, #1520, .F. ) ;
#58085=CARTESIAN_POINT ( 'NONE',  ( -12.71156169883143150, -10.76384336483936011, 33.53834819971076087 ) ) ;
#58086=CARTESIAN_POINT ( 'NONE',  ( -1.318547033612945896, -8.973038597847269315, 34.52809138561122637 ) ) ;
#58087=ORIENTED_EDGE ( 'NONE', *, *, #65855, .F. ) ;
#58088=CARTESIAN_POINT ( 'NONE',  ( -13.60754160213153163, -11.24512374952581872, 33.06303171183252942 ) ) ;
#58089=DIRECTION ( 'NONE',  ( -0.000000000000000000, -0.8660254037844399289, -0.4999999999999980016 ) ) ;
#58090=CARTESIAN_POINT ( 'NONE',  ( 2.307692307692187583, -3.300289026999228881, 32.46337939537708905 ) ) ;
#58091=EDGE_CURVE ( 'NONE', #62177, #52057, #24599, .T. ) ;
#58092=DIRECTION ( 'NONE',  ( -0.000000000000000000, 1.000000000000000000, -0.000000000000000000 ) ) ;
#58093=CARTESIAN_POINT ( 'NONE',  ( -10.61538461538461320, -8.810774026931790459, 35.74407628777942847 ) ) ;
#58094=CARTESIAN_POINT ( 'NONE',  ( -3.099977422944443006, -11.18335022499818621, 33.13157742990016885 ) ) ;
#58095=CARTESIAN_POINT ( 'NONE',  ( 15.36129493253279499, -11.46989282347013095, 32.79007818306219946 ) ) ;
#58098=CARTESIAN_POINT ( 'NONE',  ( -15.90379173393269951, -6.523592122091590895, 34.90882529074906415 ) ) ;
#58099=EDGE_CURVE ( 'NONE', #63192, #48024, #34550, .T. ) ;
#58100=CARTESIAN_POINT ( 'NONE',  ( -12.68441714396711006, -7.630691491037285168, 34.74850469731152458 ) ) ;
#58101=CARTESIAN_POINT ( 'NONE',  ( -17.32689982097166492, -4.818429247618091438, 34.26397095200675125 ) ) ;
#58103=EDGE_CURVE ( 'NONE', #15420, #69076, #72947, .T. ) ;
#58104=CARTESIAN_POINT ( 'NONE',  ( 0.4615384615384611200, -5.471508081941601098, 34.59228464037088457 ) ) ;
#58109=EDGE_LOOP ( 'NONE', ( #52506, #43919 ) ) ;
#58110=ADVANCED_FACE ( 'NONE', ( #75977 ), #50258, .F. ) ;
#58112=VERTEX_POINT ( 'NONE', #69223 ) ;
#58113=CARTESIAN_POINT ( 'NONE',  ( 14.30769230769218758, -12.27809138561165270, 31.22303859784587132 ) ) ;
#58114=CARTESIAN_POINT ( 'NONE',  ( 17.07692307692338218, -2.506253911140615021, 30.00000000000323297 ) ) ;
#58116=ORIENTED_EDGE ( 'NONE', *, *, #25752, .F. ) ;
#58117=CARTESIAN_POINT ( 'NONE',  ( -13.13466997523734037, -12.68172785388650681, 30.59649109432439218 ) ) ;
#58118=ORIENTED_EDGE ( 'NONE', *, *, #61801, .F. ) ;
#58119=CARTESIAN_POINT ( 'NONE',  ( -5.750054590621955342, -2.341251567377310217, 30.72681386836322659 ) ) ;
#58120=VERTEX_POINT ( 'NONE', #77304 ) ;
#58121=DIRECTION ( 'NONE',  ( -0.000000000000000000, 0.3420201433256694346, -0.9396926207859080948 ) ) ;
#58122=CYLINDRICAL_SURFACE ( 'NONE', #22483, 0.2500000000000008882 ) ;
#58123=EDGE_LOOP ( 'NONE', ( #30838, #78100, #62073, #59119 ) ) ;
#58124=CARTESIAN_POINT ( 'NONE',  ( 16.15384615384615330, -3.937682226553329556, 33.60647404775216529 ) ) ;
#58125=CARTESIAN_POINT ( 'NONE',  ( 11.53846153846153832, -1.790695186598648903, 34.54067556320373455 ) ) ;
#58126=EDGE_CURVE ( 'NONE', #65231, #70653, #89079, .T. ) ;
#58128=CARTESIAN_POINT ( 'NONE',  ( -5.076923076923075762, -2.499999999999998668, 29.75000000000001421 ) ) ;
#58129=CARTESIAN_POINT ( 'NONE',  ( -13.16160254052199008, -11.98016756924215009, 32.48728574198911190 ) ) ;
#58130=VERTEX_POINT ( 'NONE', #62017 ) ;
#58132=ORIENTED_EDGE ( 'NONE', *, *, #37165, .T. ) ;
#58133=CARTESIAN_POINT ( 'NONE',  ( 8.638539302563209787, -3.530157926970578952, 32.79014554554150607 ) ) ;
#58134=ORIENTED_EDGE ( 'NONE', *, *, #34902, .F. ) ;
#58135=AXIS2_PLACEMENT_3D ( 'NONE', #40980, #13062, #26578 ) ;
#58137=CARTESIAN_POINT ( 'NONE',  ( -8.835314180186648159, -9.780366693483667717, 34.19971097300155805 ) ) ;
#58138=CARTESIAN_POINT ( 'NONE',  ( 9.469380733400845074, -5.582147617184174848, 34.63737895849758530 ) ) ;
#58139=ORIENTED_EDGE ( 'NONE', *, *, #80541, .F. ) ;
#58142=CARTESIAN_POINT ( 'NONE',  ( 3.361561038594017337, -4.809403383903226192, 33.96459661697924304 ) ) ;
#58144=CARTESIAN_POINT ( 'NONE',  ( 11.76124107972994182, -11.41317474335729543, 32.86274602512330034 ) ) ;
#58145=CARTESIAN_POINT ( 'NONE',  ( 16.82689985270161515, -12.45566812827425096, 31.48439005359158926 ) ) ;
#58146=CARTESIAN_POINT ( 'NONE',  ( 14.30769230769218581, -12.16647553114689728, 32.15551576947799362 ) ) ;
#58147=FACE_BOUND ( 'NONE', #24503, .T. ) ;
#58149=CARTESIAN_POINT ( 'NONE',  ( 12.46153846153833911, -6.026961402154118019, 34.52809138561165270 ) ) ;
#58150=EDGE_CURVE ( 'NONE', #8365, #40118, #14728, .T. ) ;
#58151=CARTESIAN_POINT ( 'NONE',  ( -17.07692307692307665, -2.249999999999998668, 29.75000000000001776 ) ) ;
#58152=CARTESIAN_POINT ( 'NONE',  ( 8.769230769230768274, -3.050289026998446396, 32.03036669348365706 ) ) ;
#58153=CARTESIAN_POINT ( 'NONE',  ( 17.29970261819148902, -9.332535724633405749, 34.40230450496446224 ) ) ;
#58154=ORIENTED_EDGE ( 'NONE', *, *, #66473, .T. ) ;
#58156=CARTESIAN_POINT ( 'NONE',  ( 9.942307692307695177, -7.500000000000001776, 35.04278698407183867 ) ) ;
#58157=ORIENTED_EDGE ( 'NONE', *, *, #78957, .T. ) ;
#58162=EDGE_CURVE ( 'NONE', #22613, #49527, #56592, .T. ) ;
#58163=DIRECTION ( 'NONE',  ( -0.000000000000000000, -0.3420201433256694901, -0.9396926207859082059 ) ) ;
#58165=CARTESIAN_POINT ( 'NONE',  ( 16.82692307692307665, -7.500000000000001776, 34.75000000000000000 ) ) ;
#58166=CARTESIAN_POINT ( 'NONE',  ( -15.36091720050092846, -3.625366637846544116, 33.29286588640298561 ) ) ;
#58167=ORIENTED_EDGE ( 'NONE', *, *, #87315, .T. ) ;
#58168=DIRECTION ( 'NONE',  ( 0.000000000000000000, 0.9396926207859126468, 0.3420201433256571111 ) ) ;
#58169=CARTESIAN_POINT ( 'NONE',  ( 3.230769230769108269, -9.528491918059723176, 34.59228464037033035 ) ) ;
#58170=CARTESIAN_POINT ( 'NONE',  ( 11.76142444202302961, -7.369474270740069777, 34.74850911626239736 ) ) ;
#58171=CARTESIAN_POINT ( 'NONE',  ( 13.16113044089144068, -12.44517049084099725, 30.48991314939691932 ) ) ;
#58172=ORIENTED_EDGE ( 'NONE', *, *, #20152, .F. ) ;
#58174=ORIENTED_EDGE ( 'NONE', *, *, #78938, .F. ) ;
#58175=FACE_BOUND ( 'NONE', #87414, .T. ) ;
#58176=ORIENTED_EDGE ( 'NONE', *, *, #88949, .F. ) ;
#58177=CARTESIAN_POINT ( 'NONE',  ( 18.06606733335007675, -12.62096338111211757, 30.90682066428152908 ) ) ;
#58178=CARTESIAN_POINT ( 'NONE',  ( -13.38461538461538325, -10.51840700105979565, 33.73612834413961536 ) ) ;
#58179=ORIENTED_EDGE ( 'NONE', *, *, #70191, .F. ) ;
#58180=DIRECTION ( 'NONE',  ( 0.000000000000000000, 0.000000000000000000, 1.000000000000000000 ) ) ;
#58181=CARTESIAN_POINT ( 'NONE',  ( 6.249945409378044658, -11.56426240980093745, 33.07394671870546432 ) ) ;
#58182=CARTESIAN_POINT ( 'NONE',  ( -8.638438961405983108, -6.413143153341454017, 34.63066358083362672 ) ) ;
#58183=B_SPLINE_CURVE_WITH_KNOTS ( 'NONE', 3,
 ( #5717, #80045, #4835, #53000, #86379, #60653, #88165, #45807, #11592, #46702 ),
 .UNSPECIFIED., .F., .F.,
 ( 4, 2, 2, 2, 4 ),
 ( 0.0007817359430256216575, 0.0009771253907249856981, 0.001172514838424349847, 0.001367904286123713779, 0.001563293733823077928 ),
 .UNSPECIFIED. ) ;
#58184=CARTESIAN_POINT ( 'NONE',  ( -6.673131404728781746, -3.202959910592335202, 32.30730279482227019 ) ) ;
#58185=ORIENTED_EDGE ( 'NONE', *, *, #23485, .T. ) ;
#58186=CARTESIAN_POINT ( 'NONE',  ( -4.088590582570128973, -6.879047030191282275, 34.71129190930002295 ) ) ;
#58187=ORIENTED_EDGE ( 'NONE', *, *, #66417, .F. ) ;
#58188=CARTESIAN_POINT ( 'NONE',  ( 16.82694634598072270, -10.66389620160130036, 33.62221079203477103 ) ) ;
#58189=VERTEX_POINT ( 'NONE', #35433 ) ;
#58190=CARTESIAN_POINT ( 'NONE',  ( -7.780085495151407571, -8.973038597847271092, 34.52809138561121216 ) ) ;
#58192=CARTESIAN_POINT ( 'NONE',  ( 12.46153846153846168, -1.044019251281081972, 31.83374038241031911 ) ) ;
#58193=CARTESIAN_POINT ( 'NONE',  ( -4.153846153846273204, -12.46129190930018460, 30.37095296980731973 ) ) ;
#58194=CARTESIAN_POINT ( 'NONE',  ( 0.4615384615384611200, -12.78798330534103123, 29.99999999999997868 ) ) ;
#58195=AXIS2_PLACEMENT_3D ( 'NONE', #82784, #21056, #14310 ) ;
#58198=ORIENTED_EDGE ( 'NONE', *, *, #44725, .F. ) ;
#58199=ADVANCED_FACE ( 'NONE', ( #83642 ), #8412, .F. ) ;
#58200=B_SPLINE_CURVE_WITH_KNOTS ( 'NONE', 3,
 ( #1953, #77611, #57336, #71282, #37052, #28547, #83496, #83942, #29438, #84830 ),
 .UNSPECIFIED., .F., .F.,
 ( 4, 2, 2, 2, 4 ),
 ( 0.0007817359430256372700, 0.0009771253907250052138, 0.001172514838424373266, 0.001367904286123741101, 0.001563293733823109153 ),
 .UNSPECIFIED. ) ;
#58201=VECTOR ( 'NONE', #54257, 1000.000000000000000 ) ;
#58202=CARTESIAN_POINT ( 'NONE',  ( -15.10024352900566491, -3.816742781228458004, 33.13167719472716044 ) ) ;
#58203=FACE_OUTER_BOUND ( 'NONE', #41351, .T. ) ;
#58205=VERTEX_POINT ( 'NONE', #70550 ) ;
#58206=VERTEX_POINT ( 'NONE', #8859 ) ;
#58207=CARTESIAN_POINT ( 'NONE',  ( -11.66860874789975888, -10.88202310037935661, 33.43294751532457099 ) ) ;
#58208=CARTESIAN_POINT ( 'NONE',  ( 7.596177102105253987, -6.524016743844655686, 34.90889640711025521 ) ) ;
#58209=CARTESIAN_POINT ( 'NONE',  ( 6.250054311638314708, -11.28795663066794219, 33.01431243580653785 ) ) ;
#58210=CARTESIAN_POINT ( 'NONE',  ( 9.468822748583747284, -12.44517049084099725, 30.48991314939691932 ) ) ;
#58211=CARTESIAN_POINT ( 'NONE',  ( 6.923076923076924238, -9.584722331328613620, 36.20867863119891439 ) ) ;
#58212=EDGE_CURVE ( 'NONE', #78414, #24781, #36329, .T. ) ;
#58214=FACE_OUTER_BOUND ( 'NONE', #57085, .T. ) ;
#58215=EDGE_LOOP ( 'NONE', ( #14436, #59161 ) ) ;
#58216=LINE ( 'NONE', #50576, #53490 ) ;
#58217=CARTESIAN_POINT ( 'NONE',  ( -17.20753343654760315, -7.722926236386454590, 34.74524107206102030 ) ) ;
#58218=EDGE_CURVE ( 'NONE', #25874, #77885, #70709, .T. ) ;
#58220=B_SPLINE_CURVE_WITH_KNOTS ( 'NONE', 3,
 ( #62368, #57391, #22717, #21398, #52407, #57841, #30807, #65485, #3783, #31258 ),
 .UNSPECIFIED., .F., .F.,
 ( 4, 2, 2, 2, 4 ),
 ( 0.000000000000000000, 0.0001954339857564082062, 0.0003908679715128164124, 0.0005863019572692246186, 0.0007817359430256328248 ),
 .UNSPECIFIED. ) ;
#58221=CARTESIAN_POINT ( 'NONE',  ( -5.869952393744314989, -7.723484964179500700, 34.74522123443823318 ) ) ;
#58223=B_SPLINE_CURVE_WITH_KNOTS ( 'NONE', 3,
 ( #10218, #24159, #51614, #44872, #10659, #38126, #65585, #72791, #38577, #66031 ),
 .UNSPECIFIED., .F., .F.,
 ( 4, 2, 2, 2, 4 ),
 ( 0.000000000000000000, 0.0001954311564186873623, 0.0003908623128373747246, 0.0005862934692560620598, 0.0007817246256747494492 ),
 .UNSPECIFIED. ) ;
#58224=ORIENTED_EDGE ( 'NONE', *, *, #37749, .T. ) ;
#58227=CARTESIAN_POINT ( 'NONE',  ( -17.30040800148741553, -2.612411019501189813, 31.66733052389439962 ) ) ;
#58229=CARTESIAN_POINT ( 'NONE',  ( 10.61538461538461675, -11.91647553114624181, 32.58852847137148245 ) ) ;
#58230=ORIENTED_EDGE ( 'NONE', *, *, #88574, .F. ) ;
#58231=CARTESIAN_POINT ( 'NONE',  ( 5.777073782483852504, -9.886141570436013382, 34.14413921362392301 ) ) ;
#58233=DIRECTION ( 'NONE',  ( -0.000000000000000000, 0.7660444431189791237, -0.6427876096865379196 ) ) ;
#58235=VECTOR ( 'NONE', #72817, 1000.000000000000114 ) ;
#58236=LINE ( 'NONE', #10949, #56672 ) ;
#58237=DIRECTION ( 'NONE',  ( -0.000000000000000000, 0.3420201433256694346, -0.9396926207859080948 ) ) ;
#58238=ADVANCED_FACE ( 'NONE', ( #16050 ), #50703, .F. ) ;
#58239=EDGE_CURVE ( 'NONE', #43247, #2381, #43518, .T. ) ;
#58240=VERTEX_POINT ( 'NONE', #53266 ) ;
#58241=CARTESIAN_POINT ( 'NONE',  ( -0.6844646790546090598, -8.239355502252617924, 34.69524867566427417 ) ) ;
#58242=EDGE_LOOP ( 'NONE', ( #45571, #72088, #8251, #65497 ) ) ;
#58244=CARTESIAN_POINT ( 'NONE',  ( 4.826899839630110378, -12.22074536777954989, 31.39888409691088356 ) ) ;
#58245=CARTESIAN_POINT ( 'NONE',  ( 7.173022332454966232, -2.986452184633680673, 32.43230066228895225 ) ) ;
#58246=CARTESIAN_POINT ( 'NONE',  ( 9.822833130541335223, -2.647132371071621471, 31.75357179365171589 ) ) ;
#58247=CARTESIAN_POINT ( 'NONE',  ( 1.254467414883692067, -8.630895178749536711, 34.87696386517710323 ) ) ;
#58248=CARTESIAN_POINT ( 'NONE',  ( 15.93036122928182330, -12.11044203135681840, 32.26167407432752299 ) ) ;
#58249=VERTEX_POINT ( 'NONE', #52821 ) ;
#58250=ORIENTED_EDGE ( 'NONE', *, *, #67088, .F. ) ;
#58251=B_SPLINE_CURVE_WITH_KNOTS ( 'NONE', 3,
 ( #37726, #16568, #30090, #50779, #24206, #71072, #71954, #10265, #52567, #51663 ),
 .UNSPECIFIED., .F., .F.,
 ( 4, 2, 2, 2, 4 ),
 ( 0.0007817359430256392216, 0.0009771253907250073822, 0.001172514838424375651, 0.001367904286123743920, 0.001563293733823112189 ),
 .UNSPECIFIED. ) ;
#58252=EDGE_LOOP ( 'NONE', ( #58035, #84811 ) ) ;
#58253=EDGE_LOOP ( 'NONE', ( #44617, #7530 ) ) ;
#58254=AXIS2_PLACEMENT_3D ( 'NONE', #78008, #16313, #51850 ) ;
#58255=DIRECTION ( 'NONE',  ( 0.000000000000000000, 0.7660444431189807890, 0.6427876096865361433 ) ) ;
#58256=CARTESIAN_POINT ( 'NONE',  ( -3.361459833879538284, -6.369640206132550553, 34.87707690430378449 ) ) ;
#58257=CARTESIAN_POINT ( 'NONE',  ( -5.207399785039540596, -7.276988635370452485, 34.74523720219453793 ) ) ;
#58258=CARTESIAN_POINT ( 'NONE',  ( -13.38461538461538325, -4.098570777380720287, 33.41473453929634729 ) ) ;
#58260=ADVANCED_FACE ( 'NONE', ( #80766 ), #23242, .F. ) ;
#58261=CARTESIAN_POINT ( 'NONE',  ( 14.30769230769218758, -12.46129190930018460, 30.37095296980731973 ) ) ;
#58262=CARTESIAN_POINT ( 'NONE',  ( -5.999999999999998224, -4.661471528628507777, 34.16647553114623292 ) ) ;
#58263=CARTESIAN_POINT ( 'NONE',  ( -3.931066612577743147, -10.81320215134717344, 33.49497208177562868 ) ) ;
#58264=ORIENTED_EDGE ( 'NONE', *, *, #44168, .T. ) ;
#58265=ORIENTED_EDGE ( 'NONE', *, *, #6488, .T. ) ;
#58266=ORIENTED_EDGE ( 'NONE', *, *, #2106, .F. ) ;
#58267=CARTESIAN_POINT ( 'NONE',  ( 6.222779668978067669, -12.47679350104403007, 31.42216943046555855 ) ) ;
#58269=CARTESIAN_POINT ( 'NONE',  ( 0.4615384615383396616, -8.613356846316285953, 34.62446782046622218 ) ) ;
#58270=CARTESIAN_POINT ( 'NONE',  ( -17.77722033102192967, -11.60474049983370470, 33.02348890104160262 ) ) ;
#58271=EDGE_CURVE ( 'NONE', #81602, #5877, #66403, .T. ) ;
#58272=CYLINDRICAL_SURFACE ( 'NONE', #50371, 0.2499999999999994726 ) ;
#58273=CARTESIAN_POINT ( 'NONE',  ( 5.076923076922953193, -6.835583212225970762, 34.95778746994575670 ) ) ;
#58274=ORIENTED_EDGE ( 'NONE', *, *, #53449, .F. ) ;
#58275=ORIENTED_EDGE ( 'NONE', *, *, #35386, .T. ) ;
#58276=CARTESIAN_POINT ( 'NONE',  ( -2.307692307691999289, -2.506253911140615021, 30.00000000000323297 ) ) ;
#58277=VERTEX_POINT ( 'NONE', #19050 ) ;
#58278=FACE_BOUND ( 'NONE', #32874, .T. ) ;
#58279=B_SPLINE_CURVE_WITH_KNOTS ( 'NONE', 3,
 ( #16198, #78778, #45433, #4453, #51274, #24270, #72020, #77895, #36904, #2665 ),
 .UNSPECIFIED., .F., .F.,
 ( 4, 2, 2, 2, 4 ),
 ( 0.0007817246256747516176, 0.0009771112852218965736, 0.001172497944769041638, 0.001367884604316186702, 0.001563271263863331550 ),
 .UNSPECIFIED. ) ;
#58280=CARTESIAN_POINT ( 'NONE',  ( 13.63466980452883526, -12.41089969410671223, 31.60739465890703670 ) ) ;
#58281=LINE ( 'NONE', #17305, #24714 ) ;
#58282=ORIENTED_EDGE ( 'NONE', *, *, #50533, .T. ) ;
#58283=CARTESIAN_POINT ( 'NONE',  ( 2.084766090176161324, -8.239355502252617924, 34.69524867566427417 ) ) ;
#58284=DIRECTION ( 'NONE',  ( -0.000000000000000000, -0.5000000000000009992, -0.8660254037844380415 ) ) ;
#58285=CARTESIAN_POINT ( 'NONE',  ( -18.22348492456433178, -4.225889041578354544, 33.85425143139329407 ) ) ;
#58287=CARTESIAN_POINT ( 'NONE',  ( 12.33139125210024112, -5.195881422630166391, 34.18770438780619259 ) ) ;
#58288=CARTESIAN_POINT ( 'NONE',  ( 7.596153846153846700, -2.249999999999998668, 29.75000000000000355 ) ) ;
#58289=ORIENTED_EDGE ( 'NONE', *, *, #89105, .F. ) ;
#58291=ADVANCED_FACE ( 'NONE', ( #16492 ), #46522, .F. ) ;
#58292=CARTESIAN_POINT ( 'NONE',  ( 6.222963134266677798, -7.369474539155828730, 34.99858011523957657 ) ) ;
#58293=CARTESIAN_POINT ( 'NONE',  ( -9.692307692307691624, -9.058645607665452459, 34.76329471203371924 ) ) ;
#58294=ORIENTED_EDGE ( 'NONE', *, *, #18391, .F. ) ;
#58295=CARTESIAN_POINT ( 'NONE',  ( 7.846153846153725020, -5.219633306517616589, 34.19971097300220464 ) ) ;
#58296=CARTESIAN_POINT ( 'NONE',  ( -2.057692307692306599, -2.249999999999998668, 29.75000000000000355 ) ) ;
#58297=FACE_OUTER_BOUND ( 'NONE', #30244, .T. ) ;
#58298=CARTESIAN_POINT ( 'NONE',  ( 14.98074600654777377, -12.68155406624981119, 30.59749803192733708 ) ) ;
#58299=CARTESIAN_POINT ( 'NONE',  ( 7.846153846153725020, -8.613356846316285953, 34.62446782046622218 ) ) ;
#58300=CARTESIAN_POINT ( 'NONE',  ( 6.250054311638317373, -9.943054286541403997, 34.11300777759954883 ) ) ;
#58301=CARTESIAN_POINT ( 'NONE',  ( -14.30769230769230660, -9.058645607665452459, 34.76329471203371924 ) ) ;
#58302=CARTESIAN_POINT ( 'NONE',  ( 2.530703659305158837, -9.886259254753566594, 34.14407573483972413 ) ) ;
#58303=CARTESIAN_POINT ( 'NONE',  ( -0.3307480205715115917, -8.191423895709840863, 34.95447573519442130 ) ) ;
#58304=CARTESIAN_POINT ( 'NONE',  ( -15.45425417449318317, -11.89387501736622710, 32.13663884655806413 ) ) ;
#58305=CARTESIAN_POINT ( 'NONE',  ( -8.769230769230455635, -2.255955759149395501, 30.00000000000324363 ) ) ;
#58307=EDGE_LOOP ( 'NONE', ( #12331, #65558, #27, #80802 ) ) ;
#58308=CARTESIAN_POINT ( 'NONE',  ( 18.06525557127601900, -11.94971097300157403, 32.03036669348361443 ) ) ;
#58309=ORIENTED_EDGE ( 'NONE', *, *, #4243, .T. ) ;
#58311=ORIENTED_EDGE ( 'NONE', *, *, #87530, .F. ) ;
#58312=EDGE_CURVE ( 'NONE', #60815, #35903, #85396, .T. ) ;
#58313=CARTESIAN_POINT ( 'NONE',  ( -13.13456096470193302, -2.318338780012835443, 30.59689888758630261 ) ) ;
#58315=CARTESIAN_POINT ( 'NONE',  ( 1.384615384615264011, -12.16647553114689728, 32.15551576947799362 ) ) ;
#58317=CARTESIAN_POINT ( 'NONE',  ( -14.30769230769230660, -13.75783147151868846, 33.36296068462461051 ) ) ;
#58318=EDGE_CURVE ( 'NONE', #25852, #42793, #39447, .T. ) ;
#58319=CARTESIAN_POINT ( 'NONE',  ( -9.915792616872025178, -12.69144148231606017, 30.53333754910549303 ) ) ;
#58321=CARTESIAN_POINT ( 'NONE',  ( -12.46153846153846168, -3.937682226553329556, 33.60647404775216529 ) ) ;
#58323=DIRECTION ( 'NONE',  ( 0.000000000000000000, 0.7660444431189807890, 0.6427876096865361433 ) ) ;
#58326=CARTESIAN_POINT ( 'NONE',  ( 1.318531973659506251, -2.721908614388772296, 31.22303859784725688 ) ) ;
#58327=CARTESIAN_POINT ( 'NONE',  ( 13.31853300525525086, -3.322132147404559532, 32.92929555188719348 ) ) ;
#58328=ADVANCED_FACE ( 'NONE', ( #33886 ), #40658, .F. ) ;
#58329=CARTESIAN_POINT ( 'NONE',  ( -13.38461538461550759, -11.06231777344772027, 33.60647404775119895 ) ) ;
#58330=ORIENTED_EDGE ( 'NONE', *, *, #8671, .T. ) ;
#58332=CARTESIAN_POINT ( 'NONE',  ( -17.32689980786543060, -8.303909089506435137, 34.68538101551103381 ) ) ;
#58333=CARTESIAN_POINT ( 'NONE',  ( 1.253924781505079133, -10.70098750199973203, 33.91152734681376302 ) ) ;
#58334=DIRECTION ( 'NONE',  ( 0.000000000000000000, 0.000000000000000000, 1.000000000000000000 ) ) ;
#58335=AXIS2_PLACEMENT_3D ( 'NONE', #39685, #66240, #80216 ) ;
#58336=CARTESIAN_POINT ( 'NONE',  ( 8.639083559792549494, -11.93770438780619259, 32.05411857736982029 ) ) ;
#58337=CARTESIAN_POINT ( 'NONE',  ( -3.165514091256391715, -5.941354392334606160, 34.76329471203374055 ) ) ;
#58338=EDGE_CURVE ( 'NONE', #30672, #85857, #6429, .T. ) ;
#58339=ORIENTED_EDGE ( 'NONE', *, *, #7963, .T. ) ;
#58340=CARTESIAN_POINT ( 'NONE',  ( -1.134561072977068319, -9.943054286541400444, 34.11300777759954883 ) ) ;
#58341=ORIENTED_EDGE ( 'NONE', *, *, #75807, .F. ) ;
#58342=VERTEX_POINT ( 'NONE', #62239 ) ;
#58343=CARTESIAN_POINT ( 'NONE',  ( -9.469528023329624844, -3.020022701398813236, 32.48759521482552515 ) ) ;
#58344=CARTESIAN_POINT ( 'NONE',  ( -6.700297254098854793, -5.827830569534416583, 34.72679350104403539 ) ) ;
#58345=VECTOR ( 'NONE', #20660, 1000.000000000000114 ) ;
#58346=CARTESIAN_POINT ( 'NONE',  ( -0.7115384615384606759, -7.433932668274254141, 35.00000000000001421 ) ) ;
#58347=DIRECTION ( 'NONE',  ( 0.000000000000000000, 0.9848077530122072432, 0.1736481776669354937 ) ) ;
#58348=CARTESIAN_POINT ( 'NONE',  ( -5.300408001487407539, -8.539481045369598178, 34.89627647299170832 ) ) ;
#58349=ORIENTED_EDGE ( 'NONE', *, *, #49384, .F. ) ;
#58350=ORIENTED_EDGE ( 'NONE', *, *, #64503, .F. ) ;
#58351=VERTEX_POINT ( 'NONE', #41536 ) ;
#58352=CARTESIAN_POINT ( 'NONE',  ( -7.146003881983769901, -11.98009711892699691, 32.48740034544075428 ) ) ;
#58353=CARTESIAN_POINT ( 'NONE',  ( 8.546304551714621667, -2.758268499246657068, 31.33685645148948140 ) ) ;
#58354=CARTESIAN_POINT ( 'NONE',  ( 8.834485908743602067, -5.941354392334607049, 34.76329471203374055 ) ) ;
#58355=B_SPLINE_CURVE_WITH_KNOTS ( 'NONE', 3,
 ( #38495, #26638, #33402, #88366, #31741, #30834, #58304, #58757, #85798, #57865 ),
 .UNSPECIFIED., .F., .F.,
 ( 4, 2, 2, 2, 4 ),
 ( 0.000000000000000000, 0.0001954339857564097241, 0.0003908679715128194482, 0.0005863019572692291723, 0.0007817359430256388964 ),
 .UNSPECIFIED. ) ;
#58356=CARTESIAN_POINT ( 'NONE',  ( 1.318531973659505585, -3.513871655860377086, 32.76840700105978499 ) ) ;
#58357=CARTESIAN_POINT ( 'NONE',  ( 11.40831356872984337, -11.04286588640298561, 33.62463336215343901 ) ) ;
#58358=FACE_OUTER_BOUND ( 'NONE', #1798, .T. ) ;
#58360=EDGE_LOOP ( 'NONE', ( #70579, #81716 ) ) ;
#58362=ORIENTED_EDGE ( 'NONE', *, *, #85493, .F. ) ;
#58363=CARTESIAN_POINT ( 'NONE',  ( 2.557746619330623528, -12.41262288849542017, 30.68299917996395010 ) ) ;
#58364=VERTEX_POINT ( 'NONE', #47842 ) ;
#58365=CARTESIAN_POINT ( 'NONE',  ( 1.384615384615386802, -7.500000000000001776, 35.04278698407183867 ) ) ;
#58366=CARTESIAN_POINT ( 'NONE',  ( 9.692307692307695177, -13.20930481340135110, 34.54067556320372745 ) ) ;
#58369=ORIENTED_EDGE ( 'NONE', *, *, #10944, .T. ) ;
#58370=B_SPLINE_CURVE_WITH_KNOTS ( 'NONE', 3,
 ( #82688, #20524, #88131, #259, #27721, #19202, #33604, #53868, #55192, #41688 ),
 .UNSPECIFIED., .F., .F.,
 ( 4, 2, 2, 2, 4 ),
 ( 0.000000000000000000, 0.0001954339857564083417, 0.0003908679715128166835, 0.0005863019572692250523, 0.0007817359430256333669 ),
 .UNSPECIFIED. ) ;
#58371=CARTESIAN_POINT ( 'NONE',  ( -13.45069879557126313, -12.10708131394839349, 31.69288490824020244 ) ) ;
#58372=ORIENTED_EDGE ( 'NONE', *, *, #86954, .T. ) ;
#58373=CARTESIAN_POINT ( 'NONE',  ( -8.899378738962466784, -5.070767119584671079, 34.40440758774516183 ) ) ;
#58374=CARTESIAN_POINT ( 'NONE',  ( 10.74591031714818357, -9.417988943895561960, 34.36773134775777550 ) ) ;
#58375=B_SPLINE_CURVE_WITH_KNOTS ( 'NONE', 3,
 ( #13023, #33740, #61195, #16455, #71387, #43923, #2925, #9693, #85812, #30414 ),
 .UNSPECIFIED., .F., .F.,
 ( 4, 2, 2, 2, 4 ),
 ( 0.000000000000000000, 0.0001954339857564064444, 0.0003908679715128128888, 0.0005863019572692193060, 0.0007817359430256257775 ),
 .UNSPECIFIED. ) ;
#58377=CARTESIAN_POINT ( 'NONE',  ( 10.83834751894610093, -7.369474270740069777, 34.74850911626239736 ) ) ;
#58378=CARTESIAN_POINT ( 'NONE',  ( -6.700297381808513641, -2.600157965045225339, 30.74683119005207743 ) ) ;
#58379=CARTESIAN_POINT ( 'NONE',  ( 8.519207531937803779, -5.851115903089112003, 34.47074536777953568 ) ) ;
#58380=CARTESIAN_POINT ( 'NONE',  ( -22.75000000000000000, -10.50000000000000000, 27.25000000000000000 ) ) ;
#58382=CARTESIAN_POINT ( 'NONE',  ( -11.47239318745910452, -12.10708131394839882, 31.69288490824020954 ) ) ;
#58384=CARTESIAN_POINT ( 'NONE',  ( -8.992715693795101828, -4.225889041578353655, 33.85425143139329407 ) ) ;
#58385=VERTEX_POINT ( 'NONE', #81203 ) ;
#58386=CARTESIAN_POINT ( 'NONE',  ( -12.33101302330481808, -3.625058011473228703, 33.29252011169590020 ) ) ;
#58387=CARTESIAN_POINT ( 'NONE',  ( 15.45354877203763522, -4.387253974876679230, 33.66317474335728832 ) ) ;
#58390=CARTESIAN_POINT ( 'NONE',  ( -8.096153846153844924, -7.433932668274256805, 35.00000000000000711 ) ) ;
#58391=FACE_BOUND ( 'NONE', #12953, .T. ) ;
#58392=CARTESIAN_POINT ( 'NONE',  ( 13.31934538405906565, -2.379036618887870436, 30.90682066428147934 ) ) ;
#58393=CARTESIAN_POINT ( 'NONE',  ( 17.93472999944368240, -11.06231777344662959, 33.60647404775220082 ) ) ;
#58394=DIRECTION ( 'NONE',  ( -0.000000000000000000, -0.000000000000000000, -1.000000000000000000 ) ) ;
#58395=CARTESIAN_POINT ( 'NONE',  ( -13.63461538461538325, -2.249999999999998668, 29.75000000000000355 ) ) ;
#58396=CARTESIAN_POINT ( 'NONE',  ( 10.61538461538449418, -12.16647553114689728, 32.15551576947799362 ) ) ;
#58398=CARTESIAN_POINT ( 'NONE',  ( -14.30769230769230660, -9.819645486525091727, 36.12317359536749706 ) ) ;
#58400=VERTEX_POINT ( 'NONE', #60915 ) ;
#58401=EDGE_CURVE ( 'NONE', #10136, #51826, #5986, .T. ) ;
#58402=CARTESIAN_POINT ( 'NONE',  ( -8.069638789877794594, -11.41268669641500466, 32.86336882939237825 ) ) ;
#58404=CARTESIAN_POINT ( 'NONE',  ( -14.55771554498526932, -6.695914987888146541, 34.68535235679833306 ) ) ;
#58405=CARTESIAN_POINT ( 'NONE',  ( -7.716108683319066408, -2.504778602574660340, 29.97347330155780298 ) ) ;
#58406=CARTESIAN_POINT ( 'NONE',  ( -16.15384615384615330, -13.57706302396349152, 30.56769352161908060 ) ) ;
#58408=CARTESIAN_POINT ( 'NONE',  ( 7.780070435197966816, -4.786620604624111763, 33.94971097300155805 ) ) ;
#58411=CARTESIAN_POINT ( 'NONE',  ( -11.47331675774190352, -7.750023224968867197, 34.99404313364389907 ) ) ;
#58412=CARTESIAN_POINT ( 'NONE',  ( -14.53117723225663660, -11.60425143139329940, 33.02411095842164457 ) ) ;
#58413=VECTOR ( 'NONE', #75854, 1000.000000000000114 ) ;
#58414=CARTESIAN_POINT ( 'NONE',  ( 9.019230769230768274, -7.500000000000001776, 35.04278698407183867 ) ) ;
#58415=CARTESIAN_POINT ( 'NONE',  ( 4.826946332874483048, -9.234221910056348293, 34.70572697212741531 ) ) ;
#58416=CARTESIAN_POINT ( 'NONE',  ( 14.30769230769218758, -6.026961402154118019, 34.52809138561165270 ) ) ;
#58417=CARTESIAN_POINT ( 'NONE',  ( 4.087762742890272527, -10.51840700105979387, 33.73612834413961536 ) ) ;
#58418=B_SPLINE_CURVE_WITH_KNOTS ( 'NONE', 3,
 ( #68395, #27414, #54433, #13014, #40501, #34166, #54886, #67963, #75588, #87361 ),
 .UNSPECIFIED., .F., .F.,
 ( 4, 2, 2, 2, 4 ),
 ( 0.0007817246256747440282, 0.0009771112852218863821, 0.001172497944769028844, 0.001367884604316171307, 0.001563271263863313769 ),
 .UNSPECIFIED. ) ;
#58419=CARTESIAN_POINT ( 'NONE',  ( -18.00000000000012079, -2.892918686052166066, 31.69288490824153470 ) ) ;
#58421=DIRECTION ( 'NONE',  ( -0.000000000000000000, 0.1736481776669307198, -0.9848077530122080203 ) ) ;
#58422=ORIENTED_EDGE ( 'NONE', *, *, #87170, .T. ) ;
#58423=CARTESIAN_POINT ( 'NONE',  ( 15.16468685140909578, -11.35647404775217595, 33.31231777344666511 ) ) ;
#58424=CARTESIAN_POINT ( 'NONE',  ( 6.989145274079363368, -4.786620604624113540, 33.94971097300155805 ) ) ;
#58426=CARTESIAN_POINT ( 'NONE',  ( -10.74607521849492109, -2.494641256782728966, 31.33461815524612959 ) ) ;
#58427=CARTESIAN_POINT ( 'NONE',  ( -17.07692307692319744, -5.941354392335915335, 34.76329471203413846 ) ) ;
#58429=CARTESIAN_POINT ( 'NONE',  ( 1.607626736228236153, -4.187068189119697692, 33.49521262558774026 ) ) ;
#58430=CARTESIAN_POINT ( 'NONE',  ( 1.253923917947828537, -8.999036380462717588, 34.52022231692819076 ) ) ;
#58431=LINE ( 'NONE', #29656, #67053 ) ;
#58432=EDGE_LOOP ( 'NONE', ( #41991, #61607 ) ) ;
#58433=CARTESIAN_POINT ( 'NONE',  ( 11.76147438255493327, -4.762714258010881885, 34.23016756924214832 ) ) ;
#58434=CARTESIAN_POINT ( 'NONE',  ( -13.16183584334697443, -10.11255958852956027, 34.01340905677048454 ) ) ;
#58436=CARTESIAN_POINT ( 'NONE',  ( -14.08468095607945969, -11.24521262558773493, 33.06293181088029343 ) ) ;
#58437=EDGE_LOOP ( 'NONE', ( #24526, #54567 ) ) ;
#58438=DIRECTION ( 'NONE',  ( -0.000000000000000000, 0.3420201433256694901, -0.9396926207859082059 ) ) ;
#58439=CARTESIAN_POINT ( 'NONE',  ( 10.74617505635156789, -3.957578996910242619, 33.62503395064540257 ) ) ;
#58440=ADVANCED_FACE ( 'NONE', ( #55485 ), #74888, .F. ) ;
#58441=CARTESIAN_POINT ( 'NONE',  ( -1.161604033002533898, -5.667800583137508674, 34.40243808032445827 ) ) ;
#58442=VERTEX_POINT ( 'NONE', #19928 ) ;
#58443=EDGE_CURVE ( 'NONE', #23084, #14741, #49164, .T. ) ;
#58445=EDGE_CURVE ( 'NONE', #35007, #8069, #7310, .T. ) ;
#58446=VERTEX_POINT ( 'NONE', #28465 ) ;
#58447=B_SPLINE_CURVE_WITH_KNOTS ( 'NONE', 3,
 ( #63671, #42530, #56911, #15500, #76302, #21359, #49279, #34869, #48828, #1093 ),
 .UNSPECIFIED., .F., .F.,
 ( 4, 2, 2, 2, 4 ),
 ( 0.000000000000000000, 0.0001954339857564090194, 0.0003908679715128180387, 0.0005863019572692270039, 0.0007817359430256360774 ),
 .UNSPECIFIED. ) ;
#58448=ADVANCED_FACE ( 'NONE', ( #69450 ), #54147, .F. ) ;
#58449=CARTESIAN_POINT ( 'NONE',  ( -5.300408001487407539, -9.417330523894424488, 34.63758898049880486 ) ) ;
#58450=DIRECTION ( 'NONE',  ( 0.000000000000000000, 0.000000000000000000, 1.000000000000000000 ) ) ;
#58452=CARTESIAN_POINT ( 'NONE',  ( 4.153846153846154188, -12.78798330534102945, 29.74999999999997868 ) ) ;
#58453=CARTESIAN_POINT ( 'NONE',  ( 14.98074599347626901, -3.711651800289232028, 33.01384336483936011 ) ) ;
#58454=ORIENTED_EDGE ( 'NONE', *, *, #18541, .F. ) ;
#58455=ORIENTED_EDGE ( 'NONE', *, *, #10849, .T. ) ;
#58456=LINE ( 'NONE', #24231, #47295 ) ;
#58457=VERTEX_POINT ( 'NONE', #88859 ) ;
#58458=CARTESIAN_POINT ( 'NONE',  ( -18.00000000000012079, -2.657715359629662988, 31.77849191805970364 ) ) ;
#58460=CARTESIAN_POINT ( 'NONE',  ( 10.39245839786846837, -11.24512374952581872, 33.06303171183252942 ) ) ;
#58461=CARTESIAN_POINT ( 'NONE',  ( 13.63456079399343146, -10.18230066228895758, 34.26354781536631577 ) ) ;
#58462=EDGE_LOOP ( 'NONE', ( #28920, #17612 ) ) ;
#58463=ORIENTED_EDGE ( 'NONE', *, *, #83633, .F. ) ;
#58465=ORIENTED_EDGE ( 'NONE', *, *, #23379, .F. ) ;
#58466=CARTESIAN_POINT ( 'NONE',  ( 15.16468581981334651, -2.538708090699994813, 30.37095296980875148 ) ) ;
#58468=LINE ( 'NONE', #17056, #26022 ) ;
#58469=EDGE_CURVE ( 'NONE', #27365, #74160, #39267, .T. ) ;
#58470=CARTESIAN_POINT ( 'NONE',  ( 17.99999999999987566, -5.941354392335915335, 34.76329471203413846 ) ) ;
#58471=VERTEX_POINT ( 'NONE', #68128 ) ;
#58472=VECTOR ( 'NONE', #38959, 1000.000000000000114 ) ;
#58474=CARTESIAN_POINT ( 'NONE',  ( -1.514762594053604916, -8.587444163452046197, 34.63053765926554206 ) ) ;
#58475=CARTESIAN_POINT ( 'NONE',  ( -2.242436736416281828, -11.48612834413965977, 32.76840700105972815 ) ) ;
#58476=FACE_BOUND ( 'NONE', #18774, .T. ) ;
#58477=CARTESIAN_POINT ( 'NONE',  ( -8.769230769230768274, -2.292212530054420494, 30.41441678777542634 ) ) ;
#58478=CARTESIAN_POINT ( 'NONE',  ( 11.53846153846153832, -8.120952969808772792, 34.71129190930000163 ) ) ;
#58479=CARTESIAN_POINT ( 'NONE',  ( 8.546304551714618114, -2.554751324335735152, 30.48935550225260727 ) ) ;
#58481=CARTESIAN_POINT ( 'NONE',  ( 4.153846153846030731, -2.379036618888197729, 30.90682066428292885 ) ) ;
#58482=CARTESIAN_POINT ( 'NONE',  ( 11.47237812750566022, -11.16473453929635440, 33.15142922261925662 ) ) ;
#58484=ORIENTED_EDGE ( 'NONE', *, *, #67436, .T. ) ;
#58485=CYLINDRICAL_SURFACE ( 'NONE', #46079, 0.2500000000000002220 ) ;
#58486=CARTESIAN_POINT ( 'NONE',  ( -13.38461538461550759, -9.528491918059723176, 34.59228464037033035 ) ) ;
#58487=ORIENTED_EDGE ( 'NONE', *, *, #12885, .F. ) ;
#58489=EDGE_CURVE ( 'NONE', #72151, #79461, #29880, .T. ) ;
#58490=CARTESIAN_POINT ( 'NONE',  ( -39.05038313613820122, -2.249999999999998668, 29.75000000000000355 ) ) ;
#58491=CARTESIAN_POINT ( 'NONE',  ( -5.999999999999998224, -12.10708131394839349, 31.69288490824020244 ) ) ;
#58492=CARTESIAN_POINT ( 'NONE',  ( -6.792285115252135519, -6.413143153341454017, 34.63066358083362672 ) ) ;
#58493=CARTESIAN_POINT ( 'NONE',  ( 14.53106779346472877, -2.251407671071270489, 29.88021292934943318 ) ) ;
#58494=CARTESIAN_POINT ( 'NONE',  ( 18.00000000000000000, -13.78497067705608181, 32.30358669280327177 ) ) ;
#58495=ORIENTED_EDGE ( 'NONE', *, *, #85298, .F. ) ;
#58497=CARTESIAN_POINT ( 'NONE',  ( 18.25005441991345734, -4.074993327901525575, 33.72946981652012255 ) ) ;
#58498=CARTESIAN_POINT ( 'NONE',  ( -7.846153846153844924, -3.669653830205710676, 35.88435417666054406 ) ) ;
#58499=CARTESIAN_POINT ( 'NONE',  ( -15.23076923076922995, -12.78798330534103123, 29.99999999999997868 ) ) ;
#58500=DIRECTION ( 'NONE',  ( -0.000000000000000000, 0.3420201433256694901, -0.9396926207859082059 ) ) ;
#58504=VERTEX_POINT ( 'NONE', #50054 ) ;
#58505=B_SPLINE_CURVE_WITH_KNOTS ( 'NONE', 3,
 ( #7600, #15687, #27865, #402, #43154, #16123, #8931, #63861, #2158, #8489 ),
 .UNSPECIFIED., .F., .F.,
 ( 4, 2, 2, 2, 4 ),
 ( 0.0007817359430256388964, 0.0009771253907250073822, 0.001172514838424375868, 0.001367904286123744571, 0.001563293733823113056 ),
 .UNSPECIFIED. ) ;
#58507=EDGE_CURVE ( 'NONE', #26351, #23513, #60973, .T. ) ;
#58508=FACE_OUTER_BOUND ( 'NONE', #805, .T. ) ;
#58509=EDGE_LOOP ( 'NONE', ( #55029, #60513 ) ) ;
#58510=VECTOR ( 'NONE', #26010, 1000.000000000000000 ) ;
#58511=CARTESIAN_POINT ( 'NONE',  ( 17.29993592101647693, -4.026326845037969449, 33.68677907613345468 ) ) ;
#58512=CARTESIAN_POINT ( 'NONE',  ( 9.758376043310132530, -9.780366693483667717, 34.19971097300155805 ) ) ;
#58513=CARTESIAN_POINT ( 'NONE',  ( 14.37294787896833270, -2.892918686051625166, 31.69288490824026638 ) ) ;
#58514=EDGE_CURVE ( 'NONE', #37333, #5428, #33064, .T. ) ;
#58515=FACE_OUTER_BOUND ( 'NONE', #74484, .T. ) ;
#58517=CARTESIAN_POINT ( 'NONE',  ( 1.384615384615386802, -4.786620604624113540, 33.94971097300155094 ) ) ;
#58518=EDGE_LOOP ( 'NONE', ( #14456, #69175 ) ) ;
#58519=CARTESIAN_POINT ( 'NONE',  ( 4.218991933178116938, -7.750023238201980469, 34.74374492549440419 ) ) ;
#58520=DIRECTION ( 'NONE',  ( 0.000000000000000000, 0.1736481776669267785, -0.9848077530122087975 ) ) ;
#58521=VERTEX_POINT ( 'NONE', #83866 ) ;
#58523=CARTESIAN_POINT ( 'NONE',  ( 14.08476609017615644, -12.15238873228292071, 31.58232369045353849 ) ) ;
#58525=CARTESIAN_POINT ( 'NONE',  ( 7.846153846153846700, -13.75783147151868846, 33.36296068462461051 ) ) ;
#58526=CARTESIAN_POINT ( 'NONE',  ( -6.000000000000121680, -5.094484230521993062, 34.41647553114689373 ) ) ;
#58527=EDGE_CURVE ( 'NONE', #15410, #31669, #15835, .T. ) ;
#58528=CARTESIAN_POINT ( 'NONE',  ( 7.846153846153846700, -3.322132147404559976, 32.92929555188717927 ) ) ;
#58529=CARTESIAN_POINT ( 'NONE',  ( -7.146003140593070846, -4.887634598454295265, 34.01352882383564946 ) ) ;
#58531=ORIENTED_EDGE ( 'NONE', *, *, #79555, .T. ) ;
#58532=CARTESIAN_POINT ( 'NONE',  ( -4.403869391139117795, -5.056417327199099532, 34.11270091957320716 ) ) ;
#58533=CARTESIAN_POINT ( 'NONE',  ( -12.33149085528277844, -7.723484964179501588, 34.74522123443823318 ) ) ;
#58534=CARTESIAN_POINT ( 'NONE',  ( -4.377331078410482412, -5.827078755546623690, 34.72654668319379567 ) ) ;
#58536=ADVANCED_FACE ( 'NONE', ( #56811 ), #8198, .F. ) ;
#58537=LINE ( 'NONE', #30631, #17299 ) ;
#58539=CARTESIAN_POINT ( 'NONE',  ( -17.29984929443922681, -2.554751324335733376, 30.48935550225260727 ) ) ;
#58540=DIRECTION ( 'NONE',  ( -0.000000000000000000, -0.7660444431189791237, -0.6427876096865379196 ) ) ;
#58541=ORIENTED_EDGE ( 'NONE', *, *, #39000, .F. ) ;
#58544=EDGE_CURVE ( 'NONE', #10963, #60703, #12642, .T. ) ;
#58545=EDGE_LOOP ( 'NONE', ( #82074, #48508, #54088, #88638 ) ) ;
#58546=CARTESIAN_POINT ( 'NONE',  ( 6.673100179028331524, -6.524016743844655686, 34.90889640711025521 ) ) ;
#58547=ORIENTED_EDGE ( 'NONE', *, *, #49395, .F. ) ;
#58548=B_SPLINE_CURVE_WITH_KNOTS ( 'NONE', 3,
 ( #46157, #5611, #18691, #52452, #74077, #39850, #11934, #38510, #32633, #73184 ),
 .UNSPECIFIED., .F., .F.,
 ( 4, 2, 2, 2, 4 ),
 ( 0.0007817359430256297891, 0.0009771253907249963233, 0.001172514838424362858, 0.001367904286123729175, 0.001563293733823095709 ),
 .UNSPECIFIED. ) ;
#58550=CARTESIAN_POINT ( 'NONE',  ( -14.30769230769242917, -3.083524468854526912, 32.58852847137268327 ) ) ;
#58551=CARTESIAN_POINT ( 'NONE',  ( -1.634638608836842089, -12.07920672191015221, 32.31858351112116168 ) ) ;
#58552=EDGE_CURVE ( 'NONE', #2097, #77497, #29801, .T. ) ;
#58553=CARTESIAN_POINT ( 'NONE',  ( -0.2385256174450664790, -6.460100341425560444, 34.89618726649961644 ) ) ;
#58554=ORIENTED_EDGE ( 'NONE', *, *, #207, .F. ) ;
#58555=CARTESIAN_POINT ( 'NONE',  ( -0.7115384615384854339, -2.249999999999999112, 29.81609741502488120 ) ) ;
#58556=VERTEX_POINT ( 'NONE', #56380 ) ;
#58557=CARTESIAN_POINT ( 'NONE',  ( -11.53846153846153655, -13.53365097954675988, 30.81389545987213552 ) ) ;
#58558=ORIENTED_EDGE ( 'NONE', *, *, #75820, .F. ) ;
#58559=CARTESIAN_POINT ( 'NONE',  ( -0.5922299282060219383, -3.062553014421049546, 32.05460306192773601 ) ) ;
#58560=DIRECTION ( 'NONE',  ( 0.000000000000000000, 0.3420201433256610524, 0.9396926207859113145 ) ) ;
#58561=ADVANCED_FACE ( 'NONE', ( #43311 ), #9088, .F. ) ;
#58562=VERTEX_POINT ( 'NONE', #36977 ) ;
#58563=ADVANCED_FACE ( 'NONE', ( #2740 ), #30236, .F. ) ;
#58565=DIRECTION ( 'NONE',  ( -0.000000000000000000, -0.5000000000000009992, -0.8660254037844380415 ) ) ;
#58566=CARTESIAN_POINT ( 'NONE',  ( -11.78848477575450460, -2.823816976329319051, 31.52131813110795733 ) ) ;
#58567=CARTESIAN_POINT ( 'NONE',  ( 13.38461538461538680, -11.91647553114624181, 32.58852847137148245 ) ) ;
#58568=CARTESIAN_POINT ( 'NONE',  ( -8.096177070375304652, -12.68155406624981119, 30.59749803192733708 ) ) ;
#58569=VECTOR ( 'NONE', #46877, 1000.000000000000000 ) ;
#58570=VERTEX_POINT ( 'NONE', #12189 ) ;
#58571=ORIENTED_EDGE ( 'NONE', *, *, #5205, .T. ) ;
#58572=ORIENTED_EDGE ( 'NONE', *, *, #25118, .T. ) ;
#58573=CARTESIAN_POINT ( 'NONE',  ( 2.980746006547774218, -5.765609946408404518, 34.70566812827425451 ) ) ;
#58574=EDGE_LOOP ( 'NONE', ( #74756, #59509 ) ) ;
#58575=AXIS2_PLACEMENT_3D ( 'NONE', #9633, #11415, #31695 ) ;
#58576=ADVANCED_FACE ( 'NONE', ( #39674 ), #32012, .F. ) ;
#58577=CARTESIAN_POINT ( 'NONE',  ( -11.53846153846166089, -2.379036618888197729, 30.90682066428292885 ) ) ;
#58578=CARTESIAN_POINT ( 'NONE',  ( 9.442330948259103351, -5.643011162660950042, 34.66104346484419096 ) ) ;
#58579=ORIENTED_EDGE ( 'NONE', *, *, #15343, .T. ) ;
#58580=ORIENTED_EDGE ( 'NONE', *, *, #45472, .T. ) ;
#58581=B_SPLINE_CURVE_WITH_KNOTS ( 'NONE', 3,
 ( #40732, #13251, #27645, #88059, #26320, #178, #53787, #75395, #7386, #67753 ),
 .UNSPECIFIED., .F., .F.,
 ( 4, 2, 2, 2, 4 ),
 ( 0.000000000000000000, 0.0001954311564186868744, 0.0003908623128373737488, 0.0005862934692560606504, 0.0007817246256747474977 ),
 .UNSPECIFIED. ) ;
#58582=ORIENTED_EDGE ( 'NONE', *, *, #70331, .T. ) ;
#58583=CARTESIAN_POINT ( 'NONE',  ( 17.07692307692295586, -4.481592998941358097, 33.73612834414048933 ) ) ;
#58586=B_SPLINE_CURVE_WITH_KNOTS ( 'NONE', 3,
 ( #39275, #45564, #3245, #79808, #18108, #30716, #79358, #58182, #51861, #58627 ),
 .UNSPECIFIED., .F., .F.,
 ( 4, 2, 2, 2, 4 ),
 ( 0.0007817359430256297891, 0.0009771253907249958896, 0.001172514838424361990, 0.001367904286123728091, 0.001563293733823094191 ),
 .UNSPECIFIED. ) ;
#58587=EDGE_CURVE ( 'NONE', #35011, #4267, #65262, .T. ) ;
#58588=CARTESIAN_POINT ( 'NONE',  ( -7.846153846153844924, -2.538708090699994813, 30.37095296980875503 ) ) ;
#58589=CARTESIAN_POINT ( 'NONE',  ( -9.942307692307693401, -7.433932668274256805, 35.00000000000000711 ) ) ;
#58590=ADVANCED_FACE ( 'NONE', ( #18502 ), #52713, .F. ) ;
#58591=FACE_BOUND ( 'NONE', #34118, .T. ) ;
#58592=ORIENTED_EDGE ( 'NONE', *, *, #70727, .T. ) ;
#58594=CARTESIAN_POINT ( 'NONE',  ( 12.71159277317677549, -5.728107161865378494, 34.42597550085002922 ) ) ;
#58595=EDGE_CURVE ( 'NONE', #77057, #47782, #67134, .T. ) ;
#58596=CARTESIAN_POINT ( 'NONE',  ( 4.153846153846032507, -8.613356846316285953, 34.62446782046622218 ) ) ;
#58597=VECTOR ( 'NONE', #81783, 1000.000000000000000 ) ;
#58598=DIRECTION ( 'NONE',  ( -0.000000000000000000, -0.1736481776669307198, -0.9848077530122080203 ) ) ;
#58599=CARTESIAN_POINT ( 'NONE',  ( 8.068933387422253745, -10.81320215134717344, 33.49497208177562868 ) ) ;
#58602=ORIENTED_EDGE ( 'NONE', *, *, #65140, .F. ) ;
#58604=EDGE_CURVE ( 'NONE', #72334, #26024, #80203, .T. ) ;
#58605=FACE_OUTER_BOUND ( 'NONE', #85169, .T. ) ;
#58606=CARTESIAN_POINT ( 'NONE',  ( 5.750023269057648712, -3.137211980971221781, 32.19342716148376837 ) ) ;
#58607=LINE ( 'NONE', #31590, #38462 ) ;
#58608=CARTESIAN_POINT ( 'NONE',  ( -2.057637996053991891, -12.17597550085003455, 31.52189283813461884 ) ) ;
#58609=CARTESIAN_POINT ( 'NONE',  ( 17.14309221788574078, -7.250054483168842268, 34.74374881642865631 ) ) ;
#58610=CARTESIAN_POINT ( 'NONE',  ( -15.45425415533356173, -3.562934362175800285, 33.22335522853832401 ) ) ;
#58611=ORIENTED_EDGE ( 'NONE', *, *, #40958, .T. ) ;
#58612=CARTESIAN_POINT ( 'NONE',  ( -5.299850035829924089, -6.459968553980839800, 34.89616026154728701 ) ) ;
#58613=VECTOR ( 'NONE', #47145, 1000.000000000000000 ) ;
#58614=CARTESIAN_POINT ( 'NONE',  ( 3.230769230769231726, -10.51840700105979565, 33.73612834413961536 ) ) ;
#58616=CARTESIAN_POINT ( 'NONE',  ( -13.38461538461538325, -12.62096338111211580, 30.90682066428153263 ) ) ;
#58617=EDGE_LOOP ( 'NONE', ( #18947, #47483, #26816, #80641 ) ) ;
#58618=ORIENTED_EDGE ( 'NONE', *, *, #28675, .F. ) ;
#58619=FACE_BOUND ( 'NONE', #9720, .T. ) ;
#58620=B_SPLINE_CURVE_WITH_KNOTS ( 'NONE', 3,
 ( #11949, #73199, #38978, #86736, #61006, #88506, #88075, #39426, #25897, #6073 ),
 .UNSPECIFIED., .F., .F.,
 ( 4, 2, 2, 2, 4 ),
 ( 0.0007817359430256369448, 0.0009771253907250049969, 0.001172514838424373049, 0.001367904286123741101, 0.001563293733823109153 ),
 .UNSPECIFIED. ) ;
#58621=ORIENTED_EDGE ( 'NONE', *, *, #49266, .T. ) ;
#58622=CARTESIAN_POINT ( 'NONE',  ( 11.66898697669518192, -12.50538340440932394, 31.33453814440721885 ) ) ;
#58624=ORIENTED_EDGE ( 'NONE', *, *, #5177, .T. ) ;
#58625=CARTESIAN_POINT ( 'NONE',  ( -7.846153846153844924, -2.499999999999998668, 29.75000000000001421 ) ) ;
#58626=FACE_OUTER_BOUND ( 'NONE', #21496, .T. ) ;
#58627=CARTESIAN_POINT ( 'NONE',  ( -8.769230769230768274, -6.386643153685126251, 34.62446782046654192 ) ) ;
#58628=EDGE_CURVE ( 'NONE', #33723, #56881, #39222, .T. ) ;
#58629=CARTESIAN_POINT ( 'NONE',  ( -6.857821351800897247, -3.300289026998475705, 32.46337939537591666 ) ) ;
#58630=VERTEX_POINT ( 'NONE', #4076 ) ;
#58631=ADVANCED_FACE ( 'NONE', ( #59920 ), #85623, .F. ) ;
#58632=DIRECTION ( 'NONE',  ( -0.000000000000000000, -0.9396926207859092051, -0.3420201433256662704 ) ) ;
#58633=ORIENTED_EDGE ( 'NONE', *, *, #16623, .F. ) ;
#58634=CARTESIAN_POINT ( 'NONE',  ( 17.07692307692295586, -10.90142922262034020, 33.41473453929536674 ) ) ;
#58635=EDGE_LOOP ( 'NONE', ( #27483, #88408 ) ) ;
#58636=CARTESIAN_POINT ( 'NONE',  ( 15.45354877203763522, -8.496831190052093419, 34.64984203495476578 ) ) ;
#58638=CARTESIAN_POINT ( 'NONE',  ( -7.596099426240392916, -3.435999193479609470, 33.07426656108010832 ) ) ;
#58639=VECTOR ( 'NONE', #82478, 1000.000000000000227 ) ;
#58640=CARTESIAN_POINT ( 'NONE',  ( 0.4615384615383396616, -12.27809138561165270, 31.22303859784587132 ) ) ;
#58642=CARTESIAN_POINT ( 'NONE',  ( -9.692307692307691624, -11.91647553114624181, 32.58852847137148245 ) ) ;
#58644=ORIENTED_EDGE ( 'NONE', *, *, #64173, .F. ) ;
#58645=AXIS2_PLACEMENT_3D ( 'NONE', #6002, #19065, #12307 ) ;
#58647=DIRECTION ( 'NONE',  ( -0.000000000000000000, -0.7660444431189791237, -0.6427876096865379196 ) ) ;
#58649=ORIENTED_EDGE ( 'NONE', *, *, #5857, .F. ) ;
#58650=VECTOR ( 'NONE', #43943, 1000.000000000000000 ) ;
#58651=VERTEX_POINT ( 'NONE', #58577 ) ;
#58652=DIRECTION ( 'NONE',  ( -0.000000000000000000, 1.000000000000000000, 3.491481338843133355E-15 ) ) ;
#58653=CARTESIAN_POINT ( 'NONE',  ( 2.307692307692309264, -3.322132147404559976, 32.92929555188717927 ) ) ;
#58654=CARTESIAN_POINT ( 'NONE',  ( 17.20744851515672025, -3.625058011473227815, 33.29252011169590020 ) ) ;
#58655=DIRECTION ( 'NONE',  ( -0.000000000000000000, -0.9396926207859093161, -0.3420201433256663259 ) ) ;
#58656=CARTESIAN_POINT ( 'NONE',  ( 15.48076923077065103, -7.500000000000154543, 35.00000000000007105 ) ) ;
#58657=CARTESIAN_POINT ( 'NONE',  ( -17.07692307692307665, -11.35647404775217417, 33.31231777344666511 ) ) ;
#58659=ORIENTED_EDGE ( 'NONE', *, *, #73409, .T. ) ;
#58660=DIRECTION ( 'NONE',  ( 0.000000000000000000, 0.7660444431189822323, -0.6427876096865344779 ) ) ;
#58661=CARTESIAN_POINT ( 'NONE',  ( -0.2114841499001464675, -8.303483539816728154, 34.68545999027710991 ) ) ;
#58662=EDGE_CURVE ( 'NONE', #89067, #28242, #84598, .T. ) ;
#58663=EDGE_CURVE ( 'NONE', #3164, #17506, #56664, .T. ) ;
#58664=CARTESIAN_POINT ( 'NONE',  ( 4.283893589096606114, -7.723484941389743952, 34.99544897038808955 ) ) ;
#58665=B_SPLINE_CURVE_WITH_KNOTS ( 'NONE', 3,
 ( #24443, #23565, #42194, #71302, #69645, #14713, #44260, #28673, #64536, #10948 ),
 .UNSPECIFIED., .F., .F.,
 ( 4, 2, 2, 2, 4 ),
 ( 0.000000000000000000, 0.0001954311564186876876, 0.0003908623128373753751, 0.0005862934692560630356, 0.0007817246256747507503 ),
 .UNSPECIFIED. ) ;
#58666=CARTESIAN_POINT ( 'NONE',  ( 9.627037691751374027, -2.657715359629088780, 31.77849191805832874 ) ) ;
#58667=ORIENTED_EDGE ( 'NONE', *, *, #47485, .T. ) ;
#58668=CARTESIAN_POINT ( 'NONE',  ( 10.36536139116315880, -9.356822207818506598, 34.66110646841856635 ) ) ;
#58669=EDGE_CURVE ( 'NONE', #51593, #84770, #51352, .T. ) ;
#58670=ORIENTED_EDGE ( 'NONE', *, *, #15382, .F. ) ;
#58671=CARTESIAN_POINT ( 'NONE',  ( -17.32689982097166492, -2.544273027872574922, 31.48422191005632342 ) ) ;
#58672=CARTESIAN_POINT ( 'NONE',  ( 10.48469401227430708, -3.338472653186243644, 32.95098750199972670 ) ) ;
#58673=CARTESIAN_POINT ( 'NONE',  ( 15.36155967173618286, -4.684288915650983043, 34.18129842949671371 ) ) ;
#58674=VERTEX_POINT ( 'NONE', #79313 ) ;
#58675=EDGE_CURVE ( 'NONE', #75329, #75936, #45067, .T. ) ;
#58679=EDGE_CURVE ( 'NONE', #58941, #32595, #23313, .T. ) ;
#58680=CARTESIAN_POINT ( 'NONE',  ( 5.999999999999880096, -11.94971097300221174, 32.03036669348237098 ) ) ;
#58681=CARTESIAN_POINT ( 'NONE',  ( -5.076923076923075762, -8.164416787775445883, 34.95778746994557906 ) ) ;
#58682=ORIENTED_EDGE ( 'NONE', *, *, #60678, .T. ) ;
#58683=CARTESIAN_POINT ( 'NONE',  ( -1.318547033612945230, -3.513871655860379306, 32.76840700105978499 ) ) ;
#58684=ORIENTED_EDGE ( 'NONE', *, *, #85663, .F. ) ;
#58685=CARTESIAN_POINT ( 'NONE',  ( 8.545745825506822158, -12.44517049084099725, 30.48991314939691932 ) ) ;
#58686=EDGE_CURVE ( 'NONE', #19715, #14549, #36249, .T. ) ;
#58687=FACE_OUTER_BOUND ( 'NONE', #71567, .T. ) ;
#58688=CARTESIAN_POINT ( 'NONE',  ( -0.2385256174450663680, -2.523321265292116422, 31.42251411153756990 ) ) ;
#58689=CARTESIAN_POINT ( 'NONE',  ( 0.4615384615384611755, -1.509761064869970415, 31.06009739812519044 ) ) ;
#58690=EDGE_CURVE ( 'NONE', #53001, #48794, #34177, .T. ) ;
#58691=CARTESIAN_POINT ( 'NONE',  ( -6.222926217516144831, -4.186968288167446595, 33.49512374952580274 ) ) ;
#58693=EDGE_LOOP ( 'NONE', ( #53584, #49181, #25908, #18805 ) ) ;
#58694=ORIENTED_EDGE ( 'NONE', *, *, #46456, .F. ) ;
#58695=ORIENTED_EDGE ( 'NONE', *, *, #7622, .T. ) ;
#58696=ORIENTED_EDGE ( 'NONE', *, *, #38683, .T. ) ;
#58697=ORIENTED_EDGE ( 'NONE', *, *, #4062, .F. ) ;
#58698=EDGE_CURVE ( 'NONE', #13749, #31351, #43733, .T. ) ;
#58699=CARTESIAN_POINT ( 'NONE',  ( 13.38461538461538680, -1.951392089020283160, 34.73218667398347748 ) ) ;
#58700=CARTESIAN_POINT ( 'NONE',  ( -1.384615384615383471, -12.37446782046654192, 30.86335684631486131 ) ) ;
#58701=VECTOR ( 'NONE', #46213, 1000.000000000000000 ) ;
#58702=CARTESIAN_POINT ( 'NONE',  ( 14.98079249982687777, -4.943428324936578910, 34.04746400365624481 ) ) ;
#58703=EDGE_CURVE ( 'NONE', #49742, #6248, #47290, .T. ) ;
#58704=CARTESIAN_POINT ( 'NONE',  ( -8.769230769230768274, -1.466349020453238561, 30.81389545987213907 ) ) ;
#58705=CARTESIAN_POINT ( 'NONE',  ( -13.44988538517170440, -3.643525952247789412, 33.31231777344662959 ) ) ;
#58706=DIRECTION ( 'NONE',  ( -0.000000000000000000, -0.5000000000000009992, -0.8660254037844380415 ) ) ;
#58707=CARTESIAN_POINT ( 'NONE',  ( 5.869852790561781219, -11.93770438780619259, 32.05411857736982029 ) ) ;
#58708=CARTESIAN_POINT ( 'NONE',  ( -5.326923076923075762, -2.249999999999998668, 29.75000000000000355 ) ) ;
#58710=ORIENTED_EDGE ( 'NONE', *, *, #15801, .F. ) ;
#58711=ORIENTED_EDGE ( 'NONE', *, *, #73930, .F. ) ;
#58712=VERTEX_POINT ( 'NONE', #82430 ) ;
#58714=EDGE_CURVE ( 'NONE', #14193, #2419, #46851, .T. ) ;
#58715=ORIENTED_EDGE ( 'NONE', *, *, #61591, .T. ) ;
#58716=CARTESIAN_POINT ( 'NONE',  ( 7.846153846153846700, -3.050289026998446396, 32.03036669348365706 ) ) ;
#58717=CARTESIAN_POINT ( 'NONE',  ( -17.07692307692307665, -4.098570777380720287, 33.41473453929634729 ) ) ;
#58718=CYLINDRICAL_SURFACE ( 'NONE', #40362, 0.2499999999999986955 ) ;
#58719=CARTESIAN_POINT ( 'NONE',  ( -11.53846153846153655, -9.058645607665452459, 34.76329471203371924 ) ) ;
#58720=ORIENTED_EDGE ( 'NONE', *, *, #16793, .F. ) ;
#58721=B_SPLINE_CURVE_WITH_KNOTS ( 'NONE', 3,
 ( #70113, #57035, #35897, #64226, #83651, #41769 ),
 .UNSPECIFIED., .F., .F.,
 ( 4, 2, 4 ),
 ( 0.000000000000000000, 0.0001954784845028924105, 0.0003909569690057848211 ),
 .UNSPECIFIED. ) ;
#58722=EDGE_CURVE ( 'NONE', #18827, #78695, #6325, .T. ) ;
#58723=B_SPLINE_CURVE_WITH_KNOTS ( 'NONE', 3,
 ( #81171, #60437, #46915, #81608, #33421, #73522 ),
 .UNSPECIFIED., .F., .F.,
 ( 4, 2, 4 ),
 ( 0.000000000000000000, 0.0001954784845028924105, 0.0003909569690057848211 ),
 .UNSPECIFIED. ) ;
#58724=ORIENTED_EDGE ( 'NONE', *, *, #54803, .T. ) ;
#58725=DIRECTION ( 'NONE',  ( 0.000000000000000000, 0.9396926207859126468, -0.3420201433256571111 ) ) ;
#58727=FACE_BOUND ( 'NONE', #21195, .T. ) ;
#58728=CARTESIAN_POINT ( 'NONE',  ( -6.066083410955878108, -8.973038597847269315, 34.52809138561120506 ) ) ;
#58730=DIRECTION ( 'NONE',  ( 0.000000000000000000, 0.8660254037844377084, -0.5000000000000015543 ) ) ;
#58731=EDGE_LOOP ( 'NONE', ( #87226, #68491, #52159, #71331 ) ) ;
#58732=CARTESIAN_POINT ( 'NONE',  ( 14.08420736396836404, -2.847400154188068022, 31.58180166144859058 ) ) ;
#58734=CYLINDRICAL_SURFACE ( 'NONE', #29236, 0.2500000000000002220 ) ;
#58736=CARTESIAN_POINT ( 'NONE',  ( 12.21156173059610772, -4.943428324936578910, 34.04746400365624481 ) ) ;
#58737=CARTESIAN_POINT ( 'NONE',  ( -18.00000000000000000, -4.786620604624112651, 33.94971097300155094 ) ) ;
#58738=ADVANCED_FACE ( 'NONE', ( #62141 ), #55382, .F. ) ;
#58739=ORIENTED_EDGE ( 'NONE', *, *, #8682, .F. ) ;
#58740=AXIS2_PLACEMENT_3D ( 'NONE', #64017, #21265, #15857 ) ;
#58741=EDGE_CURVE ( 'NONE', #3368, #3730, #4742, .T. ) ;
#58743=CARTESIAN_POINT ( 'NONE',  ( -9.692307692307814193, -9.528491918059723176, 34.59228464037033035 ) ) ;
#58744=AXIS2_PLACEMENT_3D ( 'NONE', #47996, #19211, #266 ) ;
#58745=ORIENTED_EDGE ( 'NONE', *, *, #46579, .F. ) ;
#58746=CARTESIAN_POINT ( 'NONE',  ( 6.923076923076924238, -2.486705287966279876, 31.30864560766543647 ) ) ;
#58748=CARTESIAN_POINT ( 'NONE',  ( 16.15384615384615330, -2.833524468853757305, 32.15551576947925838 ) ) ;
#58749=CARTESIAN_POINT ( 'NONE',  ( 16.02369818411445834, -11.04286588640298916, 33.62463336215343901 ) ) ;
#58750=DIRECTION ( 'NONE',  ( -0.000000000000000000, 0.1736481776669307198, -0.9848077530122080203 ) ) ;
#58751=ADVANCED_FACE ( 'NONE', ( #21149 ), #48619, .F. ) ;
#58752=CARTESIAN_POINT ( 'NONE',  ( 6.792929713638702793, -9.418419913701741919, 34.36755862841477693 ) ) ;
#58756=CARTESIAN_POINT ( 'NONE',  ( 1.634669696253700621, -11.28795663066794219, 33.01431243580653785 ) ) ;
#58757=CARTESIAN_POINT ( 'NONE',  ( -15.36091644020745051, -11.93770438780619259, 32.05411857736982029 ) ) ;
#58758=CARTESIAN_POINT ( 'NONE',  ( 5.076923076923075762, -9.819645486525091727, 36.12317359536749706 ) ) ;
#58760=VERTEX_POINT ( 'NONE', #12633 ) ;
#58763=ORIENTED_EDGE ( 'NONE', *, *, #60300, .T. ) ;
#58764=DIRECTION ( 'NONE',  ( 0.000000000000000000, -6.938893903907222067E-15, 1.000000000000000000 ) ) ;
#58765=EDGE_LOOP ( 'NONE', ( #2798, #45303, #43436, #74807, #4530, #4744 ) ) ;
#58766=LINE ( 'NONE', #51538, #31116 ) ;
#58768=CARTESIAN_POINT ( 'NONE',  ( 3.100621261037536325, -2.373036134822904319, 30.88089517874952250 ) ) ;
#58769=CARTESIAN_POINT ( 'NONE',  ( -5.933932666649922361, -11.35647404775217595, 33.31231777344667222 ) ) ;
#58770=CARTESIAN_POINT ( 'NONE',  ( -5.933931648997561759, -8.973038597847269315, 34.52809138561122637 ) ) ;
#58771=CARTESIAN_POINT ( 'NONE',  ( -4.153846153846273204, -12.46129190930018460, 30.37095296980731973 ) ) ;
#58772=CARTESIAN_POINT ( 'NONE',  ( 15.23076923076923173, -8.164416787775445883, 34.95778746994557906 ) ) ;
#58773=CARTESIAN_POINT ( 'NONE',  ( -10.74553182482283198, -4.460286881179643004, 33.72017969459903242 ) ) ;
#58776=CARTESIAN_POINT ( 'NONE',  ( 18.24994540937804643, -11.56426240980093567, 33.07394671870546432 ) ) ;
#58777=CARTESIAN_POINT ( 'NONE',  ( 13.25446741488369362, -3.625366637846545892, 33.29286588640298561 ) ) ;
#58778=CARTESIAN_POINT ( 'NONE',  ( -0.4615384615385840772, -12.51329471203414379, 31.30864560766407578 ) ) ;
#58780=EDGE_LOOP ( 'NONE', ( #61351, #33092, #18032, #19908 ) ) ;
#58781=ORIENTED_EDGE ( 'NONE', *, *, #48723, .T. ) ;
#58782=DIRECTION ( 'NONE',  ( 0.000000000000000000, 0.9848077530122072432, -0.1736481776669354937 ) ) ;
#58783=CARTESIAN_POINT ( 'NONE',  ( 7.846153846153846700, -1.129524287112498415, 32.06866353760679544 ) ) ;
#58785=CARTESIAN_POINT ( 'NONE',  ( 16.40384615384757439, -7.500000000000154543, 35.00000000000007105 ) ) ;
#58790=CARTESIAN_POINT ( 'NONE',  ( 18.00000000000000000, -1.790695186598648903, 34.54067556320373455 ) ) ;
#58791=VERTEX_POINT ( 'NONE', #23355 ) ;
#58792=EDGE_CURVE ( 'NONE', #22135, #80981, #28810, .T. ) ;
#58793=ORIENTED_EDGE ( 'NONE', *, *, #47479, .F. ) ;
#58794=CARTESIAN_POINT ( 'NONE',  ( -6.000000000000119904, -6.026961402154118908, 34.52809138561165270 ) ) ;
#58795=AXIS2_PLACEMENT_3D ( 'NONE', #73052, #50976, #37032 ) ;
#58796=CARTESIAN_POINT ( 'NONE',  ( -11.31568186948346977, -11.60474049983371003, 33.02348890104160262 ) ) ;
#58797=CARTESIAN_POINT ( 'NONE',  ( 14.55769230769231015, -7.500000000000001776, 35.04278698407183867 ) ) ;
#58798=CARTESIAN_POINT ( 'NONE',  ( 0.4615384615383396616, -3.835265460704628371, 33.15142922262033665 ) ) ;
#58799=CARTESIAN_POINT ( 'NONE',  ( -13.31854703361294767, -3.050289026998446840, 32.03036669348366416 ) ) ;
#58800=AXIS2_PLACEMENT_3D ( 'NONE', #14734, #30015, #57475 ) ;
#58801=ORIENTED_EDGE ( 'NONE', *, *, #60237, .T. ) ;
#58803=EDGE_LOOP ( 'NONE', ( #55738, #46888 ) ) ;
#58805=CARTESIAN_POINT ( 'NONE',  ( 12.68491440223663957, -2.501478030877322567, 29.88021232661721172 ) ) ;
#58807=ADVANCED_FACE ( 'NONE', ( #49064 ), #1763, .F. ) ;
#58808=CARTESIAN_POINT ( 'NONE',  ( 4.153846153846154188, -3.322132147404559976, 32.92929555188717927 ) ) ;
#58810=DIRECTION ( 'NONE',  ( -0.000000000000000000, 0.5000000000000011102, -0.8660254037844380415 ) ) ;
#58811=EDGE_CURVE ( 'NONE', #57115, #59563, #73900, .T. ) ;
#58812=CARTESIAN_POINT ( 'NONE',  ( 16.15384615384603251, -9.528491918059723176, 34.59228464037033035 ) ) ;
#58813=EDGE_LOOP ( 'NONE', ( #72457, #127 ) ) ;
#58817=CARTESIAN_POINT ( 'NONE',  ( -12.52762187249433978, -11.16473453929635440, 33.15142922261925662 ) ) ;
#58818=EDGE_LOOP ( 'NONE', ( #57486, #73994, #77631, #31243 ) ) ;
#58819=CARTESIAN_POINT ( 'NONE',  ( -10.36543920600657387, -4.176053281294518804, 33.81426240980091791 ) ) ;
#58822=VERTEX_POINT ( 'NONE', #8974 ) ;
#58824=B_SPLINE_CURVE_WITH_KNOTS ( 'NONE', 3,
 ( #56632, #84119, #22836, #16524, #43990, #51169, #35474, #62927, #1238, #28722 ),
 .UNSPECIFIED., .F., .F.,
 ( 4, 2, 2, 2, 4 ),
 ( 0.000000000000000000, 0.0001954311564186868744, 0.0003908623128373737488, 0.0005862934692560606504, 0.0007817246256747474977 ),
 .UNSPECIFIED. ) ;
#58825=CARTESIAN_POINT ( 'NONE',  ( -14.43838291080261449, -12.35290016733513951, 31.75349464988449455 ) ) ;
#58826=AXIS2_PLACEMENT_3D ( 'NONE', #34260, #41917, #62174 ) ;
#58827=EDGE_LOOP ( 'NONE', ( #18810, #67630, #58455, #53427 ) ) ;
#58829=CARTESIAN_POINT ( 'NONE',  ( 10.61538461538461675, -8.973038597847269315, 34.52809138561121927 ) ) ;
#58830=FACE_OUTER_BOUND ( 'NONE', #80322, .T. ) ;
#58831=DIRECTION ( 'NONE',  ( -0.000000000000000000, 0.6427876096865404731, -0.7660444431189770143 ) ) ;
#58833=CARTESIAN_POINT ( 'NONE',  ( 5.076923076923075762, -2.538708090699994813, 30.37095296980875503 ) ) ;
#58834=CARTESIAN_POINT ( 'NONE',  ( -10.83886955910856464, -10.81261337010820256, 33.49550067578627477 ) ) ;
#58835=ORIENTED_EDGE ( 'NONE', *, *, #82177, .F. ) ;
#58836=CARTESIAN_POINT ( 'NONE',  ( 11.28848479441295005, -11.47974371597207899, 33.17467449705390692 ) ) ;
#58837=CARTESIAN_POINT ( 'NONE',  ( 6.923076923076924238, -9.058645607665452459, 34.76329471203371924 ) ) ;
#58838=EDGE_CURVE ( 'NONE', #79443, #83509, #14854, .T. ) ;
#58839=EDGE_LOOP ( 'NONE', ( #40443, #3631 ) ) ;
#58840=CARTESIAN_POINT ( 'NONE',  ( 6.673100192134570285, -5.728515186090277211, 34.42611988154120439 ) ) ;
#58841=CARTESIAN_POINT ( 'NONE',  ( 12.23867303933482553, -2.501496062324912284, 29.88072118266895671 ) ) ;
#58842=CARTESIAN_POINT ( 'NONE',  ( -15.10024379253558635, -5.915461855592780260, 34.75538340440931506 ) ) ;
#58843=CARTESIAN_POINT ( 'NONE',  ( -13.31854805126530827, -11.35647404775217595, 33.31231777344666511 ) ) ;
#58844=EDGE_CURVE ( 'NONE', #30667, #65648, #13591, .T. ) ;
#58846=ADVANCED_FACE ( 'NONE', ( #69782 ), #63005, .F. ) ;
#58847=FACE_BOUND ( 'NONE', #87869, .T. ) ;
#58848=CARTESIAN_POINT ( 'NONE',  ( 13.16113046005105325, -2.353723527008296568, 30.78948104536958752 ) ) ;
#58849=DIRECTION ( 'NONE',  ( 0.000000000000000000, 0.9396926207859126468, -0.3420201433256571111 ) ) ;
#58850=CARTESIAN_POINT ( 'NONE',  ( 16.15384615384615330, -3.050289026998446396, 32.03036669348365706 ) ) ;
#58851=CARTESIAN_POINT ( 'NONE',  ( 1.318533005255250412, -12.62096338111211580, 30.90682066428152197 ) ) ;
#58852=CARTESIAN_POINT ( 'NONE',  ( 14.24160992833217421, -10.67929555188718460, 33.92786785259543336 ) ) ;
#58853=FACE_OUTER_BOUND ( 'NONE', #39122, .T. ) ;
#58854=EDGE_CURVE ( 'NONE', #21870, #46711, #83481, .T. ) ;
#58855=DIRECTION ( 'NONE',  ( 0.000000000000000000, 0.6427876096865373645, -0.7660444431189797898 ) ) ;
#58857=EDGE_CURVE ( 'NONE', #45410, #30860, #16169, .T. ) ;
#58858=B_SPLINE_CURVE_WITH_KNOTS ( 'NONE', 3,
 ( #43886, #62814, #69590, #8788, #36259, #16861 ),
 .UNSPECIFIED., .F., .F.,
 ( 4, 2, 4 ),
 ( 0.000000000000000000, 0.0001954784845028928442, 0.0003909569690057856884 ),
 .UNSPECIFIED. ) ;
#58859=VERTEX_POINT ( 'NONE', #63460 ) ;
#58860=B_SPLINE_CURVE_WITH_KNOTS ( 'NONE', 3,
 ( #6240, #74699, #33704, #81460, #86448, #39592, #79670, #66605, #87336, #25613 ),
 .UNSPECIFIED., .F., .F.,
 ( 4, 2, 2, 2, 4 ),
 ( 0.0007817359430256306564, 0.0009771253907249969738, 0.001172514838424363291, 0.001367904286123729826, 0.001563293733823096143 ),
 .UNSPECIFIED. ) ;
#58863=DIRECTION ( 'NONE',  ( -0.000000000000000000, 1.000000000000000000, 3.491481338843133355E-15 ) ) ;
#58864=CARTESIAN_POINT ( 'NONE',  ( -4.219116599806928214, -3.300289026998414865, 32.46337939537583139 ) ) ;
#58865=CARTESIAN_POINT ( 'NONE',  ( -7.596208436775802930, -11.56426240980093745, 33.07394671870546432 ) ) ;
#58866=CARTESIAN_POINT ( 'NONE',  ( 16.94623247381277054, -8.191372820521381826, 34.95448215188423546 ) ) ;
#58867=CARTESIAN_POINT ( 'NONE',  ( 6.856994543716788293, -12.62096338111211580, 30.90682066428152197 ) ) ;
#58868=CARTESIAN_POINT ( 'NONE',  ( -11.53846153846153655, -3.937682226553329556, 33.60647404775216529 ) ) ;
#58870=CARTESIAN_POINT ( 'NONE',  ( -15.45369618967607828, -12.64616026154729411, 30.79003144601914244 ) ) ;
#58871=CARTESIAN_POINT ( 'NONE',  ( -14.37296230824862775, -11.67786785259540849, 32.92929555188721480 ) ) ;
#58872=AXIS2_PLACEMENT_3D ( 'NONE', #21041, #6222, #7544 ) ;
#58873=CARTESIAN_POINT ( 'NONE',  ( -7.780086512803768173, -9.905515769479276145, 34.41647553114623292 ) ) ;
#58875=CARTESIAN_POINT ( 'NONE',  ( 14.53047184896071897, -5.913360116392397892, 34.49180327182771322 ) ) ;
#58876=CARTESIAN_POINT ( 'NONE',  ( -11.28840722682322273, -9.943054286541403997, 34.11300777759954883 ) ) ;
#58877=VECTOR ( 'NONE', #63088, 1000.000000000000114 ) ;
#58878=CARTESIAN_POINT ( 'NONE',  ( -5.999999999999998224, -11.91647553114624181, 32.58852847137148245 ) ) ;
#58879=CARTESIAN_POINT ( 'NONE',  ( -1.134669975237341477, -12.07971442181322352, 32.31769673815850297 ) ) ;
#58880=ORIENTED_EDGE ( 'NONE', *, *, #36123, .F. ) ;
#58881=DIRECTION ( 'NONE',  ( 0.000000000000000000, 0.8660254037844377084, 0.5000000000000015543 ) ) ;
#58882=CARTESIAN_POINT ( 'NONE',  ( 7.053868730901709405, -4.809403383903225304, 33.96459661697924304 ) ) ;
#58884=CARTESIAN_POINT ( 'NONE',  ( -10.86540783960607293, -2.588893531581426988, 31.60682220781847818 ) ) ;
#58885=LINE ( 'NONE', #24659, #61344 ) ;
#58887=CARTESIAN_POINT ( 'NONE',  ( -16.40382289789474513, -4.075325502946085976, 33.72974371597207721 ) ) ;
#58889=DIRECTION ( 'NONE',  ( -0.000000000000000000, 0.5000000000000011102, -0.8660254037844380415 ) ) ;
#58890=CARTESIAN_POINT ( 'NONE',  ( 11.66850659438130755, -2.254550872974306674, 29.97347326024527092 ) ) ;
#58891=VERTEX_POINT ( 'NONE', #22480 ) ;
#58892=DIRECTION ( 'NONE',  ( 0.000000000000000000, 0.4999999999999985567, 0.8660254037844395958 ) ) ;
#58893=CARTESIAN_POINT ( 'NONE',  ( -12.46153846153846168, -8.164416787775445883, 34.95778746994557906 ) ) ;
#58894=CARTESIAN_POINT ( 'NONE',  ( -5.076923076923075762, -8.973038597847269315, 34.52809138561121927 ) ) ;
#58895=CARTESIAN_POINT ( 'NONE',  ( 8.992010310499175318, -5.114059244376869984, 34.14424750095245287 ) ) ;
#58896=VERTEX_POINT ( 'NONE', #49944 ) ;
#58898=CARTESIAN_POINT ( 'NONE',  ( -12.59222906464876779, -2.494641256782728966, 31.33461815524612959 ) ) ;
#58900=ORIENTED_EDGE ( 'NONE', *, *, #12444, .T. ) ;
#58901=ORIENTED_EDGE ( 'NONE', *, *, #64148, .T. ) ;
#58902=ORIENTED_EDGE ( 'NONE', *, *, #2428, .F. ) ;
#58903=CARTESIAN_POINT ( 'NONE',  ( 3.480823650682684178, -2.318338780012835443, 30.59689888758630261 ) ) ;
#58904=CARTESIAN_POINT ( 'NONE',  ( 6.222779668978068557, -2.353885683473779800, 30.79025554430704759 ) ) ;
#58905=CARTESIAN_POINT ( 'NONE',  ( 2.530471848960717196, -5.913360116392399668, 34.49180327182771322 ) ) ;
#58907=ORIENTED_EDGE ( 'NONE', *, *, #7090, .F. ) ;
#58908=ORIENTED_EDGE ( 'NONE', *, *, #29470, .F. ) ;
#58909=CARTESIAN_POINT ( 'NONE',  ( 15.48071474911737333, -5.057305518903948638, 34.11320923018887896 ) ) ;
#58910=ORIENTED_EDGE ( 'NONE', *, *, #71313, .F. ) ;
#58911=CARTESIAN_POINT ( 'NONE',  ( -6.923076923077045919, -4.320704448113951379, 33.92786785259630022 ) ) ;
#58912=CYLINDRICAL_SURFACE ( 'NONE', #12187, 0.2499999999999973355 ) ;
#58913=ADVANCED_FACE ( 'NONE', ( #71100 ), #50381, .F. ) ;
#58915=VECTOR ( 'NONE', #36766, 1000.000000000000000 ) ;
#58916=CARTESIAN_POINT ( 'NONE',  ( -13.38461538461538325, -13.63283147151868846, 33.57946703557072254 ) ) ;
#58917=DIRECTION ( 'NONE',  ( -0.000000000000000000, 1.000000000000000000, -0.000000000000000000 ) ) ;
#58918=VERTEX_POINT ( 'NONE', #86870 ) ;
#58919=B_SPLINE_CURVE_WITH_KNOTS ( 'NONE', 3,
 ( #62037, #55279, #346, #26932, #68798, #21043, #20177, #69681, #35456, #48072 ),
 .UNSPECIFIED., .F., .F.,
 ( 4, 2, 2, 2, 4 ),
 ( 0.000000000000000000, 0.0001954339857564077183, 0.0003908679715128154366, 0.0005863019572692231007, 0.0007817359430256308733 ),
 .UNSPECIFIED. ) ;
#58921=EDGE_LOOP ( 'NONE', ( #9765, #8539, #74357, #29354 ) ) ;
#58922=AXIS2_PLACEMENT_3D ( 'NONE', #49640, #15424, #42895 ) ;
#58923=VERTEX_POINT ( 'NONE', #64777 ) ;
#58924=CARTESIAN_POINT ( 'NONE',  ( 14.98079249982687955, -2.564618984488975517, 30.55390908950641915 ) ) ;
#58925=ORIENTED_EDGE ( 'NONE', *, *, #19806, .F. ) ;
#58927=CARTESIAN_POINT ( 'NONE',  ( 18.22301284409340028, -5.582272713120730145, 34.63742843783360570 ) ) ;
#58928=VERTEX_POINT ( 'NONE', #32345 ) ;
#58929=EDGE_CURVE ( 'NONE', #56388, #67048, #14714, .T. ) ;
#58930=CARTESIAN_POINT ( 'NONE',  ( -13.60754160213153163, -4.186968288167449259, 33.49512374952580274 ) ) ;
#58931=CARTESIAN_POINT ( 'NONE',  ( -1.384615384615505151, -8.613356846316285953, 34.62446782046622218 ) ) ;
#58932=CARTESIAN_POINT ( 'NONE',  ( -5.999999999999998224, -3.322132147404559976, 32.92929555188717927 ) ) ;
#58933=FACE_BOUND ( 'NONE', #42435, .T. ) ;
#58934=CARTESIAN_POINT ( 'NONE',  ( -16.15384615384627409, -12.27809138561165270, 31.22303859784587132 ) ) ;
#58935=CARTESIAN_POINT ( 'NONE',  ( 4.153846153846030731, -2.379036618888197729, 30.90682066428292885 ) ) ;
#58936=CARTESIAN_POINT ( 'NONE',  ( -10.36533019547115941, -10.82426656108012075, 33.81400080652039009 ) ) ;
#58937=CARTESIAN_POINT ( 'NONE',  ( 17.01165307636676260, -9.528491918058357157, 34.59228464037090589 ) ) ;
#58938=CARTESIAN_POINT ( 'NONE',  ( -8.638705330997128229, -12.15418822224088835, 32.17964115625579069 ) ) ;
#58940=CARTESIAN_POINT ( 'NONE',  ( 15.23076923076923173, -2.900454961884010974, 35.62045528018868623 ) ) ;
#58941=VERTEX_POINT ( 'NONE', #25139 ) ;
#58942=CARTESIAN_POINT ( 'NONE',  ( 10.61538461538449596, -10.90142922262034020, 33.41473453929536674 ) ) ;
#58943=CARTESIAN_POINT ( 'NONE',  ( 12.46153846153846168, -1.422936976036506707, 30.56769352161908415 ) ) ;
#58944=VERTEX_POINT ( 'NONE', #17946 ) ;
#58945=ORIENTED_EDGE ( 'NONE', *, *, #7841, .T. ) ;
#58946=CARTESIAN_POINT ( 'NONE',  ( -6.673022611438607754, -8.303483539816728154, 34.68545999027711702 ) ) ;
#58947=CARTESIAN_POINT ( 'NONE',  ( 14.98079248672063990, -2.920706130388546651, 32.31842814019191223 ) ) ;
#58948=DIRECTION ( 'NONE',  ( -0.000000000000000000, -0.3420201433256694901, -0.9396926207859082059 ) ) ;
#58949=CARTESIAN_POINT ( 'NONE',  ( 9.692307692307695177, -13.87047571288749737, 32.06866353760679544 ) ) ;
#58950=CARTESIAN_POINT ( 'NONE',  ( -11.60373153901785948, -10.33852847137145048, 34.16647553114627556 ) ) ;
#58951=ORIENTED_EDGE ( 'NONE', *, *, #50866, .T. ) ;
#58953=EDGE_CURVE ( 'NONE', #69595, #67905, #73749, .T. ) ;
#58954=EDGE_CURVE ( 'NONE', #62271, #48748, #53043, .T. ) ;
#58955=CYLINDRICAL_SURFACE ( 'NONE', #73114, 0.2499999999999998890 ) ;
#58956=CARTESIAN_POINT ( 'NONE',  ( 18.24994551834813805, -3.712312575010499494, 33.01462480002815170 ) ) ;
#58957=CARTESIAN_POINT ( 'NONE',  ( -9.915233909823838232, -4.186968288167449259, 33.49512374952580274 ) ) ;
#58958=CARTESIAN_POINT ( 'NONE',  ( 7.596130608860880429, -5.851115903089112003, 34.47074536777953568 ) ) ;
#58959=CARTESIAN_POINT ( 'NONE',  ( 10.86543892702293412, -4.235687564193448829, 33.53795663066793509 ) ) ;
#58960=( NAMED_UNIT ( * ) SI_UNIT ( $, .STERADIAN. ) SOLID_ANGLE_UNIT ( ) );
#58961=CYLINDRICAL_SURFACE ( 'NONE', #46318, 0.2500000000000008882 ) ;
#58963=ORIENTED_EDGE ( 'NONE', *, *, #936, .F. ) ;
#58965=B_SPLINE_CURVE_WITH_KNOTS ( 'NONE', 3,
 ( #56994, #50224, #70519, #44804, #72283, #64627, #43487, #8823, #85815, #29976 ),
 .UNSPECIFIED., .F., .F.,
 ( 4, 2, 2, 2, 4 ),
 ( 0.000000000000000000, 0.0001954311564186867660, 0.0003908623128373735320, 0.0005862934692560603251, 0.0007817246256747470640 ),
 .UNSPECIFIED. ) ;
#58966=CARTESIAN_POINT ( 'NONE',  ( -14.37377468705243722, -4.661471528628507777, 34.16647553114621871 ) ) ;
#58967=CARTESIAN_POINT ( 'NONE',  ( -17.77657303813842304, -7.630147231320743018, 34.74852402298682819 ) ) ;
#58968=CARTESIAN_POINT ( 'NONE',  ( 18.25005431163831204, -5.728107161865375829, 34.42597550085002922 ) ) ;
#58969=ADVANCED_FACE ( 'NONE', ( #45851 ), #31450, .F. ) ;
#58970=CARTESIAN_POINT ( 'NONE',  ( 3.930361229281820190, -10.97335522853832579, 33.68706563782419749 ) ) ;
#58971=CARTESIAN_POINT ( 'NONE',  ( 16.82692307692307665, -7.433932668274255917, 35.00000000000000711 ) ) ;
#58974=LINE ( 'NONE', #86478, #10039 ) ;
#58975=CARTESIAN_POINT ( 'NONE',  ( -8.769230769230768274, -12.62096338111211580, 30.90682066428153263 ) ) ;
#58976=CARTESIAN_POINT ( 'NONE',  ( -6.065249931774084224, -2.255955759149247619, 30.00000000000013856 ) ) ;
#58977=FACE_OUTER_BOUND ( 'NONE', #60032, .T. ) ;
#58978=CARTESIAN_POINT ( 'NONE',  ( -12.46153846153846168, -3.513871655860378418, 32.76840700105978499 ) ) ;
#58979=CARTESIAN_POINT ( 'NONE',  ( -12.71151520558705350, -8.347322224742351082, 34.93158281831414058 ) ) ;
#58980=CARTESIAN_POINT ( 'NONE',  ( -3.100243529005665355, -11.93748526763465279, 32.05452791011430946 ) ) ;
#58981=CARTESIAN_POINT ( 'NONE',  ( -0.2387589202700531599, -11.41317474335729187, 32.86274602512330034 ) ) ;
#58983=CARTESIAN_POINT ( 'NONE',  ( 9.692307692307570832, -5.094484230521993062, 34.41647553114689373 ) ) ;
#58984=CARTESIAN_POINT ( 'NONE',  ( -3.230769230769352962, -12.51329471203414379, 31.30864560766407578 ) ) ;
#58985=VERTEX_POINT ( 'NONE', #71988 ) ;
#58986=CARTESIAN_POINT ( 'NONE',  ( -16.15384615384627409, -9.528491918059723176, 34.59228464037033035 ) ) ;
#58987=CARTESIAN_POINT ( 'NONE',  ( 2.980769230769232170, -2.499999999999998668, 29.75000000000000355 ) ) ;
#58988=CARTESIAN_POINT ( 'NONE',  ( 13.16168842570853492, -6.459968553980841577, 34.89616026154728701 ) ) ;
#58990=AXIS2_PLACEMENT_3D ( 'NONE', #13897, #68842, #48559 ) ;
#58991=CIRCLE ( 'NONE', #7185, 0.2500000000000002220 ) ;
#58992=CARTESIAN_POINT ( 'NONE',  ( 5.076923076923075762, -10.05456864172156806, 36.03766855953608683 ) ) ;
#58993=CARTESIAN_POINT ( 'NONE',  ( 14.24242230713598900, -5.094484230520674117, 34.41647553114621161 ) ) ;
#58994=FACE_OUTER_BOUND ( 'NONE', #68889, .T. ) ;
#58995=ORIENTED_EDGE ( 'NONE', *, *, #66365, .F. ) ;
#58999=ORIENTED_EDGE ( 'NONE', *, *, #7841, .F. ) ;
#59000=AXIS2_PLACEMENT_3D ( 'NONE', #71893, #70123, #42665 ) ;
#59001=CYLINDRICAL_SURFACE ( 'NONE', #1114, 0.2499999999999995559 ) ;
#59002=STYLED_ITEM ( 'NONE', ( #73831 ), #63293 ) ;
#59003=ORIENTED_EDGE ( 'NONE', *, *, #85067, .T. ) ;
#59004=CARTESIAN_POINT ( 'NONE',  ( -18.06527044596078113, -11.94971097300153140, 32.03036669348370680 ) ) ;
#59005=CARTESIAN_POINT ( 'NONE',  ( -7.780085495151404906, -11.69971097300155094, 32.46337939537588113 ) ) ;
#59006=CARTESIAN_POINT ( 'NONE',  ( 15.45354877203764232, -2.847695495035523550, 31.58253572463339154 ) ) ;
#59007=EDGE_LOOP ( 'NONE', ( #82684, #42745 ) ) ;
#59008=CARTESIAN_POINT ( 'NONE',  ( -0.4615384615381466493, -2.255955759149395501, 30.00000000000324363 ) ) ;
#59009=B_SPLINE_CURVE_WITH_KNOTS ( 'NONE', 3,
 ( #58305, #51086, #43909, #38047, #17330, #45689 ),
 .UNSPECIFIED., .F., .F.,
 ( 4, 2, 4 ),
 ( 0.0003909512603273816180, 0.0005862562993132069836, 0.0007815613382990322950 ),
 .UNSPECIFIED. ) ;
#59010=ORIENTED_EDGE ( 'NONE', *, *, #47043, .T. ) ;
#59012=EDGE_LOOP ( 'NONE', ( #29839, #85515 ) ) ;
#59014=CARTESIAN_POINT ( 'NONE',  ( 0.5923302693632481741, -11.18335022499818621, 33.13157742990016885 ) ) ;
#59015=EDGE_LOOP ( 'NONE', ( #33525, #87935 ) ) ;
#59016=CARTESIAN_POINT ( 'NONE',  ( -10.61538461538461320, -13.88283147151868846, 33.14645433367849847 ) ) ;
#59017=DIRECTION ( 'NONE',  ( 0.000000000000000000, 0.8660254037844377084, -0.5000000000000015543 ) ) ;
#59018=DIRECTION ( 'NONE',  ( -0.000000000000000000, 1.000000000000000000, -0.000000000000000000 ) ) ;
#59019=EDGE_CURVE ( 'NONE', #61347, #70654, #65092, .T. ) ;
#59020=CARTESIAN_POINT ( 'NONE',  ( -5.999999999999998224, -12.29105614889573062, 35.45975837776705220 ) ) ;
#59021=CARTESIAN_POINT ( 'NONE',  ( -13.16183571563731824, -12.11081565061824250, 32.26097654155340422 ) ) ;
#59022=EDGE_LOOP ( 'NONE', ( #67187, #30684, #35839, #7524 ) ) ;
#59023=ORIENTED_EDGE ( 'NONE', *, *, #23436, .F. ) ;
#59024=EDGE_LOOP ( 'NONE', ( #62691, #53818, #74328, #61419, #23156, #81480 ) ) ;
#59025=CARTESIAN_POINT ( 'NONE',  ( 3.230769230769231726, -12.78798330534102945, 29.74999999999997868 ) ) ;
#59026=ORIENTED_EDGE ( 'NONE', *, *, #54849, .T. ) ;
#59028=EDGE_CURVE ( 'NONE', #56098, #14112, #20595, .T. ) ;
#59029=CARTESIAN_POINT ( 'NONE',  ( 5.076923076923075762, -13.63283147151868846, 33.57946703557072254 ) ) ;
#59030=CARTESIAN_POINT ( 'NONE',  ( -10.68065506134539078, -9.442884908240170461, 34.35708131394840592 ) ) ;
#59031=EDGE_CURVE ( 'NONE', #68235, #53721, #71542, .T. ) ;
#59032=ORIENTED_EDGE ( 'NONE', *, *, #14517, .T. ) ;
#59033=ORIENTED_EDGE ( 'NONE', *, *, #83874, .T. ) ;
#59034=CARTESIAN_POINT ( 'NONE',  ( 13.38461538461526423, -5.941354392335915335, 34.76329471203413846 ) ) ;
#59035=ORIENTED_EDGE ( 'NONE', *, *, #30467, .T. ) ;
#59036=CARTESIAN_POINT ( 'NONE',  ( -18.24997674404858827, -9.234221910056350069, 34.70572697212741531 ) ) ;
#59037=EDGE_CURVE ( 'NONE', #72270, #49557, #10404, .T. ) ;
#59038=CARTESIAN_POINT ( 'NONE',  ( -11.76138775597768316, -3.586966769969701208, 32.86292498521069660 ) ) ;
#59039=CARTESIAN_POINT ( 'NONE',  ( -9.561469361820931212, -7.277220318596961057, 34.99547417642776992 ) ) ;
#59040=FACE_BOUND ( 'NONE', #83286, .T. ) ;
#59041=ORIENTED_EDGE ( 'NONE', *, *, #14071, .T. ) ;
#59042=CARTESIAN_POINT ( 'NONE',  ( 7.846153846153846700, -8.973038597847269315, 34.52809138561121927 ) ) ;
#59043=CARTESIAN_POINT ( 'NONE',  ( -4.153846153846152411, -12.29105614889573062, 35.45975837776705220 ) ) ;
#59044=VECTOR ( 'NONE', #65803, 1000.000000000000000 ) ;
#59045=EDGE_CURVE ( 'NONE', #40306, #57930, #30803, .T. ) ;
#59046=CYLINDRICAL_SURFACE ( 'NONE', #84851, 0.2500000000000009437 ) ;
#59048=CARTESIAN_POINT ( 'NONE',  ( -1.515306851282943956, -2.541943142973489778, 30.39792223712631980 ) ) ;
#59049=ORIENTED_EDGE ( 'NONE', *, *, #27419, .F. ) ;
#59050=CARTESIAN_POINT ( 'NONE',  ( 9.469381474791543241, -2.554751324335735152, 30.48935550225260727 ) ) ;
#59052=EDGE_LOOP ( 'NONE', ( #8269, #75851 ) ) ;
#59054=CARTESIAN_POINT ( 'NONE',  ( 6.000000000000001776, -11.91647553114624181, 32.58852847137148245 ) ) ;
#59055=CARTESIAN_POINT ( 'NONE',  ( 10.61538461538449596, -6.026961402154118019, 34.52809138561165270 ) ) ;
#59056=DIRECTION ( 'NONE',  ( -0.000000000000000000, -1.000000000000000000, 3.491481338843133355E-15 ) ) ;
#59058=CARTESIAN_POINT ( 'NONE',  ( 1.384615384615386802, -9.780366693483667717, 34.19971097300155094 ) ) ;
#59059=CARTESIAN_POINT ( 'NONE',  ( 1.607395053593452472, -4.226511098958374291, 33.85474049983370293 ) ) ;
#59061=EDGE_CURVE ( 'NONE', #10433, #31195, #37183, .T. ) ;
#59063=CARTESIAN_POINT ( 'NONE',  ( -11.76138775597768138, -9.886141570436013382, 34.14413921362392301 ) ) ;
#59064=CARTESIAN_POINT ( 'NONE',  ( -14.30769230769199218, -2.255955759149395501, 30.00000000000324363 ) ) ;
#59066=CARTESIAN_POINT ( 'NONE',  ( 10.68145296638705410, -11.69971097300155272, 32.46337939537588113 ) ) ;
#59067=ORIENTED_EDGE ( 'NONE', *, *, #51691, .F. ) ;
#59068=EDGE_LOOP ( 'NONE', ( #1300, #5478 ) ) ;
#59069=FACE_BOUND ( 'NONE', #69954, .T. ) ;
#59070=VERTEX_POINT ( 'NONE', #75541 ) ;
#59071=ADVANCED_FACE ( 'NONE', ( #40450 ), #26480, .F. ) ;
#59072=CARTESIAN_POINT ( 'NONE',  ( 7.780070435197967704, -2.721908614388772740, 31.22303859784724622 ) ) ;
#59073=CARTESIAN_POINT ( 'NONE',  ( 5.011653076366756387, -3.083524468853724443, 32.58852847137143272 ) ) ;
#59075=ORIENTED_EDGE ( 'NONE', *, *, #4739, .F. ) ;
#59076=CYLINDRICAL_SURFACE ( 'NONE', #82722, 0.2499999999999998890 ) ;
#59077=CARTESIAN_POINT ( 'NONE',  ( -18.00000000000000000, -3.513871655860376197, 32.76840700105977788 ) ) ;
#59078=CARTESIAN_POINT ( 'NONE',  ( 5.011652630962299959, -2.892918686051582089, 31.69288490824015270 ) ) ;
#59079=DIRECTION ( 'NONE',  ( -0.000000000000000000, -0.5000000000000009992, -0.8660254037844380415 ) ) ;
#59080=CARTESIAN_POINT ( 'NONE',  ( -11.47320596718551045, -9.442884908240273489, 34.35708131394835618 ) ) ;
#59082=CARTESIAN_POINT ( 'NONE',  ( 0.4615384615384611200, -9.780366693483667717, 34.19971097300155094 ) ) ;
#59083=ORIENTED_EDGE ( 'NONE', *, *, #71660, .F. ) ;
#59084=CARTESIAN_POINT ( 'NONE',  ( -7.596099534515530216, -9.148310452688876993, 34.47095581063188519 ) ) ;
#59085=CARTESIAN_POINT ( 'NONE',  ( -12.52762084089859407, -2.833524468853757305, 32.15551576947924417 ) ) ;
#59086=CARTESIAN_POINT ( 'NONE',  ( 20.99999999999999645, -10.75000000000000000, 29.75000000000000355 ) ) ;
#59087=CARTESIAN_POINT ( 'NONE',  ( -15.23076923076922995, -2.486705287966279876, 31.30864560766543647 ) ) ;
#59088=CARTESIAN_POINT ( 'NONE',  ( -5.749999999999984013, -2.249999999999999112, 29.81603969181031033 ) ) ;
#59089=CARTESIAN_POINT ( 'NONE',  ( 5.207714884747860928, -12.38066358083363738, 30.83685684665853444 ) ) ;
#59090=AXIS2_PLACEMENT_3D ( 'NONE', #69480, #62709, #21738 ) ;
#59092=EDGE_LOOP ( 'NONE', ( #11557, #75522, #38190, #21014 ) ) ;
#59094=CARTESIAN_POINT ( 'NONE',  ( 2.438482748659259958, -3.957578996910244395, 33.62503395064540257 ) ) ;
#59095=CARTESIAN_POINT ( 'NONE',  ( 6.000000000000309086, -2.506253911140614576, 30.00000000000323297 ) ) ;
#59096=ORIENTED_EDGE ( 'NONE', *, *, #43840, .F. ) ;
#59098=CARTESIAN_POINT ( 'NONE',  ( -1.384615384615076605, -2.506253911140615021, 30.00000000000323297 ) ) ;
#59100=B_SPLINE_CURVE_WITH_KNOTS ( 'NONE', 3,
 ( #61217, #82845, #21120, #48590, #13487, #42302, #14368, #21569, #7621, #35083 ),
 .UNSPECIFIED., .F., .F.,
 ( 4, 2, 2, 2, 4 ),
 ( 0.000000000000000000, 0.0001954311564186866305, 0.0003908623128373732609, 0.0005862934692560598914, 0.0007817246256747465219 ),
 .UNSPECIFIED. ) ;
#59101=B_SPLINE_CURVE_WITH_KNOTS ( 'NONE', 3,
 ( #60260, #17952, #53050, #31003, #3530, #10747, #5326, #17054, #18395, #71993 ),
 .UNSPECIFIED., .F., .F.,
 ( 4, 2, 2, 2, 4 ),
 ( 0.0007817359430256390048, 0.0009771253907250078159, 0.001172514838424376735, 0.001367904286123745655, 0.001563293733823114574 ),
 .UNSPECIFIED. ) ;
#59102=CARTESIAN_POINT ( 'NONE',  ( 17.32686848630112308, -3.520799739797213501, 33.17531984108286025 ) ) ;
#59103=CARTESIAN_POINT ( 'NONE',  ( 9.019285189144223835, -11.47946981652013498, 33.17500667209847620 ) ) ;
#59104=CARTESIAN_POINT ( 'NONE',  ( 17.86930939688968678, -11.93127051446800380, 32.56575433478200665 ) ) ;
#59105=CARTESIAN_POINT ( 'NONE',  ( 5.777073782483853392, -8.239355502252617924, 34.69524867566427417 ) ) ;
#59106=ORIENTED_EDGE ( 'NONE', *, *, #81549, .F. ) ;
#59107=EDGE_CURVE ( 'NONE', #19283, #51157, #26923, .T. ) ;
#59108=CARTESIAN_POINT ( 'NONE',  ( -2.980823821391186623, -12.68172785388650681, 30.59649109432439218 ) ) ;
#59109=LINE ( 'NONE', #54912, #88035 ) ;
#59111=CYLINDRICAL_SURFACE ( 'NONE', #34030, 0.2499999999999986955 ) ;
#59112=CARTESIAN_POINT ( 'NONE',  ( -3.230769230769351186, -11.94971097300221174, 32.03036669348237098 ) ) ;
#59113=ORIENTED_EDGE ( 'NONE', *, *, #59795, .T. ) ;
#59114=CARTESIAN_POINT ( 'NONE',  ( 10.61538461538449418, -9.528491918059723176, 34.59228464037033035 ) ) ;
#59115=ORIENTED_EDGE ( 'NONE', *, *, #62528, .F. ) ;
#59116=CARTESIAN_POINT ( 'NONE',  ( 13.63456090296352841, -3.712312575010499494, 33.01462480002815170 ) ) ;
#59117=CARTESIAN_POINT ( 'NONE',  ( 16.40384615384615330, -2.249999999999998668, 29.75000000000000355 ) ) ;
#59118=CARTESIAN_POINT ( 'NONE',  ( 17.77651507543566822, -10.23692288466677880, 34.23039457007281072 ) ) ;
#59119=ORIENTED_EDGE ( 'NONE', *, *, #67690, .F. ) ;
#59120=CARTESIAN_POINT ( 'NONE',  ( 8.769230769230768274, -10.51840700105979565, 33.73612834413961536 ) ) ;
#59121=CARTESIAN_POINT ( 'NONE',  ( -2.530619266599154038, -6.459968553980839800, 34.89616026154728701 ) ) ;
#59123=AXIS2_PLACEMENT_3D ( 'NONE', #58398, #44007, #86360 ) ;
#59124=EDGE_CURVE ( 'NONE', #26314, #62464, #4794, .T. ) ;
#59125=CARTESIAN_POINT ( 'NONE',  ( -7.846153846153844924, -4.661471528628507777, 34.16647553114623292 ) ) ;
#59126=CYLINDRICAL_SURFACE ( 'NONE', #77112, 0.2500000000000008882 ) ;
#59127=ORIENTED_EDGE ( 'NONE', *, *, #40164, .F. ) ;
#59128=CARTESIAN_POINT ( 'NONE',  ( 8.769230769230768274, -6.386643153685126251, 34.62446782046654192 ) ) ;
#59130=CARTESIAN_POINT ( 'NONE',  ( 8.638539302563209787, -12.38065189839062263, 30.83690757178629482 ) ) ;
#59131=B_SPLINE_CURVE_WITH_KNOTS ( 'NONE', 3,
 ( #66888, #87181, #88958, #54689, #88079, #5186, #52911, #47492, #19145, #61010 ),
 .UNSPECIFIED., .F., .F.,
 ( 4, 2, 2, 2, 4 ),
 ( 0.000000000000000000, 0.0001954339857564078809, 0.0003908679715128157619, 0.0005863019572692236428, 0.0007817359430256315238 ),
 .UNSPECIFIED. ) ;
#59133=CARTESIAN_POINT ( 'NONE',  ( -0.3954711281883865337, -2.486705287966280320, 31.30864560766543647 ) ) ;
#59134=EDGE_CURVE ( 'NONE', #45405, #86404, #85521, .T. ) ;
#59135=B_SPLINE_CURVE_WITH_KNOTS ( 'NONE', 3,
 ( #70184, #8493, #35965, #89154, #41839, #27870, #70629, #63421, #1728, #27432 ),
 .UNSPECIFIED., .F., .F.,
 ( 4, 2, 2, 2, 4 ),
 ( 0.0007817246256747450040, 0.0009771112852218881168, 0.001172497944769031230, 0.001367884604316174342, 0.001563271263863317455 ),
 .UNSPECIFIED. ) ;
#59136=CARTESIAN_POINT ( 'NONE',  ( 7.596177102105255763, -12.41104346484419452, 31.60698883733904196 ) ) ;
#59138=CARTESIAN_POINT ( 'NONE',  ( -6.857009589726848375, -2.486705287966279876, 31.30864560766543647 ) ) ;
#59140=ORIENTED_EDGE ( 'NONE', *, *, #11918, .T. ) ;
#59141=EDGE_LOOP ( 'NONE', ( #581, #88504 ) ) ;
#59142=ORIENTED_EDGE ( 'NONE', *, *, #26034, .T. ) ;
#59144=ORIENTED_EDGE ( 'NONE', *, *, #18090, .F. ) ;
#59145=ORIENTED_EDGE ( 'NONE', *, *, #29124, .T. ) ;
#59146=CARTESIAN_POINT ( 'NONE',  ( -1.134561072977070095, -3.136992222400443175, 32.19305428654138979 ) ) ;
#59147=ADVANCED_FACE ( 'NONE', ( #19277 ), #46744, .F. ) ;
#59148=CARTESIAN_POINT ( 'NONE',  ( -2.307692307692305711, -3.050289026998446396, 32.03036669348365706 ) ) ;
#59149=AXIS2_PLACEMENT_3D ( 'NONE', #16236, #1833, #22550 ) ;
#59150=CARTESIAN_POINT ( 'NONE',  ( -15.45369544828537656, -10.61292498521070549, 33.66303323003028680 ) ) ;
#59152=DIRECTION ( 'NONE',  ( 0.000000000000000000, 0.4999999999999960032, -0.8660254037844410391 ) ) ;
#59153=CARTESIAN_POINT ( 'NONE',  ( -12.52762084089859762, -12.34228464037088280, 31.77849191805838558 ) ) ;
#59154=DIRECTION ( 'NONE',  ( 0.000000000000000000, 0.3420201433256641055, -0.9396926207859100932 ) ) ;
#59155=CARTESIAN_POINT ( 'NONE',  ( -7.596099534515531104, -3.136992222400443175, 32.19305428654138979 ) ) ;
#59156=DIRECTION ( 'NONE',  ( -0.000000000000000000, -0.6427876096865404731, -0.7660444431189770143 ) ) ;
#59158=ORIENTED_EDGE ( 'NONE', *, *, #54957, .T. ) ;
#59159=ORIENTED_EDGE ( 'NONE', *, *, #28518, .T. ) ;
#59160=CARTESIAN_POINT ( 'NONE',  ( 0.2115152373170035849, -2.985938066672154445, 32.43141759479405550 ) ) ;
#59161=ORIENTED_EDGE ( 'NONE', *, *, #74949, .T. ) ;
#59162=CARTESIAN_POINT ( 'NONE',  ( 6.856994543716788293, -11.35647404775217595, 33.31231777344666511 ) ) ;
#59163=CARTESIAN_POINT ( 'NONE',  ( -17.93393266664992680, -11.35647404775217240, 33.31231777344667222 ) ) ;
#59164=DIRECTION ( 'NONE',  ( 0.000000000000000000, 0.9396926207859126468, 0.3420201433256571111 ) ) ;
#59165=CARTESIAN_POINT ( 'NONE',  ( -14.55766903863466055, -9.943427161483782584, 34.11278801902876978 ) ) ;
#59166=FACE_BOUND ( 'NONE', #21244, .T. ) ;
#59167=EDGE_LOOP ( 'NONE', ( #100, #7610, #83164, #6923 ) ) ;
#59170=ORIENTED_EDGE ( 'NONE', *, *, #71313, .T. ) ;
#59171=DIRECTION ( 'NONE',  ( -0.000000000000000000, -0.1736481776669307198, -0.9848077530122080203 ) ) ;
#59172=VERTEX_POINT ( 'NONE', #88207 ) ;
#59174=FACE_BOUND ( 'NONE', #36664, .T. ) ;
#59175=CARTESIAN_POINT ( 'NONE',  ( -10.68146699474474914, -2.833524468853757305, 32.15551576947924417 ) ) ;
#59177=VERTEX_POINT ( 'NONE', #76879 ) ;
#59179=CARTESIAN_POINT ( 'NONE',  ( 8.519230769230768274, -7.500000000000001776, 35.00000000000000000 ) ) ;
#59180=ADVANCED_FACE ( 'NONE', ( #2093 ), #30020, .F. ) ;
#59181=CARTESIAN_POINT ( 'NONE',  ( -18.00000000000012079, -4.320704448113953156, 33.92786785259630022 ) ) ;
#59182=VERTEX_POINT ( 'NONE', #77755 ) ;
#59183=CARTESIAN_POINT ( 'NONE',  ( -9.442307692307691624, -7.500000000000001776, 35.04278698407183867 ) ) ;
#59184=CARTESIAN_POINT ( 'NONE',  ( -14.43838377435986864, -5.582088688514999397, 34.36776431015576350 ) ) ;
#59185=VERTEX_POINT ( 'NONE', #21932 ) ;
#59186=VECTOR ( 'NONE', #61076, 1000.000000000000000 ) ;
#59187=CARTESIAN_POINT ( 'NONE',  ( -1.450698795571263577, -5.557115091759785130, 34.35708131394839171 ) ) ;
#59188=CARTESIAN_POINT ( 'NONE',  ( -13.63461538461538325, -7.500000000000001776, 34.75000000000000000 ) ) ;
#59190=CARTESIAN_POINT ( 'NONE',  ( -12.68446542044531000, -5.582147617184174848, 34.63737895849758530 ) ) ;
#59191=CARTESIAN_POINT ( 'NONE',  ( -10.48459280755982803, -4.809403383903225304, 33.96459661697924304 ) ) ;
#59192=CARTESIAN_POINT ( 'NONE',  ( -3.230769230769229949, -2.721908614388771852, 31.22303859784724978 ) ) ;
#59194=FACE_OUTER_BOUND ( 'NONE', #77433, .T. ) ;
#59195=CARTESIAN_POINT ( 'NONE',  ( -9.692307692307691624, -6.435427911321262684, 35.78748833219616898 ) ) ;
#59196=CARTESIAN_POINT ( 'NONE',  ( -13.60754234352223335, -4.026226216239094491, 33.68668979543634379 ) ) ;
#59197=DIRECTION ( 'NONE',  ( -0.000000000000000000, -0.6427876096865404731, -0.7660444431189770143 ) ) ;
#59198=CARTESIAN_POINT ( 'NONE',  ( -3.360916440207450506, -2.619462340734462380, 30.83744416345203021 ) ) ;
#59199=CARTESIAN_POINT ( 'NONE',  ( 0.7115384615384606759, -2.499999999999998668, 29.75000000000000355 ) ) ;
#59200=FACE_OUTER_BOUND ( 'NONE', #49510, .T. ) ;
#59201=EDGE_CURVE ( 'NONE', #6421, #33663, #63014, .T. ) ;
#59203=EDGE_LOOP ( 'NONE', ( #83105, #59635, #87984, #29697 ) ) ;
#59204=CARTESIAN_POINT ( 'NONE',  ( 2.307692307692309264, -2.517432740324522911, 35.29906147534542527 ) ) ;
#59205=ORIENTED_EDGE ( 'NONE', *, *, #7197, .T. ) ;
#59207=VERTEX_POINT ( 'NONE', #84093 ) ;
#59208=CARTESIAN_POINT ( 'NONE',  ( -3.100243792535585463, -9.503571793651733657, 34.60286762892837942 ) ) ;
#59209=ORIENTED_EDGE ( 'NONE', *, *, #80541, .T. ) ;
#59210=CARTESIAN_POINT ( 'NONE',  ( 17.74999999999999289, -7.566083408709835645, 34.74999999999999289 ) ) ;
#59212=CARTESIAN_POINT ( 'NONE',  ( -13.25382494364843389, -5.496552790871120031, 34.60292014791297532 ) ) ;
#59213=CARTESIAN_POINT ( 'NONE',  ( -8.992156986746916658, -3.105860786376062332, 32.13614157043599562 ) ) ;
#59215=LINE ( 'NONE', #79044, #44612 ) ;
#59216=CARTESIAN_POINT ( 'NONE',  ( -7.846153846153844924, -8.564572088678739092, 35.78748833219616898 ) ) ;
#59217=CARTESIAN_POINT ( 'NONE',  ( -10.61538461538461320, -4.098570777380720287, 33.41473453929634729 ) ) ;
#59218=DIRECTION ( 'NONE',  ( -0.000000000000000000, -0.000000000000000000, -1.000000000000000000 ) ) ;
#59219=AXIS2_PLACEMENT_3D ( 'NONE', #20503, #13746, #41227 ) ;
#59220=B_SPLINE_CURVE_WITH_KNOTS ( 'NONE', 3,
 ( #78385, #55901, #30216, #28899, #57677, #44144, #8174, #84730, #7733, #84288 ),
 .UNSPECIFIED., .F., .F.,
 ( 4, 2, 2, 2, 4 ),
 ( 0.000000000000000000, 0.0001954311564186864407, 0.0003908623128373728815, 0.0005862934692560593493, 0.0007817246256747457630 ),
 .UNSPECIFIED. ) ;
#59222=EDGE_CURVE ( 'NONE', #18025, #88852, #49408, .T. ) ;
#59223=CARTESIAN_POINT ( 'NONE',  ( -0.5922299282060213832, -2.541943142973490666, 30.39792223712631980 ) ) ;
#59224=LINE ( 'NONE', #44358, #64963 ) ;
#59225=VECTOR ( 'NONE', #964, 1000.000000000000000 ) ;
#59226=LINE ( 'NONE', #39858, #88181 ) ;
#59227=EDGE_CURVE ( 'NONE', #46293, #54130, #26516, .T. ) ;
#59229=VERTEX_POINT ( 'NONE', #14286 ) ;
#59230=CARTESIAN_POINT ( 'NONE',  ( 6.000000000000001776, -13.75783147151868846, 33.36296068462461051 ) ) ;
#59231=CARTESIAN_POINT ( 'NONE',  ( -14.05763799605399278, -8.303483539816728154, 34.68545999027711702 ) ) ;
#59233=CARTESIAN_POINT ( 'NONE',  ( -6.223484943723949669, -3.754499324213721234, 33.06261337010820256 ) ) ;
#59234=CARTESIAN_POINT ( 'NONE',  ( 15.29693837173189053, -7.250054483168843156, 34.74374881642865631 ) ) ;
#59235=CARTESIAN_POINT ( 'NONE',  ( -4.946397638689434828, -3.068774925481847937, 32.56582465632704526 ) ) ;
#59236=EDGE_CURVE ( 'NONE', #22041, #16132, #58721, .T. ) ;
#59239=CARTESIAN_POINT ( 'NONE',  ( -1.253823576790597638, -9.804649428959606894, 34.18742332936588468 ) ) ;
#59240=ORIENTED_EDGE ( 'NONE', *, *, #49714, .F. ) ;
#59241=VERTEX_POINT ( 'NONE', #36336 ) ;
#59243=LINE ( 'NONE', #3403, #80992 ) ;
#59244=AXIS2_PLACEMENT_3D ( 'NONE', #7857, #43416, #28118 ) ;
#59246=DIRECTION ( 'NONE',  ( -0.000000000000000000, -0.5000000000000009992, -0.8660254037844380415 ) ) ;
#59247=CARTESIAN_POINT ( 'NONE',  ( 11.60452887181161508, -2.292212530054420494, 30.41441678777542990 ) ) ;
#59249=ADVANCED_FACE ( 'NONE', ( #62458 ), #63354, .F. ) ;
#59250=ORIENTED_EDGE ( 'NONE', *, *, #39995, .F. ) ;
#59251=EDGE_CURVE ( 'NONE', #70013, #79114, #61907, .T. ) ;
#59252=EDGE_LOOP ( 'NONE', ( #49086, #15213, #19744, #27741 ) ) ;
#59253=B_SPLINE_CURVE_WITH_KNOTS ( 'NONE', 3,
 ( #10332, #86459, #79682, #52643, #11224, #30160, #80125, #18427, #37345, #36908 ),
 .UNSPECIFIED., .F., .F.,
 ( 4, 2, 2, 2, 4 ),
 ( 0.0007817246256747503166, 0.0009771112852218946220, 0.001172497944769039036, 0.001367884604316183233, 0.001563271263863327647 ),
 .UNSPECIFIED. ) ;
#59255=CARTESIAN_POINT ( 'NONE',  ( -7.053224892808618307, -12.15440758774515473, 32.17923288041532004 ) ) ;
#59257=CARTESIAN_POINT ( 'NONE',  ( 4.403900573759607084, -3.435999193479609914, 33.07426656108010832 ) ) ;
#59258=CARTESIAN_POINT ( 'NONE',  ( 2.177000841024751665, -11.18331474514187995, 33.13161551792790505 ) ) ;
#59259=CARTESIAN_POINT ( 'NONE',  ( -4.219929564802034072, -8.120952969808774569, 34.71129190930000163 ) ) ;
#59260=DIRECTION ( 'NONE',  ( -0.000000000000000000, -0.9848077530122086864, -0.1736481776669273613 ) ) ;
#59261=ORIENTED_EDGE ( 'NONE', *, *, #35329, .F. ) ;
#59262=B_SPLINE_CURVE_WITH_KNOTS ( 'NONE', 3,
 ( #18477, #46827, #80637, #5851, #79732, #66206, #52243, #74308, #5408, #45931 ),
 .UNSPECIFIED., .F., .F.,
 ( 4, 2, 2, 2, 4 ),
 ( 0.000000000000000000, 0.0001954311564186874978, 0.0003908623128373749957, 0.0005862934692560624935, 0.0007817246256747499913 ),
 .UNSPECIFIED. ) ;
#59263=VERTEX_POINT ( 'NONE', #66008 ) ;
#59265=ORIENTED_EDGE ( 'NONE', *, *, #8237, .F. ) ;
#59266=CARTESIAN_POINT ( 'NONE',  ( -12.68446467905460828, -11.24512374952581872, 33.06303171183252942 ) ) ;
#59268=CARTESIAN_POINT ( 'NONE',  ( -9.915234651214539952, -10.01117774369187252, 34.36070679894347535 ) ) ;
#59269=CARTESIAN_POINT ( 'NONE',  ( -2.084679463598910321, -4.026326845037965008, 33.68677907613344047 ) ) ;
#59271=ORIENTED_EDGE ( 'NONE', *, *, #27457, .F. ) ;
#59272=CARTESIAN_POINT ( 'NONE',  ( -14.30769230769230660, -1.466349020453238561, 30.81389545987213907 ) ) ;
#59273=ORIENTED_EDGE ( 'NONE', *, *, #37373, .T. ) ;
#59274=CARTESIAN_POINT ( 'NONE',  ( 5.749976775778544713, -9.356822207818506598, 34.66110646841856635 ) ) ;
#59275=CARTESIAN_POINT ( 'NONE',  ( -1.384615384615383471, -1.367168528481310208, 33.57946703557072254 ) ) ;
#59277=FACE_BOUND ( 'NONE', #11454, .T. ) ;
#59278=CARTESIAN_POINT ( 'NONE',  ( 10.36538461538461675, -7.433931650972300353, 34.75000000000000711 ) ) ;
#59279=CARTESIAN_POINT ( 'NONE',  ( 8.069166690247241647, -2.308499170217967134, 30.53291367094873721 ) ) ;
#59281=CARTESIAN_POINT ( 'NONE',  ( 18.00000000000000000, -2.721908614388771852, 31.22303859784724978 ) ) ;
#59282=ORIENTED_EDGE ( 'NONE', *, *, #18930, .T. ) ;
#59283=CARTESIAN_POINT ( 'NONE',  ( 6.699591979352975457, -8.496056993536548418, 34.65000542017679663 ) ) ;
#59284=EDGE_CURVE ( 'NONE', #76616, #38055, #65563, .T. ) ;
#59286=EDGE_LOOP ( 'NONE', ( #48867, #21174 ) ) ;
#59287=EDGE_CURVE ( 'NONE', #28775, #24594, #42631, .T. ) ;
#59288=CARTESIAN_POINT ( 'NONE',  ( -8.703163435880695076, -3.322132147404559976, 32.92929555188717927 ) ) ;
#59289=DIRECTION ( 'NONE',  ( 0.000000000000000000, 0.3420201433256641055, -0.9396926207859100932 ) ) ;
#59291=DIRECTION ( 'NONE',  ( -0.000000000000000000, -0.9848077530122085754, -0.1736481776669273891 ) ) ;
#59292=CYLINDRICAL_SURFACE ( 'NONE', #67397, 0.2499999999999994726 ) ;
#59293=FACE_BOUND ( 'NONE', #84782, .T. ) ;
#59294=CARTESIAN_POINT ( 'NONE',  ( 17.99999999999987566, -6.026961402154118908, 34.52809138561165270 ) ) ;
#59295=DIRECTION ( 'NONE',  ( -0.000000000000000000, -0.000000000000000000, -1.000000000000000000 ) ) ;
#59296=CARTESIAN_POINT ( 'NONE',  ( -4.153846153846152411, -1.509761064869970415, 31.06009739812519044 ) ) ;
#59297=CARTESIAN_POINT ( 'NONE',  ( -11.40841393220585509, -7.723484964179501588, 34.74522123443823318 ) ) ;
#59298=CARTESIAN_POINT ( 'NONE',  ( 14.30769230769231015, -10.67929555188718282, 33.92786785259544047 ) ) ;
#59299=CARTESIAN_POINT ( 'NONE',  ( -3.903900744468109085, -10.92531984108285670, 33.72920026020278073 ) ) ;
#59300=EDGE_CURVE ( 'NONE', #41958, #2122, #43965, .T. ) ;
#59301=CARTESIAN_POINT ( 'NONE',  ( 6.130525438233646263, -5.070358843744210198, 34.40418822224088302 ) ) ;
#59303=B_SPLINE_CURVE_WITH_KNOTS ( 'NONE', 3,
 ( #27216, #14590, #82171, #75407, #34412, #42073, #61875, #190, #27656, #55127 ),
 .UNSPECIFIED., .F., .F.,
 ( 4, 2, 2, 2, 4 ),
 ( 0.0007817246256747481482, 0.0009771112852218911526, 0.001172497944769034265, 0.001367884604316177161, 0.001563271263863320274 ),
 .UNSPECIFIED. ) ;
#59304=VECTOR ( 'NONE', #24972, 1000.000000000000227 ) ;
#59305=CARTESIAN_POINT ( 'NONE',  ( -8.703975197954745724, -6.026961402152789304, 34.52809138561124769 ) ) ;
#59306=ORIENTED_EDGE ( 'NONE', *, *, #82946, .T. ) ;
#59307=AXIS2_PLACEMENT_3D ( 'NONE', #59020, #10401, #25244 ) ;
#59309=CARTESIAN_POINT ( 'NONE',  ( 2.084765348785459604, -2.308479472611653094, 30.53278059502174457 ) ) ;
#59311=CARTESIAN_POINT ( 'NONE',  ( -9.692307692307691624, -10.51840700105979565, 33.73612834413961536 ) ) ;
#59312=CARTESIAN_POINT ( 'NONE',  ( 10.83816415665302380, -12.24180327182771855, 31.33663988360758879 ) ) ;
#59313=CARTESIAN_POINT ( 'NONE',  ( -11.53846153846166089, -4.320704448113951379, 33.92786785259630022 ) ) ;
#59316=CARTESIAN_POINT ( 'NONE',  ( -5.999999999999998224, -6.435427911321262684, 35.78748833219616898 ) ) ;
#59317=CARTESIAN_POINT ( 'NONE',  ( -14.30769230769242917, -11.67786785259630911, 32.92929555188603530 ) ) ;
#59318=CARTESIAN_POINT ( 'NONE',  ( 8.096208157792160520, -11.79725096376909654, 32.30694842903959341 ) ) ;
#59319=CARTESIAN_POINT ( 'NONE',  ( 9.692307692307695177, -3.937682226553329556, 33.60647404775216529 ) ) ;
#59320=CARTESIAN_POINT ( 'NONE',  ( 14.55774661933062397, -5.728107161865378494, 34.42597550085002922 ) ) ;
#59321=CARTESIAN_POINT ( 'NONE',  ( 9.626225312947559232, -3.322132147404559532, 32.92929555188719348 ) ) ;
#59322=CARTESIAN_POINT ( 'NONE',  ( -6.065270000556321150, -12.16647553114622049, 32.15551576947930812 ) ) ;
#59323=CARTESIAN_POINT ( 'NONE',  ( 17.14217821643591932, -8.656820664281605460, 34.87096338111211224 ) ) ;
#59325=CARTESIAN_POINT ( 'NONE',  ( 16.15384615384615330, -4.661471528628507777, 34.16647553114623292 ) ) ;
#59328=EDGE_CURVE ( 'NONE', #42300, #87108, #9290, .T. ) ;
#59329=CARTESIAN_POINT ( 'NONE',  ( 5.999999999999880096, -4.481592998941358097, 33.73612834414048933 ) ) ;
#59331=ORIENTED_EDGE ( 'NONE', *, *, #66253, .F. ) ;
#59332=CARTESIAN_POINT ( 'NONE',  ( -17.75005459062195712, -6.653508905675592722, 34.93172785388651391 ) ) ;
#59333=CARTESIAN_POINT ( 'NONE',  ( -16.94639763868943660, -9.503571793651730104, 34.60286762892837942 ) ) ;
#59334=CARTESIAN_POINT ( 'NONE',  ( 8.900021210197719412, -2.494656445102012565, 31.33466734024120015 ) ) ;
#59335=VERTEX_POINT ( 'NONE', #38101 ) ;
#59336=CARTESIAN_POINT ( 'NONE',  ( -12.46153846153846168, -9.058645607665452459, 34.76329471203371924 ) ) ;
#59337=CARTESIAN_POINT ( 'NONE',  ( -3.230769230769229949, -3.513871655860378418, 32.76840700105978499 ) ) ;
#59338=CARTESIAN_POINT ( 'NONE',  ( -8.769230769230890843, -2.625532179533778709, 30.86335684631627174 ) ) ;
#59340=EDGE_CURVE ( 'NONE', #2112, #62210, #1773, .T. ) ;
#59341=ORIENTED_EDGE ( 'NONE', *, *, #36306, .F. ) ;
#59344=ADVANCED_FACE ( 'NONE', ( #45294 ), #79089, .F. ) ;
#59345=EDGE_CURVE ( 'NONE', #48076, #66517, #54417, .T. ) ;
#59346=B_SPLINE_CURVE_WITH_KNOTS ( 'NONE', 3,
 ( #38571, #46212, #51158, #11995, #78660, #37673, #3439, #58373, #85867, #38118 ),
 .UNSPECIFIED., .F., .F.,
 ( 4, 2, 2, 2, 4 ),
 ( 0.000000000000000000, 0.0001954311564186871184, 0.0003908623128373742367, 0.0005862934692560614093, 0.0007817246256747484735 ),
 .UNSPECIFIED. ) ;
#59347=CYLINDRICAL_SURFACE ( 'NONE', #61422, 0.2500000000000002220 ) ;
#59349=ORIENTED_EDGE ( 'NONE', *, *, #37752, .F. ) ;
#59350=B_SPLINE_CURVE_WITH_KNOTS ( 'NONE', 3,
 ( #16322, #37021, #64482, #16755, #44211, #71697, #33826, #60410, #40160, #61284 ),
 .UNSPECIFIED., .F., .F.,
 ( 4, 2, 2, 2, 4 ),
 ( 0.000000000000000000, 0.0001954311564186869286, 0.0003908623128373738573, 0.0005862934692560607588, 0.0007817246256747477145 ),
 .UNSPECIFIED. ) ;
#59351=ORIENTED_EDGE ( 'NONE', *, *, #30993, .F. ) ;
#59352=FACE_OUTER_BOUND ( 'NONE', #85741, .T. ) ;
#59353=CARTESIAN_POINT ( 'NONE',  ( 9.915320536401090123, -4.026326845037962343, 33.68677907613344047 ) ) ;
#59354=CARTESIAN_POINT ( 'NONE',  ( -9.627052552794857831, -12.70778746994558439, 30.41441678777536595 ) ) ;
#59355=EDGE_CURVE ( 'NONE', #3401, #6432, #53296, .T. ) ;
#59356=CARTESIAN_POINT ( 'NONE',  ( -10.36533030374629938, -3.136992222400443175, 32.19305428654138979 ) ) ;
#59357=EDGE_CURVE ( 'NONE', #34683, #4768, #68680, .T. ) ;
#59358=EDGE_CURVE ( 'NONE', #54559, #65254, #12851, .T. ) ;
#59359=ORIENTED_EDGE ( 'NONE', *, *, #38087, .F. ) ;
#59360=ORIENTED_EDGE ( 'NONE', *, *, #42615, .F. ) ;
#59361=CARTESIAN_POINT ( 'NONE',  ( 11.78840694783958298, -11.56426240980093745, 33.07394671870546432 ) ) ;
#59362=ORIENTED_EDGE ( 'NONE', *, *, #79525, .T. ) ;
#59363=LINE ( 'NONE', #67019, #53064 ) ;
#59366=AXIS2_PLACEMENT_3D ( 'NONE', #68187, #74954, #87146 ) ;
#59367=VECTOR ( 'NONE', #32898, 1000.000000000000114 ) ;
#59368=CARTESIAN_POINT ( 'NONE',  ( 10.54930120442873687, -11.16473453929635440, 33.15142922261925662 ) ) ;
#59369=CARTESIAN_POINT ( 'NONE',  ( -13.38461538461538325, -11.11383981884818262, 36.00935417666054406 ) ) ;
#59370=EDGE_LOOP ( 'NONE', ( #26360, #38681 ) ) ;
#59371=EDGE_LOOP ( 'NONE', ( #31100, #67153 ) ) ;
#59372=B_SPLINE_CURVE_WITH_KNOTS ( 'NONE', 3,
 ( #52189, #6568, #72912, #11216, #38687, #75462, #252, #45881, #4452, #34032 ),
 .UNSPECIFIED., .F., .F.,
 ( 4, 2, 2, 2, 4 ),
 ( 0.0007817359430256392216, 0.0009771253907250078159, 0.001172514838424376302, 0.001367904286123745004, 0.001563293733823113490 ),
 .UNSPECIFIED. ) ;
#59373=B_SPLINE_CURVE_WITH_KNOTS ( 'NONE', 3,
 ( #34797, #62265, #14090, #41562, #69034, #55956, #28047, #83896, #42902, #62704 ),
 .UNSPECIFIED., .F., .F.,
 ( 4, 2, 2, 2, 4 ),
 ( 0.0007817359430256372700, 0.0009771253907250054306, 0.001172514838424373483, 0.001367904286123741535, 0.001563293733823109804 ),
 .UNSPECIFIED. ) ;
#59375=CARTESIAN_POINT ( 'NONE',  ( 7.846153846153846700, -11.69971097300155272, 32.46337939537588113 ) ) ;
#59376=VERTEX_POINT ( 'NONE', #26372 ) ;
#59377=CARTESIAN_POINT ( 'NONE',  ( 16.94677510719138169, -5.915902021225892149, 34.75552854090298638 ) ) ;
#59378=B_SPLINE_CURVE_WITH_KNOTS ( 'NONE', 3,
 ( #63067, #69840, #27079, #28870, #56326, #88808, #22099, #54541, #33834, #82037 ),
 .UNSPECIFIED., .F., .F.,
 ( 4, 2, 2, 2, 4 ),
 ( 0.0007817359430256313069, 0.0009771253907249971907, 0.001172514838424363074, 0.001367904286123728958, 0.001563293733823094842 ),
 .UNSPECIFIED. ) ;
#59380=ORIENTED_EDGE ( 'NONE', *, *, #4651, .F. ) ;
#59381=CARTESIAN_POINT ( 'NONE',  ( 6.673076923076925127, -2.499999999999998668, 29.75000000000000355 ) ) ;
#59382=CARTESIAN_POINT ( 'NONE',  ( 0.4615384615384611200, -9.584722331328613620, 36.20867863119891439 ) ) ;
#59383=CARTESIAN_POINT ( 'NONE',  ( 4.403791672194295792, -2.824170634883622188, 31.52227843825338738 ) ) ;
#59384=FACE_BOUND ( 'NONE', #63998, .T. ) ;
#59385=CARTESIAN_POINT ( 'NONE',  ( -5.207613680033385428, -9.929715669179216775, 34.40415004197138416 ) ) ;
#59386=CARTESIAN_POINT ( 'NONE',  ( -12.68446467905461006, -9.086856451489515152, 34.49173150075333183 ) ) ;
#59387=EDGE_CURVE ( 'NONE', #82473, #50376, #8172, .T. ) ;
#59388=CARTESIAN_POINT ( 'NONE',  ( -7.912237257109728361, -12.10708131394839349, 31.69288490824020244 ) ) ;
#59390=CARTESIAN_POINT ( 'NONE',  ( 15.23076923076910916, -10.33852847137269571, 34.16647553114546554 ) ) ;
#59391=DIRECTION ( 'NONE',  ( -0.000000000000000000, -0.9396926207859092051, -0.3420201433256662704 ) ) ;
#59394=CARTESIAN_POINT ( 'NONE',  ( -15.09997878980228059, -11.37503395064541678, 33.29242100308974273 ) ) ;
#59395=CARTESIAN_POINT ( 'NONE',  ( 13.38461538461538680, -1.044019251281081972, 31.83374038241031911 ) ) ;
#59396=ORIENTED_EDGE ( 'NONE', *, *, #21160, .T. ) ;
#59397=VERTEX_POINT ( 'NONE', #6104 ) ;
#59399=CARTESIAN_POINT ( 'NONE',  ( -11.76138849736838488, -12.64616026154729411, 30.79003144601914244 ) ) ;
#59400=CARTESIAN_POINT ( 'NONE',  ( 0.6845513056318556222, -8.282913670948747864, 34.94150082978203642 ) ) ;
#59401=AXIS2_PLACEMENT_3D ( 'NONE', #85268, #78059, #23549 ) ;
#59403=CARTESIAN_POINT ( 'NONE',  ( 16.21910129335899597, -6.835583212224605631, 34.95778746994559327 ) ) ;
#59404=CARTESIAN_POINT ( 'NONE',  ( 16.15384615384615330, -3.513871655860378418, 32.76840700105978499 ) ) ;
#59408=CARTESIAN_POINT ( 'NONE',  ( 18.06525513951284267, -4.320704448112858032, 33.92786785259548310 ) ) ;
#59409=CARTESIAN_POINT ( 'NONE',  ( 18.25005431163831204, -3.627508038966690496, 32.91356715214248396 ) ) ;
#59410=CARTESIAN_POINT ( 'NONE',  ( -9.692307692307812417, -4.481592998941358097, 33.73612834414048933 ) ) ;
#59411=CYLINDRICAL_SURFACE ( 'NONE', #64609, 0.2499999999999979738 ) ;
#59412=CARTESIAN_POINT ( 'NONE',  ( 0.3308478584281517865, -3.338472653186242756, 32.95098750199972670 ) ) ;
#59413=SURFACE_STYLE_FILL_AREA ( #72923 ) ;
#59414=DIRECTION ( 'NONE',  ( -0.000000000000000000, -0.1736481776669307198, -0.9848077530122080203 ) ) ;
#59416=ORIENTED_EDGE ( 'NONE', *, *, #68097, .F. ) ;
#59418=CARTESIAN_POINT ( 'NONE',  ( -8.096130590202434973, -11.47974371597208076, 33.17467449705390692 ) ) ;
#59419=CARTESIAN_POINT ( 'NONE',  ( 12.33106175342199862, -7.276988635370452485, 34.74523720219453793 ) ) ;
#59420=CARTESIAN_POINT ( 'NONE',  ( 16.37685899793955357, -2.889357225399416418, 32.26129605718031002 ) ) ;
#59421=CYLINDRICAL_SURFACE ( 'NONE', #40961, 0.2500000000000012212 ) ;
#59422=CARTESIAN_POINT ( 'NONE',  ( 2.373861448654965844, -7.250054483168843156, 34.74374881642865631 ) ) ;
#59424=CARTESIAN_POINT ( 'NONE',  ( -11.53846153846153655, -9.058645607665452459, 34.76329471203371924 ) ) ;
#59426=EDGE_CURVE ( 'NONE', #31091, #9304, #70538, .T. ) ;
#59427=CYLINDRICAL_SURFACE ( 'NONE', #4158, 0.2499999999999994726 ) ;
#59428=CARTESIAN_POINT ( 'NONE',  ( 5.750023255951409951, -10.06842814019191401, 34.32929386961144758 ) ) ;
#59429=CARTESIAN_POINT ( 'NONE',  ( -9.822454901745910405, -11.47017969459904130, 32.78971311882034456 ) ) ;
#59430=CARTESIAN_POINT ( 'NONE',  ( 1.384615384615386802, -8.973038597847269315, 34.52809138561121927 ) ) ;
#59431=CARTESIAN_POINT ( 'NONE',  ( 2.307692307692309264, -3.050289026998446396, 32.03036669348365706 ) ) ;
#59432=DIRECTION ( 'NONE',  ( 0.000000000000000000, 0.3420201433256610524, 0.9396926207859113145 ) ) ;
#59433=CARTESIAN_POINT ( 'NONE',  ( -0.2114841499001473835, -11.28795663066794219, 33.01431243580653785 ) ) ;
#59434=CARTESIAN_POINT ( 'NONE',  ( 11.53846153846153832, -6.386643153685126251, 34.62446782046654192 ) ) ;
#59435=CARTESIAN_POINT ( 'NONE',  ( -3.296039231325549768, -12.51329471203370325, 31.30864560766548976 ) ) ;
#59436=ORIENTED_EDGE ( 'NONE', *, *, #84082, .T. ) ;
#59437=DIRECTION ( 'NONE',  ( -1.000000000000000000, 0.000000000000000000, 0.000000000000000000 ) ) ;
#59438=CARTESIAN_POINT ( 'NONE',  ( -13.31854805126531005, -9.905515769479276145, 34.41647553114623292 ) ) ;
#59439=CARTESIAN_POINT ( 'NONE',  ( 13.38461538461526423, -6.835583212225970762, 34.95778746994575670 ) ) ;
#59442=VECTOR ( 'NONE', #87203, 1000.000000000000000 ) ;
#59443=CARTESIAN_POINT ( 'NONE',  ( 5.076923076922953193, -10.33852847137269571, 34.16647553114546554 ) ) ;
#59444=CARTESIAN_POINT ( 'NONE',  ( -17.32694631421604115, -2.587272538249754117, 30.68239716806877837 ) ) ;
#59445=CARTESIAN_POINT ( 'NONE',  ( 10.36538461538461853, -7.433932668274256805, 35.00000000000000711 ) ) ;
#59446=ORIENTED_EDGE ( 'NONE', *, *, #8723, .F. ) ;
#59449=CARTESIAN_POINT ( 'NONE',  ( -15.29603923132555110, -4.320704448112771878, 33.92786785259540494 ) ) ;
#59450=B_SPLINE_CURVE_WITH_KNOTS ( 'NONE', 3,
 ( #48807, #62315, #49261, #13699, #6941, #76732, #42510, #34411, #632, #28102 ),
 .UNSPECIFIED., .F., .F.,
 ( 4, 2, 2, 2, 4 ),
 ( 0.000000000000000000, 0.0001954311564186865221, 0.0003908623128373730441, 0.0005862934692560595662, 0.0007817246256747460882 ),
 .UNSPECIFIED. ) ;
#59452=VECTOR ( 'NONE', #72051, 1000.000000000000000 ) ;
#59453=B_SPLINE_CURVE_WITH_KNOTS ( 'NONE', 3,
 ( #86335, #18749, #11998, #31367, #73244, #24605, #45767, #52515, #25939, #46214 ),
 .UNSPECIFIED., .F., .F.,
 ( 4, 2, 2, 2, 4 ),
 ( 0.000000000000000000, 0.0001954311564186866305, 0.0003908623128373732609, 0.0005862934692560598914, 0.0007817246256747465219 ),
 .UNSPECIFIED. ) ;
#59454=VERTEX_POINT ( 'NONE', #80889 ) ;
#59455=CARTESIAN_POINT ( 'NONE',  ( -12.46153846153846168, -1.117168528481311540, 33.14645433367849847 ) ) ;
#59457=CARTESIAN_POINT ( 'NONE',  ( -18.13069146666756382, -11.71456829005830436, 32.44064028649417253 ) ) ;
#59458=CARTESIAN_POINT ( 'NONE',  ( -1.449885385171704399, -12.16647553114622049, 32.15551576947930812 ) ) ;
#59459=EDGE_CURVE ( 'NONE', #4299, #31229, #25391, .T. ) ;
#59460=CARTESIAN_POINT ( 'NONE',  ( 15.23076923076911093, -2.892918686052165622, 31.69288490824153470 ) ) ;
#59461=VERTEX_POINT ( 'NONE', #49298 ) ;
#59462=DIRECTION ( 'NONE',  ( 0.000000000000000000, 0.6427876096865373645, -0.7660444431189797898 ) ) ;
#59463=ORIENTED_EDGE ( 'NONE', *, *, #29492, .T. ) ;
#59464=FACE_OUTER_BOUND ( 'NONE', #70182, .T. ) ;
#59465=VERTEX_POINT ( 'NONE', #228 ) ;
#59466=LINE ( 'NONE', #32883, #41409 ) ;
#59467=CARTESIAN_POINT ( 'NONE',  ( 2.307692307692309264, -3.050289026998446396, 32.03036669348365706 ) ) ;
#59469=CARTESIAN_POINT ( 'NONE',  ( 9.823098133274644539, -9.929761469519743144, 34.40412654351204225 ) ) ;
#59470=CARTESIAN_POINT ( 'NONE',  ( 0.4615384615384611200, -2.292212530054420494, 30.41441678777542634 ) ) ;
#59472=CARTESIAN_POINT ( 'NONE',  ( -5.076923076923075762, -13.88283147151868846, 33.14645433367849847 ) ) ;
#59473=EDGE_CURVE ( 'NONE', #63264, #65067, #69128, .T. ) ;
#59475=EDGE_LOOP ( 'NONE', ( #19272, #85655, #65890, #26757 ) ) ;
#59476=EDGE_LOOP ( 'NONE', ( #29735, #37445 ) ) ;
#59477=CARTESIAN_POINT ( 'NONE',  ( 3.361294932532797208, -3.816742781228458448, 33.13167719472716044 ) ) ;
#59478=ORIENTED_EDGE ( 'NONE', *, *, #51547, .F. ) ;
#59479=DIRECTION ( 'NONE',  ( -0.000000000000000000, -0.7660444431189791237, -0.6427876096865379196 ) ) ;
#59480=DIRECTION ( 'NONE',  ( -0.000000000000000000, 0.8660254037844399289, -0.4999999999999980016 ) ) ;
#59481=VERTEX_POINT ( 'NONE', #15077 ) ;
#59482=CARTESIAN_POINT ( 'NONE',  ( 15.36129466900287532, -9.503571793651731880, 34.60286762892837942 ) ) ;
#59483=ORIENTED_EDGE ( 'NONE', *, *, #26822, .T. ) ;
#59484=CARTESIAN_POINT ( 'NONE',  ( 17.14299041027315695, -9.058645607665452459, 34.76329471203371924 ) ) ;
#59485=VERTEX_POINT ( 'NONE', #50165 ) ;
#59486=CARTESIAN_POINT ( 'NONE',  ( 9.692307692307695177, -8.120952969808772792, 34.71129190930000163 ) ) ;
#59487=CARTESIAN_POINT ( 'NONE',  ( -3.230769230769229949, -12.48256725967547354, 35.29906147534542527 ) ) ;
#59488=CARTESIAN_POINT ( 'NONE',  ( -11.53846153846166089, -12.16647553114689728, 32.15551576947799362 ) ) ;
#59489=FACE_BOUND ( 'NONE', #27390, .T. ) ;
#59490=B_SPLINE_CURVE_WITH_KNOTS ( 'NONE', 3,
 ( #19342, #67085, #38275, #72946, #25206, #4944, #5387, #80157, #18896, #32852 ),
 .UNSPECIFIED., .F., .F.,
 ( 4, 2, 2, 2, 4 ),
 ( 0.000000000000000000, 0.0001954339857564080707, 0.0003908679715128161414, 0.0005863019572692241849, 0.0007817359430256322827 ),
 .UNSPECIFIED. ) ;
#59491=VECTOR ( 'NONE', #6940, 999.9999999999998863 ) ;
#59493=CARTESIAN_POINT ( 'NONE',  ( 13.63456090296352841, -9.272278438253398036, 34.42582936511637115 ) ) ;
#59494=AXIS2_PLACEMENT_3D ( 'NONE', #2863, #30356, #24475 ) ;
#59495=CARTESIAN_POINT ( 'NONE',  ( -1.384615384615383471, -2.292212530054420494, 30.41441678777542634 ) ) ;
#59496=DIRECTION ( 'NONE',  ( 0.000000000000000000, 0.000000000000000000, 1.000000000000000000 ) ) ;
#59498=CARTESIAN_POINT ( 'NONE',  ( 8.096208157792160520, -10.66356715214248396, 33.62249196103329751 ) ) ;
#59500=CARTESIAN_POINT ( 'NONE',  ( -10.36543909703647337, -4.336752205174649433, 33.62275283266504289 ) ) ;
#59502=VERTEX_POINT ( 'NONE', #21826 ) ;
#59503=CARTESIAN_POINT ( 'NONE',  ( 10.74617642320940369, -12.38066358083363738, 30.83685684665853444 ) ) ;
#59504=CARTESIAN_POINT ( 'NONE',  ( -1.514763354347078206, -5.915902021225892149, 34.75552854090298638 ) ) ;
#59505=CYLINDRICAL_SURFACE ( 'NONE', #85912, 0.2499999999999995559 ) ;
#59506=CARTESIAN_POINT ( 'NONE',  ( -4.088590582570126308, -4.481592998940251427, 33.73612834413965089 ) ) ;
#59508=CARTESIAN_POINT ( 'NONE',  ( -15.45369544828538011, -3.586966769969701208, 32.86292498521069660 ) ) ;
#59509=ORIENTED_EDGE ( 'NONE', *, *, #19631, .F. ) ;
#59510=B_SPLINE_CURVE_WITH_KNOTS ( 'NONE', 3,
 ( #8744, #70882, #35773, #2402, #49277, #28568, #84849, #37521, #23129, #56476 ),
 .UNSPECIFIED., .F., .F.,
 ( 4, 2, 2, 2, 4 ),
 ( 0.0007817359430256315238, 0.0009771253907249976244, 0.001172514838424363508, 0.001367904286123729392, 0.001563293733823095492 ),
 .UNSPECIFIED. ) ;
#59511=DIRECTION ( 'NONE',  ( 0.000000000000000000, 0.6427876096865373645, -0.7660444431189797898 ) ) ;
#59512=CARTESIAN_POINT ( 'NONE',  ( 0.6845498131513109152, -9.886259254753564818, 34.14407573483972413 ) ) ;
#59513=CARTESIAN_POINT ( 'NONE',  ( 10.54930223602447903, -2.833524468853757305, 32.15551576947924417 ) ) ;
#59514=CARTESIAN_POINT ( 'NONE',  ( -3.903900635498010363, -3.712312575010499494, 33.01462480002815170 ) ) ;
#59515=EDGE_LOOP ( 'NONE', ( #22821, #77733, #71, #21617 ) ) ;
#59516=B_SPLINE_CURVE_WITH_KNOTS ( 'NONE', 3,
 ( #32812, #5341, #45868, #25608, #66138, #87784, #26057, #81010, #59832, #80571 ),
 .UNSPECIFIED., .F., .F.,
 ( 4, 2, 2, 2, 4 ),
 ( 0.000000000000000000, 0.0001954339857564080165, 0.0003908679715128160329, 0.0005863019572692240765, 0.0007817359430256320659 ),
 .UNSPECIFIED. ) ;
#59517=ORIENTED_EDGE ( 'NONE', *, *, #20701, .F. ) ;
#59519=CARTESIAN_POINT ( 'NONE',  ( 7.623227628637697428, -2.758268499246657957, 31.33685645148948140 ) ) ;
#59520=CARTESIAN_POINT ( 'NONE',  ( -6.222828097634878652, -7.369209533119140509, 34.99857337881830688 ) ) ;
#59521=EDGE_LOOP ( 'NONE', ( #39227, #5407, #21633, #19280 ) ) ;
#59522=CARTESIAN_POINT ( 'NONE',  ( 3.164686851409094004, -12.62096338111211580, 30.90682066428152197 ) ) ;
#59523=LINE ( 'NONE', #33397, #71622 ) ;
#59524=CARTESIAN_POINT ( 'NONE',  ( 4.853438133199130533, -2.847400154188068022, 31.58180166144859058 ) ) ;
#59525=CARTESIAN_POINT ( 'NONE',  ( 1.634560793993429906, -6.653508905675590945, 34.93172785388651391 ) ) ;
#59526=DIRECTION ( 'NONE',  ( 0.000000000000000000, 0.3420201433256641055, -0.9396926207859100932 ) ) ;
#59527=VECTOR ( 'NONE', #7777, 999.9999999999998863 ) ;
#59528=ORIENTED_EDGE ( 'NONE', *, *, #46014, .T. ) ;
#59529=CARTESIAN_POINT ( 'NONE',  ( -0.2115930521604189873, -12.07971442181321997, 32.31769673815850297 ) ) ;
#59530=VERTEX_POINT ( 'NONE', #61915 ) ;
#59531=CARTESIAN_POINT ( 'NONE',  ( -5.076923076923197442, -5.219633306517616589, 34.19971097300220464 ) ) ;
#59532=EDGE_CURVE ( 'NONE', #24126, #24932, #21069, .T. ) ;
#59533=CARTESIAN_POINT ( 'NONE',  ( 13.38461538461526423, -8.656820664282941280, 34.87096338111179961 ) ) ;
#59534=DIRECTION ( 'NONE',  ( -0.000000000000000000, 0.000000000000000000, 1.000000000000000000 ) ) ;
#59536=CARTESIAN_POINT ( 'NONE',  ( -4.153846153846274980, -5.094484230521993062, 34.41647553114689373 ) ) ;
#59537=CARTESIAN_POINT ( 'NONE',  ( -8.546451100252703270, -9.418065098278013636, 34.63729479722530158 ) ) ;
#59539=ORIENTED_EDGE ( 'NONE', *, *, #11863, .F. ) ;
#59540=CARTESIAN_POINT ( 'NONE',  ( 4.853438152358745761, -12.11044203135681840, 32.26167407432752299 ) ) ;
#59541=CYLINDRICAL_SURFACE ( 'NONE', #76452, 0.2499999999999998890 ) ;
#59542=CARTESIAN_POINT ( 'NONE',  ( -0.4615384615385826339, -5.219633306517616589, 34.19971097300220464 ) ) ;
#59543=EDGE_CURVE ( 'NONE', #60046, #39792, #29044, .T. ) ;
#59544=ORIENTED_EDGE ( 'NONE', *, *, #58714, .T. ) ;
#59545=ORIENTED_EDGE ( 'NONE', *, *, #63895, .T. ) ;
#59546=CARTESIAN_POINT ( 'NONE',  ( -8.834500769787091201, -5.941354392334499579, 34.76329471203369792 ) ) ;
#59547=CARTESIAN_POINT ( 'NONE',  ( 11.28843831424008926, -4.931416488878822335, 34.32920672191015399 ) ) ;
#59548=EDGE_CURVE ( 'NONE', #56699, #39535, #16588, .T. ) ;
#59550=CARTESIAN_POINT ( 'NONE',  ( 13.13459216039393240, -2.985938066672154445, 32.43141759479405550 ) ) ;
#59551=FACE_OUTER_BOUND ( 'NONE', #35153, .T. ) ;
#59554=B_SPLINE_CURVE_WITH_KNOTS ( 'NONE', 3,
 ( #83433, #23043, #15859, #42002, #42442, #63135, #62687, #15415, #64019, #21716 ),
 .UNSPECIFIED., .F., .F.,
 ( 4, 2, 2, 2, 4 ),
 ( 0.0007817359430256294638, 0.0009771253907249950223, 0.001172514838424360472, 0.001367904286123725922, 0.001563293733823091372 ),
 .UNSPECIFIED. ) ;
#59555=CARTESIAN_POINT ( 'NONE',  ( 9.442330961365339448, -10.66389620160130036, 33.62221079203477103 ) ) ;
#59556=EDGE_CURVE ( 'NONE', #44733, #24141, #25227, .T. ) ;
#59558=DIRECTION ( 'NONE',  ( -0.000000000000000000, -0.9396926207859093161, -0.3420201433256663259 ) ) ;
#59559=EDGE_LOOP ( 'NONE', ( #4876, #79538 ) ) ;
#59560=CARTESIAN_POINT ( 'NONE',  ( 16.02315555073584363, -12.35290016733513951, 31.75349464988449455 ) ) ;
#59561=VECTOR ( 'NONE', #51340, 1000.000000000000000 ) ;
#59562=AXIS2_PLACEMENT_3D ( 'NONE', #67043, #32810, #4440 ) ;
#59563=VERTEX_POINT ( 'NONE', #36236 ) ;
#59564=CARTESIAN_POINT ( 'NONE',  ( -0.2114841499001482161, -2.779044189368093498, 31.39831045268884324 ) ) ;
#59566=CARTESIAN_POINT ( 'NONE',  ( -16.15384615384615330, -7.500000000000001776, 35.04278698407183867 ) ) ;
#59567=EDGE_LOOP ( 'NONE', ( #37656, #18760, #20213, #84202 ) ) ;
#59568=CARTESIAN_POINT ( 'NONE',  ( 0.6845498131513103601, -4.187068189119697692, 33.49521262558774026 ) ) ;
#59569=CARTESIAN_POINT ( 'NONE',  ( -11.40766973063675493, -12.38066358083363738, 30.83685684665853444 ) ) ;
#59570=DIRECTION ( 'NONE',  ( 0.000000000000000000, 0.6427876096865368094, 0.7660444431189802339 ) ) ;
#59571=CARTESIAN_POINT ( 'NONE',  ( -7.596208436775802930, -4.932303261841489928, 34.32971442181322885 ) ) ;
#59572=CARTESIAN_POINT ( 'NONE',  ( -4.946397638689433940, -11.04252011169590020, 33.62494198852677130 ) ) ;
#59573=EDGE_CURVE ( 'NONE', #14985, #8100, #48825, .T. ) ;
#59574=ORIENTED_EDGE ( 'NONE', *, *, #73987, .F. ) ;
#59577=ORIENTED_EDGE ( 'NONE', *, *, #25004, .T. ) ;
#59578=CARTESIAN_POINT ( 'NONE',  ( 5.299935921016471596, -11.43677907613344757, 33.22367315496201456 ) ) ;
#59579=DIRECTION ( 'NONE',  ( -0.000000000000000000, 0.3420201433256694346, -0.9396926207859080948 ) ) ;
#59580=CYLINDRICAL_SURFACE ( 'NONE', #65777, 0.2500000000000009437 ) ;
#59581=EDGE_CURVE ( 'NONE', #485, #15316, #29540, .T. ) ;
#59582=CARTESIAN_POINT ( 'NONE',  ( 9.692307692307695177, -2.486705287966279876, 31.30864560766543647 ) ) ;
#59583=ADVANCED_FACE ( 'NONE', ( #16396 ), #57374, .F. ) ;
#59584=CARTESIAN_POINT ( 'NONE',  ( 1.384615384615386802, -9.819645486525091727, 36.12317359536749706 ) ) ;
#59585=LINE ( 'NONE', #31679, #45058 ) ;
#59586=CARTESIAN_POINT ( 'NONE',  ( -14.05769230769230660, -7.500000000000001776, 35.04278698407183867 ) ) ;
#59587=EDGE_LOOP ( 'NONE', ( #81320, #56667, #69512, #51349 ) ) ;
#59588=VECTOR ( 'NONE', #47889, 999.9999999999998863 ) ;
#59589=ORIENTED_EDGE ( 'NONE', *, *, #10172, .T. ) ;
#59591=ORIENTED_EDGE ( 'NONE', *, *, #83418, .T. ) ;
#59592=ORIENTED_EDGE ( 'NONE', *, *, #84625, .F. ) ;
#59593=CARTESIAN_POINT ( 'NONE',  ( -5.143005456283212595, -3.937682226553329556, 33.60647404775217240 ) ) ;
#59594=CARTESIAN_POINT ( 'NONE',  ( -3.296039231325549768, -6.835583212224499938, 34.95778746994557906 ) ) ;
#59595=CARTESIAN_POINT ( 'NONE',  ( -2.438302667316833983, -7.722926236386453702, 34.74524107206102030 ) ) ;
#59596=CARTESIAN_POINT ( 'NONE',  ( -4.153846153846152411, -2.900454961884010974, 35.62045528018868623 ) ) ;
#59597=CARTESIAN_POINT ( 'NONE',  ( 13.25446817517716980, -8.587444163452046197, 34.63053765926554206 ) ) ;
#59599=CARTESIAN_POINT ( 'NONE',  ( -5.142193522883852452, -8.613356846314824011, 34.62446782046655613 ) ) ;
#59600=CARTESIAN_POINT ( 'NONE',  ( -5.299789339986176628, -2.251424796025575770, 29.88072029997477586 ) ) ;
#59602=ORIENTED_EDGE ( 'NONE', *, *, #87946, .T. ) ;
#59603=VERTEX_POINT ( 'NONE', #23153 ) ;
#59604=ORIENTED_EDGE ( 'NONE', *, *, #76660, .T. ) ;
#59605=CARTESIAN_POINT ( 'NONE',  ( -5.999999999999998224, -1.242168528481310874, 33.36296068462461051 ) ) ;
#59606=EDGE_LOOP ( 'NONE', ( #78461, #3562 ) ) ;
#59607=CARTESIAN_POINT ( 'NONE',  ( -15.93106661257773560, -6.760870238392814535, 34.69528174975672385 ) ) ;
#59608=CARTESIAN_POINT ( 'NONE',  ( -16.40386939113911779, -10.05641848906368097, 34.04755513067966177 ) ) ;
#59609=EDGE_CURVE ( 'NONE', #36772, #60982, #65904, .T. ) ;
#59610=DIRECTION ( 'NONE',  ( -0.000000000000000000, -0.9396926207859093161, -0.3420201433256663259 ) ) ;
#59611=CARTESIAN_POINT ( 'NONE',  ( 7.146088274689772923, -2.554770724473668153, 30.48948780036025852 ) ) ;
#59612=FACE_BOUND ( 'NONE', #3189, .T. ) ;
#59613=ORIENTED_EDGE ( 'NONE', *, *, #44168, .F. ) ;
#59614=VECTOR ( 'NONE', #19742, 1000.000000000000000 ) ;
#59615=B_SPLINE_CURVE_WITH_KNOTS ( 'NONE', 3,
 ( #84742, #77083, #44154, #15389, #42860, #9499 ),
 .UNSPECIFIED., .F., .F.,
 ( 4, 2, 4 ),
 ( 0.0003909569690057856884, 0.0005862646681846128607, 0.0007815723673634400329 ),
 .UNSPECIFIED. ) ;
#59618=ORIENTED_EDGE ( 'NONE', *, *, #5208, .F. ) ;
#59619=FACE_BOUND ( 'NONE', #10884, .T. ) ;
#59621=AXIS2_PLACEMENT_3D ( 'NONE', #80455, #25500, #79563 ) ;
#59622=CARTESIAN_POINT ( 'NONE',  ( -13.45069879557126313, -10.51840700105979387, 33.73612834413961536 ) ) ;
#59623=ORIENTED_EDGE ( 'NONE', *, *, #5994, .T. ) ;
#59624=DIRECTION ( 'NONE',  ( -0.000000000000000000, 0.5000000000000009992, -0.8660254037844380415 ) ) ;
#59626=CARTESIAN_POINT ( 'NONE',  ( -5.142245992415251266, -7.749976743299137993, 34.99404534957040624 ) ) ;
#59627=ORIENTED_EDGE ( 'NONE', *, *, #26214, .T. ) ;
#59628=DIRECTION ( 'NONE',  ( -0.000000000000000000, 0.6427876096865404731, -0.7660444431189770143 ) ) ;
#59629=CARTESIAN_POINT ( 'NONE',  ( 3.100077764101669686, -12.11776431015576172, 31.66791131148498906 ) ) ;
#59630=FACE_OUTER_BOUND ( 'NONE', #75981, .T. ) ;
#59631=ORIENTED_EDGE ( 'NONE', *, *, #25033, .T. ) ;
#59632=EDGE_CURVE ( 'NONE', #79092, #54595, #10979, .T. ) ;
#59633=LINE ( 'NONE', #38936, #35892 ) ;
#59634=CARTESIAN_POINT ( 'NONE',  ( -16.85414353565466428, -11.89424750095246175, 32.13594075562311758 ) ) ;
#59635=ORIENTED_EDGE ( 'NONE', *, *, #20596, .T. ) ;
#59636=CARTESIAN_POINT ( 'NONE',  ( -17.32689982097166492, -12.65889640711025521, 30.72598325615533454 ) ) ;
#59637=CARTESIAN_POINT ( 'NONE',  ( 13.25446817517716447, -2.619462340734462380, 30.83744416345203021 ) ) ;
#59638=CARTESIAN_POINT ( 'NONE',  ( -2.372962753653082402, -2.625532179533444754, 30.86335684631481513 ) ) ;
#59639=DIRECTION ( 'NONE',  ( -0.000000000000000000, -0.7660444431189791237, -0.6427876096865379196 ) ) ;
#59640=FACE_OUTER_BOUND ( 'NONE', #20249, .T. ) ;
#59641=CARTESIAN_POINT ( 'NONE',  ( -16.15384615384615330, -1.509761064869970415, 31.06009739812519044 ) ) ;
#59643=CARTESIAN_POINT ( 'NONE',  ( -8.769230769230768274, -6.435427911321262684, 35.78748833219616898 ) ) ;
#59645=FACE_OUTER_BOUND ( 'NONE', #5114, .T. ) ;
#59647=ORIENTED_EDGE ( 'NONE', *, *, #51533, .F. ) ;
#59648=CARTESIAN_POINT ( 'NONE',  ( 5.010840697562940704, -6.343179335718451384, 34.87096338111212646 ) ) ;
#59649=ORIENTED_EDGE ( 'NONE', *, *, #34560, .F. ) ;
#59650=B_SPLINE_CURVE_WITH_KNOTS ( 'NONE', 3,
 ( #24356, #51816, #44174, #57268, #15850, #3643, #9518, #44620, #71659, #9964 ),
 .UNSPECIFIED., .F., .F.,
 ( 4, 2, 2, 2, 4 ),
 ( 0.0007817359430256304396, 0.0009771253907249963233, 0.001172514838424362424, 0.001367904286123728524, 0.001563293733823094408 ),
 .UNSPECIFIED. ) ;
#59651=ADVANCED_FACE ( 'NONE', ( #10533 ), #31696, .F. ) ;
#59653=CARTESIAN_POINT ( 'NONE',  ( -16.85414340794500276, -4.226511098958372514, 33.85474049983370293 ) ) ;
#59654=VERTEX_POINT ( 'NONE', #43864 ) ;
#59658=EDGE_CURVE ( 'NONE', #62474, #60580, #1624, .T. ) ;
#59659=CARTESIAN_POINT ( 'NONE',  ( 10.86533002476265786, -2.589246495874658383, 31.60778113518102828 ) ) ;
#59660=CARTESIAN_POINT ( 'NONE',  ( -0.2387589202700531044, -5.913360116392399668, 34.49180327182771322 ) ) ;
#59661=CARTESIAN_POINT ( 'NONE',  ( -14.30769230769230660, -10.67929555188718282, 33.92786785259544047 ) ) ;
#59662=AXIS2_PLACEMENT_3D ( 'NONE', #51749, #17999, #10347 ) ;
#59664=CARTESIAN_POINT ( 'NONE',  ( 0.4615384615384611200, -11.91647553114624181, 32.58852847137148245 ) ) ;
#59665=CARTESIAN_POINT ( 'NONE',  ( 16.15384615384615330, -6.343179335718451384, 34.87096338111211935 ) ) ;
#59667=CARTESIAN_POINT ( 'NONE',  ( 5.076923076922953193, -3.083524468854526912, 32.58852847137268327 ) ) ;
#59668=CARTESIAN_POINT ( 'NONE',  ( -10.36538461538460254, -2.249999999999999112, 29.81603969181031388 ) ) ;
#59669=ADVANCED_FACE ( 'NONE', ( #84870 ), #52389, .F. ) ;
#59672=B_SPLINE_CURVE_WITH_KNOTS ( 'NONE', 3,
 ( #944, #15354, #68084, #8152, #62197, #77052, #61744, #507, #55441, #6388 ),
 .UNSPECIFIED., .F., .F.,
 ( 4, 2, 2, 2, 4 ),
 ( 0.000000000000000000, 0.0001954311564186882568, 0.0003908623128373765136, 0.0005862934692560647703, 0.0007817246256747530271 ),
 .UNSPECIFIED. ) ;
#59673=ADVANCED_FACE ( 'NONE', ( #70904 ), #9634, .F. ) ;
#59674=ORIENTED_EDGE ( 'NONE', *, *, #79521, .F. ) ;
#59675=EDGE_LOOP ( 'NONE', ( #51562, #61842, #43913, #15966 ) ) ;
#59676=CARTESIAN_POINT ( 'NONE',  ( -9.019254006523732770, -12.43535235679832596, 30.55408501211184813 ) ) ;
#59677=CARTESIAN_POINT ( 'NONE',  ( 7.622668902429899696, -11.41268669641500466, 32.86336882939237825 ) ) ;
#59678=DIRECTION ( 'NONE',  ( -0.000000000000000000, -0.5000000000000009992, -0.8660254037844380415 ) ) ;
#59679=CARTESIAN_POINT ( 'NONE',  ( -5.076923076923199218, -10.33852847137269571, 34.16647553114546554 ) ) ;
#59680=EDGE_CURVE ( 'NONE', #11769, #17756, #60853, .T. ) ;
#59681=CARTESIAN_POINT ( 'NONE',  ( 14.08420738312797837, -3.562934362175799841, 33.22335522853832401 ) ) ;
#59682=CARTESIAN_POINT ( 'NONE',  ( -9.942330916529147800, -6.652501968072648708, 34.93155406624980941 ) ) ;
#59683=B_SPLINE_CURVE_WITH_KNOTS ( 'NONE', 3,
 ( #68138, #39788, #74449, #11418, #46964, #87099, #40231, #18628, #59599, #19501 ),
 .UNSPECIFIED., .F., .F.,
 ( 4, 2, 2, 2, 4 ),
 ( 0.000000000000000000, 0.0001954339857564079894, 0.0003908679715128159787, 0.0005863019572692239681, 0.0007817359430256319575 ),
 .UNSPECIFIED. ) ;
#59684=AXIS2_PLACEMENT_3D ( 'NONE', #13003, #26076, #39159 ) ;
#59685=EDGE_CURVE ( 'NONE', #86793, #1879, #51943, .T. ) ;
#59687=CARTESIAN_POINT ( 'NONE',  ( -4.826977558574935045, -12.43552623307873972, 30.55307653245132826 ) ) ;
#59688=ORIENTED_EDGE ( 'NONE', *, *, #15278, .F. ) ;
#59689=ADVANCED_FACE ( 'NONE', ( #64124 ), #38449, .F. ) ;
#59690=VERTEX_POINT ( 'NONE', #58262 ) ;
#59691=CARTESIAN_POINT ( 'NONE',  ( 7.715463243043540587, -10.70098750199973203, 33.91152734681376302 ) ) ;
#59693=CARTESIAN_POINT ( 'NONE',  ( 9.822833394071260216, -12.27024696741798770, 31.24895572276497546 ) ) ;
#59694=EDGE_CURVE ( 'NONE', #23339, #53520, #23143, .T. ) ;
#59695=VECTOR ( 'NONE', #72101, 1000.000000000000114 ) ;
#59696=CARTESIAN_POINT ( 'NONE',  ( 1.318533005255250412, -11.35647404775217595, 33.31231777344666511 ) ) ;
#59697=CARTESIAN_POINT ( 'NONE',  ( -13.25408968285182354, -3.285477652293413264, 32.44071101563363158 ) ) ;
#59698=EDGE_LOOP ( 'NONE', ( #62873, #85250 ) ) ;
#59699=ORIENTED_EDGE ( 'NONE', *, *, #21387, .F. ) ;
#59700=EDGE_LOOP ( 'NONE', ( #59723, #55846, #52443, #87614 ) ) ;
#59701=LINE ( 'NONE', #23246, #77452 ) ;
#59703=EDGE_CURVE ( 'NONE', #18976, #54695, #59683, .T. ) ;
#59704=DIRECTION ( 'NONE',  ( -0.000000000000000000, 0.8660254037844399289, -0.4999999999999980016 ) ) ;
#59706=EDGE_CURVE ( 'NONE', #29522, #5877, #82101, .T. ) ;
#59708=ORIENTED_EDGE ( 'NONE', *, *, #2273, .T. ) ;
#59709=ORIENTED_EDGE ( 'NONE', *, *, #41274, .F. ) ;
#59710=CARTESIAN_POINT ( 'NONE',  ( 0.5920641633020259365, -11.93748526763465279, 32.05452791011430946 ) ) ;
#59711=B_SPLINE_CURVE_WITH_KNOTS ( 'NONE', 3,
 ( #7320, #28028, #6867, #55495, #68134, #82549, #27583, #12741, #60923, #14512 ),
 .UNSPECIFIED., .F., .F.,
 ( 4, 2, 2, 2, 4 ),
 ( 0.000000000000000000, 0.0001954311564186858715, 0.0003908623128373717431, 0.0005862934692560576146, 0.0007817246256747434861 ),
 .UNSPECIFIED. ) ;
#59712=AXIS2_PLACEMENT_3D ( 'NONE', #21651, #76601, #14908 ) ;
#59713=FACE_OUTER_BOUND ( 'NONE', #59203, .T. ) ;
#59714=ORIENTED_EDGE ( 'NONE', *, *, #9949, .T. ) ;
#59715=CARTESIAN_POINT ( 'NONE',  ( 1.384615384615386802, -9.780366693483667717, 34.19971097300155094 ) ) ;
#59716=CARTESIAN_POINT ( 'NONE',  ( -2.057637887778853703, -4.074993327901525575, 33.72946981652012255 ) ) ;
#59717=B_SPLINE_CURVE_WITH_KNOTS ( 'NONE', 3,
 ( #59470, #79749, #31553, #39664, #67568, #18933, #72985, #88309, #86975, #66673 ),
 .UNSPECIFIED., .F., .F.,
 ( 4, 2, 2, 2, 4 ),
 ( 0.000000000000000000, 0.0001954311564186878502, 0.0003908623128373757004, 0.0005862934692560635777, 0.0007817246256747514008 ),
 .UNSPECIFIED. ) ;
#59718=B_SPLINE_CURVE_WITH_KNOTS ( 'NONE', 3,
 ( #79269, #43697, #29753, #57659, #51306, #9042, #36511, #38279, #77488, #84710 ),
 .UNSPECIFIED., .F., .F.,
 ( 4, 2, 2, 2, 4 ),
 ( 0.0007817246256747442451, 0.0009771112852218865989, 0.001172497944769029061, 0.001367884604316171523, 0.001563271263863313986 ),
 .UNSPECIFIED. ) ;
#59720=DIRECTION ( 'NONE',  ( -0.000000000000000000, -0.000000000000000000, -1.000000000000000000 ) ) ;
#59721=ORIENTED_EDGE ( 'NONE', *, *, #17567, .F. ) ;
#59722=CARTESIAN_POINT ( 'NONE',  ( -14.53117723225664015, -12.47654668319379567, 31.42292124445336654 ) ) ;
#59723=ORIENTED_EDGE ( 'NONE', *, *, #51580, .T. ) ;
#59726=DIRECTION ( 'NONE',  ( -0.000000000000000000, -0.8660254037844397068, -0.4999999999999978906 ) ) ;
#59727=FACE_BOUND ( 'NONE', #27035, .T. ) ;
#59731=DIRECTION ( 'NONE',  ( 0.000000000000000000, 0.8660254037844377084, 0.5000000000000015543 ) ) ;
#59732=ORIENTED_EDGE ( 'NONE', *, *, #67361, .F. ) ;
#59735=FACE_OUTER_BOUND ( 'NONE', #74536, .T. ) ;
#59736=VERTEX_POINT ( 'NONE', #73581 ) ;
#59737=ADVANCED_FACE ( 'NONE', ( #11873 ), #6003, .F. ) ;
#59738=CARTESIAN_POINT ( 'NONE',  ( 17.07692307692307665, -12.10708131394839349, 31.69288490824020244 ) ) ;
#59739=CARTESIAN_POINT ( 'NONE',  ( 10.39245765647776665, -8.282780595021769443, 34.94152052738834868 ) ) ;
#59740=CARTESIAN_POINT ( 'NONE',  ( 16.82692307692307665, -7.500000000000001776, 34.75000000000000000 ) ) ;
#59741=CARTESIAN_POINT ( 'NONE',  ( 10.61538461538461675, -11.69971097300155272, 32.46337939537588113 ) ) ;
#59742=AXIS2_PLACEMENT_3D ( 'NONE', #77466, #920, #28387 ) ;
#59743=FACE_BOUND ( 'NONE', #43706, .T. ) ;
#59744=CARTESIAN_POINT ( 'NONE',  ( -7.053224892808621860, -12.50552854090298993, 31.33409797877408920 ) ) ;
#59746=CARTESIAN_POINT ( 'NONE',  ( 3.230769230769108269, -12.16647553114689728, 32.15551576947799362 ) ) ;
#59747=CARTESIAN_POINT ( 'NONE',  ( -11.76134022089018671, -7.630691491037285168, 34.74850469731152458 ) ) ;
#59748=CARTESIAN_POINT ( 'NONE',  ( -11.31568186948346977, -10.97394488606064122, 33.68653795673694873 ) ) ;
#59749=CARTESIAN_POINT ( 'NONE',  ( -4.023055712879203938, -10.70102852606553157, 33.91149625220312913 ) ) ;
#59750=CARTESIAN_POINT ( 'NONE',  ( -8.546451227962355901, -3.755027918224367323, 33.06320215134714857 ) ) ;
#59752=CARTESIAN_POINT ( 'NONE',  ( -6.989160334032801458, -8.973038597847269315, 34.52809138561120506 ) ) ;
#59753=ORIENTED_EDGE ( 'NONE', *, *, #43966, .F. ) ;
#59754=DIRECTION ( 'NONE',  ( 0.000000000000000000, 0.000000000000000000, 1.000000000000000000 ) ) ;
#59755=CYLINDRICAL_SURFACE ( 'NONE', #34074, 0.2500000000000004996 ) ;
#59756=CARTESIAN_POINT ( 'NONE',  ( -1.253823576790597860, -10.54018710029568595, 33.71981072465678864 ) ) ;
#59758=AXIS2_PLACEMENT_3D ( 'NONE', #74687, #87778, #13415 ) ;
#59759=CARTESIAN_POINT ( 'NONE',  ( 16.85343815235874132, -12.69144148231606017, 30.53333754910549303 ) ) ;
#59760=DIRECTION ( 'NONE',  ( 0.000000000000000000, 0.3420201433256641055, -0.9396926207859100932 ) ) ;
#59762=EDGE_CURVE ( 'NONE', #66117, #72102, #13474, .T. ) ;
#59763=CARTESIAN_POINT ( 'NONE',  ( 15.16468685140909400, -11.91647553114624181, 32.58852847137148245 ) ) ;
#59764=DIRECTION ( 'NONE',  ( -0.000000000000000000, -0.6427876096865404731, -0.7660444431189770143 ) ) ;
#59765=CARTESIAN_POINT ( 'NONE',  ( -12.39628332202562433, -9.528491918058460186, 34.59228464037086326 ) ) ;
#59766=CARTESIAN_POINT ( 'NONE',  ( 4.853438152358744873, -9.417330523894424488, 34.63758898049880486 ) ) ;
#59767=LINE ( 'NONE', #66068, #46855 ) ;
#59768=CARTESIAN_POINT ( 'NONE',  ( 9.442330948259101575, -3.436278759898153901, 33.07459398097509506 ) ) ;
#59769=FACE_OUTER_BOUND ( 'NONE', #55515, .T. ) ;
#59770=CARTESIAN_POINT ( 'NONE',  ( 7.911408985666682270, -9.528491918058460186, 34.59228464037086326 ) ) ;
#59771=ORIENTED_EDGE ( 'NONE', *, *, #13576, .T. ) ;
#59772=CARTESIAN_POINT ( 'NONE',  ( 6.673076923076926015, -7.566082377512563184, 35.00000000000000711 ) ) ;
#59773=CARTESIAN_POINT ( 'NONE',  ( 9.019285080869082094, -11.28795663066794575, 33.01431243580653785 ) ) ;
#59775=CARTESIAN_POINT ( 'NONE',  ( -10.68146699474474914, -9.905515769479276145, 34.41647553114623292 ) ) ;
#59776=CARTESIAN_POINT ( 'NONE',  ( -16.40386937806761836, -10.92453946501458439, 33.72985991061850086 ) ) ;
#59778=VECTOR ( 'NONE', #42927, 999.9999999999998863 ) ;
#59780=CARTESIAN_POINT ( 'NONE',  ( -12.33074802057151409, -12.62708834333097663, 30.88030960425257021 ) ) ;
#59781=CARTESIAN_POINT ( 'NONE',  ( 11.53846153846185274, -2.255955759149395501, 30.00000000000324363 ) ) ;
#59782=ORIENTED_EDGE ( 'NONE', *, *, #45977, .T. ) ;
#59783=CARTESIAN_POINT ( 'NONE',  ( -9.758390071667827570, -11.35647404775217595, 33.31231777344666511 ) ) ;
#59784=CARTESIAN_POINT ( 'NONE',  ( -2.242547526972674010, -7.750023224968865421, 34.99404313364389907 ) ) ;
#59785=CARTESIAN_POINT ( 'NONE',  ( -8.638438961405986660, -2.541949514083464479, 30.39797389878540557 ) ) ;
#59787=CARTESIAN_POINT ( 'NONE',  ( -11.53846153846166089, -2.657715359629662544, 31.77849191805970364 ) ) ;
#59788=ORIENTED_EDGE ( 'NONE', *, *, #19763, .F. ) ;
#59790=DIRECTION ( 'NONE',  ( -0.000000000000000000, 1.000000000000000000, 3.491481338843133355E-15 ) ) ;
#59792=CARTESIAN_POINT ( 'NONE',  ( 8.546303810323914618, -3.395401636524185474, 33.02366814457250399 ) ) ;
#59793=ORIENTED_EDGE ( 'NONE', *, *, #24851, .F. ) ;
#59794=EDGE_LOOP ( 'NONE', ( #55044, #6099, #73947, #61039 ) ) ;
#59795=EDGE_CURVE ( 'NONE', #19537, #73867, #25824, .T. ) ;
#59796=VERTEX_POINT ( 'NONE', #67254 ) ;
#59797=CARTESIAN_POINT ( 'NONE',  ( 5.142991427925514003, -12.10708131394839882, 31.69288490824020954 ) ) ;
#59798=CARTESIAN_POINT ( 'NONE',  ( 0.3313912521002409517, -2.619462340734462380, 30.83744416345203021 ) ) ;
#59799=ADVANCED_FACE ( 'NONE', ( #46536 ), #66361, .F. ) ;
#59800=CARTESIAN_POINT ( 'NONE',  ( -12.71156169883142617, -3.711651800289232028, 33.01384336483936011 ) ) ;
#59801=EDGE_CURVE ( 'NONE', #39037, #49681, #34998, .T. ) ;
#59802=CARTESIAN_POINT ( 'NONE',  ( -18.22520792652332844, -7.371819721847150397, 34.99865929289143196 ) ) ;
#59803=EDGE_LOOP ( 'NONE', ( #29732, #41625, #6107, #64981 ) ) ;
#59804=VECTOR ( 'NONE', #3361, 1000.000000000000227 ) ;
#59805=VERTEX_POINT ( 'NONE', #81658 ) ;
#59806=EDGE_LOOP ( 'NONE', ( #79673, #50259 ) ) ;
#59807=DIRECTION ( 'NONE',  ( 0.000000000000000000, 0.000000000000000000, 1.000000000000000000 ) ) ;
#59808=ORIENTED_EDGE ( 'NONE', *, *, #10639, .F. ) ;
#59809=CARTESIAN_POINT ( 'NONE',  ( -5.207071046654776048, -2.647304123082328875, 31.75400227202885262 ) ) ;
#59810=EDGE_CURVE ( 'NONE', #31984, #69894, #55371, .T. ) ;
#59811=CARTESIAN_POINT ( 'NONE',  ( -3.296039231325550212, -5.094484230520674117, 34.41647553114621161 ) ) ;
#59812=CARTESIAN_POINT ( 'NONE',  ( 1.515407192440172413, -10.54018710029568595, 33.71981072465678864 ) ) ;
#59813=CARTESIAN_POINT ( 'NONE',  ( -13.16160403300253634, -12.39991518177334129, 30.74647679643404530 ) ) ;
#59815=ORIENTED_EDGE ( 'NONE', *, *, #52723, .F. ) ;
#59816=VERTEX_POINT ( 'NONE', #68575 ) ;
#59817=EDGE_LOOP ( 'NONE', ( #38302, #44135 ) ) ;
#59818=CARTESIAN_POINT ( 'NONE',  ( -5.011777297591113012, -7.750023238201980469, 34.74374492549440419 ) ) ;
#59820=ORIENTED_EDGE ( 'NONE', *, *, #82307, .F. ) ;
#59821=CARTESIAN_POINT ( 'NONE',  ( 3.007284287045282500, -11.89387501736622710, 32.13663884655806413 ) ) ;
#59823=CARTESIAN_POINT ( 'NONE',  ( 16.28437185560972011, -8.586989748646450593, 34.63063291749215011 ) ) ;
#59824=CARTESIAN_POINT ( 'NONE',  ( -13.38461538461507594, -2.506253911140614576, 30.00000000000323297 ) ) ;
#59826=FACE_BOUND ( 'NONE', #67990, .T. ) ;
#59827=EDGE_CURVE ( 'NONE', #74119, #87173, #61743, .T. ) ;
#59828=DIRECTION ( 'NONE',  ( -0.000000000000000000, 0.3420201433256694901, -0.9396926207859082059 ) ) ;
#59829=CARTESIAN_POINT ( 'NONE',  ( 8.769230769230768274, -2.708943851104267164, 35.45975837776705220 ) ) ;
#59830=DIRECTION ( 'NONE',  ( -0.000000000000000000, 1.000000000000000000, 3.491481338843133355E-15 ) ) ;
#59831=CARTESIAN_POINT ( 'NONE',  ( 9.692307692307572609, -3.300289026999228881, 32.46337939537708905 ) ) ;
#59832=CARTESIAN_POINT ( 'NONE',  ( -5.142193522883852452, -3.300289026998414865, 32.46337939537583139 ) ) ;
#59834=VECTOR ( 'NONE', #50567, 1000.000000000000000 ) ;
#59836=CARTESIAN_POINT ( 'NONE',  ( 1.515140822849031954, -2.372941743896878286, 30.88044141588254377 ) ) ;
#59837=ORIENTED_EDGE ( 'NONE', *, *, #48131, .T. ) ;
#59838=CARTESIAN_POINT ( 'NONE',  ( -15.16551409125639260, -11.67786785259547777, 32.92929555188713664 ) ) ;
#59839=DIRECTION ( 'NONE',  ( 0.000000000000000000, 0.8660254037844377084, -0.5000000000000015543 ) ) ;
#59841=EDGE_LOOP ( 'NONE', ( #48111, #7583 ) ) ;
#59843=CARTESIAN_POINT ( 'NONE',  ( -17.32694631421604115, -11.37209801155882793, 32.91403422569033665 ) ) ;
#59844=EDGE_CURVE ( 'NONE', #61826, #313, #67193, .T. ) ;
#59845=CARTESIAN_POINT ( 'NONE',  ( -14.43838377435986864, -4.809359713505814149, 33.96456829005828837 ) ) ;
#59846=CARTESIAN_POINT ( 'NONE',  ( -11.53846153846153655, -5.415277668671390821, 36.20867863119892149 ) ) ;
#59847=ORIENTED_EDGE ( 'NONE', *, *, #20634, .F. ) ;
#59848=CYLINDRICAL_SURFACE ( 'NONE', #74504, 0.2499999999999998890 ) ;
#59849=CARTESIAN_POINT ( 'NONE',  ( -6.923076923076922462, -9.780366693483667717, 34.19971097300155094 ) ) ;
#59852=DIRECTION ( 'NONE',  ( 0.000000000000000000, 0.3420201433256610524, 0.9396926207859113145 ) ) ;
#59853=CARTESIAN_POINT ( 'NONE',  ( -12.68446467905460828, -4.887634598454295265, 34.01352882383564946 ) ) ;
#59854=B_SPLINE_CURVE_WITH_KNOTS ( 'NONE', 3,
 ( #75472, #13330, #66504, #39932, #87681, #40812, #60622, #59744, #88135, #20529 ),
 .UNSPECIFIED., .F., .F.,
 ( 4, 2, 2, 2, 4 ),
 ( 0.000000000000000000, 0.0001954311564186879857, 0.0003908623128373759715, 0.0005862934692560640114, 0.0007817246256747519429 ),
 .UNSPECIFIED. ) ;
#59855=CARTESIAN_POINT ( 'NONE',  ( 0.5267936010512997980, -5.094484230520773593, 34.41647553114626845 ) ) ;
#59856=CARTESIAN_POINT ( 'NONE',  ( -15.16470189741915675, -10.67929555188718282, 33.92786785259544757 ) ) ;
#59858=ORIENTED_EDGE ( 'NONE', *, *, #77924, .T. ) ;
#59859=VERTEX_POINT ( 'NONE', #50393 ) ;
#59861=CARTESIAN_POINT ( 'NONE',  ( 7.173131234715240723, -12.17597550085003633, 31.52189283813461884 ) ) ;
#59862=CARTESIAN_POINT ( 'NONE',  ( 16.40390057375960708, -2.920487667080175154, 32.31805714834170828 ) ) ;
#59863=CARTESIAN_POINT ( 'NONE',  ( -0.5920151696549253995, -7.276988635370452485, 34.74523720219453793 ) ) ;
#59864=LINE ( 'NONE', #34167, #48587 ) ;
#59866=EDGE_CURVE ( 'NONE', #35777, #45661, #26347, .T. ) ;
#59867=CARTESIAN_POINT ( 'NONE',  ( 0.7115384615383971711, -7.565270445406050648, 34.75000000000000000 ) ) ;
#59868=DIRECTION ( 'NONE',  ( -0.000000000000000000, 0.9848077530122086864, -0.1736481776669273891 ) ) ;
#59869=CARTESIAN_POINT ( 'NONE',  ( -13.45037218712969462, -7.249945686854186278, 34.74374336980224598 ) ) ;
#59870=CARTESIAN_POINT ( 'NONE',  ( 12.39626846098214052, -11.67786785259540849, 32.92929555188721480 ) ) ;
#59871=CARTESIAN_POINT ( 'NONE',  ( -6.222926217516145719, -2.758268499246657957, 31.33685645148948140 ) ) ;
#59872=CARTESIAN_POINT ( 'NONE',  ( 13.60739505359344825, -2.612705202774698421, 31.66806509827799943 ) ) ;
#59874=EDGE_CURVE ( 'NONE', #26509, #79445, #44073, .T. ) ;
#59875=CARTESIAN_POINT ( 'NONE',  ( 2.084766090176159992, -3.105860786376062332, 32.13614157043598851 ) ) ;
#59876=CARTESIAN_POINT ( 'NONE',  ( -9.692307692307691624, -3.322132147404559976, 32.92929555188717927 ) ) ;
#59877=VECTOR ( 'NONE', #35367, 1000.000000000000114 ) ;
#59878=CARTESIAN_POINT ( 'NONE',  ( 15.23076923076954614, -2.255955759149395501, 30.00000000000324363 ) ) ;
#59879=CARTESIAN_POINT ( 'NONE',  ( -7.846153846153965716, -12.46129190930018460, 30.37095296980731973 ) ) ;
#59880=VERTEX_POINT ( 'NONE', #85087 ) ;
#59882=CARTESIAN_POINT ( 'NONE',  ( 2.307692307692309264, -2.900454961884010974, 35.62045528018868623 ) ) ;
#59883=CARTESIAN_POINT ( 'NONE',  ( 18.13079044096694759, -4.684288915650984819, 34.18129842949671371 ) ) ;
#59886=DIRECTION ( 'NONE',  ( 0.000000000000000000, 0.9396926207859126468, 0.3420201433256571111 ) ) ;
#59887=CARTESIAN_POINT ( 'NONE',  ( -39.05038313613820122, -2.499999999999999556, 29.75000000000000355 ) ) ;
#59888=VERTEX_POINT ( 'NONE', #84215 ) ;
#59890=FACE_OUTER_BOUND ( 'NONE', #52905, .T. ) ;
#59891=B_SPLINE_CURVE_WITH_KNOTS ( 'NONE', 3,
 ( #71679, #9980, #50946, #31588, #58606, #9536, #64916, #23930, #37002, #65804 ),
 .UNSPECIFIED., .F., .F.,
 ( 4, 2, 2, 2, 4 ),
 ( 0.000000000000000000, 0.0001954339857564080165, 0.0003908679715128160329, 0.0005863019572692240765, 0.0007817359430256320659 ),
 .UNSPECIFIED. ) ;
#59892=VECTOR ( 'NONE', #18479, 1000.000000000000000 ) ;
#59893=EDGE_LOOP ( 'NONE', ( #9217, #68193, #76684, #56570 ) ) ;
#59894=CARTESIAN_POINT ( 'NONE',  ( -9.692307692307691624, -13.57706302396349152, 30.56769352161908060 ) ) ;
#59896=DIRECTION ( 'NONE',  ( 0.000000000000000000, 0.1736481776669267785, -0.9848077530122087975 ) ) ;
#59897=CARTESIAN_POINT ( 'NONE',  ( 13.38461538461526601, -10.21337939537710326, 33.94971097300076224 ) ) ;
#59898=LINE ( 'NONE', #86046, #67154 ) ;
#59899=VERTEX_POINT ( 'NONE', #71553 ) ;
#59900=CARTESIAN_POINT ( 'NONE',  ( -10.36543909703647159, -12.43552623307873972, 30.55307653245132826 ) ) ;
#59902=EDGE_CURVE ( 'NONE', #22022, #66369, #87622, .T. ) ;
#59903=ORIENTED_EDGE ( 'NONE', *, *, #69002, .F. ) ;
#59904=DIRECTION ( 'NONE',  ( -0.000000000000000000, 0.5000000000000011102, -0.8660254037844380415 ) ) ;
#59905=DIRECTION ( 'NONE',  ( 0.000000000000000000, 0.1736481776669267785, -0.9848077530122087975 ) ) ;
#59906=CYLINDRICAL_SURFACE ( 'NONE', #63004, 0.2499999999999994726 ) ;
#59907=CARTESIAN_POINT ( 'NONE',  ( 9.562160482869472844, -9.418419913701741919, 34.36755862841477693 ) ) ;
#59908=CARTESIAN_POINT ( 'NONE',  ( -2.980823821391187955, -4.932303261841488151, 34.32971442181322885 ) ) ;
#59911=EDGE_CURVE ( 'NONE', #8847, #34885, #2209, .T. ) ;
#59912=FACE_OUTER_BOUND ( 'NONE', #36229, .T. ) ;
#59913=EDGE_LOOP ( 'NONE', ( #46794, #52147, #31328, #17154 ) ) ;
#59916=CARTESIAN_POINT ( 'NONE',  ( -4.023320715612507925, -8.630441415882550871, 34.87705825610312615 ) ) ;
#59918=EDGE_CURVE ( 'NONE', #53138, #22316, #79658, .T. ) ;
#59919=B_SPLINE_CURVE_WITH_KNOTS ( 'NONE', 3,
 ( #23107, #37051, #37495, #2816, #30740, #30308, #58210, #85701, #23977, #17232 ),
 .UNSPECIFIED., .F., .F.,
 ( 4, 2, 2, 2, 4 ),
 ( 0.000000000000000000, 0.0001954339857564081249, 0.0003908679715128162498, 0.0005863019572692244018, 0.0007817359430256324996 ),
 .UNSPECIFIED. ) ;
#59920=FACE_OUTER_BOUND ( 'NONE', #82703, .T. ) ;
#59921=CARTESIAN_POINT ( 'NONE',  ( 3.230769230769231726, -11.33034616979429110, 35.88435417666054406 ) ) ;
#59922=EDGE_LOOP ( 'NONE', ( #86664, #40879, #9155, #87102 ) ) ;
#59923=CARTESIAN_POINT ( 'NONE',  ( -14.24162395668986925, -4.098570777380720287, 33.41473453929635440 ) ) ;
#59925=EDGE_LOOP ( 'NONE', ( #72928, #51243 ) ) ;
#59926=CARTESIAN_POINT ( 'NONE',  ( 0.2386730393348221735, -2.501496062324912284, 29.88072118266895671 ) ) ;
#59927=ORIENTED_EDGE ( 'NONE', *, *, #68323, .T. ) ;
#59928=DIRECTION ( 'NONE',  ( -0.000000000000000000, -0.000000000000000000, -1.000000000000000000 ) ) ;
#59929=AXIS2_PLACEMENT_3D ( 'NONE', #62405, #74613, #21435 ) ;
#59930=CARTESIAN_POINT ( 'NONE',  ( -11.78843826940389583, -3.627789207965226748, 32.91389620160131102 ) ) ;
#59931=CARTESIAN_POINT ( 'NONE',  ( 4.023286240232789801, -2.254533558242299396, 29.97296025877828285 ) ) ;
#59932=FACE_BOUND ( 'NONE', #15335, .T. ) ;
#59933=EDGE_CURVE ( 'NONE', #45617, #31900, #73345, .T. ) ;
#59934=CARTESIAN_POINT ( 'NONE',  ( -17.07692307692307665, -11.35647404775217417, 33.31231777344666511 ) ) ;
#59935=CARTESIAN_POINT ( 'NONE',  ( -13.38461538461538325, -2.900454961884010974, 35.62045528018868623 ) ) ;
#59936=CARTESIAN_POINT ( 'NONE',  ( 5.869439408258079638, -2.504760397472873823, 29.97295953869789997 ) ) ;
#59937=FACE_OUTER_BOUND ( 'NONE', #43443, .T. ) ;
#59938=CARTESIAN_POINT ( 'NONE',  ( 24.00000000000000000, -5.499999999999981348, 27.75000000000000000 ) ) ;
#59939=CARTESIAN_POINT ( 'NONE',  ( 8.096099364501986528, -10.76462480002816235, 33.53768742498949962 ) ) ;
#59940=ORIENTED_EDGE ( 'NONE', *, *, #54085, .F. ) ;
#59942=CIRCLE ( 'NONE', #44108, 0.2500000000000002220 ) ;
#59943=CARTESIAN_POINT ( 'NONE',  ( 10.61538461538461675, -9.780366693483667717, 34.19971097300155094 ) ) ;
#59944=EDGE_LOOP ( 'NONE', ( #53763, #55114, #31701, #59940 ) ) ;
#59945=ORIENTED_EDGE ( 'NONE', *, *, #43455, .T. ) ;
#59946=CARTESIAN_POINT ( 'NONE',  ( 10.83839596699746721, -12.39991518177334129, 30.74647679643404530 ) ) ;
#59947=CARTESIAN_POINT ( 'NONE',  ( 2.307692307692187583, -10.90142922262034020, 33.41473453929536674 ) ) ;
#59948=CARTESIAN_POINT ( 'NONE',  ( 15.23076923076910916, -8.656820664282941280, 34.87096338111179961 ) ) ;
#59949=LINE ( 'NONE', #82459, #1990 ) ;
#59950=CARTESIAN_POINT ( 'NONE',  ( 13.38461538461538680, -13.78497067705608181, 32.30358669280327177 ) ) ;
#59951=CARTESIAN_POINT ( 'NONE',  ( 1.449870524128224591, -4.320704448112861584, 33.92786785259548310 ) ) ;
#59952=ORIENTED_EDGE ( 'NONE', *, *, #74524, .F. ) ;
#59953=CARTESIAN_POINT ( 'NONE',  ( -5.207071046654771607, -5.915902021225892149, 34.75552854090298638 ) ) ;
#59954=ADVANCED_FACE ( 'NONE', ( #67037 ), #24248, .F. ) ;
#59955=CARTESIAN_POINT ( 'NONE',  ( -5.076923076923075762, -2.538708090699994813, 30.37095296980875503 ) ) ;
#59956=CARTESIAN_POINT ( 'NONE',  ( -14.05769230769229772, -2.249999999999999112, 29.81603969181032099 ) ) ;
#59957=LINE ( 'NONE', #13548, #53952 ) ;
#59958=VERTEX_POINT ( 'NONE', #38667 ) ;
#59959=B_SPLINE_CURVE_WITH_KNOTS ( 'NONE', 3,
 ( #67218, #19026, #26225, #38406, #65862, #12711, #31650, #39752, #25334, #59112 ),
 .UNSPECIFIED., .F., .F.,
 ( 4, 2, 2, 2, 4 ),
 ( 0.000000000000000000, 0.0001954339857564098054, 0.0003908679715128196108, 0.0005863019572692293891, 0.0007817359430256392216 ),
 .UNSPECIFIED. ) ;
#59960=ORIENTED_EDGE ( 'NONE', *, *, #57571, .T. ) ;
#59962=EDGE_LOOP ( 'NONE', ( #47566, #41774 ) ) ;
#59963=CARTESIAN_POINT ( 'NONE',  ( 15.45354877203763522, -6.760870238392817200, 34.69528174975672385 ) ) ;
#59964=CARTESIAN_POINT ( 'NONE',  ( -7.596099534515531104, -4.943051570960392382, 34.04725096376909477 ) ) ;
#59965=ORIENTED_EDGE ( 'NONE', *, *, #86772, .F. ) ;
#59966=DIRECTION ( 'NONE',  ( -0.000000000000000000, -0.7660444431189791237, -0.6427876096865379196 ) ) ;
#59967=CARTESIAN_POINT ( 'NONE',  ( -6.000000000000121680, -9.528491918059723176, 34.59228464037033035 ) ) ;
#59968=CARTESIAN_POINT ( 'NONE',  ( 16.08776274289027342, -8.120952969808774569, 34.71129190930000163 ) ) ;
#59969=CARTESIAN_POINT ( 'NONE',  ( -2.557669038634660996, -8.303909089506435137, 34.68538101551103381 ) ) ;
#59970=ADVANCED_FACE ( 'NONE', ( #44964 ), #66130, .T. ) ;
#59971=AXIS2_PLACEMENT_3D ( 'NONE', #15011, #56868, #76709 ) ;
#59972=CARTESIAN_POINT ( 'NONE',  ( 5.076923076923075762, -13.87047571288749737, 32.06866353760679544 ) ) ;
#59973=ORIENTED_EDGE ( 'NONE', *, *, #26120, .F. ) ;
#59974=CARTESIAN_POINT ( 'NONE',  ( -7.780898274877820597, -10.21337939537593620, 33.94971097300152252 ) ) ;
#59975=ORIENTED_EDGE ( 'NONE', *, *, #35675, .T. ) ;
#59976=CYLINDRICAL_SURFACE ( 'NONE', #82847, 0.2499999999999997502 ) ;
#59977=CARTESIAN_POINT ( 'NONE',  ( 16.08859516368491072, -2.506253911140460477, 30.00000000000013856 ) ) ;
#59978=CARTESIAN_POINT ( 'NONE',  ( -11.76194646302586833, -10.97335522853832579, 33.68706563782419749 ) ) ;
#59979=ADVANCED_FACE ( 'NONE', ( #53056 ), #80101, .F. ) ;
#59980=EDGE_CURVE ( 'NONE', #7315, #75299, #30642, .T. ) ;
#59981=CARTESIAN_POINT ( 'NONE',  ( 10.39189969082028497, -12.47654668319379567, 31.42292124445336654 ) ) ;
#59982=CARTESIAN_POINT ( 'NONE',  ( -13.38461538461538325, -5.557115091759785130, 34.35708131394839171 ) ) ;
#59984=CARTESIAN_POINT ( 'NONE',  ( -5.207071046654775159, -11.04286588640298561, 33.62463336215343901 ) ) ;
#59987=VERTEX_POINT ( 'NONE', #85526 ) ;
#59988=CARTESIAN_POINT ( 'NONE',  ( 11.60452988946397923, -2.721908614388771852, 31.22303859784725333 ) ) ;
#59990=EDGE_LOOP ( 'NONE', ( #41060, #83508, #76528, #75568 ) ) ;
#59991=ORIENTED_EDGE ( 'NONE', *, *, #65701, .T. ) ;
#59992=CARTESIAN_POINT ( 'NONE',  ( -5.750054590621955342, -12.68172785388650681, 30.59649109432439573 ) ) ;
#59993=CARTESIAN_POINT ( 'NONE',  ( -3.007989689500822017, -5.913360116392399668, 34.49180327182771322 ) ) ;
#59994=CARTESIAN_POINT ( 'NONE',  ( -0.2115384615384583999, -2.499999999999999556, 29.81604066197450109 ) ) ;
#59995=B_SPLINE_CURVE_WITH_KNOTS ( 'NONE', 3,
 ( #57946, #85426, #23707, #52516, #32265, #67820, #33143, #46215, #45768, #66933 ),
 .UNSPECIFIED., .F., .F.,
 ( 4, 2, 2, 2, 4 ),
 ( 0.0007817359430256322827, 0.0009771253907249989254, 0.001172514838424365676, 0.001367904286123732428, 0.001563293733823098962 ),
 .UNSPECIFIED. ) ;
#59996=CARTESIAN_POINT ( 'NONE',  ( 10.83816428436268176, -4.989023458446560255, 34.36081565061822118 ) ) ;
#59997=B_SPLINE_CURVE_WITH_KNOTS ( 'NONE', 3,
 ( #79346, #37458, #17650, #65814, #4114, #52751, #85220, #31599, #59066, #64927 ),
 .UNSPECIFIED., .F., .F.,
 ( 4, 2, 2, 2, 4 ),
 ( 0.0007817359430256388964, 0.0009771253907250073822, 0.001172514838424375868, 0.001367904286123744571, 0.001563293733823113056 ),
 .UNSPECIFIED. ) ;
#59999=LINE ( 'NONE', #25777, #82536 ) ;
#60000=ORIENTED_EDGE ( 'NONE', *, *, #9547, .T. ) ;
#60001=AXIS2_PLACEMENT_3D ( 'NONE', #88394, #26667, #88837 ) ;
#60002=DIRECTION ( 'NONE',  ( 0.000000000000000000, 0.1736481776669275834, 0.9848077530122086864 ) ) ;
#60004=CARTESIAN_POINT ( 'NONE',  ( 5.076923076923075762, -11.33034616979429110, 35.88435417666054406 ) ) ;
#60005=ORIENTED_EDGE ( 'NONE', *, *, #81286, .F. ) ;
#60006=CARTESIAN_POINT ( 'NONE',  ( 12.52760681254089903, -3.513871655860379306, 32.76840700105978499 ) ) ;
#60007=VECTOR ( 'NONE', #27236, 1000.000000000000114 ) ;
#60008=EDGE_LOOP ( 'NONE', ( #23117, #65746 ) ) ;
#60010=CARTESIAN_POINT ( 'NONE',  ( -13.13461538461544542, -7.565270000091922853, 34.99999999999999289 ) ) ;
#60011=CARTESIAN_POINT ( 'NONE',  ( 18.00000000000000000, -1.129524287112498415, 32.06866353760679544 ) ) ;
#60012=ORIENTED_EDGE ( 'NONE', *, *, #16208, .T. ) ;
#60014=CARTESIAN_POINT ( 'NONE',  ( 12.23805351781451201, -3.754499324213721234, 33.06261337010820256 ) ) ;
#60015=CARTESIAN_POINT ( 'NONE',  ( -6.250023224221455287, -2.341070481393820124, 30.72580821765574299 ) ) ;
#60016=CARTESIAN_POINT ( 'NONE',  ( -9.822999158975251888, -2.541943142973491554, 30.39792223712631980 ) ) ;
#60017=CARTESIAN_POINT ( 'NONE',  ( -7.623141002060451754, -4.762714258010881885, 34.23016756924214832 ) ) ;
#60019=ORIENTED_EDGE ( 'NONE', *, *, #1432, .T. ) ;
#60020=FACE_BOUND ( 'NONE', #67747, .T. ) ;
#60021=EDGE_LOOP ( 'NONE', ( #22747, #31582, #77510, #55998 ) ) ;
#60022=CARTESIAN_POINT ( 'NONE',  ( -2.307692307692305711, -2.486705287966279876, 31.30864560766543647 ) ) ;
#60023=CARTESIAN_POINT ( 'NONE',  ( 9.692307692307695177, -5.180354513474913603, 36.12317359536750416 ) ) ;
#60024=CARTESIAN_POINT ( 'NONE',  ( -3.361379590393758221, -7.722926236386453702, 34.74524107206102030 ) ) ;
#60025=CIRCLE ( 'NONE', #18305, 0.2500000000000002220 ) ;
#60027=CARTESIAN_POINT ( 'NONE',  ( 8.992242120843616959, -3.587049720035815348, 32.86302985866382897 ) ) ;
#60028=LINE ( 'NONE', #17723, #17749 ) ;
#60030=ORIENTED_EDGE ( 'NONE', *, *, #82981, .T. ) ;
#60031=ORIENTED_EDGE ( 'NONE', *, *, #80880, .T. ) ;
#60032=EDGE_LOOP ( 'NONE', ( #39195, #23322, #84292, #865 ) ) ;
#60035=CARTESIAN_POINT ( 'NONE',  ( -10.55012904410859242, -11.48612834413965977, 32.76840700105972815 ) ) ;
#60036=CARTESIAN_POINT ( 'NONE',  ( -1.384615384615505151, -12.46129190930018460, 30.37095296980731973 ) ) ;
#60037=CARTESIAN_POINT ( 'NONE',  ( -3.931066612577743147, -9.332535724633407526, 34.40230450496446224 ) ) ;
#60038=CARTESIAN_POINT ( 'NONE',  ( 3.903869422903800679, -3.137211980971221781, 32.19342716148376837 ) ) ;
#60039=FACE_OUTER_BOUND ( 'NONE', #19747, .T. ) ;
#60040=EDGE_CURVE ( 'NONE', #21841, #18937, #39579, .T. ) ;
#60042=CARTESIAN_POINT ( 'NONE',  ( -2.057746789344164107, -3.712312575010499938, 33.01462480002815170 ) ) ;
#60043=FACE_OUTER_BOUND ( 'NONE', #61837, .T. ) ;
#60044=VERTEX_POINT ( 'NONE', #37775 ) ;
#60046=VERTEX_POINT ( 'NONE', #23802 ) ;
#60047=CARTESIAN_POINT ( 'NONE',  ( -15.23076923076922995, -9.058645607665452459, 34.76329471203371924 ) ) ;
#60048=VERTEX_POINT ( 'NONE', #3539 ) ;
#60049=B_SPLINE_CURVE_WITH_KNOTS ( 'NONE', 3,
 ( #5304, #46731, #74207, #50252, #28680, #76865, #41753, #8404, #62012, #8853 ),
 .UNSPECIFIED., .F., .F.,
 ( 4, 2, 2, 2, 4 ),
 ( 0.0007817359430256303312, 0.0009771253907249965402, 0.001172514838424362641, 0.001367904286123728958, 0.001563293733823095059 ),
 .UNSPECIFIED. ) ;
#60050=CARTESIAN_POINT ( 'NONE',  ( 7.596177115211491859, -3.137211980971221781, 32.19342716148376837 ) ) ;
#60052=CARTESIAN_POINT ( 'NONE',  ( 6.000000000000001776, -5.415277668671390821, 36.20867863119892149 ) ) ;
#60053=CARTESIAN_POINT ( 'NONE',  ( -8.769230769230768274, -6.343179335718451384, 34.87096338111211935 ) ) ;
#60054=FACE_BOUND ( 'NONE', #17765, .T. ) ;
#60056=EDGE_CURVE ( 'NONE', #22892, #60384, #10230, .T. ) ;
#60057=ORIENTED_EDGE ( 'NONE', *, *, #82400, .F. ) ;
#60059=VECTOR ( 'NONE', #55500, 1000.000000000000114 ) ;
#60060=VERTEX_POINT ( 'NONE', #51713 ) ;
#60061=FACE_BOUND ( 'NONE', #71087, .T. ) ;
#60062=CARTESIAN_POINT ( 'NONE',  ( 7.596177115211490971, -11.79746400365624659, 32.30657167506340954 ) ) ;
#60063=CARTESIAN_POINT ( 'NONE',  ( 18.00000000000000000, -4.786620604624113540, 33.94971097300155094 ) ) ;
#60064=ORIENTED_EDGE ( 'NONE', *, *, #67545, .T. ) ;
#60065=CARTESIAN_POINT ( 'NONE',  ( -1.134669975237340811, -5.766571408460172243, 34.70601412856602508 ) ) ;
#60067=CARTESIAN_POINT ( 'NONE',  ( -0.6850233861027925641, -2.353723527008297012, 30.78948104536958397 ) ) ;
#60069=CARTESIAN_POINT ( 'NONE',  ( 14.53070515178570510, -3.395485233115139057, 33.02377354290275946 ) ) ;
#60070=CARTESIAN_POINT ( 'NONE',  ( 7.145856592054988354, -5.827830569534416583, 34.72679350104403539 ) ) ;
#60071=CARTESIAN_POINT ( 'NONE',  ( -9.692307692307691624, -2.538708090699994813, 30.37095296980875503 ) ) ;
#60072=EDGE_LOOP ( 'NONE', ( #88487, #14160 ) ) ;
#60073=CARTESIAN_POINT ( 'NONE',  ( 2.530705151785703766, -12.38742843783360748, 31.66772728687926985 ) ) ;
#60075=VERTEX_POINT ( 'NONE', #79215 ) ;
#60076=CARTESIAN_POINT ( 'NONE',  ( 0.3954550505825807916, -8.973038597847271092, 34.52809138561120506 ) ) ;
#60077=CARTESIAN_POINT ( 'NONE',  ( -7.846153846153530509, -2.255955759149395501, 30.00000000000324363 ) ) ;
#60078=LINE ( 'NONE', #46572, #62659 ) ;
#60079=CARTESIAN_POINT ( 'NONE',  ( 15.23076923076923173, -1.951392089020283160, 34.73218667398347748 ) ) ;
#60080=FACE_OUTER_BOUND ( 'NONE', #83761, .T. ) ;
#60081=ADVANCED_FACE ( 'NONE', ( #11196 ), #72444, .F. ) ;
#60082=ADVANCED_FACE ( 'NONE', ( #52168 ), #17960, .F. ) ;
#60083=LINE ( 'NONE', #51984, #7821 ) ;
#60084=CARTESIAN_POINT ( 'NONE',  ( 14.30769230769261569, -2.506253911140615021, 30.00000000000323297 ) ) ;
#60085=DIRECTION ( 'NONE',  ( 1.000000000000000000, 0.000000000000000000, 0.000000000000000000 ) ) ;
#60086=CARTESIAN_POINT ( 'NONE',  ( 10.61538461538461675, -9.058645607665452459, 34.76329471203371924 ) ) ;
#60087=DIRECTION ( 'NONE',  ( -0.000000000000000000, 0.9848077530122085754, -0.1736481776669273613 ) ) ;
#60090=B_SPLINE_CURVE_WITH_KNOTS ( 'NONE', 3,
 ( #12721, #40206, #12275, #67668, #26674, #60015, #87516, #5970, #54132, #67228 ),
 .UNSPECIFIED., .F., .F.,
 ( 4, 2, 2, 2, 4 ),
 ( 0.000000000000000000, 0.0001954311564186879044, 0.0003908623128373758088, 0.0005862934692560636861, 0.0007817246256747516176 ),
 .UNSPECIFIED. ) ;
#60092=ORIENTED_EDGE ( 'NONE', *, *, #77936, .T. ) ;
#60094=B_SPLINE_CURVE_WITH_KNOTS ( 'NONE', 3,
 ( #7148, #79150, #11132, #2587, #22864, #50329, #57097, #16119, #63855, #51648 ),
 .UNSPECIFIED., .F., .F.,
 ( 4, 2, 2, 2, 4 ),
 ( 0.0007817246256747472808, 0.0009771112852218905021, 0.001172497944769033832, 0.001367884604316177161, 0.001563271263863320274 ),
 .UNSPECIFIED. ) ;
#60095=AXIS2_PLACEMENT_3D ( 'NONE', #33041, #75361, #46110 ) ;
#60096=ORIENTED_EDGE ( 'NONE', *, *, #60146, .F. ) ;
#60097=CARTESIAN_POINT ( 'NONE',  ( -7.780086512803770837, -2.486705287966280320, 31.30864560766543647 ) ) ;
#60098=EDGE_LOOP ( 'NONE', ( #27940, #38828 ) ) ;
#60099=CARTESIAN_POINT ( 'NONE',  ( -5.749945580086545327, -10.06805714834173848, 34.32951233291982618 ) ) ;
#60101=CARTESIAN_POINT ( 'NONE',  ( 12.68450159580513592, -7.369474539155828730, 34.99858011523957657 ) ) ;
#60102=DIRECTION ( 'NONE',  ( -0.000000000000000000, 0.8660254037844397068, -0.4999999999999978906 ) ) ;
#60103=CARTESIAN_POINT ( 'NONE',  ( -0.2385271099256116856, -5.667800583137508674, 34.40243808032445827 ) ) ;
#60104=CARTESIAN_POINT ( 'NONE',  ( 9.823098133274648092, -2.845873456487966635, 32.17976146951972538 ) ) ;
#60105=VECTOR ( 'NONE', #43251, 1000.000000000000000 ) ;
#60106=CARTESIAN_POINT ( 'NONE',  ( -4.826977667545034656, -2.589246495874657938, 31.60778113518102828 ) ) ;
#60107=CARTESIAN_POINT ( 'NONE',  ( 0.7115928814519137946, -5.642605341092957083, 34.66089969410670335 ) ) ;
#60108=CARTESIAN_POINT ( 'NONE',  ( -14.30769230769230660, -4.661471528628507777, 34.16647553114623292 ) ) ;
#60112=VECTOR ( 'NONE', #7186, 1000.000000000000227 ) ;
#60113=CARTESIAN_POINT ( 'NONE',  ( -17.07692307692307665, -13.53365097954675988, 30.81389545987213552 ) ) ;
#60114=VERTEX_POINT ( 'NONE', #61148 ) ;
#60115=EDGE_LOOP ( 'NONE', ( #14595, #71583, #62105, #34009 ) ) ;
#60116=CARTESIAN_POINT ( 'NONE',  ( 14.08420738312797837, -8.539481045369596401, 34.89627647299170832 ) ) ;
#60117=DIRECTION ( 'NONE',  ( -0.000000000000000000, -0.8660254037844399289, -0.4999999999999980016 ) ) ;
#60118=DIRECTION ( 'NONE',  ( -0.000000000000000000, 0.1736481776669307198, -0.9848077530122080203 ) ) ;
#60119=CARTESIAN_POINT ( 'NONE',  ( -6.130147209438219669, -3.817052484675422797, 33.13202310037935661 ) ) ;
#60121=CARTESIAN_POINT ( 'NONE',  ( -0.4615384615384611200, -6.386643153685126251, 34.62446782046654192 ) ) ;
#60123=ORIENTED_EDGE ( 'NONE', *, *, #12544, .T. ) ;
#60124=CARTESIAN_POINT ( 'NONE',  ( 3.230769230769231726, -6.343179335718451384, 34.87096338111211935 ) ) ;
#60125=VERTEX_POINT ( 'NONE', #75130 ) ;
#60126=B_SPLINE_CURVE_WITH_KNOTS ( 'NONE', 3,
 ( #46705, #18796, #26442, #61102, #46264, #19240, #73293, #67423, #4385, #59325 ),
 .UNSPECIFIED., .F., .F.,
 ( 4, 2, 2, 2, 4 ),
 ( 0.0007817246256747514008, 0.0009771112852218952725, 0.001172497944769039036, 0.001367884604316182799, 0.001563271263863326779 ),
 .UNSPECIFIED. ) ;
#60128=CARTESIAN_POINT ( 'NONE',  ( 5.207714884747862705, -8.147973898785416225, 34.70805048591653730 ) ) ;
#60129=CARTESIAN_POINT ( 'NONE',  ( 5.750000000000002665, -7.433931650972300353, 34.75000000000000711 ) ) ;
#60130=CARTESIAN_POINT ( 'NONE',  ( -0.6843665591733403275, -7.369209533119137845, 34.99857337881830688 ) ) ;
#60131=CARTESIAN_POINT ( 'NONE',  ( 3.903846153846154632, -7.500000000000001776, 35.00000000000000000 ) ) ;
#60132=CARTESIAN_POINT ( 'NONE',  ( -5.326899820971668476, -8.347322224742351082, 34.93158281831414769 ) ) ;
#60133=EDGE_CURVE ( 'NONE', #72521, #51846, #41330, .T. ) ;
#60134=VERTEX_POINT ( 'NONE', #82773 ) ;
#60135=ORIENTED_EDGE ( 'NONE', *, *, #75215, .T. ) ;
#60136=ORIENTED_EDGE ( 'NONE', *, *, #13651, .T. ) ;
#60137=CARTESIAN_POINT ( 'NONE',  ( -12.46153846153846168, -11.69971097300155272, 32.46337939537588113 ) ) ;
#60138=CARTESIAN_POINT ( 'NONE',  ( 10.55011461482829560, -11.67786785259540849, 32.92929555188721480 ) ) ;
#60139=CARTESIAN_POINT ( 'NONE',  ( 16.40390057375960708, -5.642605341092955307, 34.66089969410670335 ) ) ;
#60140=CARTESIAN_POINT ( 'NONE',  ( 1.134638653673031961, -3.627789207965226748, 32.91389620160131102 ) ) ;
#60141=EDGE_CURVE ( 'NONE', #37287, #6173, #73571, .T. ) ;
#60142=VECTOR ( 'NONE', #61067, 1000.000000000000000 ) ;
#60144=FACE_OUTER_BOUND ( 'NONE', #49840, .T. ) ;
#60145=EDGE_LOOP ( 'NONE', ( #6527, #79320 ) ) ;
#60146=EDGE_CURVE ( 'NONE', #38304, #37932, #22033, .T. ) ;
#60147=ORIENTED_EDGE ( 'NONE', *, *, #24880, .F. ) ;
#60149=VECTOR ( 'NONE', #49389, 1000.000000000000114 ) ;
#60150=CARTESIAN_POINT ( 'NONE',  ( -3.360917200500930235, -2.647304123082328875, 31.75400227202885262 ) ) ;
#60151=ORIENTED_EDGE ( 'NONE', *, *, #84784, .T. ) ;
#60152=CARTESIAN_POINT ( 'NONE',  ( 1.254468175177163358, -10.19110544564091825, 33.96427741523702792 ) ) ;
#60153=CARTESIAN_POINT ( 'NONE',  ( -7.173076923076921574, -2.249999999999998668, 29.75000000000000355 ) ) ;
#60154=B_SPLINE_CURVE_WITH_KNOTS ( 'NONE', 3,
 ( #9698, #50674, #56117, #16461, #76841, #64629, #42611, #38970, #44806, #60108 ),
 .UNSPECIFIED., .F., .F.,
 ( 4, 2, 2, 2, 4 ),
 ( 0.0007817246256747484735, 0.0009771112852218922368, 0.001172497944769036217, 0.001367884604316180197, 0.001563271263863323960 ),
 .UNSPECIFIED. ) ;
#60156=EDGE_LOOP ( 'NONE', ( #46465, #32166 ) ) ;
#60157=EDGE_CURVE ( 'NONE', #78012, #72078, #70369, .T. ) ;
#60158=CARTESIAN_POINT ( 'NONE',  ( -1.161602540521988747, -11.43677907613345113, 33.22367315496201456 ) ) ;
#60160=CARTESIAN_POINT ( 'NONE',  ( 13.38461538461526423, -11.06231777344772027, 33.60647404775119895 ) ) ;
#60161=CARTESIAN_POINT ( 'NONE',  ( 9.692307692307572609, -9.442884908241554243, 34.35708131394783038 ) ) ;
#60162=FACE_BOUND ( 'NONE', #83878, .T. ) ;
#60163=CARTESIAN_POINT ( 'NONE',  ( -5.011667505647051435, -12.27809138561124591, 31.22303859784720359 ) ) ;
#60165=CARTESIAN_POINT ( 'NONE',  ( 17.07692307692295586, -3.083524468854526912, 32.58852847137268327 ) ) ;
#60166=ORIENTED_EDGE ( 'NONE', *, *, #58954, .F. ) ;
#60167=CARTESIAN_POINT ( 'NONE',  ( -11.28851612908349722, -8.476813868363244353, 34.90874843262270133 ) ) ;
#60168=CARTESIAN_POINT ( 'NONE',  ( 9.019176287578909879, -6.696923467548660192, 34.68552623307873972 ) ) ;
#60169=CARTESIAN_POINT ( 'NONE',  ( 1.384615384615386802, -11.91647553114624181, 32.58852847137148245 ) ) ;
#60172=CARTESIAN_POINT ( 'NONE',  ( -16.15384615384615330, -2.249999999999998668, 29.50000000000001421 ) ) ;
#60174=CARTESIAN_POINT ( 'NONE',  ( -16.37677311275300340, -11.98009711892700224, 32.48740034544074007 ) ) ;
#60175=CARTESIAN_POINT ( 'NONE',  ( -12.46153846153846168, -2.721908614388771852, 31.22303859784724978 ) ) ;
#60176=EDGE_CURVE ( 'NONE', #17409, #47786, #84420, .T. ) ;
#60177=FACE_BOUND ( 'NONE', #77889, .T. ) ;
#60178=CARTESIAN_POINT ( 'NONE',  ( 13.13459216039392530, -12.07920672191015221, 32.31858351112116168 ) ) ;
#60181=CARTESIAN_POINT ( 'NONE',  ( -5.869208192175211281, -9.804649428959608670, 34.18742332936588468 ) ) ;
#60182=CARTESIAN_POINT ( 'NONE',  ( -0.4615384615385826339, -12.46129190930018460, 30.37095296980731973 ) ) ;
#60183=ADVANCED_FACE ( 'NONE', ( #75998 ), #14300, .F. ) ;
#60185=VECTOR ( 'NONE', #55194, 1000.000000000000000 ) ;
#60187=ORIENTED_EDGE ( 'NONE', *, *, #68499, .F. ) ;
#60188=CARTESIAN_POINT ( 'NONE',  ( 10.55011461482829560, -12.16647553114622049, 32.15551576947930812 ) ) ;
#60189=EDGE_LOOP ( 'NONE', ( #340, #35219, #56936, #33711 ) ) ;
#60190=CARTESIAN_POINT ( 'NONE',  ( -8.769230769230768274, -13.75783147151868846, 33.36296068462461051 ) ) ;
#60191=EDGE_CURVE ( 'NONE', #16008, #28285, #49421, .T. ) ;
#60192=ORIENTED_EDGE ( 'NONE', *, *, #51056, .T. ) ;
#60193=EDGE_CURVE ( 'NONE', #35799, #19030, #85371, .T. ) ;
#60194=CARTESIAN_POINT ( 'NONE',  ( 7.623227628637698317, -9.086856451489516928, 34.49173150075333183 ) ) ;
#60195=CARTESIAN_POINT ( 'NONE',  ( 13.38461538461538680, -1.215029322943914858, 32.30358669280327177 ) ) ;
#60196=CYLINDRICAL_SURFACE ( 'NONE', #17935, 0.2499999999999994726 ) ;
#60197=ORIENTED_EDGE ( 'NONE', *, *, #34316, .T. ) ;
#60198=CARTESIAN_POINT ( 'NONE',  ( -16.21992956480203674, -2.538708090699995257, 30.37095296980875148 ) ) ;
#60199=CARTESIAN_POINT ( 'NONE',  ( -11.60454391782167249, -3.937682226553330445, 33.60647404775217240 ) ) ;
#60201=CARTESIAN_POINT ( 'NONE',  ( 2.084766090176161324, -11.76352882383564769, 32.36236540154569497 ) ) ;
#60202=DIRECTION ( 'NONE',  ( -0.000000000000000000, -0.3420201433256694901, -0.9396926207859082059 ) ) ;
#60203=CARTESIAN_POINT ( 'NONE',  ( -6.923076923076922462, -9.584722331328613620, 36.20867863119891439 ) ) ;
#60204=CARTESIAN_POINT ( 'NONE',  ( 15.23076923076911093, -6.879047030192662504, 34.71129190930017927 ) ) ;
#60205=CARTESIAN_POINT ( 'NONE',  ( -6.988347369037697376, -4.481592998940161721, 33.73612834413957984 ) ) ;
#60207=B_SPLINE_CURVE_WITH_KNOTS ( 'NONE', 3,
 ( #14120, #28078, #55988, #162, #33946, #7371, #61403, #27632, #74947, #41593 ),
 .UNSPECIFIED., .F., .F.,
 ( 4, 2, 2, 2, 4 ),
 ( 0.0007817359430256369448, 0.0009771253907250049969, 0.001172514838424373049, 0.001367904286123741101, 0.001563293733823109153 ),
 .UNSPECIFIED. ) ;
#60210=CARTESIAN_POINT ( 'NONE',  ( -1.384615384615506484, -12.16647553114689728, 32.15551576947799362 ) ) ;
#60211=ORIENTED_EDGE ( 'NONE', *, *, #62802, .F. ) ;
#60212=CYLINDRICAL_SURFACE ( 'NONE', #77276, 0.2499999999999994726 ) ;
#60213=FACE_OUTER_BOUND ( 'NONE', #63068, .T. ) ;
#60215=CARTESIAN_POINT ( 'NONE',  ( 14.30769230769231015, -1.629998284177014645, 34.34916445242399163 ) ) ;
#60217=ORIENTED_EDGE ( 'NONE', *, *, #28948, .T. ) ;
#60218=CARTESIAN_POINT ( 'NONE',  ( -0.4615384615384611200, -2.249999999999998668, 29.50000000000001421 ) ) ;
#60219=CARTESIAN_POINT ( 'NONE',  ( 9.692307692307695177, -12.62096338111211580, 30.90682066428153263 ) ) ;
#60220=CARTESIAN_POINT ( 'NONE',  ( 7.846153846153723244, -2.657715359629662544, 31.77849191805970364 ) ) ;
#60221=EDGE_LOOP ( 'NONE', ( #7564, #23337, #63377, #9414 ) ) ;
#60222=CARTESIAN_POINT ( 'NONE',  ( -7.976845312821407852, -8.147922237126337563, 34.70805685702651999 ) ) ;
#60223=CARTESIAN_POINT ( 'NONE',  ( 4.403846153846153300, -2.499999999999998668, 29.75000000000000355 ) ) ;
#60224=DIRECTION ( 'NONE',  ( -0.000000000000000000, -0.6427876096865404731, -0.7660444431189771253 ) ) ;
#60225=VECTOR ( 'NONE', #12083, 1000.000000000000000 ) ;
#60226=CARTESIAN_POINT ( 'NONE',  ( 13.38461538461538680, -5.180354513474913603, 36.12317359536750416 ) ) ;
#60227=VERTEX_POINT ( 'NONE', #22385 ) ;
#60228=VECTOR ( 'NONE', #23633, 1000.000000000000000 ) ;
#60229=CARTESIAN_POINT ( 'NONE',  ( 7.146452408849343740, -2.251407671071270489, 29.88021292934942252 ) ) ;
#60232=CARTESIAN_POINT ( 'NONE',  ( 8.703148389870632329, -3.322132147404559532, 32.92929555188719348 ) ) ;
#60233=ORIENTED_EDGE ( 'NONE', *, *, #609, .T. ) ;
#60234=ORIENTED_EDGE ( 'NONE', *, *, #36717, .T. ) ;
#60235=EDGE_CURVE ( 'NONE', #35516, #48302, #63811, .T. ) ;
#60236=ORIENTED_EDGE ( 'NONE', *, *, #8114, .T. ) ;
#60237=EDGE_CURVE ( 'NONE', #45764, #39096, #3667, .T. ) ;
#60238=CARTESIAN_POINT ( 'NONE',  ( 0.2115152242454957365, -8.432397168068783699, 34.66272746175022945 ) ) ;
#60239=CARTESIAN_POINT ( 'NONE',  ( 14.05766907039934210, -4.335965774309649134, 33.62209801155881905 ) ) ;
#60240=DIRECTION ( 'NONE',  ( 0.000000000000000000, 0.9396926207859126468, -0.3420201433256571111 ) ) ;
#60241=ADVANCED_FACE ( 'NONE', ( #8881 ), #36349, .F. ) ;
#60242=CARTESIAN_POINT ( 'NONE',  ( -5.999999999999998224, -9.780366693483667717, 34.19971097300155094 ) ) ;
#60243=ORIENTED_EDGE ( 'NONE', *, *, #21898, .T. ) ;
#60244=EDGE_LOOP ( 'NONE', ( #45179, #34294 ) ) ;
#60245=ORIENTED_EDGE ( 'NONE', *, *, #42519, .F. ) ;
#60246=CARTESIAN_POINT ( 'NONE',  ( -7.976845312821407852, -4.809359713505814149, 33.96456829005828837 ) ) ;
#60247=ORIENTED_EDGE ( 'NONE', *, *, #53042, .F. ) ;
#60249=B_SPLINE_CURVE_WITH_KNOTS ( 'NONE', 3,
 ( #36987, #16287, #50932, #15412, #71218, #8653 ),
 .UNSPECIFIED., .F., .F.,
 ( 4, 2, 4 ),
 ( 0.0003909512603273706676, 0.0005862562993131958163, 0.0007815613382990209109 ),
 .UNSPECIFIED. ) ;
#60251=CARTESIAN_POINT ( 'NONE',  ( 12.59232890250541281, -11.37503395064541678, 33.29242100308974273 ) ) ;
#60253=CARTESIAN_POINT ( 'NONE',  ( -4.403846153846151523, -7.500000000000001776, 35.00000000000000000 ) ) ;
#60254=ORIENTED_EDGE ( 'NONE', *, *, #51918, .F. ) ;
#60255=B_SPLINE_CURVE_WITH_KNOTS ( 'NONE', 3,
 ( #10380, #84726, #37393, #24775, #30211, #72515, #52241, #3162, #9485, #30639 ),
 .UNSPECIFIED., .F., .F.,
 ( 4, 2, 2, 2, 4 ),
 ( 0.000000000000000000, 0.0001954311564186872810, 0.0003908623128373745620, 0.0005862934692560618430, 0.0007817246256747491240 ),
 .UNSPECIFIED. ) ;
#60256=ADVANCED_FACE ( 'NONE', ( #2110 ), #55723, .F. ) ;
#60257=EDGE_LOOP ( 'NONE', ( #8400, #3239 ) ) ;
#60258=ORIENTED_EDGE ( 'NONE', *, *, #3206, .T. ) ;
#60260=CARTESIAN_POINT ( 'NONE',  ( 8.769230769230647482, -2.625532179533778709, 30.86335684631627174 ) ) ;
#60261=VERTEX_POINT ( 'NONE', #786 ) ;
#60262=CARTESIAN_POINT ( 'NONE',  ( 2.084765348785460937, -2.523278758544489353, 31.42238647778637528 ) ) ;
#60263=CARTESIAN_POINT ( 'NONE',  ( 12.33139125210024112, -11.47017969459903952, 32.78971311882035167 ) ) ;
#60264=CARTESIAN_POINT ( 'NONE',  ( -17.01166750564705055, -9.442884908240273489, 34.35708131394835618 ) ) ;
#60265=CARTESIAN_POINT ( 'NONE',  ( 16.40379167219429846, -3.712312575010499494, 33.01462480002815170 ) ) ;
#60267=FACE_BOUND ( 'NONE', #34139, .T. ) ;
#60268=CARTESIAN_POINT ( 'NONE',  ( -8.703163435880695076, -2.292212530054420494, 30.41441678777542990 ) ) ;
#60270=CARTESIAN_POINT ( 'NONE',  ( -8.069638789877792817, -12.24155766932282496, 31.33739205006857986 ) ) ;
#60272=CARTESIAN_POINT ( 'NONE',  ( 14.37375964104238335, -2.833524468853757750, 32.15551576947925838 ) ) ;
#60274=LINE ( 'NONE', #74246, #68303 ) ;
#60275=CARTESIAN_POINT ( 'NONE',  ( 12.59232890250541814, -2.845873456487966635, 32.17976146951972538 ) ) ;
#60276=EDGE_LOOP ( 'NONE', ( #46551, #23316, #68735, #20681, #75861, #55490 ) ) ;
#60277=CARTESIAN_POINT ( 'NONE',  ( -16.21960295636046823, -7.249945686854186278, 34.74374336980224598 ) ) ;
#60278=CARTESIAN_POINT ( 'NONE',  ( -13.16160254052198830, -4.026326845037962343, 33.68677907613344047 ) ) ;
#60279=EDGE_LOOP ( 'NONE', ( #58999, #35810, #65333, #8115, #51354, #70105 ) ) ;
#60280=ORIENTED_EDGE ( 'NONE', *, *, #88681, .T. ) ;
#60281=CARTESIAN_POINT ( 'NONE',  ( -17.14300648787895298, -11.16473453929635440, 33.15142922261925662 ) ) ;
#60282=VECTOR ( 'NONE', #48912, 1000.000000000000114 ) ;
#60283=CARTESIAN_POINT ( 'NONE',  ( 16.02369818411445834, -2.373036134822905208, 30.88089517874952250 ) ) ;
#60284=CARTESIAN_POINT ( 'NONE',  ( -2.307692307692305711, -11.35647404775217417, 33.31231777344666511 ) ) ;
#60285=ORIENTED_EDGE ( 'NONE', *, *, #26257, .T. ) ;
#60286=CARTESIAN_POINT ( 'NONE',  ( 8.638540166120462160, -12.62707690430377383, 30.88035979386743435 ) ) ;
#60287=CARTESIAN_POINT ( 'NONE',  ( 6.673100179028331524, -8.347322224742351082, 34.93158281831414769 ) ) ;
#60289=EDGE_CURVE ( 'NONE', #22236, #1002, #21948, .T. ) ;
#60290=B_SPLINE_CURVE_WITH_KNOTS ( 'NONE', 3,
 ( #71051, #44446, #72818, #59312, #64724, #24189, #3024, #77806, #2581, #57534 ),
 .UNSPECIFIED., .F., .F.,
 ( 4, 2, 2, 2, 4 ),
 ( 0.0007817359430256334753, 0.0009771253907250058643, 0.001172514838424371098, 0.001367904286123736764, 0.001563293733823101998 ),
 .UNSPECIFIED. ) ;
#60291=CARTESIAN_POINT ( 'NONE',  ( -15.29603967673000575, -6.026961402152685388, 34.52809138561120506 ) ) ;
#60292=FACE_OUTER_BOUND ( 'NONE', #22248, .T. ) ;
#60293=B_SPLINE_CURVE_WITH_KNOTS ( 'NONE', 3,
 ( #25937, #54733, #26832, #82222, #74578, #6560, #54285, #67817, #46656, #81342 ),
 .UNSPECIFIED., .F., .F.,
 ( 4, 2, 2, 2, 4 ),
 ( 0.000000000000000000, 0.0001954339857564076641, 0.0003908679715128153282, 0.0005863019572692229923, 0.0007817359430256306564 ),
 .UNSPECIFIED. ) ;
#60294=CARTESIAN_POINT ( 'NONE',  ( -8.835314180186648159, -6.386643153685125363, 34.62446782046654903 ) ) ;
#60295=CARTESIAN_POINT ( 'NONE',  ( -5.326899807865431491, -9.148715823498378086, 34.47080413974185120 ) ) ;
#60296=CARTESIAN_POINT ( 'NONE',  ( -10.39260494640654819, -11.60474049983371003, 33.02348890104160262 ) ) ;
#60297=B_SPLINE_CURVE_WITH_KNOTS ( 'NONE', 3,
 ( #57064, #70587, #63823, #49861, #70139, #9336, #42242, #22396, #35922, #41798 ),
 .UNSPECIFIED., .F., .F.,
 ( 4, 2, 2, 2, 4 ),
 ( 0.0007817359430256293554, 0.0009771253907249950223, 0.001172514838424360906, 0.001367904286123726790, 0.001563293733823092457 ),
 .UNSPECIFIED. ) ;
#60299=ORIENTED_EDGE ( 'NONE', *, *, #1363, .T. ) ;
#60300=EDGE_CURVE ( 'NONE', #57554, #62076, #16074, .T. ) ;
#60302=CARTESIAN_POINT ( 'NONE',  ( 4.826946332874485712, -10.82459398097509684, 33.81372124010185587 ) ) ;
#60303=ADVANCED_FACE ( 'NONE', ( #1223 ), #56174, .F. ) ;
#60304=CARTESIAN_POINT ( 'NONE',  ( 7.173022441425064955, -12.22109172314383052, 31.39792113162168263 ) ) ;
#60306=CARTESIAN_POINT ( 'NONE',  ( -9.692307692307814193, -8.656820664282941280, 34.87096338111179961 ) ) ;
#60307=CARTESIAN_POINT ( 'NONE',  ( -15.09997742294444834, -2.729792928343269587, 31.24908615093345077 ) ) ;
#60309=CARTESIAN_POINT ( 'NONE',  ( -16.15384615384615330, -2.721908614388771852, 31.22303859784724978 ) ) ;
#60311=CARTESIAN_POINT ( 'NONE',  ( -13.25377696660261861, -7.277220443632450575, 34.74524770363009196 ) ) ;
#60312=CARTESIAN_POINT ( 'NONE',  ( -18.06519398178334868, -12.49374608885955062, 29.99999999999984723 ) ) ;
#60313=LINE ( 'NONE', #45462, #61238 ) ;
#60314=CARTESIAN_POINT ( 'NONE',  ( 8.769230769230768274, -12.10708131394839349, 31.69288490824020244 ) ) ;
#60315=CARTESIAN_POINT ( 'NONE',  ( 5.999999999999880096, -12.27809138561165270, 31.22303859784587132 ) ) ;
#60316=CARTESIAN_POINT ( 'NONE',  ( 7.976679284387491187, -8.630441415882550871, 34.87705825610312615 ) ) ;
#60317=CARTESIAN_POINT ( 'NONE',  ( -3.480792468062195333, -8.432397168068783699, 34.66272746175022945 ) ) ;
#60318=CARTESIAN_POINT ( 'NONE',  ( -16.94639763868943660, -3.068774925481847937, 32.56582465632704526 ) ) ;
#60319=EDGE_CURVE ( 'NONE', #67219, #43247, #12297, .T. ) ;
#60321=DIRECTION ( 'NONE',  ( -0.000000000000000000, 0.1736481776669307198, -0.9848077530122080203 ) ) ;
#60322=CYLINDRICAL_SURFACE ( 'NONE', #40311, 0.2499999999999995559 ) ;
#60324=CARTESIAN_POINT ( 'NONE',  ( 5.299935921016469820, -10.01129605718032778, 34.36064277460058491 ) ) ;
#60325=DIRECTION ( 'NONE',  ( -0.000000000000000000, 0.9396926207859093161, -0.3420201433256663259 ) ) ;
#60326=EDGE_CURVE ( 'NONE', #45410, #82411, #12072, .T. ) ;
#60327=DIRECTION ( 'NONE',  ( 0.000000000000000000, 0.1736481776669267785, -0.9848077530122087975 ) ) ;
#60328=CYLINDRICAL_SURFACE ( 'NONE', #77016, 0.2499999999999979738 ) ;
#60329=ORIENTED_EDGE ( 'NONE', *, *, #46655, .F. ) ;
#60331=LINE ( 'NONE', #61212, #62777 ) ;
#60332=ORIENTED_EDGE ( 'NONE', *, *, #2536, .T. ) ;
#60333=CARTESIAN_POINT ( 'NONE',  ( -18.00000000000012079, -3.835265460704626150, 33.15142922262032954 ) ) ;
#60334=B_SPLINE_CURVE_WITH_KNOTS ( 'NONE', 3,
 ( #10980, #79880, #18629, #58263, #46095, #38450, #85753, #52839, #2864, #51483 ),
 .UNSPECIFIED., .F., .F.,
 ( 4, 2, 2, 2, 4 ),
 ( 0.0007817359430256215491, 0.0009771253907249856981, 0.001172514838424349847, 0.001367904286123713779, 0.001563293733823077928 ),
 .UNSPECIFIED. ) ;
#60335=ORIENTED_EDGE ( 'NONE', *, *, #61999, .T. ) ;
#60336=B_SPLINE_CURVE_WITH_KNOTS ( 'NONE', 3,
 ( #66531, #74174, #72383, #19234, #12039, #18340, #24647, #5272, #3479, #30949 ),
 .UNSPECIFIED., .F., .F.,
 ( 4, 2, 2, 2, 4 ),
 ( 0.000000000000000000, 0.0001954339857564065257, 0.0003908679715128130514, 0.0005863019572692196313, 0.0007817359430256261028 ),
 .UNSPECIFIED. ) ;
#60337=CARTESIAN_POINT ( 'NONE',  ( -7.780898706641009355, -6.835583212224610072, 34.95778746994559327 ) ) ;
#60338=ADVANCED_FACE ( 'NONE', ( #7853 ), #82186, .F. ) ;
#60339=CARTESIAN_POINT ( 'NONE',  ( -11.78846153846153832, -2.249999999999998668, 29.75000000000000355 ) ) ;
#60340=CARTESIAN_POINT ( 'NONE',  ( -8.096177083446805867, -3.711651800289232028, 33.01384336483936011 ) ) ;
#60341=ORIENTED_EDGE ( 'NONE', *, *, #56547, .F. ) ;
#60342=EDGE_LOOP ( 'NONE', ( #65513, #80985 ) ) ;
#60343=ADVANCED_FACE ( 'NONE', ( #12829 ), #14159, .F. ) ;
#60344=VERTEX_POINT ( 'NONE', #20475 ) ;
#60346=VECTOR ( 'NONE', #21930, 1000.000000000000000 ) ;
#60347=CARTESIAN_POINT ( 'NONE',  ( -0.6850234052624102343, -3.236172620538810385, 32.36188796281390267 ) ) ;
#60348=CARTESIAN_POINT ( 'NONE',  ( -0.2115929431903195990, -10.76462480002816235, 33.53768742498949962 ) ) ;
#60349=CARTESIAN_POINT ( 'NONE',  ( 0.4615384615384611200, -1.790695186598648903, 34.54067556320373455 ) ) ;
#60350=DIRECTION ( 'NONE',  ( 0.000000000000000000, 0.4999999999999960032, -0.8660254037844410391 ) ) ;
#60351=CARTESIAN_POINT ( 'NONE',  ( -10.86540783960606760, -12.07920672191015221, 32.31858351112116168 ) ) ;
#60352=FACE_OUTER_BOUND ( 'NONE', #48623, .T. ) ;
#60354=AXIS2_PLACEMENT_3D ( 'NONE', #66628, #5372, #88696 ) ;
#60355=VECTOR ( 'NONE', #54613, 1000.000000000000114 ) ;
#60357=CARTESIAN_POINT ( 'NONE',  ( -0.2115930521604184877, -12.45601412856602863, 31.48342859153981621 ) ) ;
#60358=VERTEX_POINT ( 'NONE', #19586 ) ;
#60360=EDGE_CURVE ( 'NONE', #66580, #87401, #48824, .T. ) ;
#60361=VERTEX_POINT ( 'NONE', #55141 ) ;
#60362=CARTESIAN_POINT ( 'NONE',  ( 1.384615384615264011, -5.941354392335915335, 34.76329471203413846 ) ) ;
#60364=CARTESIAN_POINT ( 'NONE',  ( -8.638440328263820689, -10.70102852606553157, 33.91149625220312913 ) ) ;
#60365=CARTESIAN_POINT ( 'NONE',  ( 12.68454981315131036, -3.105924265160262543, 32.13625925475356127 ) ) ;
#60366=ORIENTED_EDGE ( 'NONE', *, *, #86603, .F. ) ;
#60370=VERTEX_POINT ( 'NONE', #76299 ) ;
#60371=DIRECTION ( 'NONE',  ( 0.000000000000000000, 0.9396926207859126468, -0.3420201433256571111 ) ) ;
#60374=CARTESIAN_POINT ( 'NONE',  ( 1.515141086378949842, -6.852161475712352789, 34.70806712695775786 ) ) ;
#60375=AXIS2_PLACEMENT_3D ( 'NONE', #77478, #50437, #16652 ) ;
#60376=CARTESIAN_POINT ( 'NONE',  ( -15.90379173393269951, -10.82426656108011720, 33.81400080652039009 ) ) ;
#60377=FACE_BOUND ( 'NONE', #81714, .T. ) ;
#60380=CARTESIAN_POINT ( 'NONE',  ( 13.51514082284902862, -5.070358843744210198, 34.40418822224088302 ) ) ;
#60381=CARTESIAN_POINT ( 'NONE',  ( 3.361294669002876212, -5.070358843744209310, 34.40418822224088302 ) ) ;
#60382=CARTESIAN_POINT ( 'NONE',  ( 7.846153846153846700, -12.29105614889573062, 35.45975837776705220 ) ) ;
#60383=LINE ( 'NONE', #87897, #73539 ) ;
#60384=VERTEX_POINT ( 'NONE', #20026 ) ;
#60385=DIRECTION ( 'NONE',  ( -0.000000000000000000, -0.9848077530122085754, -0.1736481776669273613 ) ) ;
#60386=ORIENTED_EDGE ( 'NONE', *, *, #33552, .T. ) ;
#60387=VERTEX_POINT ( 'NONE', #47046 ) ;
#60388=DIRECTION ( 'NONE',  ( -0.000000000000000000, 0.9848077530122086864, -0.1736481776669273891 ) ) ;
#60389=DIRECTION ( 'NONE',  ( 0.000000000000000000, 0.1736481776669267785, -0.9848077530122087975 ) ) ;
#60390=FACE_OUTER_BOUND ( 'NONE', #51095, .T. ) ;
#60391=CARTESIAN_POINT ( 'NONE',  ( -4.087778820496076548, -9.058645607665452459, 34.76329471203371924 ) ) ;
#60393=CARTESIAN_POINT ( 'NONE',  ( -2.084912766423897335, -2.847695495035523550, 31.58253572463339154 ) ) ;
#60394=ORIENTED_EDGE ( 'NONE', *, *, #89007, .T. ) ;
#60395=CARTESIAN_POINT ( 'NONE',  ( 17.07692307692307665, -3.050289026998446396, 32.03036669348365706 ) ) ;
#60396=CARTESIAN_POINT ( 'NONE',  ( 11.31558285603289349, -7.630691491037285168, 34.74850469731152458 ) ) ;
#60397=CARTESIAN_POINT ( 'NONE',  ( -1.634592115557738312, -3.627789207965226748, 32.91389620160131102 ) ) ;
#60398=CARTESIAN_POINT ( 'NONE',  ( -15.93106648486808119, -4.226511098958372514, 33.85474049983370293 ) ) ;
#60399=ORIENTED_EDGE ( 'NONE', *, *, #38467, .T. ) ;
#60402=VECTOR ( 'NONE', #16878, 1000.000000000000000 ) ;
#60404=CIRCLE ( 'NONE', #11496, 0.2500000000000002220 ) ;
#60406=CARTESIAN_POINT ( 'NONE',  ( 0.5267940328144853357, -10.90142922261932057, 33.41473453929631887 ) ) ;
#60407=CARTESIAN_POINT ( 'NONE',  ( -18.00000000000012079, -5.219633306517615701, 34.19971097300220464 ) ) ;
#60408=EDGE_CURVE ( 'NONE', #85626, #45, #42088, .T. ) ;
#60409=VERTEX_POINT ( 'NONE', #33985 ) ;
#60410=CARTESIAN_POINT ( 'NONE',  ( 4.023698184114456566, -11.66186481527757479, 32.95055677023626117 ) ) ;
#60411=CARTESIAN_POINT ( 'NONE',  ( -5.076923076923197442, -2.892918686052165622, 31.69288490824153470 ) ) ;
#60412=CARTESIAN_POINT ( 'NONE',  ( 3.361559671736181976, -5.496552790871119143, 34.60292014791297532 ) ) ;
#60413=CARTESIAN_POINT ( 'NONE',  ( 1.607395053593452028, -6.717445702608402236, 34.94155399931962336 ) ) ;
#60415=CARTESIAN_POINT ( 'NONE',  ( -11.31545018684868964, -9.086983370893049639, 34.49168942202179267 ) ) ;
#60416=EDGE_LOOP ( 'NONE', ( #78479, #26617, #54083, #52274 ) ) ;
#60419=CARTESIAN_POINT ( 'NONE',  ( -18.00000000000000000, -13.83693561022309915, 32.05645593858272235 ) ) ;
#60422=CARTESIAN_POINT ( 'NONE',  ( -2.307692307692305711, -8.973038597847269315, 34.52809138561121927 ) ) ;
#60423=CARTESIAN_POINT ( 'NONE',  ( 1.161736702186739745, -7.630691491037286056, 34.74850469731152458 ) ) ;
#60425=CARTESIAN_POINT ( 'NONE',  ( 2.557746727605763049, -2.544122305571458575, 31.48381861865057729 ) ) ;
#60426=CARTESIAN_POINT ( 'NONE',  ( -5.143005456283212595, -10.67929555188718460, 33.92786785259543336 ) ) ;
#60427=CARTESIAN_POINT ( 'NONE',  ( -0.7115151924808159611, -12.41269422305637171, 30.68257228309993323 ) ) ;
#60428=EDGE_CURVE ( 'NONE', #22275, #78937, #7410, .T. ) ;
#60430=VERTEX_POINT ( 'NONE', #33555 ) ;
#60431=CARTESIAN_POINT ( 'NONE',  ( -7.173100147298380413, -10.92453946501458439, 33.72985991061850086 ) ) ;
#60432=LINE ( 'NONE', #40182, #16025 ) ;
#60434=LINE ( 'NONE', #53678, #34801 ) ;
#60435=VERTEX_POINT ( 'NONE', #61894 ) ;
#60436=CARTESIAN_POINT ( 'NONE',  ( 8.096099255531887806, -12.07971442181321997, 32.31769673815850297 ) ) ;
#60437=CARTESIAN_POINT ( 'NONE',  ( 2.980769230769221956, -2.499999999999999556, 29.81609845454692120 ) ) ;
#60438=CARTESIAN_POINT ( 'NONE',  ( 10.68063975489745410, -5.094484230520773593, 34.41647553114626845 ) ) ;
#60439=EDGE_CURVE ( 'NONE', #50355, #52314, #35907, .T. ) ;
#60440=CARTESIAN_POINT ( 'NONE',  ( -16.15384615384615330, -3.050289026998446396, 32.03036669348365706 ) ) ;
#60441=CARTESIAN_POINT ( 'NONE',  ( 17.75002325595141173, -2.544273027872574477, 31.48422191005632698 ) ) ;
#60442=ORIENTED_EDGE ( 'NONE', *, *, #36642, .F. ) ;
#60443=CARTESIAN_POINT ( 'NONE',  ( 5.999999999999880096, -3.835265460704628371, 33.15142922262033665 ) ) ;
#60444=CARTESIAN_POINT ( 'NONE',  ( 17.32697738856138869, -5.728107161865375829, 34.42597550085002922 ) ) ;
#60445=DIRECTION ( 'NONE',  ( 0.000000000000000000, 0.000000000000000000, 1.000000000000000000 ) ) ;
#60446=AXIS2_PLACEMENT_3D ( 'NONE', #68296, #81823, #61974 ) ;
#60447=ORIENTED_EDGE ( 'NONE', *, *, #44870, .F. ) ;
#60448=CARTESIAN_POINT ( 'NONE',  ( 12.39626846098214230, -2.657715359629088780, 31.77849191805832874 ) ) ;
#60449=EDGE_CURVE ( 'NONE', #23968, #86388, #52012, .T. ) ;
#60450=B_SPLINE_CURVE_WITH_KNOTS ( 'NONE', 3,
 ( #86933, #73390, #62516, #48562, #42276, #13455, #54894, #53999, #88264, #7596 ),
 .UNSPECIFIED., .F., .F.,
 ( 4, 2, 2, 2, 4 ),
 ( 0.0007817246256747516176, 0.0009771112852218965736, 0.001172497944769041421, 0.001367884604316186269, 0.001563271263863331333 ),
 .UNSPECIFIED. ) ;
#60451=EDGE_LOOP ( 'NONE', ( #59903, #25812 ) ) ;
#60452=FACE_OUTER_BOUND ( 'NONE', #15858, .T. ) ;
#60454=CARTESIAN_POINT ( 'NONE',  ( -1.384615384615383471, -13.20930481340135110, 34.54067556320372745 ) ) ;
#60455=ORIENTED_EDGE ( 'NONE', *, *, #47071, .F. ) ;
#60457=CARTESIAN_POINT ( 'NONE',  ( 0.4615384615384611200, -4.098570777380720287, 33.41473453929634729 ) ) ;
#60458=CARTESIAN_POINT ( 'NONE',  ( -11.53846153846153655, -13.88283147151868846, 33.14645433367849847 ) ) ;
#60460=CARTESIAN_POINT ( 'NONE',  ( -7.846153846153844924, -4.661471528628507777, 34.16647553114623292 ) ) ;
#60461=CARTESIAN_POINT ( 'NONE',  ( -0.5916864312701586304, -11.66186481527757479, 32.95055677023626117 ) ) ;
#60462=EDGE_CURVE ( 'NONE', #88588, #34081, #83522, .T. ) ;
#60463=ORIENTED_EDGE ( 'NONE', *, *, #40838, .F. ) ;
#60464=B_SPLINE_CURVE_WITH_KNOTS ( 'NONE', 3,
 ( #62047, #19295, #40024, #81894, #26496, #26053, #81452, #13418, #19736, #14304 ),
 .UNSPECIFIED., .F., .F.,
 ( 4, 2, 2, 2, 4 ),
 ( 0.000000000000000000, 0.0001954339857564091278, 0.0003908679715128182556, 0.0005863019572692274375, 0.0007817359430256365111 ),
 .UNSPECIFIED. ) ;
#60465=VECTOR ( 'NONE', #45314, 1000.000000000000114 ) ;
#60466=FACE_OUTER_BOUND ( 'NONE', #62678, .T. ) ;
#60467=ORIENTED_EDGE ( 'NONE', *, *, #87282, .F. ) ;
#60468=CARTESIAN_POINT ( 'NONE',  ( 5.207448515156718472, -11.66157788607254275, 32.95092075102925833 ) ) ;
#60469=CARTESIAN_POINT ( 'NONE',  ( -10.48459417441766561, -9.929761469519743144, 34.40412654351204225 ) ) ;
#60470=VECTOR ( 'NONE', #66171, 999.9999999999998863 ) ;
#60471=AXIS2_PLACEMENT_3D ( 'NONE', #15164, #71416, #51130 ) ;
#60472=CARTESIAN_POINT ( 'NONE',  ( 18.22301284409339672, -6.460100341425561332, 34.89618726649961644 ) ) ;
#60473=CARTESIAN_POINT ( 'NONE',  ( -6.923076923076922462, -5.557115091759785130, 34.35708131394839171 ) ) ;
#60474=DIRECTION ( 'NONE',  ( -0.000000000000000000, 1.000000000000000000, 3.491481338843133355E-15 ) ) ;
#60475=AXIS2_PLACEMENT_3D ( 'NONE', #24042, #10545, #38914 ) ;
#60477=CIRCLE ( 'NONE', #15937, 0.2500000000000002220 ) ;
#60478=EDGE_LOOP ( 'NONE', ( #80789, #61738 ) ) ;
#60479=ORIENTED_EDGE ( 'NONE', *, *, #24561, .F. ) ;
#60481=EDGE_CURVE ( 'NONE', #68101, #17484, #59510, .T. ) ;
#60482=EDGE_CURVE ( 'NONE', #72207, #64027, #47716, .T. ) ;
#60484=DIRECTION ( 'NONE',  ( -0.000000000000000000, 0.000000000000000000, 1.000000000000000000 ) ) ;
#60485=CARTESIAN_POINT ( 'NONE',  ( -6.130691466667556710, -12.38065189839062263, 30.83690757178629482 ) ) ;
#60486=CARTESIAN_POINT ( 'NONE',  ( -15.48074596171158390, -10.66389620160130036, 33.62221079203477103 ) ) ;
#60487=EDGE_CURVE ( 'NONE', #14315, #23009, #84264, .T. ) ;
#60488=CARTESIAN_POINT ( 'NONE',  ( 5.011653076366756387, -11.67786785259541027, 32.92929555188721480 ) ) ;
#60489=CARTESIAN_POINT ( 'NONE',  ( 3.361559671736181976, -9.084667340241226796, 34.75534355489798344 ) ) ;
#60490=CARTESIAN_POINT ( 'NONE',  ( -0.5922299282060186076, -11.71456829005830080, 32.44064028649416542 ) ) ;
#60491=DIRECTION ( 'NONE',  ( -0.000000000000000000, 0.6427876096865404731, -0.7660444431189770143 ) ) ;
#60492=LINE ( 'NONE', #72225, #5891 ) ;
#60493=ORIENTED_EDGE ( 'NONE', *, *, #6214, .F. ) ;
#60494=EDGE_LOOP ( 'NONE', ( #53157, #87300 ) ) ;
#60495=B_SPLINE_CURVE_WITH_KNOTS ( 'NONE', 3,
 ( #29282, #75249, #7678, #75676, #34703, #68920, #49093, #35139, #62167, #54972 ),
 .UNSPECIFIED., .F., .F.,
 ( 4, 2, 2, 2, 4 ),
 ( 0.000000000000000000, 0.0001954339857564098054, 0.0003908679715128196108, 0.0005863019572692293891, 0.0007817359430256392216 ),
 .UNSPECIFIED. ) ;
#60496=VERTEX_POINT ( 'NONE', #71304 ) ;
#60497=CARTESIAN_POINT ( 'NONE',  ( -1.634592115557738090, -11.28823185664190376, 33.01397839955799896 ) ) ;
#60498=ORIENTED_EDGE ( 'NONE', *, *, #81873, .T. ) ;
#60500=CARTESIAN_POINT ( 'NONE',  ( -7.846153846153844924, -9.058645607665452459, 34.76329471203371924 ) ) ;
#60501=B_SPLINE_CURVE_WITH_KNOTS ( 'NONE', 3,
 ( #58427, #64743, #43596, #23321, #86838, #3491, #85043, #3046, #72395, #2601 ),
 .UNSPECIFIED., .F., .F.,
 ( 4, 2, 2, 2, 4 ),
 ( 0.0007817246256747470640, 0.0009771112852218896347, 0.001172497944769032314, 0.001367884604316174993, 0.001563271263863317455 ),
 .UNSPECIFIED. ) ;
#60502=B_SPLINE_CURVE_WITH_KNOTS ( 'NONE', 3,
 ( #59082, #32500, #46466, #12237, #45570, #25753, #52768, #86580, #80258, #88367 ),
 .UNSPECIFIED., .F., .F.,
 ( 4, 2, 2, 2, 4 ),
 ( 0.000000000000000000, 0.0001954339857564091549, 0.0003908679715128183098, 0.0005863019572692274375, 0.0007817359430256366195 ),
 .UNSPECIFIED. ) ;
#60503=CARTESIAN_POINT ( 'NONE',  ( 11.47319109250076608, -3.835265460703609186, 33.15142922261924241 ) ) ;
#60504=DIRECTION ( 'NONE',  ( -0.000000000000000000, 0.1736481776669307198, -0.9848077530122080203 ) ) ;
#60505=FACE_BOUND ( 'NONE', #50119, .T. ) ;
#60507=EDGE_LOOP ( 'NONE', ( #22749, #60779, #9905, #21154 ) ) ;
#60508=DIRECTION ( 'NONE',  ( -0.000000000000000000, -0.000000000000000000, -1.000000000000000000 ) ) ;
#60509=ORIENTED_EDGE ( 'NONE', *, *, #2107, .T. ) ;
#60510=FACE_BOUND ( 'NONE', #62285, .T. ) ;
#60511=CARTESIAN_POINT ( 'NONE',  ( 9.823098133274648092, -5.496552790871120031, 34.60292014791297532 ) ) ;
#60512=CARTESIAN_POINT ( 'NONE',  ( 0.4615384615384611200, -7.500000000000001776, 35.04278698407183867 ) ) ;
#60513=ORIENTED_EDGE ( 'NONE', *, *, #29287, .F. ) ;
#60514=CARTESIAN_POINT ( 'NONE',  ( -23.00000000000000000, -4.249999999999998224, 27.25000000000000000 ) ) ;
#60515=CARTESIAN_POINT ( 'NONE',  ( 9.019230769230832223, -7.434744860731433924, 35.00000000000000711 ) ) ;
#60516=CARTESIAN_POINT ( 'NONE',  ( -4.853496678008289322, -7.630147987733840509, 34.99859428049665411 ) ) ;
#60517=ORIENTED_EDGE ( 'NONE', *, *, #44940, .T. ) ;
#60518=DIRECTION ( 'NONE',  ( -0.000000000000000000, -0.9848077530122085754, -0.1736481776669273613 ) ) ;
#60519=CARTESIAN_POINT ( 'NONE',  ( 16.15384615384615330, -1.629998284177014645, 34.34916445242399163 ) ) ;
#60520=DIRECTION ( 'NONE',  ( -0.000000000000000000, 0.6427876096865404731, -0.7660444431189771253 ) ) ;
#60521=ORIENTED_EDGE ( 'NONE', *, *, #60157, .F. ) ;
#60522=CARTESIAN_POINT ( 'NONE',  ( 13.38461538461538680, -6.435427911321262684, 35.78748833219616898 ) ) ;
#60523=CARTESIAN_POINT ( 'NONE',  ( -15.90379173393269951, -10.06805714834173138, 34.32951233291982618 ) ) ;
#60524=EDGE_LOOP ( 'NONE', ( #81254, #22013 ) ) ;
#60525=DIRECTION ( 'NONE',  ( 0.000000000000000000, 0.3420201433256610524, 0.9396926207859113145 ) ) ;
#60526=CARTESIAN_POINT ( 'NONE',  ( -0.4615384615384611200, -13.53365097954675988, 30.81389545987213552 ) ) ;
#60527=CARTESIAN_POINT ( 'NONE',  ( -8.069080805060693251, -12.38737895849757820, 31.66785238281580206 ) ) ;
#60528=CARTESIAN_POINT ( 'NONE',  ( -0.2115384615370257404, -7.500000000000155431, 34.75000000000007105 ) ) ;
#60529=DIRECTION ( 'NONE',  ( -0.000000000000000000, -0.000000000000000000, -1.000000000000000000 ) ) ;
#60530=CARTESIAN_POINT ( 'NONE',  ( 17.20771351789002424, -4.684288915650984819, 34.18129842949671371 ) ) ;
#60531=CARTESIAN_POINT ( 'NONE',  ( 0.5920638997721034968, -11.66157788607254275, 32.95092075102925833 ) ) ;
#60533=VECTOR ( 'NONE', #13000, 1000.000000000000227 ) ;
#60534=CARTESIAN_POINT ( 'NONE',  ( -16.15384615384615330, -11.69971097300155272, 32.46337939537588113 ) ) ;
#60537=ORIENTED_EDGE ( 'NONE', *, *, #87309, .T. ) ;
#60538=CARTESIAN_POINT ( 'NONE',  ( 4.946232473812769648, -6.369640206132550553, 34.87707690430378449 ) ) ;
#60541=ORIENTED_EDGE ( 'NONE', *, *, #27797, .F. ) ;
#60542=CARTESIAN_POINT ( 'NONE',  ( -3.099978789802280144, -9.084667340241226796, 34.75534355489798344 ) ) ;
#60544=CARTESIAN_POINT ( 'NONE',  ( -14.30769230769230660, -13.57706302396349152, 30.56769352161908060 ) ) ;
#60546=CARTESIAN_POINT ( 'NONE',  ( 17.77707304109314634, -4.762599654559227069, 34.23009711892697737 ) ) ;
#60547=CARTESIAN_POINT ( 'NONE',  ( -18.25002322422145440, -12.07920672191015754, 32.31858351112115457 ) ) ;
#60548=CARTESIAN_POINT ( 'NONE',  ( -0.4615384615384611200, -5.557115091759785130, 34.35708131394839171 ) ) ;
#60551=CARTESIAN_POINT ( 'NONE',  ( 9.692307692307695177, -1.117168528481311540, 33.14645433367849847 ) ) ;
#60553=ADVANCED_FACE ( 'NONE', ( #9612 ), #37074, .F. ) ;
#60555=CARTESIAN_POINT ( 'NONE',  ( 10.61538461538461675, -12.34228464037088635, 31.77849191805839268 ) ) ;
#60556=CARTESIAN_POINT ( 'NONE',  ( -17.86920955903304886, -2.295524264805589354, 30.44142389570983198 ) ) ;
#60557=CARTESIAN_POINT ( 'NONE',  ( -2.307692307692427391, -4.481592998941358097, 33.73612834414048933 ) ) ;
#60558=VERTEX_POINT ( 'NONE', #24894 ) ;
#60559=VERTEX_POINT ( 'NONE', #5077 ) ;
#60560=CARTESIAN_POINT ( 'NONE',  ( 14.05766908347085042, -8.475808217655753651, 34.90892951860618609 ) ) ;
#60561=DIRECTION ( 'NONE',  ( -0.000000000000000000, -0.7660444431189791237, -0.6427876096865379196 ) ) ;
#60563=DIRECTION ( 'NONE',  ( 0.000000000000000000, 0.1736481776669267785, -0.9848077530122087975 ) ) ;
#60565=CARTESIAN_POINT ( 'NONE',  ( 14.30769230769218581, -3.643525952248795718, 33.31231777344771672 ) ) ;
#60566=CARTESIAN_POINT ( 'NONE',  ( -39.05038313613820122, -12.50000000000000000, 29.75000000000000355 ) ) ;
#60567=VECTOR ( 'NONE', #40104, 1000.000000000000227 ) ;
#60568=EDGE_CURVE ( 'NONE', #44606, #31297, #30765, .T. ) ;
#60569=ORIENTED_EDGE ( 'NONE', *, *, #82301, .F. ) ;
#60570=CARTESIAN_POINT ( 'NONE',  ( 1.161130440891438020, -5.113361153441934093, 34.14387501736622710 ) ) ;
#60571=ORIENTED_EDGE ( 'NONE', *, *, #51457, .T. ) ;
#60573=ORIENTED_EDGE ( 'NONE', *, *, #55742, .F. ) ;
#60574=CARTESIAN_POINT ( 'NONE',  ( 5.299702618191483694, -8.496831190052096971, 34.64984203495476578 ) ) ;
#60575=CARTESIAN_POINT ( 'NONE',  ( -2.557669051740897537, -9.234221910056348293, 34.70572697212741531 ) ) ;
#60576=CARTESIAN_POINT ( 'NONE',  ( 14.05766907039934210, -5.056417327199099532, 34.11270091957321426 ) ) ;
#60578=DIRECTION ( 'NONE',  ( -0.000000000000000000, -0.5000000000000009992, -0.8660254037844380415 ) ) ;
#60580=VERTEX_POINT ( 'NONE', #58680 ) ;
#60582=EDGE_CURVE ( 'NONE', #81377, #22716, #39105, .T. ) ;
#60583=ORIENTED_EDGE ( 'NONE', *, *, #4318, .T. ) ;
#60584=EDGE_LOOP ( 'NONE', ( #40887, #73940, #42115, #5109 ) ) ;
#60585=AXIS2_PLACEMENT_3D ( 'NONE', #50552, #10016, #31167 ) ;
#60586=CARTESIAN_POINT ( 'NONE',  ( 5.934729554039225974, -2.625532179533445198, 30.86335684631481513 ) ) ;
#60588=CARTESIAN_POINT ( 'NONE',  ( 15.90384615384615330, -2.249999999999998668, 29.75000000000000355 ) ) ;
#60590=CARTESIAN_POINT ( 'NONE',  ( -15.48079246806219267, -11.37209801155882971, 32.91403422569032955 ) ) ;
#60591=CARTESIAN_POINT ( 'NONE',  ( 12.23805353697412812, -3.019605429927184392, 32.48692288466676814 ) ) ;
#60592=ORIENTED_EDGE ( 'NONE', *, *, #3523, .T. ) ;
#60593=ORIENTED_EDGE ( 'NONE', *, *, #29659, .F. ) ;
#60594=AXIS2_PLACEMENT_3D ( 'NONE', #78710, #52115, #72829 ) ;
#60595=CARTESIAN_POINT ( 'NONE',  ( 17.20771488474786892, -12.38066358083363738, 30.83685684665853444 ) ) ;
#60596=VERTEX_POINT ( 'NONE', #72642 ) ;
#60597=DIRECTION ( 'NONE',  ( -0.000000000000000000, -0.9848077530122085754, -0.1736481776669273613 ) ) ;
#60598=CARTESIAN_POINT ( 'NONE',  ( 6.673076923076925127, -7.500000000000001776, 34.75000000000000000 ) ) ;
#60600=ORIENTED_EDGE ( 'NONE', *, *, #24683, .T. ) ;
#60601=CARTESIAN_POINT ( 'NONE',  ( 7.911408985666682270, -4.320704448112861584, 33.92786785259548310 ) ) ;
#60602=VERTEX_POINT ( 'NONE', #66779 ) ;
#60604=CARTESIAN_POINT ( 'NONE',  ( 14.30769230769218581, -12.51329471203414379, 31.30864560766407578 ) ) ;
#60605=B_SPLINE_CURVE_WITH_KNOTS ( 'NONE', 3,
 ( #57967, #36811, #49880, #22849, #50313, #29192, #1702, #44005, #3014, #42697 ),
 .UNSPECIFIED., .F., .F.,
 ( 4, 2, 2, 2, 4 ),
 ( 0.0007817246256747461966, 0.0009771112852218892010, 0.001172497944769032314, 0.001367884604316175427, 0.001563271263863318323 ),
 .UNSPECIFIED. ) ;
#60606=CARTESIAN_POINT ( 'NONE',  ( -2.557692307692305267, -2.249999999999998668, 29.75000000000000355 ) ) ;
#60609=VERTEX_POINT ( 'NONE', #25347 ) ;
#60612=DIRECTION ( 'NONE',  ( -0.000000000000000000, -0.9848077530122086864, -0.1736481776669273613 ) ) ;
#60614=B_SPLINE_CURVE_WITH_KNOTS ( 'NONE', 3,
 ( #25977, #73281, #88599, #25538, #61090, #53441, #38607, #4827, #33628, #52552 ),
 .UNSPECIFIED., .F., .F.,
 ( 4, 2, 2, 2, 4 ),
 ( 0.000000000000000000, 0.0001954339857564054144, 0.0003908679715128108288, 0.0005863019572692162703, 0.0007817359430256216575 ),
 .UNSPECIFIED. ) ;
#60615=AXIS2_PLACEMENT_3D ( 'NONE', #53637, #12657, #5902 ) ;
#60616=DIRECTION ( 'NONE',  ( -0.000000000000000000, 0.5000000000000009992, -0.8660254037844380415 ) ) ;
#60617=CARTESIAN_POINT ( 'NONE',  ( -3.930833309752758797, -10.01129605718032778, 34.36064277460058491 ) ) ;
#60618=CARTESIAN_POINT ( 'NONE',  ( -16.28440606745951413, -2.254533558242299396, 29.97296025877828640 ) ) ;
#60619=FACE_OUTER_BOUND ( 'NONE', #20502, .T. ) ;
#60620=DIRECTION ( 'NONE',  ( -0.000000000000000000, 1.000000000000000000, 3.491481338843133355E-15 ) ) ;
#60621=FACE_BOUND ( 'NONE', #75611, .T. ) ;
#60622=CARTESIAN_POINT ( 'NONE',  ( -7.146561847641256016, -12.47654668319379567, 31.42292124445336654 ) ) ;
#60623=DIRECTION ( 'NONE',  ( 1.000000000000000000, 0.000000000000000000, 0.000000000000000000 ) ) ;
#60624=B_SPLINE_CURVE_WITH_KNOTS ( 'NONE', 3,
 ( #89176, #31658, #11839, #20257, #39314, #37971, #6731, #58673, #27456, #32537 ),
 .UNSPECIFIED., .F., .F.,
 ( 4, 2, 2, 2, 4 ),
 ( 0.0007817246256747484735, 0.0009771112852218931041, 0.001172497944769037735, 0.001367884604316182365, 0.001563271263863326996 ),
 .UNSPECIFIED. ) ;
#60625=CARTESIAN_POINT ( 'NONE',  ( -15.09997878980228059, -4.684288915650983043, 34.18129842949671371 ) ) ;
#60626=CARTESIAN_POINT ( 'NONE',  ( -8.519285250882624894, -11.86320923018887541, 32.19269448109604781 ) ) ;
#60627=CARTESIAN_POINT ( 'NONE',  ( -9.692307692307691624, -10.51840700105979565, 33.73612834413961536 ) ) ;
#60629=LINE ( 'NONE', #11119, #79316 ) ;
#60631=ORIENTED_EDGE ( 'NONE', *, *, #10967, .F. ) ;
#60632=CARTESIAN_POINT ( 'NONE',  ( -12.71153846153846345, -7.433932668274256805, 35.00000000000000711 ) ) ;
#60633=ORIENTED_EDGE ( 'NONE', *, *, #70817, .T. ) ;
#60634=CARTESIAN_POINT ( 'NONE',  ( 0.3962680155776852065, -6.879047030191174805, 34.71129190930000163 ) ) ;
#60635=ORIENTED_EDGE ( 'NONE', *, *, #68694, .T. ) ;
#60636=CARTESIAN_POINT ( 'NONE',  ( 7.912221179503920787, -9.905515769479276145, 34.41647553114623292 ) ) ;
#60637=CARTESIAN_POINT ( 'NONE',  ( 2.307692307692186251, -12.16647553114689728, 32.15551576947799362 ) ) ;
#60640=CARTESIAN_POINT ( 'NONE',  ( 17.07692307692307665, -12.62096338111211580, 30.90682066428153263 ) ) ;
#60641=CARTESIAN_POINT ( 'NONE',  ( 5.076923076922953193, -12.16647553114689728, 32.15551576947799362 ) ) ;
#60643=ADVANCED_FACE ( 'NONE', ( #86627 ), #17252, .F. ) ;
#60644=CARTESIAN_POINT ( 'NONE',  ( 4.153846153846154188, -10.51840700105979565, 33.73612834413961536 ) ) ;
#60645=CARTESIAN_POINT ( 'NONE',  ( 4.853996859406927378, -4.887634598454295265, 34.01352882383564946 ) ) ;
#60646=CARTESIAN_POINT ( 'NONE',  ( 7.976679547917413515, -11.93748526763465279, 32.05452791011430946 ) ) ;
#60648=CARTESIAN_POINT ( 'NONE',  ( -1.161602540521988747, -6.460100341425561332, 34.89618726649961644 ) ) ;
#60650=EDGE_CURVE ( 'NONE', #15793, #39836, #58236, .T. ) ;
#60652=CARTESIAN_POINT ( 'NONE',  ( 2.980769230769232170, -7.433932668274255029, 35.00000000000000711 ) ) ;
#60653=CARTESIAN_POINT ( 'NONE',  ( -11.28840722682322628, -10.66356715214248396, 33.62249196103329751 ) ) ;
#60654=EDGE_LOOP ( 'NONE', ( #23050, #44771, #7627, #6790 ) ) ;
#60655=CARTESIAN_POINT ( 'NONE',  ( 6.673076923076925127, -7.500000000000001776, 35.00000000000000000 ) ) ;
#60656=FACE_OUTER_BOUND ( 'NONE', #83547, .T. ) ;
#60658=AXIS2_PLACEMENT_3D ( 'NONE', #62923, #84558, #56185 ) ;
#60659=EDGE_CURVE ( 'NONE', #73792, #52382, #87388, .T. ) ;
#60660=DIRECTION ( 'NONE',  ( -0.000000000000000000, 0.9848077530122086864, -0.1736481776669273891 ) ) ;
#60661=CARTESIAN_POINT ( 'NONE',  ( 5.207713517890026012, -6.369690395747422684, 34.87708834333098196 ) ) ;
#60662=ORIENTED_EDGE ( 'NONE', *, *, #88611, .T. ) ;
#60663=LINE ( 'NONE', #81399, #57217 ) ;
#60664=CARTESIAN_POINT ( 'NONE',  ( 9.562159722575998444, -12.70455904226513866, 30.44083106164009322 ) ) ;
#60666=ORIENTED_EDGE ( 'NONE', *, *, #75764, .T. ) ;
#60668=EDGE_CURVE ( 'NONE', #49648, #32624, #80755, .T. ) ;
#60669=CARTESIAN_POINT ( 'NONE',  ( 15.23076923076910916, -5.941354392335915335, 34.76329471203413846 ) ) ;
#60671=B_SPLINE_CURVE_WITH_KNOTS ( 'NONE', 3,
 ( #48369, #25558, #60222, #80965, #46716, #75848, #69092, #7399, #34855, #30319 ),
 .UNSPECIFIED., .F., .F.,
 ( 4, 2, 2, 2, 4 ),
 ( 0.000000000000000000, 0.0001954339857564078809, 0.0003908679715128157619, 0.0005863019572692236428, 0.0007817359430256315238 ),
 .UNSPECIFIED. ) ;
#60672=B_SPLINE_CURVE_WITH_KNOTS ( 'NONE', 3,
 ( #59381, #86884, #73344, #78759, #10307, #3538 ),
 .UNSPECIFIED., .F., .F.,
 ( 4, 2, 4 ),
 ( 0.000000000000000000, 0.0001954784845028908113, 0.0003909569690057816227 ),
 .UNSPECIFIED. ) ;
#60673=LINE ( 'NONE', #18809, #14105 ) ;
#60674=VERTEX_POINT ( 'NONE', #18599 ) ;
#60675=DIRECTION ( 'NONE',  ( 0.000000000000000000, 0.7660444431189822323, -0.6427876096865344779 ) ) ;
#60676=CARTESIAN_POINT ( 'NONE',  ( -13.45069879557126669, -11.69971097300155272, 32.46337939537587403 ) ) ;
#60677=DIRECTION ( 'NONE',  ( -0.000000000000000000, 1.000000000000000000, -0.000000000000000000 ) ) ;
#60678=EDGE_CURVE ( 'NONE', #32941, #57045, #35848, .T. ) ;
#60679=ORIENTED_EDGE ( 'NONE', *, *, #32625, .T. ) ;
#60680=ORIENTED_EDGE ( 'NONE', *, *, #25204, .T. ) ;
#60681=EDGE_LOOP ( 'NONE', ( #7705, #386 ) ) ;
#60682=EDGE_LOOP ( 'NONE', ( #37302, #54324, #10435, #62731 ) ) ;
#60683=CARTESIAN_POINT ( 'NONE',  ( -9.822454901745910405, -2.882441371585227508, 31.66841991370172238 ) ) ;
#60684=CARTESIAN_POINT ( 'NONE',  ( -2.057637996053991447, -5.728107161865378494, 34.42597550085002922 ) ) ;
#60685=CARTESIAN_POINT ( 'NONE',  ( -7.911423846710166075, -12.70778746994557551, 30.41441678777548319 ) ) ;
#60687=CARTESIAN_POINT ( 'NONE',  ( -16.82697755857493505, -5.057305518903949526, 34.11320923018887896 ) ) ;
#60689=ADVANCED_FACE ( 'NONE', ( #65876 ), #43215, .F. ) ;
#60690=EDGE_LOOP ( 'NONE', ( #15507, #7205 ) ) ;
#60691=ORIENTED_EDGE ( 'NONE', *, *, #13046, .T. ) ;
#60692=CARTESIAN_POINT ( 'NONE',  ( -13.38461538461538325, -11.69971097300155272, 32.46337939537588113 ) ) ;
#60693=EDGE_CURVE ( 'NONE', #43000, #42649, #23373, .T. ) ;
#60694=VERTEX_POINT ( 'NONE', #29709 ) ;
#60695=FACE_OUTER_BOUND ( 'NONE', #29803, .T. ) ;
#60696=LINE ( 'NONE', #88205, #83949 ) ;
#60697=EDGE_CURVE ( 'NONE', #16683, #32754, #3984, .T. ) ;
#60698=EDGE_CURVE ( 'NONE', #51973, #20058, #20680, .T. ) ;
#60699=B_SPLINE_CURVE_WITH_KNOTS ( 'NONE', 3,
 ( #54050, #32457, #59926, #39680, #27034, #45965 ),
 .UNSPECIFIED., .F., .F.,
 ( 4, 2, 4 ),
 ( 1.084202172485504434E-19, 0.0001954784845028911637, 0.0003909569690057822190 ),
 .UNSPECIFIED. ) ;
#60701=CARTESIAN_POINT ( 'NONE',  ( -5.749945688361685292, -4.235687564193446164, 33.53795663066793509 ) ) ;
#60702=ORIENTED_EDGE ( 'NONE', *, *, #86940, .T. ) ;
#60703=VERTEX_POINT ( 'NONE', #37328 ) ;
#60704=ORIENTED_EDGE ( 'NONE', *, *, #80829, .F. ) ;
#60705=CARTESIAN_POINT ( 'NONE',  ( 14.53070515178570332, -10.77377354290276124, 33.85451476688484718 ) ) ;
#60706=CARTESIAN_POINT ( 'NONE',  ( -2.307692307692305711, -2.721908614388771852, 31.22303859784724978 ) ) ;
#60707=VERTEX_POINT ( 'NONE', #56727 ) ;
#60708=CARTESIAN_POINT ( 'NONE',  ( 3.100622021331010725, -11.93770438780619259, 32.05411857736982029 ) ) ;
#60709=B_SPLINE_CURVE_WITH_KNOTS ( 'NONE', 3,
 ( #738, #19679, #26884, #14253, #67427, #41732, #28200, #40845, #68311, #55671 ),
 .UNSPECIFIED., .F., .F.,
 ( 4, 2, 2, 2, 4 ),
 ( 0.0007817246256747525934, 0.0009771112852218970073, 0.001172497944769041204, 0.001367884604316185401, 0.001563271263863329815 ),
 .UNSPECIFIED. ) ;
#60710=FACE_OUTER_BOUND ( 'NONE', #47627, .T. ) ;
#60712=CARTESIAN_POINT ( 'NONE',  ( -11.28840711854808632, -4.074993327901527351, 33.72946981652012255 ) ) ;
#60713=CARTESIAN_POINT ( 'NONE',  ( 8.900022577055556994, -12.38066358083363738, 30.83685684665853444 ) ) ;
#60714=CARTESIAN_POINT ( 'NONE',  ( 0.2115152373170033906, -9.356822207818506598, 34.66110646841856635 ) ) ;
#60715=FACE_BOUND ( 'NONE', #45647, .T. ) ;
#60716=CARTESIAN_POINT ( 'NONE',  ( -15.45425415533356350, -8.539481045369596401, 34.89627647299170832 ) ) ;
#60717=CARTESIAN_POINT ( 'NONE',  ( -1.253823576790597638, -11.71459661697925903, 32.44059661609676937 ) ) ;
#60718=AXIS2_PLACEMENT_3D ( 'NONE', #72809, #44889, #37695 ) ;
#60719=DIRECTION ( 'NONE',  ( -0.000000000000000000, -0.8660254037844399289, -0.4999999999999980016 ) ) ;
#60720=DIRECTION ( 'NONE',  ( -0.000000000000000000, 0.3420201433256694901, -0.9396926207859082059 ) ) ;
#60721=CARTESIAN_POINT ( 'NONE',  ( 6.699591998512590685, -10.97335522853832579, 33.68706563782419749 ) ) ;
#60722=VECTOR ( 'NONE', #72864, 1000.000000000000000 ) ;
#60724=DIRECTION ( 'NONE',  ( 0.000000000000000000, 0.8660254037844377084, 0.5000000000000015543 ) ) ;
#60725=ORIENTED_EDGE ( 'NONE', *, *, #64523, .T. ) ;
#60726=CARTESIAN_POINT ( 'NONE',  ( -16.37667284632515674, -7.369208160676171460, 34.74850200257122879 ) ) ;
#60727=DIRECTION ( 'NONE',  ( 0.000000000000000000, 0.1736481776669275834, 0.9848077530122086864 ) ) ;
#60728=ORIENTED_EDGE ( 'NONE', *, *, #88529, .T. ) ;
#60729=VERTEX_POINT ( 'NONE', #15752 ) ;
#60730=CYLINDRICAL_SURFACE ( 'NONE', #69376, 0.2499999999999997502 ) ;
#60731=CARTESIAN_POINT ( 'NONE',  ( 16.08857615328984281, -2.379036618887870436, 30.90682066428148644 ) ) ;
#60732=CARTESIAN_POINT ( 'NONE',  ( -14.98076923076916778, -7.434744429011176159, 34.75000000000000711 ) ) ;
#60733=ORIENTED_EDGE ( 'NONE', *, *, #31684, .T. ) ;
#60735=CARTESIAN_POINT ( 'NONE',  ( -15.90379184220783948, -11.28795663066794575, 33.01431243580653785 ) ) ;
#60737=FACE_BOUND ( 'NONE', #25350, .T. ) ;
#60738=CARTESIAN_POINT ( 'NONE',  ( -14.53117723225664015, -4.225889041578353655, 33.85425143139329407 ) ) ;
#60739=CARTESIAN_POINT ( 'NONE',  ( 5.934729999443682402, -6.835583212224499938, 34.95778746994557906 ) ) ;
#60740=CARTESIAN_POINT ( 'NONE',  ( 8.069165197766697162, -9.086983370893049639, 34.49168942202179267 ) ) ;
#60741=CARTESIAN_POINT ( 'NONE',  ( 2.438484115517094430, -4.809403383903226192, 33.96459661697924304 ) ) ;
#60743=CARTESIAN_POINT ( 'NONE',  ( -14.55769230769230660, -7.500000000000001776, 35.00000000000000000 ) ) ;
#60746=ORIENTED_EDGE ( 'NONE', *, *, #82400, .T. ) ;
#60747=ORIENTED_EDGE ( 'NONE', *, *, #1187, .F. ) ;
#60748=CARTESIAN_POINT ( 'NONE',  ( 4.946232473812770536, -10.70098750199973203, 33.91152734681376302 ) ) ;
#60749=CARTESIAN_POINT ( 'NONE',  ( -4.219929564802033184, -12.37446782046654192, 30.86335684631486487 ) ) ;
#60751=CARTESIAN_POINT ( 'NONE',  ( 17.07692307692339284, -2.255955759149395501, 30.00000000000324363 ) ) ;
#60752=CARTESIAN_POINT ( 'NONE',  ( 5.076923076923075762, -1.466349020453238561, 30.81389545987213907 ) ) ;
#60754=EDGE_CURVE ( 'NONE', #73212, #52584, #72007, .T. ) ;
#60755=CARTESIAN_POINT ( 'NONE',  ( -1.515305987725693138, -3.957541250942359756, 33.62499894934981626 ) ) ;
#60757=LINE ( 'NONE', #79705, #77523 ) ;
#60758=CARTESIAN_POINT ( 'NONE',  ( -0.4615384615384611200, -13.63283147151868846, 33.57946703557072254 ) ) ;
#60759=CARTESIAN_POINT ( 'NONE',  ( -6.250023237292966272, -2.823816976329319495, 31.52131813110795733 ) ) ;
#60760=FACE_OUTER_BOUND ( 'NONE', #56074, .T. ) ;
#60761=AXIS2_PLACEMENT_3D ( 'NONE', #41820, #70610, #20648 ) ;
#60763=CARTESIAN_POINT ( 'NONE',  ( -6.923076923077045919, -3.643525952248796163, 33.31231777344771672 ) ) ;
#60764=CARTESIAN_POINT ( 'NONE',  ( -7.780898274877819709, -12.46129190930001052, 30.37095296980870174 ) ) ;
#60765=ORIENTED_EDGE ( 'NONE', *, *, #57563, .T. ) ;
#60766=CARTESIAN_POINT ( 'NONE',  ( 1.134638653673031738, -2.564618984488975961, 30.55390908950641915 ) ) ;
#60767=CARTESIAN_POINT ( 'NONE',  ( -17.29985003582992320, -6.459968553980840689, 34.89616026154728701 ) ) ;
#60768=B_SPLINE_CURVE_WITH_KNOTS ( 'NONE', 3,
 ( #54318, #33619, #67402, #52984, #80482, #32723, #45792, #18329, #60634, #53432 ),
 .UNSPECIFIED., .F., .F.,
 ( 4, 2, 2, 2, 4 ),
 ( 0.000000000000000000, 0.0001954339857564076099, 0.0003908679715128152198, 0.0005863019572692228839, 0.0007817359430256304396 ),
 .UNSPECIFIED. ) ;
#60770=EDGE_CURVE ( 'NONE', #72857, #37303, #81957, .T. ) ;
#60772=CYLINDRICAL_SURFACE ( 'NONE', #41242, 0.2500000000000008882 ) ;
#60773=LINE ( 'NONE', #5839, #6866 ) ;
#60774=CARTESIAN_POINT ( 'NONE',  ( 20.74999999999998224, -12.50000000000000000, 27.25000000000000000 ) ) ;
#60775=ORIENTED_EDGE ( 'NONE', *, *, #54293, .F. ) ;
#60777=CARTESIAN_POINT ( 'NONE',  ( -14.37377468705243722, -5.471508081941602875, 34.59228464037088457 ) ) ;
#60778=EDGE_CURVE ( 'NONE', #275, #62404, #29306, .T. ) ;
#60779=ORIENTED_EDGE ( 'NONE', *, *, #34103, .T. ) ;
#60780=CARTESIAN_POINT ( 'NONE',  ( -11.28846153846152589, -2.249999999999999112, 29.81603969181031744 ) ) ;
#60781=CARTESIAN_POINT ( 'NONE',  ( -2.307692307692305711, -2.538708090699994813, 30.37095296980875503 ) ) ;
#60782=EDGE_LOOP ( 'NONE', ( #87639, #52886 ) ) ;
#60783=CARTESIAN_POINT ( 'NONE',  ( 14.08420736396836226, -2.599994579823202923, 30.74605699353653776 ) ) ;
#60785=CARTESIAN_POINT ( 'NONE',  ( -20.74999999999999289, -7.500000000000000000, 29.75000000000000355 ) ) ;
#60786=ADVANCED_FACE ( 'NONE', ( #71120 ), #36891, .F. ) ;
#60787=VERTEX_POINT ( 'NONE', #2650 ) ;
#60790=ORIENTED_EDGE ( 'NONE', *, *, #55943, .F. ) ;
#60791=ADVANCED_FACE ( 'NONE', ( #57610 ), #64794, .F. ) ;
#60792=CARTESIAN_POINT ( 'NONE',  ( -8.096130590202436750, -2.318417181685855422, 30.59732222474233865 ) ) ;
#60793=CARTESIAN_POINT ( 'NONE',  ( -0.3962828902624368488, -10.90142922261932057, 33.41473453929631887 ) ) ;
#60794=CARTESIAN_POINT ( 'NONE',  ( 9.562159722575998444, -3.069018819979302926, 32.56621877034667278 ) ) ;
#60795=CARTESIAN_POINT ( 'NONE',  ( -17.32694631421604115, -5.851115903089112003, 34.47074536777953568 ) ) ;
#60796=ADVANCED_FACE ( 'NONE', ( #31014 ), #72449, .F. ) ;
#60797=CARTESIAN_POINT ( 'NONE',  ( 9.692307692307572609, -9.442884908241554243, 34.35708131394783038 ) ) ;
#60798=CARTESIAN_POINT ( 'NONE',  ( 6.988332062589762472, -8.656820664281605460, 34.87096338111211224 ) ) ;
#60799=LINE ( 'NONE', #79302, #56723 ) ;
#60800=VECTOR ( 'NONE', #30226, 1000.000000000000000 ) ;
#60801=CYLINDRICAL_SURFACE ( 'NONE', #1762, 0.2500000000000002220 ) ;
#60802=ADVANCED_FACE ( 'NONE', ( #19739 ), #32366, .F. ) ;
#60803=ORIENTED_EDGE ( 'NONE', *, *, #83293, .F. ) ;
#60804=B_SPLINE_CURVE_WITH_KNOTS ( 'NONE', 3,
 ( #7039, #51427, #37950, #25326, #58208, #44685, #86600, #87050, #80278, #64508 ),
 .UNSPECIFIED., .F., .F.,
 ( 4, 2, 2, 2, 4 ),
 ( 0.000000000000000000, 0.0001954311564186869015, 0.0003908623128373738030, 0.0005862934692560607588, 0.0007817246256747476061 ),
 .UNSPECIFIED. ) ;
#60805=EDGE_LOOP ( 'NONE', ( #82486, #18830, #4879, #54428 ) ) ;
#60806=CARTESIAN_POINT ( 'NONE',  ( 7.145856592054990131, -12.69155399931963046, 30.53255429739158444 ) ) ;
#60807=ORIENTED_EDGE ( 'NONE', *, *, #83019, .T. ) ;
#60808=EDGE_CURVE ( 'NONE', #64117, #44046, #86442, .T. ) ;
#60809=EDGE_CURVE ( 'NONE', #3657, #69245, #4560, .T. ) ;
#60810=CARTESIAN_POINT ( 'NONE',  ( -8.519285359852727169, -10.92531984108285670, 33.72920026020278073 ) ) ;
#60811=CARTESIAN_POINT ( 'NONE',  ( 12.59206416330202494, -3.285477652293413264, 32.44071101563363158 ) ) ;
#60812=EDGE_LOOP ( 'NONE', ( #1765, #22622 ) ) ;
#60813=CARTESIAN_POINT ( 'NONE',  ( -14.05774678934416499, -4.336752205174649433, 33.62275283266504289 ) ) ;
#60814=AXIS2_PLACEMENT_3D ( 'NONE', #9175, #83950, #29883 ) ;
#60815=VERTEX_POINT ( 'NONE', #19297 ) ;
#60816=CARTESIAN_POINT ( 'NONE',  ( 11.76147289007438523, -2.554770724473668153, 30.48948780036025852 ) ) ;
#60817=EDGE_LOOP ( 'NONE', ( #43635, #51591, #37700, #70359 ) ) ;
#60818=AXIS2_PLACEMENT_3D ( 'NONE', #84709, #21660, #77487 ) ;
#60819=CARTESIAN_POINT ( 'NONE',  ( -18.13069060311030967, -9.084618155246140248, 34.75535874321725771 ) ) ;
#60820=CARTESIAN_POINT ( 'NONE',  ( -12.33074802057151409, -9.929761469519743144, 34.40412654351204225 ) ) ;
#60821=EDGE_CURVE ( 'NONE', #59736, #26488, #45389, .T. ) ;
#60822=CARTESIAN_POINT ( 'NONE',  ( 10.86543892702293057, -4.943051570960394159, 34.04725096376909477 ) ) ;
#60823=FACE_BOUND ( 'NONE', #82095, .T. ) ;
#60824=DIRECTION ( 'NONE',  ( 0.000000000000000000, 0.4999999999999985567, 0.8660254037844395958 ) ) ;
#60825=CARTESIAN_POINT ( 'NONE',  ( -7.846153846153844924, -4.945431358278436385, 36.03766855953609394 ) ) ;
#60827=CARTESIAN_POINT ( 'NONE',  ( -5.749999999999999112, -2.499999999999998668, 29.75000000000000355 ) ) ;
#60828=ADVANCED_FACE ( 'NONE', ( #87330 ), #80569, .F. ) ;
#60829=CARTESIAN_POINT ( 'NONE',  ( 10.86538461538605205, -7.500000000000155431, 34.75000000000007105 ) ) ;
#60830=CARTESIAN_POINT ( 'NONE',  ( 15.90386942290380290, -4.236021600441997492, 33.53823185664189310 ) ) ;
#60831=CARTESIAN_POINT ( 'NONE',  ( -11.66915214157184622, -3.338472653186243644, 32.95098750199972670 ) ) ;
#60833=VERTEX_POINT ( 'NONE', #47200 ) ;
#60834=DIRECTION ( 'NONE',  ( -0.000000000000000000, 0.6427876096865404731, -0.7660444431189771253 ) ) ;
#60835=CARTESIAN_POINT ( 'NONE',  ( -14.05774678934416499, -12.43552623307873972, 30.55307653245132826 ) ) ;
#60836=LINE ( 'NONE', #74810, #11136 ) ;
#60837=CARTESIAN_POINT ( 'NONE',  ( -4.088591014333315066, -9.528491918058460186, 34.59228464037085615 ) ) ;
#60838=B_SPLINE_CURVE_WITH_KNOTS ( 'NONE', 3,
 ( #23575, #15503, #43848, #57805, #58245, #43417, #36221, #64111, #63676, #2409 ),
 .UNSPECIFIED., .F., .F.,
 ( 4, 2, 2, 2, 4 ),
 ( 0.0007817246256747447872, 0.0009771112852218874663, 0.001172497944769030362, 0.001367884604316173258, 0.001563271263863315937 ),
 .UNSPECIFIED. ) ;
#60840=CARTESIAN_POINT ( 'NONE',  ( 1.634560793993430350, -4.176053281294515251, 33.81426240980091791 ) ) ;
#60841=VERTEX_POINT ( 'NONE', #12983 ) ;
#60842=ADVANCED_FACE ( 'NONE', ( #31926 ), #74242, .F. ) ;
#60843=CARTESIAN_POINT ( 'NONE',  ( -13.38461538461538325, -1.951392089020283160, 34.73218667398347748 ) ) ;
#60845=CARTESIAN_POINT ( 'NONE',  ( 16.85399611801622655, -4.026226216239093603, 33.68668979543632958 ) ) ;
#60846=CARTESIAN_POINT ( 'NONE',  ( -7.146003881983771677, -6.459968553980839800, 34.89616026154728701 ) ) ;
#60847=ORIENTED_EDGE ( 'NONE', *, *, #66974, .T. ) ;
#60848=EDGE_CURVE ( 'NONE', #81591, #36076, #79865, .T. ) ;
#60849=ORIENTED_EDGE ( 'NONE', *, *, #88439, .F. ) ;
#60851=ORIENTED_EDGE ( 'NONE', *, *, #83977, .T. ) ;
#60852=EDGE_CURVE ( 'NONE', #85711, #40118, #50804, .T. ) ;
#60853=CIRCLE ( 'NONE', #59494, 0.2500000000000002220 ) ;
#60854=CARTESIAN_POINT ( 'NONE',  ( 15.29683758177167086, -6.386643153685127139, 34.62446782046654192 ) ) ;
#60855=ORIENTED_EDGE ( 'NONE', *, *, #10671, .F. ) ;
#60856=LINE ( 'NONE', #19871, #5048 ) ;
#60857=DIRECTION ( 'NONE',  ( -0.000000000000000000, 1.000000000000000000, -0.000000000000000000 ) ) ;
#60858=CARTESIAN_POINT ( 'NONE',  ( -5.299849294439221481, -4.186968288167446595, 33.49512374952580274 ) ) ;
#60859=CARTESIAN_POINT ( 'NONE',  ( 11.53846153846153832, -1.215029322943914858, 32.30358669280327177 ) ) ;
#60860=VECTOR ( 'NONE', #19925, 1000.000000000000000 ) ;
#60861=EDGE_CURVE ( 'NONE', #76945, #84175, #73806, .T. ) ;
#60862=CARTESIAN_POINT ( 'NONE',  ( -1.384615384615383471, -8.564572088678739092, 35.78748833219616898 ) ) ;
#60863=ORIENTED_EDGE ( 'NONE', *, *, #14535, .T. ) ;
#60864=CARTESIAN_POINT ( 'NONE',  ( 22.75000000000000000, -4.499999999999999112, 27.25000000000000000 ) ) ;
#60865=CARTESIAN_POINT ( 'NONE',  ( -0.2387587925603967820, -12.11081565061823717, 32.26097654155341843 ) ) ;
#60866=ORIENTED_EDGE ( 'NONE', *, *, #54818, .F. ) ;
#60868=CARTESIAN_POINT ( 'NONE',  ( 16.15384615384645883, -2.506253911140615021, 30.00000000000323297 ) ) ;
#60869=CARTESIAN_POINT ( 'NONE',  ( 1.634615384615323075, -7.565270445406050648, 34.75000000000000000 ) ) ;
#60870=DIRECTION ( 'NONE',  ( -0.000000000000000000, -0.1736481776669307198, -0.9848077530122080203 ) ) ;
#60871=CARTESIAN_POINT ( 'NONE',  ( -6.000000000000121680, -11.06231777344772027, 33.60647404775119895 ) ) ;
#60872=CARTESIAN_POINT ( 'NONE',  ( -8.769230769230768274, -9.058645607665452459, 34.76329471203371924 ) ) ;
#60873=CARTESIAN_POINT ( 'NONE',  ( -0.5922299282060203840, -12.38065189839062263, 30.83690757178629482 ) ) ;
#60875=ORIENTED_EDGE ( 'NONE', *, *, #13069, .F. ) ;
#60877=CARTESIAN_POINT ( 'NONE',  ( 12.59206389977210705, -5.070358843744210198, 34.40418822224088302 ) ) ;
#60878=ORIENTED_EDGE ( 'NONE', *, *, #24995, .F. ) ;
#60879=VERTEX_POINT ( 'NONE', #61154 ) ;
#60880=CARTESIAN_POINT ( 'NONE',  ( 7.976944287120795174, -11.93129842949671726, 32.56571108434900452 ) ) ;
#60881=CARTESIAN_POINT ( 'NONE',  ( -3.230769230769351186, -6.026961402154118908, 34.52809138561165270 ) ) ;
#60882=B_SPLINE_CURVE_WITH_KNOTS ( 'NONE', 3,
 ( #63179, #62730, #55983, #42483, #55539, #47895, #34381, #7804, #1492, #28978 ),
 .UNSPECIFIED., .F., .F.,
 ( 4, 2, 2, 2, 4 ),
 ( 0.0007817246256747448956, 0.0009771112852218876831, 0.001172497944769030362, 0.001367884604316173258, 0.001563271263863315937 ),
 .UNSPECIFIED. ) ;
#60883=EDGE_CURVE ( 'NONE', #45658, #36243, #88666, .T. ) ;
#60885=CARTESIAN_POINT ( 'NONE',  ( -5.076923076922769340, -2.506253911140614576, 30.00000000000323297 ) ) ;
#60886=CIRCLE ( 'NONE', #32151, 0.2500000000000002220 ) ;
#60887=CARTESIAN_POINT ( 'NONE',  ( 0.7115928814519132395, -2.318338780012835443, 30.59689888758630261 ) ) ;
#60888=ORIENTED_EDGE ( 'NONE', *, *, #71630, .F. ) ;
#60889=CARTESIAN_POINT ( 'NONE',  ( 9.561616225640134914, -10.54014554554150607, 33.71984207302941883 ) ) ;
#60890=CARTESIAN_POINT ( 'NONE',  ( 17.29970261819148902, -5.913360116392396115, 34.49180327182771322 ) ) ;
#60891=FACE_OUTER_BOUND ( 'NONE', #11377, .T. ) ;
#60892=ORIENTED_EDGE ( 'NONE', *, *, #64573, .T. ) ;
#60893=LINE ( 'NONE', #13596, #9644 ) ;
#60894=ORIENTED_EDGE ( 'NONE', *, *, #44686, .F. ) ;
#60897=DIRECTION ( 'NONE',  ( 0.000000000000000000, 0.6427876096865368094, 0.7660444431189802339 ) ) ;
#60899=CARTESIAN_POINT ( 'NONE',  ( 3.230769230769110045, -12.27809138561165270, 31.22303859784587132 ) ) ;
#60900=CARTESIAN_POINT ( 'NONE',  ( -11.53846153846165912, -12.46129190930018460, 30.37095296980731973 ) ) ;
#60901=CARTESIAN_POINT ( 'NONE',  ( -9.942330929600657896, -2.587272538249755893, 30.68239716806877837 ) ) ;
#60902=CARTESIAN_POINT ( 'NONE',  ( 2.307692307692186251, -4.320704448113951379, 33.92786785259630022 ) ) ;
#60903=DIRECTION ( 'NONE',  ( -0.000000000000000000, 0.1736481776669307198, -0.9848077530122080203 ) ) ;
#60904=ORIENTED_EDGE ( 'NONE', *, *, #72083, .F. ) ;
#60905=CARTESIAN_POINT ( 'NONE',  ( 2.307692307692309264, -12.78798330534102945, 29.74999999999997868 ) ) ;
#60907=B_SPLINE_CURVE_WITH_KNOTS ( 'NONE', 3,
 ( #6826, #5955, #82060, #34299, #60441, #81612, #54119, #77, #87958, #47367 ),
 .UNSPECIFIED., .F., .F.,
 ( 4, 2, 2, 2, 4 ),
 ( 0.000000000000000000, 0.0001954311564186867389, 0.0003908623128373734778, 0.0005862934692560602167, 0.0007817246256747469556 ),
 .UNSPECIFIED. ) ;
#60908=CARTESIAN_POINT ( 'NONE',  ( 6.923076923076924238, -1.044019251281081972, 31.83374038241031911 ) ) ;
#60909=CIRCLE ( 'NONE', #46516, 0.2500000000000002220 ) ;
#60911=ADVANCED_FACE ( 'NONE', ( #21052 ), #55729, .F. ) ;
#60912=VECTOR ( 'NONE', #84546, 1000.000000000000227 ) ;
#60913=CARTESIAN_POINT ( 'NONE',  ( -18.06608237936013239, -10.67929555188718460, 33.92786785259543336 ) ) ;
#60914=ADVANCED_FACE ( 'NONE', ( #49427 ), #8000, .F. ) ;
#60915=CARTESIAN_POINT ( 'NONE',  ( 5.999999999999878320, -12.70778746994576025, 30.41441678777401236 ) ) ;
#60916=CARTESIAN_POINT ( 'NONE',  ( 7.173131234715239835, -9.943054286541403997, 34.11300777759954883 ) ) ;
#60917=EDGE_LOOP ( 'NONE', ( #59359, #8915 ) ) ;
#60918=EDGE_LOOP ( 'NONE', ( #40768, #18460, #6403, #30783 ) ) ;
#60920=VERTEX_POINT ( 'NONE', #20188 ) ;
#60921=EDGE_LOOP ( 'NONE', ( #34628, #20060, #14856, #64193 ) ) ;
#60923=CARTESIAN_POINT ( 'NONE',  ( 15.16549923021291058, -3.643525952247789412, 33.31231777344662959 ) ) ;
#60924=EDGE_CURVE ( 'NONE', #20422, #71376, #47653, .T. ) ;
#60925=CARTESIAN_POINT ( 'NONE',  ( -11.53846153846153655, -5.471508081941601098, 34.59228464037088457 ) ) ;
#60926=CARTESIAN_POINT ( 'NONE',  ( -7.912236225513978205, -3.322132147404559532, 32.92929555188719348 ) ) ;
#60927=CARTESIAN_POINT ( 'NONE',  ( -5.326899807865431491, -10.66389620160130036, 33.62221079203477103 ) ) ;
#60928=B_SPLINE_CURVE_WITH_KNOTS ( 'NONE', 3,
 ( #250, #27275, #81789, #76345, #47539, #61057, #75031, #47982, #14652, #69591 ),
 .UNSPECIFIED., .F., .F.,
 ( 4, 2, 2, 2, 4 ),
 ( 0.000000000000000000, 0.0001954311564186862239, 0.0003908623128373724478, 0.0005862934692560586988, 0.0007817246256747448956 ),
 .UNSPECIFIED. ) ;
#60929=CARTESIAN_POINT ( 'NONE',  ( 4.153846153846154188, -2.499999999999998668, 29.75000000000001421 ) ) ;
#60930=CARTESIAN_POINT ( 'NONE',  ( -5.010854725920638408, -4.098570777380720287, 33.41473453929635440 ) ) ;
#60931=CARTESIAN_POINT ( 'NONE',  ( -4.826977667545033768, -11.56426240980093745, 33.07394671870546432 ) ) ;
#60932=EDGE_LOOP ( 'NONE', ( #41304, #28678 ) ) ;
#60933=VERTEX_POINT ( 'NONE', #42674 ) ;
#60935=CARTESIAN_POINT ( 'NONE',  ( 2.177000841024749889, -2.541943142973489778, 30.39792223712631980 ) ) ;
#60936=EDGE_LOOP ( 'NONE', ( #31537, #69051, #42457, #69865, #81415, #29763 ) ) ;
#60937=AXIS2_PLACEMENT_3D ( 'NONE', #57184, #84675, #21178 ) ;
#60938=DIRECTION ( 'NONE',  ( 0.000000000000000000, 0.1736481776669267785, -0.9848077530122087975 ) ) ;
#60939=CARTESIAN_POINT ( 'NONE',  ( -8.069638789877792817, -4.386631170607604879, 33.66268669641500111 ) ) ;
#60941=CARTESIAN_POINT ( 'NONE',  ( -10.74607608205217346, -3.530157926970578952, 32.79014554554150607 ) ) ;
#60942=FACE_BOUND ( 'NONE', #24328, .T. ) ;
#60943=EDGE_LOOP ( 'NONE', ( #88651, #72351, #78751, #20863 ) ) ;
#60944=CARTESIAN_POINT ( 'NONE',  ( 16.82694634598072625, -6.567427716900048118, 34.66269422305636283 ) ) ;
#60945=CARTESIAN_POINT ( 'NONE',  ( -3.164700879766791708, -6.386643153685127139, 34.62446782046654192 ) ) ;
#60946=ORIENTED_EDGE ( 'NONE', *, *, #61348, .F. ) ;
#60947=CARTESIAN_POINT ( 'NONE',  ( 5.010840697562938928, -2.292212530054419606, 30.41441678777542634 ) ) ;
#60948=EDGE_CURVE ( 'NONE', #43471, #34591, #83068, .T. ) ;
#60950=FACE_BOUND ( 'NONE', #89133, .T. ) ;
#60951=CARTESIAN_POINT ( 'NONE',  ( -9.692307692307691624, -2.292212530054420494, 30.41441678777542634 ) ) ;
#60952=CARTESIAN_POINT ( 'NONE',  ( 18.13079180782478872, -4.809403383903225304, 33.96459661697925014 ) ) ;
#60953=VERTEX_POINT ( 'NONE', #48083 ) ;
#60954=CYLINDRICAL_SURFACE ( 'NONE', #41993, 0.2500000000000009437 ) ;
#60955=DIRECTION ( 'NONE',  ( -0.000000000000000000, -0.000000000000000000, -1.000000000000000000 ) ) ;
#60956=CARTESIAN_POINT ( 'NONE',  ( -0.5922290646487694543, -2.295517848115769421, 30.44137282052137294 ) ) ;
#60957=ORIENTED_EDGE ( 'NONE', *, *, #52575, .T. ) ;
#60958=CYLINDRICAL_SURFACE ( 'NONE', #82506, 0.2500000000000008882 ) ;
#60959=LINE ( 'NONE', #74935, #11192 ) ;
#60960=CARTESIAN_POINT ( 'NONE',  ( -3.360916440207447398, -2.882441371585227508, 31.66841991370171527 ) ) ;
#60961=CARTESIAN_POINT ( 'NONE',  ( -7.846153846153965716, -2.892918686052166066, 31.69288490824153470 ) ) ;
#60962=ORIENTED_EDGE ( 'NONE', *, *, #53694, .F. ) ;
#60964=CARTESIAN_POINT ( 'NONE',  ( 12.52673144983311637, -2.255955759149235629, 29.99999999999988987 ) ) ;
#60965=DIRECTION ( 'NONE',  ( 0.000000000000000000, 0.4999999999999960032, -0.8660254037844410391 ) ) ;
#60966=VERTEX_POINT ( 'NONE', #793 ) ;
#60967=CARTESIAN_POINT ( 'NONE',  ( -4.826977667545032880, -3.520799739797213501, 33.17531984108286025 ) ) ;
#60968=CARTESIAN_POINT ( 'NONE',  ( -4.403869391139117795, -2.587272538249754117, 30.68239716806877837 ) ) ;
#60969=CARTESIAN_POINT ( 'NONE',  ( -8.096177070375301099, -12.45566812827425096, 31.48439005359158926 ) ) ;
#60970=CARTESIAN_POINT ( 'NONE',  ( 13.63456090296352841, -12.43552623307873972, 30.55307653245132826 ) ) ;
#60971=CARTESIAN_POINT ( 'NONE',  ( -6.673076923076859401, -7.434744860731433924, 35.00000000000000711 ) ) ;
#60972=CARTESIAN_POINT ( 'NONE',  ( 15.00728430620490350, -5.827078755546623690, 34.72654668319379567 ) ) ;
#60973=B_SPLINE_CURVE_WITH_KNOTS ( 'NONE', 3,
 ( #70786, #37422, #63570, #49172, #84311, #1874, #63121, #55927, #83419, #15844 ),
 .UNSPECIFIED., .F., .F.,
 ( 4, 2, 2, 2, 4 ),
 ( 0.0007817246256747447872, 0.0009771112852218874663, 0.001172497944769030362, 0.001367884604316173258, 0.001563271263863315937 ),
 .UNSPECIFIED. ) ;
#60974=CARTESIAN_POINT ( 'NONE',  ( 6.249945518348144269, -11.86320923018887541, 32.19269448109604781 ) ) ;
#60975=CARTESIAN_POINT ( 'NONE',  ( 16.15384615384615330, -5.557115091759785130, 34.35708131394839171 ) ) ;
#60976=EDGE_CURVE ( 'NONE', #19826, #53468, #69693, .T. ) ;
#60979=EDGE_LOOP ( 'NONE', ( #22044, #11947 ) ) ;
#60980=AXIS2_PLACEMENT_3D ( 'NONE', #14048, #41522, #83407 ) ;
#60981=CARTESIAN_POINT ( 'NONE',  ( 4.826899852701618698, -6.652501968072646932, 34.93155406624980941 ) ) ;
#60982=VERTEX_POINT ( 'NONE', #62917 ) ;
#60985=ORIENTED_EDGE ( 'NONE', *, *, #33667, .F. ) ;
#60986=CARTESIAN_POINT ( 'NONE',  ( -11.53846153846166089, -2.379036618888197729, 30.90682066428292885 ) ) ;
#60987=ORIENTED_EDGE ( 'NONE', *, *, #59358, .F. ) ;
#60988=CARTESIAN_POINT ( 'NONE',  ( -4.403822897894741573, -2.544273027872574922, 31.48422191005632342 ) ) ;
#60990=CARTESIAN_POINT ( 'NONE',  ( 12.23871036390358569, -7.369209533119137845, 34.99857337881830688 ) ) ;
#60992=CARTESIAN_POINT ( 'NONE',  ( 5.776515056276056548, -11.41268669641500466, 32.86336882939237825 ) ) ;
#60994=FACE_OUTER_BOUND ( 'NONE', #43387, .T. ) ;
#60995=CARTESIAN_POINT ( 'NONE',  ( -13.60754160213153163, -2.554751324335734708, 30.48935550225260727 ) ) ;
#60998=EDGE_CURVE ( 'NONE', #67793, #16935, #74438, .T. ) ;
#60999=ADVANCED_FACE ( 'NONE', ( #68809 ), #7108, .F. ) ;
#61000=CARTESIAN_POINT ( 'NONE',  ( -0.5276218724943432248, -2.538708090699994813, 30.37095296980875148 ) ) ;
#61001=CARTESIAN_POINT ( 'NONE',  ( -14.37294329785354918, -2.506253911140460922, 30.00000000000013856 ) ) ;
#61002=CARTESIAN_POINT ( 'NONE',  ( -2.530618525208451874, -4.186968288167446595, 33.49512374952580274 ) ) ;
#61003=ADVANCED_FACE ( 'NONE', ( #64691 ), #22829, .F. ) ;
#61004=EDGE_LOOP ( 'NONE', ( #32524, #76723 ) ) ;
#61006=CARTESIAN_POINT ( 'NONE',  ( -9.442362173959550020, -3.712312575010499049, 33.01462480002815170 ) ) ;
#61007=FACE_OUTER_BOUND ( 'NONE', #35632, .T. ) ;
#61008=CARTESIAN_POINT ( 'NONE',  ( 17.07692307692307665, -2.249999999999998668, 29.75000000000001776 ) ) ;
#61009=CARTESIAN_POINT ( 'NONE',  ( -16.02305434602136458, -12.38066358083363738, 30.83685684665853444 ) ) ;
#61010=CARTESIAN_POINT ( 'NONE',  ( 8.769230769230647482, -4.481592998941358097, 33.73612834414048933 ) ) ;
#61011=CARTESIAN_POINT ( 'NONE',  ( -6.000000000000119904, -8.613356846316285953, 34.62446782046622218 ) ) ;
#61012=AXIS2_PLACEMENT_3D ( 'NONE', #31155, #80253, #44659 ) ;
#61013=CARTESIAN_POINT ( 'NONE',  ( -2.531177232256637044, -8.539481045369598178, 34.89627647299170832 ) ) ;
#61014=ORIENTED_EDGE ( 'NONE', *, *, #25633, .F. ) ;
#61015=CARTESIAN_POINT ( 'NONE',  ( -6.792551221313363641, -10.19071101563364756, 33.96452234770658407 ) ) ;
#61017=ORIENTED_EDGE ( 'NONE', *, *, #1946, .F. ) ;
#61018=ADVANCED_FACE ( 'NONE', ( #51160 ), #1680, .F. ) ;
#61019=CARTESIAN_POINT ( 'NONE',  ( 16.28437159207980045, -9.503571793651730104, 34.60286762892837942 ) ) ;
#61020=CARTESIAN_POINT ( 'NONE',  ( 4.023154687178593925, -2.541943142973490666, 30.39792223712631980 ) ) ;
#61021=CARTESIAN_POINT ( 'NONE',  ( -0.4615384615385826339, -6.879047030192662504, 34.71129190930017927 ) ) ;
#61022=CARTESIAN_POINT ( 'NONE',  ( 5.076923076923075762, -1.129524287112498415, 32.06866353760679544 ) ) ;
#61023=CARTESIAN_POINT ( 'NONE',  ( -7.846153846153965716, -9.442884908241554243, 34.35708131394783038 ) ) ;
#61024=EDGE_CURVE ( 'NONE', #85855, #36501, #84191, .T. ) ;
#61025=ORIENTED_EDGE ( 'NONE', *, *, #58587, .T. ) ;
#61026=ADVANCED_FACE ( 'NONE', ( #71022 ), #65137, .F. ) ;
#61027=ORIENTED_EDGE ( 'NONE', *, *, #55257, .F. ) ;
#61028=ORIENTED_EDGE ( 'NONE', *, *, #23669, .F. ) ;
#61029=ORIENTED_EDGE ( 'NONE', *, *, #4202, .F. ) ;
#61030=VECTOR ( 'NONE', #72224, 1000.000000000000227 ) ;
#61031=CARTESIAN_POINT ( 'NONE',  ( 17.07692307692295586, -10.33852847137269571, 34.16647553114546554 ) ) ;
#61032=FACE_OUTER_BOUND ( 'NONE', #15269, .T. ) ;
#61035=VECTOR ( 'NONE', #15167, 1000.000000000000000 ) ;
#61036=VECTOR ( 'NONE', #5825, 1000.000000000000000 ) ;
#61037=CARTESIAN_POINT ( 'NONE',  ( -16.37733107841048508, -2.353723527008297012, 30.78948104536958752 ) ) ;
#61038=CARTESIAN_POINT ( 'NONE',  ( -10.48459280755982981, -12.11778462344220841, 31.66786338562085135 ) ) ;
#61039=ORIENTED_EDGE ( 'NONE', *, *, #23589, .F. ) ;
#61041=ORIENTED_EDGE ( 'NONE', *, *, #11342, .T. ) ;
#61042=ADVANCED_FACE ( 'NONE', ( #78662 ), #56625, .F. ) ;
#61043=CARTESIAN_POINT ( 'NONE',  ( -10.39237326377176274, -11.76359900205217457, 32.36225158514719880 ) ) ;
#61044=ORIENTED_EDGE ( 'NONE', *, *, #55425, .T. ) ;
#61045=CARTESIAN_POINT ( 'NONE',  ( 9.561617089197390840, -8.191372820521381826, 34.95448215188423546 ) ) ;
#61046=CARTESIAN_POINT ( 'NONE',  ( -10.61538461538461320, -7.500000000000001776, 35.04278698407183867 ) ) ;
#61048=VERTEX_POINT ( 'NONE', #22392 ) ;
#61049=CARTESIAN_POINT ( 'NONE',  ( -1.384615384615383471, -2.486705287966279876, 31.30864560766543647 ) ) ;
#61050=ORIENTED_EDGE ( 'NONE', *, *, #50321, .F. ) ;
#61051=CYLINDRICAL_SURFACE ( 'NONE', #35670, 0.2499999999999995559 ) ;
#61052=FACE_BOUND ( 'NONE', #10891, .T. ) ;
#61054=FACE_OUTER_BOUND ( 'NONE', #9119, .T. ) ;
#61056=EDGE_CURVE ( 'NONE', #69885, #63541, #11105, .T. ) ;
#61057=CARTESIAN_POINT ( 'NONE',  ( 8.519207545009310323, -12.07920672191015221, 32.31858351112116168 ) ) ;
#61058=CARTESIAN_POINT ( 'NONE',  ( -14.17690049986752321, -2.541949514083464479, 30.39797389878540557 ) ) ;
#61059=EDGE_CURVE ( 'NONE', #74128, #70315, #10213, .T. ) ;
#61060=CARTESIAN_POINT ( 'NONE',  ( -13.60749406704403519, -7.630691491037285168, 34.74850469731152458 ) ) ;
#61061=DIRECTION ( 'NONE',  ( -0.000000000000000000, -0.8660254037844399289, -0.4999999999999980016 ) ) ;
#61062=ORIENTED_EDGE ( 'NONE', *, *, #70101, .F. ) ;
#61063=VECTOR ( 'NONE', #35949, 1000.000000000000114 ) ;
#61064=CARTESIAN_POINT ( 'NONE',  ( -18.13014796973170206, -12.70455904226513866, 30.44083106164009322 ) ) ;
#61065=CARTESIAN_POINT ( 'NONE',  ( -5.750054590621955342, -4.176053281294514363, 33.81426240980091791 ) ) ;
#61066=LINE ( 'NONE', #56085, #68574 ) ;
#61067=DIRECTION ( 'NONE',  ( -0.000000000000000000, 0.1736481776669307198, -0.9848077530122080203 ) ) ;
#61068=CARTESIAN_POINT ( 'NONE',  ( -1.384615384615383471, -2.499999999999998668, 29.75000000000001421 ) ) ;
#61069=FACE_BOUND ( 'NONE', #3496, .T. ) ;
#61071=CARTESIAN_POINT ( 'NONE',  ( 16.94677510719138169, -3.069018819979304702, 32.56621877034667278 ) ) ;
#61074=FACE_OUTER_BOUND ( 'NONE', #2103, .T. ) ;
#61075=CARTESIAN_POINT ( 'NONE',  ( -11.40767109749459074, -10.70102852606553157, 33.91149625220312913 ) ) ;
#61076=DIRECTION ( 'NONE',  ( 1.000000000000000000, 0.000000000000000000, 0.000000000000000000 ) ) ;
#61078=EDGE_LOOP ( 'NONE', ( #16107, #80682 ) ) ;
#61080=ORIENTED_EDGE ( 'NONE', *, *, #3845, .T. ) ;
#61081=CARTESIAN_POINT ( 'NONE',  ( 1.134615384615377698, -2.499999999999999556, 29.81609845454692120 ) ) ;
#61082=ORIENTED_EDGE ( 'NONE', *, *, #48272, .T. ) ;
#61083=CARTESIAN_POINT ( 'NONE',  ( -11.53846153846153655, -2.721908614388771852, 31.22303859784724978 ) ) ;
#61084=CARTESIAN_POINT ( 'NONE',  ( -18.13014720943822056, -2.619462340734461048, 30.83744416345203021 ) ) ;
#61085=CARTESIAN_POINT ( 'NONE',  ( 18.00000000000000000, -2.249999999999998668, 29.50000000000001421 ) ) ;
#61087=CARTESIAN_POINT ( 'NONE',  ( 16.94677510719138169, -12.70455904226513866, 30.44083106164009322 ) ) ;
#61088=CARTESIAN_POINT ( 'NONE',  ( -9.822918051932216343, -7.722926236386453702, 34.74524107206102030 ) ) ;
#61090=CARTESIAN_POINT ( 'NONE',  ( 14.05771557674995620, -10.66389620160130036, 33.62221079203477103 ) ) ;
#61091=CARTESIAN_POINT ( 'NONE',  ( 4.946775867484854317, -5.195881422630167279, 34.18770438780618548 ) ) ;
#61092=CARTESIAN_POINT ( 'NONE',  ( -4.946397638689433940, -12.15418822224088657, 32.17964115625579069 ) ) ;
#61093=CARTESIAN_POINT ( 'NONE',  ( 3.230769230769231726, -10.89733346790207413, 36.13435417666054406 ) ) ;
#61094=DIRECTION ( 'NONE',  ( -0.000000000000000000, -0.8660254037844399289, -0.4999999999999980016 ) ) ;
#61095=CARTESIAN_POINT ( 'NONE',  ( -5.934744428723972121, -10.90142922261932057, 33.41473453929631887 ) ) ;
#61097=EDGE_CURVE ( 'NONE', #79197, #84840, #77628, .T. ) ;
#61099=CARTESIAN_POINT ( 'NONE',  ( -14.98076923076922995, -7.500000000000001776, 35.04278698407183867 ) ) ;
#61101=ORIENTED_EDGE ( 'NONE', *, *, #81425, .T. ) ;
#61102=CARTESIAN_POINT ( 'NONE',  ( 16.37662582282421653, -4.989023458446561143, 34.36081565061822118 ) ) ;
#61104=AXIS2_PLACEMENT_3D ( 'NONE', #58625, #45115, #51859 ) ;
#61105=DIRECTION ( 'NONE',  ( 0.000000000000000000, 0.000000000000000000, 1.000000000000000000 ) ) ;
#61107=EDGE_LOOP ( 'NONE', ( #42499, #48706, #7179, #54150 ) ) ;
#61110=CARTESIAN_POINT ( 'NONE',  ( 2.057715576749954867, -2.779195860258149242, 31.39871582349837453 ) ) ;
#61112=FACE_OUTER_BOUND ( 'NONE', #6626, .T. ) ;
#61113=CARTESIAN_POINT ( 'NONE',  ( 15.45354889974729495, -5.827830569534417471, 34.72679350104403539 ) ) ;
#61114=LINE ( 'NONE', #34969, #74477 ) ;
#61115=ORIENTED_EDGE ( 'NONE', *, *, #71775, .F. ) ;
#61116=CARTESIAN_POINT ( 'NONE',  ( 3.230769230769108269, -2.657715359629662544, 31.77849191805970364 ) ) ;
#61117=CARTESIAN_POINT ( 'NONE',  ( -9.942307692307691624, -2.499999999999998668, 29.75000000000000355 ) ) ;
#61118=CARTESIAN_POINT ( 'NONE',  ( 8.639082799499075094, -3.625366637846545892, 33.29286588640298561 ) ) ;
#61119=ORIENTED_EDGE ( 'NONE', *, *, #667, .T. ) ;
#61120=EDGE_LOOP ( 'NONE', ( #84635, #29057 ) ) ;
#61121=ORIENTED_EDGE ( 'NONE', *, *, #35386, .F. ) ;
#61122=VERTEX_POINT ( 'NONE', #71453 ) ;
#61123=CARTESIAN_POINT ( 'NONE',  ( -9.692307692307812417, -2.892918686052166066, 31.69288490824153470 ) ) ;
#61124=CARTESIAN_POINT ( 'NONE',  ( 14.17754509825408960, -4.460286881179643004, 33.72017969459903242 ) ) ;
#61125=CARTESIAN_POINT ( 'NONE',  ( -11.31568186948346977, -3.563462043263030399, 33.22394488606062879 ) ) ;
#61126=CARTESIAN_POINT ( 'NONE',  ( 11.53846153846153832, -2.499999999999998668, 29.75000000000001421 ) ) ;
#61127=CARTESIAN_POINT ( 'NONE',  ( 16.15384615384615330, -4.786620604624113540, 33.94971097300155094 ) ) ;
#61128=ORIENTED_EDGE ( 'NONE', *, *, #43677, .T. ) ;
#61129=VERTEX_POINT ( 'NONE', #11545 ) ;
#61130=EDGE_LOOP ( 'NONE', ( #41538, #74045, #16248, #55893 ) ) ;
#61131=CARTESIAN_POINT ( 'NONE',  ( -16.15384615384615330, -6.189225973068211317, 35.74407628777942847 ) ) ;
#61132=VERTEX_POINT ( 'NONE', #66932 ) ;
#61133=CARTESIAN_POINT ( 'NONE',  ( -4.853910232829682592, -12.38742843783360748, 31.66772728687926985 ) ) ;
#61134=CARTESIAN_POINT ( 'NONE',  ( -3.360917200500922686, -12.15440758774515473, 32.17923288041532004 ) ) ;
#61136=CARTESIAN_POINT ( 'NONE',  ( 16.02369818411446190, -11.66186481527757479, 32.95055677023626117 ) ) ;
#61139=ORIENTED_EDGE ( 'NONE', *, *, #40838, .T. ) ;
#61140=CARTESIAN_POINT ( 'NONE',  ( 10.74617642320940369, -10.54018710029568595, 33.71981072465678864 ) ) ;
#61142=ORIENTED_EDGE ( 'NONE', *, *, #87847, .T. ) ;
#61143=CARTESIAN_POINT ( 'NONE',  ( -11.47320639894870276, -12.70778746994558439, 30.41441678777536595 ) ) ;
#61145=CARTESIAN_POINT ( 'NONE',  ( -17.07692307692319744, -3.643525952248796163, 33.31231777344771672 ) ) ;
#61146=ORIENTED_EDGE ( 'NONE', *, *, #31815, .T. ) ;
#61147=CARTESIAN_POINT ( 'NONE',  ( 1.384615384615386802, -11.11383981884818262, 36.00935417666054406 ) ) ;
#61148=CARTESIAN_POINT ( 'NONE',  ( -6.923076923076922462, -12.37446782046654192, 30.86335684631486131 ) ) ;
#61149=CARTESIAN_POINT ( 'NONE',  ( -17.07692307692319744, -11.06231777344772027, 33.60647404775119895 ) ) ;
#61150=FACE_BOUND ( 'NONE', #36338, .T. ) ;
#61151=CARTESIAN_POINT ( 'NONE',  ( 10.86543892702293057, -9.943054286541403997, 34.11300777759954883 ) ) ;
#61154=CARTESIAN_POINT ( 'NONE',  ( -9.942307692307691624, -7.500000000000001776, 34.75000000000000000 ) ) ;
#61155=CARTESIAN_POINT ( 'NONE',  ( 9.627037246346917598, -3.300289026998414865, 32.46337939537583139 ) ) ;
#61157=DIRECTION ( 'NONE',  ( 0.000000000000000000, 0.9848077530122072432, -0.1736481776669354937 ) ) ;
#61158=CARTESIAN_POINT ( 'NONE',  ( -11.53846153846153655, -1.466349020453238561, 30.81389545987213907 ) ) ;
#61159=ORIENTED_EDGE ( 'NONE', *, *, #45103, .F. ) ;
#61160=CARTESIAN_POINT ( 'NONE',  ( 14.30769230769231015, -12.37446782046654192, 30.86335684631486131 ) ) ;
#61161=B_SPLINE_CURVE_WITH_KNOTS ( 'NONE', 3,
 ( #28005, #14046, #34312, #75311, #13604, #82522, #7296, #20801, #41520, #62227 ),
 .UNSPECIFIED., .F., .F.,
 ( 4, 2, 2, 2, 4 ),
 ( 0.000000000000000000, 0.0001954339857564082333, 0.0003908679715128164666, 0.0005863019572692247270, 0.0007817359430256329332 ),
 .UNSPECIFIED. ) ;
#61162=CIRCLE ( 'NONE', #12314, 0.2500000000000002220 ) ;
#61163=ORIENTED_EDGE ( 'NONE', *, *, #69296, .T. ) ;
#61165=B_SPLINE_CURVE_WITH_KNOTS ( 'NONE', 3,
 ( #5536, #73557, #59130, #24901, #52815, #73995, #58685, #45620, #11853, #39770 ),
 .UNSPECIFIED., .F., .F.,
 ( 4, 2, 2, 2, 4 ),
 ( 0.000000000000000000, 0.0001954339857564081249, 0.0003908679715128162498, 0.0005863019572692244018, 0.0007817359430256324996 ),
 .UNSPECIFIED. ) ;
#61166=CARTESIAN_POINT ( 'NONE',  ( -14.43783951713053249, -5.195881422630166391, 34.18770438780619259 ) ) ;
#61167=FACE_OUTER_BOUND ( 'NONE', #11344, .T. ) ;
#61168=VERTEX_POINT ( 'NONE', #25053 ) ;
#61170=CARTESIAN_POINT ( 'NONE',  ( -4.153846153846274980, -9.528491918059723176, 34.59228464037033035 ) ) ;
#61171=FACE_BOUND ( 'NONE', #23641, .T. ) ;
#61172=CARTESIAN_POINT ( 'NONE',  ( -4.153846153846152411, -2.499999999999998668, 29.75000000000001421 ) ) ;
#61173=CYLINDRICAL_SURFACE ( 'NONE', #14308, 0.2499999999999993616 ) ;
#61174=CARTESIAN_POINT ( 'NONE',  ( 7.846153846153725020, -9.442884908241554243, 34.35708131394783038 ) ) ;
#61176=CARTESIAN_POINT ( 'NONE',  ( -5.300408020647025431, -9.331801661448606566, 34.40259984581193464 ) ) ;
#61180=ORIENTED_EDGE ( 'NONE', *, *, #7492, .T. ) ;
#61181=ORIENTED_EDGE ( 'NONE', *, *, #52052, .F. ) ;
#61182=DIRECTION ( 'NONE',  ( -0.000000000000000000, 0.7660444431189791237, -0.6427876096865379196 ) ) ;
#61183=CARTESIAN_POINT ( 'NONE',  ( -17.86920955903305597, -3.338503747796863319, 32.95102852606552801 ) ) ;
#61184=CARTESIAN_POINT ( 'NONE',  ( 10.61538461538461675, -2.538708090699994813, 30.37095296980875503 ) ) ;
#61185=CARTESIAN_POINT ( 'NONE',  ( 6.792929713638700129, -12.27039167877662251, 31.24851455888617835 ) ) ;
#61186=FACE_OUTER_BOUND ( 'NONE', #88314, .T. ) ;
#61188=DIRECTION ( 'NONE',  ( 0.000000000000000000, 0.8660254037844377084, 0.5000000000000015543 ) ) ;
#61189=CYLINDRICAL_SURFACE ( 'NONE', #24432, 0.2499999999999997502 ) ;
#61190=AXIS2_PLACEMENT_3D ( 'NONE', #21442, #34515, #12910 ) ;
#61191=CARTESIAN_POINT ( 'NONE',  ( 7.846153846153723244, -3.643525952248796163, 33.31231777344771672 ) ) ;
#61192=DIRECTION ( 'NONE',  ( -0.000000000000000000, -0.7660444431189791237, -0.6427876096865379196 ) ) ;
#61193=CARTESIAN_POINT ( 'NONE',  ( 9.942362003946008997, -2.779044189368095719, 31.39831045268885745 ) ) ;
#61194=CARTESIAN_POINT ( 'NONE',  ( 7.846153846153846700, -2.499999999999998668, 29.75000000000001421 ) ) ;
#61195=CARTESIAN_POINT ( 'NONE',  ( 6.792385456409367528, -11.18331474514187995, 33.13161551792790505 ) ) ;
#61196=EDGE_CURVE ( 'NONE', #77096, #39874, #59453, .T. ) ;
#61197=DIRECTION ( 'NONE',  ( 0.000000000000000000, 0.6427876096865373645, -0.7660444431189797898 ) ) ;
#61198=CARTESIAN_POINT ( 'NONE',  ( 12.46153846153833911, -2.892918686052165622, 31.69288490824153470 ) ) ;
#61199=ORIENTED_EDGE ( 'NONE', *, *, #37757, .T. ) ;
#61200=CARTESIAN_POINT ( 'NONE',  ( 9.019176178608811156, -4.932303261841489928, 34.32971442181322885 ) ) ;
#61201=LINE ( 'NONE', #54008, #69024 ) ;
#61203=EDGE_CURVE ( 'NONE', #69402, #38647, #17490, .T. ) ;
#61204=B_SPLINE_CURVE_WITH_KNOTS ( 'NONE', 3,
 ( #46935, #87073, #80752, #80301, #45612, #73088, #33439, #39760, #18596, #46059 ),
 .UNSPECIFIED., .F., .F.,
 ( 4, 2, 2, 2, 4 ),
 ( 0.0007817246256747459798, 0.0009771112852218896347, 0.001172497944769033398, 0.001367884604316177161, 0.001563271263863320708 ),
 .UNSPECIFIED. ) ;
#61205=ADVANCED_FACE ( 'NONE', ( #58830 ), #66490, .F. ) ;
#61206=CARTESIAN_POINT ( 'NONE',  ( -9.692307692307814193, -11.06231777344772027, 33.60647404775119895 ) ) ;
#61207=DIRECTION ( 'NONE',  ( 0.000000000000000000, 0.8660254037844377084, 0.5000000000000015543 ) ) ;
#61208=CARTESIAN_POINT ( 'NONE',  ( 10.61538461538449596, -6.026961402154118019, 34.52809138561165270 ) ) ;
#61210=VERTEX_POINT ( 'NONE', #60606 ) ;
#61212=CARTESIAN_POINT ( 'NONE',  ( -16.15384615384615330, -4.102666532097928531, 36.13435417666054406 ) ) ;
#61213=VERTEX_POINT ( 'NONE', #32691 ) ;
#61214=CARTESIAN_POINT ( 'NONE',  ( -16.02305434602136458, -9.804649428959608670, 34.18742332936588468 ) ) ;
#61215=CARTESIAN_POINT ( 'NONE',  ( 0.3313912521002425060, -2.882441371585227508, 31.66841991370171527 ) ) ;
#61216=EDGE_LOOP ( 'NONE', ( #60803, #4056, #50362, #20734 ) ) ;
#61217=CARTESIAN_POINT ( 'NONE',  ( -10.61538461538461320, -3.937682226553329556, 33.60647404775216529 ) ) ;
#61218=CARTESIAN_POINT ( 'NONE',  ( 8.545745844666436497, -6.716662450894489211, 34.94144148231605840 ) ) ;
#61219=AXIS2_PLACEMENT_3D ( 'NONE', #20282, #57517, #16092 ) ;
#61220=CARTESIAN_POINT ( 'NONE',  ( 15.23076923076923173, -2.721908614388771852, 31.22303859784724978 ) ) ;
#61221=ORIENTED_EDGE ( 'NONE', *, *, #48318, .F. ) ;
#61222=ORIENTED_EDGE ( 'NONE', *, *, #80077, .T. ) ;
#61223=ORIENTED_EDGE ( 'NONE', *, *, #62683, .F. ) ;
#61224=CARTESIAN_POINT ( 'NONE',  ( -15.16470189741915320, -3.937682226553329556, 33.60647404775216529 ) ) ;
#61225=CARTESIAN_POINT ( 'NONE',  ( -0.4615384615384611200, -10.51840700105979565, 33.73612834413961536 ) ) ;
#61226=DIRECTION ( 'NONE',  ( 0.000000000000000000, 0.8660254037844377084, 0.5000000000000015543 ) ) ;
#61227=CARTESIAN_POINT ( 'NONE',  ( 9.627037691751374027, -9.528491918058357157, 34.59228464037090589 ) ) ;
#61228=VECTOR ( 'NONE', #9423, 1000.000000000000227 ) ;
#61229=CARTESIAN_POINT ( 'NONE',  ( -2.531177251416254492, -5.912607949931405038, 34.49155766932282319 ) ) ;
#61230=FACE_OUTER_BOUND ( 'NONE', #4470, .T. ) ;
#61232=CYLINDRICAL_SURFACE ( 'NONE', #70829, 0.2499999999999994726 ) ;
#61233=ADVANCED_FACE ( 'NONE', ( #60162, #52957, #87666, #4791, #53405, #80906, #32264, #19189, #88121, #59727, #52071, #3881, #72344, #10654, #74132, #12429, #38121, #17860, #65581, #45313, #72786, #11096, #38573, #66027, #4336, #31823, #59277, #86783, #56071, #68698, #48868, #61490, #21401, #47088, #75026, #28151, #75901, #27708, #75457, #20946, #14202, #76339, #7889, #35355, #88997, #41677, #83109, #82675, #6119, #74579, #40352, #62370, #55179, #14647, #69145, #55620, #7451, #42130, #27270, #13314, #48417, #69584, #33593, #54734, #245, #40795, #34906, #13753, #62809, #41235, #1128, #61052, #684, #28608, #19626, #6999, #12867, #67819, #34471, #88557, #26833, #54287, #81784, #20074, #47532, #82223, #68259, #61931, #6561, #20512, #34025, #47976, #15981, #2881, #71348, #77668, #84888, #71794, #22719, #35813, #42566, #9654, #29497, #44304, #43446, #36691, #2015, #30810, #70921, #23607, #36254, #85325, #21844, #49751, #30373, #50636, #2444, #50184, #23171, #78115, #9230, #10099, #37563, #63708, #16416, #57843, #57393, #70027, #64142, #43882, #37118, #29936, #65028, #29062, #3339, #83563, #63267, #49319, #64583, #51058, #1574, #78552, #16857, #76796, #15093, #8337, #56517, #77226, #84007, #8782, #22287, #15536, #43005, #70478, #56950, #84446, #65487, #32591, #53302, #65923, #87565, #73600, #39807, #17303, #67275, #74037, #18200, #32159, #38922, #39370, #12328, #44761, #59619, #24051, #5570, #72240, #52856, #85770, #51500, #11893, #66827, #72689, #58278, #3785, #73139, #10552, #86679, #17757, #31263, #60061, #80803, #4233, #25845, #19086, #58727, #38471, #46113, #79003, #38022, #86226, #24495, #5125, #18651, #45662, #51962, #46554, #87119, #79458, #45211, #10998, #80353, #31716, #25397, #59174, #24944, #11439, #52410, #79898, #66380, #4687, #6022, #34807, #13217, #88454, #6895, #27167, #28059, #47429, #62274, #88022, #74924, #40696, #54185, #14544, #27610, #7352, #33922, #21293, #61383, #74471, #81238, #20851, #68160, #83009, #54627, #75363, #6463, #69485, #82124, #590, #88897, #55523, #60510, #26724, #41571, #144, #41133, #20417, #34364, #55083, #47882, #48765, #76236, #13654, #82579, #42026, #61833, #19523, #26282, #53750, #75796, #68598, #33043, #46984, #12766, #67718, #48321, #14101, #40253, #33491, #60950, #69044, #81681, #19962, #8239, #36161, #50091, #16318, #57298, #84347, #62714, #43783, #36592, #76692, #83461, #7788, #2341, #28506, #64044, #1030, #63163, #63609, #83906, #55966, #14995, #49657, #84791, #9552, #77131, #1477, #71245, #42468, #44205, #69928, #29835, #70378, #23075, #50960, #1914, #85223, #2776, #37017, #21743, #15441, #42915, #28964, #78449, #50532, #64478, #8685, #49216, #35712, #15884, #29402, #56851, #16750, #35254, #56418, #22191, #22623, #77576, #43348, #30277, #57746, #70826, #9130, #23504, #78013, #40485, #10450, #44652, #40045, #53530, #9992, #72137, #81914, #86568, #38364, #71692, #81027, #58175, #67949, #79350, #12999, #6252, #17195, #51853, #60737, #54418, #3237, #37462, #64932, #30708, #33277, #23942, #72586, #17653, #24837, #85665, #26518, #61171, #19756, #20203, #51393, #67506, #19316, #46785, #4119, #81471, #88244, #65818, #74262, #88684, #10892, #78898, #37920, #65383, #33715, #47218, #31603, #59069, #45110, #3676, #12559, #26961, #24388, #74712, #31147, #58619, #86113, #5800, #53981, #14324, #48995, #42253, #62495, #29188, #82353, #35936, #56640, #34151, #55305, #809, #61618, #1246, #63389, #28276, #83234, #7129, #84133, #76474, #8016, #21520, #35483, #82796, #8463, #41809, #55746, #21070, #47668, #7574, #20635, #69710, #48538, #14776, #1697, #69271, #75154, #42692, #62064, #62934, #28736, #15220, #13438, #40917, #76020, #56199, #27840, #68381, #35035, #83689, #89123, #6679, #21973, #49444, #27399, #376, #76917, #70152, #54869, #48100, #75575, #13877, #41358, #68824, #34598, #84571, #31382, #37239, #78232, #22409, #85007, #22845, #57521, #44001, #58847, #37690, #3896, #70599, #49874, #57076, #77354, #15661, #71918, #63837, #23288, #30056, #64711, #8904, #65156, #10672, #58391, #51177, #2132, #36374, #43131, #16980, #29620, #78685, #50309, #77792, #3010, #30923, #85887, #16096, #43562, #71037, #44429, #50748, #10231, #65596, #16533, #17429, #36807, #24172, #9350, #64265, #30492, #2565, #3457, #38138, #57963, #85443, #71470, #9778, #51624, #79128, #23723, #44884, #72361, #47103, #39490, #5683, #33159, #4355, #33607, #59293, #80921, #59743, #53419, #40373, #80469, #74595, #81358, #11565, #19207, #32708, #53873, #12882, #67833, #39045, #60621, #87237, #79580, #72803, #31838, #26406, #5244, #39931, #19642, #11111, #66503, #66950, #80016, #60177, #18765, #6133, #46231, #86353, #38587, #46672, #12013, #66042, #67389, #24623, #87680, #25955, #45780, #52089, #74149, #12445, #88134, #17876, #32278, #45331, #73719, #86800, #4808, #25070, #52532, #18317, #73259, #52972, #25516, #55635, #75918, #42584, #6577, #49336, #70044, #13329, #8354, #42147, #28168, #40811, #75471, #13769, #7907, #7013, #28626, #89013, #54754, #20089, #41252, #61069, #68274, #14218, #47552, #262, #20528, #34044, #35372, #56088, #68717, #1145, #83583, #88576, #75043, #83126, #69164, #34923, #14665, #76814, #41691, #7469, #47992, #26848, #702, #21417, #62386, #48886, #34487, #21859, #55196, #76357, #61952, #54305, #20961, #15111, #27724, #62825, #69602, #81800, #82691, #61506, #27287, #48432, #82240, #71366, #3358, #24075, #51522, #77684, #43462, #72261, #84906, #65049, #15997, #37586, #63283, #2029 ), #85343, .F. ) ;
#61234=ORIENTED_EDGE ( 'NONE', *, *, #36357, .F. ) ;
#61235=ORIENTED_EDGE ( 'NONE', *, *, #61460, .F. ) ;
#61236=CARTESIAN_POINT ( 'NONE',  ( -0.2114841499001473557, -12.17597550085003455, 31.52189283813461884 ) ) ;
#61237=ORIENTED_EDGE ( 'NONE', *, *, #75042, .T. ) ;
#61238=VECTOR ( 'NONE', #25648, 1000.000000000000000 ) ;
#61239=CARTESIAN_POINT ( 'NONE',  ( -5.999999999999998224, -12.78798330534102945, 29.74999999999997868 ) ) ;
#61240=CARTESIAN_POINT ( 'NONE',  ( 2.307692307692309264, -1.129524287112498415, 32.06866353760679544 ) ) ;
#61242=CARTESIAN_POINT ( 'NONE',  ( 15.29602437028206907, -9.528491918058460186, 34.59228464037086326 ) ) ;
#61243=EDGE_CURVE ( 'NONE', #8131, #58342, #66943, .T. ) ;
#61245=VERTEX_POINT ( 'NONE', #29081 ) ;
#61246=CARTESIAN_POINT ( 'NONE',  ( 17.32697749683652688, -9.233818618650598609, 34.70587769442853698 ) ) ;
#61247=ORIENTED_EDGE ( 'NONE', *, *, #76329, .F. ) ;
#61248=CARTESIAN_POINT ( 'NONE',  ( -10.74586132350107981, -7.276988635370452485, 34.74523720219453793 ) ) ;
#61249=VERTEX_POINT ( 'NONE', #56535 ) ;
#61250=CARTESIAN_POINT ( 'NONE',  ( -12.21159305216042057, -10.18230066228895758, 34.26354781536631577 ) ) ;
#61251=CARTESIAN_POINT ( 'NONE',  ( 12.33139049180676672, -2.373036134822904319, 30.88089517874952250 ) ) ;
#61252=FACE_BOUND ( 'NONE', #78088, .T. ) ;
#61253=CARTESIAN_POINT ( 'NONE',  ( 5.934729999443682402, -2.379036618887870436, 30.90682066428147934 ) ) ;
#61254=CARTESIAN_POINT ( 'NONE',  ( -8.769230769230768274, -11.11383981884818262, 36.00935417666054406 ) ) ;
#61255=EDGE_CURVE ( 'NONE', #76768, #4390, #46525, .T. ) ;
#61256=LINE ( 'NONE', #33365, #75505 ) ;
#61257=CARTESIAN_POINT ( 'NONE',  ( -13.38461538461538325, -2.292212530054420494, 30.41441678777542634 ) ) ;
#61258=FACE_OUTER_BOUND ( 'NONE', #69177, .T. ) ;
#61259=CARTESIAN_POINT ( 'NONE',  ( -13.13461538461538325, -2.499999999999998668, 29.75000000000000355 ) ) ;
#61260=EDGE_CURVE ( 'NONE', #40886, #22606, #9977, .T. ) ;
#61262=VERTEX_POINT ( 'NONE', #84463 ) ;
#61263=LINE ( 'NONE', #54969, #18753 ) ;
#61264=CARTESIAN_POINT ( 'NONE',  ( 2.557637826040450424, -10.76462480002816235, 33.53768742498949962 ) ) ;
#61265=B_SPLINE_CURVE_WITH_KNOTS ( 'NONE', 3,
 ( #22705, #77652, #43432, #36674, #57375, #2429, #29921, #84871, #23154, #50620 ),
 .UNSPECIFIED., .F., .F.,
 ( 4, 2, 2, 2, 4 ),
 ( 0.0007817359430256365111, 0.0009771253907250043464, 0.001172514838424372399, 0.001367904286123740234, 0.001563293733823108069 ),
 .UNSPECIFIED. ) ;
#61266=CARTESIAN_POINT ( 'NONE',  ( 3.100078627658922503, -3.338472653186242756, 32.95098750199972670 ) ) ;
#61267=DIRECTION ( 'NONE',  ( -0.000000000000000000, 0.1736481776669307198, -0.9848077530122080203 ) ) ;
#61268=CARTESIAN_POINT ( 'NONE',  ( 6.923076923076800782, -5.094484230521993062, 34.41647553114689373 ) ) ;
#61269=CARTESIAN_POINT ( 'NONE',  ( -12.39628332202562433, -5.094484230520773593, 34.41647553114626845 ) ) ;
#61270=ORIENTED_EDGE ( 'NONE', *, *, #15242, .F. ) ;
#61271=CARTESIAN_POINT ( 'NONE',  ( -11.78843826940389405, -12.17611988154120972, 31.52148481390971213 ) ) ;
#61272=CARTESIAN_POINT ( 'NONE',  ( 14.98079248672064345, -4.075325502946081535, 33.72974371597206300 ) ) ;
#61274=EDGE_CURVE ( 'NONE', #3673, #41031, #86268, .T. ) ;
#61278=ORIENTED_EDGE ( 'NONE', *, *, #46259, .F. ) ;
#61279=EDGE_CURVE ( 'NONE', #63347, #41758, #16876, .T. ) ;
#61280=CARTESIAN_POINT ( 'NONE',  ( 16.15384615384615330, -2.499999999999998668, 29.50000000000001066 ) ) ;
#61281=ORIENTED_EDGE ( 'NONE', *, *, #70350, .F. ) ;
#61282=EDGE_CURVE ( 'NONE', #12918, #41880, #54016, .T. ) ;
#61284=CARTESIAN_POINT ( 'NONE',  ( 4.153846153846030731, -11.67786785259630911, 32.92929555188603530 ) ) ;
#61285=CARTESIAN_POINT ( 'NONE',  ( 15.16549878480845770, -9.442884908240170461, 34.35708131394840592 ) ) ;
#61286=CARTESIAN_POINT ( 'NONE',  ( 3.480823650682683734, -5.642605341092957083, 34.66089969410670335 ) ) ;
#61287=CARTESIAN_POINT ( 'NONE',  ( 1.384615384615386802, -6.343179335718451384, 34.87096338111211935 ) ) ;
#61288=CARTESIAN_POINT ( 'NONE',  ( -11.53846153846165912, -6.879047030192662504, 34.71129190930017927 ) ) ;
#61290=CARTESIAN_POINT ( 'NONE',  ( 4.376857505459002873, -4.187068189119697692, 33.49521262558774026 ) ) ;
#61292=ORIENTED_EDGE ( 'NONE', *, *, #11963, .T. ) ;
#61293=CARTESIAN_POINT ( 'NONE',  ( -6.923076923077045919, -5.941354392335915335, 34.76329471203413846 ) ) ;
#61294=CARTESIAN_POINT ( 'NONE',  ( -3.230769230769352962, -2.657715359629662544, 31.77849191805970364 ) ) ;
#61295=CARTESIAN_POINT ( 'NONE',  ( -10.86538461538461320, -7.500000000000001776, 35.00000000000000000 ) ) ;
#61297=DIRECTION ( 'NONE',  ( -0.000000000000000000, 0.8660254037844397068, -0.4999999999999978906 ) ) ;
#61298=EDGE_CURVE ( 'NONE', #71149, #53698, #13182, .T. ) ;
#61300=CARTESIAN_POINT ( 'NONE',  ( 12.68431800280686517, -11.41317474335729543, 32.86274602512330034 ) ) ;
#61302=ORIENTED_EDGE ( 'NONE', *, *, #40439, .T. ) ;
#61303=CARTESIAN_POINT ( 'NONE',  ( -13.38461538461538325, -8.120952969808772792, 34.71129190930000163 ) ) ;
#61304=CARTESIAN_POINT ( 'NONE',  ( -15.23076923076922995, -1.129524287112498415, 32.06866353760679544 ) ) ;
#61306=AXIS2_PLACEMENT_3D ( 'NONE', #73304, #11608, #39088 ) ;
#61307=EDGE_LOOP ( 'NONE', ( #44188, #61660 ) ) ;
#61308=EDGE_CURVE ( 'NONE', #82157, #70706, #60083, .T. ) ;
#61309=ORIENTED_EDGE ( 'NONE', *, *, #46415, .F. ) ;
#61310=CARTESIAN_POINT ( 'NONE',  ( 9.692307692307572609, -2.625532179533778709, 30.86335684631627174 ) ) ;
#61311=CARTESIAN_POINT ( 'NONE',  ( -5.299849294439222369, -6.503392248772476236, 34.64988816332204635 ) ) ;
#61312=VECTOR ( 'NONE', #26231, 1000.000000000000000 ) ;
#61313=CARTESIAN_POINT ( 'NONE',  ( -10.86536135943320502, -2.318417181685855422, 30.59732222474233865 ) ) ;
#61314=DIRECTION ( 'NONE',  ( -0.000000000000000000, -0.6427876096865404731, -0.7660444431189771253 ) ) ;
#61315=CARTESIAN_POINT ( 'NONE',  ( -14.37296230824862953, -3.083524468853724443, 32.58852847137143272 ) ) ;
#61316=VERTEX_POINT ( 'NONE', #88045 ) ;
#61317=CARTESIAN_POINT ( 'NONE',  ( 12.46153846153877609, -2.255955759149395501, 30.00000000000324363 ) ) ;
#61318=CARTESIAN_POINT ( 'NONE',  ( -12.46153846153846168, -5.180354513474913603, 36.12317359536750416 ) ) ;
#61319=CARTESIAN_POINT ( 'NONE',  ( 1.634615384615386580, -2.499999999999998668, 29.75000000000000355 ) ) ;
#61320=ORIENTED_EDGE ( 'NONE', *, *, #35663, .F. ) ;
#61321=CARTESIAN_POINT ( 'NONE',  ( -4.153846153846152411, -3.937682226553329556, 33.60647404775216529 ) ) ;
#61322=ORIENTED_EDGE ( 'NONE', *, *, #66349, .T. ) ;
#61323=CARTESIAN_POINT ( 'NONE',  ( -16.37677237136229991, -5.667676309546437530, 34.40238873228292249 ) ) ;
#61325=CARTESIAN_POINT ( 'NONE',  ( -5.776987155906605054, -11.98016756924215009, 32.48728574198911190 ) ) ;
#61326=ORIENTED_EDGE ( 'NONE', *, *, #14276, .T. ) ;
#61328=DIRECTION ( 'NONE',  ( -0.000000000000000000, 0.8660254037844397068, -0.4999999999999978906 ) ) ;
#61329=CARTESIAN_POINT ( 'NONE',  ( -11.60454494941741999, -6.386643153685125363, 34.62446782046654903 ) ) ;
#61330=EDGE_CURVE ( 'NONE', #82159, #72717, #74059, .T. ) ;
#61331=CARTESIAN_POINT ( 'NONE',  ( 6.923076923076924238, -12.34228464037088635, 31.77849191805839268 ) ) ;
#61332=CARTESIAN_POINT ( 'NONE',  ( 18.00000000000000000, -8.564572088678739092, 35.78748833219616898 ) ) ;
#61333=EDGE_CURVE ( 'NONE', #75057, #16191, #41097, .T. ) ;
#61334=VECTOR ( 'NONE', #83602, 1000.000000000000227 ) ;
#61335=ORIENTED_EDGE ( 'NONE', *, *, #84358, .F. ) ;
#61336=FACE_BOUND ( 'NONE', #5718, .T. ) ;
#61337=ORIENTED_EDGE ( 'NONE', *, *, #45977, .F. ) ;
#61338=CARTESIAN_POINT ( 'NONE',  ( -8.519285250882628446, -4.336752205174649433, 33.62275283266504289 ) ) ;
#61339=ADVANCED_FACE ( 'NONE', ( #66402 ), #11019, .F. ) ;
#61340=ADVANCED_FACE ( 'NONE', ( #19546 ), #25419, .T. ) ;
#61341=DIRECTION ( 'NONE',  ( 0.000000000000000000, 0.9396926207859126468, -0.3420201433256571111 ) ) ;
#61342=ADVANCED_FACE ( 'NONE', ( #5148 ), #38042, .F. ) ;
#61343=CARTESIAN_POINT ( 'NONE',  ( -18.22292695890684655, -10.77366814457252175, 33.85459836347580875 ) ) ;
#61344=VECTOR ( 'NONE', #57553, 1000.000000000000000 ) ;
#61346=CARTESIAN_POINT ( 'NONE',  ( -11.40793583669797506, -2.619367082507849442, 30.83698974864643461 ) ) ;
#61347=VERTEX_POINT ( 'NONE', #80377 ) ;
#61348=EDGE_CURVE ( 'NONE', #65223, #82999, #86700, .T. ) ;
#61349=ORIENTED_EDGE ( 'NONE', *, *, #7910, .T. ) ;
#61351=ORIENTED_EDGE ( 'NONE', *, *, #58021, .F. ) ;
#61352=CARTESIAN_POINT ( 'NONE',  ( -5.011667505647053211, -5.219633306516380244, 34.19971097300157936 ) ) ;
#61353=CARTESIAN_POINT ( 'NONE',  ( -16.94687791408830080, -2.504778602574659896, 29.97347330155780654 ) ) ;
#61354=CARTESIAN_POINT ( 'NONE',  ( 4.946775107191379028, -11.66186481527757479, 32.95055677023626117 ) ) ;
#61355=VERTEX_POINT ( 'NONE', #67298 ) ;
#61356=B_SPLINE_CURVE_WITH_KNOTS ( 'NONE', 3,
 ( #54244, #40312, #67774, #81740, #20024, #6521, #22679, #84401, #63218, #8295 ),
 .UNSPECIFIED., .F., .F.,
 ( 4, 2, 2, 2, 4 ),
 ( 0.0007817359430256282712, 0.0009771253907249945886, 0.001172514838424360689, 0.001367904286123726790, 0.001563293733823093107 ),
 .UNSPECIFIED. ) ;
#61357=CARTESIAN_POINT ( 'NONE',  ( -13.38461538461538325, -6.435427911321262684, 35.78748833219616898 ) ) ;
#61358=CARTESIAN_POINT ( 'NONE',  ( -2.307692307692305711, -13.20930481340135110, 34.54067556320372745 ) ) ;
#61359=DIRECTION ( 'NONE',  ( 0.000000000000000000, 0.7660444431189822323, -0.6427876096865344779 ) ) ;
#61360=CARTESIAN_POINT ( 'NONE',  ( 11.53846153846153832, -9.780366693483667717, 34.19971097300155094 ) ) ;
#61361=VERTEX_POINT ( 'NONE', #87141 ) ;
#61362=B_SPLINE_CURVE_WITH_KNOTS ( 'NONE', 3,
 ( #34379, #61844, #86487, #4494, #81055, #74289, #12588, #53562, #18459, #31519 ),
 .UNSPECIFIED., .F., .F.,
 ( 4, 2, 2, 2, 4 ),
 ( 0.000000000000000000, 0.0001954339857564078538, 0.0003908679715128157077, 0.0005863019572692235344, 0.0007817359430256314154 ),
 .UNSPECIFIED. ) ;
#61363=EDGE_CURVE ( 'NONE', #10767, #34572, #24966, .T. ) ;
#61364=VERTEX_POINT ( 'NONE', #11460 ) ;
#61365=AXIS2_PLACEMENT_3D ( 'NONE', #52700, #44597, #85605 ) ;
#61366=ORIENTED_EDGE ( 'NONE', *, *, #26554, .F. ) ;
#61367=DIRECTION ( 'NONE',  ( -0.000000000000000000, -0.1736481776669307198, -0.9848077530122080203 ) ) ;
#61368=EDGE_CURVE ( 'NONE', #13051, #27912, #25865, .T. ) ;
#61369=CARTESIAN_POINT ( 'NONE',  ( -1.450697763975518528, -2.486705287966279876, 31.30864560766542937 ) ) ;
#61370=CARTESIAN_POINT ( 'NONE',  ( -7.623141002060451754, -9.172514111537584114, 34.72667873470787470 ) ) ;
#61371=CARTESIAN_POINT ( 'NONE',  ( 16.08852214104184242, -7.749976730030849303, 34.74374725381503737 ) ) ;
#61372=CARTESIAN_POINT ( 'NONE',  ( -9.915792636031639518, -6.760086850603066466, 34.69517049084099369 ) ) ;
#61373=FACE_BOUND ( 'NONE', #43156, .T. ) ;
#61374=ORIENTED_EDGE ( 'NONE', *, *, #15790, .T. ) ;
#61376=CARTESIAN_POINT ( 'NONE',  ( 15.23076923076923173, -2.721908614388771852, 31.22303859784724978 ) ) ;
#61377=CARTESIAN_POINT ( 'NONE',  ( 17.07692307692295586, -6.879047030192662504, 34.71129190930017927 ) ) ;
#61378=CYLINDRICAL_SURFACE ( 'NONE', #49595, 0.2499999999999994726 ) ;
#61379=VERTEX_POINT ( 'NONE', #13676 ) ;
#61380=CARTESIAN_POINT ( 'NONE',  ( 17.20771351789003489, -5.496552790871120031, 34.60292014791297532 ) ) ;
#61381=B_SPLINE_CURVE_WITH_KNOTS ( 'NONE', 3,
 ( #10694, #38160, #52112, #39513, #39069, #86374, #38610, #30947, #46255, #65618 ),
 .UNSPECIFIED., .F., .F.,
 ( 4, 2, 2, 2, 4 ),
 ( 0.0007817246256747517261, 0.0009771112852218961399, 0.001172497944769040771, 0.001367884604316185401, 0.001563271263863329815 ),
 .UNSPECIFIED. ) ;
#61383=FACE_BOUND ( 'NONE', #43476, .T. ) ;
#61384=CARTESIAN_POINT ( 'NONE',  ( 9.626224281351813516, -5.557115091759785130, 34.35708131394839171 ) ) ;
#61385=ORIENTED_EDGE ( 'NONE', *, *, #6508, .T. ) ;
#61386=DIRECTION ( 'NONE',  ( -0.000000000000000000, -0.9848077530122086864, -0.1736481776669273613 ) ) ;
#61387=CARTESIAN_POINT ( 'NONE',  ( -12.59222906464876779, -11.93127051446799847, 32.56575433478202797 ) ) ;
#61388=CARTESIAN_POINT ( 'NONE',  ( 1.161689167099237752, -3.105860786376062332, 32.13614157043599562 ) ) ;
#61390=CARTESIAN_POINT ( 'NONE',  ( -8.769230769230892619, -3.643525952248795718, 33.31231777344771672 ) ) ;
#61391=FACE_OUTER_BOUND ( 'NONE', #35789, .T. ) ;
#61392=CARTESIAN_POINT ( 'NONE',  ( 6.923076923076802558, -12.46129190930018460, 30.37095296980731973 ) ) ;
#61393=CARTESIAN_POINT ( 'NONE',  ( 2.438217745925950641, -3.068774925481847493, 32.56582465632704526 ) ) ;
#61395=CARTESIAN_POINT ( 'NONE',  ( 13.38461538461538680, -5.557115091759785130, 34.35708131394839171 ) ) ;
#61396=CARTESIAN_POINT ( 'NONE',  ( 2.438482748659259958, -3.338503747796865984, 32.95102852606552801 ) ) ;
#61397=CARTESIAN_POINT ( 'NONE',  ( -8.899377978668990608, -3.817052484675422797, 33.13202310037935661 ) ) ;
#61398=VERTEX_POINT ( 'NONE', #75817 ) ;
#61399=CARTESIAN_POINT ( 'NONE',  ( 5.076923076923075762, -5.557115091759785130, 34.35708131394839171 ) ) ;
#61400=CARTESIAN_POINT ( 'NONE',  ( 15.90382292962469890, -4.175268141568689195, 33.81360843649122216 ) ) ;
#61401=CARTESIAN_POINT ( 'NONE',  ( 6.000000000000001776, -8.973038597847269315, 34.52809138561121927 ) ) ;
#61402=CARTESIAN_POINT ( 'NONE',  ( 13.51514108637895006, -12.45806712695776319, 30.39783852428763922 ) ) ;
#61403=CARTESIAN_POINT ( 'NONE',  ( -13.16160403300253634, -3.587049720035815348, 32.86302985866382897 ) ) ;
#61405=CARTESIAN_POINT ( 'NONE',  ( -12.46153846153846168, -10.67929555188718282, 33.92786785259544047 ) ) ;
#61406=CARTESIAN_POINT ( 'NONE',  ( -1.450698795571263577, -4.786620604624113540, 33.94971097300155805 ) ) ;
#61407=CARTESIAN_POINT ( 'NONE',  ( -16.85391172531022619, -8.239487800360276282, 34.69522927552633718 ) ) ;
#61408=EDGE_CURVE ( 'NONE', #25915, #22155, #163, .T. ) ;
#61409=EDGE_CURVE ( 'NONE', #41880, #12918, #16595, .T. ) ;
#61410=B_SPLINE_CURVE_WITH_KNOTS ( 'NONE', 3,
 ( #22425, #77369, #13895, #21538, #42708, #76490, #83251, #56655, #49460, #1713 ),
 .UNSPECIFIED., .F., .F.,
 ( 4, 2, 2, 2, 4 ),
 ( 0.0007817359430256301143, 0.0009771253907249963233, 0.001172514838424362641, 0.001367904286123728958, 0.001563293733823095059 ),
 .UNSPECIFIED. ) ;
#61411=CYLINDRICAL_SURFACE ( 'NONE', #59366, 0.2499999999999995559 ) ;
#61414=VECTOR ( 'NONE', #71415, 1000.000000000000227 ) ;
#61415=B_SPLINE_CURVE_WITH_KNOTS ( 'NONE', 3,
 ( #14871, #13969, #82001, #8107, #464, #68468, #35579, #49535, #76111, #55838 ),
 .UNSPECIFIED., .F., .F.,
 ( 4, 2, 2, 2, 4 ),
 ( 0.000000000000000000, 0.0001954311564186865763, 0.0003908623128373731525, 0.0005862934692560596746, 0.0007817246256747463051 ),
 .UNSPECIFIED. ) ;
#61416=CARTESIAN_POINT ( 'NONE',  ( -8.769230769230890843, -12.27809138561165270, 31.22303859784587132 ) ) ;
#61418=EDGE_CURVE ( 'NONE', #6801, #27837, #86510, .T. ) ;
#61419=ORIENTED_EDGE ( 'NONE', *, *, #70181, .T. ) ;
#61421=EDGE_CURVE ( 'NONE', #81196, #86663, #55989, .T. ) ;
#61422=AXIS2_PLACEMENT_3D ( 'NONE', #51677, #17482, #44933 ) ;
#61423=VERTEX_POINT ( 'NONE', #14121 ) ;
#61426=CARTESIAN_POINT ( 'NONE',  ( 14.55763782604045176, -11.37275283266504111, 32.91324779482534524 ) ) ;
#61427=LINE ( 'NONE', #68201, #72613 ) ;
#61428=CARTESIAN_POINT ( 'NONE',  ( 3.007284287045282500, -8.496056993536548418, 34.65000542017679663 ) ) ;
#61429=DIRECTION ( 'NONE',  ( 0.000000000000000000, 1.000000000000000000, 0.000000000000000000 ) ) ;
#61430=CARTESIAN_POINT ( 'NONE',  ( -11.53846153846165912, -11.48612834414049644, 32.76840700105863391 ) ) ;
#61431=DIRECTION ( 'NONE',  ( -0.000000000000000000, 0.1736481776669307198, -0.9848077530122080203 ) ) ;
#61432=EDGE_CURVE ( 'NONE', #42225, #17613, #1632, .T. ) ;
#61433=LINE ( 'NONE', #20011, #42214 ) ;
#61434=CYLINDRICAL_SURFACE ( 'NONE', #34780, 0.2499999999999995559 ) ;
#61435=CARTESIAN_POINT ( 'NONE',  ( -17.75005459062195712, -2.341251567377310217, 30.72681386836322659 ) ) ;
#61436=EDGE_CURVE ( 'NONE', #62595, #52583, #14563, .T. ) ;
#61440=CARTESIAN_POINT ( 'NONE',  ( -17.86943940825808852, -12.49523960252712484, 29.97295953869786800 ) ) ;
#61441=CARTESIAN_POINT ( 'NONE',  ( 0.4615384615384611200, -11.91647553114624181, 32.58852847137148245 ) ) ;
#61442=DIRECTION ( 'NONE',  ( 0.000000000000000000, 0.6427876096865368094, 0.7660444431189802339 ) ) ;
#61443=EDGE_CURVE ( 'NONE', #11769, #52068, #88920, .T. ) ;
#61444=DIRECTION ( 'NONE',  ( 0.000000000000000000, 0.7660444431189807890, 0.6427876096865361433 ) ) ;
#61445=CARTESIAN_POINT ( 'NONE',  ( 14.24242230713598900, -3.643525952247789412, 33.31231777344662959 ) ) ;
#61446=B_SPLINE_CURVE_WITH_KNOTS ( 'NONE', 3,
 ( #9443, #84677, #65259, #36040, #17083, #3116, #79236, #8566, #63495, #77460 ),
 .UNSPECIFIED., .F., .F.,
 ( 4, 2, 2, 2, 4 ),
 ( 0.0007817246256747463051, 0.0009771112852218896347, 0.001172497944769033181, 0.001367884604316176728, 0.001563271263863320057 ),
 .UNSPECIFIED. ) ;
#61447=DIRECTION ( 'NONE',  ( 0.000000000000000000, 0.9848077530122072432, -0.1736481776669354937 ) ) ;
#61448=CARTESIAN_POINT ( 'NONE',  ( -0.4615384615384611200, -12.09954503811598769, 35.62045528018868623 ) ) ;
#61449=EDGE_CURVE ( 'NONE', #64747, #46752, #53137, .T. ) ;
#61450=ORIENTED_EDGE ( 'NONE', *, *, #16167, .F. ) ;
#61451=DIRECTION ( 'NONE',  ( -0.000000000000000000, -0.9848077530122086864, -0.1736481776669273891 ) ) ;
#61454=CARTESIAN_POINT ( 'NONE',  ( 5.076923076922953193, -11.06231777344772027, 33.60647404775119895 ) ) ;
#61455=CARTESIAN_POINT ( 'NONE',  ( -18.25000000000001066, -12.75000000000000178, 29.81889780837731152 ) ) ;
#61456=CARTESIAN_POINT ( 'NONE',  ( -4.153846153846152411, -11.91647553114624181, 32.58852847137148245 ) ) ;
#61458=CARTESIAN_POINT ( 'NONE',  ( -12.46153846153846168, -12.10708131394839349, 31.69288490824020244 ) ) ;
#61459=ORIENTED_EDGE ( 'NONE', *, *, #34619, .T. ) ;
#61460=EDGE_CURVE ( 'NONE', #63896, #64886, #72428, .T. ) ;
#61461=EDGE_LOOP ( 'NONE', ( #36694, #64653, #44975, #74642 ) ) ;
#61462=AXIS2_PLACEMENT_3D ( 'NONE', #38305, #3619, #51333 ) ;
#61463=EDGE_LOOP ( 'NONE', ( #68257, #44460 ) ) ;
#61464=EDGE_LOOP ( 'NONE', ( #29586, #24229 ) ) ;
#61465=EDGE_CURVE ( 'NONE', #861, #63608, #69654, .T. ) ;
#61466=CARTESIAN_POINT ( 'NONE',  ( 17.14217821643591932, -10.33852847137154107, 34.16647553114620450 ) ) ;
#61467=CARTESIAN_POINT ( 'NONE',  ( 4.853996859406927378, -10.61292498521070549, 33.66303323003028680 ) ) ;
#61468=AXIS2_PLACEMENT_3D ( 'NONE', #68231, #8304, #55146 ) ;
#61469=CARTESIAN_POINT ( 'NONE',  ( -3.296852641725110722, -9.780366693483667717, 34.19971097300155805 ) ) ;
#61470=B_SPLINE_CURVE_WITH_KNOTS ( 'NONE', 3,
 ( #59404, #80120, #52639, #19308, #40910, #5352, #39599, #18423, #53075, #12554 ),
 .UNSPECIFIED., .F., .F.,
 ( 4, 2, 2, 2, 4 ),
 ( 0.000000000000000000, 0.0001954339857564093717, 0.0003908679715128187434, 0.0005863019572692280881, 0.0007817359430256374869 ),
 .UNSPECIFIED. ) ;
#61471=CARTESIAN_POINT ( 'NONE',  ( -15.45369544828537656, -11.24512374952581872, 33.06303171183252942 ) ) ;
#61473=CARTESIAN_POINT ( 'NONE',  ( -15.48074597481781822, -2.544273027872575366, 31.48422191005632342 ) ) ;
#61475=ORIENTED_EDGE ( 'NONE', *, *, #34606, .F. ) ;
#61476=ADVANCED_FACE ( 'NONE', ( #16336 ), #50111, .F. ) ;
#61477=ORIENTED_EDGE ( 'NONE', *, *, #71839, .T. ) ;
#61478=ORIENTED_EDGE ( 'NONE', *, *, #82885, .T. ) ;
#61479=DIRECTION ( 'NONE',  ( -0.000000000000000000, 0.6427876096865404731, -0.7660444431189770143 ) ) ;
#61480=ORIENTED_EDGE ( 'NONE', *, *, #20852, .F. ) ;
#61481=ADVANCED_FACE ( 'NONE', ( #64067 ), #57762, .F. ) ;
#61482=CARTESIAN_POINT ( 'NONE',  ( -8.769230769230892619, -3.643525952248795718, 33.31231777344771672 ) ) ;
#61483=CARTESIAN_POINT ( 'NONE',  ( -12.33101302330482341, -12.15418822224088835, 32.17964115625579069 ) ) ;
#61484=B_SPLINE_CURVE_WITH_KNOTS ( 'NONE', 3,
 ( #59849, #32827, #54868, #88243, #46338, #18868, #26071, #26515, #39603, #73826 ),
 .UNSPECIFIED., .F., .F.,
 ( 4, 2, 2, 2, 4 ),
 ( 0.000000000000000000, 0.0001954339857564091278, 0.0003908679715128182556, 0.0005863019572692274375, 0.0007817359430256365111 ),
 .UNSPECIFIED. ) ;
#61487=CARTESIAN_POINT ( 'NONE',  ( -3.165513659493205623, -12.46129190930001052, 30.37095296980870174 ) ) ;
#61488=ORIENTED_EDGE ( 'NONE', *, *, #17655, .F. ) ;
#61490=FACE_BOUND ( 'NONE', #77645, .T. ) ;
#61491=DIRECTION ( 'NONE',  ( 0.000000000000000000, -6.938893903907222067E-15, 1.000000000000000000 ) ) ;
#61492=AXIS2_PLACEMENT_3D ( 'NONE', #36372, #2130, #2563 ) ;
#61493=CARTESIAN_POINT ( 'NONE',  ( 8.703147358274890166, -4.786620604624113540, 33.94971097300155805 ) ) ;
#61494=ORIENTED_EDGE ( 'NONE', *, *, #36232, .F. ) ;
#61495=CARTESIAN_POINT ( 'NONE',  ( -9.757577692864012775, -5.094484230520674117, 34.41647553114621161 ) ) ;
#61497=B_SPLINE_CURVE_WITH_KNOTS ( 'NONE', 3,
 ( #67321, #81728, #38973, #20012, #73649, #12813, #47475, #81288, #74973, #60555 ),
 .UNSPECIFIED., .F., .F.,
 ( 4, 2, 2, 2, 4 ),
 ( 0.0007817246256747524850, 0.0009771112852218972241, 0.001172497944769042072, 0.001367884604316186702, 0.001563271263863331550 ),
 .UNSPECIFIED. ) ;
#61498=CARTESIAN_POINT ( 'NONE',  ( 16.15384615384603251, -6.835583212225970762, 34.95778746994575670 ) ) ;
#61500=VERTEX_POINT ( 'NONE', #69948 ) ;
#61501=CARTESIAN_POINT ( 'NONE',  ( 11.60452988946397745, -3.050289026998446840, 32.03036669348366416 ) ) ;
#61502=CARTESIAN_POINT ( 'NONE',  ( -7.623374304885434327, -11.41317474335729543, 32.86274602512330034 ) ) ;
#61503=CARTESIAN_POINT ( 'NONE',  ( -16.21909608562023664, -2.255955759149247175, 30.00000000000014211 ) ) ;
#61505=DIRECTION ( 'NONE',  ( 0.000000000000000000, 0.7660444431189822323, -0.6427876096865344779 ) ) ;
#61506=FACE_BOUND ( 'NONE', #11081, .T. ) ;
#61507=CARTESIAN_POINT ( 'NONE',  ( 1.634615384616805889, -7.500000000000154543, 35.00000000000007105 ) ) ;
#61508=CARTESIAN_POINT ( 'NONE',  ( -17.32689982097166492, -10.82459398097509684, 33.81372124010185587 ) ) ;
#61510=CARTESIAN_POINT ( 'NONE',  ( 5.326868486301119532, -2.341251567377310217, 30.72681386836322659 ) ) ;
#61511=DIRECTION ( 'NONE',  ( -0.000000000000000000, -0.1736481776669307198, -0.9848077530122080203 ) ) ;
#61512=CARTESIAN_POINT ( 'NONE',  ( 15.23076923076911093, -10.21337939537710326, 33.94971097300076224 ) ) ;
#61513=CARTESIAN_POINT ( 'NONE',  ( 5.999999999999878320, -8.656820664282941280, 34.87096338111179961 ) ) ;
#61515=ORIENTED_EDGE ( 'NONE', *, *, #48386, .T. ) ;
#61516=CARTESIAN_POINT ( 'NONE',  ( 1.384615384615265343, -12.27809138561165270, 31.22303859784587132 ) ) ;
#61517=ORIENTED_EDGE ( 'NONE', *, *, #53337, .F. ) ;
#61518=CARTESIAN_POINT ( 'NONE',  ( 0.7115384615384637845, -2.499999999999999556, 29.81604066197450109 ) ) ;
#61519=ORIENTED_EDGE ( 'NONE', *, *, #22803, .T. ) ;
#61520=CARTESIAN_POINT ( 'NONE',  ( 12.46153846153846168, -13.53365097954675988, 30.81389545987213552 ) ) ;
#61521=EDGE_CURVE ( 'NONE', #51057, #7803, #64931, .T. ) ;
#61522=CARTESIAN_POINT ( 'NONE',  ( -14.30769230769230660, -3.937682226553329556, 33.60647404775216529 ) ) ;
#61524=EDGE_LOOP ( 'NONE', ( #82844, #413, #45276, #22523 ) ) ;
#61525=CARTESIAN_POINT ( 'NONE',  ( 18.25000000000006395, -7.434744860731433924, 35.00000000000000711 ) ) ;
#61527=CARTESIAN_POINT ( 'NONE',  ( 12.71153846153846168, -2.499999999999998668, 29.75000000000000355 ) ) ;
#61528=CARTESIAN_POINT ( 'NONE',  ( 4.853438133199127869, -5.113361153441932316, 34.14387501736621999 ) ) ;
#61530=CARTESIAN_POINT ( 'NONE',  ( 10.39245765647776309, -2.523278758544489797, 31.42238647778637528 ) ) ;
#61531=CARTESIAN_POINT ( 'NONE',  ( -12.21159305216042057, -8.476813868363244353, 34.90874843262270133 ) ) ;
#61533=ADVANCED_FACE ( 'NONE', ( #56438 ), #50977, .F. ) ;
#61535=CARTESIAN_POINT ( 'NONE',  ( 5.776515075435668223, -2.612411019501189813, 31.66733052389439962 ) ) ;
#61536=CARTESIAN_POINT ( 'NONE',  ( 14.17700084102474989, -5.582088688514999397, 34.36776431015576350 ) ) ;
#61537=ORIENTED_EDGE ( 'NONE', *, *, #41274, .T. ) ;
#61538=EDGE_CURVE ( 'NONE', #62944, #10070, #7999, .T. ) ;
#61539=CARTESIAN_POINT ( 'NONE',  ( -18.00000000000000000, -12.46687347288208159, 35.28035834855298702 ) ) ;
#61540=B_SPLINE_CURVE_WITH_KNOTS ( 'NONE', 3,
 ( #81863, #34101, #20150, #89072, #69658, #7964, #82744, #40869, #47618, #62013 ),
 .UNSPECIFIED., .F., .F.,
 ( 4, 2, 2, 2, 4 ),
 ( 0.0007817359430256288133, 0.0009771253907249948054, 0.001172514838424360689, 0.001367904286123726573, 0.001563293733823092457 ),
 .UNSPECIFIED. ) ;
#61542=CARTESIAN_POINT ( 'NONE',  ( -11.53846153846153655, -12.10708131394839349, 31.69288490824020244 ) ) ;
#61543=CARTESIAN_POINT ( 'NONE',  ( -16.37677311275299985, -10.77366814457252175, 33.85459836347579454 ) ) ;
#61544=EDGE_LOOP ( 'NONE', ( #88745, #28789, #72748, #48627 ) ) ;
#61545=CARTESIAN_POINT ( 'NONE',  ( -6.923076923076922462, -6.386643153685126251, 34.62446782046654192 ) ) ;
#61546=CARTESIAN_POINT ( 'NONE',  ( 16.37685899793955357, -2.523321265292116866, 31.42251411153756990 ) ) ;
#61547=CARTESIAN_POINT ( 'NONE',  ( -17.01075393596041962, -7.250054483168842268, 34.74374881642865631 ) ) ;
#61549=DIRECTION ( 'NONE',  ( -0.000000000000000000, -0.8660254037844399289, -0.4999999999999980016 ) ) ;
#61550=AXIS2_PLACEMENT_3D ( 'NONE', #13817, #75088, #75965 ) ;
#61551=CARTESIAN_POINT ( 'NONE',  ( 15.29602437028207085, -5.941354392334607049, 34.76329471203374055 ) ) ;
#61552=CARTESIAN_POINT ( 'NONE',  ( 16.15384615384603251, -9.442884908241554243, 34.35708131394783038 ) ) ;
#61553=EDGE_CURVE ( 'NONE', #2810, #10613, #12306, .T. ) ;
#61554=CARTESIAN_POINT ( 'NONE',  ( 4.826899839630110378, -4.335965774309649134, 33.62209801155881905 ) ) ;
#61555=FACE_OUTER_BOUND ( 'NONE', #3942, .T. ) ;
#61556=CARTESIAN_POINT ( 'NONE',  ( 8.769230769230768274, -6.189225973068211317, 35.74407628777942847 ) ) ;
#61557=VERTEX_POINT ( 'NONE', #3255 ) ;
#61558=ORIENTED_EDGE ( 'NONE', *, *, #27988, .F. ) ;
#61560=EDGE_CURVE ( 'NONE', #10726, #28342, #9129, .T. ) ;
#61565=EDGE_CURVE ( 'NONE', #10638, #22672, #5039, .T. ) ;
#61569=CARTESIAN_POINT ( 'NONE',  ( 15.93091993633000847, -4.887634598454295265, 34.01352882383564946 ) ) ;
#61570=VERTEX_POINT ( 'NONE', #58640 ) ;
#61571=CLOSED_SHELL ( 'NONE', ( #29021, #8123, #64879, #72068, #21945, #43758, #82758, #21399, #23546, #28045, #22779, #62403, #38079, #50279, #49066, #44772, #6081, #39011, #78515, #9838, #65211, #40559, #70379, #38796, #55964, #80781, #82516, #28862, #22767, #30883, #64528, #78949, #88992, #58440, #20704, #42516, #63668, #85161, #22543, #27636, #10111, #30664, #56910, #35565, #77662, #49982, #66279, #2946, #29252, #10022, #78153, #14658, #84438, #54808, #55936, #37650, #63080, #23372, #33238, #81444, #56008, #18664, #36303, #74776, #74303, #39840, #1000, #26776, #34078, #71530, #7919, #621, #43406, #31215, #5238, #49487, #29080, #28796, #69596, #18898, #37323, #65286, #21765, #67784, #57582, #18927, #73562, #55010, #9827, #27364, #31070, #85272, #1722, #57560, #55813, #21525, #6953, #18493, #19385, #72744, #9240, #3511, #22208, #40697, #25392, #36056, #33235, #31313, #20822, #62963, #67911, #73436, #18292, #15221, #56954, #29845, #29090, #65827, #59799, #60802, #41146, #68115, #6160, #7536, #22563, #18993, #19168, #51148, #15897, #1939, #9112, #6514, #608, #13107, #17766, #84456, #49721, #76392, #51422, #30355, #60643, #3186, #8952, #3743, #34668, #26548, #57714, #3951, #20063, #76878, #62880, #18039, #15201, #66302, #52156, #33440, #25290, #12098, #10223, #38113, #60303, #49717, #32025, #39917, #45713, #17141, #66221, #14697, #66927, #86274, #77312, #10799, #44298, #57009, #15352, #47351, #53978, #80679, #75540, #74728, #22805, #49782, #81225, #72903, #85825, #85248, #10143, #37902, #45834, #43062, #64137, #44303, #62094, #8177, #53118, #9509, #6310, #2964, #31763, #42747, #27499, #10444, #43912, #3330, #75614, #66305, #83539, #33541, #86660, #41208, #56120, #88996, #74535, #38754, #58969, #43246, #84393, #87864, #69947, #31790, #78281, #86849, #14155, #45404, #51437, #83952, #39333, #44250, #76257, #17215, #4245, #6959, #70957, #58260, #21113, #44967, #2661, #43944, #73360, #63141, #76668, #83426, #34334, #73461, #15421, #59180, #70314, #59071, #39565, #53710, #75879, #71909, #55213, #56058, #9621, #30980, #54991, #63697, #70865, #83077, #79971, #66906, #74503, #45560, #60338, #39154, #68286, #12496, #49223, #46704, #83359, #10649, #59583, #72512, #5447, #35276, #41362, #63511, #77766, #10187, #34441, #27800, #30545, #59954, #12363, #45244, #82957, #43268, #30721, #18462, #16469, #19428, #61866, #2205, #21295, #77228, #2440, #46624, #44000, #86145, #14477, #69255, #43081, #83006, #6753, #13802, #48269, #71426, #86649, #38255, #37049, #28266, #76624, #64766, #40357, #85731, #10177, #8896, #29901, #32873, #47477, #77778, #60842, #57347, #71264, #70089, #3396, #54948, #10400, #31333, #34324, #5767, #23621, #34852, #29027, #15327, #2461, #83841, #60796, #11849, #66294, #15851, #48381, #26685, #46602, #71777, #55246, #40967, #15061, #64047, #26354, #27254, #81206, #10434, #52753, #11222, #3597, #4171, #77247, #74201, #78147, #15838, #21263, #74281, #50198, #7431, #57910, #21892, #20762, #34768, #55487, #34641, #26607, #88751, #51652, #75314, #26330, #21547, #66905, #70050, #71070, #67979, #71644, #9189, #74109, #9705, #82906, #49287, #13188, #40639, #87301, #87209, #57300, #39318, #14322, #43101, #17307, #40836, #80324, #17950, #35145, #57733, #18524, #14148, #74031, #38787, #43703, #64840, #40977, #9597, #49075, #76823, #28784, #16309, #47268, #43214, #46111, #89156, #16129, #22929, #40758, #77782, #53196, #40005, #43790, #65010, #81628, #51598, #24171, #62665, #82890, #86433, #15719, #79629, #65724, #19575, #60241, #76152, #26631, #33655, #7702, #5918, #50992, #53812, #81168, #40046, #37063, #88164, #86382, #3002, #59673, #22526, #62895, #30787, #20325, #81849, #73399, #40023, #64315, #21661, #71891, #50846, #51886, #62990, #44299, #87061, #81316, #39981, #28788, #31238, #40913, #40753, #17927, #44753, #10962, #86658, #67331, #57511, #50415, #58291, #68305, #7891, #15005, #1044, #47417, #67617, #67709, #60082, #41954, #53660, #71176, #13157, #85962, #20004, #62925, #8687, #2676, #39260, #64253, #243, #67879, #10818, #38482, #86790, #20686, #8422, #35524, #47694, #72157, #42802, #23852, #10789, #48252, #56508, #28355, #32968, #63718, #88052, #30106, #53255, #10415, #33424, #76300, #21638, #52309, #17450, #33656, #311, #68532, #27710, #72463, #88019, #23264, #41790, #7028, #61881, #56566, #84773, #34669, #56946, #40983, #36009, #26140, #81986, #50485, #3078, #7277, #21873, #45609, #51462, #4352, #30753, #45321, #51903, #45849, #84905, #46234, #4752, #3650, #51447, #86545, #12477, #12197, #31676, #67600, #9028, #49685, #9520, #60791, #51551, #52502, #37215, #50853, #34149, #72249, #17256, #70202, #78038, #66848, #43613, #14396, #38992, #32768, #29018, #64202, #84153, #319, #27247, #74255, #80857, #78533, #70939, #33527, #25904, #50692, #69116, #34043, #87449, #61476, #77832, #36227, #55211, #347, #50610, #13190, #10192, #48739, #31516, #5829, #5880, #51934, #40860, #36469, #37788, #34552, #32119, #22271, #20645, #6551, #25691, #19695, #31847, #5700, #947, #708, #26679, #67072, #79927, #24014, #37734, #46328, #32110, #8045, #78529, #51817, #55670, #54357, #76826, #49958, #84182, #20262, #36867, #54121, #9247, #53234, #61533, #27130, #21129, #21609, #36573, #81063, #43991, #46732, #6876, #4875, #16811, #36195, #14921, #84680, #74485, #65213, #46755, #35430, #56993, #34470, #1200, #47136, #75022, #20544, #55841, #52077, #86063, #74214, #25699, #18511, #69787, #33989, #494, #12388, #5231, #67259, #73684, #48993, #23775, #89078, #57681, #56934, #5810, #67581, #64769, #23739, #55282, #32347, #87950, #32896, #38730, #36780, #40338, #16605, #45627, #19750, #32942, #60183, #12815, #79378, #76311, #75921, #87339, #6189, #61869, #39584, #50363, #32909, #46607, #24906, #4086, #7539, #27697, #65884, #31145, #39365, #87659, #3796, #61233, #28674, #45293, #36377, #19550, #71021, #54964, #84031, #76647, #58631, #84304, #69036, #3627, #72848, #27098, #57034, #71173, #66809, #7977, #3923, #17381, #39742, #32360, #22891, #58561, #77174, #59147, #34126, #85034, #72567, #6743, #28337, #16802, #34328, #57692, #9526, #14443, #26295, #3037, #56378, #44370, #81876, #7696, #71825, #77931, #62036, #48863, #19268, #85224, #31460, #49193, #81333, #34981, #82993, #84275, #49398, #28933, #68693, #63810, #51368, #5083, #12968, #56111, #17382, #16059, #32179, #73208, #24169, #12568, #53541, #22813, #37724, #82064, #42113, #53746, #44493, #37908, #29897, #58751, #84492, #7944, #2399, #63317, #5593, #15023, #44793, #65146, #41177, #56050, #7877, #42645, #74965, #86969, #53262, #11706, #26622, #45045, #31303, #16566, #81762, #37316, #4569, #80291, #23901, #67938, #42282, #83526, #59979, #14093, #63017, #154, #30178, #10091, #4178, #80893, #72324, #45515, #62327, #3072, #83444, #7288, #42134, #79149, #44936, #1085, #5188, #54087, #10657, #63549, #10548, #65330, #38935, #39479, #41597, #26153, #12991, #86537, #13313, #58590, #58199, #66569, #45297, #54046, #50786, #76889, #25916, #39472, #87961, #66959, #49981, #80139, #47193, #63994, #62908, #14511, #8077, #7482, #58448, #21926, #43328, #15124, #83616, #1866, #55562, #72052, #3782, #83574, #22487, #24573, #64327, #1723, #7412, #13178, #28729, #77320, #12205, #17392, #26601, #43414, #61339, #52060, #72887, #78178, #8551, #19891, #28261, #39232, #21304, #26193, #8071, #32429, #9207, #34221, #62449, #64622, #10708, #61481, #26940, #45602, #6000, #9930, #35009, #36771, #31883, #81659, #28357, #56822, #70596, #85511, #58110, #20904, #5079, #6712, #29039, #71814, #29346, #23235, #4090, #42912, #58328, #41198, #75284, #89170, #66775, #23054, #75098, #48680, #26933, #80198, #83036, #77676, #76881, #14196, #14441, #33290, #9420, #27996, #35515, #17363, #16733, #2883, #71874, #11781, #58738, #15193, #60828, #7063, #50216, #60553, #29394, #50919, #23954, #76258, #81550, #6971, #9732, #35099, #4345, #86089, #46451, #30679, #87391, #67111, #12608, #36557, #24796, #37398, #15781, #39376, #78496, #11712, #21808, #88295, #21376, #6179, #65118, #9103, #23888, #12615, #73711, #14058, #62811, #80299, #47601, #333, #5305, #85548, #18777, #56447, #74431, #8051, #53368, #43384, #72640, #1355, #47849, #58846, #6704, #29983, #72793, #22418, #63382, #43285, #83908, #39485, #8195, #15516, #50308, #74997, #12874, #70909, #59249, #59689, #53852, #75591, #7097, #88930, #23245, #43012, #65627, #80178, #59344, #57156, #13484, #60081, #59669, #47722, #25195, #2715, #59737, #78378, #61018, #37482, #54298, #63688, #20995, #65438, #77306, #25524, #16639, #60343, #46630, #65741, #48481, #30043, #24383, #53548, #30113, #40003, #45206, #61026, #13469, #43297, #51599, #39165, #61913, #14618, #41957, #81940, #32667, #31814, #24686, #82830, #50016, #36623, #78998, #84996, #17833, #75506, #12609, #84006, #11551, #24004, #58536, #74559, #56333, #35886, #43892, #32236, #14715, #13608, #37070, #35218, #25576, #75624, #4088, #79794, #51709, #61205, #79135, #70217, #42126, #46139, #18364, #54703, #20439, #42219, #80817, #70137, #58238, #88298, #46643, #77408, #52163, #18342, #45189, #69836, #54373, #25428, #6077, #19574, #61342, #9700, #71222, #57424, #25679, #32600, #20224, #64326, #42379, #68555, #47006, #72505, #62542, #49612, #63775, #10975, #47180, #62299, #58807, #1375, #15063, #68031, #37180, #47536, #51083, #57816, #72034, #11793, #42065, #75364, #13826, #26111, #57578, #58563, #52565, #9500, #74948, #46720, #17918, #24494, #71883, #40874, #88888, #978, #4030, #80602, #26934, #1321, #36109, #69208, #42910, #88390, #2041, #18885, #83399, #54035, #75338, #34397, #55150, #17792, #27554, #33908, #63277, #52461, #28856, #35277, #67336, #40131, #62137, #8044, #86186, #68432, #3434, #87899, #80028, #64298, #24391, #72751, #337, #13722, #1399, #77042, #73205, #46425, #85876, #74917, #70324, #62868, #83429, #12310, #79765, #15769, #56915, #54369, #60999, #88448, #17979, #65404, #27226, #10828, #53821, #12081, #78073, #81134, #85179, #11240, #4289, #6249, #65024, #14068, #76284, #48063, #66856, #65898, #3777, #68103, #79053, #86316, #2141, #52346, #87540, #51606, #60786, #6500, #47712, #57216, #23037, #39268, #21200, #49823, #62596, #79195, #15214, #21124, #58576, #56491, #57414, #41729, #33369, #61003, #9311, #13870, #52244, #38866, #71744, #73035, #35089, #57402, #31747, #32777, #66014, #54411, #51355, #808, #86377, #77133, #15054, #17931, #36545, #52169, #12358, #73881, #43262, #31355, #60911, #56715, #2593, #56223, #24379, #13467, #14177, #44681, #8710, #7325, #24797, #5603, #4534, #56294, #69771, #59651, #54425, #60256, #16536, #85656, #29404, #79363, #28016, #67537, #25637, #31186, #22996, #32642, #26783, #50799, #17323, #53881, #71962, #1367, #89086, #48711, #8225, #86799, #52824, #5968, #42304, #63544, #77849, #66462, #563, #10216, #63190, #79810, #22870, #72265, #15945, #82538, #63594, #23396, #26369, #9948, #47203, #71756, #36736, #41446, #38180, #49689, #78305, #17533, #42005, #54282, #25129, #12198, #76315, #75521, #37994, #16674, #83580, #44262, #79597, #85174, #68566, #74531, #2777, #87307, #58046, #60689, #21925, #51830, #26793, #45569, #80089, #58913, #15852, #23502, #41754, #56383, #73311, #83626, #69086, #80640, #68726, #64652, #323, #75049, #43577, #40348, #81739, #76966, #928, #72953, #30293, #19924, #29159, #35028, #64667, #88831, #83404, #72779, #61042, #10727, #10036, #18126, #62785, #79625, #32861, #7295, #56494, #80801, #3568, #77963, #4301, #56471, #46747, #84550, #38738, #11463, #65306, #16903, #44823, #51923, #39558, #39820, #40844, #27658, #14702, #75058, #76957, #7594, #18259, #48532, #8961, #1581, #44452, #77533, #82225, #16454, #80194, #78049, #70655, #29006, #66887, #1403, #60914, #41742, #7629, #54178, #68938, #71549, #79289, #61340, #27231, #37220, #46368, #72242, #3973, #64910, #59970, #23770, #17026, #56202 ) ) ;
#61572=ORIENTED_EDGE ( 'NONE', *, *, #88949, .T. ) ;
#61574=ORIENTED_EDGE ( 'NONE', *, *, #65771, .T. ) ;
#61575=CARTESIAN_POINT ( 'NONE',  ( -12.46153846153846168, -3.886160181151819604, 36.00935417666054406 ) ) ;
#61576=EDGE_LOOP ( 'NONE', ( #87856, #29164 ) ) ;
#61577=CARTESIAN_POINT ( 'NONE',  ( -1.608100309179717025, -3.019605429927184836, 32.48692288466676814 ) ) ;
#61578=B_SPLINE_CURVE_WITH_KNOTS ( 'NONE', 3,
 ( #30255, #9973, #57722, #62690, #85204, #36138, #15862, #1010, #23483, #50939 ),
 .UNSPECIFIED., .F., .F.,
 ( 4, 2, 2, 2, 4 ),
 ( 0.0007817359430256318490, 0.0009771253907249984917, 0.001172514838424365026, 0.001367904286123731560, 0.001563293733823098311 ),
 .UNSPECIFIED. ) ;
#61579=CARTESIAN_POINT ( 'NONE',  ( -3.480792454990688789, -12.07920672191015221, 32.31858351112116168 ) ) ;
#61580=CARTESIAN_POINT ( 'NONE',  ( 6.923076923076924238, -4.661471528628507777, 34.16647553114623292 ) ) ;
#61581=CYLINDRICAL_SURFACE ( 'NONE', #53969, 0.2499999999999986955 ) ;
#61583=EDGE_CURVE ( 'NONE', #61584, #19974, #38147, .T. ) ;
#61584=VERTEX_POINT ( 'NONE', #32505 ) ;
#61585=ORIENTED_EDGE ( 'NONE', *, *, #69200, .T. ) ;
#61586=CARTESIAN_POINT ( 'NONE',  ( -4.853496115061506799, -7.630147231320743018, 34.74852402298682819 ) ) ;
#61588=ORIENTED_EDGE ( 'NONE', *, *, #27948, .T. ) ;
#61589=CARTESIAN_POINT ( 'NONE',  ( 4.153846153846154188, -8.973038597847269315, 34.52809138561121927 ) ) ;
#61591=EDGE_CURVE ( 'NONE', #77888, #4198, #54251, .T. ) ;
#61592=CARTESIAN_POINT ( 'NONE',  ( -17.20707104665477161, -3.625366637846545448, 33.29286588640298561 ) ) ;
#61593=VERTEX_POINT ( 'NONE', #59087 ) ;
#61595=CARTESIAN_POINT ( 'NONE',  ( 0.4615384615384611200, -9.058645607665452459, 34.76329471203371924 ) ) ;
#61596=EDGE_CURVE ( 'NONE', #70222, #12394, #70377, .T. ) ;
#61597=AXIS2_PLACEMENT_3D ( 'NONE', #43232, #36479, #34708 ) ;
#61598=FACE_BOUND ( 'NONE', #29747, .T. ) ;
#61599=EDGE_CURVE ( 'NONE', #28595, #67660, #28424, .T. ) ;
#61600=CARTESIAN_POINT ( 'NONE',  ( -15.29685161012936767, -8.164416787775445883, 34.95778746994557906 ) ) ;
#61601=CARTESIAN_POINT ( 'NONE',  ( 0.4615384615384611200, -6.343179335718451384, 34.87096338111211935 ) ) ;
#61604=CARTESIAN_POINT ( 'NONE',  ( 18.06525557127601900, -4.481592998940251427, 33.73612834413965089 ) ) ;
#61605=CARTESIAN_POINT ( 'NONE',  ( 2.307692307692309264, -8.810774026931790459, 35.74407628777942847 ) ) ;
#61606=CARTESIAN_POINT ( 'NONE',  ( -3.903791733932698182, -11.47946981652013498, 33.17500667209846910 ) ) ;
#61607=ORIENTED_EDGE ( 'NONE', *, *, #77019, .T. ) ;
#61608=CARTESIAN_POINT ( 'NONE',  ( -8.769230769230768274, -2.249999999999998668, 29.50000000000001421 ) ) ;
#61610=ORIENTED_EDGE ( 'NONE', *, *, #56714, .T. ) ;
#61611=B_SPLINE_CURVE_WITH_KNOTS ( 'NONE', 3,
 ( #68038, #20, #80674, #33363, #33798, #54959, #19399, #12203, #46866, #74350 ),
 .UNSPECIFIED., .F., .F.,
 ( 4, 2, 2, 2, 4 ),
 ( 0.000000000000000000, 0.0001954311564186862510, 0.0003908623128373725020, 0.0005862934692560588072, 0.0007817246256747450040 ),
 .UNSPECIFIED. ) ;
#61612=CARTESIAN_POINT ( 'NONE',  ( 14.05771557674995442, -9.943427161483782584, 34.11278801902876978 ) ) ;
#61613=CARTESIAN_POINT ( 'NONE',  ( -7.596099426240392027, -2.318338780012835443, 30.59689888758630261 ) ) ;
#61614=B_SPLINE_CURVE_WITH_KNOTS ( 'NONE', 3,
 ( #826, #29634, #50324, #49459, #76489, #43144 ),
 .UNSPECIFIED., .F., .F.,
 ( 4, 2, 4 ),
 ( 3.879202041849148443E-17, 0.0001954756301637101349, 0.0003909512603273815096 ),
 .UNSPECIFIED. ) ;
#61615=EDGE_LOOP ( 'NONE', ( #10907, #11865, #43811, #9024, #32420, #86689 ) ) ;
#61616=CARTESIAN_POINT ( 'NONE',  ( -16.08859058257013430, -11.48612834413965977, 32.76840700105972815 ) ) ;
#61618=FACE_BOUND ( 'NONE', #70885, .T. ) ;
#61619=CARTESIAN_POINT ( 'NONE',  ( -18.13014720943822056, -3.285722584762971632, 32.44110544564090759 ) ) ;
#61620=CARTESIAN_POINT ( 'NONE',  ( 15.48071474911736978, -12.22109172314383052, 31.39792113162168263 ) ) ;
#61621=CARTESIAN_POINT ( 'NONE',  ( 2.057669083470851756, -6.652501968072646932, 34.93155406624980941 ) ) ;
#61624=CARTESIAN_POINT ( 'NONE',  ( 2.307692307692186251, -11.06231777344772027, 33.60647404775119895 ) ) ;
#61626=EDGE_LOOP ( 'NONE', ( #68078, #71870, #22699, #28991 ) ) ;
#61627=ORIENTED_EDGE ( 'NONE', *, *, #69225, .F. ) ;
#61629=CARTESIAN_POINT ( 'NONE',  ( -12.39628332202562433, -5.941354392334607049, 34.76329471203374055 ) ) ;
#61630=DIRECTION ( 'NONE',  ( 0.000000000000000000, 0.1736481776669275834, 0.9848077530122086864 ) ) ;
#61631=CARTESIAN_POINT ( 'NONE',  ( -4.153846153846152411, -12.34228464037088635, 31.77849191805839268 ) ) ;
#61632=CARTESIAN_POINT ( 'NONE',  ( -0.2115384615370257404, -7.500000000000155431, 34.75000000000007105 ) ) ;
#61633=CARTESIAN_POINT ( 'NONE',  ( -15.00775787915638482, -2.758310577978207778, 31.33698337089302299 ) ) ;
#61635=CARTESIAN_POINT ( 'NONE',  ( -1.607542343522233796, -4.026226216239095379, 33.68668979543632958 ) ) ;
#61636=CARTESIAN_POINT ( 'NONE',  ( 1.384615384615264011, -10.33852847137269571, 34.16647553114546554 ) ) ;
#61637=VECTOR ( 'NONE', #9306, 1000.000000000000227 ) ;
#61638=CARTESIAN_POINT ( 'NONE',  ( 4.153846153846154188, -1.422936976036506707, 30.56769352161908415 ) ) ;
#61641=VECTOR ( 'NONE', #86704, 1000.000000000000000 ) ;
#61642=CARTESIAN_POINT ( 'NONE',  ( 7.780071466793711643, -8.164416787775445883, 34.95778746994557906 ) ) ;
#61643=CARTESIAN_POINT ( 'NONE',  ( -4.826923076923076650, -7.500000000000001776, 35.04278698407183867 ) ) ;
#61644=CYLINDRICAL_SURFACE ( 'NONE', #69221, 0.2500000000000008882 ) ;
#61645=CARTESIAN_POINT ( 'NONE',  ( 3.230769230769231726, -13.53365097954675988, 30.81389545987213552 ) ) ;
#61646=ORIENTED_EDGE ( 'NONE', *, *, #19631, .T. ) ;
#61647=CARTESIAN_POINT ( 'NONE',  ( 8.899756207464411872, -5.070358843744210198, 34.40418822224088302 ) ) ;
#61650=CARTESIAN_POINT ( 'NONE',  ( -9.757577692864012775, -11.06231777344662781, 33.60647404775220082 ) ) ;
#61651=CARTESIAN_POINT ( 'NONE',  ( -17.86920819217521483, -10.54018710029568595, 33.71981072465678864 ) ) ;
#61652=FACE_OUTER_BOUND ( 'NONE', #66236, .T. ) ;
#61653=CARTESIAN_POINT ( 'NONE',  ( -1.254089682851819987, -4.459921816937788996, 33.71989282347011851 ) ) ;
#61654=EDGE_LOOP ( 'NONE', ( #82572, #29294, #86668, #80739, #70393, #5543, #15952, #34712, #14289, #19468, #78019, #17044, #16711, #80777, #18989, #61349 ) ) ;
#61656=CARTESIAN_POINT ( 'NONE',  ( 16.82694633287448838, -2.544273027872574477, 31.48422191005632698 ) ) ;
#61657=ORIENTED_EDGE ( 'NONE', *, *, #52028, .F. ) ;
#61658=CARTESIAN_POINT ( 'NONE',  ( -11.53846153846122391, -2.255955759149395501, 30.00000000000324363 ) ) ;
#61659=CARTESIAN_POINT ( 'NONE',  ( 13.31853300525525086, -9.058645607665454236, 34.76329471203372634 ) ) ;
#61660=ORIENTED_EDGE ( 'NONE', *, *, #35094, .F. ) ;
#61662=CARTESIAN_POINT ( 'NONE',  ( -7.780085495151404906, -2.538708090699994813, 30.37095296980875503 ) ) ;
#61663=CARTESIAN_POINT ( 'NONE',  ( 2.307692307692309264, -1.215029322943914858, 32.30358669280327177 ) ) ;
#61664=ORIENTED_EDGE ( 'NONE', *, *, #27988, .T. ) ;
#61665=EDGE_LOOP ( 'NONE', ( #23357, #72085 ) ) ;
#61666=CYLINDRICAL_SURFACE ( 'NONE', #49859, 0.2500000000000002220 ) ;
#61669=ORIENTED_EDGE ( 'NONE', *, *, #11173, .T. ) ;
#61670=CARTESIAN_POINT ( 'NONE',  ( -15.23076923076935252, -4.320704448113951379, 33.92786785259630022 ) ) ;
#61671=CARTESIAN_POINT ( 'NONE',  ( 18.06606733335007675, -9.905515769479276145, 34.41647553114623292 ) ) ;
#61672=CARTESIAN_POINT ( 'NONE',  ( 9.468822767743363400, -9.417330523894424488, 34.63758898049880486 ) ) ;
#61673=CYLINDRICAL_SURFACE ( 'NONE', #16021, 0.2499999999999995559 ) ;
#61674=FACE_OUTER_BOUND ( 'NONE', #50299, .T. ) ;
#61675=CARTESIAN_POINT ( 'NONE',  ( 13.60762673622823549, -3.105924265160262543, 32.13625925475356127 ) ) ;
#61676=CARTESIAN_POINT ( 'NONE',  ( -0.4615384615385840772, -12.51329471203414379, 31.30864560766407578 ) ) ;
#61677=ORIENTED_EDGE ( 'NONE', *, *, #69226, .F. ) ;
#61678=EDGE_CURVE ( 'NONE', #11687, #23012, #27531, .T. ) ;
#61679=EDGE_LOOP ( 'NONE', ( #82874, #65623, #88152, #41232 ) ) ;
#61680=CARTESIAN_POINT ( 'NONE',  ( 7.173022332454968009, -12.68172785388650681, 30.59649109432439573 ) ) ;
#61681=EDGE_LOOP ( 'NONE', ( #71065, #8681, #37872, #15610 ) ) ;
#61683=AXIS2_PLACEMENT_3D ( 'NONE', #56810, #15843, #64003 ) ;
#61684=CARTESIAN_POINT ( 'NONE',  ( 11.76147438255493327, -3.395485233115139057, 33.02377354290275946 ) ) ;
#61685=CARTESIAN_POINT ( 'NONE',  ( 6.066067333350078528, -9.905515769479277921, 34.41647553114623292 ) ) ;
#61686=ORIENTED_EDGE ( 'NONE', *, *, #41708, .F. ) ;
#61687=CARTESIAN_POINT ( 'NONE',  ( 8.069165197766697162, -8.239487800360276282, 34.69522927552633718 ) ) ;
#61688=AXIS2_PLACEMENT_3D ( 'NONE', #47185, #20605, #12971 ) ;
#61691=EDGE_LOOP ( 'NONE', ( #3342, #12453, #19701, #67620, #76485, #61159 ) ) ;
#61692=VECTOR ( 'NONE', #61977, 1000.000000000000000 ) ;
#61693=CARTESIAN_POINT ( 'NONE',  ( -14.08467946359891165, -11.98016756924215009, 32.48728574198911190 ) ) ;
#61694=EDGE_CURVE ( 'NONE', #49073, #15199, #7713, .T. ) ;
#61695=EDGE_CURVE ( 'NONE', #19526, #82761, #76757, .T. ) ;
#61696=ORIENTED_EDGE ( 'NONE', *, *, #58445, .T. ) ;
#61697=CARTESIAN_POINT ( 'NONE',  ( -12.39628332202562433, -10.33852847137154107, 34.16647553114620450 ) ) ;
#61698=CARTESIAN_POINT ( 'NONE',  ( -9.019207500173122227, -2.779195860258146578, 31.39871582349836032 ) ) ;
#61699=FACE_BOUND ( 'NONE', #23157, .T. ) ;
#61700=CARTESIAN_POINT ( 'NONE',  ( -14.55766905174089665, -9.234221910056348293, 34.70572697212741531 ) ) ;
#61701=DIRECTION ( 'NONE',  ( 0.000000000000000000, 0.9848077530122072432, 0.1736481776669354937 ) ) ;
#61702=CARTESIAN_POINT ( 'NONE',  ( 9.561617089197387287, -2.295517848115769421, 30.44137282052137294 ) ) ;
#61703=CARTESIAN_POINT ( 'NONE',  ( 10.54930223602447903, -9.905515769479276145, 34.41647553114623292 ) ) ;
#61704=EDGE_CURVE ( 'NONE', #21602, #65648, #68510, .T. ) ;
#61706=DIRECTION ( 'NONE',  ( -0.000000000000000000, 0.5000000000000011102, -0.8660254037844380415 ) ) ;
#61707=CARTESIAN_POINT ( 'NONE',  ( -6.250000000000007994, -2.499999999999999556, 29.81609845454692120 ) ) ;
#61708=EDGE_CURVE ( 'NONE', #30802, #77995, #37016, .T. ) ;
#61709=ORIENTED_EDGE ( 'NONE', *, *, #75225, .F. ) ;
#61710=ORIENTED_EDGE ( 'NONE', *, *, #56614, .F. ) ;
#61711=CYLINDRICAL_SURFACE ( 'NONE', #1525, 0.2500000000000009437 ) ;
#61712=FACE_OUTER_BOUND ( 'NONE', #85592, .T. ) ;
#61713=CARTESIAN_POINT ( 'NONE',  ( -9.626240358957616650, -12.34228464037088813, 31.77849191805839268 ) ) ;
#61714=CARTESIAN_POINT ( 'NONE',  ( -3.903900744468109529, -9.357781135181031829, 34.66075350412533851 ) ) ;
#61716=LINE ( 'NONE', #33, #7307 ) ;
#61717=ORIENTED_EDGE ( 'NONE', *, *, #73658, .F. ) ;
#61718=CARTESIAN_POINT ( 'NONE',  ( 2.057715576749954867, -9.148715823498378086, 34.47080413974185120 ) ) ;
#61719=CARTESIAN_POINT ( 'NONE',  ( 3.361294932532793656, -11.46989282347013095, 32.79007818306219946 ) ) ;
#61720=FACE_OUTER_BOUND ( 'NONE', #88021, .T. ) ;
#61721=CARTESIAN_POINT ( 'NONE',  ( -7.146561847641254239, -6.716662450894490100, 34.94144148231605840 ) ) ;
#61722=ORIENTED_EDGE ( 'NONE', *, *, #29568, .T. ) ;
#61723=AXIS2_PLACEMENT_3D ( 'NONE', #14562, #21312, #69064 ) ;
#61724=ORIENTED_EDGE ( 'NONE', *, *, #57670, .F. ) ;
#61725=B_SPLINE_CURVE_WITH_KNOTS ( 'NONE', 3,
 ( #14122, #69506, #1499, #62737, #28984, #56439, #82598, #1053, #55990, #83482 ),
 .UNSPECIFIED., .F., .F.,
 ( 4, 2, 2, 2, 4 ),
 ( 0.0007817246256747484735, 0.0009771112852218920199, 0.001172497944769035783, 0.001367884604316179330, 0.001563271263863322876 ),
 .UNSPECIFIED. ) ;
#61727=VERTEX_POINT ( 'NONE', #19442 ) ;
#61728=CARTESIAN_POINT ( 'NONE',  ( 0.2387117690594567077, -7.369208160676172348, 34.74850200257122879 ) ) ;
#61729=ORIENTED_EDGE ( 'NONE', *, *, #82547, .T. ) ;
#61730=DIRECTION ( 'NONE',  ( -0.000000000000000000, 0.3420201433256694346, -0.9396926207859080948 ) ) ;
#61732=CARTESIAN_POINT ( 'NONE',  ( 4.853438133199126980, -6.760086850603068243, 34.69517049084099369 ) ) ;
#61734=CARTESIAN_POINT ( 'NONE',  ( 12.46153846153846168, -9.780366693483667717, 34.19971097300155094 ) ) ;
#61736=CARTESIAN_POINT ( 'NONE',  ( 18.00000000000000000, -1.044019251281081972, 31.83374038241031911 ) ) ;
#61737=CARTESIAN_POINT ( 'NONE',  ( 6.000000000000001776, -13.04860791097971706, 34.73218667398347037 ) ) ;
#61738=ORIENTED_EDGE ( 'NONE', *, *, #36881, .T. ) ;
#61740=CARTESIAN_POINT ( 'NONE',  ( -10.61538461538473399, -3.835265460704628371, 33.15142922262033665 ) ) ;
#61741=CARTESIAN_POINT ( 'NONE',  ( -13.44988583057615905, -5.219633306516282545, 34.19971097300152962 ) ) ;
#61742=CARTESIAN_POINT ( 'NONE',  ( 8.835298102580845025, -11.91647553114624358, 32.58852847137148245 ) ) ;
#61743=B_SPLINE_CURVE_WITH_KNOTS ( 'NONE', 3,
 ( #75342, #49955, #20396, #48297, #41111, #71112 ),
 .UNSPECIFIED., .F., .F.,
 ( 4, 2, 4 ),
 ( 4.220987180333914613E-17, 0.0001954756301637170196, 0.0003909512603273918637 ),
 .UNSPECIFIED. ) ;
#61744=CARTESIAN_POINT ( 'NONE',  ( -9.915792616872026954, -12.47654668319379567, 31.42292124445336654 ) ) ;
#61746=CARTESIAN_POINT ( 'NONE',  ( -0.5916864312701615169, -2.647304123082328875, 31.75400227202885262 ) ) ;
#61748=EDGE_LOOP ( 'NONE', ( #67730, #687, #45240, #74018, #78308, #51019 ) ) ;
#61749=CARTESIAN_POINT ( 'NONE',  ( 5.076923076923075762, -3.322132147404559976, 32.92929555188717927 ) ) ;
#61750=CARTESIAN_POINT ( 'NONE',  ( 0.5923302693632463978, -3.062576670634119758, 32.05464942895959979 ) ) ;
#61751=AXIS2_PLACEMENT_3D ( 'NONE', #44992, #31493, #71138 ) ;
#61752=CARTESIAN_POINT ( 'NONE',  ( 9.758375025657770152, -2.833524468853757750, 32.15551576947925838 ) ) ;
#61753=ORIENTED_EDGE ( 'NONE', *, *, #30547, .F. ) ;
#61756=AXIS2_PLACEMENT_3D ( 'NONE', #86366, #53888, #46247 ) ;
#61757=EDGE_CURVE ( 'NONE', #80981, #64802, #44499, .T. ) ;
#61759=LINE ( 'NONE', #12257, #77590 ) ;
#61760=CARTESIAN_POINT ( 'NONE',  ( -0.4615384615385840772, -11.06231777344772027, 33.60647404775119895 ) ) ;
#61761=VECTOR ( 'NONE', #56455, 999.9999999999998863 ) ;
#61762=CARTESIAN_POINT ( 'NONE',  ( -14.30769230769242917, -3.083524468854526912, 32.58852847137268327 ) ) ;
#61764=CARTESIAN_POINT ( 'NONE',  ( -15.29685264172511161, -2.721908614388770964, 31.22303859784723912 ) ) ;
#61765=CARTESIAN_POINT ( 'NONE',  ( 3.453548772037640546, -12.24180327182771855, 31.33663988360758168 ) ) ;
#61766=CARTESIAN_POINT ( 'NONE',  ( 18.06606733335007675, -12.34228464037088813, 31.77849191805839268 ) ) ;
#61768=CARTESIAN_POINT ( 'NONE',  ( -8.992058866865649591, -7.369209533119140509, 34.99857337881830688 ) ) ;
#61769=EDGE_CURVE ( 'NONE', #38026, #59454, #69254, .T. ) ;
#61770=ORIENTED_EDGE ( 'NONE', *, *, #1281, .F. ) ;
#61771=CARTESIAN_POINT ( 'NONE',  ( 12.68431813051652313, -12.47679350104403007, 31.42216943046555855 ) ) ;
#61772=CARTESIAN_POINT ( 'NONE',  ( 11.47319153790521717, -2.657715359629088780, 31.77849191805832874 ) ) ;
#61774=EDGE_CURVE ( 'NONE', #37061, #73584, #68956, .T. ) ;
#61775=CARTESIAN_POINT ( 'NONE',  ( -17.75005459062195712, -10.18230066228896646, 34.26354781536631577 ) ) ;
#61776=CARTESIAN_POINT ( 'NONE',  ( 11.53846153846141753, -4.481592998941358097, 33.73612834414048933 ) ) ;
#61777=CARTESIAN_POINT ( 'NONE',  ( 13.13463865367303285, -6.567427716900048118, 34.66269422305636283 ) ) ;
#61778=B_SPLINE_CURVE_WITH_KNOTS ( 'NONE', 3,
 ( #87997, #53725, #19497, #88425, #26697, #54156, #81652, #74899, #19935, #13191 ),
 .UNSPECIFIED., .F., .F.,
 ( 4, 2, 2, 2, 4 ),
 ( 0.0007817246256747485819, 0.0009771112852218918031, 0.001172497944769034916, 0.001367884604316178029, 0.001563271263863321358 ),
 .UNSPECIFIED. ) ;
#61779=LINE ( 'NONE', #26677, #16108 ) ;
#61781=B_SPLINE_CURVE_WITH_KNOTS ( 'NONE', 3,
 ( #72220, #39349, #71772, #4210, #10080, #66806, #86205, #79438, #38000, #17736 ),
 .UNSPECIFIED., .F., .F.,
 ( 4, 2, 2, 2, 4 ),
 ( 0.0007817359430256285964, 0.0009771253907249943717, 0.001172514838424360039, 0.001367904286123725706, 0.001563293733823091372 ),
 .UNSPECIFIED. ) ;
#61782=B_SPLINE_CURVE_WITH_KNOTS ( 'NONE', 3,
 ( #29842, #84355, #70388, #15892, #64484, #29411, #2789, #8249, #14552, #22198 ),
 .UNSPECIFIED., .F., .F.,
 ( 4, 2, 2, 2, 4 ),
 ( 0.000000000000000000, 0.0001954311564186876334, 0.0003908623128373752667, 0.0005862934692560629272, 0.0007817246256747505334 ),
 .UNSPECIFIED. ) ;
#61783=ORIENTED_EDGE ( 'NONE', *, *, #28570, .T. ) ;
#61784=EDGE_CURVE ( 'NONE', #3322, #24141, #26644, .T. ) ;
#61785=FACE_BOUND ( 'NONE', #66865, .T. ) ;
#61787=CARTESIAN_POINT ( 'NONE',  ( -9.019207513279360100, -12.41104346484419452, 31.60698883733904196 ) ) ;
#61788=VECTOR ( 'NONE', #20429, 1000.000000000000114 ) ;
#61789=EDGE_CURVE ( 'NONE', #49742, #74216, #4817, .T. ) ;
#61790=CARTESIAN_POINT ( 'NONE',  ( 18.06606835100244268, -12.10708131394839882, 31.69288490824020954 ) ) ;
#61791=DIRECTION ( 'NONE',  ( 0.000000000000000000, 1.000000000000000000, 0.000000000000000000 ) ) ;
#61792=CARTESIAN_POINT ( 'NONE',  ( -6.223484943723949669, -12.24155766932282496, 31.33739205006857986 ) ) ;
#61793=VERTEX_POINT ( 'NONE', #9908 ) ;
#61794=ORIENTED_EDGE ( 'NONE', *, *, #1475, .F. ) ;
#61795=ORIENTED_EDGE ( 'NONE', *, *, #25008, .T. ) ;
#61796=DIRECTION ( 'NONE',  ( -0.000000000000000000, -0.9396926207859092051, -0.3420201433256662704 ) ) ;
#61797=ORIENTED_EDGE ( 'NONE', *, *, #29058, .F. ) ;
#61798=EDGE_CURVE ( 'NONE', #39836, #60358, #57444, .T. ) ;
#61800=CARTESIAN_POINT ( 'NONE',  ( -17.20707104665477161, -10.31621877034669588, 34.18098118002070152 ) ) ;
#61801=EDGE_CURVE ( 'NONE', #40219, #85070, #5947, .T. ) ;
#61802=FACE_OUTER_BOUND ( 'NONE', #2636, .T. ) ;
#61803=CARTESIAN_POINT ( 'NONE',  ( -2.307692307692305711, -12.78798330534102945, 29.74999999999997868 ) ) ;
#61804=CARTESIAN_POINT ( 'NONE',  ( -13.63461538461538325, -7.500000000000001776, 35.04278698407183867 ) ) ;
#61805=AXIS2_PLACEMENT_3D ( 'NONE', #84465, #59197, #39832 ) ;
#61806=CIRCLE ( 'NONE', #82025, 0.2500000000000002220 ) ;
#61807=EDGE_CURVE ( 'NONE', #70953, #68235, #31602, .T. ) ;
#61809=CARTESIAN_POINT ( 'NONE',  ( -2.307692307692427391, -5.219633306517616589, 34.19971097300220464 ) ) ;
#61810=EDGE_CURVE ( 'NONE', #69536, #32821, #84274, .T. ) ;
#61811=CARTESIAN_POINT ( 'NONE',  ( 17.75002326905764605, -2.564618984488975517, 30.55390908950641915 ) ) ;
#61812=CARTESIAN_POINT ( 'NONE',  ( -8.546217925137375104, -2.889357225399414197, 32.26129605718031002 ) ) ;
#61815=AXIS2_PLACEMENT_3D ( 'NONE', #36407, #56669, #76947 ) ;
#61816=VERTEX_POINT ( 'NONE', #70289 ) ;
#61817=VECTOR ( 'NONE', #66815, 1000.000000000000000 ) ;
#61818=CYLINDRICAL_SURFACE ( 'NONE', #74775, 0.2499999999999995559 ) ;
#61819=CARTESIAN_POINT ( 'NONE',  ( 1.384615384615386802, -10.05456864172156806, 36.03766855953608683 ) ) ;
#61820=CARTESIAN_POINT ( 'NONE',  ( -6.000000000000119904, -3.835265460704628371, 33.15142922262033665 ) ) ;
#61821=B_SPLINE_CURVE_WITH_KNOTS ( 'NONE', 3,
 ( #34054, #21871, #42157, #75480, #7480, #14229, #89024, #712, #82251, #61516 ),
 .UNSPECIFIED., .F., .F.,
 ( 4, 2, 2, 2, 4 ),
 ( 0.000000000000000000, 0.0001954339857564058210, 0.0003908679715128116419, 0.0005863019572692174629, 0.0007817359430256232838 ),
 .UNSPECIFIED. ) ;
#61823=CARTESIAN_POINT ( 'NONE',  ( -9.758391103263569732, -6.386643153685125363, 34.62446782046654903 ) ) ;
#61824=FACE_BOUND ( 'NONE', #22340, .T. ) ;
#61825=CARTESIAN_POINT ( 'NONE',  ( -7.053224892808616531, -3.625366637846544560, 33.29286588640298561 ) ) ;
#61826=VERTEX_POINT ( 'NONE', #49575 ) ;
#61827=DIRECTION ( 'NONE',  ( 0.000000000000000000, 0.9848077530122072432, 0.1736481776669354937 ) ) ;
#61828=CARTESIAN_POINT ( 'NONE',  ( -9.692307692307691624, -13.88283147151868846, 33.14645433367849847 ) ) ;
#61829=CARTESIAN_POINT ( 'NONE',  ( -1.384615384615383471, -3.322132147404559976, 32.92929555188717927 ) ) ;
#61831=FACE_OUTER_BOUND ( 'NONE', #73613, .T. ) ;
#61833=FACE_BOUND ( 'NONE', #9453, .T. ) ;
#61834=FACE_OUTER_BOUND ( 'NONE', #38774, .T. ) ;
#61837=EDGE_LOOP ( 'NONE', ( #76721, #50597, #41116, #35604 ) ) ;
#61838=CYLINDRICAL_SURFACE ( 'NONE', #86824, 0.2499999999999973355 ) ;
#61839=CARTESIAN_POINT ( 'NONE',  ( 14.53047197667037338, -3.563462043263030399, 33.22394488606062879 ) ) ;
#61840=CARTESIAN_POINT ( 'NONE',  ( -16.37677237136229991, -12.39988816332205701, 30.74660775122750778 ) ) ;
#61841=CARTESIAN_POINT ( 'NONE',  ( -7.053768389744480061, -10.54014554554150607, 33.71984207302941883 ) ) ;
#61842=ORIENTED_EDGE ( 'NONE', *, *, #37138, .T. ) ;
#61843=CARTESIAN_POINT ( 'NONE',  ( 16.28437185560972011, -10.88167719472716399, 33.43325721877153711 ) ) ;
#61844=CARTESIAN_POINT ( 'NONE',  ( -15.29685264172511161, -8.120952969808774569, 34.71129190930000163 ) ) ;
#61845=CYLINDRICAL_SURFACE ( 'NONE', #62847, 0.2500000000000009437 ) ;
#61846=VERTEX_POINT ( 'NONE', #36933 ) ;
#61847=DIRECTION ( 'NONE',  ( -0.000000000000000000, 0.6427876096865404731, -0.7660444431189771253 ) ) ;
#61848=CARTESIAN_POINT ( 'NONE',  ( -14.30769230769230660, -2.486705287966279876, 31.30864560766543647 ) ) ;
#61849=CARTESIAN_POINT ( 'NONE',  ( 16.28437159207980045, -12.15418822224088657, 32.17964115625579069 ) ) ;
#61850=CARTESIAN_POINT ( 'NONE',  ( -10.48459280755983158, -2.541949514083464479, 30.39797389878540557 ) ) ;
#61851=EDGE_CURVE ( 'NONE', #31297, #56029, #63818, .T. ) ;
#61852=CARTESIAN_POINT ( 'NONE',  ( 14.98074600654777733, -5.765609946408404518, 34.70566812827425451 ) ) ;
#61853=CARTESIAN_POINT ( 'NONE',  ( 8.769230769230768274, -13.20930481340135110, 34.54067556320372745 ) ) ;
#61857=ORIENTED_EDGE ( 'NONE', *, *, #25203, .F. ) ;
#61859=ORIENTED_EDGE ( 'NONE', *, *, #24456, .F. ) ;
#61861=DIRECTION ( 'NONE',  ( 0.000000000000000000, 0.000000000000000000, 1.000000000000000000 ) ) ;
#61863=CARTESIAN_POINT ( 'NONE',  ( -4.219928533206287469, -2.486705287966279432, 31.30864560766542937 ) ) ;
#61865=CARTESIAN_POINT ( 'NONE',  ( 17.86930939688969033, -4.684245665217972032, 34.18127051446801090 ) ) ;
#61866=ADVANCED_FACE ( 'NONE', ( #77923 ), #16228, .F. ) ;
#61867=CARTESIAN_POINT ( 'NONE',  ( -11.53846153846153655, -9.905515769479276145, 34.41647553114623292 ) ) ;
#61868=CARTESIAN_POINT ( 'NONE',  ( 6.130525701763568591, -3.285477652293412820, 32.44071101563363158 ) ) ;
#61869=ADVANCED_FACE ( 'NONE', ( #30618 ), #45910, .F. ) ;
#61870=CARTESIAN_POINT ( 'NONE',  ( 1.161130460051053248, -2.612411019501189813, 31.66733052389439962 ) ) ;
#61871=CARTESIAN_POINT ( 'NONE',  ( 9.915087361285756629, -12.47679350104403007, 31.42216943046555855 ) ) ;
#61872=CARTESIAN_POINT ( 'NONE',  ( -11.66915300512910214, -4.809359713505814149, 33.96456829005828837 ) ) ;
#61874=CARTESIAN_POINT ( 'NONE',  ( 10.39189967166066708, -2.599994579823202923, 30.74605699353653776 ) ) ;
#61875=CARTESIAN_POINT ( 'NONE',  ( -16.85391023282967993, -10.77377354290276301, 33.85451476688484718 ) ) ;
#61876=VECTOR ( 'NONE', #69257, 1000.000000000000114 ) ;
#61877=DIRECTION ( 'NONE',  ( -0.000000000000000000, 0.7660444431189791237, -0.6427876096865379196 ) ) ;
#61878=CARTESIAN_POINT ( 'NONE',  ( -13.16183584334697798, -11.41317474335729543, 32.86274602512330034 ) ) ;
#61881=ADVANCED_FACE ( 'NONE', ( #24757 ), #4490, .F. ) ;
#61883=ORIENTED_EDGE ( 'NONE', *, *, #40597, .T. ) ;
#61884=CARTESIAN_POINT ( 'NONE',  ( -18.00000000000030553, -12.49374608885938542, 30.00000000000319744 ) ) ;
#61885=CARTESIAN_POINT ( 'NONE',  ( 11.78846153846295763, -7.500000000000154543, 35.00000000000007105 ) ) ;
#61886=CARTESIAN_POINT ( 'NONE',  ( -18.00000000000000000, -12.27536236210233866, 35.44105525097462106 ) ) ;
#61887=CARTESIAN_POINT ( 'NONE',  ( 3.230769230769231726, -2.499999999999998668, 29.50000000000001066 ) ) ;
#61888=EDGE_CURVE ( 'NONE', #57222, #26954, #43415, .T. ) ;
#61890=CARTESIAN_POINT ( 'NONE',  ( 9.757562831820530747, -11.67786785259547777, 32.92929555188713664 ) ) ;
#61892=CARTESIAN_POINT ( 'NONE',  ( -9.469294848214296678, -10.77377354290276124, 33.85451476688484718 ) ) ;
#61894=CARTESIAN_POINT ( 'NONE',  ( 6.923076923076924238, -4.786620604624113540, 33.94971097300155094 ) ) ;
#61895=ORIENTED_EDGE ( 'NONE', *, *, #13976, .F. ) ;
#61896=EDGE_CURVE ( 'NONE', #67262, #10170, #14377, .T. ) ;
#61897=CARTESIAN_POINT ( 'NONE',  ( 12.46153846153876898, -2.506253911140615021, 30.00000000000323297 ) ) ;
#61898=ORIENTED_EDGE ( 'NONE', *, *, #54184, .F. ) ;
#61899=CARTESIAN_POINT ( 'NONE',  ( -2.307692307692427391, -6.879047030192662504, 34.71129190930017927 ) ) ;
#61900=CARTESIAN_POINT ( 'NONE',  ( -5.076923076923197442, -2.625532179533778709, 30.86335684631627174 ) ) ;
#61901=CARTESIAN_POINT ( 'NONE',  ( 11.78851585009985214, -10.66356715214248752, 33.62249196103329751 ) ) ;
#61902=CARTESIAN_POINT ( 'NONE',  ( 4.023698184114458343, -6.809168938359898782, 34.95455904226513866 ) ) ;
#61904=ORIENTED_EDGE ( 'NONE', *, *, #28301, .F. ) ;
#61905=EDGE_LOOP ( 'NONE', ( #80441, #86119, #34551, #16210 ) ) ;
#61906=ORIENTED_EDGE ( 'NONE', *, *, #72529, .F. ) ;
#61907=B_SPLINE_CURVE_WITH_KNOTS ( 'NONE', 3,
 ( #772, #9310, #7537, #28239, #55710, #21483, #76434, #14738, #69671, #35444 ),
 .UNSPECIFIED., .F., .F.,
 ( 4, 2, 2, 2, 4 ),
 ( 0.0007817359430256304396, 0.0009771253907249963233, 0.001172514838424362424, 0.001367904286123728524, 0.001563293733823094408 ),
 .UNSPECIFIED. ) ;
#61908=VERTEX_POINT ( 'NONE', #37823 ) ;
#61910=LINE ( 'NONE', #77647, #42991 ) ;
#61911=CARTESIAN_POINT ( 'NONE',  ( -16.02305571287920571, -9.084667340241228572, 34.75534355489798344 ) ) ;
#61912=CARTESIAN_POINT ( 'NONE',  ( -3.296039676730006196, -10.21337939537584383, 33.94971097300158647 ) ) ;
#61913=ADVANCED_FACE ( 'NONE', ( #11248 ), #86937, .F. ) ;
#61915=CARTESIAN_POINT ( 'NONE',  ( -5.999999999999998224, -11.35647404775217417, 33.31231777344666511 ) ) ;
#61916=EDGE_CURVE ( 'NONE', #30008, #31103, #79711, .T. ) ;
#61917=CARTESIAN_POINT ( 'NONE',  ( 12.39545608217832395, -2.833524468853757305, 32.15551576947924417 ) ) ;
#61918=ORIENTED_EDGE ( 'NONE', *, *, #46933, .F. ) ;
#61919=ORIENTED_EDGE ( 'NONE', *, *, #10905, .T. ) ;
#61920=ORIENTED_EDGE ( 'NONE', *, *, #19799, .F. ) ;
#61921=CARTESIAN_POINT ( 'NONE',  ( 17.32697738856138869, -12.41262288849542017, 30.68299917996395010 ) ) ;
#61922=ORIENTED_EDGE ( 'NONE', *, *, #70162, .T. ) ;
#61923=CARTESIAN_POINT ( 'NONE',  ( 17.20744851515672025, -11.04252011169589842, 33.62494198852677840 ) ) ;
#61924=CARTESIAN_POINT ( 'NONE',  ( -4.826868765284762830, -11.28795663066794219, 33.01431243580653785 ) ) ;
#61927=VECTOR ( 'NONE', #38139, 1000.000000000000114 ) ;
#61928=EDGE_CURVE ( 'NONE', #74382, #55112, #8959, .T. ) ;
#61930=LINE ( 'NONE', #33591, #58597 ) ;
#61931=FACE_BOUND ( 'NONE', #66570, .T. ) ;
#61932=CARTESIAN_POINT ( 'NONE',  ( -5.869209559033045309, -2.845873456487966635, 32.17976146951972538 ) ) ;
#61933=VECTOR ( 'NONE', #80845, 1000.000000000000000 ) ;
#61934=AXIS2_PLACEMENT_3D ( 'NONE', #36143, #57283, #23057 ) ;
#61935=CARTESIAN_POINT ( 'NONE',  ( 13.38461538461538680, -6.435427911321262684, 35.78748833219616898 ) ) ;
#61936=VERTEX_POINT ( 'NONE', #53105 ) ;
#61938=CARTESIAN_POINT ( 'NONE',  ( 11.53846153846153832, -12.78798330534103123, 29.99999999999997868 ) ) ;
#61939=CARTESIAN_POINT ( 'NONE',  ( 6.857806922520602200, -12.16647553114622049, 32.15551576947930812 ) ) ;
#61940=CARTESIAN_POINT ( 'NONE',  ( -17.07692307692307665, -12.62096338111211580, 30.90682066428153263 ) ) ;
#61941=CARTESIAN_POINT ( 'NONE',  ( 12.46153846153846168, -11.69971097300155272, 32.46337939537588113 ) ) ;
#61942=ORIENTED_EDGE ( 'NONE', *, *, #31373, .T. ) ;
#61943=VECTOR ( 'NONE', #21615, 1000.000000000000114 ) ;
#61945=CARTESIAN_POINT ( 'NONE',  ( -3.931066484868084299, -10.23759521482555357, 34.22997729860117033 ) ) ;
#61946=CARTESIAN_POINT ( 'NONE',  ( 17.20744877868663281, -10.19071101563364401, 33.96452234770658407 ) ) ;
#61947=CARTESIAN_POINT ( 'NONE',  ( -2.531177251416254936, -10.81261337010820256, 33.49550067578627477 ) ) ;
#61948=B_SPLINE_CURVE_WITH_KNOTS ( 'NONE', 3,
 ( #22984, #16665, #23854, #17569, #2698, #84267, #37375, #22546, #30194, #50013 ),
 .UNSPECIFIED., .F., .F.,
 ( 4, 2, 2, 2, 4 ),
 ( 0.000000000000000000, 0.0001954339857564081791, 0.0003908679715128163582, 0.0005863019572692245102, 0.0007817359430256327164 ),
 .UNSPECIFIED. ) ;
#61949=CYLINDRICAL_SURFACE ( 'NONE', #9845, 0.2499999999999979738 ) ;
#61950=B_SPLINE_CURVE_WITH_KNOTS ( 'NONE', 3,
 ( #76806, #36264, #30383, #43891, #8792, #56959, #50192, #16867, #64151, #77678 ),
 .UNSPECIFIED., .F., .F.,
 ( 4, 2, 2, 2, 4 ),
 ( 0.0007817359430256388964, 0.0009771253907250075990, 0.001172514838424376085, 0.001367904286123744571, 0.001563293733823113273 ),
 .UNSPECIFIED. ) ;
#61951=EDGE_CURVE ( 'NONE', #13845, #53903, #38024, .T. ) ;
#61952=FACE_BOUND ( 'NONE', #43512, .T. ) ;
#61953=CARTESIAN_POINT ( 'NONE',  ( -6.792551484843276199, -12.70449254468099198, 30.44128974285582956 ) ) ;
#61954=CARTESIAN_POINT ( 'NONE',  ( 16.82689985270161870, -2.985938066672154889, 32.43141759479405550 ) ) ;
#61955=DIRECTION ( 'NONE',  ( -0.000000000000000000, 0.3420201433256694346, -0.9396926207859080948 ) ) ;
#61957=CARTESIAN_POINT ( 'NONE',  ( -2.307692307692428724, -8.656820664282941280, 34.87096338111179961 ) ) ;
#61958=CARTESIAN_POINT ( 'NONE',  ( -5.076923076923075762, -12.34228464037088635, 31.77849191805839268 ) ) ;
#61960=ORIENTED_EDGE ( 'NONE', *, *, #67001, .T. ) ;
#61961=EDGE_CURVE ( 'NONE', #47861, #78029, #64759, .T. ) ;
#61962=CARTESIAN_POINT ( 'NONE',  ( -5.999999999999998224, -10.67929555188718282, 33.92786785259544047 ) ) ;
#61965=CARTESIAN_POINT ( 'NONE',  ( -13.31936024510254413, -11.06231777344671130, 33.60647404775212976 ) ) ;
#61967=CARTESIAN_POINT ( 'NONE',  ( -11.40793583669797684, -2.882268652242222284, 31.66798894389554064 ) ) ;
#61968=CARTESIAN_POINT ( 'NONE',  ( 14.30769230769231015, -3.937682226553329556, 33.60647404775216529 ) ) ;
#61969=CARTESIAN_POINT ( 'NONE',  ( 5.933917620639864943, -8.164416787775445883, 34.95778746994557906 ) ) ;
#61970=ORIENTED_EDGE ( 'NONE', *, *, #9611, .F. ) ;
#61971=CARTESIAN_POINT ( 'NONE',  ( -15.23076923076922995, -4.786620604624113540, 33.94971097300155094 ) ) ;
#61973=CARTESIAN_POINT ( 'NONE',  ( -15.45425415533356173, -9.417330523894424488, 34.63758898049880486 ) ) ;
#61974=DIRECTION ( 'NONE',  ( 0.000000000000000000, 0.4999999999999985567, 0.8660254037844395958 ) ) ;
#61976=CARTESIAN_POINT ( 'NONE',  ( 12.23861224402230974, -2.758268499246657068, 31.33685645148948140 ) ) ;
#61977=DIRECTION ( 'NONE',  ( -0.000000000000000000, 0.1736481776669307198, -0.9848077530122080203 ) ) ;
#61978=CARTESIAN_POINT ( 'NONE',  ( -12.39547112818838492, -8.164416787775445883, 34.95778746994558617 ) ) ;
#61980=AXIS2_PLACEMENT_3D ( 'NONE', #19255, #3943, #52137 ) ;
#61982=CARTESIAN_POINT ( 'NONE',  ( -10.55012904410859420, -2.892918686051626498, 31.69288490824026638 ) ) ;
#61983=CARTESIAN_POINT ( 'NONE',  ( 10.68064018666063575, -11.48612834413965977, 32.76840700105972815 ) ) ;
#61984=EDGE_CURVE ( 'NONE', #68144, #8709, #4643, .T. ) ;
#61985=EDGE_LOOP ( 'NONE', ( #82441, #41577 ) ) ;
#61987=CARTESIAN_POINT ( 'NONE',  ( 8.992242120843618736, -9.886259254753566594, 34.14407573483972413 ) ) ;
#61989=B_SPLINE_CURVE_WITH_KNOTS ( 'NONE', 3,
 ( #20889, #88940, #20008, #7828, #68638, #21334, #61870, #48359, #28546, #33963 ),
 .UNSPECIFIED., .F., .F.,
 ( 4, 2, 2, 2, 4 ),
 ( 0.000000000000000000, 0.0001954311564186863865, 0.0003908623128373727731, 0.0005862934692560591325, 0.0007817246256747455461 ),
 .UNSPECIFIED. ) ;
#61990=CARTESIAN_POINT ( 'NONE',  ( -17.74994568836168440, -12.41262288849542017, 30.68299917996395010 ) ) ;
#61991=LINE ( 'NONE', #739, #12435 ) ;
#61992=VERTEX_POINT ( 'NONE', #26096 ) ;
#61993=CARTESIAN_POINT ( 'NONE',  ( 6.792466563452393302, -7.722926236386453702, 34.74524107206102030 ) ) ;
#61994=CARTESIAN_POINT ( 'NONE',  ( -0.3962828902624376815, -10.21337939537593442, 33.94971097300152252 ) ) ;
#61995=CARTESIAN_POINT ( 'NONE',  ( 2.307692307692187583, -2.892918686052166066, 31.69288490824153470 ) ) ;
#61996=ORIENTED_EDGE ( 'NONE', *, *, #61097, .T. ) ;
#61997=CARTESIAN_POINT ( 'NONE',  ( -5.326899807865430603, -5.728515186090277211, 34.42611988154120439 ) ) ;
#61998=B_SPLINE_CURVE_WITH_KNOTS ( 'NONE', 3,
 ( #813, #63392, #69715, #56203, #84136, #21976, #77357, #49447, #76920, #1701 ),
 .UNSPECIFIED., .F., .F.,
 ( 4, 2, 2, 2, 4 ),
 ( 0.0007817359430256395469, 0.0009771253907250080327, 0.001172514838424376735, 0.001367904286123745438, 0.001563293733823113924 ),
 .UNSPECIFIED. ) ;
#61999=EDGE_CURVE ( 'NONE', #32338, #49839, #73406, .T. ) ;
#62000=CARTESIAN_POINT ( 'NONE',  ( 4.946447891847356004, -7.276987145209185215, 34.99546412871779211 ) ) ;
#62002=CARTESIAN_POINT ( 'NONE',  ( -17.07692307692319744, -2.892918686052165622, 31.69288490824153470 ) ) ;
#62003=B_SPLINE_CURVE_WITH_KNOTS ( 'NONE', 3,
 ( #81948, #21104, #20672, #47701, #47254, #74746, #76056, #14355, #81503, #41843 ),
 .UNSPECIFIED., .F., .F.,
 ( 4, 2, 2, 2, 4 ),
 ( 0.0007817246256747460882, 0.0009771112852218887673, 0.001172497944769031663, 0.001367884604316174559, 0.001563271263863317238 ),
 .UNSPECIFIED. ) ;
#62004=CARTESIAN_POINT ( 'NONE',  ( -13.44988583057616083, -11.94971097300153140, 32.03036669348370680 ) ) ;
#62005=AXIS2_PLACEMENT_3D ( 'NONE', #52328, #32071, #52774 ) ;
#62006=ORIENTED_EDGE ( 'NONE', *, *, #57948, .T. ) ;
#62007=ORIENTED_EDGE ( 'NONE', *, *, #667, .F. ) ;
#62008=ORIENTED_EDGE ( 'NONE', *, *, #4164, .F. ) ;
#62010=VECTOR ( 'NONE', #15893, 1000.000000000000000 ) ;
#62011=CARTESIAN_POINT ( 'NONE',  ( -16.37677311275300340, -3.395401636524186362, 33.02366814457250399 ) ) ;
#62012=CARTESIAN_POINT ( 'NONE',  ( -6.857008572074484221, -4.098570777380720287, 33.41473453929635440 ) ) ;
#62013=CARTESIAN_POINT ( 'NONE',  ( 9.692307692307695177, -4.786620604624113540, 33.94971097300155094 ) ) ;
#62014=CARTESIAN_POINT ( 'NONE',  ( 11.53846153846141576, -10.33852847137269571, 34.16647553114546554 ) ) ;
#62015=CIRCLE ( 'NONE', #13099, 0.2500000000000002220 ) ;
#62016=VERTEX_POINT ( 'NONE', #74738 ) ;
#62017=CARTESIAN_POINT ( 'NONE',  ( 15.23076923076923173, -9.780366693483667717, 34.19971097300155094 ) ) ;
#62018=ORIENTED_EDGE ( 'NONE', *, *, #67818, .T. ) ;
#62019=VERTEX_POINT ( 'NONE', #13461 ) ;
#62020=ORIENTED_EDGE ( 'NONE', *, *, #74137, .T. ) ;
#62022=ORIENTED_EDGE ( 'NONE', *, *, #5351, .F. ) ;
#62023=CARTESIAN_POINT ( 'NONE',  ( 6.000000000000001776, -10.89733346790207413, 36.13435417666054406 ) ) ;
#62024=B_SPLINE_CURVE_WITH_KNOTS ( 'NONE', 3,
 ( #72079, #25232, #80182, #86965, #31542, #11727, #3617, #25677, #53134, #80642 ),
 .UNSPECIFIED., .F., .F.,
 ( 4, 2, 2, 2, 4 ),
 ( 0.000000000000000000, 0.0001954311564186875520, 0.0003908623128373751041, 0.0005862934692560627103, 0.0007817246256747502082 ),
 .UNSPECIFIED. ) ;
#62025=DIRECTION ( 'NONE',  ( -0.000000000000000000, 0.7660444431189791237, -0.6427876096865379196 ) ) ;
#62026=EDGE_CURVE ( 'NONE', #10, #49638, #32550, .T. ) ;
#62027=CARTESIAN_POINT ( 'NONE',  ( 5.934729999443682402, -4.320704448112771878, 33.92786785259540494 ) ) ;
#62028=CARTESIAN_POINT ( 'NONE',  ( -5.999999999999998224, -4.098570777380720287, 33.41473453929634729 ) ) ;
#62029=EDGE_CURVE ( 'NONE', #84688, #21487, #32851, .T. ) ;
#62030=VERTEX_POINT ( 'NONE', #75599 ) ;
#62031=VERTEX_POINT ( 'NONE', #67528 ) ;
#62032=ORIENTED_EDGE ( 'NONE', *, *, #15087, .F. ) ;
#62033=CARTESIAN_POINT ( 'NONE',  ( -9.442362173959550020, -5.852078868378309373, 34.47109172314383585 ) ) ;
#62034=DIRECTION ( 'NONE',  ( -0.000000000000000000, 0.7660444431189791237, -0.6427876096865379196 ) ) ;
#62035=EDGE_LOOP ( 'NONE', ( #86038, #5855, #88453, #2870 ) ) ;
#62036=ADVANCED_FACE ( 'NONE', ( #20229 ), #33303, .F. ) ;
#62037=CARTESIAN_POINT ( 'NONE',  ( 6.923076923076924238, -6.386643153685126251, 34.62446782046654192 ) ) ;
#62038=CIRCLE ( 'NONE', #30344, 0.2500000000000002220 ) ;
#62040=ORIENTED_EDGE ( 'NONE', *, *, #70420, .T. ) ;
#62041=VECTOR ( 'NONE', #9156, 1000.000000000000000 ) ;
#62042=CARTESIAN_POINT ( 'NONE',  ( 8.769230769230768274, -12.37446782046654192, 30.86335684631486131 ) ) ;
#62043=EDGE_CURVE ( 'NONE', #76426, #14630, #6275, .T. ) ;
#62044=DIRECTION ( 'NONE',  ( -0.000000000000000000, -0.9396926207859092051, -0.3420201433256662704 ) ) ;
#62045=EDGE_LOOP ( 'NONE', ( #16826, #70376, #8508, #24850 ) ) ;
#62046=FACE_BOUND ( 'NONE', #20516, .T. ) ;
#62047=CARTESIAN_POINT ( 'NONE',  ( -0.4615384615384611200, -9.780366693483667717, 34.19971097300155094 ) ) ;
#62048=DIRECTION ( 'NONE',  ( -0.000000000000000000, -0.9848077530122086864, -0.1736481776669273613 ) ) ;
#62049=CARTESIAN_POINT ( 'NONE',  ( 6.923076923076924238, -11.11383981884818262, 36.00935417666054406 ) ) ;
#62050=CARTESIAN_POINT ( 'NONE',  ( -14.30769230769230660, -12.29105614889573062, 35.45975837776705220 ) ) ;
#62051=CARTESIAN_POINT ( 'NONE',  ( -0.4615384615385826339, -12.27809138561165270, 31.22303859784587132 ) ) ;
#62052=CARTESIAN_POINT ( 'NONE',  ( -4.853911725310227077, -10.61302985866383963, 33.66295027996417843 ) ) ;
#62053=CARTESIAN_POINT ( 'NONE',  ( 13.38461538461569411, -2.506253911140615021, 30.00000000000323297 ) ) ;
#62054=ORIENTED_EDGE ( 'NONE', *, *, #19375, .T. ) ;
#62055=CARTESIAN_POINT ( 'NONE',  ( -2.372962308248625529, -4.320704448112771878, 33.92786785259540494 ) ) ;
#62056=CARTESIAN_POINT ( 'NONE',  ( -8.096153846153844924, -2.499999999999998668, 29.75000000000000355 ) ) ;
#62057=ORIENTED_EDGE ( 'NONE', *, *, #19204, .F. ) ;
#62058=B_SPLINE_CURVE_WITH_KNOTS ( 'NONE', 3,
 ( #72188, #5070, #25789, #17705, #53247, #78952, #24438, #65435, #60010, #18144 ),
 .UNSPECIFIED., .F., .F.,
 ( 4, 2, 2, 2, 4 ),
 ( 0.000000000000000000, 0.0001954311584214072923, 0.0003908623168428145846, 0.0005862934752642218498, 0.0007817246336856291692 ),
 .UNSPECIFIED. ) ;
#62060=CARTESIAN_POINT ( 'NONE',  ( 13.38461538461538680, -1.129524287112498415, 32.06866353760679544 ) ) ;
#62061=ORIENTED_EDGE ( 'NONE', *, *, #77878, .F. ) ;
#62062=CARTESIAN_POINT ( 'NONE',  ( -9.757577692864012775, -9.528491918058357157, 34.59228464037090589 ) ) ;
#62063=CARTESIAN_POINT ( 'NONE',  ( 2.307692307692186251, -5.094484230521993062, 34.41647553114689373 ) ) ;
#62064=FACE_BOUND ( 'NONE', #18746, .T. ) ;
#62066=CARTESIAN_POINT ( 'NONE',  ( 15.48082354240754732, -12.17597550085003810, 31.52189283813460463 ) ) ;
#62067=CARTESIAN_POINT ( 'NONE',  ( -8.769230769230768274, -6.386643153685126251, 34.62446782046654192 ) ) ;
#62068=CARTESIAN_POINT ( 'NONE',  ( 1.515140822849032398, -12.70449254468099198, 30.44128974285582956 ) ) ;
#62071=CARTESIAN_POINT ( 'NONE',  ( -14.08467946359890988, -5.582272713120729257, 34.63742843783360570 ) ) ;
#62073=ORIENTED_EDGE ( 'NONE', *, *, #72925, .F. ) ;
#62074=EDGE_CURVE ( 'NONE', #39806, #88852, #58375, .T. ) ;
#62076=VERTEX_POINT ( 'NONE', #72280 ) ;
#62077=DIRECTION ( 'NONE',  ( 0.000000000000000000, 0.3420201433256641055, -0.9396926207859100932 ) ) ;
#62078=CARTESIAN_POINT ( 'NONE',  ( -15.23076923076935252, -5.941354392335915335, 34.76329471203413846 ) ) ;
#62079=CARTESIAN_POINT ( 'NONE',  ( -9.469528151039281028, -9.332535724633409302, 34.40230450496446934 ) ) ;
#62080=CARTESIAN_POINT ( 'NONE',  ( -8.992157728137614825, -8.282780595021769443, 34.94152052738834158 ) ) ;
#62083=AXIS2_PLACEMENT_3D ( 'NONE', #4381, #65621, #16559 ) ;
#62085=CARTESIAN_POINT ( 'NONE',  ( 16.15384615384615330, -13.20930481340135110, 34.54067556320372745 ) ) ;
#62086=EDGE_CURVE ( 'NONE', #3191, #59530, #30473, .T. ) ;
#62087=CARTESIAN_POINT ( 'NONE',  ( 6.222779668978068557, -4.226511098958374291, 33.85474049983370293 ) ) ;
#62088=CARTESIAN_POINT ( 'NONE',  ( 17.77707304109314279, -4.026226216239093603, 33.68668979543632958 ) ) ;
#62089=CARTESIAN_POINT ( 'NONE',  ( -1.254567949364932211, -7.723484941389743952, 34.99544897038808955 ) ) ;
#62090=CARTESIAN_POINT ( 'NONE',  ( 5.076923076923075762, -4.102666532097928531, 36.13435417666054406 ) ) ;
#62091=CARTESIAN_POINT ( 'NONE',  ( -0.4615384615384611200, -3.937682226553329556, 33.60647404775216529 ) ) ;
#62092=CARTESIAN_POINT ( 'NONE',  ( 15.23076923076923173, -13.78497067705608181, 32.30358669280327177 ) ) ;
#62093=EDGE_CURVE ( 'NONE', #37921, #68993, #86267, .T. ) ;
#62094=ADVANCED_FACE ( 'NONE', ( #49020 ), #23649, .F. ) ;
#62096=ORIENTED_EDGE ( 'NONE', *, *, #9223, .F. ) ;
#62097=CARTESIAN_POINT ( 'NONE',  ( 4.088575707885377497, -5.219633306516282545, 34.19971097300152252 ) ) ;
#62098=CARTESIAN_POINT ( 'NONE',  ( 6.923076923076800782, -11.06231777344772027, 33.60647404775119895 ) ) ;
#62101=CARTESIAN_POINT ( 'NONE',  ( -16.15384615384615330, -5.180354513474913603, 36.12317359536750416 ) ) ;
#62102=ORIENTED_EDGE ( 'NONE', *, *, #54730, .F. ) ;
#62103=CARTESIAN_POINT ( 'NONE',  ( -13.38461538461550582, -11.94971097300221174, 32.03036669348237098 ) ) ;
#62104=CARTESIAN_POINT ( 'NONE',  ( -14.37377571864818293, -12.10708131394839349, 31.69288490824020244 ) ) ;
#62105=ORIENTED_EDGE ( 'NONE', *, *, #32772, .T. ) ;
#62106=CARTESIAN_POINT ( 'NONE',  ( 9.758375025657770152, -12.62096338111211757, 30.90682066428152908 ) ) ;
#62107=CARTESIAN_POINT ( 'NONE',  ( 12.71159288145191724, -5.642605341092957971, 34.66089969410670335 ) ) ;
#62108=EDGE_CURVE ( 'NONE', #85233, #25506, #67020, .T. ) ;
#62109=EDGE_LOOP ( 'NONE', ( #63441, #32053, #23941, #11882 ) ) ;
#62111=CARTESIAN_POINT ( 'NONE',  ( 13.38461538461526423, -9.528491918059723176, 34.59228464037033035 ) ) ;
#62112=B_SPLINE_CURVE_WITH_KNOTS ( 'NONE', 3,
 ( #27964, #68502, #55431, #33831, #62623, #27076, #54538, #34274, #13560, #41042 ),
 .UNSPECIFIED., .F., .F.,
 ( 4, 2, 2, 2, 4 ),
 ( 0.0007817359430256315238, 0.0009771253907249976244, 0.001172514838424363508, 0.001367904286123729392, 0.001563293733823095492 ),
 .UNSPECIFIED. ) ;
#62113=ORIENTED_EDGE ( 'NONE', *, *, #31738, .F. ) ;
#62114=AXIS2_PLACEMENT_3D ( 'NONE', #73591, #18639, #37555 ) ;
#62115=CARTESIAN_POINT ( 'NONE',  ( 16.82694634598072625, -11.28823185664190376, 33.01397839955799896 ) ) ;
#62116=EDGE_CURVE ( 'NONE', #88566, #32155, #10058, .T. ) ;
#62117=EDGE_CURVE ( 'NONE', #49489, #44980, #77696, .T. ) ;
#62118=CARTESIAN_POINT ( 'NONE',  ( -15.29652265908256048, -7.249945578846652694, 34.99404164642496795 ) ) ;
#62119=CARTESIAN_POINT ( 'NONE',  ( 2.241609928332172430, -12.62096338111211580, 30.90682066428152197 ) ) ;
#62120=ORIENTED_EDGE ( 'NONE', *, *, #33109, .T. ) ;
#62121=VERTEX_POINT ( 'NONE', #38059 ) ;
#62122=CARTESIAN_POINT ( 'NONE',  ( -10.36543920600657209, -2.341251567377310217, 30.72681386836322659 ) ) ;
#62123=EDGE_CURVE ( 'NONE', #22049, #72929, #28300, .T. ) ;
#62125=CARTESIAN_POINT ( 'NONE',  ( -15.10024379253558457, -4.299079248970732792, 33.91157788607253565 ) ) ;
#62126=CARTESIAN_POINT ( 'NONE',  ( -1.134669866267241867, -2.587454068350147907, 30.68340429815432202 ) ) ;
#62127=DIRECTION ( 'NONE',  ( -0.000000000000000000, -0.000000000000000000, -1.000000000000000000 ) ) ;
#62128=B_SPLINE_CURVE_WITH_KNOTS ( 'NONE', 3,
 ( #24934, #79449, #78992, #10089, #85762, #59608, #73129, #52399, #23599, #51050 ),
 .UNSPECIFIED., .F., .F.,
 ( 4, 2, 2, 2, 4 ),
 ( 0.000000000000000000, 0.0001954339857564089923, 0.0003908679715128179845, 0.0005863019572692270039, 0.0007817359430256359690 ),
 .UNSPECIFIED. ) ;
#62129=DIRECTION ( 'NONE',  ( 0.000000000000000000, 0.9396926207859126468, -0.3420201433256571111 ) ) ;
#62130=CARTESIAN_POINT ( 'NONE',  ( -4.219116599806928214, -6.879047030191174805, 34.71129190930000163 ) ) ;
#62131=CARTESIAN_POINT ( 'NONE',  ( 1.253924781505078911, -2.295517848115769421, 30.44137282052137294 ) ) ;
#62132=CARTESIAN_POINT ( 'NONE',  ( 15.93091919493930320, -12.64616026154729411, 30.79003144601914244 ) ) ;
#62133=EDGE_LOOP ( 'NONE', ( #76885, #43031 ) ) ;
#62134=ORIENTED_EDGE ( 'NONE', *, *, #49170, .T. ) ;
#62136=VERTEX_POINT ( 'NONE', #69737 ) ;
#62137=ADVANCED_FACE ( 'NONE', ( #78154 ), #35511, .F. ) ;
#62138=CARTESIAN_POINT ( 'NONE',  ( 16.85399611801622655, -2.308479472611653094, 30.53278059502174457 ) ) ;
#62140=VECTOR ( 'NONE', #79303, 1000.000000000000114 ) ;
#62141=FACE_OUTER_BOUND ( 'NONE', #9990, .T. ) ;
#62142=CARTESIAN_POINT ( 'NONE',  ( 14.30769230769218581, -6.835583212225970762, 34.95778746994575670 ) ) ;
#62144=FACE_OUTER_BOUND ( 'NONE', #31064, .T. ) ;
#62145=AXIS2_PLACEMENT_3D ( 'NONE', #81729, #26333, #4737 ) ;
#62146=ORIENTED_EDGE ( 'NONE', *, *, #30730, .F. ) ;
#62147=CARTESIAN_POINT ( 'NONE',  ( -12.21153846153845990, -2.499999999999999556, 29.81604066197449754 ) ) ;
#62149=CARTESIAN_POINT ( 'NONE',  ( -11.53846153846153655, -6.435427911321262684, 35.78748833219616898 ) ) ;
#62150=ORIENTED_EDGE ( 'NONE', *, *, #26712, .T. ) ;
#62151=CARTESIAN_POINT ( 'NONE',  ( -4.153846153846274980, -4.320704448113951379, 33.92786785259630022 ) ) ;
#62152=CARTESIAN_POINT ( 'NONE',  ( -8.899922235898324985, -2.729777683071817229, 31.24903638046269450 ) ) ;
#62153=FACE_BOUND ( 'NONE', #47171, .T. ) ;
#62154=CARTESIAN_POINT ( 'NONE',  ( 5.777073041093152561, -2.308479472611653094, 30.53278059502174457 ) ) ;
#62155=CARTESIAN_POINT ( 'NONE',  ( -11.60373153901785948, -6.835583212224499938, 34.95778746994557906 ) ) ;
#62156=CARTESIAN_POINT ( 'NONE',  ( -16.02305571287920571, -4.684288915650984819, 34.18129842949671371 ) ) ;
#62157=CARTESIAN_POINT ( 'NONE',  ( -0.3954711281883858676, -2.833524468853757750, 32.15551576947925838 ) ) ;
#62158=CARTESIAN_POINT ( 'NONE',  ( -2.980823712421087901, -3.202959910592335202, 32.30730279482227019 ) ) ;
#62159=CARTESIAN_POINT ( 'NONE',  ( -4.377331097570100304, -11.41268669641500466, 32.86336882939237825 ) ) ;
#62160=CARTESIAN_POINT ( 'NONE',  ( -14.05763799605399278, -3.627508038966690496, 32.91356715214248396 ) ) ;
#62161=VERTEX_POINT ( 'NONE', #66869 ) ;
#62163=DIRECTION ( 'NONE',  ( -0.000000000000000000, -0.000000000000000000, 1.000000000000000000 ) ) ;
#62164=CARTESIAN_POINT ( 'NONE',  ( 14.98079249982687955, -12.17611988154120972, 31.52148481390971213 ) ) ;
#62165=EDGE_CURVE ( 'NONE', #88652, #81428, #26324, .T. ) ;
#62166=VECTOR ( 'NONE', #46559, 1000.000000000000000 ) ;
#62167=CARTESIAN_POINT ( 'NONE',  ( -12.52680890749923570, -2.625532179533444754, 30.86335684631481513 ) ) ;
#62168=CARTESIAN_POINT ( 'NONE',  ( -8.769230769230768274, -10.89733346790207413, 36.13435417666054406 ) ) ;
#62169=CARTESIAN_POINT ( 'NONE',  ( 15.48082354240754555, -3.627508038966690496, 32.91356715214248396 ) ) ;
#62172=CYLINDRICAL_SURFACE ( 'NONE', #61597, 0.2499999999999986955 ) ;
#62173=CARTESIAN_POINT ( 'NONE',  ( 3.361561038594018225, -11.18335022499818621, 33.13157742990016885 ) ) ;
#62174=DIRECTION ( 'NONE',  ( 0.000000000000000000, 0.3420201433256610524, 0.9396926207859113145 ) ) ;
#62175=LINE ( 'NONE', #49103, #7935 ) ;
#62176=VECTOR ( 'NONE', #52580, 1000.000000000000227 ) ;
#62177=VERTEX_POINT ( 'NONE', #66422 ) ;
#62178=ORIENTED_EDGE ( 'NONE', *, *, #68149, .T. ) ;
#62179=EDGE_LOOP ( 'NONE', ( #62781, #46330, #60386, #86752 ) ) ;
#62181=EDGE_CURVE ( 'NONE', #11993, #27559, #48659, .T. ) ;
#62182=ORIENTED_EDGE ( 'NONE', *, *, #45066, .T. ) ;
#62183=CARTESIAN_POINT ( 'NONE',  ( -9.442362282929646966, -10.18230066228895758, 34.26354781536631577 ) ) ;
#62184=DIRECTION ( 'NONE',  ( 0.000000000000000000, 0.000000000000000000, 1.000000000000000000 ) ) ;
#62187=EDGE_CURVE ( 'NONE', #56825, #35354, #7840, .T. ) ;
#62188=CARTESIAN_POINT ( 'NONE',  ( -11.31545018684868786, -6.503523203565941380, 34.64991518177335195 ) ) ;
#62190=CARTESIAN_POINT ( 'NONE',  ( 4.219914504848592429, -4.098570777380720287, 33.41473453929635440 ) ) ;
#62192=ORIENTED_EDGE ( 'NONE', *, *, #10334, .F. ) ;
#62194=CARTESIAN_POINT ( 'NONE',  ( -10.39260507411620260, -3.755027918224367323, 33.06320215134714857 ) ) ;
#62195=FACE_OUTER_BOUND ( 'NONE', #52148, .T. ) ;
#62196=CARTESIAN_POINT ( 'NONE',  ( 9.758376043310132530, -10.51840700105979565, 33.73612834413962247 ) ) ;
#62197=CARTESIAN_POINT ( 'NONE',  ( -9.942284436356281674, -12.41104346484419452, 31.60698883733904196 ) ) ;
#62198=EDGE_CURVE ( 'NONE', #35844, #61936, #41185, .T. ) ;
#62199=CARTESIAN_POINT ( 'NONE',  ( 9.468822748583747284, -10.11188796281391511, 34.01382737946119050 ) ) ;
#62200=CARTESIAN_POINT ( 'NONE',  ( -0.4615384615385840772, -2.657715359629662544, 31.77849191805970364 ) ) ;
#62201=B_SPLINE_CURVE_WITH_KNOTS ( 'NONE', 3,
 ( #80832, #74063, #47011, #19115, #53778, #5598, #27196, #54652, #82151, #40724 ),
 .UNSPECIFIED., .F., .F.,
 ( 4, 2, 2, 2, 4 ),
 ( 0.0007817359430256294638, 0.0009771253907249974075, 0.001172514838424365460, 0.001367904286123733295, 0.001563293733823094191 ),
 .UNSPECIFIED. ) ;
#62204=LINE ( 'NONE', #27979, #66200 ) ;
#62205=CARTESIAN_POINT ( 'NONE',  ( 0.7115927731767749398, -3.136992222400443175, 32.19305428654138979 ) ) ;
#62207=VECTOR ( 'NONE', #552, 1000.000000000000227 ) ;
#62208=DIRECTION ( 'NONE',  ( -0.000000000000000000, 0.6427876096865404731, -0.7660444431189770143 ) ) ;
#62209=VERTEX_POINT ( 'NONE', #11481 ) ;
#62210=VERTEX_POINT ( 'NONE', #11933 ) ;
#62211=CARTESIAN_POINT ( 'NONE',  ( 2.084864210057430167, -7.369209533119137845, 34.99857337881830688 ) ) ;
#62212=CARTESIAN_POINT ( 'NONE',  ( -3.296852641725108501, -10.51840700105979387, 33.73612834413961536 ) ) ;
#62213=VECTOR ( 'NONE', #24442, 1000.000000000000000 ) ;
#62214=CARTESIAN_POINT ( 'NONE',  ( 8.769230769230768274, -1.044019251281081972, 31.83374038241031911 ) ) ;
#62215=CARTESIAN_POINT ( 'NONE',  ( 14.24160889673642849, -3.050289026998445951, 32.03036669348365706 ) ) ;
#62217=CARTESIAN_POINT ( 'NONE',  ( -15.23076923076935074, -2.892918686052166066, 31.69288490824153470 ) ) ;
#62218=EDGE_CURVE ( 'NONE', #21962, #46929, #2549, .T. ) ;
#62219=CARTESIAN_POINT ( 'NONE',  ( 3.230769230769231726, -12.10708131394839349, 31.69288490824020244 ) ) ;
#62220=CARTESIAN_POINT ( 'NONE',  ( 24.00000000000000000, -9.499999999999982236, 27.25000000000000000 ) ) ;
#62223=ORIENTED_EDGE ( 'NONE', *, *, #69729, .T. ) ;
#62226=ORIENTED_EDGE ( 'NONE', *, *, #48234, .T. ) ;
#62227=CARTESIAN_POINT ( 'NONE',  ( 7.846153846153725020, -12.27809138561165270, 31.22303859784587132 ) ) ;
#62228=CARTESIAN_POINT ( 'NONE',  ( -14.55771553191376277, -2.341070481393819236, 30.72580821765574299 ) ) ;
#62229=CARTESIAN_POINT ( 'NONE',  ( -11.66915300512910214, -6.413092428213692742, 34.63065189839063152 ) ) ;
#62230=B_SPLINE_CURVE_WITH_KNOTS ( 'NONE', 3,
 ( #74801, #54510, #75667, #13970, #41448, #68912, #80678, #18962, #46427, #12206 ),
 .UNSPECIFIED., .F., .F.,
 ( 4, 2, 2, 2, 4 ),
 ( 0.000000000000000000, 0.0001954339857564076099, 0.0003908679715128152198, 0.0005863019572692228839, 0.0007817359430256304396 ),
 .UNSPECIFIED. ) ;
#62231=VECTOR ( 'NONE', #36718, 1000.000000000000000 ) ;
#62232=DIRECTION ( 'NONE',  ( 0.000000000000000000, 0.4999999999999960032, -0.8660254037844410391 ) ) ;
#62234=ORIENTED_EDGE ( 'NONE', *, *, #50180, .T. ) ;
#62235=FACE_BOUND ( 'NONE', #77642, .T. ) ;
#62236=ORIENTED_EDGE ( 'NONE', *, *, #13069, .T. ) ;
#62238=CARTESIAN_POINT ( 'NONE',  ( -12.46153846153846168, -1.129524287112498415, 32.06866353760679544 ) ) ;
#62239=CARTESIAN_POINT ( 'NONE',  ( 8.769230769230768274, -3.937682226553329556, 33.60647404775216529 ) ) ;
#62240=CARTESIAN_POINT ( 'NONE',  ( -11.28840722682322628, -2.564540009722895419, 30.55348353981670684 ) ) ;
#62241=ORIENTED_EDGE ( 'NONE', *, *, #32323, .F. ) ;
#62242=ORIENTED_EDGE ( 'NONE', *, *, #32277, .T. ) ;
#62243=ORIENTED_EDGE ( 'NONE', *, *, #14252, .F. ) ;
#62245=ORIENTED_EDGE ( 'NONE', *, *, #80843, .T. ) ;
#62246=CARTESIAN_POINT ( 'NONE',  ( -13.38461538461550582, -3.300289026999228881, 32.46337939537708905 ) ) ;
#62247=CARTESIAN_POINT ( 'NONE',  ( 13.38461538461538680, -9.058645607665452459, 34.76329471203371924 ) ) ;
#62248=CYLINDRICAL_SURFACE ( 'NONE', #17024, 0.2499999999999979738 ) ;
#62249=DIRECTION ( 'NONE',  ( 0.000000000000000000, 0.4999999999999985567, 0.8660254037844395958 ) ) ;
#62250=AXIS2_PLACEMENT_3D ( 'NONE', #18389, #58030, #44953 ) ;
#62252=CARTESIAN_POINT ( 'NONE',  ( 15.29602480204525605, -9.442884908240273489, 34.35708131394835618 ) ) ;
#62253=CARTESIAN_POINT ( 'NONE',  ( -18.25000000000000355, -7.500000000000000000, 35.00000000000000000 ) ) ;
#62254=CARTESIAN_POINT ( 'NONE',  ( 11.40831432902331954, -10.19110544564092002, 33.96427741523702792 ) ) ;
#62255=VERTEX_POINT ( 'NONE', #79938 ) ;
#62256=ORIENTED_EDGE ( 'NONE', *, *, #81144, .T. ) ;
#62257=VECTOR ( 'NONE', #33990, 1000.000000000000114 ) ;
#62259=DIRECTION ( 'NONE',  ( -0.000000000000000000, 0.7660444431189791237, -0.6427876096865379196 ) ) ;
#62260=CYLINDRICAL_SURFACE ( 'NONE', #30252, 0.2499999999999995559 ) ;
#62262=DIRECTION ( 'NONE',  ( -0.000000000000000000, -0.7660444431189791237, -0.6427876096865379196 ) ) ;
#62263=CARTESIAN_POINT ( 'NONE',  ( -6.792285115252135519, -3.530189275343204702, 32.79018710029569661 ) ) ;
#62264=FACE_BOUND ( 'NONE', #79766, .T. ) ;
#62265=CARTESIAN_POINT ( 'NONE',  ( 9.757563263583719504, -3.835265460703683349, 33.15142922261929925 ) ) ;
#62266=VERTEX_POINT ( 'NONE', #74512 ) ;
#62267=CYLINDRICAL_SURFACE ( 'NONE', #83160, 0.2499999999999979738 ) ;
#62268=CARTESIAN_POINT ( 'NONE',  ( 0.4615384615384611200, -9.780366693483667717, 34.19971097300155094 ) ) ;
#62269=DIRECTION ( 'NONE',  ( 0.000000000000000000, 0.7660444431189807890, 0.6427876096865361433 ) ) ;
#62270=CARTESIAN_POINT ( 'NONE',  ( 1.384615384615386802, -9.819645486525091727, 36.12317359536749706 ) ) ;
#62271=VERTEX_POINT ( 'NONE', #12807 ) ;
#62272=CARTESIAN_POINT ( 'NONE',  ( 18.25005431163831204, -12.41262288849542017, 30.68299917996395010 ) ) ;
#62273=ORIENTED_EDGE ( 'NONE', *, *, #34632, .T. ) ;
#62274=FACE_BOUND ( 'NONE', #28137, .T. ) ;
#62275=DIRECTION ( 'NONE',  ( 0.000000000000000000, 0.6427876096865373645, -0.7660444431189797898 ) ) ;
#62276=EDGE_CURVE ( 'NONE', #71689, #88631, #83137, .T. ) ;
#62277=CARTESIAN_POINT ( 'NONE',  ( -12.46153846153846168, -8.120952969808772792, 34.71129190930000163 ) ) ;
#62280=EDGE_CURVE ( 'NONE', #21769, #5919, #45251, .T. ) ;
#62281=CARTESIAN_POINT ( 'NONE',  ( 5.076923076922954969, -3.300289026999228881, 32.46337939537708905 ) ) ;
#62282=CARTESIAN_POINT ( 'NONE',  ( -3.296039231325549768, -2.379036618887870880, 30.90682066428147934 ) ) ;
#62283=CARTESIAN_POINT ( 'NONE',  ( -16.40386939113911779, -12.43535235679832596, 30.55408501211184813 ) ) ;
#62284=CARTESIAN_POINT ( 'NONE',  ( -13.38461538461538325, -12.48256725967547354, 35.29906147534542527 ) ) ;
#62285=EDGE_LOOP ( 'NONE', ( #13291, #44171 ) ) ;
#62286=CARTESIAN_POINT ( 'NONE',  ( -7.846153846153967493, -10.33852847137269571, 34.16647553114546554 ) ) ;
#62288=CARTESIAN_POINT ( 'NONE',  ( -15.93106648486808119, -10.23759521482555357, 34.22997729860117033 ) ) ;
#62289=DIRECTION ( 'NONE',  ( 0.000000000000000000, 0.4999999999999985567, 0.8660254037844395958 ) ) ;
#62291=ORIENTED_EDGE ( 'NONE', *, *, #79797, .F. ) ;
#62292=CARTESIAN_POINT ( 'NONE',  ( 9.469479594672815637, -7.369209533119137845, 34.99857337881830688 ) ) ;
#62293=CARTESIAN_POINT ( 'NONE',  ( -4.153846153846152411, -2.721908614388771852, 31.22303859784724978 ) ) ;
#62294=CARTESIAN_POINT ( 'NONE',  ( 5.011653076366757276, -2.657715359629089225, 31.77849191805834295 ) ) ;
#62296=CARTESIAN_POINT ( 'NONE',  ( 9.757563263583717728, -9.442884908240273489, 34.35708131394835618 ) ) ;
#62297=DIRECTION ( 'NONE',  ( -0.000000000000000000, 0.7660444431189791237, -0.6427876096865379196 ) ) ;
#62298=FACE_OUTER_BOUND ( 'NONE', #8940, .T. ) ;
#62299=ADVANCED_FACE ( 'NONE', ( #14136 ), #82618, .F. ) ;
#62300=LINE ( 'NONE', #83032, #3238 ) ;
#62302=ORIENTED_EDGE ( 'NONE', *, *, #82787, .T. ) ;
#62303=CARTESIAN_POINT ( 'NONE',  ( -17.32692307692307665, -2.249999999999998668, 29.75000000000000355 ) ) ;
#62304=ORIENTED_EDGE ( 'NONE', *, *, #45057, .F. ) ;
#62305=ORIENTED_EDGE ( 'NONE', *, *, #24779, .T. ) ;
#62306=CARTESIAN_POINT ( 'NONE',  ( -11.28851612908349722, -2.341251567377310217, 30.72681386836322659 ) ) ;
#62307=EDGE_LOOP ( 'NONE', ( #47665, #86549, #49062, #13944 ) ) ;
#62308=DIRECTION ( 'NONE',  ( -0.000000000000000000, -0.5000000000000009992, -0.8660254037844380415 ) ) ;
#62310=DIRECTION ( 'NONE',  ( 0.000000000000000000, 0.9396926207859126468, 0.3420201433256571111 ) ) ;
#62311=CARTESIAN_POINT ( 'NONE',  ( -11.78848477575450282, -11.37209801155882971, 32.91403422569032955 ) ) ;
#62313=CARTESIAN_POINT ( 'NONE',  ( 2.307692307692309264, -9.780366693483667717, 34.19971097300155094 ) ) ;
#62314=CARTESIAN_POINT ( 'NONE',  ( -4.403869391139116907, -3.711651800289232916, 33.01384336483936011 ) ) ;
#62315=CARTESIAN_POINT ( 'NONE',  ( 6.856994543716788293, -9.905515769479276145, 34.41647553114623292 ) ) ;
#62316=CARTESIAN_POINT ( 'NONE',  ( 11.31553532094539172, -10.61292498521070549, 33.66303323003028680 ) ) ;
#62321=B_SPLINE_CURVE_WITH_KNOTS ( 'NONE', 3,
 ( #86652, #5102, #5548, #59595, #73115, #12743, #79434, #31692, #46959, #72663 ),
 .UNSPECIFIED., .F., .F.,
 ( 4, 2, 2, 2, 4 ),
 ( 0.000000000000000000, 0.0001954339881912774070, 0.0003908679763825548140, 0.0005863019645738322752, 0.0007817359527651096280 ),
 .UNSPECIFIED. ) ;
#62322=CARTESIAN_POINT ( 'NONE',  ( -13.16160403300253634, -11.24521262558773493, 33.06293181088029343 ) ) ;
#62324=VECTOR ( 'NONE', #5106, 1000.000000000000114 ) ;
#62325=ORIENTED_EDGE ( 'NONE', *, *, #47773, .T. ) ;
#62326=EDGE_LOOP ( 'NONE', ( #83168, #55064 ) ) ;
#62327=ADVANCED_FACE ( 'NONE', ( #28543 ), #68636, .F. ) ;
#62328=CARTESIAN_POINT ( 'NONE',  ( -18.06527000055631760, -2.657715359629089669, 31.77849191805835005 ) ) ;
#62329=CARTESIAN_POINT ( 'NONE',  ( 1.449870524128224591, -3.643525952247864463, 33.31231777344670064 ) ) ;
#62330=DIRECTION ( 'NONE',  ( -0.000000000000000000, 1.000000000000000000, 3.491481338843133355E-15 ) ) ;
#62331=CARTESIAN_POINT ( 'NONE',  ( -5.076923076923075762, -2.517432740324522911, 35.29906147534542527 ) ) ;
#62332=EDGE_CURVE ( 'NONE', #12780, #31146, #1065, .T. ) ;
#62333=CARTESIAN_POINT ( 'NONE',  ( 12.33084699487090674, -8.999036380462717588, 34.52022231692819076 ) ) ;
#62334=CARTESIAN_POINT ( 'NONE',  ( -6.250023237292963607, -8.432397168068783699, 34.66272746175022945 ) ) ;
#62335=CARTESIAN_POINT ( 'NONE',  ( -1.384615384615383471, -5.180354513474913603, 36.12317359536750416 ) ) ;
#62336=ORIENTED_EDGE ( 'NONE', *, *, #15597, .T. ) ;
#62337=CARTESIAN_POINT ( 'NONE',  ( 16.08857570788537572, -2.892918686051582533, 31.69288490824015980 ) ) ;
#62338=ORIENTED_EDGE ( 'NONE', *, *, #44581, .T. ) ;
#62339=CARTESIAN_POINT ( 'NONE',  ( 9.915319043920545639, -11.76359900205217635, 32.36225158514719880 ) ) ;
#62340=CARTESIAN_POINT ( 'NONE',  ( 6.923076923076800782, -6.835583212225970762, 34.95778746994575670 ) ) ;
#62341=CARTESIAN_POINT ( 'NONE',  ( -0.2387589202700526325, -6.760870238392817200, 34.69528174975673096 ) ) ;
#62342=DIRECTION ( 'NONE',  ( -0.000000000000000000, -0.9396926207859093161, -0.3420201433256663259 ) ) ;
#62343=CARTESIAN_POINT ( 'NONE',  ( -13.60754234352223335, -2.523278758544489797, 31.42238647778637528 ) ) ;
#62344=ORIENTED_EDGE ( 'NONE', *, *, #85734, .F. ) ;
#62345=CIRCLE ( 'NONE', #22046, 0.2500000000000002220 ) ;
#62346=AXIS2_PLACEMENT_3D ( 'NONE', #61022, #62342, #55148 ) ;
#62347=ORIENTED_EDGE ( 'NONE', *, *, #79035, .F. ) ;
#62348=EDGE_CURVE ( 'NONE', #34190, #14282, #335, .T. ) ;
#62349=ORIENTED_EDGE ( 'NONE', *, *, #29526, .F. ) ;
#62350=EDGE_LOOP ( 'NONE', ( #73634, #41264 ) ) ;
#62351=LINE ( 'NONE', #34886, #24265 ) ;
#62352=CARTESIAN_POINT ( 'NONE',  ( 7.623227628637698317, -3.586966769969700763, 32.86292498521069660 ) ) ;
#62353=LINE ( 'NONE', #28131, #63860 ) ;
#62354=CARTESIAN_POINT ( 'NONE',  ( 2.177545098254091371, -11.47017969459903952, 32.78971311882034456 ) ) ;
#62355=CARTESIAN_POINT ( 'NONE',  ( 4.403791672194296680, -6.696923467548660192, 34.68552623307873972 ) ) ;
#62356=DIRECTION ( 'NONE',  ( -0.000000000000000000, 0.3420201433256694901, -0.9396926207859082059 ) ) ;
#62357=EDGE_LOOP ( 'NONE', ( #20049, #82531 ) ) ;
#62358=ORIENTED_EDGE ( 'NONE', *, *, #49818, .T. ) ;
#62359=EDGE_CURVE ( 'NONE', #71793, #5237, #61427, .T. ) ;
#62360=ORIENTED_EDGE ( 'NONE', *, *, #86022, .F. ) ;
#62361=CARTESIAN_POINT ( 'NONE',  ( 4.284371592079798674, -4.299079248970732792, 33.91157788607253565 ) ) ;
#62362=ORIENTED_EDGE ( 'NONE', *, *, #1445, .T. ) ;
#62363=CARTESIAN_POINT ( 'NONE',  ( 10.36540788444226102, -12.41269422305637171, 30.68257228309993323 ) ) ;
#62364=CARTESIAN_POINT ( 'NONE',  ( -2.242436736416281384, -9.442884908240271713, 34.35708131394835618 ) ) ;
#62366=ORIENTED_EDGE ( 'NONE', *, *, #7182, .F. ) ;
#62367=ORIENTED_EDGE ( 'NONE', *, *, #49514, .T. ) ;
#62368=CARTESIAN_POINT ( 'NONE',  ( -2.307692307692305711, -12.37446782046654192, 30.86335684631486131 ) ) ;
#62369=VERTEX_POINT ( 'NONE', #182 ) ;
#62370=FACE_BOUND ( 'NONE', #141, .T. ) ;
#62371=CARTESIAN_POINT ( 'NONE',  ( -5.999999999999998224, -2.833524468853757305, 32.15551576947925838 ) ) ;
#62372=VECTOR ( 'NONE', #27229, 1000.000000000000227 ) ;
#62376=CARTESIAN_POINT ( 'NONE',  ( -16.08859101433330707, -12.70778746994558439, 30.41441678777537305 ) ) ;
#62377=EDGE_CURVE ( 'NONE', #54531, #59736, #40735, .T. ) ;
#62379=CARTESIAN_POINT ( 'NONE',  ( -1.134615384613964384, -7.500000000000154543, 35.00000000000007105 ) ) ;
#62380=ORIENTED_EDGE ( 'NONE', *, *, #2536, .F. ) ;
#62381=CARTESIAN_POINT ( 'NONE',  ( 11.53846153846141753, -3.300289026999228881, 32.46337939537708905 ) ) ;
#62382=CARTESIAN_POINT ( 'NONE',  ( -5.869209559033047974, -3.957578996910242619, 33.62503395064540257 ) ) ;
#62383=CARTESIAN_POINT ( 'NONE',  ( 0.4615384615384611200, -11.69971097300155272, 32.46337939537588113 ) ) ;
#62384=DIRECTION ( 'NONE',  ( 0.000000000000000000, 0.000000000000000000, 1.000000000000000000 ) ) ;
#62385=CARTESIAN_POINT ( 'NONE',  ( -0.2115384615385252354, -7.565270445406050648, 34.75000000000000000 ) ) ;
#62386=FACE_BOUND ( 'NONE', #11840, .T. ) ;
#62387=LINE ( 'NONE', #703, #20361 ) ;
#62388=CARTESIAN_POINT ( 'NONE',  ( -4.153846153845845102, -2.506253911140614576, 30.00000000000323297 ) ) ;
#62389=EDGE_CURVE ( 'NONE', #51433, #47287, #52956, .T. ) ;
#62390=CARTESIAN_POINT ( 'NONE',  ( -6.989160334032800570, -12.10708131394839349, 31.69288490824020244 ) ) ;
#62391=CARTESIAN_POINT ( 'NONE',  ( -10.61538461538461320, -6.189225973068211317, 35.74407628777942847 ) ) ;
#62392=CARTESIAN_POINT ( 'NONE',  ( 8.992010310499178871, -2.847695495035523550, 31.58253572463339154 ) ) ;
#62393=CARTESIAN_POINT ( 'NONE',  ( -18.13069146666756382, -9.804603061927748442, 34.18744698557895845 ) ) ;
#62395=ORIENTED_EDGE ( 'NONE', *, *, #3737, .T. ) ;
#62396=CARTESIAN_POINT ( 'NONE',  ( -9.019230769230770051, -7.433931650972299465, 34.75000000000000711 ) ) ;
#62397=VERTEX_POINT ( 'NONE', #75398 ) ;
#62398=EDGE_CURVE ( 'NONE', #86296, #64502, #78819, .T. ) ;
#62399=CARTESIAN_POINT ( 'NONE',  ( 3.230769230769231726, -6.681629849574314051, 35.83090037661290239 ) ) ;
#62400=ORIENTED_EDGE ( 'NONE', *, *, #60040, .T. ) ;
#62401=CARTESIAN_POINT ( 'NONE',  ( 17.77707378248384629, -12.15238873228291716, 31.58232369045353849 ) ) ;
#62402=CARTESIAN_POINT ( 'NONE',  ( -18.06608341095587278, -2.538708090699994813, 30.37095296980875503 ) ) ;
#62403=ADVANCED_FACE ( 'NONE', ( #87894 ), #26158, .F. ) ;
#62404=VERTEX_POINT ( 'NONE', #67593 ) ;
#62405=CARTESIAN_POINT ( 'NONE',  ( 14.30769230769231015, -11.11383981884818262, 36.00935417666054406 ) ) ;
#62407=CARTESIAN_POINT ( 'NONE',  ( 4.153846153846032507, -9.442884908241554243, 34.35708131394783038 ) ) ;
#62408=CARTESIAN_POINT ( 'NONE',  ( -5.207071046654774271, -3.069018819979302926, 32.56621877034667278 ) ) ;
#62409=VECTOR ( 'NONE', #49645, 1000.000000000000000 ) ;
#62411=CARTESIAN_POINT ( 'NONE',  ( -17.07692307692307665, -12.34228464037088635, 31.77849191805839268 ) ) ;
#62412=FACE_OUTER_BOUND ( 'NONE', #60189, .T. ) ;
#62413=LINE ( 'NONE', #41722, #20999 ) ;
#62415=CARTESIAN_POINT ( 'NONE',  ( -18.22292695890684655, -11.43668979543635089, 33.22377378376089752 ) ) ;
#62416=DIRECTION ( 'NONE',  ( 0.000000000000000000, 0.7660444431189822323, -0.6427876096865344779 ) ) ;
#62418=VERTEX_POINT ( 'NONE', #66702 ) ;
#62422=CARTESIAN_POINT ( 'NONE',  ( -8.899378738962466784, -11.66186481527757302, 32.95055677023626117 ) ) ;
#62423=ORIENTED_EDGE ( 'NONE', *, *, #89130, .T. ) ;
#62424=CARTESIAN_POINT ( 'NONE',  ( 12.46153846153846168, -8.164416787775445883, 34.95778746994557906 ) ) ;
#62425=CARTESIAN_POINT ( 'NONE',  ( -17.07692307692307665, -9.058645607665452459, 34.76329471203371924 ) ) ;
#62426=CARTESIAN_POINT ( 'NONE',  ( -17.29974976940208364, -7.369208160676171460, 34.74850200257122879 ) ) ;
#62428=CARTESIAN_POINT ( 'NONE',  ( 7.846153846153846700, -1.242168528481310874, 33.36296068462461051 ) ) ;
#62429=EDGE_CURVE ( 'NONE', #82187, #59241, #61256, .T. ) ;
#62430=CARTESIAN_POINT ( 'NONE',  ( 13.38461538461526601, -2.625532179533778709, 30.86335684631627174 ) ) ;
#62431=CARTESIAN_POINT ( 'NONE',  ( 3.230769230769231726, -3.050289026998446396, 32.03036669348365706 ) ) ;
#62432=CARTESIAN_POINT ( 'NONE',  ( 5.076923076923075762, -4.098570777380720287, 33.41473453929634729 ) ) ;
#62433=DIRECTION ( 'NONE',  ( -0.000000000000000000, 0.1736481776669307198, -0.9848077530122080203 ) ) ;
#62435=ORIENTED_EDGE ( 'NONE', *, *, #50980, .F. ) ;
#62436=ORIENTED_EDGE ( 'NONE', *, *, #84193, .T. ) ;
#62439=ORIENTED_EDGE ( 'NONE', *, *, #87629, .T. ) ;
#62440=VECTOR ( 'NONE', #30575, 999.9999999999998863 ) ;
#62442=CARTESIAN_POINT ( 'NONE',  ( -4.088590582570128973, -3.300289026998475705, 32.46337939537591666 ) ) ;
#62444=CARTESIAN_POINT ( 'NONE',  ( -3.230769230769229949, -12.78798330534103123, 29.99999999999997868 ) ) ;
#62445=CARTESIAN_POINT ( 'NONE',  ( 17.07692307692307665, -5.180354513474913603, 36.12317359536750416 ) ) ;
#62447=CARTESIAN_POINT ( 'NONE',  ( 2.307692307692309264, -13.49023893513002648, 31.06009739812518688 ) ) ;
#62449=ADVANCED_FACE ( 'NONE', ( #5450 ), #32028, .F. ) ;
#62450=ORIENTED_EDGE ( 'NONE', *, *, #52722, .T. ) ;
#62451=EDGE_LOOP ( 'NONE', ( #37104, #70853, #68609, #61450 ) ) ;
#62453=ORIENTED_EDGE ( 'NONE', *, *, #28301, .T. ) ;
#62454=CARTESIAN_POINT ( 'NONE',  ( -3.230769230769351186, -2.625532179533779154, 30.86335684631627174 ) ) ;
#62456=CYLINDRICAL_SURFACE ( 'NONE', #65206, 0.2499999999999997502 ) ;
#62458=FACE_OUTER_BOUND ( 'NONE', #40429, .T. ) ;
#62459=CARTESIAN_POINT ( 'NONE',  ( -4.826923076921640465, -7.500000000000155431, 34.75000000000007105 ) ) ;
#62460=ORIENTED_EDGE ( 'NONE', *, *, #35714, .T. ) ;
#62461=EDGE_LOOP ( 'NONE', ( #51959, #71619, #64506, #9872 ) ) ;
#62462=EDGE_CURVE ( 'NONE', #62255, #36439, #5759, .T. ) ;
#62464=VERTEX_POINT ( 'NONE', #40573 ) ;
#62465=CARTESIAN_POINT ( 'NONE',  ( -1.384615384615383471, -12.78798330534103123, 29.99999999999997868 ) ) ;
#62466=CARTESIAN_POINT ( 'NONE',  ( -10.39260494640654819, -2.612705202774698421, 31.66806509827799943 ) ) ;
#62467=ORIENTED_EDGE ( 'NONE', *, *, #73094, .F. ) ;
#62468=CARTESIAN_POINT ( 'NONE',  ( -2.241623956689867914, -8.120952969808772792, 34.71129190929999453 ) ) ;
#62470=VERTEX_POINT ( 'NONE', #88770 ) ;
#62473=B_SPLINE_CURVE_WITH_KNOTS ( 'NONE', 3,
 ( #69352, #16598, #9411, #7649, #35109, #62572, #55825, #10741, #72876, #11637 ),
 .UNSPECIFIED., .F., .F.,
 ( 4, 2, 2, 2, 4 ),
 ( 0.000000000000000000, 0.0001954311564186863323, 0.0003908623128373726646, 0.0005862934692560590241, 0.0007817246256747453293 ),
 .UNSPECIFIED. ) ;
#62474=VERTEX_POINT ( 'NONE', #80220 ) ;
#62475=FACE_BOUND ( 'NONE', #3279, .T. ) ;
#62476=CARTESIAN_POINT ( 'NONE',  ( -18.00000000000012079, -8.613356846316285953, 34.62446782046622218 ) ) ;
#62477=CARTESIAN_POINT ( 'NONE',  ( 13.60762822870878352, -6.460100341425560444, 34.89618726649961644 ) ) ;
#62480=CARTESIAN_POINT ( 'NONE',  ( 4.946231610255516387, -9.804603061927743113, 34.18744698557895845 ) ) ;
#62481=B_SPLINE_CURVE_WITH_KNOTS ( 'NONE', 3,
 ( #15128, #62402, #42163, #1160, #42601, #8369, #83143, #61084, #28642, #55215 ),
 .UNSPECIFIED., .F., .F.,
 ( 4, 2, 2, 2, 4 ),
 ( 0.000000000000000000, 0.0001954339857564088296, 0.0003908679715128176592, 0.0005863019572692264618, 0.0007817359430256353185 ),
 .UNSPECIFIED. ) ;
#62482=DIRECTION ( 'NONE',  ( -0.000000000000000000, 0.9396926207859093161, -0.3420201433256663259 ) ) ;
#62483=CARTESIAN_POINT ( 'NONE',  ( -2.531177251416255825, -3.754499324213721234, 33.06261337010820256 ) ) ;
#62485=CARTESIAN_POINT ( 'NONE',  ( 0.4615384615384611755, -1.951392089020283160, 34.73218667398347748 ) ) ;
#62486=CARTESIAN_POINT ( 'NONE',  ( 13.13461538461538680, -7.500000000000001776, 34.75000000000000000 ) ) ;
#62487=EDGE_CURVE ( 'NONE', #71584, #70102, #3509, .T. ) ;
#62488=VERTEX_POINT ( 'NONE', #34692 ) ;
#62489=DIRECTION ( 'NONE',  ( 0.000000000000000000, 0.4999999999999960032, -0.8660254037844410391 ) ) ;
#62490=CARTESIAN_POINT ( 'NONE',  ( 5.076923076923075762, -13.78497067705608181, 32.30358669280327177 ) ) ;
#62492=CARTESIAN_POINT ( 'NONE',  ( 10.61538461538461675, -13.53365097954675988, 30.81389545987213552 ) ) ;
#62493=CARTESIAN_POINT ( 'NONE',  ( 2.557746727605762160, -4.818054556918156983, 34.26375889529406749 ) ) ;
#62494=VECTOR ( 'NONE', #1342, 999.9999999999998863 ) ;
#62495=FACE_BOUND ( 'NONE', #82609, .T. ) ;
#62496=DIRECTION ( 'NONE',  ( 0.000000000000000000, 0.1736481776669275834, 0.9848077530122086864 ) ) ;
#62497=DIRECTION ( 'NONE',  ( -0.000000000000000000, 0.8660254037844397068, -0.4999999999999978906 ) ) ;
#62498=CARTESIAN_POINT ( 'NONE',  ( 11.53846153846153832, -13.20930481340135110, 34.54067556320372745 ) ) ;
#62499=CARTESIAN_POINT ( 'NONE',  ( -15.36091644020745051, -9.418419913701741919, 34.36755862841477693 ) ) ;
#62500=CARTESIAN_POINT ( 'NONE',  ( -15.16551365949320562, -6.879047030191282275, 34.71129190930002295 ) ) ;
#62501=DIRECTION ( 'NONE',  ( 0.000000000000000000, 0.4999999999999960032, -0.8660254037844410391 ) ) ;
#62504=VECTOR ( 'NONE', #20593, 1000.000000000000000 ) ;
#62507=CARTESIAN_POINT ( 'NONE',  ( 6.923076923076924238, -1.129524287112498415, 32.06866353760679544 ) ) ;
#62508=CARTESIAN_POINT ( 'NONE',  ( -17.07692307692307665, -3.513871655860378418, 32.76840700105978499 ) ) ;
#62509=CARTESIAN_POINT ( 'NONE',  ( 14.53047197667037338, -9.418065098278013636, 34.63729479722530158 ) ) ;
#62511=CARTESIAN_POINT ( 'NONE',  ( -13.25382494364843389, -2.494656445102012565, 31.33466734024120015 ) ) ;
#62514=CARTESIAN_POINT ( 'NONE',  ( 2.242442375918224151, -2.255955759149247619, 30.00000000000013856 ) ) ;
#62515=LINE ( 'NONE', #55326, #21645 ) ;
#62516=CARTESIAN_POINT ( 'NONE',  ( -4.946397638689432164, -2.372941743896878286, 30.88044141588254377 ) ) ;
#62517=CARTESIAN_POINT ( 'NONE',  ( -15.16470087976679615, -11.16473453929635440, 33.15142922261926373 ) ) ;
#62519=CARTESIAN_POINT ( 'NONE',  ( 9.822833394071256663, -11.46989282347013095, 32.79007818306219946 ) ) ;
#62520=CARTESIAN_POINT ( 'NONE',  ( -14.08491276642389423, -3.236590943229499029, 32.36255958852954251 ) ) ;
#62521=EDGE_CURVE ( 'NONE', #72856, #13730, #17577, .T. ) ;
#62522=B_SPLINE_CURVE_WITH_KNOTS ( 'NONE', 3,
 ( #39348, #46534, #12305, #66805, #60038, #32565, #39786, #41108, #87545, #47403 ),
 .UNSPECIFIED., .F., .F.,
 ( 4, 2, 2, 2, 4 ),
 ( 0.000000000000000000, 0.0001954339857564080165, 0.0003908679715128160329, 0.0005863019572692240765, 0.0007817359430256320659 ),
 .UNSPECIFIED. ) ;
#62523=CARTESIAN_POINT ( 'NONE',  ( -13.38461538461550582, -3.835265460704628371, 33.15142922262033665 ) ) ;
#62525=CYLINDRICAL_SURFACE ( 'NONE', #3899, 0.2499999999999995559 ) ;
#62526=CARTESIAN_POINT ( 'NONE',  ( -17.07692307692307665, -6.681629849574314051, 35.83090037661290239 ) ) ;
#62528=EDGE_CURVE ( 'NONE', #85539, #18924, #42345, .T. ) ;
#62529=CARTESIAN_POINT ( 'NONE',  ( -5.750054590621955342, -12.45601412856602863, 31.48342859153981621 ) ) ;
#62530=CARTESIAN_POINT ( 'NONE',  ( -18.00000000000000000, -10.51840700105979387, 33.73612834413961536 ) ) ;
#62531=ORIENTED_EDGE ( 'NONE', *, *, #32903, .T. ) ;
#62532=CARTESIAN_POINT ( 'NONE',  ( -16.15384615384584777, -2.506253911140615021, 30.00000000000323297 ) ) ;
#62533=CARTESIAN_POINT ( 'NONE',  ( -1.384615384615505151, -4.481592998941358097, 33.73612834414048933 ) ) ;
#62534=ORIENTED_EDGE ( 'NONE', *, *, #52134, .F. ) ;
#62535=CARTESIAN_POINT ( 'NONE',  ( 9.692307692307695177, -12.62096338111211580, 30.90682066428153263 ) ) ;
#62536=CARTESIAN_POINT ( 'NONE',  ( 12.68431813051652313, -5.827830569534417471, 34.72679350104403539 ) ) ;
#62537=EDGE_CURVE ( 'NONE', #58896, #80991, #70025, .T. ) ;
#62538=ORIENTED_EDGE ( 'NONE', *, *, #1322, .T. ) ;
#62539=CARTESIAN_POINT ( 'NONE',  ( -39.05038313613820122, -12.75000000000000178, 29.75000000000000355 ) ) ;
#62540=AXIS2_PLACEMENT_3D ( 'NONE', #31633, #87046, #86141 ) ;
#62542=ADVANCED_FACE ( 'NONE', ( #41008 ), #83327, .F. ) ;
#62545=CARTESIAN_POINT ( 'NONE',  ( -15.48076923076922995, -7.500000000000001776, 35.00000000000000000 ) ) ;
#62546=LINE ( 'NONE', #7625, #87358 ) ;
#62547=ORIENTED_EDGE ( 'NONE', *, *, #42683, .T. ) ;
#62549=EDGE_CURVE ( 'NONE', #39262, #25331, #61415, .T. ) ;
#62550=CARTESIAN_POINT ( 'NONE',  ( -6.857821783564084228, -8.656820664281605460, 34.87096338111211224 ) ) ;
#62552=CARTESIAN_POINT ( 'NONE',  ( 3.230769230769231726, -11.91647553114624181, 32.58852847137148245 ) ) ;
#62553=CARTESIAN_POINT ( 'NONE',  ( 12.52760681254089725, -8.973038597847271092, 34.52809138561121216 ) ) ;
#62554=CARTESIAN_POINT ( 'NONE',  ( 2.557637717070352146, -11.56426240980093567, 33.07394671870546432 ) ) ;
#62555=CARTESIAN_POINT ( 'NONE',  ( -2.372962753653081958, -6.026961402152685388, 34.52809138561120506 ) ) ;
#62557=CARTESIAN_POINT ( 'NONE',  ( 0.7115384615385238476, -7.434744860731433036, 35.00000000000000000 ) ) ;
#62558=B_SPLINE_CURVE_WITH_KNOTS ( 'NONE', 3,
 ( #6778, #20738, #82011, #76575, #49545, #77020, #48205, #14423, #61713, #68479 ),
 .UNSPECIFIED., .F., .F.,
 ( 4, 2, 2, 2, 4 ),
 ( 0.0007817246256747530271, 0.0009771112852218978746, 0.001172497944769042939, 0.001367884604316188003, 0.001563271263863332851 ),
 .UNSPECIFIED. ) ;
#62559=B_SPLINE_CURVE_WITH_KNOTS ( 'NONE', 3,
 ( #68054, #5906, #32478, #60393, #33382, #52745, #73924, #87911, #45990, #81129 ),
 .UNSPECIFIED., .F., .F.,
 ( 4, 2, 2, 2, 4 ),
 ( 0.0007817359430256294638, 0.0009771253907249937212, 0.001172514838424358087, 0.001367904286123722453, 0.001563293733823093758 ),
 .UNSPECIFIED. ) ;
#62560=DIRECTION ( 'NONE',  ( -0.000000000000000000, 1.000000000000000000, 3.491481338843133355E-15 ) ) ;
#62561=B_SPLINE_CURVE_WITH_KNOTS ( 'NONE', 3,
 ( #966, #70758, #64418, #77073, #69867, #15378, #36532, #35192, #28436, #15820 ),
 .UNSPECIFIED., .F., .F.,
 ( 4, 2, 2, 2, 4 ),
 ( 0.0007817359430256282712, 0.0009771253907249939381, 0.001172514838424359388, 0.001367904286123725055, 0.001563293733823090722 ),
 .UNSPECIFIED. ) ;
#62562=B_SPLINE_CURVE_WITH_KNOTS ( 'NONE', 3,
 ( #74838, #75703, #83364, #35619, #14006, #41045, #68077, #41483, #41933, #6382 ),
 .UNSPECIFIED., .F., .F.,
 ( 4, 2, 2, 2, 4 ),
 ( 0.0007817359430256388964, 0.0009771253907250075990, 0.001172514838424376085, 0.001367904286123744571, 0.001563293733823113273 ),
 .UNSPECIFIED. ) ;
#62563=VERTEX_POINT ( 'NONE', #6767 ) ;
#62565=CARTESIAN_POINT ( 'NONE',  ( 9.562160482869472844, -4.460286881179643004, 33.72017969459903242 ) ) ;
#62567=EDGE_CURVE ( 'NONE', #51593, #67601, #74348, .T. ) ;
#62568=CARTESIAN_POINT ( 'NONE',  ( -18.25000000000000000, -7.500000000000001776, 35.00000000000000000 ) ) ;
#62569=EDGE_LOOP ( 'NONE', ( #4102, #37727, #7862, #9689 ) ) ;
#62570=EDGE_CURVE ( 'NONE', #69653, #30568, #24885, .T. ) ;
#62571=CARTESIAN_POINT ( 'NONE',  ( -18.00000000000000000, -3.050289026998447284, 32.03036669348365706 ) ) ;
#62572=CARTESIAN_POINT ( 'NONE',  ( -8.096177070375302876, -10.18141759479407327, 34.26406193332782379 ) ) ;
#62573=AXIS2_PLACEMENT_3D ( 'NONE', #85956, #44060, #25588 ) ;
#62574=EDGE_LOOP ( 'NONE', ( #77033, #64481 ) ) ;
#62575=DIRECTION ( 'NONE',  ( -0.000000000000000000, -0.7660444431189791237, -0.6427876096865379196 ) ) ;
#62577=ORIENTED_EDGE ( 'NONE', *, *, #88235, .T. ) ;
#62578=CARTESIAN_POINT ( 'NONE',  ( -16.37733109757010652, -3.754499324213721234, 33.06261337010820256 ) ) ;
#62579=EDGE_LOOP ( 'NONE', ( #1442, #2745, #89069, #47662 ) ) ;
#62580=CARTESIAN_POINT ( 'NONE',  ( -10.86538461538461320, -7.433931650972299465, 34.75000000000000711 ) ) ;
#62581=ORIENTED_EDGE ( 'NONE', *, *, #19900, .F. ) ;
#62582=EDGE_CURVE ( 'NONE', #59899, #87868, #86166, .T. ) ;
#62583=DIRECTION ( 'NONE',  ( -0.000000000000000000, 0.9396926207859092051, -0.3420201433256662704 ) ) ;
#62584=CARTESIAN_POINT ( 'NONE',  ( 10.61538461538449596, -5.219633306517616589, 34.19971097300220464 ) ) ;
#62585=FACE_BOUND ( 'NONE', #73474, .T. ) ;
#62586=FACE_OUTER_BOUND ( 'NONE', #4367, .T. ) ;
#62587=FACE_OUTER_BOUND ( 'NONE', #35027, .T. ) ;
#62588=B_SPLINE_CURVE_WITH_KNOTS ( 'NONE', 3,
 ( #63831, #3892, #36369, #43994, #3453, #9772, #16527, #79124, #71914, #24166 ),
 .UNSPECIFIED., .F., .F.,
 ( 4, 2, 2, 2, 4 ),
 ( 0.0007817359430256282712, 0.0009771253907249941549, 0.001172514838424359822, 0.001367904286123725489, 0.001563293733823091372 ),
 .UNSPECIFIED. ) ;
#62589=CARTESIAN_POINT ( 'NONE',  ( 15.48082365068268551, -2.544122305571458575, 31.48381861865057729 ) ) ;
#62590=CARTESIAN_POINT ( 'NONE',  ( 0.5267314498331145955, -2.255955759149235629, 29.99999999999988631 ) ) ;
#62591=CARTESIAN_POINT ( 'NONE',  ( -3.230769230769229949, -3.050289026998446396, 32.03036669348365706 ) ) ;
#62592=CARTESIAN_POINT ( 'NONE',  ( 2.307692307692309264, -11.11383981884818262, 36.00935417666054406 ) ) ;
#62594=FACE_OUTER_BOUND ( 'NONE', #68473, .T. ) ;
#62595=VERTEX_POINT ( 'NONE', #23947 ) ;
#62596=ADVANCED_FACE ( 'NONE', ( #37468 ), #24844, .F. ) ;
#62597=EDGE_LOOP ( 'NONE', ( #77114, #31635 ) ) ;
#62598=CARTESIAN_POINT ( 'NONE',  ( -1.319360245102545015, -5.094484230520773593, 34.41647553114626845 ) ) ;
#62599=CARTESIAN_POINT ( 'NONE',  ( 16.40390046548447245, -12.17597550085003633, 31.52189283813461884 ) ) ;
#62600=EDGE_CURVE ( 'NONE', #67350, #9817, #15075, .T. ) ;
#62601=CARTESIAN_POINT ( 'NONE',  ( -11.76138775597768671, -11.76352882383564769, 32.36236540154569497 ) ) ;
#62602=CARTESIAN_POINT ( 'NONE',  ( -16.85391023282967993, -10.01129605718032423, 34.36064277460058491 ) ) ;
#62603=CARTESIAN_POINT ( 'NONE',  ( 15.45354877203763877, -3.755027918224367767, 33.06320215134714857 ) ) ;
#62606=ORIENTED_EDGE ( 'NONE', *, *, #11437, .T. ) ;
#62607=DIRECTION ( 'NONE',  ( -0.000000000000000000, -0.1736481776669307198, -0.9848077530122080203 ) ) ;
#62608=CARTESIAN_POINT ( 'NONE',  ( 3.453780582382079967, -11.24521262558773671, 33.06293181088029343 ) ) ;
#62609=CARTESIAN_POINT ( 'NONE',  ( -3.361459833879538728, -11.37499894934982514, 33.29245874905763003 ) ) ;
#62611=CARTESIAN_POINT ( 'NONE',  ( -10.61538461538473399, -6.026961402154118019, 34.52809138561165270 ) ) ;
#62612=ORIENTED_EDGE ( 'NONE', *, *, #9339, .F. ) ;
#62613=EDGE_CURVE ( 'NONE', #11687, #52584, #38086, .T. ) ;
#62614=VERTEX_POINT ( 'NONE', #24396 ) ;
#62615=EDGE_LOOP ( 'NONE', ( #16854, #12629 ) ) ;
#62616=CARTESIAN_POINT ( 'NONE',  ( -6.923076923076922462, -8.120952969808772792, 34.71129190930000163 ) ) ;
#62618=CARTESIAN_POINT ( 'NONE',  ( -9.692307692307691624, -9.905515769479276145, 34.41647553114623292 ) ) ;
#62619=CARTESIAN_POINT ( 'NONE',  ( -17.07692307692307665, -3.050289026998446396, 32.03036669348365706 ) ) ;
#62620=B_SPLINE_CURVE_WITH_KNOTS ( 'NONE', 3,
 ( #50228, #9274, #50676, #17353, #58776, #78601, #44808, #72287, #87609, #25889 ),
 .UNSPECIFIED., .F., .F.,
 ( 4, 2, 2, 2, 4 ),
 ( 0.0007817246256747489071, 0.0009771112852218922368, 0.001172497944769035350, 0.001367884604316178679, 0.001563271263863322009 ),
 .UNSPECIFIED. ) ;
#62621=CARTESIAN_POINT ( 'NONE',  ( 18.00000000000000000, -8.973038597847269315, 34.52809138561121927 ) ) ;
#62622=CARTESIAN_POINT ( 'NONE',  ( -2.057746789344164995, -5.057305518903949526, 34.11320923018887896 ) ) ;
#62623=CARTESIAN_POINT ( 'NONE',  ( 14.55763782604044998, -4.336752205174649433, 33.62275283266504289 ) ) ;
#62624=VERTEX_POINT ( 'NONE', #85670 ) ;
#62625=CARTESIAN_POINT ( 'NONE',  ( 4.153846153846032507, -4.481592998941358097, 33.73612834414048933 ) ) ;
#62626=CARTESIAN_POINT ( 'NONE',  ( -0.6844654204453102242, -5.582147617184174848, 34.63737895849758530 ) ) ;
#62627=VERTEX_POINT ( 'NONE', #4585 ) ;
#62628=CARTESIAN_POINT ( 'NONE',  ( -9.469296340694841163, -4.187068189119699468, 33.49521262558774026 ) ) ;
#62629=DIRECTION ( 'NONE',  ( -0.000000000000000000, 0.9848077530122086864, -0.1736481776669273891 ) ) ;
#62630=CARTESIAN_POINT ( 'NONE',  ( -17.14219307747939425, -12.16647553114622049, 32.15551576947930812 ) ) ;
#62631=CARTESIAN_POINT ( 'NONE',  ( 6.249945409378045547, -9.357781135181031829, 34.66075350412533851 ) ) ;
#62632=DIRECTION ( 'NONE',  ( -0.000000000000000000, 1.000000000000000000, -0.000000000000000000 ) ) ;
#62633=CARTESIAN_POINT ( 'NONE',  ( -3.480792454990688789, -10.92453946501458439, 33.72985991061850086 ) ) ;
#62634=LINE ( 'NONE', #49130, #14863 ) ;
#62636=ORIENTED_EDGE ( 'NONE', *, *, #30057, .T. ) ;
#62637=CARTESIAN_POINT ( 'NONE',  ( -4.946084746436313573, -7.277220318596959281, 34.99547417642776992 ) ) ;
#62638=CARTESIAN_POINT ( 'NONE',  ( 12.68455130563185662, -4.762714258010881885, 34.23016756924214832 ) ) ;
#62639=DIRECTION ( 'NONE',  ( -0.000000000000000000, -0.7660444431189791237, -0.6427876096865379196 ) ) ;
#62641=ORIENTED_EDGE ( 'NONE', *, *, #31804, .T. ) ;
#62642=DIRECTION ( 'NONE',  ( -0.000000000000000000, -0.5000000000000009992, -0.8660254037844380415 ) ) ;
#62644=VECTOR ( 'NONE', #46210, 1000.000000000000000 ) ;
#62645=CARTESIAN_POINT ( 'NONE',  ( -1.384615384615383471, -6.386643153685126251, 34.62446782046654192 ) ) ;
#62646=CARTESIAN_POINT ( 'NONE',  ( 14.17700084102474989, -3.062553014421049546, 32.05460306192773601 ) ) ;
#62647=EDGE_CURVE ( 'NONE', #71008, #41980, #1280, .T. ) ;
#62648=ORIENTED_EDGE ( 'NONE', *, *, #34899, .F. ) ;
#62649=CARTESIAN_POINT ( 'NONE',  ( -16.28399412357784826, -6.809168938359901446, 34.95455904226513866 ) ) ;
#62650=LINE ( 'NONE', #2718, #87228 ) ;
#62651=CARTESIAN_POINT ( 'NONE',  ( -2.307692307692305711, -5.471508081941601098, 34.59228464037088457 ) ) ;
#62652=EDGE_LOOP ( 'NONE', ( #38322, #40609, #6847, #83139 ) ) ;
#62653=EDGE_CURVE ( 'NONE', #55982, #5477, #51824, .T. ) ;
#62654=FACE_OUTER_BOUND ( 'NONE', #6110, .T. ) ;
#62655=B_SPLINE_CURVE_WITH_KNOTS ( 'NONE', 3,
 ( #68304, #12914, #80499, #74177, #46260, #66534, #6607, #54336, #60652, #73750 ),
 .UNSPECIFIED., .F., .F.,
 ( 4, 2, 2, 2, 4 ),
 ( 0.0007817246336856284103, 0.0009771112958940092897, 0.001172497958102390169, 0.001367884620310771265, 0.001563271282519152145 ),
 .UNSPECIFIED. ) ;
#62656=ORIENTED_EDGE ( 'NONE', *, *, #62165, .T. ) ;
#62658=CARTESIAN_POINT ( 'NONE',  ( -10.86540785267758125, -2.823816976329319051, 31.52131813110795733 ) ) ;
#62659=VECTOR ( 'NONE', #74491, 1000.000000000000000 ) ;
#62660=ORIENTED_EDGE ( 'NONE', *, *, #13104, .F. ) ;
#62661=FACE_OUTER_BOUND ( 'NONE', #28329, .T. ) ;
#62662=CARTESIAN_POINT ( 'NONE',  ( 4.376858997939548246, -9.172514111537584114, 34.72667873470787470 ) ) ;
#62663=CARTESIAN_POINT ( 'NONE',  ( -10.74607608205217346, -5.582088688514999397, 34.36776431015576350 ) ) ;
#62664=VECTOR ( 'NONE', #31861, 1000.000000000000227 ) ;
#62665=ADVANCED_FACE ( 'NONE', ( #17661 ), #59076, .F. ) ;
#62666=DIRECTION ( 'NONE',  ( 0.000000000000000000, 0.1736481776669267785, -0.9848077530122087975 ) ) ;
#62668=VERTEX_POINT ( 'NONE', #38820 ) ;
#62669=EDGE_LOOP ( 'NONE', ( #6294, #13408 ) ) ;
#62670=FACE_BOUND ( 'NONE', #20925, .T. ) ;
#62671=ORIENTED_EDGE ( 'NONE', *, *, #31751, .F. ) ;
#62673=EDGE_CURVE ( 'NONE', #74204, #61048, #50964, .T. ) ;
#62674=CARTESIAN_POINT ( 'NONE',  ( 6.923076923077238654, -2.255955759149395501, 30.00000000000324363 ) ) ;
#62675=EDGE_CURVE ( 'NONE', #66285, #65590, #59350, .T. ) ;
#62678=EDGE_LOOP ( 'NONE', ( #55673, #15383, #66115, #76571, #20898, #47811, #76076, #68462, #41246, #72340, #31203, #7770, #47508, #40097, #26858, #73252, #15024, #56678, #53228, #16361, #47608, #13116, #16621, #4669, #8202, #33401, #25036, #21153, #76087, #85430, #50807, #64369, #69411, #18817, #59416, #35340, #10717, #77865, #69838, #8512, #63127, #1242, #77036, #52614, #82739, #41314, #50004, #33648, #30770, #25568, #30299, #74698, #75571, #29629, #33683, #13565, #7022, #45966, #33106, #43980, #52480, #8655, #65366, #65879, #8958, #72813, #82092, #24762, #38769, #61898, #69882, #13309, #75976, #67734, #85807, #73597, #45842, #84981, #25041, #18199, #17831, #9002, #77556, #70856, #38071, #17192, #65483, #39295, #81664, #4161, #73932, #74110, #16388, #56349, #77867, #75502, #8054, #84751, #24018, #46384, #52403, #42079, #76312, #86450, #78719, #16125, #68553, #41555, #7787, #7824, #49473, #75548, #24959, #64077, #48414, #47733, #30372, #71294, #52715, #70121, #68756, #40328, #63891, #41515, #69373, #37414, #8414 ) ) ;
#62679=ORIENTED_EDGE ( 'NONE', *, *, #59980, .T. ) ;
#62681=CARTESIAN_POINT ( 'NONE',  ( -0.3307466537136761753, -3.062576670634119758, 32.05464942895959979 ) ) ;
#62682=ORIENTED_EDGE ( 'NONE', *, *, #31916, .F. ) ;
#62683=EDGE_CURVE ( 'NONE', #10877, #87392, #87467, .T. ) ;
#62684=CARTESIAN_POINT ( 'NONE',  ( 0.4615384615383382183, -10.33852847137269571, 34.16647553114546554 ) ) ;
#62685=CARTESIAN_POINT ( 'NONE',  ( -6.923076923076607159, -2.255955759149395501, 30.00000000000324363 ) ) ;
#62686=CARTESIAN_POINT ( 'NONE',  ( 13.51514082284902862, -11.66157788607254098, 32.95092075102925833 ) ) ;
#62687=CARTESIAN_POINT ( 'NONE',  ( 8.992242120843618736, -9.086983370893049639, 34.49168942202179267 ) ) ;
#62688=FACE_OUTER_BOUND ( 'NONE', #14573, .T. ) ;
#62690=CARTESIAN_POINT ( 'NONE',  ( 11.76124107972994359, -8.496831190052093419, 34.64984203495476578 ) ) ;
#62691=ORIENTED_EDGE ( 'NONE', *, *, #29609, .F. ) ;
#62692=AXIS2_PLACEMENT_3D ( 'NONE', #59272, #30904, #52067 ) ;
#62693=ORIENTED_EDGE ( 'NONE', *, *, #75688, .T. ) ;
#62695=ORIENTED_EDGE ( 'NONE', *, *, #11925, .F. ) ;
#62696=CARTESIAN_POINT ( 'NONE',  ( -5.999999999999998224, -6.435427911321262684, 35.78748833219616898 ) ) ;
#62699=CARTESIAN_POINT ( 'NONE',  ( -13.51476259405360203, -6.001485441113819874, 34.52039167877662607 ) ) ;
#62700=CARTESIAN_POINT ( 'NONE',  ( -17.93474486048716088, -5.941354392334603496, 34.76329471203374055 ) ) ;
#62701=CARTESIAN_POINT ( 'NONE',  ( -6.792551221313355647, -3.816742781228458448, 33.13167719472716044 ) ) ;
#62702=EDGE_CURVE ( 'NONE', #2541, #41728, #37807, .T. ) ;
#62703=DIRECTION ( 'NONE',  ( 0.000000000000000000, 0.000000000000000000, -1.000000000000000000 ) ) ;
#62704=CARTESIAN_POINT ( 'NONE',  ( 9.692307692307695177, -3.513871655860378418, 32.76840700105978499 ) ) ;
#62706=ORIENTED_EDGE ( 'NONE', *, *, #74069, .F. ) ;
#62707=CARTESIAN_POINT ( 'NONE',  ( 17.32686848630112308, -12.07971442181321997, 32.31769673815850297 ) ) ;
#62708=CARTESIAN_POINT ( 'NONE',  ( -0.4615384615384611200, -8.973038597847269315, 34.52809138561121927 ) ) ;
#62709=DIRECTION ( 'NONE',  ( -0.000000000000000000, 0.8660254037844399289, -0.4999999999999980016 ) ) ;
#62710=CARTESIAN_POINT ( 'NONE',  ( 6.923076923076924238, -9.058645607665452459, 34.76329471203371924 ) ) ;
#62711=VERTEX_POINT ( 'NONE', #87026 ) ;
#62712=CYLINDRICAL_SURFACE ( 'NONE', #2525, 0.2499999999999986955 ) ;
#62713=VERTEX_POINT ( 'NONE', #39273 ) ;
#62714=FACE_BOUND ( 'NONE', #11174, .T. ) ;
#62715=CARTESIAN_POINT ( 'NONE',  ( -15.90384615384615330, -2.499999999999998668, 29.75000000000000355 ) ) ;
#62717=CARTESIAN_POINT ( 'NONE',  ( 4.219913487196228274, -2.486705287966279876, 31.30864560766543647 ) ) ;
#62718=CARTESIAN_POINT ( 'NONE',  ( -7.053553631193387297, -7.276988635370452485, 34.74523720219453793 ) ) ;
#62719=EDGE_LOOP ( 'NONE', ( #15323, #86282, #67842, #5287 ) ) ;
#62720=CARTESIAN_POINT ( 'NONE',  ( -12.59168567097668401, -10.19110544564092002, 33.96427741523702792 ) ) ;
#62721=CARTESIAN_POINT ( 'NONE',  ( -3.480792454990687013, -2.341070481393819236, 30.72580821765574299 ) ) ;
#62723=DIRECTION ( 'NONE',  ( 0.000000000000000000, 0.6427876096865373645, -0.7660444431189797898 ) ) ;
#62725=B_SPLINE_CURVE_WITH_KNOTS ( 'NONE', 3,
 ( #11886, #88014, #26274, #19078, #61371, #88883, #68150, #5562, #80345, #46104 ),
 .UNSPECIFIED., .F., .F.,
 ( 4, 2, 2, 2, 4 ),
 ( 0.000000000000000000, 0.0001954339881912783286, 0.0003908679763825566571, 0.0005863019645738349857, 0.0007817359527651133143 ),
 .UNSPECIFIED. ) ;
#62726=AXIS2_PLACEMENT_3D ( 'NONE', #55136, #88508, #61442 ) ;
#62727=CARTESIAN_POINT ( 'NONE',  ( 12.71153846153847766, -2.249999999999999112, 29.81603969181029967 ) ) ;
#62729=B_SPLINE_CURVE_WITH_KNOTS ( 'NONE', 3,
 ( #18387, #46743, #31449, #79645, #45848, #4882, #73329, #32344, #59811, #12517 ),
 .UNSPECIFIED., .F., .F.,
 ( 4, 2, 2, 2, 4 ),
 ( 0.000000000000000000, 0.0001954311564186874978, 0.0003908623128373749957, 0.0005862934692560624935, 0.0007817246256747499913 ),
 .UNSPECIFIED. ) ;
#62730=CARTESIAN_POINT ( 'NONE',  ( 4.219101293358991533, -3.083524468853784839, 32.58852847137153930 ) ) ;
#62731=ORIENTED_EDGE ( 'NONE', *, *, #20149, .F. ) ;
#62732=CARTESIAN_POINT ( 'NONE',  ( 17.32692307692449418, -7.500000000000154543, 35.00000000000007105 ) ) ;
#62733=CARTESIAN_POINT ( 'NONE',  ( -4.283993363284368527, -2.882441371585227063, 31.66841991370171527 ) ) ;
#62734=CARTESIAN_POINT ( 'NONE',  ( -18.00000000000000000, -12.75000000000000711, 29.49999999999997868 ) ) ;
#62735=DIRECTION ( 'NONE',  ( 1.000000000000000000, 0.000000000000000000, 0.000000000000000000 ) ) ;
#62736=CARTESIAN_POINT ( 'NONE',  ( 15.23076923076923173, -5.471508081941601098, 34.59228464037088457 ) ) ;
#62737=CARTESIAN_POINT ( 'NONE',  ( -5.777220331021931443, -6.717445702608402236, 34.94155399931962336 ) ) ;
#62738=CARTESIAN_POINT ( 'NONE',  ( 16.40379167219429490, -5.852078868378311149, 34.47109172314383585 ) ) ;
#62739=CARTESIAN_POINT ( 'NONE',  ( -18.00000000000000000, -12.50000000000000000, 29.74999999999997868 ) ) ;
#62741=VERTEX_POINT ( 'NONE', #73497 ) ;
#62742=CARTESIAN_POINT ( 'NONE',  ( -17.86920819217521483, -8.999086150933472084, 34.52020707165672064 ) ) ;
#62743=ORIENTED_EDGE ( 'NONE', *, *, #70715, .T. ) ;
#62744=ORIENTED_EDGE ( 'NONE', *, *, #69652, .T. ) ;
#62745=DIRECTION ( 'NONE',  ( 0.000000000000000000, 1.000000000000000000, 0.000000000000000000 ) ) ;
#62746=VERTEX_POINT ( 'NONE', #5482 ) ;
#62747=CARTESIAN_POINT ( 'NONE',  ( -5.934744860487158213, -12.70778746994558439, 30.41441678777537305 ) ) ;
#62748=CARTESIAN_POINT ( 'NONE',  ( -7.846153846153967493, -8.656820664282941280, 34.87096338111179961 ) ) ;
#62749=CARTESIAN_POINT ( 'NONE',  ( 6.250054311638314708, -3.136992222400443175, 32.19305428654138979 ) ) ;
#62750=DIRECTION ( 'NONE',  ( -0.000000000000000000, -0.7660444431189791237, -0.6427876096865379196 ) ) ;
#62751=CARTESIAN_POINT ( 'NONE',  ( 6.223011351612851350, -2.554770724473668153, 30.48948780036025852 ) ) ;
#62752=CARTESIAN_POINT ( 'NONE',  ( 8.638539302563209787, -11.18331474514187995, 33.13161551792790505 ) ) ;
#62753=CARTESIAN_POINT ( 'NONE',  ( 16.08776274289027697, -11.69971097300155272, 32.46337939537587403 ) ) ;
#62754=CARTESIAN_POINT ( 'NONE',  ( 6.856994543716784740, -12.34228464037088280, 31.77849191805838558 ) ) ;
#62755=VECTOR ( 'NONE', #43378, 1000.000000000000227 ) ;
#62756=DIRECTION ( 'NONE',  ( -0.000000000000000000, -0.1736481776669307198, -0.9848077530122080203 ) ) ;
#62757=CARTESIAN_POINT ( 'NONE',  ( -2.057637887778853258, -2.920487667080175154, 32.31805714834170828 ) ) ;
#62758=CARTESIAN_POINT ( 'NONE',  ( 6.000000000000001776, -11.35647404775217417, 33.31231777344666511 ) ) ;
#62759=CARTESIAN_POINT ( 'NONE',  ( 11.78840705680968171, -5.057305518903948638, 34.11320923018887896 ) ) ;
#62761=ORIENTED_EDGE ( 'NONE', *, *, #19951, .F. ) ;
#62762=DIRECTION ( 'NONE',  ( -0.000000000000000000, -0.1736481776669307198, -0.9848077530122080203 ) ) ;
#62763=CARTESIAN_POINT ( 'NONE',  ( 0.000000000000000000, 0.000000000000000000, 0.000000000000000000 ) ) ;
#62764=CARTESIAN_POINT ( 'NONE',  ( -3.007757879156382153, -2.758310577978208666, 31.33698337089302299 ) ) ;
#62765=DIRECTION ( 'NONE',  ( -0.000000000000000000, -0.6427876096865404731, -0.7660444431189771253 ) ) ;
#62766=EDGE_LOOP ( 'NONE', ( #1154, #57376 ) ) ;
#62768=CARTESIAN_POINT ( 'NONE',  ( -4.153846153846273204, -6.879047030192662504, 34.71129190930017927 ) ) ;
#62769=CARTESIAN_POINT ( 'NONE',  ( -9.626240358957616650, -10.67929555188718282, 33.92786785259544757 ) ) ;
#62770=DIRECTION ( 'NONE',  ( -0.000000000000000000, -0.5000000000000009992, -0.8660254037844380415 ) ) ;
#62771=ORIENTED_EDGE ( 'NONE', *, *, #79541, .T. ) ;
#62772=CARTESIAN_POINT ( 'NONE',  ( -14.55771553191376277, -12.68155406624981119, 30.59749803192733708 ) ) ;
#62773=EDGE_LOOP ( 'NONE', ( #53946, #3138, #4996, #84863 ) ) ;
#62774=CARTESIAN_POINT ( 'NONE',  ( 16.15384615384615330, -9.058645607665452459, 34.76329471203371924 ) ) ;
#62776=CARTESIAN_POINT ( 'NONE',  ( 4.284684484332913712, -7.277220318596959281, 34.99547417642776992 ) ) ;
#62777=VECTOR ( 'NONE', #87844, 1000.000000000000000 ) ;
#62778=LINE ( 'NONE', #28578, #8531 ) ;
#62780=CARTESIAN_POINT ( 'NONE',  ( -6.857821783564084228, -2.657715359629131857, 31.77849191805844242 ) ) ;
#62781=ORIENTED_EDGE ( 'NONE', *, *, #26914, .F. ) ;
#62782=ORIENTED_EDGE ( 'NONE', *, *, #86108, .T. ) ;
#62783=VERTEX_POINT ( 'NONE', #81583 ) ;
#62784=ORIENTED_EDGE ( 'NONE', *, *, #1993, .T. ) ;
#62785=ADVANCED_FACE ( 'NONE', ( #41036 ), #47336, .F. ) ;
#62786=CARTESIAN_POINT ( 'NONE',  ( -5.999999999999998224, -11.16473453929635440, 33.15142922261926373 ) ) ;
#62787=CYLINDRICAL_SURFACE ( 'NONE', #70446, 0.2499999999999995837 ) ;
#62788=CARTESIAN_POINT ( 'NONE',  ( -12.23875879256039667, -12.47679350104403007, 31.42216943046555855 ) ) ;
#62789=CARTESIAN_POINT ( 'NONE',  ( -16.15384615384627409, -11.67786785259630911, 32.92929555188603530 ) ) ;
#62790=CARTESIAN_POINT ( 'NONE',  ( 16.15384615384615330, -2.900454961884010974, 35.62045528018868623 ) ) ;
#62791=CARTESIAN_POINT ( 'NONE',  ( 14.55774661933062575, -9.943054286541403997, 34.11300777759954883 ) ) ;
#62793=ORIENTED_EDGE ( 'NONE', *, *, #20541, .T. ) ;
#62794=ORIENTED_EDGE ( 'NONE', *, *, #88523, .F. ) ;
#62795=DIRECTION ( 'NONE',  ( -0.000000000000000000, 0.7660444431189791237, -0.6427876096865379196 ) ) ;
#62796=ORIENTED_EDGE ( 'NONE', *, *, #75872, .F. ) ;
#62797=CARTESIAN_POINT ( 'NONE',  ( 16.37685750545900376, -8.239487800360276282, 34.69522927552633718 ) ) ;
#62798=CARTESIAN_POINT ( 'NONE',  ( 13.60762822870878530, -4.026326845037962343, 33.68677907613344047 ) ) ;
#62799=CARTESIAN_POINT ( 'NONE',  ( 9.627037246346919375, -2.625532179533445198, 30.86335684631481513 ) ) ;
#62800=EDGE_CURVE ( 'NONE', #30672, #14427, #18515, .T. ) ;
#62801=CARTESIAN_POINT ( 'NONE',  ( 13.51540719244017374, -8.147973898785416225, 34.70805048591653730 ) ) ;
#62802=EDGE_CURVE ( 'NONE', #81013, #46051, #60856, .T. ) ;
#62803=ORIENTED_EDGE ( 'NONE', *, *, #17005, .T. ) ;
#62804=ORIENTED_EDGE ( 'NONE', *, *, #87452, .F. ) ;
#62805=CARTESIAN_POINT ( 'NONE',  ( 3.903869409797561474, -4.075325502946086864, 33.72974371597207721 ) ) ;
#62806=B_SPLINE_CURVE_WITH_KNOTS ( 'NONE', 3,
 ( #58528, #4031, #85578, #17568, #50877, #79714, #23853, #72949, #72053, #24303 ),
 .UNSPECIFIED., .F., .F.,
 ( 4, 2, 2, 2, 4 ),
 ( 0.000000000000000000, 0.0001954311564186858986, 0.0003908623128373717973, 0.0005862934692560577230, 0.0007817246256747435946 ),
 .UNSPECIFIED. ) ;
#62807=AXIS2_PLACEMENT_3D ( 'NONE', #15273, #35993, #75631 ) ;
#62808=EDGE_LOOP ( 'NONE', ( #73143, #5517, #47963, #80201 ) ) ;
#62809=FACE_BOUND ( 'NONE', #81095, .T. ) ;
#62810=CARTESIAN_POINT ( 'NONE',  ( 4.826899852701619587, -4.931416488878822335, 34.32920672191015399 ) ) ;
#62811=ADVANCED_FACE ( 'NONE', ( #26632 ), #40599, .F. ) ;
#62813=EDGE_LOOP ( 'NONE', ( #79548, #58372 ) ) ;
#62814=CARTESIAN_POINT ( 'NONE',  ( -4.403846153846163070, -2.499999999999999556, 29.81609845454692120 ) ) ;
#62815=FACE_OUTER_BOUND ( 'NONE', #55377, .T. ) ;
#62817=DIRECTION ( 'NONE',  ( 0.000000000000000000, 0.9396926207859126468, -0.3420201433256571111 ) ) ;
#62818=CARTESIAN_POINT ( 'NONE',  ( -17.01085472592063397, -2.538708090699994813, 30.37095296980875503 ) ) ;
#62819=ORIENTED_EDGE ( 'NONE', *, *, #44983, .F. ) ;
#62820=CARTESIAN_POINT ( 'NONE',  ( 5.999999999999880096, -8.613356846316285953, 34.62446782046622218 ) ) ;
#62821=CARTESIAN_POINT ( 'NONE',  ( 3.230769230769110045, -4.481592998941358097, 33.73612834414048933 ) ) ;
#62822=FACE_OUTER_BOUND ( 'NONE', #39676, .T. ) ;
#62824=CARTESIAN_POINT ( 'NONE',  ( -15.16551365949320562, -11.94971097300157403, 32.03036669348361443 ) ) ;
#62825=FACE_BOUND ( 'NONE', #10763, .T. ) ;
#62826=CARTESIAN_POINT ( 'NONE',  ( 5.010839665967195877, -11.16473453929635440, 33.15142922261925662 ) ) ;
#62828=CARTESIAN_POINT ( 'NONE',  ( 11.66898697669518548, -12.15418822224088657, 32.17964115625579069 ) ) ;
#62829=CARTESIAN_POINT ( 'NONE',  ( -11.53846153846165912, -11.48612834414049644, 32.76840700105863391 ) ) ;
#62830=CARTESIAN_POINT ( 'NONE',  ( -18.25002322422145085, -2.985938066672159330, 32.43141759479405550 ) ) ;
#62831=CARTESIAN_POINT ( 'NONE',  ( -39.05038313613820122, -2.249999999999998668, 29.75000000000000355 ) ) ;
#62833=ORIENTED_EDGE ( 'NONE', *, *, #46126, .T. ) ;
#62834=B_SPLINE_CURVE_WITH_KNOTS ( 'NONE', 3,
 ( #17780, #45234, #23630, #85344, #65946, #86701, #51081, #36707, #2463, #24967 ),
 .UNSPECIFIED., .F., .F.,
 ( 4, 2, 2, 2, 4 ),
 ( 0.000000000000000000, 0.0001954339857564080707, 0.0003908679715128161414, 0.0005863019572692241849, 0.0007817359430256322827 ),
 .UNSPECIFIED. ) ;
#62835=LINE ( 'NONE', #55646, #69193 ) ;
#62837=LINE ( 'NONE', #62399, #17625 ) ;
#62838=AXIS2_PLACEMENT_3D ( 'NONE', #60011, #65436, #45607 ) ;
#62839=ORIENTED_EDGE ( 'NONE', *, *, #26025, .T. ) ;
#62840=CARTESIAN_POINT ( 'NONE',  ( -11.31568199719312418, -2.847695495035523550, 31.58253572463339154 ) ) ;
#62841=FACE_OUTER_BOUND ( 'NONE', #24688, .T. ) ;
#62842=ORIENTED_EDGE ( 'NONE', *, *, #55866, .T. ) ;
#62843=CARTESIAN_POINT ( 'NONE',  ( -9.442307692307755573, -7.565270445406050648, 34.75000000000000000 ) ) ;
#62846=CARTESIAN_POINT ( 'NONE',  ( 16.15384615384603251, -8.656820664282941280, 34.87096338111179961 ) ) ;
#62847=AXIS2_PLACEMENT_3D ( 'NONE', #70396, #35728, #62289 ) ;
#62848=CARTESIAN_POINT ( 'NONE',  ( 10.61538461538461675, -13.37000171582298513, 34.34916445242398453 ) ) ;
#62849=CARTESIAN_POINT ( 'NONE',  ( 11.28843830116857383, -2.823816976329317274, 31.52131813110795733 ) ) ;
#62850=LINE ( 'NONE', #69627, #2223 ) ;
#62851=CARTESIAN_POINT ( 'NONE',  ( 14.30769230769231015, -1.242168528481310874, 33.36296068462461051 ) ) ;
#62853=CARTESIAN_POINT ( 'NONE',  ( -15.23076923076922995, -11.35647404775217417, 33.31231777344666511 ) ) ;
#62854=CARTESIAN_POINT ( 'NONE',  ( 10.86543892702293057, -11.28795663066794575, 33.01431243580653785 ) ) ;
#62856=B_SPLINE_CURVE_WITH_KNOTS ( 'NONE', 3,
 ( #5183, #32651, #87618, #52024, #66441, #6076, #25003, #61009, #19581, #25454 ),
 .UNSPECIFIED., .F., .F.,
 ( 4, 2, 2, 2, 4 ),
 ( 0.0007817359430256328248, 0.0009771253907249997928, 0.001172514838424366544, 0.001367904286123733295, 0.001563293733823100263 ),
 .UNSPECIFIED. ) ;
#62857=CARTESIAN_POINT ( 'NONE',  ( -13.38461538461550759, -12.70778746994576025, 30.41441678777401236 ) ) ;
#62858=B_SPLINE_CURVE_WITH_KNOTS ( 'NONE', 3,
 ( #65044, #3354, #51979, #65502, #30826, #72704, #11014, #59637, #79475, #16872 ),
 .UNSPECIFIED., .F., .F.,
 ( 4, 2, 2, 2, 4 ),
 ( 0.000000000000000000, 0.0001954339857564097512, 0.0003908679715128195024, 0.0005863019572692292807, 0.0007817359430256390048 ),
 .UNSPECIFIED. ) ;
#62860=CARTESIAN_POINT ( 'NONE',  ( 5.999999999999880096, -4.481592998941358097, 33.73612834414048933 ) ) ;
#62862=ORIENTED_EDGE ( 'NONE', *, *, #11789, .F. ) ;
#62863=CARTESIAN_POINT ( 'NONE',  ( 6.673076923076925127, -7.566083408709834757, 34.74999999999999289 ) ) ;
#62864=CARTESIAN_POINT ( 'NONE',  ( 1.134615384615387246, -7.500000000000001776, 35.00000000000000000 ) ) ;
#62865=CARTESIAN_POINT ( 'NONE',  ( -16.82692307692164135, -7.500000000000155431, 34.75000000000007105 ) ) ;
#62866=CARTESIAN_POINT ( 'NONE',  ( -14.55771554498526932, -11.86270091957321249, 32.19358267280087915 ) ) ;
#62867=CARTESIAN_POINT ( 'NONE',  ( 9.692307692307570832, -12.16647553114689728, 32.15551576947799362 ) ) ;
#62868=ADVANCED_FACE ( 'NONE', ( #54090 ), #67179, .F. ) ;
#62871=CYLINDRICAL_SURFACE ( 'NONE', #37965, 0.2499999999999997502 ) ;
#62872=VECTOR ( 'NONE', #48647, 1000.000000000000227 ) ;
#62873=ORIENTED_EDGE ( 'NONE', *, *, #82463, .F. ) ;
#62874=ORIENTED_EDGE ( 'NONE', *, *, #1948, .T. ) ;
#62875=VECTOR ( 'NONE', #30622, 1000.000000000000000 ) ;
#62876=ORIENTED_EDGE ( 'NONE', *, *, #27684, .F. ) ;
#62878=CARTESIAN_POINT ( 'NONE',  ( -16.40386937806761125, -3.520140089381496473, 33.17453946501458262 ) ) ;
#62879=CARTESIAN_POINT ( 'NONE',  ( -4.153846153846152411, -3.050289026998446396, 32.03036669348365706 ) ) ;
#62880=ADVANCED_FACE ( 'NONE', ( #76593 ), #27517, .F. ) ;
#62881=CARTESIAN_POINT ( 'NONE',  ( 2.177000841024750333, -5.582088688514999397, 34.36776431015576350 ) ) ;
#62882=DIRECTION ( 'NONE',  ( 1.000000000000000000, 0.000000000000000000, 0.000000000000000000 ) ) ;
#62883=B_SPLINE_CURVE_WITH_KNOTS ( 'NONE', 3,
 ( #3977, #39126, #85086, #4895, #16609, #50824, #23366, #51253, #44072, #31008 ),
 .UNSPECIFIED., .F., .F.,
 ( 4, 2, 2, 2, 4 ),
 ( 0.0007817246256747473893, 0.0009771112852218909357, 0.001172497944769034482, 0.001367884604316178246, 0.001563271263863321792 ),
 .UNSPECIFIED. ) ;
#62885=CARTESIAN_POINT ( 'NONE',  ( 17.29970274590113632, -11.60474049983370648, 33.02348890104160262 ) ) ;
#62886=ORIENTED_EDGE ( 'NONE', *, *, #85621, .T. ) ;
#62887=B_SPLINE_CURVE_WITH_KNOTS ( 'NONE', 3,
 ( #39456, #65562, #66912, #53388, #5207, #17842, #38552, #37653, #52050, #65113 ),
 .UNSPECIFIED., .F., .F.,
 ( 4, 2, 2, 2, 4 ),
 ( 0.0007817246256747453293, 0.0009771112852218889842, 0.001172497944769032531, 0.001367884604316176294, 0.001563271263863319840 ),
 .UNSPECIFIED. ) ;
#62889=EDGE_CURVE ( 'NONE', #60384, #22892, #4471, .T. ) ;
#62890=ORIENTED_EDGE ( 'NONE', *, *, #66072, .T. ) ;
#62891=CARTESIAN_POINT ( 'NONE',  ( 13.31853300525525086, -4.661471528628507777, 34.16647553114621871 ) ) ;
#62892=ORIENTED_EDGE ( 'NONE', *, *, #37619, .T. ) ;
#62893=LINE ( 'NONE', #7084, #15732 ) ;
#62894=CARTESIAN_POINT ( 'NONE',  ( 6.066067333350076751, -2.486705287966279876, 31.30864560766543647 ) ) ;
#62895=ADVANCED_FACE ( 'NONE', ( #63058 ), #15338, .F. ) ;
#62896=AXIS2_PLACEMENT_3D ( 'NONE', #28363, #13525, #88768 ) ;
#62897=CARTESIAN_POINT ( 'NONE',  ( -9.822999158975251888, -8.147922237126337563, 34.70805685702651999 ) ) ;
#62898=CARTESIAN_POINT ( 'NONE',  ( 10.61538461538461675, -13.20930481340135110, 34.54067556320372745 ) ) ;
#62899=ORIENTED_EDGE ( 'NONE', *, *, #85997, .F. ) ;
#62900=VERTEX_POINT ( 'NONE', #56754 ) ;
#62902=CARTESIAN_POINT ( 'NONE',  ( -14.55769230769230305, -7.566083408709835645, 34.74999999999999289 ) ) ;
#62903=CARTESIAN_POINT ( 'NONE',  ( 11.60371667797437567, -5.941354392334607049, 34.76329471203374055 ) ) ;
#62904=ORIENTED_EDGE ( 'NONE', *, *, #3108, .T. ) ;
#62905=CARTESIAN_POINT ( 'NONE',  ( -6.988347369037698265, -12.46129190929999986, 30.37095296980880832 ) ) ;
#62906=CARTESIAN_POINT ( 'NONE',  ( -11.28851612908349722, -12.68172785388650681, 30.59649109432439218 ) ) ;
#62907=CARTESIAN_POINT ( 'NONE',  ( 7.145856464345331283, -11.89424750095246175, 32.13594075562311758 ) ) ;
#62908=ADVANCED_FACE ( 'NONE', ( #34270 ), #82913, .F. ) ;
#62909=VERTEX_POINT ( 'NONE', #63508 ) ;
#62910=EDGE_CURVE ( 'NONE', #68389, #72129, #13086, .T. ) ;
#62911=CARTESIAN_POINT ( 'NONE',  ( 9.692307692307695177, -1.951392089020283160, 34.73218667398347748 ) ) ;
#62913=ORIENTED_EDGE ( 'NONE', *, *, #33870, .F. ) ;
#62914=FACE_BOUND ( 'NONE', #61576, .T. ) ;
#62916=CARTESIAN_POINT ( 'NONE',  ( 13.51540582558234149, -6.369690395747422684, 34.87708834333098196 ) ) ;
#62917=CARTESIAN_POINT ( 'NONE',  ( -23.00000000000000000, -9.499999999999982236, 27.74999999999999645 ) ) ;
#62918=B_SPLINE_CURVE_WITH_KNOTS ( 'NONE', 3,
 ( #34082, #74187, #33645, #27329, #18802, #39083, #66544, #25996, #39532, #4844 ),
 .UNSPECIFIED., .F., .F.,
 ( 4, 2, 2, 2, 4 ),
 ( 0.0007817359430256319575, 0.0009771253907249984917, 0.001172514838424365026, 0.001367904286123731343, 0.001563293733823097878 ),
 .UNSPECIFIED. ) ;
#62919=LINE ( 'NONE', #8446, #61876 ) ;
#62920=LINE ( 'NONE', #1233, #2323 ) ;
#62921=EDGE_CURVE ( 'NONE', #59502, #79391, #47531, .T. ) ;
#62923=CARTESIAN_POINT ( 'NONE',  ( 4.153846153846154188, -1.466349020453238561, 30.81389545987213907 ) ) ;
#62924=VERTEX_POINT ( 'NONE', #55427 ) ;
#62925=ADVANCED_FACE ( 'NONE', ( #21196 ), #48664, .F. ) ;
#62926=CARTESIAN_POINT ( 'NONE',  ( 14.37376065869474751, -12.37446782046654192, 30.86335684631486842 ) ) ;
#62927=CARTESIAN_POINT ( 'NONE',  ( -6.130147969731695845, -11.66186481527757479, 32.95055677023626117 ) ) ;
#62928=VERTEX_POINT ( 'NONE', #930 ) ;
#62930=CARTESIAN_POINT ( 'NONE',  ( -18.00000000000000000, -1.459774944578025924, 30.56119799385072611 ) ) ;
#62931=EDGE_LOOP ( 'NONE', ( #80115, #36141 ) ) ;
#62932=CARTESIAN_POINT ( 'NONE',  ( -13.25408994638174320, -11.66157788607254098, 32.95092075102925833 ) ) ;
#62933=CARTESIAN_POINT ( 'NONE',  ( 4.403791672194294016, -10.05730279482229683, 34.04704008940765902 ) ) ;
#62934=FACE_BOUND ( 'NONE', #3585, .T. ) ;
#62936=CARTESIAN_POINT ( 'NONE',  ( -16.85391172531022619, -12.39991518177334129, 30.74647679643404530 ) ) ;
#62937=CARTESIAN_POINT ( 'NONE',  ( 1.634669804528839476, -12.65882529074907126, 30.72640787790839312 ) ) ;
#62938=CARTESIAN_POINT ( 'NONE',  ( -2.980823712421087013, -11.86320923018887719, 32.19269448109604781 ) ) ;
#62939=CARTESIAN_POINT ( 'NONE',  ( 7.173022441425065843, -12.43552623307873972, 30.55307653245132826 ) ) ;
#62943=ORIENTED_EDGE ( 'NONE', *, *, #47824, .F. ) ;
#62944=VERTEX_POINT ( 'NONE', #28398 ) ;
#62945=CARTESIAN_POINT ( 'NONE',  ( -9.942284436356281674, -2.318417181685855422, 30.59732222474233865 ) ) ;
#62946=CARTESIAN_POINT ( 'NONE',  ( -10.39260494640654642, -8.540255544307065350, 34.89611431652622286 ) ) ;
#62947=CARTESIAN_POINT ( 'NONE',  ( 14.43848274865925774, -9.084667340241226796, 34.75534355489798344 ) ) ;
#62948=CARTESIAN_POINT ( 'NONE',  ( -8.834500769787091201, -8.656820664281498878, 34.87096338111211935 ) ) ;
#62951=CARTESIAN_POINT ( 'NONE',  ( 0.4615384615384611200, -3.937682226553329556, 33.60647404775216529 ) ) ;
#62952=LINE ( 'NONE', #63409, #34541 ) ;
#62953=DIRECTION ( 'NONE',  ( -0.000000000000000000, -0.6427876096865404731, -0.7660444431189771253 ) ) ;
#62954=CARTESIAN_POINT ( 'NONE',  ( 17.93472999944368240, -8.656820664281497102, 34.87096338111211935 ) ) ;
#62956=CARTESIAN_POINT ( 'NONE',  ( 18.22277954126840172, -10.11255958852955672, 34.01340905677048454 ) ) ;
#62957=CARTESIAN_POINT ( 'NONE',  ( 6.000000000000001776, -2.708943851104267164, 35.45975837776705220 ) ) ;
#62958=EDGE_CURVE ( 'NONE', #11362, #49139, #55869, .T. ) ;
#62959=CARTESIAN_POINT ( 'NONE',  ( 15.23076923076923173, -3.937682226553329556, 33.60647404775216529 ) ) ;
#62960=CARTESIAN_POINT ( 'NONE',  ( 11.53846153846153832, -10.67929555188718282, 33.92786785259544047 ) ) ;
#62961=B_SPLINE_CURVE_WITH_KNOTS ( 'NONE', 3,
 ( #74250, #12549, #44977, #65692, #3991, #31479, #24723, #52181, #61662, #88728 ),
 .UNSPECIFIED., .F., .F.,
 ( 4, 2, 2, 2, 4 ),
 ( 0.0007817359430256392216, 0.0009771253907250082495, 0.001172514838424377169, 0.001367904286123746305, 0.001563293733823115225 ),
 .UNSPECIFIED. ) ;
#62962=EDGE_LOOP ( 'NONE', ( #37643, #39425, #77263, #24242 ) ) ;
#62963=ADVANCED_FACE ( 'NONE', ( #49114 ), #78794, .F. ) ;
#62964=B_SPLINE_CURVE_WITH_KNOTS ( 'NONE', 3,
 ( #55512, #50519, #29390, #69474, #69916, #36580, #14982, #1018, #50078, #83894 ),
 .UNSPECIFIED., .F., .F.,
 ( 4, 2, 2, 2, 4 ),
 ( 0.000000000000000000, 0.0001954339857564065528, 0.0003908679715128131056, 0.0005863019572692196313, 0.0007817359430256262112 ),
 .UNSPECIFIED. ) ;
#62965=CARTESIAN_POINT ( 'NONE',  ( 2.057669083470853089, -3.520140089381496473, 33.17453946501458262 ) ) ;
#62966=CARTESIAN_POINT ( 'NONE',  ( 18.25000000000000000, -2.499999999999998668, 29.75000000000000355 ) ) ;
#62969=CYLINDRICAL_SURFACE ( 'NONE', #5874, 0.2499999999999998890 ) ;
#62971=ORIENTED_EDGE ( 'NONE', *, *, #24561, .T. ) ;
#62973=CARTESIAN_POINT ( 'NONE',  ( -9.442362173959551797, -5.057305518903948638, 34.11320923018887896 ) ) ;
#62974=VERTEX_POINT ( 'NONE', #72036 ) ;
#62975=CARTESIAN_POINT ( 'NONE',  ( 9.561747100565771262, -2.504760397472875155, 29.97295953869789997 ) ) ;
#62976=CARTESIAN_POINT ( 'NONE',  ( 12.46153846153846168, -5.471508081941601098, 34.59228464037088457 ) ) ;
#62977=ORIENTED_EDGE ( 'NONE', *, *, #17742, .T. ) ;
#62978=CARTESIAN_POINT ( 'NONE',  ( -5.207614543590632472, -11.18331474514187995, 33.13161551792790505 ) ) ;
#62979=EDGE_CURVE ( 'NONE', #60060, #23103, #77532, .T. ) ;
#62980=CARTESIAN_POINT ( 'NONE',  ( 13.16113046005105858, -9.417330523894424488, 34.63758898049880486 ) ) ;
#62981=VERTEX_POINT ( 'NONE', #3575 ) ;
#62982=CARTESIAN_POINT ( 'NONE',  ( 7.846153846153846700, -5.180354513474913603, 36.12317359536750416 ) ) ;
#62983=DIRECTION ( 'NONE',  ( 0.000000000000000000, 1.000000000000000000, 0.000000000000000000 ) ) ;
#62984=AXIS2_PLACEMENT_3D ( 'NONE', #74416, #73981, #26229 ) ;
#62985=CARTESIAN_POINT ( 'NONE',  ( -9.692307692307384315, -2.506253911140614576, 30.00000000000323297 ) ) ;
#62986=ORIENTED_EDGE ( 'NONE', *, *, #27373, .T. ) ;
#62987=EDGE_LOOP ( 'NONE', ( #5665, #88054, #7333, #73097 ) ) ;
#62988=CARTESIAN_POINT ( 'NONE',  ( -10.39260494640654819, -2.353885683473779800, 30.79025554430704403 ) ) ;
#62989=ORIENTED_EDGE ( 'NONE', *, *, #1872, .F. ) ;
#62990=ADVANCED_FACE ( 'NONE', ( #65279 ), #2241, .F. ) ;
#62991=CARTESIAN_POINT ( 'NONE',  ( 5.207713517890025123, -4.684288915650984819, 34.18129842949671371 ) ) ;
#62995=CARTESIAN_POINT ( 'NONE',  ( 1.134592160393928628, -2.341070481393820124, 30.72580821765574299 ) ) ;
#62996=CARTESIAN_POINT ( 'NONE',  ( 3.230769230769108269, -10.33852847137269571, 34.16647553114546554 ) ) ;
#62997=VERTEX_POINT ( 'NONE', #58078 ) ;
#62998=EDGE_LOOP ( 'NONE', ( #61895, #44607 ) ) ;
#62999=CARTESIAN_POINT ( 'NONE',  ( -1.254567778359700680, -7.723484964179500700, 34.74522123443823318 ) ) ;
#63000=ORIENTED_EDGE ( 'NONE', *, *, #51046, .F. ) ;
#63002=CARTESIAN_POINT ( 'NONE',  ( 16.85343815235874132, -2.353723527008297012, 30.78948104536958752 ) ) ;
#63003=VERTEX_POINT ( 'NONE', #36920 ) ;
#63004=AXIS2_PLACEMENT_3D ( 'NONE', #46837, #68438, #61226 ) ;
#63005=CYLINDRICAL_SURFACE ( 'NONE', #82412, 0.2499999999999993616 ) ;
#63006=CARTESIAN_POINT ( 'NONE',  ( 5.076923076923075762, -3.513871655860378418, 32.76840700105978499 ) ) ;
#63007=ORIENTED_EDGE ( 'NONE', *, *, #2822, .F. ) ;
#63008=CARTESIAN_POINT ( 'NONE',  ( 7.911409417429871027, -8.613356846314928816, 34.62446782046653482 ) ) ;
#63009=VERTEX_POINT ( 'NONE', #86471 ) ;
#63010=CARTESIAN_POINT ( 'NONE',  ( -14.30769230769242917, -5.094484230521993062, 34.41647553114689373 ) ) ;
#63011=ORIENTED_EDGE ( 'NONE', *, *, #11939, .F. ) ;
#63012=CYLINDRICAL_SURFACE ( 'NONE', #64645, 0.2499999999999973355 ) ;
#63013=B_SPLINE_CURVE_WITH_KNOTS ( 'NONE', 3,
 ( #88246, #74264, #81029, #4921, #67063, #25180, #40048, #53532, #60739, #12125 ),
 .UNSPECIFIED., .F., .F.,
 ( 4, 2, 2, 2, 4 ),
 ( 0.000000000000000000, 0.0001954311564186871184, 0.0003908623128373742367, 0.0005862934692560614093, 0.0007817246256747484735 ),
 .UNSPECIFIED. ) ;
#63014=B_SPLINE_CURVE_WITH_KNOTS ( 'NONE', 3,
 ( #28695, #84531, #62897, #1211, #8423, #49836, #1661, #82759, #48957, #56604 ),
 .UNSPECIFIED., .F., .F.,
 ( 4, 2, 2, 2, 4 ),
 ( 0.000000000000000000, 0.0001954339857564078809, 0.0003908679715128157619, 0.0005863019572692236428, 0.0007817359430256315238 ),
 .UNSPECIFIED. ) ;
#63015=EDGE_CURVE ( 'NONE', #65460, #86922, #31169, .T. ) ;
#63017=ADVANCED_FACE ( 'NONE', ( #63946 ), #9025, .F. ) ;
#63018=CARTESIAN_POINT ( 'NONE',  ( 6.923076923076924238, -13.95598074871891292, 31.83374038241031911 ) ) ;
#63019=LINE ( 'NONE', #70685, #61228 ) ;
#63020=FACE_BOUND ( 'NONE', #38919, .T. ) ;
#63022=CARTESIAN_POINT ( 'NONE',  ( -11.78848476268299628, -6.652501968072648708, 34.93155406624980941 ) ) ;
#63024=CARTESIAN_POINT ( 'NONE',  ( 9.469380733400845074, -2.308479472611653094, 30.53278059502174457 ) ) ;
#63025=CARTESIAN_POINT ( 'NONE',  ( -0.2115930521604183767, -2.986452184633680229, 32.43230066228893804 ) ) ;
#63026=AXIS2_PLACEMENT_3D ( 'NONE', #51870, #38834, #78916 ) ;
#63027=CARTESIAN_POINT ( 'NONE',  ( -3.007757879156382153, -3.105924265160262543, 32.13625925475356127 ) ) ;
#63028=CARTESIAN_POINT ( 'NONE',  ( -16.40382288478850725, -8.303909089506435137, 34.68538101551103381 ) ) ;
#63029=EDGE_LOOP ( 'NONE', ( #51235, #27954, #57758, #64553 ) ) ;
#63030=EDGE_CURVE ( 'NONE', #52057, #62177, #41005, .T. ) ;
#63031=CARTESIAN_POINT ( 'NONE',  ( -14.30769230769230660, -13.20930481340135110, 34.54067556320372745 ) ) ;
#63033=ORIENTED_EDGE ( 'NONE', *, *, #38191, .T. ) ;
#63035=FACE_OUTER_BOUND ( 'NONE', #18383, .T. ) ;
#63036=CARTESIAN_POINT ( 'NONE',  ( 15.23076923076911093, -12.27809138561165270, 31.22303859784587132 ) ) ;
#63037=VECTOR ( 'NONE', #18456, 1000.000000000000114 ) ;
#63038=CYLINDRICAL_SURFACE ( 'NONE', #74408, 0.2500000000000004996 ) ;
#63039=CARTESIAN_POINT ( 'NONE',  ( -10.61538461538461320, -11.69971097300155272, 32.46337939537588113 ) ) ;
#63040=CARTESIAN_POINT ( 'NONE',  ( 1.607395053593450918, -10.97394488606064122, 33.68653795673694873 ) ) ;
#63041=CARTESIAN_POINT ( 'NONE',  ( 9.692307692307572609, -2.625532179533778709, 30.86335684631627174 ) ) ;
#63043=CARTESIAN_POINT ( 'NONE',  ( -18.25002323729296450, -5.851115903089110226, 34.47074536777953568 ) ) ;
#63044=AXIS2_PLACEMENT_3D ( 'NONE', #81636, #40653, #13173 ) ;
#63045=CARTESIAN_POINT ( 'NONE',  ( -14.37296230824862775, -10.33852847137145048, 34.16647553114627556 ) ) ;
#63046=CARTESIAN_POINT ( 'NONE',  ( -12.71156168575992318, -11.56360843649121684, 33.07473185843129926 ) ) ;
#63047=CARTESIAN_POINT ( 'NONE',  ( -8.703975629717932705, -2.657715359629131857, 31.77849191805844242 ) ) ;
#63048=FACE_OUTER_BOUND ( 'NONE', #56980, .T. ) ;
#63050=EDGE_CURVE ( 'NONE', #78447, #40455, #2390, .T. ) ;
#63051=DIRECTION ( 'NONE',  ( -0.000000000000000000, 0.9396926207859093161, -0.3420201433256663259 ) ) ;
#63053=EDGE_LOOP ( 'NONE', ( #43734, #29493 ) ) ;
#63054=CARTESIAN_POINT ( 'NONE',  ( -5.999999999999998224, -3.937682226553329556, 33.60647404775216529 ) ) ;
#63055=EDGE_CURVE ( 'NONE', #28342, #10726, #79774, .T. ) ;
#63056=ORIENTED_EDGE ( 'NONE', *, *, #47736, .T. ) ;
#63057=B_SPLINE_CURVE_WITH_KNOTS ( 'NONE', 3,
 ( #17532, #16195, #31026, #3558, #50840, #30585, #9875, #78776, #10771, #72462 ),
 .UNSPECIFIED., .F., .F.,
 ( 4, 2, 2, 2, 4 ),
 ( 0.000000000000000000, 0.0001954339857564054686, 0.0003908679715128109372, 0.0005863019572692163787, 0.0007817359430256218744 ),
 .UNSPECIFIED. ) ;
#63058=FACE_OUTER_BOUND ( 'NONE', #22451, .T. ) ;
#63060=DIRECTION ( 'NONE',  ( -0.000000000000000000, -0.3420201433256694901, -0.9396926207859082059 ) ) ;
#63061=CARTESIAN_POINT ( 'NONE',  ( 7.846153846153723244, -6.835583212225970762, 34.95778746994575670 ) ) ;
#63062=DIRECTION ( 'NONE',  ( 0.000000000000000000, -6.938893903907222067E-15, 1.000000000000000000 ) ) ;
#63063=B_SPLINE_CURVE_WITH_KNOTS ( 'NONE', 3,
 ( #57032, #42650, #16940, #15618, #8864, #44390, #71877, #3417, #85848, #23247 ),
 .UNSPECIFIED., .F., .F.,
 ( 4, 2, 2, 2, 4 ),
 ( 0.0007817359430256323911, 0.0009771253907249991422, 0.001172514838424365893, 0.001367904286123732644, 0.001563293733823099396 ),
 .UNSPECIFIED. ) ;
#63064=CARTESIAN_POINT ( 'NONE',  ( 0.7115928814519135726, -9.233818618650603938, 34.70587769442853698 ) ) ;
#63066=CARTESIAN_POINT ( 'NONE',  ( 5.999999999999880096, -12.46129190930018460, 30.37095296980731973 ) ) ;
#63067=CARTESIAN_POINT ( 'NONE',  ( -13.38461538461550582, -4.481592998941358097, 33.73612834414048933 ) ) ;
#63068=EDGE_LOOP ( 'NONE', ( #37335, #28000, #31262, #2812 ) ) ;
#63069=CARTESIAN_POINT ( 'NONE',  ( -5.076923076922769340, -2.506253911140614576, 30.00000000000323297 ) ) ;
#63070=CARTESIAN_POINT ( 'NONE',  ( -5.076923076923075762, -13.95598074871891292, 31.83374038241031911 ) ) ;
#63071=CARTESIAN_POINT ( 'NONE',  ( 17.01165263096229907, -3.835265460703609186, 33.15142922261924241 ) ) ;
#63072=CARTESIAN_POINT ( 'NONE',  ( 15.48071464014727461, -2.986452184633680673, 32.43230066228895225 ) ) ;
#63073=EDGE_CURVE ( 'NONE', #83315, #72489, #33291, .T. ) ;
#63074=CARTESIAN_POINT ( 'NONE',  ( -2.242437168179467033, -2.379036618887895305, 30.90682066428159303 ) ) ;
#63075=LINE ( 'NONE', #28877, #68003 ) ;
#63076=DIRECTION ( 'NONE',  ( -0.000000000000000000, 1.000000000000000000, 3.491481338843133355E-15 ) ) ;
#63078=ORIENTED_EDGE ( 'NONE', *, *, #49611, .T. ) ;
#63080=ADVANCED_FACE ( 'NONE', ( #81039 ), #4477, .F. ) ;
#63081=CARTESIAN_POINT ( 'NONE',  ( -16.82697755857493505, -10.76462480002816413, 33.53768742498949962 ) ) ;
#63082=CARTESIAN_POINT ( 'NONE',  ( -17.14219307747939069, -5.094484230520675894, 34.41647553114621161 ) ) ;
#63083=CARTESIAN_POINT ( 'NONE',  ( 7.976945653978632755, -2.541949514083463590, 30.39797389878540557 ) ) ;
#63084=CARTESIAN_POINT ( 'NONE',  ( -7.715363405186889345, -2.845873456487966635, 32.17976146951973249 ) ) ;
#63087=CARTESIAN_POINT ( 'NONE',  ( -5.207070286361298095, -6.852621066184267029, 34.70813303252209181 ) ) ;
#63088=DIRECTION ( 'NONE',  ( -0.000000000000000000, -0.9396926207859092051, -0.3420201433256662704 ) ) ;
#63089=EDGE_CURVE ( 'NONE', #31532, #8324, #67984, .T. ) ;
#63090=CARTESIAN_POINT ( 'NONE',  ( -9.692307692307691624, -12.78798330534102767, 29.49999999999997868 ) ) ;
#63091=ORIENTED_EDGE ( 'NONE', *, *, #41668, .F. ) ;
#63092=CARTESIAN_POINT ( 'NONE',  ( -23.00000000000000000, -5.499999999999981348, 27.75000000000000000 ) ) ;
#63093=CARTESIAN_POINT ( 'NONE',  ( -5.999999999999690914, -2.506253911140614576, 30.00000000000323297 ) ) ;
#63094=EDGE_CURVE ( 'NONE', #26115, #28684, #57112, .T. ) ;
#63095=CARTESIAN_POINT ( 'NONE',  ( 3.230769230769231726, -2.249999999999998668, 29.75000000000001776 ) ) ;
#63096=DIRECTION ( 'NONE',  ( -0.000000000000000000, 0.8660254037844397068, -0.4999999999999978906 ) ) ;
#63097=B_SPLINE_CURVE_WITH_KNOTS ( 'NONE', 3,
 ( #50084, #20845, #48314, #14988, #14094, #22185, #69922, #49651, #75787, #62708 ),
 .UNSPECIFIED., .F., .F.,
 ( 4, 2, 2, 2, 4 ),
 ( 0.0007817359430256294638, 0.0009771253907249952391, 0.001172514838424361123, 0.001367904286123726790, 0.001563293733823092673 ),
 .UNSPECIFIED. ) ;
#63099=CARTESIAN_POINT ( 'NONE',  ( -6.700064078983528404, -6.460100341425561332, 34.89618726649961644 ) ) ;
#63100=ORIENTED_EDGE ( 'NONE', *, *, #17584, .F. ) ;
#63101=B_SPLINE_CURVE_WITH_KNOTS ( 'NONE', 3,
 ( #74748, #67097, #54454, #5399, #87840, #13037, #75189, #19350, #13477, #6716 ),
 .UNSPECIFIED., .F., .F.,
 ( 4, 2, 2, 2, 4 ),
 ( 0.0007817246256747484735, 0.0009771112852218922368, 0.001172497944769036217, 0.001367884604316180197, 0.001563271263863323960 ),
 .UNSPECIFIED. ) ;
#63102=VECTOR ( 'NONE', #3693, 1000.000000000000227 ) ;
#63103=CARTESIAN_POINT ( 'NONE',  ( 1.384615384615386802, -12.34228464037088635, 31.77849191805839268 ) ) ;
#63104=CARTESIAN_POINT ( 'NONE',  ( -4.023007735833388665, -7.277220443632450575, 34.74524770363009196 ) ) ;
#63105=ORIENTED_EDGE ( 'NONE', *, *, #82408, .T. ) ;
#63106=CYLINDRICAL_SURFACE ( 'NONE', #80721, 0.2500000000000009437 ) ;
#63107=CARTESIAN_POINT ( 'NONE',  ( 4.153846153846030731, -9.528491918059723176, 34.59228464037033035 ) ) ;
#63108=EDGE_CURVE ( 'NONE', #36685, #10416, #65714, .T. ) ;
#63109=CARTESIAN_POINT ( 'NONE',  ( -11.53846153846165912, -6.879047030192662504, 34.71129190930017927 ) ) ;
#63110=AXIS2_PLACEMENT_3D ( 'NONE', #4769, #66463, #71876 ) ;
#63111=EDGE_CURVE ( 'NONE', #18498, #56760, #25190, .T. ) ;
#63112=VECTOR ( 'NONE', #78158, 1000.000000000000114 ) ;
#63113=DIRECTION ( 'NONE',  ( -0.000000000000000000, -0.1736481776669307198, -0.9848077530122080203 ) ) ;
#63114=CARTESIAN_POINT ( 'NONE',  ( 3.230769230769231726, -12.37446782046654192, 30.86335684631486131 ) ) ;
#63115=ORIENTED_EDGE ( 'NONE', *, *, #5799, .T. ) ;
#63116=ORIENTED_EDGE ( 'NONE', *, *, #34999, .T. ) ;
#63117=FACE_BOUND ( 'NONE', #36344, .T. ) ;
#63118=EDGE_LOOP ( 'NONE', ( #59714, #54594, #25432, #88793 ) ) ;
#63119=CARTESIAN_POINT ( 'NONE',  ( 15.16549878480845770, -12.46129190929999986, 30.37095296980880832 ) ) ;
#63120=CARTESIAN_POINT ( 'NONE',  ( 6.673076923076925127, -2.249999999999998668, 29.75000000000000355 ) ) ;
#63121=CARTESIAN_POINT ( 'NONE',  ( 6.223012844093399387, -2.889357225399416862, 32.26129605718031002 ) ) ;
#63122=CARTESIAN_POINT ( 'NONE',  ( -17.07692307692307665, -2.833524468853757305, 32.15551576947925838 ) ) ;
#63125=ORIENTED_EDGE ( 'NONE', *, *, #15856, .F. ) ;
#63126=CARTESIAN_POINT ( 'NONE',  ( 13.16173670218674374, -7.630691491037285168, 34.74850469731152458 ) ) ;
#63127=ORIENTED_EDGE ( 'NONE', *, *, #79220, .F. ) ;
#63128=B_SPLINE_CURVE_WITH_KNOTS ( 'NONE', 3,
 ( #32200, #32631, #60101, #67755, #26765, #82616, #12806, #60990, #20455, #55119 ),
 .UNSPECIFIED., .F., .F.,
 ( 4, 2, 2, 2, 4 ),
 ( 0.0007817246336856289524, 0.0009771112958940101571, 0.001172497958102391253, 0.001367884620310772350, 0.001563271282519153446 ),
 .UNSPECIFIED. ) ;
#63129=CARTESIAN_POINT ( 'NONE',  ( 13.16113044089144068, -2.847400154188068022, 31.58180166144859058 ) ) ;
#63130=AXIS2_PLACEMENT_3D ( 'NONE', #2336, #63604, #36586 ) ;
#63131=CARTESIAN_POINT ( 'NONE',  ( 16.94677510719138169, -3.625366637846545448, 33.29286588640298561 ) ) ;
#63132=B_SPLINE_CURVE_WITH_KNOTS ( 'NONE', 3,
 ( #31085, #58555, #86048, #24325, #51787, #59008 ),
 .UNSPECIFIED., .F., .F.,
 ( 4, 2, 4 ),
 ( 4.224605973302673136E-17, 0.0001954756301637175888, 0.0003909512603273928937 ),
 .UNSPECIFIED. ) ;
#63133=CARTESIAN_POINT ( 'NONE',  ( -18.25002322422145440, -6.652501968072647820, 34.93155406624980941 ) ) ;
#63134=ORIENTED_EDGE ( 'NONE', *, *, #61243, .F. ) ;
#63135=CARTESIAN_POINT ( 'NONE',  ( 9.019285080869083870, -9.148310452688876993, 34.47095581063188519 ) ) ;
#63136=EDGE_CURVE ( 'NONE', #27202, #53025, #9892, .T. ) ;
#63137=CARTESIAN_POINT ( 'NONE',  ( -15.09997878980228059, -3.338503747796866872, 32.95102852606553512 ) ) ;
#63139=CARTESIAN_POINT ( 'NONE',  ( -11.60373198442231590, -3.300289026998414865, 32.46337939537583139 ) ) ;
#63141=ADVANCED_FACE ( 'NONE', ( #5371 ), #87813, .F. ) ;
#63142=B_SPLINE_CURVE_WITH_KNOTS ( 'NONE', 3,
 ( #10595, #3380, #31758, #16899, #64626, #23651, #45253, #17345, #11038, #72726 ),
 .UNSPECIFIED., .F., .F.,
 ( 4, 2, 2, 2, 4 ),
 ( 0.000000000000000000, 0.0001954311564186864407, 0.0003908623128373728815, 0.0005862934692560593493, 0.0007817246256747457630 ),
 .UNSPECIFIED. ) ;
#63143=ORIENTED_EDGE ( 'NONE', *, *, #58507, .T. ) ;
#63144=ORIENTED_EDGE ( 'NONE', *, *, #38418, .T. ) ;
#63146=CARTESIAN_POINT ( 'NONE',  ( -7.846153846153844924, -6.386643153685126251, 34.62446782046654192 ) ) ;
#63147=CARTESIAN_POINT ( 'NONE',  ( 10.61538461538449418, -2.379036618888197729, 30.90682066428292885 ) ) ;
#63148=EDGE_CURVE ( 'NONE', #77307, #72978, #82967, .T. ) ;
#63149=LINE ( 'NONE', #51380, #26958 ) ;
#63150=CARTESIAN_POINT ( 'NONE',  ( 12.68455130563185662, -12.64618726649961289, 30.78989965857442712 ) ) ;
#63151=FACE_BOUND ( 'NONE', #78836, .T. ) ;
#63152=CARTESIAN_POINT ( 'NONE',  ( 8.519254025182180001, -10.82459398097509329, 33.81372124010185587 ) ) ;
#63153=EDGE_LOOP ( 'NONE', ( #22190, #22838 ) ) ;
#63155=CARTESIAN_POINT ( 'NONE',  ( 9.692307692307695177, -8.120952969808772792, 34.71129190930000163 ) ) ;
#63157=DIRECTION ( 'NONE',  ( -0.000000000000000000, -0.1736481776669307198, -0.9848077530122080203 ) ) ;
#63158=ORIENTED_EDGE ( 'NONE', *, *, #64025, .T. ) ;
#63160=CARTESIAN_POINT ( 'NONE',  ( 6.065255139512840898, -11.06231777344671130, 33.60647404775212976 ) ) ;
#63161=B_SPLINE_CURVE_WITH_KNOTS ( 'NONE', 3,
 ( #75366, #67280, #67722, #26729, #5575, #68601, #74041, #69048, #146, #88027 ),
 .UNSPECIFIED., .F., .F.,
 ( 4, 2, 2, 2, 4 ),
 ( 0.0007817359527651090859, 0.0009771254036996478414, 0.001172514854634186489, 0.001367904305568725136, 0.001563293756503263783 ),
 .UNSPECIFIED. ) ;
#63162=ORIENTED_EDGE ( 'NONE', *, *, #85858, .F. ) ;
#63163=FACE_BOUND ( 'NONE', #76301, .T. ) ;
#63165=EDGE_CURVE ( 'NONE', #64018, #88485, #45290, .T. ) ;
#63166=CARTESIAN_POINT ( 'NONE',  ( -7.053224892808618307, -10.31621877034669588, 34.18098118002070152 ) ) ;
#63167=CARTESIAN_POINT ( 'NONE',  ( 12.46153846153846168, -5.557115091759785130, 34.35708131394839171 ) ) ;
#63168=VERTEX_POINT ( 'NONE', #28288 ) ;
#63169=CARTESIAN_POINT ( 'NONE',  ( -14.43838377435986864, -12.38065189839062263, 30.83690757178629482 ) ) ;
#63170=CARTESIAN_POINT ( 'NONE',  ( -6.000000000000121680, -9.528491918059723176, 34.59228464037033035 ) ) ;
#63171=CYLINDRICAL_SURFACE ( 'NONE', #61012, 0.2500000000000009437 ) ;
#63173=ORIENTED_EDGE ( 'NONE', *, *, #22544, .F. ) ;
#63177=ORIENTED_EDGE ( 'NONE', *, *, #55257, .T. ) ;
#63179=CARTESIAN_POINT ( 'NONE',  ( 4.153846153846030731, -3.083524468854526912, 32.58852847137268327 ) ) ;
#63180=VERTEX_POINT ( 'NONE', #62508 ) ;
#63181=CARTESIAN_POINT ( 'NONE',  ( 11.60371710973756620, -6.879047030191282275, 34.71129190930002295 ) ) ;
#63182=CARTESIAN_POINT ( 'NONE',  ( -13.38461538461538325, -4.786620604624113540, 33.94971097300155094 ) ) ;
#63183=DIRECTION ( 'NONE',  ( 0.000000000000000000, 0.8660254037844377084, 0.5000000000000015543 ) ) ;
#63184=CARTESIAN_POINT ( 'NONE',  ( -12.46153846153858424, -11.06231777344772027, 33.60647404775119895 ) ) ;
#63185=CARTESIAN_POINT ( 'NONE',  ( -8.096177083446809419, -10.76384336483936011, 33.53834819971076087 ) ) ;
#63186=CARTESIAN_POINT ( 'NONE',  ( -11.53846153846166089, -9.528491918059723176, 34.59228464037033035 ) ) ;
#63187=CARTESIAN_POINT ( 'NONE',  ( 7.846153846153846700, -4.098570777380720287, 33.41473453929634729 ) ) ;
#63189=ORIENTED_EDGE ( 'NONE', *, *, #67981, .T. ) ;
#63190=ADVANCED_FACE ( 'NONE', ( #35947 ), #40930, .F. ) ;
#63191=CARTESIAN_POINT ( 'NONE',  ( -16.28399412357785536, -5.070767119584671079, 34.40440758774516183 ) ) ;
#63192=VERTEX_POINT ( 'NONE', #20650 ) ;
#63193=ORIENTED_EDGE ( 'NONE', *, *, #44843, .F. ) ;
#63194=EDGE_CURVE ( 'NONE', #60729, #74862, #19624, .T. ) ;
#63195=CARTESIAN_POINT ( 'NONE',  ( -16.21992853320628925, -9.058645607665454236, 34.76329471203372634 ) ) ;
#63196=ORIENTED_EDGE ( 'NONE', *, *, #84001, .T. ) ;
#63197=CARTESIAN_POINT ( 'NONE',  ( 10.83839745947800992, -8.282913670948747864, 34.94150082978203642 ) ) ;
#63198=CARTESIAN_POINT ( 'NONE',  ( 6.065255571276024327, -3.300289026998475705, 32.46337939537591666 ) ) ;
#63199=CARTESIAN_POINT ( 'NONE',  ( -11.78843826940389583, -11.28823185664190376, 33.01397839955799896 ) ) ;
#63200=DIRECTION ( 'NONE',  ( 0.000000000000000000, 0.1736481776669275834, 0.9848077530122086864 ) ) ;
#63201=CARTESIAN_POINT ( 'NONE',  ( -10.61538461538461320, -3.322132147404559976, 32.92929555188717927 ) ) ;
#63202=CARTESIAN_POINT ( 'NONE',  ( 6.923076923076924238, -11.16473453929635440, 33.15142922261926373 ) ) ;
#63203=CARTESIAN_POINT ( 'NONE',  ( -15.23076923076935252, -8.656820664282941280, 34.87096338111179961 ) ) ;
#63204=FACE_OUTER_BOUND ( 'NONE', #20414, .T. ) ;
#63205=CARTESIAN_POINT ( 'NONE',  ( -2.084679463598908544, -2.889357225399416862, 32.26129605718031002 ) ) ;
#63206=EDGE_CURVE ( 'NONE', #72231, #41905, #75305, .T. ) ;
#63207=EDGE_CURVE ( 'NONE', #68579, #74314, #46267, .T. ) ;
#63208=CARTESIAN_POINT ( 'NONE',  ( 13.38461538461538680, -3.669653830205710676, 35.88435417666054406 ) ) ;
#63210=CARTESIAN_POINT ( 'NONE',  ( 9.692307692307695177, -2.249999999999998668, 29.50000000000001421 ) ) ;
#63211=EDGE_LOOP ( 'NONE', ( #70809, #57488 ) ) ;
#63213=CARTESIAN_POINT ( 'NONE',  ( 12.52760579488853665, -2.486705287966280320, 31.30864560766543647 ) ) ;
#63215=CARTESIAN_POINT ( 'NONE',  ( 3.480714640147274608, -10.92531984108285670, 33.72920026020278073 ) ) ;
#63216=CARTESIAN_POINT ( 'NONE',  ( 12.46153846153833911, -10.90142922262034020, 33.41473453929536674 ) ) ;
#63217=EDGE_LOOP ( 'NONE', ( #64462, #64059, #40221, #61920 ) ) ;
#63218=CARTESIAN_POINT ( 'NONE',  ( 6.066068351002440906, -4.786620604624113540, 33.94971097300155805 ) ) ;
#63220=CARTESIAN_POINT ( 'NONE',  ( -10.74607521849492109, -12.62707690430377383, 30.88035979386743435 ) ) ;
#63221=B_SPLINE_CURVE_WITH_KNOTS ( 'NONE', 3,
 ( #45224, #39383, #66393, #46567, #25409, #73616, #60073, #74051, #67290, #46998 ),
 .UNSPECIFIED., .F., .F.,
 ( 4, 2, 2, 2, 4 ),
 ( 0.0007817246256747528103, 0.0009771112852218980915, 0.001172497944769043156, 0.001367884604316188437, 0.001563271263863333718 ),
 .UNSPECIFIED. ) ;
#63222=CARTESIAN_POINT ( 'NONE',  ( -12.39628289026243557, -10.90142922261932057, 33.41473453929631887 ) ) ;
#63223=EDGE_CURVE ( 'NONE', #52323, #49979, #170, .T. ) ;
#63224=EDGE_CURVE ( 'NONE', #2856, #86167, #38770, .T. ) ;
#63225=ORIENTED_EDGE ( 'NONE', *, *, #36519, .F. ) ;
#63226=CARTESIAN_POINT ( 'NONE',  ( 18.06606733335007675, -3.322132147404559532, 32.92929555188717927 ) ) ;
#63227=ORIENTED_EDGE ( 'NONE', *, *, #41158, .T. ) ;
#63230=VECTOR ( 'NONE', #28170, 1000.000000000000114 ) ;
#63232=CARTESIAN_POINT ( 'NONE',  ( 15.36129466900288065, -3.625058011473228703, 33.29252011169590020 ) ) ;
#63233=CARTESIAN_POINT ( 'NONE',  ( -1.634638608836841200, -9.356822207818506598, 34.66110646841856635 ) ) ;
#63234=B_SPLINE_CURVE_WITH_KNOTS ( 'NONE', 3,
 ( #42558, #70913, #16405, #50175, #50628, #2008, #78106, #49744, #63259, #70470 ),
 .UNSPECIFIED., .F., .F.,
 ( 4, 2, 2, 2, 4 ),
 ( 0.0007817359430256252354, 0.0009771253907249898181, 0.001172514838424354401, 0.001367904286123718983, 0.001563293733823083566 ),
 .UNSPECIFIED. ) ;
#63235=CARTESIAN_POINT ( 'NONE',  ( -9.915792616872025178, -8.539481045369596401, 34.89627647299170832 ) ) ;
#63236=FACE_OUTER_BOUND ( 'NONE', #81462, .T. ) ;
#63239=EDGE_LOOP ( 'NONE', ( #69785, #114, #28371, #36583 ) ) ;
#63240=B_SPLINE_CURVE_WITH_KNOTS ( 'NONE', 3,
 ( #88642, #55264, #81427, #47173, #32781, #5755 ),
 .UNSPECIFIED., .F., .F.,
 ( 4, 2, 4 ),
 ( 0.0003909569690057860679, 0.0005862646681846136196, 0.0007815723673634411171 ),
 .UNSPECIFIED. ) ;
#63241=CIRCLE ( 'NONE', #25836, 5.250000000000000888 ) ;
#63242=VERTEX_POINT ( 'NONE', #37253 ) ;
#63243=B_SPLINE_CURVE_WITH_KNOTS ( 'NONE', 3,
 ( #18023, #17121, #44577, #45479, #37385, #10375, #37838, #66651, #78374, #64854 ),
 .UNSPECIFIED., .F., .F.,
 ( 4, 2, 2, 2, 4 ),
 ( 0.000000000000000000, 0.0001954311564186863052, 0.0003908623128373726104, 0.0005862934692560589156, 0.0007817246256747452209 ),
 .UNSPECIFIED. ) ;
#63244=ORIENTED_EDGE ( 'NONE', *, *, #63941, .F. ) ;
#63245=VERTEX_POINT ( 'NONE', #49887 ) ;
#63246=CARTESIAN_POINT ( 'NONE',  ( -10.83886953994894853, -12.47654668319379567, 31.42292124445336654 ) ) ;
#63247=CARTESIAN_POINT ( 'NONE',  ( -12.59168643127016196, -12.70455904226513866, 30.44083106164009322 ) ) ;
#63248=CARTESIAN_POINT ( 'NONE',  ( 17.07692307692295586, -4.481592998941358097, 33.73612834414048933 ) ) ;
#63249=EDGE_CURVE ( 'NONE', #2005, #81618, #78474, .T. ) ;
#63250=CARTESIAN_POINT ( 'NONE',  ( 0.4615384615384611200, -12.34228464037088635, 31.77849191805839268 ) ) ;
#63251=CARTESIAN_POINT ( 'NONE',  ( 17.99999999999987566, -3.083524468854526912, 32.58852847137268327 ) ) ;
#63254=ORIENTED_EDGE ( 'NONE', *, *, #61196, .T. ) ;
#63255=EDGE_LOOP ( 'NONE', ( #50563, #73059, #62671, #21019 ) ) ;
#63256=CARTESIAN_POINT ( 'NONE',  ( -3.230769230769229949, -10.51840700105979565, 33.73612834413961536 ) ) ;
#63257=ORIENTED_EDGE ( 'NONE', *, *, #30603, .F. ) ;
#63258=DIRECTION ( 'NONE',  ( 0.000000000000000000, 0.4999999999999985567, 0.8660254037844395958 ) ) ;
#63259=CARTESIAN_POINT ( 'NONE',  ( -8.703162418228332697, -11.16473453929635440, 33.15142922261926373 ) ) ;
#63260=FACE_OUTER_BOUND ( 'NONE', #42928, .T. ) ;
#63262=ORIENTED_EDGE ( 'NONE', *, *, #62117, .T. ) ;
#63263=B_SPLINE_CURVE_WITH_KNOTS ( 'NONE', 3,
 ( #70239, #8547, #36022, #85088, #1777, #29268, #22494, #77437, #15748, #8991 ),
 .UNSPECIFIED., .F., .F.,
 ( 4, 2, 2, 2, 4 ),
 ( 0.000000000000000000, 0.0001954311564186864949, 0.0003908623128373729899, 0.0005862934692560594577, 0.0007817246256747459798 ),
 .UNSPECIFIED. ) ;
#63264=VERTEX_POINT ( 'NONE', #37703 ) ;
#63265=CARTESIAN_POINT ( 'NONE',  ( -17.86947456176635640, -3.068774925481849269, 32.56582465632704526 ) ) ;
#63266=ORIENTED_EDGE ( 'NONE', *, *, #19822, .T. ) ;
#63267=FACE_BOUND ( 'NONE', #36127, .T. ) ;
#63268=CARTESIAN_POINT ( 'NONE',  ( -6.000000000000121680, -4.320704448113951379, 33.92786785259630022 ) ) ;
#63269=CARTESIAN_POINT ( 'NONE',  ( 7.976944287120798727, -5.496552790871120031, 34.60292014791297532 ) ) ;
#63270=ORIENTED_EDGE ( 'NONE', *, *, #2639, .F. ) ;
#63271=CARTESIAN_POINT ( 'NONE',  ( 16.37662569511456212, -11.41317474335729543, 32.86274602512330034 ) ) ;
#63272=CARTESIAN_POINT ( 'NONE',  ( 11.40831356872984514, -6.809168938359901446, 34.95455904226513866 ) ) ;
#63273=LINE ( 'NONE', #70484, #14833 ) ;
#63275=CARTESIAN_POINT ( 'NONE',  ( 7.846153846153725020, -2.625532179533779154, 30.86335684631627174 ) ) ;
#63276=ORIENTED_EDGE ( 'NONE', *, *, #10896, .F. ) ;
#63277=ADVANCED_FACE ( 'NONE', ( #16110 ), #2578, .F. ) ;
#63278=CARTESIAN_POINT ( 'NONE',  ( -0.6844179782760478892, -7.630690623152301733, 34.99857592706774057 ) ) ;
#63279=DIRECTION ( 'NONE',  ( -0.000000000000000000, -0.6427876096865404731, -0.7660444431189771253 ) ) ;
#63281=CARTESIAN_POINT ( 'NONE',  ( 13.51514082284903040, -2.372941743896879174, 30.88044141588253666 ) ) ;
#63282=CARTESIAN_POINT ( 'NONE',  ( 15.23076923076923173, -2.708943851104267164, 35.45975837776705220 ) ) ;
#63283=FACE_BOUND ( 'NONE', #19656, .T. ) ;
#63284=CARTESIAN_POINT ( 'NONE',  ( 5.011652630962300847, -11.48612834413959582, 32.76840700105983473 ) ) ;
#63285=CARTESIAN_POINT ( 'NONE',  ( 7.146088274689772923, -3.105924265160262543, 32.13625925475356127 ) ) ;
#63287=CARTESIAN_POINT ( 'NONE',  ( -14.55766905174090020, -3.436278759898153901, 33.07459398097509506 ) ) ;
#63289=CARTESIAN_POINT ( 'NONE',  ( 15.23076923076923173, -9.780366693483667717, 34.19971097300155094 ) ) ;
#63290=CARTESIAN_POINT ( 'NONE',  ( -10.68065461594093435, -6.835583212224499938, 34.95778746994557906 ) ) ;
#63292=EDGE_LOOP ( 'NONE', ( #70732, #46858, #13247, #2299 ) ) ;
#63293=ADVANCED_BREP_SHAPE_REPRESENTATION ( '', ( #307, #83448 ), #14453 ) ;
#63294=CARTESIAN_POINT ( 'NONE',  ( 16.15384615384615330, -3.322132147404559976, 32.92929555188717927 ) ) ;
#63296=AXIS2_PLACEMENT_3D ( 'NONE', #25384, #52846, #60938 ) ;
#63297=CARTESIAN_POINT ( 'NONE',  ( -13.16183571563731647, -9.418065098278013636, 34.63729479722530158 ) ) ;
#63299=EDGE_CURVE ( 'NONE', #18589, #69653, #43574, .T. ) ;
#63300=CARTESIAN_POINT ( 'NONE',  ( -1.384615384615506484, -4.320704448113951379, 33.92786785259630022 ) ) ;
#63301=CARTESIAN_POINT ( 'NONE',  ( 4.826899852701617810, -12.07920672191015221, 32.31858351112116168 ) ) ;
#63302=EDGE_LOOP ( 'NONE', ( #35458, #64118, #1886, #54448 ) ) ;
#63303=CARTESIAN_POINT ( 'NONE',  ( -8.096177083446811196, -5.851115903089112003, 34.47074536777953568 ) ) ;
#63305=DIRECTION ( 'NONE',  ( -0.000000000000000000, -0.8660254037844397068, -0.4999999999999978906 ) ) ;
#63306=CIRCLE ( 'NONE', #14387, 0.2500000000000002220 ) ;
#63308=CYLINDRICAL_SURFACE ( 'NONE', #11595, 0.2499999999999994726 ) ;
#63309=VECTOR ( 'NONE', #2986, 1000.000000000000227 ) ;
#63311=CARTESIAN_POINT ( 'NONE',  ( -5.076923076923075762, -1.044019251281081972, 31.83374038241031911 ) ) ;
#63315=CARTESIAN_POINT ( 'NONE',  ( 11.28843831424008393, -5.765609946408404518, 34.70566812827425451 ) ) ;
#63316=CARTESIAN_POINT ( 'NONE',  ( 14.43821800945587519, -10.88167719472716399, 33.43325721877153711 ) ) ;
#63317=ADVANCED_FACE ( 'NONE', ( #65170 ), #9362, .F. ) ;
#63318=B_SPLINE_CURVE_WITH_KNOTS ( 'NONE', 3,
 ( #8264, #42052, #22647, #1502, #21317, #613, #15464, #167, #55108, #63187 ),
 .UNSPECIFIED., .F., .F.,
 ( 4, 2, 2, 2, 4 ),
 ( 0.0007817359430256304396, 0.0009771253907249961065, 0.001172514838424361773, 0.001367904286123727440, 0.001563293733823093107 ),
 .UNSPECIFIED. ) ;
#63319=CYLINDRICAL_SURFACE ( 'NONE', #3270, 0.2499999999999994726 ) ;
#63321=CARTESIAN_POINT ( 'NONE',  ( 0.4615384615384611200, -2.708943851104267164, 35.45975837776705220 ) ) ;
#63322=VERTEX_POINT ( 'NONE', #51638 ) ;
#63323=CARTESIAN_POINT ( 'NONE',  ( 1.384615384615264011, -8.656820664282941280, 34.87096338111179961 ) ) ;
#63325=DIRECTION ( 'NONE',  ( -0.000000000000000000, 0.9848077530122085754, -0.1736481776669273613 ) ) ;
#63326=CARTESIAN_POINT ( 'NONE',  ( 8.519254025182178225, -5.643011162660950042, 34.66104346484419096 ) ) ;
#63327=CARTESIAN_POINT ( 'NONE',  ( -16.37733109757010652, -10.81261337010820256, 33.49550067578627477 ) ) ;
#63328=CARTESIAN_POINT ( 'NONE',  ( -12.46153846153846168, -6.681629849574314051, 35.83090037661290239 ) ) ;
#63330=EDGE_CURVE ( 'NONE', #20258, #45665, #18353, .T. ) ;
#63331=EDGE_CURVE ( 'NONE', #75513, #47058, #67798, .T. ) ;
#63333=ORIENTED_EDGE ( 'NONE', *, *, #50777, .T. ) ;
#63334=VECTOR ( 'NONE', #31306, 1000.000000000000227 ) ;
#63335=ORIENTED_EDGE ( 'NONE', *, *, #9004, .F. ) ;
#63337=LINE ( 'NONE', #49821, #40066 ) ;
#63338=CARTESIAN_POINT ( 'NONE',  ( 16.15384615384615330, -2.721908614388771852, 31.22303859784724978 ) ) ;
#63340=CARTESIAN_POINT ( 'NONE',  ( 10.86543903529806876, -10.06805714834173493, 34.32951233291982618 ) ) ;
#63341=B_SPLINE_CURVE_WITH_KNOTS ( 'NONE', 3,
 ( #64021, #35690, #8212, #56396, #84767, #36993, #2318, #28479, #22599, #15860 ),
 .UNSPECIFIED., .F., .F.,
 ( 4, 2, 2, 2, 4 ),
 ( 0.000000000000000000, 0.0001954311564186871184, 0.0003908623128373742367, 0.0005862934692560614093, 0.0007817246256747484735 ),
 .UNSPECIFIED. ) ;
#63342=VERTEX_POINT ( 'NONE', #45344 ) ;
#63343=DIRECTION ( 'NONE',  ( -0.000000000000000000, -0.8660254037844399289, -0.4999999999999980016 ) ) ;
#63344=ORIENTED_EDGE ( 'NONE', *, *, #3949, .T. ) ;
#63345=ORIENTED_EDGE ( 'NONE', *, *, #88535, .T. ) ;
#63346=VECTOR ( 'NONE', #75027, 1000.000000000000227 ) ;
#63347=VERTEX_POINT ( 'NONE', #32291 ) ;
#63349=ORIENTED_EDGE ( 'NONE', *, *, #62116, .F. ) ;
#63350=CYLINDRICAL_SURFACE ( 'NONE', #4282, 0.2500000000000008882 ) ;
#63351=CARTESIAN_POINT ( 'NONE',  ( -10.74553182482283198, -5.195881422630166391, 34.18770438780619259 ) ) ;
#63352=AXIS2_PLACEMENT_3D ( 'NONE', #42051, #88922, #67742 ) ;
#63353=VECTOR ( 'NONE', #77891, 1000.000000000000000 ) ;
#63354=CYLINDRICAL_SURFACE ( 'NONE', #9104, 0.2499999999999997502 ) ;
#63355=EDGE_LOOP ( 'NONE', ( #52369, #20078 ) ) ;
#63356=AXIS2_PLACEMENT_3D ( 'NONE', #41614, #68203, #69082 ) ;
#63358=ORIENTED_EDGE ( 'NONE', *, *, #64546, .T. ) ;
#63359=CARTESIAN_POINT ( 'NONE',  ( -9.692307692307691624, -5.557115091759785130, 34.35708131394839171 ) ) ;
#63360=CARTESIAN_POINT ( 'NONE',  ( 11.66925197942849302, -5.496552790871120031, 34.60292014791297532 ) ) ;
#63362=CARTESIAN_POINT ( 'NONE',  ( -7.053224132515141243, -12.45813303252208648, 30.39737893381572675 ) ) ;
#63363=CARTESIAN_POINT ( 'NONE',  ( 11.53846153846153832, -7.500000000000001776, 35.04278698407183867 ) ) ;
#63364=CARTESIAN_POINT ( 'NONE',  ( 2.557637717070352590, -9.357781135181031829, 34.66075350412533851 ) ) ;
#63365=EDGE_LOOP ( 'NONE', ( #27352, #21397, #81093, #61859 ) ) ;
#63366=CARTESIAN_POINT ( 'NONE',  ( -11.47320596718551933, -5.219633306516380244, 34.19971097300157936 ) ) ;
#63368=ORIENTED_EDGE ( 'NONE', *, *, #88415, .F. ) ;
#63369=FACE_BOUND ( 'NONE', #21383, .T. ) ;
#63370=CARTESIAN_POINT ( 'NONE',  ( -18.00000000000000000, -1.812984705146277520, 34.52197243641129631 ) ) ;
#63371=CARTESIAN_POINT ( 'NONE',  ( -13.13461538461538325, -7.500000000000001776, 35.04278698407183867 ) ) ;
#63373=DIRECTION ( 'NONE',  ( -0.000000000000000000, -0.9396926207859092051, -0.3420201433256662704 ) ) ;
#63374=LINE ( 'NONE', #65139, #32493 ) ;
#63375=CARTESIAN_POINT ( 'NONE',  ( 15.23076923076923173, -1.242168528481310874, 33.36296068462461051 ) ) ;
#63376=CARTESIAN_POINT ( 'NONE',  ( -2.530618525208453651, -3.586966769969700763, 32.86292498521069660 ) ) ;
#63377=ORIENTED_EDGE ( 'NONE', *, *, #88070, .F. ) ;
#63378=CARTESIAN_POINT ( 'NONE',  ( -11.53846153846165912, -4.481592998941358097, 33.73612834414048933 ) ) ;
#63379=FACE_OUTER_BOUND ( 'NONE', #48488, .T. ) ;
#63381=EDGE_CURVE ( 'NONE', #30821, #36751, #31260, .T. ) ;
#63382=ADVANCED_FACE ( 'NONE', ( #53887 ), #59755, .F. ) ;
#63383=LINE ( 'NONE', #57515, #7728 ) ;
#63384=CARTESIAN_POINT ( 'NONE',  ( -14.05774689831426372, -9.357781135181031829, 34.66075350412533851 ) ) ;
#63385=CARTESIAN_POINT ( 'NONE',  ( 3.007942538290226508, -7.369208160676173236, 34.74850200257122879 ) ) ;
#63386=CARTESIAN_POINT ( 'NONE',  ( 2.307692307692309264, -5.471508081941601098, 34.59228464037088457 ) ) ;
#63388=CARTESIAN_POINT ( 'NONE',  ( -8.835314180186649935, -5.557115091759785130, 34.35708131394839171 ) ) ;
#63389=FACE_BOUND ( 'NONE', #68459, .T. ) ;
#63391=CARTESIAN_POINT ( 'NONE',  ( -16.94639737515951694, -12.45806712695776319, 30.39783852428763566 ) ) ;
#63392=CARTESIAN_POINT ( 'NONE',  ( -16.08859058257013075, -2.625532179533469623, 30.86335684631491105 ) ) ;
#63393=CARTESIAN_POINT ( 'NONE',  ( -5.010855743573000787, -9.905515769479277921, 34.41647553114623292 ) ) ;
#63394=CARTESIAN_POINT ( 'NONE',  ( -12.52762187249434156, -4.098570777380719399, 33.41473453929634729 ) ) ;
#63395=AXIS2_PLACEMENT_3D ( 'NONE', #34802, #27605, #27162 ) ;
#63396=CARTESIAN_POINT ( 'NONE',  ( -17.93393164899756087, -4.786620604624112651, 33.94971097300155805 ) ) ;
#63398=ORIENTED_EDGE ( 'NONE', *, *, #12493, .F. ) ;
#63399=EDGE_LOOP ( 'NONE', ( #27617, #82938, #58697, #63899 ) ) ;
#63400=EDGE_CURVE ( 'NONE', #74750, #75555, #50560, .T. ) ;
#63401=LINE ( 'NONE', #83700, #3203 ) ;
#63402=CARTESIAN_POINT ( 'NONE',  ( -12.21159305216042057, -6.653508905675592722, 34.93172785388651391 ) ) ;
#63403=CARTESIAN_POINT ( 'NONE',  ( 14.43821774592595197, -9.503571793651731880, 34.60286762892837942 ) ) ;
#63404=DIRECTION ( 'NONE',  ( 0.000000000000000000, 0.1736481776669275834, 0.9848077530122086864 ) ) ;
#63405=CARTESIAN_POINT ( 'NONE',  ( -13.31854805126531005, -2.486705287966280320, 31.30864560766543647 ) ) ;
#63407=B_SPLINE_CURVE_WITH_KNOTS ( 'NONE', 3,
 ( #73233, #45302, #17399, #64678, #24593, #10200, #30460, #66476, #79551, #65123 ),
 .UNSPECIFIED., .F., .F.,
 ( 4, 2, 2, 2, 4 ),
 ( 0.000000000000000000, 0.0001954311564186862781, 0.0003908623128373725562, 0.0005862934692560588072, 0.0007817246256747451124 ),
 .UNSPECIFIED. ) ;
#63408=CARTESIAN_POINT ( 'NONE',  ( 4.023369445729690241, -7.276988635370452485, 34.74523720219453793 ) ) ;
#63409=CARTESIAN_POINT ( 'NONE',  ( 11.53846153846153832, -1.367168528481310208, 33.57946703557072254 ) ) ;
#63410=CARTESIAN_POINT ( 'NONE',  ( 17.07692307692307665, -2.499999999999998668, 29.75000000000001421 ) ) ;
#63411=CARTESIAN_POINT ( 'NONE',  ( 15.23076923076923173, -3.322132147404559976, 32.92929555188717927 ) ) ;
#63413=CARTESIAN_POINT ( 'NONE',  ( -4.826868657009622865, -6.523592122091591783, 34.90882529074906415 ) ) ;
#63414=DIRECTION ( 'NONE',  ( 0.000000000000000000, 0.4999999999999960032, -0.8660254037844410391 ) ) ;
#63416=EDGE_CURVE ( 'NONE', #69312, #63565, #54880, .T. ) ;
#63417=CARTESIAN_POINT ( 'NONE',  ( 14.08476609017615644, -6.503392248772476236, 34.64988816332204635 ) ) ;
#63418=AXIS2_PLACEMENT_3D ( 'NONE', #77061, #76615, #42400 ) ;
#63419=ORIENTED_EDGE ( 'NONE', *, *, #60754, .T. ) ;
#63420=CARTESIAN_POINT ( 'NONE',  ( 2.241609928332174206, -3.322132147404559976, 32.92929555188719348 ) ) ;
#63421=CARTESIAN_POINT ( 'NONE',  ( 10.74617505635156789, -5.496552790871120031, 34.60292014791297532 ) ) ;
#63423=AXIS2_PLACEMENT_3D ( 'NONE', #26041, #74229, #66585 ) ;
#63424=AXIS2_PLACEMENT_3D ( 'NONE', #35142, #42359, #21624 ) ;
#63425=CARTESIAN_POINT ( 'NONE',  ( 8.834424751014125832, -2.506253911140448043, 29.99999999999988631 ) ) ;
#63426=CARTESIAN_POINT ( 'NONE',  ( -16.08859101433330707, -2.657715359629131857, 31.77849191805844242 ) ) ;
#63427=ORIENTED_EDGE ( 'NONE', *, *, #16028, .T. ) ;
#63428=CARTESIAN_POINT ( 'NONE',  ( -9.692307692307691624, -5.180354513474913603, 36.12317359536750416 ) ) ;
#63429=DIRECTION ( 'NONE',  ( -0.000000000000000000, -0.5000000000000009992, -0.8660254037844380415 ) ) ;
#63430=VERTEX_POINT ( 'NONE', #86815 ) ;
#63431=CARTESIAN_POINT ( 'NONE',  ( 7.145856464345333059, -3.755027918224367767, 33.06320215134714857 ) ) ;
#63432=CARTESIAN_POINT ( 'NONE',  ( -4.826868765284761054, -9.943054286541403997, 34.11300777759954883 ) ) ;
#63434=CARTESIAN_POINT ( 'NONE',  ( -5.326899807865430603, -12.17611988154120972, 31.52148481390971213 ) ) ;
#63435=CARTESIAN_POINT ( 'NONE',  ( 10.86533002476265963, -10.92531984108285670, 33.72920026020278073 ) ) ;
#63436=ORIENTED_EDGE ( 'NONE', *, *, #43863, .F. ) ;
#63437=CARTESIAN_POINT ( 'NONE',  ( 8.899756207464411872, -2.372941743896879174, 30.88044141588253666 ) ) ;
#63441=ORIENTED_EDGE ( 'NONE', *, *, #10205, .F. ) ;
#63444=CARTESIAN_POINT ( 'NONE',  ( -6.700297254098854793, -8.540255544307065350, 34.89611431652622286 ) ) ;
#63445=EDGE_LOOP ( 'NONE', ( #9646, #43163, #3781, #75888 ) ) ;
#63446=EDGE_CURVE ( 'NONE', #27850, #9213, #1109, .T. ) ;
#63447=B_SPLINE_CURVE_WITH_KNOTS ( 'NONE', 3,
 ( #47252, #73403, #11709, #74744, #87833, #46814, #13470, #80618, #40948, #26102 ),
 .UNSPECIFIED., .F., .F.,
 ( 4, 2, 2, 2, 4 ),
 ( 0.000000000000000000, 0.0001954339857564093175, 0.0003908679715128186350, 0.0005863019572692279796, 0.0007817359430256372700 ),
 .UNSPECIFIED. ) ;
#63448=CARTESIAN_POINT ( 'NONE',  ( 12.59206416330202671, -9.417988943895561960, 34.36773134775777550 ) ) ;
#63449=FACE_OUTER_BOUND ( 'NONE', #87636, .T. ) ;
#63450=EDGE_CURVE ( 'NONE', #1602, #3325, #82807, .T. ) ;
#63452=DIRECTION ( 'NONE',  ( 0.000000000000000000, 0.1736481776669275834, 0.9848077530122086864 ) ) ;
#63453=AXIS2_PLACEMENT_3D ( 'NONE', #80648, #81530, #18931 ) ;
#63454=EDGE_LOOP ( 'NONE', ( #32009, #32686, #78870, #27937 ) ) ;
#63455=ORIENTED_EDGE ( 'NONE', *, *, #86640, .F. ) ;
#63456=CARTESIAN_POINT ( 'NONE',  ( -2.530520405327184807, -7.369209533119137845, 34.99857337881830688 ) ) ;
#63457=VERTEX_POINT ( 'NONE', #75059 ) ;
#63458=CARTESIAN_POINT ( 'NONE',  ( 16.21904013562951263, -2.506253911140448043, 29.99999999999988631 ) ) ;
#63459=EDGE_LOOP ( 'NONE', ( #55436, #15097, #26681, #78987 ) ) ;
#63460=CARTESIAN_POINT ( 'NONE',  ( -18.00000000000000000, -5.471508081941599322, 34.59228464037088457 ) ) ;
#63461=CARTESIAN_POINT ( 'NONE',  ( 10.36538461538461675, -2.499999999999998668, 29.75000000000000355 ) ) ;
#63462=ORIENTED_EDGE ( 'NONE', *, *, #24560, .T. ) ;
#63463=CARTESIAN_POINT ( 'NONE',  ( 8.068933387422255521, -8.496831190052093419, 34.64984203495476578 ) ) ;
#63465=CARTESIAN_POINT ( 'NONE',  ( -6.673022611438608642, -11.28795663066794219, 33.01431243580653785 ) ) ;
#63466=ORIENTED_EDGE ( 'NONE', *, *, #1090, .F. ) ;
#63469=CARTESIAN_POINT ( 'NONE',  ( -15.90390063549801347, -3.712312575010499494, 33.01462480002815170 ) ) ;
#63470=ORIENTED_EDGE ( 'NONE', *, *, #31288, .T. ) ;
#63471=B_SPLINE_CURVE_WITH_KNOTS ( 'NONE', 3,
 ( #33773, #67122, #13059, #7188, #74320, #34658, #81528, #34208, #32886, #430 ),
 .UNSPECIFIED., .F., .F.,
 ( 4, 2, 2, 2, 4 ),
 ( 0.000000000000000000, 0.0001954311564186869286, 0.0003908623128373738573, 0.0005862934692560607588, 0.0007817246256747477145 ),
 .UNSPECIFIED. ) ;
#63472=B_SPLINE_CURVE_WITH_KNOTS ( 'NONE', 3,
 ( #28056, #21741, #82577, #70375, #77573, #49655, #76690, #14993, #77129, #42911 ),
 .UNSPECIFIED., .F., .F.,
 ( 4, 2, 2, 2, 4 ),
 ( 0.000000000000000000, 0.0001954311564186879315, 0.0003908623128373758630, 0.0005862934692560637946, 0.0007817246256747517261 ),
 .UNSPECIFIED. ) ;
#63473=AXIS2_PLACEMENT_3D ( 'NONE', #61853, #62297, #27634 ) ;
#63474=CARTESIAN_POINT ( 'NONE',  ( 16.08857570788537572, -12.46129190929999986, 30.37095296980880832 ) ) ;
#63475=CARTESIAN_POINT ( 'NONE',  ( 17.86985203026830149, -12.50552854090298638, 31.33409797877408920 ) ) ;
#63476=FACE_BOUND ( 'NONE', #52029, .T. ) ;
#63477=CARTESIAN_POINT ( 'NONE',  ( -9.692307692307814193, -4.320704448113951379, 33.92786785259630022 ) ) ;
#63478=CARTESIAN_POINT ( 'NONE',  ( -11.78843828251013015, -6.524016743844655686, 34.90889640711025521 ) ) ;
#63479=VECTOR ( 'NONE', #68914, 1000.000000000000227 ) ;
#63480=CARTESIAN_POINT ( 'NONE',  ( 15.23076923076910916, -2.657715359629662544, 31.77849191805970364 ) ) ;
#63481=LINE ( 'NONE', #27933, #28847 ) ;
#63482=CARTESIAN_POINT ( 'NONE',  ( -11.53846153846165912, -3.300289026999228881, 32.46337939537708905 ) ) ;
#63483=CARTESIAN_POINT ( 'NONE',  ( -16.28399412357785536, -2.647304123082328875, 31.75400227202885262 ) ) ;
#63485=CARTESIAN_POINT ( 'NONE',  ( 10.39189967166066708, -10.11188796281391511, 34.01382737946119050 ) ) ;
#63486=EDGE_LOOP ( 'NONE', ( #20330, #74070, #64126, #61017 ) ) ;
#63488=VECTOR ( 'NONE', #22435, 1000.000000000000114 ) ;
#63489=EDGE_CURVE ( 'NONE', #63457, #86663, #72889, .T. ) ;
#63490=CARTESIAN_POINT ( 'NONE',  ( -5.207071046654769830, -12.15440758774515473, 32.17923288041532004 ) ) ;
#63491=CARTESIAN_POINT ( 'NONE',  ( 16.37662569511455857, -12.24180327182771855, 31.33663988360758168 ) ) ;
#63492=LINE ( 'NONE', #21177, #62872 ) ;
#63493=CARTESIAN_POINT ( 'NONE',  ( -15.23076923076922995, -1.422936976036506707, 30.56769352161908415 ) ) ;
#63494=CARTESIAN_POINT ( 'NONE',  ( -10.39260494640654819, -12.47679350104403007, 31.42216943046555855 ) ) ;
#63495=CARTESIAN_POINT ( 'NONE',  ( 14.37375964104238513, -11.35647404775217595, 33.31231777344666511 ) ) ;
#63497=CARTESIAN_POINT ( 'NONE',  ( 13.13459214732242408, -5.056417327199099532, 34.11270091957321426 ) ) ;
#63498=CARTESIAN_POINT ( 'NONE',  ( 0.4615384615384611200, -8.973038597847269315, 34.52809138561121927 ) ) ;
#63499=CARTESIAN_POINT ( 'NONE',  ( -12.71151520558705172, -11.47974371597208076, 33.17467449705390692 ) ) ;
#63500=CARTESIAN_POINT ( 'NONE',  ( -16.82692307692165556, -7.500000000000154543, 35.00000000000007105 ) ) ;
#63501=CYLINDRICAL_SURFACE ( 'NONE', #4606, 0.2500000000000002220 ) ;
#63503=ORIENTED_EDGE ( 'NONE', *, *, #33980, .F. ) ;
#63504=ORIENTED_EDGE ( 'NONE', *, *, #23061, .F. ) ;
#63505=EDGE_CURVE ( 'NONE', #41484, #36333, #41268, .T. ) ;
#63507=EDGE_LOOP ( 'NONE', ( #79651, #31352, #76701, #58339, #53706, #48951 ) ) ;
#63508=CARTESIAN_POINT ( 'NONE',  ( 16.15384615384603251, -11.06231777344772027, 33.60647404775119895 ) ) ;
#63509=CARTESIAN_POINT ( 'NONE',  ( 8.769230769230768274, -13.78497067705608181, 32.30358669280327177 ) ) ;
#63510=LINE ( 'NONE', #76140, #26484 ) ;
#63511=ADVANCED_FACE ( 'NONE', ( #68732 ), #54767, .F. ) ;
#63512=DIRECTION ( 'NONE',  ( -0.000000000000000000, -0.9396926207859092051, -0.3420201433256662704 ) ) ;
#63514=DIRECTION ( 'NONE',  ( -0.000000000000000000, 0.1736481776669307198, -0.9848077530122080203 ) ) ;
#63515=ORIENTED_EDGE ( 'NONE', *, *, #56967, .F. ) ;
#63516=DIRECTION ( 'NONE',  ( -0.000000000000000000, -0.9396926207859093161, -0.3420201433256663259 ) ) ;
#63517=CARTESIAN_POINT ( 'NONE',  ( -1.319359813339359366, -9.442884908240271713, 34.35708131394835618 ) ) ;
#63518=ORIENTED_EDGE ( 'NONE', *, *, #28620, .F. ) ;
#63519=CARTESIAN_POINT ( 'NONE',  ( 3.007843013253082454, -12.39988816332205701, 30.74660775122750778 ) ) ;
#63520=CARTESIAN_POINT ( 'NONE',  ( -0.6850233861027927862, -4.225889041578354544, 33.85425143139329407 ) ) ;
#63523=CARTESIAN_POINT ( 'NONE',  ( 6.856994543716787405, -3.322132147404559976, 32.92929555188719348 ) ) ;
#63527=ORIENTED_EDGE ( 'NONE', *, *, #50424, .F. ) ;
#63528=CARTESIAN_POINT ( 'NONE',  ( -1.161835843346975539, -11.41317474335729187, 32.86274602512330034 ) ) ;
#63529=CARTESIAN_POINT ( 'NONE',  ( -1.134560964701930796, -3.435999193479609470, 33.07426656108011542 ) ) ;
#63531=EDGE_CURVE ( 'NONE', #998, #47096, #41966, .T. ) ;
#63532=CARTESIAN_POINT ( 'NONE',  ( 0.2115152373170033073, -5.765609946408404518, 34.70566812827425451 ) ) ;
#63533=CARTESIAN_POINT ( 'NONE',  ( -7.715628407920204879, -3.068774925481847493, 32.56582465632704526 ) ) ;
#63536=CARTESIAN_POINT ( 'NONE',  ( -2.307692307692427391, -3.300289026999228881, 32.46337939537708905 ) ) ;
#63537=EDGE_CURVE ( 'NONE', #65576, #46336, #28641, .T. ) ;
#63538=EDGE_LOOP ( 'NONE', ( #76570, #25049, #35437, #77859 ) ) ;
#63540=CYLINDRICAL_SURFACE ( 'NONE', #28445, 0.2499999999999986955 ) ;
#63541=VERTEX_POINT ( 'NONE', #49353 ) ;
#63543=CARTESIAN_POINT ( 'NONE',  ( 4.153846153846032507, -3.835265460704628371, 33.15142922262033665 ) ) ;
#63544=ADVANCED_FACE ( 'NONE', ( #76830 ), #13344, .F. ) ;
#63545=CARTESIAN_POINT ( 'NONE',  ( 8.769230769230768274, -12.78798330534103123, 29.99999999999997868 ) ) ;
#63546=LINE ( 'NONE', #14934, #63769 ) ;
#63548=CARTESIAN_POINT ( 'NONE',  ( 7.846153846153846700, -8.164416787775445883, 34.95778746994557906 ) ) ;
#63549=ADVANCED_FACE ( 'NONE', ( #20545 ), #82704, .F. ) ;
#63550=AXIS2_PLACEMENT_3D ( 'NONE', #25058, #52520, #44417 ) ;
#63551=ORIENTED_EDGE ( 'NONE', *, *, #57127, .F. ) ;
#63552=CARTESIAN_POINT ( 'NONE',  ( 12.21156171748987163, -12.01397095200674059, 32.43157075238190146 ) ) ;
#63553=CARTESIAN_POINT ( 'NONE',  ( -10.83831083290075981, -2.758268499246657068, 31.33685645148948140 ) ) ;
#63554=ORIENTED_EDGE ( 'NONE', *, *, #43191, .F. ) ;
#63555=EDGE_CURVE ( 'NONE', #54624, #38474, #10853, .T. ) ;
#63556=CARTESIAN_POINT ( 'NONE',  ( -5.749945688361685292, -11.28795663066794219, 33.01431243580653785 ) ) ;
#63558=CYLINDRICAL_SURFACE ( 'NONE', #9228, 0.2499999999999994726 ) ;
#63559=VECTOR ( 'NONE', #70076, 1000.000000000000227 ) ;
#63560=DIRECTION ( 'NONE',  ( 0.000000000000000000, 0.3420201433256610524, 0.9396926207859113145 ) ) ;
#63562=ORIENTED_EDGE ( 'NONE', *, *, #12424, .F. ) ;
#63563=EDGE_LOOP ( 'NONE', ( #89076, #996 ) ) ;
#63564=FACE_BOUND ( 'NONE', #15431, .T. ) ;
#63565=VERTEX_POINT ( 'NONE', #44344 ) ;
#63566=CARTESIAN_POINT ( 'NONE',  ( 15.00728428704528561, -12.44517049084099725, 30.48991314939691932 ) ) ;
#63567=EDGE_CURVE ( 'NONE', #16683, #83747, #34452, .T. ) ;
#63568=CARTESIAN_POINT ( 'NONE',  ( -20.74999999999999645, -4.499999999999999112, 29.75000000000000355 ) ) ;
#63570=CARTESIAN_POINT ( 'NONE',  ( 6.130525438233644486, -3.068774925481847937, 32.56582465632704526 ) ) ;
#63571=CARTESIAN_POINT ( 'NONE',  ( -14.17716660592874689, -9.417988943895561960, 34.36773134775777550 ) ) ;
#63572=B_SPLINE_CURVE_WITH_KNOTS ( 'NONE', 3,
 ( #34449, #53384, #19166, #74113, #12407, #39891, #33120, #47064, #60586, #81322 ),
 .UNSPECIFIED., .F., .F.,
 ( 4, 2, 2, 2, 4 ),
 ( 0.000000000000000000, 0.0001954339857564099951, 0.0003908679715128199903, 0.0005863019572692300396, 0.0007817359430256399806 ),
 .UNSPECIFIED. ) ;
#63573=ORIENTED_EDGE ( 'NONE', *, *, #25311, .T. ) ;
#63574=ORIENTED_EDGE ( 'NONE', *, *, #59866, .T. ) ;
#63575=VERTEX_POINT ( 'NONE', #16449 ) ;
#63578=VERTEX_POINT ( 'NONE', #79037 ) ;
#63579=EDGE_CURVE ( 'NONE', #46007, #69974, #22652, .T. ) ;
#63580=CARTESIAN_POINT ( 'NONE',  ( 13.13459214732242053, -2.823816976329317274, 31.52131813110795733 ) ) ;
#63581=CARTESIAN_POINT ( 'NONE',  ( -2.531177232256638820, -12.47654668319379567, 31.42292124445336654 ) ) ;
#63582=EDGE_CURVE ( 'NONE', #84853, #63945, #9722, .T. ) ;
#63583=CARTESIAN_POINT ( 'NONE',  ( -17.30040800148741198, -3.019605429927187501, 32.48692288466676814 ) ) ;
#63584=ORIENTED_EDGE ( 'NONE', *, *, #77344, .F. ) ;
#63585=CARTESIAN_POINT ( 'NONE',  ( -8.546217925137373328, -4.026326845037962343, 33.68677907613344047 ) ) ;
#63586=EDGE_CURVE ( 'NONE', #30665, #18168, #67130, .T. ) ;
#63588=CARTESIAN_POINT ( 'NONE',  ( -17.74989548036563036, -7.568793089027813004, 35.00000000000000711 ) ) ;
#63590=EDGE_LOOP ( 'NONE', ( #83548, #34062, #12, #34681 ) ) ;
#63591=ORIENTED_EDGE ( 'NONE', *, *, #39750, .T. ) ;
#63592=EDGE_LOOP ( 'NONE', ( #86978, #22419 ) ) ;
#63593=CARTESIAN_POINT ( 'NONE',  ( 3.100159575565149428, -7.722926974430166069, 34.99546784045485737 ) ) ;
#63594=ADVANCED_FACE ( 'NONE', ( #44795 ), #2478, .F. ) ;
#63596=CARTESIAN_POINT ( 'NONE',  ( -9.692307692307814193, -8.656820664282941280, 34.87096338111179961 ) ) ;
#63597=CYLINDRICAL_SURFACE ( 'NONE', #87409, 0.2499999999999986955 ) ;
#63598=LINE ( 'NONE', #82996, #62409 ) ;
#63599=FACE_BOUND ( 'NONE', #65455, .T. ) ;
#63600=DIRECTION ( 'NONE',  ( -0.000000000000000000, 0.9396926207859092051, -0.3420201433256662704 ) ) ;
#63601=VERTEX_POINT ( 'NONE', #65066 ) ;
#63604=DIRECTION ( 'NONE',  ( -0.000000000000000000, 0.3420201433256694346, -0.9396926207859080948 ) ) ;
#63605=CARTESIAN_POINT ( 'NONE',  ( -11.40793583669797151, -3.816742781228458004, 33.13167719472716044 ) ) ;
#63606=EDGE_LOOP ( 'NONE', ( #5850, #71850 ) ) ;
#63608=VERTEX_POINT ( 'NONE', #84040 ) ;
#63609=FACE_BOUND ( 'NONE', #60690, .T. ) ;
#63610=B_SPLINE_CURVE_WITH_KNOTS ( 'NONE', 3,
 ( #42511, #76282, #48366, #35757, #34851, #62757, #63205, #633, #69528, #1522 ),
 .UNSPECIFIED., .F., .F.,
 ( 4, 2, 2, 2, 4 ),
 ( 0.0007817246256747446788, 0.0009771112852218872494, 0.001172497944769029929, 0.001367884604316172391, 0.001563271263863315070 ),
 .UNSPECIFIED. ) ;
#63611=CARTESIAN_POINT ( 'NONE',  ( -16.85414353565466072, -4.387253974876675677, 33.66317474335728832 ) ) ;
#63613=B_SPLINE_CURVE_WITH_KNOTS ( 'NONE', 3,
 ( #17097, #3576, #9897, #23404, #72037, #50862, #36496, #44551, #52208, #10346 ),
 .UNSPECIFIED., .F., .F.,
 ( 4, 2, 2, 2, 4 ),
 ( 0.0007817359430256360774, 0.0009771253907250041296, 0.001172514838424371965, 0.001367904286123740017, 0.001563293733823108069 ),
 .UNSPECIFIED. ) ;
#63614=CARTESIAN_POINT ( 'NONE',  ( 14.30769230769231015, -1.044019251281081972, 31.83374038241031911 ) ) ;
#63615=CARTESIAN_POINT ( 'NONE',  ( 14.05771557674995442, -11.79746400365624659, 32.30657167506340954 ) ) ;
#63616=ORIENTED_EDGE ( 'NONE', *, *, #44942, .T. ) ;
#63617=CARTESIAN_POINT ( 'NONE',  ( 11.78851595837499211, -10.82426656108012075, 33.81400080652039009 ) ) ;
#63618=CARTESIAN_POINT ( 'NONE',  ( -18.00000000000000000, -3.937682226553330445, 33.60647404775216529 ) ) ;
#63619=CARTESIAN_POINT ( 'NONE',  ( -10.61538461538461320, -1.422936976036506707, 30.56769352161908415 ) ) ;
#63621=CARTESIAN_POINT ( 'NONE',  ( -5.076923076923199218, -5.941354392335915335, 34.76329471203413846 ) ) ;
#63622=VERTEX_POINT ( 'NONE', #63300 ) ;
#63624=FACE_OUTER_BOUND ( 'NONE', #71597, .T. ) ;
#63626=CARTESIAN_POINT ( 'NONE',  ( 13.63456090296352485, -12.22109172314383052, 31.39792113162168263 ) ) ;
#63627=ORIENTED_EDGE ( 'NONE', *, *, #16714, .T. ) ;
#63628=CARTESIAN_POINT ( 'NONE',  ( 11.76147289007438701, -6.503523203565941380, 34.64991518177335195 ) ) ;
#63629=CARTESIAN_POINT ( 'NONE',  ( -10.68065506134539078, -12.46129190929999986, 30.37095296980880832 ) ) ;
#63630=CYLINDRICAL_SURFACE ( 'NONE', #81764, 0.2499999999999994726 ) ;
#63631=DIRECTION ( 'NONE',  ( -0.000000000000000000, -0.3420201433256694901, -0.9396926207859082059 ) ) ;
#63632=CARTESIAN_POINT ( 'NONE',  ( 9.019230769230784261, -2.249999999999997780, 29.81603969181030322 ) ) ;
#63633=CARTESIAN_POINT ( 'NONE',  ( 18.00000000000000000, -4.661471528628507777, 34.16647553114623292 ) ) ;
#63634=CARTESIAN_POINT ( 'NONE',  ( 12.23865977910981506, -7.630691491037285168, 34.74850469731152458 ) ) ;
#63637=VERTEX_POINT ( 'NONE', #56550 ) ;
#63638=CARTESIAN_POINT ( 'NONE',  ( -0.5916856709766816769, -6.001485441113819874, 34.52039167877662607 ) ) ;
#63642=ORIENTED_EDGE ( 'NONE', *, *, #20116, .T. ) ;
#63643=CARTESIAN_POINT ( 'NONE',  ( 16.94677586748485965, -5.195881422630167279, 34.18770438780618548 ) ) ;
#63644=DIRECTION ( 'NONE',  ( 0.000000000000000000, 0.7660444431189807890, 0.6427876096865361433 ) ) ;
#63645=CARTESIAN_POINT ( 'NONE',  ( 0.7115384615398802071, -7.500000000000154543, 35.00000000000007105 ) ) ;
#63646=CARTESIAN_POINT ( 'NONE',  ( 10.61538461538461675, -6.343179335718451384, 34.87096338111211935 ) ) ;
#63647=CARTESIAN_POINT ( 'NONE',  ( -9.019207513279360100, -2.544273027872575366, 31.48422191005632342 ) ) ;
#63648=CARTESIAN_POINT ( 'NONE',  ( 20.74999999999999645, -2.499999999999999556, 29.75000000000000355 ) ) ;
#63650=CYLINDRICAL_SURFACE ( 'NONE', #36489, 0.2499999999999995559 ) ;
#63651=CARTESIAN_POINT ( 'NONE',  ( -8.769230769230892619, -2.379036618888197729, 30.90682066428292885 ) ) ;
#63653=EDGE_CURVE ( 'NONE', #56750, #32572, #70509, .T. ) ;
#63654=B_SPLINE_CURVE_WITH_KNOTS ( 'NONE', 3,
 ( #13451, #18886, #5817, #53995, #20653, #33294 ),
 .UNSPECIFIED., .F., .F.,
 ( 4, 2, 4 ),
 ( 0.0003909512603273828648, 0.0005862562993132068752, 0.0007815613382990308855 ),
 .UNSPECIFIED. ) ;
#63655=B_SPLINE_CURVE_WITH_KNOTS ( 'NONE', 3,
 ( #62476, #89103, #69252, #67926, #35017, #6231, #53508, #88664, #81005, #46764 ),
 .UNSPECIFIED., .F., .F.,
 ( 4, 2, 2, 2, 4 ),
 ( 0.0007817359430256328248, 0.0009771253907249995759, 0.001172514838424366327, 0.001367904286123732861, 0.001563293733823099612 ),
 .UNSPECIFIED. ) ;
#63656=FACE_OUTER_BOUND ( 'NONE', #3772, .T. ) ;
#63657=B_SPLINE_CURVE_WITH_KNOTS ( 'NONE', 3,
 ( #5786, #34138, #54406, #47205, #40905, #5344, #12987, #60275, #75563, #40032 ),
 .UNSPECIFIED., .F., .F.,
 ( 4, 2, 2, 2, 4 ),
 ( 0.0007817246256747440282, 0.0009771112852218863821, 0.001172497944769028844, 0.001367884604316171307, 0.001563271263863313769 ),
 .UNSPECIFIED. ) ;
#63658=FACE_OUTER_BOUND ( 'NONE', #24725, .T. ) ;
#63659=EDGE_CURVE ( 'NONE', #33070, #84431, #63743, .T. ) ;
#63660=ORIENTED_EDGE ( 'NONE', *, *, #75116, .T. ) ;
#63661=CARTESIAN_POINT ( 'NONE',  ( 15.10062202133100939, -11.47017969459903952, 32.78971311882035167 ) ) ;
#63662=CARTESIAN_POINT ( 'NONE',  ( -2.307692307692305711, -8.973038597847269315, 34.52809138561121927 ) ) ;
#63663=CARTESIAN_POINT ( 'NONE',  ( 12.68454981315131214, -10.61302985866384141, 33.66295027996417843 ) ) ;
#63664=VERTEX_POINT ( 'NONE', #22753 ) ;
#63665=EDGE_CURVE ( 'NONE', #74089, #41980, #19121, .T. ) ;
#63667=CARTESIAN_POINT ( 'NONE',  ( -17.07692307692319744, -3.835265460704628815, 33.15142922262033665 ) ) ;
#63668=ADVANCED_FACE ( 'NONE', ( #25430 ), #66416, .F. ) ;
#63669=CARTESIAN_POINT ( 'NONE',  ( -12.39547011053602432, -10.51840700105979565, 33.73612834413962247 ) ) ;
#63670=EDGE_LOOP ( 'NONE', ( #57914, #679 ) ) ;
#63671=CARTESIAN_POINT ( 'NONE',  ( -13.38461538461538325, -9.780366693483667717, 34.19971097300155094 ) ) ;
#63672=ORIENTED_EDGE ( 'NONE', *, *, #58091, .T. ) ;
#63673=EDGE_CURVE ( 'NONE', #41990, #6248, #66684, .T. ) ;
#63674=CARTESIAN_POINT ( 'NONE',  ( 9.942253210655835005, -11.86320923018887719, 32.19269448109604070 ) ) ;
#63675=AXIS2_PLACEMENT_3D ( 'NONE', #59584, #57917, #70993 ) ;
#63676=CARTESIAN_POINT ( 'NONE',  ( 6.989144256426999213, -2.833524468853757750, 32.15551576947925838 ) ) ;
#63677=DIRECTION ( 'NONE',  ( -0.000000000000000000, 1.000000000000000000, -0.000000000000000000 ) ) ;
#63678=CARTESIAN_POINT ( 'NONE',  ( -12.46153846153846168, -3.937682226553329556, 33.60647404775216529 ) ) ;
#63679=CARTESIAN_POINT ( 'NONE',  ( 1.384615384615386802, -13.53365097954675988, 30.81389545987213552 ) ) ;
#63680=B_SPLINE_CURVE_WITH_KNOTS ( 'NONE', 3,
 ( #85102, #77453, #78327, #56737, #57179, #56298, #84232, #49543, #15317, #42794 ),
 .UNSPECIFIED., .F., .F.,
 ( 4, 2, 2, 2, 4 ),
 ( 0.0007817359430256372700, 0.0009771253907250054306, 0.001172514838424373483, 0.001367904286123741535, 0.001563293733823109804 ),
 .UNSPECIFIED. ) ;
#63681=ORIENTED_EDGE ( 'NONE', *, *, #24896, .F. ) ;
#63682=B_SPLINE_CURVE_WITH_KNOTS ( 'NONE', 3,
 ( #45151, #18585, #51436, #10934, #73076, #79395, #58221, #37960, #12262, #79841 ),
 .UNSPECIFIED., .F., .F.,
 ( 4, 2, 2, 2, 4 ),
 ( 0.000000000000000000, 0.0001954339881912772715, 0.0003908679763825545429, 0.0005863019645738318415, 0.0007817359527651090859 ),
 .UNSPECIFIED. ) ;
#63683=B_SPLINE_CURVE_WITH_KNOTS ( 'NONE', 3,
 ( #81590, #11800, #4133, #39279, #66736, #18113, #38376, #65830, #81152, #5034 ),
 .UNSPECIFIED., .F., .F.,
 ( 4, 2, 2, 2, 4 ),
 ( 0.0007817246256747504250, 0.0009771112852218954894, 0.001172497944769040554, 0.001367884604316185401, 0.001563271263863330466 ),
 .UNSPECIFIED. ) ;
#63684=EDGE_LOOP ( 'NONE', ( #29806, #20507 ) ) ;
#63685=ORIENTED_EDGE ( 'NONE', *, *, #11488, .F. ) ;
#63686=DIRECTION ( 'NONE',  ( 0.000000000000000000, 0.3420201433256641055, -0.9396926207859100932 ) ) ;
#63687=CARTESIAN_POINT ( 'NONE',  ( 16.15384615384603251, -5.941354392335915335, 34.76329471203413846 ) ) ;
#63688=ADVANCED_FACE ( 'NONE', ( #73636 ), #73178, .F. ) ;
#63689=CARTESIAN_POINT ( 'NONE',  ( -4.377331078410485077, -12.47654668319379567, 31.42292124445336654 ) ) ;
#63690=CARTESIAN_POINT ( 'NONE',  ( 11.40777007179397984, -12.11776431015576172, 31.66791131148498906 ) ) ;
#63691=CARTESIAN_POINT ( 'NONE',  ( 7.715678661078126943, -7.276987145209185215, 34.99546412871779211 ) ) ;
#63692=CARTESIAN_POINT ( 'NONE',  ( 17.99999999999987566, -12.46129190930018460, 30.37095296980731973 ) ) ;
#63693=ORIENTED_EDGE ( 'NONE', *, *, #13412, .F. ) ;
#63694=VERTEX_POINT ( 'NONE', #52446 ) ;
#63695=VERTEX_POINT ( 'NONE', #5605 ) ;
#63696=CARTESIAN_POINT ( 'NONE',  ( 12.52760681254089903, -8.120952969808772792, 34.71129190929999453 ) ) ;
#63697=ADVANCED_FACE ( 'NONE', ( #19557 ), #80388, .F. ) ;
#63698=ORIENTED_EDGE ( 'NONE', *, *, #5566, .T. ) ;
#63700=CARTESIAN_POINT ( 'NONE',  ( -9.758391103263571509, -8.973038597847271092, 34.52809138561120506 ) ) ;
#63701=CARTESIAN_POINT ( 'NONE',  ( -10.39237177129122003, -6.460100341425560444, 34.89618726649961644 ) ) ;
#63704=EDGE_CURVE ( 'NONE', #54661, #85662, #5433, .T. ) ;
#63705=ORIENTED_EDGE ( 'NONE', *, *, #45844, .T. ) ;
#63706=CARTESIAN_POINT ( 'NONE',  ( 4.854043560185492545, -7.630690623152302621, 34.99857592706774057 ) ) ;
#63707=ORIENTED_EDGE ( 'NONE', *, *, #36863, .F. ) ;
#63708=FACE_BOUND ( 'NONE', #53686, .T. ) ;
#63709=B_SPLINE_CURVE_WITH_KNOTS ( 'NONE', 3,
 ( #370, #76910, #82348, #35930, #63384, #70146, #8458, #1692, #29182, #56635 ),
 .UNSPECIFIED., .F., .F.,
 ( 4, 2, 2, 2, 4 ),
 ( 0.0007817246256747460882, 0.0009771112852218900684, 0.001172497944769033832, 0.001367884604316177595, 0.001563271263863321575 ),
 .UNSPECIFIED. ) ;
#63711=FACE_OUTER_BOUND ( 'NONE', #52689, .T. ) ;
#63712=VERTEX_POINT ( 'NONE', #45696 ) ;
#63713=CARTESIAN_POINT ( 'NONE',  ( 15.48076923077065103, -7.500000000000154543, 35.00000000000007105 ) ) ;
#63714=CARTESIAN_POINT ( 'NONE',  ( 3.296024802045256941, -3.300289026998474817, 32.46337939537591666 ) ) ;
#63716=CARTESIAN_POINT ( 'NONE',  ( -11.53846153846153655, -5.557115091759785130, 34.35708131394839171 ) ) ;
#63717=CARTESIAN_POINT ( 'NONE',  ( 4.219914504848592429, -3.050289026998446840, 32.03036669348366416 ) ) ;
#63718=ADVANCED_FACE ( 'NONE', ( #3818 ), #46150, .F. ) ;
#63719=CARTESIAN_POINT ( 'NONE',  ( 4.153846153846154188, -4.098570777380720287, 33.41473453929634729 ) ) ;
#63720=CARTESIAN_POINT ( 'NONE',  ( -7.846153846153965716, -6.879047030192662504, 34.71129190930017927 ) ) ;
#63722=B_SPLINE_CURVE_WITH_KNOTS ( 'NONE', 3,
 ( #52514, #79998, #11095, #25052, #19187, #80454, #12428, #46657, #41564, #38572 ),
 .UNSPECIFIED., .F., .F.,
 ( 4, 2, 2, 2, 4 ),
 ( 0.000000000000000000, 0.0001954311564186867931, 0.0003908623128373735862, 0.0005862934692560603251, 0.0007817246256747473893 ),
 .UNSPECIFIED. ) ;
#63724=EDGE_CURVE ( 'NONE', #25656, #22888, #64581, .T. ) ;
#63725=CARTESIAN_POINT ( 'NONE',  ( -18.22348494372394967, -6.760086850603067354, 34.69517049084099369 ) ) ;
#63726=EDGE_CURVE ( 'NONE', #17306, #879, #28086, .T. ) ;
#63727=CARTESIAN_POINT ( 'NONE',  ( 8.900021210197719412, -3.957578996910242619, 33.62503395064540257 ) ) ;
#63728=CARTESIAN_POINT ( 'NONE',  ( 17.14299142792552288, -3.513871655860379306, 32.76840700105978499 ) ) ;
#63729=CARTESIAN_POINT ( 'NONE',  ( 11.53846153846141753, -4.481592998941358097, 33.73612834414048933 ) ) ;
#63730=CARTESIAN_POINT ( 'NONE',  ( 1.384615384615386802, -11.16473453929635440, 33.15142922261926373 ) ) ;
#63732=CARTESIAN_POINT ( 'NONE',  ( 8.834486340506794377, -2.892918686051625166, 31.69288490824026638 ) ) ;
#63733=CARTESIAN_POINT ( 'NONE',  ( 13.13461538461538325, -7.566082377512564960, 35.00000000000000711 ) ) ;
#63735=EDGE_CURVE ( 'NONE', #58651, #14505, #7664, .T. ) ;
#63739=ORIENTED_EDGE ( 'NONE', *, *, #64682, .F. ) ;
#63741=CARTESIAN_POINT ( 'NONE',  ( 9.469381474791545017, -6.503392248772476236, 34.64988816332204635 ) ) ;
#63743=LINE ( 'NONE', #2044, #2364 ) ;
#63744=CARTESIAN_POINT ( 'NONE',  ( 17.14299041027315695, -2.833524468853757750, 32.15551576947925838 ) ) ;
#63746=CARTESIAN_POINT ( 'NONE',  ( -6.130147209438219669, -11.93770438780619259, 32.05411857736982029 ) ) ;
#63748=CARTESIAN_POINT ( 'NONE',  ( 5.999999999999878320, -6.835583212225970762, 34.95778746994575670 ) ) ;
#63750=DIRECTION ( 'NONE',  ( 0.000000000000000000, 0.000000000000000000, 1.000000000000000000 ) ) ;
#63751=CARTESIAN_POINT ( 'NONE',  ( 18.00000000000000000, -2.292212530054420494, 30.41441678777542634 ) ) ;
#63752=CARTESIAN_POINT ( 'NONE',  ( 15.00728430620490172, -8.539481045369596401, 34.89627647299170832 ) ) ;
#63753=CARTESIAN_POINT ( 'NONE',  ( 11.47319109250076430, -2.892918686051582533, 31.69288490824015980 ) ) ;
#63754=CARTESIAN_POINT ( 'NONE',  ( -13.51530598772569114, -11.93127051446799847, 32.56575433478202797 ) ) ;
#63756=CARTESIAN_POINT ( 'NONE',  ( -9.915233909823841785, -3.586966769969701208, 32.86292498521069660 ) ) ;
#63757=CARTESIAN_POINT ( 'NONE',  ( 10.68145296638705410, -11.16473453929635440, 33.15142922261926373 ) ) ;
#63760=EDGE_CURVE ( 'NONE', #13945, #36896, #76415, .T. ) ;
#63762=ORIENTED_EDGE ( 'NONE', *, *, #46483, .T. ) ;
#63763=LINE ( 'NONE', #300, #2493 ) ;
#63764=CARTESIAN_POINT ( 'NONE',  ( 12.33084785842815378, -8.191372820521381826, 34.95448215188423546 ) ) ;
#63765=CARTESIAN_POINT ( 'NONE',  ( -9.019254006523732770, -11.37209801155882971, 32.91403422569032955 ) ) ;
#63767=CARTESIAN_POINT ( 'NONE',  ( -16.21911659980693443, -10.90142922261923886, 33.41473453929638993 ) ) ;
#63768=CARTESIAN_POINT ( 'NONE',  ( -8.992156986746914882, -8.239355502252617924, 34.69524867566427417 ) ) ;
#63769=VECTOR ( 'NONE', #51331, 1000.000000000000000 ) ;
#63770=EDGE_CURVE ( 'NONE', #5574, #61908, #3337, .T. ) ;
#63771=VECTOR ( 'NONE', #16821, 1000.000000000000227 ) ;
#63772=CARTESIAN_POINT ( 'NONE',  ( -8.769230769230768274, -1.117168528481311540, 33.14645433367849847 ) ) ;
#63773=EDGE_LOOP ( 'NONE', ( #57570, #61234 ) ) ;
#63774=ORIENTED_EDGE ( 'NONE', *, *, #43191, .T. ) ;
#63775=ADVANCED_FACE ( 'NONE', ( #67751 ), #14131, .F. ) ;
#63776=B_SPLINE_CURVE_WITH_KNOTS ( 'NONE', 3,
 ( #15606, #22356, #30442, #23239, #71417, #65101, #30005, #9299, #50700, #79077 ),
 .UNSPECIFIED., .F., .F.,
 ( 4, 2, 2, 2, 4 ),
 ( 0.0007817359430256391132, 0.0009771253907250075990, 0.001172514838424375868, 0.001367904286123744354, 0.001563293733823112840 ),
 .UNSPECIFIED. ) ;
#63777=ORIENTED_EDGE ( 'NONE', *, *, #86960, .T. ) ;
#63779=CARTESIAN_POINT ( 'NONE',  ( -3.230769230769229949, -9.905515769479276145, 34.41647553114623292 ) ) ;
#63780=CARTESIAN_POINT ( 'NONE',  ( -5.076923076923075762, -13.53365097954675988, 30.81389545987213552 ) ) ;
#63781=CARTESIAN_POINT ( 'NONE',  ( -6.066083410955878108, -3.050289026998445951, 32.03036669348365706 ) ) ;
#63782=DIRECTION ( 'NONE',  ( -0.000000000000000000, 1.000000000000000000, 3.491481338843133355E-15 ) ) ;
#63784=EDGE_CURVE ( 'NONE', #74008, #56240, #51328, .T. ) ;
#63785=CARTESIAN_POINT ( 'NONE',  ( 17.07692307692307665, -9.584722331328613620, 36.20867863119891439 ) ) ;
#63786=VERTEX_POINT ( 'NONE', #13687 ) ;
#63787=VERTEX_POINT ( 'NONE', #82158 ) ;
#63788=CARTESIAN_POINT ( 'NONE',  ( -4.153846153846152411, -8.973038597847269315, 34.52809138561121927 ) ) ;
#63789=ORIENTED_EDGE ( 'NONE', *, *, #48060, .F. ) ;
#63791=CARTESIAN_POINT ( 'NONE',  ( -10.61538461538473399, -5.219633306517616589, 34.19971097300220464 ) ) ;
#63794=CARTESIAN_POINT ( 'NONE',  ( -3.230769230769229949, -13.20930481340135110, 34.54067556320372745 ) ) ;
#63795=EDGE_CURVE ( 'NONE', #16341, #72329, #24023, .T. ) ;
#63796=FACE_OUTER_BOUND ( 'NONE', #63902, .T. ) ;
#63797=ORIENTED_EDGE ( 'NONE', *, *, #74221, .T. ) ;
#63798=ORIENTED_EDGE ( 'NONE', *, *, #64812, .T. ) ;
#63800=ORIENTED_EDGE ( 'NONE', *, *, #47975, .T. ) ;
#63801=CARTESIAN_POINT ( 'NONE',  ( -2.084912638714238486, -3.563462043263030399, 33.22394488606062879 ) ) ;
#63802=CARTESIAN_POINT ( 'NONE',  ( 1.134638653673032183, -8.303909089506435137, 34.68538101551103381 ) ) ;
#63803=ORIENTED_EDGE ( 'NONE', *, *, #67069, .T. ) ;
#63805=CYLINDRICAL_SURFACE ( 'NONE', #20172, 0.2500000000000002220 ) ;
#63807=EDGE_LOOP ( 'NONE', ( #44374, #89095 ) ) ;
#63808=EDGE_CURVE ( 'NONE', #78559, #53313, #68630, .T. ) ;
#63809=B_SPLINE_CURVE_WITH_KNOTS ( 'NONE', 3,
 ( #66328, #13492, #40970, #31202, #24439, #51907, #59118, #24889, #73085, #11383 ),
 .UNSPECIFIED., .F., .F.,
 ( 4, 2, 2, 2, 4 ),
 ( 0.000000000000000000, 0.0001954311564186867660, 0.0003908623128373735320, 0.0005862934692560603251, 0.0007817246256747470640 ),
 .UNSPECIFIED. ) ;
#63810=ADVANCED_FACE ( 'NONE', ( #28540 ), #34840, .F. ) ;
#63811=LINE ( 'NONE', #69685, #76739 ) ;
#63812=CARTESIAN_POINT ( 'NONE',  ( 4.854056813859977559, -2.251424796025575770, 29.88072029997477586 ) ) ;
#63813=B_SPLINE_CURVE_WITH_KNOTS ( 'NONE', 3,
 ( #59390, #18410, #66601, #12542, #33260, #67045, #67490, #5784, #73352, #12109 ),
 .UNSPECIFIED., .F., .F.,
 ( 4, 2, 2, 2, 4 ),
 ( 0.0007817246256747452209, 0.0009771112852218887673, 0.001172497944769032531, 0.001367884604316176294, 0.001563271263863319840 ),
 .UNSPECIFIED. ) ;
#63815=FACE_BOUND ( 'NONE', #4538, .T. ) ;
#63816=DIRECTION ( 'NONE',  ( 0.000000000000000000, -1.000000000000000000, 0.000000000000000000 ) ) ;
#63817=CARTESIAN_POINT ( 'NONE',  ( -6.923076923077044142, -2.892918686052165622, 31.69288490824153470 ) ) ;
#63818=B_SPLINE_CURVE_WITH_KNOTS ( 'NONE', 3,
 ( #8595, #57656, #36072, #22541, #2694, #63959, #29750, #57214, #30190, #22979 ),
 .UNSPECIFIED., .F., .F.,
 ( 4, 2, 2, 2, 4 ),
 ( 0.000000000000000000, 0.0001954339857564078809, 0.0003908679715128157619, 0.0005863019572692236428, 0.0007817359430256315238 ),
 .UNSPECIFIED. ) ;
#63819=DIRECTION ( 'NONE',  ( 0.000000000000000000, 0.3420201433256610524, 0.9396926207859113145 ) ) ;
#63820=DIRECTION ( 'NONE',  ( 0.000000000000000000, 0.7660444431189807890, 0.6427876096865361433 ) ) ;
#63821=CARTESIAN_POINT ( 'NONE',  ( -6.673131404728780858, -2.587454068350147462, 30.68340429815432202 ) ) ;
#63822=CARTESIAN_POINT ( 'NONE',  ( -8.769230769230768274, -11.16473453929635440, 33.15142922261926373 ) ) ;
#63823=CARTESIAN_POINT ( 'NONE',  ( -16.02332045208259359, -9.417988943895561960, 34.36773134775778260 ) ) ;
#63825=FACE_OUTER_BOUND ( 'NONE', #72423, .T. ) ;
#63826=CYLINDRICAL_SURFACE ( 'NONE', #78079, 0.2499999999999995559 ) ;
#63828=ORIENTED_EDGE ( 'NONE', *, *, #31634, .F. ) ;
#63829=VECTOR ( 'NONE', #37451, 1000.000000000000114 ) ;
#63830=CARTESIAN_POINT ( 'NONE',  ( -16.15384615384615330, -12.62096338111211580, 30.90682066428153263 ) ) ;
#63831=CARTESIAN_POINT ( 'NONE',  ( -5.076923076923197442, -6.026961402154118908, 34.52809138561165270 ) ) ;
#63832=CARTESIAN_POINT ( 'NONE',  ( 3.480769230769294786, -7.434744429011176159, 34.75000000000000711 ) ) ;
#63833=CARTESIAN_POINT ( 'NONE',  ( 2.177544337960614307, -5.915902021225892149, 34.75552854090298638 ) ) ;
#63834=CARTESIAN_POINT ( 'NONE',  ( -10.36543920600657209, -2.986452184633680229, 32.43230066228895225 ) ) ;
#63836=CARTESIAN_POINT ( 'NONE',  ( -5.076923076923075762, -2.538708090699994813, 30.37095296980875503 ) ) ;
#63837=FACE_BOUND ( 'NONE', #44362, .T. ) ;
#63838=CARTESIAN_POINT ( 'NONE',  ( 11.53846153846153832, -6.343179335718451384, 34.87096338111211935 ) ) ;
#63839=CARTESIAN_POINT ( 'NONE',  ( 1.515407192440171968, -2.541949514083463590, 30.39797389878540557 ) ) ;
#63840=FACE_OUTER_BOUND ( 'NONE', #81315, .T. ) ;
#63841=CARTESIAN_POINT ( 'NONE',  ( -7.846153846153967493, -12.70778746994576025, 30.41441678777401236 ) ) ;
#63842=CARTESIAN_POINT ( 'NONE',  ( -12.59168567097668401, -4.460286881179643004, 33.72017969459903242 ) ) ;
#63843=CARTESIAN_POINT ( 'NONE',  ( 8.899756470994335089, -10.88167719472716399, 33.43325721877153711 ) ) ;
#63845=ORIENTED_EDGE ( 'NONE', *, *, #56806, .F. ) ;
#63846=ORIENTED_EDGE ( 'NONE', *, *, #38194, .T. ) ;
#63847=DIRECTION ( 'NONE',  ( 0.000000000000000000, 0.000000000000000000, -1.000000000000000000 ) ) ;
#63848=CARTESIAN_POINT ( 'NONE',  ( -4.219929564802031408, -3.050289026998445951, 32.03036669348365706 ) ) ;
#63849=CARTESIAN_POINT ( 'NONE',  ( -8.769230769230768274, -12.78798330534102945, 29.74999999999997868 ) ) ;
#63850=CARTESIAN_POINT ( 'NONE',  ( -0.6844654204453105573, -2.889293201056495786, 32.26117774369186009 ) ) ;
#63851=CARTESIAN_POINT ( 'NONE',  ( 3.100622021331013833, -11.47017969459903952, 32.78971311882034456 ) ) ;
#63853=CARTESIAN_POINT ( 'NONE',  ( -8.519285250882631999, -2.824170634883621744, 31.52227843825338738 ) ) ;
#63854=LINE ( 'NONE', #35506, #44544 ) ;
#63855=CARTESIAN_POINT ( 'NONE',  ( 3.296836564119306257, -3.937682226553329556, 33.60647404775216529 ) ) ;
#63856=CARTESIAN_POINT ( 'NONE',  ( -1.634638621908349077, -12.43535235679832596, 30.55408501211184813 ) ) ;
#63857=CARTESIAN_POINT ( 'NONE',  ( -3.480745974817822663, -4.075325502946086864, 33.72974371597207721 ) ) ;
#63858=CYLINDRICAL_SURFACE ( 'NONE', #31017, 0.2499999999999994726 ) ;
#63859=B_SPLINE_CURVE_WITH_KNOTS ( 'NONE', 3,
 ( #85563, #72484, #24745, #11691, #17098, #64827, #58080, #51291, #38263, #72038 ),
 .UNSPECIFIED., .F., .F.,
 ( 4, 2, 2, 2, 4 ),
 ( 0.000000000000000000, 0.0001954339857564071491, 0.0003908679715128142982, 0.0005863019572692214744, 0.0007817359430256285964 ),
 .UNSPECIFIED. ) ;
#63860=VECTOR ( 'NONE', #69126, 1000.000000000000227 ) ;
#63861=CARTESIAN_POINT ( 'NONE',  ( 14.43848411551709709, -11.71459661697925903, 32.44059661609676937 ) ) ;
#63862=LINE ( 'NONE', #85033, #51351 ) ;
#63864=CARTESIAN_POINT ( 'NONE',  ( -7.846153846153844924, -2.249999999999998668, 29.50000000000001421 ) ) ;
#63865=CARTESIAN_POINT ( 'NONE',  ( -5.869209559033048862, -2.494656445102013453, 31.33466734024120015 ) ) ;
#63867=CARTESIAN_POINT ( 'NONE',  ( 0.7114838709165042241, -3.520799739797213945, 33.17531984108286025 ) ) ;
#63868=CARTESIAN_POINT ( 'NONE',  ( -15.93106648486808119, -2.612705202774696200, 31.66806509827799943 ) ) ;
#63869=ORIENTED_EDGE ( 'NONE', *, *, #18055, .T. ) ;
#63870=CARTESIAN_POINT ( 'NONE',  ( -16.37671157604979300, -2.501496062324912284, 29.88072118266895671 ) ) ;
#63871=DIRECTION ( 'NONE',  ( 0.000000000000000000, -6.938893903907222067E-15, 1.000000000000000000 ) ) ;
#63872=ORIENTED_EDGE ( 'NONE', *, *, #18021, .F. ) ;
#63873=CARTESIAN_POINT ( 'NONE',  ( 7.053602624840491053, -3.816742781228458448, 33.13167719472716044 ) ) ;
#63874=FACE_OUTER_BOUND ( 'NONE', #349, .T. ) ;
#63875=ORIENTED_EDGE ( 'NONE', *, *, #75421, .F. ) ;
#63877=CARTESIAN_POINT ( 'NONE',  ( 9.019285080869083870, -4.943051570960394159, 34.04725096376909477 ) ) ;
#63878=ORIENTED_EDGE ( 'NONE', *, *, #81549, .T. ) ;
#63879=CARTESIAN_POINT ( 'NONE',  ( -12.46153846153846168, -2.292212530054420494, 30.41441678777542634 ) ) ;
#63882=EDGE_LOOP ( 'NONE', ( #76115, #50580 ) ) ;
#63883=ORIENTED_EDGE ( 'NONE', *, *, #46475, .T. ) ;
#63885=DIRECTION ( 'NONE',  ( 0.000000000000000000, 0.4999999999999960032, -0.8660254037844410391 ) ) ;
#63886=CARTESIAN_POINT ( 'NONE',  ( 2.372947447205147942, -11.67786785259547777, 32.92929555188713664 ) ) ;
#63888=AXIS2_PLACEMENT_3D ( 'NONE', #52966, #77894, #25509 ) ;
#63889=CARTESIAN_POINT ( 'NONE',  ( -17.30040802064702987, -6.760086850603066466, 34.69517049084099369 ) ) ;
#63890=VERTEX_POINT ( 'NONE', #1509 ) ;
#63891=ORIENTED_EDGE ( 'NONE', *, *, #20694, .F. ) ;
#63894=CARTESIAN_POINT ( 'NONE',  ( 12.71159288145191724, -11.47946981652013498, 33.17500667209847620 ) ) ;
#63895=EDGE_CURVE ( 'NONE', #47746, #221, #79435, .T. ) ;
#63896=VERTEX_POINT ( 'NONE', #44570 ) ;
#63898=CARTESIAN_POINT ( 'NONE',  ( 7.912222197156284054, -4.786620604624113540, 33.94971097300155805 ) ) ;
#63899=ORIENTED_EDGE ( 'NONE', *, *, #73577, .F. ) ;
#63900=ORIENTED_EDGE ( 'NONE', *, *, #37718, .F. ) ;
#63901=CARTESIAN_POINT ( 'NONE',  ( -12.46153846153846168, -4.786620604624113540, 33.94971097300155094 ) ) ;
#63902=EDGE_LOOP ( 'NONE', ( #53925, #84749, #30531, #13299 ) ) ;
#63903=CARTESIAN_POINT ( 'NONE',  ( 4.403791672194294904, -5.057305518903949526, 34.11320923018887896 ) ) ;
#63904=VECTOR ( 'NONE', #46428, 1000.000000000000227 ) ;
#63905=CARTESIAN_POINT ( 'NONE',  ( -5.300408020647026319, -10.11188796281391511, 34.01382737946119050 ) ) ;
#63908=CARTESIAN_POINT ( 'NONE',  ( 15.36156103859402045, -3.062576670634119758, 32.05464942895959979 ) ) ;
#63909=B_SPLINE_CURVE_WITH_KNOTS ( 'NONE', 3,
 ( #55913, #49158, #76640, #1420, #28913, #1862, #63993, #65329, #70322, #2290 ),
 .UNSPECIFIED., .F., .F.,
 ( 4, 2, 2, 2, 4 ),
 ( 0.000000000000000000, 0.0001954339857564076912, 0.0003908679715128153282, 0.0005863019572692228839, 0.0007817359430256304396 ),
 .UNSPECIFIED. ) ;
#63910=CARTESIAN_POINT ( 'NONE',  ( -14.24162497434223162, -12.62096338111211757, 30.90682066428152908 ) ) ;
#63911=CARTESIAN_POINT ( 'NONE',  ( -13.38461538461538325, -13.53365097954675988, 30.81389545987213552 ) ) ;
#63912=FACE_BOUND ( 'NONE', #83203, .T. ) ;
#63913=VECTOR ( 'NONE', #4067, 1000.000000000000000 ) ;
#63914=CARTESIAN_POINT ( 'NONE',  ( -8.546451100252703270, -2.353885683473779800, 30.79025554430704403 ) ) ;
#63915=CARTESIAN_POINT ( 'NONE',  ( -11.66915214157184977, -6.369640206132551441, 34.87707690430378449 ) ) ;
#63917=DIRECTION ( 'NONE',  ( -0.000000000000000000, 1.000000000000000000, 3.491481338843133355E-15 ) ) ;
#63919=CARTESIAN_POINT ( 'NONE',  ( 4.219913487196230939, -2.292212530054420494, 30.41441678777542990 ) ) ;
#63921=CARTESIAN_POINT ( 'NONE',  ( -7.846153846153844924, -11.33034616979429110, 35.88435417666054406 ) ) ;
#63922=ORIENTED_EDGE ( 'NONE', *, *, #66275, .F. ) ;
#63923=DIRECTION ( 'NONE',  ( -0.000000000000000000, -0.9396926207859093161, -0.3420201433256663259 ) ) ;
#63924=ORIENTED_EDGE ( 'NONE', *, *, #51314, .F. ) ;
#63925=VERTEX_POINT ( 'NONE', #42498 ) ;
#63926=CARTESIAN_POINT ( 'NONE',  ( -8.769230769230768274, -8.810774026931790459, 35.74407628777942847 ) ) ;
#63927=CARTESIAN_POINT ( 'NONE',  ( -3.360917200500924906, -5.915902021225892149, 34.75552854090298638 ) ) ;
#63928=CARTESIAN_POINT ( 'NONE',  ( 2.307692307692187583, -2.625532179533779154, 30.86335684631627174 ) ) ;
#63929=CARTESIAN_POINT ( 'NONE',  ( 8.069166690247241647, -3.395485233115139057, 33.02377354290275946 ) ) ;
#63930=CARTESIAN_POINT ( 'NONE',  ( -12.23875879256039667, -2.612705202774698421, 31.66806509827799943 ) ) ;
#63931=LINE ( 'NONE', #58494, #1577 ) ;
#63932=EDGE_LOOP ( 'NONE', ( #78668, #6625 ) ) ;
#63934=FACE_OUTER_BOUND ( 'NONE', #34431, .T. ) ;
#63935=CARTESIAN_POINT ( 'NONE',  ( -15.23076923076922995, -9.780366693483667717, 34.19971097300155094 ) ) ;
#63936=DIRECTION ( 'NONE',  ( 1.000000000000000000, 0.000000000000000000, 0.000000000000000000 ) ) ;
#63937=CARTESIAN_POINT ( 'NONE',  ( 15.23076923076923173, -12.34228464037088635, 31.77849191805839268 ) ) ;
#63938=DIRECTION ( 'NONE',  ( 0.000000000000000000, -6.938893903907222067E-15, 1.000000000000000000 ) ) ;
#63940=ORIENTED_EDGE ( 'NONE', *, *, #63808, .F. ) ;
#63941=EDGE_CURVE ( 'NONE', #57554, #52054, #47197, .T. ) ;
#63942=ORIENTED_EDGE ( 'NONE', *, *, #17477, .T. ) ;
#63943=EDGE_CURVE ( 'NONE', #45833, #71793, #11812, .T. ) ;
#63944=CARTESIAN_POINT ( 'NONE',  ( -6.222926958906846551, -4.026226216239095379, 33.68668979543632958 ) ) ;
#63945=VERTEX_POINT ( 'NONE', #24308 ) ;
#63946=FACE_OUTER_BOUND ( 'NONE', #29017, .T. ) ;
#63947=LINE ( 'NONE', #45453, #3974 ) ;
#63949=CARTESIAN_POINT ( 'NONE',  ( -4.853910232829680815, -3.395485233115139057, 33.02377354290275946 ) ) ;
#63951=CARTESIAN_POINT ( 'NONE',  ( 0.5920638997721058283, -9.503571793651733657, 34.60286762892837942 ) ) ;
#63952=AXIS2_PLACEMENT_3D ( 'NONE', #40933, #12137, #12575 ) ;
#63953=ORIENTED_EDGE ( 'NONE', *, *, #63207, .T. ) ;
#63954=CARTESIAN_POINT ( 'NONE',  ( -12.71151519248081563, -10.66389620160130036, 33.62221079203477103 ) ) ;
#63955=CARTESIAN_POINT ( 'NONE',  ( -2.176900499867520544, -10.54018710029568595, 33.71981072465678864 ) ) ;
#63956=VERTEX_POINT ( 'NONE', #50881 ) ;
#63957=CARTESIAN_POINT ( 'NONE',  ( 3.164686851409094004, -12.34228464037088280, 31.77849191805838558 ) ) ;
#63958=CARTESIAN_POINT ( 'NONE',  ( -17.14300545628321615, -11.91647553114624181, 32.58852847137148245 ) ) ;
#63959=CARTESIAN_POINT ( 'NONE',  ( 11.28843830116857383, -4.335965774309649134, 33.62209801155881905 ) ) ;
#63960=DIRECTION ( 'NONE',  ( 0.000000000000000000, 0.9848077530122072432, 0.1736481776669354937 ) ) ;
#63961=DIRECTION ( 'NONE',  ( 0.000000000000000000, 0.9396926207859126468, 0.3420201433256571111 ) ) ;
#63962=CARTESIAN_POINT ( 'NONE',  ( -6.988347369037697376, -5.219633306516282545, 34.19971097300152252 ) ) ;
#63964=EDGE_LOOP ( 'NONE', ( #29495, #66379 ) ) ;
#63965=CARTESIAN_POINT ( 'NONE',  ( -12.46153846153846168, -13.87047571288749737, 32.06866353760679544 ) ) ;
#63966=CARTESIAN_POINT ( 'NONE',  ( -1.608100328339334029, -12.24155766932282496, 31.33739205006857986 ) ) ;
#63968=CARTESIAN_POINT ( 'NONE',  ( -3.454254174493178731, -9.331801661448606566, 34.40259984581193464 ) ) ;
#63969=CARTESIAN_POINT ( 'NONE',  ( 9.562159722575998444, -6.809168938359901446, 34.95455904226513866 ) ) ;
#63970=ORIENTED_EDGE ( 'NONE', *, *, #18021, .T. ) ;
#63972=LINE ( 'NONE', #14926, #21055 ) ;
#63973=ORIENTED_EDGE ( 'NONE', *, *, #37752, .T. ) ;
#63974=CARTESIAN_POINT ( 'NONE',  ( -18.00000000000012079, -5.094484230521992174, 34.41647553114689373 ) ) ;
#63975=EDGE_LOOP ( 'NONE', ( #33476, #64377, #50544, #33846 ) ) ;
#63977=CARTESIAN_POINT ( 'NONE',  ( 17.74997676270703550, -6.695914987888146541, 34.68535235679833306 ) ) ;
#63978=CARTESIAN_POINT ( 'NONE',  ( -17.32694630114453105, -2.341070481393820124, 30.72580821765574299 ) ) ;
#63979=AXIS2_PLACEMENT_3D ( 'NONE', #49430, #62482, #84114 ) ;
#63980=CARTESIAN_POINT ( 'NONE',  ( -8.769230769230892619, -5.941354392335915335, 34.76329471203413846 ) ) ;
#63982=ORIENTED_EDGE ( 'NONE', *, *, #76449, .F. ) ;
#63983=CARTESIAN_POINT ( 'NONE',  ( -3.230769230769229949, -2.292212530054420494, 30.41441678777542634 ) ) ;
#63984=B_SPLINE_CURVE_WITH_KNOTS ( 'NONE', 3,
 ( #18007, #50443, #16657, #58088, #23846, #51299, #70733, #57212, #31055, #9036 ),
 .UNSPECIFIED., .F., .F.,
 ( 4, 2, 2, 2, 4 ),
 ( 0.000000000000000000, 0.0001954339857564063089, 0.0003908679715128126177, 0.0005863019572692189808, 0.0007817359430256252354 ),
 .UNSPECIFIED. ) ;
#63985=AXIS2_PLACEMENT_3D ( 'NONE', #42814, #8583, #49993 ) ;
#63986=EDGE_LOOP ( 'NONE', ( #70717, #35471, #35539, #79406 ) ) ;
#63988=CARTESIAN_POINT ( 'NONE',  ( 4.826946332874483936, -5.643011162660950042, 34.66104346484419096 ) ) ;
#63989=ORIENTED_EDGE ( 'NONE', *, *, #30188, .T. ) ;
#63990=AXIS2_PLACEMENT_3D ( 'NONE', #73576, #24471, #38898 ) ;
#63991=CARTESIAN_POINT ( 'NONE',  ( 11.66898697669518548, -12.70449254468099198, 30.44128974285582956 ) ) ;
#63993=CARTESIAN_POINT ( 'NONE',  ( 0.2380535178145126718, -4.386631170607604879, 33.66268669641500111 ) ) ;
#63994=ADVANCED_FACE ( 'NONE', ( #65300 ), #52226, .F. ) ;
#63995=CYLINDRICAL_SURFACE ( 'NONE', #52034, 0.2500000000000008882 ) ;
#63996=CARTESIAN_POINT ( 'NONE',  ( -4.826923076921640465, -7.500000000000155431, 34.75000000000007105 ) ) ;
#63998=EDGE_LOOP ( 'NONE', ( #47520, #6638 ) ) ;
#63999=FACE_BOUND ( 'NONE', #44750, .T. ) ;
#64000=ORIENTED_EDGE ( 'NONE', *, *, #4410, .T. ) ;
#64001=CARTESIAN_POINT ( 'NONE',  ( 6.923076923076924238, -6.189225973068211317, 35.74407628777942847 ) ) ;
#64002=EDGE_CURVE ( 'NONE', #37932, #38304, #64423, .T. ) ;
#64003=DIRECTION ( 'NONE',  ( 0.000000000000000000, 0.9848077530122072432, 0.1736481776669354937 ) ) ;
#64004=DIRECTION ( 'NONE',  ( 0.000000000000000000, 0.4999999999999960032, -0.8660254037844410391 ) ) ;
#64006=EDGE_CURVE ( 'NONE', #65220, #30240, #29773, .T. ) ;
#64007=ORIENTED_EDGE ( 'NONE', *, *, #47267, .F. ) ;
#64009=VERTEX_POINT ( 'NONE', #52673 ) ;
#64010=CARTESIAN_POINT ( 'NONE',  ( 16.85343813319912698, -4.386631170607603991, 33.66268669641500111 ) ) ;
#64011=VERTEX_POINT ( 'NONE', #4948 ) ;
#64013=B_SPLINE_CURVE_WITH_KNOTS ( 'NONE', 3,
 ( #68665, #61455, #88966, #48388, #54700, #1096 ),
 .UNSPECIFIED., .F., .F.,
 ( 4, 2, 4 ),
 ( 0.000000000000000000, 0.2500000000000000000, 0.5000000000000000000 ),
 .UNSPECIFIED. ) ;
#64015=CARTESIAN_POINT ( 'NONE',  ( 2.980792499826877773, -2.779195860258149242, 31.39871582349837453 ) ) ;
#64016=DIRECTION ( 'NONE',  ( -0.000000000000000000, 0.7660444431189791237, -0.6427876096865379196 ) ) ;
#64017=CARTESIAN_POINT ( 'NONE',  ( 9.692307692307695177, -1.129524287112498415, 32.06866353760679544 ) ) ;
#64018=VERTEX_POINT ( 'NONE', #81058 ) ;
#64019=CARTESIAN_POINT ( 'NONE',  ( 8.835299120233205628, -8.973038597847271092, 34.52809138561121216 ) ) ;
#64020=EDGE_CURVE ( 'NONE', #57330, #5010, #32413, .T. ) ;
#64021=CARTESIAN_POINT ( 'NONE',  ( -5.999999999999998224, -6.343179335718451384, 34.87096338111211935 ) ) ;
#64022=CYLINDRICAL_SURFACE ( 'NONE', #4919, 0.2500000000000008882 ) ;
#64023=CARTESIAN_POINT ( 'NONE',  ( 8.899756207464411872, -6.808710257144161559, 34.95449254468098843 ) ) ;
#64024=ORIENTED_EDGE ( 'NONE', *, *, #66590, .T. ) ;
#64025=EDGE_CURVE ( 'NONE', #55155, #20155, #71928, .T. ) ;
#64026=VERTEX_POINT ( 'NONE', #67091 ) ;
#64027=VERTEX_POINT ( 'NONE', #88274 ) ;
#64029=CARTESIAN_POINT ( 'NONE',  ( 10.48523664565292002, -2.373036134822904319, 30.88089517874952250 ) ) ;
#64030=CARTESIAN_POINT ( 'NONE',  ( -15.90384615384615330, -7.500000000000001776, 35.04278698407183867 ) ) ;
#64031=CARTESIAN_POINT ( 'NONE',  ( 12.59232890250541281, -12.62708834333097663, 30.88030960425257021 ) ) ;
#64032=FACE_BOUND ( 'NONE', #44645, .T. ) ;
#64033=CARTESIAN_POINT ( 'NONE',  ( -15.29685161012936412, -3.322132147404559532, 32.92929555188719348 ) ) ;
#64034=ORIENTED_EDGE ( 'NONE', *, *, #30257, .T. ) ;
#64036=EDGE_CURVE ( 'NONE', #40036, #10299, #66644, .T. ) ;
#64037=CARTESIAN_POINT ( 'NONE',  ( -3.099977422944443450, -2.541949514083463590, 30.39797389878540557 ) ) ;
#64038=CARTESIAN_POINT ( 'NONE',  ( 9.442330948259105128, -12.01397095200674059, 32.43157075238190146 ) ) ;
#64039=CARTESIAN_POINT ( 'NONE',  ( -17.07692307692319744, -11.94971097300221174, 32.03036669348237098 ) ) ;
#64040=CARTESIAN_POINT ( 'NONE',  ( -11.47239318745910097, -3.513871655860379306, 32.76840700105978499 ) ) ;
#64041=ORIENTED_EDGE ( 'NONE', *, *, #10368, .T. ) ;
#64042=CARTESIAN_POINT ( 'NONE',  ( 2.307692307692309264, -11.69971097300155272, 32.46337939537588113 ) ) ;
#64043=ORIENTED_EDGE ( 'NONE', *, *, #48885, .T. ) ;
#64044=FACE_BOUND ( 'NONE', #52859, .T. ) ;
#64045=CARTESIAN_POINT ( 'NONE',  ( 11.53846153846153832, -2.833524468853757305, 32.15551576947925838 ) ) ;
#64046=B_SPLINE_CURVE_WITH_KNOTS ( 'NONE', 3,
 ( #48996, #48539, #69712, #9351, #28277, #36808, #2133, #56200, #8464, #29621 ),
 .UNSPECIFIED., .F., .F.,
 ( 4, 2, 2, 2, 4 ),
 ( 0.000000000000000000, 0.0001954311564186867931, 0.0003908623128373735862, 0.0005862934692560603251, 0.0007817246256747471724 ),
 .UNSPECIFIED. ) ;
#64047=ADVANCED_FACE ( 'NONE', ( #75183 ), #40080, .F. ) ;
#64048=CARTESIAN_POINT ( 'NONE',  ( 4.153846153846030731, -2.657715359629662988, 31.77849191805970364 ) ) ;
#64049=CARTESIAN_POINT ( 'NONE',  ( 14.24242186173153257, -11.94971097300153140, 32.03036669348370680 ) ) ;
#64050=EDGE_CURVE ( 'NONE', #54951, #13992, #42913, .T. ) ;
#64051=B_SPLINE_CURVE_WITH_KNOTS ( 'NONE', 3,
 ( #2135, #71041, #57966, #57524, #9353, #72364, #57080, #65599, #84575, #77795 ),
 .UNSPECIFIED., .F., .F.,
 ( 4, 2, 2, 2, 4 ),
 ( 0.000000000000000000, 0.0001954311564186868473, 0.0003908623128373736946, 0.0005862934692560605419, 0.0007817246256747473893 ),
 .UNSPECIFIED. ) ;
#64052=ORIENTED_EDGE ( 'NONE', *, *, #11293, .F. ) ;
#64054=B_SPLINE_CURVE_WITH_KNOTS ( 'NONE', 3,
 ( #47380, #7292, #40203, #26670, #68541, #53697, #55034, #19032, #40642, #48264 ),
 .UNSPECIFIED., .F., .F.,
 ( 4, 2, 2, 2, 4 ),
 ( 0.0007817246256747473893, 0.0009771112852218909357, 0.001172497944769034482, 0.001367884604316178246, 0.001563271263863321792 ),
 .UNSPECIFIED. ) ;
#64055=CARTESIAN_POINT ( 'NONE',  ( 5.207714884747860928, -3.062576670634119758, 32.05464942895959979 ) ) ;
#64056=CARTESIAN_POINT ( 'NONE',  ( 4.826923076923077538, -7.433931650972300353, 34.75000000000000711 ) ) ;
#64057=CARTESIAN_POINT ( 'NONE',  ( -10.61538461538473399, -3.835265460704628371, 33.15142922262033665 ) ) ;
#64058=CARTESIAN_POINT ( 'NONE',  ( -6.923076923076922462, -3.050289026998446396, 32.03036669348365706 ) ) ;
#64059=ORIENTED_EDGE ( 'NONE', *, *, #55926, .T. ) ;
#64060=FACE_OUTER_BOUND ( 'NONE', #39163, .T. ) ;
#64061=ORIENTED_EDGE ( 'NONE', *, *, #19183, .T. ) ;
#64062=CARTESIAN_POINT ( 'NONE',  ( 13.60739492588379385, -12.24180327182771855, 31.33663988360758879 ) ) ;
#64063=EDGE_LOOP ( 'NONE', ( #2354, #83731, #74788, #13369 ) ) ;
#64064=CARTESIAN_POINT ( 'NONE',  ( 3.296837581771671299, -2.538708090699994813, 30.37095296980875503 ) ) ;
#64065=CARTESIAN_POINT ( 'NONE',  ( -6.857821351800897247, -11.94971097300157403, 32.03036669348361443 ) ) ;
#64066=CARTESIAN_POINT ( 'NONE',  ( 13.25446817517716980, -9.418419913701741919, 34.36755862841477693 ) ) ;
#64067=FACE_OUTER_BOUND ( 'NONE', #38470, .T. ) ;
#64068=CYLINDRICAL_SURFACE ( 'NONE', #60585, 0.2499999999999986955 ) ;
#64069=CARTESIAN_POINT ( 'NONE',  ( 11.53846153846141753, -8.613356846316285953, 34.62446782046622218 ) ) ;
#64070=LINE ( 'NONE', #65403, #44952 ) ;
#64072=ORIENTED_EDGE ( 'NONE', *, *, #87775, .F. ) ;
#64073=DIRECTION ( 'NONE',  ( 0.000000000000000000, 0.3420201433256641055, -0.9396926207859100932 ) ) ;
#64074=LINE ( 'NONE', #10021, #43839 ) ;
#64075=VERTEX_POINT ( 'NONE', #26101 ) ;
#64076=EDGE_LOOP ( 'NONE', ( #13782, #69349, #84951, #45340, #83981, #37443 ) ) ;
#64077=ORIENTED_EDGE ( 'NONE', *, *, #28038, .F. ) ;
#64078=CARTESIAN_POINT ( 'NONE',  ( -10.68146802634049308, -11.16473453929635440, 33.15142922261925662 ) ) ;
#64079=CARTESIAN_POINT ( 'NONE',  ( 3.007843013253082454, -9.886141570436013382, 34.14413921362392301 ) ) ;
#64080=AXIS2_PLACEMENT_3D ( 'NONE', #73646, #10151, #79503 ) ;
#64081=CARTESIAN_POINT ( 'NONE',  ( 0.3309288063343787667, -7.722926974430166069, 34.99546784045485737 ) ) ;
#64082=CARTESIAN_POINT ( 'NONE',  ( 10.86543903529806876, -6.523592122091592671, 34.90882529074906415 ) ) ;
#64083=CARTESIAN_POINT ( 'NONE',  ( -16.40382288478850725, -3.137211980971222225, 32.19342716148376837 ) ) ;
#64084=DIRECTION ( 'NONE',  ( -0.000000000000000000, 0.5000000000000011102, -0.8660254037844381525 ) ) ;
#64085=DIRECTION ( 'NONE',  ( -1.000000000000000000, 0.000000000000000000, 0.000000000000000000 ) ) ;
#64086=ORIENTED_EDGE ( 'NONE', *, *, #69152, .F. ) ;
#64087=EDGE_CURVE ( 'NONE', #10994, #84179, #46371, .T. ) ;
#64090=B_SPLINE_CURVE_WITH_KNOTS ( 'NONE', 3,
 ( #52631, #11665, #31934, #45426, #18859, #39141, #67495, #11210, #80576, #4909 ),
 .UNSPECIFIED., .F., .F.,
 ( 4, 2, 2, 2, 4 ),
 ( 0.0007817246256747434861, 0.0009771112852218861652, 0.001172497944769028844, 0.001367884604316171740, 0.001563271263863314419 ),
 .UNSPECIFIED. ) ;
#64091=CYLINDRICAL_SURFACE ( 'NONE', #78104, 0.2499999999999997502 ) ;
#64092=EDGE_CURVE ( 'NONE', #67350, #64228, #74291, .T. ) ;
#64093=ORIENTED_EDGE ( 'NONE', *, *, #22035, .T. ) ;
#64095=B_SPLINE_CURVE_WITH_KNOTS ( 'NONE', 3,
 ( #78001, #56407, #22180, #2330, #28493, #77561, #42899, #15428, #1901, #84779 ),
 .UNSPECIFIED., .F., .F.,
 ( 4, 2, 2, 2, 4 ),
 ( 0.0007817246256747455461, 0.0009771112852218883336, 0.001172497944769031230, 0.001367884604316174126, 0.001563271263863317022 ),
 .UNSPECIFIED. ) ;
#64096=EDGE_CURVE ( 'NONE', #15414, #67575, #56928, .T. ) ;
#64097=EDGE_CURVE ( 'NONE', #21125, #81602, #81945, .T. ) ;
#64098=EDGE_LOOP ( 'NONE', ( #10523, #43376 ) ) ;
#64099=CARTESIAN_POINT ( 'NONE',  ( 12.39545608217832395, -9.058645607665454236, 34.76329471203372634 ) ) ;
#64100=CARTESIAN_POINT ( 'NONE',  ( 3.361559671736181976, -10.70102852606553157, 33.91149625220312913 ) ) ;
#64101=DIRECTION ( 'NONE',  ( 0.000000000000000000, 0.1736481776669267785, -0.9848077530122087975 ) ) ;
#64102=ORIENTED_EDGE ( 'NONE', *, *, #17589, .T. ) ;
#64103=CARTESIAN_POINT ( 'NONE',  ( 12.68431813051652668, -10.97394488606064122, 33.68653795673694873 ) ) ;
#64105=EDGE_CURVE ( 'NONE', #25692, #7689, #49454, .T. ) ;
#64106=CARTESIAN_POINT ( 'NONE',  ( -3.100243529005665355, -12.27024696741798770, 31.24895572276497546 ) ) ;
#64107=EDGE_LOOP ( 'NONE', ( #86746, #70053 ) ) ;
#64109=EDGE_LOOP ( 'NONE', ( #64043, #55488 ) ) ;
#64111=CARTESIAN_POINT ( 'NONE',  ( 7.053867364043877153, -2.845873456487966635, 32.17976146951972538 ) ) ;
#64112=CARTESIAN_POINT ( 'NONE',  ( -5.999999999999998224, -2.538708090699994813, 30.37095296980875503 ) ) ;
#64113=FACE_OUTER_BOUND ( 'NONE', #57125, .T. ) ;
#64114=CARTESIAN_POINT ( 'NONE',  ( -17.86920955903305597, -12.35292014791297710, 31.75344720912887198 ) ) ;
#64115=EDGE_CURVE ( 'NONE', #45555, #42060, #45134, .T. ) ;
#64117=VERTEX_POINT ( 'NONE', #56668 ) ;
#64118=ORIENTED_EDGE ( 'NONE', *, *, #58552, .T. ) ;
#64120=FACE_OUTER_BOUND ( 'NONE', #30103, .T. ) ;
#64121=CARTESIAN_POINT ( 'NONE',  ( -4.403869378067610363, -12.45566812827425096, 31.48439005359158926 ) ) ;
#64123=VECTOR ( 'NONE', #66636, 1000.000000000000114 ) ;
#64124=FACE_OUTER_BOUND ( 'NONE', #30459, .T. ) ;
#64125=CARTESIAN_POINT ( 'NONE',  ( 8.769230769230768274, -11.33034616979429110, 35.88435417666054406 ) ) ;
#64126=ORIENTED_EDGE ( 'NONE', *, *, #67277, .F. ) ;
#64128=AXIS2_PLACEMENT_3D ( 'NONE', #61008, #26782, #81737 ) ;
#64129=EDGE_LOOP ( 'NONE', ( #33191, #11069 ) ) ;
#64130=CARTESIAN_POINT ( 'NONE',  ( 11.53846153846141753, -9.442884908241554243, 34.35708131394783038 ) ) ;
#64131=ORIENTED_EDGE ( 'NONE', *, *, #12709, .T. ) ;
#64132=CARTESIAN_POINT ( 'NONE',  ( -6.000000000000121680, -12.70778746994576025, 30.41441678777401236 ) ) ;
#64133=CARTESIAN_POINT ( 'NONE',  ( -5.207071046654772495, -12.70455904226513866, 30.44083106164009322 ) ) ;
#64134=CARTESIAN_POINT ( 'NONE',  ( 13.60762673622823549, -8.239487800360276282, 34.69522927552633718 ) ) ;
#64135=EDGE_LOOP ( 'NONE', ( #32471, #86064, #44619, #1094 ) ) ;
#64136=EDGE_CURVE ( 'NONE', #73637, #20256, #17222, .T. ) ;
#64137=ADVANCED_FACE ( 'NONE', ( #41389 ), #62525, .F. ) ;
#64138=ORIENTED_EDGE ( 'NONE', *, *, #48045, .T. ) ;
#64139=CARTESIAN_POINT ( 'NONE',  ( 4.826923076923076650, -7.500000000000001776, 35.00000000000000000 ) ) ;
#64140=ORIENTED_EDGE ( 'NONE', *, *, #84118, .F. ) ;
#64142=FACE_BOUND ( 'NONE', #35184, .T. ) ;
#64143=CARTESIAN_POINT ( 'NONE',  ( 3.453548899747295842, -2.612705202774697533, 31.66806509827799943 ) ) ;
#64144=CARTESIAN_POINT ( 'NONE',  ( -3.903791842207839480, -11.79725096376909654, 32.30694842903960762 ) ) ;
#64145=EDGE_LOOP ( 'NONE', ( #13777, #61918 ) ) ;
#64146=CARTESIAN_POINT ( 'NONE',  ( -14.17716686945866122, -8.630441415882550871, 34.87705825610312615 ) ) ;
#64147=DIRECTION ( 'NONE',  ( 0.000000000000000000, 0.8660254037844377084, -0.5000000000000015543 ) ) ;
#64148=EDGE_CURVE ( 'NONE', #78555, #44484, #22475, .T. ) ;
#64149=CARTESIAN_POINT ( 'NONE',  ( 1.318533005255251744, -3.322132147404559976, 32.92929555188719348 ) ) ;
#64150=CARTESIAN_POINT ( 'NONE',  ( -11.66860874789975888, -6.001485441113819874, 34.52039167877662607 ) ) ;
#64151=CARTESIAN_POINT ( 'NONE',  ( -13.31854703361294590, -11.69971097300155272, 32.46337939537588113 ) ) ;
#64152=CARTESIAN_POINT ( 'NONE',  ( -6.700297381808512753, -9.332535724633407526, 34.40230450496446224 ) ) ;
#64153=EDGE_CURVE ( 'NONE', #22567, #70591, #75133, .T. ) ;
#64154=CARTESIAN_POINT ( 'NONE',  ( -15.23076923076922995, -5.557115091759785130, 34.35708131394839171 ) ) ;
#64156=CARTESIAN_POINT ( 'NONE',  ( -6.130691466667558487, -5.582088688514999397, 34.36776431015576350 ) ) ;
#64158=CYLINDRICAL_SURFACE ( 'NONE', #31522, 0.2499999999999998890 ) ;
#64159=VECTOR ( 'NONE', #35730, 1000.000000000000114 ) ;
#64160=CARTESIAN_POINT ( 'NONE',  ( -13.16183571563731824, -12.47679350104403007, 31.42216943046555855 ) ) ;
#64161=CARTESIAN_POINT ( 'NONE',  ( -17.07692307692307665, -3.937682226553329556, 33.60647404775216529 ) ) ;
#64163=CARTESIAN_POINT ( 'NONE',  ( -1.134669975237340367, -9.357781135181031829, 34.66075350412533851 ) ) ;
#64164=CYLINDRICAL_SURFACE ( 'NONE', #77456, 0.2499999999999973355 ) ;
#64165=CARTESIAN_POINT ( 'NONE',  ( -18.00000000000012079, -3.083524468854528244, 32.58852847137268327 ) ) ;
#64167=CARTESIAN_POINT ( 'NONE',  ( -2.372962308248625529, -5.941354392334500467, 34.76329471203369792 ) ) ;
#64169=ORIENTED_EDGE ( 'NONE', *, *, #22877, .F. ) ;
#64170=CARTESIAN_POINT ( 'NONE',  ( 18.25005431163831560, -11.79725096376909299, 32.30694842903960762 ) ) ;
#64171=ORIENTED_EDGE ( 'NONE', *, *, #43484, .T. ) ;
#64172=CARTESIAN_POINT ( 'NONE',  ( -2.373774687052442545, -2.833524468853757305, 32.15551576947924417 ) ) ;
#64173=EDGE_CURVE ( 'NONE', #1510, #47623, #3175, .T. ) ;
#64174=ORIENTED_EDGE ( 'NONE', *, *, #47625, .F. ) ;
#64175=CARTESIAN_POINT ( 'NONE',  ( -13.16183571563731647, -2.353885683473779800, 30.79025554430704403 ) ) ;
#64176=ORIENTED_EDGE ( 'NONE', *, *, #75872, .T. ) ;
#64177=CARTESIAN_POINT ( 'NONE',  ( -6.065270445960775803, -11.94971097300153140, 32.03036669348370680 ) ) ;
#64179=CARTESIAN_POINT ( 'NONE',  ( -6.000000000000119904, -4.481592998941358097, 33.73612834414048933 ) ) ;
#64180=CARTESIAN_POINT ( 'NONE',  ( -3.007756386675836779, -12.38742843783360748, 31.66772728687926985 ) ) ;
#64181=CARTESIAN_POINT ( 'NONE',  ( 6.923076923076924238, -8.973038597847269315, 34.52809138561121927 ) ) ;
#64182=DIRECTION ( 'NONE',  ( 0.000000000000000000, 0.1736481776669275834, 0.9848077530122086864 ) ) ;
#64184=CARTESIAN_POINT ( 'NONE',  ( -13.44988538517170440, -12.16647553114622049, 32.15551576947930812 ) ) ;
#64188=CARTESIAN_POINT ( 'NONE',  ( -2.084679463598912097, -11.98016756924214832, 32.48728574198911190 ) ) ;
#64189=CARTESIAN_POINT ( 'NONE',  ( -23.00000000000000000, -7.500000000000000000, 29.75000000000000355 ) ) ;
#64191=EDGE_CURVE ( 'NONE', #4986, #74135, #85471, .T. ) ;
#64192=CARTESIAN_POINT ( 'NONE',  ( -10.36533019547115941, -5.642605341092957971, 34.66089969410670335 ) ) ;
#64193=ORIENTED_EDGE ( 'NONE', *, *, #67377, .F. ) ;
#64194=AXIS2_PLACEMENT_3D ( 'NONE', #28777, #14821, #28318 ) ;
#64195=FACE_OUTER_BOUND ( 'NONE', #51815, .T. ) ;
#64196=CARTESIAN_POINT ( 'NONE',  ( 16.02369894440793274, -12.27039167877662251, 31.24851455888617835 ) ) ;
#64197=CARTESIAN_POINT ( 'NONE',  ( 1.161689167099238418, -12.39988816332205701, 30.74660775122750778 ) ) ;
#64198=DIRECTION ( 'NONE',  ( -0.000000000000000000, -0.000000000000000000, -1.000000000000000000 ) ) ;
#64199=CARTESIAN_POINT ( 'NONE',  ( -1.384615384615383471, -10.51840700105979565, 33.73612834413961536 ) ) ;
#64200=VECTOR ( 'NONE', #69873, 1000.000000000000227 ) ;
#64201=CARTESIAN_POINT ( 'NONE',  ( -8.769230769230768274, -8.120952969808772792, 34.71129190930000163 ) ) ;
#64202=ADVANCED_FACE ( 'NONE', ( #84602 ), #11140, .F. ) ;
#64204=EDGE_CURVE ( 'NONE', #42820, #51792, #79158, .T. ) ;
#64205=VECTOR ( 'NONE', #21641, 1000.000000000000227 ) ;
#64206=EDGE_LOOP ( 'NONE', ( #28014, #88560, #45021, #44055 ) ) ;
#64207=CARTESIAN_POINT ( 'NONE',  ( -10.74599427058869416, -7.722926974430166069, 34.99546784045485737 ) ) ;
#64208=VERTEX_POINT ( 'NONE', #44028 ) ;
#64209=EDGE_LOOP ( 'NONE', ( #44338, #15779, #49149, #64565 ) ) ;
#64210=B_SPLINE_CURVE_WITH_KNOTS ( 'NONE', 3,
 ( #4688, #80354, #33492, #81239, #81682, #39371, #87566, #4234, #31717, #60951 ),
 .UNSPECIFIED., .F., .F.,
 ( 4, 2, 2, 2, 4 ),
 ( 0.0007817246256747504250, 0.0009771112852218954894, 0.001172497944769040554, 0.001367884604316185401, 0.001563271263863330466 ),
 .UNSPECIFIED. ) ;
#64211=CARTESIAN_POINT ( 'NONE',  ( -5.999999999999998224, -12.62096338111211580, 30.90682066428153263 ) ) ;
#64212=CARTESIAN_POINT ( 'NONE',  ( 16.21910172512217940, -2.892918686051626498, 31.69288490824026638 ) ) ;
#64213=B_SPLINE_CURVE_WITH_KNOTS ( 'NONE', 3,
 ( #24003, #81527, #74768, #80189, #18490, #45944, #73435, #39210, #4974, #32441 ),
 .UNSPECIFIED., .F., .F.,
 ( 4, 2, 2, 2, 4 ),
 ( 0.0007817359430256297891, 0.0009771253907249958896, 0.001172514838424361990, 0.001367904286123728091, 0.001563293733823094191 ),
 .UNSPECIFIED. ) ;
#64214=CARTESIAN_POINT ( 'NONE',  ( -13.16160403300253279, -9.086983370893049639, 34.49168942202179267 ) ) ;
#64215=CARTESIAN_POINT ( 'NONE',  ( 17.74997676270703550, -9.271318131107980420, 34.42618302367067429 ) ) ;
#64216=EDGE_CURVE ( 'NONE', #22286, #79691, #44461, .T. ) ;
#64217=VERTEX_POINT ( 'NONE', #44915 ) ;
#64219=CARTESIAN_POINT ( 'NONE',  ( -6.673131404728780858, -5.852078868378311149, 34.47109172314383585 ) ) ;
#64221=AXIS2_PLACEMENT_3D ( 'NONE', #29970, #16013, #8817 ) ;
#64222=VERTEX_POINT ( 'NONE', #78713 ) ;
#64223=FACE_OUTER_BOUND ( 'NONE', #6839, .T. ) ;
#64225=CARTESIAN_POINT ( 'NONE',  ( -16.15384615384615330, -4.098570777380720287, 33.41473453929634729 ) ) ;
#64226=CARTESIAN_POINT ( 'NONE',  ( 2.177131715950388458, -2.504760397472875155, 29.97295953869789997 ) ) ;
#64227=CARTESIAN_POINT ( 'NONE',  ( 3.230769230769231726, -6.386643153685126251, 34.62446782046654192 ) ) ;
#64228=VERTEX_POINT ( 'NONE', #63864 ) ;
#64231=VERTEX_POINT ( 'NONE', #57108 ) ;
#64232=CARTESIAN_POINT ( 'NONE',  ( 4.403791672194295792, -11.37275283266503756, 32.91324779482534524 ) ) ;
#64233=ORIENTED_EDGE ( 'NONE', *, *, #23436, .T. ) ;
#64236=CARTESIAN_POINT ( 'NONE',  ( 9.692307692307695177, -4.945431358278436385, 36.03766855953609394 ) ) ;
#64237=EDGE_LOOP ( 'NONE', ( #56265, #59604, #51995, #71309 ) ) ;
#64238=B_SPLINE_CURVE_WITH_KNOTS ( 'NONE', 3,
 ( #24119, #38089, #59693, #38996, #46187, #11964, #45734, #72311, #39441, #80875 ),
 .UNSPECIFIED., .F., .F.,
 ( 4, 2, 2, 2, 4 ),
 ( 0.0007817359430256334753, 0.0009771253907250058643, 0.001172514838424371098, 0.001367904286123736764, 0.001563293733823101998 ),
 .UNSPECIFIED. ) ;
#64239=CARTESIAN_POINT ( 'NONE',  ( -11.31545018684868786, -4.887748414852792322, 34.01359900205216746 ) ) ;
#64240=LINE ( 'NONE', #21949, #16599 ) ;
#64242=FACE_BOUND ( 'NONE', #88410, .T. ) ;
#64243=CARTESIAN_POINT ( 'NONE',  ( 15.29602437028207085, -11.67786785259547777, 32.92929555188713664 ) ) ;
#64244=CARTESIAN_POINT ( 'NONE',  ( -17.07692307692307665, -6.189225973068211317, 35.74407628777942847 ) ) ;
#64246=CARTESIAN_POINT ( 'NONE',  ( 6.000000000000001776, -10.05456864172156806, 36.03766855953608683 ) ) ;
#64247=FACE_OUTER_BOUND ( 'NONE', #27393, .T. ) ;
#64248=AXIS2_PLACEMENT_3D ( 'NONE', #68653, #28563, #61444 ) ;
#64249=CARTESIAN_POINT ( 'NONE',  ( 5.076923076922954969, -2.625532179533778709, 30.86335684631627174 ) ) ;
#64250=DIRECTION ( 'NONE',  ( 0.000000000000000000, 0.000000000000000000, -1.000000000000000000 ) ) ;
#64251=ORIENTED_EDGE ( 'NONE', *, *, #35737, .F. ) ;
#64252=CARTESIAN_POINT ( 'NONE',  ( 17.07692307692307665, -13.63283147151868846, 33.57946703557072254 ) ) ;
#64253=ADVANCED_FACE ( 'NONE', ( #17010 ), #50338, .F. ) ;
#64254=CARTESIAN_POINT ( 'NONE',  ( -16.94613263595612906, -6.369690395747424461, 34.87708834333098196 ) ) ;
#64255=ORIENTED_EDGE ( 'NONE', *, *, #1175, .F. ) ;
#64256=AXIS2_PLACEMENT_3D ( 'NONE', #24629, #51184, #23729 ) ;
#64259=CARTESIAN_POINT ( 'NONE',  ( 16.85399611801622655, -10.77366814457252175, 33.85459836347580875 ) ) ;
#64261=CARTESIAN_POINT ( 'NONE',  ( -15.16551409125639260, -5.941354392334607049, 34.76329471203374055 ) ) ;
#64262=CARTESIAN_POINT ( 'NONE',  ( -7.780086512803768173, -10.67929555188718282, 33.92786785259544757 ) ) ;
#64263=CYLINDRICAL_SURFACE ( 'NONE', #61492, 0.2499999999999998890 ) ;
#64264=CARTESIAN_POINT ( 'NONE',  ( -8.834501215191545853, -6.026961402152685388, 34.52809138561120506 ) ) ;
#64265=FACE_BOUND ( 'NONE', #64519, .T. ) ;
#64266=CARTESIAN_POINT ( 'NONE',  ( -2.531177251416254492, -6.760086850603068243, 34.69517049084099369 ) ) ;
#64267=LINE ( 'NONE', #30494, #86280 ) ;
#64272=EDGE_CURVE ( 'NONE', #8206, #68769, #67643, .T. ) ;
#64273=DIRECTION ( 'NONE',  ( -0.000000000000000000, 1.000000000000000000, 3.491481338843133355E-15 ) ) ;
#64275=ORIENTED_EDGE ( 'NONE', *, *, #77455, .F. ) ;
#64276=LINE ( 'NONE', #85453, #32019 ) ;
#64277=DIRECTION ( 'NONE',  ( -0.000000000000000000, -0.9848077530122085754, -0.1736481776669273613 ) ) ;
#64278=CARTESIAN_POINT ( 'NONE',  ( -9.561515884482904681, -8.999086150933475636, 34.52020707165672775 ) ) ;
#64279=CARTESIAN_POINT ( 'NONE',  ( -20.74999999999999645, -12.50000000000000000, 29.75000000000000355 ) ) ;
#64280=CYLINDRICAL_SURFACE ( 'NONE', #19851, 0.2500000000000008882 ) ;
#64282=CARTESIAN_POINT ( 'NONE',  ( -2.437840277424000224, -3.625366637846545448, 33.29286588640298561 ) ) ;
#64283=CARTESIAN_POINT ( 'NONE',  ( -11.53846153846166089, -3.643525952248795718, 33.31231777344771672 ) ) ;
#64284=EDGE_CURVE ( 'NONE', #2304, #70411, #38597, .T. ) ;
#64285=CARTESIAN_POINT ( 'NONE',  ( -7.846153846153844924, -2.833524468853757305, 32.15551576947925838 ) ) ;
#64286=CARTESIAN_POINT ( 'NONE',  ( -0.4615384615385840772, -2.657715359629662544, 31.77849191805970364 ) ) ;
#64287=B_SPLINE_CURVE_WITH_KNOTS ( 'NONE', 3,
 ( #61829, #45317, #139, #72790, #11099, #69040, #38576, #4340, #81676, #31826 ),
 .UNSPECIFIED., .F., .F.,
 ( 4, 2, 2, 2, 4 ),
 ( 0.000000000000000000, 0.0001954311564186861426, 0.0003908623128373722852, 0.0005862934692560583735, 0.0007817246256747445703 ),
 .UNSPECIFIED. ) ;
#64289=CARTESIAN_POINT ( 'NONE',  ( 12.21156171748987163, -12.65889640711025521, 30.72598325615533454 ) ) ;
#64290=B_SPLINE_CURVE_WITH_KNOTS ( 'NONE', 3,
 ( #71075, #85482, #10269, #70638, #43599, #8500, #58000, #65196, #37280, #57556 ),
 .UNSPECIFIED., .F., .F.,
 ( 4, 2, 2, 2, 4 ),
 ( 0.000000000000000000, 0.0001954339857564070678, 0.0003908679715128141356, 0.0005863019572692211492, 0.0007817359430256282712 ),
 .UNSPECIFIED. ) ;
#64293=ORIENTED_EDGE ( 'NONE', *, *, #5948, .T. ) ;
#64294=CARTESIAN_POINT ( 'NONE',  ( 3.230769230769231726, -12.34228464037088635, 31.77849191805839268 ) ) ;
#64295=CARTESIAN_POINT ( 'NONE',  ( -1.515175298228748080, -2.254533558242299396, 29.97296025877828285 ) ) ;
#64296=CIRCLE ( 'NONE', #77294, 0.2500000000000002220 ) ;
#64298=ADVANCED_FACE ( 'NONE', ( #31868 ), #47139, .F. ) ;
#64299=CARTESIAN_POINT ( 'NONE',  ( -2.557669051740897537, -4.818429247618089661, 34.26397095200675125 ) ) ;
#64300=DIRECTION ( 'NONE',  ( 1.000000000000000000, 0.000000000000000000, 0.000000000000000000 ) ) ;
#64302=CARTESIAN_POINT ( 'NONE',  ( -16.28399412357784826, -4.299443229763728169, 33.91186481527756058 ) ) ;
#64303=CARTESIAN_POINT ( 'NONE',  ( 12.39545505058258001, -5.557115091759785130, 34.35708131394839171 ) ) ;
#64304=ORIENTED_EDGE ( 'NONE', *, *, #82211, .F. ) ;
#64305=DIRECTION ( 'NONE',  ( -0.000000000000000000, 1.000000000000000000, -0.000000000000000000 ) ) ;
#64307=DIRECTION ( 'NONE',  ( -0.000000000000000000, -0.5000000000000009992, -0.8660254037844380415 ) ) ;
#64308=AXIS2_PLACEMENT_3D ( 'NONE', #6038, #74940, #60965 ) ;
#64309=CARTESIAN_POINT ( 'NONE',  ( 11.53846153846153832, -4.945431358278436385, 36.03766855953609394 ) ) ;
#64310=FACE_OUTER_BOUND ( 'NONE', #53829, .T. ) ;
#64312=CARTESIAN_POINT ( 'NONE',  ( -11.78848477575450282, -4.335965774309649134, 33.62209801155881905 ) ) ;
#64313=CARTESIAN_POINT ( 'NONE',  ( 5.206968132842848540, -2.254550872974306674, 29.97347326024527447 ) ) ;
#64314=B_SPLINE_CURVE_WITH_KNOTS ( 'NONE', 3,
 ( #71982, #24684, #73323, #10288, #11626, #58453, #39103, #16587, #71533, #79637 ),
 .UNSPECIFIED., .F., .F.,
 ( 4, 2, 2, 2, 4 ),
 ( 0.000000000000000000, 0.0001954339857564093175, 0.0003908679715128186350, 0.0005863019572692279796, 0.0007817359430256372700 ),
 .UNSPECIFIED. ) ;
#64315=ADVANCED_FACE ( 'NONE', ( #33192 ), #60212, .F. ) ;
#64317=EDGE_LOOP ( 'NONE', ( #87154, #34247, #39446, #5222, #69561, #14128 ) ) ;
#64318=EDGE_LOOP ( 'NONE', ( #4320, #37738 ) ) ;
#64319=EDGE_LOOP ( 'NONE', ( #16949, #5158 ) ) ;
#64321=CARTESIAN_POINT ( 'NONE',  ( -9.942284423250047354, -9.943427161483782584, 34.11278801902876978 ) ) ;
#64322=CARTESIAN_POINT ( 'NONE',  ( 13.45068271796546178, -3.322132147404559976, 32.92929555188717927 ) ) ;
#64323=CARTESIAN_POINT ( 'NONE',  ( -4.088591014333314178, -12.70778746994558439, 30.41441678777537305 ) ) ;
#64324=EDGE_CURVE ( 'NONE', #11896, #50121, #60126, .T. ) ;
#64325=CARTESIAN_POINT ( 'NONE',  ( 3.230769230769231726, -9.905515769479276145, 34.41647553114623292 ) ) ;
#64326=ADVANCED_FACE ( 'NONE', ( #26882 ), #81393, .F. ) ;
#64327=ADVANCED_FACE ( 'NONE', ( #88167 ), #74180, .F. ) ;
#64328=ORIENTED_EDGE ( 'NONE', *, *, #74064, .T. ) ;
#64330=ORIENTED_EDGE ( 'NONE', *, *, #53172, .T. ) ;
#64331=CARTESIAN_POINT ( 'NONE',  ( 5.076923076922954969, -3.835265460704628371, 33.15142922262033665 ) ) ;
#64332=EDGE_LOOP ( 'NONE', ( #67342, #87768, #66568, #46682 ) ) ;
#64333=EDGE_CURVE ( 'NONE', #20169, #61249, #54698, .T. ) ;
#64334=CARTESIAN_POINT ( 'NONE',  ( 5.076923076923075762, -1.215029322943914858, 32.30358669280327177 ) ) ;
#64335=CARTESIAN_POINT ( 'NONE',  ( 7.622668921589517588, -12.11044203135681840, 32.26167407432752299 ) ) ;
#64336=CARTESIAN_POINT ( 'NONE',  ( 14.30769230769231015, -1.215029322943914858, 32.30358669280327177 ) ) ;
#64337=EDGE_LOOP ( 'NONE', ( #23458, #1527 ) ) ;
#64338=B_SPLINE_CURVE_WITH_KNOTS ( 'NONE', 3,
 ( #7306, #20379, #33450, #54587, #61787, #14054, #55045, #55483, #35212, #12731 ),
 .UNSPECIFIED., .F., .F.,
 ( 4, 2, 2, 2, 4 ),
 ( 0.000000000000000000, 0.0001954311564186882568, 0.0003908623128373765136, 0.0005862934692560647703, 0.0007817246256747530271 ),
 .UNSPECIFIED. ) ;
#64339=ORIENTED_EDGE ( 'NONE', *, *, #86184, .T. ) ;
#64340=DIRECTION ( 'NONE',  ( 0.000000000000000000, 0.8660254037844377084, 0.5000000000000015543 ) ) ;
#64341=EDGE_LOOP ( 'NONE', ( #56107, #85100, #65130, #6929 ) ) ;
#64342=FACE_OUTER_BOUND ( 'NONE', #47377, .T. ) ;
#64344=CARTESIAN_POINT ( 'NONE',  ( -5.143006487878958310, -9.780366693483667717, 34.19971097300155805 ) ) ;
#64345=ORIENTED_EDGE ( 'NONE', *, *, #35769, .T. ) ;
#64346=CARTESIAN_POINT ( 'NONE',  ( 17.86930853333243618, -10.54014554554151140, 33.71984207302941883 ) ) ;
#64348=CARTESIAN_POINT ( 'NONE',  ( 17.77707304109314634, -12.38737895849757820, 31.66785238281580206 ) ) ;
#64349=VECTOR ( 'NONE', #76900, 999.9999999999998863 ) ;
#64350=FACE_BOUND ( 'NONE', #47838, .T. ) ;
#64351=CARTESIAN_POINT ( 'NONE',  ( 7.846153846153846700, -12.34228464037088635, 31.77849191805839268 ) ) ;
#64352=CARTESIAN_POINT ( 'NONE',  ( 4.153846153846154188, -2.292212530054420494, 30.41441678777542634 ) ) ;
#64353=DIRECTION ( 'NONE',  ( 0.000000000000000000, 0.7660444431189822323, -0.6427876096865344779 ) ) ;
#64354=CARTESIAN_POINT ( 'NONE',  ( 5.076923076923075762, -12.62096338111211580, 30.90682066428153263 ) ) ;
#64355=CARTESIAN_POINT ( 'NONE',  ( -16.15384615384615330, -2.833524468853757305, 32.15551576947925838 ) ) ;
#64356=CARTESIAN_POINT ( 'NONE',  ( 17.86985203026830504, -6.809168938359901446, 34.95455904226513866 ) ) ;
#64357=FACE_OUTER_BOUND ( 'NONE', #21360, .T. ) ;
#64358=VERTEX_POINT ( 'NONE', #12919 ) ;
#64359=CIRCLE ( 'NONE', #80202, 0.2500000000000002220 ) ;
#64360=CARTESIAN_POINT ( 'NONE',  ( -16.15384615384615330, -3.322132147404559976, 32.92929555188717927 ) ) ;
#64361=ORIENTED_EDGE ( 'NONE', *, *, #4419, .T. ) ;
#64362=ORIENTED_EDGE ( 'NONE', *, *, #32794, .F. ) ;
#64363=CARTESIAN_POINT ( 'NONE',  ( -1.161602540521989857, -4.762714258010882773, 34.23016756924214832 ) ) ;
#64365=CARTESIAN_POINT ( 'NONE',  ( -5.999999999999998224, -6.386643153685126251, 34.62446782046654192 ) ) ;
#64366=CARTESIAN_POINT ( 'NONE',  ( 14.37294744720514572, -4.320704448112861584, 33.92786785259548310 ) ) ;
#64367=CARTESIAN_POINT ( 'NONE',  ( 1.318531973659506029, -6.386643153685125363, 34.62446782046654903 ) ) ;
#64368=CARTESIAN_POINT ( 'NONE',  ( 1.254468175177164913, -11.93770438780619259, 32.05411857736982029 ) ) ;
#64369=ORIENTED_EDGE ( 'NONE', *, *, #81657, .F. ) ;
#64370=DIRECTION ( 'NONE',  ( -0.000000000000000000, -0.000000000000000000, -1.000000000000000000 ) ) ;
#64371=CARTESIAN_POINT ( 'NONE',  ( 6.673053685783957967, -3.711651800289232916, 33.01384336483936011 ) ) ;
#64372=CARTESIAN_POINT ( 'NONE',  ( -12.68446542044531000, -11.43668979543635089, 33.22377378376089752 ) ) ;
#64373=CARTESIAN_POINT ( 'NONE',  ( -12.46153846153846168, -9.584722331328613620, 36.20867863119891439 ) ) ;
#64374=CARTESIAN_POINT ( 'NONE',  ( -11.76132696066517802, -2.501496062324912284, 29.88072118266895671 ) ) ;
#64375=B_SPLINE_CURVE_WITH_KNOTS ( 'NONE', 3,
 ( #14409, #82881, #47753, #7218, #19839, #35121, #27042, #5886, #48629, #76106 ),
 .UNSPECIFIED., .F., .F.,
 ( 4, 2, 2, 2, 4 ),
 ( 0.000000000000000000, 0.0001954339857564086670, 0.0003908679715128173340, 0.0005863019572692260281, 0.0007817359430256346680 ),
 .UNSPECIFIED. ) ;
#64377=ORIENTED_EDGE ( 'NONE', *, *, #15956, .T. ) ;
#64378=ORIENTED_EDGE ( 'NONE', *, *, #4583, .T. ) ;
#64381=ORIENTED_EDGE ( 'NONE', *, *, #24529, .T. ) ;
#64382=CARTESIAN_POINT ( 'NONE',  ( -7.146561866800870355, -2.599994579823202923, 30.74605699353653776 ) ) ;
#64383=CARTESIAN_POINT ( 'NONE',  ( 18.24994551834813805, -5.852078868378311149, 34.47109172314383585 ) ) ;
#64384=CARTESIAN_POINT ( 'NONE',  ( 4.153846153846154188, -10.67929555188718282, 33.92786785259544047 ) ) ;
#64385=B_SPLINE_CURVE_WITH_KNOTS ( 'NONE', 3,
 ( #57900, #58337, #37631, #30866, #24110, #51560, #17365, #44822, #1640, #38530 ),
 .UNSPECIFIED., .F., .F.,
 ( 4, 2, 2, 2, 4 ),
 ( 0.0007817246256747458714, 0.0009771112852218889842, 0.001172497944769032097, 0.001367884604316175210, 0.001563271263863318323 ),
 .UNSPECIFIED. ) ;
#64386=CARTESIAN_POINT ( 'NONE',  ( 2.177215599575844873, -7.276988635370450709, 34.74523720219453793 ) ) ;
#64388=CYLINDRICAL_SURFACE ( 'NONE', #47457, 0.2500000000000002220 ) ;
#64390=LINE ( 'NONE', #30181, #87580 ) ;
#64391=CARTESIAN_POINT ( 'NONE',  ( 11.53846153846153832, -10.05456864172156806, 36.03766855953608683 ) ) ;
#64392=VERTEX_POINT ( 'NONE', #52562 ) ;
#64393=CARTESIAN_POINT ( 'NONE',  ( -9.757630607799864464, -7.749976743299138882, 34.99404534957040624 ) ) ;
#64394=CARTESIAN_POINT ( 'NONE',  ( -12.21159294319032007, -3.712312575010499049, 33.01462480002815170 ) ) ;
#64395=DIRECTION ( 'NONE',  ( -0.000000000000000000, 0.7660444431189791237, -0.6427876096865379196 ) ) ;
#64396=CARTESIAN_POINT ( 'NONE',  ( 11.53846153846153832, -8.164416787775445883, 34.95778746994557906 ) ) ;
#64397=AXIS2_PLACEMENT_3D ( 'NONE', #10940, #45604, #38411 ) ;
#64398=CARTESIAN_POINT ( 'NONE',  ( -12.71156169883143150, -12.43535235679832596, 30.55408501211184813 ) ) ;
#64403=CARTESIAN_POINT ( 'NONE',  ( -1.318548051265309384, -3.322132147404559976, 32.92929555188717927 ) ) ;
#64406=CARTESIAN_POINT ( 'NONE',  ( -15.90390074446811042, -11.56426240980093567, 33.07394671870546432 ) ) ;
#64407=CARTESIAN_POINT ( 'NONE',  ( -3.230769230769352962, -11.06231777344772027, 33.60647404775119895 ) ) ;
#64408=ORIENTED_EDGE ( 'NONE', *, *, #83767, .F. ) ;
#64410=CARTESIAN_POINT ( 'NONE',  ( 3.230769230769110045, -9.442884908241554243, 34.35708131394783038 ) ) ;
#64411=VERTEX_POINT ( 'NONE', #80047 ) ;
#64412=FACE_OUTER_BOUND ( 'NONE', #38342, .T. ) ;
#64413=ORIENTED_EDGE ( 'NONE', *, *, #17813, .F. ) ;
#64414=VECTOR ( 'NONE', #80252, 1000.000000000000227 ) ;
#64415=DIRECTION ( 'NONE',  ( -0.000000000000000000, -0.6427876096865404731, -0.7660444431189771253 ) ) ;
#64416=CARTESIAN_POINT ( 'NONE',  ( -17.14219307747939425, -2.379036618887870880, 30.90682066428148644 ) ) ;
#64417=EDGE_CURVE ( 'NONE', #75871, #62121, #26792, .T. ) ;
#64418=CARTESIAN_POINT ( 'NONE',  ( 7.976679547917409963, -6.001044277235011215, 34.52024696741798948 ) ) ;
#64419=CARTESIAN_POINT ( 'NONE',  ( -4.376773112753000738, -11.43668979543635089, 33.22377378376089752 ) ) ;
#64420=VERTEX_POINT ( 'NONE', #87268 ) ;
#64421=CARTESIAN_POINT ( 'NONE',  ( -2.530619266599153150, -11.98009711892699691, 32.48740034544075428 ) ) ;
#64422=VECTOR ( 'NONE', #40587, 1000.000000000000227 ) ;
#64423=B_SPLINE_CURVE_WITH_KNOTS ( 'NONE', 3,
 ( #76722, #17116, #37378, #3596, #31065, #58532, #86029, #47251, #18901, #34181 ),
 .UNSPECIFIED., .F., .F.,
 ( 4, 2, 2, 2, 4 ),
 ( 0.000000000000000000, 0.0001954339857564070678, 0.0003908679715128141356, 0.0005863019572692211492, 0.0007817359430256282712 ),
 .UNSPECIFIED. ) ;
#64424=VERTEX_POINT ( 'NONE', #25547 ) ;
#64426=CARTESIAN_POINT ( 'NONE',  ( 5.750000000000003553, -7.566083408709834757, 34.74999999999999289 ) ) ;
#64427=VERTEX_POINT ( 'NONE', #62857 ) ;
#64429=CARTESIAN_POINT ( 'NONE',  ( 5.076923076923075762, -8.318370150425687726, 35.83090037661290239 ) ) ;
#64430=CARTESIAN_POINT ( 'NONE',  ( -14.53117725141625627, -10.81261337010820256, 33.49550067578627477 ) ) ;
#64432=CARTESIAN_POINT ( 'NONE',  ( 13.51514082284903040, -12.15418822224088657, 32.17964115625579069 ) ) ;
#64433=CARTESIAN_POINT ( 'NONE',  ( -18.13069146666756382, -4.118384482072086072, 33.43331474514187818 ) ) ;
#64435=EDGE_CURVE ( 'NONE', #9551, #68708, #69194, .T. ) ;
#64436=ORIENTED_EDGE ( 'NONE', *, *, #77936, .F. ) ;
#64437=VERTEX_POINT ( 'NONE', #75953 ) ;
#64438=FACE_BOUND ( 'NONE', #51270, .T. ) ;
#64439=EDGE_LOOP ( 'NONE', ( #38436, #13645, #45935, #70269 ) ) ;
#64440=CARTESIAN_POINT ( 'NONE',  ( 8.545745825506818605, -3.754499324213721234, 33.06261337010820256 ) ) ;
#64442=AXIS2_PLACEMENT_3D ( 'NONE', #80375, #52431, #24514 ) ;
#64443=DIRECTION ( 'NONE',  ( -0.000000000000000000, -0.8660254037844397068, -0.4999999999999978906 ) ) ;
#64444=CARTESIAN_POINT ( 'NONE',  ( -2.084912638714238931, -10.23759521482555357, 34.22997729860117033 ) ) ;
#64445=VERTEX_POINT ( 'NONE', #20561 ) ;
#64446=ORIENTED_EDGE ( 'NONE', *, *, #66862, .F. ) ;
#64447=CARTESIAN_POINT ( 'NONE',  ( 9.692307692307570832, -5.941354392335915335, 34.76329471203413846 ) ) ;
#64448=B_SPLINE_CURVE_WITH_KNOTS ( 'NONE', 3,
 ( #82888, #7669, #35130, #56290, #55400, #48636, #28830, #76113, #69801, #14415 ),
 .UNSPECIFIED., .F., .F.,
 ( 4, 2, 2, 2, 4 ),
 ( 0.0007817359430256215491, 0.0009771253907249856981, 0.001172514838424349847, 0.001367904286123713779, 0.001563293733823077928 ),
 .UNSPECIFIED. ) ;
#64449=ORIENTED_EDGE ( 'NONE', *, *, #26926, .T. ) ;
#64450=B_SPLINE_CURVE_WITH_KNOTS ( 'NONE', 3,
 ( #48018, #55225, #75495, #27753, #13796, #7495, #41280, #47131, #14243, #74621 ),
 .UNSPECIFIED., .F., .F.,
 ( 4, 2, 2, 2, 4 ),
 ( 0.0007817359430256294638, 0.0009771253907249937212, 0.001172514838424358087, 0.001367904286123722453, 0.001563293733823093758 ),
 .UNSPECIFIED. ) ;
#64451=DIRECTION ( 'NONE',  ( -0.000000000000000000, -0.3420201433256694901, -0.9396926207859082059 ) ) ;
#64452=DIRECTION ( 'NONE',  ( -0.000000000000000000, 0.7660444431189791237, -0.6427876096865379196 ) ) ;
#64453=CARTESIAN_POINT ( 'NONE',  ( 16.85399611801622655, -3.395401636524186362, 33.02366814457250399 ) ) ;
#64454=FACE_BOUND ( 'NONE', #27033, .T. ) ;
#64455=EDGE_LOOP ( 'NONE', ( #42542, #79672 ) ) ;
#64456=DIRECTION ( 'NONE',  ( -0.000000000000000000, 0.5000000000000011102, -0.8660254037844380415 ) ) ;
#64458=CARTESIAN_POINT ( 'NONE',  ( 7.846153846154153122, -2.506253911140614576, 30.00000000000323297 ) ) ;
#64459=CYLINDRICAL_SURFACE ( 'NONE', #173, 0.2499999999999994726 ) ;
#64460=EDGE_LOOP ( 'NONE', ( #43179, #46170 ) ) ;
#64462=ORIENTED_EDGE ( 'NONE', *, *, #87379, .T. ) ;
#64465=CARTESIAN_POINT ( 'NONE',  ( -3.230769230769229949, -12.78798330534102945, 29.74999999999997868 ) ) ;
#64466=DIRECTION ( 'NONE',  ( -0.000000000000000000, -0.000000000000000000, -1.000000000000000000 ) ) ;
#64467=LINE ( 'NONE', #45098, #78225 ) ;
#64468=CARTESIAN_POINT ( 'NONE',  ( -18.13069060311031322, -5.496505350115500121, 34.60290016733514307 ) ) ;
#64469=CARTESIAN_POINT ( 'NONE',  ( -11.76194646302587010, -2.353723527008296568, 30.78948104536958752 ) ) ;
#64471=CARTESIAN_POINT ( 'NONE',  ( -39.05038313613820122, -2.499999999999999556, 29.75000000000000355 ) ) ;
#64472=CARTESIAN_POINT ( 'NONE',  ( -0.2385256174450659516, -3.395485233115138168, 33.02377354290276656 ) ) ;
#64473=CARTESIAN_POINT ( 'NONE',  ( 4.153846153846154188, -8.973038597847269315, 34.52809138561121927 ) ) ;
#64474=CARTESIAN_POINT ( 'NONE',  ( -13.38461538461550759, -12.70778746994576025, 30.41441678777401236 ) ) ;
#64475=ORIENTED_EDGE ( 'NONE', *, *, #69668, .T. ) ;
#64477=VERTEX_POINT ( 'NONE', #734 ) ;
#64478=FACE_BOUND ( 'NONE', #80225, .T. ) ;
#64479=FACE_OUTER_BOUND ( 'NONE', #54861, .T. ) ;
#64480=CARTESIAN_POINT ( 'NONE',  ( 12.21151522424549718, -12.22074536777954989, 31.39888409691088356 ) ) ;
#64481=ORIENTED_EDGE ( 'NONE', *, *, #51644, .T. ) ;
#64482=CARTESIAN_POINT ( 'NONE',  ( 4.023155550735845409, -11.37499894934982514, 33.29245874905763003 ) ) ;
#64483=CARTESIAN_POINT ( 'NONE',  ( 6.250054419913455561, -11.47946981652013498, 33.17500667209846910 ) ) ;
#64484=CARTESIAN_POINT ( 'NONE',  ( 8.519254025182178225, -2.318417181685855422, 30.59732222474233865 ) ) ;
#64486=ORIENTED_EDGE ( 'NONE', *, *, #26545, .F. ) ;
#64488=CARTESIAN_POINT ( 'NONE',  ( -9.692307692307814193, -3.083524468854526912, 32.58852847137268327 ) ) ;
#64489=ORIENTED_EDGE ( 'NONE', *, *, #47177, .F. ) ;
#64490=CARTESIAN_POINT ( 'NONE',  ( 13.63456079399343146, -8.476813868363244353, 34.90874843262270133 ) ) ;
#64491=ORIENTED_EDGE ( 'NONE', *, *, #82386, .T. ) ;
#64492=CARTESIAN_POINT ( 'NONE',  ( 7.780883400193070898, -10.90142922261923886, 33.41473453929638993 ) ) ;
#64493=CARTESIAN_POINT ( 'NONE',  ( 15.00728428704528383, -2.847400154188068022, 31.58180166144859058 ) ) ;
#64494=CARTESIAN_POINT ( 'NONE',  ( -7.846153846153844924, -3.322132147404559976, 32.92929555188717927 ) ) ;
#64495=CARTESIAN_POINT ( 'NONE',  ( 12.71148397988660150, -4.336752205174649433, 33.62275283266504289 ) ) ;
#64496=CARTESIAN_POINT ( 'NONE',  ( -14.30769230769242917, -8.656820664282941280, 34.87096338111179961 ) ) ;
#64497=CARTESIAN_POINT ( 'NONE',  ( 6.065255571276026103, -2.892918686051625166, 31.69288490824025928 ) ) ;
#64499=EDGE_LOOP ( 'NONE', ( #58580, #51961, #1, #82007 ) ) ;
#64500=CARTESIAN_POINT ( 'NONE',  ( 5.999999999999878320, -10.33852847137269571, 34.16647553114546554 ) ) ;
#64501=CARTESIAN_POINT ( 'NONE',  ( 5.869309396889695662, -8.191372820521381826, 34.95448215188423546 ) ) ;
#64502=VERTEX_POINT ( 'NONE', #89045 ) ;
#64503=EDGE_CURVE ( 'NONE', #35268, #65460, #85891, .T. ) ;
#64506=ORIENTED_EDGE ( 'NONE', *, *, #36861, .T. ) ;
#64508=CARTESIAN_POINT ( 'NONE',  ( 7.846153846153723244, -6.835583212225970762, 34.95778746994575670 ) ) ;
#64509=B_SPLINE_CURVE_WITH_KNOTS ( 'NONE', 3,
 ( #38868, #80300, #73547, #39316, #5526, #32993, #32104, #5073, #66776, #81629 ),
 .UNSPECIFIED., .F., .F.,
 ( 4, 2, 2, 2, 4 ),
 ( 0.0007817246256747484735, 0.0009771112852218922368, 0.001172497944769036217, 0.001367884604316180197, 0.001563271263863323960 ),
 .UNSPECIFIED. ) ;
#64510=EDGE_CURVE ( 'NONE', #42382, #24770, #1173, .T. ) ;
#64511=B_SPLINE_CURVE_WITH_KNOTS ( 'NONE', 3,
 ( #55716, #62903, #84099, #23256, #22377, #49415, #50272, #63360, #9747, #78205 ),
 .UNSPECIFIED., .F., .F.,
 ( 4, 2, 2, 2, 4 ),
 ( 0.0007817246256747450040, 0.0009771112852218881168, 0.001172497944769031230, 0.001367884604316174342, 0.001563271263863317455 ),
 .UNSPECIFIED. ) ;
#64512=CARTESIAN_POINT ( 'NONE',  ( 6.249945518348143381, -11.37275283266503756, 32.91324779482534524 ) ) ;
#64513=VECTOR ( 'NONE', #40986, 1000.000000000000227 ) ;
#64515=CARTESIAN_POINT ( 'NONE',  ( -16.15384615384615330, -12.62096338111211580, 30.90682066428153263 ) ) ;
#64517=AXIS2_PLACEMENT_3D ( 'NONE', #78690, #51628, #38142 ) ;
#64518=CARTESIAN_POINT ( 'NONE',  ( 5.869390344795919923, -7.722926974430166069, 34.99546784045485737 ) ) ;
#64519=EDGE_LOOP ( 'NONE', ( #7509, #28331 ) ) ;
#64520=LINE ( 'NONE', #2820, #72134 ) ;
#64523=EDGE_CURVE ( 'NONE', #33427, #68692, #34076, .T. ) ;
#64524=DIRECTION ( 'NONE',  ( 0.000000000000000000, 0.4999999999999985567, 0.8660254037844395958 ) ) ;
#64527=CARTESIAN_POINT ( 'NONE',  ( -17.32692307692308376, -2.250000000000000000, 29.81609741502490607 ) ) ;
#64528=ADVANCED_FACE ( 'NONE', ( #27324 ), #63319, .F. ) ;
#64529=ORIENTED_EDGE ( 'NONE', *, *, #56684, .F. ) ;
#64530=CARTESIAN_POINT ( 'NONE',  ( -17.14300545628320904, -2.486705287966280320, 31.30864560766543647 ) ) ;
#64532=CARTESIAN_POINT ( 'NONE',  ( 3.453548899747295398, -10.97394488606064122, 33.68653795673694873 ) ) ;
#64533=CARTESIAN_POINT ( 'NONE',  ( 6.223012844093396723, -12.64618726649961289, 30.78989965857442712 ) ) ;
#64535=CARTESIAN_POINT ( 'NONE',  ( -1.515305987725692027, -12.62707690430377383, 30.88035979386743435 ) ) ;
#64536=CARTESIAN_POINT ( 'NONE',  ( 10.55011461482829738, -12.70778746994557551, 30.41441678777548319 ) ) ;
#64537=CARTESIAN_POINT ( 'NONE',  ( -12.71153846153846168, -7.500000000000001776, 34.75000000000000000 ) ) ;
#64538=CARTESIAN_POINT ( 'NONE',  ( -3.007757879156380376, -12.15243808032445827, 31.58219941686247978 ) ) ;
#64540=ORIENTED_EDGE ( 'NONE', *, *, #7844, .T. ) ;
#64543=ORIENTED_EDGE ( 'NONE', *, *, #53178, .F. ) ;
#64544=CARTESIAN_POINT ( 'NONE',  ( 6.923076923076924238, -6.435427911321262684, 35.78748833219616898 ) ) ;
#64545=CARTESIAN_POINT ( 'NONE',  ( -3.454254174493180507, -12.24155766932282496, 31.33739205006857986 ) ) ;
#64546=EDGE_CURVE ( 'NONE', #64975, #535, #49800, .T. ) ;
#64547=CARTESIAN_POINT ( 'NONE',  ( -6.000000000000119904, -2.625532179533778709, 30.86335684631627174 ) ) ;
#64549=CARTESIAN_POINT ( 'NONE',  ( -14.08468095607945791, -9.886259254753566594, 34.14407573483972413 ) ) ;
#64550=CARTESIAN_POINT ( 'NONE',  ( -17.77698715590660328, -12.38742843783360925, 31.66772728687926985 ) ) ;
#64552=ORIENTED_EDGE ( 'NONE', *, *, #77035, .T. ) ;
#64553=ORIENTED_EDGE ( 'NONE', *, *, #47781, .F. ) ;
#64554=CARTESIAN_POINT ( 'NONE',  ( -1.384615384615383471, -12.29105614889573062, 35.45975837776705220 ) ) ;
#64555=CARTESIAN_POINT ( 'NONE',  ( 11.28848479441294828, -9.234221910056348293, 34.70572697212741531 ) ) ;
#64556=CARTESIAN_POINT ( 'NONE',  ( -4.023055712879203938, -6.369690395747422684, 34.87708834333098196 ) ) ;
#64557=CARTESIAN_POINT ( 'NONE',  ( 15.23076923076923173, -1.215029322943914858, 32.30358669280327177 ) ) ;
#64558=B_SPLINE_CURVE_WITH_KNOTS ( 'NONE', 3,
 ( #84487, #22762, #2488, #43488, #57435, #23212, #71391, #37167, #64628, #2931 ),
 .UNSPECIFIED., .F., .F.,
 ( 4, 2, 2, 2, 4 ),
 ( 0.000000000000000000, 0.0001954311564186871184, 0.0003908623128373742367, 0.0005862934692560614093, 0.0007817246256747484735 ),
 .UNSPECIFIED. ) ;
#64559=CARTESIAN_POINT ( 'NONE',  ( 7.846153846153723244, -12.70778746994576025, 30.41441678777401236 ) ) ;
#64560=CARTESIAN_POINT ( 'NONE',  ( 11.47237812750566022, -12.10708131394839349, 31.69288490824020244 ) ) ;
#64562=DIRECTION ( 'NONE',  ( -0.000000000000000000, 1.000000000000000000, 3.491481338843133355E-15 ) ) ;
#64563=CARTESIAN_POINT ( 'NONE',  ( 16.82692307692306244, -2.249999999999998668, 29.81609741502487410 ) ) ;
#64564=VERTEX_POINT ( 'NONE', #34957 ) ;
#64565=ORIENTED_EDGE ( 'NONE', *, *, #80002, .F. ) ;
#64566=ORIENTED_EDGE ( 'NONE', *, *, #27874, .F. ) ;
#64567=VECTOR ( 'NONE', #20059, 1000.000000000000114 ) ;
#64568=CARTESIAN_POINT ( 'NONE',  ( 6.000000000000001776, -12.34228464037088635, 31.77849191805839268 ) ) ;
#64569=ORIENTED_EDGE ( 'NONE', *, *, #12454, .T. ) ;
#64570=CARTESIAN_POINT ( 'NONE',  ( -10.61538461538461320, -11.35647404775217417, 33.31231777344666511 ) ) ;
#64571=CARTESIAN_POINT ( 'NONE',  ( -10.61538461538461320, -6.343179335718451384, 34.87096338111211935 ) ) ;
#64573=EDGE_CURVE ( 'NONE', #38795, #79333, #82276, .T. ) ;
#64574=CARTESIAN_POINT ( 'NONE',  ( 1.384615384615264011, -5.094484230521993062, 34.41647553114689373 ) ) ;
#64576=ORIENTED_EDGE ( 'NONE', *, *, #41106, .T. ) ;
#64577=AXIS2_PLACEMENT_3D ( 'NONE', #45900, #37361, #30176 ) ;
#64578=B_SPLINE_CURVE_WITH_KNOTS ( 'NONE', 3,
 ( #43444, #83106, #83561, #49749, #77223, #15534 ),
 .UNSPECIFIED., .F., .F.,
 ( 4, 2, 4 ),
 ( 0.0003909569690057776653, 0.0005862646681846002839, 0.0007815723673634227941 ),
 .UNSPECIFIED. ) ;
#64579=ORIENTED_EDGE ( 'NONE', *, *, #12816, .F. ) ;
#64580=CARTESIAN_POINT ( 'NONE',  ( -11.66860950819323151, -12.15440758774515473, 32.17923288041532004 ) ) ;
#64581=B_SPLINE_CURVE_WITH_KNOTS ( 'NONE', 3,
 ( #31298, #5159, #12365, #72719, #53785, #32627, #4266, #11030, #60097, #25876 ),
 .UNSPECIFIED., .F., .F.,
 ( 4, 2, 2, 2, 4 ),
 ( 0.0007817246256747446788, 0.0009771112852218874663, 0.001172497944769030362, 0.001367884604316173258, 0.001563271263863315937 ),
 .UNSPECIFIED. ) ;
#64582=ORIENTED_EDGE ( 'NONE', *, *, #22668, .T. ) ;
#64583=FACE_BOUND ( 'NONE', #29804, .T. ) ;
#64584=CARTESIAN_POINT ( 'NONE',  ( 3.296836564119305812, -2.486705287966280320, 31.30864560766543647 ) ) ;
#64585=CARTESIAN_POINT ( 'NONE',  ( -14.55771553191376277, -6.652501968072648708, 34.93155406624980941 ) ) ;
#64587=CARTESIAN_POINT ( 'NONE',  ( -15.00775787915638126, -4.887748414852792322, 34.01359900205216746 ) ) ;
#64588=CARTESIAN_POINT ( 'NONE',  ( 4.946232473812769648, -8.191372820521381826, 34.95448215188423546 ) ) ;
#64589=CARTESIAN_POINT ( 'NONE',  ( 10.54930120442873864, -2.721908614388770964, 31.22303859784723912 ) ) ;
#64590=ORIENTED_EDGE ( 'NONE', *, *, #78093, .F. ) ;
#64592=CARTESIAN_POINT ( 'NONE',  ( -16.85414353565466783, -2.600157965045223563, 30.74683119005207033 ) ) ;
#64593=EDGE_CURVE ( 'NONE', #60344, #86735, #11634, .T. ) ;
#64596=CARTESIAN_POINT ( 'NONE',  ( 3.453548772037639214, -8.496831190052096971, 34.64984203495476578 ) ) ;
#64597=DIRECTION ( 'NONE',  ( -0.000000000000000000, -0.1736481776669307198, -0.9848077530122080203 ) ) ;
#64598=CARTESIAN_POINT ( 'NONE',  ( 2.307692307692186251, -12.16647553114689728, 32.15551576947799362 ) ) ;
#64599=CARTESIAN_POINT ( 'NONE',  ( 15.90382292962469535, -2.985938066672154889, 32.43141759479405550 ) ) ;
#64601=DIRECTION ( 'NONE',  ( -0.000000000000000000, 1.000000000000000000, 3.491481338843133355E-15 ) ) ;
#64602=CARTESIAN_POINT ( 'NONE',  ( 7.976679284387489410, -3.068774925481848825, 32.56582465632704526 ) ) ;
#64603=DIRECTION ( 'NONE',  ( -0.000000000000000000, -0.1736481776669307198, -0.9848077530122080203 ) ) ;
#64604=CARTESIAN_POINT ( 'NONE',  ( 2.438218009455871638, -10.19071101563364401, 33.96452234770658407 ) ) ;
#64605=CARTESIAN_POINT ( 'NONE',  ( 8.769230769231075584, -2.506253911140615021, 30.00000000000323297 ) ) ;
#64606=CARTESIAN_POINT ( 'NONE',  ( -2.557692307692305267, -7.500000000000001776, 35.04278698407183867 ) ) ;
#64607=CARTESIAN_POINT ( 'NONE',  ( 6.000000000000001776, -11.91647553114624181, 32.58852847137148245 ) ) ;
#64608=DIRECTION ( 'NONE',  ( -0.000000000000000000, 0.9396926207859092051, -0.3420201433256662704 ) ) ;
#64609=AXIS2_PLACEMENT_3D ( 'NONE', #53082, #38250, #30595 ) ;
#64611=VERTEX_POINT ( 'NONE', #85824 ) ;
#64613=EDGE_LOOP ( 'NONE', ( #27662, #12550 ) ) ;
#64614=CARTESIAN_POINT ( 'NONE',  ( -2.437840277424005553, -3.069018819979302926, 32.56621877034667278 ) ) ;
#64617=DIRECTION ( 'NONE',  ( -0.000000000000000000, -0.5000000000000009992, -0.8660254037844380415 ) ) ;
#64618=ORIENTED_EDGE ( 'NONE', *, *, #40063, .T. ) ;
#64619=CARTESIAN_POINT ( 'NONE',  ( 5.869852030268300602, -11.04286588640298561, 33.62463336215343901 ) ) ;
#64621=CARTESIAN_POINT ( 'NONE',  ( 7.716005876422151744, -8.630895178749533159, 34.87696386517710323 ) ) ;
#64622=ADVANCED_FACE ( 'NONE', ( #72291 ), #57442, .F. ) ;
#64623=CARTESIAN_POINT ( 'NONE',  ( -4.854143535654667829, -2.847695495035524882, 31.58253572463339509 ) ) ;
#64624=B_SPLINE_CURVE_WITH_KNOTS ( 'NONE', 3,
 ( #37022, #2788, #85230, #16756, #72144, #51860, #38821, #10900, #10000, #23081 ),
 .UNSPECIFIED., .F., .F.,
 ( 4, 2, 2, 2, 4 ),
 ( 0.000000000000000000, 0.0001954339857564053873, 0.0003908679715128107746, 0.0005863019572692161618, 0.0007817359430256215491 ),
 .UNSPECIFIED. ) ;
#64625=CARTESIAN_POINT ( 'NONE',  ( -18.00000000000012079, -12.51329471203414379, 31.30864560766407578 ) ) ;
#64626=CARTESIAN_POINT ( 'NONE',  ( -6.249976744048588273, -2.544273027872574922, 31.48422191005632342 ) ) ;
#64627=CARTESIAN_POINT ( 'NONE',  ( -16.40386937806761125, -10.18141759479407327, 34.26406193332782379 ) ) ;
#64628=CARTESIAN_POINT ( 'NONE',  ( -13.44988538517170440, -8.656820664281498878, 34.87096338111211935 ) ) ;
#64629=CARTESIAN_POINT ( 'NONE',  ( -14.05763788777885281, -4.818054556918156983, 34.26375889529406749 ) ) ;
#64631=CYLINDRICAL_SURFACE ( 'NONE', #79347, 0.2500000000000002220 ) ;
#64634=CYLINDRICAL_SURFACE ( 'NONE', #29206, 0.2499999999999994726 ) ;
#64637=VECTOR ( 'NONE', #28692, 1000.000000000000114 ) ;
#64638=VERTEX_POINT ( 'NONE', #43495 ) ;
#64639=LINE ( 'NONE', #3838, #81730 ) ;
#64640=CARTESIAN_POINT ( 'NONE',  ( -6.923076923077045919, -11.06231777344772027, 33.60647404775119895 ) ) ;
#64641=CARTESIAN_POINT ( 'NONE',  ( -9.019207500173124004, -11.28823185664190376, 33.01397839955799896 ) ) ;
#64642=CARTESIAN_POINT ( 'NONE',  ( 16.08852323835397513, -7.749976743299138882, 34.99404534957040624 ) ) ;
#64643=AXIS2_PLACEMENT_3D ( 'NONE', #65609, #23737, #30937 ) ;
#64645=AXIS2_PLACEMENT_3D ( 'NONE', #49072, #55391, #68460 ) ;
#64646=CARTESIAN_POINT ( 'NONE',  ( -14.30769230769242917, -4.320704448113951379, 33.92786785259630022 ) ) ;
#64647=AXIS2_PLACEMENT_3D ( 'NONE', #17018, #44470, #66545 ) ;
#64648=EDGE_CURVE ( 'NONE', #7426, #9090, #33168, .T. ) ;
#64650=CARTESIAN_POINT ( 'NONE',  ( 4.153846153846032507, -11.48612834414049644, 32.76840700105863391 ) ) ;
#64651=ORIENTED_EDGE ( 'NONE', *, *, #16746, .F. ) ;
#64652=ADVANCED_FACE ( 'NONE', ( #31317 ), #3388, .F. ) ;
#64653=ORIENTED_EDGE ( 'NONE', *, *, #29626, .T. ) ;
#64654=CARTESIAN_POINT ( 'NONE',  ( -5.869208192175211281, -5.582136614379148654, 34.36778462344220486 ) ) ;
#64656=CARTESIAN_POINT ( 'NONE',  ( -15.36145983387954139, -10.70098750199973203, 33.91152734681376302 ) ) ;
#64657=EDGE_CURVE ( 'NONE', #60044, #52756, #69689, .T. ) ;
#64659=CARTESIAN_POINT ( 'NONE',  ( 17.77707378248384629, -9.086856451489516928, 34.49173150075333183 ) ) ;
#64660=VERTEX_POINT ( 'NONE', #58778 ) ;
#64661=CARTESIAN_POINT ( 'NONE',  ( -14.17716660592874156, -12.27024696741798948, 31.24895572276497546 ) ) ;
#64662=EDGE_LOOP ( 'NONE', ( #24886, #49511 ) ) ;
#64663=B_SPLINE_CURVE_WITH_KNOTS ( 'NONE', 3,
 ( #54076, #13109, #68485, #6362, #54977, #12664, #74815, #13986, #80696, #32937 ),
 .UNSPECIFIED., .F., .F.,
 ( 4, 2, 2, 2, 4 ),
 ( 0.0007817246256747491240, 0.0009771112852218931041, 0.001172497944769036867, 0.001367884604316180631, 0.001563271263863324611 ),
 .UNSPECIFIED. ) ;
#64664=ORIENTED_EDGE ( 'NONE', *, *, #56967, .T. ) ;
#64665=CARTESIAN_POINT ( 'NONE',  ( 1.161130440891439797, -11.41268669641500466, 32.86336882939237825 ) ) ;
#64666=CYLINDRICAL_SURFACE ( 'NONE', #38815, 0.2499999999999993616 ) ;
#64667=ADVANCED_FACE ( 'NONE', ( #24549 ), #64634, .F. ) ;
#64669=DIRECTION ( 'NONE',  ( -0.000000000000000000, -0.9848077530122086864, -0.1736481776669273613 ) ) ;
#64670=EDGE_CURVE ( 'NONE', #38977, #33880, #72871, .T. ) ;
#64671=CARTESIAN_POINT ( 'NONE',  ( -16.94639737515951339, -3.285477652293413264, 32.44071101563363158 ) ) ;
#64672=DIRECTION ( 'NONE',  ( -0.000000000000000000, -0.9396926207859092051, -0.3420201433256662704 ) ) ;
#64673=ORIENTED_EDGE ( 'NONE', *, *, #60191, .T. ) ;
#64674=B_SPLINE_CURVE_WITH_KNOTS ( 'NONE', 3,
 ( #64851, #2702, #85584, #30199, #29757, #29320, #57663, #8158, #15360, #78370 ),
 .UNSPECIFIED., .F., .F.,
 ( 4, 2, 2, 2, 4 ),
 ( 0.000000000000000000, 0.0001954339857564073659, 0.0003908679715128147319, 0.0005863019572692221250, 0.0007817359430256294638 ),
 .UNSPECIFIED. ) ;
#64675=VERTEX_POINT ( 'NONE', #58329 ) ;
#64677=ORIENTED_EDGE ( 'NONE', *, *, #36292, .T. ) ;
#64678=CARTESIAN_POINT ( 'NONE',  ( -13.60754234352223335, -5.582147617184174848, 34.63737895849758530 ) ) ;
#64679=VERTEX_POINT ( 'NONE', #17355 ) ;
#64681=CARTESIAN_POINT ( 'NONE',  ( 6.000000000000001776, -12.48256725967547354, 35.29906147534542527 ) ) ;
#64682=EDGE_CURVE ( 'NONE', #81662, #45538, #4765, .T. ) ;
#64683=DIRECTION ( 'NONE',  ( -0.000000000000000000, 0.3420201433256694901, -0.9396926207859082059 ) ) ;
#64686=DIRECTION ( 'NONE',  ( 0.000000000000000000, 0.1736481776669275834, 0.9848077530122086864 ) ) ;
#64687=ORIENTED_EDGE ( 'NONE', *, *, #83593, .F. ) ;
#64688=EDGE_CURVE ( 'NONE', #15080, #8255, #48156, .T. ) ;
#64689=CARTESIAN_POINT ( 'NONE',  ( 2.557637826040449980, -9.272278438253398036, 34.42582936511637826 ) ) ;
#64691=FACE_OUTER_BOUND ( 'NONE', #71890, .T. ) ;
#64692=LINE ( 'NONE', #30041, #56152 ) ;
#64693=AXIS2_PLACEMENT_3D ( 'NONE', #54307, #20091, #69604 ) ;
#64694=CARTESIAN_POINT ( 'NONE',  ( 4.826899839630109490, -3.202444869320336451, 32.30641848906366675 ) ) ;
#64696=EDGE_CURVE ( 'NONE', #53579, #32375, #47034, .T. ) ;
#64697=CARTESIAN_POINT ( 'NONE',  ( -0.7115152055870525016, -12.41104346484419452, 31.60698883733904196 ) ) ;
#64698=CARTESIAN_POINT ( 'NONE',  ( -9.692307692307691624, -7.500000000000001776, 35.04278698407183867 ) ) ;
#64699=ORIENTED_EDGE ( 'NONE', *, *, #32784, .T. ) ;
#64700=CARTESIAN_POINT ( 'NONE',  ( -10.83886955910856464, -10.11188796281391511, 34.01382737946119050 ) ) ;
#64703=ORIENTED_EDGE ( 'NONE', *, *, #31598, .F. ) ;
#64704=EDGE_CURVE ( 'NONE', #88692, #85285, #41791, .T. ) ;
#64705=CARTESIAN_POINT ( 'NONE',  ( -16.21911615440246734, -12.70778746994557551, 30.41441678777548319 ) ) ;
#64706=CARTESIAN_POINT ( 'NONE',  ( 16.82689985270161870, -10.92453946501459328, 33.72985991061849376 ) ) ;
#64707=CARTESIAN_POINT ( 'NONE',  ( 16.08776377448601735, -6.343179335718451384, 34.87096338111212646 ) ) ;
#64708=CARTESIAN_POINT ( 'NONE',  ( -7.623374177175779032, -10.97394488606064122, 33.68653795673694873 ) ) ;
#64709=CARTESIAN_POINT ( 'NONE',  ( -0.3310127597748990236, -12.45806712695776319, 30.39783852428763922 ) ) ;
#64710=CARTESIAN_POINT ( 'NONE',  ( 7.715462379486287325, -8.147922237126337563, 34.70805685702651999 ) ) ;
#64711=FACE_BOUND ( 'NONE', #74370, .T. ) ;
#64712=CARTESIAN_POINT ( 'NONE',  ( 5.299702745901139878, -5.827830569534416583, 34.72679350104403539 ) ) ;
#64713=CYLINDRICAL_SURFACE ( 'NONE', #38813, 0.2499999999999986955 ) ;
#64715=DIRECTION ( 'NONE',  ( -0.000000000000000000, -0.9848077530122085754, -0.1736481776669273613 ) ) ;
#64719=ORIENTED_EDGE ( 'NONE', *, *, #17285, .T. ) ;
#64720=DIRECTION ( 'NONE',  ( -0.000000000000000000, 0.9848077530122086864, -0.1736481776669273891 ) ) ;
#64721=CARTESIAN_POINT ( 'NONE',  ( -5.076923076923075762, -3.050289026998446396, 32.03036669348365706 ) ) ;
#64722=CARTESIAN_POINT ( 'NONE',  ( -0.6844654204453108903, -3.395401636524185474, 33.02366814457250399 ) ) ;
#64724=CARTESIAN_POINT ( 'NONE',  ( 10.86533013373275836, -12.22109172314383052, 31.39792113162168263 ) ) ;
#64725=LINE ( 'NONE', #21206, #28229 ) ;
#64727=EDGE_CURVE ( 'NONE', #64009, #32057, #45261, .T. ) ;
#64728=CARTESIAN_POINT ( 'NONE',  ( -8.638705067467206788, -2.882268652242222284, 31.66798894389554064 ) ) ;
#64730=CARTESIAN_POINT ( 'NONE',  ( -17.01085472592063752, -5.557115091759786019, 34.35708131394839882 ) ) ;
#64731=CARTESIAN_POINT ( 'NONE',  ( 17.74997677577853850, -8.475808217655753651, 34.90892951860618609 ) ) ;
#64733=CARTESIAN_POINT ( 'NONE',  ( 4.023154687178598365, -10.54014554554150607, 33.71984207302941883 ) ) ;
#64734=CARTESIAN_POINT ( 'NONE',  ( -6.130147969731692292, -12.15440758774515473, 32.17923288041532004 ) ) ;
#64735=CARTESIAN_POINT ( 'NONE',  ( 17.14299041027315695, -2.486705287966280320, 31.30864560766543647 ) ) ;
#64736=ORIENTED_EDGE ( 'NONE', *, *, #43963, .T. ) ;
#64738=CARTESIAN_POINT ( 'NONE',  ( 17.14217821643591932, -12.70778746994558439, 30.41441678777537305 ) ) ;
#64739=CARTESIAN_POINT ( 'NONE',  ( 6.988332494352946789, -5.219633306516380244, 34.19971097300157936 ) ) ;
#64741=B_SPLINE_CURVE_WITH_KNOTS ( 'NONE', 3,
 ( #27860, #37264, #44022, #57539, #30078, #50330, #71492, #22865, #16120, #8928 ),
 .UNSPECIFIED., .F., .F.,
 ( 4, 2, 2, 2, 4 ),
 ( 0.000000000000000000, 0.0001954311564186868473, 0.0003908623128373736946, 0.0005862934692560605419, 0.0007817246256747473893 ),
 .UNSPECIFIED. ) ;
#64742=CARTESIAN_POINT ( 'NONE',  ( 7.146089767170319185, -10.77377354290276301, 33.85451476688484718 ) ) ;
#64743=CARTESIAN_POINT ( 'NONE',  ( -17.01166793741023042, -5.941354392334603496, 34.76329471203374055 ) ) ;
#64744=EDGE_LOOP ( 'NONE', ( #80026, #23899, #48385, #16795 ) ) ;
#64745=CARTESIAN_POINT ( 'NONE',  ( -6.857009589726848375, -9.905515769479277921, 34.41647553114623292 ) ) ;
#64746=LINE ( 'NONE', #30964, #22429 ) ;
#64747=VERTEX_POINT ( 'NONE', #31769 ) ;
#64748=CARTESIAN_POINT ( 'NONE',  ( 11.78840694783958298, -4.932303261841489928, 34.32971442181322885 ) ) ;
#64749=FACE_OUTER_BOUND ( 'NONE', #13613, .T. ) ;
#64750=CARTESIAN_POINT ( 'NONE',  ( -8.519285250882626670, -2.587454068350147018, 30.68340429815432202 ) ) ;
#64751=DIRECTION ( 'NONE',  ( -0.000000000000000000, -0.5000000000000009992, -0.8660254037844380415 ) ) ;
#64752=ORIENTED_EDGE ( 'NONE', *, *, #5063, .F. ) ;
#64754=CARTESIAN_POINT ( 'NONE',  ( -15.90390063549801347, -3.202959910592335202, 32.30730279482227019 ) ) ;
#64755=VECTOR ( 'NONE', #5783, 1000.000000000000000 ) ;
#64756=CARTESIAN_POINT ( 'NONE',  ( -11.53846153846153655, -6.386643153685126251, 34.62446782046654192 ) ) ;
#64757=ORIENTED_EDGE ( 'NONE', *, *, #69921, .T. ) ;
#64758=EDGE_LOOP ( 'NONE', ( #76200, #88987, #33351, #28832 ) ) ;
#64759=B_SPLINE_CURVE_WITH_KNOTS ( 'NONE', 3,
 ( #37370, #64841, #27424, #88706, #68406, #7152, #81495, #40943, #34624, #19782 ),
 .UNSPECIFIED., .F., .F.,
 ( 4, 2, 2, 2, 4 ),
 ( 0.000000000000000000, 0.0001954311564186865492, 0.0003908623128373730983, 0.0005862934692560596746, 0.0007817246256747461966 ),
 .UNSPECIFIED. ) ;
#64760=EDGE_CURVE ( 'NONE', #7820, #29336, #11493, .T. ) ;
#64763=VECTOR ( 'NONE', #49822, 999.9999999999998863 ) ;
#64765=CARTESIAN_POINT ( 'NONE',  ( 6.250054419913455561, -2.318338780012835443, 30.59689888758630261 ) ) ;
#64766=ADVANCED_FACE ( 'NONE', ( #53800 ), #72734, .F. ) ;
#64767=CARTESIAN_POINT ( 'NONE',  ( 17.07692307692307665, -1.422936976036506707, 30.56769352161908415 ) ) ;
#64769=ADVANCED_FACE ( 'NONE', ( #4281 ), #5618, .F. ) ;
#64770=CARTESIAN_POINT ( 'NONE',  ( -6.923076923076922462, -13.63283147151868846, 33.57946703557072254 ) ) ;
#64771=ORIENTED_EDGE ( 'NONE', *, *, #5740, .T. ) ;
#64773=CARTESIAN_POINT ( 'NONE',  ( 4.403791563224197070, -5.766571408460171355, 34.70601412856602508 ) ) ;
#64774=ORIENTED_EDGE ( 'NONE', *, *, #39423, .T. ) ;
#64776=DIRECTION ( 'NONE',  ( -0.000000000000000000, 0.9848077530122086864, -0.1736481776669273891 ) ) ;
#64777=CARTESIAN_POINT ( 'NONE',  ( -17.07692307692319744, -8.613356846316285953, 34.62446782046622218 ) ) ;
#64778=CARTESIAN_POINT ( 'NONE',  ( 16.02315555073584363, -11.37499894934982514, 33.29245874905763003 ) ) ;
#64779=ORIENTED_EDGE ( 'NONE', *, *, #19024, .F. ) ;
#64780=ORIENTED_EDGE ( 'NONE', *, *, #19997, .T. ) ;
#64781=CARTESIAN_POINT ( 'NONE',  ( -3.230769230769229949, -10.51840700105979565, 33.73612834413961536 ) ) ;
#64782=ORIENTED_EDGE ( 'NONE', *, *, #43455, .F. ) ;
#64783=B_SPLINE_CURVE_WITH_KNOTS ( 'NONE', 3,
 ( #34996, #770, #28237, #21482, #68346, #14737, #69669, #81430, #62894, #19718 ),
 .UNSPECIFIED., .F., .F.,
 ( 4, 2, 2, 2, 4 ),
 ( 0.0007817246256747457630, 0.0009771112852218887673, 0.001172497944769031880, 0.001367884604316174993, 0.001563271263863318106 ),
 .UNSPECIFIED. ) ;
#64784=CARTESIAN_POINT ( 'NONE',  ( -14.30769230769230660, -11.91647553114624181, 32.58852847137148245 ) ) ;
#64785=CARTESIAN_POINT ( 'NONE',  ( -9.692307692307691624, -2.249999999999998668, 29.75000000000001776 ) ) ;
#64786=ORIENTED_EDGE ( 'NONE', *, *, #6475, .F. ) ;
#64788=CARTESIAN_POINT ( 'NONE',  ( -14.05763788777885637, -12.65882529074907126, 30.72640787790839312 ) ) ;
#64789=LINE ( 'NONE', #49956, #66967 ) ;
#64790=FACE_BOUND ( 'NONE', #56339, .T. ) ;
#64791=EDGE_CURVE ( 'NONE', #49542, #19289, #59226, .T. ) ;
#64792=CARTESIAN_POINT ( 'NONE',  ( 7.976944287120795174, -12.35292014791297710, 31.75344720912887198 ) ) ;
#64793=CARTESIAN_POINT ( 'NONE',  ( 3.903822929624695792, -2.341070481393820124, 30.72580821765574299 ) ) ;
#64794=CYLINDRICAL_SURFACE ( 'NONE', #76798, 0.2499999999999995559 ) ;
#64795=FACE_OUTER_BOUND ( 'NONE', #65018, .T. ) ;
#64796=CARTESIAN_POINT ( 'NONE',  ( -0.4615384615384611200, -11.11383981884818262, 36.00935417666054406 ) ) ;
#64797=CARTESIAN_POINT ( 'NONE',  ( -7.846153846153844924, -3.050289026998446396, 32.03036669348365706 ) ) ;
#64798=CARTESIAN_POINT ( 'NONE',  ( 1.384615384615386802, -2.292212530054420494, 30.41441678777542634 ) ) ;
#64799=VERTEX_POINT ( 'NONE', #45712 ) ;
#64800=CARTESIAN_POINT ( 'NONE',  ( -12.46153846153846168, -2.708943851104267164, 35.45975837776705220 ) ) ;
#64802=VERTEX_POINT ( 'NONE', #32212 ) ;
#64803=CARTESIAN_POINT ( 'NONE',  ( 5.777073782483853392, -6.503392248772476236, 34.64988816332204635 ) ) ;
#64804=CARTESIAN_POINT ( 'NONE',  ( 15.16468685140909400, -2.833524468853757305, 32.15551576947924417 ) ) ;
#64806=CARTESIAN_POINT ( 'NONE',  ( -11.53846153846153655, -10.51840700105979565, 33.73612834413961536 ) ) ;
#64807=CARTESIAN_POINT ( 'NONE',  ( -14.05763799605399100, -2.779044189368095275, 31.39831045268885745 ) ) ;
#64809=CARTESIAN_POINT ( 'NONE',  ( -0.2387589202700515223, -11.89424750095246175, 32.13594075562311758 ) ) ;
#64812=EDGE_CURVE ( 'NONE', #35909, #20857, #87171, .T. ) ;
#64813=EDGE_CURVE ( 'NONE', #28639, #41851, #4117, .T. ) ;
#64814=CARTESIAN_POINT ( 'NONE',  ( 6.673100192134568509, -3.627789207965226748, 32.91389620160131102 ) ) ;
#64815=CARTESIAN_POINT ( 'NONE',  ( 17.29993442853592711, -6.503523203565941380, 34.64991518177335195 ) ) ;
#64817=CARTESIAN_POINT ( 'NONE',  ( -7.846153846153844924, -13.57706302396349152, 30.56769352161908060 ) ) ;
#64819=ORIENTED_EDGE ( 'NONE', *, *, #19082, .F. ) ;
#64820=VECTOR ( 'NONE', #52391, 1000.000000000000114 ) ;
#64821=VECTOR ( 'NONE', #18534, 1000.000000000000114 ) ;
#64822=ORIENTED_EDGE ( 'NONE', *, *, #53239, .T. ) ;
#64823=CARTESIAN_POINT ( 'NONE',  ( 14.30769230769218581, -12.51329471203414379, 31.30864560766407578 ) ) ;
#64824=ORIENTED_EDGE ( 'NONE', *, *, #72289, .F. ) ;
#64825=CARTESIAN_POINT ( 'NONE',  ( -4.153846153846152411, -12.37446782046654192, 30.86335684631486131 ) ) ;
#64826=DIRECTION ( 'NONE',  ( -0.000000000000000000, 1.000000000000000000, 3.491481338843133355E-15 ) ) ;
#64827=CARTESIAN_POINT ( 'NONE',  ( -16.40386939113911779, -5.056417327199097755, 34.11270091957320716 ) ) ;
#64828=CARTESIAN_POINT ( 'NONE',  ( 5.869440086386637390, -2.254533558242299396, 29.97296025877828285 ) ) ;
#64832=DIRECTION ( 'NONE',  ( 0.000000000000000000, 0.9848077530122072432, 0.1736481776669354937 ) ) ;
#64833=VERTEX_POINT ( 'NONE', #53357 ) ;
#64835=CARTESIAN_POINT ( 'NONE',  ( -2.241624974342230292, -12.62096338111211757, 30.90682066428152908 ) ) ;
#64836=ORIENTED_EDGE ( 'NONE', *, *, #37866, .T. ) ;
#64837=CARTESIAN_POINT ( 'NONE',  ( -17.07692307692307665, -6.343179335718451384, 34.87096338111211935 ) ) ;
#64838=CARTESIAN_POINT ( 'NONE',  ( 14.30769230769231015, -12.10708131394839349, 31.69288490824020244 ) ) ;
#64839=EDGE_CURVE ( 'NONE', #43442, #12296, #87919, .T. ) ;
#64840=ADVANCED_FACE ( 'NONE', ( #81731 ), #41182, .F. ) ;
#64841=CARTESIAN_POINT ( 'NONE',  ( -3.296851610129365451, -9.905515769479276145, 34.41647553114623292 ) ) ;
#64843=CARTESIAN_POINT ( 'NONE',  ( 7.846153846153846700, -2.499999999999998668, 29.75000000000001421 ) ) ;
#64844=CARTESIAN_POINT ( 'NONE',  ( -4.153846153846273204, -9.442884908241554243, 34.35708131394783038 ) ) ;
#64845=CARTESIAN_POINT ( 'NONE',  ( -6.923076923076922462, -4.786620604624113540, 33.94971097300155094 ) ) ;
#64847=ORIENTED_EDGE ( 'NONE', *, *, #72228, .T. ) ;
#64848=EDGE_CURVE ( 'NONE', #11070, #48730, #37460, .T. ) ;
#64849=CARTESIAN_POINT ( 'NONE',  ( -15.90390074446811042, -6.653508905675593610, 34.93172785388651391 ) ) ;
#64850=CARTESIAN_POINT ( 'NONE',  ( 8.900022577055556994, -11.71459661697925903, 32.44059661609676937 ) ) ;
#64851=CARTESIAN_POINT ( 'NONE',  ( -13.38461538461538325, -8.973038597847269315, 34.52809138561121927 ) ) ;
#64853=LINE ( 'NONE', #3155, #69125 ) ;
#64854=CARTESIAN_POINT ( 'NONE',  ( 8.769230769230645706, -10.33852847137269571, 34.16647553114546554 ) ) ;
#64855=ORIENTED_EDGE ( 'NONE', *, *, #65167, .F. ) ;
#64857=CARTESIAN_POINT ( 'NONE',  ( -1.450698795571264466, -9.780366693483667717, 34.19971097300155805 ) ) ;
#64858=EDGE_LOOP ( 'NONE', ( #85948, #8513 ) ) ;
#64859=CARTESIAN_POINT ( 'NONE',  ( 6.699591998512592461, -6.716662450894490100, 34.94144148231605840 ) ) ;
#64862=CARTESIAN_POINT ( 'NONE',  ( 12.46153846153846168, -2.721908614388771852, 31.22303859784724978 ) ) ;
#64863=DIRECTION ( 'NONE',  ( -1.000000000000000000, 0.000000000000000000, 0.000000000000000000 ) ) ;
#64864=CARTESIAN_POINT ( 'NONE',  ( -0.2387587925603952832, -6.717445702608402236, 34.94155399931962336 ) ) ;
#64865=ORIENTED_EDGE ( 'NONE', *, *, #76130, .F. ) ;
#64868=ORIENTED_EDGE ( 'NONE', *, *, #7950, .T. ) ;
#64869=CARTESIAN_POINT ( 'NONE',  ( 13.31936545284130169, -2.255955759149247619, 30.00000000000013856 ) ) ;
#64870=VECTOR ( 'NONE', #48577, 1000.000000000000227 ) ;
#64871=EDGE_CURVE ( 'NONE', #47629, #61347, #21345, .T. ) ;
#64872=VERTEX_POINT ( 'NONE', #28555 ) ;
#64874=CARTESIAN_POINT ( 'NONE',  ( 2.557746619330623528, -3.136992222400443175, 32.19305428654138979 ) ) ;
#64875=ORIENTED_EDGE ( 'NONE', *, *, #42512, .F. ) ;
#64876=CARTESIAN_POINT ( 'NONE',  ( -6.223484924564331777, -10.97335522853832579, 33.68706563782419749 ) ) ;
#64877=CARTESIAN_POINT ( 'NONE',  ( -12.71156169883143150, -5.851115903089112003, 34.47074536777953568 ) ) ;
#64878=DIRECTION ( 'NONE',  ( -0.000000000000000000, -0.9396926207859093161, -0.3420201433256663259 ) ) ;
#64879=ADVANCED_FACE ( 'NONE', ( #192 ), #56014, .F. ) ;
#64880=CARTESIAN_POINT ( 'NONE',  ( 4.826899839630111266, -9.271318131107980420, 34.42618302367067429 ) ) ;
#64881=LINE ( 'NONE', #79752, #27775 ) ;
#64882=ORIENTED_EDGE ( 'NONE', *, *, #16825, .T. ) ;
#64883=ORIENTED_EDGE ( 'NONE', *, *, #81712, .T. ) ;
#64885=FACE_BOUND ( 'NONE', #8577, .T. ) ;
#64886=VERTEX_POINT ( 'NONE', #27659 ) ;
#64887=CARTESIAN_POINT ( 'NONE',  ( -7.976301815885541657, -5.915902021225889484, 34.75552854090298638 ) ) ;
#64888=ORIENTED_EDGE ( 'NONE', *, *, #69648, .T. ) ;
#64889=B_SPLINE_CURVE_WITH_KNOTS ( 'NONE', 3,
 ( #72093, #85612, #53929, #61125, #31097, #88634, #78845, #72536, #45060, #33224 ),
 .UNSPECIFIED., .F., .F.,
 ( 4, 2, 2, 2, 4 ),
 ( 0.0007817246256747434861, 0.0009771112852218859484, 0.001172497944769028411, 0.001367884604316171090, 0.001563271263863313552 ),
 .UNSPECIFIED. ) ;
#64891=CARTESIAN_POINT ( 'NONE',  ( 13.60762673622823549, -10.61302985866384141, 33.66295027996417843 ) ) ;
#64892=CARTESIAN_POINT ( 'NONE',  ( 0.4615384615384611200, -12.62096338111211580, 30.90682066428153263 ) ) ;
#64893=EDGE_LOOP ( 'NONE', ( #61025, #50838 ) ) ;
#64895=ORIENTED_EDGE ( 'NONE', *, *, #5838, .F. ) ;
#64896=EDGE_CURVE ( 'NONE', #56712, #78354, #78296, .T. ) ;
#64897=ORIENTED_EDGE ( 'NONE', *, *, #72331, .F. ) ;
#64898=LINE ( 'NONE', #36559, #3668 ) ;
#64899=ORIENTED_EDGE ( 'NONE', *, *, #68375, .F. ) ;
#64900=CARTESIAN_POINT ( 'NONE',  ( 11.78840705680968348, -11.37275283266504111, 32.91324779482534524 ) ) ;
#64901=DIRECTION ( 'NONE',  ( 0.000000000000000000, 0.6427876096865373645, -0.7660444431189797898 ) ) ;
#64902=CARTESIAN_POINT ( 'NONE',  ( -2.373774687052442989, -12.34228464037088280, 31.77849191805838558 ) ) ;
#64903=FACE_BOUND ( 'NONE', #80976, .T. ) ;
#64904=VERTEX_POINT ( 'NONE', #76285 ) ;
#64905=LINE ( 'NONE', #10425, #87415 ) ;
#64906=DIRECTION ( 'NONE',  ( -0.000000000000000000, 0.5000000000000011102, -0.8660254037844381525 ) ) ;
#64907=CARTESIAN_POINT ( 'NONE',  ( 2.307692307692186251, -8.656820664282941280, 34.87096338111179961 ) ) ;
#64908=CARTESIAN_POINT ( 'NONE',  ( -1.384615384615383471, -2.538708090699994813, 30.37095296980875503 ) ) ;
#64909=ORIENTED_EDGE ( 'NONE', *, *, #68429, .F. ) ;
#64910=ADVANCED_FACE ( 'NONE', ( #14146 ), #20466, .T. ) ;
#64911=FACE_OUTER_BOUND ( 'NONE', #3003, .T. ) ;
#64912=ORIENTED_EDGE ( 'NONE', *, *, #88303, .F. ) ;
#64913=EDGE_CURVE ( 'NONE', #79882, #55035, #42514, .T. ) ;
#64914=ORIENTED_EDGE ( 'NONE', *, *, #80015, .T. ) ;
#64915=CARTESIAN_POINT ( 'NONE',  ( -7.912237257109724808, -6.386643153685125363, 34.62446782046654903 ) ) ;
#64916=CARTESIAN_POINT ( 'NONE',  ( 5.776515056276054771, -3.236172620538810385, 32.36188796281390267 ) ) ;
#64918=CARTESIAN_POINT ( 'NONE',  ( -8.703975629717929152, -12.51329471203373700, 31.30864560766537963 ) ) ;
#64919=CARTESIAN_POINT ( 'NONE',  ( -13.51530598772569469, -2.845849958028613624, 32.17971566917920967 ) ) ;
#64920=CARTESIAN_POINT ( 'NONE',  ( 7.846153846153846700, -12.37446782046654192, 30.86335684631486131 ) ) ;
#64921=CARTESIAN_POINT ( 'NONE',  ( -2.372962753653082402, -10.21337939537584383, 33.94971097300158647 ) ) ;
#64922=ORIENTED_EDGE ( 'NONE', *, *, #37093, .F. ) ;
#64923=CARTESIAN_POINT ( 'NONE',  ( -5.999999999999998224, -8.564572088678739092, 35.78748833219616898 ) ) ;
#64925=CARTESIAN_POINT ( 'NONE',  ( -11.78848477575450282, -10.05641848906368097, 34.04755513067966177 ) ) ;
#64926=DIRECTION ( 'NONE',  ( -0.000000000000000000, 1.000000000000000000, 3.491481338843133355E-15 ) ) ;
#64927=CARTESIAN_POINT ( 'NONE',  ( 10.61538461538461675, -11.69971097300155272, 32.46337939537588113 ) ) ;
#64928=VECTOR ( 'NONE', #11357, 1000.000000000000227 ) ;
#64929=ORIENTED_EDGE ( 'NONE', *, *, #79170, .T. ) ;
#64930=VERTEX_POINT ( 'NONE', #28104 ) ;
#64931=B_SPLINE_CURVE_WITH_KNOTS ( 'NONE', 3,
 ( #36609, #15903, #37480, #35733, #8261, #57318, #1936, #37035, #71710, #29422 ),
 .UNSPECIFIED., .F., .F.,
 ( 4, 2, 2, 2, 4 ),
 ( 0.0007817359430256293554, 0.0009771253907249941549, 0.001172514838424358954, 0.001367904286123723537, 0.001563293733823095276 ),
 .UNSPECIFIED. ) ;
#64932=FACE_BOUND ( 'NONE', #47050, .T. ) ;
#64933=ORIENTED_EDGE ( 'NONE', *, *, #48444, .T. ) ;
#64934=CARTESIAN_POINT ( 'NONE',  ( -18.00000000000000711, -2.252971138473345292, 29.99985851721553942 ) ) ;
#64935=CARTESIAN_POINT ( 'NONE',  ( 4.826899852701618698, -2.985938066672154445, 32.43141759479405550 ) ) ;
#64937=CARTESIAN_POINT ( 'NONE',  ( 8.769230769230768274, -11.11383981884818262, 36.00935417666054406 ) ) ;
#64938=CARTESIAN_POINT ( 'NONE',  ( -2.084680956079457026, -4.187068189119697692, 33.49521262558774026 ) ) ;
#64939=CARTESIAN_POINT ( 'NONE',  ( -7.912237257109724808, -11.69971097300155272, 32.46337939537587403 ) ) ;
#64940=CARTESIAN_POINT ( 'NONE',  ( -1.161835715637317579, -4.226511098958374291, 33.85474049983370293 ) ) ;
#64942=CARTESIAN_POINT ( 'NONE',  ( 4.153846153846154188, -1.129524287112498415, 32.06866353760679544 ) ) ;
#64943=ORIENTED_EDGE ( 'NONE', *, *, #1452, .T. ) ;
#64944=CARTESIAN_POINT ( 'NONE',  ( 17.01083966596719321, -10.51840700105979565, 33.73612834413961536 ) ) ;
#64946=CARTESIAN_POINT ( 'NONE',  ( -7.846153846153965716, -9.442884908241554243, 34.35708131394783038 ) ) ;
#64947=CARTESIAN_POINT ( 'NONE',  ( -12.46153846153846168, -2.833524468853757305, 32.15551576947925838 ) ) ;
#64948=LINE ( 'NONE', #79369, #15602 ) ;
#64949=EDGE_CURVE ( 'NONE', #64502, #60134, #7837, .T. ) ;
#64950=CARTESIAN_POINT ( 'NONE',  ( 12.59233026936325217, -4.118422570099828484, 33.43335022499816489 ) ) ;
#64951=LINE ( 'NONE', #3256, #26075 ) ;
#64952=LINE ( 'NONE', #57322, #14758 ) ;
#64954=VERTEX_POINT ( 'NONE', #88948 ) ;
#64955=CARTESIAN_POINT ( 'NONE',  ( -0.7115616988314271696, -5.851115903089112003, 34.47074536777953568 ) ) ;
#64956=CARTESIAN_POINT ( 'NONE',  ( 5.934729999443682402, -8.656820664281497102, 34.87096338111211935 ) ) ;
#64958=ORIENTED_EDGE ( 'NONE', *, *, #43185, .T. ) ;
#64959=VERTEX_POINT ( 'NONE', #47480 ) ;
#64960=FACE_OUTER_BOUND ( 'NONE', #36650, .T. ) ;
#64963=VECTOR ( 'NONE', #10155, 1000.000000000000000 ) ;
#64964=B_SPLINE_CURVE_WITH_KNOTS ( 'NONE', 3,
 ( #10088, #37554, #65019, #3327, #30798, #26272, #73590, #87109, #67263, #5560 ),
 .UNSPECIFIED., .F., .F.,
 ( 4, 2, 2, 2, 4 ),
 ( 0.0007817359430256386795, 0.0009771253907250069485, 0.001172514838424375217, 0.001367904286123743486, 0.001563293733823111755 ),
 .UNSPECIFIED. ) ;
#64965=FACE_OUTER_BOUND ( 'NONE', #21288, .T. ) ;
#64967=CARTESIAN_POINT ( 'NONE',  ( 17.86985203026830504, -12.15440758774515473, 32.17923288041532004 ) ) ;
#64968=B_SPLINE_CURVE_WITH_KNOTS ( 'NONE', 3,
 ( #7421, #40323, #1545, #71318, #50153, #15065, #64550, #64114, #56488, #49286 ),
 .UNSPECIFIED., .F., .F.,
 ( 4, 2, 2, 2, 4 ),
 ( 0.0007817246256747532440, 0.0009771112852218978746, 0.001172497944769042288, 0.001367884604316186702, 0.001563271263863331333 ),
 .UNSPECIFIED. ) ;
#64969=DIRECTION ( 'NONE',  ( 0.000000000000000000, 0.000000000000000000, -1.000000000000000000 ) ) ;
#64970=ORIENTED_EDGE ( 'NONE', *, *, #48215, .T. ) ;
#64971=CARTESIAN_POINT ( 'NONE',  ( 6.130525701763565927, -10.88167719472716399, 33.43325721877153711 ) ) ;
#64972=CARTESIAN_POINT ( 'NONE',  ( -1.607541602131530967, -6.503392248772476236, 34.64988816332204635 ) ) ;
#64973=CARTESIAN_POINT ( 'NONE',  ( 3.903846153846154632, -7.566082377512563184, 35.00000000000000711 ) ) ;
#64974=CARTESIAN_POINT ( 'NONE',  ( 12.21156173059610772, -11.79746400365624659, 32.30657167506340954 ) ) ;
#64975=VERTEX_POINT ( 'NONE', #26777 ) ;
#64976=CARTESIAN_POINT ( 'NONE',  ( -5.999999999999998224, -11.91647553114624181, 32.58852847137148245 ) ) ;
#64977=ORIENTED_EDGE ( 'NONE', *, *, #33829, .F. ) ;
#64978=CARTESIAN_POINT ( 'NONE',  ( -17.93393266664992680, -8.164416787775447659, 34.95778746994558617 ) ) ;
#64979=CARTESIAN_POINT ( 'NONE',  ( -1.607541602131531633, -9.086856451489515152, 34.49173150075333183 ) ) ;
#64980=CARTESIAN_POINT ( 'NONE',  ( 3.903846153846154632, -7.500000000000001776, 34.75000000000000000 ) ) ;
#64981=ORIENTED_EDGE ( 'NONE', *, *, #48021, .F. ) ;
#64982=CARTESIAN_POINT ( 'NONE',  ( -1.450697763975519639, -12.62096338111211580, 30.90682066428152197 ) ) ;
#64983=CARTESIAN_POINT ( 'NONE',  ( 5.076923076923075762, -8.120952969808772792, 34.71129190930000163 ) ) ;
#64984=CARTESIAN_POINT ( 'NONE',  ( -17.20761454359064047, -3.530157926970578508, 32.79014554554150607 ) ) ;
#64985=CARTESIAN_POINT ( 'NONE',  ( -7.715628407920200438, -5.070358843744210198, 34.40418822224088302 ) ) ;
#64986=CARTESIAN_POINT ( 'NONE',  ( -5.076923076923199218, -8.656820664282941280, 34.87096338111179961 ) ) ;
#64987=ORIENTED_EDGE ( 'NONE', *, *, #45015, .F. ) ;
#64988=CARTESIAN_POINT ( 'NONE',  ( 7.623226887246995709, -11.43668979543635089, 33.22377378376089752 ) ) ;
#64990=AXIS2_PLACEMENT_3D ( 'NONE', #12261, #11827, #65859 ) ;
#64992=B_SPLINE_CURVE_WITH_KNOTS ( 'NONE', 3,
 ( #80748, #39312, #18143, #32534, #59116, #66770, #5965, #87510, #46930, #19031 ),
 .UNSPECIFIED., .F., .F.,
 ( 4, 2, 2, 2, 4 ),
 ( 0.0007817359430256372700, 0.0009771253907250054306, 0.001172514838424373483, 0.001367904286123741535, 0.001563293733823109804 ),
 .UNSPECIFIED. ) ;
#64993=CARTESIAN_POINT ( 'NONE',  ( 2.307692307692309264, -1.951392089020283160, 34.73218667398347748 ) ) ;
#64994=CARTESIAN_POINT ( 'NONE',  ( 9.915087361285756629, -2.612705202774698421, 31.66806509827799943 ) ) ;
#64995=B_SPLINE_CURVE_WITH_KNOTS ( 'NONE', 3,
 ( #87676, #45777, #17425, #11562, #11108, #25512, #32274, #79577, #38584, #73256 ),
 .UNSPECIFIED., .F., .F.,
 ( 4, 2, 2, 2, 4 ),
 ( 0.000000000000000000, 0.0001954339857564053873, 0.0003908679715128107746, 0.0005863019572692161618, 0.0007817359430256215491 ),
 .UNSPECIFIED. ) ;
#64996=CARTESIAN_POINT ( 'NONE',  ( -9.915234651214539952, -8.282780595021769443, 34.94152052738834158 ) ) ;
#64997=CARTESIAN_POINT ( 'NONE',  ( 15.00728428704528561, -11.89387501736622710, 32.13663884655806413 ) ) ;
#64998=ORIENTED_EDGE ( 'NONE', *, *, #46376, .F. ) ;
#64999=ORIENTED_EDGE ( 'NONE', *, *, #76538, .T. ) ;
#65001=ORIENTED_EDGE ( 'NONE', *, *, #39404, .F. ) ;
#65002=VERTEX_POINT ( 'NONE', #75408 ) ;
#65003=CARTESIAN_POINT ( 'NONE',  ( 12.59233026936325039, -11.71459661697925903, 32.44059661609676937 ) ) ;
#65004=CARTESIAN_POINT ( 'NONE',  ( 13.60739492588379385, -10.11255958852956027, 34.01340905677048454 ) ) ;
#65005=CARTESIAN_POINT ( 'NONE',  ( -4.946084658910312903, -7.277220443632450575, 34.74524770363009196 ) ) ;
#65006=DIRECTION ( 'NONE',  ( -0.000000000000000000, 0.8660254037844397068, -0.4999999999999978906 ) ) ;
#65007=CARTESIAN_POINT ( 'NONE',  ( -13.16183584334697265, -5.913360116392397892, 34.49180327182771322 ) ) ;
#65008=VECTOR ( 'NONE', #30597, 1000.000000000000227 ) ;
#65009=CARTESIAN_POINT ( 'NONE',  ( 8.545745825506822158, -9.331801661448606566, 34.40259984581193464 ) ) ;
#65010=ADVANCED_FACE ( 'NONE', ( #33970 ), #47927, .F. ) ;
#65011=DIRECTION ( 'NONE',  ( -0.000000000000000000, -0.9396926207859093161, -0.3420201433256663259 ) ) ;
#65012=CARTESIAN_POINT ( 'NONE',  ( -7.846153846153965716, -3.300289026999228881, 32.46337939537708905 ) ) ;
#65013=ORIENTED_EDGE ( 'NONE', *, *, #39404, .T. ) ;
#65014=EDGE_CURVE ( 'NONE', #67905, #69595, #27734, .T. ) ;
#65015=ORIENTED_EDGE ( 'NONE', *, *, #28412, .T. ) ;
#65016=ORIENTED_EDGE ( 'NONE', *, *, #51108, .F. ) ;
#65017=CYLINDRICAL_SURFACE ( 'NONE', #38826, 0.2499999999999994726 ) ;
#65018=EDGE_LOOP ( 'NONE', ( #71752, #22583, #70023, #80882 ) ) ;
#65019=CARTESIAN_POINT ( 'NONE',  ( 16.28437185560972011, -11.93748526763465279, 32.05452791011430946 ) ) ;
#65020=CARTESIAN_POINT ( 'NONE',  ( -17.75005459062195712, -11.56426240980093567, 33.07394671870546432 ) ) ;
#65021=CARTESIAN_POINT ( 'NONE',  ( -1.134615384615383915, -2.249999999999998668, 29.75000000000000355 ) ) ;
#65022=CARTESIAN_POINT ( 'NONE',  ( 9.692307692307695177, -13.20930481340135110, 34.54067556320372745 ) ) ;
#65024=ADVANCED_FACE ( 'NONE', ( #63656 ), #10038, .F. ) ;
#65025=ORIENTED_EDGE ( 'NONE', *, *, #65816, .F. ) ;
#65026=LINE ( 'NONE', #10097, #15488 ) ;
#65027=ORIENTED_EDGE ( 'NONE', *, *, #16677, .T. ) ;
#65028=FACE_BOUND ( 'NONE', #63882, .T. ) ;
#65030=CARTESIAN_POINT ( 'NONE',  ( 16.08857570788537572, -6.879047030191174805, 34.71129190930000163 ) ) ;
#65032=CARTESIAN_POINT ( 'NONE',  ( 17.86930853333243974, -2.729777683071817229, 31.24903638046269450 ) ) ;
#65033=LINE ( 'NONE', #22293, #21646 ) ;
#65034=CARTESIAN_POINT ( 'NONE',  ( 2.084207383127976598, -11.60425143139329940, 33.02411095842164457 ) ) ;
#65035=EDGE_LOOP ( 'NONE', ( #86181, #60197, #6331, #76084 ) ) ;
#65036=CARTESIAN_POINT ( 'NONE',  ( -11.78843828251013015, -4.818429247618089661, 34.26397095200675125 ) ) ;
#65037=DIRECTION ( 'NONE',  ( 0.000000000000000000, 0.4999999999999960032, -0.8660254037844410391 ) ) ;
#65038=EDGE_LOOP ( 'NONE', ( #70924, #64449, #22375, #56031 ) ) ;
#65039=DIRECTION ( 'NONE',  ( 0.000000000000000000, 0.1736481776669275834, 0.9848077530122086864 ) ) ;
#65040=CARTESIAN_POINT ( 'NONE',  ( 10.61538461538449596, -11.94971097300221174, 32.03036669348237098 ) ) ;
#65041=AXIS2_PLACEMENT_3D ( 'NONE', #60190, #11577, #39059 ) ;
#65042=ORIENTED_EDGE ( 'NONE', *, *, #47370, .F. ) ;
#65044=CARTESIAN_POINT ( 'NONE',  ( 13.38461538461538680, -2.538708090699994813, 30.37095296980875503 ) ) ;
#65045=CARTESIAN_POINT ( 'NONE',  ( 6.923076923076924238, -3.937682226553329556, 33.60647404775216529 ) ) ;
#65046=CARTESIAN_POINT ( 'NONE',  ( 8.096153846155281997, -7.500000000000155431, 34.75000000000007105 ) ) ;
#65047=CARTESIAN_POINT ( 'NONE',  ( 9.692307692307695177, -12.34228464037088635, 31.77849191805839268 ) ) ;
#65048=EDGE_CURVE ( 'NONE', #67006, #25149, #65381, .T. ) ;
#65049=FACE_BOUND ( 'NONE', #88843, .T. ) ;
#65051=CARTESIAN_POINT ( 'NONE',  ( 7.053602624840490165, -3.285477652293412820, 32.44071101563363158 ) ) ;
#65052=CARTESIAN_POINT ( 'NONE',  ( -1.161602540521988525, -9.172514111537584114, 34.72667873470787470 ) ) ;
#65053=CARTESIAN_POINT ( 'NONE',  ( -18.00000000000000000, -4.949874560955057845, 36.02546096051201374 ) ) ;
#65054=CARTESIAN_POINT ( 'NONE',  ( 9.019176287578909879, -2.824170634883621744, 31.52227843825338738 ) ) ;
#65055=EDGE_CURVE ( 'NONE', #61936, #69536, #78944, .T. ) ;
#65056=CARTESIAN_POINT ( 'NONE',  ( 13.16173586787780359, -7.630690623152299956, 34.99857592706774057 ) ) ;
#65059=B_SPLINE_CURVE_WITH_KNOTS ( 'NONE', 3,
 ( #16888, #29965, #43916, #57425, #84919, #23202, #50663, #71378, #9685, #13137 ),
 .UNSPECIFIED., .F., .F.,
 ( 4, 2, 2, 2, 4 ),
 ( 0.000000000000000000, 0.0001954339857564074473, 0.0003908679715128148945, 0.0005863019572692223418, 0.0007817359430256297891 ),
 .UNSPECIFIED. ) ;
#65061=CARTESIAN_POINT ( 'NONE',  ( -0.4615384615384611200, -10.05456864172156806, 36.03766855953608683 ) ) ;
#65062=ORIENTED_EDGE ( 'NONE', *, *, #42893, .T. ) ;
#65064=EDGE_CURVE ( 'NONE', #57769, #77586, #28882, .T. ) ;
#65065=VERTEX_POINT ( 'NONE', #57785 ) ;
#65066=CARTESIAN_POINT ( 'NONE',  ( 1.384615384615265343, -5.219633306517616589, 34.19971097300220464 ) ) ;
#65067=VERTEX_POINT ( 'NONE', #2386 ) ;
#65068=CARTESIAN_POINT ( 'NONE',  ( -18.00000000000000000, -12.37446782046654192, 30.86335684631486131 ) ) ;
#65070=CARTESIAN_POINT ( 'NONE',  ( -17.77698864838715309, -5.667800583137508674, 34.40243808032445827 ) ) ;
#65071=CARTESIAN_POINT ( 'NONE',  ( -9.942284436356281674, -12.65889640711025521, 30.72598325615533454 ) ) ;
#65072=CARTESIAN_POINT ( 'NONE',  ( -16.15384615384615330, -2.249999999999998668, 29.75000000000001776 ) ) ;
#65073=CARTESIAN_POINT ( 'NONE',  ( 17.86985203026830504, -2.373036134822905208, 30.88089517874952250 ) ) ;
#65075=DIRECTION ( 'NONE',  ( 1.000000000000000000, 0.000000000000000000, 0.000000000000000000 ) ) ;
#65076=CARTESIAN_POINT ( 'NONE',  ( 5.999999999999880096, -4.481592998941358097, 33.73612834414048933 ) ) ;
#65080=CARTESIAN_POINT ( 'NONE',  ( 14.53070365930516061, -3.105924265160262543, 32.13625925475356127 ) ) ;
#65082=VECTOR ( 'NONE', #25696, 1000.000000000000227 ) ;
#65083=ORIENTED_EDGE ( 'NONE', *, *, #55707, .T. ) ;
#65084=CARTESIAN_POINT ( 'NONE',  ( -13.38461538461538325, -6.343179335718451384, 34.87096338111211935 ) ) ;
#65085=CARTESIAN_POINT ( 'NONE',  ( 15.90382291655318880, -12.22074536777955345, 31.39888409691088356 ) ) ;
#65086=CARTESIAN_POINT ( 'NONE',  ( 9.915319043920545639, -6.503523203565941380, 34.64991518177335195 ) ) ;
#65087=CARTESIAN_POINT ( 'NONE',  ( 18.22277954126840172, -10.81320215134717166, 33.49497208177562868 ) ) ;
#65089=VECTOR ( 'NONE', #12177, 1000.000000000000114 ) ;
#65090=CARTESIAN_POINT ( 'NONE',  ( 2.242421861731533905, -12.27809138561121394, 31.22303859784730307 ) ) ;
#65091=EDGE_CURVE ( 'NONE', #16329, #61210, #55094, .T. ) ;
#65092=B_SPLINE_CURVE_WITH_KNOTS ( 'NONE', 3,
 ( #73332, #59368, #72430, #58460, #39115, #37309, #66578, #3524, #4884, #85513 ),
 .UNSPECIFIED., .F., .F.,
 ( 4, 2, 2, 2, 4 ),
 ( 0.000000000000000000, 0.0001954339857564063360, 0.0003908679715128126719, 0.0005863019572692189808, 0.0007817359430256253438 ),
 .UNSPECIFIED. ) ;
#65093=VERTEX_POINT ( 'NONE', #8731 ) ;
#65094=B_SPLINE_CURVE_WITH_KNOTS ( 'NONE', 3,
 ( #84174, #7170, #35976, #42295, #68863, #63432, #77393, #56680, #15260, #34642 ),
 .UNSPECIFIED., .F., .F.,
 ( 4, 2, 2, 2, 4 ),
 ( 0.0007817359430256365111, 0.0009771253907250043464, 0.001172514838424372399, 0.001367904286123740234, 0.001563293733823108069 ),
 .UNSPECIFIED. ) ;
#65095=CARTESIAN_POINT ( 'NONE',  ( 7.780883845597524662, -3.083524468853724887, 32.58852847137143272 ) ) ;
#65096=VERTEX_POINT ( 'NONE', #23988 ) ;
#65097=ORIENTED_EDGE ( 'NONE', *, *, #11656, .T. ) ;
#65098=DIRECTION ( 'NONE',  ( 1.000000000000000000, -0.000000000000000000, -0.000000000000000000 ) ) ;
#65099=CARTESIAN_POINT ( 'NONE',  ( -6.065270000556318486, -12.70778746994557551, 30.41441678777548319 ) ) ;
#65100=LINE ( 'NONE', #31336, #77578 ) ;
#65101=CARTESIAN_POINT ( 'NONE',  ( 1.634669696253700399, -11.79725096376909654, 32.30694842903960762 ) ) ;
#65102=CARTESIAN_POINT ( 'NONE',  ( -13.38461538461538325, -3.050289026998446396, 32.03036669348365706 ) ) ;
#65104=ORIENTED_EDGE ( 'NONE', *, *, #74326, .T. ) ;
#65105=VECTOR ( 'NONE', #88502, 1000.000000000000000 ) ;
#65106=CARTESIAN_POINT ( 'NONE',  ( 9.019176287578909879, -3.712312575010499494, 33.01462480002815170 ) ) ;
#65107=CIRCLE ( 'NONE', #55097, 0.2500000000000002220 ) ;
#65108=EDGE_LOOP ( 'NONE', ( #9221, #45210, #57788, #84608 ) ) ;
#65109=ORIENTED_EDGE ( 'NONE', *, *, #70964, .F. ) ;
#65110=CARTESIAN_POINT ( 'NONE',  ( 1.134638653673032405, -11.28823185664190376, 33.01397839955799896 ) ) ;
#65111=DIRECTION ( 'NONE',  ( 0.000000000000000000, 0.8660254037844377084, 0.5000000000000015543 ) ) ;
#65112=LINE ( 'NONE', #84965, #70996 ) ;
#65113=CARTESIAN_POINT ( 'NONE',  ( -8.769230769230768274, -9.905515769479276145, 34.41647553114623292 ) ) ;
#65115=CARTESIAN_POINT ( 'NONE',  ( -4.376772371362299019, -8.239355502252617924, 34.69524867566427417 ) ) ;
#65116=LINE ( 'NONE', #85410, #88389 ) ;
#65117=EDGE_LOOP ( 'NONE', ( #31364, #65715 ) ) ;
#65118=ADVANCED_FACE ( 'NONE', ( #36637 ), #64091, .F. ) ;
#65119=ORIENTED_EDGE ( 'NONE', *, *, #6786, .F. ) ;
#65121=B_SPLINE_CURVE_WITH_KNOTS ( 'NONE', 3,
 ( #27546, #88382, #40627, #41504, #74857, #73963, #54560, #54113, #68523, #47812 ),
 .UNSPECIFIED., .F., .F.,
 ( 4, 2, 2, 2, 4 ),
 ( 0.000000000000000000, 0.0001954339857564097241, 0.0003908679715128194482, 0.0005863019572692291723, 0.0007817359430256388964 ),
 .UNSPECIFIED. ) ;
#65122=EDGE_LOOP ( 'NONE', ( #4756, #27538 ) ) ;
#65123=CARTESIAN_POINT ( 'NONE',  ( -13.38461538461550759, -5.941354392335915335, 34.76329471203413846 ) ) ;
#65124=ORIENTED_EDGE ( 'NONE', *, *, #3444, .T. ) ;
#65125=CARTESIAN_POINT ( 'NONE',  ( -10.48485917715096960, -4.299079248970732792, 33.91157788607253565 ) ) ;
#65126=CARTESIAN_POINT ( 'NONE',  ( 6.130791807824786943, -12.38066358083363738, 30.83685684665853444 ) ) ;
#65127=B_SPLINE_CURVE_WITH_KNOTS ( 'NONE', 3,
 ( #35425, #83635, #21914, #49388, #76864, #15162, #85391, #86298, #51128, #16927 ),
 .UNSPECIFIED., .F., .F.,
 ( 4, 2, 2, 2, 4 ),
 ( 0.0007817359430256390048, 0.0009771253907250075990, 0.001172514838424376085, 0.001367904286123744571, 0.001563293733823113056 ),
 .UNSPECIFIED. ) ;
#65128=B_SPLINE_CURVE_WITH_KNOTS ( 'NONE', 3,
 ( #1585, #29070, #57404, #64592, #71357, #43014, #71804, #56525, #62818, #85335 ),
 .UNSPECIFIED., .F., .F.,
 ( 4, 2, 2, 2, 4 ),
 ( 0.0007817359430256395469, 0.0009771253907250080327, 0.001172514838424376735, 0.001367904286123745438, 0.001563293733823113924 ),
 .UNSPECIFIED. ) ;
#65130=ORIENTED_EDGE ( 'NONE', *, *, #30188, .F. ) ;
#65131=EDGE_CURVE ( 'NONE', #32626, #63712, #49305, .T. ) ;
#65132=CARTESIAN_POINT ( 'NONE',  ( 10.74591005361826035, -2.372941743896879174, 30.88044141588253666 ) ) ;
#65133=VERTEX_POINT ( 'NONE', #4168 ) ;
#65134=CARTESIAN_POINT ( 'NONE',  ( 5.750023255951409951, -9.234221910056348293, 34.70572697212741531 ) ) ;
#65135=FACE_OUTER_BOUND ( 'NONE', #47640, .T. ) ;
#65136=VECTOR ( 'NONE', #30380, 1000.000000000000227 ) ;
#65137=CYLINDRICAL_SURFACE ( 'NONE', #50920, 0.2499999999999995837 ) ;
#65138=CARTESIAN_POINT ( 'NONE',  ( -2.307692307692428724, -3.083524468854526912, 32.58852847137268327 ) ) ;
#65139=CARTESIAN_POINT ( 'NONE',  ( -9.692307692307691624, -10.05456864172156806, 36.03766855953608683 ) ) ;
#65140=EDGE_CURVE ( 'NONE', #74204, #43756, #89022, .T. ) ;
#65142=CARTESIAN_POINT ( 'NONE',  ( 8.638539302563209787, -5.582088688514999397, 34.36776431015576350 ) ) ;
#65143=CARTESIAN_POINT ( 'NONE',  ( -10.74553182482283198, -10.88202310037935661, 33.43294751532457099 ) ) ;
#65144=ORIENTED_EDGE ( 'NONE', *, *, #28836, .F. ) ;
#65145=CARTESIAN_POINT ( 'NONE',  ( -11.28840722682322628, -4.235687564193445276, 33.53795663066793509 ) ) ;
#65146=ADVANCED_FACE ( 'NONE', ( #65428 ), #87505, .F. ) ;
#65147=CARTESIAN_POINT ( 'NONE',  ( 9.019285080869080318, -6.567000820036036579, 34.66262288849541306 ) ) ;
#65148=ORIENTED_EDGE ( 'NONE', *, *, #54589, .F. ) ;
#65149=AXIS2_PLACEMENT_3D ( 'NONE', #9616, #2844, #30336 ) ;
#65150=CARTESIAN_POINT ( 'NONE',  ( -16.37677311275299985, -12.64616026154729411, 30.79003144601914244 ) ) ;
#65151=CARTESIAN_POINT ( 'NONE',  ( -16.15384615384615330, -11.69971097300155272, 32.46337939537588113 ) ) ;
#65152=CARTESIAN_POINT ( 'NONE',  ( 5.076923076923075762, -12.78798330534102945, 29.74999999999997868 ) ) ;
#65153=CARTESIAN_POINT ( 'NONE',  ( -16.15384615384627409, -12.16647553114689728, 32.15551576947799362 ) ) ;
#65154=CARTESIAN_POINT ( 'NONE',  ( -7.623190711887172455, -7.369474539155828730, 34.99858011523957657 ) ) ;
#65155=EDGE_CURVE ( 'NONE', #24781, #22672, #36353, .T. ) ;
#65156=FACE_BOUND ( 'NONE', #65858, .T. ) ;
#65157=CARTESIAN_POINT ( 'NONE',  ( 5.142990410273152513, -5.471508081941601098, 34.59228464037088457 ) ) ;
#65158=CARTESIAN_POINT ( 'NONE',  ( 1.634560902963529072, -2.587454068350147907, 30.68340429815432202 ) ) ;
#65159=DIRECTION ( 'NONE',  ( -0.000000000000000000, 0.9848077530122086864, -0.1736481776669273891 ) ) ;
#65160=CARTESIAN_POINT ( 'NONE',  ( -11.66907189808606482, -7.722926236386453702, 34.74524107206102030 ) ) ;
#65161=LINE ( 'NONE', #71476, #33417 ) ;
#65162=CARTESIAN_POINT ( 'NONE',  ( 12.39626801557768587, -12.46129190929999986, 30.37095296980880832 ) ) ;
#65165=ORIENTED_EDGE ( 'NONE', *, *, #38871, .T. ) ;
#65166=FACE_OUTER_BOUND ( 'NONE', #85599, .T. ) ;
#65167=EDGE_CURVE ( 'NONE', #82613, #34578, #59959, .T. ) ;
#65168=EDGE_CURVE ( 'NONE', #10775, #77057, #8442, .T. ) ;
#65169=B_SPLINE_CURVE_WITH_KNOTS ( 'NONE', 3,
 ( #84466, #22742, #71819, #10124, #53777, #32183, #31740, #73168, #86703, #60534 ),
 .UNSPECIFIED., .F., .F.,
 ( 4, 2, 2, 2, 4 ),
 ( 0.0007817359430256384627, 0.0009771253907250067317, 0.001172514838424375001, 0.001367904286123743270, 0.001563293733823111539 ),
 .UNSPECIFIED. ) ;
#65170=FACE_OUTER_BOUND ( 'NONE', #68551, .T. ) ;
#65171=CARTESIAN_POINT ( 'NONE',  ( -7.846153846153537614, -2.506253911140614576, 30.00000000000323297 ) ) ;
#65172=CARTESIAN_POINT ( 'NONE',  ( 16.82694633287449193, -8.347322224742351082, 34.93158281831414769 ) ) ;
#65173=CARTESIAN_POINT ( 'NONE',  ( 6.673053698855465399, -12.68155406624981119, 30.59749803192733708 ) ) ;
#65176=B_SPLINE_CURVE_WITH_KNOTS ( 'NONE', 3,
 ( #46931, #20369, #82520, #81625, #68984, #87971, #61325, #88842, #27113, #75309 ),
 .UNSPECIFIED., .F., .F.,
 ( 4, 2, 2, 2, 4 ),
 ( 0.0007817246256747446788, 0.0009771112852218879000, 0.001172497944769031013, 0.001367884604316174126, 0.001563271263863317238 ),
 .UNSPECIFIED. ) ;
#65177=CARTESIAN_POINT ( 'NONE',  ( -2.438382910802615822, -3.338472653186242756, 32.95098750199972670 ) ) ;
#65178=CARTESIAN_POINT ( 'NONE',  ( 0.5923302693632473970, -3.530189275343204702, 32.79018710029569661 ) ) ;
#65180=CARTESIAN_POINT ( 'NONE',  ( -16.82697755857493505, -5.852078868378312038, 34.47109172314383585 ) ) ;
#65181=CARTESIAN_POINT ( 'NONE',  ( 5.010840697562940704, -9.058645607665454236, 34.76329471203372634 ) ) ;
#65183=CARTESIAN_POINT ( 'NONE',  ( 10.61538461538492406, -2.506253911140615021, 30.00000000000323297 ) ) ;
#65184=DIRECTION ( 'NONE',  ( -0.000000000000000000, -0.9848077530122086864, -0.1736481776669273613 ) ) ;
#65185=CARTESIAN_POINT ( 'NONE',  ( 14.24160889673642849, -6.386643153685125363, 34.62446782046654903 ) ) ;
#65186=VERTEX_POINT ( 'NONE', #32529 ) ;
#65188=CARTESIAN_POINT ( 'NONE',  ( -1.384615384615069056, -2.255955759149395501, 30.00000000000324363 ) ) ;
#65190=CARTESIAN_POINT ( 'NONE',  ( -10.83886953994894675, -10.23692288466677880, 34.23039457007281072 ) ) ;
#65192=ORIENTED_EDGE ( 'NONE', *, *, #66124, .F. ) ;
#65193=EDGE_CURVE ( 'NONE', #52884, #41653, #5065, .T. ) ;
#65194=CARTESIAN_POINT ( 'NONE',  ( -18.22348494372394967, -9.331801661448606566, 34.40259984581193464 ) ) ;
#65195=CARTESIAN_POINT ( 'NONE',  ( -1.134561072977069429, -6.567000820036038355, 34.66262288849541306 ) ) ;
#65196=CARTESIAN_POINT ( 'NONE',  ( 4.023698944407932743, -6.001485441113818986, 34.52039167877662607 ) ) ;
#65198=FACE_OUTER_BOUND ( 'NONE', #53850, .T. ) ;
#65199=DIRECTION ( 'NONE',  ( -0.000000000000000000, 0.3420201433256694346, -0.9396926207859080948 ) ) ;
#65200=CARTESIAN_POINT ( 'NONE',  ( 0.4615384615384611200, -13.20930481340135110, 34.54067556320372745 ) ) ;
#65201=CARTESIAN_POINT ( 'NONE',  ( -15.48076923076922995, -2.249999999999998668, 29.75000000000000355 ) ) ;
#65202=ORIENTED_EDGE ( 'NONE', *, *, #23669, .T. ) ;
#65203=CARTESIAN_POINT ( 'NONE',  ( 2.530703659305159725, -12.15243808032445827, 31.58219941686247978 ) ) ;
#65204=EDGE_CURVE ( 'NONE', #86321, #57810, #53588, .T. ) ;
#65205=CARTESIAN_POINT ( 'NONE',  ( 10.83816428436268353, -4.226511098958373402, 33.85474049983370293 ) ) ;
#65206=AXIS2_PLACEMENT_3D ( 'NONE', #83197, #62025, #42213 ) ;
#65207=LINE ( 'NONE', #18369, #12506 ) ;
#65209=EDGE_LOOP ( 'NONE', ( #46085, #79805, #55697, #13225 ) ) ;
#65210=B_SPLINE_CURVE_WITH_KNOTS ( 'NONE', 3,
 ( #24617, #6470, #88906, #31377, #6031, #31832, #46993, #19533, #54634, #75369 ),
 .UNSPECIFIED., .F., .F.,
 ( 4, 2, 2, 2, 4 ),
 ( 0.000000000000000000, 0.0001954339857564091278, 0.0003908679715128182556, 0.0005863019572692274375, 0.0007817359430256365111 ),
 .UNSPECIFIED. ) ;
#65211=ADVANCED_FACE ( 'NONE', ( #55028 ), #27556, .F. ) ;
#65213=ADVANCED_FACE ( 'NONE', ( #60891 ), #7284, .F. ) ;
#65214=AXIS2_PLACEMENT_3D ( 'NONE', #3978, #86437, #24708 ) ;
#65215=DIRECTION ( 'NONE',  ( -0.000000000000000000, -0.1736481776669307198, -0.9848077530122080203 ) ) ;
#65216=CARTESIAN_POINT ( 'NONE',  ( 9.692307692307695177, -3.937682226553329556, 33.60647404775216529 ) ) ;
#65217=CARTESIAN_POINT ( 'NONE',  ( 2.373760658694747061, -5.557115091759786019, 34.35708131394839882 ) ) ;
#65218=EDGE_CURVE ( 'NONE', #82401, #57426, #55644, .T. ) ;
#65219=CARTESIAN_POINT ( 'NONE',  ( 2.307692307692309264, -6.189225973068211317, 35.74407628777942847 ) ) ;
#65220=VERTEX_POINT ( 'NONE', #61319 ) ;
#65221=ORIENTED_EDGE ( 'NONE', *, *, #17848, .T. ) ;
#65223=VERTEX_POINT ( 'NONE', #54124 ) ;
#65224=B_SPLINE_CURVE_WITH_KNOTS ( 'NONE', 3,
 ( #10894, #45558, #24841, #65385, #85667, #64934 ),
 .UNSPECIFIED., .F., .F.,
 ( 4, 2, 4 ),
 ( 0.000000000000000000, 0.2499999999999978906, 0.4999999999999957812 ),
 .UNSPECIFIED. ) ;
#65225=CARTESIAN_POINT ( 'NONE',  ( 9.915087233576103998, -12.44528174975671853, 30.48912976160716681 ) ) ;
#65226=B_SPLINE_CURVE_WITH_KNOTS ( 'NONE', 3,
 ( #4797, #79571, #5234, #33148, #60167, #46663, #17867, #66495, #80006, #45320 ),
 .UNSPECIFIED., .F., .F.,
 ( 4, 2, 2, 2, 4 ),
 ( 0.0007817246256747484735, 0.0009771112852218928873, 0.001172497944769037084, 0.001367884604316181498, 0.001563271263863325912 ),
 .UNSPECIFIED. ) ;
#65227=CARTESIAN_POINT ( 'NONE',  ( -8.703162418228330921, -12.37446782046654192, 30.86335684631486842 ) ) ;
#65228=CARTESIAN_POINT ( 'NONE',  ( 13.51514082284903218, -10.31582465632705237, 34.18122507451815295 ) ) ;
#65229=ORIENTED_EDGE ( 'NONE', *, *, #69921, .F. ) ;
#65230=EDGE_CURVE ( 'NONE', #50666, #56147, #24550, .T. ) ;
#65231=VERTEX_POINT ( 'NONE', #67658 ) ;
#65232=EDGE_CURVE ( 'NONE', #59481, #4425, #66513, .T. ) ;
#65233=VECTOR ( 'NONE', #7340, 1000.000000000000114 ) ;
#65234=ORIENTED_EDGE ( 'NONE', *, *, #33504, .T. ) ;
#65235=CARTESIAN_POINT ( 'NONE',  ( -13.13461538461537259, -2.249999999999999112, 29.81603969181032454 ) ) ;
#65236=VERTEX_POINT ( 'NONE', #62220 ) ;
#65237=CARTESIAN_POINT ( 'NONE',  ( -0.6844646790546077275, -10.61292498521070549, 33.66303323003028680 ) ) ;
#65239=ORIENTED_EDGE ( 'NONE', *, *, #84572, .T. ) ;
#65240=CARTESIAN_POINT ( 'NONE',  ( -13.38461538461538325, -4.098570777380720287, 33.41473453929634729 ) ) ;
#65241=DIRECTION ( 'NONE',  ( -0.000000000000000000, -0.1736481776669307198, -0.9848077530122080203 ) ) ;
#65242=CARTESIAN_POINT ( 'NONE',  ( -6.000000000000121680, -3.643525952248796163, 33.31231777344771672 ) ) ;
#65243=FACE_BOUND ( 'NONE', #89177, .T. ) ;
#65244=CARTESIAN_POINT ( 'NONE',  ( 15.00784301325307979, -5.667676309546437530, 34.40238873228292249 ) ) ;
#65245=CARTESIAN_POINT ( 'NONE',  ( 2.530703659305157949, -8.239487800360276282, 34.69522927552633718 ) ) ;
#65246=CARTESIAN_POINT ( 'NONE',  ( 13.25446741488368829, -12.70455904226513866, 30.44083106164009322 ) ) ;
#65248=DIRECTION ( 'NONE',  ( 0.000000000000000000, 0.8660254037844377084, 0.5000000000000015543 ) ) ;
#65249=CARTESIAN_POINT ( 'NONE',  ( 17.77651507543566822, -6.716662450894490988, 34.94144148231605840 ) ) ;
#65251=ORIENTED_EDGE ( 'NONE', *, *, #37149, .F. ) ;
#65252=CARTESIAN_POINT ( 'NONE',  ( 10.54930120442873331, -10.51840700105979387, 33.73612834413961536 ) ) ;
#65253=ORIENTED_EDGE ( 'NONE', *, *, #38015, .F. ) ;
#65254=VERTEX_POINT ( 'NONE', #49148 ) ;
#65255=CARTESIAN_POINT ( 'NONE',  ( -2.307692307692305711, -1.044019251281081972, 31.83374038241031911 ) ) ;
#65256=CARTESIAN_POINT ( 'NONE',  ( 10.61538461538461675, -12.62096338111211580, 30.90682066428153263 ) ) ;
#65257=CARTESIAN_POINT ( 'NONE',  ( -5.933931648997561759, -6.386643153685127139, 34.62446782046654192 ) ) ;
#65259=CARTESIAN_POINT ( 'NONE',  ( 14.43821774592595197, -11.66157788607254098, 32.95092075102925833 ) ) ;
#65262=B_SPLINE_CURVE_WITH_KNOTS ( 'NONE', 3,
 ( #4990, #58137, #25251, #3636, #65781, #32451, #10854, #38323, #72996, #86984 ),
 .UNSPECIFIED., .F., .F.,
 ( 4, 2, 2, 2, 4 ),
 ( 0.000000000000000000, 0.0001954339857564090194, 0.0003908679715128180387, 0.0005863019572692270039, 0.0007817359430256360774 ),
 .UNSPECIFIED. ) ;
#65264=EDGE_CURVE ( 'NONE', #46286, #2856, #967, .T. ) ;
#65265=EDGE_CURVE ( 'NONE', #25396, #31453, #82, .T. ) ;
#65266=CARTESIAN_POINT ( 'NONE',  ( 0.2115152373170028632, -12.68155406624981119, 30.59749803192733708 ) ) ;
#65267=DIRECTION ( 'NONE',  ( 0.000000000000000000, 0.9848077530122072432, 0.1736481776669354937 ) ) ;
#65268=CARTESIAN_POINT ( 'NONE',  ( 0.3962684609821410242, -3.643525952247789412, 33.31231777344662959 ) ) ;
#65270=DIRECTION ( 'NONE',  ( 0.000000000000000000, 0.7660444431189822323, -0.6427876096865344779 ) ) ;
#65275=AXIS2_PLACEMENT_3D ( 'NONE', #74692, #17966, #81454 ) ;
#65276=CARTESIAN_POINT ( 'NONE',  ( -14.30769230769242917, -5.094484230521993062, 34.41647553114689373 ) ) ;
#65277=EDGE_CURVE ( 'NONE', #72566, #26386, #50209, .T. ) ;
#65279=FACE_OUTER_BOUND ( 'NONE', #55230, .T. ) ;
#65281=CARTESIAN_POINT ( 'NONE',  ( 4.023155550735848074, -10.70098750199973203, 33.91152734681376302 ) ) ;
#65282=CARTESIAN_POINT ( 'NONE',  ( 3.230769230769231726, -12.29105614889573062, 35.45975837776705220 ) ) ;
#65284=CARTESIAN_POINT ( 'NONE',  ( -13.51476259405360203, -8.587444163452046197, 34.63053765926554206 ) ) ;
#65285=EDGE_LOOP ( 'NONE', ( #7986, #48642, #24830, #85434 ) ) ;
#65286=ADVANCED_FACE ( 'NONE', ( #1410 ), #42411, .F. ) ;
#65287=FACE_OUTER_BOUND ( 'NONE', #18041, .T. ) ;
#65288=CARTESIAN_POINT ( 'NONE',  ( -1.384615384615505151, -9.442884908241554243, 34.35708131394783038 ) ) ;
#65289=ORIENTED_EDGE ( 'NONE', *, *, #78573, .T. ) ;
#65290=CARTESIAN_POINT ( 'NONE',  ( -9.468881293392906073, -7.630147987733840509, 34.99859428049665411 ) ) ;
#65291=CARTESIAN_POINT ( 'NONE',  ( 3.361561038594015116, -2.729792928343269587, 31.24908615093345077 ) ) ;
#65293=FACE_OUTER_BOUND ( 'NONE', #4624, .T. ) ;
#65294=CARTESIAN_POINT ( 'NONE',  ( 10.61538461538449596, -2.892918686052165622, 31.69288490824153470 ) ) ;
#65295=CARTESIAN_POINT ( 'NONE',  ( -3.230769230769351186, -11.48612834414049644, 32.76840700105863391 ) ) ;
#65297=EDGE_CURVE ( 'NONE', #76436, #25676, #63546, .T. ) ;
#65299=ORIENTED_EDGE ( 'NONE', *, *, #3736, .T. ) ;
#65300=FACE_OUTER_BOUND ( 'NONE', #20717, .T. ) ;
#65301=CARTESIAN_POINT ( 'NONE',  ( -12.71153846153846168, -7.500000000000001776, 34.75000000000000000 ) ) ;
#65304=CARTESIAN_POINT ( 'NONE',  ( -15.93106648486808119, -11.60474049983370648, 33.02348890104160262 ) ) ;
#65305=CARTESIAN_POINT ( 'NONE',  ( 2.307692307692309264, -11.91647553114624181, 32.58852847137148245 ) ) ;
#65306=ADVANCED_FACE ( 'NONE', ( #83845 ), #85600, .F. ) ;
#65307=ORIENTED_EDGE ( 'NONE', *, *, #27918, .F. ) ;
#65309=CARTESIAN_POINT ( 'NONE',  ( -15.23076923076922995, -3.937682226553329556, 33.60647404775216529 ) ) ;
#65310=B_SPLINE_CURVE_WITH_KNOTS ( 'NONE', 3,
 ( #16954, #77764, #15631, #43975, #57048, #3432, #10204, #65126, #51152, #83662 ),
 .UNSPECIFIED., .F., .F.,
 ( 4, 2, 2, 2, 4 ),
 ( 0.0007817359430256322827, 0.0009771253907249989254, 0.001172514838424365676, 0.001367904286123732428, 0.001563293733823098962 ),
 .UNSPECIFIED. ) ;
#65311=ORIENTED_EDGE ( 'NONE', *, *, #31104, .F. ) ;
#65312=VECTOR ( 'NONE', #60612, 999.9999999999998863 ) ;
#65313=DIRECTION ( 'NONE',  ( 0.000000000000000000, 0.9848077530122072432, 0.1736481776669354937 ) ) ;
#65314=ORIENTED_EDGE ( 'NONE', *, *, #23798, .T. ) ;
#65316=CARTESIAN_POINT ( 'NONE',  ( -1.634592128663974187, -12.01397095200673881, 32.43157075238190146 ) ) ;
#65317=CARTESIAN_POINT ( 'NONE',  ( -1.607541602131530745, -4.186968288167446595, 33.49512374952580274 ) ) ;
#65318=ORIENTED_EDGE ( 'NONE', *, *, #46259, .T. ) ;
#65319=CARTESIAN_POINT ( 'NONE',  ( -10.61538461538461320, -12.37446782046654192, 30.86335684631486131 ) ) ;
#65321=CARTESIAN_POINT ( 'NONE',  ( -18.00000000000000000, -12.10708131394839349, 31.69288490824020244 ) ) ;
#65322=EDGE_CURVE ( 'NONE', #66893, #67169, #42848, .T. ) ;
#65325=CARTESIAN_POINT ( 'NONE',  ( 0.4615384615384611200, -11.16473453929635440, 33.15142922261926373 ) ) ;
#65326=VERTEX_POINT ( 'NONE', #49598 ) ;
#65327=CARTESIAN_POINT ( 'NONE',  ( -5.869474298236436738, -11.46989282347013095, 32.79007818306219946 ) ) ;
#65328=CARTESIAN_POINT ( 'NONE',  ( -24.00000000000000000, 0.000000000000000000, 0.000000000000000000 ) ) ;
#65329=CARTESIAN_POINT ( 'NONE',  ( 0.3313912521002408407, -4.460286881179643892, 33.72017969459903952 ) ) ;
#65330=ADVANCED_FACE ( 'NONE', ( #8624 ), #28900, .F. ) ;
#65332=CARTESIAN_POINT ( 'NONE',  ( -7.976844449264153702, -12.62707690430377383, 30.88035979386743435 ) ) ;
#65333=ORIENTED_EDGE ( 'NONE', *, *, #52743, .T. ) ;
#65334=ORIENTED_EDGE ( 'NONE', *, *, #39444, .T. ) ;
#65335=EDGE_CURVE ( 'NONE', #23814, #50087, #36955, .T. ) ;
#65336=ORIENTED_EDGE ( 'NONE', *, *, #75899, .F. ) ;
#65337=CARTESIAN_POINT ( 'NONE',  ( 3.007284306204901281, -5.827078755546623690, 34.72654668319379567 ) ) ;
#65338=VERTEX_POINT ( 'NONE', #71626 ) ;
#65341=VECTOR ( 'NONE', #72708, 1000.000000000000000 ) ;
#65342=B_SPLINE_CURVE_WITH_KNOTS ( 'NONE', 3,
 ( #21542, #14344, #54893, #62087, #49016, #22431, #76495, #21090, #14800, #70175 ),
 .UNSPECIFIED., .F., .F.,
 ( 4, 2, 2, 2, 4 ),
 ( 0.0007817246256747473893, 0.0009771112852218905021, 0.001172497944769033615, 0.001367884604316176944, 0.001563271263863320057 ),
 .UNSPECIFIED. ) ;
#65343=CARTESIAN_POINT ( 'NONE',  ( 8.769230769230768274, -13.20930481340135110, 34.54067556320372745 ) ) ;
#65344=CYLINDRICAL_SURFACE ( 'NONE', #75515, 0.2500000000000009437 ) ;
#65345=VERTEX_POINT ( 'NONE', #77509 ) ;
#65346=EDGE_CURVE ( 'NONE', #64886, #63896, #1884, .T. ) ;
#65347=ORIENTED_EDGE ( 'NONE', *, *, #49318, .T. ) ;
#65348=EDGE_CURVE ( 'NONE', #64427, #83601, #31890, .T. ) ;
#65349=ORIENTED_EDGE ( 'NONE', *, *, #19806, .T. ) ;
#65350=CARTESIAN_POINT ( 'NONE',  ( 15.23076923076923173, -10.51840700105979565, 33.73612834413961536 ) ) ;
#65351=VERTEX_POINT ( 'NONE', #84731 ) ;
#65352=DIRECTION ( 'NONE',  ( 0.000000000000000000, 0.9396926207859126468, -0.3420201433256571111 ) ) ;
#65354=CARTESIAN_POINT ( 'NONE',  ( 17.07692307692307665, -2.833524468853757305, 32.15551576947925838 ) ) ;
#65355=CARTESIAN_POINT ( 'NONE',  ( 0.2115152242454959031, -5.056417327199099532, 34.11270091957321426 ) ) ;
#65356=B_SPLINE_CURVE_WITH_KNOTS ( 'NONE', 3,
 ( #68651, #6074, #40308, #41628, #76291, #33095, #40750, #88507, #88076, #67333 ),
 .UNSPECIFIED., .F., .F.,
 ( 4, 2, 2, 2, 4 ),
 ( 0.0007817246256747448956, 0.0009771112852218876831, 0.001172497944769030579, 0.001367884604316173475, 0.001563271263863316371 ),
 .UNSPECIFIED. ) ;
#65357=FACE_BOUND ( 'NONE', #19033, .T. ) ;
#65360=CARTESIAN_POINT ( 'NONE',  ( 13.60762673622823726, -9.086983370893049639, 34.49168942202179267 ) ) ;
#65361=DIRECTION ( 'NONE',  ( 0.000000000000000000, 0.9848077530122072432, -0.1736481776669354937 ) ) ;
#65362=CARTESIAN_POINT ( 'NONE',  ( -13.38461538461538325, -2.721908614388771852, 31.22303859784724978 ) ) ;
#65364=ORIENTED_EDGE ( 'NONE', *, *, #9294, .T. ) ;
#65366=ORIENTED_EDGE ( 'NONE', *, *, #33984, .F. ) ;
#65367=ORIENTED_EDGE ( 'NONE', *, *, #77275, .T. ) ;
#65368=CARTESIAN_POINT ( 'NONE',  ( -0.7115151924808159611, -9.148715823498378086, 34.47080413974185120 ) ) ;
#65369=CARTESIAN_POINT ( 'NONE',  ( -1.384615384615506484, -5.941354392335915335, 34.76329471203413846 ) ) ;
#65370=DIRECTION ( 'NONE',  ( -0.000000000000000000, -0.1736481776669307198, -0.9848077530122080203 ) ) ;
#65372=DIRECTION ( 'NONE',  ( -0.000000000000000000, -0.9848077530122086864, -0.1736481776669273613 ) ) ;
#65373=CARTESIAN_POINT ( 'NONE',  ( -12.21148414990014963, -4.235687564193447052, 33.53795663066793509 ) ) ;
#65374=ORIENTED_EDGE ( 'NONE', *, *, #70616, .T. ) ;
#65375=CARTESIAN_POINT ( 'NONE',  ( 6.673053698855461846, -2.588893531581426544, 31.60682220781847818 ) ) ;
#65376=CARTESIAN_POINT ( 'NONE',  ( -0.3307480205715102595, -3.338503747796865095, 32.95102852606552801 ) ) ;
#65378=CARTESIAN_POINT ( 'NONE',  ( -4.087777802843714170, -3.513871655860379306, 32.76840700105978499 ) ) ;
#65379=B_SPLINE_CURVE_WITH_KNOTS ( 'NONE', 3,
 ( #24410, #44225, #44674, #51874, #17675, #71712, #9574, #30729, #37037, #10017 ),
 .UNSPECIFIED., .F., .F.,
 ( 4, 2, 2, 2, 4 ),
 ( 0.000000000000000000, 0.0001954311564186862510, 0.0003908623128373725020, 0.0005862934692560588072, 0.0007817246256747450040 ),
 .UNSPECIFIED. ) ;
#65380=VERTEX_POINT ( 'NONE', #57242 ) ;
#65381=B_SPLINE_CURVE_WITH_KNOTS ( 'NONE', 3,
 ( #43825, #77618, #77175, #15484, #64974, #57344, #16360, #37961, #70425, #50134 ),
 .UNSPECIFIED., .F., .F.,
 ( 4, 2, 2, 2, 4 ),
 ( 0.000000000000000000, 0.0001954339857564097241, 0.0003908679715128194482, 0.0005863019572692291723, 0.0007817359430256388964 ),
 .UNSPECIFIED. ) ;
#65382=ORIENTED_EDGE ( 'NONE', *, *, #65852, .F. ) ;
#65383=FACE_BOUND ( 'NONE', #26135, .T. ) ;
#65384=ORIENTED_EDGE ( 'NONE', *, *, #25664, .T. ) ;
#65385=CARTESIAN_POINT ( 'NONE',  ( -17.87165453592967879, -2.254606617072892671, 29.97517285561840339 ) ) ;
#65386=CARTESIAN_POINT ( 'NONE',  ( -1.319360245102545681, -2.379036618887895305, 30.90682066428159303 ) ) ;
#65387=ORIENTED_EDGE ( 'NONE', *, *, #72458, .F. ) ;
#65388=CARTESIAN_POINT ( 'NONE',  ( -3.453695448285377445, -12.39988816332205701, 30.74660775122750778 ) ) ;
#65389=CARTESIAN_POINT ( 'NONE',  ( 15.23076923076910916, -3.083524468854526912, 32.58852847137268327 ) ) ;
#65390=CARTESIAN_POINT ( 'NONE',  ( 15.90386942290380290, -8.303909089506435137, 34.68538101551103381 ) ) ;
#65391=CARTESIAN_POINT ( 'NONE',  ( 4.376625822824220080, -6.717445702608402236, 34.94155399931962336 ) ) ;
#65392=VERTEX_POINT ( 'NONE', #50467 ) ;
#65393=CARTESIAN_POINT ( 'NONE',  ( -3.903900635498010807, -6.696923467548660192, 34.68552623307873972 ) ) ;
#65394=ORIENTED_EDGE ( 'NONE', *, *, #57592, .T. ) ;
#65395=EDGE_CURVE ( 'NONE', #10508, #6055, #9397, .T. ) ;
#65397=ORIENTED_EDGE ( 'NONE', *, *, #46940, .T. ) ;
#65398=CARTESIAN_POINT ( 'NONE',  ( -8.769230769230768274, -9.780366693483667717, 34.19971097300155094 ) ) ;
#65399=CARTESIAN_POINT ( 'NONE',  ( -12.52680846209478460, -3.083524468853724443, 32.58852847137143272 ) ) ;
#65400=CYLINDRICAL_SURFACE ( 'NONE', #55906, 0.2500000000000002220 ) ;
#65401=CARTESIAN_POINT ( 'NONE',  ( 10.54930223602447903, -12.34228464037088280, 31.77849191805838558 ) ) ;
#65403=CARTESIAN_POINT ( 'NONE',  ( 4.153846153846154188, -9.584722331328613620, 36.20867863119891439 ) ) ;
#65404=ADVANCED_FACE ( 'NONE', ( #38747 ), #18481, .F. ) ;
#65406=ORIENTED_EDGE ( 'NONE', *, *, #38853, .T. ) ;
#65407=DIRECTION ( 'NONE',  ( -0.000000000000000000, 0.9396926207859092051, -0.3420201433256662704 ) ) ;
#65408=CARTESIAN_POINT ( 'NONE',  ( -18.00000000000000000, -6.190371309867714444, 35.73758076001107042 ) ) ;
#65411=B_SPLINE_CURVE_WITH_KNOTS ( 'NONE', 3,
 ( #40577, #68045, #81562, #11767, #59500, #47312, #46431, #74805, #73915, #13095 ),
 .UNSPECIFIED., .F., .F.,
 ( 4, 2, 2, 2, 4 ),
 ( 0.0007817359430256313069, 0.0009771253907249971907, 0.001172514838424363074, 0.001367904286123728958, 0.001563293733823094842 ),
 .UNSPECIFIED. ) ;
#65412=ORIENTED_EDGE ( 'NONE', *, *, #84715, .T. ) ;
#65413=ORIENTED_EDGE ( 'NONE', *, *, #39982, .T. ) ;
#65414=CARTESIAN_POINT ( 'NONE',  ( -1.607480806819022945, -2.501496062324912284, 29.88072118266895671 ) ) ;
#65415=CARTESIAN_POINT ( 'NONE',  ( 11.53846153846141576, -5.094484230521993062, 34.41647553114689373 ) ) ;
#65416=CARTESIAN_POINT ( 'NONE',  ( 17.29970274590113632, -3.563462043263029955, 33.22394488606062879 ) ) ;
#65417=B_SPLINE_CURVE_WITH_KNOTS ( 'NONE', 3,
 ( #11084, #79987, #32250, #75769, #80443, #45754 ),
 .UNSPECIFIED., .F., .F.,
 ( 4, 2, 4 ),
 ( 0.0003909569690057805385, 0.0005862646681846044039, 0.0007815723673634283235 ),
 .UNSPECIFIED. ) ;
#65418=CARTESIAN_POINT ( 'NONE',  ( 10.61538461538461675, -3.886160181151819604, 36.00935417666054406 ) ) ;
#65419=CARTESIAN_POINT ( 'NONE',  ( 15.93036122928182330, -10.23692288466677880, 34.23039457007281072 ) ) ;
#65421=B_SPLINE_CURVE_WITH_KNOTS ( 'NONE', 3,
 ( #54623, #40692, #6458, #33918, #47878, #27163, #82119, #75359, #13649, #29831 ),
 .UNSPECIFIED., .F., .F.,
 ( 4, 2, 2, 2, 4 ),
 ( 0.000000000000000000, 0.0001954339857564054957, 0.0003908679715128109914, 0.0005863019572692164871, 0.0007817359430256219828 ),
 .UNSPECIFIED. ) ;
#65422=CARTESIAN_POINT ( 'NONE',  ( -16.85414340794500276, -11.60474049983370648, 33.02348890104160262 ) ) ;
#65423=CARTESIAN_POINT ( 'NONE',  ( -7.146561866800870355, -11.89387501736622710, 32.13663884655806413 ) ) ;
#65424=VERTEX_POINT ( 'NONE', #66210 ) ;
#65426=CARTESIAN_POINT ( 'NONE',  ( -0.2115929431903199320, -8.433404298154338008, 34.66254593164986630 ) ) ;
#65427=CARTESIAN_POINT ( 'NONE',  ( 7.053867364043874488, -6.369690395747422684, 34.87708834333098196 ) ) ;
#65428=FACE_OUTER_BOUND ( 'NONE', #25249, .T. ) ;
#65429=VERTEX_POINT ( 'NONE', #32435 ) ;
#65430=CARTESIAN_POINT ( 'NONE',  ( 12.33139049180676139, -2.647304123082328875, 31.75400227202885972 ) ) ;
#65431=EDGE_CURVE ( 'NONE', #64420, #47909, #10512, .T. ) ;
#65432=EDGE_LOOP ( 'NONE', ( #82867, #16840 ) ) ;
#65433=CARTESIAN_POINT ( 'NONE',  ( 9.019285189144218506, -2.920487667080175598, 32.31805714834170828 ) ) ;
#65435=CARTESIAN_POINT ( 'NONE',  ( -13.16118898570059947, -7.630147987733840509, 34.99859428049665411 ) ) ;
#65436=DIRECTION ( 'NONE',  ( -0.000000000000000000, -0.9396926207859093161, -0.3420201433256663259 ) ) ;
#65437=EDGE_LOOP ( 'NONE', ( #13250, #61588, #58172, #78488 ) ) ;
#65438=ADVANCED_FACE ( 'NONE', ( #18922 ), #45494, .F. ) ;
#65439=CARTESIAN_POINT ( 'NONE',  ( -1.384615384615383471, -12.62096338111211580, 30.90682066428153263 ) ) ;
#65440=DIRECTION ( 'NONE',  ( -0.000000000000000000, -0.9848077530122085754, -0.1736481776669273613 ) ) ;
#65441=AXIS2_PLACEMENT_3D ( 'NONE', #64785, #3090, #10305 ) ;
#65442=CARTESIAN_POINT ( 'NONE',  ( 9.019230769230704325, -7.565270445406050648, 34.75000000000000000 ) ) ;
#65444=EDGE_CURVE ( 'NONE', #27705, #56750, #62024, .T. ) ;
#65445=EDGE_LOOP ( 'NONE', ( #4148, #81539, #85085, #1579 ) ) ;
#65446=CARTESIAN_POINT ( 'NONE',  ( -0.5922299282060203840, -8.147922237126337563, 34.70805685702651999 ) ) ;
#65447=EDGE_LOOP ( 'NONE', ( #74562, #19943, #29413, #3947 ) ) ;
#65448=CARTESIAN_POINT ( 'NONE',  ( 2.307692307692186251, -12.70778746994576025, 30.41441678777401236 ) ) ;
#65449=CARTESIAN_POINT ( 'NONE',  ( -9.442362173959551797, -12.22109172314383052, 31.39792113162168263 ) ) ;
#65450=CARTESIAN_POINT ( 'NONE',  ( -13.51476259405360558, -2.882441371585227508, 31.66841991370172238 ) ) ;
#65451=CARTESIAN_POINT ( 'NONE',  ( 7.780071466793708979, -12.34228464037088280, 31.77849191805838558 ) ) ;
#65453=CARTESIAN_POINT ( 'NONE',  ( 16.15384615384615330, -11.91647553114624181, 32.58852847137148245 ) ) ;
#65455=EDGE_LOOP ( 'NONE', ( #15122, #47696 ) ) ;
#65456=ORIENTED_EDGE ( 'NONE', *, *, #7387, .T. ) ;
#65457=ORIENTED_EDGE ( 'NONE', *, *, #72789, .F. ) ;
#65458=EDGE_CURVE ( 'NONE', #27369, #75057, #63132, .T. ) ;
#65460=VERTEX_POINT ( 'NONE', #72522 ) ;
#65463=CARTESIAN_POINT ( 'NONE',  ( -10.61538461538473399, -8.613356846316285953, 34.62446782046622218 ) ) ;
#65464=CARTESIAN_POINT ( 'NONE',  ( -3.453696189676077832, -6.459968553980839800, 34.89616026154728701 ) ) ;
#65465=CARTESIAN_POINT ( 'NONE',  ( -4.153846153846152411, -6.343179335718451384, 34.87096338111211935 ) ) ;
#65466=EDGE_CURVE ( 'NONE', #27738, #39506, #49106, .T. ) ;
#65467=CARTESIAN_POINT ( 'NONE',  ( -6.000000000000119904, -5.219633306517616589, 34.19971097300220464 ) ) ;
#65468=CARTESIAN_POINT ( 'NONE',  ( 7.780883845597526438, -12.70778746994557551, 30.41441678777548319 ) ) ;
#65470=DIRECTION ( 'NONE',  ( 0.000000000000000000, 0.3420201433256610524, 0.9396926207859113145 ) ) ;
#65471=CARTESIAN_POINT ( 'NONE',  ( -17.86920819217521483, -6.413143153341454017, 34.63066358083362672 ) ) ;
#65472=CARTESIAN_POINT ( 'NONE',  ( -4.219929564802034072, -9.780366693483667717, 34.19971097300155805 ) ) ;
#65473=VERTEX_POINT ( 'NONE', #43993 ) ;
#65474=AXIS2_PLACEMENT_3D ( 'NONE', #62898, #76435, #51478 ) ;
#65475=EDGE_LOOP ( 'NONE', ( #73666, #49919, #53212, #34375 ) ) ;
#65476=ORIENTED_EDGE ( 'NONE', *, *, #73728, .F. ) ;
#65477=CARTESIAN_POINT ( 'NONE',  ( 0.2115617174898691832, -2.920706130388546651, 32.31842814019191223 ) ) ;
#65478=VERTEX_POINT ( 'NONE', #70145 ) ;
#65479=CARTESIAN_POINT ( 'NONE',  ( 3.230769230769231726, -5.415277668671390821, 36.20867863119892149 ) ) ;
#65480=CARTESIAN_POINT ( 'NONE',  ( -17.74994558008654622, -11.47946981652013321, 33.17500667209846910 ) ) ;
#65481=CARTESIAN_POINT ( 'NONE',  ( -1.514763354347081092, -5.070767119584671967, 34.40440758774516183 ) ) ;
#65482=CARTESIAN_POINT ( 'NONE',  ( -11.31544869436814338, -9.172514111537584114, 34.72667873470787470 ) ) ;
#65483=ORIENTED_EDGE ( 'NONE', *, *, #81712, .F. ) ;
#65484=ORIENTED_EDGE ( 'NONE', *, *, #12855, .T. ) ;
#65485=CARTESIAN_POINT ( 'NONE',  ( -2.437839517130525824, -12.45813303252208648, 30.39737893381572675 ) ) ;
#65486=ORIENTED_EDGE ( 'NONE', *, *, #87282, .T. ) ;
#65487=FACE_BOUND ( 'NONE', #72878, .T. ) ;
#65488=CARTESIAN_POINT ( 'NONE',  ( 15.23076923076923173, -9.780366693483667717, 34.19971097300155094 ) ) ;
#65489=CARTESIAN_POINT ( 'NONE',  ( 16.15384615384615330, -6.386643153685126251, 34.62446782046654192 ) ) ;
#65490=VERTEX_POINT ( 'NONE', #85000 ) ;
#65491=CARTESIAN_POINT ( 'NONE',  ( 14.05771557674995798, -2.779195860258146578, 31.39871582349836032 ) ) ;
#65492=CARTESIAN_POINT ( 'NONE',  ( -6.792286482109973988, -2.295524264805589354, 30.44142389570982488 ) ) ;
#65493=CARTESIAN_POINT ( 'NONE',  ( -9.692307692307691624, -13.49023893513002648, 31.06009739812518688 ) ) ;
#65494=ORIENTED_EDGE ( 'NONE', *, *, #54246, .F. ) ;
#65495=CARTESIAN_POINT ( 'NONE',  ( 18.25000000000141753, -7.500000000000154543, 35.00000000000007105 ) ) ;
#65496=DIRECTION ( 'NONE',  ( -0.000000000000000000, 1.000000000000000000, 3.491481338843133355E-15 ) ) ;
#65497=ORIENTED_EDGE ( 'NONE', *, *, #51398, .F. ) ;
#65498=CARTESIAN_POINT ( 'NONE',  ( 3.230769230769110045, -8.613356846316285953, 34.62446782046622218 ) ) ;
#65499=LINE ( 'NONE', #5141, #45610 ) ;
#65500=EDGE_LOOP ( 'NONE', ( #33869, #81858, #12941, #88458 ) ) ;
#65501=CARTESIAN_POINT ( 'NONE',  ( 7.173022332454966232, -2.589246495874657938, 31.60778113518102828 ) ) ;
#65502=CARTESIAN_POINT ( 'NONE',  ( 13.16168916709923664, -2.554751324335735152, 30.48935550225260727 ) ) ;
#65504=CARTESIAN_POINT ( 'NONE',  ( 7.715677138037380978, -7.276988635370448932, 34.74523720219453793 ) ) ;
#65505=FACE_OUTER_BOUND ( 'NONE', #30437, .T. ) ;
#65506=CARTESIAN_POINT ( 'NONE',  ( 6.857806477116148436, -9.442884908240170461, 34.35708131394840592 ) ) ;
#65507=CARTESIAN_POINT ( 'NONE',  ( -8.769230769230455635, -2.255955759149395501, 30.00000000000324363 ) ) ;
#65509=CARTESIAN_POINT ( 'NONE',  ( 1.384615384615265343, -11.48612834414049644, 32.76840700105863391 ) ) ;
#65510=CARTESIAN_POINT ( 'NONE',  ( 3.480769230769230838, -2.499999999999998668, 29.75000000000000355 ) ) ;
#65511=CARTESIAN_POINT ( 'NONE',  ( -10.68065506134539078, -8.613356846314824011, 34.62446782046655613 ) ) ;
#65513=ORIENTED_EDGE ( 'NONE', *, *, #87657, .F. ) ;
#65514=CARTESIAN_POINT ( 'NONE',  ( 17.99999999999987566, -11.94971097300221174, 32.03036669348237098 ) ) ;
#65516=B_SPLINE_CURVE_WITH_KNOTS ( 'NONE', 3,
 ( #35067, #48572, #13910, #84162, #49904, #34630, #77383, #54902, #82384, #7606 ),
 .UNSPECIFIED., .F., .F.,
 ( 4, 2, 2, 2, 4 ),
 ( 0.0007817359430256398721, 0.0009771253907250084664, 0.001172514838424377169, 0.001367904286123745872, 0.001563293733823114574 ),
 .UNSPECIFIED. ) ;
#65517=ORIENTED_EDGE ( 'NONE', *, *, #28306, .F. ) ;
#65518=CARTESIAN_POINT ( 'NONE',  ( -2.057637996053991447, -12.41262288849542017, 30.68299917996395010 ) ) ;
#65519=ORIENTED_EDGE ( 'NONE', *, *, #35893, .F. ) ;
#65520=LINE ( 'NONE', #4268, #39764 ) ;
#65522=CARTESIAN_POINT ( 'NONE',  ( -15.23076923076935074, -4.481592998941358097, 33.73612834414048933 ) ) ;
#65523=CARTESIAN_POINT ( 'NONE',  ( -6.000000000000121680, -11.67786785259630911, 32.92929555188603530 ) ) ;
#65524=CARTESIAN_POINT ( 'NONE',  ( -5.749945688361683516, -9.148310452688871663, 34.47095581063188519 ) ) ;
#65525=CARTESIAN_POINT ( 'NONE',  ( -14.37377468705243899, -10.67929555188718460, 33.92786785259543336 ) ) ;
#65526=CYLINDRICAL_SURFACE ( 'NONE', #67684, 0.2500000000000009437 ) ;
#65527=CARTESIAN_POINT ( 'NONE',  ( -7.780898274877821486, -2.892918686051624722, 31.69288490824025928 ) ) ;
#65528=CYLINDRICAL_SURFACE ( 'NONE', #64080, 0.2499999999999995837 ) ;
#65530=VECTOR ( 'NONE', #73000, 1000.000000000000227 ) ;
#65531=DIRECTION ( 'NONE',  ( -0.000000000000000000, 1.000000000000000000, 3.491481338843133355E-15 ) ) ;
#65532=CARTESIAN_POINT ( 'NONE',  ( 13.25392478150507891, -3.338472653186243644, 32.95098750199972670 ) ) ;
#65533=CARTESIAN_POINT ( 'NONE',  ( 14.37294787896833270, -3.300289026998473041, 32.46337939537591666 ) ) ;
#65534=EDGE_CURVE ( 'NONE', #5535, #57873, #88856, .T. ) ;
#65537=CARTESIAN_POINT ( 'NONE',  ( 0.4615384615384611200, -6.435427911321262684, 35.78748833219616898 ) ) ;
#65538=CARTESIAN_POINT ( 'NONE',  ( 7.780070435197966816, -11.16473453929635440, 33.15142922261925662 ) ) ;
#65541=CARTESIAN_POINT ( 'NONE',  ( 14.17700170458200404, -3.338472653186243644, 32.95098750199972670 ) ) ;
#65542=DIRECTION ( 'NONE',  ( 0.000000000000000000, 0.1736481776669267785, -0.9848077530122087975 ) ) ;
#65544=EDGE_LOOP ( 'NONE', ( #53047, #21012, #8082, #77461 ) ) ;
#65545=CARTESIAN_POINT ( 'NONE',  ( -1.134669866267242755, -10.05730279482229683, 34.04704008940765902 ) ) ;
#65546=ORIENTED_EDGE ( 'NONE', *, *, #36721, .F. ) ;
#65547=ORIENTED_EDGE ( 'NONE', *, *, #13104, .T. ) ;
#65548=CARTESIAN_POINT ( 'NONE',  ( 7.622668921589514035, -10.97335522853832579, 33.68706563782419749 ) ) ;
#65549=CARTESIAN_POINT ( 'NONE',  ( -6.673022503163469565, -5.642605341092957083, 34.66089969410670335 ) ) ;
#65550=CARTESIAN_POINT ( 'NONE',  ( -9.442253380669381357, -6.567000820036036579, 34.66262288849541306 ) ) ;
#65551=CARTESIAN_POINT ( 'NONE',  ( -6.222926217516147496, -3.105860786376062332, 32.13614157043599562 ) ) ;
#65552=CARTESIAN_POINT ( 'NONE',  ( -13.13466986626724164, -3.202959910592335646, 32.30730279482227019 ) ) ;
#65553=AXIS2_PLACEMENT_3D ( 'NONE', #4954, #86950, #32419 ) ;
#65554=EDGE_LOOP ( 'NONE', ( #57971, #68227, #14773, #67352 ) ) ;
#65556=EDGE_CURVE ( 'NONE', #53195, #82297, #63383, .T. ) ;
#65558=ORIENTED_EDGE ( 'NONE', *, *, #82910, .T. ) ;
#65559=CARTESIAN_POINT ( 'NONE',  ( 13.13459216039393240, -4.931416488878822335, 34.32920672191015399 ) ) ;
#65560=CARTESIAN_POINT ( 'NONE',  ( -16.15384615384627409, -9.528491918059723176, 34.59228464037033035 ) ) ;
#65561=CARTESIAN_POINT ( 'NONE',  ( 9.692307692307695177, -11.16473453929635440, 33.15142922261926373 ) ) ;
#65562=CARTESIAN_POINT ( 'NONE',  ( -8.703975629717932705, -10.33852847137154107, 34.16647553114620450 ) ) ;
#65563=LINE ( 'NONE', #72326, #39331 ) ;
#65564=CARTESIAN_POINT ( 'NONE',  ( 17.74997676270703550, -8.432397168068783699, 34.66272746175022945 ) ) ;
#65566=EDGE_CURVE ( 'NONE', #88377, #20922, #53402, .T. ) ;
#65567=ORIENTED_EDGE ( 'NONE', *, *, #70060, .T. ) ;
#65569=ORIENTED_EDGE ( 'NONE', *, *, #78241, .F. ) ;
#65570=CARTESIAN_POINT ( 'NONE',  ( 15.36156103859402222, -5.582136614379148654, 34.36778462344220486 ) ) ;
#65571=ORIENTED_EDGE ( 'NONE', *, *, #15634, .T. ) ;
#65572=CARTESIAN_POINT ( 'NONE',  ( -10.61538461538473577, -4.320704448113951379, 33.92786785259630022 ) ) ;
#65573=DIRECTION ( 'NONE',  ( -0.000000000000000000, -0.3420201433256694346, -0.9396926207859080948 ) ) ;
#65576=VERTEX_POINT ( 'NONE', #77347 ) ;
#65577=CARTESIAN_POINT ( 'NONE',  ( 10.83816428436268176, -2.353885683473779800, 30.79025554430704403 ) ) ;
#65578=EDGE_LOOP ( 'NONE', ( #30407, #62243 ) ) ;
#65579=DIRECTION ( 'NONE',  ( -0.000000000000000000, 0.9848077530122086864, -0.1736481776669273891 ) ) ;
#65580=DIRECTION ( 'NONE',  ( -0.000000000000000000, 0.9848077530122086864, -0.1736481776669273891 ) ) ;
#65581=FACE_BOUND ( 'NONE', #77743, .T. ) ;
#65582=CARTESIAN_POINT ( 'NONE',  ( 5.869852030268303267, -12.50552854090298993, 31.33409797877408920 ) ) ;
#65583=CARTESIAN_POINT ( 'NONE',  ( 8.068933515131908152, -2.353885683473779800, 30.79025554430704403 ) ) ;
#65584=CARTESIAN_POINT ( 'NONE',  ( -3.230769230769229949, -3.322132147404559976, 32.92929555188717927 ) ) ;
#65585=CARTESIAN_POINT ( 'NONE',  ( -3.454254155333561283, -8.539481045369598178, 34.89627647299170832 ) ) ;
#65586=ORIENTED_EDGE ( 'NONE', *, *, #74511, .F. ) ;
#65587=CARTESIAN_POINT ( 'NONE',  ( 11.28843831424007860, -11.56360843649121861, 33.07473185843129926 ) ) ;
#65590=VERTEX_POINT ( 'NONE', #30485 ) ;
#65591=CARTESIAN_POINT ( 'NONE',  ( -12.46153846153846168, -9.780366693483667717, 34.19971097300155094 ) ) ;
#65592=CARTESIAN_POINT ( 'NONE',  ( 12.46153846153876898, -2.506253911140615021, 30.00000000000323297 ) ) ;
#65593=FACE_OUTER_BOUND ( 'NONE', #3447, .T. ) ;
#65594=CARTESIAN_POINT ( 'NONE',  ( 11.31497659473759043, -5.912607949931405926, 34.49155766932282319 ) ) ;
#65595=CYLINDRICAL_SURFACE ( 'NONE', #51553, 0.2500000000000009437 ) ;
#65596=FACE_BOUND ( 'NONE', #15022, .T. ) ;
#65597=CARTESIAN_POINT ( 'NONE',  ( 18.00000000000000000, -12.37446782046654192, 30.86335684631486131 ) ) ;
#65598=CARTESIAN_POINT ( 'NONE',  ( -10.54921800879297322, -7.250054591869670162, 34.99404684341514127 ) ) ;
#65599=CARTESIAN_POINT ( 'NONE',  ( -18.13014796973169851, -8.630895178749536711, 34.87696386517710323 ) ) ;
#65600=CARTESIAN_POINT ( 'NONE',  ( 18.22301135161285046, -11.24521262558773493, 33.06293181088029343 ) ) ;
#65601=CARTESIAN_POINT ( 'NONE',  ( 0.7115928814519136836, -2.920487667080175154, 32.31805714834170828 ) ) ;
#65602=CARTESIAN_POINT ( 'NONE',  ( 0.4615384615387678746, -2.506253911140615021, 30.00000000000323297 ) ) ;
#65603=FACE_OUTER_BOUND ( 'NONE', #39694, .T. ) ;
#65606=DIRECTION ( 'NONE',  ( -0.000000000000000000, -0.6427876096865404731, -0.7660444431189770143 ) ) ;
#65607=AXIS2_PLACEMENT_3D ( 'NONE', #3938, #30096, #57559 ) ;
#65608=CARTESIAN_POINT ( 'NONE',  ( 8.096099255531889582, -10.18230066228896114, 34.26354781536631577 ) ) ;
#65609=CARTESIAN_POINT ( 'NONE',  ( -2.307692307692305711, -3.886160181151819604, 36.00935417666054406 ) ) ;
#65610=CARTESIAN_POINT ( 'NONE',  ( -9.942330929600657896, -10.76384336483936011, 33.53834819971076087 ) ) ;
#65612=CYLINDRICAL_SURFACE ( 'NONE', #72853, 2.000000000000001776 ) ;
#65614=EDGE_CURVE ( 'NONE', #81377, #46553, #57957, .T. ) ;
#65615=CARTESIAN_POINT ( 'NONE',  ( -1.515090569691102562, -7.276987145209184327, 34.99546412871779211 ) ) ;
#65616=CARTESIAN_POINT ( 'NONE',  ( 0.5920641633020268246, -3.816742781228458448, 33.13167719472716044 ) ) ;
#65617=CARTESIAN_POINT ( 'NONE',  ( 11.40785188325745558, -7.722926974430166069, 34.99546784045485737 ) ) ;
#65618=CARTESIAN_POINT ( 'NONE',  ( 5.076923076923075762, -12.62096338111211580, 30.90682066428153263 ) ) ;
#65619=CARTESIAN_POINT ( 'NONE',  ( 8.546304551714619890, -9.886141570436013382, 34.14413921362392301 ) ) ;
#65620=CARTESIAN_POINT ( 'NONE',  ( 4.153846153846154188, -10.51840700105979565, 33.73612834413961536 ) ) ;
#65621=DIRECTION ( 'NONE',  ( -0.000000000000000000, 0.6427876096865404731, -0.7660444431189770143 ) ) ;
#65622=CARTESIAN_POINT ( 'NONE',  ( 7.912221179503920787, -9.058645607665452459, 34.76329471203371924 ) ) ;
#65623=ORIENTED_EDGE ( 'NONE', *, *, #77415, .T. ) ;
#65624=CARTESIAN_POINT ( 'NONE',  ( 3.453548899747294953, -12.47679350104403007, 31.42216943046555855 ) ) ;
#65625=CARTESIAN_POINT ( 'NONE',  ( 14.30769230769218758, -6.026961402154118019, 34.52809138561165270 ) ) ;
#65627=ADVANCED_FACE ( 'NONE', ( #29181 ), #10224, .F. ) ;
#65628=LINE ( 'NONE', #72394, #50468 ) ;
#65629=LINE ( 'NONE', #3931, #21036 ) ;
#65631=CARTESIAN_POINT ( 'NONE',  ( -6.923076923077045919, -10.33852847137269571, 34.16647553114546554 ) ) ;
#65632=CARTESIAN_POINT ( 'NONE',  ( -12.46153846153858424, -12.70778746994576025, 30.41441678777401236 ) ) ;
#65633=CARTESIAN_POINT ( 'NONE',  ( 11.53846153846153832, -2.833524468853757305, 32.15551576947925838 ) ) ;
#65634=ORIENTED_EDGE ( 'NONE', *, *, #35774, .F. ) ;
#65635=CARTESIAN_POINT ( 'NONE',  ( -13.60754234352223335, -10.01117774369187252, 34.36070679894347535 ) ) ;
#65636=CARTESIAN_POINT ( 'NONE',  ( 17.32692307692449418, -7.500000000000154543, 35.00000000000007105 ) ) ;
#65637=EDGE_CURVE ( 'NONE', #18061, #32348, #5086, .T. ) ;
#65638=B_SPLINE_CURVE_WITH_KNOTS ( 'NONE', 3,
 ( #80444, #58817, #51149, #59266, #87210, #52505, #39017, #71889, #31356, #10643 ),
 .UNSPECIFIED., .F., .F.,
 ( 4, 2, 2, 2, 4 ),
 ( 0.000000000000000000, 0.0001954339857564063089, 0.0003908679715128126177, 0.0005863019572692189808, 0.0007817359430256252354 ),
 .UNSPECIFIED. ) ;
#65639=CARTESIAN_POINT ( 'NONE',  ( -8.546451227962355901, -2.600157965045224451, 30.74683119005207743 ) ) ;
#65640=CARTESIAN_POINT ( 'NONE',  ( -14.17690049986751966, -11.18335022499818621, 33.13157742990016885 ) ) ;
#65641=ORIENTED_EDGE ( 'NONE', *, *, #40883, .F. ) ;
#65642=DIRECTION ( 'NONE',  ( -0.000000000000000000, -0.3420201433256694901, -0.9396926207859082059 ) ) ;
#65646=ORIENTED_EDGE ( 'NONE', *, *, #81933, .F. ) ;
#65647=ORIENTED_EDGE ( 'NONE', *, *, #71932, .F. ) ;
#65648=VERTEX_POINT ( 'NONE', #72798 ) ;
#65649=EDGE_CURVE ( 'NONE', #15172, #41806, #85637, .T. ) ;
#65650=CARTESIAN_POINT ( 'NONE',  ( -9.758391103263573285, -2.721908614388770964, 31.22303859784723912 ) ) ;
#65651=CARTESIAN_POINT ( 'NONE',  ( 16.15384615384615330, -1.951392089020283160, 34.73218667398347748 ) ) ;
#65652=AXIS2_PLACEMENT_3D ( 'NONE', #85478, #9380, #66080 ) ;
#65653=CARTESIAN_POINT ( 'NONE',  ( -5.999999999999998224, -13.78497067705608181, 32.30358669280327177 ) ) ;
#65654=CARTESIAN_POINT ( 'NONE',  ( 3.230769230769231726, -12.78798330534103123, 29.99999999999997868 ) ) ;
#65655=EDGE_CURVE ( 'NONE', #4047, #40157, #13226, .T. ) ;
#65656=ORIENTED_EDGE ( 'NONE', *, *, #87641, .F. ) ;
#65657=VECTOR ( 'NONE', #19792, 1000.000000000000000 ) ;
#65658=VERTEX_POINT ( 'NONE', #79575 ) ;
#65659=CARTESIAN_POINT ( 'NONE',  ( -18.00000000000012079, -8.656820664282943056, 34.87096338111179961 ) ) ;
#65661=ORIENTED_EDGE ( 'NONE', *, *, #70651, .T. ) ;
#65662=CARTESIAN_POINT ( 'NONE',  ( -14.24162497434223162, -11.35647404775217595, 33.31231777344666511 ) ) ;
#65664=EDGE_CURVE ( 'NONE', #36550, #16329, #62345, .T. ) ;
#65665=AXIS2_PLACEMENT_3D ( 'NONE', #45083, #74349, #39688 ) ;
#65666=EDGE_CURVE ( 'NONE', #71441, #23412, #54529, .T. ) ;
#65667=CARTESIAN_POINT ( 'NONE',  ( 1.384615384615386802, -10.51840700105979565, 33.73612834413961536 ) ) ;
#65668=CYLINDRICAL_SURFACE ( 'NONE', #46775, 0.2499999999999994726 ) ;
#65669=ORIENTED_EDGE ( 'NONE', *, *, #5798, .T. ) ;
#65670=ORIENTED_EDGE ( 'NONE', *, *, #7098, .T. ) ;
#65673=CARTESIAN_POINT ( 'NONE',  ( 5.326868595271217366, -5.057305518903949526, 34.11320923018887896 ) ) ;
#65674=ORIENTED_EDGE ( 'NONE', *, *, #44589, .T. ) ;
#65675=CARTESIAN_POINT ( 'NONE',  ( 2.980792499826877329, -11.79746400365624659, 32.30657167506340954 ) ) ;
#65676=CARTESIAN_POINT ( 'NONE',  ( 18.24994540937804643, -5.766571408460170467, 34.70601412856602508 ) ) ;
#65679=CARTESIAN_POINT ( 'NONE',  ( -8.835314180186646382, -10.51840700105979387, 33.73612834413961536 ) ) ;
#65680=CARTESIAN_POINT ( 'NONE',  ( 10.61538461538461675, -8.810774026931790459, 35.74407628777942847 ) ) ;
#65681=CARTESIAN_POINT ( 'NONE',  ( -6.923076923076922462, -12.78798330534102945, 29.74999999999997868 ) ) ;
#65682=FACE_BOUND ( 'NONE', #87344, .T. ) ;
#65683=CARTESIAN_POINT ( 'NONE',  ( -15.23076923076922995, -8.164416787775445883, 34.95778746994557906 ) ) ;
#65684=CARTESIAN_POINT ( 'NONE',  ( 9.561830984191230343, -7.276988635370452485, 34.74523720219453793 ) ) ;
#65685=CARTESIAN_POINT ( 'NONE',  ( -9.692307692307691624, -12.48256725967547354, 35.29906147534542527 ) ) ;
#65686=CARTESIAN_POINT ( 'NONE',  ( 3.296024370282069516, -3.643525952247864463, 33.31231777344670064 ) ) ;
#65687=CARTESIAN_POINT ( 'NONE',  ( -5.934744428723975673, -2.892918686051625166, 31.69288490824025928 ) ) ;
#65688=CARTESIAN_POINT ( 'NONE',  ( 6.923076923076924238, -12.34228464037088635, 31.77849191805839268 ) ) ;
#65690=ORIENTED_EDGE ( 'NONE', *, *, #58595, .F. ) ;
#65691=CARTESIAN_POINT ( 'NONE',  ( -16.08859101433330707, -3.643525952247864019, 33.31231777344670064 ) ) ;
#65692=CARTESIAN_POINT ( 'NONE',  ( -7.623374304885434327, -2.600157965045225339, 30.74683119005207743 ) ) ;
#65693=ORIENTED_EDGE ( 'NONE', *, *, #23928, .F. ) ;
#65694=ORIENTED_EDGE ( 'NONE', *, *, #61896, .F. ) ;
#65695=CARTESIAN_POINT ( 'NONE',  ( 5.933916589044120116, -6.386643153685125363, 34.62446782046654903 ) ) ;
#65696=CARTESIAN_POINT ( 'NONE',  ( 10.61538461538461675, -11.91647553114624181, 32.58852847137148245 ) ) ;
#65698=CARTESIAN_POINT ( 'NONE',  ( -17.07692307692307665, -1.790695186598648903, 34.54067556320373455 ) ) ;
#65701=EDGE_CURVE ( 'NONE', #83312, #4579, #65210, .T. ) ;
#65702=VECTOR ( 'NONE', #37062, 1000.000000000000227 ) ;
#65703=CARTESIAN_POINT ( 'NONE',  ( -18.00000000000000000, -13.92244064605451648, 31.82153278338624602 ) ) ;
#65706=CARTESIAN_POINT ( 'NONE',  ( 14.30769230769218581, -12.70778746994576025, 30.41441678777401236 ) ) ;
#65707=B_SPLINE_CURVE_WITH_KNOTS ( 'NONE', 3,
 ( #51055, #79000, #38468, #72238, #65920, #45659, #71792, #78113, #38019, #66378 ),
 .UNSPECIFIED., .F., .F.,
 ( 4, 2, 2, 2, 4 ),
 ( 0.000000000000000000, 0.0001954311564186872268, 0.0003908623128373744536, 0.0005862934692560616261, 0.0007817246256747489071 ),
 .UNSPECIFIED. ) ;
#65708=LINE ( 'NONE', #58499, #81944 ) ;
#65709=LINE ( 'NONE', #2671, #20910 ) ;
#65710=DIRECTION ( 'NONE',  ( -0.000000000000000000, -0.7660444431189791237, -0.6427876096865379196 ) ) ;
#65711=AXIS2_PLACEMENT_3D ( 'NONE', #80530, #20147, #39100 ) ;
#65713=ORIENTED_EDGE ( 'NONE', *, *, #32269, .T. ) ;
#65714=B_SPLINE_CURVE_WITH_KNOTS ( 'NONE', 3,
 ( #20216, #39167, #11235, #40499, #39614, #46796, #33728, #61183, #26082, #66166 ),
 .UNSPECIFIED., .F., .F.,
 ( 4, 2, 2, 2, 4 ),
 ( 0.0007817246256747459798, 0.0009771112852218885505, 0.001172497944769031013, 0.001367884604316173475, 0.001563271263863315937 ),
 .UNSPECIFIED. ) ;
#65715=ORIENTED_EDGE ( 'NONE', *, *, #72984, .T. ) ;
#65717=CARTESIAN_POINT ( 'NONE',  ( 14.05766908347085042, -12.45566812827425451, 31.48439005359158926 ) ) ;
#65720=LINE ( 'NONE', #57641, #71857 ) ;
#65721=CARTESIAN_POINT ( 'NONE',  ( 3.230769230769231726, -4.098570777380720287, 33.41473453929634729 ) ) ;
#65722=CARTESIAN_POINT ( 'NONE',  ( 17.20776140740982996, -7.277220318596959281, 34.99547417642776992 ) ) ;
#65724=ADVANCED_FACE ( 'NONE', ( #33499 ), #60958, .F. ) ;
#65725=DIRECTION ( 'NONE',  ( 0.000000000000000000, 0.8660254037844377084, 0.5000000000000015543 ) ) ;
#65726=CARTESIAN_POINT ( 'NONE',  ( -20.75000000000000355, -2.499999999999999556, 27.25000000000000000 ) ) ;
#65727=CARTESIAN_POINT ( 'NONE',  ( 16.85343813319912343, -12.24155766932282496, 31.33739205006857986 ) ) ;
#65728=LINE ( 'NONE', #17559, #15168 ) ;
#65729=CYLINDRICAL_SURFACE ( 'NONE', #68451, 0.2499999999999994726 ) ;
#65730=DIRECTION ( 'NONE',  ( -0.000000000000000000, 0.7660444431189791237, -0.6427876096865379196 ) ) ;
#65731=DIRECTION ( 'NONE',  ( -0.000000000000000000, -0.9396926207859093161, -0.3420201433256663259 ) ) ;
#65732=CARTESIAN_POINT ( 'NONE',  ( 5.076923076923075762, -13.95598074871891292, 31.83374038241031911 ) ) ;
#65733=CARTESIAN_POINT ( 'NONE',  ( 10.61538461538461675, -2.721908614388771852, 31.22303859784724978 ) ) ;
#65734=CARTESIAN_POINT ( 'NONE',  ( -3.230769230769229949, -11.16473453929635440, 33.15142922261926373 ) ) ;
#65735=CARTESIAN_POINT ( 'NONE',  ( -7.053224132515143907, -5.195881422630167279, 34.18770438780618548 ) ) ;
#65736=EDGE_LOOP ( 'NONE', ( #54982, #61374 ) ) ;
#65737=CARTESIAN_POINT ( 'NONE',  ( -16.28399412357784826, -9.504002272028873932, 34.60269587691767867 ) ) ;
#65738=CARTESIAN_POINT ( 'NONE',  ( 1.161689167099238418, -5.667676309546437530, 34.40238873228292249 ) ) ;
#65739=CYLINDRICAL_SURFACE ( 'NONE', #80780, 0.2500000000000012212 ) ;
#65741=ADVANCED_FACE ( 'NONE', ( #34371 ), #61838, .F. ) ;
#65742=CARTESIAN_POINT ( 'NONE',  ( -14.24243673641628050, -5.219633306516380244, 34.19971097300157936 ) ) ;
#65743=AXIS2_PLACEMENT_3D ( 'NONE', #7997, #63816, #50284 ) ;
#65744=CARTESIAN_POINT ( 'NONE',  ( 14.08420738312797837, -4.988325925672468131, 34.36044203135681130 ) ) ;
#65745=CARTESIAN_POINT ( 'NONE',  ( 5.142990410273151625, -3.937682226553329556, 33.60647404775216529 ) ) ;
#65746=ORIENTED_EDGE ( 'NONE', *, *, #84084, .F. ) ;
#65748=CARTESIAN_POINT ( 'NONE',  ( -12.46153846153815437, -2.506253911140614576, 30.00000000000323297 ) ) ;
#65750=ORIENTED_EDGE ( 'NONE', *, *, #7814, .T. ) ;
#65751=DIRECTION ( 'NONE',  ( -0.000000000000000000, 0.1736481776669307198, -0.9848077530122080203 ) ) ;
#65752=B_SPLINE_CURVE_WITH_KNOTS ( 'NONE', 3,
 ( #50465, #71185, #3166, #50031, #28897, #2717, #72076, #9488, #30215, #63543 ),
 .UNSPECIFIED., .F., .F.,
 ( 4, 2, 2, 2, 4 ),
 ( 0.000000000000000000, 0.0001954339857564092633, 0.0003908679715128185266, 0.0005863019572692277628, 0.0007817359430256370532 ),
 .UNSPECIFIED. ) ;
#65754=LINE ( 'NONE', #72518, #20465 ) ;
#65755=CARTESIAN_POINT ( 'NONE',  ( 2.980769230769232170, -2.249999999999998668, 29.75000000000000355 ) ) ;
#65756=VECTOR ( 'NONE', #3926, 1000.000000000000227 ) ;
#65757=CARTESIAN_POINT ( 'NONE',  ( 4.153846153846154188, -7.500000000000001776, 35.04278698407183867 ) ) ;
#65758=ORIENTED_EDGE ( 'NONE', *, *, #83753, .T. ) ;
#65759=CARTESIAN_POINT ( 'NONE',  ( -10.48485891362105171, -12.45806712695776319, 30.39783852428763922 ) ) ;
#65760=ORIENTED_EDGE ( 'NONE', *, *, #19426, .F. ) ;
#65762=ORIENTED_EDGE ( 'NONE', *, *, #82173, .F. ) ;
#65763=CARTESIAN_POINT ( 'NONE',  ( 13.60762673622823726, -11.76359900205217635, 32.36225158514719880 ) ) ;
#65764=CARTESIAN_POINT ( 'NONE',  ( 2.307692307692187583, -3.300289026999228881, 32.46337939537708905 ) ) ;
#65765=ORIENTED_EDGE ( 'NONE', *, *, #11072, .T. ) ;
#65766=CARTESIAN_POINT ( 'NONE',  ( -10.86536135943320502, -12.01397095200674059, 32.43157075238190146 ) ) ;
#65767=CARTESIAN_POINT ( 'NONE',  ( 10.68064018666064108, -3.300289026998473041, 32.46337939537591666 ) ) ;
#65769=DIRECTION ( 'NONE',  ( -0.000000000000000000, 0.8660254037844399289, -0.4999999999999980016 ) ) ;
#65771=EDGE_CURVE ( 'NONE', #86292, #18500, #18016, .T. ) ;
#65773=ORIENTED_EDGE ( 'NONE', *, *, #75090, .T. ) ;
#65774=ORIENTED_EDGE ( 'NONE', *, *, #42740, .F. ) ;
#65775=CARTESIAN_POINT ( 'NONE',  ( 3.230769230769231726, -3.513871655860378418, 32.76840700105978499 ) ) ;
#65776=ORIENTED_EDGE ( 'NONE', *, *, #20152, .T. ) ;
#65777=AXIS2_PLACEMENT_3D ( 'NONE', #87083, #39332, #12288 ) ;
#65779=EDGE_CURVE ( 'NONE', #17845, #55623, #44789, .T. ) ;
#65781=CARTESIAN_POINT ( 'NONE',  ( -9.019207500173124004, -9.943427161483782584, 34.11278801902876978 ) ) ;
#65782=CARTESIAN_POINT ( 'NONE',  ( 6.222779668978068557, -10.23759521482555357, 34.22997729860117033 ) ) ;
#65783=ORIENTED_EDGE ( 'NONE', *, *, #56798, .F. ) ;
#65785=CARTESIAN_POINT ( 'NONE',  ( -0.4615384615384611200, -5.415277668671390821, 36.20867863119892149 ) ) ;
#65787=CARTESIAN_POINT ( 'NONE',  ( -10.48459280755982626, -8.999086150933475636, 34.52020707165672775 ) ) ;
#65788=CARTESIAN_POINT ( 'NONE',  ( -7.911424292114618950, -2.625532179533444754, 30.86335684631481513 ) ) ;
#65789=EDGE_CURVE ( 'NONE', #62210, #2112, #73853, .T. ) ;
#65790=CARTESIAN_POINT ( 'NONE',  ( 12.33139125210024112, -2.619462340734462380, 30.83744416345203021 ) ) ;
#65791=FACE_BOUND ( 'NONE', #53089, .T. ) ;
#65793=LINE ( 'NONE', #11758, #83060 ) ;
#65794=DIRECTION ( 'NONE',  ( -0.000000000000000000, 0.6427876096865404731, -0.7660444431189770143 ) ) ;
#65795=CARTESIAN_POINT ( 'NONE',  ( -14.30769230769242739, -6.026961402154118019, 34.52809138561165270 ) ) ;
#65796=EDGE_CURVE ( 'NONE', #65067, #56939, #8286, .T. ) ;
#65797=CARTESIAN_POINT ( 'NONE',  ( 2.307692307692309264, -8.164416787775445883, 34.95778746994557906 ) ) ;
#65798=FACE_OUTER_BOUND ( 'NONE', #279, .T. ) ;
#65799=ORIENTED_EDGE ( 'NONE', *, *, #216, .F. ) ;
#65800=CARTESIAN_POINT ( 'NONE',  ( -7.173100160369890510, -6.695914987888143877, 34.68535235679833306 ) ) ;
#65801=ORIENTED_EDGE ( 'NONE', *, *, #72545, .T. ) ;
#65803=DIRECTION ( 'NONE',  ( -0.000000000000000000, -0.1736481776669307198, -0.9848077530122080203 ) ) ;
#65804=CARTESIAN_POINT ( 'NONE',  ( 5.999999999999880096, -3.300289026999228881, 32.46337939537708905 ) ) ;
#65805=CARTESIAN_POINT ( 'NONE',  ( -8.546451100252705047, -12.47679350104403007, 31.42216943046555855 ) ) ;
#65806=CARTESIAN_POINT ( 'NONE',  ( -2.307692307692305711, -12.10708131394839349, 31.69288490824020244 ) ) ;
#65807=CARTESIAN_POINT ( 'NONE',  ( 1.634669696253702176, -9.943054286541400444, 34.11300777759954883 ) ) ;
#65808=CARTESIAN_POINT ( 'NONE',  ( 14.24242230713598900, -3.083524468853724443, 32.58852847137143272 ) ) ;
#65809=ORIENTED_EDGE ( 'NONE', *, *, #71040, .T. ) ;
#65811=DIRECTION ( 'NONE',  ( -0.000000000000000000, -0.7660444431189791237, -0.6427876096865379196 ) ) ;
#65812=CARTESIAN_POINT ( 'NONE',  ( 13.38461538461538680, -3.886160181151819604, 36.00935417666054406 ) ) ;
#65814=CARTESIAN_POINT ( 'NONE',  ( 10.83816415665302202, -11.89424750095246175, 32.13594075562310337 ) ) ;
#65815=ORIENTED_EDGE ( 'NONE', *, *, #66571, .F. ) ;
#65816=EDGE_CURVE ( 'NONE', #56815, #42102, #20071, .T. ) ;
#65818=FACE_BOUND ( 'NONE', #88253, .T. ) ;
#65819=ORIENTED_EDGE ( 'NONE', *, *, #82345, .F. ) ;
#65820=CARTESIAN_POINT ( 'NONE',  ( 7.715462379486289102, -2.729777683071817229, 31.24903638046268739 ) ) ;
#65821=CARTESIAN_POINT ( 'NONE',  ( -5.933833393408360024, -7.250054591869668386, 34.99404684341514127 ) ) ;
#65822=ORIENTED_EDGE ( 'NONE', *, *, #37262, .F. ) ;
#65823=CARTESIAN_POINT ( 'NONE',  ( -7.780085495151407571, -4.098570777380720287, 33.41473453929635440 ) ) ;
#65824=LINE ( 'NONE', #51400, #41423 ) ;
#65826=DIRECTION ( 'NONE',  ( 0.000000000000000000, 0.000000000000000000, 1.000000000000000000 ) ) ;
#65827=ADVANCED_FACE ( 'NONE', ( #1920 ), #56858, .F. ) ;
#65828=CARTESIAN_POINT ( 'NONE',  ( -0.5916856709766792344, -11.47017969459903952, 32.78971311882034456 ) ) ;
#65829=VERTEX_POINT ( 'NONE', #14750 ) ;
#65830=CARTESIAN_POINT ( 'NONE',  ( -15.09997878980228414, -2.295524264805589354, 30.44142389570982488 ) ) ;
#65831=ORIENTED_EDGE ( 'NONE', *, *, #34103, .F. ) ;
#65832=CARTESIAN_POINT ( 'NONE',  ( -7.596208327805705096, -9.272278438253398036, 34.42582936511637115 ) ) ;
#65833=CARTESIAN_POINT ( 'NONE',  ( 15.23076923076923173, -2.721908614388771852, 31.22303859784724978 ) ) ;
#65834=CARTESIAN_POINT ( 'NONE',  ( -6.923076923076922462, -5.557115091759785130, 34.35708131394839171 ) ) ;
#65835=CIRCLE ( 'NONE', #16977, 0.2500000000000002220 ) ;
#65836=CARTESIAN_POINT ( 'NONE',  ( 18.24994551834813805, -8.433404298154332679, 34.66254593164985920 ) ) ;
#65838=EDGE_CURVE ( 'NONE', #57810, #69549, #48074, .T. ) ;
#65839=CARTESIAN_POINT ( 'NONE',  ( 5.326868595271218254, -12.43552623307873972, 30.55307653245132826 ) ) ;
#65841=EDGE_LOOP ( 'NONE', ( #45307, #27607 ) ) ;
#65842=AXIS2_PLACEMENT_3D ( 'NONE', #28364, #22497, #8994 ) ;
#65844=CARTESIAN_POINT ( 'NONE',  ( 2.307692307692186251, -4.320704448113951379, 33.92786785259630022 ) ) ;
#65846=B_SPLINE_CURVE_WITH_KNOTS ( 'NONE', 3,
 ( #25985, #20123, #61536, #53448, #81389, #12044, #75072, #4834, #39072, #40840 ),
 .UNSPECIFIED., .F., .F.,
 ( 4, 2, 2, 2, 4 ),
 ( 0.000000000000000000, 0.0001954339857564074473, 0.0003908679715128148945, 0.0005863019572692223418, 0.0007817359430256297891 ),
 .UNSPECIFIED. ) ;
#65847=ORIENTED_EDGE ( 'NONE', *, *, #17590, .T. ) ;
#65848=AXIS2_PLACEMENT_3D ( 'NONE', #67996, #88725, #38740 ) ;
#65850=CARTESIAN_POINT ( 'NONE',  ( -1.634615384615383027, -2.499999999999998668, 29.75000000000000355 ) ) ;
#65852=EDGE_CURVE ( 'NONE', #58944, #17200, #56601, .T. ) ;
#65853=CARTESIAN_POINT ( 'NONE',  ( 16.15384615384615330, -1.422936976036506707, 30.56769352161908415 ) ) ;
#65854=CARTESIAN_POINT ( 'NONE',  ( 10.61538461538449596, -4.481592998941358097, 33.73612834414048933 ) ) ;
#65855=EDGE_CURVE ( 'NONE', #83084, #39482, #36208, .T. ) ;
#65857=DIRECTION ( 'NONE',  ( 0.000000000000000000, 0.000000000000000000, 1.000000000000000000 ) ) ;
#65858=EDGE_LOOP ( 'NONE', ( #34248, #14558 ) ) ;
#65859=DIRECTION ( 'NONE',  ( 0.000000000000000000, 0.9848077530122072432, -0.1736481776669354937 ) ) ;
#65860=CARTESIAN_POINT ( 'NONE',  ( 8.703147358274890166, -8.120952969808774569, 34.71129190930000163 ) ) ;
#65861=CYLINDRICAL_SURFACE ( 'NONE', #52734, 0.2500000000000004996 ) ;
#65862=CARTESIAN_POINT ( 'NONE',  ( -3.480745961711584791, -11.79746400365624659, 32.30657167506340954 ) ) ;
#65863=EDGE_LOOP ( 'NONE', ( #6596, #44815, #69746, #48371 ) ) ;
#65864=CARTESIAN_POINT ( 'NONE',  ( 12.21156171748987163, -2.544273027872575366, 31.48422191005632342 ) ) ;
#65865=B_SPLINE_CURVE_WITH_KNOTS ( 'NONE', 3,
 ( #58975, #17558, #18005, #45460, #72940, #11244, #38713, #4486, #31962, #45906 ),
 .UNSPECIFIED., .F., .F.,
 ( 4, 2, 2, 2, 4 ),
 ( 0.000000000000000000, 0.0001954311564186876876, 0.0003908623128373753751, 0.0005862934692560630356, 0.0007817246256747507503 ),
 .UNSPECIFIED. ) ;
#65866=ORIENTED_EDGE ( 'NONE', *, *, #61056, .T. ) ;
#65867=AXIS2_PLACEMENT_3D ( 'NONE', #68713, #7011, #12880 ) ;
#65868=CARTESIAN_POINT ( 'NONE',  ( 1.634615384616822320, -7.500000000000155431, 34.75000000000007105 ) ) ;
#65869=CARTESIAN_POINT ( 'NONE',  ( 16.21903914214080800, -2.255955759149236073, 29.99999999999988276 ) ) ;
#65870=DIRECTION ( 'NONE',  ( -0.000000000000000000, -0.000000000000000000, -1.000000000000000000 ) ) ;
#65871=ORIENTED_EDGE ( 'NONE', *, *, #50501, .T. ) ;
#65872=CARTESIAN_POINT ( 'NONE',  ( -11.53846153846153655, -13.20930481340135110, 34.54067556320372745 ) ) ;
#65874=DIRECTION ( 'NONE',  ( -0.000000000000000000, 0.7660444431189791237, -0.6427876096865379196 ) ) ;
#65875=VECTOR ( 'NONE', #46943, 999.9999999999998863 ) ;
#65876=FACE_OUTER_BOUND ( 'NONE', #37661, .T. ) ;
#65877=CARTESIAN_POINT ( 'NONE',  ( 3.480714640147274164, -2.986452184633681117, 32.43230066228895225 ) ) ;
#65878=VECTOR ( 'NONE', #23013, 1000.000000000000227 ) ;
#65879=ORIENTED_EDGE ( 'NONE', *, *, #61333, .F. ) ;
#65881=ORIENTED_EDGE ( 'NONE', *, *, #247, .F. ) ;
#65883=CARTESIAN_POINT ( 'NONE',  ( 4.853996859406927378, -12.15238873228292071, 31.58232369045353849 ) ) ;
#65884=ADVANCED_FACE ( 'NONE', ( #7099 ), #6654, .F. ) ;
#65885=CARTESIAN_POINT ( 'NONE',  ( 7.846153846153846700, -11.35647404775217417, 33.31231777344666511 ) ) ;
#65887=EDGE_CURVE ( 'NONE', #34465, #15080, #42229, .T. ) ;
#65888=DIRECTION ( 'NONE',  ( 0.000000000000000000, 1.000000000000000000, 0.000000000000000000 ) ) ;
#65889=CARTESIAN_POINT ( 'NONE',  ( 15.16549878480845415, -11.94971097300153140, 32.03036669348370680 ) ) ;
#65890=ORIENTED_EDGE ( 'NONE', *, *, #61368, .T. ) ;
#65891=VERTEX_POINT ( 'NONE', #76450 ) ;
#65892=EDGE_CURVE ( 'NONE', #47638, #52597, #41331, .T. ) ;
#65893=EDGE_LOOP ( 'NONE', ( #49007, #32469 ) ) ;
#65895=VERTEX_POINT ( 'NONE', #20609 ) ;
#65896=CARTESIAN_POINT ( 'NONE',  ( -1.161604033002535230, -3.105924265160262099, 32.13625925475356127 ) ) ;
#65897=CARTESIAN_POINT ( 'NONE',  ( -1.254089682851821097, -12.45806712695776319, 30.39783852428763922 ) ) ;
#65898=ADVANCED_FACE ( 'NONE', ( #60710 ), #27813, .F. ) ;
#65900=CARTESIAN_POINT ( 'NONE',  ( -15.29603967673000575, -10.90142922261923886, 33.41473453929638993 ) ) ;
#65901=CARTESIAN_POINT ( 'NONE',  ( -6.923076923076922462, -3.050289026998446396, 32.03036669348365706 ) ) ;
#65902=DIRECTION ( 'NONE',  ( -0.000000000000000000, 1.000000000000000000, 3.491481338843133355E-15 ) ) ;
#65903=CARTESIAN_POINT ( 'NONE',  ( -12.52680846209478283, -12.51329471203370325, 31.30864560766548976 ) ) ;
#65904=LINE ( 'NONE', #3765, #17720 ) ;
#65906=CARTESIAN_POINT ( 'NONE',  ( 0.3308469948709003572, -3.062553014421049546, 32.05460306192773601 ) ) ;
#65907=ORIENTED_EDGE ( 'NONE', *, *, #18303, .T. ) ;
#65908=EDGE_LOOP ( 'NONE', ( #84186, #12226, #76094, #16824 ) ) ;
#65909=VERTEX_POINT ( 'NONE', #68799 ) ;
#65910=CARTESIAN_POINT ( 'NONE',  ( 0.2380535369741321461, -12.11044203135681840, 32.26167407432752299 ) ) ;
#65911=VERTEX_POINT ( 'NONE', #26490 ) ;
#65912=CARTESIAN_POINT ( 'NONE',  ( 6.923076923076924238, -11.35647404775217417, 33.31231777344666511 ) ) ;
#65913=CARTESIAN_POINT ( 'NONE',  ( 18.22337548577241861, -2.251407671071268712, 29.88021292934942963 ) ) ;
#65914=B_SPLINE_CURVE_WITH_KNOTS ( 'NONE', 3,
 ( #7201, #4, #12292, #75645, #40989, #82866, #1317, #28808, #443, #13948 ),
 .UNSPECIFIED., .F., .F.,
 ( 4, 2, 2, 2, 4 ),
 ( 0.000000000000000000, 0.0001954311564186875792, 0.0003908623128373751583, 0.0005862934692560627103, 0.0007817246256747503166 ),
 .UNSPECIFIED. ) ;
#65915=CARTESIAN_POINT ( 'NONE',  ( -13.38461538461538325, -3.886160181151819604, 36.00935417666054406 ) ) ;
#65916=CARTESIAN_POINT ( 'NONE',  ( 7.053868730901709405, -2.541949514083464479, 30.39797389878540557 ) ) ;
#65917=FACE_BOUND ( 'NONE', #19491, .T. ) ;
#65918=ORIENTED_EDGE ( 'NONE', *, *, #46375, .F. ) ;
#65920=CARTESIAN_POINT ( 'NONE',  ( -17.32689982097166492, -11.47974371597207899, 33.17467449705390692 ) ) ;
#65921=EDGE_CURVE ( 'NONE', #34858, #2073, #69244, .T. ) ;
#65922=VERTEX_POINT ( 'NONE', #68356 ) ;
#65923=FACE_BOUND ( 'NONE', #6676, .T. ) ;
#65924=DIRECTION ( 'NONE',  ( -0.000000000000000000, 0.1736481776669307198, -0.9848077530122080203 ) ) ;
#65925=AXIS2_PLACEMENT_3D ( 'NONE', #26200, #20334, #41049 ) ;
#65926=CARTESIAN_POINT ( 'NONE',  ( -4.023054346021367245, -11.71459661697925903, 32.44059661609676937 ) ) ;
#65927=ORIENTED_EDGE ( 'NONE', *, *, #87169, .F. ) ;
#65928=CARTESIAN_POINT ( 'NONE',  ( 2.307692307692187583, -8.613356846316285953, 34.62446782046622218 ) ) ;
#65930=DIRECTION ( 'NONE',  ( -0.000000000000000000, -0.6427876096865404731, -0.7660444431189770143 ) ) ;
#65931=ORIENTED_EDGE ( 'NONE', *, *, #55165, .T. ) ;
#65932=CARTESIAN_POINT ( 'NONE',  ( -11.60454391782167427, -4.661471528628507777, 34.16647553114621871 ) ) ;
#65933=CARTESIAN_POINT ( 'NONE',  ( -14.30769230769230660, -5.557115091759785130, 34.35708131394839171 ) ) ;
#65934=ORIENTED_EDGE ( 'NONE', *, *, #31168, .F. ) ;
#65935=AXIS2_PLACEMENT_3D ( 'NONE', #88305, #88736, #60350 ) ;
#65937=CARTESIAN_POINT ( 'NONE',  ( -2.557715544985271983, -11.37209801155882971, 32.91403422569032955 ) ) ;
#65938=DIRECTION ( 'NONE',  ( -0.000000000000000000, 0.6427876096865404731, -0.7660444431189770143 ) ) ;
#65940=CARTESIAN_POINT ( 'NONE',  ( 18.13079180782478872, -6.413143153341454017, 34.63066358083362672 ) ) ;
#65941=CARTESIAN_POINT ( 'NONE',  ( -12.46153846153858247, -2.625532179533778709, 30.86335684631627174 ) ) ;
#65942=CARTESIAN_POINT ( 'NONE',  ( -2.307692307692427391, -2.625532179533779154, 30.86335684631627174 ) ) ;
#65943=CARTESIAN_POINT ( 'NONE',  ( 5.076923076923075762, -1.951392089020283160, 34.73218667398347748 ) ) ;
#65944=CARTESIAN_POINT ( 'NONE',  ( -16.02332045208259359, -4.459921816937789885, 33.71989282347011851 ) ) ;
#65945=CARTESIAN_POINT ( 'NONE',  ( -0.3314934056186895073, -2.254550872974307119, 29.97347326024527447 ) ) ;
#65946=CARTESIAN_POINT ( 'NONE',  ( 4.826946345980720920, -12.41269422305637171, 30.68257228309993323 ) ) ;
#65947=CARTESIAN_POINT ( 'NONE',  ( -16.94639737515951339, -8.586989748646450593, 34.63063291749215011 ) ) ;
#65948=EDGE_CURVE ( 'NONE', #65909, #40661, #6209, .T. ) ;
#65949=VECTOR ( 'NONE', #7413, 1000.000000000000114 ) ;
#65950=EDGE_CURVE ( 'NONE', #84284, #81366, #33690, .T. ) ;
#65951=CARTESIAN_POINT ( 'NONE',  ( 17.07692307692307665, -4.098570777380720287, 33.41473453929634729 ) ) ;
#65952=CARTESIAN_POINT ( 'NONE',  ( 3.454145171467415398, -2.501478030877322567, 29.88021232661720816 ) ) ;
#65953=DIRECTION ( 'NONE',  ( 0.000000000000000000, 1.000000000000000000, 0.000000000000000000 ) ) ;
#65955=ORIENTED_EDGE ( 'NONE', *, *, #10786, .T. ) ;
#65957=EDGE_LOOP ( 'NONE', ( #82395, #404 ) ) ;
#65958=B_SPLINE_CURVE_WITH_KNOTS ( 'NONE', 3,
 ( #78961, #71308, #57801, #85286, #17257, #44717, #23571, #23131, #58683, #15944 ),
 .UNSPECIFIED., .F., .F.,
 ( 4, 2, 2, 2, 4 ),
 ( 0.0007817359430256371616, 0.0009771253907250052138, 0.001172514838424373266, 0.001367904286123741318, 0.001563293733823109370 ),
 .UNSPECIFIED. ) ;
#65959=ORIENTED_EDGE ( 'NONE', *, *, #88306, .F. ) ;
#65960=CARTESIAN_POINT ( 'NONE',  ( -3.230769230769352962, -9.528491918059723176, 34.59228464037033035 ) ) ;
#65961=ORIENTED_EDGE ( 'NONE', *, *, #925, .F. ) ;
#65962=CARTESIAN_POINT ( 'NONE',  ( 17.77712131757136049, -7.630691491037286056, 34.74850469731152458 ) ) ;
#65964=CYLINDRICAL_SURFACE ( 'NONE', #67428, 0.2500000000000009437 ) ;
#65965=EDGE_CURVE ( 'NONE', #19849, #33151, #54466, .T. ) ;
#65966=CARTESIAN_POINT ( 'NONE',  ( -18.22292695890684655, -11.98009711892699691, 32.48740034544075428 ) ) ;
#65967=CARTESIAN_POINT ( 'NONE',  ( 9.915087361285756629, -9.418065098278013636, 34.63729479722530158 ) ) ;
#65968=FACE_OUTER_BOUND ( 'NONE', #41906, .T. ) ;
#65969=DIRECTION ( 'NONE',  ( -0.000000000000000000, 0.6427876096865404731, -0.7660444431189771253 ) ) ;
#65970=CYLINDRICAL_SURFACE ( 'NONE', #71787, 0.2499999999999986955 ) ;
#65971=CARTESIAN_POINT ( 'NONE',  ( -1.384615384615383471, -7.500000000000001776, 35.04278698407183867 ) ) ;
#65973=EDGE_CURVE ( 'NONE', #42127, #29932, #36347, .T. ) ;
#65975=CARTESIAN_POINT ( 'NONE',  ( 1.254468175177168465, -2.882441371585227952, 31.66841991370172948 ) ) ;
#65976=FACE_OUTER_BOUND ( 'NONE', #72509, .T. ) ;
#65977=CARTESIAN_POINT ( 'NONE',  ( 2.307692307692309264, -8.564572088678739092, 35.78748833219616898 ) ) ;
#65978=EDGE_CURVE ( 'NONE', #25175, #64975, #74897, .T. ) ;
#65979=ORIENTED_EDGE ( 'NONE', *, *, #63249, .F. ) ;
#65980=EDGE_LOOP ( 'NONE', ( #48729, #22853, #54410, #50626, #61722, #52376 ) ) ;
#65982=CARTESIAN_POINT ( 'NONE',  ( -17.14219352288385778, -8.613356846314824011, 34.62446782046655613 ) ) ;
#65983=CARTESIAN_POINT ( 'NONE',  ( 11.53846153846153832, -10.51840700105979565, 33.73612834413961536 ) ) ;
#65984=LINE ( 'NONE', #38527, #41266 ) ;
#65985=CARTESIAN_POINT ( 'NONE',  ( 4.153846153846154188, -3.322132147404559976, 32.92929555188717927 ) ) ;
#65986=FACE_OUTER_BOUND ( 'NONE', #29221, .T. ) ;
#65988=CARTESIAN_POINT ( 'NONE',  ( 7.715463243043537034, -2.845849958028613624, 32.17971566917920967 ) ) ;
#65990=ORIENTED_EDGE ( 'NONE', *, *, #53093, .T. ) ;
#65991=EDGE_CURVE ( 'NONE', #84238, #32965, #70575, .T. ) ;
#65993=CARTESIAN_POINT ( 'NONE',  ( 3.903869422903798458, -2.564618984488975961, 30.55390908950641915 ) ) ;
#65995=DIRECTION ( 'NONE',  ( 0.000000000000000000, 0.9848077530122072432, -0.1736481776669354937 ) ) ;
#65996=CARTESIAN_POINT ( 'NONE',  ( -5.207071046654770718, -8.630895178749536711, 34.87696386517710323 ) ) ;
#65997=VECTOR ( 'NONE', #89082, 1000.000000000000114 ) ;
#65999=AXIS2_PLACEMENT_3D ( 'NONE', #14801, #26540, #14345 ) ;
#66001=ORIENTED_EDGE ( 'NONE', *, *, #5748, .T. ) ;
#66004=B_SPLINE_CURVE_WITH_KNOTS ( 'NONE', 3,
 ( #26470, #3630, #10846, #59021, #44603, #67453, #58129, #26909, #9947, #38317 ),
 .UNSPECIFIED., .F., .F.,
 ( 4, 2, 2, 2, 4 ),
 ( 0.0007817246256747447872, 0.0009771112852218876831, 0.001172497944769030579, 0.001367884604316173475, 0.001563271263863316371 ),
 .UNSPECIFIED. ) ;
#66006=B_SPLINE_CURVE_WITH_KNOTS ( 'NONE', 3,
 ( #36561, #29807, #45075, #30245, #50061, #85192, #23470, #50929, #17162, #78417 ),
 .UNSPECIFIED., .F., .F.,
 ( 4, 2, 2, 2, 4 ),
 ( 0.000000000000000000, 0.0001954339857564091278, 0.0003908679715128182556, 0.0005863019572692274375, 0.0007817359430256365111 ),
 .UNSPECIFIED. ) ;
#66007=CARTESIAN_POINT ( 'NONE',  ( 10.39189969082028675, -4.988325925672468131, 34.36044203135681130 ) ) ;
#66008=CARTESIAN_POINT ( 'NONE',  ( 6.923076923076800782, -8.656820664282941280, 34.87096338111179961 ) ) ;
#66009=CARTESIAN_POINT ( 'NONE',  ( 5.869308533332443290, -12.38065189839062263, 30.83690757178629482 ) ) ;
#66010=VERTEX_POINT ( 'NONE', #23700 ) ;
#66011=ORIENTED_EDGE ( 'NONE', *, *, #23985, .T. ) ;
#66012=CYLINDRICAL_SURFACE ( 'NONE', #45996, 0.2499999999999994726 ) ;
#66013=ORIENTED_EDGE ( 'NONE', *, *, #31118, .T. ) ;
#66014=ADVANCED_FACE ( 'NONE', ( #84980 ), #8878, .F. ) ;
#66015=CARTESIAN_POINT ( 'NONE',  ( -5.869474298236434073, -3.285477652293412820, 32.44071101563363158 ) ) ;
#66016=ORIENTED_EDGE ( 'NONE', *, *, #65666, .T. ) ;
#66017=CARTESIAN_POINT ( 'NONE',  ( 8.769230769230645706, -2.379036618888197729, 30.90682066428292885 ) ) ;
#66018=CARTESIAN_POINT ( 'NONE',  ( -7.145943186140023329, -2.251424796025575770, 29.88072029997477586 ) ) ;
#66021=LINE ( 'NONE', #52952, #54089 ) ;
#66022=CIRCLE ( 'NONE', #24307, 2.000000000000001776 ) ;
#66023=ORIENTED_EDGE ( 'NONE', *, *, #28746, .T. ) ;
#66024=CARTESIAN_POINT ( 'NONE',  ( 7.846153846154160227, -2.255955759149395501, 30.00000000000324363 ) ) ;
#66025=CYLINDRICAL_SURFACE ( 'NONE', #27090, 0.2499999999999998890 ) ;
#66026=B_SPLINE_CURVE_WITH_KNOTS ( 'NONE', 3,
 ( #88373, #73954, #39729, #5498, #54103, #60425, #27974, #62, #41940, #7265 ),
 .UNSPECIFIED., .F., .F.,
 ( 4, 2, 2, 2, 4 ),
 ( 0.0007817246256747455461, 0.0009771112852218883336, 0.001172497944769031230, 0.001367884604316174126, 0.001563271263863317022 ),
 .UNSPECIFIED. ) ;
#66027=FACE_BOUND ( 'NONE', #63592, .T. ) ;
#66028=CARTESIAN_POINT ( 'NONE',  ( -0.4615384615384611200, -11.35647404775217417, 33.31231777344666511 ) ) ;
#66029=CARTESIAN_POINT ( 'NONE',  ( 7.976679284387489410, -2.372941743896879174, 30.88044141588253666 ) ) ;
#66030=FACE_OUTER_BOUND ( 'NONE', #50271, .T. ) ;
#66031=CARTESIAN_POINT ( 'NONE',  ( -3.230769230769352962, -8.656820664282941280, 34.87096338111179961 ) ) ;
#66032=ORIENTED_EDGE ( 'NONE', *, *, #6162, .F. ) ;
#66033=EDGE_CURVE ( 'NONE', #5283, #86522, #15632, .T. ) ;
#66034=LINE ( 'NONE', #38129, #28866 ) ;
#66035=CARTESIAN_POINT ( 'NONE',  ( 8.769230769230768274, -6.386643153685126251, 34.62446782046654192 ) ) ;
#66036=ORIENTED_EDGE ( 'NONE', *, *, #79281, .F. ) ;
#66037=CARTESIAN_POINT ( 'NONE',  ( -8.519285359852727169, -3.520799739797214389, 33.17531984108286025 ) ) ;
#66038=LINE ( 'NONE', #12439, #9883 ) ;
#66039=CARTESIAN_POINT ( 'NONE',  ( -15.23076923076922995, -11.11383981884818262, 36.00935417666054406 ) ) ;
#66040=DIRECTION ( 'NONE',  ( -0.000000000000000000, -0.000000000000000000, -1.000000000000000000 ) ) ;
#66041=CARTESIAN_POINT ( 'NONE',  ( 12.33084699487090319, -4.118384482072086072, 33.43331474514187107 ) ) ;
#66042=FACE_BOUND ( 'NONE', #7, .T. ) ;
#66043=CYLINDRICAL_SURFACE ( 'NONE', #47606, 0.2500000000000002220 ) ;
#66045=EDGE_CURVE ( 'NONE', #34824, #2196, #26464, .T. ) ;
#66046=CARTESIAN_POINT ( 'NONE',  ( -3.230769230769229949, -10.89733346790207413, 36.13435417666054406 ) ) ;
#66047=CARTESIAN_POINT ( 'NONE',  ( 3.230769230769110045, -4.481592998941358097, 33.73612834414048933 ) ) ;
#66048=DIRECTION ( 'NONE',  ( -0.000000000000000000, -0.3420201433256694901, -0.9396926207859082059 ) ) ;
#66049=CARTESIAN_POINT ( 'NONE',  ( 15.93091993633000136, -10.61292498521070549, 33.66303323003028680 ) ) ;
#66050=FACE_OUTER_BOUND ( 'NONE', #60682, .T. ) ;
#66051=B_SPLINE_CURVE_WITH_KNOTS ( 'NONE', 3,
 ( #75914, #7009, #5678, #61945, #33603, #40368, #60617, #14212, #68270, #69160 ),
 .UNSPECIFIED., .F., .F.,
 ( 4, 2, 2, 2, 4 ),
 ( 0.0007817246256747460882, 0.0009771112852218892010, 0.001172497944769032314, 0.001367884604316175210, 0.001563271263863318323 ),
 .UNSPECIFIED. ) ;
#66055=AXIS2_PLACEMENT_3D ( 'NONE', #62238, #19048, #87987 ) ;
#66056=CARTESIAN_POINT ( 'NONE',  ( -4.153846153846152411, -11.69971097300155272, 32.46337939537588113 ) ) ;
#66058=CARTESIAN_POINT ( 'NONE',  ( -1.254089682851819987, -10.88167719472716399, 33.43325721877153711 ) ) ;
#66060=CARTESIAN_POINT ( 'NONE',  ( 7.596177115211490083, -4.943428324936578910, 34.04746400365624481 ) ) ;
#66061=CYLINDRICAL_SURFACE ( 'NONE', #5220, 0.2500000000000012212 ) ;
#66063=CARTESIAN_POINT ( 'NONE',  ( 2.242421861731533017, -11.94971097300153140, 32.03036669348370680 ) ) ;
#66064=CARTESIAN_POINT ( 'NONE',  ( 8.703148389870632329, -2.486705287966279432, 31.30864560766542937 ) ) ;
#66065=CIRCLE ( 'NONE', #20044, 2.000000000000001776 ) ;
#66067=CARTESIAN_POINT ( 'NONE',  ( -5.076923076923075762, -4.786620604624113540, 33.94971097300155094 ) ) ;
#66068=CARTESIAN_POINT ( 'NONE',  ( -3.230769230769229949, -13.04860791097971706, 34.73218667398347037 ) ) ;
#66069=CARTESIAN_POINT ( 'NONE',  ( -11.47239318745909742, -9.780366693483667717, 34.19971097300155805 ) ) ;
#66071=EDGE_CURVE ( 'NONE', #10540, #2738, #16510, .T. ) ;
#66072=EDGE_CURVE ( 'NONE', #19388, #2266, #86615, .T. ) ;
#66073=CARTESIAN_POINT ( 'NONE',  ( -2.307692307691991296, -2.255955759149395501, 30.00000000000324363 ) ) ;
#66075=ORIENTED_EDGE ( 'NONE', *, *, #37618, .T. ) ;
#66076=CARTESIAN_POINT ( 'NONE',  ( 6.700197406339339246, -7.630690623152302621, 34.99857592706774057 ) ) ;
#66079=CARTESIAN_POINT ( 'NONE',  ( -10.61538461538461320, -9.905515769479276145, 34.41647553114623292 ) ) ;
#66080=DIRECTION ( 'NONE',  ( 0.000000000000000000, 0.9396926207859126468, 0.3420201433256571111 ) ) ;
#66081=ORIENTED_EDGE ( 'NONE', *, *, #74403, .F. ) ;
#66084=CARTESIAN_POINT ( 'NONE',  ( -7.780086512803768173, -12.34228464037088813, 31.77849191805839268 ) ) ;
#66086=DIRECTION ( 'NONE',  ( 0.000000000000000000, 0.000000000000000000, 1.000000000000000000 ) ) ;
#66087=CYLINDRICAL_SURFACE ( 'NONE', #28262, 0.2499999999999994726 ) ;
#66088=CYLINDRICAL_SURFACE ( 'NONE', #42038, 0.2499999999999995559 ) ;
#66089=B_SPLINE_CURVE_WITH_KNOTS ( 'NONE', 3,
 ( #13083, #54954, #20288, #27925, #46420, #55393, #39683, #12199, #73903, #12643 ),
 .UNSPECIFIED., .F., .F.,
 ( 4, 2, 2, 2, 4 ),
 ( 0.000000000000000000, 0.0001954339857564071762, 0.0003908679715128143524, 0.0005863019572692215828, 0.0007817359430256287049 ),
 .UNSPECIFIED. ) ;
#66091=EDGE_LOOP ( 'NONE', ( #57232, #24318, #68670, #13493 ) ) ;
#66092=DIRECTION ( 'NONE',  ( 0.000000000000000000, 0.9396926207859126468, -0.3420201433256571111 ) ) ;
#66093=B_SPLINE_CURVE_WITH_KNOTS ( 'NONE', 3,
 ( #85749, #4664, #87098, #78532, #79877, #16835, #72666, #24474, #78981, #17282 ),
 .UNSPECIFIED., .F., .F.,
 ( 4, 2, 2, 2, 4 ),
 ( 0.000000000000000000, 0.0001954339857564070949, 0.0003908679715128141898, 0.0005863019572692212576, 0.0007817359430256283796 ),
 .UNSPECIFIED. ) ;
#66094=B_SPLINE_CURVE_WITH_KNOTS ( 'NONE', 3,
 ( #48223, #33828, #20757, #60858, #13558, #67181, #47789, #68498, #13121, #74831 ),
 .UNSPECIFIED., .F., .F.,
 ( 4, 2, 2, 2, 4 ),
 ( 0.000000000000000000, 0.0001954339857564075828, 0.0003908679715128151656, 0.0005863019572692227755, 0.0007817359430256303312 ),
 .UNSPECIFIED. ) ;
#66095=CARTESIAN_POINT ( 'NONE',  ( -12.46153846153858424, -2.657715359629662544, 31.77849191805970364 ) ) ;
#66096=FACE_OUTER_BOUND ( 'NONE', #37272, .T. ) ;
#66097=ORIENTED_EDGE ( 'NONE', *, *, #1993, .F. ) ;
#66100=EDGE_LOOP ( 'NONE', ( #17483, #43140 ) ) ;
#66101=DIRECTION ( 'NONE',  ( 0.000000000000000000, 0.6427876096865368094, 0.7660444431189802339 ) ) ;
#66102=CARTESIAN_POINT ( 'NONE',  ( 9.757562831820530747, -4.320704448112861584, 33.92786785259548310 ) ) ;
#66103=CARTESIAN_POINT ( 'NONE',  ( -12.59222992820602194, -3.530157926970578952, 32.79014554554150607 ) ) ;
#66104=CARTESIAN_POINT ( 'NONE',  ( -17.14219352288385778, -6.879047030191174805, 34.71129190930000163 ) ) ;
#66105=VERTEX_POINT ( 'NONE', #30901 ) ;
#66107=VERTEX_POINT ( 'NONE', #73237 ) ;
#66108=CARTESIAN_POINT ( 'NONE',  ( -1.161835843346975317, -5.114059244376869984, 34.14424750095245287 ) ) ;
#66110=CARTESIAN_POINT ( 'NONE',  ( -6.857821783564084228, -4.320704448112861584, 33.92786785259548310 ) ) ;
#66111=DIRECTION ( 'NONE',  ( 0.000000000000000000, 0.4999999999999985567, 0.8660254037844395958 ) ) ;
#66112=AXIS2_PLACEMENT_3D ( 'NONE', #15555, #2902, #22307 ) ;
#66113=CARTESIAN_POINT ( 'NONE',  ( 1.384615384615265343, -10.90142922262034020, 33.41473453929536674 ) ) ;
#66114=CARTESIAN_POINT ( 'NONE',  ( 6.000000000000001776, -2.249999999999998668, 29.75000000000001776 ) ) ;
#66115=ORIENTED_EDGE ( 'NONE', *, *, #26646, .F. ) ;
#66116=B_SPLINE_CURVE_WITH_KNOTS ( 'NONE', 3,
 ( #61401, #41152, #53320, #54646, #88475, #80823, #13673, #74944, #13237, #55100 ),
 .UNSPECIFIED., .F., .F.,
 ( 4, 2, 2, 2, 4 ),
 ( 0.000000000000000000, 0.0001954339857564073659, 0.0003908679715128147319, 0.0005863019572692221250, 0.0007817359430256294638 ),
 .UNSPECIFIED. ) ;
#66117=VERTEX_POINT ( 'NONE', #66925 ) ;
#66119=ORIENTED_EDGE ( 'NONE', *, *, #85300, .F. ) ;
#66120=CARTESIAN_POINT ( 'NONE',  ( 6.923076923076924238, -3.322132147404559976, 32.92929555188717927 ) ) ;
#66121=VERTEX_POINT ( 'NONE', #38565 ) ;
#66124=EDGE_CURVE ( 'NONE', #10850, #79237, #10206, .T. ) ;
#66125=DIRECTION ( 'NONE',  ( -0.000000000000000000, -0.9848077530122086864, -0.1736481776669273613 ) ) ;
#66126=B_SPLINE_CURVE_WITH_KNOTS ( 'NONE', 3,
 ( #20098, #59305, #45790, #87689, #11575, #6143, #46243, #81812, #39057, #47114 ),
 .UNSPECIFIED., .F., .F.,
 ( 4, 2, 2, 2, 4 ),
 ( 0.0007817359430256297891, 0.0009771253907249961065, 0.001172514838424362424, 0.001367904286123728741, 0.001563293733823095059 ),
 .UNSPECIFIED. ) ;
#66127=CARTESIAN_POINT ( 'NONE',  ( 12.23861224402231151, -11.24512374952581872, 33.06303171183252942 ) ) ;
#66128=ORIENTED_EDGE ( 'NONE', *, *, #51414, .F. ) ;
#66130=PLANE ( 'NONE',  #56603 ) ;
#66131=CARTESIAN_POINT ( 'NONE',  ( 4.284371855609716562, -2.882268652242224505, 31.66798894389554064 ) ) ;
#66132=FACE_BOUND ( 'NONE', #56357, .T. ) ;
#66134=CARTESIAN_POINT ( 'NONE',  ( 11.47319109250076430, -8.613356846314824011, 34.62446782046655613 ) ) ;
#66136=DIRECTION ( 'NONE',  ( 0.000000000000000000, 0.4999999999999960032, -0.8660254037844410391 ) ) ;
#66137=CARTESIAN_POINT ( 'NONE',  ( 16.85343815235874132, -9.417330523894424488, 34.63758898049880486 ) ) ;
#66138=CARTESIAN_POINT ( 'NONE',  ( -5.326899807865430603, -3.137211980971221781, 32.19342716148376837 ) ) ;
#66139=CYLINDRICAL_SURFACE ( 'NONE', #46700, 0.2500000000000009437 ) ;
#66140=CARTESIAN_POINT ( 'NONE',  ( -6.923076923077044142, -6.026961402154118908, 34.52809138561165270 ) ) ;
#66141=ORIENTED_EDGE ( 'NONE', *, *, #12821, .T. ) ;
#66143=EDGE_CURVE ( 'NONE', #58556, #33472, #39399, .T. ) ;
#66144=DIRECTION ( 'NONE',  ( -0.000000000000000000, -0.1736481776669307198, -0.9848077530122080203 ) ) ;
#66146=ORIENTED_EDGE ( 'NONE', *, *, #72289, .T. ) ;
#66147=LINE ( 'NONE', #18420, #57575 ) ;
#66148=CARTESIAN_POINT ( 'NONE',  ( 7.846153846153846700, -12.62096338111211580, 30.90682066428153263 ) ) ;
#66149=CARTESIAN_POINT ( 'NONE',  ( -16.82686865700962286, -12.65882529074907126, 30.72640787790838601 ) ) ;
#66150=CARTESIAN_POINT ( 'NONE',  ( 14.37288529598696307, -2.255955759149235629, 29.99999999999988987 ) ) ;
#66151=CARTESIAN_POINT ( 'NONE',  ( 15.23076923076923173, -10.05456864172156806, 36.03766855953608683 ) ) ;
#66153=LINE ( 'NONE', #65703, #57197 ) ;
#66154=DIRECTION ( 'NONE',  ( 0.000000000000000000, 0.6427876096865373645, -0.7660444431189797898 ) ) ;
#66155=CARTESIAN_POINT ( 'NONE',  ( 18.13052570176356681, -3.816742781228458448, 33.13167719472716044 ) ) ;
#66156=CARTESIAN_POINT ( 'NONE',  ( 12.46153846153846168, -2.708943851104267164, 35.45975837776705220 ) ) ;
#66157=DIRECTION ( 'NONE',  ( 0.000000000000000000, 0.8660254037844377084, 0.5000000000000015543 ) ) ;
#66158=EDGE_CURVE ( 'NONE', #66781, #82483, #77973, .T. ) ;
#66160=CYLINDRICAL_SURFACE ( 'NONE', #6086, 0.2499999999999995559 ) ;
#66161=AXIS2_PLACEMENT_3D ( 'NONE', #60862, #19875, #52 ) ;
#66163=ORIENTED_EDGE ( 'NONE', *, *, #57592, .F. ) ;
#66164=ORIENTED_EDGE ( 'NONE', *, *, #55918, .F. ) ;
#66165=CARTESIAN_POINT ( 'NONE',  ( -8.069080805060693251, -11.43668979543635089, 33.22377378376089752 ) ) ;
#66166=CARTESIAN_POINT ( 'NONE',  ( -18.00000000000000000, -3.322132147404558200, 32.92929555188717217 ) ) ;
#66167=CARTESIAN_POINT ( 'NONE',  ( 10.83839596699746544, -2.554770724473668153, 30.48948780036025852 ) ) ;
#66168=CARTESIAN_POINT ( 'NONE',  ( -14.30769230769230660, -6.386643153685126251, 34.62446782046654192 ) ) ;
#66169=CARTESIAN_POINT ( 'NONE',  ( 17.29988621118975800, -7.369474539155830506, 34.99858011523957657 ) ) ;
#66171=DIRECTION ( 'NONE',  ( -0.000000000000000000, 0.3420201433256694901, -0.9396926207859082059 ) ) ;
#66172=DIRECTION ( 'NONE',  ( -0.000000000000000000, -0.9396926207859093161, -0.3420201433256663259 ) ) ;
#66174=CARTESIAN_POINT ( 'NONE',  ( -2.307692307692305711, -5.415277668671390821, 36.20867863119892149 ) ) ;
#66175=CYLINDRICAL_SURFACE ( 'NONE', #85693, 0.2500000000000012212 ) ;
#66176=DIRECTION ( 'NONE',  ( 0.000000000000000000, 0.4999999999999960032, -0.8660254037844410391 ) ) ;
#66177=CARTESIAN_POINT ( 'NONE',  ( -12.52680846209478460, -8.656820664281498878, 34.87096338111211935 ) ) ;
#66178=CARTESIAN_POINT ( 'NONE',  ( 8.096208266067295156, -8.346898887586323923, 34.93166121998716278 ) ) ;
#66179=EDGE_CURVE ( 'NONE', #74977, #33753, #18956, .T. ) ;
#66180=CARTESIAN_POINT ( 'NONE',  ( -6.065270445960774914, -10.21337939537584383, 33.94971097300158647 ) ) ;
#66181=AXIS2_PLACEMENT_3D ( 'NONE', #32692, #18301, #80456 ) ;
#66182=CARTESIAN_POINT ( 'NONE',  ( 9.692307692307695177, -4.661471528628507777, 34.16647553114623292 ) ) ;
#66183=CARTESIAN_POINT ( 'NONE',  ( -3.480792454990687901, -12.45566812827425096, 31.48439005359158926 ) ) ;
#66184=EDGE_CURVE ( 'NONE', #37534, #31340, #7159, .T. ) ;
#66185=ORIENTED_EDGE ( 'NONE', *, *, #39750, .F. ) ;
#66186=CARTESIAN_POINT ( 'NONE',  ( -16.37677311275299985, -9.172386477786394821, 34.72672124145550043 ) ) ;
#66187=CARTESIAN_POINT ( 'NONE',  ( 18.22277966897806678, -4.989023458446561143, 34.36081565061822118 ) ) ;
#66188=CARTESIAN_POINT ( 'NONE',  ( -4.153846153846152411, -5.471508081941601098, 34.59228464037088457 ) ) ;
#66190=CIRCLE ( 'NONE', #77699, 0.2500000000000002220 ) ;
#66193=CARTESIAN_POINT ( 'NONE',  ( 3.230769230769231726, -1.790695186598648903, 34.54067556320373455 ) ) ;
#66194=CYLINDRICAL_SURFACE ( 'NONE', #3412, 0.2500000000000012212 ) ;
#66195=EDGE_CURVE ( 'NONE', #19174, #42436, #42563, .T. ) ;
#66196=CARTESIAN_POINT ( 'NONE',  ( 5.076923076923075762, -3.937682226553329556, 33.60647404775216529 ) ) ;
#66197=VERTEX_POINT ( 'NONE', #39362 ) ;
#66200=VECTOR ( 'NONE', #55448, 999.9999999999998863 ) ;
#66201=ORIENTED_EDGE ( 'NONE', *, *, #51024, .T. ) ;
#66202=VECTOR ( 'NONE', #23699, 1000.000000000000114 ) ;
#66203=CARTESIAN_POINT ( 'NONE',  ( -18.00000000000000000, -3.513871655860376197, 32.76840700105977788 ) ) ;
#66205=VERTEX_POINT ( 'NONE', #10093 ) ;
#66206=CARTESIAN_POINT ( 'NONE',  ( 2.980746006547774218, -4.931416488878823223, 34.32920672191015399 ) ) ;
#66208=FACE_OUTER_BOUND ( 'NONE', #48220, .T. ) ;
#66209=ORIENTED_EDGE ( 'NONE', *, *, #29680, .T. ) ;
#66210=CARTESIAN_POINT ( 'NONE',  ( 8.769230769230768274, -11.69971097300155272, 32.46337939537588113 ) ) ;
#66212=CARTESIAN_POINT ( 'NONE',  ( 11.40831432902331599, -3.817052484675422797, 33.13202310037935661 ) ) ;
#66213=ORIENTED_EDGE ( 'NONE', *, *, #34843, .F. ) ;
#66214=CARTESIAN_POINT ( 'NONE',  ( 13.44987095589141113, -11.94971097300157403, 32.03036669348361443 ) ) ;
#66215=CARTESIAN_POINT ( 'NONE',  ( 2.530703659305157505, -3.105924265160262543, 32.13625925475356127 ) ) ;
#66218=CARTESIAN_POINT ( 'NONE',  ( 7.173022332454967120, -8.476813868363244353, 34.90874843262270133 ) ) ;
#66219=CARTESIAN_POINT ( 'NONE',  ( 11.53846153846153832, -11.69971097300155272, 32.46337939537588113 ) ) ;
#66220=CYLINDRICAL_SURFACE ( 'NONE', #69350, 0.2500000000000009437 ) ;
#66221=ADVANCED_FACE ( 'NONE', ( #31252 ), #44755, .F. ) ;
#66222=ORIENTED_EDGE ( 'NONE', *, *, #43206, .T. ) ;
#66224=B_SPLINE_CURVE_WITH_KNOTS ( 'NONE', 3,
 ( #73864, #60777, #5403, #88722, #20245, #67544, #47707, #32869, #74752, #6720 ),
 .UNSPECIFIED., .F., .F.,
 ( 4, 2, 2, 2, 4 ),
 ( 0.000000000000000000, 0.0001954311564186862781, 0.0003908623128373725562, 0.0005862934692560588072, 0.0007817246256747451124 ),
 .UNSPECIFIED. ) ;
#66226=CARTESIAN_POINT ( 'NONE',  ( 3.453780582382080411, -3.587049720035815348, 32.86302985866382897 ) ) ;
#66227=ORIENTED_EDGE ( 'NONE', *, *, #70021, .T. ) ;
#66228=CIRCLE ( 'NONE', #4384, 0.2500000000000002220 ) ;
#66229=DIRECTION ( 'NONE',  ( -0.000000000000000000, -1.000000000000000000, 3.491481338843133355E-15 ) ) ;
#66230=CARTESIAN_POINT ( 'NONE',  ( 1.607394925883795844, -2.847695495035523106, 31.58253572463339154 ) ) ;
#66231=ORIENTED_EDGE ( 'NONE', *, *, #86420, .T. ) ;
#66232=FACE_OUTER_BOUND ( 'NONE', #70368, .T. ) ;
#66234=EDGE_LOOP ( 'NONE', ( #75961, #76994, #54262, #23201 ) ) ;
#66235=CARTESIAN_POINT ( 'NONE',  ( 11.60371710973756620, -2.625532179533470512, 30.86335684631491105 ) ) ;
#66236=EDGE_LOOP ( 'NONE', ( #35648, #34028, #43449, #63225 ) ) ;
#66237=LINE ( 'NONE', #81107, #76170 ) ;
#66239=CARTESIAN_POINT ( 'NONE',  ( -7.846153846153965716, -2.625532179533778709, 30.86335684631627174 ) ) ;
#66240=DIRECTION ( 'NONE',  ( -0.000000000000000000, -0.1736481776669307198, -0.9848077530122080203 ) ) ;
#66241=FACE_BOUND ( 'NONE', #83355, .T. ) ;
#66242=CARTESIAN_POINT ( 'NONE',  ( 2.084813625263661763, -7.630691491037286056, 34.74850469731152458 ) ) ;
#66243=CARTESIAN_POINT ( 'NONE',  ( 13.38461538461538680, -8.973038597847269315, 34.52809138561121927 ) ) ;
#66246=EDGE_CURVE ( 'NONE', #78733, #66604, #51955, .T. ) ;
#66247=CARTESIAN_POINT ( 'NONE',  ( 13.63466980452883881, -4.818054556918156983, 34.26375889529406749 ) ) ;
#66248=DIRECTION ( 'NONE',  ( 0.000000000000000000, 0.8660254037844377084, 0.5000000000000015543 ) ) ;
#66249=DIRECTION ( 'NONE',  ( -0.000000000000000000, 0.7660444431189791237, -0.6427876096865379196 ) ) ;
#66250=DIRECTION ( 'NONE',  ( 0.000000000000000000, 0.6427876096865373645, -0.7660444431189797898 ) ) ;
#66251=EDGE_LOOP ( 'NONE', ( #71449, #64552, #59732, #77105 ) ) ;
#66252=CARTESIAN_POINT ( 'NONE',  ( -7.053224132515142131, -6.852621066184267029, 34.70813303252209181 ) ) ;
#66253=EDGE_CURVE ( 'NONE', #69827, #88074, #45202, .T. ) ;
#66254=ORIENTED_EDGE ( 'NONE', *, *, #9256, .F. ) ;
#66255=ORIENTED_EDGE ( 'NONE', *, *, #39991, .T. ) ;
#66256=AXIS2_PLACEMENT_3D ( 'NONE', #69262, #89113, #8006 ) ;
#66257=B_SPLINE_CURVE_WITH_KNOTS ( 'NONE', 3,
 ( #14683, #7926, #28644, #61088, #35392, #34942, #19662, #75063, #62843, #89032 ),
 .UNSPECIFIED., .F., .F.,
 ( 4, 2, 2, 2, 4 ),
 ( 0.000000000000000000, 0.0001954339881912776238, 0.0003908679763825552477, 0.0005863019645738329257, 0.0007817359527651104954 ),
 .UNSPECIFIED. ) ;
#66258=CARTESIAN_POINT ( 'NONE',  ( 5.776515075435673552, -12.11044203135681840, 32.26167407432752299 ) ) ;
#66259=CARTESIAN_POINT ( 'NONE',  ( 10.83816415665302380, -5.913360116392397892, 34.49180327182771322 ) ) ;
#66260=CARTESIAN_POINT ( 'NONE',  ( -3.930419754931365972, -7.630147987733840509, 34.99859428049665411 ) ) ;
#66261=CARTESIAN_POINT ( 'NONE',  ( -2.177166605928741117, -12.27024696741798770, 31.24895572276497546 ) ) ;
#66263=CARTESIAN_POINT ( 'NONE',  ( -15.29685264172511161, -3.513871655860377086, 32.76840700105978499 ) ) ;
#66264=B_SPLINE_CURVE_WITH_KNOTS ( 'NONE', 3,
 ( #8224, #48754, #35700, #42454, #57286, #76224, #63150, #64031, #70813, #1465 ),
 .UNSPECIFIED., .F., .F.,
 ( 4, 2, 2, 2, 4 ),
 ( 0.0007817246256747507503, 0.0009771112852218959231, 0.001172497944769040987, 0.001367884604316186052, 0.001563271263863331116 ),
 .UNSPECIFIED. ) ;
#66265=ORIENTED_EDGE ( 'NONE', *, *, #39559, .F. ) ;
#66266=CARTESIAN_POINT ( 'NONE',  ( 16.82689983963011926, -5.851115903089112003, 34.47074536777953568 ) ) ;
#66267=CARTESIAN_POINT ( 'NONE',  ( 18.00000000000000000, -3.322132147404559976, 32.92929555188717927 ) ) ;
#66268=CARTESIAN_POINT ( 'NONE',  ( 2.557637717070352590, -12.68172785388650681, 30.59649109432439218 ) ) ;
#66269=EDGE_CURVE ( 'NONE', #65254, #50483, #17838, .T. ) ;
#66270=CARTESIAN_POINT ( 'NONE',  ( 4.854044394494430037, -7.630691491037286056, 34.74850469731152458 ) ) ;
#66272=ORIENTED_EDGE ( 'NONE', *, *, #38226, .F. ) ;
#66274=VERTEX_POINT ( 'NONE', #58273 ) ;
#66275=EDGE_CURVE ( 'NONE', #8133, #29891, #87741, .T. ) ;
#66276=CARTESIAN_POINT ( 'NONE',  ( -1.384615384615383471, -3.886160181151819604, 36.00935417666054406 ) ) ;
#66277=CARTESIAN_POINT ( 'NONE',  ( -13.13466986626724342, -10.76462480002816235, 33.53768742498949962 ) ) ;
#66278=ORIENTED_EDGE ( 'NONE', *, *, #42408, .F. ) ;
#66279=ADVANCED_FACE ( 'NONE', ( #26716 ), #74914, .F. ) ;
#66280=CARTESIAN_POINT ( 'NONE',  ( -7.596208327805704208, -4.336752205174649433, 33.62275283266504289 ) ) ;
#66281=CARTESIAN_POINT ( 'NONE',  ( -2.057746789344164551, -4.336752205174647656, 33.62275283266504289 ) ) ;
#66282=CARTESIAN_POINT ( 'NONE',  ( 0.6845498131513105822, -12.15243808032445827, 31.58219941686247978 ) ) ;
#66283=CARTESIAN_POINT ( 'NONE',  ( 14.05769230769230838, -7.500000000000001776, 34.75000000000000000 ) ) ;
#66284=CARTESIAN_POINT ( 'NONE',  ( -11.40793583669797506, -9.417988943895561960, 34.36773134775777550 ) ) ;
#66285=VERTEX_POINT ( 'NONE', #75782 ) ;
#66286=CARTESIAN_POINT ( 'NONE',  ( -7.596099534515528440, -9.943054286541403997, 34.11300777759954883 ) ) ;
#66287=ORIENTED_EDGE ( 'NONE', *, *, #17243, .F. ) ;
#66288=CARTESIAN_POINT ( 'NONE',  ( -7.715362038329057981, -8.999086150933475636, 34.52020707165672775 ) ) ;
#66289=CARTESIAN_POINT ( 'NONE',  ( 0.2115384615384615641, -7.500000000000001776, 35.00000000000000000 ) ) ;
#66290=CYLINDRICAL_SURFACE ( 'NONE', #63026, 0.2499999999999995559 ) ;
#66293=CARTESIAN_POINT ( 'NONE',  ( -8.546217925137375104, -8.282913670948747864, 34.94150082978203642 ) ) ;
#66294=ADVANCED_FACE ( 'NONE', ( #133 ), #19514, .F. ) ;
#66295=CARTESIAN_POINT ( 'NONE',  ( 18.06606835100244268, -2.538708090699994813, 30.37095296980875503 ) ) ;
#66296=VECTOR ( 'NONE', #8052, 1000.000000000000227 ) ;
#66298=ORIENTED_EDGE ( 'NONE', *, *, #67683, .T. ) ;
#66301=CARTESIAN_POINT ( 'NONE',  ( -12.46153846153858424, -6.835583212225970762, 34.95778746994575670 ) ) ;
#66302=ADVANCED_FACE ( 'NONE', ( #46977 ), #19079, .F. ) ;
#66303=B_SPLINE_CURVE_WITH_KNOTS ( 'NONE', 3,
 ( #23211, #44352, #16459, #84931, #24095, #51103 ),
 .UNSPECIFIED., .F., .F.,
 ( 4, 2, 4 ),
 ( 0.5000001263146904851, 0.7500000631573452425, 1.000000000000000000 ),
 .UNSPECIFIED. ) ;
#66304=VERTEX_POINT ( 'NONE', #12322 ) ;
#66305=ADVANCED_FACE ( 'NONE', ( #82113 ), #67268, .F. ) ;
#66307=CARTESIAN_POINT ( 'NONE',  ( 9.915320536401090123, -3.395485233115139057, 33.02377354290275946 ) ) ;
#66308=CARTESIAN_POINT ( 'NONE',  ( -14.08491263871424160, -2.612705202774698421, 31.66806509827799943 ) ) ;
#66311=CARTESIAN_POINT ( 'NONE',  ( 17.77707304109313924, -11.98009711892700224, 32.48740034544074007 ) ) ;
#66312=DIRECTION ( 'NONE',  ( 0.000000000000000000, 0.8660254037844377084, 0.5000000000000015543 ) ) ;
#66313=VERTEX_POINT ( 'NONE', #20406 ) ;
#66314=CARTESIAN_POINT ( 'NONE',  ( 9.468822748583747284, -10.81261337010820256, 33.49550067578627477 ) ) ;
#66315=AXIS2_PLACEMENT_3D ( 'NONE', #6809, #34283, #35627 ) ;
#66316=CARTESIAN_POINT ( 'NONE',  ( -2.057637996053990115, -9.943054286541407549, 34.11300777759954883 ) ) ;
#66318=EDGE_CURVE ( 'NONE', #19392, #37313, #9226, .T. ) ;
#66319=CARTESIAN_POINT ( 'NONE',  ( 16.82689983963011926, -9.271318131107980420, 34.42618302367067429 ) ) ;
#66320=EDGE_LOOP ( 'NONE', ( #57827, #63591, #77490, #34788 ) ) ;
#66321=CARTESIAN_POINT ( 'NONE',  ( 10.48469401227430708, -9.084618155246140248, 34.75535874321725771 ) ) ;
#66322=VECTOR ( 'NONE', #71563, 1000.000000000000227 ) ;
#66323=VECTOR ( 'NONE', #73151, 1000.000000000000000 ) ;
#66324=ORIENTED_EDGE ( 'NONE', *, *, #9715, .T. ) ;
#66325=CARTESIAN_POINT ( 'NONE',  ( 1.450784525578043382, -7.250054483168843156, 34.74374881642865631 ) ) ;
#66326=CARTESIAN_POINT ( 'NONE',  ( 10.61538461538461675, -3.322132147404559976, 32.92929555188717927 ) ) ;
#66327=EDGE_CURVE ( 'NONE', #54986, #75871, #14088, .T. ) ;
#66328=CARTESIAN_POINT ( 'NONE',  ( 18.00000000000000000, -9.905515769479276145, 34.41647553114623292 ) ) ;
#66329=ORIENTED_EDGE ( 'NONE', *, *, #10859, .T. ) ;
#66330=CARTESIAN_POINT ( 'NONE',  ( 12.21156173059610772, -3.627789207965226748, 32.91389620160131102 ) ) ;
#66331=CARTESIAN_POINT ( 'NONE',  ( 5.934729554039226862, -10.21337939537584383, 33.94971097300158647 ) ) ;
#66333=VECTOR ( 'NONE', #12229, 999.9999999999998863 ) ;
#66334=CARTESIAN_POINT ( 'NONE',  ( -6.065270000556318486, -5.941354392334500467, 34.76329471203369792 ) ) ;
#66335=CARTESIAN_POINT ( 'NONE',  ( -3.164700879766791708, -12.37446782046654192, 30.86335684631486842 ) ) ;
#66337=ORIENTED_EDGE ( 'NONE', *, *, #80623, .T. ) ;
#66338=CARTESIAN_POINT ( 'NONE',  ( -3.931066484868084299, -12.47679350104403007, 31.42216943046555855 ) ) ;
#66339=EDGE_LOOP ( 'NONE', ( #8135, #85059 ) ) ;
#66340=CARTESIAN_POINT ( 'NONE',  ( 11.28846153846153832, -7.500000000000001776, 34.75000000000000000 ) ) ;
#66341=EDGE_CURVE ( 'NONE', #78622, #67447, #14643, .T. ) ;
#66342=CARTESIAN_POINT ( 'NONE',  ( -10.61538461538430589, -2.506253911140614576, 30.00000000000323297 ) ) ;
#66343=EDGE_CURVE ( 'NONE', #61908, #5574, #10339, .T. ) ;
#66344=CARTESIAN_POINT ( 'NONE',  ( -13.38461538461550582, -2.892918686052166066, 31.69288490824153470 ) ) ;
#66346=CYLINDRICAL_SURFACE ( 'NONE', #27834, 0.2500000000000002220 ) ;
#66348=VERTEX_POINT ( 'NONE', #15873 ) ;
#66349=EDGE_CURVE ( 'NONE', #89174, #75689, #62964, .T. ) ;
#66350=ORIENTED_EDGE ( 'NONE', *, *, #43427, .T. ) ;
#66352=ORIENTED_EDGE ( 'NONE', *, *, #86324, .T. ) ;
#66353=ORIENTED_EDGE ( 'NONE', *, *, #51990, .F. ) ;
#66354=CARTESIAN_POINT ( 'NONE',  ( 20.74999999999999645, -4.499999999999999112, 27.25000000000000000 ) ) ;
#66355=CARTESIAN_POINT ( 'NONE',  ( -11.60373198442231590, -9.442884908240170461, 34.35708131394840592 ) ) ;
#66356=AXIS2_PLACEMENT_3D ( 'NONE', #11923, #40285, #32191 ) ;
#66357=CARTESIAN_POINT ( 'NONE',  ( -10.61538461538461320, -4.661471528628507777, 34.16647553114623292 ) ) ;
#66358=CARTESIAN_POINT ( 'NONE',  ( -6.988347369037697376, -3.300289026998414865, 32.46337939537583139 ) ) ;
#66359=CARTESIAN_POINT ( 'NONE',  ( -13.31854703361294590, -5.557115091759786019, 34.35708131394839882 ) ) ;
#66360=CARTESIAN_POINT ( 'NONE',  ( -12.59168643127016196, -12.50552854090298993, 31.33409797877408920 ) ) ;
#66361=CYLINDRICAL_SURFACE ( 'NONE', #86859, 0.2499999999999995559 ) ;
#66362=CARTESIAN_POINT ( 'NONE',  ( 9.442284468086239002, -10.18141759479407327, 34.26406193332782379 ) ) ;
#66363=CARTESIAN_POINT ( 'NONE',  ( 8.068933515131909928, -4.989023458446560255, 34.36081565061822118 ) ) ;
#66364=EDGE_LOOP ( 'NONE', ( #19602, #87466 ) ) ;
#66365=EDGE_CURVE ( 'NONE', #25943, #34857, #34795, .T. ) ;
#66366=ORIENTED_EDGE ( 'NONE', *, *, #13930, .T. ) ;
#66367=ORIENTED_EDGE ( 'NONE', *, *, #30539, .T. ) ;
#66368=CARTESIAN_POINT ( 'NONE',  ( 11.78840694783958121, -2.589246495874658383, 31.60778113518102828 ) ) ;
#66369=VERTEX_POINT ( 'NONE', #9116 ) ;
#66370=CARTESIAN_POINT ( 'NONE',  ( -16.08777780284371772, -6.386643153685127139, 34.62446782046654192 ) ) ;
#66371=CYLINDRICAL_SURFACE ( 'NONE', #62114, 0.2499999999999994726 ) ;
#66372=B_SPLINE_CURVE_WITH_KNOTS ( 'NONE', 3,
 ( #30324, #37067, #35766, #56470, #8292, #35308, #62764, #22238, #83960, #78499 ),
 .UNSPECIFIED., .F., .F.,
 ( 4, 2, 2, 2, 4 ),
 ( 0.0007817359430256294638, 0.0009771253907249937212, 0.001172514838424358087, 0.001367904286123722453, 0.001563293733823093758 ),
 .UNSPECIFIED. ) ;
#66373=FACE_OUTER_BOUND ( 'NONE', #54026, .T. ) ;
#66374=CARTESIAN_POINT ( 'NONE',  ( -14.53061852520844965, -9.886141570436013382, 34.14413921362392301 ) ) ;
#66375=FACE_BOUND ( 'NONE', #71949, .T. ) ;
#66376=ORIENTED_EDGE ( 'NONE', *, *, #10333, .T. ) ;
#66377=VERTEX_POINT ( 'NONE', #36147 ) ;
#66378=CARTESIAN_POINT ( 'NONE',  ( -17.07692307692319744, -11.67786785259630911, 32.92929555188603530 ) ) ;
#66379=ORIENTED_EDGE ( 'NONE', *, *, #79384, .F. ) ;
#66380=FACE_BOUND ( 'NONE', #16086, .T. ) ;
#66381=CARTESIAN_POINT ( 'NONE',  ( 9.942362112221147186, -5.642605341092957971, 34.66089969410670335 ) ) ;
#66383=ORIENTED_EDGE ( 'NONE', *, *, #77213, .F. ) ;
#66384=CARTESIAN_POINT ( 'NONE',  ( -14.98082371242108835, -12.22109172314383052, 31.39792113162168263 ) ) ;
#66385=CARTESIAN_POINT ( 'NONE',  ( -1.608100309179714582, -8.539481045369598178, 34.89627647299170832 ) ) ;
#66386=CARTESIAN_POINT ( 'NONE',  ( 2.084765348785460048, -11.43668979543635089, 33.22377378376089752 ) ) ;
#66388=CARTESIAN_POINT ( 'NONE',  ( 12.23861224402231151, -4.887634598454295265, 34.01352882383564946 ) ) ;
#66389=CARTESIAN_POINT ( 'NONE',  ( -14.30769230769242739, -6.026961402154118019, 34.52809138561165270 ) ) ;
#66390=DIRECTION ( 'NONE',  ( -0.000000000000000000, 0.8660254037844397068, -0.4999999999999978906 ) ) ;
#66392=VECTOR ( 'NONE', #34050, 1000.000000000000114 ) ;
#66393=CARTESIAN_POINT ( 'NONE',  ( 2.438217745925951085, -12.50538340440932217, 31.33453814440721885 ) ) ;
#66394=CARTESIAN_POINT ( 'NONE',  ( -16.94639737515951339, -11.93748526763465279, 32.05452791011430946 ) ) ;
#66395=ORIENTED_EDGE ( 'NONE', *, *, #83228, .F. ) ;
#66396=CARTESIAN_POINT ( 'NONE',  ( 0.4615384615384611200, -8.973038597847269315, 34.52809138561121927 ) ) ;
#66397=CARTESIAN_POINT ( 'NONE',  ( 14.30769230769231015, -8.120952969808772792, 34.71129190930000163 ) ) ;
#66398=CARTESIAN_POINT ( 'NONE',  ( -2.531177251416254492, -2.599994579823203367, 30.74605699353653776 ) ) ;
#66399=CARTESIAN_POINT ( 'NONE',  ( -8.703162418228332697, -8.973038597847271092, 34.52809138561121216 ) ) ;
#66400=B_SPLINE_CURVE_WITH_KNOTS ( 'NONE', 3,
 ( #46884, #32482, #20313, #46443, #82018, #74367, #59512, #25734, #27064, #73487 ),
 .UNSPECIFIED., .F., .F.,
 ( 4, 2, 2, 2, 4 ),
 ( 0.0007817359430256366195, 0.0009771253907250045632, 0.001172514838424372615, 0.001367904286123740668, 0.001563293733823108720 ),
 .UNSPECIFIED. ) ;
#66401=CARTESIAN_POINT ( 'NONE',  ( -7.173076923076921574, -7.500000000000001776, 35.00000000000000000 ) ) ;
#66402=FACE_OUTER_BOUND ( 'NONE', #24575, .T. ) ;
#66403=B_SPLINE_CURVE_WITH_KNOTS ( 'NONE', 3,
 ( #11859, #5540, #64661, #33008, #10181, #39335, #57469, #66790, #78189, #5092 ),
 .UNSPECIFIED., .F., .F.,
 ( 4, 2, 2, 2, 4 ),
 ( 0.0007817359430256333669, 0.0009771253907250056474, 0.001172514838424370881, 0.001367904286123736331, 0.001563293733823101564 ),
 .UNSPECIFIED. ) ;
#66404=CARTESIAN_POINT ( 'NONE',  ( 0.5267936010512991318, -11.67786785259547777, 32.92929555188713664 ) ) ;
#66405=CARTESIAN_POINT ( 'NONE',  ( 8.703960768674447124, -3.083524468853724443, 32.58852847137143272 ) ) ;
#66406=EDGE_CURVE ( 'NONE', #33660, #12785, #63598, .T. ) ;
#66408=CARTESIAN_POINT ( 'NONE',  ( -14.98071481085577972, -2.544122305571458575, 31.48381861865057729 ) ) ;
#66409=CARTESIAN_POINT ( 'NONE',  ( 12.39626846098214230, -5.094484230520674117, 34.41647553114621161 ) ) ;
#66411=EDGE_LOOP ( 'NONE', ( #71242, #25669, #72167, #60366 ) ) ;
#66412=CARTESIAN_POINT ( 'NONE',  ( -12.59222992820602194, -8.147922237126337563, 34.70805685702651999 ) ) ;
#66413=ORIENTED_EDGE ( 'NONE', *, *, #56441, .F. ) ;
#66415=ORIENTED_EDGE ( 'NONE', *, *, #66246, .T. ) ;
#66416=CYLINDRICAL_SURFACE ( 'NONE', #13881, 0.2500000000000002220 ) ;
#66417=EDGE_CURVE ( 'NONE', #38481, #36016, #66264, .T. ) ;
#66418=ORIENTED_EDGE ( 'NONE', *, *, #48367, .F. ) ;
#66419=CARTESIAN_POINT ( 'NONE',  ( 18.13004760625567968, -7.723484964179501588, 34.74522123443823318 ) ) ;
#66421=CARTESIAN_POINT ( 'NONE',  ( -18.00000000000000000, -4.661471528628506000, 34.16647553114623292 ) ) ;
#66422=CARTESIAN_POINT ( 'NONE',  ( -17.74999999999856115, -7.500000000000155431, 34.75000000000007105 ) ) ;
#66423=CARTESIAN_POINT ( 'NONE',  ( 9.758375025657770152, -9.058645607665452459, 34.76329471203371924 ) ) ;
#66424=CARTESIAN_POINT ( 'NONE',  ( 16.15384615384615330, -13.75783147151868846, 33.36296068462461051 ) ) ;
#66425=LINE ( 'NONE', #79501, #53269 ) ;
#66426=LINE ( 'NONE', #37612, #37267 ) ;
#66427=CARTESIAN_POINT ( 'NONE',  ( -7.780085495151409347, -12.10708131394839882, 31.69288490824020954 ) ) ;
#66428=EDGE_CURVE ( 'NONE', #69663, #31874, #64095, .T. ) ;
#66429=VECTOR ( 'NONE', #77998, 1000.000000000000227 ) ;
#66431=CARTESIAN_POINT ( 'NONE',  ( 17.14217821643591932, -2.379036618887895305, 30.90682066428158592 ) ) ;
#66432=CARTESIAN_POINT ( 'NONE',  ( 18.00000000000000000, -12.10708131394839349, 31.69288490824020244 ) ) ;
#66433=AXIS2_PLACEMENT_3D ( 'NONE', #36092, #16251, #1849 ) ;
#66434=EDGE_CURVE ( 'NONE', #68701, #59603, #25337, .T. ) ;
#66437=ORIENTED_EDGE ( 'NONE', *, *, #48234, .F. ) ;
#66438=CARTESIAN_POINT ( 'NONE',  ( -11.31568199719312773, -5.913360116392397892, 34.49180327182771322 ) ) ;
#66439=CARTESIAN_POINT ( 'NONE',  ( -14.17716660592874689, -8.586989748646452369, 34.63063291749215011 ) ) ;
#66441=CARTESIAN_POINT ( 'NONE',  ( -15.90390063549801347, -12.43552623307873972, 30.55307653245132826 ) ) ;
#66443=CARTESIAN_POINT ( 'NONE',  ( -0.5922299282060191628, -6.413092428213692742, 34.63065189839063152 ) ) ;
#66444=B_SPLINE_CURVE_WITH_KNOTS ( 'NONE', 3,
 ( #6321, #34672, #27908, #43193, #43626, #16161, #62999, #15282, #8969, #29249 ),
 .UNSPECIFIED., .F., .F.,
 ( 4, 2, 2, 2, 4 ),
 ( 0.000000000000000000, 0.0001954339881912774612, 0.0003908679763825549224, 0.0005863019645738323836, 0.0007817359527651098448 ),
 .UNSPECIFIED. ) ;
#66445=VERTEX_POINT ( 'NONE', #28044 ) ;
#66446=CARTESIAN_POINT ( 'NONE',  ( 3.100621261037536325, -6.809168938359898782, 34.95455904226513866 ) ) ;
#66447=EDGE_LOOP ( 'NONE', ( #10242, #52141, #29365, #10387 ) ) ;
#66448=EDGE_CURVE ( 'NONE', #38559, #47058, #84336, .T. ) ;
#66449=ORIENTED_EDGE ( 'NONE', *, *, #20750, .T. ) ;
#66450=AXIS2_PLACEMENT_3D ( 'NONE', #8468, #35941, #84138 ) ;
#66451=CARTESIAN_POINT ( 'NONE',  ( -5.999999999999998224, -5.557115091759785130, 34.35708131394839171 ) ) ;
#66452=AXIS2_PLACEMENT_3D ( 'NONE', #34761, #40208, #62232 ) ;
#66454=CARTESIAN_POINT ( 'NONE',  ( -9.561515884482904681, -6.413143153341454017, 34.63066358083362672 ) ) ;
#66455=LINE ( 'NONE', #38543, #1930 ) ;
#66456=CARTESIAN_POINT ( 'NONE',  ( 13.25446741488368829, -5.915902021225889484, 34.75552854090298638 ) ) ;
#66459=EDGE_CURVE ( 'NONE', #9541, #11982, #35241, .T. ) ;
#66460=ORIENTED_EDGE ( 'NONE', *, *, #83911, .F. ) ;
#66462=ADVANCED_FACE ( 'NONE', ( #24375 ), #25282, .F. ) ;
#66463=DIRECTION ( 'NONE',  ( 0.000000000000000000, 1.000000000000000000, 0.000000000000000000 ) ) ;
#66465=B_SPLINE_CURVE_WITH_KNOTS ( 'NONE', 3,
 ( #60460, #19477, #54581, #46937, #74423, #94, #55040, #82526, #14049, #41525 ),
 .UNSPECIFIED., .F., .F.,
 ( 4, 2, 2, 2, 4 ),
 ( 0.000000000000000000, 0.0001954311564186871184, 0.0003908623128373742367, 0.0005862934692560614093, 0.0007817246256747484735 ),
 .UNSPECIFIED. ) ;
#66466=DIRECTION ( 'NONE',  ( -0.000000000000000000, 0.1736481776669307198, -0.9848077530122080203 ) ) ;
#66468=B_SPLINE_CURVE_WITH_KNOTS ( 'NONE', 3,
 ( #51051, #17296, #51954, #73131, #72680, #65021 ),
 .UNSPECIFIED., .F., .F.,
 ( 4, 2, 4 ),
 ( 0.0003909512603273872016, 0.0005862562993132132720, 0.0007815613382990393423 ),
 .UNSPECIFIED. ) ;
#66469=CARTESIAN_POINT ( 'NONE',  ( -3.903846153846215472, -7.565270445406050648, 34.75000000000000000 ) ) ;
#66470=CARTESIAN_POINT ( 'NONE',  ( 18.00000000000000000, -8.120952969808772792, 34.71129190930000163 ) ) ;
#66471=ORIENTED_EDGE ( 'NONE', *, *, #65534, .F. ) ;
#66472=B_SPLINE_CURVE_WITH_KNOTS ( 'NONE', 3,
 ( #3941, #85488, #23331, #22453, #57562, #78274, #71515, #9823, #49918, #85053 ),
 .UNSPECIFIED., .F., .F.,
 ( 4, 2, 2, 2, 4 ),
 ( 0.000000000000000000, 0.0001954339857564080707, 0.0003908679715128161414, 0.0005863019572692241849, 0.0007817359430256322827 ),
 .UNSPECIFIED. ) ;
#66473=EDGE_CURVE ( 'NONE', #76426, #30118, #4925, .T. ) ;
#66474=ORIENTED_EDGE ( 'NONE', *, *, #83296, .T. ) ;
#66475=CARTESIAN_POINT ( 'NONE',  ( 0.4615384615383396616, -11.94971097300221174, 32.03036669348237098 ) ) ;
#66476=CARTESIAN_POINT ( 'NONE',  ( -13.51476335434708353, -5.915902021225889484, 34.75552854090298638 ) ) ;
#66477=ORIENTED_EDGE ( 'NONE', *, *, #17507, .T. ) ;
#66478=CYLINDRICAL_SURFACE ( 'NONE', #47896, 0.2499999999999995837 ) ;
#66479=CARTESIAN_POINT ( 'NONE',  ( -6.923076923076607159, -2.255955759149395501, 30.00000000000324363 ) ) ;
#66481=EDGE_CURVE ( 'NONE', #12502, #71930, #64467, .T. ) ;
#66483=VERTEX_POINT ( 'NONE', #10881 ) ;
#66484=CARTESIAN_POINT ( 'NONE',  ( 10.86543903529806876, -2.318338780012835443, 30.59689888758630261 ) ) ;
#66485=ORIENTED_EDGE ( 'NONE', *, *, #35443, .T. ) ;
#66487=B_SPLINE_CURVE_WITH_KNOTS ( 'NONE', 3,
 ( #18254, #65538, #79059, #66884, #73655, #87176, #59677, #79954, #39427, #52470 ),
 .UNSPECIFIED., .F., .F.,
 ( 4, 2, 2, 2, 4 ),
 ( 0.000000000000000000, 0.0001954339857564064173, 0.0003908679715128128345, 0.0005863019572692191976, 0.0007817359430256256691 ),
 .UNSPECIFIED. ) ;
#66489=FACE_OUTER_BOUND ( 'NONE', #18543, .T. ) ;
#66490=CYLINDRICAL_SURFACE ( 'NONE', #59621, 0.2500000000000008882 ) ;
#66491=FACE_OUTER_BOUND ( 'NONE', #54006, .T. ) ;
#66492=CYLINDRICAL_SURFACE ( 'NONE', #47358, 0.2499999999999995559 ) ;
#66493=CARTESIAN_POINT ( 'NONE',  ( 0.4615384615384611200, -11.11383981884818262, 36.00935417666054406 ) ) ;
#66494=EDGE_LOOP ( 'NONE', ( #71621, #54809 ) ) ;
#66495=CARTESIAN_POINT ( 'NONE',  ( -11.40767109749459074, -8.191423895709840863, 34.95447573519442130 ) ) ;
#66496=CARTESIAN_POINT ( 'NONE',  ( 11.40790162484817216, -2.254533558242299396, 29.97296025877828285 ) ) ;
#66497=DIRECTION ( 'NONE',  ( 1.000000000000000000, 0.000000000000000000, 0.000000000000000000 ) ) ;
#66498=ORIENTED_EDGE ( 'NONE', *, *, #87240, .F. ) ;
#66499=CARTESIAN_POINT ( 'NONE',  ( -9.469528023329623068, -4.989023458446560255, 34.36081565061822118 ) ) ;
#66500=CARTESIAN_POINT ( 'NONE',  ( 14.55763771707035303, -10.18230066228895758, 34.26354781536631577 ) ) ;
#66501=CARTESIAN_POINT ( 'NONE',  ( 11.28848480751918437, -5.728515186090277211, 34.42611988154120439 ) ) ;
#66502=CARTESIAN_POINT ( 'NONE',  ( 9.019176178608812933, -10.18230066228895758, 34.26354781536631577 ) ) ;
#66503=FACE_BOUND ( 'NONE', #75409, .T. ) ;
#66504=CARTESIAN_POINT ( 'NONE',  ( -7.053767526187231240, -12.35290016733513951, 31.75349464988449455 ) ) ;
#66505=LINE ( 'NONE', #25072, #33090 ) ;
#66506=B_SPLINE_CURVE_WITH_KNOTS ( 'NONE', 3,
 ( #74388, #54545, #33407, #60, #18559, #46023, #39283, #11804, #61741, #73952 ),
 .UNSPECIFIED., .F., .F.,
 ( 4, 2, 2, 2, 4 ),
 ( 0.000000000000000000, 0.0001954339857564071762, 0.0003908679715128143524, 0.0005863019572692215828, 0.0007817359430256287049 ),
 .UNSPECIFIED. ) ;
#66507=LINE ( 'NONE', #33610, #39650 ) ;
#66508=CARTESIAN_POINT ( 'NONE',  ( 1.161130460051055024, -12.69144148231606017, 30.53333754910549303 ) ) ;
#66509=CARTESIAN_POINT ( 'NONE',  ( 2.307692307692186251, -5.094484230521993062, 34.41647553114689373 ) ) ;
#66510=CARTESIAN_POINT ( 'NONE',  ( 16.15384615384603251, -10.90142922262034020, 33.41473453929536674 ) ) ;
#66511=CARTESIAN_POINT ( 'NONE',  ( 13.31934538405906565, -2.657715359629088780, 31.77849191805832874 ) ) ;
#66513=B_SPLINE_CURVE_WITH_KNOTS ( 'NONE', 3,
 ( #19902, #6831, #41512, #68979, #74866, #82514, #82067, #47373, #20363, #55902 ),
 .UNSPECIFIED., .F., .F.,
 ( 4, 2, 2, 2, 4 ),
 ( 0.0007817246256747519429, 0.0009771112852218970073, 0.001172497944769042288, 0.001367884604316187353, 0.001563271263863332417 ),
 .UNSPECIFIED. ) ;
#66514=EDGE_CURVE ( 'NONE', #32981, #76146, #50051, .T. ) ;
#66515=VECTOR ( 'NONE', #50981, 1000.000000000000227 ) ;
#66516=CARTESIAN_POINT ( 'NONE',  ( 1.384615384615386802, -1.790695186598648903, 34.54067556320373455 ) ) ;
#66517=VERTEX_POINT ( 'NONE', #10439 ) ;
#66520=CARTESIAN_POINT ( 'NONE',  ( -4.023320452082587373, -12.27024696741798770, 31.24895572276497546 ) ) ;
#66521=DIRECTION ( 'NONE',  ( -0.000000000000000000, -0.9396926207859092051, -0.3420201433256662704 ) ) ;
#66523=CARTESIAN_POINT ( 'NONE',  ( 6.000000000000001776, -2.517432740324522911, 35.29906147534542527 ) ) ;
#66524=CARTESIAN_POINT ( 'NONE',  ( -12.46153846153846168, -6.343179335718451384, 34.87096338111211935 ) ) ;
#66526=CIRCLE ( 'NONE', #47814, 0.2500000000000002220 ) ;
#66527=CARTESIAN_POINT ( 'NONE',  ( 15.23076923076923173, -11.91647553114624181, 32.58852847137148245 ) ) ;
#66528=CYLINDRICAL_SURFACE ( 'NONE', #27406, 0.2499999999999979738 ) ;
#66529=CARTESIAN_POINT ( 'NONE',  ( 17.07692307692307665, -12.78798330534103123, 29.99999999999997868 ) ) ;
#66530=CARTESIAN_POINT ( 'NONE',  ( 4.826899852701619587, -9.356822207818506598, 34.66110646841856635 ) ) ;
#66531=CARTESIAN_POINT ( 'NONE',  ( 0.4615384615384611200, -11.16473453929635440, 33.15142922261926373 ) ) ;
#66532=CARTESIAN_POINT ( 'NONE',  ( 12.46153846153846168, -13.75783147151868846, 33.36296068462461051 ) ) ;
#66533=EDGE_CURVE ( 'NONE', #66936, #16713, #18532, .T. ) ;
#66534=CARTESIAN_POINT ( 'NONE',  ( 3.165015802455898974, -7.249945578846654470, 34.99404164642496795 ) ) ;
#66535=DIRECTION ( 'NONE',  ( 0.000000000000000000, 0.8660254037844377084, 0.5000000000000015543 ) ) ;
#66536=ORIENTED_EDGE ( 'NONE', *, *, #39897, .F. ) ;
#66538=CARTESIAN_POINT ( 'NONE',  ( 17.14299142792551578, -2.721908614388772296, 31.22303859784725333 ) ) ;
#66539=CYLINDRICAL_SURFACE ( 'NONE', #31681, 0.2500000000000004996 ) ;
#66541=CARTESIAN_POINT ( 'NONE',  ( -15.16557624247457348, -2.255955759149234741, 29.99999999999988631 ) ) ;
#66542=CARTESIAN_POINT ( 'NONE',  ( -16.21911615440246734, -11.06231777344663136, 33.60647404775220082 ) ) ;
#66543=ORIENTED_EDGE ( 'NONE', *, *, #37205, .T. ) ;
#66544=CARTESIAN_POINT ( 'NONE',  ( 7.146088274689774700, -8.239487800360276282, 34.69522927552633718 ) ) ;
#66545=DIRECTION ( 'NONE',  ( 0.000000000000000000, 0.000000000000000000, 1.000000000000000000 ) ) ;
#66546=CARTESIAN_POINT ( 'NONE',  ( 11.78846153846155431, -2.249999999999999112, 29.81603969181029967 ) ) ;
#66547=VERTEX_POINT ( 'NONE', #31591 ) ;
#66548=CARTESIAN_POINT ( 'NONE',  ( -9.758390071667825794, -3.322132147404559532, 32.92929555188719348 ) ) ;
#66549=CARTESIAN_POINT ( 'NONE',  ( -3.100243529005665355, -3.816742781228458448, 33.13167719472716044 ) ) ;
#66550=CARTESIAN_POINT ( 'NONE',  ( -8.703975197954740395, -2.625532179533470512, 30.86335684631491105 ) ) ;
#66551=CARTESIAN_POINT ( 'NONE',  ( -16.28432133892187395, -7.276987145209182550, 34.99546412871779211 ) ) ;
#66553=VERTEX_POINT ( 'NONE', #3224 ) ;
#66554=B_SPLINE_CURVE_WITH_KNOTS ( 'NONE', 3,
 ( #59781, #53461, #58890, #31877, #66546, #4846 ),
 .UNSPECIFIED., .F., .F.,
 ( 4, 2, 4 ),
 ( 0.0003909512603273880690, 0.0005862562993132132720, 0.0007815613382990384750 ),
 .UNSPECIFIED. ) ;
#66555=LINE ( 'NONE', #32328, #82313 ) ;
#66556=DIRECTION ( 'NONE',  ( 1.000000000000000000, 0.000000000000000000, 0.000000000000000000 ) ) ;
#66557=CARTESIAN_POINT ( 'NONE',  ( 14.98079248672063990, -10.06842814019191401, 34.32929386961144758 ) ) ;
#66558=ORIENTED_EDGE ( 'NONE', *, *, #71450, .F. ) ;
#66559=ORIENTED_EDGE ( 'NONE', *, *, #71381, .F. ) ;
#66561=VERTEX_POINT ( 'NONE', #11320 ) ;
#66562=CARTESIAN_POINT ( 'NONE',  ( 12.52679360105129724, -10.33852847137154107, 34.16647553114620450 ) ) ;
#66563=CARTESIAN_POINT ( 'NONE',  ( 9.915087361285760181, -4.226511098958373402, 33.85474049983370293 ) ) ;
#66564=EDGE_CURVE ( 'NONE', #62997, #39886, #16810, .T. ) ;
#66565=CARTESIAN_POINT ( 'NONE',  ( 13.31934493865461455, -11.48612834413959582, 32.76840700105983473 ) ) ;
#66566=CARTESIAN_POINT ( 'NONE',  ( -17.07692307692319744, -5.219633306517616589, 34.19971097300220464 ) ) ;
#66567=ORIENTED_EDGE ( 'NONE', *, *, #65131, .F. ) ;
#66568=ORIENTED_EDGE ( 'NONE', *, *, #40372, .T. ) ;
#66569=ADVANCED_FACE ( 'NONE', ( #9982 ), #12217, .F. ) ;
#66570=EDGE_LOOP ( 'NONE', ( #73887, #65674 ) ) ;
#66571=EDGE_CURVE ( 'NONE', #12150, #6421, #87448, .T. ) ;
#66572=CARTESIAN_POINT ( 'NONE',  ( 11.78851595837499566, -11.47946981652013498, 33.17500667209847620 ) ) ;
#66573=ORIENTED_EDGE ( 'NONE', *, *, #80871, .T. ) ;
#66574=CARTESIAN_POINT ( 'NONE',  ( -16.21911615440246734, -12.51329471203370325, 31.30864560766548976 ) ) ;
#66575=DIRECTION ( 'NONE',  ( 0.000000000000000000, -6.938893903907222067E-15, 1.000000000000000000 ) ) ;
#66577=AXIS2_PLACEMENT_3D ( 'NONE', #37196, #30009, #46075 ) ;
#66578=CARTESIAN_POINT ( 'NONE',  ( 10.39189967166066708, -11.41268669641499756, 32.86336882939238535 ) ) ;
#66579=CARTESIAN_POINT ( 'NONE',  ( -1.384615384615383471, -12.62096338111211580, 30.90682066428153263 ) ) ;
#66580=VERTEX_POINT ( 'NONE', #26170 ) ;
#66581=EDGE_CURVE ( 'NONE', #46498, #22155, #53353, .T. ) ;
#66582=AXIS2_PLACEMENT_3D ( 'NONE', #58125, #84741, #51799 ) ;
#66585=DIRECTION ( 'NONE',  ( 0.000000000000000000, 0.9396926207859126468, 0.3420201433256571111 ) ) ;
#66586=CARTESIAN_POINT ( 'NONE',  ( -13.16123989884296286, -2.251407671071268712, 29.88021292934942963 ) ) ;
#66587=ORIENTED_EDGE ( 'NONE', *, *, #7865, .F. ) ;
#66588=B_SPLINE_CURVE_WITH_KNOTS ( 'NONE', 3,
 ( #82467, #68928, #40152, #88350, #82019, #48212, #67613, #54078, #7239, #55418 ),
 .UNSPECIFIED., .F., .F.,
 ( 4, 2, 2, 2, 4 ),
 ( 0.000000000000000000, 0.0001954339857564083417, 0.0003908679715128166835, 0.0005863019572692250523, 0.0007817359430256333669 ),
 .UNSPECIFIED. ) ;
#66589=CARTESIAN_POINT ( 'NONE',  ( -10.86538461538462563, -2.249999999999999556, 29.81609741502489541 ) ) ;
#66590=EDGE_CURVE ( 'NONE', #30707, #53458, #47769, .T. ) ;
#66591=EDGE_CURVE ( 'NONE', #64427, #80479, #12660, .T. ) ;
#66592=FACE_OUTER_BOUND ( 'NONE', #18167, .T. ) ;
#66593=CARTESIAN_POINT ( 'NONE',  ( -13.51476259405360381, -4.460286881179643004, 33.72017969459903242 ) ) ;
#66594=DIRECTION ( 'NONE',  ( -0.000000000000000000, 0.6427876096865404731, -0.7660444431189771253 ) ) ;
#66595=CARTESIAN_POINT ( 'NONE',  ( 10.61538461538461675, -8.318370150425687726, 35.83090037661290239 ) ) ;
#66596=FACE_BOUND ( 'NONE', #51144, .T. ) ;
#66597=CARTESIAN_POINT ( 'NONE',  ( -0.5276218724943423366, -4.098570777380720287, 33.41473453929634729 ) ) ;
#66598=CARTESIAN_POINT ( 'NONE',  ( -12.59168567097668401, -9.418419913701741919, 34.36755862841477693 ) ) ;
#66599=CARTESIAN_POINT ( 'NONE',  ( -8.769230769230890843, -4.481592998941358097, 33.73612834414048933 ) ) ;
#66600=FACE_OUTER_BOUND ( 'NONE', #82699, .T. ) ;
#66601=CARTESIAN_POINT ( 'NONE',  ( 15.36129466900287888, -10.31582465632705237, 34.18122507451815295 ) ) ;
#66602=CARTESIAN_POINT ( 'NONE',  ( 0.2115617305961068617, -12.17611988154120972, 31.52148481390971213 ) ) ;
#66603=CARTESIAN_POINT ( 'NONE',  ( 12.46153846153833911, -9.442884908241554243, 34.35708131394783038 ) ) ;
#66604=VERTEX_POINT ( 'NONE', #80691 ) ;
#66605=CARTESIAN_POINT ( 'NONE',  ( 2.438484115517096651, -6.413143153341454017, 34.63066358083362672 ) ) ;
#66606=DIRECTION ( 'NONE',  ( -0.000000000000000000, -0.9848077530122086864, -0.1736481776669273613 ) ) ;
#66607=VERTEX_POINT ( 'NONE', #13541 ) ;
#66608=ORIENTED_EDGE ( 'NONE', *, *, #73890, .T. ) ;
#66609=CARTESIAN_POINT ( 'NONE',  ( 0.5920638997721051622, -8.630441415882550871, 34.87705825610312615 ) ) ;
#66611=AXIS2_PLACEMENT_3D ( 'NONE', #30193, #1387, #57658 ) ;
#66612=CARTESIAN_POINT ( 'NONE',  ( -0.5920990532803821482, -2.504760397472875155, 29.97295953869789997 ) ) ;
#66613=CARTESIAN_POINT ( 'NONE',  ( -11.53846153846165912, -5.219633306517616589, 34.19971097300220464 ) ) ;
#66614=CARTESIAN_POINT ( 'NONE',  ( -11.53846153846166089, -10.33852847137269571, 34.16647553114546554 ) ) ;
#66615=VERTEX_POINT ( 'NONE', #81127 ) ;
#66616=CARTESIAN_POINT ( 'NONE',  ( 14.30769230769231015, -8.973038597847269315, 34.52809138561121927 ) ) ;
#66618=CARTESIAN_POINT ( 'NONE',  ( 18.22277954126840172, -3.755027918224367767, 33.06320215134714857 ) ) ;
#66619=DIRECTION ( 'NONE',  ( -1.000000000000000000, 0.000000000000000000, 0.000000000000000000 ) ) ;
#66620=LINE ( 'NONE', #4922, #89152 ) ;
#66621=DIRECTION ( 'NONE',  ( -0.000000000000000000, 0.3420201433256694346, -0.9396926207859080948 ) ) ;
#66622=CARTESIAN_POINT ( 'NONE',  ( -16.85391023282967637, -2.523321265292116866, 31.42251411153756990 ) ) ;
#66624=ORIENTED_EDGE ( 'NONE', *, *, #59201, .T. ) ;
#66626=CARTESIAN_POINT ( 'NONE',  ( 5.076923076922954969, -6.879047030192662504, 34.71129190930017927 ) ) ;
#66627=DIRECTION ( 'NONE',  ( 0.000000000000000000, 0.3420201433256610524, 0.9396926207859113145 ) ) ;
#66628=CARTESIAN_POINT ( 'NONE',  ( -3.230769230769229949, -9.819645486525091727, 36.12317359536749706 ) ) ;
#66629=CARTESIAN_POINT ( 'NONE',  ( 6.699591979352973681, -12.24155766932282496, 31.33739205006857986 ) ) ;
#66630=CARTESIAN_POINT ( 'NONE',  ( 5.326868486301119532, -3.520799739797213501, 33.17531984108286025 ) ) ;
#66632=CARTESIAN_POINT ( 'NONE',  ( -9.019253993452226226, -10.18141759479407327, 34.26406193332782379 ) ) ;
#66633=CARTESIAN_POINT ( 'NONE',  ( -17.07692307692307665, -4.661471528628507777, 34.16647553114623292 ) ) ;
#66634=CARTESIAN_POINT ( 'NONE',  ( -1.384615384615383471, -3.886160181151819604, 36.00935417666054406 ) ) ;
#66636=DIRECTION ( 'NONE',  ( -0.000000000000000000, -0.9396926207859092051, -0.3420201433256662704 ) ) ;
#66637=CARTESIAN_POINT ( 'NONE',  ( 15.16549923021291235, -12.51329471203370325, 31.30864560766548976 ) ) ;
#66638=CARTESIAN_POINT ( 'NONE',  ( -3.480769230769229061, -7.500000000000001776, 34.75000000000000000 ) ) ;
#66639=CARTESIAN_POINT ( 'NONE',  ( 7.053867364043874488, -2.295524264805589354, 30.44142389570982488 ) ) ;
#66640=CARTESIAN_POINT ( 'NONE',  ( -2.307692307692305711, -5.180354513474913603, 36.12317359536750416 ) ) ;
#66641=LINE ( 'NONE', #4946, #1062 ) ;
#66642=ORIENTED_EDGE ( 'NONE', *, *, #40114, .F. ) ;
#66643=B_SPLINE_CURVE_WITH_KNOTS ( 'NONE', 3,
 ( #78978, #48506, #1212, #51037, #55711, #28696, #21933, #83200, #56160, #49409 ),
 .UNSPECIFIED., .F., .F.,
 ( 4, 2, 2, 2, 4 ),
 ( 0.0007817246336856289524, 0.0009771112958940101571, 0.001172497958102391253, 0.001367884620310772350, 0.001563271282519153446 ),
 .UNSPECIFIED. ) ;
#66644=LINE ( 'NONE', #88711, #8231 ) ;
#66646=CARTESIAN_POINT ( 'NONE',  ( -4.403822897894745125, -5.643011162660950042, 34.66104346484419096 ) ) ;
#66649=B_SPLINE_CURVE_WITH_KNOTS ( 'NONE', 3,
 ( #3151, #45024, #85583, #72059, #52227, #57662, #10370, #3598, #59438, #37831 ),
 .UNSPECIFIED., .F., .F.,
 ( 4, 2, 2, 2, 4 ),
 ( 0.0007817246256747453293, 0.0009771112852218889842, 0.001172497944769032531, 0.001367884604316176294, 0.001563271263863319840 ),
 .UNSPECIFIED. ) ;
#66650=CARTESIAN_POINT ( 'NONE',  ( 13.63456090296352841, -5.057305518903948638, 34.11320923018887896 ) ) ;
#66651=CARTESIAN_POINT ( 'NONE',  ( 8.639082799499075094, -10.31621877034669588, 34.18098118002070152 ) ) ;
#66652=CARTESIAN_POINT ( 'NONE',  ( 17.07692307692307665, -12.62096338111211580, 30.90682066428153263 ) ) ;
#66653=VERTEX_POINT ( 'NONE', #54070 ) ;
#66655=CARTESIAN_POINT ( 'NONE',  ( 17.86930853333243618, -3.530157926970578508, 32.79014554554150607 ) ) ;
#66656=EDGE_LOOP ( 'NONE', ( #15909, #88520 ) ) ;
#66657=CARTESIAN_POINT ( 'NONE',  ( -17.93474442872397034, -3.835265460703682017, 33.15142922261929925 ) ) ;
#66658=EDGE_LOOP ( 'NONE', ( #4947, #53408 ) ) ;
#66659=FACE_OUTER_BOUND ( 'NONE', #58765, .T. ) ;
#66660=CARTESIAN_POINT ( 'NONE',  ( -15.29685161012936589, -2.833524468853757305, 32.15551576947924417 ) ) ;
#66661=CARTESIAN_POINT ( 'NONE',  ( -15.23076923076891553, -2.255955759149395501, 30.00000000000324363 ) ) ;
#66663=CARTESIAN_POINT ( 'NONE',  ( -10.39260507411620438, -12.44528174975671853, 30.48912976160716681 ) ) ;
#66667=EDGE_LOOP ( 'NONE', ( #25063, #73772, #61857, #23887 ) ) ;
#66668=CARTESIAN_POINT ( 'NONE',  ( 2.242422307135989890, -9.528491918058357157, 34.59228464037090589 ) ) ;
#66669=CARTESIAN_POINT ( 'NONE',  ( 12.59233026936325039, -12.11778462344221019, 31.66786338562085135 ) ) ;
#66671=CARTESIAN_POINT ( 'NONE',  ( -10.61538461538461320, -2.538708090699994813, 30.37095296980875503 ) ) ;
#66672=CARTESIAN_POINT ( 'NONE',  ( 9.915087361285761958, -10.23759521482555357, 34.22997729860117033 ) ) ;
#66673=CARTESIAN_POINT ( 'NONE',  ( 0.4615384615383382183, -2.379036618888197285, 30.90682066428292885 ) ) ;
#66676=CARTESIAN_POINT ( 'NONE',  ( 18.00000000000000000, -2.499999999999998668, 29.75000000000001421 ) ) ;
#66677=VERTEX_POINT ( 'NONE', #26614 ) ;
#66678=ORIENTED_EDGE ( 'NONE', *, *, #74300, .T. ) ;
#66679=B_SPLINE_CURVE_WITH_KNOTS ( 'NONE', 3,
 ( #5796, #61616, #54415, #27397, #81912, #60735, #13875, #26514, #40482, #374 ),
 .UNSPECIFIED., .F., .F.,
 ( 4, 2, 2, 2, 4 ),
 ( 0.0007817359430256251270, 0.0009771253907249900349, 0.001172514838424354834, 0.001367904286123719851, 0.001563293733823084650 ),
 .UNSPECIFIED. ) ;
#66681=ORIENTED_EDGE ( 'NONE', *, *, #78093, .T. ) ;
#66683=ORIENTED_EDGE ( 'NONE', *, *, #54892, .T. ) ;
#66684=B_SPLINE_CURVE_WITH_KNOTS ( 'NONE', 3,
 ( #46591, #80838, #38504, #24531, #51998, #65518, #32196, #10588, #11475, #24980 ),
 .UNSPECIFIED., .F., .F.,
 ( 4, 2, 2, 2, 4 ),
 ( 0.0007817359430256328248, 0.0009771253907249995759, 0.001172514838424366327, 0.001367904286123733078, 0.001563293733823099829 ),
 .UNSPECIFIED. ) ;
#66685=CARTESIAN_POINT ( 'NONE',  ( -14.05763788777885637, -10.82426656108012075, 33.81400080652039009 ) ) ;
#66686=LINE ( 'NONE', #59921, #59695 ) ;
#66687=EDGE_LOOP ( 'NONE', ( #56228, #70609, #78549, #12627 ) ) ;
#66688=CARTESIAN_POINT ( 'NONE',  ( 14.55763771707034948, -12.07971442181322352, 32.31769673815850297 ) ) ;
#66689=ORIENTED_EDGE ( 'NONE', *, *, #40936, .T. ) ;
#66690=CARTESIAN_POINT ( 'NONE',  ( 11.66898724022510159, -2.619367082507849442, 30.83698974864643461 ) ) ;
#66691=VERTEX_POINT ( 'NONE', #39252 ) ;
#66692=CARTESIAN_POINT ( 'NONE',  ( -9.442307692307679190, -2.249999999999999112, 29.81603969181031033 ) ) ;
#66693=EDGE_CURVE ( 'NONE', #82761, #65424, #59949, .T. ) ;
#66695=CARTESIAN_POINT ( 'NONE',  ( -8.096177083446809419, -2.587272538249755893, 30.68239716806877837 ) ) ;
#66696=CARTESIAN_POINT ( 'NONE',  ( -9.442307692306272315, -7.500000000000154543, 35.00000000000007105 ) ) ;
#66697=FACE_BOUND ( 'NONE', #14554, .T. ) ;
#66698=AXIS2_PLACEMENT_3D ( 'NONE', #13587, #19897, #26220 ) ;
#66700=CARTESIAN_POINT ( 'NONE',  ( 1.161787286980507705, -7.369209533119137845, 34.99857337881830688 ) ) ;
#66701=VECTOR ( 'NONE', #10081, 1000.000000000000114 ) ;
#66702=CARTESIAN_POINT ( 'NONE',  ( -14.30769230769242917, -4.320704448113951379, 33.92786785259630022 ) ) ;
#66703=EDGE_CURVE ( 'NONE', #45365, #20449, #36128, .T. ) ;
#66704=CYLINDRICAL_SURFACE ( 'NONE', #24448, 0.2499999999999995559 ) ;
#66706=CARTESIAN_POINT ( 'NONE',  ( 10.61538461538449418, -11.06231777344772027, 33.60647404775119895 ) ) ;
#66707=EDGE_LOOP ( 'NONE', ( #53649, #55025, #14878, #50095 ) ) ;
#66708=DIRECTION ( 'NONE',  ( 0.000000000000000000, 0.4999999999999960032, -0.8660254037844410391 ) ) ;
#66709=EDGE_LOOP ( 'NONE', ( #2325, #55540 ) ) ;
#66710=ORIENTED_EDGE ( 'NONE', *, *, #86211, .F. ) ;
#66711=CARTESIAN_POINT ( 'NONE',  ( -0.6850234052624096792, -9.331801661448606566, 34.40259984581193464 ) ) ;
#66712=CARTESIAN_POINT ( 'NONE',  ( -14.17716660592874689, -12.45806712695776319, 30.39783852428763922 ) ) ;
#66713=CARTESIAN_POINT ( 'NONE',  ( -3.230769230769229949, -5.180354513474913603, 36.12317359536750416 ) ) ;
#66714=CARTESIAN_POINT ( 'NONE',  ( 3.361561038594017337, -10.54018710029568595, 33.71981072465678864 ) ) ;
#66715=CARTESIAN_POINT ( 'NONE',  ( 16.85399685940693004, -8.239355502252617924, 34.69524867566427417 ) ) ;
#66716=CARTESIAN_POINT ( 'NONE',  ( -12.46153846153846168, -4.098570777380720287, 33.41473453929634729 ) ) ;
#66717=VERTEX_POINT ( 'NONE', #32930 ) ;
#66718=CARTESIAN_POINT ( 'NONE',  ( 16.82694634598072270, -5.728515186090277211, 34.42611988154120439 ) ) ;
#66719=CARTESIAN_POINT ( 'NONE',  ( -5.010854725920637520, -2.538708090699994813, 30.37095296980875503 ) ) ;
#66720=CARTESIAN_POINT ( 'NONE',  ( 10.39245765647776309, -2.889293201056495786, 32.26117774369186009 ) ) ;
#66721=CARTESIAN_POINT ( 'NONE',  ( -16.08859101433330707, -4.320704448112858032, 33.92786785259548310 ) ) ;
#66722=ORIENTED_EDGE ( 'NONE', *, *, #14287, .F. ) ;
#66723=ORIENTED_EDGE ( 'NONE', *, *, #80323, .T. ) ;
#66725=ORIENTED_EDGE ( 'NONE', *, *, #55181, .T. ) ;
#66726=CARTESIAN_POINT ( 'NONE',  ( 18.13079044096694759, -12.62708834333097663, 30.88030960425256310 ) ) ;
#66727=CARTESIAN_POINT ( 'NONE',  ( 4.946232473812766983, -2.845849958028613624, 32.17971566917920967 ) ) ;
#66728=EDGE_LOOP ( 'NONE', ( #27759, #83333 ) ) ;
#66730=CARTESIAN_POINT ( 'NONE',  ( -6.130690603110307890, -9.084618155246140248, 34.75535874321725771 ) ) ;
#66732=CARTESIAN_POINT ( 'NONE',  ( -2.530618525208452763, -8.239355502252617924, 34.69524867566427417 ) ) ;
#66733=CARTESIAN_POINT ( 'NONE',  ( -0.4615384615385826339, -2.625532179533779598, 30.86335684631627174 ) ) ;
#66735=ORIENTED_EDGE ( 'NONE', *, *, #15698, .F. ) ;
#66736=CARTESIAN_POINT ( 'NONE',  ( -14.98082382139119062, -2.341251567377310217, 30.72681386836322659 ) ) ;
#66737=ORIENTED_EDGE ( 'NONE', *, *, #48596, .T. ) ;
#66738=CARTESIAN_POINT ( 'NONE',  ( -8.769230769230890843, -10.21337939537710326, 33.94971097300076224 ) ) ;
#66739=DIRECTION ( 'NONE',  ( -0.000000000000000000, -0.000000000000000000, -1.000000000000000000 ) ) ;
#66741=CARTESIAN_POINT ( 'NONE',  ( 18.13052570176355971, -8.586989748646450593, 34.63063291749215011 ) ) ;
#66742=CARTESIAN_POINT ( 'NONE',  ( -3.931066484868086075, -4.989023458446560255, 34.36081565061822118 ) ) ;
#66743=CARTESIAN_POINT ( 'NONE',  ( -5.299850035829924977, -10.77366814457252175, 33.85459836347579454 ) ) ;
#66744=DIRECTION ( 'NONE',  ( -0.000000000000000000, 0.5000000000000011102, -0.8660254037844381525 ) ) ;
#66747=DIRECTION ( 'NONE',  ( 0.000000000000000000, 0.1736481776669275834, 0.9848077530122086864 ) ) ;
#66748=CARTESIAN_POINT ( 'NONE',  ( 8.096153846153782752, -7.565270000091922853, 34.99999999999999289 ) ) ;
#66749=CARTESIAN_POINT ( 'NONE',  ( -11.53846153846165912, -9.442884908241554243, 34.35708131394783038 ) ) ;
#66750=ORIENTED_EDGE ( 'NONE', *, *, #11680, .T. ) ;
#66751=ORIENTED_EDGE ( 'NONE', *, *, #12041, .F. ) ;
#66752=CARTESIAN_POINT ( 'NONE',  ( -8.769230769230768274, -5.471508081941601098, 34.59228464037088457 ) ) ;
#66753=CARTESIAN_POINT ( 'NONE',  ( 11.47319153790521717, -12.70778746994557551, 30.41441678777548319 ) ) ;
#66754=CARTESIAN_POINT ( 'NONE',  ( -0.5916864312701568540, -9.504002272028875709, 34.60269587691767867 ) ) ;
#66755=EDGE_CURVE ( 'NONE', #47148, #43255, #71521, .T. ) ;
#66756=CARTESIAN_POINT ( 'NONE',  ( -10.83886953994894853, -2.353723527008296568, 30.78948104536958752 ) ) ;
#66757=FACE_OUTER_BOUND ( 'NONE', #73111, .T. ) ;
#66758=DIRECTION ( 'NONE',  ( -0.000000000000000000, -0.7660444431189791237, -0.6427876096865379196 ) ) ;
#66759=B_SPLINE_CURVE_WITH_KNOTS ( 'NONE', 3,
 ( #47005, #12790, #54206, #40275, #4253, #33514, #67297, #73625, #39828, #5591 ),
 .UNSPECIFIED., .F., .F.,
 ( 4, 2, 2, 2, 4 ),
 ( 0.000000000000000000, 0.0001954311564186863594, 0.0003908623128373726104, 0.0005862934692560589156, 0.0007817246256747452209 ),
 .UNSPECIFIED. ) ;
#66760=EDGE_LOOP ( 'NONE', ( #10481, #7385, #9649, #21740 ) ) ;
#66761=CARTESIAN_POINT ( 'NONE',  ( -16.40386937806761125, -6.652501968072647820, 34.93155406624980941 ) ) ;
#66764=CARTESIAN_POINT ( 'NONE',  ( 4.153846153846030731, -8.656820664282941280, 34.87096338111179961 ) ) ;
#66766=CARTESIAN_POINT ( 'NONE',  ( 12.68454981315131036, -3.587049720035815348, 32.86302985866382897 ) ) ;
#66768=EDGE_CURVE ( 'NONE', #87399, #51804, #34988, .T. ) ;
#66769=ORIENTED_EDGE ( 'NONE', *, *, #23330, .T. ) ;
#66770=CARTESIAN_POINT ( 'NONE',  ( 13.63466969625370062, -3.627508038966690496, 32.91356715214248396 ) ) ;
#66771=CARTESIAN_POINT ( 'NONE',  ( 10.61538461538449418, -3.643525952248795718, 33.31231777344771672 ) ) ;
#66772=DIRECTION ( 'NONE',  ( -1.000000000000000000, 0.000000000000000000, 0.000000000000000000 ) ) ;
#66774=B_SPLINE_CURVE_WITH_KNOTS ( 'NONE', 3,
 ( #40195, #87059, #53238, #19022, #31646, #11373, #46922, #38852, #25779, #60443 ),
 .UNSPECIFIED., .F., .F.,
 ( 4, 2, 2, 2, 4 ),
 ( 0.000000000000000000, 0.0001954339857564093175, 0.0003908679715128186350, 0.0005863019572692279796, 0.0007817359430256372700 ),
 .UNSPECIFIED. ) ;
#66775=ADVANCED_FACE ( 'NONE', ( #7233 ), #35591, .F. ) ;
#66776=CARTESIAN_POINT ( 'NONE',  ( -13.31854805126531005, -4.661471528628508665, 34.16647553114624003 ) ) ;
#66777=CYLINDRICAL_SURFACE ( 'NONE', #14769, 0.2499999999999986955 ) ;
#66778=DIRECTION ( 'NONE',  ( 0.000000000000000000, 0.9848077530122072432, 0.1736481776669354937 ) ) ;
#66779=CARTESIAN_POINT ( 'NONE',  ( -17.07692307692319744, -12.51329471203414379, 31.30864560766407578 ) ) ;
#66780=CARTESIAN_POINT ( 'NONE',  ( -4.946132635956126400, -8.191423895709842640, 34.95447573519442130 ) ) ;
#66781=VERTEX_POINT ( 'NONE', #63039 ) ;
#66782=EDGE_CURVE ( 'NONE', #72551, #85757, #48206, .T. ) ;
#66784=ORIENTED_EDGE ( 'NONE', *, *, #9186, .T. ) ;
#66785=CARTESIAN_POINT ( 'NONE',  ( 5.076923076922953193, -11.67786785259630911, 32.92929555188603530 ) ) ;
#66787=EDGE_CURVE ( 'NONE', #85159, #61364, #76576, .T. ) ;
#66788=CARTESIAN_POINT ( 'NONE',  ( -11.78846153846153832, -7.500000000000001776, 35.00000000000000000 ) ) ;
#66790=CARTESIAN_POINT ( 'NONE',  ( -14.17690049986752143, -12.11778462344220841, 31.66786338562085135 ) ) ;
#66793=ORIENTED_EDGE ( 'NONE', *, *, #11994, .F. ) ;
#66794=VECTOR ( 'NONE', #83118, 999.9999999999998863 ) ;
#66795=ORIENTED_EDGE ( 'NONE', *, *, #11265, .F. ) ;
#66796=ORIENTED_EDGE ( 'NONE', *, *, #59801, .T. ) ;
#66797=EDGE_LOOP ( 'NONE', ( #51247, #447 ) ) ;
#66798=ORIENTED_EDGE ( 'NONE', *, *, #32787, .F. ) ;
#66799=EDGE_CURVE ( 'NONE', #72105, #78212, #21622, .T. ) ;
#66800=CARTESIAN_POINT ( 'NONE',  ( -16.21992956480203318, -3.513871655860377086, 32.76840700105978499 ) ) ;
#66802=EDGE_CURVE ( 'NONE', #19490, #35011, #84235, .T. ) ;
#66803=B_SPLINE_CURVE_WITH_KNOTS ( 'NONE', 3,
 ( #70338, #29802, #21704, #64444, #43312, #8645, #28926, #29361, #23464, #30237 ),
 .UNSPECIFIED., .F., .F.,
 ( 4, 2, 2, 2, 4 ),
 ( 0.0007817246256747461966, 0.0009771112852218892010, 0.001172497944769032314, 0.001367884604316175427, 0.001563271263863318323 ),
 .UNSPECIFIED. ) ;
#66804=CARTESIAN_POINT ( 'NONE',  ( -10.48459417441766561, -4.684288915650983043, 34.18129842949671371 ) ) ;
#66805=CARTESIAN_POINT ( 'NONE',  ( 3.930919936330004472, -3.105860786376062332, 32.13614157043599562 ) ) ;
#66806=CARTESIAN_POINT ( 'NONE',  ( 0.7115927731767758280, -4.943051570960395047, 34.04725096376909477 ) ) ;
#66809=ADVANCED_FACE ( 'NONE', ( #14883 ), #83789, .F. ) ;
#66810=CARTESIAN_POINT ( 'NONE',  ( 17.74997676270703550, -2.587272538249754117, 30.68239716806877837 ) ) ;
#66811=CARTESIAN_POINT ( 'NONE',  ( 6.923076923076924238, -1.422936976036506707, 30.56769352161908415 ) ) ;
#66813=ORIENTED_EDGE ( 'NONE', *, *, #22721, .F. ) ;
#66814=ORIENTED_EDGE ( 'NONE', *, *, #57473, .F. ) ;
#66815=DIRECTION ( 'NONE',  ( -1.000000000000000000, -0.000000000000000000, -0.000000000000000000 ) ) ;
#66816=ORIENTED_EDGE ( 'NONE', *, *, #25976, .F. ) ;
#66817=CARTESIAN_POINT ( 'NONE',  ( 6.792928953345226617, -11.66186481527757479, 32.95055677023626117 ) ) ;
#66818=CARTESIAN_POINT ( 'NONE',  ( -5.749945688361685292, -3.627508038966690496, 32.91356715214248396 ) ) ;
#66820=CARTESIAN_POINT ( 'NONE',  ( -11.47320639894870276, -9.528491918058460186, 34.59228464037086326 ) ) ;
#66821=FACE_BOUND ( 'NONE', #112, .T. ) ;
#66822=VERTEX_POINT ( 'NONE', #49546 ) ;
#66824=CARTESIAN_POINT ( 'NONE',  ( 17.29993592101647693, -5.582272713120730145, 34.63742843783360570 ) ) ;
#66827=FACE_BOUND ( 'NONE', #60145, .T. ) ;
#66828=CARTESIAN_POINT ( 'NONE',  ( -10.83886953994894675, -3.019605429927184836, 32.48692288466676814 ) ) ;
#66829=VECTOR ( 'NONE', #60870, 1000.000000000000000 ) ;
#66830=DIRECTION ( 'NONE',  ( -0.000000000000000000, -0.9396926207859093161, -0.3420201433256663259 ) ) ;
#66831=ORIENTED_EDGE ( 'NONE', *, *, #18294, .T. ) ;
#66833=CARTESIAN_POINT ( 'NONE',  ( -1.449885385171703067, -8.656820664281497102, 34.87096338111211935 ) ) ;
#66834=LINE ( 'NONE', #65493, #22024 ) ;
#66835=VERTEX_POINT ( 'NONE', #49976 ) ;
#66837=CARTESIAN_POINT ( 'NONE',  ( -14.43783951713053249, -6.001485441113819874, 34.52039167877662607 ) ) ;
#66838=CARTESIAN_POINT ( 'NONE',  ( 11.53846153846153832, -3.669653830205710676, 35.88435417666054406 ) ) ;
#66840=FACE_OUTER_BOUND ( 'NONE', #74217, .T. ) ;
#66842=ORIENTED_EDGE ( 'NONE', *, *, #76373, .T. ) ;
#66843=CARTESIAN_POINT ( 'NONE',  ( 8.769230769230645706, -11.67786785259630911, 32.92929555188603530 ) ) ;
#66844=CARTESIAN_POINT ( 'NONE',  ( -12.33101275977489841, -2.619367082507849442, 30.83698974864643461 ) ) ;
#66845=CARTESIAN_POINT ( 'NONE',  ( -14.53117723225664371, -2.612411019501189369, 31.66733052389439962 ) ) ;
#66846=CARTESIAN_POINT ( 'NONE',  ( -12.46153846153846168, -5.415277668671390821, 36.20867863119892149 ) ) ;
#66847=CARTESIAN_POINT ( 'NONE',  ( 13.38461538461538680, -2.249999999999998668, 29.75000000000001776 ) ) ;
#66848=ADVANCED_FACE ( 'NONE', ( #15764 ), #70703, .F. ) ;
#66849=CARTESIAN_POINT ( 'NONE',  ( 17.29993592101647337, -4.762714258010882773, 34.23016756924214832 ) ) ;
#66850=CARTESIAN_POINT ( 'NONE',  ( -1.515306851282941958, -4.809359713505814149, 33.96456829005828837 ) ) ;
#66851=FACE_OUTER_BOUND ( 'NONE', #79291, .T. ) ;
#66852=B_SPLINE_CURVE_WITH_KNOTS ( 'NONE', 3,
 ( #19499, #12744, #46960, #6001, #68136, #5103, #80783, #68571, #27586, #33897 ),
 .UNSPECIFIED., .F., .F.,
 ( 4, 2, 2, 2, 4 ),
 ( 0.0007817359430256326080, 0.0009771253907250047801, 0.001172514838424369796, 0.001367904286123735030, 0.001563293733823100046 ),
 .UNSPECIFIED. ) ;
#66853=B_SPLINE_CURVE_WITH_KNOTS ( 'NONE', 3,
 ( #22827, #69691, #83670, #9758, #28256, #70581, #84551, #1677, #37223, #21953 ),
 .UNSPECIFIED., .F., .F.,
 ( 4, 2, 2, 2, 4 ),
 ( 0.000000000000000000, 0.0001954311564186871184, 0.0003908623128373742367, 0.0005862934692560614093, 0.0007817246256747484735 ),
 .UNSPECIFIED. ) ;
#66854=CARTESIAN_POINT ( 'NONE',  ( -39.05038313613820122, -2.249999999999998668, 29.75000000000000355 ) ) ;
#66856=ADVANCED_FACE ( 'NONE', ( #29721 ), #82897, .F. ) ;
#66857=B_SPLINE_CURVE_WITH_KNOTS ( 'NONE', 3,
 ( #23710, #2554, #31371, #73247, #30045, #85874, #58834, #65143, #23276, #24609 ),
 .UNSPECIFIED., .F., .F.,
 ( 4, 2, 2, 2, 4 ),
 ( 0.000000000000000000, 0.0001954339857564054144, 0.0003908679715128108288, 0.0005863019572692162703, 0.0007817359430256216575 ),
 .UNSPECIFIED. ) ;
#66859=ORIENTED_EDGE ( 'NONE', *, *, #53764, .T. ) ;
#66860=CYLINDRICAL_SURFACE ( 'NONE', #20342, 0.2499999999999993616 ) ;
#66861=EDGE_LOOP ( 'NONE', ( #56924, #53339 ) ) ;
#66862=EDGE_CURVE ( 'NONE', #25698, #36076, #14424, .T. ) ;
#66864=DIRECTION ( 'NONE',  ( -0.000000000000000000, 0.9848077530122086864, -0.1736481776669273891 ) ) ;
#66865=EDGE_LOOP ( 'NONE', ( #20427, #21427 ) ) ;
#66866=CARTESIAN_POINT ( 'NONE',  ( -6.000000000000121680, -10.33852847137269571, 34.16647553114546554 ) ) ;
#66868=CARTESIAN_POINT ( 'NONE',  ( -13.13466997523734214, -5.766571408460171355, 34.70601412856602508 ) ) ;
#66869=CARTESIAN_POINT ( 'NONE',  ( -16.82692307692307665, -2.499999999999998668, 29.75000000000000355 ) ) ;
#66870=LINE ( 'NONE', #5166, #61933 ) ;
#66871=DIRECTION ( 'NONE',  ( -0.000000000000000000, 0.1736481776669307198, -0.9848077530122080203 ) ) ;
#66872=EDGE_CURVE ( 'NONE', #42322, #40124, #73781, .T. ) ;
#66873=VECTOR ( 'NONE', #3023, 1000.000000000000114 ) ;
#66874=CARTESIAN_POINT ( 'NONE',  ( -10.48459417441766206, -3.338503747796866872, 32.95102852606553512 ) ) ;
#66876=CARTESIAN_POINT ( 'NONE',  ( 5.750023269057646935, -4.236021600441998380, 33.53823185664189310 ) ) ;
#66878=DIRECTION ( 'NONE',  ( -0.000000000000000000, -0.5000000000000009992, -0.8660254037844380415 ) ) ;
#66879=CARTESIAN_POINT ( 'NONE',  ( -17.86947456176635640, -2.372941743896879174, 30.88044141588254377 ) ) ;
#66881=ORIENTED_EDGE ( 'NONE', *, *, #85686, .F. ) ;
#66882=ORIENTED_EDGE ( 'NONE', *, *, #36085, .F. ) ;
#66883=DIRECTION ( 'NONE',  ( 0.000000000000000000, 0.4999999999999985567, 0.8660254037844395958 ) ) ;
#66884=CARTESIAN_POINT ( 'NONE',  ( 7.623227628637697428, -11.24512374952581872, 33.06303171183252942 ) ) ;
#66885=CARTESIAN_POINT ( 'NONE',  ( 16.40379156322419973, -12.45601412856602686, 31.48342859153981621 ) ) ;
#66886=DIRECTION ( 'NONE',  ( -0.000000000000000000, -0.3420201433256694346, -0.9396926207859080948 ) ) ;
#66887=ADVANCED_FACE ( 'NONE', ( #2664 ), #39481, .F. ) ;
#66888=CARTESIAN_POINT ( 'NONE',  ( 8.769230769230768274, -4.098570777380720287, 33.41473453929634729 ) ) ;
#66889=CARTESIAN_POINT ( 'NONE',  ( -9.915792616872025178, -6.716662450894489211, 34.94144148231605840 ) ) ;
#66891=EDGE_LOOP ( 'NONE', ( #68595, #40326, #67136, #57297 ) ) ;
#66892=CARTESIAN_POINT ( 'NONE',  ( 16.02315468717859659, -2.729777683071817229, 31.24903638046269450 ) ) ;
#66893=VERTEX_POINT ( 'NONE', #60169 ) ;
#66895=CARTESIAN_POINT ( 'NONE',  ( 16.21910129335899597, -9.528491918058456633, 34.59228464037085615 ) ) ;
#66896=AXIS2_PLACEMENT_3D ( 'NONE', #20456, #74967, #47469 ) ;
#66898=CARTESIAN_POINT ( 'NONE',  ( -0.7115384615384606759, -7.500000000000001776, 35.00000000000000000 ) ) ;
#66899=CIRCLE ( 'NONE', #28065, 0.2500000000000002220 ) ;
#66900=CARTESIAN_POINT ( 'NONE',  ( 11.78840694783958476, -2.341251567377310217, 30.72681386836322659 ) ) ;
#66901=CARTESIAN_POINT ( 'NONE',  ( -5.076923076923199218, -8.656820664282941280, 34.87096338111179961 ) ) ;
#66902=ORIENTED_EDGE ( 'NONE', *, *, #48332, .F. ) ;
#66903=ORIENTED_EDGE ( 'NONE', *, *, #82454, .T. ) ;
#66904=VERTEX_POINT ( 'NONE', #33150 ) ;
#66905=ADVANCED_FACE ( 'NONE', ( #18759 ), #45774, .F. ) ;
#66906=ADVANCED_FACE ( 'NONE', ( #30156 ), #66941, .F. ) ;
#66907=CARTESIAN_POINT ( 'NONE',  ( 0.4615384615384611200, -4.098570777380720287, 33.41473453929634729 ) ) ;
#66908=CARTESIAN_POINT ( 'NONE',  ( 10.61538461538461675, -11.35647404775217417, 33.31231777344666511 ) ) ;
#66910=EDGE_CURVE ( 'NONE', #14505, #48663, #12006, .T. ) ;
#66911=B_SPLINE_CURVE_WITH_KNOTS ( 'NONE', 3,
 ( #32933, #57185, #21623, #63040, #56302, #29722, #14425, #55412, #75678, #77459 ),
 .UNSPECIFIED., .F., .F.,
 ( 4, 2, 2, 2, 4 ),
 ( 0.0007817246256747461966, 0.0009771112852218889842, 0.001172497944769031880, 0.001367884604316174776, 0.001563271263863317672 ),
 .UNSPECIFIED. ) ;
#66912=CARTESIAN_POINT ( 'NONE',  ( -8.638705330997126453, -10.31582465632705237, 34.18122507451815295 ) ) ;
#66913=CARTESIAN_POINT ( 'NONE',  ( -16.94613126909829504, -3.062576670634119758, 32.05464942895959979 ) ) ;
#66914=EDGE_CURVE ( 'NONE', #37313, #41563, #50410, .T. ) ;
#66915=CARTESIAN_POINT ( 'NONE',  ( 17.77651505627605033, -8.496056993536548418, 34.65000542017679663 ) ) ;
#66916=EDGE_LOOP ( 'NONE', ( #28772, #36834 ) ) ;
#66917=ORIENTED_EDGE ( 'NONE', *, *, #81522, .F. ) ;
#66919=VECTOR ( 'NONE', #13127, 1000.000000000000227 ) ;
#66920=CARTESIAN_POINT ( 'NONE',  ( 11.31553532094538994, -9.086856451489515152, 34.49173150075333183 ) ) ;
#66921=EDGE_LOOP ( 'NONE', ( #9093, #27686 ) ) ;
#66922=DIRECTION ( 'NONE',  ( -0.000000000000000000, -0.000000000000000000, -1.000000000000000000 ) ) ;
#66923=CARTESIAN_POINT ( 'NONE',  ( -2.176901866725355461, -3.957578996910244395, 33.62503395064540257 ) ) ;
#66924=B_SPLINE_CURVE_WITH_KNOTS ( 'NONE', 3,
 ( #87329, #25605, #80568, #59386, #74691, #53509, #46317, #66598, #12539, #67927 ),
 .UNSPECIFIED., .F., .F.,
 ( 4, 2, 2, 2, 4 ),
 ( 0.000000000000000000, 0.0001954339857564073659, 0.0003908679715128147319, 0.0005863019572692221250, 0.0007817359430256294638 ),
 .UNSPECIFIED. ) ;
#66925=CARTESIAN_POINT ( 'NONE',  ( 4.153846153846154188, -2.499999999999998668, 29.50000000000001066 ) ) ;
#66926=EDGE_LOOP ( 'NONE', ( #54770, #49617 ) ) ;
#66927=ADVANCED_FACE ( 'NONE', ( #59735 ), #32271, .F. ) ;
#66928=CARTESIAN_POINT ( 'NONE',  ( 3.360814286689004504, -2.254550872974306674, 29.97347326024527447 ) ) ;
#66929=VERTEX_POINT ( 'NONE', #37341 ) ;
#66930=DIRECTION ( 'NONE',  ( 0.000000000000000000, 0.9848077530122072432, -0.1736481776669354937 ) ) ;
#66931=DIRECTION ( 'NONE',  ( 0.000000000000000000, 0.3420201433256641055, -0.9396926207859100932 ) ) ;
#66932=CARTESIAN_POINT ( 'NONE',  ( 17.07692307692307665, -12.34228464037088635, 31.77849191805839268 ) ) ;
#66933=CARTESIAN_POINT ( 'NONE',  ( -6.923076923076922462, -12.37446782046654192, 30.86335684631486131 ) ) ;
#66934=FACE_OUTER_BOUND ( 'NONE', #52020, .T. ) ;
#66935=CYLINDRICAL_SURFACE ( 'NONE', #18941, 0.2499999999999979738 ) ;
#66936=VERTEX_POINT ( 'NONE', #4800 ) ;
#66937=EDGE_CURVE ( 'NONE', #45196, #22351, #40442, .T. ) ;
#66938=CARTESIAN_POINT ( 'NONE',  ( 9.692307692307695177, -1.242168528481310874, 33.36296068462461051 ) ) ;
#66940=B_SPLINE_CURVE_WITH_KNOTS ( 'NONE', 3,
 ( #37170, #11043, #84936, #38067, #38516, #22765, #9701, #86276, #57886, #23215 ),
 .UNSPECIFIED., .F., .F.,
 ( 4, 2, 2, 2, 4 ),
 ( 0.0007817246256747446788, 0.0009771112852218874663, 0.001172497944769030145, 0.001367884604316172825, 0.001563271263863315720 ),
 .UNSPECIFIED. ) ;
#66941=CYLINDRICAL_SURFACE ( 'NONE', #2053, 0.2499999999999973355 ) ;
#66942=ORIENTED_EDGE ( 'NONE', *, *, #38313, .T. ) ;
#66943=B_SPLINE_CURVE_WITH_KNOTS ( 'NONE', 3,
 ( #70492, #50652, #9248, #1593, #36706, #79023, #44781, #63727, #8800, #35828 ),
 .UNSPECIFIED., .F., .F.,
 ( 4, 2, 2, 2, 4 ),
 ( 0.0007817246256747464135, 0.0009771112852218900684, 0.001172497944769033615, 0.001367884604316177161, 0.001563271263863320925 ),
 .UNSPECIFIED. ) ;
#66944=DIRECTION ( 'NONE',  ( -0.000000000000000000, -0.9848077530122086864, -0.1736481776669273613 ) ) ;
#66945=CARTESIAN_POINT ( 'NONE',  ( 10.48523664565292002, -8.630895178749533159, 34.87696386517710323 ) ) ;
#66947=CARTESIAN_POINT ( 'NONE',  ( -0.6844171439671091761, -7.630691491037286056, 34.74850469731152458 ) ) ;
#66948=EDGE_CURVE ( 'NONE', #70315, #68861, #48067, .T. ) ;
#66949=VECTOR ( 'NONE', #47107, 1000.000000000000000 ) ;
#66950=FACE_BOUND ( 'NONE', #47368, .T. ) ;
#66951=CARTESIAN_POINT ( 'NONE',  ( -4.153846153846152411, -5.557115091759785130, 34.35708131394839171 ) ) ;
#66952=DIRECTION ( 'NONE',  ( 0.000000000000000000, 0.1736481776669275834, 0.9848077530122086864 ) ) ;
#66953=CARTESIAN_POINT ( 'NONE',  ( 2.084207383127978819, -10.23692288466677880, 34.23039457007281072 ) ) ;
#66954=CARTESIAN_POINT ( 'NONE',  ( -17.86920819217521483, -11.18335022499818265, 33.13157742990017596 ) ) ;
#66955=CARTESIAN_POINT ( 'NONE',  ( -9.469296340694842939, -10.61302985866383963, 33.66295027996417843 ) ) ;
#66956=CARTESIAN_POINT ( 'NONE',  ( -39.05038313613820122, -2.499999999999999556, 29.75000000000000355 ) ) ;
#66958=ORIENTED_EDGE ( 'NONE', *, *, #43640, .T. ) ;
#66959=ADVANCED_FACE ( 'NONE', ( #19196 ), #39922, .F. ) ;
#66960=CARTESIAN_POINT ( 'NONE',  ( 10.39245765647776487, -11.98009711892699514, 32.48740034544076138 ) ) ;
#66962=LINE ( 'NONE', #88589, #55039 ) ;
#66963=ORIENTED_EDGE ( 'NONE', *, *, #8118, .T. ) ;
#66964=CARTESIAN_POINT ( 'NONE',  ( -3.903900635498009919, -12.22109172314383052, 31.39792113162168263 ) ) ;
#66967=VECTOR ( 'NONE', #9860, 1000.000000000000000 ) ;
#66968=ORIENTED_EDGE ( 'NONE', *, *, #38351, .F. ) ;
#66969=CARTESIAN_POINT ( 'NONE',  ( -16.15384615384615330, -2.538708090699994813, 30.37095296980875503 ) ) ;
#66970=CARTESIAN_POINT ( 'NONE',  ( 6.066067333350077639, -3.322132147404559976, 32.92929555188717927 ) ) ;
#66972=CARTESIAN_POINT ( 'NONE',  ( 15.16549923021291413, -12.16647553114622049, 32.15551576947930812 ) ) ;
#66973=CARTESIAN_POINT ( 'NONE',  ( -14.30769230769230660, -11.35647404775217417, 33.31231777344666511 ) ) ;
#66974=EDGE_CURVE ( 'NONE', #23956, #64904, #74140, .T. ) ;
#66975=CARTESIAN_POINT ( 'NONE',  ( 6.923076923076924238, -1.117168528481311540, 33.14645433367849847 ) ) ;
#66976=CARTESIAN_POINT ( 'NONE',  ( 5.999999999999878320, -12.51329471203414379, 31.30864560766407578 ) ) ;
#66977=CARTESIAN_POINT ( 'NONE',  ( 7.053602624840489277, -4.459921816937789885, 33.71989282347011851 ) ) ;
#66980=DIRECTION ( 'NONE',  ( -0.000000000000000000, -0.9848077530122085754, -0.1736481776669273613 ) ) ;
#66981=EDGE_CURVE ( 'NONE', #57772, #25798, #56534, .T. ) ;
#66982=CARTESIAN_POINT ( 'NONE',  ( 14.30769230769231015, -1.509761064869970415, 31.06009739812519044 ) ) ;
#66983=VERTEX_POINT ( 'NONE', #9878 ) ;
#66985=DIRECTION ( 'NONE',  ( 0.000000000000000000, 0.000000000000000000, 1.000000000000000000 ) ) ;
#66986=B_SPLINE_CURVE_WITH_KNOTS ( 'NONE', 3,
 ( #57365, #77639, #43850, #56487, #22257, #71317, #50152, #58247, #15949, #43419 ),
 .UNSPECIFIED., .F., .F.,
 ( 4, 2, 2, 2, 4 ),
 ( 0.000000000000000000, 0.0001954311564186874436, 0.0003908623128373748873, 0.0005862934692560622767, 0.0007817246256747497745 ),
 .UNSPECIFIED. ) ;
#66989=CARTESIAN_POINT ( 'NONE',  ( -16.37733107841048863, -10.97335522853832579, 33.68706563782419749 ) ) ;
#66992=LINE ( 'NONE', #47596, #58613 ) ;
#66993=CARTESIAN_POINT ( 'NONE',  ( 9.442284468086237226, -12.68155406624981119, 30.59749803192733708 ) ) ;
#66994=CARTESIAN_POINT ( 'NONE',  ( 4.853996118016225658, -12.38737895849757820, 31.66785238281580206 ) ) ;
#66996=CARTESIAN_POINT ( 'NONE',  ( 11.66898724022510514, -5.195472089885680766, 34.18748526763464923 ) ) ;
#66997=DIRECTION ( 'NONE',  ( 0.000000000000000000, 0.9396926207859126468, -0.3420201433256571111 ) ) ;
#66999=FACE_OUTER_BOUND ( 'NONE', #18437, .T. ) ;
#67000=CARTESIAN_POINT ( 'NONE',  ( 11.66925334628632882, -8.999086150933475636, 34.52020707165672775 ) ) ;
#67001=EDGE_CURVE ( 'NONE', #33434, #76071, #41684, .T. ) ;
#67002=ORIENTED_EDGE ( 'NONE', *, *, #35179, .T. ) ;
#67003=DIRECTION ( 'NONE',  ( -0.000000000000000000, -0.9396926207859092051, -0.3420201433256662704 ) ) ;
#67004=CARTESIAN_POINT ( 'NONE',  ( -15.48074597481782178, -11.47974371597208076, 33.17467449705390692 ) ) ;
#67006=VERTEX_POINT ( 'NONE', #61941 ) ;
#67007=ORIENTED_EDGE ( 'NONE', *, *, #77635, .F. ) ;
#67008=ORIENTED_EDGE ( 'NONE', *, *, #38982, .F. ) ;
#67009=CARTESIAN_POINT ( 'NONE',  ( -3.230769230769229949, -12.09954503811598769, 35.62045528018868623 ) ) ;
#67010=FACE_OUTER_BOUND ( 'NONE', #83903, .T. ) ;
#67011=LINE ( 'NONE', #5307, #40926 ) ;
#67012=CARTESIAN_POINT ( 'NONE',  ( 14.30769230769231015, -13.87047571288749737, 32.06866353760679544 ) ) ;
#67013=EDGE_LOOP ( 'NONE', ( #40236, #27572, #68340, #71344 ) ) ;
#67014=AXIS2_PLACEMENT_3D ( 'NONE', #73160, #69061, #33059 ) ;
#67015=VERTEX_POINT ( 'NONE', #14208 ) ;
#67016=ORIENTED_EDGE ( 'NONE', *, *, #73315, .T. ) ;
#67017=CARTESIAN_POINT ( 'NONE',  ( -7.053767526187229464, -2.494641256782728966, 31.33461815524612959 ) ) ;
#67019=CARTESIAN_POINT ( 'NONE',  ( 18.00000000000000000, -13.49023893513002648, 31.06009739812518688 ) ) ;
#67020=B_SPLINE_CURVE_WITH_KNOTS ( 'NONE', 3,
 ( #51100, #49469, #17343, #64623, #7599, #3825, #71836, #42279, #21996, #44801 ),
 .UNSPECIFIED., .F., .F.,
 ( 4, 2, 2, 2, 4 ),
 ( 0.0007817359430256294638, 0.0009771253907249974075, 0.001172514838424365460, 0.001367904286123733295, 0.001563293733823094191 ),
 .UNSPECIFIED. ) ;
#67021=DIRECTION ( 'NONE',  ( -0.000000000000000000, 0.8660254037844399289, -0.4999999999999980016 ) ) ;
#67023=CARTESIAN_POINT ( 'NONE',  ( 7.173131342990377135, -4.818054556918156095, 34.26375889529406749 ) ) ;
#67024=DIRECTION ( 'NONE',  ( -0.000000000000000000, -0.9396926207859093161, -0.3420201433256663259 ) ) ;
#67025=EDGE_CURVE ( 'NONE', #79443, #35898, #44714, .T. ) ;
#67026=VECTOR ( 'NONE', #4785, 1000.000000000000000 ) ;
#67030=CARTESIAN_POINT ( 'NONE',  ( 14.55763771707035303, -10.92531984108285670, 33.72920026020278073 ) ) ;
#67032=EDGE_LOOP ( 'NONE', ( #11277, #20589 ) ) ;
#67033=EDGE_CURVE ( 'NONE', #88230, #51973, #7006, .T. ) ;
#67034=CARTESIAN_POINT ( 'NONE',  ( -10.74594452899797936, -2.254533558242300284, 29.97296025877828285 ) ) ;
#67035=CARTESIAN_POINT ( 'NONE',  ( -0.4615384615384611200, -4.661471528628507777, 34.16647553114623292 ) ) ;
#67036=LINE ( 'NONE', #53956, #56102 ) ;
#67037=FACE_OUTER_BOUND ( 'NONE', #34218, .T. ) ;
#67038=EDGE_CURVE ( 'NONE', #11273, #28791, #67825, .T. ) ;
#67039=LINE ( 'NONE', #52619, #23791 ) ;
#67040=FACE_BOUND ( 'NONE', #35561, .T. ) ;
#67041=CARTESIAN_POINT ( 'NONE',  ( -0.6850234052624097902, -4.386631170607604879, 33.66268669641500111 ) ) ;
#67043=CARTESIAN_POINT ( 'NONE',  ( -5.999999999999998224, -2.708943851104267164, 35.45975837776705220 ) ) ;
#67045=CARTESIAN_POINT ( 'NONE',  ( 15.48082365068268018, -10.06805714834173493, 34.32951233291982618 ) ) ;
#67046=CARTESIAN_POINT ( 'NONE',  ( -4.403846153846151523, -7.500000000000001776, 35.00000000000000000 ) ) ;
#67047=DIRECTION ( 'NONE',  ( -0.000000000000000000, -0.9848077530122085754, -0.1736481776669273613 ) ) ;
#67048=VERTEX_POINT ( 'NONE', #253 ) ;
#67050=DIRECTION ( 'NONE',  ( 0.000000000000000000, 0.8660254037844377084, 0.5000000000000015543 ) ) ;
#67051=ORIENTED_EDGE ( 'NONE', *, *, #66782, .T. ) ;
#67052=ORIENTED_EDGE ( 'NONE', *, *, #11437, .F. ) ;
#67053=VECTOR ( 'NONE', #70193, 1000.000000000000227 ) ;
#67054=CARTESIAN_POINT ( 'NONE',  ( -6.923076923077044142, -5.219633306517616589, 34.19971097300220464 ) ) ;
#67055=EDGE_CURVE ( 'NONE', #40219, #26904, #6569, .T. ) ;
#67056=B_SPLINE_CURVE_WITH_KNOTS ( 'NONE', 3,
 ( #29813, #1449, #84324, #28031, #36134, #16291, #63585, #69013, #28939, #1887 ),
 .UNSPECIFIED., .F., .F.,
 ( 4, 2, 2, 2, 4 ),
 ( 0.0007817246256747465219, 0.0009771112852218900684, 0.001172497944769033615, 0.001367884604316177378, 0.001563271263863320925 ),
 .UNSPECIFIED. ) ;
#67057=DIRECTION ( 'NONE',  ( 0.000000000000000000, 0.3420201433256610524, 0.9396926207859113145 ) ) ;
#67058=DIRECTION ( 'NONE',  ( -0.000000000000000000, 0.5000000000000011102, -0.8660254037844381525 ) ) ;
#67059=ORIENTED_EDGE ( 'NONE', *, *, #37154, .T. ) ;
#67060=CARTESIAN_POINT ( 'NONE',  ( 13.38461538461526601, -2.892918686052165622, 31.69288490824153470 ) ) ;
#67061=CARTESIAN_POINT ( 'NONE',  ( 6.923076923076924238, -13.78497067705608181, 32.30358669280327177 ) ) ;
#67062=LINE ( 'NONE', #67950, #38948 ) ;
#67063=CARTESIAN_POINT ( 'NONE',  ( 5.750023255951410839, -6.524016743844655686, 34.90889640711025521 ) ) ;
#67065=CARTESIAN_POINT ( 'NONE',  ( 0.5920638997721049401, -5.070358843744209310, 34.40418822224088302 ) ) ;
#67066=CARTESIAN_POINT ( 'NONE',  ( -10.55012947587177941, -11.67786785259547777, 32.92929555188713664 ) ) ;
#67068=ORIENTED_EDGE ( 'NONE', *, *, #24063, .T. ) ;
#67069=EDGE_CURVE ( 'NONE', #20099, #58521, #27505, .T. ) ;
#67070=VERTEX_POINT ( 'NONE', #62379 ) ;
#67072=ADVANCED_FACE ( 'NONE', ( #82232 ), #48876, .F. ) ;
#67073=CARTESIAN_POINT ( 'NONE',  ( 6.923076923076924238, -12.10708131394839349, 31.69288490824020244 ) ) ;
#67074=CARTESIAN_POINT ( 'NONE',  ( 10.68145296638705410, -2.538708090699994813, 30.37095296980875503 ) ) ;
#67076=CARTESIAN_POINT ( 'NONE',  ( -3.454254174493178287, -5.912607949931405038, 34.49155766932282319 ) ) ;
#67078=DIRECTION ( 'NONE',  ( -0.000000000000000000, 0.1736481776669307198, -0.9848077530122080203 ) ) ;
#67079=CARTESIAN_POINT ( 'NONE',  ( 14.05766908347085042, -6.652501968072648708, 34.93155406624980941 ) ) ;
#67080=DIRECTION ( 'NONE',  ( -0.000000000000000000, 1.000000000000000000, 3.491481338843133355E-15 ) ) ;
#67081=CARTESIAN_POINT ( 'NONE',  ( 12.33139049180676494, -11.66186481527757302, 32.95055677023626117 ) ) ;
#67082=CARTESIAN_POINT ( 'NONE',  ( 9.823099500132478568, -2.729792928343269587, 31.24908615093345077 ) ) ;
#67083=CARTESIAN_POINT ( 'NONE',  ( 8.639083559792545941, -12.27039167877662251, 31.24851455888617835 ) ) ;
#67084=CARTESIAN_POINT ( 'NONE',  ( 5.869308533332440625, -12.11776431015576172, 31.66791131148498906 ) ) ;
#67085=CARTESIAN_POINT ( 'NONE',  ( 4.087762742890272527, -12.37446782046654192, 30.86335684631486487 ) ) ;
#67086=VECTOR ( 'NONE', #50219, 1000.000000000000227 ) ;
#67088=EDGE_CURVE ( 'NONE', #879, #17306, #12511, .T. ) ;
#67089=CARTESIAN_POINT ( 'NONE',  ( -7.596099534515530216, -12.41262288849542017, 30.68299917996395010 ) ) ;
#67090=ORIENTED_EDGE ( 'NONE', *, *, #74654, .F. ) ;
#67091=CARTESIAN_POINT ( 'NONE',  ( 8.769230769230768274, -12.62096338111211580, 30.90682066428153263 ) ) ;
#67092=CARTESIAN_POINT ( 'NONE',  ( -17.14300545628320904, -6.343179335718451384, 34.87096338111212646 ) ) ;
#67093=CARTESIAN_POINT ( 'NONE',  ( 6.000000000000001776, -2.486705287966279876, 31.30864560766543647 ) ) ;
#67095=B_SPLINE_CURVE_WITH_KNOTS ( 'NONE', 3,
 ( #77632, #79415, #17715, #43410, #70884, #50598 ),
 .UNSPECIFIED., .F., .F.,
 ( 4, 2, 4 ),
 ( 0.000000000000000000, 0.0001954784845028902421, 0.0003909569690057804843 ),
 .UNSPECIFIED. ) ;
#67096=CARTESIAN_POINT ( 'NONE',  ( 5.299702745901139878, -10.23759521482555357, 34.22997729860117033 ) ) ;
#67097=CARTESIAN_POINT ( 'NONE',  ( -11.47320639894870276, -5.094484230520773593, 34.41647553114626845 ) ) ;
#67098=B_SPLINE_CURVE_WITH_KNOTS ( 'NONE', 3,
 ( #24070, #39387, #44777, #80373, #38487, #87137, #24512, #17319, #38940, #66397 ),
 .UNSPECIFIED., .F., .F.,
 ( 4, 2, 2, 2, 4 ),
 ( 0.0007817359430256318490, 0.0009771253907249984917, 0.001172514838424365026, 0.001367904286123731560, 0.001563293733823098311 ),
 .UNSPECIFIED. ) ;
#67099=CARTESIAN_POINT ( 'NONE',  ( -0.4615384615385826339, -2.625532179533779598, 30.86335684631627174 ) ) ;
#67100=ORIENTED_EDGE ( 'NONE', *, *, #44105, .F. ) ;
#67102=CARTESIAN_POINT ( 'NONE',  ( -20.75000000000000355, -12.50000000000000000, 27.25000000000000000 ) ) ;
#67103=AXIS2_PLACEMENT_3D ( 'NONE', #19680, #5282, #74632 ) ;
#67104=EDGE_CURVE ( 'NONE', #14267, #53679, #14587, .T. ) ;
#67105=VERTEX_POINT ( 'NONE', #49328 ) ;
#67106=CARTESIAN_POINT ( 'NONE',  ( 0.4615384615384611200, -2.721908614388771852, 31.22303859784724978 ) ) ;
#67107=EDGE_LOOP ( 'NONE', ( #60332, #38400, #22068, #6745 ) ) ;
#67108=B_SPLINE_CURVE_WITH_KNOTS ( 'NONE', 3,
 ( #53226, #18568, #46481, #46911, #10918, #87948, #45583, #11814, #39292, #38389 ),
 .UNSPECIFIED., .F., .F.,
 ( 4, 2, 2, 2, 4 ),
 ( 0.0007817359430256315238, 0.0009771253907249980580, 0.001172514838424364592, 0.001367904286123730910, 0.001563293733823097444 ),
 .UNSPECIFIED. ) ;
#67109=DIRECTION ( 'NONE',  ( -0.000000000000000000, 1.000000000000000000, 3.491481338843133355E-15 ) ) ;
#67110=EDGE_CURVE ( 'NONE', #11909, #72772, #2892, .T. ) ;
#67111=ADVANCED_FACE ( 'NONE', ( #57852 ), #37129, .F. ) ;
#67112=CARTESIAN_POINT ( 'NONE',  ( -7.846153846153965716, -11.94971097300221174, 32.03036669348237098 ) ) ;
#67113=DIRECTION ( 'NONE',  ( 0.000000000000000000, 0.000000000000000000, -1.000000000000000000 ) ) ;
#67114=ORIENTED_EDGE ( 'NONE', *, *, #26646, .T. ) ;
#67115=ORIENTED_EDGE ( 'NONE', *, *, #16666, .F. ) ;
#67116=EDGE_CURVE ( 'NONE', #43361, #48748, #61950, .T. ) ;
#67117=ORIENTED_EDGE ( 'NONE', *, *, #49762, .F. ) ;
#67118=CARTESIAN_POINT ( 'NONE',  ( -16.02305571287920216, -2.295524264805590686, 30.44142389570982488 ) ) ;
#67119=CARTESIAN_POINT ( 'NONE',  ( 7.146089767170319185, -11.43677907613344757, 33.22367315496201456 ) ) ;
#67121=CYLINDRICAL_SURFACE ( 'NONE', #85849, 0.2499999999999994726 ) ;
#67122=CARTESIAN_POINT ( 'NONE',  ( -1.450697763975519416, -11.35647404775217595, 33.31231777344666511 ) ) ;
#67123=CARTESIAN_POINT ( 'NONE',  ( -10.74607521849492109, -11.93127051446799847, 32.56575433478202797 ) ) ;
#67124=CARTESIAN_POINT ( 'NONE',  ( -6.923076923076922462, -8.973038597847269315, 34.52809138561121927 ) ) ;
#67125=CARTESIAN_POINT ( 'NONE',  ( 12.52679403281448600, -5.219633306516380244, 34.19971097300157936 ) ) ;
#67126=VECTOR ( 'NONE', #73084, 1000.000000000000227 ) ;
#67127=CARTESIAN_POINT ( 'NONE',  ( -12.46153846153858247, -6.879047030192662504, 34.71129190930017927 ) ) ;
#67128=ORIENTED_EDGE ( 'NONE', *, *, #79566, .F. ) ;
#67130=CIRCLE ( 'NONE', #23965, 0.2500000000000002220 ) ;
#67131=VERTEX_POINT ( 'NONE', #21852 ) ;
#67132=CARTESIAN_POINT ( 'NONE',  ( -3.930833309752757021, -8.282913670948747864, 34.94150082978203642 ) ) ;
#67134=LINE ( 'NONE', #4535, #29173 ) ;
#67135=LINE ( 'NONE', #23903, #15152 ) ;
#67136=ORIENTED_EDGE ( 'NONE', *, *, #57838, .F. ) ;
#67137=CARTESIAN_POINT ( 'NONE',  ( 15.36155967173618286, -9.084667340241226796, 34.75534355489798344 ) ) ;
#67138=EDGE_LOOP ( 'NONE', ( #39563, #66415, #64752, #35086 ) ) ;
#67139=CARTESIAN_POINT ( 'NONE',  ( -10.74553182482283198, -3.285722584762969856, 32.44110544564090759 ) ) ;
#67140=ORIENTED_EDGE ( 'NONE', *, *, #70707, .F. ) ;
#67141=CARTESIAN_POINT ( 'NONE',  ( 10.86538461538461675, -7.500000000000001776, 35.04278698407183867 ) ) ;
#67142=CIRCLE ( 'NONE', #32668, 0.2500000000000002220 ) ;
#67143=CARTESIAN_POINT ( 'NONE',  ( 1.449870955891410684, -6.879047030191282275, 34.71129190930002295 ) ) ;
#67144=CARTESIAN_POINT ( 'NONE',  ( 0.3308469948709023556, -4.809359713505814149, 33.96456829005828837 ) ) ;
#67145=B_SPLINE_CURVE_WITH_KNOTS ( 'NONE', 3,
 ( #86364, #37250, #72814, #36818, #3909, #30067, #58402, #30935, #24635, #71482 ),
 .UNSPECIFIED., .F., .F.,
 ( 4, 2, 2, 2, 4 ),
 ( 0.000000000000000000, 0.0001954339857564063089, 0.0003908679715128126177, 0.0005863019572692189808, 0.0007817359430256252354 ),
 .UNSPECIFIED. ) ;
#67146=FACE_BOUND ( 'NONE', #72274, .T. ) ;
#67147=CARTESIAN_POINT ( 'NONE',  ( 2.557692307693744560, -7.500000000000155431, 34.75000000000007105 ) ) ;
#67148=DIRECTION ( 'NONE',  ( -0.000000000000000000, 1.000000000000000000, -0.000000000000000000 ) ) ;
#67149=CARTESIAN_POINT ( 'NONE',  ( 5.777134577796363857, -2.501496062324911840, 29.88072118266895671 ) ) ;
#67150=CARTESIAN_POINT ( 'NONE',  ( -13.38461538461550582, -12.27809138561165270, 31.22303859784587132 ) ) ;
#67151=CARTESIAN_POINT ( 'NONE',  ( 10.36538461538461675, -7.500000000000001776, 34.75000000000000000 ) ) ;
#67152=CARTESIAN_POINT ( 'NONE',  ( 0.4615384615384611200, -13.20930481340135110, 34.54067556320372745 ) ) ;
#67153=ORIENTED_EDGE ( 'NONE', *, *, #36123, .T. ) ;
#67154=VECTOR ( 'NONE', #72973, 1000.000000000000000 ) ;
#67155=CARTESIAN_POINT ( 'NONE',  ( -3.230769230769229949, -1.129524287112498415, 32.06866353760679544 ) ) ;
#67156=EDGE_LOOP ( 'NONE', ( #76869, #79756, #27052, #86879 ) ) ;
#67157=VERTEX_POINT ( 'NONE', #15102 ) ;
#67158=CARTESIAN_POINT ( 'NONE',  ( 5.933917620639864943, -11.91647553114624181, 32.58852847137148245 ) ) ;
#67159=CARTESIAN_POINT ( 'NONE',  ( -5.999999999999998224, -8.318370150425687726, 35.83090037661290239 ) ) ;
#67160=CARTESIAN_POINT ( 'NONE',  ( 2.057692307692309708, -7.500000000000001776, 35.04278698407183867 ) ) ;
#67161=CARTESIAN_POINT ( 'NONE',  ( -14.37377468705243899, -11.91647553114624181, 32.58852847137148245 ) ) ;
#67162=CARTESIAN_POINT ( 'NONE',  ( -17.29985003582992320, -12.38737895849757820, 31.66785238281580206 ) ) ;
#67163=CARTESIAN_POINT ( 'NONE',  ( -13.38461538461550582, -2.892918686052166066, 31.69288490824153470 ) ) ;
#67164=ORIENTED_EDGE ( 'NONE', *, *, #29798, .T. ) ;
#67165=CARTESIAN_POINT ( 'NONE',  ( -8.096153846153844924, -7.500000000000001776, 35.00000000000000000 ) ) ;
#67166=CARTESIAN_POINT ( 'NONE',  ( 15.10062126103753855, -4.299443229763728169, 33.91186481527756058 ) ) ;
#67167=CARTESIAN_POINT ( 'NONE',  ( -14.53117725141625627, -8.496056993536548418, 34.65000542017679663 ) ) ;
#67168=CARTESIAN_POINT ( 'NONE',  ( -6.989159302437059296, -6.343179335718451384, 34.87096338111212646 ) ) ;
#67169=VERTEX_POINT ( 'NONE', #84455 ) ;
#67170=VERTEX_POINT ( 'NONE', #2023 ) ;
#67171=B_SPLINE_CURVE_WITH_KNOTS ( 'NONE', 3,
 ( #7811, #49677, #28528, #15462, #42933, #7374, #69949, #70402, #8704, #34388 ),
 .UNSPECIFIED., .F., .F.,
 ( 4, 2, 2, 2, 4 ),
 ( 0.0007817246256747472808, 0.0009771112852218905021, 0.001172497944769033832, 0.001367884604316177161, 0.001563271263863320274 ),
 .UNSPECIFIED. ) ;
#67173=ORIENTED_EDGE ( 'NONE', *, *, #34013, .F. ) ;
#67174=VECTOR ( 'NONE', #68217, 1000.000000000000114 ) ;
#67177=EDGE_CURVE ( 'NONE', #88629, #84284, #47924, .T. ) ;
#67178=VERTEX_POINT ( 'NONE', #63275 ) ;
#67179=CYLINDRICAL_SURFACE ( 'NONE', #88456, 0.2499999999999998890 ) ;
#67180=CARTESIAN_POINT ( 'NONE',  ( 14.55774672760576394, -5.642605341092957971, 34.66089969410670335 ) ) ;
#67181=CARTESIAN_POINT ( 'NONE',  ( -5.326946314216042033, -4.335965774309649134, 33.62209801155881905 ) ) ;
#67182=CARTESIAN_POINT ( 'NONE',  ( 9.019285189144222059, -3.435999193479609914, 33.07426656108010832 ) ) ;
#67185=ORIENTED_EDGE ( 'NONE', *, *, #21630, .T. ) ;
#67186=CARTESIAN_POINT ( 'NONE',  ( -7.780085495151405794, -9.780366693483667717, 34.19971097300155805 ) ) ;
#67187=ORIENTED_EDGE ( 'NONE', *, *, #61449, .T. ) ;
#67188=CARTESIAN_POINT ( 'NONE',  ( 13.38461538461538680, -3.937682226553329556, 33.60647404775216529 ) ) ;
#67189=CARTESIAN_POINT ( 'NONE',  ( 8.899756207464413649, -12.50538340440932394, 31.33453814440721885 ) ) ;
#67190=DIRECTION ( 'NONE',  ( -0.000000000000000000, -0.5000000000000009992, -0.8660254037844380415 ) ) ;
#67191=B_SPLINE_CURVE_WITH_KNOTS ( 'NONE', 3,
 ( #44449, #3916, #31402, #58870, #86371, #52108, #79598, #77808, #17894, #45351 ),
 .UNSPECIFIED., .F., .F.,
 ( 4, 2, 2, 2, 4 ),
 ( 0.000000000000000000, 0.0001954311564186876876, 0.0003908623128373753751, 0.0005862934692560630356, 0.0007817246256747507503 ),
 .UNSPECIFIED. ) ;
#67192=CARTESIAN_POINT ( 'NONE',  ( 18.00000000000000000, -8.120952969808772792, 34.71129190930000163 ) ) ;
#67193=B_SPLINE_CURVE_WITH_KNOTS ( 'NONE', 3,
 ( #34341, #77436, #122, #22492, #29267, #2644, #84652, #29704, #30137, #57604 ),
 .UNSPECIFIED., .F., .F.,
 ( 4, 2, 2, 2, 4 ),
 ( 0.0007817359430256257775, 0.0009771253907249911191, 0.001172514838424356352, 0.001367904286123721586, 0.001563293733823086819 ),
 .UNSPECIFIED. ) ;
#67194=DIRECTION ( 'NONE',  ( 0.000000000000000000, 0.1736481776669275834, 0.9848077530122086864 ) ) ;
#67195=EDGE_CURVE ( 'NONE', #13888, #87291, #65128, .T. ) ;
#67196=AXIS2_PLACEMENT_3D ( 'NONE', #6054, #7384, #69077 ) ;
#67198=B_SPLINE_CURVE_WITH_KNOTS ( 'NONE', 3,
 ( #37628, #10608, #85381, #2069, #2501, #77285, #37179, #44366, #23226, #31324 ),
 .UNSPECIFIED., .F., .F.,
 ( 4, 2, 2, 2, 4 ),
 ( 0.0007817359430256294638, 0.0009771253907249974075, 0.001172514838424365460, 0.001367904286123733295, 0.001563293733823094191 ),
 .UNSPECIFIED. ) ;
#67199=CARTESIAN_POINT ( 'NONE',  ( -0.7115152055870509473, -2.544273027872575366, 31.48422191005632342 ) ) ;
#67201=ORIENTED_EDGE ( 'NONE', *, *, #57163, .F. ) ;
#67202=CARTESIAN_POINT ( 'NONE',  ( 11.53846153846153832, -2.721908614388771852, 31.22303859784724978 ) ) ;
#67203=CARTESIAN_POINT ( 'NONE',  ( 2.557637717070352590, -4.176053281294514363, 33.81426240980091791 ) ) ;
#67206=CARTESIAN_POINT ( 'NONE',  ( 2.530655441958984397, -7.369474539155830506, 34.99858011523957657 ) ) ;
#67207=CARTESIAN_POINT ( 'NONE',  ( -12.71151519248081740, -3.137211980971221781, 32.19342716148376837 ) ) ;
#67208=CARTESIAN_POINT ( 'NONE',  ( -0.4615384615384611200, -9.058645607665452459, 34.76329471203371924 ) ) ;
#67209=CARTESIAN_POINT ( 'NONE',  ( -9.019207513279360100, -10.82459398097509329, 33.81372124010185587 ) ) ;
#67211=CARTESIAN_POINT ( 'NONE',  ( 0.5267936010512991318, -2.379036618887895305, 30.90682066428159303 ) ) ;
#67212=EDGE_LOOP ( 'NONE', ( #85154, #58908 ) ) ;
#67213=VECTOR ( 'NONE', #76167, 1000.000000000000000 ) ;
#67214=CARTESIAN_POINT ( 'NONE',  ( -3.100243792535588128, -12.70449254468099198, 30.44128974285582956 ) ) ;
#67216=EDGE_CURVE ( 'NONE', #37079, #47404, #82403, .T. ) ;
#67217=CARTESIAN_POINT ( 'NONE',  ( 7.145856592054988354, -6.717445702608402236, 34.94155399931962336 ) ) ;
#67218=CARTESIAN_POINT ( 'NONE',  ( -3.230769230769229949, -11.69971097300155272, 32.46337939537588113 ) ) ;
#67219=VERTEX_POINT ( 'NONE', #50644 ) ;
#67220=CARTESIAN_POINT ( 'NONE',  ( 12.52679403281448423, -3.835265460703683349, 33.15142922261929925 ) ) ;
#67221=AXIS2_PLACEMENT_3D ( 'NONE', #57373, #84868, #78094 ) ;
#67222=ORIENTED_EDGE ( 'NONE', *, *, #10470, .F. ) ;
#67226=VERTEX_POINT ( 'NONE', #22731 ) ;
#67227=CARTESIAN_POINT ( 'NONE',  ( 0.5276068125408992504, -4.098570777380720287, 33.41473453929635440 ) ) ;
#67228=CARTESIAN_POINT ( 'NONE',  ( -6.000000000000121680, -2.379036618888197729, 30.90682066428292885 ) ) ;
#67229=CYLINDRICAL_SURFACE ( 'NONE', #88328, 0.2499999999999997502 ) ;
#67230=B_SPLINE_CURVE_WITH_KNOTS ( 'NONE', 3,
 ( #36083, #55894, #77063, #50458, #50023, #49587, #48690, #29325, #28889, #43275 ),
 .UNSPECIFIED., .F., .F.,
 ( 4, 2, 2, 2, 4 ),
 ( 0.000000000000000000, 0.0001954311564186869557, 0.0003908623128373738030, 0.0005862934692560607588, 0.0007817246256747476061 ),
 .UNSPECIFIED. ) ;
#67231=B_SPLINE_CURVE_WITH_KNOTS ( 'NONE', 3,
 ( #44515, #65679, #57600, #25150, #78309, #45860, #52167, #9858, #31464, #24707 ),
 .UNSPECIFIED., .F., .F.,
 ( 4, 2, 2, 2, 4 ),
 ( 0.000000000000000000, 0.0001954339857564054144, 0.0003908679715128108288, 0.0005863019572692162703, 0.0007817359430256216575 ),
 .UNSPECIFIED. ) ;
#67232=FACE_OUTER_BOUND ( 'NONE', #54707, .T. ) ;
#67233=CARTESIAN_POINT ( 'NONE',  ( -0.5268084620947819374, -11.67786785259541027, 32.92929555188721480 ) ) ;
#67234=B_SPLINE_CURVE_WITH_KNOTS ( 'NONE', 3,
 ( #8093, #68455, #54946, #49520, #35566, #1326, #76993, #13954, #21596, #6752 ),
 .UNSPECIFIED., .F., .F.,
 ( 4, 2, 2, 2, 4 ),
 ( 0.0007817359430256297891, 0.0009771253907249961065, 0.001172514838424362424, 0.001367904286123728741, 0.001563293733823095059 ),
 .UNSPECIFIED. ) ;
#67235=EDGE_LOOP ( 'NONE', ( #18207, #55313, #25141, #33652 ) ) ;
#67236=CARTESIAN_POINT ( 'NONE',  ( -3.903791733932700847, -12.41089969410671223, 31.60739465890703670 ) ) ;
#67239=CARTESIAN_POINT ( 'NONE',  ( -10.39237177129122003, -10.01129605718032600, 34.36064277460058491 ) ) ;
#67240=CARTESIAN_POINT ( 'NONE',  ( -13.60754160213152808, -2.758268499246657068, 31.33685645148948140 ) ) ;
#67242=CARTESIAN_POINT ( 'NONE',  ( 6.250054311638317373, -9.148310452688871663, 34.47095581063188519 ) ) ;
#67244=FACE_OUTER_BOUND ( 'NONE', #70895, .T. ) ;
#67245=ORIENTED_EDGE ( 'NONE', *, *, #72348, .T. ) ;
#67247=ORIENTED_EDGE ( 'NONE', *, *, #59473, .F. ) ;
#67249=CARTESIAN_POINT ( 'NONE',  ( -10.48459280755982626, -11.18335022499818621, 33.13157742990016885 ) ) ;
#67250=CARTESIAN_POINT ( 'NONE',  ( -3.230769230769229949, -6.343179335718451384, 34.87096338111211935 ) ) ;
#67251=CARTESIAN_POINT ( 'NONE',  ( -15.36146069743679021, -10.54014554554150607, 33.71984207302941883 ) ) ;
#67252=DIRECTION ( 'NONE',  ( -0.000000000000000000, 0.9396926207859093161, -0.3420201433256663259 ) ) ;
#67253=CARTESIAN_POINT ( 'NONE',  ( 17.77707378248384629, -9.886141570436013382, 34.14413921362392301 ) ) ;
#67254=CARTESIAN_POINT ( 'NONE',  ( -10.36538461538461320, -2.499999999999998668, 29.75000000000000355 ) ) ;
#67256=CARTESIAN_POINT ( 'NONE',  ( 6.923076923076802558, -12.46129190930018460, 30.37095296980731973 ) ) ;
#67258=EDGE_LOOP ( 'NONE', ( #37892, #79885, #8147, #71204 ) ) ;
#67259=ADVANCED_FACE ( 'NONE', ( #43454 ), #2454, .F. ) ;
#67261=CARTESIAN_POINT ( 'NONE',  ( 2.241608896736426271, -2.538708090699994813, 30.37095296980875148 ) ) ;
#67262=VERTEX_POINT ( 'NONE', #52866 ) ;
#67263=CARTESIAN_POINT ( 'NONE',  ( 16.21991450484859953, -11.69971097300155272, 32.46337939537588113 ) ) ;
#67264=CARTESIAN_POINT ( 'NONE',  ( -7.596099426240392027, -9.233818618650603938, 34.70587769442853698 ) ) ;
#67266=CARTESIAN_POINT ( 'NONE',  ( 12.46153846153833911, -8.656820664282941280, 34.87096338111179961 ) ) ;
#67267=AXIS2_PLACEMENT_3D ( 'NONE', #85212, #65370, #78884 ) ;
#67268=CYLINDRICAL_SURFACE ( 'NONE', #40832, 0.2499999999999995559 ) ;
#67269=FACE_BOUND ( 'NONE', #60451, .T. ) ;
#67270=ORIENTED_EDGE ( 'NONE', *, *, #73799, .F. ) ;
#67271=VERTEX_POINT ( 'NONE', #52423 ) ;
#67272=CARTESIAN_POINT ( 'NONE',  ( -5.010854725920638408, -6.386643153685127139, 34.62446782046654192 ) ) ;
#67275=FACE_BOUND ( 'NONE', #478, .T. ) ;
#67276=CARTESIAN_POINT ( 'NONE',  ( 9.822833130541342328, -5.915461855592780260, 34.75538340440931506 ) ) ;
#67277=EDGE_CURVE ( 'NONE', #43616, #14619, #57655, .T. ) ;
#67278=CARTESIAN_POINT ( 'NONE',  ( -13.63459211555773720, -10.66389620160130036, 33.62221079203477103 ) ) ;
#67279=ORIENTED_EDGE ( 'NONE', *, *, #60056, .T. ) ;
#67280=CARTESIAN_POINT ( 'NONE',  ( -5.749999999999936051, -7.434744429011176159, 34.75000000000000711 ) ) ;
#67281=CARTESIAN_POINT ( 'NONE',  ( -6.700297254098854793, -2.353885683473779800, 30.79025554430704759 ) ) ;
#67282=AXIS2_PLACEMENT_3D ( 'NONE', #17920, #45375, #72849 ) ;
#67284=ORIENTED_EDGE ( 'NONE', *, *, #55863, .F. ) ;
#67285=EDGE_CURVE ( 'NONE', #68032, #10589, #69675, .T. ) ;
#67286=FACE_OUTER_BOUND ( 'NONE', #38547, .T. ) ;
#67287=CARTESIAN_POINT ( 'NONE',  ( 17.99999999999987566, -11.06231777344772027, 33.60647404775119895 ) ) ;
#67288=CARTESIAN_POINT ( 'NONE',  ( 2.530471976670372491, -3.020022701398814124, 32.48759521482552515 ) ) ;
#67289=ORIENTED_EDGE ( 'NONE', *, *, #81140, .T. ) ;
#67290=CARTESIAN_POINT ( 'NONE',  ( 2.373759641042385571, -12.34228464037088813, 31.77849191805839268 ) ) ;
#67291=CYLINDRICAL_SURFACE ( 'NONE', #64308, 0.2500000000000004996 ) ;
#67292=ORIENTED_EDGE ( 'NONE', *, *, #11058, .T. ) ;
#67293=CARTESIAN_POINT ( 'NONE',  ( -12.68502338610279168, -5.827078755546623690, 34.72654668319379567 ) ) ;
#67295=CARTESIAN_POINT ( 'NONE',  ( 0.4615384615384611200, -10.67929555188718282, 33.92786785259544047 ) ) ;
#67296=CARTESIAN_POINT ( 'NONE',  ( -5.011667505647054099, -8.613356846314928816, 34.62446782046653482 ) ) ;
#67297=CARTESIAN_POINT ( 'NONE',  ( 0.2380535369741272611, -2.612411019501190701, 31.66733052389439962 ) ) ;
#67298=CARTESIAN_POINT ( 'NONE',  ( 15.23076923076923173, -2.538708090699994813, 30.37095296980875503 ) ) ;
#67299=CARTESIAN_POINT ( 'NONE',  ( 14.17713171595038446, -2.504760397472875155, 29.97295953869789997 ) ) ;
#67300=CARTESIAN_POINT ( 'NONE',  ( -15.48079246806219267, -12.43535235679832596, 30.55408501211184813 ) ) ;
#67301=EDGE_CURVE ( 'NONE', #3308, #6564, #23190, .T. ) ;
#67302=CARTESIAN_POINT ( 'NONE',  ( -3.230769230769229949, -2.538708090699994813, 30.37095296980875503 ) ) ;
#67303=CARTESIAN_POINT ( 'NONE',  ( -12.46153846153858247, -11.48612834414049644, 32.76840700105863391 ) ) ;
#67306=CARTESIAN_POINT ( 'NONE',  ( -12.46153846153846168, -8.120952969808772792, 34.71129190930000163 ) ) ;
#67307=ORIENTED_EDGE ( 'NONE', *, *, #41617, .F. ) ;
#67308=ORIENTED_EDGE ( 'NONE', *, *, #77542, .T. ) ;
#67309=CARTESIAN_POINT ( 'NONE',  ( -3.007756386675835447, -9.172514111537584114, 34.72667873470787470 ) ) ;
#67310=VERTEX_POINT ( 'NONE', #38480 ) ;
#67313=CARTESIAN_POINT ( 'NONE',  ( 13.44987095589141113, -2.892918686051625166, 31.69288490824026638 ) ) ;
#67314=DIRECTION ( 'NONE',  ( -0.000000000000000000, -0.6427876096865404731, -0.7660444431189770143 ) ) ;
#67315=CARTESIAN_POINT ( 'NONE',  ( 9.692307692307570832, -9.528491918059723176, 34.59228464037033035 ) ) ;
#67316=VECTOR ( 'NONE', #12031, 1000.000000000000227 ) ;
#67317=CARTESIAN_POINT ( 'NONE',  ( -10.48485917715096782, -3.625058011473228703, 33.29252011169590020 ) ) ;
#67318=DIRECTION ( 'NONE',  ( 0.000000000000000000, 0.3420201433256641055, -0.9396926207859100932 ) ) ;
#67319=CARTESIAN_POINT ( 'NONE',  ( 2.241608896736428047, -9.780366693483667717, 34.19971097300155805 ) ) ;
#67321=CARTESIAN_POINT ( 'NONE',  ( 10.61538461538449418, -12.51329471203414379, 31.30864560766407578 ) ) ;
#67322=CARTESIAN_POINT ( 'NONE',  ( -4.219116154402474450, -12.16647553114622049, 32.15551576947930812 ) ) ;
#67323=EDGE_CURVE ( 'NONE', #43106, #21818, #55414, .T. ) ;
#67324=AXIS2_PLACEMENT_3D ( 'NONE', #18253, #74978, #80860 ) ;
#67325=EDGE_CURVE ( 'NONE', #84179, #37632, #21121, .T. ) ;
#67326=CARTESIAN_POINT ( 'NONE',  ( 5.776515075435673552, -3.562934362175799841, 33.22335522853832401 ) ) ;
#67327=B_SPLINE_CURVE_WITH_KNOTS ( 'NONE', 3,
 ( #44106, #71585, #9894, #66165, #59418, #79248, #79695, #17996, #51287, #50859 ),
 .UNSPECIFIED., .F., .F.,
 ( 4, 2, 2, 2, 4 ),
 ( 0.000000000000000000, 0.0001954311564186865763, 0.0003908623128373731525, 0.0005862934692560596746, 0.0007817246256747463051 ),
 .UNSPECIFIED. ) ;
#67328=B_SPLINE_CURVE_WITH_KNOTS ( 'NONE', 3,
 ( #63378, #29178, #57953, #8893, #9338, #65145, #36798, #2556, #16523, #85432 ),
 .UNSPECIFIED., .F., .F.,
 ( 4, 2, 2, 2, 4 ),
 ( 0.0007817359430256313069, 0.0009771253907249971907, 0.001172514838424363291, 0.001367904286123729392, 0.001563293733823095276 ),
 .UNSPECIFIED. ) ;
#67329=ORIENTED_EDGE ( 'NONE', *, *, #76632, .F. ) ;
#67330=VERTEX_POINT ( 'NONE', #58288 ) ;
#67331=ADVANCED_FACE ( 'NONE', ( #25854 ), #80813, .F. ) ;
#67332=CARTESIAN_POINT ( 'NONE',  ( 14.30769230769218581, -8.656820664282941280, 34.87096338111179961 ) ) ;
#67333=CARTESIAN_POINT ( 'NONE',  ( 15.23076923076923173, -11.91647553114624181, 32.58852847137148245 ) ) ;
#67334=FACE_OUTER_BOUND ( 'NONE', #19245, .T. ) ;
#67335=CARTESIAN_POINT ( 'NONE',  ( -6.222926217516147496, -3.586966769969700763, 32.86292498521069660 ) ) ;
#67336=ADVANCED_FACE ( 'NONE', ( #72251 ), #10561, .F. ) ;
#67337=CARTESIAN_POINT ( 'NONE',  ( -9.692307692307812417, -4.481592998941358097, 33.73612834414048933 ) ) ;
#67338=DIRECTION ( 'NONE',  ( 0.000000000000000000, 0.9396926207859126468, 0.3420201433256571111 ) ) ;
#67340=CARTESIAN_POINT ( 'NONE',  ( 1.161689167099238418, -4.887634598454295265, 34.01352882383564946 ) ) ;
#67341=VERTEX_POINT ( 'NONE', #51972 ) ;
#67342=ORIENTED_EDGE ( 'NONE', *, *, #9072, .F. ) ;
#67343=CARTESIAN_POINT ( 'NONE',  ( 17.74997676270703550, -3.202444869320336451, 32.30641848906366675 ) ) ;
#67344=CARTESIAN_POINT ( 'NONE',  ( 4.087762742890270751, -2.538708090699994813, 30.37095296980875148 ) ) ;
#67345=CARTESIAN_POINT ( 'NONE',  ( 11.53846153846153832, -10.51840700105979565, 33.73612834413961536 ) ) ;
#67346=VECTOR ( 'NONE', #43951, 1000.000000000000000 ) ;
#67348=CYLINDRICAL_SURFACE ( 'NONE', #85345, 0.2499999999999993616 ) ;
#67349=ORIENTED_EDGE ( 'NONE', *, *, #24867, .T. ) ;
#67350=VERTEX_POINT ( 'NONE', #75371 ) ;
#67351=EDGE_CURVE ( 'NONE', #48154, #19870, #45683, .T. ) ;
#67352=ORIENTED_EDGE ( 'NONE', *, *, #70116, .F. ) ;
#67353=VERTEX_POINT ( 'NONE', #55090 ) ;
#67354=CARTESIAN_POINT ( 'NONE',  ( 17.29970274590113632, -10.23759521482555357, 34.22997729860117033 ) ) ;
#67355=CARTESIAN_POINT ( 'NONE',  ( 10.36536139116315880, -11.56360843649121861, 33.07473185843129926 ) ) ;
#67356=CARTESIAN_POINT ( 'NONE',  ( 4.219101293358989757, -3.643525952247864463, 33.31231777344670064 ) ) ;
#67357=CARTESIAN_POINT ( 'NONE',  ( 2.057715576749955311, -11.28823185664190376, 33.01397839955799896 ) ) ;
#67358=DIRECTION ( 'NONE',  ( -0.000000000000000000, -0.9848077530122086864, -0.1736481776669273613 ) ) ;
#67359=CARTESIAN_POINT ( 'NONE',  ( -4.153846153846152411, -10.51840700105979565, 33.73612834413961536 ) ) ;
#67360=VERTEX_POINT ( 'NONE', #13228 ) ;
#67361=EDGE_CURVE ( 'NONE', #24082, #25133, #48859, .T. ) ;
#67362=ORIENTED_EDGE ( 'NONE', *, *, #12444, .F. ) ;
#67364=CARTESIAN_POINT ( 'NONE',  ( -3.480745974817819555, -2.544273027872574922, 31.48422191005632342 ) ) ;
#67365=EDGE_LOOP ( 'NONE', ( #54041, #74839 ) ) ;
#67366=CARTESIAN_POINT ( 'NONE',  ( -9.757578138268467427, -5.219633306516282545, 34.19971097300152962 ) ) ;
#67367=CYLINDRICAL_SURFACE ( 'NONE', #73418, 0.2499999999999997502 ) ;
#67369=EDGE_LOOP ( 'NONE', ( #41226, #68342, #6223, #32645 ) ) ;
#67371=CARTESIAN_POINT ( 'NONE',  ( -3.230769230769351186, -12.46129190930018460, 30.37095296980731973 ) ) ;
#67372=ORIENTED_EDGE ( 'NONE', *, *, #51343, .T. ) ;
#67373=CARTESIAN_POINT ( 'NONE',  ( 8.096099364501988305, -12.22109172314383230, 31.39792113162168263 ) ) ;
#67374=CARTESIAN_POINT ( 'NONE',  ( 17.14217821643591932, -12.16647553114626490, 32.15551576947920864 ) ) ;
#67375=CARTESIAN_POINT ( 'NONE',  ( -12.39628289026243557, -12.46129190930001052, 30.37095296980870174 ) ) ;
#67376=CARTESIAN_POINT ( 'NONE',  ( -7.146561866800873020, -3.754499324213721234, 33.06261337010820256 ) ) ;
#67377=EDGE_CURVE ( 'NONE', #52302, #70228, #28457, .T. ) ;
#67378=DIRECTION ( 'NONE',  ( -0.000000000000000000, 1.000000000000000000, -0.000000000000000000 ) ) ;
#67379=EDGE_LOOP ( 'NONE', ( #54847, #52868 ) ) ;
#67380=FACE_OUTER_BOUND ( 'NONE', #37027, .T. ) ;
#67381=EDGE_CURVE ( 'NONE', #42328, #72479, #68169, .T. ) ;
#67382=DIRECTION ( 'NONE',  ( 1.000000000000000000, 0.000000000000000000, 0.000000000000000000 ) ) ;
#67383=ORIENTED_EDGE ( 'NONE', *, *, #45022, .T. ) ;
#67384=FACE_OUTER_BOUND ( 'NONE', #4718, .T. ) ;
#67385=CARTESIAN_POINT ( 'NONE',  ( -7.623142494540996239, -11.24521262558773493, 33.06293181088029343 ) ) ;
#67386=CARTESIAN_POINT ( 'NONE',  ( 17.07692307692295586, -10.21337939537710326, 33.94971097300076224 ) ) ;
#67387=LINE ( 'NONE', #20087, #32838 ) ;
#67388=CARTESIAN_POINT ( 'NONE',  ( -0.3963926822064974820, -7.750023238201980469, 34.74374492549440419 ) ) ;
#67389=FACE_BOUND ( 'NONE', #30276, .T. ) ;
#67390=CARTESIAN_POINT ( 'NONE',  ( 5.934729999443681514, -5.094484230520674117, 34.41647553114621161 ) ) ;
#67391=CARTESIAN_POINT ( 'NONE',  ( 4.153846153846154188, -12.62096338111211580, 30.90682066428153263 ) ) ;
#67392=EDGE_CURVE ( 'NONE', #41347, #76970, #53164, .T. ) ;
#67393=CARTESIAN_POINT ( 'NONE',  ( -9.561517251340744039, -11.93129842949671726, 32.56571108434900452 ) ) ;
#67395=DIRECTION ( 'NONE',  ( -0.000000000000000000, -0.9848077530122085754, -0.1736481776669273613 ) ) ;
#67396=CARTESIAN_POINT ( 'NONE',  ( 15.23076923076911093, -11.94971097300221174, 32.03036669348237098 ) ) ;
#67397=AXIS2_PLACEMENT_3D ( 'NONE', #26405, #5243, #88573 ) ;
#67400=CARTESIAN_POINT ( 'NONE',  ( -7.146003140593069958, -9.086856451489516928, 34.49173150075333183 ) ) ;
#67401=ORIENTED_EDGE ( 'NONE', *, *, #5641, .T. ) ;
#67402=CARTESIAN_POINT ( 'NONE',  ( 0.3308469948709031883, -6.413092428213692742, 34.63065189839063152 ) ) ;
#67403=ORIENTED_EDGE ( 'NONE', *, *, #28940, .T. ) ;
#67404=CARTESIAN_POINT ( 'NONE',  ( 7.780883400193070898, -9.442884908240170461, 34.35708131394840592 ) ) ;
#67405=DIRECTION ( 'NONE',  ( -0.000000000000000000, -0.9396926207859092051, -0.3420201433256662704 ) ) ;
#67406=EDGE_CURVE ( 'NONE', #763, #72305, #48329, .T. ) ;
#67407=CARTESIAN_POINT ( 'NONE',  ( -5.011667937410237528, -9.528491918058460186, 34.59228464037085615 ) ) ;
#67408=ORIENTED_EDGE ( 'NONE', *, *, #75753, .F. ) ;
#67409=CARTESIAN_POINT ( 'NONE',  ( -10.61538461538473577, -12.16647553114689728, 32.15551576947799362 ) ) ;
#67410=CARTESIAN_POINT ( 'NONE',  ( 1.134638640566796086, -12.01397095200673881, 32.43157075238190146 ) ) ;
#67412=CARTESIAN_POINT ( 'NONE',  ( 8.769230769230647482, -5.219633306517616589, 34.19971097300220464 ) ) ;
#67414=CARTESIAN_POINT ( 'NONE',  ( 7.911409417429869251, -11.94971097300157403, 32.03036669348361443 ) ) ;
#67416=CARTESIAN_POINT ( 'NONE',  ( -16.15384615384615330, -2.499999999999998668, 29.75000000000001421 ) ) ;
#67417=CARTESIAN_POINT ( 'NONE',  ( -8.992715712954719720, -9.331801661448606566, 34.40259984581193464 ) ) ;
#67419=CARTESIAN_POINT ( 'NONE',  ( 14.30769230769231015, -9.905515769479276145, 34.41647553114623292 ) ) ;
#67420=EDGE_CURVE ( 'NONE', #11924, #72078, #41142, .T. ) ;
#67421=CARTESIAN_POINT ( 'NONE',  ( 17.07692307692295586, -8.656820664282941280, 34.87096338111179961 ) ) ;
#67422=ORIENTED_EDGE ( 'NONE', *, *, #11963, .F. ) ;
#67423=CARTESIAN_POINT ( 'NONE',  ( 16.28463659481310444, -4.684288915650984819, 34.18129842949671371 ) ) ;
#67424=DIRECTION ( 'NONE',  ( -0.000000000000000000, 0.5000000000000011102, -0.8660254037844381525 ) ) ;
#67426=EDGE_CURVE ( 'NONE', #72305, #35045, #11220, .T. ) ;
#67427=CARTESIAN_POINT ( 'NONE',  ( -15.90390074446811042, -12.45601412856602686, 31.48342859153981621 ) ) ;
#67428=AXIS2_PLACEMENT_3D ( 'NONE', #58317, #38058, #18239 ) ;
#67429=CARTESIAN_POINT ( 'NONE',  ( -16.40382289789473802, -10.82459398097509684, 33.81372124010185587 ) ) ;
#67430=ORIENTED_EDGE ( 'NONE', *, *, #60861, .T. ) ;
#67431=CARTESIAN_POINT ( 'NONE',  ( 7.846153846153846700, -4.786620604624113540, 33.94971097300155094 ) ) ;
#67432=CARTESIAN_POINT ( 'NONE',  ( 18.00000000000000000, -4.945431358278436385, 36.03766855953609394 ) ) ;
#67433=CARTESIAN_POINT ( 'NONE',  ( 8.096208266067300485, -2.544122305571458131, 31.48381861865057729 ) ) ;
#67434=VERTEX_POINT ( 'NONE', #50540 ) ;
#67435=CARTESIAN_POINT ( 'NONE',  ( 12.46153846153846168, -12.37446782046654192, 30.86335684631486131 ) ) ;
#67436=EDGE_CURVE ( 'NONE', #37313, #19392, #32764, .T. ) ;
#67437=CARTESIAN_POINT ( 'NONE',  ( 4.826923076923076650, -7.433932668274256805, 35.00000000000000711 ) ) ;
#67438=CIRCLE ( 'NONE', #34317, 0.2500000000000002220 ) ;
#67439=CARTESIAN_POINT ( 'NONE',  ( -11.60373153901786125, -2.657715359629089225, 31.77849191805832874 ) ) ;
#67440=VERTEX_POINT ( 'NONE', #23082 ) ;
#67442=CARTESIAN_POINT ( 'NONE',  ( -1.384615384615383471, -2.708943851104267164, 35.45975837776705220 ) ) ;
#67443=CARTESIAN_POINT ( 'NONE',  ( 6.673100192134568509, -4.943428324936578910, 34.04746400365624481 ) ) ;
#67444=AXIS2_PLACEMENT_3D ( 'NONE', #37581, #2895, #23624 ) ;
#67445=CARTESIAN_POINT ( 'NONE',  ( -13.25382494364843389, -8.191423895709840863, 34.95447573519442130 ) ) ;
#67447=VERTEX_POINT ( 'NONE', #64057 ) ;
#67448=EDGE_CURVE ( 'NONE', #52128, #50940, #1922, .T. ) ;
#67449=ORIENTED_EDGE ( 'NONE', *, *, #49188, .F. ) ;
#67450=CYLINDRICAL_SURFACE ( 'NONE', #78639, 0.2499999999999997502 ) ;
#67451=CARTESIAN_POINT ( 'NONE',  ( 0.3954550505825790707, -2.538708090699994813, 30.37095296980875148 ) ) ;
#67453=CARTESIAN_POINT ( 'NONE',  ( -13.13456096470193302, -12.01375889529407281, 32.43194544308182969 ) ) ;
#67454=CARTESIAN_POINT ( 'NONE',  ( -7.846153846153844924, -10.67929555188718282, 33.92786785259544047 ) ) ;
#67455=CARTESIAN_POINT ( 'NONE',  ( -7.846153846153844924, -12.48256725967547354, 35.29906147534542527 ) ) ;
#67456=ORIENTED_EDGE ( 'NONE', *, *, #45524, .F. ) ;
#67457=EDGE_CURVE ( 'NONE', #81768, #26583, #76787, .T. ) ;
#67459=ORIENTED_EDGE ( 'NONE', *, *, #14517, .F. ) ;
#67460=LINE ( 'NONE', #61131, #57334 ) ;
#67461=ORIENTED_EDGE ( 'NONE', *, *, #63331, .F. ) ;
#67462=B_SPLINE_CURVE_WITH_KNOTS ( 'NONE', 3,
 ( #7457, #26839, #690, #69153, #41243, #28158, #6567, #81349, #34031, #20518 ),
 .UNSPECIFIED., .F., .F.,
 ( 4, 2, 2, 2, 4 ),
 ( 0.0007817246256747483650, 0.0009771112852218926705, 0.001172497944769037084, 0.001367884604316181498, 0.001563271263863325695 ),
 .UNSPECIFIED. ) ;
#67463=CYLINDRICAL_SURFACE ( 'NONE', #70382, 0.2499999999999995559 ) ;
#67464=VECTOR ( 'NONE', #82146, 1000.000000000000000 ) ;
#67465=EDGE_CURVE ( 'NONE', #88230, #18284, #61782, .T. ) ;
#67466=DIRECTION ( 'NONE',  ( -0.000000000000000000, 0.6427876096865404731, -0.7660444431189770143 ) ) ;
#67468=DIRECTION ( 'NONE',  ( 0.000000000000000000, 0.3420201433256641055, -0.9396926207859100932 ) ) ;
#67469=CARTESIAN_POINT ( 'NONE',  ( -5.869474298236435850, -4.459921816937789885, 33.71989282347011851 ) ) ;
#67470=ORIENTED_EDGE ( 'NONE', *, *, #89173, .F. ) ;
#67471=B_SPLINE_CURVE_WITH_KNOTS ( 'NONE', 3,
 ( #66973, #73743, #25090, #51196, #5268, #30945, #58412, #38608, #58871, #59317 ),
 .UNSPECIFIED., .F., .F.,
 ( 4, 2, 2, 2, 4 ),
 ( 0.000000000000000000, 0.0001954311564186865763, 0.0003908623128373731525, 0.0005862934692560596746, 0.0007817246256747463051 ),
 .UNSPECIFIED. ) ;
#67472=ORIENTED_EDGE ( 'NONE', *, *, #1243, .F. ) ;
#67473=EDGE_CURVE ( 'NONE', #40783, #14918, #8693, .T. ) ;
#67474=ORIENTED_EDGE ( 'NONE', *, *, #19312, .F. ) ;
#67475=CARTESIAN_POINT ( 'NONE',  ( -7.846153846153844924, -3.937682226553329556, 33.60647404775216529 ) ) ;
#67476=DIRECTION ( 'NONE',  ( -0.000000000000000000, 0.5000000000000011102, -0.8660254037844381525 ) ) ;
#67478=CARTESIAN_POINT ( 'NONE',  ( 4.153846153846154188, -4.786620604624113540, 33.94971097300155094 ) ) ;
#67480=ORIENTED_EDGE ( 'NONE', *, *, #19763, .T. ) ;
#67481=CARTESIAN_POINT ( 'NONE',  ( -11.31568186948346622, -4.226511098958373402, 33.85474049983370293 ) ) ;
#67482=CARTESIAN_POINT ( 'NONE',  ( 16.15384615384615330, -3.513871655860378418, 32.76840700105978499 ) ) ;
#67483=CARTESIAN_POINT ( 'NONE',  ( -0.4615384615385826339, -11.48612834414049644, 32.76840700105863391 ) ) ;
#67484=FACE_BOUND ( 'NONE', #88241, .T. ) ;
#67485=CARTESIAN_POINT ( 'NONE',  ( -15.36091720050093024, -8.630895178749533159, 34.87696386517710323 ) ) ;
#67486=CYLINDRICAL_SURFACE ( 'NONE', #37040, 0.2499999999999979738 ) ;
#67487=CARTESIAN_POINT ( 'NONE',  ( -8.899922235898328537, -4.118384482072085184, 33.43331474514187107 ) ) ;
#67488=CARTESIAN_POINT ( 'NONE',  ( -7.053687282701448069, -7.722926236386453702, 34.74524107206102030 ) ) ;
#67489=VECTOR ( 'NONE', #185, 1000.000000000000000 ) ;
#67490=CARTESIAN_POINT ( 'NONE',  ( 15.45378207486262667, -10.01129605718032600, 34.36064277460058491 ) ) ;
#67491=CARTESIAN_POINT ( 'NONE',  ( -4.284321338921872169, -7.276987145209185215, 34.99546412871779211 ) ) ;
#67492=CARTESIAN_POINT ( 'NONE',  ( 5.076923076923075762, -11.69971097300155272, 32.46337939537588113 ) ) ;
#67493=VERTEX_POINT ( 'NONE', #57307 ) ;
#67494=CARTESIAN_POINT ( 'NONE',  ( -14.98071481085577972, -11.47946981652013498, 33.17500667209847620 ) ) ;
#67495=CARTESIAN_POINT ( 'NONE',  ( 12.68455130563185662, -3.395485233115139057, 33.02377354290275946 ) ) ;
#67497=EDGE_CURVE ( 'NONE', #69896, #28781, #12351, .T. ) ;
#67498=ORIENTED_EDGE ( 'NONE', *, *, #63055, .T. ) ;
#67500=CARTESIAN_POINT ( 'NONE',  ( 0.7114838709165038910, -8.476813868363244353, 34.90874843262270133 ) ) ;
#67501=CARTESIAN_POINT ( 'NONE',  ( -13.63459212866397685, -4.818429247618089661, 34.26397095200675125 ) ) ;
#67502=CARTESIAN_POINT ( 'NONE',  ( -11.78848476268299628, -10.18141759479407327, 34.26406193332782379 ) ) ;
#67504=CARTESIAN_POINT ( 'NONE',  ( -9.942284436356281674, -9.234221910056348293, 34.70572697212741531 ) ) ;
#67505=CARTESIAN_POINT ( 'NONE',  ( -4.153846153846152411, -9.058645607665452459, 34.76329471203371924 ) ) ;
#67506=FACE_BOUND ( 'NONE', #53780, .T. ) ;
#67507=CARTESIAN_POINT ( 'NONE',  ( -15.36146069743679199, -5.582088688514999397, 34.36776431015576350 ) ) ;
#67509=DIRECTION ( 'NONE',  ( 0.000000000000000000, 1.000000000000000000, 0.000000000000000000 ) ) ;
#67510=CARTESIAN_POINT ( 'NONE',  ( 2.438218009455872082, -5.195472089885680766, 34.18748526763464923 ) ) ;
#67512=CARTESIAN_POINT ( 'NONE',  ( -10.36533019547115941, -11.47946981652013498, 33.17500667209847620 ) ) ;
#67514=VERTEX_POINT ( 'NONE', #55976 ) ;
#67515=VERTEX_POINT ( 'NONE', #69493 ) ;
#67516=CARTESIAN_POINT ( 'NONE',  ( -15.23076923076922995, -13.88283147151868846, 33.14645433367849847 ) ) ;
#67517=CARTESIAN_POINT ( 'NONE',  ( 12.21153846153846168, -7.433931650972300353, 34.75000000000000711 ) ) ;
#67518=CARTESIAN_POINT ( 'NONE',  ( 4.153846153846030731, -10.33852847137269571, 34.16647553114546554 ) ) ;
#67519=LINE ( 'NONE', #81928, #13620 ) ;
#67520=CARTESIAN_POINT ( 'NONE',  ( -9.692307692307691624, -2.249999999999998668, 29.50000000000001421 ) ) ;
#67522=CARTESIAN_POINT ( 'NONE',  ( -9.019207513279361876, -10.06842814019191401, 34.32929386961144758 ) ) ;
#67523=CARTESIAN_POINT ( 'NONE',  ( -5.999999999999998224, -8.164416787775445883, 34.95778746994557906 ) ) ;
#67524=DIRECTION ( 'NONE',  ( -0.000000000000000000, 0.8660254037844399289, -0.4999999999999980016 ) ) ;
#67525=CARTESIAN_POINT ( 'NONE',  ( 13.31934538405906743, -10.33852847137145048, 34.16647553114627556 ) ) ;
#67526=LINE ( 'NONE', #4941, #22421 ) ;
#67528=CARTESIAN_POINT ( 'NONE',  ( 9.692307692307695177, -3.937682226553329556, 33.60647404775216529 ) ) ;
#67529=B_SPLINE_CURVE_WITH_KNOTS ( 'NONE', 3,
 ( #35554, #21138, #71092, #48608, #8081, #9402 ),
 .UNSPECIFIED., .F., .F.,
 ( 4, 2, 4 ),
 ( 0.0003909569690057776653, 0.0005862646681846002839, 0.0007815723673634227941 ),
 .UNSPECIFIED. ) ;
#67530=FACE_OUTER_BOUND ( 'NONE', #10897, .T. ) ;
#67531=DIRECTION ( 'NONE',  ( -0.000000000000000000, -0.000000000000000000, -1.000000000000000000 ) ) ;
#67532=VERTEX_POINT ( 'NONE', #76699 ) ;
#67533=VECTOR ( 'NONE', #12342, 1000.000000000000227 ) ;
#67534=CARTESIAN_POINT ( 'NONE',  ( -4.854143535654665165, -11.89424750095246175, 32.13594075562311758 ) ) ;
#67535=FACE_OUTER_BOUND ( 'NONE', #87514, .T. ) ;
#67537=ADVANCED_FACE ( 'NONE', ( #35722 ), #63171, .F. ) ;
#67538=CARTESIAN_POINT ( 'NONE',  ( 13.44987095589141113, -5.219633306516380244, 34.19971097300157936 ) ) ;
#67539=DIRECTION ( 'NONE',  ( -0.000000000000000000, -0.1736481776669307198, -0.9848077530122080203 ) ) ;
#67540=CARTESIAN_POINT ( 'NONE',  ( 4.153846153846154188, -1.466349020453238561, 30.81389545987213907 ) ) ;
#67541=CARTESIAN_POINT ( 'NONE',  ( 10.86538461538468070, -7.434744860731433924, 35.00000000000000711 ) ) ;
#67542=EDGE_LOOP ( 'NONE', ( #65961, #76691, #35189, #54177 ) ) ;
#67544=CARTESIAN_POINT ( 'NONE',  ( -14.55771553191376633, -5.765609946408404518, 34.70566812827425451 ) ) ;
#67545=EDGE_CURVE ( 'NONE', #13172, #36624, #17778, .T. ) ;
#67546=ORIENTED_EDGE ( 'NONE', *, *, #71450, .T. ) ;
#67547=CYLINDRICAL_SURFACE ( 'NONE', #39144, 0.2500000000000009437 ) ;
#67548=DIRECTION ( 'NONE',  ( -0.000000000000000000, 0.9848077530122085754, -0.1736481776669273613 ) ) ;
#67550=B_SPLINE_CURVE_WITH_KNOTS ( 'NONE', 3,
 ( #84807, #78026, #43358, #23085, #56863, #83918, #70840, #8696, #9141, #64488 ),
 .UNSPECIFIED., .F., .F.,
 ( 4, 2, 2, 2, 4 ),
 ( 0.000000000000000000, 0.0001954311564186860613, 0.0003908623128373721225, 0.0005862934692560581567, 0.0007817246256747442451 ),
 .UNSPECIFIED. ) ;
#67551=ORIENTED_EDGE ( 'NONE', *, *, #65277, .F. ) ;
#67552=FACE_OUTER_BOUND ( 'NONE', #82951, .T. ) ;
#67553=CARTESIAN_POINT ( 'NONE',  ( 8.769230769230768274, -6.343179335718451384, 34.87096338111211935 ) ) ;
#67554=CYLINDRICAL_SURFACE ( 'NONE', #24000, 0.2499999999999997502 ) ;
#67555=EDGE_LOOP ( 'NONE', ( #70985, #3507, #1236, #8988 ) ) ;
#67556=VERTEX_POINT ( 'NONE', #17203 ) ;
#67557=AXIS2_PLACEMENT_3D ( 'NONE', #31529, #4501, #78821 ) ;
#67558=EDGE_CURVE ( 'NONE', #82155, #10320, #58586, .T. ) ;
#67559=ORIENTED_EDGE ( 'NONE', *, *, #85554, .T. ) ;
#67560=VECTOR ( 'NONE', #10445, 1000.000000000000114 ) ;
#67561=AXIS2_PLACEMENT_3D ( 'NONE', #18173, #45637, #73113 ) ;
#67562=CARTESIAN_POINT ( 'NONE',  ( 13.38461538461538680, -11.69971097300155272, 32.46337939537588113 ) ) ;
#67563=CARTESIAN_POINT ( 'NONE',  ( 7.173131342990377135, -11.47946981652013498, 33.17500667209846910 ) ) ;
#67564=CARTESIAN_POINT ( 'NONE',  ( -18.00000000000000000, -11.10434399251292881, 35.99290692298802696 ) ) ;
#67565=CARTESIAN_POINT ( 'NONE',  ( 9.442330948259103351, -9.234221910056348293, 34.70572697212741531 ) ) ;
#67566=CYLINDRICAL_SURFACE ( 'NONE', #34729, 0.2500000000000002220 ) ;
#67567=CARTESIAN_POINT ( 'NONE',  ( -3.099978789802282364, -4.684288915650983043, 34.18129842949671371 ) ) ;
#67568=CARTESIAN_POINT ( 'NONE',  ( 0.2115617174898694330, -2.318417181685854533, 30.59732222474233865 ) ) ;
#67569=AXIS2_PLACEMENT_3D ( 'NONE', #63849, #10245, #10686 ) ;
#67570=DIRECTION ( 'NONE',  ( -0.000000000000000000, -0.000000000000000000, -1.000000000000000000 ) ) ;
#67571=EDGE_LOOP ( 'NONE', ( #14897, #64673, #84089, #49155 ) ) ;
#67572=ORIENTED_EDGE ( 'NONE', *, *, #80404, .F. ) ;
#67573=EDGE_LOOP ( 'NONE', ( #3869, #51504, #10852, #24634 ) ) ;
#67575=VERTEX_POINT ( 'NONE', #10001 ) ;
#67576=EDGE_CURVE ( 'NONE', #12730, #64872, #3718, .T. ) ;
#67577=CARTESIAN_POINT ( 'NONE',  ( -15.23076923076922995, -13.75783147151868846, 33.36296068462461051 ) ) ;
#67578=CARTESIAN_POINT ( 'NONE',  ( 16.15384615384615330, -2.833524468853757305, 32.15551576947925838 ) ) ;
#67579=ORIENTED_EDGE ( 'NONE', *, *, #55524, .T. ) ;
#67580=CARTESIAN_POINT ( 'NONE',  ( 14.43821774592595197, -12.15418822224088657, 32.17964115625579069 ) ) ;
#67581=ADVANCED_FACE ( 'NONE', ( #78456 ), #4127, .F. ) ;
#67582=ORIENTED_EDGE ( 'NONE', *, *, #77646, .F. ) ;
#67583=CARTESIAN_POINT ( 'NONE',  ( 11.53846153846153832, -2.538708090699994813, 30.37095296980875503 ) ) ;
#67584=ORIENTED_EDGE ( 'NONE', *, *, #26398, .F. ) ;
#67585=CARTESIAN_POINT ( 'NONE',  ( -18.06527000055631405, -9.528491918058357157, 34.59228464037090589 ) ) ;
#67586=EDGE_CURVE ( 'NONE', #61570, #61361, #4858, .T. ) ;
#67587=EDGE_CURVE ( 'NONE', #1344, #67131, #86536, .T. ) ;
#67588=CARTESIAN_POINT ( 'NONE',  ( -6.923076923077045919, -5.094484230521993062, 34.41647553114689373 ) ) ;
#67589=CARTESIAN_POINT ( 'NONE',  ( 12.39545608217832218, -2.292212530054419606, 30.41441678777542634 ) ) ;
#67590=FACE_BOUND ( 'NONE', #52500, .T. ) ;
#67591=CARTESIAN_POINT ( 'NONE',  ( -14.43838291080261627, -9.084618155246140248, 34.75535874321725771 ) ) ;
#67593=CARTESIAN_POINT ( 'NONE',  ( -15.23076923076922995, -10.51840700105979565, 33.73612834413961536 ) ) ;
#67594=B_SPLINE_CURVE_WITH_KNOTS ( 'NONE', 3,
 ( #75942, #76839, #14241, #8378, #41719, #83149 ),
 .UNSPECIFIED., .F., .F.,
 ( 4, 2, 4 ),
 ( 0.0003909512603273914300, 0.0005862562993132194519, 0.0007815613382990475822 ),
 .UNSPECIFIED. ) ;
#67598=CARTESIAN_POINT ( 'NONE',  ( -0.4615384615384611200, -2.708943851104267164, 35.45975837776705220 ) ) ;
#67599=ORIENTED_EDGE ( 'NONE', *, *, #28940, .F. ) ;
#67600=ADVANCED_FACE ( 'NONE', ( #25748 ), #40162, .F. ) ;
#67601=VERTEX_POINT ( 'NONE', #19873 ) ;
#67602=CARTESIAN_POINT ( 'NONE',  ( 12.46153846153846168, -13.04860791097971706, 34.73218667398347037 ) ) ;
#67603=CYLINDRICAL_SURFACE ( 'NONE', #17492, 0.2500000000000008882 ) ;
#67604=CARTESIAN_POINT ( 'NONE',  ( 15.29683656411930848, -8.164416787775445883, 34.95778746994558617 ) ) ;
#67605=CARTESIAN_POINT ( 'NONE',  ( 3.296837581771668635, -10.51840700105979565, 33.73612834413962247 ) ) ;
#67607=CARTESIAN_POINT ( 'NONE',  ( -17.20761368003338632, -12.35290016733513951, 31.75349464988449455 ) ) ;
#67609=EDGE_CURVE ( 'NONE', #47795, #18497, #9170, .T. ) ;
#67611=CARTESIAN_POINT ( 'NONE',  ( -5.326946301144534601, -5.765609946408404518, 34.70566812827425451 ) ) ;
#67613=CARTESIAN_POINT ( 'NONE',  ( -8.992715712954719720, -12.24155766932282496, 31.33739205006857986 ) ) ;
#67614=AXIS2_PLACEMENT_3D ( 'NONE', #42923, #20862, #62723 ) ;
#67615=CARTESIAN_POINT ( 'NONE',  ( -0.4615384615384611200, -5.180354513474913603, 36.12317359536750416 ) ) ;
#67616=ORIENTED_EDGE ( 'NONE', *, *, #10532, .F. ) ;
#67617=ADVANCED_FACE ( 'NONE', ( #39719 ), #19432, .F. ) ;
#67620=ORIENTED_EDGE ( 'NONE', *, *, #50952, .T. ) ;
#67621=CARTESIAN_POINT ( 'NONE',  ( 0.5277076025011177007, -7.250054483168842268, 34.74374881642865631 ) ) ;
#67622=EDGE_LOOP ( 'NONE', ( #88233, #16507, #72540, #72720 ) ) ;
#67623=CARTESIAN_POINT ( 'NONE',  ( -16.15384615384615330, -4.786620604624113540, 33.94971097300155094 ) ) ;
#67624=CARTESIAN_POINT ( 'NONE',  ( -5.142193522883851564, -2.892918686051582089, 31.69288490824015270 ) ) ;
#67625=CARTESIAN_POINT ( 'NONE',  ( 3.230769230769231726, -5.471508081941601098, 34.59228464037088457 ) ) ;
#67626=CARTESIAN_POINT ( 'NONE',  ( -2.307692307692427391, -8.613356846316285953, 34.62446782046622218 ) ) ;
#67627=VECTOR ( 'NONE', #79273, 1000.000000000000227 ) ;
#67628=VECTOR ( 'NONE', #14876, 1000.000000000000000 ) ;
#67629=CYLINDRICAL_SURFACE ( 'NONE', #51739, 0.2500000000000008882 ) ;
#67630=ORIENTED_EDGE ( 'NONE', *, *, #29071, .T. ) ;
#67632=CARTESIAN_POINT ( 'NONE',  ( -0.3307480205715130350, -11.93129842949671726, 32.56571108434900452 ) ) ;
#67633=ORIENTED_EDGE ( 'NONE', *, *, #67891, .T. ) ;
#67634=CARTESIAN_POINT ( 'NONE',  ( -5.207613680033385428, -2.295517848115769421, 30.44137282052136939 ) ) ;
#67635=CARTESIAN_POINT ( 'NONE',  ( 9.019285189144222059, -12.41089969410671223, 31.60739465890703670 ) ) ;
#67636=CARTESIAN_POINT ( 'NONE',  ( -11.60454391782167249, -10.67929555188718460, 33.92786785259543336 ) ) ;
#67637=CARTESIAN_POINT ( 'NONE',  ( -16.02379871859570670, -7.723484941389743952, 34.99544897038808955 ) ) ;
#67638=CARTESIAN_POINT ( 'NONE',  ( 13.38461538461526423, -4.320704448113951379, 33.92786785259630022 ) ) ;
#67639=CARTESIAN_POINT ( 'NONE',  ( -5.326899820971668476, -10.82459398097509684, 33.81372124010185587 ) ) ;
#67640=CARTESIAN_POINT ( 'NONE',  ( -0.4615384615384611200, -2.486705287966279876, 31.30864560766543647 ) ) ;
#67642=VERTEX_POINT ( 'NONE', #46895 ) ;
#67643=B_SPLINE_CURVE_WITH_KNOTS ( 'NONE', 3,
 ( #3485, #10701, #38167, #65624, #2596, #43592, #71066, #36835, #23753, #64294 ),
 .UNSPECIFIED., .F., .F.,
 ( 4, 2, 2, 2, 4 ),
 ( 0.0007817246256747528103, 0.0009771112852218980915, 0.001172497944769043156, 0.001367884604316188437, 0.001563271263863333718 ),
 .UNSPECIFIED. ) ;
#67645=DIRECTION ( 'NONE',  ( -0.000000000000000000, -0.3420201433256694346, -0.9396926207859080948 ) ) ;
#67646=EDGE_CURVE ( 'NONE', #54317, #79691, #66094, .T. ) ;
#67647=EDGE_LOOP ( 'NONE', ( #55878, #23895, #58684, #16446 ) ) ;
#67648=EDGE_LOOP ( 'NONE', ( #24974, #51997 ) ) ;
#67650=CARTESIAN_POINT ( 'NONE',  ( -12.52680890749923570, -3.300289026998414865, 32.46337939537583139 ) ) ;
#67651=CARTESIAN_POINT ( 'NONE',  ( 10.68145194873469173, -4.661471528628508665, 34.16647553114624003 ) ) ;
#67653=EDGE_CURVE ( 'NONE', #66313, #45635, #27339, .T. ) ;
#67654=CARTESIAN_POINT ( 'NONE',  ( -14.55771553191376633, -2.985938066672154445, 32.43141759479405550 ) ) ;
#67655=EDGE_LOOP ( 'NONE', ( #50146, #65412, #83632, #52268 ) ) ;
#67656=FACE_OUTER_BOUND ( 'NONE', #1078, .T. ) ;
#67657=CARTESIAN_POINT ( 'NONE',  ( -5.076923076923075762, -1.509761064869970415, 31.06009739812519044 ) ) ;
#67658=CARTESIAN_POINT ( 'NONE',  ( 17.07692307692295586, -11.67786785259630911, 32.92929555188603530 ) ) ;
#67659=AXIS2_PLACEMENT_3D ( 'NONE', #29205, #37260, #15240 ) ;
#67660=VERTEX_POINT ( 'NONE', #6798 ) ;
#67661=EDGE_CURVE ( 'NONE', #82873, #42667, #19836, .T. ) ;
#67662=DIRECTION ( 'NONE',  ( 0.000000000000000000, 0.9396926207859126468, 0.3420201433256571111 ) ) ;
#67664=CARTESIAN_POINT ( 'NONE',  ( -0.2385271099256129623, -2.758310577978207334, 31.33698337089303010 ) ) ;
#67665=FACE_OUTER_BOUND ( 'NONE', #14471, .T. ) ;
#67666=ORIENTED_EDGE ( 'NONE', *, *, #13053, .T. ) ;
#67667=CARTESIAN_POINT ( 'NONE',  ( 0.5923302693632478411, -4.118422570099827595, 33.43335022499816489 ) ) ;
#67668=CARTESIAN_POINT ( 'NONE',  ( -6.222926958906846551, -2.308479472611653094, 30.53278059502174457 ) ) ;
#67669=CARTESIAN_POINT ( 'NONE',  ( -6.857821783564084228, -12.51329471203373700, 31.30864560766537963 ) ) ;
#67670=EDGE_CURVE ( 'NONE', #65590, #44756, #82479, .T. ) ;
#67671=CARTESIAN_POINT ( 'NONE',  ( 7.173131342990377135, -12.41089969410671223, 31.60739465890703670 ) ) ;
#67672=CARTESIAN_POINT ( 'NONE',  ( -1.634638608836842089, -10.92453946501458439, 33.72985991061850086 ) ) ;
#67673=ORIENTED_EDGE ( 'NONE', *, *, #38090, .F. ) ;
#67674=FACE_BOUND ( 'NONE', #69025, .T. ) ;
#67675=ORIENTED_EDGE ( 'NONE', *, *, #55342, .T. ) ;
#67676=CARTESIAN_POINT ( 'NONE',  ( -4.403846153846151523, -7.500000000000001776, 34.75000000000000000 ) ) ;
#67677=CARTESIAN_POINT ( 'NONE',  ( -10.61538461538461320, -2.249999999999998668, 29.75000000000001776 ) ) ;
#67679=CARTESIAN_POINT ( 'NONE',  ( -18.00000000000000000, -10.67929555188718282, 33.92786785259543336 ) ) ;
#67681=CARTESIAN_POINT ( 'NONE',  ( 17.07692307692307665, -1.790695186598648903, 34.54067556320373455 ) ) ;
#67682=CARTESIAN_POINT ( 'NONE',  ( 5.326923076923075762, -2.249999999999998668, 29.75000000000000355 ) ) ;
#67683=EDGE_CURVE ( 'NONE', #20327, #82892, #63510, .T. ) ;
#67684=AXIS2_PLACEMENT_3D ( 'NONE', #84486, #30851, #64182 ) ;
#67685=AXIS2_PLACEMENT_3D ( 'NONE', #66938, #52964, #47093 ) ;
#67686=EDGE_LOOP ( 'NONE', ( #78975, #55721 ) ) ;
#67688=ORIENTED_EDGE ( 'NONE', *, *, #76937, .T. ) ;
#67689=ORIENTED_EDGE ( 'NONE', *, *, #4966, .T. ) ;
#67690=EDGE_CURVE ( 'NONE', #75887, #79557, #70278, .T. ) ;
#67692=CARTESIAN_POINT ( 'NONE',  ( -6.249976730942353953, -12.41269422305637171, 30.68257228309993323 ) ) ;
#67693=CARTESIAN_POINT ( 'NONE',  ( -4.087777802843714170, -8.973038597847269315, 34.52809138561122637 ) ) ;
#67694=CARTESIAN_POINT ( 'NONE',  ( -8.096177070375302876, -3.520140089381495585, 33.17453946501458262 ) ) ;
#67695=CARTESIAN_POINT ( 'NONE',  ( 11.40831432902331954, -2.619462340734462380, 30.83744416345203021 ) ) ;
#67698=CARTESIAN_POINT ( 'NONE',  ( -5.076923076923199218, -11.67786785259630911, 32.92929555188603530 ) ) ;
#67699=ORIENTED_EDGE ( 'NONE', *, *, #16028, .F. ) ;
#67701=VERTEX_POINT ( 'NONE', #62621 ) ;
#67702=CARTESIAN_POINT ( 'NONE',  ( -11.60373198442231590, -12.46129190929999986, 30.37095296980880832 ) ) ;
#67703=VERTEX_POINT ( 'NONE', #21198 ) ;
#67704=CARTESIAN_POINT ( 'NONE',  ( -3.165514091256391271, -10.33852847137154107, 34.16647553114620450 ) ) ;
#67705=DIRECTION ( 'NONE',  ( -0.000000000000000000, 0.6427876096865404731, -0.7660444431189770143 ) ) ;
#67706=B_SPLINE_CURVE_WITH_KNOTS ( 'NONE', 3,
 ( #25735, #18538, #45995, #53192, #80698, #18979, #67167, #26177, #41466, #33386 ),
 .UNSPECIFIED., .F., .F.,
 ( 4, 2, 2, 2, 4 ),
 ( 0.000000000000000000, 0.0001954339857564078809, 0.0003908679715128157619, 0.0005863019572692236428, 0.0007817359430256315238 ),
 .UNSPECIFIED. ) ;
#67707=CARTESIAN_POINT ( 'NONE',  ( -0.4615384615385840772, -2.379036618888197285, 30.90682066428292885 ) ) ;
#67709=ADVANCED_FACE ( 'NONE', ( #16217 ), #42376, .F. ) ;
#67710=FACE_BOUND ( 'NONE', #62350, .T. ) ;
#67711=ORIENTED_EDGE ( 'NONE', *, *, #61984, .T. ) ;
#67713=FACE_OUTER_BOUND ( 'NONE', #57871, .T. ) ;
#67715=VERTEX_POINT ( 'NONE', #71152 ) ;
#67716=CARTESIAN_POINT ( 'NONE',  ( 6.000000000000001776, -9.905515769479276145, 34.41647553114623292 ) ) ;
#67717=ORIENTED_EDGE ( 'NONE', *, *, #57485, .F. ) ;
#67718=FACE_BOUND ( 'NONE', #69072, .T. ) ;
#67719=CARTESIAN_POINT ( 'NONE',  ( 7.846153846153846700, -11.69971097300155272, 32.46337939537588113 ) ) ;
#67720=CARTESIAN_POINT ( 'NONE',  ( 15.16468685140909400, -6.343179335718451384, 34.87096338111212646 ) ) ;
#67721=ORIENTED_EDGE ( 'NONE', *, *, #7073, .F. ) ;
#67722=CARTESIAN_POINT ( 'NONE',  ( -5.777037096438515817, -7.369474270740069777, 34.74850911626239736 ) ) ;
#67724=CARTESIAN_POINT ( 'NONE',  ( 1.254468175177166467, -3.285722584762969856, 32.44110544564090759 ) ) ;
#67725=ORIENTED_EDGE ( 'NONE', *, *, #55007, .F. ) ;
#67726=DIRECTION ( 'NONE',  ( 0.000000000000000000, 0.000000000000000000, 1.000000000000000000 ) ) ;
#67727=CARTESIAN_POINT ( 'NONE',  ( -7.846153846153967493, -8.656820664282941280, 34.87096338111179961 ) ) ;
#67728=CARTESIAN_POINT ( 'NONE',  ( 18.25005441991345734, -10.82426656108011720, 33.81400080652039009 ) ) ;
#67729=CARTESIAN_POINT ( 'NONE',  ( -7.976845312821404299, -2.729777683071817229, 31.24903638046269450 ) ) ;
#67730=ORIENTED_EDGE ( 'NONE', *, *, #34592, .F. ) ;
#67731=B_SPLINE_CURVE_WITH_KNOTS ( 'NONE', 3,
 ( #83549, #43437, #56506, #7441, #21833, #49303, #76782, #36242, #63696, #15082 ),
 .UNSPECIFIED., .F., .F.,
 ( 4, 2, 2, 2, 4 ),
 ( 0.0007817359430256318490, 0.0009771253907249984917, 0.001172514838424365026, 0.001367904286123731560, 0.001563293733823098311 ),
 .UNSPECIFIED. ) ;
#67732=CARTESIAN_POINT ( 'NONE',  ( -2.307692307692305711, -11.16473453929635440, 33.15142922261926373 ) ) ;
#67734=ORIENTED_EDGE ( 'NONE', *, *, #49220, .F. ) ;
#67735=DIRECTION ( 'NONE',  ( -0.000000000000000000, -0.8660254037844397068, -0.4999999999999978906 ) ) ;
#67737=CARTESIAN_POINT ( 'NONE',  ( -13.38461538461550582, -5.219633306517616589, 34.19971097300220464 ) ) ;
#67738=CARTESIAN_POINT ( 'NONE',  ( -4.826868765284761942, -8.303483539816728154, 34.68545999027711702 ) ) ;
#67739=DIRECTION ( 'NONE',  ( -0.000000000000000000, -0.3420201433256694346, -0.9396926207859080948 ) ) ;
#67740=CARTESIAN_POINT ( 'NONE',  ( 15.16468685140909400, -5.471508081941602875, 34.59228464037088457 ) ) ;
#67741=CARTESIAN_POINT ( 'NONE',  ( 0.2115384615384615641, -7.500000000000001776, 34.75000000000000000 ) ) ;
#67742=DIRECTION ( 'NONE',  ( 0.000000000000000000, 0.4999999999999985567, 0.8660254037844395958 ) ) ;
#67743=DIRECTION ( 'NONE',  ( 0.000000000000000000, 0.6427876096865373645, -0.7660444431189797898 ) ) ;
#67746=CARTESIAN_POINT ( 'NONE',  ( 5.076923076923075762, -6.343179335718451384, 34.87096338111211935 ) ) ;
#67747=EDGE_LOOP ( 'NONE', ( #87855, #86005 ) ) ;
#67748=VECTOR ( 'NONE', #87101, 1000.000000000000227 ) ;
#67749=VECTOR ( 'NONE', #45434, 1000.000000000000000 ) ;
#67751=FACE_OUTER_BOUND ( 'NONE', #25528, .T. ) ;
#67752=ORIENTED_EDGE ( 'NONE', *, *, #19460, .T. ) ;
#67753=CARTESIAN_POINT ( 'NONE',  ( -5.076923076923199218, -11.67786785259630911, 32.92929555188603530 ) ) ;
#67755=CARTESIAN_POINT ( 'NONE',  ( 12.59237679202522031, -7.277220318596961057, 34.99547417642776992 ) ) ;
#67756=CARTESIAN_POINT ( 'NONE',  ( -9.019207500173124004, -3.137211980971221781, 32.19342716148376837 ) ) ;
#67757=CARTESIAN_POINT ( 'NONE',  ( -3.165513659493205623, -9.442884908240271713, 34.35708131394835618 ) ) ;
#67758=VECTOR ( 'NONE', #22627, 1000.000000000000114 ) ;
#67759=CARTESIAN_POINT ( 'NONE',  ( -5.076923076923199218, -2.657715359629662988, 31.77849191805970364 ) ) ;
#67760=CARTESIAN_POINT ( 'NONE',  ( -7.846153846153537614, -2.506253911140614576, 30.00000000000323297 ) ) ;
#67762=CARTESIAN_POINT ( 'NONE',  ( 6.792928953345224841, -12.50552854090298993, 31.33409797877408920 ) ) ;
#67763=CARTESIAN_POINT ( 'NONE',  ( 1.384615384615265343, -12.27809138561165270, 31.22303859784587132 ) ) ;
#67765=CARTESIAN_POINT ( 'NONE',  ( 1.384615384615386802, -11.33034616979429110, 35.88435417666054406 ) ) ;
#67766=ORIENTED_EDGE ( 'NONE', *, *, #25211, .T. ) ;
#67768=B_SPLINE_CURVE_WITH_KNOTS ( 'NONE', 3,
 ( #48902, #68290, #6593, #49354, #55652, #56106, #83600, #27305, #13784, #54768 ),
 .UNSPECIFIED., .F., .F.,
 ( 4, 2, 2, 2, 4 ),
 ( 0.0007817246256747470640, 0.0009771112852218898515, 0.001172497944769032531, 0.001367884604316175427, 0.001563271263863318106 ),
 .UNSPECIFIED. ) ;
#67769=CARTESIAN_POINT ( 'NONE',  ( -8.899922235898328537, -12.38065189839062263, 30.83690757178629482 ) ) ;
#67770=CARTESIAN_POINT ( 'NONE',  ( 0.4615384615384611200, -11.69971097300155272, 32.46337939537588113 ) ) ;
#67771=CYLINDRICAL_SURFACE ( 'NONE', #45429, 0.2499999999999973355 ) ;
#67772=CARTESIAN_POINT ( 'NONE',  ( 6.250000000000017764, -2.249999999999999112, 29.81603969181031033 ) ) ;
#67773=B_SPLINE_CURVE_WITH_KNOTS ( 'NONE', 3,
 ( #70306, #27550, #82943, #8618, #36089, #29329, #84283, #21226, #34298, #50027 ),
 .UNSPECIFIED., .F., .F.,
 ( 4, 2, 2, 2, 4 ),
 ( 0.000000000000000000, 0.0001954311584214072381, 0.0003908623168428144762, 0.0005862934752642217414, 0.0007817246336856289524 ),
 .UNSPECIFIED. ) ;
#67774=CARTESIAN_POINT ( 'NONE',  ( 6.130525701763564150, -5.195472089885680766, 34.18748526763464923 ) ) ;
#67775=FACE_OUTER_BOUND ( 'NONE', #68068, .T. ) ;
#67778=EDGE_LOOP ( 'NONE', ( #44664, #1919, #20017, #73230 ) ) ;
#67782=ORIENTED_EDGE ( 'NONE', *, *, #35859, .T. ) ;
#67783=CARTESIAN_POINT ( 'NONE',  ( -8.546217925137376881, -4.762714258010881885, 34.23016756924214832 ) ) ;
#67784=ADVANCED_FACE ( 'NONE', ( #49563 ), #55871, .F. ) ;
#67785=CARTESIAN_POINT ( 'NONE',  ( -2.373774687052442545, -9.058645607665454236, 34.76329471203372634 ) ) ;
#67786=CARTESIAN_POINT ( 'NONE',  ( 14.24242186173153435, -5.219633306516282545, 34.19971097300152962 ) ) ;
#67788=CARTESIAN_POINT ( 'NONE',  ( 3.100078627658924280, -8.191372820521381826, 34.95448215188423546 ) ) ;
#67789=CARTESIAN_POINT ( 'NONE',  ( 5.749976762707035505, -2.823816976329319495, 31.52131813110795733 ) ) ;
#67790=ORIENTED_EDGE ( 'NONE', *, *, #42597, .F. ) ;
#67791=ORIENTED_EDGE ( 'NONE', *, *, #47507, .F. ) ;
#67792=ORIENTED_EDGE ( 'NONE', *, *, #74010, .F. ) ;
#67793=VERTEX_POINT ( 'NONE', #49995 ) ;
#67794=B_SPLINE_CURVE_WITH_KNOTS ( 'NONE', 3,
 ( #6735, #26575, #54478, #27900, #67565, #81976, #61672, #75211, #61227, #18929 ),
 .UNSPECIFIED., .F., .F.,
 ( 4, 2, 2, 2, 4 ),
 ( 0.000000000000000000, 0.0001954311564186864949, 0.0003908623128373729899, 0.0005862934692560594577, 0.0007817246256747459798 ),
 .UNSPECIFIED. ) ;
#67796=CARTESIAN_POINT ( 'NONE',  ( 18.00000000000000000, -2.292212530054420494, 30.41441678777542634 ) ) ;
#67797=CARTESIAN_POINT ( 'NONE',  ( 7.780883400193072674, -3.835265460703609186, 33.15142922261924241 ) ) ;
#67798=B_SPLINE_CURVE_WITH_KNOTS ( 'NONE', 3,
 ( #12027, #12897, #72815, #60194, #46685, #80936, #5259, #39945, #67404, #5701 ),
 .UNSPECIFIED., .F., .F.,
 ( 4, 2, 2, 2, 4 ),
 ( 0.000000000000000000, 0.0001954339857564073659, 0.0003908679715128147319, 0.0005863019572692221250, 0.0007817359430256294638 ),
 .UNSPECIFIED. ) ;
#67800=AXIS2_PLACEMENT_3D ( 'NONE', #53516, #12546, #60724 ) ;
#67801=CARTESIAN_POINT ( 'NONE',  ( -16.21992853320628925, -2.292212530054420050, 30.41441678777542634 ) ) ;
#67803=CARTESIAN_POINT ( 'NONE',  ( 12.21151523731700550, -2.985938066672154445, 32.43141759479405550 ) ) ;
#67804=EDGE_LOOP ( 'NONE', ( #75347, #1949 ) ) ;
#67805=ORIENTED_EDGE ( 'NONE', *, *, #2586, .T. ) ;
#67806=VERTEX_POINT ( 'NONE', #83358 ) ;
#67807=LINE ( 'NONE', #47965, #64567 ) ;
#67808=EDGE_LOOP ( 'NONE', ( #63982, #63270 ) ) ;
#67809=FACE_OUTER_BOUND ( 'NONE', #23074, .T. ) ;
#67810=DIRECTION ( 'NONE',  ( 0.000000000000000000, 0.8660254037844377084, -0.5000000000000015543 ) ) ;
#67813=VERTEX_POINT ( 'NONE', #36922 ) ;
#67814=EDGE_CURVE ( 'NONE', #73573, #12391, #29303, .T. ) ;
#67817=CARTESIAN_POINT ( 'NONE',  ( 2.177545098254088707, -6.852621066184267029, 34.70813303252209181 ) ) ;
#67818=EDGE_CURVE ( 'NONE', #54248, #28816, #29575, .T. ) ;
#67819=FACE_BOUND ( 'NONE', #53972, .T. ) ;
#67820=CARTESIAN_POINT ( 'NONE',  ( -6.673022611438608642, -12.41262288849542017, 30.68299917996395010 ) ) ;
#67821=EDGE_CURVE ( 'NONE', #75335, #76807, #43250, .T. ) ;
#67822=LINE ( 'NONE', #32695, #49151 ) ;
#67823=ORIENTED_EDGE ( 'NONE', *, *, #88056, .T. ) ;
#67824=CARTESIAN_POINT ( 'NONE',  ( -12.71153846153846168, -7.500000000000001776, 34.75000000000000000 ) ) ;
#67825=LINE ( 'NONE', #12875, #66794 ) ;
#67826=ORIENTED_EDGE ( 'NONE', *, *, #55493, .F. ) ;
#67828=CARTESIAN_POINT ( 'NONE',  ( 1.384615384615386802, -1.129524287112498415, 32.06866353760679544 ) ) ;
#67829=CARTESIAN_POINT ( 'NONE',  ( -5.934744860487159102, -4.320704448112861584, 33.92786785259548310 ) ) ;
#67831=CARTESIAN_POINT ( 'NONE',  ( -2.307692307692428724, -9.528491918059723176, 34.59228464037033035 ) ) ;
#67832=CARTESIAN_POINT ( 'NONE',  ( 10.48523740594639619, -11.93770438780619259, 32.05411857736982029 ) ) ;
#67833=FACE_BOUND ( 'NONE', #74005, .T. ) ;
#67835=LINE ( 'NONE', #46674, #73330 ) ;
#67836=CARTESIAN_POINT ( 'NONE',  ( 2.307692307692309264, -4.102666532097928531, 36.13435417666054406 ) ) ;
#67838=CARTESIAN_POINT ( 'NONE',  ( -2.057746898314263273, -12.45601412856602686, 31.48342859153981621 ) ) ;
#67839=VECTOR ( 'NONE', #7498, 1000.000000000000227 ) ;
#67840=CARTESIAN_POINT ( 'NONE',  ( 8.992010438208831502, -12.69155399931963046, 30.53255429739157734 ) ) ;
#67842=ORIENTED_EDGE ( 'NONE', *, *, #50890, .F. ) ;
#67843=CARTESIAN_POINT ( 'NONE',  ( 18.00000000000000000, -9.905515769479276145, 34.41647553114623292 ) ) ;
#67844=ORIENTED_EDGE ( 'NONE', *, *, #59284, .F. ) ;
#67845=CARTESIAN_POINT ( 'NONE',  ( -1.384615384615383471, -10.05456864172156806, 36.03766855953608683 ) ) ;
#67846=ORIENTED_EDGE ( 'NONE', *, *, #37356, .T. ) ;
#67847=CARTESIAN_POINT ( 'NONE',  ( 16.37685899793954292, -12.64618726649961289, 30.78989965857442712 ) ) ;
#67850=ORIENTED_EDGE ( 'NONE', *, *, #14640, .T. ) ;
#67851=CARTESIAN_POINT ( 'NONE',  ( -10.39237177129122003, -11.98016756924215009, 32.48728574198911190 ) ) ;
#67852=CARTESIAN_POINT ( 'NONE',  ( 6.000000000000001776, -10.67929555188718282, 33.92786785259544047 ) ) ;
#67854=CARTESIAN_POINT ( 'NONE',  ( 4.403791672194295792, -10.76462480002816235, 33.53768742498949962 ) ) ;
#67855=CARTESIAN_POINT ( 'NONE',  ( 8.703960768674448900, -2.657715359629088780, 31.77849191805832874 ) ) ;
#67857=CARTESIAN_POINT ( 'NONE',  ( 1.318533005255250634, -4.661471528628507777, 34.16647553114621871 ) ) ;
#67858=CARTESIAN_POINT ( 'NONE',  ( -0.3954701105360229896, -4.098570777380720287, 33.41473453929635440 ) ) ;
#67859=CARTESIAN_POINT ( 'NONE',  ( 9.692307692307695177, -3.322132147404559976, 32.92929555188717927 ) ) ;
#67862=CARTESIAN_POINT ( 'NONE',  ( 5.299935921016470708, -2.523321265292115090, 31.42251411153756280 ) ) ;
#67863=CARTESIAN_POINT ( 'NONE',  ( 7.146088274689773812, -11.24521262558773671, 33.06293181088029343 ) ) ;
#67864=ORIENTED_EDGE ( 'NONE', *, *, #49833, .T. ) ;
#67865=DIRECTION ( 'NONE',  ( -0.000000000000000000, 0.9396926207859093161, -0.3420201433256663259 ) ) ;
#67868=CARTESIAN_POINT ( 'NONE',  ( -17.93393164899756087, -12.37446782046654192, 30.86335684631486842 ) ) ;
#67869=CARTESIAN_POINT ( 'NONE',  ( -5.142193522883852452, -2.625532179533445198, 30.86335684631481513 ) ) ;
#67874=CARTESIAN_POINT ( 'NONE',  ( 1.384615384615386802, -5.471508081941601098, 34.59228464037088457 ) ) ;
#67875=ORIENTED_EDGE ( 'NONE', *, *, #15778, .T. ) ;
#67876=DIRECTION ( 'NONE',  ( -0.000000000000000000, -0.5000000000000009992, -0.8660254037844380415 ) ) ;
#67877=CARTESIAN_POINT ( 'NONE',  ( 4.854094979288197997, -7.369209533119140509, 34.99857337881830688 ) ) ;
#67878=VECTOR ( 'NONE', #56892, 1000.000000000000000 ) ;
#67879=ADVANCED_FACE ( 'NONE', ( #69396 ), #7700, .F. ) ;
#67880=CARTESIAN_POINT ( 'NONE',  ( -12.71156168575991785, -4.931416488878822335, 34.32920672191015399 ) ) ;
#67881=VERTEX_POINT ( 'NONE', #29739 ) ;
#67882=B_SPLINE_CURVE_WITH_KNOTS ( 'NONE', 3,
 ( #79238, #78783, #50847, #17085, #86909, #44539, #4459, #45887, #25177, #30592 ),
 .UNSPECIFIED., .F., .F.,
 ( 4, 2, 2, 2, 4 ),
 ( 0.0007817246256747469556, 0.0009771112852218889842, 0.001172497944769031013, 0.001367884604316173041, 0.001563271263863315070 ),
 .UNSPECIFIED. ) ;
#67883=CARTESIAN_POINT ( 'NONE',  ( -9.469528023329626620, -2.612705202774698421, 31.66806509827799943 ) ) ;
#67884=DIRECTION ( 'NONE',  ( 0.000000000000000000, 0.9848077530122072432, 0.1736481776669354937 ) ) ;
#67885=CARTESIAN_POINT ( 'NONE',  ( -13.16160254052199008, -8.282913670948747864, 34.94150082978203642 ) ) ;
#67886=VERTEX_POINT ( 'NONE', #22968 ) ;
#67888=ORIENTED_EDGE ( 'NONE', *, *, #55333, .T. ) ;
#67890=VERTEX_POINT ( 'NONE', #77912 ) ;
#67891=EDGE_CURVE ( 'NONE', #81961, #38938, #35158, .T. ) ;
#67892=CARTESIAN_POINT ( 'NONE',  ( 5.299934428535926223, -12.15243808032446005, 31.58219941686247978 ) ) ;
#67893=CARTESIAN_POINT ( 'NONE',  ( 14.17700084102475344, -4.118384482072086072, 33.43331474514187107 ) ) ;
#67894=EDGE_CURVE ( 'NONE', #86167, #2856, #84302, .T. ) ;
#67895=CARTESIAN_POINT ( 'NONE',  ( -16.28453675695647007, -2.845849958028613624, 32.17971566917920967 ) ) ;
#67897=B_SPLINE_CURVE_WITH_KNOTS ( 'NONE', 3,
 ( #29259, #71105, #22485, #8981, #78302, #83762, #36449, #57154, #85517, #63901 ),
 .UNSPECIFIED., .F., .F.,
 ( 4, 2, 2, 2, 4 ),
 ( 0.0007817359430256287049, 0.0009771253907249945886, 0.001172514838424360255, 0.001367904286123725922, 0.001563293733823091806 ),
 .UNSPECIFIED. ) ;
#67898=CARTESIAN_POINT ( 'NONE',  ( 5.142991427925513115, -5.557115091759786019, 34.35708131394839882 ) ) ;
#67899=AXIS2_PLACEMENT_3D ( 'NONE', #16213, #49112, #49991 ) ;
#67900=ORIENTED_EDGE ( 'NONE', *, *, #50384, .T. ) ;
#67903=VERTEX_POINT ( 'NONE', #73384 ) ;
#67904=CARTESIAN_POINT ( 'NONE',  ( -6.923076923076922462, -2.486705287966279876, 31.30864560766543647 ) ) ;
#67905=VERTEX_POINT ( 'NONE', #25192 ) ;
#67906=CARTESIAN_POINT ( 'NONE',  ( -5.076923076923199218, -12.51329471203414379, 31.30864560766407578 ) ) ;
#67907=CYLINDRICAL_SURFACE ( 'NONE', #88269, 0.2499999999999973355 ) ;
#67908=EDGE_CURVE ( 'NONE', #41728, #2541, #63859, .T. ) ;
#67910=DIRECTION ( 'NONE',  ( -0.000000000000000000, 0.9848077530122086864, -0.1736481776669273891 ) ) ;
#67911=ADVANCED_FACE ( 'NONE', ( #45002 ), #79698, .F. ) ;
#67913=ORIENTED_EDGE ( 'NONE', *, *, #2471, .F. ) ;
#67914=VERTEX_POINT ( 'NONE', #65721 ) ;
#67915=CARTESIAN_POINT ( 'NONE',  ( -16.15384615384615330, -8.120952969808772792, 34.71129190930000163 ) ) ;
#67916=CYLINDRICAL_SURFACE ( 'NONE', #51647, 0.2499999999999994726 ) ;
#67917=ORIENTED_EDGE ( 'NONE', *, *, #26377, .F. ) ;
#67918=CARTESIAN_POINT ( 'NONE',  ( 9.562160482869472844, -11.93770438780619259, 32.05411857736982029 ) ) ;
#67919=CARTESIAN_POINT ( 'NONE',  ( -17.20761368003338987, -3.338472653186243200, 32.95098750199972670 ) ) ;
#67920=EDGE_CURVE ( 'NONE', #80449, #81210, #543, .T. ) ;
#67921=EDGE_LOOP ( 'NONE', ( #55008, #788 ) ) ;
#67923=CARTESIAN_POINT ( 'NONE',  ( -18.00000000000000000, -2.538708090699994813, 30.37095296980875858 ) ) ;
#67925=FACE_BOUND ( 'NONE', #44764, .T. ) ;
#67926=CARTESIAN_POINT ( 'NONE',  ( -17.77722045873158763, -8.496831190052089866, 34.64984203495476578 ) ) ;
#67927=CARTESIAN_POINT ( 'NONE',  ( -12.46153846153858247, -9.442884908241554243, 34.35708131394783038 ) ) ;
#67928=B_SPLINE_CURVE_WITH_KNOTS ( 'NONE', 3,
 ( #33321, #26563, #54018, #82396, #27003, #6295, #20682, #61214, #48145, #54462 ),
 .UNSPECIFIED., .F., .F.,
 ( 4, 2, 2, 2, 4 ),
 ( 0.0007817359430256359690, 0.0009771253907250036959, 0.001172514838424371314, 0.001367904286123738933, 0.001563293733823106768 ),
 .UNSPECIFIED. ) ;
#67930=CARTESIAN_POINT ( 'NONE',  ( 11.76124107972994537, -12.44528174975671853, 30.48912976160716681 ) ) ;
#67931=PLANE ( 'NONE',  #2903 ) ;
#67932=CARTESIAN_POINT ( 'NONE',  ( 6.673100179028333301, -10.82459398097509684, 33.81372124010185587 ) ) ;
#67933=AXIS2_PLACEMENT_3D ( 'NONE', #9946, #25688, #16701 ) ;
#67934=EDGE_CURVE ( 'NONE', #13671, #19193, #74551, .T. ) ;
#67935=CARTESIAN_POINT ( 'NONE',  ( -0.4615384615384611200, -1.044019251281081972, 31.83374038241031911 ) ) ;
#67936=CARTESIAN_POINT ( 'NONE',  ( 7.146452863775108355, -2.501478030877322567, 29.88021232661720816 ) ) ;
#67937=ORIENTED_EDGE ( 'NONE', *, *, #68657, .T. ) ;
#67938=ADVANCED_FACE ( 'NONE', ( #11237 ), #59421, .F. ) ;
#67939=CARTESIAN_POINT ( 'NONE',  ( -15.16470189741915320, -11.35647404775217595, 33.31231777344666511 ) ) ;
#67940=CARTESIAN_POINT ( 'NONE',  ( 0.3313904918067619998, -11.04286588640298561, 33.62463336215343901 ) ) ;
#67941=ORIENTED_EDGE ( 'NONE', *, *, #55368, .F. ) ;
#67944=CARTESIAN_POINT ( 'NONE',  ( -15.45369544828537833, -2.554751324335734708, 30.48935550225260727 ) ) ;
#67946=ORIENTED_EDGE ( 'NONE', *, *, #32699, .F. ) ;
#67947=FACE_OUTER_BOUND ( 'NONE', #56451, .T. ) ;
#67948=CARTESIAN_POINT ( 'NONE',  ( 6.857806922520603976, -8.656820664281497102, 34.87096338111211935 ) ) ;
#67949=FACE_BOUND ( 'NONE', #69957, .T. ) ;
#67950=CARTESIAN_POINT ( 'NONE',  ( -14.30769230769230660, -13.49023893513002648, 31.06009739812518688 ) ) ;
#67951=CARTESIAN_POINT ( 'NONE',  ( -16.82692307692306954, -2.249999999999999112, 29.81603969181033165 ) ) ;
#67953=CARTESIAN_POINT ( 'NONE',  ( 0.4615384615384611200, -4.661471528628507777, 34.16647553114623292 ) ) ;
#67955=CARTESIAN_POINT ( 'NONE',  ( -14.43830196289638579, -7.722926974430166069, 34.99546784045485737 ) ) ;
#67957=ORIENTED_EDGE ( 'NONE', *, *, #52110, .T. ) ;
#67958=B_SPLINE_CURVE_WITH_KNOTS ( 'NONE', 3,
 ( #25199, #4939, #87820, #12142, #33299, #31509, #65727, #39174, #40068, #10800 ),
 .UNSPECIFIED., .F., .F.,
 ( 4, 2, 2, 2, 4 ),
 ( 0.000000000000000000, 0.0001954339857564084773, 0.0003908679715128169545, 0.0005863019572692254860, 0.0007817359430256339090 ),
 .UNSPECIFIED. ) ;
#67959=ORIENTED_EDGE ( 'NONE', *, *, #2312, .T. ) ;
#67960=CARTESIAN_POINT ( 'NONE',  ( 4.826899852701617810, -10.92453946501458439, 33.72985991061850086 ) ) ;
#67961=CARTESIAN_POINT ( 'NONE',  ( -4.403822884788507253, -12.41269422305637171, 30.68257228309993323 ) ) ;
#67962=CARTESIAN_POINT ( 'NONE',  ( 16.37662582282421297, -3.020022701398814569, 32.48759521482552515 ) ) ;
#67963=CARTESIAN_POINT ( 'NONE',  ( 10.74617505635157144, -2.845873456487966635, 32.17976146951972538 ) ) ;
#67964=CARTESIAN_POINT ( 'NONE',  ( -3.480792468062196221, -5.851115903089112003, 34.47074536777953568 ) ) ;
#67966=CARTESIAN_POINT ( 'NONE',  ( -8.769230769230768274, -9.905515769479276145, 34.41647553114623292 ) ) ;
#67967=CARTESIAN_POINT ( 'NONE',  ( 1.253924781505077801, -9.929715669179220328, 34.40415004197138416 ) ) ;
#67968=CARTESIAN_POINT ( 'NONE',  ( 17.74997677577854560, -4.175268141568689195, 33.81360843649122216 ) ) ;
#67969=CARTESIAN_POINT ( 'NONE',  ( -14.98082371242109012, -11.37275283266504111, 32.91324779482534524 ) ) ;
#67970=CARTESIAN_POINT ( 'NONE',  ( -9.692307692307691624, -11.16473453929635440, 33.15142922261926373 ) ) ;
#67971=CARTESIAN_POINT ( 'NONE',  ( 8.546304551714618114, -12.15238873228292071, 31.58232369045353849 ) ) ;
#67972=VECTOR ( 'NONE', #84583, 1000.000000000000000 ) ;
#67973=CARTESIAN_POINT ( 'NONE',  ( 6.000000000000001776, -12.10708131394839349, 31.69288490824020244 ) ) ;
#67974=EDGE_CURVE ( 'NONE', #23594, #19289, #29421, .T. ) ;
#67975=LINE ( 'NONE', #6277, #27567 ) ;
#67976=B_SPLINE_CURVE_WITH_KNOTS ( 'NONE', 3,
 ( #23838, #86009, #44112, #64828, #57643, #85126 ),
 .UNSPECIFIED., .F., .F.,
 ( 4, 2, 4 ),
 ( 4.220987180333914613E-17, 0.0001954756301637177243, 0.0003909512603273932732 ),
 .UNSPECIFIED. ) ;
#67977=CARTESIAN_POINT ( 'NONE',  ( -3.454254155333563059, -12.47654668319379567, 31.42292124445336654 ) ) ;
#67978=EDGE_LOOP ( 'NONE', ( #68767, #1991, #12438, #39139 ) ) ;
#67979=ADVANCED_FACE ( 'NONE', ( #37360 ), #3131, .F. ) ;
#67980=CARTESIAN_POINT ( 'NONE',  ( -14.30769230769230660, -4.945431358278436385, 36.03766855953609394 ) ) ;
#67981=EDGE_CURVE ( 'NONE', #20157, #39109, #67519, .T. ) ;
#67984=B_SPLINE_CURVE_WITH_KNOTS ( 'NONE', 3,
 ( #53992, #25638, #54431, #73382, #81926, #47231, #73837, #19329, #74723, #40058 ),
 .UNSPECIFIED., .F., .F.,
 ( 4, 2, 2, 2, 4 ),
 ( 0.0007817359430256301143, 0.0009771253907249963233, 0.001172514838424362641, 0.001367904286123728958, 0.001563293733823095276 ),
 .UNSPECIFIED. ) ;
#67985=EDGE_CURVE ( 'NONE', #66983, #7925, #20218, .T. ) ;
#67986=CARTESIAN_POINT ( 'NONE',  ( 3.903822929624696680, -4.931416488878822335, 34.32920672191015399 ) ) ;
#67987=CYLINDRICAL_SURFACE ( 'NONE', #71434, 0.2499999999999995559 ) ;
#67988=DIRECTION ( 'NONE',  ( 0.000000000000000000, 0.1736481776669267785, -0.9848077530122087975 ) ) ;
#67989=CARTESIAN_POINT ( 'NONE',  ( -14.30769230769242739, -12.27809138561165270, 31.22303859784587132 ) ) ;
#67990=EDGE_LOOP ( 'NONE', ( #36980, #38690 ) ) ;
#67992=CARTESIAN_POINT ( 'NONE',  ( 3.296024370282069071, -8.656820664281605460, 34.87096338111211224 ) ) ;
#67993=ORIENTED_EDGE ( 'NONE', *, *, #27039, .F. ) ;
#67994=FACE_OUTER_BOUND ( 'NONE', #71676, .T. ) ;
#67996=CARTESIAN_POINT ( 'NONE',  ( 11.53846153846153832, -1.790695186598648903, 34.54067556320373455 ) ) ;
#67998=CARTESIAN_POINT ( 'NONE',  ( 7.622668902429897919, -4.386631170607603991, 33.66268669641500111 ) ) ;
#67999=CARTESIAN_POINT ( 'NONE',  ( -16.08870037451418966, -7.750023238201980469, 34.74374492549440419 ) ) ;
#68000=CARTESIAN_POINT ( 'NONE',  ( 2.084765348785459604, -12.64616026154729411, 30.79003144601913533 ) ) ;
#68002=VERTEX_POINT ( 'NONE', #82368 ) ;
#68003=VECTOR ( 'NONE', #13572, 1000.000000000000227 ) ;
#68004=EDGE_LOOP ( 'NONE', ( #78210, #45427 ) ) ;
#68005=VECTOR ( 'NONE', #87085, 1000.000000000000000 ) ;
#68006=CARTESIAN_POINT ( 'NONE',  ( -8.096177070375304652, -2.341070481393819236, 30.72580821765574299 ) ) ;
#68007=FACE_OUTER_BOUND ( 'NONE', #7968, .T. ) ;
#68009=CARTESIAN_POINT ( 'NONE',  ( -17.14219352288385778, -6.026961402152685388, 34.52809138561120506 ) ) ;
#68010=DIRECTION ( 'NONE',  ( -0.000000000000000000, -0.3420201433256694901, -0.9396926207859082059 ) ) ;
#68011=CARTESIAN_POINT ( 'NONE',  ( 20.74999999999999645, -4.500000000000000000, 29.75000000000000355 ) ) ;
#68012=EDGE_CURVE ( 'NONE', #53025, #27202, #78847, .T. ) ;
#68013=CARTESIAN_POINT ( 'NONE',  ( 17.07692307692307665, -3.322132147404559976, 32.92929555188717927 ) ) ;
#68015=B_SPLINE_CURVE_WITH_KNOTS ( 'NONE', 3,
 ( #67727, #19096, #39379, #27176, #88031, #40706, #81248, #6032, #47888, #53310 ),
 .UNSPECIFIED., .F., .F.,
 ( 4, 2, 2, 2, 4 ),
 ( 0.0007817246256747484735, 0.0009771112852218926705, 0.001172497944769037084, 0.001367884604316181498, 0.001563271263863325695 ),
 .UNSPECIFIED. ) ;
#68016=EDGE_CURVE ( 'NONE', #65133, #62019, #42335, .T. ) ;
#68017=CARTESIAN_POINT ( 'NONE',  ( -0.3962833220256225530, -12.51329471203373700, 31.30864560766537963 ) ) ;
#68019=ORIENTED_EDGE ( 'NONE', *, *, #41888, .F. ) ;
#68020=CARTESIAN_POINT ( 'NONE',  ( 18.00000000000000000, -9.058645607665452459, 34.76329471203371924 ) ) ;
#68021=EDGE_LOOP ( 'NONE', ( #23927, #67752 ) ) ;
#68022=CARTESIAN_POINT ( 'NONE',  ( -13.45036881292871556, -7.249945578846652694, 34.99404164642496795 ) ) ;
#68023=CARTESIAN_POINT ( 'NONE',  ( 12.46153846153833911, -3.300289026999228881, 32.46337939537708905 ) ) ;
#68025=CARTESIAN_POINT ( 'NONE',  ( -14.30769230769230660, -4.098570777380720287, 33.41473453929634729 ) ) ;
#68026=AXIS2_PLACEMENT_3D ( 'NONE', #48368, #20015, #82174 ) ;
#68028=CARTESIAN_POINT ( 'NONE',  ( 17.14217821643591932, -9.528491918058456633, 34.59228464037085615 ) ) ;
#68029=VERTEX_POINT ( 'NONE', #87815 ) ;
#68030=LINE ( 'NONE', #39231, #30126 ) ;
#68031=ADVANCED_FACE ( 'NONE', ( #88697 ), #53546, .F. ) ;
#68032=VERTEX_POINT ( 'NONE', #4933 ) ;
#68033=EDGE_CURVE ( 'NONE', #77653, #43710, #8985, .T. ) ;
#68034=CARTESIAN_POINT ( 'NONE',  ( -16.28399336328437386, -6.852621066184266141, 34.70813303252209181 ) ) ;
#68035=CARTESIAN_POINT ( 'NONE',  ( 12.21156171748987163, -2.318417181685855422, 30.59732222474233865 ) ) ;
#68036=FACE_BOUND ( 'NONE', #16482, .T. ) ;
#68037=CARTESIAN_POINT ( 'NONE',  ( 0.4615384615384611200, -13.75783147151868846, 33.36296068462461051 ) ) ;
#68038=CARTESIAN_POINT ( 'NONE',  ( 16.15384615384615330, -3.322132147404559976, 32.92929555188717927 ) ) ;
#68039=EDGE_CURVE ( 'NONE', #45648, #37486, #58418, .T. ) ;
#68040=CARTESIAN_POINT ( 'NONE',  ( 18.00000000000000000, -5.180354513474913603, 36.12317359536750416 ) ) ;
#68041=CARTESIAN_POINT ( 'NONE',  ( 10.39245765647776309, -10.01117774369187252, 34.36070679894347535 ) ) ;
#68042=DIRECTION ( 'NONE',  ( -0.000000000000000000, 0.6427876096865404731, -0.7660444431189771253 ) ) ;
#68045=CARTESIAN_POINT ( 'NONE',  ( -10.55012904410858532, -4.481592998940250538, 33.73612834413965089 ) ) ;
#68047=EDGE_LOOP ( 'NONE', ( #71994, #53181, #18938, #59360 ) ) ;
#68048=LINE ( 'NONE', #55406, #70561 ) ;
#68049=CARTESIAN_POINT ( 'NONE',  ( -18.22292695890684655, -10.01117774369187252, 34.36070679894347535 ) ) ;
#68050=EDGE_CURVE ( 'NONE', #77161, #38977, #80599, .T. ) ;
#68051=CARTESIAN_POINT ( 'NONE',  ( -3.903846153846215472, -7.565270000091922853, 34.99999999999999289 ) ) ;
#68053=DIRECTION ( 'NONE',  ( 0.000000000000000000, 0.000000000000000000, 1.000000000000000000 ) ) ;
#68054=CARTESIAN_POINT ( 'NONE',  ( -2.307692307692427391, -2.892918686052166066, 31.69288490824153470 ) ) ;
#68056=CARTESIAN_POINT ( 'NONE',  ( 2.084766090176160436, -9.086856451489515152, 34.49173150075333183 ) ) ;
#68057=CARTESIAN_POINT ( 'NONE',  ( 14.05771557674995442, -11.28823185664190376, 33.01397839955799896 ) ) ;
#68058=CARTESIAN_POINT ( 'NONE',  ( -3.453696189676077832, -11.43668979543635089, 33.22377378376089752 ) ) ;
#68059=CARTESIAN_POINT ( 'NONE',  ( -16.02305571287919861, -3.957578996910245284, 33.62503395064540257 ) ) ;
#68060=VERTEX_POINT ( 'NONE', #60306 ) ;
#68061=EDGE_CURVE ( 'NONE', #45177, #62016, #48698, .T. ) ;
#68064=ORIENTED_EDGE ( 'NONE', *, *, #12709, .F. ) ;
#68066=CARTESIAN_POINT ( 'NONE',  ( 10.54930223602447903, -3.937682226553330445, 33.60647404775217240 ) ) ;
#68068=EDGE_LOOP ( 'NONE', ( #1440, #57256, #2965, #23297 ) ) ;
#68069=CARTESIAN_POINT ( 'NONE',  ( 4.403846153846153300, -7.500000000000001776, 35.04278698407183867 ) ) ;
#68070=LINE ( 'NONE', #26190, #87478 ) ;
#68071=CARTESIAN_POINT ( 'NONE',  ( 3.480714640147274608, -10.18230066228895758, 34.26354781536631577 ) ) ;
#68072=CARTESIAN_POINT ( 'NONE',  ( 1.515405825582336607, -6.369690395747424461, 34.87708834333098196 ) ) ;
#68073=AXIS2_PLACEMENT_3D ( 'NONE', #66640, #37825, #71602 ) ;
#68074=DIRECTION ( 'NONE',  ( -0.000000000000000000, 0.3420201433256694346, -0.9396926207859080948 ) ) ;
#68075=EDGE_LOOP ( 'NONE', ( #51225, #75207 ) ) ;
#68076=CARTESIAN_POINT ( 'NONE',  ( 11.47321054830029752, -2.506253911140460922, 30.00000000000013856 ) ) ;
#68077=CARTESIAN_POINT ( 'NONE',  ( -12.23852710992561121, -11.76359900205217457, 32.36225158514719880 ) ) ;
#68078=ORIENTED_EDGE ( 'NONE', *, *, #74069, .T. ) ;
#68079=CARTESIAN_POINT ( 'NONE',  ( -16.15384615384615330, -11.91647553114624181, 32.58852847137148245 ) ) ;
#68080=CARTESIAN_POINT ( 'NONE',  ( -2.372962753653081958, -9.442884908240170461, 34.35708131394840592 ) ) ;
#68081=LINE ( 'NONE', #25757, #6980 ) ;
#68082=DIRECTION ( 'NONE',  ( 1.000000000000000000, 0.000000000000000000, 0.000000000000000000 ) ) ;
#68083=EDGE_CURVE ( 'NONE', #58457, #48900, #82062, .T. ) ;
#68084=CARTESIAN_POINT ( 'NONE',  ( -9.822998295417995962, -12.35290016733513951, 31.75349464988449455 ) ) ;
#68085=FACE_OUTER_BOUND ( 'NONE', #17745, .T. ) ;
#68086=CARTESIAN_POINT ( 'NONE',  ( -10.61538461538461320, -1.629998284177014645, 34.34916445242399163 ) ) ;
#68088=EDGE_LOOP ( 'NONE', ( #12404, #47076 ) ) ;
#68089=EDGE_CURVE ( 'NONE', #22486, #12820, #1712, .T. ) ;
#68090=CARTESIAN_POINT ( 'NONE',  ( 14.98079249982687777, -8.303909089506435137, 34.68538101551103381 ) ) ;
#68091=CARTESIAN_POINT ( 'NONE',  ( 1.254467414883691401, -9.504002272028875709, 34.60269587691767867 ) ) ;
#68092=ORIENTED_EDGE ( 'NONE', *, *, #71828, .F. ) ;
#68093=EDGE_LOOP ( 'NONE', ( #80792, #37645 ) ) ;
#68094=CARTESIAN_POINT ( 'NONE',  ( -5.934744428723973897, -2.625532179533470512, 30.86335684631491105 ) ) ;
#68095=CARTESIAN_POINT ( 'NONE',  ( -12.68446467905460473, -3.105860786376062332, 32.13614157043599562 ) ) ;
#68096=CARTESIAN_POINT ( 'NONE',  ( -8.899378738962470337, -11.04286588640298561, 33.62463336215343901 ) ) ;
#68097=EDGE_CURVE ( 'NONE', #87048, #74753, #61614, .T. ) ;
#68098=CYLINDRICAL_SURFACE ( 'NONE', #9661, 0.2500000000000009437 ) ;
#68100=CARTESIAN_POINT ( 'NONE',  ( 0.5920638997721057173, -2.372941743896879174, 30.88044141588254377 ) ) ;
#68101=VERTEX_POINT ( 'NONE', #83249 ) ;
#68102=CARTESIAN_POINT ( 'NONE',  ( 17.07692307692307665, -3.050289026998446396, 32.03036669348365706 ) ) ;
#68103=ADVANCED_FACE ( 'NONE', ( #1260 ), #8477, .F. ) ;
#68104=CARTESIAN_POINT ( 'NONE',  ( -14.43783951713052716, -2.882441371585227508, 31.66841991370172238 ) ) ;
#68105=DIRECTION ( 'NONE',  ( 0.000000000000000000, 0.3420201433256610524, 0.9396926207859113145 ) ) ;
#68107=CARTESIAN_POINT ( 'NONE',  ( -8.703064162639128298, -7.250054591869670162, 34.99404684341514127 ) ) ;
#68108=B_SPLINE_CURVE_WITH_KNOTS ( 'NONE', 3,
 ( #66073, #86830, #80044, #18344, #45806, #73289 ),
 .UNSPECIFIED., .F., .F.,
 ( 4, 2, 4 ),
 ( 0.0003909512603273928395, 0.0005862562993132216203, 0.0007815613382990504012 ),
 .UNSPECIFIED. ) ;
#68109=VERTEX_POINT ( 'NONE', #29201 ) ;
#68111=CARTESIAN_POINT ( 'NONE',  ( 11.40831356872983982, -2.647304123082328875, 31.75400227202885972 ) ) ;
#68112=ORIENTED_EDGE ( 'NONE', *, *, #48862, .T. ) ;
#68113=CYLINDRICAL_SURFACE ( 'NONE', #7338, 0.2500000000000012212 ) ;
#68114=CARTESIAN_POINT ( 'NONE',  ( -11.28840722682322628, -12.41262288849542017, 30.68299917996395010 ) ) ;
#68115=ADVANCED_FACE ( 'NONE', ( #56654 ), #83703, .F. ) ;
#68116=DIRECTION ( 'NONE',  ( -0.000000000000000000, -0.9848077530122086864, -0.1736481776669273613 ) ) ;
#68117=EDGE_CURVE ( 'NONE', #24060, #87089, #69120, .T. ) ;
#68119=CARTESIAN_POINT ( 'NONE',  ( -0.6844654204453102242, -11.43668979543635089, 33.22377378376089752 ) ) ;
#68120=VECTOR ( 'NONE', #5094, 1000.000000000000000 ) ;
#68121=ORIENTED_EDGE ( 'NONE', *, *, #58053, .F. ) ;
#68122=CARTESIAN_POINT ( 'NONE',  ( -3.930833309752758797, -12.38742843783360748, 31.66772728687926985 ) ) ;
#68123=ORIENTED_EDGE ( 'NONE', *, *, #42638, .F. ) ;
#68124=CARTESIAN_POINT ( 'NONE',  ( -8.638705067467205012, -4.459921816937791661, 33.71989282347011851 ) ) ;
#68125=AXIS2_PLACEMENT_3D ( 'NONE', #73526, #10930, #3715 ) ;
#68126=DIRECTION ( 'NONE',  ( -0.000000000000000000, -0.3420201433256694901, -0.9396926207859082059 ) ) ;
#68127=CARTESIAN_POINT ( 'NONE',  ( 18.06525557127602255, -12.27809138561124591, 31.22303859784720359 ) ) ;
#68128=CARTESIAN_POINT ( 'NONE',  ( -20.75000000000000000, -12.50000000000000000, 29.75000000000000355 ) ) ;
#68129=CARTESIAN_POINT ( 'NONE',  ( 17.07692307692295586, -2.625532179533778709, 30.86335684631627174 ) ) ;
#68130=ORIENTED_EDGE ( 'NONE', *, *, #59933, .F. ) ;
#68131=ORIENTED_EDGE ( 'NONE', *, *, #53833, .T. ) ;
#68134=CARTESIAN_POINT ( 'NONE',  ( 14.98079248672063990, -3.436278759898153901, 33.07459398097509506 ) ) ;
#68135=CARTESIAN_POINT ( 'NONE',  ( 1.634560902963529294, -3.712312575010499938, 33.01462480002815170 ) ) ;
#68136=CARTESIAN_POINT ( 'NONE',  ( 6.249945518348142492, -12.22109172314383052, 31.39792113162168263 ) ) ;
#68137=CARTESIAN_POINT ( 'NONE',  ( 17.74997676270703550, -10.05641848906368097, 34.04755513067966177 ) ) ;
#68138=CARTESIAN_POINT ( 'NONE',  ( -5.076923076923075762, -8.120952969808772792, 34.71129190930000163 ) ) ;
#68139=FACE_OUTER_BOUND ( 'NONE', #1789, .T. ) ;
#68140=CARTESIAN_POINT ( 'NONE',  ( -5.299849294439222369, -3.586966769969700763, 32.86292498521069660 ) ) ;
#68141=ORIENTED_EDGE ( 'NONE', *, *, #62549, .F. ) ;
#68142=EDGE_CURVE ( 'NONE', #75030, #603, #71341, .T. ) ;
#68143=ORIENTED_EDGE ( 'NONE', *, *, #48272, .F. ) ;
#68144=VERTEX_POINT ( 'NONE', #52104 ) ;
#68145=CARTESIAN_POINT ( 'NONE',  ( -18.00000000000000000, -8.563426751879235965, 35.78099280442780383 ) ) ;
#68146=VECTOR ( 'NONE', #59720, 1000.000000000000000 ) ;
#68147=CARTESIAN_POINT ( 'NONE',  ( -20.75000000000000000, -2.499999999999999556, 29.75000000000000355 ) ) ;
#68148=CARTESIAN_POINT ( 'NONE',  ( -7.780898706641007578, -9.528491918058460186, 34.59228464037086326 ) ) ;
#68149=EDGE_CURVE ( 'NONE', #13706, #42649, #49814, .T. ) ;
#68150=CARTESIAN_POINT ( 'NONE',  ( 16.28389376010183653, -7.723484964179501588, 34.74522123443823318 ) ) ;
#68151=CARTESIAN_POINT ( 'NONE',  ( -10.68146802634049486, -3.513871655860377086, 32.76840700105978499 ) ) ;
#68152=FACE_BOUND ( 'NONE', #75830, .T. ) ;
#68153=ORIENTED_EDGE ( 'NONE', *, *, #52963, .F. ) ;
#68154=CARTESIAN_POINT ( 'NONE',  ( -1.161604033002535230, -2.758310577978207334, 31.33698337089302299 ) ) ;
#68155=CARTESIAN_POINT ( 'NONE',  ( -3.230769230769351186, -6.879047030192662504, 34.71129190930017927 ) ) ;
#68157=EDGE_CURVE ( 'NONE', #14741, #48597, #31398, .T. ) ;
#68159=ORIENTED_EDGE ( 'NONE', *, *, #20498, .T. ) ;
#68160=FACE_BOUND ( 'NONE', #37635, .T. ) ;
#68162=EDGE_LOOP ( 'NONE', ( #9071, #85875 ) ) ;
#68163=CARTESIAN_POINT ( 'NONE',  ( -12.39547011053602432, -8.120952969808772792, 34.71129190929999453 ) ) ;
#68165=DIRECTION ( 'NONE',  ( 0.000000000000000000, 0.7660444431189807890, 0.6427876096865361433 ) ) ;
#68166=VERTEX_POINT ( 'NONE', #79593 ) ;
#68169=LINE ( 'NONE', #20425, #59588 ) ;
#68170=CARTESIAN_POINT ( 'NONE',  ( -7.912237257109724808, -2.721908614388770964, 31.22303859784723912 ) ) ;
#68171=EDGE_LOOP ( 'NONE', ( #47647, #172 ) ) ;
#68172=EDGE_CURVE ( 'NONE', #20922, #76970, #16995, .T. ) ;
#68173=CARTESIAN_POINT ( 'NONE',  ( -4.854143407945010757, -4.989023458446560255, 34.36081565061822118 ) ) ;
#68174=CARTESIAN_POINT ( 'NONE',  ( 2.307692307692186251, -3.643525952248796163, 33.31231777344771672 ) ) ;
#68175=CARTESIAN_POINT ( 'NONE',  ( 1.607628228708781748, -2.889357225399415086, 32.26129605718031002 ) ) ;
#68176=VERTEX_POINT ( 'NONE', #3471 ) ;
#68177=CARTESIAN_POINT ( 'NONE',  ( -13.38461538461538325, -1.629998284177014645, 34.34916445242399163 ) ) ;
#68178=CARTESIAN_POINT ( 'NONE',  ( 9.626554263994364646, -7.249945578846651806, 34.99404164642496795 ) ) ;
#68179=CARTESIAN_POINT ( 'NONE',  ( -13.13466986626724342, -5.057305518903948638, 34.11320923018887896 ) ) ;
#68180=CARTESIAN_POINT ( 'NONE',  ( 13.44987095589141113, -12.46129190930001052, 30.37095296980870174 ) ) ;
#68182=CARTESIAN_POINT ( 'NONE',  ( 16.82694633287449193, -4.818429247618089661, 34.26397095200675125 ) ) ;
#68183=COLOUR_RGB ( '', 0.31764706, 0.68627451, 0.89019608) ;
#68184=CARTESIAN_POINT ( 'NONE',  ( 5.076923076922953193, -5.941354392335915335, 34.76329471203413846 ) ) ;
#68186=CARTESIAN_POINT ( 'NONE',  ( -16.94613126909829148, -8.147973898785416225, 34.70805048591653730 ) ) ;
#68187=CARTESIAN_POINT ( 'NONE',  ( -8.769230769230768274, -8.564572088678739092, 35.78748833219616898 ) ) ;
#68189=VERTEX_POINT ( 'NONE', #43576 ) ;
#68192=CYLINDRICAL_SURFACE ( 'NONE', #70666, 0.2499999999999997502 ) ;
#68193=ORIENTED_EDGE ( 'NONE', *, *, #13372, .T. ) ;
#68194=EDGE_LOOP ( 'NONE', ( #32778, #85689, #42337, #9193 ) ) ;
#68195=EDGE_CURVE ( 'NONE', #15069, #18273, #68268, .T. ) ;
#68197=ORIENTED_EDGE ( 'NONE', *, *, #2075, .F. ) ;
#68198=CARTESIAN_POINT ( 'NONE',  ( 1.634560793993429240, -12.07971442181322352, 32.31769673815850297 ) ) ;
#68200=CARTESIAN_POINT ( 'NONE',  ( 17.93391762063986050, -4.661471528628507777, 34.16647553114621871 ) ) ;
#68201=CARTESIAN_POINT ( 'NONE',  ( -16.15384615384615330, -10.05456864172156806, 36.03766855953608683 ) ) ;
#68202=CARTESIAN_POINT ( 'NONE',  ( -16.08859058257012720, -6.026961402152789304, 34.52809138561124769 ) ) ;
#68203=DIRECTION ( 'NONE',  ( 0.000000000000000000, 1.000000000000000000, 0.000000000000000000 ) ) ;
#68204=CARTESIAN_POINT ( 'NONE',  ( -13.60810032833933292, -2.599994579823203367, 30.74605699353653776 ) ) ;
#68205=CARTESIAN_POINT ( 'NONE',  ( 2.530471848960717196, -11.41317474335729187, 32.86274602512330034 ) ) ;
#68208=CARTESIAN_POINT ( 'NONE',  ( -13.38461538461538325, -6.386643153685126251, 34.62446782046654192 ) ) ;
#68209=EDGE_CURVE ( 'NONE', #28816, #28226, #37705, .T. ) ;
#68211=B_SPLINE_CURVE_WITH_KNOTS ( 'NONE', 3,
 ( #16799, #30757, #57351, #44253, #9602, #70875, #71739, #10044, #64978, #78951 ),
 .UNSPECIFIED., .F., .F.,
 ( 4, 2, 2, 2, 4 ),
 ( 0.0007817246256747473893, 0.0009771112852218900684, 0.001172497944769032964, 0.001367884604316175860, 0.001563271263863318539 ),
 .UNSPECIFIED. ) ;
#68212=ORIENTED_EDGE ( 'NONE', *, *, #57952, .T. ) ;
#68213=ORIENTED_EDGE ( 'NONE', *, *, #20280, .F. ) ;
#68214=CARTESIAN_POINT ( 'NONE',  ( -15.16551365949320562, -8.613356846314928816, 34.62446782046653482 ) ) ;
#68215=CARTESIAN_POINT ( 'NONE',  ( 0.7115928814519144607, -12.01375889529407637, 32.43194544308182969 ) ) ;
#68217=DIRECTION ( 'NONE',  ( -0.000000000000000000, 0.9396926207859092051, -0.3420201433256662704 ) ) ;
#68219=EDGE_CURVE ( 'NONE', #74128, #58471, #17444, .T. ) ;
#68220=CARTESIAN_POINT ( 'NONE',  ( 3.230769230769231726, -4.661471528628507777, 34.16647553114623292 ) ) ;
#68222=B_SPLINE_CURVE_WITH_KNOTS ( 'NONE', 3,
 ( #20538, #68728, #7023, #42595, #34498, #21428, #56099, #14675, #69174, #61962 ),
 .UNSPECIFIED., .F., .F.,
 ( 4, 2, 2, 2, 4 ),
 ( 0.0007817246256747461966, 0.0009771112852218892010, 0.001172497944769032314, 0.001367884604316175427, 0.001563271263863318323 ),
 .UNSPECIFIED. ) ;
#68223=EDGE_CURVE ( 'NONE', #4955, #84646, #25095, .T. ) ;
#68224=EDGE_CURVE ( 'NONE', #80982, #27279, #73443, .T. ) ;
#68225=ORIENTED_EDGE ( 'NONE', *, *, #45952, .T. ) ;
#68226=DIRECTION ( 'NONE',  ( 0.000000000000000000, 0.8660254037844377084, -0.5000000000000015543 ) ) ;
#68227=ORIENTED_EDGE ( 'NONE', *, *, #42740, .T. ) ;
#68228=EDGE_CURVE ( 'NONE', #28534, #65186, #7864, .T. ) ;
#68230=CARTESIAN_POINT ( 'NONE',  ( -14.37344911020661620, -7.249945686854186278, 34.74374336980224598 ) ) ;
#68231=CARTESIAN_POINT ( 'NONE',  ( -9.692307692307691624, -1.466349020453238561, 30.81389545987213907 ) ) ;
#68233=CARTESIAN_POINT ( 'NONE',  ( 3.007842271862381622, -8.282780595021769443, 34.94152052738834868 ) ) ;
#68234=CARTESIAN_POINT ( 'NONE',  ( -17.07692307692307665, -3.669653830205710676, 35.88435417666054406 ) ) ;
#68235=VERTEX_POINT ( 'NONE', #39947 ) ;
#68236=ORIENTED_EDGE ( 'NONE', *, *, #59918, .F. ) ;
#68237=ORIENTED_EDGE ( 'NONE', *, *, #58527, .T. ) ;
#68238=VERTEX_POINT ( 'NONE', #61085 ) ;
#68240=CARTESIAN_POINT ( 'NONE',  ( -6.223484924564330001, -4.988325925672468131, 34.36044203135681130 ) ) ;
#68241=CARTESIAN_POINT ( 'NONE',  ( -16.02332071561251325, -9.503571793651730104, 34.60286762892837942 ) ) ;
#68242=CARTESIAN_POINT ( 'NONE',  ( 14.17700170458200581, -2.494641256782728966, 31.33461815524612959 ) ) ;
#68244=CARTESIAN_POINT ( 'NONE',  ( 2.084207363968361815, -11.41268669641500466, 32.86336882939237825 ) ) ;
#68245=CARTESIAN_POINT ( 'NONE',  ( 17.86930853333243974, -4.809359713505814149, 33.96456829005828837 ) ) ;
#68246=CARTESIAN_POINT ( 'NONE',  ( -10.39237326377176274, -12.15243808032446005, 31.58219941686247978 ) ) ;
#68248=EDGE_LOOP ( 'NONE', ( #52686, #54574 ) ) ;
#68249=ORIENTED_EDGE ( 'NONE', *, *, #55165, .F. ) ;
#68250=CARTESIAN_POINT ( 'NONE',  ( 11.31497659473759043, -9.331801661448606566, 34.40259984581193464 ) ) ;
#68251=EDGE_LOOP ( 'NONE', ( #55263, #44651 ) ) ;
#68253=CARTESIAN_POINT ( 'NONE',  ( -12.23852561744506673, -11.98016756924215009, 32.48728574198911190 ) ) ;
#68255=ORIENTED_EDGE ( 'NONE', *, *, #80910, .T. ) ;
#68256=CARTESIAN_POINT ( 'NONE',  ( 8.769230769230768274, -6.435427911321262684, 35.78748833219616898 ) ) ;
#68257=ORIENTED_EDGE ( 'NONE', *, *, #42333, .T. ) ;
#68258=CARTESIAN_POINT ( 'NONE',  ( 8.069165197766697162, -12.15243808032445827, 31.58219941686247978 ) ) ;
#68259=FACE_BOUND ( 'NONE', #49803, .T. ) ;
#68260=CARTESIAN_POINT ( 'NONE',  ( -4.826977558574935934, -12.22109172314383052, 31.39792113162168263 ) ) ;
#68261=CARTESIAN_POINT ( 'NONE',  ( 8.519207531937803779, -5.056417327199099532, 34.11270091957321426 ) ) ;
#68262=ORIENTED_EDGE ( 'NONE', *, *, #68050, .T. ) ;
#68263=CARTESIAN_POINT ( 'NONE',  ( -9.942284436356285227, -4.818429247618089661, 34.26397095200675125 ) ) ;
#68264=CARTESIAN_POINT ( 'NONE',  ( -9.019230769230768274, -2.249999999999998668, 29.75000000000000355 ) ) ;
#68265=CARTESIAN_POINT ( 'NONE',  ( -13.13461538461544897, -7.565270445406050648, 34.75000000000000000 ) ) ;
#68266=CARTESIAN_POINT ( 'NONE',  ( 14.08420738312798015, -9.417330523894424488, 34.63758898049880486 ) ) ;
#68267=ORIENTED_EDGE ( 'NONE', *, *, #31233, .T. ) ;
#68268=CIRCLE ( 'NONE', #39555, 2.000000000000001776 ) ;
#68269=CARTESIAN_POINT ( 'NONE',  ( -0.7115384615384606759, -7.500000000000001776, 35.00000000000000000 ) ) ;
#68270=CARTESIAN_POINT ( 'NONE',  ( -4.087778820496077437, -9.905515769479277921, 34.41647553114623292 ) ) ;
#68271=CARTESIAN_POINT ( 'NONE',  ( 17.07692307692307665, -9.780366693483667717, 34.19971097300155094 ) ) ;
#68272=FACE_OUTER_BOUND ( 'NONE', #9021, .T. ) ;
#68273=CARTESIAN_POINT ( 'NONE',  ( -10.61538461538461320, -8.318370150425687726, 35.83090037661290239 ) ) ;
#68274=FACE_BOUND ( 'NONE', #39572, .T. ) ;
#68275=CARTESIAN_POINT ( 'NONE',  ( 1.134615384615387246, -7.566082377512563184, 35.00000000000000711 ) ) ;
#68276=CARTESIAN_POINT ( 'NONE',  ( 17.01084069756293715, -2.833524468853757305, 32.15551576947924417 ) ) ;
#68277=CARTESIAN_POINT ( 'NONE',  ( -5.999999999999998224, -2.249999999999998668, 29.50000000000001421 ) ) ;
#68278=CARTESIAN_POINT ( 'NONE',  ( -8.703975197954745724, -11.94971097300157403, 32.03036669348361443 ) ) ;
#68279=CARTESIAN_POINT ( 'NONE',  ( -9.469528151039277475, -10.81320215134717344, 33.49497208177562868 ) ) ;
#68280=CARTESIAN_POINT ( 'NONE',  ( -7.846153846153844924, -3.937682226553329556, 33.60647404775216529 ) ) ;
#68282=ORIENTED_EDGE ( 'NONE', *, *, #11310, .T. ) ;
#68283=B_SPLINE_CURVE_WITH_KNOTS ( 'NONE', 3,
 ( #27085, #13571, #69848, #47800, #21210, #55003, #69407, #48678, #82043, #76151 ),
 .UNSPECIFIED., .F., .F.,
 ( 4, 2, 2, 2, 4 ),
 ( 0.000000000000000000, 0.0001954339857564073388, 0.0003908679715128146777, 0.0005863019572692220165, 0.0007817359430256293554 ),
 .UNSPECIFIED. ) ;
#68285=ORIENTED_EDGE ( 'NONE', *, *, #55304, .T. ) ;
#68286=ADVANCED_FACE ( 'NONE', ( #33176 ), #88151, .F. ) ;
#68287=CARTESIAN_POINT ( 'NONE',  ( -18.25002322422145085, -3.520140089381496917, 33.17453946501457551 ) ) ;
#68288=ORIENTED_EDGE ( 'NONE', *, *, #1182, .F. ) ;
#68290=CARTESIAN_POINT ( 'NONE',  ( -16.08859101433330707, -12.16647553114626490, 32.15551576947920864 ) ) ;
#68291=CARTESIAN_POINT ( 'NONE',  ( -4.853910232829680815, -9.172514111537584114, 34.72667873470787470 ) ) ;
#68293=CARTESIAN_POINT ( 'NONE',  ( -15.45369544828537656, -4.887634598454295265, 34.01352882383564946 ) ) ;
#68295=CARTESIAN_POINT ( 'NONE',  ( -10.48485917715097138, -12.70449254468099198, 30.44128974285582956 ) ) ;
#68296=CARTESIAN_POINT ( 'NONE',  ( 7.846153846153846700, -13.75783147151868846, 33.36296068462461051 ) ) ;
#68297=CARTESIAN_POINT ( 'NONE',  ( -5.076923076923075762, -12.37446782046654192, 30.86335684631486131 ) ) ;
#68298=CARTESIAN_POINT ( 'NONE',  ( 3.903822916553188804, -11.86270091957321249, 32.19358267280087915 ) ) ;
#68299=CYLINDRICAL_SURFACE ( 'NONE', #13742, 0.2500000000000004996 ) ;
#68300=DIRECTION ( 'NONE',  ( -0.000000000000000000, 0.1736481776669307198, -0.9848077530122080203 ) ) ;
#68301=B_SPLINE_CURVE_WITH_KNOTS ( 'NONE', 3,
 ( #35830, #50201, #65051, #70494, #30394, #3360, #63285, #17326, #77686, #44783 ),
 .UNSPECIFIED., .F., .F.,
 ( 4, 2, 2, 2, 4 ),
 ( 0.0007817359430256320659, 0.0009771253907249987086, 0.001172514838424365460, 0.001367904286123731994, 0.001563293733823098745 ),
 .UNSPECIFIED. ) ;
#68303=VECTOR ( 'NONE', #25161, 1000.000000000000000 ) ;
#68304=CARTESIAN_POINT ( 'NONE',  ( 3.480769230770650147, -7.500000000000154543, 35.00000000000007105 ) ) ;
#68305=ADVANCED_FACE ( 'NONE', ( #39062 ), #60196, .F. ) ;
#68306=B_SPLINE_CURVE_WITH_KNOTS ( 'NONE', 3,
 ( #18131, #86148, #23535, #71721, #38394, #59547, #52788, #9583, #10483, #65415 ),
 .UNSPECIFIED., .F., .F.,
 ( 4, 2, 2, 2, 4 ),
 ( 0.000000000000000000, 0.0001954311564186871184, 0.0003908623128373742367, 0.0005862934692560614093, 0.0007817246256747484735 ),
 .UNSPECIFIED. ) ;
#68308=DIRECTION ( 'NONE',  ( -0.000000000000000000, -0.000000000000000000, -1.000000000000000000 ) ) ;
#68310=AXIS2_PLACEMENT_3D ( 'NONE', #41384, #88268, #68850 ) ;
#68311=CARTESIAN_POINT ( 'NONE',  ( -16.08777882049607655, -12.34228464037088813, 31.77849191805839268 ) ) ;
#68312=CARTESIAN_POINT ( 'NONE',  ( 17.29970261819148902, -11.89424750095246175, 32.13594075562311758 ) ) ;
#68313=ORIENTED_EDGE ( 'NONE', *, *, #64813, .F. ) ;
#68314=DIRECTION ( 'NONE',  ( 0.000000000000000000, -6.938893903907222067E-15, 1.000000000000000000 ) ) ;
#68315=CARTESIAN_POINT ( 'NONE',  ( 6.923076923076802558, -11.48612834414049644, 32.76840700105863391 ) ) ;
#68317=ORIENTED_EDGE ( 'NONE', *, *, #40594, .F. ) ;
#68318=CARTESIAN_POINT ( 'NONE',  ( 8.545745844666438273, -5.827078755546623690, 34.72654668319379567 ) ) ;
#68319=CARTESIAN_POINT ( 'NONE',  ( 2.242421861731532573, -12.46129190929999986, 30.37095296980880832 ) ) ;
#68320=CARTESIAN_POINT ( 'NONE',  ( 15.93036121012220541, -9.331801661448606566, 34.40259984581193464 ) ) ;
#68321=CARTESIAN_POINT ( 'NONE',  ( 15.23076923076911093, -2.625532179533778709, 30.86335684631627174 ) ) ;
#68322=CARTESIAN_POINT ( 'NONE',  ( -13.51530685128294174, -11.71456829005830080, 32.44064028649416542 ) ) ;
#68323=EDGE_CURVE ( 'NONE', #18936, #36238, #45512, .T. ) ;
#68325=CARTESIAN_POINT ( 'NONE',  ( -13.13456096470193302, -8.346898887586323923, 34.93166121998716278 ) ) ;
#68326=EDGE_LOOP ( 'NONE', ( #39704, #20787, #57471, #3890 ) ) ;
#68327=ORIENTED_EDGE ( 'NONE', *, *, #48257, .T. ) ;
#68328=EDGE_LOOP ( 'NONE', ( #40579, #15454 ) ) ;
#68329=VERTEX_POINT ( 'NONE', #80485 ) ;
#68331=CARTESIAN_POINT ( 'NONE',  ( -13.51476259405360558, -3.817052484675422797, 33.13202310037935661 ) ) ;
#68332=CARTESIAN_POINT ( 'NONE',  ( 14.08476609017615644, -4.186968288167450147, 33.49512374952580274 ) ) ;
#68334=CARTESIAN_POINT ( 'NONE',  ( 4.153846153846030731, -12.70778746994576025, 30.41441678777401236 ) ) ;
#68336=B_SPLINE_CURVE_WITH_KNOTS ( 'NONE', 3,
 ( #37430, #4998, #37889, #59038, #59930, #30681, #73004, #31572, #80669, #86993 ),
 .UNSPECIFIED., .F., .F.,
 ( 4, 2, 2, 2, 4 ),
 ( 0.000000000000000000, 0.0001954339857564092362, 0.0003908679715128184724, 0.0005863019572692276544, 0.0007817359430256369448 ),
 .UNSPECIFIED. ) ;
#68337=VECTOR ( 'NONE', #70285, 1000.000000000000227 ) ;
#68338=LINE ( 'NONE', #47169, #19010 ) ;
#68339=B_SPLINE_CURVE_WITH_KNOTS ( 'NONE', 3,
 ( #12623, #25242, #38314, #18047, #10843, #46401, #73439, #86518, #11737, #87407 ),
 .UNSPECIFIED., .F., .F.,
 ( 4, 2, 2, 2, 4 ),
 ( 0.0007817246256747461966, 0.0009771112852218889842, 0.001172497944769031880, 0.001367884604316174776, 0.001563271263863317672 ),
 .UNSPECIFIED. ) ;
#68340=ORIENTED_EDGE ( 'NONE', *, *, #18625, .T. ) ;
#68341=ORIENTED_EDGE ( 'NONE', *, *, #79189, .F. ) ;
#68342=ORIENTED_EDGE ( 'NONE', *, *, #82182, .T. ) ;
#68343=CARTESIAN_POINT ( 'NONE',  ( -7.173100147298383078, -2.588893531581426544, 31.60682220781847818 ) ) ;
#68344=ORIENTED_EDGE ( 'NONE', *, *, #6097, .F. ) ;
#68345=CARTESIAN_POINT ( 'NONE',  ( -5.076923076923075762, -12.34228464037088635, 31.77849191805839268 ) ) ;
#68346=CARTESIAN_POINT ( 'NONE',  ( 6.249945409378044658, -2.589246495874657938, 31.60778113518102828 ) ) ;
#68347=CARTESIAN_POINT ( 'NONE',  ( -12.46153846153846168, -12.10708131394839349, 31.69288490824020244 ) ) ;
#68349=ORIENTED_EDGE ( 'NONE', *, *, #2471, .T. ) ;
#68351=ORIENTED_EDGE ( 'NONE', *, *, #17549, .T. ) ;
#68352=CARTESIAN_POINT ( 'NONE',  ( -5.207533436547604921, -7.722926236386453702, 34.74524107206102030 ) ) ;
#68353=CARTESIAN_POINT ( 'NONE',  ( 17.07692307692295586, -12.16647553114689728, 32.15551576947799362 ) ) ;
#68354=ORIENTED_EDGE ( 'NONE', *, *, #66459, .F. ) ;
#68355=CARTESIAN_POINT ( 'NONE',  ( 13.13461538461538858, -2.499999999999999556, 29.81609845454691765 ) ) ;
#68356=CARTESIAN_POINT ( 'NONE',  ( 1.384615384615386802, -8.120952969808772792, 34.71129190930000163 ) ) ;
#68358=CARTESIAN_POINT ( 'NONE',  ( 16.15384615384603251, -3.835265460704628815, 33.15142922262033665 ) ) ;
#68359=CARTESIAN_POINT ( 'NONE',  ( 12.71148387091650278, -9.357781135181031829, 34.66075350412533851 ) ) ;
#68360=FACE_BOUND ( 'NONE', #85452, .T. ) ;
#68361=LINE ( 'NONE', #27383, #71527 ) ;
#68362=CARTESIAN_POINT ( 'NONE',  ( -6.066082379360135945, -12.34228464037088280, 31.77849191805838558 ) ) ;
#68364=B_SPLINE_CURVE_WITH_KNOTS ( 'NONE', 3,
 ( #63323, #75510, #21456, #54791, #82726, #35864, #8837, #42184, #68757, #69201 ),
 .UNSPECIFIED., .F., .F.,
 ( 4, 2, 2, 2, 4 ),
 ( 0.0007817246256747497745, 0.0009771112852218937547, 0.001172497944769037518, 0.001367884604316181498, 0.001563271263863325478 ),
 .UNSPECIFIED. ) ;
#68365=CARTESIAN_POINT ( 'NONE',  ( 0.7115384615398802071, -7.500000000000154543, 35.00000000000007105 ) ) ;
#68366=DIRECTION ( 'NONE',  ( -1.000000000000000000, 0.000000000000000000, 0.000000000000000000 ) ) ;
#68367=CARTESIAN_POINT ( 'NONE',  ( -4.023054346021369021, -2.729792928343270919, 31.24908615093345077 ) ) ;
#68368=CARTESIAN_POINT ( 'NONE',  ( -4.023320715612509701, -11.66157788607254275, 32.95092075102925833 ) ) ;
#68369=ORIENTED_EDGE ( 'NONE', *, *, #35874, .F. ) ;
#68371=AXIS2_PLACEMENT_3D ( 'NONE', #14288, #41770, #21484 ) ;
#68372=CARTESIAN_POINT ( 'NONE',  ( 13.63461538461544897, -7.434744429011176159, 34.75000000000000711 ) ) ;
#68373=B_SPLINE_CURVE_WITH_KNOTS ( 'NONE', 3,
 ( #46054, #65869, #30758, #85717, #4175, #59117 ),
 .UNSPECIFIED., .F., .F.,
 ( 4, 2, 4 ),
 ( 0.0003909512603273990194, 0.0005862562993132244393, 0.0007815613382990498591 ),
 .UNSPECIFIED. ) ;
#68374=VERTEX_POINT ( 'NONE', #12462 ) ;
#68375=EDGE_CURVE ( 'NONE', #43958, #80807, #77731, .T. ) ;
#68376=CARTESIAN_POINT ( 'NONE',  ( -15.48074596171158213, -2.564618984488975073, 30.55390908950641915 ) ) ;
#68377=CARTESIAN_POINT ( 'NONE',  ( 9.442330961365341224, -2.779195860258146578, 31.39871582349836032 ) ) ;
#68379=CARTESIAN_POINT ( 'NONE',  ( 11.28843831424008570, -10.18141759479407327, 34.26406193332782379 ) ) ;
#68380=CYLINDRICAL_SURFACE ( 'NONE', #83213, 0.2500000000000009437 ) ;
#68381=FACE_BOUND ( 'NONE', #50212, .T. ) ;
#68382=CARTESIAN_POINT ( 'NONE',  ( -14.43838291080261627, -3.957541250942358424, 33.62499894934981626 ) ) ;
#68383=CARTESIAN_POINT ( 'NONE',  ( 4.023155550735846298, -12.35290016733513951, 31.75349464988449455 ) ) ;
#68384=CARTESIAN_POINT ( 'NONE',  ( 2.242422307135989890, -6.835583212224499938, 34.95778746994557906 ) ) ;
#68385=CARTESIAN_POINT ( 'NONE',  ( 2.557637826040450424, -5.057305518903949526, 34.11320923018887896 ) ) ;
#68387=CARTESIAN_POINT ( 'NONE',  ( 2.177001704582002262, -10.70098750199973203, 33.91152734681376302 ) ) ;
#68389=VERTEX_POINT ( 'NONE', #6150 ) ;
#68390=ORIENTED_EDGE ( 'NONE', *, *, #74524, .T. ) ;
#68391=EDGE_CURVE ( 'NONE', #23252, #60384, #20107, .T. ) ;
#68392=CARTESIAN_POINT ( 'NONE',  ( -12.46153846153858424, -5.941354392335915335, 34.76329471203413846 ) ) ;
#68393=CARTESIAN_POINT ( 'NONE',  ( -10.55012947587177941, -8.656820664281605460, 34.87096338111211224 ) ) ;
#68394=CARTESIAN_POINT ( 'NONE',  ( 6.989243529668563326, -7.250054591869668386, 34.99404684341514127 ) ) ;
#68395=CARTESIAN_POINT ( 'NONE',  ( 10.61538461538449418, -3.083524468854526912, 32.58852847137268327 ) ) ;
#68397=CARTESIAN_POINT ( 'NONE',  ( 5.076923076922953193, -3.643525952248796163, 33.31231777344771672 ) ) ;
#68400=CARTESIAN_POINT ( 'NONE',  ( 1.134592160393929516, -10.18141759479407327, 34.26406193332782379 ) ) ;
#68401=VECTOR ( 'NONE', #21887, 1000.000000000000227 ) ;
#68402=CARTESIAN_POINT ( 'NONE',  ( 7.715463243043539698, -5.496505350115500121, 34.60290016733514307 ) ) ;
#68403=LINE ( 'NONE', #76044, #26676 ) ;
#68406=CARTESIAN_POINT ( 'NONE',  ( -3.480745974817821775, -10.06842814019191401, 34.32929386961144758 ) ) ;
#68407=CARTESIAN_POINT ( 'NONE',  ( -3.454254174493179175, -8.496056993536548418, 34.65000542017679663 ) ) ;
#68408=EDGE_CURVE ( 'NONE', #70248, #53579, #1497, .T. ) ;
#68409=CARTESIAN_POINT ( 'NONE',  ( 12.68431800280687050, -2.847695495035523550, 31.58253572463339154 ) ) ;
#68410=B_SPLINE_CURVE_WITH_KNOTS ( 'NONE', 3,
 ( #70868, #36203, #77170, #78052, #9168, #37498 ),
 .UNSPECIFIED., .F., .F.,
 ( 4, 2, 4 ),
 ( 4.221881728299276106E-17, 0.0001954756301637148241, 0.0003909512603273874185 ),
 .UNSPECIFIED. ) ;
#68411=EDGE_LOOP ( 'NONE', ( #58185, #30977, #21326, #31332 ) ) ;
#68412=CARTESIAN_POINT ( 'NONE',  ( -14.30769230769230660, -13.95598074871891292, 31.83374038241031911 ) ) ;
#68413=CARTESIAN_POINT ( 'NONE',  ( -4.153846153846152411, -1.117168528481311540, 33.14645433367849847 ) ) ;
#68416=CARTESIAN_POINT ( 'NONE',  ( -9.822455662039393687, -11.04286588640298561, 33.62463336215343901 ) ) ;
#68417=CARTESIAN_POINT ( 'NONE',  ( -5.749999999998578915, -7.500000000000154543, 35.00000000000007105 ) ) ;
#68418=CARTESIAN_POINT ( 'NONE',  ( -3.230769230769229949, -1.129524287112498415, 32.06866353760679544 ) ) ;
#68419=CARTESIAN_POINT ( 'NONE',  ( -14.37296275365308240, -12.27809138561121394, 31.22303859784730307 ) ) ;
#68423=EDGE_LOOP ( 'NONE', ( #77128, #60000 ) ) ;
#68424=CARTESIAN_POINT ( 'NONE',  ( -11.28846153846153655, -2.249999999999998668, 29.75000000000000355 ) ) ;
#68426=ORIENTED_EDGE ( 'NONE', *, *, #39774, .T. ) ;
#68428=CARTESIAN_POINT ( 'NONE',  ( 2.557746727605762160, -8.346898887586323923, 34.93166121998716278 ) ) ;
#68429=EDGE_CURVE ( 'NONE', #50723, #17200, #64074, .T. ) ;
#68430=DIRECTION ( 'NONE',  ( 1.000000000000000000, 0.000000000000000000, 0.000000000000000000 ) ) ;
#68431=ORIENTED_EDGE ( 'NONE', *, *, #31168, .T. ) ;
#68432=ADVANCED_FACE ( 'NONE', ( #85252 ), #48009, .F. ) ;
#68433=ORIENTED_EDGE ( 'NONE', *, *, #2614, .T. ) ;
#68434=CARTESIAN_POINT ( 'NONE',  ( 3.007842271862381178, -2.889293201056495786, 32.26117774369186009 ) ) ;
#68435=EDGE_LOOP ( 'NONE', ( #17367, #12515 ) ) ;
#68436=CARTESIAN_POINT ( 'NONE',  ( 3.480714640147273720, -12.07971442181321997, 32.31769673815850297 ) ) ;
#68437=EDGE_CURVE ( 'NONE', #3673, #31209, #43373, .T. ) ;
#68438=DIRECTION ( 'NONE',  ( -0.000000000000000000, 0.5000000000000011102, -0.8660254037844381525 ) ) ;
#68439=CYLINDRICAL_SURFACE ( 'NONE', #65935, 0.2500000000000004996 ) ;
#68440=EDGE_CURVE ( 'NONE', #48065, #51319, #75486, .T. ) ;
#68441=AXIS2_PLACEMENT_3D ( 'NONE', #81892, #6657, #82774 ) ;
#68442=CARTESIAN_POINT ( 'NONE',  ( -6.700064078983527516, -11.43677907613344757, 33.22367315496201456 ) ) ;
#68443=CARTESIAN_POINT ( 'NONE',  ( -7.846153846153844924, -12.29105614889573062, 35.45975837776705220 ) ) ;
#68444=CARTESIAN_POINT ( 'NONE',  ( 13.51540719244017374, -3.062576670634119758, 32.05464942895959979 ) ) ;
#68445=CARTESIAN_POINT ( 'NONE',  ( -12.59222992820602194, -6.413092428213692742, 34.63065189839063152 ) ) ;
#68446=VERTEX_POINT ( 'NONE', #78476 ) ;
#68447=ORIENTED_EDGE ( 'NONE', *, *, #25418, .F. ) ;
#68448=CARTESIAN_POINT ( 'NONE',  ( 6.923076923076800782, -12.70778746994576025, 30.41441678777401236 ) ) ;
#68449=ORIENTED_EDGE ( 'NONE', *, *, #70968, .T. ) ;
#68450=CARTESIAN_POINT ( 'NONE',  ( 7.846153846153846700, -2.486705287966279876, 31.30864560766543647 ) ) ;
#68451=AXIS2_PLACEMENT_3D ( 'NONE', #22976, #85573, #79263 ) ;
#68452=CARTESIAN_POINT ( 'NONE',  ( -8.769230769230892619, -11.06231777344772027, 33.60647404775119895 ) ) ;
#68453=CARTESIAN_POINT ( 'NONE',  ( 11.60371710973756620, -12.27809138561124591, 31.22303859784720359 ) ) ;
#68454=ORIENTED_EDGE ( 'NONE', *, *, #1561, .T. ) ;
#68455=CARTESIAN_POINT ( 'NONE',  ( -12.39628289026243557, -6.026961402152789304, 34.52809138561124769 ) ) ;
#68456=CIRCLE ( 'NONE', #38315, 2.000000000000001776 ) ;
#68457=ORIENTED_EDGE ( 'NONE', *, *, #62123, .F. ) ;
#68458=CYLINDRICAL_SURFACE ( 'NONE', #16589, 0.2500000000000002220 ) ;
#68459=EDGE_LOOP ( 'NONE', ( #56252, #88468 ) ) ;
#68460=DIRECTION ( 'NONE',  ( 0.000000000000000000, 0.7660444431189807890, 0.6427876096865361433 ) ) ;
#68462=ORIENTED_EDGE ( 'NONE', *, *, #33145, .F. ) ;
#68463=CARTESIAN_POINT ( 'NONE',  ( -4.283994123577849145, -4.299443229763728169, 33.91186481527756058 ) ) ;
#68464=CARTESIAN_POINT ( 'NONE',  ( -8.835314180186649935, -2.721908614388770964, 31.22303859784723912 ) ) ;
#68465=FACE_BOUND ( 'NONE', #76100, .T. ) ;
#68466=CARTESIAN_POINT ( 'NONE',  ( -0.4615384615385826339, -5.219633306517616589, 34.19971097300220464 ) ) ;
#68467=DIRECTION ( 'NONE',  ( -0.000000000000000000, -0.3420201433256694346, -0.9396926207859080948 ) ) ;
#68468=CARTESIAN_POINT ( 'NONE',  ( 9.442284468086237226, -11.56360843649121861, 33.07473185843129926 ) ) ;
#68472=CARTESIAN_POINT ( 'NONE',  ( 14.37375964104238335, -6.343179335718452272, 34.87096338111212646 ) ) ;
#68473=EDGE_LOOP ( 'NONE', ( #45394, #87846, #67090, #30520, #86648, #42010 ) ) ;
#68475=ORIENTED_EDGE ( 'NONE', *, *, #24115, .T. ) ;
#68476=EDGE_CURVE ( 'NONE', #73234, #10850, #372, .T. ) ;
#68477=CARTESIAN_POINT ( 'NONE',  ( 15.23076923076923173, -13.53365097954675988, 30.81389545987213552 ) ) ;
#68478=DIRECTION ( 'NONE',  ( -1.000000000000000000, 0.000000000000000000, 0.000000000000000000 ) ) ;
#68479=CARTESIAN_POINT ( 'NONE',  ( -9.692307692307691624, -12.34228464037088635, 31.77849191805839268 ) ) ;
#68480=DIRECTION ( 'NONE',  ( 0.000000000000000000, 0.3420201433256641055, -0.9396926207859100932 ) ) ;
#68481=CARTESIAN_POINT ( 'NONE',  ( -17.14300545628321260, -12.34228464037088280, 31.77849191805838558 ) ) ;
#68482=CARTESIAN_POINT ( 'NONE',  ( 11.53846153846153832, -10.89733346790207413, 36.13435417666054406 ) ) ;
#68483=EDGE_LOOP ( 'NONE', ( #76227, #57482 ) ) ;
#68485=CARTESIAN_POINT ( 'NONE',  ( -5.869474561766354626, -8.630441415882550871, 34.87705825610312615 ) ) ;
#68486=CARTESIAN_POINT ( 'NONE',  ( 11.78846153846297362, -7.500000000000155431, 34.75000000000007105 ) ) ;
#68487=CARTESIAN_POINT ( 'NONE',  ( 16.94623247381276343, -3.957541250942358424, 33.62499894934981626 ) ) ;
#68489=EDGE_LOOP ( 'NONE', ( #82298, #53067, #44595, #65384, #56778, #52606 ) ) ;
#68490=ORIENTED_EDGE ( 'NONE', *, *, #191, .F. ) ;
#68491=ORIENTED_EDGE ( 'NONE', *, *, #68707, .T. ) ;
#68492=EDGE_CURVE ( 'NONE', #69035, #81618, #29863, .T. ) ;
#68493=CARTESIAN_POINT ( 'NONE',  ( 15.45378058238208219, -6.503523203565941380, 34.64991518177335195 ) ) ;
#68494=ORIENTED_EDGE ( 'NONE', *, *, #88423, .F. ) ;
#68496=CARTESIAN_POINT ( 'NONE',  ( -15.93106661257773560, -5.114059244376869096, 34.14424750095245287 ) ) ;
#68497=CARTESIAN_POINT ( 'NONE',  ( -6.250023224221455287, -9.356822207818506598, 34.66110646841856635 ) ) ;
#68498=CARTESIAN_POINT ( 'NONE',  ( -5.207070286361298095, -4.460286881179643004, 33.72017969459903242 ) ) ;
#68499=EDGE_CURVE ( 'NONE', #57235, #1867, #87502, .T. ) ;
#68500=CARTESIAN_POINT ( 'NONE',  ( -2.241623956689868358, -4.786620604624113540, 33.94971097300155805 ) ) ;
#68501=B_SPLINE_CURVE_WITH_KNOTS ( 'NONE', 3,
 ( #22756, #21880, #2480, #2048, #16451, #84925, #70512, #63746, #64177, #3374 ),
 .UNSPECIFIED., .F., .F.,
 ( 4, 2, 2, 2, 4 ),
 ( 0.000000000000000000, 0.0001954339857564097512, 0.0003908679715128195024, 0.0005863019572692292807, 0.0007817359430256390048 ),
 .UNSPECIFIED. ) ;
#68502=CARTESIAN_POINT ( 'NONE',  ( 14.37294787896833448, -4.481592998940250538, 33.73612834413965089 ) ) ;
#68503=ORIENTED_EDGE ( 'NONE', *, *, #26181, .T. ) ;
#68505=CYLINDRICAL_SURFACE ( 'NONE', #18004, 0.2499999999999986955 ) ;
#68507=CARTESIAN_POINT ( 'NONE',  ( -4.153846153846152411, -1.242168528481310874, 33.36296068462461051 ) ) ;
#68508=CARTESIAN_POINT ( 'NONE',  ( 15.90384615384615330, -2.499999999999998668, 29.75000000000000355 ) ) ;
#68509=DIRECTION ( 'NONE',  ( -0.000000000000000000, -0.000000000000000000, -1.000000000000000000 ) ) ;
#68510=LINE ( 'NONE', #55440, #16486 ) ;
#68511=CARTESIAN_POINT ( 'NONE',  ( -14.30769230769242739, -6.879047030192662504, 34.71129190930017927 ) ) ;
#68512=CARTESIAN_POINT ( 'NONE',  ( 9.561616225640136690, -9.804603061927743113, 34.18744698557895845 ) ) ;
#68513=EDGE_CURVE ( 'NONE', #55920, #13845, #84373, .T. ) ;
#68514=CARTESIAN_POINT ( 'NONE',  ( -0.4615384615385826339, -12.46129190930018460, 30.37095296980731973 ) ) ;
#68516=ORIENTED_EDGE ( 'NONE', *, *, #6713, .T. ) ;
#68517=LINE ( 'NONE', #20776, #30208 ) ;
#68518=CARTESIAN_POINT ( 'NONE',  ( 0.6843180028068713838, -3.236590943229497697, 32.36255958852954251 ) ) ;
#68519=CARTESIAN_POINT ( 'NONE',  ( 9.823098133274644539, -10.70102852606553157, 33.91149625220312913 ) ) ;
#68521=EDGE_LOOP ( 'NONE', ( #13688, #38860, #10862, #36514 ) ) ;
#68523=CARTESIAN_POINT ( 'NONE',  ( -12.52680890749923925, -11.94971097300153140, 32.03036669348370680 ) ) ;
#68524=CARTESIAN_POINT ( 'NONE',  ( 11.40777093535123221, -12.62707690430377383, 30.88035979386743435 ) ) ;
#68525=VECTOR ( 'NONE', #69977, 1000.000000000000114 ) ;
#68526=CARTESIAN_POINT ( 'NONE',  ( 2.557746727605760384, -10.82426656108011720, 33.81400080652039009 ) ) ;
#68528=CARTESIAN_POINT ( 'NONE',  ( -14.53117723225663838, -3.019605429927184836, 32.48692288466676814 ) ) ;
#68529=ORIENTED_EDGE ( 'NONE', *, *, #16413, .F. ) ;
#68531=CARTESIAN_POINT ( 'NONE',  ( 5.999999999999880096, -6.026961402154118908, 34.52809138561165270 ) ) ;
#68532=ADVANCED_FACE ( 'NONE', ( #58203 ), #24415, .F. ) ;
#68534=FACE_OUTER_BOUND ( 'NONE', #53735, .T. ) ;
#68535=CARTESIAN_POINT ( 'NONE',  ( 17.07692307692307665, -13.87047571288749737, 32.06866353760679544 ) ) ;
#68536=ORIENTED_EDGE ( 'NONE', *, *, #14725, .T. ) ;
#68537=CARTESIAN_POINT ( 'NONE',  ( -17.07692307692319744, -12.16647553114689728, 32.15551576947799362 ) ) ;
#68539=VERTEX_POINT ( 'NONE', #32513 ) ;
#68540=CARTESIAN_POINT ( 'NONE',  ( 12.46153846153833911, -12.51329471203414379, 31.30864560766407578 ) ) ;
#68541=CARTESIAN_POINT ( 'NONE',  ( 11.78840694783958298, -6.653508905675592722, 34.93172785388651391 ) ) ;
#68543=EDGE_CURVE ( 'NONE', #70102, #83933, #78680, .T. ) ;
#68544=B_SPLINE_CURVE_WITH_KNOTS ( 'NONE', 3,
 ( #2184, #44487, #29675, #37298, #52143, #58903, #57136, #71977, #50800, #23341 ),
 .UNSPECIFIED., .F., .F.,
 ( 4, 2, 2, 2, 4 ),
 ( 0.0007817246256747516176, 0.0009771112852218965736, 0.001172497944769041638, 0.001367884604316186702, 0.001563271263863331550 ),
 .UNSPECIFIED. ) ;
#68545=CARTESIAN_POINT ( 'NONE',  ( 18.00000000000000000, -1.242168528481310874, 33.36296068462461051 ) ) ;
#68546=CARTESIAN_POINT ( 'NONE',  ( -8.769230769230890843, -2.625532179533778709, 30.86335684631627174 ) ) ;
#68547=CARTESIAN_POINT ( 'NONE',  ( 1.384615384615265343, -4.481592998941358097, 33.73612834414048933 ) ) ;
#68548=CARTESIAN_POINT ( 'NONE',  ( 11.47319153790522073, -12.51329471203370325, 31.30864560766548976 ) ) ;
#68549=CARTESIAN_POINT ( 'NONE',  ( 3.453548772037640546, -12.44528174975671853, 30.48912976160716681 ) ) ;
#68550=AXIS2_PLACEMENT_3D ( 'NONE', #4610, #32081, #25325 ) ;
#68551=EDGE_LOOP ( 'NONE', ( #64909, #62358, #11474, #18128 ) ) ;
#68552=FACE_BOUND ( 'NONE', #79552, .T. ) ;
#68553=ORIENTED_EDGE ( 'NONE', *, *, #41158, .F. ) ;
#68554=FACE_OUTER_BOUND ( 'NONE', #4072, .T. ) ;
#68555=ADVANCED_FACE ( 'NONE', ( #4145 ), #51421, .F. ) ;
#68556=CARTESIAN_POINT ( 'NONE',  ( 17.99999999999987566, -12.27809138561165270, 31.22303859784587132 ) ) ;
#68557=EDGE_CURVE ( 'NONE', #75533, #27477, #82994, .T. ) ;
#68559=DIRECTION ( 'NONE',  ( -0.000000000000000000, -0.8660254037844399289, -0.4999999999999980016 ) ) ;
#68560=CARTESIAN_POINT ( 'NONE',  ( 14.30769230769231015, -2.721908614388771852, 31.22303859784724978 ) ) ;
#68561=ORIENTED_EDGE ( 'NONE', *, *, #84542, .T. ) ;
#68562=ORIENTED_EDGE ( 'NONE', *, *, #36151, .T. ) ;
#68563=ORIENTED_EDGE ( 'NONE', *, *, #1439, .F. ) ;
#68564=LINE ( 'NONE', #1880, #87977 ) ;
#68565=VERTEX_POINT ( 'NONE', #3702 ) ;
#68566=ADVANCED_FACE ( 'NONE', ( #10919 ), #86594, .F. ) ;
#68568=B_SPLINE_CURVE_WITH_KNOTS ( 'NONE', 3,
 ( #47660, #68372, #14314, #35026, #34590, #41801, #69263, #75145, #7566, #62486 ),
 .UNSPECIFIED., .F., .F.,
 ( 4, 2, 2, 2, 4 ),
 ( 0.0007817359527651101701, 0.0009771254036996489256, 0.001172514854634187790, 0.001367904305568726653, 0.001563293756503265517 ),
 .UNSPECIFIED. ) ;
#68569=CYLINDRICAL_SURFACE ( 'NONE', #19506, 0.2499999999999986955 ) ;
#68571=CARTESIAN_POINT ( 'NONE',  ( 6.130791807824788719, -12.11778462344220841, 31.66786338562085135 ) ) ;
#68573=CARTESIAN_POINT ( 'NONE',  ( 5.076923076923075762, -3.886160181151819604, 36.00935417666054406 ) ) ;
#68574=VECTOR ( 'NONE', #28623, 1000.000000000000227 ) ;
#68575=CARTESIAN_POINT ( 'NONE',  ( -4.153846153846152411, -5.471508081941601098, 34.59228464037088457 ) ) ;
#68576=CARTESIAN_POINT ( 'NONE',  ( 15.23076923076923173, -13.20930481340135110, 34.54067556320372745 ) ) ;
#68577=CARTESIAN_POINT ( 'NONE',  ( 17.20744877868664346, -2.619367082507847666, 30.83698974864643461 ) ) ;
#68578=EDGE_LOOP ( 'NONE', ( #68064, #26504 ) ) ;
#68579=VERTEX_POINT ( 'NONE', #66301 ) ;
#68580=ORIENTED_EDGE ( 'NONE', *, *, #44242, .T. ) ;
#68581=CARTESIAN_POINT ( 'NONE',  ( -13.63463860883684120, -12.45566812827425451, 31.48439005359158926 ) ) ;
#68583=CARTESIAN_POINT ( 'NONE',  ( 0.4615384615384611200, -6.435427911321262684, 35.78748833219616898 ) ) ;
#68584=LINE ( 'NONE', #5116, #13186 ) ;
#68585=CARTESIAN_POINT ( 'NONE',  ( 1.384615384615264011, -12.51329471203414379, 31.30864560766407578 ) ) ;
#68586=DIRECTION ( 'NONE',  ( -0.000000000000000000, -0.1736481776669307198, -0.9848077530122080203 ) ) ;
#68587=FACE_BOUND ( 'NONE', #9405, .T. ) ;
#68588=CARTESIAN_POINT ( 'NONE',  ( -7.173053667125516064, -3.436278759898155677, 33.07459398097509506 ) ) ;
#68589=ORIENTED_EDGE ( 'NONE', *, *, #44498, .F. ) ;
#68592=DIRECTION ( 'NONE',  ( -0.000000000000000000, -0.5000000000000009992, -0.8660254037844380415 ) ) ;
#68593=CARTESIAN_POINT ( 'NONE',  ( -6.923076923076922462, -7.500000000000001776, 35.04278698407183867 ) ) ;
#68594=CARTESIAN_POINT ( 'NONE',  ( -3.361459833879539616, -3.338472653186242756, 32.95098750199972670 ) ) ;
#68595=ORIENTED_EDGE ( 'NONE', *, *, #41749, .T. ) ;
#68596=CARTESIAN_POINT ( 'NONE',  ( 17.14299041027315695, -5.471508081941601098, 34.59228464037088457 ) ) ;
#68597=EDGE_LOOP ( 'NONE', ( #40873, #29136 ) ) ;
#68598=FACE_BOUND ( 'NONE', #48895, .T. ) ;
#68599=DIRECTION ( 'NONE',  ( 0.000000000000000000, 0.6427876096865373645, -0.7660444431189797898 ) ) ;
#68600=B_SPLINE_CURVE_WITH_KNOTS ( 'NONE', 3,
 ( #3990, #65691, #44527, #78772, #23813, #2220, #43655, #51267, #9434, #64360 ),
 .UNSPECIFIED., .F., .F.,
 ( 4, 2, 2, 2, 4 ),
 ( 0.0007817246256747452209, 0.0009771112852218879000, 0.001172497944769030362, 0.001367884604316172825, 0.001563271263863315504 ),
 .UNSPECIFIED. ) ;
#68601=CARTESIAN_POINT ( 'NONE',  ( -6.065756802514307822, -7.249945686854186278, 34.74374336980224598 ) ) ;
#68602=CARTESIAN_POINT ( 'NONE',  ( 0.4615384615384611200, -3.886160181151819604, 36.00935417666054406 ) ) ;
#68603=EDGE_LOOP ( 'NONE', ( #85729, #67292 ) ) ;
#68604=CARTESIAN_POINT ( 'NONE',  ( 6.923076923076802558, -6.026961402154118908, 34.52809138561165270 ) ) ;
#68606=CARTESIAN_POINT ( 'NONE',  ( 18.22301284409339672, -10.77377354290276301, 33.85451476688484718 ) ) ;
#68608=CARTESIAN_POINT ( 'NONE',  ( 2.307692307692186251, -3.083524468854526912, 32.58852847137268327 ) ) ;
#68609=ORIENTED_EDGE ( 'NONE', *, *, #1208, .T. ) ;
#68610=DIRECTION ( 'NONE',  ( -0.000000000000000000, -0.6427876096865404731, -0.7660444431189770143 ) ) ;
#68611=CARTESIAN_POINT ( 'NONE',  ( 2.530705151785704654, -3.395485233115138168, 33.02377354290276656 ) ) ;
#68612=B_SPLINE_CURVE_WITH_KNOTS ( 'NONE', 3,
 ( #68155, #74919, #86787, #25057, #52519, #19518, #33485, #13212, #60945, #88450 ),
 .UNSPECIFIED., .F., .F.,
 ( 4, 2, 2, 2, 4 ),
 ( 0.0007817359430256306564, 0.0009771253907249969738, 0.001172514838424363291, 0.001367904286123729826, 0.001563293733823096143 ),
 .UNSPECIFIED. ) ;
#68613=CARTESIAN_POINT ( 'NONE',  ( -8.992156986746916658, -3.586966769969701208, 32.86292498521069660 ) ) ;
#68615=DIRECTION ( 'NONE',  ( 0.000000000000000000, 0.1736481776669275834, 0.9848077530122086864 ) ) ;
#68617=CARTESIAN_POINT ( 'NONE',  ( 13.38461538461538680, -12.37446782046654192, 30.86335684631486131 ) ) ;
#68618=CYLINDRICAL_SURFACE ( 'NONE', #61723, 0.2499999999999995559 ) ;
#68619=VECTOR ( 'NONE', #77176, 999.9999999999998863 ) ;
#68620=CARTESIAN_POINT ( 'NONE',  ( -13.25382494364843389, -3.338503747796866872, 32.95102852606553512 ) ) ;
#68621=CARTESIAN_POINT ( 'NONE',  ( -7.846153846153965716, -10.90142922262034020, 33.41473453929536674 ) ) ;
#68622=CARTESIAN_POINT ( 'NONE',  ( -16.37733107841048508, -8.539481045369598178, 34.89627647299170832 ) ) ;
#68625=ORIENTED_EDGE ( 'NONE', *, *, #71723, .F. ) ;
#68628=VERTEX_POINT ( 'NONE', #66749 ) ;
#68630=LINE ( 'NONE', #54219, #32655 ) ;
#68631=AXIS2_PLACEMENT_3D ( 'NONE', #53583, #46830, #82848 ) ;
#68632=EDGE_LOOP ( 'NONE', ( #45522, #87058 ) ) ;
#68633=CARTESIAN_POINT ( 'NONE',  ( 14.17754509825408960, -8.587444163452046197, 34.63053765926554206 ) ) ;
#68635=CARTESIAN_POINT ( 'NONE',  ( 13.38461538461538680, -2.721908614388771852, 31.22303859784724978 ) ) ;
#68636=CYLINDRICAL_SURFACE ( 'NONE', #2143, 0.2500000000000002220 ) ;
#68637=FACE_OUTER_BOUND ( 'NONE', #60943, .T. ) ;
#68638=CARTESIAN_POINT ( 'NONE',  ( 1.134638640566797196, -2.544273027872574922, 31.48422191005632342 ) ) ;
#68639=DIRECTION ( 'NONE',  ( -0.000000000000000000, -0.7660444431189791237, -0.6427876096865379196 ) ) ;
#68640=CARTESIAN_POINT ( 'NONE',  ( 2.307692307692187583, -10.21337939537710326, 33.94971097300076224 ) ) ;
#68642=DIRECTION ( 'NONE',  ( 0.000000000000000000, 0.1736481776669275834, 0.9848077530122086864 ) ) ;
#68643=DIRECTION ( 'NONE',  ( -0.000000000000000000, -0.3420201433256694901, -0.9396926207859082059 ) ) ;
#68644=B_SPLINE_CURVE_WITH_KNOTS ( 'NONE', 3,
 ( #64325, #35999, #1310, #57140, #77414, #2188, #82861, #22469, #875, #62996 ),
 .UNSPECIFIED., .F., .F.,
 ( 4, 2, 2, 2, 4 ),
 ( 0.000000000000000000, 0.0001954311564186865492, 0.0003908623128373730983, 0.0005862934692560596746, 0.0007817246256747461966 ),
 .UNSPECIFIED. ) ;
#68645=CARTESIAN_POINT ( 'NONE',  ( 14.53106824839049160, -2.501478030877322567, 29.88021232661721172 ) ) ;
#68646=CARTESIAN_POINT ( 'NONE',  ( -9.757577692864012775, -11.67786785259540849, 32.92929555188721480 ) ) ;
#68647=EDGE_CURVE ( 'NONE', #46832, #48838, #23766, .T. ) ;
#68649=ORIENTED_EDGE ( 'NONE', *, *, #18267, .F. ) ;
#68650=CARTESIAN_POINT ( 'NONE',  ( -18.13069060311030611, -2.494641256782729855, 31.33461815524612959 ) ) ;
#68651=CARTESIAN_POINT ( 'NONE',  ( 15.23076923076910916, -12.16647553114689728, 32.15551576947799362 ) ) ;
#68652=LINE ( 'NONE', #26341, #77144 ) ;
#68653=CARTESIAN_POINT ( 'NONE',  ( 15.23076923076923173, -12.29105614889573062, 35.45975837776705220 ) ) ;
#68655=LINE ( 'NONE', #21354, #23358 ) ;
#68656=CARTESIAN_POINT ( 'NONE',  ( -9.469528023329624844, -10.97394488606064122, 33.68653795673694873 ) ) ;
#68657=EDGE_CURVE ( 'NONE', #1046, #85754, #75499, .T. ) ;
#68659=AXIS2_PLACEMENT_3D ( 'NONE', #67540, #51887, #60327 ) ;
#68660=VERTEX_POINT ( 'NONE', #85084 ) ;
#68661=CARTESIAN_POINT ( 'NONE',  ( -14.55766905174089665, -12.65889640711025521, 30.72598325615533454 ) ) ;
#68662=VERTEX_POINT ( 'NONE', #42775 ) ;
#68663=EDGE_CURVE ( 'NONE', #78118, #88590, #5629, .T. ) ;
#68664=CARTESIAN_POINT ( 'NONE',  ( 5.326977388561390470, -8.303483539816728154, 34.68545999027711702 ) ) ;
#68665=CARTESIAN_POINT ( 'NONE',  ( -18.25000000000000000, -12.75000000000000888, 29.74999999999997868 ) ) ;
#68666=CARTESIAN_POINT ( 'NONE',  ( -6.988399838569097966, -7.749976743299137993, 34.99404534957040624 ) ) ;
#68667=CARTESIAN_POINT ( 'NONE',  ( -15.45425417449318317, -3.236172620538810385, 32.36188796281390267 ) ) ;
#68669=ORIENTED_EDGE ( 'NONE', *, *, #34115, .T. ) ;
#68670=ORIENTED_EDGE ( 'NONE', *, *, #27210, .F. ) ;
#68671=AXIS2_PLACEMENT_3D ( 'NONE', #36579, #10880, #38352 ) ;
#68672=ORIENTED_EDGE ( 'NONE', *, *, #39991, .F. ) ;
#68673=ORIENTED_EDGE ( 'NONE', *, *, #25267, .T. ) ;
#68674=CYLINDRICAL_SURFACE ( 'NONE', #8483, 0.2500000000000004996 ) ;
#68675=CARTESIAN_POINT ( 'NONE',  ( 7.846153846153725020, -3.835265460704628371, 33.15142922262033665 ) ) ;
#68677=EDGE_CURVE ( 'NONE', #23762, #45514, #84129, .T. ) ;
#68679=CARTESIAN_POINT ( 'NONE',  ( 16.40379167219429846, -10.05730279482229683, 34.04704008940765902 ) ) ;
#68680=LINE ( 'NONE', #32675, #59442 ) ;
#68681=CARTESIAN_POINT ( 'NONE',  ( 16.15384615384615330, -13.88283147151868846, 33.14645433367849847 ) ) ;
#68682=AXIS2_PLACEMENT_3D ( 'NONE', #81611, #87957, #46040 ) ;
#68683=ORIENTED_EDGE ( 'NONE', *, *, #20649, .T. ) ;
#68684=ORIENTED_EDGE ( 'NONE', *, *, #73101, .F. ) ;
#68685=ORIENTED_EDGE ( 'NONE', *, *, #87296, .T. ) ;
#68686=FACE_OUTER_BOUND ( 'NONE', #30723, .T. ) ;
#68688=ORIENTED_EDGE ( 'NONE', *, *, #36763, .F. ) ;
#68689=CYLINDRICAL_SURFACE ( 'NONE', #47714, 0.2499999999999986955 ) ;
#68690=DIRECTION ( 'NONE',  ( -0.000000000000000000, 0.5000000000000011102, -0.8660254037844381525 ) ) ;
#68692=VERTEX_POINT ( 'NONE', #57159 ) ;
#68693=ADVANCED_FACE ( 'NONE', ( #50822 ), #70681, .F. ) ;
#68694=EDGE_CURVE ( 'NONE', #88462, #27552, #47584, .T. ) ;
#68696=CARTESIAN_POINT ( 'NONE',  ( -13.38461538461550582, -4.481592998941358097, 33.73612834414048933 ) ) ;
#68697=B_SPLINE_CURVE_WITH_KNOTS ( 'NONE', 3,
 ( #40645, #88846, #19036, #73986, #46504, #26234 ),
 .UNSPECIFIED., .F., .F.,
 ( 4, 2, 4 ),
 ( 2.110382192020081086E-17, 0.0001954756301636924353, 0.0003909512603273637287 ),
 .UNSPECIFIED. ) ;
#68698=FACE_BOUND ( 'NONE', #61985, .T. ) ;
#68699=CARTESIAN_POINT ( 'NONE',  ( -5.076923076923075762, -4.661471528628507777, 34.16647553114623292 ) ) ;
#68700=CARTESIAN_POINT ( 'NONE',  ( -4.219928533206287469, -9.905515769479276145, 34.41647553114623292 ) ) ;
#68701=VERTEX_POINT ( 'NONE', #15744 ) ;
#68702=CARTESIAN_POINT ( 'NONE',  ( 7.846153846153846700, -7.500000000000001776, 35.04278698407183867 ) ) ;
#68703=CARTESIAN_POINT ( 'NONE',  ( 6.699591998512594238, -12.11044203135681840, 32.26167407432752299 ) ) ;
#68704=B_SPLINE_CURVE_WITH_KNOTS ( 'NONE', 3,
 ( #26004, #46279, #86848, #74641, #39091, #38631, #66551, #4852, #5292, #53467 ),
 .UNSPECIFIED., .F., .F.,
 ( 4, 2, 2, 2, 4 ),
 ( 0.0007817246336856291692, 0.0009771112958940103739, 0.001172497958102391470, 0.001367884620310772566, 0.001563271282519153663 ),
 .UNSPECIFIED. ) ;
#68705=FACE_OUTER_BOUND ( 'NONE', #12942, .T. ) ;
#68706=CARTESIAN_POINT ( 'NONE',  ( 14.24160992833217065, -9.058645607665454236, 34.76329471203372634 ) ) ;
#68707=EDGE_CURVE ( 'NONE', #4668, #75052, #55070, .T. ) ;
#68708=VERTEX_POINT ( 'NONE', #17509 ) ;
#68710=CARTESIAN_POINT ( 'NONE',  ( 16.28468457185891438, -7.277220443632451463, 34.74524770363009196 ) ) ;
#68711=DIRECTION ( 'NONE',  ( 0.000000000000000000, 0.8660254037844377084, 0.5000000000000015543 ) ) ;
#68712=CARTESIAN_POINT ( 'NONE',  ( 4.403791563224196182, -11.56426240980093745, 33.07394671870546432 ) ) ;
#68713=CARTESIAN_POINT ( 'NONE',  ( 9.692307692307695177, -11.11383981884818262, 36.00935417666054406 ) ) ;
#68715=CARTESIAN_POINT ( 'NONE',  ( -15.16470087976679082, -11.69971097300155272, 32.46337939537588113 ) ) ;
#68717=FACE_BOUND ( 'NONE', #20193, .T. ) ;
#68718=CARTESIAN_POINT ( 'NONE',  ( -7.846153846153844924, -1.466349020453238561, 30.81389545987213907 ) ) ;
#68719=CARTESIAN_POINT ( 'NONE',  ( 16.94623247381276343, -2.845849958028613624, 32.17971566917920967 ) ) ;
#68720=VECTOR ( 'NONE', #36640, 1000.000000000000227 ) ;
#68721=CARTESIAN_POINT ( 'NONE',  ( 5.207713517890025123, -9.084667340241226796, 34.75534355489798344 ) ) ;
#68722=CARTESIAN_POINT ( 'NONE',  ( -5.933931648997559982, -9.780366693483667717, 34.19971097300155805 ) ) ;
#68723=CARTESIAN_POINT ( 'NONE',  ( -2.307692307692305711, -12.34228464037088635, 31.77849191805839268 ) ) ;
#68724=LINE ( 'NONE', #62831, #39090 ) ;
#68726=ADVANCED_FACE ( 'NONE', ( #66592 ), #17956, .F. ) ;
#68728=CARTESIAN_POINT ( 'NONE',  ( -5.934744860487159102, -11.06231777344671130, 33.60647404775212976 ) ) ;
#68730=CARTESIAN_POINT ( 'NONE',  ( -1.384615384615383471, -12.48256725967547354, 35.29906147534542527 ) ) ;
#68731=ORIENTED_EDGE ( 'NONE', *, *, #51414, .T. ) ;
#68732=FACE_OUTER_BOUND ( 'NONE', #75704, .T. ) ;
#68733=FACE_OUTER_BOUND ( 'NONE', #63217, .T. ) ;
#68734=CARTESIAN_POINT ( 'NONE',  ( -9.627052552794857831, -11.67786785259547777, 32.92929555188713664 ) ) ;
#68735=ORIENTED_EDGE ( 'NONE', *, *, #83977, .F. ) ;
#68736=CARTESIAN_POINT ( 'NONE',  ( 17.86952481492428291, -7.276987145209182550, 34.99546412871779211 ) ) ;
#68738=CARTESIAN_POINT ( 'NONE',  ( -15.36145983387954139, -9.084618155246140248, 34.75535874321725771 ) ) ;
#68739=CARTESIAN_POINT ( 'NONE',  ( 23.00000000000000000, -4.249999999999998224, 29.75000000000000355 ) ) ;
#68741=CARTESIAN_POINT ( 'NONE',  ( 8.769230769230768274, -9.584722331328613620, 36.20867863119891439 ) ) ;
#68742=CARTESIAN_POINT ( 'NONE',  ( -12.46153846153858424, -8.656820664282941280, 34.87096338111179961 ) ) ;
#68743=CARTESIAN_POINT ( 'NONE',  ( -6.923076923076922462, -2.249999999999998668, 29.50000000000001421 ) ) ;
#68746=CARTESIAN_POINT ( 'NONE',  ( -10.61538461538473399, -2.892918686052166066, 31.69288490824153470 ) ) ;
#68747=CARTESIAN_POINT ( 'NONE',  ( -11.53846153846165912, -6.879047030192662504, 34.71129190930017927 ) ) ;
#68748=B_SPLINE_CURVE_WITH_KNOTS ( 'NONE', 3,
 ( #24168, #4806, #73715, #60174, #12011, #53417, #16978, #10228, #37688, #65153 ),
 .UNSPECIFIED., .F., .F.,
 ( 4, 2, 2, 2, 4 ),
 ( 0.000000000000000000, 0.0001954311564186867660, 0.0003908623128373735320, 0.0005862934692560603251, 0.0007817246256747470640 ),
 .UNSPECIFIED. ) ;
#68749=ORIENTED_EDGE ( 'NONE', *, *, #52608, .F. ) ;
#68750=CARTESIAN_POINT ( 'NONE',  ( 8.992010310499175318, -10.11255958852956027, 34.01340905677048454 ) ) ;
#68751=AXIS2_PLACEMENT_3D ( 'NONE', #30039, #65580, #17859 ) ;
#68753=EDGE_CURVE ( 'NONE', #69788, #49089, #38987, .T. ) ;
#68754=CARTESIAN_POINT ( 'NONE',  ( 6.923076923076924238, -2.292212530054420494, 30.41441678777542634 ) ) ;
#68755=CARTESIAN_POINT ( 'NONE',  ( -8.834500769787091201, -3.643525952247789412, 33.31231777344662959 ) ) ;
#68756=ORIENTED_EDGE ( 'NONE', *, *, #16666, .T. ) ;
#68757=CARTESIAN_POINT ( 'NONE',  ( 1.450682717965462443, -8.164416787775445883, 34.95778746994558617 ) ) ;
#68759=CARTESIAN_POINT ( 'NONE',  ( 3.930361229281822855, -9.417330523894424488, 34.63758898049880486 ) ) ;
#68760=EDGE_LOOP ( 'NONE', ( #2296, #25926, #60341, #25968 ) ) ;
#68761=CARTESIAN_POINT ( 'NONE',  ( -8.096153846153843148, -7.566083408709834757, 34.74999999999999289 ) ) ;
#68763=CARTESIAN_POINT ( 'NONE',  ( -17.01075647033143667, -7.250054591869668386, 34.99404684341514127 ) ) ;
#68765=CARTESIAN_POINT ( 'NONE',  ( 10.61538461538461675, -1.951392089020283160, 34.73218667398347748 ) ) ;
#68766=DIRECTION ( 'NONE',  ( -0.000000000000000000, 0.1736481776669307198, -0.9848077530122080203 ) ) ;
#68767=ORIENTED_EDGE ( 'NONE', *, *, #48883, .T. ) ;
#68768=ORIENTED_EDGE ( 'NONE', *, *, #56783, .T. ) ;
#68769=VERTEX_POINT ( 'NONE', #39577 ) ;
#68770=AXIS2_PLACEMENT_3D ( 'NONE', #80467, #59291, #52086 ) ;
#68771=DIRECTION ( 'NONE',  ( -0.000000000000000000, -0.6427876096865404731, -0.7660444431189770143 ) ) ;
#68772=CARTESIAN_POINT ( 'NONE',  ( -2.307692307692305711, -5.557115091759785130, 34.35708131394839171 ) ) ;
#68773=LINE ( 'NONE', #62444, #6185 ) ;
#68774=CARTESIAN_POINT ( 'NONE',  ( -8.069638770718178478, -10.97335522853832579, 33.68706563782419749 ) ) ;
#68775=B_SPLINE_CURVE_WITH_KNOTS ( 'NONE', 3,
 ( #69936, #15003, #61841, #76244, #43356, #34816, #70836, #8694, #35265, #8250 ),
 .UNSPECIFIED., .F., .F.,
 ( 4, 2, 2, 2, 4 ),
 ( 0.000000000000000000, 0.0001954339857564053873, 0.0003908679715128107746, 0.0005863019572692161618, 0.0007817359430256215491 ),
 .UNSPECIFIED. ) ;
#68776=VECTOR ( 'NONE', #62127, 1000.000000000000000 ) ;
#68778=B_SPLINE_CURVE_WITH_KNOTS ( 'NONE', 3,
 ( #84768, #42444, #14972, #48298, #15418, #42006, #21268, #41550, #56830, #28480 ),
 .UNSPECIFIED., .F., .F.,
 ( 4, 2, 2, 2, 4 ),
 ( 0.0007817359430256297891, 0.0009771253907249958896, 0.001172514838424361990, 0.001367904286123728091, 0.001563293733823094191 ),
 .UNSPECIFIED. ) ;
#68779=CARTESIAN_POINT ( 'NONE',  ( 17.07692307692307665, -11.35647404775217417, 33.31231777344666511 ) ) ;
#68780=ORIENTED_EDGE ( 'NONE', *, *, #15433, .F. ) ;
#68781=ORIENTED_EDGE ( 'NONE', *, *, #22016, .T. ) ;
#68783=ORIENTED_EDGE ( 'NONE', *, *, #27322, .F. ) ;
#68785=EDGE_LOOP ( 'NONE', ( #83836, #81398, #7805, #58925 ) ) ;
#68786=CARTESIAN_POINT ( 'NONE',  ( -3.230769230769229949, -2.249999999999998668, 29.75000000000001776 ) ) ;
#68788=CARTESIAN_POINT ( 'NONE',  ( -10.61538461538461320, -11.33034616979429110, 35.88435417666054406 ) ) ;
#68790=LINE ( 'NONE', #12088, #84205 ) ;
#68791=EDGE_LOOP ( 'NONE', ( #33012, #36121 ) ) ;
#68792=EDGE_CURVE ( 'NONE', #64437, #46179, #46472, .T. ) ;
#68794=ORIENTED_EDGE ( 'NONE', *, *, #63223, .T. ) ;
#68796=FACE_OUTER_BOUND ( 'NONE', #14493, .T. ) ;
#68797=ORIENTED_EDGE ( 'NONE', *, *, #11368, .F. ) ;
#68798=CARTESIAN_POINT ( 'NONE',  ( 6.673100192134570285, -6.567427716900047230, 34.66269422305636283 ) ) ;
#68799=CARTESIAN_POINT ( 'NONE',  ( -0.4615384615384611200, -6.343179335718451384, 34.87096338111211935 ) ) ;
#68800=VERTEX_POINT ( 'NONE', #87774 ) ;
#68802=CARTESIAN_POINT ( 'NONE',  ( -3.930834802233303282, -4.887748414852792322, 34.01359900205216746 ) ) ;
#68803=CARTESIAN_POINT ( 'NONE',  ( 12.71159288145191013, -9.233818618650603938, 34.70587769442853698 ) ) ;
#68805=EDGE_LOOP ( 'NONE', ( #19724, #7822 ) ) ;
#68806=FACE_BOUND ( 'NONE', #25009, .T. ) ;
#68807=CARTESIAN_POINT ( 'NONE',  ( -15.48074597481782178, -8.347322224742351082, 34.93158281831414058 ) ) ;
#68808=CARTESIAN_POINT ( 'NONE',  ( 15.90382292962469535, -2.588893531581426100, 31.60682220781849239 ) ) ;
#68809=FACE_OUTER_BOUND ( 'NONE', #31299, .T. ) ;
#68810=DIRECTION ( 'NONE',  ( 0.000000000000000000, 0.7660444431189807890, 0.6427876096865361433 ) ) ;
#68812=FACE_OUTER_BOUND ( 'NONE', #27523, .T. ) ;
#68815=CARTESIAN_POINT ( 'NONE',  ( -7.911423846710166075, -6.835583212224499938, 34.95778746994557906 ) ) ;
#68816=CARTESIAN_POINT ( 'NONE',  ( 0.4615384615384611200, -10.67929555188718282, 33.92786785259544047 ) ) ;
#68817=ORIENTED_EDGE ( 'NONE', *, *, #44206, .F. ) ;
#68819=CARTESIAN_POINT ( 'NONE',  ( 10.61538461538461675, -8.164416787775445883, 34.95778746994557906 ) ) ;
#68821=CARTESIAN_POINT ( 'NONE',  ( -12.46153846153858424, -2.379036618888197729, 30.90682066428292885 ) ) ;
#68822=EDGE_CURVE ( 'NONE', #5428, #37333, #15374, .T. ) ;
#68823=CYLINDRICAL_SURFACE ( 'NONE', #71690, 0.2499999999999998890 ) ;
#68824=FACE_BOUND ( 'NONE', #39997, .T. ) ;
#68825=CARTESIAN_POINT ( 'NONE',  ( -18.25002323729296805, -3.202444869320337784, 32.30641848906366675 ) ) ;
#68827=CARTESIAN_POINT ( 'NONE',  ( 10.39189967166066708, -8.496056993536548418, 34.65000542017679663 ) ) ;
#68828=CYLINDRICAL_SURFACE ( 'NONE', #23722, 0.2499999999999995559 ) ;
#68829=CARTESIAN_POINT ( 'NONE',  ( -8.769230769230890843, -12.27809138561165270, 31.22303859784587132 ) ) ;
#68833=VERTEX_POINT ( 'NONE', #51866 ) ;
#68834=AXIS2_PLACEMENT_3D ( 'NONE', #40510, #26543, #26986 ) ;
#68835=CARTESIAN_POINT ( 'NONE',  ( -4.153846153846152411, -9.780366693483667717, 34.19971097300155094 ) ) ;
#68836=CARTESIAN_POINT ( 'NONE',  ( -15.45369618967607828, -5.582147617184174848, 34.63737895849758530 ) ) ;
#68837=DIRECTION ( 'NONE',  ( -0.000000000000000000, 0.9396926207859093161, -0.3420201433256663259 ) ) ;
#68838=CARTESIAN_POINT ( 'NONE',  ( -8.769230769230768274, -8.164416787775445883, 34.95778746994557906 ) ) ;
#68839=CARTESIAN_POINT ( 'NONE',  ( -13.25408994638174498, -2.647132371071621471, 31.75357179365171589 ) ) ;
#68841=B_SPLINE_CURVE_WITH_KNOTS ( 'NONE', 3,
 ( #11643, #38213, #39121, #32352, #65673, #3970, #80557, #87318, #25595, #52161 ),
 .UNSPECIFIED., .F., .F.,
 ( 4, 2, 2, 2, 4 ),
 ( 0.0007817359430256282712, 0.0009771253907249945886, 0.001172514838424360689, 0.001367904286123726790, 0.001563293733823093107 ),
 .UNSPECIFIED. ) ;
#68842=DIRECTION ( 'NONE',  ( 0.000000000000000000, -8.673617379884033500E-16, 1.000000000000000000 ) ) ;
#68844=CIRCLE ( 'NONE', #63110, 0.2500000000000002220 ) ;
#68845=CARTESIAN_POINT ( 'NONE',  ( 6.923076923076924238, -2.538708090699994813, 30.37095296980875503 ) ) ;
#68847=CARTESIAN_POINT ( 'NONE',  ( 10.61538461538461675, -3.322132147404559976, 32.92929555188717927 ) ) ;
#68848=CARTESIAN_POINT ( 'NONE',  ( 5.142178216435913107, -8.656820664281605460, 34.87096338111211224 ) ) ;
#68849=VECTOR ( 'NONE', #1598, 1000.000000000000000 ) ;
#68850=DIRECTION ( 'NONE',  ( 0.000000000000000000, -6.938893903907222067E-15, 1.000000000000000000 ) ) ;
#68851=CARTESIAN_POINT ( 'NONE',  ( -8.546217925137373328, -11.43677907613344757, 33.22367315496202167 ) ) ;
#68852=CARTESIAN_POINT ( 'NONE',  ( 12.52760681254090080, -2.721908614388771852, 31.22303859784725333 ) ) ;
#68853=ORIENTED_EDGE ( 'NONE', *, *, #13912, .T. ) ;
#68854=DIRECTION ( 'NONE',  ( 0.000000000000000000, 0.9848077530122072432, -0.1736481776669354937 ) ) ;
#68857=CARTESIAN_POINT ( 'NONE',  ( -9.758390071667827570, -10.67929555188718460, 33.92786785259543336 ) ) ;
#68858=CARTESIAN_POINT ( 'NONE',  ( -18.00000000000012079, -10.21337939537710504, 33.94971097300076224 ) ) ;
#68859=FACE_OUTER_BOUND ( 'NONE', #12120, .T. ) ;
#68860=CARTESIAN_POINT ( 'NONE',  ( 7.623227628637697428, -2.554751324335733820, 30.48935550225260727 ) ) ;
#68861=VERTEX_POINT ( 'NONE', #86128 ) ;
#68863=CARTESIAN_POINT ( 'NONE',  ( -4.826977558574935934, -10.05730279482229683, 34.04704008940765902 ) ) ;
#68864=ORIENTED_EDGE ( 'NONE', *, *, #43333, .F. ) ;
#68865=CARTESIAN_POINT ( 'NONE',  ( 11.76147438255493149, -9.172514111537584114, 34.72667873470787470 ) ) ;
#68866=CARTESIAN_POINT ( 'NONE',  ( 8.096153846155281997, -7.500000000000155431, 34.75000000000007105 ) ) ;
#68867=ORIENTED_EDGE ( 'NONE', *, *, #79450, .T. ) ;
#68868=CARTESIAN_POINT ( 'NONE',  ( 7.596130608860880429, -4.335965774309649134, 33.62209801155881905 ) ) ;
#68869=CARTESIAN_POINT ( 'NONE',  ( 8.519254025182176449, -6.524016743844655686, 34.90889640711025521 ) ) ;
#68870=CARTESIAN_POINT ( 'NONE',  ( -15.00775787915638304, -12.39991518177334129, 30.74647679643404530 ) ) ;
#68871=EDGE_LOOP ( 'NONE', ( #70753, #85274 ) ) ;
#68872=ORIENTED_EDGE ( 'NONE', *, *, #66782, .F. ) ;
#68873=CARTESIAN_POINT ( 'NONE',  ( 15.36156103859402045, -10.54018710029568595, 33.71981072465678864 ) ) ;
#68874=VECTOR ( 'NONE', #55634, 1000.000000000000000 ) ;
#68875=ORIENTED_EDGE ( 'NONE', *, *, #36881, .F. ) ;
#68876=CARTESIAN_POINT ( 'NONE',  ( 7.780071466793711643, -9.058645607665454236, 34.76329471203372634 ) ) ;
#68877=CARTESIAN_POINT ( 'NONE',  ( -7.053224892808619195, -2.373036134822904319, 30.88089517874952250 ) ) ;
#68879=CARTESIAN_POINT ( 'NONE',  ( -6.857009589726846599, -11.35647404775217595, 33.31231777344667222 ) ) ;
#68880=CARTESIAN_POINT ( 'NONE',  ( -0.2387587925603955330, -5.827830569534416583, 34.72679350104403539 ) ) ;
#68881=CARTESIAN_POINT ( 'NONE',  ( -2.372942239466390824, -2.255955759149247619, 30.00000000000013856 ) ) ;
#68882=CARTESIAN_POINT ( 'NONE',  ( -0.2385256174450668676, -12.38742843783360748, 31.66772728687926985 ) ) ;
#68885=CARTESIAN_POINT ( 'NONE',  ( 18.22277966897806678, -9.418065098278011860, 34.63729479722530158 ) ) ;
#68886=ORIENTED_EDGE ( 'NONE', *, *, #73500, .F. ) ;
#68887=CARTESIAN_POINT ( 'NONE',  ( 17.07692307692307665, -2.292212530054420494, 30.41441678777542634 ) ) ;
#68888=EDGE_CURVE ( 'NONE', #32448, #19849, #50972, .T. ) ;
#68889=EDGE_LOOP ( 'NONE', ( #840, #35695, #862, #45982 ) ) ;
#68891=CARTESIAN_POINT ( 'NONE',  ( 9.692307692307695177, -1.629998284177014645, 34.34916445242399163 ) ) ;
#68892=DIRECTION ( 'NONE',  ( 1.000000000000000000, 0.000000000000000000, 0.000000000000000000 ) ) ;
#68893=EDGE_CURVE ( 'NONE', #72630, #58205, #53951, .T. ) ;
#68894=ORIENTED_EDGE ( 'NONE', *, *, #19900, .T. ) ;
#68895=DIRECTION ( 'NONE',  ( -0.000000000000000000, 0.9396926207859093161, -0.3420201433256663259 ) ) ;
#68896=VECTOR ( 'NONE', #75547, 1000.000000000000000 ) ;
#68897=ORIENTED_EDGE ( 'NONE', *, *, #9600, .F. ) ;
#68898=DIRECTION ( 'NONE',  ( -1.000000000000000000, 0.000000000000000000, 0.000000000000000000 ) ) ;
#68899=VERTEX_POINT ( 'NONE', #10465 ) ;
#68901=CARTESIAN_POINT ( 'NONE',  ( -12.68502338610279168, -3.562934362175800285, 33.22335522853832401 ) ) ;
#68902=ORIENTED_EDGE ( 'NONE', *, *, #83019, .F. ) ;
#68904=EDGE_CURVE ( 'NONE', #74960, #19286, #71183, .T. ) ;
#68905=CARTESIAN_POINT ( 'NONE',  ( 1.384615384615265343, -6.879047030192662504, 34.71129190930017927 ) ) ;
#68906=B_SPLINE_CURVE_WITH_KNOTS ( 'NONE', 3,
 ( #30813, #70923, #45214, #72691, #38025, #64144, #3787, #65926, #16859, #37121 ),
 .UNSPECIFIED., .F., .F.,
 ( 4, 2, 2, 2, 4 ),
 ( 0.0007817359430256390048, 0.0009771253907250075990, 0.001172514838424376085, 0.001367904286123744571, 0.001563293733823113056 ),
 .UNSPECIFIED. ) ;
#68907=LINE ( 'NONE', #28359, #30998 ) ;
#68908=FACE_BOUND ( 'NONE', #48570, .T. ) ;
#68909=CYLINDRICAL_SURFACE ( 'NONE', #51370, 0.2499999999999979738 ) ;
#68910=CARTESIAN_POINT ( 'NONE',  ( -6.857008572074485997, -12.10708131394839882, 31.69288490824020954 ) ) ;
#68911=CARTESIAN_POINT ( 'NONE',  ( 4.284637961670939355, -12.38066358083363738, 30.83685684665853444 ) ) ;
#68912=CARTESIAN_POINT ( 'NONE',  ( -3.480792468062195333, -4.335965774309649134, 33.62209801155881905 ) ) ;
#68914=DIRECTION ( 'NONE',  ( -0.000000000000000000, 0.7660444431189791237, -0.6427876096865379196 ) ) ;
#68915=CARTESIAN_POINT ( 'NONE',  ( 7.846153846153846700, -3.322132147404559976, 32.92929555188717927 ) ) ;
#68916=EDGE_LOOP ( 'NONE', ( #57830, #85766 ) ) ;
#68917=ORIENTED_EDGE ( 'NONE', *, *, #8407, .T. ) ;
#68918=DIRECTION ( 'NONE',  ( 0.000000000000000000, 0.1736481776669275834, 0.9848077530122086864 ) ) ;
#68920=CARTESIAN_POINT ( 'NONE',  ( -12.71156169883142617, -2.587272538249755893, 30.68239716806877837 ) ) ;
#68921=CARTESIAN_POINT ( 'NONE',  ( -7.846153846153844924, -13.87047571288749737, 32.06866353760679544 ) ) ;
#68922=CARTESIAN_POINT ( 'NONE',  ( -23.00000000000000000, -4.249999999999998224, 29.75000000000000355 ) ) ;
#68923=LINE ( 'NONE', #71574, #40432 ) ;
#68924=VERTEX_POINT ( 'NONE', #3250 ) ;
#68926=CARTESIAN_POINT ( 'NONE',  ( -5.207613680033383652, -5.496505350115500121, 34.60290016733514307 ) ) ;
#68928=CARTESIAN_POINT ( 'NONE',  ( -8.835314180186649935, -12.10708131394839349, 31.69288490824020244 ) ) ;
#68930=CARTESIAN_POINT ( 'NONE',  ( 3.007284287045282944, -3.236172620538810385, 32.36188796281390267 ) ) ;
#68931=ORIENTED_EDGE ( 'NONE', *, *, #78288, .T. ) ;
#68932=CIRCLE ( 'NONE', #25738, 0.2500000000000002220 ) ;
#68933=ORIENTED_EDGE ( 'NONE', *, *, #21066, .F. ) ;
#68937=CARTESIAN_POINT ( 'NONE',  ( 15.29602480204525605, -6.879047030191282275, 34.71129190930002295 ) ) ;
#68938=ADVANCED_FACE ( 'NONE', ( #50103 ), #16330, .F. ) ;
#68939=ORIENTED_EDGE ( 'NONE', *, *, #1290, .T. ) ;
#68940=CARTESIAN_POINT ( 'NONE',  ( -9.627052552794857831, -10.33852847137154107, 34.16647553114620450 ) ) ;
#68941=CARTESIAN_POINT ( 'NONE',  ( -17.20707028636129721, -3.285722584762970744, 32.44110544564090048 ) ) ;
#68942=DIRECTION ( 'NONE',  ( -0.000000000000000000, 0.7660444431189791237, -0.6427876096865379196 ) ) ;
#68944=B_SPLINE_CURVE_WITH_KNOTS ( 'NONE', 3,
 ( #69154, #32379, #61060, #79677, #25172, #13321, #20080, #40803, #68265, #47984 ),
 .UNSPECIFIED., .F., .F.,
 ( 4, 2, 2, 2, 4 ),
 ( 0.000000000000000000, 0.0001954339881912776238, 0.0003908679763825552477, 0.0005863019645738329257, 0.0007817359527651104954 ),
 .UNSPECIFIED. ) ;
#68945=CARTESIAN_POINT ( 'NONE',  ( -11.28840722682322273, -6.567000820036036579, 34.66262288849541306 ) ) ;
#68946=ORIENTED_EDGE ( 'NONE', *, *, #66862, .T. ) ;
#68947=CARTESIAN_POINT ( 'NONE',  ( 4.219039142140807996, -2.255955759149235629, 29.99999999999988631 ) ) ;
#68948=B_SPLINE_CURVE_WITH_KNOTS ( 'NONE', 3,
 ( #86045, #66660, #31990, #45039, #86962, #18478, #73423, #19361, #11724, #46828 ),
 .UNSPECIFIED., .F., .F.,
 ( 4, 2, 2, 2, 4 ),
 ( 0.000000000000000000, 0.0001954311564186860613, 0.0003908623128373721225, 0.0005862934692560581567, 0.0007817246256747442451 ),
 .UNSPECIFIED. ) ;
#68949=DIRECTION ( 'NONE',  ( 0.000000000000000000, 0.9396926207859126468, 0.3420201433256571111 ) ) ;
#68950=ORIENTED_EDGE ( 'NONE', *, *, #4618, .T. ) ;
#68951=CARTESIAN_POINT ( 'NONE',  ( -16.94613263595612551, -8.191423895709842640, 34.95447573519442130 ) ) ;
#68954=B_SPLINE_CURVE_WITH_KNOTS ( 'NONE', 3,
 ( #9829, #17924, #3061, #38187, #85937, #39095, #24221, #30541, #58012, #38637 ),
 .UNSPECIFIED., .F., .F.,
 ( 4, 2, 2, 2, 4 ),
 ( 0.000000000000000000, 0.0001954339857564091820, 0.0003908679715128183640, 0.0005863019572692275460, 0.0007817359430256367279 ),
 .UNSPECIFIED. ) ;
#68955=B_SPLINE_CURVE_WITH_KNOTS ( 'NONE', 3,
 ( #51199, #57540, #15245, #36830, #30079, #49467 ),
 .UNSPECIFIED., .F., .F.,
 ( 4, 2, 4 ),
 ( 0.0003909569690057842790, 0.0005862646681846108007, 0.0007815723673634373224 ),
 .UNSPECIFIED. ) ;
#68956=LINE ( 'NONE', #7264, #665 ) ;
#68958=CARTESIAN_POINT ( 'NONE',  ( -3.230769230769229949, -10.67929555188718282, 33.92786785259544047 ) ) ;
#68959=DIRECTION ( 'NONE',  ( 0.000000000000000000, 0.3420201433256610524, 0.9396926207859113145 ) ) ;
#68961=ORIENTED_EDGE ( 'NONE', *, *, #23061, .T. ) ;
#68962=CARTESIAN_POINT ( 'NONE',  ( -15.48074597481782178, -6.524016743844655686, 34.90889640711025521 ) ) ;
#68966=CARTESIAN_POINT ( 'NONE',  ( 9.942253101685738059, -2.986452184633680673, 32.43230066228895225 ) ) ;
#68967=EDGE_LOOP ( 'NONE', ( #46526, #58659, #68894, #85377 ) ) ;
#68968=ORIENTED_EDGE ( 'NONE', *, *, #55863, .T. ) ;
#68969=CARTESIAN_POINT ( 'NONE',  ( -5.869474298236436738, -2.619367082507848554, 30.83698974864644171 ) ) ;
#68970=CARTESIAN_POINT ( 'NONE',  ( -16.02332045208259359, -12.27024696741798770, 31.24895572276497546 ) ) ;
#68973=CARTESIAN_POINT ( 'NONE',  ( -4.403822884788508141, -10.66389620160130036, 33.62221079203477103 ) ) ;
#68975=ORIENTED_EDGE ( 'NONE', *, *, #63224, .T. ) ;
#68976=EDGE_CURVE ( 'NONE', #57354, #41209, #1311, .T. ) ;
#68977=CARTESIAN_POINT ( 'NONE',  ( 12.23867219847536170, -2.251424796025574881, 29.88072029997477230 ) ) ;
#68978=CARTESIAN_POINT ( 'NONE',  ( 3.453780582382081743, -12.15243808032445827, 31.58219941686247978 ) ) ;
#68979=CARTESIAN_POINT ( 'NONE',  ( 5.299702745901141654, -12.47679350104403007, 31.42216943046555855 ) ) ;
#68980=ORIENTED_EDGE ( 'NONE', *, *, #30140, .F. ) ;
#68982=VERTEX_POINT ( 'NONE', #44666 ) ;
#68984=CARTESIAN_POINT ( 'NONE',  ( -5.750054590621957118, -12.07971442181322352, 32.31769673815850297 ) ) ;
#68986=DIRECTION ( 'NONE',  ( -0.000000000000000000, 1.000000000000000000, 3.491481338843133355E-15 ) ) ;
#68987=CYLINDRICAL_SURFACE ( 'NONE', #85295, 0.2499999999999993616 ) ;
#68988=CARTESIAN_POINT ( 'NONE',  ( 1.254468175177166689, -4.460286881179644780, 33.72017969459903242 ) ) ;
#68990=LINE ( 'NONE', #12725, #40555 ) ;
#68991=CARTESIAN_POINT ( 'NONE',  ( 3.453780582382079523, -12.39991518177334129, 30.74647679643404530 ) ) ;
#68992=B_SPLINE_CURVE_WITH_KNOTS ( 'NONE', 3,
 ( #7683, #84239, #22517, #35144, #57188, #76580, #83345, #14887, #69816, #8126 ),
 .UNSPECIFIED., .F., .F.,
 ( 4, 2, 2, 2, 4 ),
 ( 0.000000000000000000, 0.0001954311564186858715, 0.0003908623128373717431, 0.0005862934692560576146, 0.0007817246256747434861 ),
 .UNSPECIFIED. ) ;
#68993=VERTEX_POINT ( 'NONE', #47344 ) ;
#68994=FACE_BOUND ( 'NONE', #56675, .T. ) ;
#68995=ORIENTED_EDGE ( 'NONE', *, *, #26907, .T. ) ;
#68999=CARTESIAN_POINT ( 'NONE',  ( 18.06606733335007675, -6.343179335718452272, 34.87096338111212646 ) ) ;
#69000=DIRECTION ( 'NONE',  ( 0.000000000000000000, 0.6427876096865373645, -0.7660444431189797898 ) ) ;
#69001=CARTESIAN_POINT ( 'NONE',  ( -6.130147209438221445, -12.27039167877662251, 31.24851455888617835 ) ) ;
#69002=EDGE_CURVE ( 'NONE', #13933, #41455, #24916, .T. ) ;
#69003=VERTEX_POINT ( 'NONE', #10906 ) ;
#69004=VERTEX_POINT ( 'NONE', #54097 ) ;
#69005=ORIENTED_EDGE ( 'NONE', *, *, #38422, .T. ) ;
#69006=CARTESIAN_POINT ( 'NONE',  ( -10.86540783960607115, -8.475808217655753651, 34.90892951860618609 ) ) ;
#69007=ORIENTED_EDGE ( 'NONE', *, *, #24124, .T. ) ;
#69008=AXIS2_PLACEMENT_3D ( 'NONE', #51831, #64906, #66248 ) ;
#69009=EDGE_CURVE ( 'NONE', #8333, #72105, #63683, .T. ) ;
#69010=DIRECTION ( 'NONE',  ( 0.000000000000000000, 0.4999999999999985567, 0.8660254037844395958 ) ) ;
#69011=CARTESIAN_POINT ( 'NONE',  ( 1.450683735617825265, -3.513871655860379306, 32.76840700105978499 ) ) ;
#69012=CARTESIAN_POINT ( 'NONE',  ( -18.13014796973169851, -6.809168938359903223, 34.95455904226513866 ) ) ;
#69013=CARTESIAN_POINT ( 'NONE',  ( -8.638440328263817136, -3.957578996910242619, 33.62503395064540257 ) ) ;
#69014=CIRCLE ( 'NONE', #80546, 2.000000000000001776 ) ;
#69016=EDGE_CURVE ( 'NONE', #22109, #45697, #60502, .T. ) ;
#69017=DIRECTION ( 'NONE',  ( -0.000000000000000000, -0.5000000000000009992, -0.8660254037844380415 ) ) ;
#69018=CARTESIAN_POINT ( 'NONE',  ( -14.24243716817946925, -12.70778746994558439, 30.41441678777536595 ) ) ;
#69019=CARTESIAN_POINT ( 'NONE',  ( 3.930361229281820190, -2.612411019501189813, 31.66733052389439962 ) ) ;
#69020=CARTESIAN_POINT ( 'NONE',  ( -5.326946314216042033, -3.711651800289232916, 33.01384336483936011 ) ) ;
#69021=EDGE_LOOP ( 'NONE', ( #4110, #69484, #21490, #21682 ) ) ;
#69022=EDGE_CURVE ( 'NONE', #20097, #44863, #17426, .T. ) ;
#69023=EDGE_LOOP ( 'NONE', ( #20707, #64345 ) ) ;
#69024=VECTOR ( 'NONE', #19787, 1000.000000000000000 ) ;
#69025=EDGE_LOOP ( 'NONE', ( #39601, #83453 ) ) ;
#69027=FACE_OUTER_BOUND ( 'NONE', #34275, .T. ) ;
#69028=CARTESIAN_POINT ( 'NONE',  ( -1.514763354347083535, -2.647304123082328875, 31.75400227202885262 ) ) ;
#69029=CARTESIAN_POINT ( 'NONE',  ( 1.607395053593451140, -11.60474049983370648, 33.02348890104160262 ) ) ;
#69031=CARTESIAN_POINT ( 'NONE',  ( -17.75005459062195712, -5.766571408460170467, 34.70601412856602508 ) ) ;
#69032=CARTESIAN_POINT ( 'NONE',  ( 1.384615384615386802, -2.708943851104267164, 35.45975837776705220 ) ) ;
#69033=FACE_BOUND ( 'NONE', #37013, .T. ) ;
#69034=CARTESIAN_POINT ( 'NONE',  ( 9.942253210655836781, -3.712312575010499494, 33.01462480002815170 ) ) ;
#69035=VERTEX_POINT ( 'NONE', #5489 ) ;
#69036=ADVANCED_FACE ( 'NONE', ( #32955 ), #11345, .F. ) ;
#69037=CARTESIAN_POINT ( 'NONE',  ( -10.61538461538429878, -2.255955759149395501, 30.00000000000324363 ) ) ;
#69038=DIRECTION ( 'NONE',  ( 0.000000000000000000, 0.6427876096865368094, 0.7660444431189802339 ) ) ;
#69040=CARTESIAN_POINT ( 'NONE',  ( -1.634638608836840534, -3.520140089381497361, 33.17453946501458262 ) ) ;
#69041=EDGE_LOOP ( 'NONE', ( #9746, #22986, #49516, #33118 ) ) ;
#69042=CARTESIAN_POINT ( 'NONE',  ( -18.13014720943822056, -8.587444163452046197, 34.63053765926554206 ) ) ;
#69043=ORIENTED_EDGE ( 'NONE', *, *, #6268, .T. ) ;
#69044=FACE_BOUND ( 'NONE', #37489, .T. ) ;
#69045=B_SPLINE_CURVE_WITH_KNOTS ( 'NONE', 3,
 ( #26453, #12932, #54797, #87730, #40419, #6181, #62000, #67877, #67437, #73766 ),
 .UNSPECIFIED., .F., .F.,
 ( 4, 2, 2, 2, 4 ),
 ( 0.0007817246336856291692, 0.0009771112958940103739, 0.001172497958102391470, 0.001367884620310772566, 0.001563271282519153879 ),
 .UNSPECIFIED. ) ;
#69047=B_SPLINE_CURVE_WITH_KNOTS ( 'NONE', 3,
 ( #32397, #13013, #40500, #67962, #6264, #59862, #59420, #8476, #7142, #55320 ),
 .UNSPECIFIED., .F., .F.,
 ( 4, 2, 2, 2, 4 ),
 ( 0.0007817246256747550871, 0.0009771112852218989588, 0.001172497944769042939, 0.001367884604316186702, 0.001563271263863330682 ),
 .UNSPECIFIED. ) ;
#69048=CARTESIAN_POINT ( 'NONE',  ( -6.222826692479002553, -7.369208160676172348, 34.74850200257122879 ) ) ;
#69049=CARTESIAN_POINT ( 'NONE',  ( 16.85399611801622299, -11.98009711892700224, 32.48740034544074007 ) ) ;
#69050=EDGE_CURVE ( 'NONE', #62981, #88144, #79820, .T. ) ;
#69051=ORIENTED_EDGE ( 'NONE', *, *, #50479, .F. ) ;
#69052=CARTESIAN_POINT ( 'NONE',  ( 11.76124120743960333, -10.97394488606064122, 33.68653795673694873 ) ) ;
#69053=CARTESIAN_POINT ( 'NONE',  ( 15.48071464014727283, -2.341251567377310217, 30.72681386836322659 ) ) ;
#69054=CARTESIAN_POINT ( 'NONE',  ( -3.361460697436787104, -2.729777683071816785, 31.24903638046268739 ) ) ;
#69055=CARTESIAN_POINT ( 'NONE',  ( 6.249945518348143381, -3.712312575010499494, 33.01462480002815170 ) ) ;
#69057=CARTESIAN_POINT ( 'NONE',  ( 13.31934493865461278, -6.026961402152685388, 34.52809138561120506 ) ) ;
#69058=CARTESIAN_POINT ( 'NONE',  ( 2.438217745925954194, -3.625058011473228259, 33.29252011169590020 ) ) ;
#69060=ORIENTED_EDGE ( 'NONE', *, *, #80951, .F. ) ;
#69061=DIRECTION ( 'NONE',  ( -0.000000000000000000, -0.000000000000000000, -1.000000000000000000 ) ) ;
#69062=CARTESIAN_POINT ( 'NONE',  ( -10.83831083290076158, -12.39988816332205701, 30.74660775122750778 ) ) ;
#69063=CARTESIAN_POINT ( 'NONE',  ( 4.946232473812771424, -2.494641256782728966, 31.33461815524612959 ) ) ;
#69064=DIRECTION ( 'NONE',  ( 0.000000000000000000, 0.9848077530122072432, -0.1736481776669354937 ) ) ;
#69065=CARTESIAN_POINT ( 'NONE',  ( 16.85343815235874132, -4.988325925672468131, 34.36044203135681130 ) ) ;
#69066=CARTESIAN_POINT ( 'NONE',  ( 8.992606255003186888, -2.251407671071268712, 29.88021292934942963 ) ) ;
#69067=CARTESIAN_POINT ( 'NONE',  ( -16.28453675695646652, -8.191372820521381826, 34.95448215188424967 ) ) ;
#69068=LINE ( 'NONE', #28987, #21955 ) ;
#69069=EDGE_CURVE ( 'NONE', #11070, #71689, #34277, .T. ) ;
#69070=VECTOR ( 'NONE', #18995, 999.9999999999998863 ) ;
#69072=EDGE_LOOP ( 'NONE', ( #42221, #6759 ) ) ;
#69073=CARTESIAN_POINT ( 'NONE',  ( 17.86985279056177944, -4.460286881179643004, 33.72017969459903242 ) ) ;
#69074=ORIENTED_EDGE ( 'NONE', *, *, #71759, .F. ) ;
#69076=VERTEX_POINT ( 'NONE', #8146 ) ;
#69077=DIRECTION ( 'NONE',  ( 0.000000000000000000, 0.7660444431189822323, -0.6427876096865344779 ) ) ;
#69078=ORIENTED_EDGE ( 'NONE', *, *, #61465, .F. ) ;
#69079=DIRECTION ( 'NONE',  ( 0.000000000000000000, 0.9848077530122072432, -0.1736481776669354937 ) ) ;
#69080=DIRECTION ( 'NONE',  ( -0.000000000000000000, 1.000000000000000000, 3.491481338843133355E-15 ) ) ;
#69081=CARTESIAN_POINT ( 'NONE',  ( 7.846153846153846700, -2.292212530054420494, 30.41441678777542634 ) ) ;
#69082=DIRECTION ( 'NONE',  ( 0.000000000000000000, 0.000000000000000000, 1.000000000000000000 ) ) ;
#69083=LINE ( 'NONE', #48803, #86219 ) ;
#69084=CARTESIAN_POINT ( 'NONE',  ( -11.76194648218548622, -5.113361153441934093, 34.14387501736622710 ) ) ;
#69085=CARTESIAN_POINT ( 'NONE',  ( -4.376772371362300795, -3.586966769969700763, 32.86292498521069660 ) ) ;
#69086=ADVANCED_FACE ( 'NONE', ( #48228 ), #68505, .F. ) ;
#69087=DIRECTION ( 'NONE',  ( -0.000000000000000000, -0.9848077530122085754, -0.1736481776669273613 ) ) ;
#69088=CARTESIAN_POINT ( 'NONE',  ( 13.38461538461526601, -5.219633306517616589, 34.19971097300220464 ) ) ;
#69089=B_SPLINE_CURVE_WITH_KNOTS ( 'NONE', 3,
 ( #16963, #17858, #18298, #72784, #64689, #87219, #23704, #52954, #86780, #44410 ),
 .UNSPECIFIED., .F., .F.,
 ( 4, 2, 2, 2, 4 ),
 ( 0.0007817359430256293554, 0.0009771253907249952391, 0.001172514838424361123, 0.001367904286123727007, 0.001563293733823092890 ),
 .UNSPECIFIED. ) ;
#69091=CARTESIAN_POINT ( 'NONE',  ( 5.142178216435913107, -11.06231777344671130, 33.60647404775212976 ) ) ;
#69092=CARTESIAN_POINT ( 'NONE',  ( -8.069638789877792817, -8.496056993536548418, 34.65000542017679663 ) ) ;
#69093=EDGE_CURVE ( 'NONE', #36228, #80445, #3533, .T. ) ;
#69094=AXIS2_PLACEMENT_3D ( 'NONE', #59316, #25089, #80037 ) ;
#69096=EDGE_CURVE ( 'NONE', #68565, #67330, #36700, .T. ) ;
#69097=ORIENTED_EDGE ( 'NONE', *, *, #46026, .F. ) ;
#69098=ORIENTED_EDGE ( 'NONE', *, *, #19694, .F. ) ;
#69099=CYLINDRICAL_SURFACE ( 'NONE', #38567, 0.2499999999999995559 ) ;
#69100=CARTESIAN_POINT ( 'NONE',  ( 16.15384615384615330, -12.48256725967547354, 35.29906147534542527 ) ) ;
#69102=CARTESIAN_POINT ( 'NONE',  ( -11.40762312044877014, -7.277220443632450575, 34.74524770363009196 ) ) ;
#69104=CARTESIAN_POINT ( 'NONE',  ( -6.222926217516146608, -8.239355502252617924, 34.69524867566427417 ) ) ;
#69105=EDGE_CURVE ( 'NONE', #12728, #49110, #62562, .T. ) ;
#69106=MECHANICAL_DESIGN_GEOMETRIC_PRESENTATION_REPRESENTATION('',(#59002),#13047);
#69107=CARTESIAN_POINT ( 'NONE',  ( -2.372962308248625529, -8.656820664281497102, 34.87096338111211935 ) ) ;
#69108=VERTEX_POINT ( 'NONE', #7259 ) ;
#69109=CARTESIAN_POINT ( 'NONE',  ( -14.30769230769230660, -12.62096338111211580, 30.90682066428153263 ) ) ;
#69110=ORIENTED_EDGE ( 'NONE', *, *, #75319, .F. ) ;
#69111=CARTESIAN_POINT ( 'NONE',  ( 13.25392478150508069, -12.35290016733513951, 31.75349464988449455 ) ) ;
#69113=CARTESIAN_POINT ( 'NONE',  ( -6.699650524162136023, -7.630147987733840509, 34.99859428049665411 ) ) ;
#69116=ADVANCED_FACE ( 'NONE', ( #49122 ), #21204, .F. ) ;
#69119=B_SPLINE_CURVE_WITH_KNOTS ( 'NONE', 3,
 ( #83879, #22598, #29376, #43322, #70801, #2316, #7324, #34783, #82980, #48741 ),
 .UNSPECIFIED., .F., .F.,
 ( 4, 2, 2, 2, 4 ),
 ( 0.0007817246256747530271, 0.0009771112852218974409, 0.001172497944769041638, 0.001367884604316185835, 0.001563271263863330249 ),
 .UNSPECIFIED. ) ;
#69120=B_SPLINE_CURVE_WITH_KNOTS ( 'NONE', 3,
 ( #70613, #36388, #42269, #63850, #27854, #2148, #41375, #56213, #69726, #8031 ),
 .UNSPECIFIED., .F., .F.,
 ( 4, 2, 2, 2, 4 ),
 ( 0.000000000000000000, 0.0001954311564186863323, 0.0003908623128373726646, 0.0005862934692560590241, 0.0007817246256747453293 ),
 .UNSPECIFIED. ) ;
#69121=EDGE_LOOP ( 'NONE', ( #86629, #24416, #49936, #31849 ) ) ;
#69122=ORIENTED_EDGE ( 'NONE', *, *, #40533, .T. ) ;
#69123=CARTESIAN_POINT ( 'NONE',  ( 5.076923076923075762, -2.708943851104267164, 35.45975837776705220 ) ) ;
#69124=CARTESIAN_POINT ( 'NONE',  ( 7.715462379486285549, -3.530157926970578508, 32.79014554554150607 ) ) ;
#69125=VECTOR ( 'NONE', #8608, 1000.000000000000227 ) ;
#69126=DIRECTION ( 'NONE',  ( -0.000000000000000000, 0.6427876096865404731, -0.7660444431189771253 ) ) ;
#69127=DIRECTION ( 'NONE',  ( -0.000000000000000000, 0.7660444431189791237, -0.6427876096865379196 ) ) ;
#69128=LINE ( 'NONE', #34455, #50732 ) ;
#69129=CARTESIAN_POINT ( 'NONE',  ( -15.45425415533356528, -2.612411019501189369, 31.66733052389439962 ) ) ;
#69130=VERTEX_POINT ( 'NONE', #42384 ) ;
#69131=ORIENTED_EDGE ( 'NONE', *, *, #25687, .F. ) ;
#69132=EDGE_LOOP ( 'NONE', ( #21828, #40260, #24699, #43654 ) ) ;
#69134=ORIENTED_EDGE ( 'NONE', *, *, #41622, .F. ) ;
#69135=CYLINDRICAL_SURFACE ( 'NONE', #59219, 0.2500000000000009437 ) ;
#69136=CARTESIAN_POINT ( 'NONE',  ( 6.989246064039581263, -7.250054483168843156, 34.74374881642865631 ) ) ;
#69138=ORIENTED_EDGE ( 'NONE', *, *, #38720, .T. ) ;
#69139=EDGE_CURVE ( 'NONE', #22888, #4743, #34724, .T. ) ;
#69140=VECTOR ( 'NONE', #46673, 1000.000000000000227 ) ;
#69142=FACE_OUTER_BOUND ( 'NONE', #79380, .T. ) ;
#69144=EDGE_CURVE ( 'NONE', #28039, #39612, #55435, .T. ) ;
#69145=FACE_BOUND ( 'NONE', #26807, .T. ) ;
#69146=CARTESIAN_POINT ( 'NONE',  ( 6.699591979352975457, -4.386631170607603991, 33.66268669641500111 ) ) ;
#69147=AXIS2_PLACEMENT_3D ( 'NONE', #50124, #84828, #63644 ) ;
#69149=CYLINDRICAL_SURFACE ( 'NONE', #8914, 0.2499999999999995559 ) ;
#69150=ORIENTED_EDGE ( 'NONE', *, *, #42770, .F. ) ;
#69151=CARTESIAN_POINT ( 'NONE',  ( -9.822998295418001291, -4.684245665217972032, 34.18127051446801090 ) ) ;
#69152=EDGE_CURVE ( 'NONE', #76205, #32515, #59378, .T. ) ;
#69153=CARTESIAN_POINT ( 'NONE',  ( 8.992010438208831502, -8.540255544307065350, 34.89611431652622286 ) ) ;
#69154=CARTESIAN_POINT ( 'NONE',  ( -13.63461538461538325, -7.500000000000001776, 34.75000000000000000 ) ) ;
#69156=ORIENTED_EDGE ( 'NONE', *, *, #80072, .F. ) ;
#69157=AXIS2_PLACEMENT_3D ( 'NONE', #68602, #81686, #20421 ) ;
#69158=EDGE_CURVE ( 'NONE', #45937, #64075, #88443, .T. ) ;
#69159=CARTESIAN_POINT ( 'NONE',  ( 12.46153846153833911, -11.48612834414049644, 32.76840700105863391 ) ) ;
#69160=CARTESIAN_POINT ( 'NONE',  ( -4.153846153846152411, -9.905515769479276145, 34.41647553114623292 ) ) ;
#69162=CARTESIAN_POINT ( 'NONE',  ( -2.241624974342230292, -9.058645607665452459, 34.76329471203371924 ) ) ;
#69163=FACE_OUTER_BOUND ( 'NONE', #84185, .T. ) ;
#69164=FACE_BOUND ( 'NONE', #20751, .T. ) ;
#69165=CARTESIAN_POINT ( 'NONE',  ( 4.826946345980721809, -11.28823185664190376, 33.01397839955799896 ) ) ;
#69166=CARTESIAN_POINT ( 'NONE',  ( -17.29985003582992320, -10.77366814457252175, 33.85459836347579454 ) ) ;
#69167=CARTESIAN_POINT ( 'NONE',  ( 5.076923076922953193, -2.379036618888197729, 30.90682066428292885 ) ) ;
#69168=CARTESIAN_POINT ( 'NONE',  ( -1.384615384615383471, -4.661471528628507777, 34.16647553114623292 ) ) ;
#69169=CARTESIAN_POINT ( 'NONE',  ( 2.557637717070352590, -6.653508905675590945, 34.93172785388651391 ) ) ;
#69170=EDGE_CURVE ( 'NONE', #87106, #5632, #85571, .T. ) ;
#69171=CARTESIAN_POINT ( 'NONE',  ( -18.06527044596078113, -10.21337939537584560, 33.94971097300158647 ) ) ;
#69173=ORIENTED_EDGE ( 'NONE', *, *, #24273, .F. ) ;
#69174=CARTESIAN_POINT ( 'NONE',  ( -5.933932666649923249, -10.67929555188718282, 33.92786785259544757 ) ) ;
#69175=ORIENTED_EDGE ( 'NONE', *, *, #44181, .F. ) ;
#69176=CARTESIAN_POINT ( 'NONE',  ( -15.16470087976679260, -4.098570777380720287, 33.41473453929635440 ) ) ;
#69177=EDGE_LOOP ( 'NONE', ( #76649, #59396, #52738, #62862 ) ) ;
#69178=CARTESIAN_POINT ( 'NONE',  ( -11.40793610022789828, -6.808710257144161559, 34.95449254468098843 ) ) ;
#69179=CARTESIAN_POINT ( 'NONE',  ( -7.911424292114620727, -10.21337939537584383, 33.94971097300158647 ) ) ;
#69180=ORIENTED_EDGE ( 'NONE', *, *, #37717, .T. ) ;
#69181=DIRECTION ( 'NONE',  ( -0.000000000000000000, 0.8660254037844397068, -0.4999999999999978906 ) ) ;
#69183=CARTESIAN_POINT ( 'NONE',  ( 4.087762742890273415, -8.973038597847269315, 34.52809138561120506 ) ) ;
#69184=CARTESIAN_POINT ( 'NONE',  ( -7.053224892808620083, -12.70455904226513866, 30.44083106164009322 ) ) ;
#69185=LINE ( 'NONE', #62848, #23053 ) ;
#69186=CARTESIAN_POINT ( 'NONE',  ( -17.07692307692307665, -1.367168528481310208, 33.57946703557072254 ) ) ;
#69187=CARTESIAN_POINT ( 'NONE',  ( -1.134669975237340589, -6.653508905675590945, 34.93172785388651391 ) ) ;
#69188=CARTESIAN_POINT ( 'NONE',  ( -5.999999999999998224, -10.51840700105979565, 33.73612834413961536 ) ) ;
#69190=CARTESIAN_POINT ( 'NONE',  ( -9.692307692307691624, -3.513871655860378418, 32.76840700105978499 ) ) ;
#69191=CARTESIAN_POINT ( 'NONE',  ( 1.384615384615265343, -11.94971097300221174, 32.03036669348237098 ) ) ;
#69192=EDGE_LOOP ( 'NONE', ( #81547, #53749 ) ) ;
#69193=VECTOR ( 'NONE', #28636, 1000.000000000000227 ) ;
#69194=LINE ( 'NONE', #22336, #87323 ) ;
#69196=EDGE_CURVE ( 'NONE', #24412, #28929, #29246, .T. ) ;
#69198=LINE ( 'NONE', #28201, #48376 ) ;
#69199=EDGE_LOOP ( 'NONE', ( #50900, #18425 ) ) ;
#69200=EDGE_CURVE ( 'NONE', #74216, #49742, #4511, .T. ) ;
#69201=CARTESIAN_POINT ( 'NONE',  ( 1.384615384615386802, -8.164416787775445883, 34.95778746994557906 ) ) ;
#69202=CARTESIAN_POINT ( 'NONE',  ( 16.28437159207980045, -2.647132371071621471, 31.75357179365173010 ) ) ;
#69203=CARTESIAN_POINT ( 'NONE',  ( -16.94608465891031557, -7.277220443632451463, 34.74524770363009196 ) ) ;
#69204=ORIENTED_EDGE ( 'NONE', *, *, #17818, .F. ) ;
#69205=CYLINDRICAL_SURFACE ( 'NONE', #45501, 0.2500000000000004996 ) ;
#69206=CARTESIAN_POINT ( 'NONE',  ( -16.21992956480203318, -10.51840700105979565, 33.73612834413961536 ) ) ;
#69207=CARTESIAN_POINT ( 'NONE',  ( 16.02315468717859304, -8.999036380462719364, 34.52022231692819076 ) ) ;
#69208=ADVANCED_FACE ( 'NONE', ( #17104 ), #44559, .F. ) ;
#69209=CARTESIAN_POINT ( 'NONE',  ( 0.4615384615383396616, -12.46129190930018460, 30.37095296980731973 ) ) ;
#69210=FACE_OUTER_BOUND ( 'NONE', #70108, .T. ) ;
#69211=EDGE_CURVE ( 'NONE', #87523, #8641, #77481, .T. ) ;
#69212=ORIENTED_EDGE ( 'NONE', *, *, #658, .F. ) ;
#69213=ORIENTED_EDGE ( 'NONE', *, *, #28539, .T. ) ;
#69214=ORIENTED_EDGE ( 'NONE', *, *, #28878, .F. ) ;
#69215=VECTOR ( 'NONE', #72011, 1000.000000000000227 ) ;
#69217=CARTESIAN_POINT ( 'NONE',  ( -4.087777802843713282, -3.050289026998446840, 32.03036669348366416 ) ) ;
#69218=CYLINDRICAL_SURFACE ( 'NONE', #44984, 0.2499999999999986955 ) ;
#69219=DIRECTION ( 'NONE',  ( 0.000000000000000000, 0.4999999999999985567, 0.8660254037844395958 ) ) ;
#69220=EDGE_CURVE ( 'NONE', #35285, #43192, #35625, .T. ) ;
#69221=AXIS2_PLACEMENT_3D ( 'NONE', #13905, #87827, #6705 ) ;
#69222=ORIENTED_EDGE ( 'NONE', *, *, #49098, .T. ) ;
#69223=CARTESIAN_POINT ( 'NONE',  ( -12.46153846153858424, -5.094484230521993062, 34.41647553114689373 ) ) ;
#69224=ORIENTED_EDGE ( 'NONE', *, *, #62181, .F. ) ;
#69225=EDGE_CURVE ( 'NONE', #48928, #50148, #78356, .T. ) ;
#69226=EDGE_CURVE ( 'NONE', #62924, #3792, #77046, .T. ) ;
#69229=CARTESIAN_POINT ( 'NONE',  ( 8.638540166120463937, -12.35290016733513951, 31.75349464988449455 ) ) ;
#69230=ORIENTED_EDGE ( 'NONE', *, *, #82677, .F. ) ;
#69231=CARTESIAN_POINT ( 'NONE',  ( -0.6850234052624097902, -5.113361153441934093, 34.14387501736622710 ) ) ;
#69232=EDGE_CURVE ( 'NONE', #74248, #29230, #12010, .T. ) ;
#69233=CARTESIAN_POINT ( 'NONE',  ( -3.480745974817820887, -12.01397095200673881, 32.43157075238190146 ) ) ;
#69234=B_SPLINE_CURVE_WITH_KNOTS ( 'NONE', 3,
 ( #79584, #25074, #80473, #10676, #45784, #37694, #16984, #79132, #18769, #44433 ),
 .UNSPECIFIED., .F., .F.,
 ( 4, 2, 2, 2, 4 ),
 ( 0.0007817359430256232838, 0.0009771253907249928539, 0.001172514838424355485, 0.001367904286123718116, 0.001563293733823080747 ),
 .UNSPECIFIED. ) ;
#69236=CARTESIAN_POINT ( 'NONE',  ( 1.384615384615386802, -4.786620604624113540, 33.94971097300155094 ) ) ;
#69237=VERTEX_POINT ( 'NONE', #22974 ) ;
#69238=ORIENTED_EDGE ( 'NONE', *, *, #56547, .T. ) ;
#69240=CARTESIAN_POINT ( 'NONE',  ( -14.05769230769237055, -7.565270445406050648, 34.75000000000000000 ) ) ;
#69242=ORIENTED_EDGE ( 'NONE', *, *, #81799, .T. ) ;
#69244=LINE ( 'NONE', #35010, #69558 ) ;
#69245=VERTEX_POINT ( 'NONE', #16224 ) ;
#69246=B_SPLINE_CURVE_WITH_KNOTS ( 'NONE', 3,
 ( #71405, #9710, #71854, #65087, #30430, #29992, #2945, #36314, #3394, #51119 ),
 .UNSPECIFIED., .F., .F.,
 ( 4, 2, 2, 2, 4 ),
 ( 0.0007817359430256221996, 0.0009771253907249863487, 0.001172514838424350498, 0.001367904286123714647, 0.001563293733823078796 ),
 .UNSPECIFIED. ) ;
#69247=AXIS2_PLACEMENT_3D ( 'NONE', #23530, #50985, #15468 ) ;
#69248=CARTESIAN_POINT ( 'NONE',  ( -4.153846153846273204, -5.219633306517616589, 34.19971097300220464 ) ) ;
#69249=CARTESIAN_POINT ( 'NONE',  ( 12.68455130563185662, -9.172514111537584114, 34.72667873470787470 ) ) ;
#69250=ORIENTED_EDGE ( 'NONE', *, *, #27313, .F. ) ;
#69251=FACE_BOUND ( 'NONE', #15058, .T. ) ;
#69252=CARTESIAN_POINT ( 'NONE',  ( -17.86947429823644029, -8.586989748646450593, 34.63063291749215011 ) ) ;
#69253=CARTESIAN_POINT ( 'NONE',  ( -24.00000000000000000, -5.499999999999981348, 27.75000000000000000 ) ) ;
#69254=B_SPLINE_CURVE_WITH_KNOTS ( 'NONE', 3,
 ( #14461, #40174, #82490, #47799, #21209, #75280, #67637, #41939, #20769, #33408 ),
 .UNSPECIFIED., .F., .F.,
 ( 4, 2, 2, 2, 4 ),
 ( 0.000000000000000000, 0.0001954311584214072923, 0.0003908623168428145846, 0.0005862934752642218498, 0.0007817246336856291692 ),
 .UNSPECIFIED. ) ;
#69255=ADVANCED_FACE ( 'NONE', ( #71158 ), #2690, .F. ) ;
#69256=CARTESIAN_POINT ( 'NONE',  ( 3.230769230769231726, -8.973038597847269315, 34.52809138561121927 ) ) ;
#69257=DIRECTION ( 'NONE',  ( -0.000000000000000000, 0.5000000000000011102, -0.8660254037844380415 ) ) ;
#69259=DIRECTION ( 'NONE',  ( -0.000000000000000000, 0.1736481776669307198, -0.9848077530122080203 ) ) ;
#69260=CARTESIAN_POINT ( 'NONE',  ( 0.7115384615384606759, -2.249999999999998668, 29.75000000000000355 ) ) ;
#69261=EDGE_LOOP ( 'NONE', ( #66567, #675, #35438, #65347, #6431, #38070 ) ) ;
#69262=CARTESIAN_POINT ( 'NONE',  ( -16.15384615384615330, -13.20930481340135110, 34.54067556320372745 ) ) ;
#69263=CARTESIAN_POINT ( 'NONE',  ( 13.25413867649892552, -7.276988635370452485, 34.74523720219453793 ) ) ;
#69264=EDGE_LOOP ( 'NONE', ( #14994, #48972 ) ) ;
#69265=EDGE_CURVE ( 'NONE', #76524, #12327, #14065, .T. ) ;
#69266=CARTESIAN_POINT ( 'NONE',  ( 8.638539302563209787, -3.062553014421049546, 32.05460306192773601 ) ) ;
#69267=CARTESIAN_POINT ( 'NONE',  ( -4.403869378067608586, -3.520140089381497361, 33.17453946501458262 ) ) ;
#69268=ORIENTED_EDGE ( 'NONE', *, *, #34369, .T. ) ;
#69269=FACE_OUTER_BOUND ( 'NONE', #45182, .T. ) ;
#69271=FACE_BOUND ( 'NONE', #41014, .T. ) ;
#69272=CARTESIAN_POINT ( 'NONE',  ( 7.846153846153846700, -2.708943851104267164, 35.45975837776705220 ) ) ;
#69273=CARTESIAN_POINT ( 'NONE',  ( 4.153846153846154188, -12.34228464037088635, 31.77849191805839268 ) ) ;
#69274=FACE_OUTER_BOUND ( 'NONE', #19905, .T. ) ;
#69279=EDGE_CURVE ( 'NONE', #71146, #52853, #206, .T. ) ;
#69280=DIRECTION ( 'NONE',  ( -0.000000000000000000, 0.8660254037844397068, -0.4999999999999978906 ) ) ;
#69282=ORIENTED_EDGE ( 'NONE', *, *, #75265, .T. ) ;
#69283=VECTOR ( 'NONE', #87669, 1000.000000000000227 ) ;
#69284=ORIENTED_EDGE ( 'NONE', *, *, #28238, .F. ) ;
#69285=CARTESIAN_POINT ( 'NONE',  ( -23.00000000000000000, -9.499999999999982236, 27.74999999999999645 ) ) ;
#69286=CARTESIAN_POINT ( 'NONE',  ( -0.7115616988314267255, -2.823816976329320827, 31.52131813110797154 ) ) ;
#69287=CARTESIAN_POINT ( 'NONE',  ( 1.607628228708781748, -9.172514111537584114, 34.72667873470787470 ) ) ;
#69288=CARTESIAN_POINT ( 'NONE',  ( -1.514762594053604250, -3.285722584762969856, 32.44110544564090759 ) ) ;
#69289=CARTESIAN_POINT ( 'NONE',  ( -9.692307692307814193, -12.51329471203414379, 31.30864560766407578 ) ) ;
#69291=VECTOR ( 'NONE', #16140, 1000.000000000000114 ) ;
#69292=B_SPLINE_CURVE_WITH_KNOTS ( 'NONE', 3,
 ( #41624, #66548, #20897, #56016, #18806, #6946, #34416, #87728, #83504, #21790 ),
 .UNSPECIFIED., .F., .F.,
 ( 4, 2, 2, 2, 4 ),
 ( 0.000000000000000000, 0.0001954311564186858715, 0.0003908623128373717431, 0.0005862934692560576146, 0.0007817246256747434861 ),
 .UNSPECIFIED. ) ;
#69293=CYLINDRICAL_SURFACE ( 'NONE', #82024, 0.2499999999999986955 ) ;
#69294=B_SPLINE_CURVE_WITH_KNOTS ( 'NONE', 3,
 ( #42120, #33251, #46311, #67481, #12101, #60712, #21836, #76784, #88219, #2871 ),
 .UNSPECIFIED., .F., .F.,
 ( 4, 2, 2, 2, 4 ),
 ( 0.0007817246256747465219, 0.0009771112852218900684, 0.001172497944769033615, 0.001367884604316177378, 0.001563271263863320925 ),
 .UNSPECIFIED. ) ;
#69295=CARTESIAN_POINT ( 'NONE',  ( 1.254467414883691401, -10.31621877034669588, 34.18098118002070152 ) ) ;
#69296=EDGE_CURVE ( 'NONE', #18061, #86451, #80608, .T. ) ;
#69297=CARTESIAN_POINT ( 'NONE',  ( -17.30040802064702987, -5.113361153441931428, 34.14387501736621999 ) ) ;
#69298=CARTESIAN_POINT ( 'NONE',  ( 7.780071466793711643, -5.471508081941601986, 34.59228464037088457 ) ) ;
#69300=LINE ( 'NONE', #76498, #19527 ) ;
#69301=B_SPLINE_CURVE_WITH_KNOTS ( 'NONE', 3,
 ( #67454, #88195, #26471, #13830, #82745, #20151, #68774, #48494, #21018, #40870 ),
 .UNSPECIFIED., .F., .F.,
 ( 4, 2, 2, 2, 4 ),
 ( 0.000000000000000000, 0.0001954311564186863323, 0.0003908623128373726646, 0.0005862934692560590241, 0.0007817246256747453293 ),
 .UNSPECIFIED. ) ;
#69302=CARTESIAN_POINT ( 'NONE',  ( -9.915234651214539952, -12.64616026154729411, 30.79003144601914244 ) ) ;
#69303=CARTESIAN_POINT ( 'NONE',  ( 10.86538461538603606, -7.500000000000154543, 35.00000000000007105 ) ) ;
#69304=CARTESIAN_POINT ( 'NONE',  ( -12.46153846153815437, -2.506253911140614576, 30.00000000000323297 ) ) ;
#69306=CARTESIAN_POINT ( 'NONE',  ( -0.2385271099256121019, -3.587049720035815348, 32.86302985866382897 ) ) ;
#69307=CARTESIAN_POINT ( 'NONE',  ( -0.4615384615384611200, -9.905515769479276145, 34.41647553114623292 ) ) ;
#69309=EDGE_CURVE ( 'NONE', #8757, #29571, #50595, .T. ) ;
#69310=CARTESIAN_POINT ( 'NONE',  ( -6.000000000000121680, -12.51329471203414379, 31.30864560766407578 ) ) ;
#69312=VERTEX_POINT ( 'NONE', #26092 ) ;
#69314=CARTESIAN_POINT ( 'NONE',  ( -14.55766903863466055, -12.17611988154120972, 31.52148481390971213 ) ) ;
#69315=VERTEX_POINT ( 'NONE', #11245 ) ;
#69316=CARTESIAN_POINT ( 'NONE',  ( 6.923076923076802558, -3.835265460704628371, 33.15142922262033665 ) ) ;
#69317=EDGE_CURVE ( 'NONE', #86321, #32791, #38714, .T. ) ;
#69318=CARTESIAN_POINT ( 'NONE',  ( 12.68455130563185840, -5.582272713120729257, 34.63742843783360570 ) ) ;
#69319=ORIENTED_EDGE ( 'NONE', *, *, #23441, .T. ) ;
#69320=CARTESIAN_POINT ( 'NONE',  ( 5.076923076923075762, -13.20930481340135110, 34.54067556320372745 ) ) ;
#69322=ORIENTED_EDGE ( 'NONE', *, *, #8517, .F. ) ;
#69324=CARTESIAN_POINT ( 'NONE',  ( 14.05771557674995265, -2.564618984488975517, 30.55390908950641915 ) ) ;
#69325=CARTESIAN_POINT ( 'NONE',  ( 7.846153846153846700, -12.34228464037088635, 31.77849191805839268 ) ) ;
#69326=EDGE_CURVE ( 'NONE', #86793, #47021, #78511, .T. ) ;
#69328=ORIENTED_EDGE ( 'NONE', *, *, #68142, .F. ) ;
#69329=ORIENTED_EDGE ( 'NONE', *, *, #87668, .F. ) ;
#69330=CARTESIAN_POINT ( 'NONE',  ( 2.980746006547773330, -2.985938066672154445, 32.43141759479405550 ) ) ;
#69331=ORIENTED_EDGE ( 'NONE', *, *, #56584, .F. ) ;
#69332=DIRECTION ( 'NONE',  ( -0.000000000000000000, 0.9848077530122086864, -0.1736481776669273891 ) ) ;
#69333=CARTESIAN_POINT ( 'NONE',  ( 15.29683656411930848, -12.62096338111211757, 30.90682066428152908 ) ) ;
#69335=B_SPLINE_CURVE_WITH_KNOTS ( 'NONE', 3,
 ( #71915, #63832, #29183, #50744, #43995, #2128, #70147, #63385, #1693, #84566 ),
 .UNSPECIFIED., .F., .F.,
 ( 4, 2, 2, 2, 4 ),
 ( 0.0007817359527651096280, 0.0009771254036996484919, 0.001172514854634187573, 0.001367904305568726653, 0.001563293756503265517 ),
 .UNSPECIFIED. ) ;
#69336=FACE_OUTER_BOUND ( 'NONE', #39339, .T. ) ;
#69337=DIRECTION ( 'NONE',  ( 0.000000000000000000, 0.7660444431189807890, 0.6427876096865361433 ) ) ;
#69338=CARTESIAN_POINT ( 'NONE',  ( 0.7115384615398802071, -7.500000000000154543, 35.00000000000007105 ) ) ;
#69339=EDGE_CURVE ( 'NONE', #88144, #23339, #51757, .T. ) ;
#69340=CARTESIAN_POINT ( 'NONE',  ( 3.230769230769231726, -13.53365097954675988, 30.81389545987213552 ) ) ;
#69341=EDGE_CURVE ( 'NONE', #75936, #60370, #25888, .T. ) ;
#69342=EDGE_CURVE ( 'NONE', #75886, #88472, #65728, .T. ) ;
#69343=ORIENTED_EDGE ( 'NONE', *, *, #13606, .T. ) ;
#69345=CARTESIAN_POINT ( 'NONE',  ( -0.2385271099256117133, -12.15243808032445827, 31.58219941686247978 ) ) ;
#69346=ORIENTED_EDGE ( 'NONE', *, *, #42587, .T. ) ;
#69347=CARTESIAN_POINT ( 'NONE',  ( 17.07692307692295586, -2.379036618888197729, 30.90682066428292885 ) ) ;
#69349=ORIENTED_EDGE ( 'NONE', *, *, #42587, .F. ) ;
#69350=AXIS2_PLACEMENT_3D ( 'NONE', #4527, #65769, #4068 ) ;
#69352=CARTESIAN_POINT ( 'NONE',  ( -7.846153846153844924, -9.905515769479276145, 34.41647553114623292 ) ) ;
#69353=VERTEX_POINT ( 'NONE', #86480 ) ;
#69354=CARTESIAN_POINT ( 'NONE',  ( -9.692307692307384315, -2.506253911140614576, 30.00000000000323297 ) ) ;
#69356=ORIENTED_EDGE ( 'NONE', *, *, #74797, .F. ) ;
#69357=CARTESIAN_POINT ( 'NONE',  ( -16.15384615384615330, -3.513871655860378418, 32.76840700105978499 ) ) ;
#69358=ORIENTED_EDGE ( 'NONE', *, *, #62549, .T. ) ;
#69359=CARTESIAN_POINT ( 'NONE',  ( -12.59168643127015841, -3.625366637846544116, 33.29286588640298561 ) ) ;
#69360=ORIENTED_EDGE ( 'NONE', *, *, #87170, .F. ) ;
#69361=CARTESIAN_POINT ( 'NONE',  ( 17.74997676270703550, -10.76384336483936011, 33.53834819971076087 ) ) ;
#69362=CARTESIAN_POINT ( 'NONE',  ( -8.834501215191544077, -2.892918686051582977, 31.69288490824015980 ) ) ;
#69363=FACE_BOUND ( 'NONE', #9100, .T. ) ;
#69367=DIRECTION ( 'NONE',  ( 0.000000000000000000, 0.3420201433256641055, -0.9396926207859100932 ) ) ;
#69368=CARTESIAN_POINT ( 'NONE',  ( -17.14219307747939425, -8.656820664281497102, 34.87096338111211935 ) ) ;
#69369=CARTESIAN_POINT ( 'NONE',  ( 10.36536139116315525, -10.92453946501458795, 33.72985991061850086 ) ) ;
#69370=ORIENTED_EDGE ( 'NONE', *, *, #63665, .F. ) ;
#69371=CARTESIAN_POINT ( 'NONE',  ( -14.24243673641627339, -3.835265460703683349, 33.15142922261929925 ) ) ;
#69372=EDGE_LOOP ( 'NONE', ( #12750, #61883 ) ) ;
#69373=ORIENTED_EDGE ( 'NONE', *, *, #86095, .T. ) ;
#69374=CARTESIAN_POINT ( 'NONE',  ( 6.923076923076802558, -5.219633306517616589, 34.19971097300220464 ) ) ;
#69375=CARTESIAN_POINT ( 'NONE',  ( 13.38461538461538680, -1.242168528481310874, 33.36296068462461051 ) ) ;
#69376=AXIS2_PLACEMENT_3D ( 'NONE', #88236, #25617, #42135 ) ;
#69377=CARTESIAN_POINT ( 'NONE',  ( 2.307692307692187583, -12.46129190930018460, 30.37095296980731973 ) ) ;
#69378=CARTESIAN_POINT ( 'NONE',  ( -16.94639763868943660, -10.31582465632704704, 34.18122507451815295 ) ) ;
#69379=CARTESIAN_POINT ( 'NONE',  ( -10.54931728203453822, -12.34228464037088813, 31.77849191805839268 ) ) ;
#69380=CARTESIAN_POINT ( 'NONE',  ( 13.38461538461526601, -11.48612834414049644, 32.76840700105863391 ) ) ;
#69381=EDGE_LOOP ( 'NONE', ( #76659, #41475, #35974, #76655 ) ) ;
#69382=CARTESIAN_POINT ( 'NONE',  ( 13.16113044089144068, -5.113361153441934093, 34.14387501736622710 ) ) ;
#69383=LINE ( 'NONE', #49983, #56034 ) ;
#69384=CARTESIAN_POINT ( 'NONE',  ( 17.01165307636676260, -4.320704448112772766, 33.92786785259540494 ) ) ;
#69386=LINE ( 'NONE', #35149, #80805 ) ;
#69387=AXIS2_PLACEMENT_3D ( 'NONE', #40094, #67109, #18916 ) ;
#69388=EDGE_LOOP ( 'NONE', ( #76958, #70333, #9893, #60147 ) ) ;
#69389=ORIENTED_EDGE ( 'NONE', *, *, #63249, .T. ) ;
#69392=CARTESIAN_POINT ( 'NONE',  ( -6.130690603110309667, -3.957541250942359756, 33.62499894934981626 ) ) ;
#69393=ORIENTED_EDGE ( 'NONE', *, *, #936, .T. ) ;
#69394=DIRECTION ( 'NONE',  ( 0.000000000000000000, 0.8660254037844377084, 0.5000000000000015543 ) ) ;
#69395=CARTESIAN_POINT ( 'NONE',  ( -12.39547011053602432, -6.386643153685127139, 34.62446782046654192 ) ) ;
#69396=FACE_OUTER_BOUND ( 'NONE', #85222, .T. ) ;
#69398=CARTESIAN_POINT ( 'NONE',  ( 12.21151522424549896, -10.05641848906368097, 34.04755513067966177 ) ) ;
#69399=ORIENTED_EDGE ( 'NONE', *, *, #29382, .F. ) ;
#69400=CARTESIAN_POINT ( 'NONE',  ( 11.28846153846153832, -2.499999999999998668, 29.75000000000000355 ) ) ;
#69401=CARTESIAN_POINT ( 'NONE',  ( -0.6850233861027916760, -5.827078755546623690, 34.72654668319379567 ) ) ;
#69402=VERTEX_POINT ( 'NONE', #80151 ) ;
#69403=CARTESIAN_POINT ( 'NONE',  ( 2.307692307692309264, -6.343179335718451384, 34.87096338111211935 ) ) ;
#69404=CARTESIAN_POINT ( 'NONE',  ( -17.07692307692307665, -8.120952969808772792, 34.71129190930000163 ) ) ;
#69405=CARTESIAN_POINT ( 'NONE',  ( 16.85399685940691938, -3.586966769969702540, 32.86292498521069660 ) ) ;
#69406=CARTESIAN_POINT ( 'NONE',  ( 8.900021210197715860, -11.93129842949671726, 32.56571108434900452 ) ) ;
#69407=CARTESIAN_POINT ( 'NONE',  ( -12.68502340526240957, -2.847400154188067578, 31.58180166144859058 ) ) ;
#69408=CARTESIAN_POINT ( 'NONE',  ( 18.00000000000000000, -12.29105614889573062, 35.45975837776705220 ) ) ;
#69409=CARTESIAN_POINT ( 'NONE',  ( -12.59168567097668401, -12.45813303252208648, 30.39737893381572675 ) ) ;
#69411=ORIENTED_EDGE ( 'NONE', *, *, #16208, .F. ) ;
#69412=DIRECTION ( 'NONE',  ( -0.000000000000000000, 0.9848077530122085754, -0.1736481776669273613 ) ) ;
#69415=DIRECTION ( 'NONE',  ( 0.000000000000000000, 0.7660444431189807890, 0.6427876096865361433 ) ) ;
#69416=CARTESIAN_POINT ( 'NONE',  ( -3.100243792535588128, -11.04252011169590020, 33.62494198852677130 ) ) ;
#69417=ORIENTED_EDGE ( 'NONE', *, *, #18090, .T. ) ;
#69418=CARTESIAN_POINT ( 'NONE',  ( -9.692307692307691624, -3.513871655860378418, 32.76840700105978499 ) ) ;
#69419=CARTESIAN_POINT ( 'NONE',  ( -16.08859058257012720, -12.27809138561124591, 31.22303859784720359 ) ) ;
#69420=VECTOR ( 'NONE', #85487, 1000.000000000000000 ) ;
#69421=CARTESIAN_POINT ( 'NONE',  ( -0.6850233861027934523, -12.69144148231606017, 30.53333754910549303 ) ) ;
#69422=CARTESIAN_POINT ( 'NONE',  ( 14.08476609017615644, -3.105860786376062332, 32.13614157043599562 ) ) ;
#69424=CARTESIAN_POINT ( 'NONE',  ( -12.33101275977490197, -9.417988943895561960, 34.36773134775777550 ) ) ;
#69425=EDGE_CURVE ( 'NONE', #69684, #7426, #68403, .T. ) ;
#69426=DIRECTION ( 'NONE',  ( 0.000000000000000000, 0.8660254037844377084, -0.5000000000000015543 ) ) ;
#69427=CARTESIAN_POINT ( 'NONE',  ( -14.05769230769224265, -7.434744860731433924, 35.00000000000000711 ) ) ;
#69428=ORIENTED_EDGE ( 'NONE', *, *, #34021, .T. ) ;
#69429=FACE_OUTER_BOUND ( 'NONE', #36069, .T. ) ;
#69430=EDGE_LOOP ( 'NONE', ( #16778, #62693, #42265, #68249 ) ) ;
#69432=CARTESIAN_POINT ( 'NONE',  ( 4.826899852701619587, -5.765609946408404518, 34.70566812827425451 ) ) ;
#69434=LINE ( 'NONE', #20371, #79286 ) ;
#69435=CARTESIAN_POINT ( 'NONE',  ( -8.769230769230768274, -2.538708090699994813, 30.37095296980875503 ) ) ;
#69436=CARTESIAN_POINT ( 'NONE',  ( 13.25446817517716447, -6.852621066184266141, 34.70813303252209181 ) ) ;
#69437=VECTOR ( 'NONE', #18701, 1000.000000000000227 ) ;
#69438=AXIS2_PLACEMENT_3D ( 'NONE', #10243, #45341, #79139 ) ;
#69440=CARTESIAN_POINT ( 'NONE',  ( -18.00000000000000000, -2.833524468853757305, 32.15551576947926549 ) ) ;
#69441=EDGE_CURVE ( 'NONE', #74870, #38427, #69735, .T. ) ;
#69442=EDGE_CURVE ( 'NONE', #2529, #85483, #5465, .T. ) ;
#69443=EDGE_LOOP ( 'NONE', ( #42448, #34756 ) ) ;
#69444=ORIENTED_EDGE ( 'NONE', *, *, #20584, .T. ) ;
#69445=FACE_BOUND ( 'NONE', #25278, .T. ) ;
#69446=ORIENTED_EDGE ( 'NONE', *, *, #11144, .T. ) ;
#69447=DIRECTION ( 'NONE',  ( -0.000000000000000000, -0.9848077530122086864, -0.1736481776669273613 ) ) ;
#69449=CARTESIAN_POINT ( 'NONE',  ( -5.076923076923075762, -11.91647553114624181, 32.58852847137148245 ) ) ;
#69450=FACE_OUTER_BOUND ( 'NONE', #65500, .T. ) ;
#69451=CARTESIAN_POINT ( 'NONE',  ( 6.923076923076924238, -9.780366693483667717, 34.19971097300155094 ) ) ;
#69453=EDGE_LOOP ( 'NONE', ( #88823, #11956 ) ) ;
#69454=VERTEX_POINT ( 'NONE', #81935 ) ;
#69456=ORIENTED_EDGE ( 'NONE', *, *, #45283, .T. ) ;
#69458=CARTESIAN_POINT ( 'NONE',  ( -9.442307692306256328, -7.500000000000155431, 34.75000000000007105 ) ) ;
#69459=CARTESIAN_POINT ( 'NONE',  ( -18.00000000000012079, -11.48612834414049644, 32.76840700105863391 ) ) ;
#69460=VECTOR ( 'NONE', #76908, 1000.000000000000000 ) ;
#69461=CARTESIAN_POINT ( 'NONE',  ( -1.161652481053898844, -7.369474270740069777, 34.74850911626239736 ) ) ;
#69463=DIRECTION ( 'NONE',  ( 0.000000000000000000, 1.000000000000000000, 0.000000000000000000 ) ) ;
#69464=CARTESIAN_POINT ( 'NONE',  ( -14.30769230769230660, -4.661471528628507777, 34.16647553114623292 ) ) ;
#69465=CARTESIAN_POINT ( 'NONE',  ( -5.076923076923197442, -3.835265460704628371, 33.15142922262033665 ) ) ;
#69467=EDGE_LOOP ( 'NONE', ( #35841, #8567, #46056, #1377, #67472, #50210 ) ) ;
#69468=CIRCLE ( 'NONE', #70894, 2.000000000000001776 ) ;
#69469=EDGE_LOOP ( 'NONE', ( #53935, #48346, #65406, #44494 ) ) ;
#69470=CARTESIAN_POINT ( 'NONE',  ( 3.360816666019682764, -7.723484941389743952, 34.99544897038808955 ) ) ;
#69471=DIRECTION ( 'NONE',  ( 0.000000000000000000, 0.9848077530122072432, -0.1736481776669354937 ) ) ;
#69472=CARTESIAN_POINT ( 'NONE',  ( 10.48469401227430886, -2.295517848115769421, 30.44137282052137294 ) ) ;
#69473=DIRECTION ( 'NONE',  ( 0.000000000000000000, 0.4999999999999985567, 0.8660254037844395958 ) ) ;
#69474=CARTESIAN_POINT ( 'NONE',  ( -3.453695448285377445, -11.24512374952581872, 33.06303171183252942 ) ) ;
#69475=FACE_BOUND ( 'NONE', #20383, .T. ) ;
#69476=CARTESIAN_POINT ( 'NONE',  ( 16.15384615384603251, -3.300289026999228437, 32.46337939537709616 ) ) ;
#69477=ORIENTED_EDGE ( 'NONE', *, *, #17759, .F. ) ;
#69478=CARTESIAN_POINT ( 'NONE',  ( -7.911476761646023093, -7.749976743299138882, 34.99404534957040624 ) ) ;
#69479=CARTESIAN_POINT ( 'NONE',  ( 9.442284468086237226, -12.07920672191015221, 32.31858351112116168 ) ) ;
#69480=CARTESIAN_POINT ( 'NONE',  ( 3.230769230769231726, -13.75783147151868846, 33.36296068462461051 ) ) ;
#69481=CARTESIAN_POINT ( 'NONE',  ( 5.076923076923075762, -12.29105614889573062, 35.45975837776705220 ) ) ;
#69483=CARTESIAN_POINT ( 'NONE',  ( 2.557637826040451756, -11.86320923018887719, 32.19269448109604781 ) ) ;
#69484=ORIENTED_EDGE ( 'NONE', *, *, #15509, .T. ) ;
#69485=FACE_BOUND ( 'NONE', #59817, .T. ) ;
#69487=B_SPLINE_CURVE_WITH_KNOTS ( 'NONE', 3,
 ( #22675, #77622, #36210, #10499, #37968, #37066, #15931, #63661, #23994, #84842 ),
 .UNSPECIFIED., .F., .F.,
 ( 4, 2, 2, 2, 4 ),
 ( 0.000000000000000000, 0.0001954339857564063360, 0.0003908679715128126719, 0.0005863019572692189808, 0.0007817359430256253438 ),
 .UNSPECIFIED. ) ;
#69488=CARTESIAN_POINT ( 'NONE',  ( 17.07692307692307665, -11.69971097300155272, 32.46337939537588113 ) ) ;
#69489=CARTESIAN_POINT ( 'NONE',  ( -12.46153846153858424, -12.16647553114689728, 32.15551576947799362 ) ) ;
#69490=ORIENTED_EDGE ( 'NONE', *, *, #62921, .T. ) ;
#69491=DIRECTION ( 'NONE',  ( -0.000000000000000000, 0.6427876096865404731, -0.7660444431189770143 ) ) ;
#69492=CARTESIAN_POINT ( 'NONE',  ( -17.93393266664992325, -3.937682226553330445, 33.60647404775216529 ) ) ;
#69493=CARTESIAN_POINT ( 'NONE',  ( 3.230769230769231726, -11.16473453929635440, 33.15142922261926373 ) ) ;
#69494=CARTESIAN_POINT ( 'NONE',  ( -17.86920955903305597, -12.62708834333097663, 30.88030960425256310 ) ) ;
#69498=ORIENTED_EDGE ( 'NONE', *, *, #3173, .T. ) ;
#69499=CARTESIAN_POINT ( 'NONE',  ( 16.02337096877043621, -7.276987145209182550, 34.99546412871779211 ) ) ;
#69500=ORIENTED_EDGE ( 'NONE', *, *, #74949, .F. ) ;
#69501=CARTESIAN_POINT ( 'NONE',  ( -18.13049666469081700, -12.75000000000001066, 29.52694327409752262 ) ) ;
#69502=CARTESIAN_POINT ( 'NONE',  ( -4.403869391139119571, -2.823816976329319495, 31.52131813110795733 ) ) ;
#69503=CARTESIAN_POINT ( 'NONE',  ( 13.13459214732242408, -9.271318131107980420, 34.42618302367067429 ) ) ;
#69506=CARTESIAN_POINT ( 'NONE',  ( -5.934744860487159102, -6.835583212224609184, 34.95778746994559327 ) ) ;
#69507=CARTESIAN_POINT ( 'NONE',  ( 16.21910172512217585, -6.026961402152790193, 34.52809138561124769 ) ) ;
#69508=CARTESIAN_POINT ( 'NONE',  ( 12.68496542340003508, -7.630147231320743018, 34.74852402298682819 ) ) ;
#69510=EDGE_LOOP ( 'NONE', ( #9718, #6627 ) ) ;
#69511=CYLINDRICAL_SURFACE ( 'NONE', #33252, 0.2499999999999998890 ) ;
#69512=ORIENTED_EDGE ( 'NONE', *, *, #8745, .T. ) ;
#69513=EDGE_CURVE ( 'NONE', #18739, #47404, #41382, .T. ) ;
#69514=ORIENTED_EDGE ( 'NONE', *, *, #8728, .F. ) ;
#69515=CARTESIAN_POINT ( 'NONE',  ( -17.07692307692307665, -2.499999999999998668, 29.75000000000001421 ) ) ;
#69516=ORIENTED_EDGE ( 'NONE', *, *, #87775, .T. ) ;
#69517=DIRECTION ( 'NONE',  ( 0.000000000000000000, 0.1736481776669267785, -0.9848077530122087975 ) ) ;
#69518=UNCERTAINTY_MEASURE_WITH_UNIT (LENGTH_MEASURE( 1.000000000000000082E-05 ), #80625, 'distance_accuracy_value', 'NONE');
#69520=CARTESIAN_POINT ( 'NONE',  ( -11.31568186948346622, -10.23759521482555357, 34.22997729860117033 ) ) ;
#69521=DIRECTION ( 'NONE',  ( -0.000000000000000000, 0.3420201433256694346, -0.9396926207859080948 ) ) ;
#69522=CARTESIAN_POINT ( 'NONE',  ( -7.173053667125516064, -9.234221910056348293, 34.70572697212741531 ) ) ;
#69523=CARTESIAN_POINT ( 'NONE',  ( -5.076923076923075762, -5.415277668671390821, 36.20867863119892149 ) ) ;
#69524=CARTESIAN_POINT ( 'NONE',  ( -8.769230769230768274, -2.486705287966279876, 31.30864560766543647 ) ) ;
#69527=CARTESIAN_POINT ( 'NONE',  ( -8.769230769230768274, -4.661471528628507777, 34.16647553114623292 ) ) ;
#69528=CARTESIAN_POINT ( 'NONE',  ( -2.241624974342230292, -2.833524468853757750, 32.15551576947925838 ) ) ;
#69529=B_SPLINE_CURVE_WITH_KNOTS ( 'NONE', 3,
 ( #6967, #26357, #6532, #47055, #68666, #76307, #54702, #69113, #47944, #48390 ),
 .UNSPECIFIED., .F., .F.,
 ( 4, 2, 2, 2, 4 ),
 ( 0.000000000000000000, 0.0001954311584214072923, 0.0003908623168428145846, 0.0005862934752642218498, 0.0007817246336856291692 ),
 .UNSPECIFIED. ) ;
#69531=DIRECTION ( 'NONE',  ( 0.000000000000000000, 0.000000000000000000, -1.000000000000000000 ) ) ;
#69532=CARTESIAN_POINT ( 'NONE',  ( -1.634615384615383027, -2.499999999999998668, 29.75000000000000355 ) ) ;
#69533=VECTOR ( 'NONE', #16787, 999.9999999999998863 ) ;
#69534=EDGE_CURVE ( 'NONE', #53330, #67070, #32427, .T. ) ;
#69535=AXIS2_PLACEMENT_3D ( 'NONE', #61358, #33467, #39350 ) ;
#69536=VERTEX_POINT ( 'NONE', #40508 ) ;
#69537=VERTEX_POINT ( 'NONE', #35059 ) ;
#69538=CARTESIAN_POINT ( 'NONE',  ( 3.100621261037532772, -11.04286588640298561, 33.62463336215343901 ) ) ;
#69540=CARTESIAN_POINT ( 'NONE',  ( -11.78846153846153832, -7.500000000000001776, 34.75000000000000000 ) ) ;
#69543=CARTESIAN_POINT ( 'NONE',  ( -18.00000000000000000, -6.436573248120765811, 35.78099280442780383 ) ) ;
#69544=CARTESIAN_POINT ( 'NONE',  ( -2.437840277424001112, -8.630895178749536711, 34.87696386517710323 ) ) ;
#69545=EDGE_CURVE ( 'NONE', #17317, #22911, #79638, .T. ) ;
#69547=CARTESIAN_POINT ( 'NONE',  ( 18.06525513951284267, -3.643525952247864019, 33.31231777344670064 ) ) ;
#69548=EDGE_CURVE ( 'NONE', #32348, #23528, #42277, .T. ) ;
#69549=VERTEX_POINT ( 'NONE', #26984 ) ;
#69550=CARTESIAN_POINT ( 'NONE',  ( 10.61538461538449596, -8.613356846316285953, 34.62446782046622218 ) ) ;
#69553=CARTESIAN_POINT ( 'NONE',  ( -1.634592128663975297, -9.234221910056348293, 34.70572697212741531 ) ) ;
#69554=EDGE_CURVE ( 'NONE', #1510, #87031, #28758, .T. ) ;
#69555=CARTESIAN_POINT ( 'NONE',  ( 3.930361229281821966, -6.716662450894490100, 34.94144148231605840 ) ) ;
#69556=CARTESIAN_POINT ( 'NONE',  ( -2.980769230769293454, -7.565270000091922853, 34.99999999999999289 ) ) ;
#69557=ORIENTED_EDGE ( 'NONE', *, *, #83227, .F. ) ;
#69558=VECTOR ( 'NONE', #83209, 1000.000000000000000 ) ;
#69559=ORIENTED_EDGE ( 'NONE', *, *, #27337, .T. ) ;
#69560=ORIENTED_EDGE ( 'NONE', *, *, #17231, .F. ) ;
#69561=ORIENTED_EDGE ( 'NONE', *, *, #42720, .T. ) ;
#69562=LINE ( 'NONE', #661, #41523 ) ;
#69563=CARTESIAN_POINT ( 'NONE',  ( -2.530619266599156258, -10.01117774369187252, 34.36070679894347535 ) ) ;
#69564=DIRECTION ( 'NONE',  ( 0.000000000000000000, 0.7660444431189822323, -0.6427876096865344779 ) ) ;
#69566=CARTESIAN_POINT ( 'NONE',  ( 4.153846153846032507, -6.879047030192662504, 34.71129190930017927 ) ) ;
#69567=CARTESIAN_POINT ( 'NONE',  ( 14.30769230769218758, -10.21337939537710326, 33.94971097300076224 ) ) ;
#69569=ORIENTED_EDGE ( 'NONE', *, *, #33136, .F. ) ;
#69570=ORIENTED_EDGE ( 'NONE', *, *, #17135, .F. ) ;
#69571=DIRECTION ( 'NONE',  ( 0.000000000000000000, 0.6427876096865368094, 0.7660444431189802339 ) ) ;
#69572=ORIENTED_EDGE ( 'NONE', *, *, #9194, .T. ) ;
#69574=CARTESIAN_POINT ( 'NONE',  ( -5.143005456283213483, -12.62096338111211580, 30.90682066428152197 ) ) ;
#69575=DIRECTION ( 'NONE',  ( 0.000000000000000000, 0.000000000000000000, 1.000000000000000000 ) ) ;
#69579=EDGE_CURVE ( 'NONE', #80708, #39037, #68955, .T. ) ;
#69580=ORIENTED_EDGE ( 'NONE', *, *, #63073, .F. ) ;
#69581=CARTESIAN_POINT ( 'NONE',  ( -18.00000000000012079, -3.083524468854528244, 32.58852847137268327 ) ) ;
#69583=EDGE_LOOP ( 'NONE', ( #13445, #11163 ) ) ;
#69584=FACE_BOUND ( 'NONE', #73175, .T. ) ;
#69585=CARTESIAN_POINT ( 'NONE',  ( 5.076923076923075762, -4.661471528628507777, 34.16647553114623292 ) ) ;
#69587=VECTOR ( 'NONE', #63917, 1000.000000000000000 ) ;
#69589=ORIENTED_EDGE ( 'NONE', *, *, #583, .T. ) ;
#69590=CARTESIAN_POINT ( 'NONE',  ( -4.376711576049792995, -2.501496062324911840, 29.88072118266895671 ) ) ;
#69591=CARTESIAN_POINT ( 'NONE',  ( 8.769230769230645706, -12.16647553114689728, 32.15551576947799362 ) ) ;
#69592=CARTESIAN_POINT ( 'NONE',  ( -1.384615384615383471, -10.67929555188718282, 33.92786785259544047 ) ) ;
#69593=CARTESIAN_POINT ( 'NONE',  ( 4.023698944407935407, -11.47017969459903952, 32.78971311882034456 ) ) ;
#69594=CARTESIAN_POINT ( 'NONE',  ( 8.769230769230768274, -1.422936976036506707, 30.56769352161908415 ) ) ;
#69595=VERTEX_POINT ( 'NONE', #57099 ) ;
#69596=ADVANCED_FACE ( 'NONE', ( #43151 ), #84156, .F. ) ;
#69597=CARTESIAN_POINT ( 'NONE',  ( 6.000000000000001776, -8.120952969808772792, 34.71129190930000163 ) ) ;
#69598=DIRECTION ( 'NONE',  ( 0.000000000000000000, -6.938893903907222067E-15, 1.000000000000000000 ) ) ;
#69599=DIRECTION ( 'NONE',  ( 0.000000000000000000, 0.6427876096865368094, 0.7660444431189802339 ) ) ;
#69600=CARTESIAN_POINT ( 'NONE',  ( 15.90386940979756503, -10.82459398097509862, 33.81372124010183455 ) ) ;
#69601=CYLINDRICAL_SURFACE ( 'NONE', #27141, 0.2500000000000012212 ) ;
#69602=FACE_BOUND ( 'NONE', #43679, .T. ) ;
#69603=CARTESIAN_POINT ( 'NONE',  ( 17.29970261819148902, -3.755027918224367767, 33.06320215134714857 ) ) ;
#69604=DIRECTION ( 'NONE',  ( 0.000000000000000000, 0.8660254037844377084, -0.5000000000000015543 ) ) ;
#69605=CARTESIAN_POINT ( 'NONE',  ( -14.30769230769230660, -3.322132147404559976, 32.92929555188717927 ) ) ;
#69606=CARTESIAN_POINT ( 'NONE',  ( -11.40793583669797506, -11.46989282347013095, 32.79007818306219946 ) ) ;
#69607=CARTESIAN_POINT ( 'NONE',  ( 5.776515056276054771, -10.81261337010820256, 33.49550067578627477 ) ) ;
#69608=DIRECTION ( 'NONE',  ( -0.000000000000000000, -0.5000000000000009992, -0.8660254037844380415 ) ) ;
#69610=ORIENTED_EDGE ( 'NONE', *, *, #45739, .T. ) ;
#69611=CARTESIAN_POINT ( 'NONE',  ( -8.519230769229334754, -7.500000000000155431, 34.75000000000007105 ) ) ;
#69612=ORIENTED_EDGE ( 'NONE', *, *, #81758, .F. ) ;
#69613=CARTESIAN_POINT ( 'NONE',  ( -11.53846153846153655, -5.471508081941601098, 34.59228464037088457 ) ) ;
#69614=ORIENTED_EDGE ( 'NONE', *, *, #238, .T. ) ;
#69615=CARTESIAN_POINT ( 'NONE',  ( -3.903791842207838592, -12.17597550085003633, 31.52189283813461884 ) ) ;
#69616=CARTESIAN_POINT ( 'NONE',  ( 14.24160992833217065, -3.937682226553330445, 33.60647404775217240 ) ) ;
#69620=EDGE_CURVE ( 'NONE', #48440, #74923, #44455, .T. ) ;
#69621=CARTESIAN_POINT ( 'NONE',  ( -10.36543920600657209, -12.68172785388650681, 30.59649109432439218 ) ) ;
#69622=FACE_OUTER_BOUND ( 'NONE', #79963, .T. ) ;
#69623=B_SPLINE_CURVE_WITH_KNOTS ( 'NONE', 3,
 ( #44054, #85072, #57585, #36004, #23350, #15727, #69776, #63456, #1757, #22472 ),
 .UNSPECIFIED., .F., .F.,
 ( 4, 2, 2, 2, 4 ),
 ( 0.0007817246336856284103, 0.0009771112958940092897, 0.001172497958102390169, 0.001367884620310771265, 0.001563271282519152145 ),
 .UNSPECIFIED. ) ;
#69625=FACE_OUTER_BOUND ( 'NONE', #54502, .T. ) ;
#69626=LINE ( 'NONE', #70961, #80427 ) ;
#69627=CARTESIAN_POINT ( 'NONE',  ( 16.15384615384615330, -9.584722331328613620, 36.20867863119891439 ) ) ;
#69628=DIRECTION ( 'NONE',  ( -0.000000000000000000, -0.7660444431189791237, -0.6427876096865379196 ) ) ;
#69630=CARTESIAN_POINT ( 'NONE',  ( 11.28848479441294828, -5.643011162660950042, 34.66104346484419096 ) ) ;
#69631=CARTESIAN_POINT ( 'NONE',  ( 17.99999999999987566, -4.481592998941358097, 33.73612834414048933 ) ) ;
#69634=CARTESIAN_POINT ( 'NONE',  ( -10.36543920600657209, -5.766571408460171355, 34.70601412856602508 ) ) ;
#69635=CARTESIAN_POINT ( 'NONE',  ( 1.384615384615386802, -1.951392089020283160, 34.73218667398347748 ) ) ;
#69636=ORIENTED_EDGE ( 'NONE', *, *, #53224, .F. ) ;
#69637=CARTESIAN_POINT ( 'NONE',  ( -17.77698864838714243, -2.758310577978209110, 31.33698337089303010 ) ) ;
#69638=FACE_OUTER_BOUND ( 'NONE', #33998, .T. ) ;
#69639=DIRECTION ( 'NONE',  ( -0.000000000000000000, 0.000000000000000000, 1.000000000000000000 ) ) ;
#69640=ORIENTED_EDGE ( 'NONE', *, *, #74511, .T. ) ;
#69641=CARTESIAN_POINT ( 'NONE',  ( -14.43838377435986686, -11.71456829005830080, 32.44064028649416542 ) ) ;
#69643=DIRECTION ( 'NONE',  ( 0.000000000000000000, -6.938893903907222067E-15, 1.000000000000000000 ) ) ;
#69644=LINE ( 'NONE', #7953, #56261 ) ;
#69645=CARTESIAN_POINT ( 'NONE',  ( 10.36540787133602670, -12.65889640711025521, 30.72598325615533454 ) ) ;
#69648=EDGE_CURVE ( 'NONE', #7735, #62030, #51689, .T. ) ;
#69649=ORIENTED_EDGE ( 'NONE', *, *, #52110, .F. ) ;
#69650=CARTESIAN_POINT ( 'NONE',  ( -0.2387589202700516056, -10.81320215134717344, 33.49497208177562868 ) ) ;
#69651=ORIENTED_EDGE ( 'NONE', *, *, #32681, .T. ) ;
#69652=EDGE_CURVE ( 'NONE', #63192, #10084, #15192, .T. ) ;
#69653=VERTEX_POINT ( 'NONE', #30516 ) ;
#69654=CIRCLE ( 'NONE', #23677, 0.2500000000000002220 ) ;
#69655=CARTESIAN_POINT ( 'NONE',  ( -13.60810032833933469, -3.754499324213721234, 33.06261337010820256 ) ) ;
#69656=CARTESIAN_POINT ( 'NONE',  ( -3.931066612577741370, -3.236590943229499029, 32.36255958852953540 ) ) ;
#69657=EDGE_CURVE ( 'NONE', #38188, #68176, #30187, .T. ) ;
#69658=CARTESIAN_POINT ( 'NONE',  ( 9.942253210655836781, -5.057305518903948638, 34.11320923018887896 ) ) ;
#69659=CARTESIAN_POINT ( 'NONE',  ( 13.38461538461538680, -8.164416787775445883, 34.95778746994557906 ) ) ;
#69660=ORIENTED_EDGE ( 'NONE', *, *, #15104, .F. ) ;
#69661=CARTESIAN_POINT ( 'NONE',  ( 17.29993592101647693, -11.43677907613345113, 33.22367315496201456 ) ) ;
#69663=VERTEX_POINT ( 'NONE', #57985 ) ;
#69664=VERTEX_POINT ( 'NONE', #85465 ) ;
#69666=ORIENTED_EDGE ( 'NONE', *, *, #83336, .T. ) ;
#69667=CARTESIAN_POINT ( 'NONE',  ( -6.923076923076922462, -2.292212530054420494, 30.41441678777542634 ) ) ;
#69668=EDGE_CURVE ( 'NONE', #14315, #75360, #17003, .T. ) ;
#69669=CARTESIAN_POINT ( 'NONE',  ( 6.223012844093396723, -2.523321265292115090, 31.42251411153756280 ) ) ;
#69671=CARTESIAN_POINT ( 'NONE',  ( -3.164700879766792152, -4.098570777380720287, 33.41473453929635440 ) ) ;
#69673=ORIENTED_EDGE ( 'NONE', *, *, #19172, .F. ) ;
#69674=ORIENTED_EDGE ( 'NONE', *, *, #88254, .T. ) ;
#69675=CIRCLE ( 'NONE', #84048, 2.000000000000001776 ) ;
#69677=CARTESIAN_POINT ( 'NONE',  ( -9.626239341305252495, -5.557115091759786019, 34.35708131394839882 ) ) ;
#69678=CARTESIAN_POINT ( 'NONE',  ( -2.557715544985270650, -2.823816976329320827, 31.52131813110797154 ) ) ;
#69679=VERTEX_POINT ( 'NONE', #24196 ) ;
#69680=CARTESIAN_POINT ( 'NONE',  ( -7.146003140593069958, -12.39988816332205701, 30.74660775122750778 ) ) ;
#69681=CARTESIAN_POINT ( 'NONE',  ( 6.792929713638703682, -6.852621066184267029, 34.70813303252209181 ) ) ;
#69682=EDGE_CURVE ( 'NONE', #50475, #26485, #60336, .T. ) ;
#69683=CARTESIAN_POINT ( 'NONE',  ( -14.53117725141625094, -2.599994579823203367, 30.74605699353653776 ) ) ;
#69684=VERTEX_POINT ( 'NONE', #4379 ) ;
#69685=CARTESIAN_POINT ( 'NONE',  ( -14.30769230769230660, -8.318370150425687726, 35.83090037661290239 ) ) ;
#69687=EDGE_LOOP ( 'NONE', ( #26528, #28917, #66942, #13506, #52076, #12501 ) ) ;
#69688=FACE_BOUND ( 'NONE', #43068, .T. ) ;
#69689=B_SPLINE_CURVE_WITH_KNOTS ( 'NONE', 3,
 ( #70969, #86279, #71847, #23218, #37172, #50678, #84493, #79052, #50230, #9703 ),
 .UNSPECIFIED., .F., .F.,
 ( 4, 2, 2, 2, 4 ),
 ( 0.000000000000000000, 0.0001954311564186862510, 0.0003908623128373725020, 0.0005862934692560588072, 0.0007817246256747450040 ),
 .UNSPECIFIED. ) ;
#69690=EDGE_CURVE ( 'NONE', #3690, #89174, #59767, .T. ) ;
#69691=CARTESIAN_POINT ( 'NONE',  ( -10.68146699474474914, -4.661471528628507777, 34.16647553114621871 ) ) ;
#69692=CARTESIAN_POINT ( 'NONE',  ( 13.44987052412822059, -6.835583212224610072, 34.95778746994559327 ) ) ;
#69693=LINE ( 'NONE', #6662, #10633 ) ;
#69694=CARTESIAN_POINT ( 'NONE',  ( -13.38461538461538325, -2.249999999999998668, 29.50000000000001421 ) ) ;
#69696=CARTESIAN_POINT ( 'NONE',  ( 14.30769230769231015, -12.34228464037088635, 31.77849191805839268 ) ) ;
#69697=CARTESIAN_POINT ( 'NONE',  ( -2.373775718648187816, -3.513871655860377086, 32.76840700105978499 ) ) ;
#69699=DIRECTION ( 'NONE',  ( 0.000000000000000000, 0.7660444431189807890, 0.6427876096865361433 ) ) ;
#69700=CARTESIAN_POINT ( 'NONE',  ( 2.307692307692309264, -13.53365097954675988, 30.81389545987213552 ) ) ;
#69701=B_SPLINE_CURVE_WITH_KNOTS ( 'NONE', 3,
 ( #35615, #83813, #63951, #49566, #9462, #63064, #49999, #29743, #23408, #58083 ),
 .UNSPECIFIED., .F., .F.,
 ( 4, 2, 2, 2, 4 ),
 ( 0.0007817246256747472808, 0.0009771112852218907189, 0.001172497944769034265, 0.001367884604316177595, 0.001563271263863321141 ),
 .UNSPECIFIED. ) ;
#69702=ORIENTED_EDGE ( 'NONE', *, *, #67038, .T. ) ;
#69703=EDGE_CURVE ( 'NONE', #77971, #84339, #9752, .T. ) ;
#69704=FACE_OUTER_BOUND ( 'NONE', #79455, .T. ) ;
#69705=CARTESIAN_POINT ( 'NONE',  ( -4.377331078410482412, -3.562934362175799841, 33.22335522853832401 ) ) ;
#69706=ORIENTED_EDGE ( 'NONE', *, *, #67420, .T. ) ;
#69707=CARTESIAN_POINT ( 'NONE',  ( 8.096208266067295156, -6.523592122091591783, 34.90882529074906415 ) ) ;
#69708=CARTESIAN_POINT ( 'NONE',  ( -4.284536756956461190, -2.295517848115769421, 30.44137282052136939 ) ) ;
#69710=FACE_BOUND ( 'NONE', #70457, .T. ) ;
#69711=EDGE_CURVE ( 'NONE', #2618, #71762, #4832, .T. ) ;
#69712=CARTESIAN_POINT ( 'NONE',  ( -1.515305987725691139, -6.369640206132550553, 34.87707690430378449 ) ) ;
#69713=DIRECTION ( 'NONE',  ( -0.000000000000000000, -0.9396926207859092051, -0.3420201433256662704 ) ) ;
#69714=CARTESIAN_POINT ( 'NONE',  ( -6.857008572074484221, -8.973038597847269315, 34.52809138561122637 ) ) ;
#69715=CARTESIAN_POINT ( 'NONE',  ( -16.02332045208259004, -2.619367082507847222, 30.83698974864643461 ) ) ;
#69716=CARTESIAN_POINT ( 'NONE',  ( -5.076923076923075762, -9.905515769479276145, 34.41647553114623292 ) ) ;
#69717=CARTESIAN_POINT ( 'NONE',  ( -12.52680890749923570, -4.481592998940162609, 33.73612834413957984 ) ) ;
#69718=CARTESIAN_POINT ( 'NONE',  ( -14.24162497434223340, -5.471508081941601098, 34.59228464037088457 ) ) ;
#69720=ORIENTED_EDGE ( 'NONE', *, *, #82345, .T. ) ;
#69721=VECTOR ( 'NONE', #51238, 1000.000000000000000 ) ;
#69722=ORIENTED_EDGE ( 'NONE', *, *, #82454, .F. ) ;
#69723=CARTESIAN_POINT ( 'NONE',  ( 16.08776377448601735, -9.058645607665454236, 34.76329471203372634 ) ) ;
#69724=CARTESIAN_POINT ( 'NONE',  ( -12.46153846153858424, -6.835583212225970762, 34.95778746994575670 ) ) ;
#69725=CARTESIAN_POINT ( 'NONE',  ( -7.846153846153844924, -13.37000171582298513, 34.34916445242398453 ) ) ;
#69726=CARTESIAN_POINT ( 'NONE',  ( -0.5268084620947811603, -3.083524468853724443, 32.58852847137143272 ) ) ;
#69727=CARTESIAN_POINT ( 'NONE',  ( -1.134615384615383915, -7.500000000000001776, 35.04278698407183867 ) ) ;
#69729=EDGE_CURVE ( 'NONE', #64747, #53433, #25093, .T. ) ;
#69731=CARTESIAN_POINT ( 'NONE',  ( 4.153846153846154188, -11.91647553114624181, 32.58852847137148245 ) ) ;
#69732=EDGE_CURVE ( 'NONE', #42058, #75680, #43099, .T. ) ;
#69733=CARTESIAN_POINT ( 'NONE',  ( 9.442284468086237226, -10.92453946501458795, 33.72985991061850086 ) ) ;
#69734=DIRECTION ( 'NONE',  ( 0.000000000000000000, -6.938893903907222067E-15, 1.000000000000000000 ) ) ;
#69735=LINE ( 'NONE', #41830, #84177 ) ;
#69737=CARTESIAN_POINT ( 'NONE',  ( -6.000000000000121680, -12.51329471203414379, 31.30864560766407578 ) ) ;
#69738=CARTESIAN_POINT ( 'NONE',  ( 10.36538461538461675, -7.500000000000001776, 35.00000000000000000 ) ) ;
#69739=DIRECTION ( 'NONE',  ( 0.000000000000000000, 0.3420201433256610524, 0.9396926207859113145 ) ) ;
#69740=ORIENTED_EDGE ( 'NONE', *, *, #13780, .F. ) ;
#69741=CARTESIAN_POINT ( 'NONE',  ( 12.46153846153846168, -3.937682226553329556, 33.60647404775216529 ) ) ;
#69742=CARTESIAN_POINT ( 'NONE',  ( -12.21153846153702638, -7.500000000000155431, 34.75000000000007105 ) ) ;
#69744=CARTESIAN_POINT ( 'NONE',  ( 3.903869409797562806, -4.818429247618089661, 34.26397095200675125 ) ) ;
#69745=FACE_OUTER_BOUND ( 'NONE', #76217, .T. ) ;
#69746=ORIENTED_EDGE ( 'NONE', *, *, #6984, .F. ) ;
#69747=CARTESIAN_POINT ( 'NONE',  ( -6.923076923076922462, -10.89733346790207413, 36.13435417666054406 ) ) ;
#69748=CARTESIAN_POINT ( 'NONE',  ( -9.469296340694841163, -4.887748414852792322, 34.01359900205216746 ) ) ;
#69750=DIRECTION ( 'NONE',  ( -0.000000000000000000, 0.6427876096865404731, -0.7660444431189771253 ) ) ;
#69751=CARTESIAN_POINT ( 'NONE',  ( -9.442253272394237840, -5.642605341092957971, 34.66089969410670335 ) ) ;
#69753=DIRECTION ( 'NONE',  ( -0.000000000000000000, -0.000000000000000000, -1.000000000000000000 ) ) ;
#69757=CARTESIAN_POINT ( 'NONE',  ( -15.23076923076922995, -4.661471528628507777, 34.16647553114623292 ) ) ;
#69758=CARTESIAN_POINT ( 'NONE',  ( -11.78848476268299450, -12.45566812827425451, 31.48439005359158926 ) ) ;
#69759=DIRECTION ( 'NONE',  ( 0.000000000000000000, 0.000000000000000000, 1.000000000000000000 ) ) ;
#69760=ORIENTED_EDGE ( 'NONE', *, *, #59340, .F. ) ;
#69761=ORIENTED_EDGE ( 'NONE', *, *, #30612, .T. ) ;
#69762=CARTESIAN_POINT ( 'NONE',  ( 6.223011351612852238, -6.503523203565942268, 34.64991518177335195 ) ) ;
#69763=EDGE_CURVE ( 'NONE', #86735, #60344, #22685, .T. ) ;
#69764=VERTEX_POINT ( 'NONE', #38161 ) ;
#69765=CARTESIAN_POINT ( 'NONE',  ( 7.846153846153846700, -2.833524468853757305, 32.15551576947925838 ) ) ;
#69766=CARTESIAN_POINT ( 'NONE',  ( -7.146003881983771677, -2.308479472611653094, 30.53278059502174457 ) ) ;
#69768=EDGE_CURVE ( 'NONE', #13588, #363, #38800, .T. ) ;
#69769=CYLINDRICAL_SURFACE ( 'NONE', #56489, 0.2500000000000004996 ) ;
#69770=CARTESIAN_POINT ( 'NONE',  ( 17.07692307692307665, -1.044019251281081972, 31.83374038241031911 ) ) ;
#69771=ADVANCED_FACE ( 'NONE', ( #83151 ), #68299, .F. ) ;
#69772=CARTESIAN_POINT ( 'NONE',  ( 13.38461538461538680, -12.78798330534103123, 29.99999999999997868 ) ) ;
#69773=B_SPLINE_CURVE_WITH_KNOTS ( 'NONE', 3,
 ( #78337, #57630, #36045, #64372, #63499, #63046, #50417, #29728, #28846, #56307 ),
 .UNSPECIFIED., .F., .F.,
 ( 4, 2, 2, 2, 4 ),
 ( 0.000000000000000000, 0.0001954311564186865763, 0.0003908623128373731525, 0.0005862934692560596746, 0.0007817246256747463051 ),
 .UNSPECIFIED. ) ;
#69774=ORIENTED_EDGE ( 'NONE', *, *, #58099, .F. ) ;
#69775=ORIENTED_EDGE ( 'NONE', *, *, #79918, .T. ) ;
#69776=CARTESIAN_POINT ( 'NONE',  ( -2.438167492768025024, -7.276987145209184327, 34.99546412871779211 ) ) ;
#69778=EDGE_CURVE ( 'NONE', #4584, #58033, #82714, .T. ) ;
#69779=CARTESIAN_POINT ( 'NONE',  ( 7.596130621932386973, -2.588893531581426988, 31.60682220781847818 ) ) ;
#69780=ORIENTED_EDGE ( 'NONE', *, *, #17439, .F. ) ;
#69781=EDGE_CURVE ( 'NONE', #45658, #54250, #38181, .T. ) ;
#69782=FACE_OUTER_BOUND ( 'NONE', #7571, .T. ) ;
#69783=CARTESIAN_POINT ( 'NONE',  ( 8.068933387422255521, -5.114059244376869984, 34.14424750095245287 ) ) ;
#69785=ORIENTED_EDGE ( 'NONE', *, *, #38663, .T. ) ;
#69787=ADVANCED_FACE ( 'NONE', ( #6603 ), #33185, .F. ) ;
#69788=VERTEX_POINT ( 'NONE', #12472 ) ;
#69790=ORIENTED_EDGE ( 'NONE', *, *, #33358, .T. ) ;
#69791=CARTESIAN_POINT ( 'NONE',  ( -14.30769230769242917, -12.16647553114689728, 32.15551576947799362 ) ) ;
#69793=CARTESIAN_POINT ( 'NONE',  ( 17.86985279056177944, -10.88202310037936194, 33.43294751532457099 ) ) ;
#69794=CARTESIAN_POINT ( 'NONE',  ( 17.75002325595141173, -12.41104346484419452, 31.60698883733904196 ) ) ;
#69795=FACE_BOUND ( 'NONE', #10555, .T. ) ;
#69796=EDGE_CURVE ( 'NONE', #85539, #33270, #83787, .T. ) ;
#69797=CARTESIAN_POINT ( 'NONE',  ( -11.60454494941742176, -2.538708090699994813, 30.37095296980875148 ) ) ;
#69798=CARTESIAN_POINT ( 'NONE',  ( -18.00000000000000000, -3.895656007487076078, 35.99290692298802696 ) ) ;
#69799=CARTESIAN_POINT ( 'NONE',  ( -16.08859101433330707, -5.094484230520771817, 34.41647553114626845 ) ) ;
#69800=CARTESIAN_POINT ( 'NONE',  ( 12.21156171748986985, -3.436278759898153901, 33.07459398097509506 ) ) ;
#69801=CARTESIAN_POINT ( 'NONE',  ( 5.142991427925513115, -10.51840700105979565, 33.73612834413962247 ) ) ;
#69802=CARTESIAN_POINT ( 'NONE',  ( -39.05038313613820122, -2.499999999999999556, 29.75000000000000355 ) ) ;
#69804=EDGE_CURVE ( 'NONE', #55112, #74382, #10718, .T. ) ;
#69805=CARTESIAN_POINT ( 'NONE',  ( 10.36540788444226102, -9.943427161483782584, 34.11278801902876978 ) ) ;
#69806=EDGE_LOOP ( 'NONE', ( #14081, #58132, #55529, #74327 ) ) ;
#69807=ORIENTED_EDGE ( 'NONE', *, *, #63194, .T. ) ;
#69808=AXIS2_PLACEMENT_3D ( 'NONE', #37475, #57757, #3689 ) ;
#69809=CARTESIAN_POINT ( 'NONE',  ( 7.622668902429897919, -6.760086850603068243, 34.69517049084099369 ) ) ;
#69810=DIRECTION ( 'NONE',  ( -0.000000000000000000, 0.9396926207859093161, -0.3420201433256663259 ) ) ;
#69811=DIRECTION ( 'NONE',  ( 0.000000000000000000, 0.4999999999999960032, -0.8660254037844410391 ) ) ;
#69813=CARTESIAN_POINT ( 'NONE',  ( -10.36543920600657209, -12.45601412856602686, 31.48342859153981621 ) ) ;
#69814=CARTESIAN_POINT ( 'NONE',  ( -12.33101302330481808, -5.070358843744210198, 34.40418822224088302 ) ) ;
#69815=ORIENTED_EDGE ( 'NONE', *, *, #72413, .F. ) ;
#69816=CARTESIAN_POINT ( 'NONE',  ( 11.47319153790521717, -3.643525952247789412, 33.31231777344662959 ) ) ;
#69817=EDGE_CURVE ( 'NONE', #71873, #16707, #11848, .T. ) ;
#69818=EDGE_CURVE ( 'NONE', #1987, #59805, #64450, .T. ) ;
#69819=CARTESIAN_POINT ( 'NONE',  ( -6.130691466667556710, -6.413092428213692742, 34.63065189839063152 ) ) ;
#69820=CARTESIAN_POINT ( 'NONE',  ( -10.48459280755982803, -9.804649428959608670, 34.18742332936588468 ) ) ;
#69821=CARTESIAN_POINT ( 'NONE',  ( -12.46153846153858424, -9.528491918059723176, 34.59228464037033035 ) ) ;
#69824=FACE_OUTER_BOUND ( 'NONE', #1115, .T. ) ;
#69825=ORIENTED_EDGE ( 'NONE', *, *, #80127, .T. ) ;
#69826=B_SPLINE_CURVE_WITH_KNOTS ( 'NONE', 3,
 ( #17826, #79965, #59691, #78623, #24567, #44376, #65548, #4758, #25463, #38540 ),
 .UNSPECIFIED., .F., .F.,
 ( 4, 2, 2, 2, 4 ),
 ( 0.000000000000000000, 0.0001954311564186863323, 0.0003908623128373726646, 0.0005862934692560590241, 0.0007817246256747453293 ),
 .UNSPECIFIED. ) ;
#69827=VERTEX_POINT ( 'NONE', #41721 ) ;
#69828=B_SPLINE_CURVE_WITH_KNOTS ( 'NONE', 3,
 ( #77492, #55889, #15804, #28883, #68962, #83376, #21664, #49134, #8602, #36077 ),
 .UNSPECIFIED., .F., .F.,
 ( 4, 2, 2, 2, 4 ),
 ( 0.000000000000000000, 0.0001954311564186868744, 0.0003908623128373737488, 0.0005862934692560606504, 0.0007817246256747474977 ),
 .UNSPECIFIED. ) ;
#69829=CARTESIAN_POINT ( 'NONE',  ( -6.130147969731695845, -4.299443229763728169, 33.91186481527756058 ) ) ;
#69830=ORIENTED_EDGE ( 'NONE', *, *, #55992, .F. ) ;
#69831=CARTESIAN_POINT ( 'NONE',  ( -1.253823576790597638, -8.147973898785416225, 34.70805048591653730 ) ) ;
#69832=FACE_OUTER_BOUND ( 'NONE', #87132, .T. ) ;
#69833=CARTESIAN_POINT ( 'NONE',  ( 6.000000000000001776, -1.044019251281081972, 31.83374038241031911 ) ) ;
#69834=CARTESIAN_POINT ( 'NONE',  ( 3.230769230769110045, -10.90142922262034020, 33.41473453929536674 ) ) ;
#69835=CARTESIAN_POINT ( 'NONE',  ( 5.076923076923075762, -12.78798330534102945, 29.74999999999997868 ) ) ;
#69836=ADVANCED_FACE ( 'NONE', ( #62412 ), #6159, .F. ) ;
#69837=CARTESIAN_POINT ( 'NONE',  ( -16.82692307692307665, -2.249999999999998668, 29.75000000000000355 ) ) ;
#69838=ORIENTED_EDGE ( 'NONE', *, *, #22314, .F. ) ;
#69839=DIRECTION ( 'NONE',  ( 0.000000000000000000, 0.6427876096865373645, -0.7660444431189797898 ) ) ;
#69840=CARTESIAN_POINT ( 'NONE',  ( -13.31935981333935537, -4.481592998940250538, 33.73612834413965089 ) ) ;
#69841=ORIENTED_EDGE ( 'NONE', *, *, #83520, .T. ) ;
#69843=CARTESIAN_POINT ( 'NONE',  ( -10.39237326377176451, -3.587049720035815348, 32.86302985866382897 ) ) ;
#69844=CYLINDRICAL_SURFACE ( 'NONE', #87567, 0.2500000000000002220 ) ;
#69846=EDGE_CURVE ( 'NONE', #58822, #73958, #43047, .T. ) ;
#69847=CARTESIAN_POINT ( 'NONE',  ( -2.307692307692428724, -12.70778746994576025, 30.41441678777401236 ) ) ;
#69848=CARTESIAN_POINT ( 'NONE',  ( -12.59222992820601661, -2.729777683071817229, 31.24903638046269450 ) ) ;
#69849=AXIS2_PLACEMENT_3D ( 'NONE', #3013, #45334, #30495 ) ;
#69851=CARTESIAN_POINT ( 'NONE',  ( -5.999999999999998224, -13.20930481340135110, 34.54067556320372745 ) ) ;
#69853=ORIENTED_EDGE ( 'NONE', *, *, #35497, .T. ) ;
#69854=EDGE_CURVE ( 'NONE', #29911, #54514, #15036, .T. ) ;
#69855=CARTESIAN_POINT ( 'NONE',  ( -1.254089682851821985, -11.46989282347013095, 32.79007818306219946 ) ) ;
#69856=CARTESIAN_POINT ( 'NONE',  ( 15.23076923076910916, -3.643525952248795718, 33.31231777344771672 ) ) ;
#69857=CARTESIAN_POINT ( 'NONE',  ( 7.976679547917409963, -2.619367082507848998, 30.83698974864644171 ) ) ;
#69858=CARTESIAN_POINT ( 'NONE',  ( -7.780086512803769061, -2.833524468853757750, 32.15551576947925838 ) ) ;
#69859=VERTEX_POINT ( 'NONE', #70962 ) ;
#69861=LINE ( 'NONE', #1843, #953 ) ;
#69862=AXIS2_PLACEMENT_3D ( 'NONE', #84763, #29373, #78421 ) ;
#69863=CARTESIAN_POINT ( 'NONE',  ( -0.5276208408985972875, -12.62096338111211580, 30.90682066428152197 ) ) ;
#69864=CARTESIAN_POINT ( 'NONE',  ( -4.376772371362299019, -10.61292498521070549, 33.66303323003028680 ) ) ;
#69865=ORIENTED_EDGE ( 'NONE', *, *, #57702, .T. ) ;
#69866=CARTESIAN_POINT ( 'NONE',  ( -12.23875892027004753, -9.332535724633409302, 34.40230450496446934 ) ) ;
#69867=CARTESIAN_POINT ( 'NONE',  ( 8.096099364501986528, -5.852078868378312038, 34.47109172314383585 ) ) ;
#69868=CARTESIAN_POINT ( 'NONE',  ( 14.30769230769231015, -12.29105614889573062, 35.45975837776705220 ) ) ;
#69869=ORIENTED_EDGE ( 'NONE', *, *, #42997, .F. ) ;
#69870=CARTESIAN_POINT ( 'NONE',  ( -2.557715531913763662, -12.07920672191015221, 32.31858351112116168 ) ) ;
#69871=ORIENTED_EDGE ( 'NONE', *, *, #42215, .F. ) ;
#69872=CARTESIAN_POINT ( 'NONE',  ( -16.15384615384615330, -5.557115091759785130, 34.35708131394839171 ) ) ;
#69873=DIRECTION ( 'NONE',  ( -0.000000000000000000, 0.8660254037844397068, -0.4999999999999978906 ) ) ;
#69875=ORIENTED_EDGE ( 'NONE', *, *, #53472, .T. ) ;
#69876=CARTESIAN_POINT ( 'NONE',  ( 10.83839745947801170, -11.43677907613344757, 33.22367315496202167 ) ) ;
#69877=CARTESIAN_POINT ( 'NONE',  ( -9.019254006523732770, -2.587272538249755893, 30.68239716806877837 ) ) ;
#69878=CARTESIAN_POINT ( 'NONE',  ( -6.700297254098854793, -12.47679350104403007, 31.42216943046555855 ) ) ;
#69880=CARTESIAN_POINT ( 'NONE',  ( -11.53846153846153655, -5.471508081941601098, 34.59228464037088457 ) ) ;
#69881=CARTESIAN_POINT ( 'NONE',  ( -18.06527044596078113, -4.481592998940164385, 33.73612834413957984 ) ) ;
#69882=ORIENTED_EDGE ( 'NONE', *, *, #30600, .F. ) ;
#69883=ORIENTED_EDGE ( 'NONE', *, *, #27426, .F. ) ;
#69884=FACE_BOUND ( 'NONE', #50178, .T. ) ;
#69885=VERTEX_POINT ( 'NONE', #57884 ) ;
#69886=CARTESIAN_POINT ( 'NONE',  ( -8.546219417617917813, -4.187068189119699468, 33.49521262558774026 ) ) ;
#69887=LINE ( 'NONE', #29799, #5636 ) ;
#69888=CARTESIAN_POINT ( 'NONE',  ( 9.627037246346921151, -12.27809138561121394, 31.22303859784730307 ) ) ;
#69889=CARTESIAN_POINT ( 'NONE',  ( -14.24162395668986925, -8.973038597847271092, 34.52809138561121216 ) ) ;
#69890=B_SPLINE_CURVE_WITH_KNOTS ( 'NONE', 3,
 ( #88467, #88033, #81250, #26736, #19973, #47442, #74937, #69494, #22199, #22632 ),
 .UNSPECIFIED., .F., .F.,
 ( 4, 2, 2, 2, 4 ),
 ( 0.0007817246256747517261, 0.0009771112852218957062, 0.001172497944769039686, 0.001367884604316183667, 0.001563271263863327647 ),
 .UNSPECIFIED. ) ;
#69892=EDGE_CURVE ( 'NONE', #32510, #2169, #2056, .T. ) ;
#69893=ORIENTED_EDGE ( 'NONE', *, *, #54732, .T. ) ;
#69894=VERTEX_POINT ( 'NONE', #2932 ) ;
#69895=CARTESIAN_POINT ( 'NONE',  ( -0.2114841499001473557, -3.136992222400443175, 32.19305428654138979 ) ) ;
#69896=VERTEX_POINT ( 'NONE', #15138 ) ;
#69897=VECTOR ( 'NONE', #82236, 1000.000000000000000 ) ;
#69898=CARTESIAN_POINT ( 'NONE',  ( 3.100622021331012501, -2.882441371585227508, 31.66841991370171527 ) ) ;
#69899=CARTESIAN_POINT ( 'NONE',  ( 1.384615384615386802, -3.513871655860378418, 32.76840700105978499 ) ) ;
#69900=CARTESIAN_POINT ( 'NONE',  ( -18.22348494372394967, -11.41268669641500111, 32.86336882939238535 ) ) ;
#69901=ORIENTED_EDGE ( 'NONE', *, *, #66143, .T. ) ;
#69902=FACE_OUTER_BOUND ( 'NONE', #42250, .T. ) ;
#69903=CARTESIAN_POINT ( 'NONE',  ( 6.923076923076924238, -1.242168528481310874, 33.36296068462461051 ) ) ;
#69904=FACE_OUTER_BOUND ( 'NONE', #32014, .T. ) ;
#69905=CARTESIAN_POINT ( 'NONE',  ( -11.78848477575450460, -3.202444869320336451, 32.30641848906366675 ) ) ;
#69906=ORIENTED_EDGE ( 'NONE', *, *, #29526, .T. ) ;
#69907=EDGE_CURVE ( 'NONE', #11752, #1726, #29978, .T. ) ;
#69910=EDGE_LOOP ( 'NONE', ( #81579, #22200, #17372, #8025 ) ) ;
#69911=CARTESIAN_POINT ( 'NONE',  ( 4.153846153846154188, -2.833524468853757305, 32.15551576947925838 ) ) ;
#69914=CARTESIAN_POINT ( 'NONE',  ( 11.53846153846153832, -1.117168528481311540, 33.14645433367849847 ) ) ;
#69915=CARTESIAN_POINT ( 'NONE',  ( 11.28848479441294828, -2.318417181685855422, 30.59732222474233865 ) ) ;
#69916=CARTESIAN_POINT ( 'NONE',  ( -3.480745961711583902, -11.28823185664190376, 33.01397839955799896 ) ) ;
#69917=FACE_BOUND ( 'NONE', #85760, .T. ) ;
#69918=CARTESIAN_POINT ( 'NONE',  ( 8.096099364501990081, -11.37275283266504111, 32.91324779482534524 ) ) ;
#69919=ORIENTED_EDGE ( 'NONE', *, *, #21795, .F. ) ;
#69920=CARTESIAN_POINT ( 'NONE',  ( 17.14217864819909920, -10.90142922261932057, 33.41473453929631887 ) ) ;
#69921=EDGE_CURVE ( 'NONE', #69537, #12402, #62850, .T. ) ;
#69922=CARTESIAN_POINT ( 'NONE',  ( -0.2385271099256112415, -9.086983370893047862, 34.49168942202179267 ) ) ;
#69923=CARTESIAN_POINT ( 'NONE',  ( 4.153846153846032507, -9.442884908241554243, 34.35708131394783038 ) ) ;
#69924=FACE_OUTER_BOUND ( 'NONE', #26100, .T. ) ;
#69925=ORIENTED_EDGE ( 'NONE', *, *, #65838, .F. ) ;
#69926=CARTESIAN_POINT ( 'NONE',  ( 2.307692307692187583, -11.94971097300221174, 32.03036669348237098 ) ) ;
#69927=ORIENTED_EDGE ( 'NONE', *, *, #81121, .F. ) ;
#69928=FACE_BOUND ( 'NONE', #31621, .T. ) ;
#69929=CARTESIAN_POINT ( 'NONE',  ( 16.15384615384603251, -3.643525952248796163, 33.31231777344771672 ) ) ;
#69930=CARTESIAN_POINT ( 'NONE',  ( -6.923076923077045919, -10.33852847137269571, 34.16647553114546554 ) ) ;
#69931=CARTESIAN_POINT ( 'NONE',  ( 5.076923076922953193, -10.33852847137269571, 34.16647553114546554 ) ) ;
#69932=VERTEX_POINT ( 'NONE', #15580 ) ;
#69933=CARTESIAN_POINT ( 'NONE',  ( 0.2115152242454954312, -10.76384336483936011, 33.53834819971076087 ) ) ;
#69934=CARTESIAN_POINT ( 'NONE',  ( 15.23076923076910916, -2.379036618888197729, 30.90682066428292885 ) ) ;
#69935=CARTESIAN_POINT ( 'NONE',  ( 8.519254025182176449, -8.347322224742351082, 34.93158281831414769 ) ) ;
#69936=CARTESIAN_POINT ( 'NONE',  ( -6.923076923076922462, -10.51840700105979565, 33.73612834413961536 ) ) ;
#69937=EDGE_LOOP ( 'NONE', ( #34735, #21045 ) ) ;
#69939=CYLINDRICAL_SURFACE ( 'NONE', #28693, 0.2499999999999979738 ) ;
#69940=ORIENTED_EDGE ( 'NONE', *, *, #45022, .F. ) ;
#69941=CARTESIAN_POINT ( 'NONE',  ( 17.07692307692295586, -12.27809138561165270, 31.22303859784587132 ) ) ;
#69942=VERTEX_POINT ( 'NONE', #84933 ) ;
#69943=CARTESIAN_POINT ( 'NONE',  ( -18.00000000104979492, -12.75000000000000355, 29.50000000010276935 ) ) ;
#69944=CARTESIAN_POINT ( 'NONE',  ( -1.608100309179716803, -12.47654668319379567, 31.42292124445336654 ) ) ;
#69945=CARTESIAN_POINT ( 'NONE',  ( 13.31934493865461278, -9.442884908240170461, 34.35708131394840592 ) ) ;
#69947=ADVANCED_FACE ( 'NONE', ( #78159 ), #70072, .F. ) ;
#69948=CARTESIAN_POINT ( 'NONE',  ( 9.692307692307570832, -5.094484230521993062, 34.41647553114689373 ) ) ;
#69949=CARTESIAN_POINT ( 'NONE',  ( -3.007756386675834559, -4.026326845037965008, 33.68677907613344047 ) ) ;
#69950=CARTESIAN_POINT ( 'NONE',  ( 0.2115384615384615641, -7.500000000000001776, 34.75000000000000000 ) ) ;
#69951=CARTESIAN_POINT ( 'NONE',  ( 14.17700084102474811, -3.530157926970578952, 32.79014554554150607 ) ) ;
#69954=EDGE_LOOP ( 'NONE', ( #32974, #12761 ) ) ;
#69955=CARTESIAN_POINT ( 'NONE',  ( -17.93474442872397034, -9.442884908240273489, 34.35708131394837039 ) ) ;
#69956=EDGE_LOOP ( 'NONE', ( #81924, #42330, #40010, #61960, #23772, #81081 ) ) ;
#69957=EDGE_LOOP ( 'NONE', ( #46370, #61222 ) ) ;
#69958=CARTESIAN_POINT ( 'NONE',  ( -16.15384615384627409, -6.835583212225970762, 34.95778746994575670 ) ) ;
#69959=EDGE_LOOP ( 'NONE', ( #64140, #66784, #76707, #19824 ) ) ;
#69960=CARTESIAN_POINT ( 'NONE',  ( -6.000000000000121680, -2.379036618888197729, 30.90682066428292885 ) ) ;
#69961=B_SPLINE_CURVE_WITH_KNOTS ( 'NONE', 3,
 ( #68531, #41959, #35190, #21677, #55026, #6829, #54568, #76627, #49146, #14032 ),
 .UNSPECIFIED., .F., .F.,
 ( 4, 2, 2, 2, 4 ),
 ( 0.0007817359430256282712, 0.0009771253907249941549, 0.001172514838424359822, 0.001367904286123725489, 0.001563293733823091372 ),
 .UNSPECIFIED. ) ;
#69962=B_SPLINE_CURVE_WITH_KNOTS ( 'NONE', 3,
 ( #70120, #25040, #11534, #16951, #3870, #44853, #44400, #65570, #72333, #45756 ),
 .UNSPECIFIED., .F., .F.,
 ( 4, 2, 2, 2, 4 ),
 ( 0.0007817359430256297891, 0.0009771253907249958896, 0.001172514838424362207, 0.001367904286123728524, 0.001563293733823094625 ),
 .UNSPECIFIED. ) ;
#69963=CARTESIAN_POINT ( 'NONE',  ( 10.61538461538461675, -9.819645486525091727, 36.12317359536749706 ) ) ;
#69964=CARTESIAN_POINT ( 'NONE',  ( -11.60454494941741999, -11.16473453929635440, 33.15142922261925662 ) ) ;
#69965=CARTESIAN_POINT ( 'NONE',  ( 1.384615384615386802, -13.53365097954675988, 30.81389545987213552 ) ) ;
#69966=CARTESIAN_POINT ( 'NONE',  ( 12.46153846153846168, -10.51840700105979565, 33.73612834413961536 ) ) ;
#69967=CARTESIAN_POINT ( 'NONE',  ( 17.32697749683652688, -8.346898887586322147, 34.93166121998716278 ) ) ;
#69968=DIRECTION ( 'NONE',  ( -0.000000000000000000, 0.1736481776669307198, -0.9848077530122080203 ) ) ;
#69969=CARTESIAN_POINT ( 'NONE',  ( 2.307692307692309264, -9.780366693483667717, 34.19971097300155094 ) ) ;
#69970=CARTESIAN_POINT ( 'NONE',  ( 17.93391658904411656, -11.69971097300155272, 32.46337939537587403 ) ) ;
#69971=DIRECTION ( 'NONE',  ( -0.000000000000000000, -0.5000000000000009992, -0.8660254037844380415 ) ) ;
#69972=LINE ( 'NONE', #1963, #68619 ) ;
#69973=ORIENTED_EDGE ( 'NONE', *, *, #66948, .T. ) ;
#69974=VERTEX_POINT ( 'NONE', #23213 ) ;
#69975=CARTESIAN_POINT ( 'NONE',  ( 3.230769230769108269, -11.06231777344772027, 33.60647404775119895 ) ) ;
#69976=DIRECTION ( 'NONE',  ( -0.000000000000000000, 0.8660254037844399289, -0.4999999999999980016 ) ) ;
#69977=DIRECTION ( 'NONE',  ( -0.000000000000000000, 0.5000000000000011102, -0.8660254037844380415 ) ) ;
#69978=CARTESIAN_POINT ( 'NONE',  ( -2.307692307692305711, -2.499999999999998668, 29.75000000000001421 ) ) ;
#69980=CARTESIAN_POINT ( 'NONE',  ( -15.90379173393269596, -8.346898887586322147, 34.93166121998716278 ) ) ;
#69981=CARTESIAN_POINT ( 'NONE',  ( -13.51476335434708353, -11.04286588640298561, 33.62463336215343901 ) ) ;
#69982=CARTESIAN_POINT ( 'NONE',  ( -3.165513659493205623, -12.27809138561124591, 31.22303859784720359 ) ) ;
#69983=ORIENTED_EDGE ( 'NONE', *, *, #31649, .T. ) ;
#69984=CARTESIAN_POINT ( 'NONE',  ( 0.5267940328144853357, -6.026961402152789304, 34.52809138561124769 ) ) ;
#69985=VERTEX_POINT ( 'NONE', #29538 ) ;
#69986=B_SPLINE_CURVE_WITH_KNOTS ( 'NONE', 3,
 ( #27476, #20276, #6, #46852, #75223, #21150, #87877, #74335, #12634, #13511 ),
 .UNSPECIFIED., .F., .F.,
 ( 4, 2, 2, 2, 4 ),
 ( 0.000000000000000000, 0.0001954339857564072033, 0.0003908679715128144066, 0.0005863019572692215828, 0.0007817359430256288133 ),
 .UNSPECIFIED. ) ;
#69987=B_SPLINE_CURVE_WITH_KNOTS ( 'NONE', 3,
 ( #85382, #16917, #65541, #3842, #46176, #11953, #59681, #33982, #61445, #60565 ),
 .UNSPECIFIED., .F., .F.,
 ( 4, 2, 2, 2, 4 ),
 ( 0.000000000000000000, 0.0001954311564186858715, 0.0003908623128373717431, 0.0005862934692560576146, 0.0007817246256747434861 ),
 .UNSPECIFIED. ) ;
#69992=CARTESIAN_POINT ( 'NONE',  ( -14.08468095607945969, -11.76359900205217457, 32.36225158514719880 ) ) ;
#69993=CARTESIAN_POINT ( 'NONE',  ( 17.99999999999987566, -8.656820664282941280, 34.87096338111179961 ) ) ;
#69994=B_SPLINE_CURVE_WITH_KNOTS ( 'NONE', 3,
 ( #59879, #60764, #26547, #86942, #79715, #67089, #5389, #52224, #54005, #73400 ),
 .UNSPECIFIED., .F., .F.,
 ( 4, 2, 2, 2, 4 ),
 ( 0.0007817359430256327164, 0.0009771253907249995759, 0.001172514838424366544, 0.001367904286123733295, 0.001563293733823100263 ),
 .UNSPECIFIED. ) ;
#69995=ORIENTED_EDGE ( 'NONE', *, *, #42513, .T. ) ;
#69996=EDGE_CURVE ( 'NONE', #52292, #38569, #8825, .T. ) ;
#69997=ORIENTED_EDGE ( 'NONE', *, *, #33731, .T. ) ;
#69998=EDGE_CURVE ( 'NONE', #62271, #66561, #3204, .T. ) ;
#70000=ORIENTED_EDGE ( 'NONE', *, *, #83557, .T. ) ;
#70002=CARTESIAN_POINT ( 'NONE',  ( -6.130147209438217004, -11.47017969459903952, 32.78971311882034456 ) ) ;
#70003=CARTESIAN_POINT ( 'NONE',  ( -16.82686876528476105, -3.627508038966690496, 32.91356715214248396 ) ) ;
#70004=CARTESIAN_POINT ( 'NONE',  ( -12.39547112818838492, -12.34228464037088813, 31.77849191805839268 ) ) ;
#70005=CARTESIAN_POINT ( 'NONE',  ( -2.241624974342229848, -11.35647404775217595, 33.31231777344667222 ) ) ;
#70006=EDGE_CURVE ( 'NONE', #49403, #33332, #60154, .T. ) ;
#70007=CARTESIAN_POINT ( 'NONE',  ( -17.75005448165186195, -4.336752205174650321, 33.62275283266504289 ) ) ;
#70008=FACE_OUTER_BOUND ( 'NONE', #39782, .T. ) ;
#70009=ORIENTED_EDGE ( 'NONE', *, *, #87442, .F. ) ;
#70010=ORIENTED_EDGE ( 'NONE', *, *, #82498, .T. ) ;
#70013=VERTEX_POINT ( 'NONE', #87607 ) ;
#70015=CARTESIAN_POINT ( 'NONE',  ( -10.54931728203453822, -6.343179335718452272, 34.87096338111212646 ) ) ;
#70016=CARTESIAN_POINT ( 'NONE',  ( 9.468822748583747284, -2.599994579823202923, 30.74605699353653776 ) ) ;
#70018=CARTESIAN_POINT ( 'NONE',  ( 13.38461538461538680, -8.120952969808772792, 34.71129190930000163 ) ) ;
#70019=ORIENTED_EDGE ( 'NONE', *, *, #11480, .F. ) ;
#70020=B_SPLINE_CURVE_WITH_KNOTS ( 'NONE', 3,
 ( #82813, #56214, #21987, #84588, #70171, #28291, #7144, #14340, #8478, #2150 ),
 .UNSPECIFIED., .F., .F.,
 ( 4, 2, 2, 2, 4 ),
 ( 0.000000000000000000, 0.0001954339857564084502, 0.0003908679715128169003, 0.0005863019572692253776, 0.0007817359430256338006 ),
 .UNSPECIFIED. ) ;
#70021=EDGE_CURVE ( 'NONE', #36076, #81591, #56964, .T. ) ;
#70022=B_SPLINE_CURVE_WITH_KNOTS ( 'NONE', 3,
 ( #40473, #20622, #25610, #67936, #53066, #26059 ),
 .UNSPECIFIED., .F., .F.,
 ( 4, 2, 4 ),
 ( 0.0003909569690057816227, 0.0005862646681846067891, 0.0007815723673634319014 ),
 .UNSPECIFIED. ) ;
#70023=ORIENTED_EDGE ( 'NONE', *, *, #60650, .T. ) ;
#70024=CARTESIAN_POINT ( 'NONE',  ( -7.846153846153844924, -12.78798330534102945, 29.74999999999997868 ) ) ;
#70025=B_SPLINE_CURVE_WITH_KNOTS ( 'NONE', 3,
 ( #1339, #69799, #21166, #7222, #77008, #47757, #20295, #62156, #42784, #54960 ),
 .UNSPECIFIED., .F., .F.,
 ( 4, 2, 2, 2, 4 ),
 ( 0.0007817246256747514008, 0.0009771112852218952725, 0.001172497944769039253, 0.001367884604316183233, 0.001563271263863327213 ),
 .UNSPECIFIED. ) ;
#70026=ORIENTED_EDGE ( 'NONE', *, *, #85193, .F. ) ;
#70027=FACE_BOUND ( 'NONE', #71244, .T. ) ;
#70028=CARTESIAN_POINT ( 'NONE',  ( -6.923076923076922462, -13.04860791097971706, 34.73218667398347037 ) ) ;
#70029=CARTESIAN_POINT ( 'NONE',  ( 0.4615384615383396616, -11.48612834414049644, 32.76840700105863391 ) ) ;
#70031=CARTESIAN_POINT ( 'NONE',  ( 15.00794113313435219, -7.369209533119137845, 34.99857337881830688 ) ) ;
#70032=CARTESIAN_POINT ( 'NONE',  ( 16.15384615384603251, -4.481592998941358097, 33.73612834414048933 ) ) ;
#70033=VECTOR ( 'NONE', #19362, 1000.000000000000227 ) ;
#70034=CARTESIAN_POINT ( 'NONE',  ( -1.384615384615383471, -4.102666532097928531, 36.13435417666054406 ) ) ;
#70035=CARTESIAN_POINT ( 'NONE',  ( 4.023154687178596589, -11.18331474514187995, 33.13161551792790505 ) ) ;
#70036=CARTESIAN_POINT ( 'NONE',  ( 4.376857505459001096, -3.105924265160262543, 32.13625925475356127 ) ) ;
#70038=CARTESIAN_POINT ( 'NONE',  ( -11.31568186948347154, -12.47679350104403007, 31.42216943046555855 ) ) ;
#70041=DIRECTION ( 'NONE',  ( -0.000000000000000000, 0.8660254037844399289, -0.4999999999999980016 ) ) ;
#70043=EDGE_CURVE ( 'NONE', #28560, #65473, #52899, .T. ) ;
#70044=FACE_BOUND ( 'NONE', #71177, .T. ) ;
#70045=CARTESIAN_POINT ( 'NONE',  ( 17.32697738856138869, -3.627508038966690496, 32.91356715214248396 ) ) ;
#70046=CARTESIAN_POINT ( 'NONE',  ( 11.53846153846153832, -12.37446782046654192, 30.86335684631486131 ) ) ;
#70047=CARTESIAN_POINT ( 'NONE',  ( 11.66925197942848769, -11.93129842949671726, 32.56571108434900452 ) ) ;
#70048=CARTESIAN_POINT ( 'NONE',  ( -3.360917200500929791, -3.069018819979302926, 32.56621877034667278 ) ) ;
#70050=ADVANCED_FACE ( 'NONE', ( #4732 ), #87163, .F. ) ;
#70051=LINE ( 'NONE', #29520, #70699 ) ;
#70053=ORIENTED_EDGE ( 'NONE', *, *, #83416, .T. ) ;
#70055=ORIENTED_EDGE ( 'NONE', *, *, #58239, .T. ) ;
#70056=CARTESIAN_POINT ( 'NONE',  ( -13.25382494364843389, -10.70102852606553157, 33.91149625220312913 ) ) ;
#70057=EDGE_CURVE ( 'NONE', #80983, #2346, #86273, .T. ) ;
#70058=VECTOR ( 'NONE', #15750, 1000.000000000000000 ) ;
#70060=EDGE_CURVE ( 'NONE', #41484, #45738, #45167, .T. ) ;
#70061=CARTESIAN_POINT ( 'NONE',  ( 0.4615384615384611755, -1.215029322943914858, 32.30358669280327177 ) ) ;
#70062=DIRECTION ( 'NONE',  ( -0.000000000000000000, -0.5000000000000009992, -0.8660254037844380415 ) ) ;
#70063=VERTEX_POINT ( 'NONE', #59665 ) ;
#70064=CARTESIAN_POINT ( 'NONE',  ( -8.096130577096198877, -5.728515186090277211, 34.42611988154120439 ) ) ;
#70067=B_SPLINE_CURVE_WITH_KNOTS ( 'NONE', 3,
 ( #36474, #57183, #77457, #17534, #44985, #44090, #22950, #15763, #65257, #64365 ),
 .UNSPECIFIED., .F., .F.,
 ( 4, 2, 2, 2, 4 ),
 ( 0.0007817359430256308733, 0.0009771253907249971907, 0.001172514838424363725, 0.001367904286123730259, 0.001563293733823096577 ),
 .UNSPECIFIED. ) ;
#70068=CARTESIAN_POINT ( 'NONE',  ( 1.384615384615264011, -12.51329471203414379, 31.30864560766407578 ) ) ;
#70069=CARTESIAN_POINT ( 'NONE',  ( 7.146088274689774700, -9.086983370893049639, 34.49168942202179267 ) ) ;
#70070=CARTESIAN_POINT ( 'NONE',  ( -5.076923076923197442, -12.46129190930018460, 30.37095296980731973 ) ) ;
#70071=LINE ( 'NONE', #63311, #63112 ) ;
#70072=CYLINDRICAL_SURFACE ( 'NONE', #28138, 0.2500000000000008882 ) ;
#70073=B_SPLINE_CURVE_WITH_KNOTS ( 'NONE', 3,
 ( #31797, #67356, #31346, #25479, #52933, #59257, #53386, #25921, #45745, #58808 ),
 .UNSPECIFIED., .F., .F.,
 ( 4, 2, 2, 2, 4 ),
 ( 0.0007817246256747444619, 0.0009771112852218868158, 0.001172497944769029061, 0.001367884604316171523, 0.001563271263863313769 ),
 .UNSPECIFIED. ) ;
#70076=DIRECTION ( 'NONE',  ( -0.000000000000000000, -0.6427876096865404731, -0.7660444431189771253 ) ) ;
#70077=AXIS2_PLACEMENT_3D ( 'NONE', #73402, #80162, #46813 ) ;
#70080=DIRECTION ( 'NONE',  ( -0.000000000000000000, -0.1736481776669307198, -0.9848077530122080203 ) ) ;
#70081=ORIENTED_EDGE ( 'NONE', *, *, #59680, .F. ) ;
#70082=DIRECTION ( 'NONE',  ( -0.000000000000000000, -0.3420201433256694346, -0.9396926207859080948 ) ) ;
#70083=CARTESIAN_POINT ( 'NONE',  ( -3.230769230769352962, -5.941354392335915335, 34.76329471203413846 ) ) ;
#70084=DIRECTION ( 'NONE',  ( 0.000000000000000000, 0.6427876096865373645, -0.7660444431189797898 ) ) ;
#70085=DIRECTION ( 'NONE',  ( 0.000000000000000000, 0.1736481776669275834, 0.9848077530122086864 ) ) ;
#70087=CARTESIAN_POINT ( 'NONE',  ( 9.692307692307695177, -11.16473453929635440, 33.15142922261926373 ) ) ;
#70088=CYLINDRICAL_SURFACE ( 'NONE', #47645, 0.2499999999999973355 ) ;
#70089=ADVANCED_FACE ( 'NONE', ( #52009 ), #65528, .F. ) ;
#70090=VECTOR ( 'NONE', #64466, 1000.000000000000000 ) ;
#70091=ORIENTED_EDGE ( 'NONE', *, *, #31671, .T. ) ;
#70092=ORIENTED_EDGE ( 'NONE', *, *, #63555, .F. ) ;
#70093=VECTOR ( 'NONE', #88429, 1000.000000000000000 ) ;
#70094=VERTEX_POINT ( 'NONE', #11486 ) ;
#70095=CARTESIAN_POINT ( 'NONE',  ( -13.63459211555773720, -3.627789207965226748, 32.91389620160131102 ) ) ;
#70096=CARTESIAN_POINT ( 'NONE',  ( 3.230769230769108269, -5.941354392335915335, 34.76329471203413846 ) ) ;
#70097=CARTESIAN_POINT ( 'NONE',  ( 6.673053698855467175, -2.985938066672154445, 32.43141759479405550 ) ) ;
#70098=VECTOR ( 'NONE', #8933, 1000.000000000000000 ) ;
#70099=DIRECTION ( 'NONE',  ( -0.000000000000000000, 0.3420201433256694346, -0.9396926207859080948 ) ) ;
#70100=CARTESIAN_POINT ( 'NONE',  ( 13.13463864056679498, -8.347322224742351082, 34.93158281831414769 ) ) ;
#70101=EDGE_CURVE ( 'NONE', #73925, #11539, #71967, .T. ) ;
#70102=VERTEX_POINT ( 'NONE', #38514 ) ;
#70104=ORIENTED_EDGE ( 'NONE', *, *, #85504, .T. ) ;
#70105=ORIENTED_EDGE ( 'NONE', *, *, #37861, .F. ) ;
#70106=VERTEX_POINT ( 'NONE', #3383 ) ;
#70107=CARTESIAN_POINT ( 'NONE',  ( -15.29685264172511161, -12.10708131394839349, 31.69288490824020244 ) ) ;
#70108=EDGE_LOOP ( 'NONE', ( #43294, #22129, #52441, #86319 ) ) ;
#70109=CARTESIAN_POINT ( 'NONE',  ( 2.307692307692309264, -1.629998284177014645, 34.34916445242399163 ) ) ;
#70110=CARTESIAN_POINT ( 'NONE',  ( -10.36538461538467715, -7.565270445406050648, 34.75000000000000000 ) ) ;
#70112=AXIS2_PLACEMENT_3D ( 'NONE', #45532, #24815, #4549 ) ;
#70113=CARTESIAN_POINT ( 'NONE',  ( 2.057692307692309708, -2.499999999999998668, 29.75000000000000355 ) ) ;
#70114=CARTESIAN_POINT ( 'NONE',  ( -4.826923076923014477, -7.434744429011176159, 34.75000000000000711 ) ) ;
#70116=EDGE_CURVE ( 'NONE', #19898, #48076, #85817, .T. ) ;
#70117=ORIENTED_EDGE ( 'NONE', *, *, #69817, .F. ) ;
#70118=VERTEX_POINT ( 'NONE', #86726 ) ;
#70119=CARTESIAN_POINT ( 'NONE',  ( -14.43830266731683132, -7.722926236386453702, 34.74524107206102030 ) ) ;
#70120=CARTESIAN_POINT ( 'NONE',  ( 15.23076923076911093, -6.026961402154118019, 34.52809138561165270 ) ) ;
#70121=ORIENTED_EDGE ( 'NONE', *, *, #30369, .F. ) ;
#70122=CARTESIAN_POINT ( 'NONE',  ( 1.634560902963527740, -9.272278438253398036, 34.42582936511637826 ) ) ;
#70123=DIRECTION ( 'NONE',  ( -0.000000000000000000, 0.3420201433256694346, -0.9396926207859080948 ) ) ;
#70124=CARTESIAN_POINT ( 'NONE',  ( 7.053868730901712070, -11.71459661697925903, 32.44059661609676937 ) ) ;
#70125=ORIENTED_EDGE ( 'NONE', *, *, #69317, .T. ) ;
#70126=AXIS2_PLACEMENT_3D ( 'NONE', #22661, #50570, #57777 ) ;
#70128=CARTESIAN_POINT ( 'NONE',  ( -11.31568199719312773, -5.114059244376869984, 34.14424750095245287 ) ) ;
#70129=DIRECTION ( 'NONE',  ( 1.000000000000000000, 0.000000000000000000, 0.000000000000000000 ) ) ;
#70130=EDGE_LOOP ( 'NONE', ( #43853, #81402, #9444, #41995 ) ) ;
#70131=FACE_BOUND ( 'NONE', #20048, .T. ) ;
#70132=DIRECTION ( 'NONE',  ( -0.000000000000000000, -0.7660444431189792347, -0.6427876096865379196 ) ) ;
#70133=CARTESIAN_POINT ( 'NONE',  ( -18.24997674404858827, -12.41104346484419452, 31.60698883733904196 ) ) ;
#70134=DIRECTION ( 'NONE',  ( 0.000000000000000000, 0.8660254037844377084, 0.5000000000000015543 ) ) ;
#70135=DIRECTION ( 'NONE',  ( -0.000000000000000000, 1.000000000000000000, 3.491481338843133355E-15 ) ) ;
#70136=CARTESIAN_POINT ( 'NONE',  ( -6.923076923076922462, -2.538708090699994813, 30.37095296980875503 ) ) ;
#70137=ADVANCED_FACE ( 'NONE', ( #19130 ), #40297, .F. ) ;
#70138=CARTESIAN_POINT ( 'NONE',  ( -4.946131269098289707, -10.54018710029568595, 33.71981072465678864 ) ) ;
#70139=CARTESIAN_POINT ( 'NONE',  ( -15.90390063549801347, -9.272278438253401589, 34.42582936511637826 ) ) ;
#70140=VERTEX_POINT ( 'NONE', #27652 ) ;
#70141=CARTESIAN_POINT ( 'NONE',  ( -2.307692307692305711, -3.937682226553329556, 33.60647404775216529 ) ) ;
#70142=EDGE_CURVE ( 'NONE', #37962, #4784, #54229, .T. ) ;
#70143=FACE_OUTER_BOUND ( 'NONE', #31811, .T. ) ;
#70144=EDGE_LOOP ( 'NONE', ( #23349, #7081, #82325, #87500 ) ) ;
#70145=CARTESIAN_POINT ( 'NONE',  ( -10.61538461538461320, -8.973038597847269315, 34.52809138561121927 ) ) ;
#70146=CARTESIAN_POINT ( 'NONE',  ( -14.05763788777885637, -9.233818618650603938, 34.70587769442853698 ) ) ;
#70147=CARTESIAN_POINT ( 'NONE',  ( 3.100292522652767335, -7.276988635370450709, 34.74523720219453793 ) ) ;
#70149=CARTESIAN_POINT ( 'NONE',  ( 17.86985279056177944, -6.001485441113818986, 34.52039167877662607 ) ) ;
#70150=CARTESIAN_POINT ( 'NONE',  ( -8.769230769230768274, -5.557115091759785130, 34.35708131394839171 ) ) ;
#70152=FACE_BOUND ( 'NONE', #32607, .T. ) ;
#70153=CYLINDRICAL_SURFACE ( 'NONE', #98, 0.2499999999999998890 ) ;
#70155=CARTESIAN_POINT ( 'NONE',  ( 1.634560793993430350, -12.68172785388650681, 30.59649109432439573 ) ) ;
#70156=CARTESIAN_POINT ( 'NONE',  ( -17.86947429823644029, -11.46989282347012740, 32.79007818306219946 ) ) ;
#70157=CARTESIAN_POINT ( 'NONE',  ( 7.715593254411924562, -2.504760397472875155, 29.97295953869789997 ) ) ;
#70159=VECTOR ( 'NONE', #40900, 1000.000000000000227 ) ;
#70161=ORIENTED_EDGE ( 'NONE', *, *, #24880, .T. ) ;
#70162=EDGE_CURVE ( 'NONE', #81839, #12293, #77402, .T. ) ;
#70163=B_SPLINE_CURVE_WITH_KNOTS ( 'NONE', 3,
 ( #44458, #79154, #31410, #10698, #17900, #52558, #30082, #24198, #50771, #58419 ),
 .UNSPECIFIED., .F., .F.,
 ( 4, 2, 2, 2, 4 ),
 ( 0.000000000000000000, 0.0001954339857564132749, 0.0003908679715128195566, 0.0005863019572692258112, 0.0007817359430256319575 ),
 .UNSPECIFIED. ) ;
#70164=ORIENTED_EDGE ( 'NONE', *, *, #68195, .F. ) ;
#70165=CARTESIAN_POINT ( 'NONE',  ( 5.326868595271218254, -6.696923467548660192, 34.68552623307873972 ) ) ;
#70167=VECTOR ( 'NONE', #2271, 1000.000000000000227 ) ;
#70168=CARTESIAN_POINT ( 'NONE',  ( -15.29685161012936412, -5.471508081941602875, 34.59228464037088457 ) ) ;
#70169=CARTESIAN_POINT ( 'NONE',  ( 14.37294744720514572, -9.528491918058460186, 34.59228464037086326 ) ) ;
#70170=CARTESIAN_POINT ( 'NONE',  ( -16.85414353565466428, -11.41317474335729543, 32.86274602512330034 ) ) ;
#70171=CARTESIAN_POINT ( 'NONE',  ( -16.40382288478850725, -12.17611988154120795, 31.52148481390971213 ) ) ;
#70173=DIRECTION ( 'NONE',  ( -0.000000000000000000, 0.3420201433256694346, -0.9396926207859080948 ) ) ;
#70174=CYLINDRICAL_SURFACE ( 'NONE', #46047, 0.2500000000000004996 ) ;
#70175=CARTESIAN_POINT ( 'NONE',  ( 6.000000000000001776, -3.937682226553329556, 33.60647404775216529 ) ) ;
#70176=CARTESIAN_POINT ( 'NONE',  ( -3.165514091256391715, -12.16647553114626490, 32.15551576947920864 ) ) ;
#70177=CARTESIAN_POINT ( 'NONE',  ( -3.480792454990686124, -4.175268141568689195, 33.81360843649122216 ) ) ;
#70178=CARTESIAN_POINT ( 'NONE',  ( 16.37685750545900376, -4.887748414852792322, 34.01359900205217457 ) ) ;
#70179=CARTESIAN_POINT ( 'NONE',  ( 12.52760579488853665, -2.292212530054420494, 30.41441678777542990 ) ) ;
#70181=EDGE_CURVE ( 'NONE', #50406, #6751, #47473, .T. ) ;
#70182=EDGE_LOOP ( 'NONE', ( #6408, #47938, #88108, #20949 ) ) ;
#70183=CARTESIAN_POINT ( 'NONE',  ( -14.37296275365308240, -3.835265460703609186, 33.15142922261924241 ) ) ;
#70184=CARTESIAN_POINT ( 'NONE',  ( 10.61538461538449418, -5.941354392335915335, 34.76329471203413846 ) ) ;
#70186=B_SPLINE_CURVE_WITH_KNOTS ( 'NONE', 3,
 ( #63841, #42258, #56644, #77796, #2136, #83693, #35489, #85011, #2569, #16101 ),
 .UNSPECIFIED., .F., .F.,
 ( 4, 2, 2, 2, 4 ),
 ( 0.0007817246256747509671, 0.0009771112852218959231, 0.001172497944769040987, 0.001367884604316185835, 0.001563271263863330899 ),
 .UNSPECIFIED. ) ;
#70187=CARTESIAN_POINT ( 'NONE',  ( 0.6843181305165275674, -3.563462043263030399, 33.22394488606062879 ) ) ;
#70188=VECTOR ( 'NONE', #18867, 1000.000000000000227 ) ;
#70189=CARTESIAN_POINT ( 'NONE',  ( 4.153846153846032507, -10.21337939537710326, 33.94971097300076224 ) ) ;
#70190=ORIENTED_EDGE ( 'NONE', *, *, #81140, .F. ) ;
#70191=EDGE_CURVE ( 'NONE', #13277, #2439, #16143, .T. ) ;
#70192=CARTESIAN_POINT ( 'NONE',  ( -9.915792616872023402, -5.827078755546623690, 34.72654668319379567 ) ) ;
#70193=DIRECTION ( 'NONE',  ( -0.000000000000000000, -0.8660254037844397068, -0.4999999999999978906 ) ) ;
#70194=VERTEX_POINT ( 'NONE', #53349 ) ;
#70195=CARTESIAN_POINT ( 'NONE',  ( 9.942362112221147186, -12.65882529074907126, 30.72640787790839312 ) ) ;
#70196=CARTESIAN_POINT ( 'NONE',  ( -22.75000000000000000, -7.500000000000000000, 29.75000000000000355 ) ) ;
#70197=ORIENTED_EDGE ( 'NONE', *, *, #64097, .T. ) ;
#70198=CARTESIAN_POINT ( 'NONE',  ( -5.207070286361299871, -12.27039167877662251, 31.24851455888617835 ) ) ;
#70199=CARTESIAN_POINT ( 'NONE',  ( 7.715543486529319317, -7.722926236386456367, 34.74524107206103452 ) ) ;
#70200=EDGE_LOOP ( 'NONE', ( #5007, #72598 ) ) ;
#70201=LINE ( 'NONE', #50790, #1748 ) ;
#70202=ADVANCED_FACE ( 'NONE', ( #55124 ), #47030, .F. ) ;
#70203=CARTESIAN_POINT ( 'NONE',  ( 16.15384615384615330, -2.499999999999998668, 29.75000000000001421 ) ) ;
#70204=AXIS2_PLACEMENT_3D ( 'NONE', #34754, #28907, #13161 ) ;
#70205=B_SPLINE_CURVE_WITH_KNOTS ( 'NONE', 3,
 ( #6480, #22969, #9460, #88915, #19981, #47447, #43684, #49564, #16218, #22094 ),
 .UNSPECIFIED., .F., .F.,
 ( 4, 2, 2, 2, 4 ),
 ( 0.0007817359430256216575, 0.0009771253907249856981, 0.001172514838424349847, 0.001367904286123713779, 0.001563293733823077928 ),
 .UNSPECIFIED. ) ;
#70206=CARTESIAN_POINT ( 'NONE',  ( 9.822833130541338775, -6.808710257144161559, 34.95449254468098843 ) ) ;
#70207=ORIENTED_EDGE ( 'NONE', *, *, #68492, .F. ) ;
#70208=ORIENTED_EDGE ( 'NONE', *, *, #10164, .F. ) ;
#70209=CARTESIAN_POINT ( 'NONE',  ( -6.923076923077045919, -8.656820664282941280, 34.87096338111179961 ) ) ;
#70210=B_SPLINE_CURVE_WITH_KNOTS ( 'NONE', 3,
 ( #19403, #46871, #1343, #23377, #1785, #69369, #43653, #71124, #36466, #35131 ),
 .UNSPECIFIED., .F., .F.,
 ( 4, 2, 2, 2, 4 ),
 ( 0.000000000000000000, 0.0001954311564186862781, 0.0003908623128373725562, 0.0005862934692560588072, 0.0007817246256747451124 ),
 .UNSPECIFIED. ) ;
#70211=EDGE_CURVE ( 'NONE', #39096, #45764, #12950, .T. ) ;
#70212=ORIENTED_EDGE ( 'NONE', *, *, #7073, .T. ) ;
#70214=CARTESIAN_POINT ( 'NONE',  ( 5.076923076922953193, -5.094484230521993062, 34.41647553114689373 ) ) ;
#70215=CARTESIAN_POINT ( 'NONE',  ( 13.38461538461538680, -3.322132147404559976, 32.92929555188717927 ) ) ;
#70217=ADVANCED_FACE ( 'NONE', ( #33537 ), #26770, .F. ) ;
#70218=CARTESIAN_POINT ( 'NONE',  ( 7.846153846153725020, -2.892918686052165622, 31.69288490824153470 ) ) ;
#70219=ORIENTED_EDGE ( 'NONE', *, *, #60487, .T. ) ;
#70220=ORIENTED_EDGE ( 'NONE', *, *, #5379, .F. ) ;
#70221=DIRECTION ( 'NONE',  ( 0.000000000000000000, 0.7660444431189807890, 0.6427876096865361433 ) ) ;
#70222=VERTEX_POINT ( 'NONE', #63201 ) ;
#70223=VECTOR ( 'NONE', #30907, 1000.000000000000227 ) ;
#70224=CARTESIAN_POINT ( 'NONE',  ( 16.37722209454433653, -2.501478030877322567, 29.88021232661721172 ) ) ;
#70226=CARTESIAN_POINT ( 'NONE',  ( 7.846153846153723244, -12.16647553114689728, 32.15551576947799362 ) ) ;
#70227=LINE ( 'NONE', #64336, #19455 ) ;
#70228=VERTEX_POINT ( 'NONE', #84383 ) ;
#70230=DIRECTION ( 'NONE',  ( 0.000000000000000000, 0.3420201433256610524, 0.9396926207859113145 ) ) ;
#70231=EDGE_LOOP ( 'NONE', ( #8516, #3073 ) ) ;
#70232=CARTESIAN_POINT ( 'NONE',  ( -8.703162418228330921, -8.120952969808772792, 34.71129190929999453 ) ) ;
#70233=ORIENTED_EDGE ( 'NONE', *, *, #67586, .F. ) ;
#70234=B_SPLINE_CURVE_WITH_KNOTS ( 'NONE', 3,
 ( #86190, #16822, #11861, #45626, #37987, #85737, #10067, #73106, #39337, #11402 ),
 .UNSPECIFIED., .F., .F.,
 ( 4, 2, 2, 2, 4 ),
 ( 0.000000000000000000, 0.0001954339857564079623, 0.0003908679715128159245, 0.0005863019572692238597, 0.0007817359430256318490 ),
 .UNSPECIFIED. ) ;
#70235=DIRECTION ( 'NONE',  ( -0.000000000000000000, 0.5000000000000011102, -0.8660254037844380415 ) ) ;
#70237=ORIENTED_EDGE ( 'NONE', *, *, #45902, .T. ) ;
#70238=CARTESIAN_POINT ( 'NONE',  ( 4.153846153846154188, -13.75783147151868846, 33.36296068462461051 ) ) ;
#70239=CARTESIAN_POINT ( 'NONE',  ( 6.923076923076924238, -5.471508081941601098, 34.59228464037088457 ) ) ;
#70240=FACE_BOUND ( 'NONE', #66709, .T. ) ;
#70242=DIRECTION ( 'NONE',  ( 1.000000000000000000, 0.000000000000000000, 0.000000000000000000 ) ) ;
#70243=CARTESIAN_POINT ( 'NONE',  ( 9.626225312947553903, -2.292212530054419606, 30.41441678777542634 ) ) ;
#70244=CARTESIAN_POINT ( 'NONE',  ( -17.01085574357299990, -12.34228464037088813, 31.77849191805839268 ) ) ;
#70245=VECTOR ( 'NONE', #59639, 1000.000000000000227 ) ;
#70246=CARTESIAN_POINT ( 'NONE',  ( -3.099977422944445671, -3.062576670634119758, 32.05464942895959979 ) ) ;
#70247=CARTESIAN_POINT ( 'NONE',  ( 11.53846153846153832, -13.20930481340135110, 34.54067556320372745 ) ) ;
#70248=VERTEX_POINT ( 'NONE', #22227 ) ;
#70249=CARTESIAN_POINT ( 'NONE',  ( -14.30769230769230660, -3.513871655860378418, 32.76840700105978499 ) ) ;
#70250=ORIENTED_EDGE ( 'NONE', *, *, #79544, .F. ) ;
#70251=VERTEX_POINT ( 'NONE', #8278 ) ;
#70253=CARTESIAN_POINT ( 'NONE',  ( -5.076923076923199218, -12.16647553114689728, 32.15551576947799362 ) ) ;
#70254=CARTESIAN_POINT ( 'NONE',  ( -3.480745974817821775, -5.643011162660950042, 34.66104346484419096 ) ) ;
#70256=CARTESIAN_POINT ( 'NONE',  ( 15.23076923076923173, -8.164416787775445883, 34.95778746994557906 ) ) ;
#70258=CARTESIAN_POINT ( 'NONE',  ( 0.4615384615383396616, -2.625532179533779154, 30.86335684631627174 ) ) ;
#70259=CARTESIAN_POINT ( 'NONE',  ( -4.088591014333315066, -3.643525952247864463, 33.31231777344670064 ) ) ;
#70260=EDGE_LOOP ( 'NONE', ( #27455, #66831 ) ) ;
#70261=FACE_OUTER_BOUND ( 'NONE', #53284, .T. ) ;
#70262=AXIS2_PLACEMENT_3D ( 'NONE', #78513, #37979, #31668 ) ;
#70263=EDGE_CURVE ( 'NONE', #2917, #37415, #76280, .T. ) ;
#70264=CARTESIAN_POINT ( 'NONE',  ( -14.43784027742400156, -10.31621877034669588, 34.18098118002070152 ) ) ;
#70265=CARTESIAN_POINT ( 'NONE',  ( -10.54931626438217585, -9.780366693483667717, 34.19971097300155805 ) ) ;
#70266=CARTESIAN_POINT ( 'NONE',  ( 3.165498784808455923, -3.300289026998414865, 32.46337939537583139 ) ) ;
#70267=CARTESIAN_POINT ( 'NONE',  ( 13.63466980452883881, -5.642605341092957971, 34.66089969410670335 ) ) ;
#70268=CARTESIAN_POINT ( 'NONE',  ( 3.007842271862383399, -11.98009711892699691, 32.48740034544075428 ) ) ;
#70269=ORIENTED_EDGE ( 'NONE', *, *, #69768, .F. ) ;
#70270=EDGE_CURVE ( 'NONE', #14815, #53666, #19340, .T. ) ;
#70271=B_SPLINE_CURVE_WITH_KNOTS ( 'NONE', 3,
 ( #38354, #50949, #78440, #44193, #58609, #52744, #72127, #10440, #9983, #58165 ),
 .UNSPECIFIED., .F., .F.,
 ( 4, 2, 2, 2, 4 ),
 ( 0.0007817359527651133143, 0.0009771254036996530456, 0.001172514854634192777, 0.001367904305568732291, 0.001563293756503272023 ),
 .UNSPECIFIED. ) ;
#70272=ORIENTED_EDGE ( 'NONE', *, *, #38404, .F. ) ;
#70274=EDGE_CURVE ( 'NONE', #84739, #29700, #35435, .T. ) ;
#70275=VERTEX_POINT ( 'NONE', #51775 ) ;
#70276=DIRECTION ( 'NONE',  ( 0.000000000000000000, 0.9396926207859126468, 0.3420201433256571111 ) ) ;
#70277=DIRECTION ( 'NONE',  ( 0.000000000000000000, 0.4999999999999985567, 0.8660254037844395958 ) ) ;
#70278=LINE ( 'NONE', #14902, #42381 ) ;
#70279=CARTESIAN_POINT ( 'NONE',  ( -5.076923076923075762, -3.322132147404559976, 32.92929555188717927 ) ) ;
#70280=CARTESIAN_POINT ( 'NONE',  ( -17.32689982097166492, -9.234221910056350069, 34.70572697212741531 ) ) ;
#70281=CARTESIAN_POINT ( 'NONE',  ( 8.639083559792549494, -6.852621066184266141, 34.70813303252209181 ) ) ;
#70282=ORIENTED_EDGE ( 'NONE', *, *, #72896, .F. ) ;
#70283=EDGE_CURVE ( 'NONE', #25143, #45049, #31114, .T. ) ;
#70284=DIRECTION ( 'NONE',  ( -0.000000000000000000, -0.6427876096865404731, -0.7660444431189771253 ) ) ;
#70285=DIRECTION ( 'NONE',  ( -0.000000000000000000, -0.6427876096865404731, -0.7660444431189771253 ) ) ;
#70286=ORIENTED_EDGE ( 'NONE', *, *, #33394, .F. ) ;
#70287=DIRECTION ( 'NONE',  ( -0.000000000000000000, 0.1736481776669307198, -0.9848077530122080203 ) ) ;
#70288=CARTESIAN_POINT ( 'NONE',  ( -17.20707104665477161, -12.15440758774515473, 32.17923288041532004 ) ) ;
#70289=CARTESIAN_POINT ( 'NONE',  ( -10.61538461538473399, -11.48612834414049644, 32.76840700105863391 ) ) ;
#70290=CARTESIAN_POINT ( 'NONE',  ( 0.4615384615383396616, -2.892918686052166066, 31.69288490824153470 ) ) ;
#70292=EDGE_CURVE ( 'NONE', #2182, #82908, #47244, .T. ) ;
#70294=EDGE_LOOP ( 'NONE', ( #42140, #48841, #9515, #88623 ) ) ;
#70295=AXIS2_PLACEMENT_3D ( 'NONE', #61068, #88133, #73258 ) ;
#70296=FACE_OUTER_BOUND ( 'NONE', #75021, .T. ) ;
#70297=CARTESIAN_POINT ( 'NONE',  ( -4.153846153846152411, -9.584722331328613620, 36.20867863119891439 ) ) ;
#70299=CARTESIAN_POINT ( 'NONE',  ( 13.13461538461538680, -7.500000000000001776, 35.00000000000000000 ) ) ;
#70300=CARTESIAN_POINT ( 'NONE',  ( -7.623374177175779920, -3.020022701398814124, 32.48759521482552515 ) ) ;
#70301=ORIENTED_EDGE ( 'NONE', *, *, #89047, .T. ) ;
#70303=CARTESIAN_POINT ( 'NONE',  ( 11.31553457955468645, -4.026226216239094491, 33.68668979543634379 ) ) ;
#70304=ORIENTED_EDGE ( 'NONE', *, *, #8448, .F. ) ;
#70305=CARTESIAN_POINT ( 'NONE',  ( -1.161835843346974428, -6.760870238392817200, 34.69528174975672385 ) ) ;
#70306=CARTESIAN_POINT ( 'NONE',  ( 9.442307692307693401, -7.500000000000001776, 35.00000000000000000 ) ) ;
#70307=ORIENTED_EDGE ( 'NONE', *, *, #49351, .T. ) ;
#70308=DIRECTION ( 'NONE',  ( -0.000000000000000000, 0.1736481776669307198, -0.9848077530122080203 ) ) ;
#70310=CARTESIAN_POINT ( 'NONE',  ( -8.546451100252703270, -5.827830569534417471, 34.72679350104403539 ) ) ;
#70311=CARTESIAN_POINT ( 'NONE',  ( -13.16160254052199008, -12.64618726649961289, 30.78989965857442712 ) ) ;
#70312=ORIENTED_EDGE ( 'NONE', *, *, #85376, .F. ) ;
#70313=CARTESIAN_POINT ( 'NONE',  ( -3.099978789802282364, -2.295524264805589354, 30.44142389570982488 ) ) ;
#70314=ADVANCED_FACE ( 'NONE', ( #79278 ), #5400, .F. ) ;
#70315=VERTEX_POINT ( 'NONE', #60774 ) ;
#70316=CIRCLE ( 'NONE', #58795, 0.2500000000000002220 ) ;
#70317=CARTESIAN_POINT ( 'NONE',  ( 4.153846153846032507, -5.219633306517616589, 34.19971097300220464 ) ) ;
#70318=CARTESIAN_POINT ( 'NONE',  ( 6.250000000001437961, -7.500000000000155431, 34.75000000000007105 ) ) ;
#70319=EDGE_LOOP ( 'NONE', ( #82974, #11423, #54697, #66917 ) ) ;
#70320=CARTESIAN_POINT ( 'NONE',  ( 10.61538461538461675, -11.35647404775217417, 33.31231777344666511 ) ) ;
#70321=CARTESIAN_POINT ( 'NONE',  ( -8.835314180186649935, -2.538708090699994813, 30.37095296980875148 ) ) ;
#70322=CARTESIAN_POINT ( 'NONE',  ( 0.3962680155776846513, -4.481592998940160832, 33.73612834413957984 ) ) ;
#70324=ADVANCED_FACE ( 'NONE', ( #11716 ), #60328, .F. ) ;
#70326=DIRECTION ( 'NONE',  ( -0.000000000000000000, 0.6427876096865404731, -0.7660444431189770143 ) ) ;
#70327=CARTESIAN_POINT ( 'NONE',  ( 3.480769230769230838, -2.249999999999998668, 29.75000000000000355 ) ) ;
#70329=VERTEX_POINT ( 'NONE', #87841 ) ;
#70330=VERTEX_POINT ( 'NONE', #73412 ) ;
#70331=EDGE_CURVE ( 'NONE', #52128, #16142, #84902, .T. ) ;
#70332=FACE_BOUND ( 'NONE', #63211, .T. ) ;
#70333=ORIENTED_EDGE ( 'NONE', *, *, #59222, .T. ) ;
#70335=B_SPLINE_CURVE_WITH_KNOTS ( 'NONE', 3,
 ( #75050, #35379, #82697, #41698, #76363, #269, #35834, #76820, #63290, #34929 ),
 .UNSPECIFIED., .F., .F.,
 ( 4, 2, 2, 2, 4 ),
 ( 0.000000000000000000, 0.0001954311564186868744, 0.0003908623128373737488, 0.0005862934692560606504, 0.0007817246256747474977 ),
 .UNSPECIFIED. ) ;
#70336=CARTESIAN_POINT ( 'NONE',  ( 7.846153846153723244, -12.70778746994576025, 30.41441678777401236 ) ) ;
#70337=CARTESIAN_POINT ( 'NONE',  ( 9.692307692307695177, -12.10708131394839349, 31.69288490824020244 ) ) ;
#70338=CARTESIAN_POINT ( 'NONE',  ( -2.307692307692428724, -10.33852847137269571, 34.16647553114546554 ) ) ;
#70339=EDGE_CURVE ( 'NONE', #88089, #70832, #79477, .T. ) ;
#70340=EDGE_LOOP ( 'NONE', ( #12220, #83832 ) ) ;
#70341=ORIENTED_EDGE ( 'NONE', *, *, #64812, .F. ) ;
#70342=EDGE_LOOP ( 'NONE', ( #71411, #54198 ) ) ;
#70343=CARTESIAN_POINT ( 'NONE',  ( -2.980714810855777053, -11.47946981652013498, 33.17500667209846910 ) ) ;
#70344=EDGE_CURVE ( 'NONE', #49728, #49386, #88543, .T. ) ;
#70346=VERTEX_POINT ( 'NONE', #46819 ) ;
#70347=LINE ( 'NONE', #30247, #45941 ) ;
#70348=VECTOR ( 'NONE', #76583, 1000.000000000000114 ) ;
#70349=CARTESIAN_POINT ( 'NONE',  ( -15.23076923076935252, -11.67786785259630911, 32.92929555188603530 ) ) ;
#70350=EDGE_CURVE ( 'NONE', #8229, #56240, #25218, .T. ) ;
#70351=CARTESIAN_POINT ( 'NONE',  ( 13.51540582558233972, -11.37503395064541678, 33.29242100308974273 ) ) ;
#70352=ORIENTED_EDGE ( 'NONE', *, *, #85284, .F. ) ;
#70353=B_SPLINE_CURVE_WITH_KNOTS ( 'NONE', 3,
 ( #38945, #66404, #60531, #27193, #6046, #46576, #19547, #47009, #25866, #80827 ),
 .UNSPECIFIED., .F., .F.,
 ( 4, 2, 2, 2, 4 ),
 ( 0.0007817246256747473893, 0.0009771112852218907189, 0.001172497944769034049, 0.001367884604316177378, 0.001563271263863320708 ),
 .UNSPECIFIED. ) ;
#70354=CARTESIAN_POINT ( 'NONE',  ( 13.13463865367303463, -10.66389620160130036, 33.62221079203477103 ) ) ;
#70356=CARTESIAN_POINT ( 'NONE',  ( 4.088576153289834814, -2.657715359629089225, 31.77849191805834295 ) ) ;
#70357=CARTESIAN_POINT ( 'NONE',  ( 8.769230769230645706, -6.835583212225970762, 34.95778746994575670 ) ) ;
#70358=ORIENTED_EDGE ( 'NONE', *, *, #1312, .T. ) ;
#70359=ORIENTED_EDGE ( 'NONE', *, *, #2937, .F. ) ;
#70360=ORIENTED_EDGE ( 'NONE', *, *, #847, .T. ) ;
#70361=CARTESIAN_POINT ( 'NONE',  ( -4.153846153846273204, -10.21337939537710326, 33.94971097300076224 ) ) ;
#70362=CARTESIAN_POINT ( 'NONE',  ( 12.23805351781451201, -6.760086850603066466, 34.69517049084099369 ) ) ;
#70363=CARTESIAN_POINT ( 'NONE',  ( 10.61538461538461675, -6.386643153685126251, 34.62446782046654192 ) ) ;
#70364=LINE ( 'NONE', #56838, #51344 ) ;
#70365=CARTESIAN_POINT ( 'NONE',  ( -6.700065571464073777, -3.587049720035815348, 32.86302985866382897 ) ) ;
#70366=FACE_BOUND ( 'NONE', #84790, .T. ) ;
#70367=CARTESIAN_POINT ( 'NONE',  ( 8.769230769230768274, -10.67929555188718282, 33.92786785259544047 ) ) ;
#70368=EDGE_LOOP ( 'NONE', ( #51741, #27685, #59952, #58793 ) ) ;
#70369=B_SPLINE_CURVE_WITH_KNOTS ( 'NONE', 3,
 ( #68358, #88661, #7101, #6656, #60265, #6228, #53505, #20182, #47648, #67482 ),
 .UNSPECIFIED., .F., .F.,
 ( 4, 2, 2, 2, 4 ),
 ( 0.0007817359430256374869, 0.0009771253907250054306, 0.001172514838424373266, 0.001367904286123741101, 0.001563293733823109153 ),
 .UNSPECIFIED. ) ;
#70370=CARTESIAN_POINT ( 'NONE',  ( 17.29993592101647337, -11.98016756924215187, 32.48728574198911190 ) ) ;
#70371=DIRECTION ( 'NONE',  ( -0.000000000000000000, -0.9396926207859092051, -0.3420201433256662704 ) ) ;
#70372=CARTESIAN_POINT ( 'NONE',  ( 11.47270473594723228, -7.249945686854186278, 34.74374336980224598 ) ) ;
#70375=CARTESIAN_POINT ( 'NONE',  ( 4.853996118016226546, -12.64616026154729411, 30.79003144601913533 ) ) ;
#70376=ORIENTED_EDGE ( 'NONE', *, *, #86120, .T. ) ;
#70377=B_SPLINE_CURVE_WITH_KNOTS ( 'NONE', 3,
 ( #32070, #19002, #73953, #51872, #24408, #79370, #78917, #45575, #11350, #72602 ),
 .UNSPECIFIED., .F., .F.,
 ( 4, 2, 2, 2, 4 ),
 ( 0.000000000000000000, 0.0001954311564186858715, 0.0003908623128373717431, 0.0005862934692560576146, 0.0007817246256747434861 ),
 .UNSPECIFIED. ) ;
#70378=FACE_BOUND ( 'NONE', #12364, .T. ) ;
#70379=ADVANCED_FACE ( 'NONE', ( #58994 ), #25665, .F. ) ;
#70380=CARTESIAN_POINT ( 'NONE',  ( 5.076923076922954969, -6.026961402154118908, 34.52809138561165270 ) ) ;
#70382=AXIS2_PLACEMENT_3D ( 'NONE', #88202, #11179, #53489 ) ;
#70383=CARTESIAN_POINT ( 'NONE',  ( 16.85343813319913053, -11.89387501736623420, 32.13663884655804992 ) ) ;
#70384=CARTESIAN_POINT ( 'NONE',  ( 14.05766907039934210, -11.86270091957321249, 32.19358267280087915 ) ) ;
#70385=ORIENTED_EDGE ( 'NONE', *, *, #81758, .T. ) ;
#70387=CARTESIAN_POINT ( 'NONE',  ( -3.361459833879538284, -2.295517848115769421, 30.44137282052137294 ) ) ;
#70388=CARTESIAN_POINT ( 'NONE',  ( 8.638540166120460384, -2.295517848115769421, 30.44137282052137294 ) ) ;
#70390=ORIENTED_EDGE ( 'NONE', *, *, #86250, .T. ) ;
#70391=VECTOR ( 'NONE', #33687, 1000.000000000000114 ) ;
#70392=DIRECTION ( 'NONE',  ( 0.000000000000000000, 0.8660254037844377084, 0.5000000000000015543 ) ) ;
#70393=ORIENTED_EDGE ( 'NONE', *, *, #16956, .F. ) ;
#70394=EDGE_CURVE ( 'NONE', #8812, #19730, #53797, .T. ) ;
#70396=CARTESIAN_POINT ( 'NONE',  ( 18.00000000000000000, -13.75783147151868846, 33.36296068462461051 ) ) ;
#70397=ORIENTED_EDGE ( 'NONE', *, *, #52134, .T. ) ;
#70398=CARTESIAN_POINT ( 'NONE',  ( 11.78840705680968171, -6.696923467548660192, 34.68552623307873972 ) ) ;
#70399=CARTESIAN_POINT ( 'NONE',  ( -10.86540785267757947, -12.43535235679832596, 30.55408501211184813 ) ) ;
#70400=DIRECTION ( 'NONE',  ( 0.000000000000000000, 0.8660254037844377084, 0.5000000000000015543 ) ) ;
#70401=CARTESIAN_POINT ( 'NONE',  ( -15.48076923076922995, -7.566082377512564960, 35.00000000000000711 ) ) ;
#70402=CARTESIAN_POINT ( 'NONE',  ( -3.099978789802278811, -3.957578996910244395, 33.62503395064540257 ) ) ;
#70403=CARTESIAN_POINT ( 'NONE',  ( 8.703960768674447124, -4.320704448112771878, 33.92786785259540494 ) ) ;
#70404=DIRECTION ( 'NONE',  ( -0.000000000000000000, -0.3420201433256694901, -0.9396926207859082059 ) ) ;
#70405=EDGE_CURVE ( 'NONE', #9565, #3410, #49493, .T. ) ;
#70408=CYLINDRICAL_SURFACE ( 'NONE', #85074, 0.2500000000000012212 ) ;
#70410=ORIENTED_EDGE ( 'NONE', *, *, #27443, .F. ) ;
#70411=VERTEX_POINT ( 'NONE', #66652 ) ;
#70412=EDGE_LOOP ( 'NONE', ( #80135, #27831 ) ) ;
#70413=CARTESIAN_POINT ( 'NONE',  ( 10.61538461538449418, -8.656820664282941280, 34.87096338111179961 ) ) ;
#70415=B_SPLINE_CURVE_WITH_KNOTS ( 'NONE', 3,
 ( #15381, #29337, #77954, #49150, #71189, #50899, #55904, #77076, #57682, #44147 ),
 .UNSPECIFIED., .F., .F.,
 ( 4, 2, 2, 2, 4 ),
 ( 0.0007817246256747442451, 0.0009771112852218865989, 0.001172497944769029061, 0.001367884604316171523, 0.001563271263863313986 ),
 .UNSPECIFIED. ) ;
#70416=B_SPLINE_CURVE_WITH_KNOTS ( 'NONE', 3,
 ( #24811, #4087, #24358, #17627, #17164, #58145, #79770, #44621, #10421, #72555 ),
 .UNSPECIFIED., .F., .F.,
 ( 4, 2, 2, 2, 4 ),
 ( 0.000000000000000000, 0.0001954311564186880399, 0.0003908623128373760799, 0.0005862934692560641198, 0.0007817246256747521597 ),
 .UNSPECIFIED. ) ;
#70418=DIRECTION ( 'NONE',  ( -0.000000000000000000, 0.1736481776669307198, -0.9848077530122080203 ) ) ;
#70419=CARTESIAN_POINT ( 'NONE',  ( -8.992157728137614825, -2.523278758544489797, 31.42238647778637528 ) ) ;
#70420=EDGE_CURVE ( 'NONE', #84034, #30710, #35526, .T. ) ;
#70421=CARTESIAN_POINT ( 'NONE',  ( 17.14299041027315695, -8.164416787775445883, 34.95778746994558617 ) ) ;
#70422=CARTESIAN_POINT ( 'NONE',  ( 5.934677084507826272, -7.749976743299137993, 34.99404534957040624 ) ) ;
#70423=CARTESIAN_POINT ( 'NONE',  ( 6.000000000000001776, -12.78798330534103123, 29.99999999999997868 ) ) ;
#70424=CARTESIAN_POINT ( 'NONE',  ( 17.93472955403922242, -11.94971097300153140, 32.03036669348370680 ) ) ;
#70425=CARTESIAN_POINT ( 'NONE',  ( 12.39626801557768410, -11.94971097300153140, 32.03036669348370680 ) ) ;
#70426=VECTOR ( 'NONE', #18871, 999.9999999999998863 ) ;
#70429=ORIENTED_EDGE ( 'NONE', *, *, #74410, .T. ) ;
#70430=CARTESIAN_POINT ( 'NONE',  ( 8.900021210197722965, -2.845873456487966635, 32.17976146951972538 ) ) ;
#70431=CARTESIAN_POINT ( 'NONE',  ( -16.08865316555149860, -2.255955759149234741, 29.99999999999988276 ) ) ;
#70433=CARTESIAN_POINT ( 'NONE',  ( -2.530519000171310484, -7.369208160676173236, 34.74850200257122879 ) ) ;
#70436=EDGE_CURVE ( 'NONE', #5877, #81602, #41832, .T. ) ;
#70438=CARTESIAN_POINT ( 'NONE',  ( -17.14219352288385778, -3.835265460703609186, 33.15142922261924241 ) ) ;
#70439=CARTESIAN_POINT ( 'NONE',  ( -9.561517251340742263, -3.338503747796866872, 32.95102852606553512 ) ) ;
#70440=EDGE_CURVE ( 'NONE', #11287, #82297, #7369, .T. ) ;
#70441=ORIENTED_EDGE ( 'NONE', *, *, #79894, .F. ) ;
#70442=CARTESIAN_POINT ( 'NONE',  ( 0.5923302693632478411, -5.582136614379148654, 34.36778462344220486 ) ) ;
#70443=EDGE_CURVE ( 'NONE', #35844, #32821, #28774, .T. ) ;
#70444=ORIENTED_EDGE ( 'NONE', *, *, #23564, .F. ) ;
#70445=CARTESIAN_POINT ( 'NONE',  ( 10.61538461538461675, -8.120952969808772792, 34.71129190930000163 ) ) ;
#70446=AXIS2_PLACEMENT_3D ( 'NONE', #47065, #26810, #33575 ) ;
#70447=CARTESIAN_POINT ( 'NONE',  ( -3.360916440207453615, -12.27039167877662251, 31.24851455888617835 ) ) ;
#70448=CARTESIAN_POINT ( 'NONE',  ( -15.23076923076922995, -1.215029322943914858, 32.30358669280327177 ) ) ;
#70449=CARTESIAN_POINT ( 'NONE',  ( -9.757577692864012775, -8.656820664281498878, 34.87096338111211935 ) ) ;
#70450=DIRECTION ( 'NONE',  ( -0.000000000000000000, -0.9848077530122085754, -0.1736481776669273613 ) ) ;
#70454=B_SPLINE_CURVE_WITH_KNOTS ( 'NONE', 3,
 ( #32288, #59752, #33616, #67400, #53428, #12455, #26857, #87247, #54316, #18775 ),
 .UNSPECIFIED., .F., .F.,
 ( 4, 2, 2, 2, 4 ),
 ( 0.000000000000000000, 0.0001954339857564073659, 0.0003908679715128147319, 0.0005863019572692221250, 0.0007817359430256294638 ),
 .UNSPECIFIED. ) ;
#70455=EDGE_CURVE ( 'NONE', #86919, #23926, #7612, .T. ) ;
#70456=ORIENTED_EDGE ( 'NONE', *, *, #31478, .F. ) ;
#70457=EDGE_LOOP ( 'NONE', ( #77097, #50835 ) ) ;
#70458=CARTESIAN_POINT ( 'NONE',  ( 13.25446817517716980, -3.285722584762969856, 32.44110544564090759 ) ) ;
#70459=CARTESIAN_POINT ( 'NONE',  ( 13.44987095589141113, -10.21337939537593620, 33.94971097300152252 ) ) ;
#70461=CARTESIAN_POINT ( 'NONE',  ( -2.242437168179467477, -11.67786785259547777, 32.92929555188713664 ) ) ;
#70462=CARTESIAN_POINT ( 'NONE',  ( 4.376625695114563008, -6.760870238392817200, 34.69528174975672385 ) ) ;
#70464=ORIENTED_EDGE ( 'NONE', *, *, #57939, .T. ) ;
#70466=ORIENTED_EDGE ( 'NONE', *, *, #6851, .F. ) ;
#70468=ORIENTED_EDGE ( 'NONE', *, *, #4957, .F. ) ;
#70469=DIRECTION ( 'NONE',  ( 0.000000000000000000, 0.3420201433256641055, -0.9396926207859100932 ) ) ;
#70470=CARTESIAN_POINT ( 'NONE',  ( -8.769230769230768274, -11.16473453929635440, 33.15142922261926373 ) ) ;
#70472=EDGE_LOOP ( 'NONE', ( #233, #1655 ) ) ;
#70473=B_SPLINE_CURVE_WITH_KNOTS ( 'NONE', 3,
 ( #45164, #83629, #16807, #72192, #751, #72638, #37518, #10049, #3287, #44709 ),
 .UNSPECIFIED., .F., .F.,
 ( 4, 2, 2, 2, 4 ),
 ( 0.000000000000000000, 0.0001954339857564093175, 0.0003908679715128186350, 0.0005863019572692279796, 0.0007817359430256372700 ),
 .UNSPECIFIED. ) ;
#70475=EDGE_LOOP ( 'NONE', ( #72774, #62344 ) ) ;
#70476=CARTESIAN_POINT ( 'NONE',  ( 12.46153846153846168, -2.538708090699994813, 30.37095296980875503 ) ) ;
#70477=ORIENTED_EDGE ( 'NONE', *, *, #43766, .T. ) ;
#70478=FACE_BOUND ( 'NONE', #21981, .T. ) ;
#70479=FACE_OUTER_BOUND ( 'NONE', #32895, .T. ) ;
#70480=DIRECTION ( 'NONE',  ( 0.000000000000000000, 0.9848077530122072432, -0.1736481776669354937 ) ) ;
#70481=VERTEX_POINT ( 'NONE', #82390 ) ;
#70482=LINE ( 'NONE', #49323, #76520 ) ;
#70483=FACE_OUTER_BOUND ( 'NONE', #2920, .T. ) ;
#70484=CARTESIAN_POINT ( 'NONE',  ( -1.384615384615383471, -5.415277668671390821, 36.20867863119892149 ) ) ;
#70485=CARTESIAN_POINT ( 'NONE',  ( -15.45425417449318317, -6.760086850603066466, 34.69517049084099369 ) ) ;
#70486=CARTESIAN_POINT ( 'NONE',  ( 4.153846153846032507, -3.300289026999228881, 32.46337939537708905 ) ) ;
#70487=LINE ( 'NONE', #72256, #74647 ) ;
#70488=CARTESIAN_POINT ( 'NONE',  ( 16.15384615384615330, -1.215029322943914858, 32.30358669280327177 ) ) ;
#70489=CARTESIAN_POINT ( 'NONE',  ( 16.21910172512217585, -9.442884908240273489, 34.35708131394835618 ) ) ;
#70490=DIRECTION ( 'NONE',  ( -0.000000000000000000, 0.9396926207859092051, -0.3420201433256662704 ) ) ;
#70491=LINE ( 'NONE', #75917, #80329 ) ;
#70492=CARTESIAN_POINT ( 'NONE',  ( 8.769230769230645706, -4.320704448113951379, 33.92786785259630022 ) ) ;
#70493=FACE_OUTER_BOUND ( 'NONE', #51266, .T. ) ;
#70494=CARTESIAN_POINT ( 'NONE',  ( 7.145856464345332171, -3.236590943229499029, 32.36255958852954251 ) ) ;
#70495=AXIS2_PLACEMENT_3D ( 'NONE', #20947, #14203, #8338 ) ;
#70496=CARTESIAN_POINT ( 'NONE',  ( 1.607626736228236153, -11.24521262558773671, 33.06293181088029343 ) ) ;
#70497=CARTESIAN_POINT ( 'NONE',  ( -11.31568199719312773, -11.41317474335729543, 32.86274602512330034 ) ) ;
#70498=CARTESIAN_POINT ( 'NONE',  ( 5.869308533332445066, -10.54014554554150607, 33.71984207302941883 ) ) ;
#70499=CARTESIAN_POINT ( 'NONE',  ( 12.46153846153846168, -12.78798330534103123, 29.99999999999997868 ) ) ;
#70501=ORIENTED_EDGE ( 'NONE', *, *, #52608, .T. ) ;
#70502=B_SPLINE_CURVE_WITH_KNOTS ( 'NONE', 3,
 ( #12673, #75692, #87923, #41474, #67621, #75264, #5917, #61728, #26186, #53654 ),
 .UNSPECIFIED., .F., .F.,
 ( 4, 2, 2, 2, 4 ),
 ( 0.0007817359527651098448, 0.0009771254036996487088, 0.001172514854634187573, 0.001367904305568726437, 0.001563293756503265301 ),
 .UNSPECIFIED. ) ;
#70503=CARTESIAN_POINT ( 'NONE',  ( -4.023320715612507925, -5.915461855592777596, 34.75538340440931506 ) ) ;
#70504=ORIENTED_EDGE ( 'NONE', *, *, #40121, .F. ) ;
#70505=AXIS2_PLACEMENT_3D ( 'NONE', #82710, #35394, #42169 ) ;
#70506=AXIS2_PLACEMENT_3D ( 'NONE', #79657, #37321, #23801 ) ;
#70507=CARTESIAN_POINT ( 'NONE',  ( -15.00775787915638304, -4.187068189119696804, 33.49521262558774026 ) ) ;
#70509=LINE ( 'NONE', #8814, #41213 ) ;
#70510=CARTESIAN_POINT ( 'NONE',  ( 14.17754433796061875, -2.373036134822904319, 30.88089517874952250 ) ) ;
#70512=CARTESIAN_POINT ( 'NONE',  ( -6.223484943723947893, -11.89387501736622710, 32.13663884655806413 ) ) ;
#70514=CARTESIAN_POINT ( 'NONE',  ( 6.130790440966952026, -6.369690395747422684, 34.87708834333098196 ) ) ;
#70515=AXIS2_PLACEMENT_3D ( 'NONE', #19241, #67424, #47140 ) ;
#70516=CARTESIAN_POINT ( 'NONE',  ( -7.846153846153967493, -4.320704448113951379, 33.92786785259630022 ) ) ;
#70517=CARTESIAN_POINT ( 'NONE',  ( -5.300408001487409315, -3.019605429927184836, 32.48692288466676814 ) ) ;
#70519=CARTESIAN_POINT ( 'NONE',  ( -16.28453675695646652, -9.929715669179216775, 34.40415004197138416 ) ) ;
#70520=DIRECTION ( 'NONE',  ( 0.000000000000000000, 0.9396926207859126468, -0.3420201433256571111 ) ) ;
#70521=DIRECTION ( 'NONE',  ( -0.000000000000000000, 0.9396926207859093161, -0.3420201433256663259 ) ) ;
#70524=CARTESIAN_POINT ( 'NONE',  ( -18.13014796973170206, -11.66186481527757124, 32.95055677023626117 ) ) ;
#70526=CARTESIAN_POINT ( 'NONE',  ( 13.63456090296352841, -4.336752205174649433, 33.62275283266504289 ) ) ;
#70528=EDGE_CURVE ( 'NONE', #53886, #81564, #83724, .T. ) ;
#70530=ORIENTED_EDGE ( 'NONE', *, *, #86178, .F. ) ;
#70531=CARTESIAN_POINT ( 'NONE',  ( 7.173076923076860290, -7.565270445406050648, 34.75000000000000000 ) ) ;
#70532=CYLINDRICAL_SURFACE ( 'NONE', #40242, 0.2500000000000008882 ) ;
#70533=CYLINDRICAL_SURFACE ( 'NONE', #8094, 0.2499999999999998890 ) ;
#70534=CARTESIAN_POINT ( 'NONE',  ( 1.514660547450164874, -2.504778602574659896, 29.97347330155780298 ) ) ;
#70535=CARTESIAN_POINT ( 'NONE',  ( -3.007757879156381708, -4.887748414852789658, 34.01359900205216746 ) ) ;
#70536=CARTESIAN_POINT ( 'NONE',  ( -9.692307692307814193, -12.16647553114689728, 32.15551576947799362 ) ) ;
#70537=CARTESIAN_POINT ( 'NONE',  ( 8.638539302563215116, -10.54014554554150607, 33.71984207302941883 ) ) ;
#70538=B_SPLINE_CURVE_WITH_KNOTS ( 'NONE', 3,
 ( #20054, #39457, #68245, #5209, #5652, #19608, #74560, #87646, #47515, #47070 ),
 .UNSPECIFIED., .F., .F.,
 ( 4, 2, 2, 2, 4 ),
 ( 0.000000000000000000, 0.0001954339857564071491, 0.0003908679715128142982, 0.0005863019572692214744, 0.0007817359430256285964 ),
 .UNSPECIFIED. ) ;
#70539=EDGE_CURVE ( 'NONE', #85237, #327, #4160, .T. ) ;
#70540=ORIENTED_EDGE ( 'NONE', *, *, #2061, .F. ) ;
#70542=AXIS2_PLACEMENT_3D ( 'NONE', #18906, #19349, #59886 ) ;
#70543=ORIENTED_EDGE ( 'NONE', *, *, #76773, .T. ) ;
#70544=CARTESIAN_POINT ( 'NONE',  ( -5.076923076923075762, -5.471508081941601098, 34.59228464037088457 ) ) ;
#70545=CARTESIAN_POINT ( 'NONE',  ( 6.792929713638705458, -2.882441371585227063, 31.66841991370171527 ) ) ;
#70546=CARTESIAN_POINT ( 'NONE',  ( -15.29603923132555288, -11.06231777344662781, 33.60647404775220082 ) ) ;
#70547=CARTESIAN_POINT ( 'NONE',  ( -6.065270445960775803, -3.300289026998414865, 32.46337939537583139 ) ) ;
#70548=CARTESIAN_POINT ( 'NONE',  ( -39.05038313613820122, -2.499999999999999556, 29.75000000000000355 ) ) ;
#70549=ORIENTED_EDGE ( 'NONE', *, *, #55422, .F. ) ;
#70550=CARTESIAN_POINT ( 'NONE',  ( 13.38461538461538680, -8.164416787775445883, 34.95778746994557906 ) ) ;
#70551=ORIENTED_EDGE ( 'NONE', *, *, #42171, .T. ) ;
#70552=EDGE_CURVE ( 'NONE', #55385, #88074, #17080, .T. ) ;
#70553=ORIENTED_EDGE ( 'NONE', *, *, #47230, .F. ) ;
#70554=AXIS2_PLACEMENT_3D ( 'NONE', #57299, #73369, #17987 ) ;
#70555=CARTESIAN_POINT ( 'NONE',  ( 8.545745844666434721, -12.47654668319379567, 31.42292124445336654 ) ) ;
#70556=ORIENTED_EDGE ( 'NONE', *, *, #71119, .T. ) ;
#70557=DIRECTION ( 'NONE',  ( 0.000000000000000000, 0.1736481776669267785, -0.9848077530122087975 ) ) ;
#70559=CYLINDRICAL_SURFACE ( 'NONE', #58065, 0.2500000000000002220 ) ;
#70561=VECTOR ( 'NONE', #62163, 1000.000000000000000 ) ;
#70562=EDGE_CURVE ( 'NONE', #49738, #67178, #9589, .T. ) ;
#70563=CARTESIAN_POINT ( 'NONE',  ( 4.087762742890272527, -4.098570777380720287, 33.41473453929634729 ) ) ;
#70564=CARTESIAN_POINT ( 'NONE',  ( -16.08777882049607655, -5.471508081941601098, 34.59228464037088457 ) ) ;
#70565=EDGE_LOOP ( 'NONE', ( #2190, #342 ) ) ;
#70567=AXIS2_PLACEMENT_3D ( 'NONE', #2450, #58284, #64147 ) ;
#70568=B_SPLINE_CURVE_WITH_KNOTS ( 'NONE', 3,
 ( #65560, #31345, #68241, #55158, #88976, #83088, #14624, #61911, #76317, #27249 ),
 .UNSPECIFIED., .F., .F.,
 ( 4, 2, 2, 2, 4 ),
 ( 0.0007817246256747481482, 0.0009771112852218911526, 0.001172497944769034049, 0.001367884604316176944, 0.001563271263863319840 ),
 .UNSPECIFIED. ) ;
#70570=LINE ( 'NONE', #62465, #54736 ) ;
#70572=ORIENTED_EDGE ( 'NONE', *, *, #25531, .F. ) ;
#70573=FACE_OUTER_BOUND ( 'NONE', #43015, .T. ) ;
#70574=CARTESIAN_POINT ( 'NONE',  ( 4.826946345980720032, -3.627789207965226748, 32.91389620160131102 ) ) ;
#70575=LINE ( 'NONE', #9753, #49381 ) ;
#70576=ORIENTED_EDGE ( 'NONE', *, *, #9686, .F. ) ;
#70578=CARTESIAN_POINT ( 'NONE',  ( 15.00784227186237985, -2.523278758544489797, 31.42238647778637528 ) ) ;
#70579=ORIENTED_EDGE ( 'NONE', *, *, #36721, .T. ) ;
#70580=FACE_BOUND ( 'NONE', #74909, .T. ) ;
#70581=CARTESIAN_POINT ( 'NONE',  ( -10.86540783960607115, -4.931416488878822335, 34.32920672191015399 ) ) ;
#70582=CARTESIAN_POINT ( 'NONE',  ( 17.86985203026830149, -12.70455904226513866, 30.44083106164009322 ) ) ;
#70583=CARTESIAN_POINT ( 'NONE',  ( 2.242422307135989445, -12.51329471203370325, 31.30864560766548976 ) ) ;
#70585=CARTESIAN_POINT ( 'NONE',  ( -10.74607521849492464, -5.496505350115501010, 34.60290016733514307 ) ) ;
#70586=CARTESIAN_POINT ( 'NONE',  ( 8.769230769230768274, -5.557115091759785130, 34.35708131394839171 ) ) ;
#70587=CARTESIAN_POINT ( 'NONE',  ( -16.08859058257012720, -9.442884908240273489, 34.35708131394835618 ) ) ;
#70588=EDGE_LOOP ( 'NONE', ( #86515, #49831 ) ) ;
#70590=CARTESIAN_POINT ( 'NONE',  ( 4.826946332874483936, -4.075325502946086864, 33.72974371597207721 ) ) ;
#70591=VERTEX_POINT ( 'NONE', #50782 ) ;
#70592=CARTESIAN_POINT ( 'NONE',  ( -12.46153846153846168, -3.322132147404559976, 32.92929555188717927 ) ) ;
#70593=CARTESIAN_POINT ( 'NONE',  ( 14.30769230769231015, -9.780366693483667717, 34.19971097300155094 ) ) ;
#70594=CARTESIAN_POINT ( 'NONE',  ( -16.08859058257012720, -10.90142922261932057, 33.41473453929631887 ) ) ;
#70595=CARTESIAN_POINT ( 'NONE',  ( -17.07692307692307665, -10.67929555188718282, 33.92786785259544047 ) ) ;
#70596=ADVANCED_FACE ( 'NONE', ( #36843 ), #9816, .F. ) ;
#70598=CARTESIAN_POINT ( 'NONE',  ( 2.557637717070351702, -4.932303261841488151, 34.32971442181322885 ) ) ;
#70599=FACE_BOUND ( 'NONE', #14639, .T. ) ;
#70600=FACE_OUTER_BOUND ( 'NONE', #61681, .T. ) ;
#70601=CARTESIAN_POINT ( 'NONE',  ( 15.23076923076923173, -2.499999999999998668, 29.75000000000001421 ) ) ;
#70603=FACE_OUTER_BOUND ( 'NONE', #24344, .T. ) ;
#70604=CARTESIAN_POINT ( 'NONE',  ( -6.923076923077044142, -5.219633306517616589, 34.19971097300220464 ) ) ;
#70605=AXIS2_PLACEMENT_3D ( 'NONE', #71953, #78717, #1282 ) ;
#70606=CARTESIAN_POINT ( 'NONE',  ( 1.134615384615366374, -2.249999999999999112, 29.81609741502488120 ) ) ;
#70609=ORIENTED_EDGE ( 'NONE', *, *, #80583, .T. ) ;
#70610=DIRECTION ( 'NONE',  ( -0.000000000000000000, -0.9848077530122085754, -0.1736481776669273613 ) ) ;
#70611=CARTESIAN_POINT ( 'NONE',  ( -4.283993363284373856, -3.285722584762969856, 32.44110544564090759 ) ) ;
#70612=CARTESIAN_POINT ( 'NONE',  ( -7.596099426240391139, -11.47946981652013498, 33.17500667209846910 ) ) ;
#70613=CARTESIAN_POINT ( 'NONE',  ( -0.4615384615384611200, -2.833524468853757305, 32.15551576947925838 ) ) ;
#70614=CARTESIAN_POINT ( 'NONE',  ( 12.46153846153846168, -2.499999999999998668, 29.75000000000001421 ) ) ;
#70616=EDGE_CURVE ( 'NONE', #52843, #74684, #25709, .T. ) ;
#70617=CARTESIAN_POINT ( 'NONE',  ( -11.76134105519912154, -7.630690623152299956, 34.99857592706774057 ) ) ;
#70618=CARTESIAN_POINT ( 'NONE',  ( 18.00000000000000000, -3.050289026998446396, 32.03036669348365706 ) ) ;
#70619=CARTESIAN_POINT ( 'NONE',  ( -17.20761454359063691, -4.809359713505814149, 33.96456829005828837 ) ) ;
#70620=CARTESIAN_POINT ( 'NONE',  ( -1.514762594053604028, -12.45813303252208648, 30.39737893381572675 ) ) ;
#70621=DIRECTION ( 'NONE',  ( -0.000000000000000000, -0.8660254037844397068, -0.4999999999999978906 ) ) ;
#70622=DIRECTION ( 'NONE',  ( -0.000000000000000000, 0.7660444431189791237, -0.6427876096865379196 ) ) ;
#70623=B_SPLINE_CURVE_WITH_KNOTS ( 'NONE', 3,
 ( #59443, #80166, #26105, #67096, #4952, #32863, #60324, #87838, #33749, #20239 ),
 .UNSPECIFIED., .F., .F.,
 ( 4, 2, 2, 2, 4 ),
 ( 0.0007817246256747460882, 0.0009771112852218892010, 0.001172497944769032314, 0.001367884604316175210, 0.001563271263863318323 ),
 .UNSPECIFIED. ) ;
#70624=CARTESIAN_POINT ( 'NONE',  ( 12.46153846153846168, -2.292212530054420494, 30.41441678777542634 ) ) ;
#70625=AXIS2_PLACEMENT_3D ( 'NONE', #2343, #80128, #79685 ) ;
#70628=CARTESIAN_POINT ( 'NONE',  ( 2.057715563643716550, -3.436278759898155233, 33.07459398097509506 ) ) ;
#70629=CARTESIAN_POINT ( 'NONE',  ( 10.83839745947801170, -5.582272713120729257, 34.63742843783360570 ) ) ;
#70632=VECTOR ( 'NONE', #41143, 1000.000000000000000 ) ;
#70633=EDGE_CURVE ( 'NONE', #27791, #2893, #58431, .T. ) ;
#70634=DIRECTION ( 'NONE',  ( 0.000000000000000000, 0.6427876096865373645, -0.7660444431189797898 ) ) ;
#70635=CARTESIAN_POINT ( 'NONE',  ( 3.230769230769231726, -13.88283147151868846, 33.14645433367849847 ) ) ;
#70636=EDGE_LOOP ( 'NONE', ( #65866, #43344, #38440, #10139 ) ) ;
#70637=CARTESIAN_POINT ( 'NONE',  ( -7.173053667125516064, -2.920706130388546651, 32.31842814019191223 ) ) ;
#70638=CARTESIAN_POINT ( 'NONE',  ( 3.930919936330004472, -5.667676309546437530, 34.40238873228292249 ) ) ;
#70639=ORIENTED_EDGE ( 'NONE', *, *, #18969, .F. ) ;
#70640=CARTESIAN_POINT ( 'NONE',  ( -5.999999999999998224, -3.322132147404559976, 32.92929555188717927 ) ) ;
#70641=CARTESIAN_POINT ( 'NONE',  ( 16.82689985270161870, -2.588893531581426100, 31.60682220781849239 ) ) ;
#70642=EDGE_CURVE ( 'NONE', #15672, #49031, #64290, .T. ) ;
#70643=EDGE_LOOP ( 'NONE', ( #30526, #55790 ) ) ;
#70644=CARTESIAN_POINT ( 'NONE',  ( -13.31935981333935537, -2.625532179533470512, 30.86335684631491105 ) ) ;
#70645=VECTOR ( 'NONE', #64273, 1000.000000000000000 ) ;
#70646=CARTESIAN_POINT ( 'NONE',  ( 7.846153846153846700, -13.53365097954675988, 30.81389545987213552 ) ) ;
#70647=EDGE_LOOP ( 'NONE', ( #5430, #18986, #32795, #83594 ) ) ;
#70648=CARTESIAN_POINT ( 'NONE',  ( -11.60373198442231413, -4.481592998940162609, 33.73612834413957984 ) ) ;
#70651=EDGE_CURVE ( 'NONE', #48397, #41602, #85047, .T. ) ;
#70652=ORIENTED_EDGE ( 'NONE', *, *, #3514, .T. ) ;
#70653=VERTEX_POINT ( 'NONE', #16571 ) ;
#70654=VERTEX_POINT ( 'NONE', #71508 ) ;
#70655=ADVANCED_FACE ( 'NONE', ( #3049 ), #15257, .F. ) ;
#70656=CARTESIAN_POINT ( 'NONE',  ( -7.146561847641254239, -2.353723527008295680, 30.78948104536958752 ) ) ;
#70657=CARTESIAN_POINT ( 'NONE',  ( -15.29603923132555110, -2.379036618887870436, 30.90682066428147934 ) ) ;
#70658=EDGE_CURVE ( 'NONE', #10983, #67914, #64746, .T. ) ;
#70659=CARTESIAN_POINT ( 'NONE',  ( -3.230769230769352962, -8.656820664282941280, 34.87096338111179961 ) ) ;
#70660=CYLINDRICAL_SURFACE ( 'NONE', #8973, 0.2500000000000009437 ) ;
#70662=ORIENTED_EDGE ( 'NONE', *, *, #32935, .F. ) ;
#70663=ORIENTED_EDGE ( 'NONE', *, *, #86954, .F. ) ;
#70664=CARTESIAN_POINT ( 'NONE',  ( 17.07692307692295586, -5.219633306517616589, 34.19971097300220464 ) ) ;
#70665=ORIENTED_EDGE ( 'NONE', *, *, #68904, .T. ) ;
#70666=AXIS2_PLACEMENT_3D ( 'NONE', #20446, #55996, #47908 ) ;
#70667=B_SPLINE_CURVE_WITH_KNOTS ( 'NONE', 3,
 ( #38475, #37569, #87124, #73144, #66384, #87570, #38027, #30815, #79462, #11897 ),
 .UNSPECIFIED., .F., .F.,
 ( 4, 2, 2, 2, 4 ),
 ( 0.0007817359430256333669, 0.0009771253907250056474, 0.001172514838424370881, 0.001367904286123736331, 0.001563293733823101564 ),
 .UNSPECIFIED. ) ;
#70668=CYLINDRICAL_SURFACE ( 'NONE', #7871, 0.2500000000000009437 ) ;
#70669=ORIENTED_EDGE ( 'NONE', *, *, #59980, .F. ) ;
#70670=EDGE_CURVE ( 'NONE', #3335, #88199, #50347, .T. ) ;
#70672=CARTESIAN_POINT ( 'NONE',  ( 15.29596221906388287, -2.255955759149235629, 29.99999999999988987 ) ) ;
#70673=CARTESIAN_POINT ( 'NONE',  ( 7.846153846153725020, -5.219633306517616589, 34.19971097300220464 ) ) ;
#70674=ORIENTED_EDGE ( 'NONE', *, *, #18391, .T. ) ;
#70675=VERTEX_POINT ( 'NONE', #44471 ) ;
#70676=B_SPLINE_CURVE_WITH_KNOTS ( 'NONE', 3,
 ( #23826, #51281, #79241, #38251, #31496, #58959, #86463, #79688, #45443, #72922 ),
 .UNSPECIFIED., .F., .F.,
 ( 4, 2, 2, 2, 4 ),
 ( 0.0007817359430256315238, 0.0009771253907249976244, 0.001172514838424363508, 0.001367904286123729392, 0.001563293733823095492 ),
 .UNSPECIFIED. ) ;
#70677=CARTESIAN_POINT ( 'NONE',  ( 9.942307692309114486, -7.500000000000154543, 35.00000000000007105 ) ) ;
#70678=VERTEX_POINT ( 'NONE', #29223 ) ;
#70679=B_SPLINE_CURVE_WITH_KNOTS ( 'NONE', 3,
 ( #48374, #34861, #6075, #88955, #33096, #20902, #28110, #199, #27224, #41190 ),
 .UNSPECIFIED., .F., .F.,
 ( 4, 2, 2, 2, 4 ),
 ( 0.0007817246256747446788, 0.0009771112852218879000, 0.001172497944769031013, 0.001367884604316174126, 0.001563271263863317238 ),
 .UNSPECIFIED. ) ;
#70680=CARTESIAN_POINT ( 'NONE',  ( 4.153846153846032507, -5.219633306517616589, 34.19971097300220464 ) ) ;
#70681=CYLINDRICAL_SURFACE ( 'NONE', #19476, 0.2499999999999986955 ) ;
#70682=ORIENTED_EDGE ( 'NONE', *, *, #49330, .F. ) ;
#70683=CARTESIAN_POINT ( 'NONE',  ( 15.00728430620490172, -2.353723527008296568, 30.78948104536958752 ) ) ;
#70684=CARTESIAN_POINT ( 'NONE',  ( 15.23076923076911093, -9.442884908241554243, 34.35708131394783038 ) ) ;
#70685=CARTESIAN_POINT ( 'NONE',  ( 8.769230769230768274, -12.48256725967547354, 35.29906147534542527 ) ) ;
#70686=FACE_BOUND ( 'NONE', #7960, .T. ) ;
#70687=CARTESIAN_POINT ( 'NONE',  ( -8.638705330997126453, -2.372941743896879174, 30.88044141588253666 ) ) ;
#70689=VECTOR ( 'NONE', #19964, 1000.000000000000000 ) ;
#70690=CARTESIAN_POINT ( 'NONE',  ( 8.769230769230768274, -2.538708090699994813, 30.37095296980875503 ) ) ;
#70691=CARTESIAN_POINT ( 'NONE',  ( -9.692307692307691624, -12.34228464037088635, 31.77849191805839268 ) ) ;
#70692=CARTESIAN_POINT ( 'NONE',  ( -16.15384615384627409, -3.083524468854526912, 32.58852847137268327 ) ) ;
#70693=CARTESIAN_POINT ( 'NONE',  ( -5.010855743573002563, -3.937682226553329556, 33.60647404775216529 ) ) ;
#70694=FACE_OUTER_BOUND ( 'NONE', #5213, .T. ) ;
#70696=FACE_OUTER_BOUND ( 'NONE', #78858, .T. ) ;
#70697=EDGE_LOOP ( 'NONE', ( #45376, #4590 ) ) ;
#70698=EDGE_LOOP ( 'NONE', ( #88148, #10712, #41098, #55734 ) ) ;
#70699=VECTOR ( 'NONE', #64608, 1000.000000000000114 ) ;
#70700=CARTESIAN_POINT ( 'NONE',  ( 1.384615384615386802, -11.16473453929635440, 33.15142922261926373 ) ) ;
#70701=CARTESIAN_POINT ( 'NONE',  ( 16.15384615384603251, -12.27809138561165270, 31.22303859784587132 ) ) ;
#70702=CARTESIAN_POINT ( 'NONE',  ( 11.28843831424008926, -8.475808217655753651, 34.90892951860618609 ) ) ;
#70703=CYLINDRICAL_SURFACE ( 'NONE', #75349, 0.2500000000000008882 ) ;
#70704=CARTESIAN_POINT ( 'NONE',  ( -10.48459417441766561, -12.35292014791297710, 31.75344720912887198 ) ) ;
#70705=CARTESIAN_POINT ( 'NONE',  ( -4.023055712879200385, -3.338503747796866872, 32.95102852606553512 ) ) ;
#70706=VERTEX_POINT ( 'NONE', #84170 ) ;
#70707=EDGE_CURVE ( 'NONE', #25698, #55151, #80429, .T. ) ;
#70708=CARTESIAN_POINT ( 'NONE',  ( -18.06527044596078113, -6.026961402152683611, 34.52809138561120506 ) ) ;
#70709=B_SPLINE_CURVE_WITH_KNOTS ( 'NONE', 3,
 ( #39777, #87988, #73563, #12290, #64219, #74001, #18612, #84959, #51135, #60473 ),
 .UNSPECIFIED., .F., .F.,
 ( 4, 2, 2, 2, 4 ),
 ( 0.0007817359430256282712, 0.0009771253907249941549, 0.001172514838424359822, 0.001367904286123725489, 0.001563293733823091372 ),
 .UNSPECIFIED. ) ;
#70710=CARTESIAN_POINT ( 'NONE',  ( 3.296024802045255164, -11.48612834413965977, 32.76840700105972815 ) ) ;
#70711=CARTESIAN_POINT ( 'NONE',  ( 17.07692307692295586, -6.879047030192662504, 34.71129190930017927 ) ) ;
#70712=CARTESIAN_POINT ( 'NONE',  ( -8.546451100252703270, -2.612705202774698421, 31.66806509827799943 ) ) ;
#70713=LINE ( 'NONE', #9888, #16106 ) ;
#70714=EDGE_CURVE ( 'NONE', #53248, #60559, #66554, .T. ) ;
#70715=EDGE_CURVE ( 'NONE', #4425, #59481, #76101, .T. ) ;
#70717=ORIENTED_EDGE ( 'NONE', *, *, #18455, .T. ) ;
#70718=ORIENTED_EDGE ( 'NONE', *, *, #77908, .F. ) ;
#70719=EDGE_CURVE ( 'NONE', #78911, #88008, #32090, .T. ) ;
#70720=CARTESIAN_POINT ( 'NONE',  ( -7.715628407920203102, -12.15418822224088657, 32.17964115625579069 ) ) ;
#70722=CARTESIAN_POINT ( 'NONE',  ( 10.61538461538461675, -9.819645486525091727, 36.12317359536749706 ) ) ;
#70723=DIRECTION ( 'NONE',  ( -0.000000000000000000, 1.000000000000000000, -0.000000000000000000 ) ) ;
#70725=CARTESIAN_POINT ( 'NONE',  ( -0.4615384615384611200, -11.91647553114624181, 32.58852847137148245 ) ) ;
#70727=EDGE_CURVE ( 'NONE', #62488, #62470, #39598, .T. ) ;
#70728=CARTESIAN_POINT ( 'NONE',  ( 14.30769230769231015, -6.343179335718451384, 34.87096338111211935 ) ) ;
#70730=CARTESIAN_POINT ( 'NONE',  ( -12.68446467905460473, -10.61292498521070549, 33.66303323003028680 ) ) ;
#70731=DIRECTION ( 'NONE',  ( -0.000000000000000000, 1.000000000000000000, 3.491481338843133355E-15 ) ) ;
#70732=ORIENTED_EDGE ( 'NONE', *, *, #45014, .T. ) ;
#70733=CARTESIAN_POINT ( 'NONE',  ( -13.60810032833933292, -11.41268669641500466, 32.86336882939237825 ) ) ;
#70734=DIRECTION ( 'NONE',  ( -0.000000000000000000, -0.000000000000000000, -1.000000000000000000 ) ) ;
#70735=AXIS2_PLACEMENT_3D ( 'NONE', #18190, #24484, #57834 ) ;
#70736=CARTESIAN_POINT ( 'NONE',  ( -3.230769230769229949, -4.786620604624113540, 33.94971097300155094 ) ) ;
#70737=CARTESIAN_POINT ( 'NONE',  ( 6.673053698855467175, -3.520140089381497361, 33.17453946501458262 ) ) ;
#70738=CARTESIAN_POINT ( 'NONE',  ( -3.453597328404108602, -7.369209533119137845, 34.99857337881830688 ) ) ;
#70739=CARTESIAN_POINT ( 'NONE',  ( 15.48071474911737511, -11.37275283266504111, 32.91324779482534524 ) ) ;
#70740=VECTOR ( 'NONE', #79, 1000.000000000000000 ) ;
#70742=ORIENTED_EDGE ( 'NONE', *, *, #73136, .F. ) ;
#70743=CARTESIAN_POINT ( 'NONE',  ( -3.100243792535585907, -6.808710257144159783, 34.95449254468098843 ) ) ;
#70744=CARTESIAN_POINT ( 'NONE',  ( 4.403900573759606196, -10.82426656108011720, 33.81400080652039009 ) ) ;
#70746=CARTESIAN_POINT ( 'NONE',  ( 0.3954560821783252300, -5.471508081941601986, 34.59228464037088457 ) ) ;
#70747=CARTESIAN_POINT ( 'NONE',  ( -16.15384615384615330, -13.78497067705608181, 32.30358669280327177 ) ) ;
#70748=ORIENTED_EDGE ( 'NONE', *, *, #81885, .F. ) ;
#70750=CARTESIAN_POINT ( 'NONE',  ( -3.360916440207450062, -10.88202310037936194, 33.43294751532457099 ) ) ;
#70751=EDGE_CURVE ( 'NONE', #22972, #35664, #982, .T. ) ;
#70752=B_SPLINE_CURVE_WITH_KNOTS ( 'NONE', 3,
 ( #70680, #8983, #36880, #36452, #63903, #2204, #57157, #84647, #22926, #67478 ),
 .UNSPECIFIED., .F., .F.,
 ( 4, 2, 2, 2, 4 ),
 ( 0.0007817359430256280543, 0.0009771253907249941549, 0.001172514838424360472, 0.001367904286123726790, 0.001563293733823092890 ),
 .UNSPECIFIED. ) ;
#70753=ORIENTED_EDGE ( 'NONE', *, *, #4682, .F. ) ;
#70754=CARTESIAN_POINT ( 'NONE',  ( -0.7115616857599195155, -10.92453946501458439, 33.72985991061850086 ) ) ;
#70756=CARTESIAN_POINT ( 'NONE',  ( 17.93391658904412012, -6.386643153685125363, 34.62446782046654903 ) ) ;
#70757=CARTESIAN_POINT ( 'NONE',  ( 10.61538461538493117, -2.255955759149395501, 30.00000000000324363 ) ) ;
#70758=CARTESIAN_POINT ( 'NONE',  ( 7.911409417429871027, -6.026961402152789304, 34.52809138561124769 ) ) ;
#70759=CARTESIAN_POINT ( 'NONE',  ( 17.07692307692307665, -13.20930481340135110, 34.54067556320372745 ) ) ;
#70760=VERTEX_POINT ( 'NONE', #80055 ) ;
#70761=CARTESIAN_POINT ( 'NONE',  ( -2.980823821391186623, -2.341251567377310217, 30.72681386836322659 ) ) ;
#70763=ORIENTED_EDGE ( 'NONE', *, *, #79878, .T. ) ;
#70764=CIRCLE ( 'NONE', #17725, 0.2500000000000002220 ) ;
#70765=CARTESIAN_POINT ( 'NONE',  ( 12.46153846153846168, -11.91647553114624181, 32.58852847137148245 ) ) ;
#70766=CARTESIAN_POINT ( 'NONE',  ( 0.7114838709165044461, -10.18230066228895758, 34.26354781536631577 ) ) ;
#70767=ORIENTED_EDGE ( 'NONE', *, *, #12299, .F. ) ;
#70768=CARTESIAN_POINT ( 'NONE',  ( -16.15384615384615330, -13.63283147151868846, 33.57946703557072254 ) ) ;
#70769=FACE_OUTER_BOUND ( 'NONE', #84735, .T. ) ;
#70770=CARTESIAN_POINT ( 'NONE',  ( -11.60373198442231413, -2.892918686051582977, 31.69288490824015980 ) ) ;
#70772=CARTESIAN_POINT ( 'NONE',  ( 1.134592160393929294, -6.652501968072646932, 34.93155406624980941 ) ) ;
#70773=CARTESIAN_POINT ( 'NONE',  ( -3.903791733932699515, -4.074993327901525575, 33.72946981652012255 ) ) ;
#70776=EDGE_LOOP ( 'NONE', ( #46308, #11288 ) ) ;
#70777=VERTEX_POINT ( 'NONE', #45819 ) ;
#70778=FACE_BOUND ( 'NONE', #74456, .T. ) ;
#70779=ORIENTED_EDGE ( 'NONE', *, *, #15284, .F. ) ;
#70780=CARTESIAN_POINT ( 'NONE',  ( -8.769230769230768274, -4.098570777380720287, 33.41473453929634729 ) ) ;
#70781=B_SPLINE_CURVE_WITH_KNOTS ( 'NONE', 3,
 ( #47655, #75139, #37227, #57947, #50289, #64694, #2119, #17414, #16083, #2995 ),
 .UNSPECIFIED., .F., .F.,
 ( 4, 2, 2, 2, 4 ),
 ( 0.000000000000000000, 0.0001954339857564080165, 0.0003908679715128160329, 0.0005863019572692240765, 0.0007817359430256320659 ),
 .UNSPECIFIED. ) ;
#70782=EDGE_CURVE ( 'NONE', #6671, #33723, #53618, .T. ) ;
#70783=B_SPLINE_CURVE_WITH_KNOTS ( 'NONE', 3,
 ( #11586, #80945, #61092, #19232, #80494, #74172, #12908, #4830, #88601, #26872 ),
 .UNSPECIFIED., .F., .F.,
 ( 4, 2, 2, 2, 4 ),
 ( 0.0007817246256747446788, 0.0009771112852218879000, 0.001172497944769031013, 0.001367884604316174126, 0.001563271263863317238 ),
 .UNSPECIFIED. ) ;
#70784=CARTESIAN_POINT ( 'NONE',  ( -7.846153846153967493, -6.835583212225970762, 34.95778746994575670 ) ) ;
#70785=EDGE_CURVE ( 'NONE', #59805, #1987, #3034, .T. ) ;
#70786=CARTESIAN_POINT ( 'NONE',  ( 5.999999999999878320, -3.083524468854526912, 32.58852847137268327 ) ) ;
#70787=DIRECTION ( 'NONE',  ( -0.000000000000000000, 0.5000000000000011102, -0.8660254037844381525 ) ) ;
#70788=ORIENTED_EDGE ( 'NONE', *, *, #86411, .F. ) ;
#70789=VERTEX_POINT ( 'NONE', #47598 ) ;
#70790=EDGE_CURVE ( 'NONE', #7689, #62944, #75960, .T. ) ;
#70791=CARTESIAN_POINT ( 'NONE',  ( 16.94623161025551639, -4.118384482072086072, 33.43331474514187107 ) ) ;
#70792=ORIENTED_EDGE ( 'NONE', *, *, #47863, .F. ) ;
#70793=VECTOR ( 'NONE', #48218, 1000.000000000000114 ) ;
#70795=CARTESIAN_POINT ( 'NONE',  ( 13.13463865367303640, -2.779195860258146578, 31.39871582349836032 ) ) ;
#70797=EDGE_CURVE ( 'NONE', #22972, #79057, #41296, .T. ) ;
#70798=DIRECTION ( 'NONE',  ( 0.000000000000000000, 0.6427876096865368094, 0.7660444431189802339 ) ) ;
#70799=DIRECTION ( 'NONE',  ( -0.000000000000000000, 1.000000000000000000, 3.491481338843133355E-15 ) ) ;
#70800=ORIENTED_EDGE ( 'NONE', *, *, #58811, .T. ) ;
#70801=CARTESIAN_POINT ( 'NONE',  ( 16.40379156322419973, -2.341251567377310217, 30.72681386836322659 ) ) ;
#70802=CARTESIAN_POINT ( 'NONE',  ( -15.23076923076922995, -3.322132147404559976, 32.92929555188717927 ) ) ;
#70804=CARTESIAN_POINT ( 'NONE',  ( -17.87165453593004827, -7.725172855618575696, 34.99539338292708379 ) ) ;
#70805=CARTESIAN_POINT ( 'NONE',  ( -1.134560964701931018, -2.920487667080174710, 32.31805714834170828 ) ) ;
#70808=ORIENTED_EDGE ( 'NONE', *, *, #24501, .F. ) ;
#70809=ORIENTED_EDGE ( 'NONE', *, *, #9949, .F. ) ;
#70810=CYLINDRICAL_SURFACE ( 'NONE', #61934, 0.2499999999999979738 ) ;
#70811=CARTESIAN_POINT ( 'NONE',  ( 2.307692307692187583, -2.625532179533779154, 30.86335684631627174 ) ) ;
#70812=CARTESIAN_POINT ( 'NONE',  ( 15.93091993633000136, -5.667676309546437530, 34.40238873228292249 ) ) ;
#70813=CARTESIAN_POINT ( 'NONE',  ( 12.52760579488853665, -12.62096338111211757, 30.90682066428152908 ) ) ;
#70814=CARTESIAN_POINT ( 'NONE',  ( -7.846153846153844924, -1.629998284177014645, 34.34916445242399163 ) ) ;
#70815=CARTESIAN_POINT ( 'NONE',  ( -2.437839517130528044, -10.19110544564092002, 33.96427741523702792 ) ) ;
#70816=ORIENTED_EDGE ( 'NONE', *, *, #68408, .F. ) ;
#70817=EDGE_CURVE ( 'NONE', #86112, #81662, #27768, .T. ) ;
#70818=CARTESIAN_POINT ( 'NONE',  ( 17.07692307692307665, -11.91647553114624181, 32.58852847137148245 ) ) ;
#70819=CARTESIAN_POINT ( 'NONE',  ( 9.561617089197390840, -11.93127051446799847, 32.56575433478202797 ) ) ;
#70820=CARTESIAN_POINT ( 'NONE',  ( 11.28846153846153832, -7.433931650972300353, 34.75000000000000711 ) ) ;
#70821=CARTESIAN_POINT ( 'NONE',  ( -11.28840722682322628, -3.627508038966690496, 32.91356715214248396 ) ) ;
#70822=EDGE_LOOP ( 'NONE', ( #15209, #21389 ) ) ;
#70823=CARTESIAN_POINT ( 'NONE',  ( 2.438218009455874302, -11.93748526763465279, 32.05452791011430946 ) ) ;
#70824=EDGE_CURVE ( 'NONE', #4668, #75533, #55238, .T. ) ;
#70825=VERTEX_POINT ( 'NONE', #54793 ) ;
#70826=FACE_BOUND ( 'NONE', #58432, .T. ) ;
#70827=CARTESIAN_POINT ( 'NONE',  ( 4.826946345980721809, -5.728515186090277211, 34.42611988154120439 ) ) ;
#70829=AXIS2_PLACEMENT_3D ( 'NONE', #74777, #13063, #19374 ) ;
#70830=CYLINDRICAL_SURFACE ( 'NONE', #73693, 0.2500000000000004996 ) ;
#70832=VERTEX_POINT ( 'NONE', #6176 ) ;
#70833=CARTESIAN_POINT ( 'NONE',  ( -12.59222992820602371, -9.804603061927743113, 34.18744698557895845 ) ) ;
#70834=CARTESIAN_POINT ( 'NONE',  ( 4.946446368806611815, -7.276988635370452485, 34.74523720219453793 ) ) ;
#70835=CARTESIAN_POINT ( 'NONE',  ( -9.942330929600657896, -3.202444869320336451, 32.30641848906366675 ) ) ;
#70836=CARTESIAN_POINT ( 'NONE',  ( -7.146561866800870355, -10.81261337010820256, 33.49550067578627477 ) ) ;
#70837=ORIENTED_EDGE ( 'NONE', *, *, #28675, .T. ) ;
#70838=VECTOR ( 'NONE', #60224, 1000.000000000000227 ) ;
#70840=CARTESIAN_POINT ( 'NONE',  ( -9.915792616872025178, -3.019605429927184836, 32.48692288466676814 ) ) ;
#70841=ORIENTED_EDGE ( 'NONE', *, *, #15165, .F. ) ;
#70843=ORIENTED_EDGE ( 'NONE', *, *, #51791, .T. ) ;
#70844=CARTESIAN_POINT ( 'NONE',  ( 7.846153846153725020, -10.90142922262034020, 33.41473453929536674 ) ) ;
#70845=CARTESIAN_POINT ( 'NONE',  ( -6.923076923076922462, -11.69971097300155272, 32.46337939537588113 ) ) ;
#70846=DIRECTION ( 'NONE',  ( -0.000000000000000000, 0.5000000000000011102, -0.8660254037844381525 ) ) ;
#70847=CARTESIAN_POINT ( 'NONE',  ( 12.68454981315131214, -4.187068189119697692, 33.49521262558774026 ) ) ;
#70849=CARTESIAN_POINT ( 'NONE',  ( -11.78843828251013015, -9.234221910056348293, 34.70572697212741531 ) ) ;
#70850=EDGE_CURVE ( 'NONE', #63664, #74128, #68456, .T. ) ;
#70853=ORIENTED_EDGE ( 'NONE', *, *, #80528, .T. ) ;
#70854=CARTESIAN_POINT ( 'NONE',  ( 16.15384615384615330, -8.973038597847269315, 34.52809138561121927 ) ) ;
#70855=CARTESIAN_POINT ( 'NONE',  ( 13.13461538461538680, -7.500000000000001776, 35.00000000000000000 ) ) ;
#70856=ORIENTED_EDGE ( 'NONE', *, *, #58675, .F. ) ;
#70857=ORIENTED_EDGE ( 'NONE', *, *, #14187, .T. ) ;
#70859=CARTESIAN_POINT ( 'NONE',  ( 4.153846153846154188, -12.10708131394839349, 31.69288490824020244 ) ) ;
#70860=EDGE_CURVE ( 'NONE', #20749, #11535, #72911, .T. ) ;
#70861=CARTESIAN_POINT ( 'NONE',  ( -4.854143407945007205, -12.69155399931963046, 30.53255429739158444 ) ) ;
#70862=CARTESIAN_POINT ( 'NONE',  ( 0.2115384615384615363, -7.566082377512563184, 35.00000000000000711 ) ) ;
#70863=FACE_OUTER_BOUND ( 'NONE', #56710, .T. ) ;
#70864=CARTESIAN_POINT ( 'NONE',  ( -13.25382494364843389, -6.369690395747422684, 34.87708834333098196 ) ) ;
#70865=ADVANCED_FACE ( 'NONE', ( #27331 ), #82285, .F. ) ;
#70866=CARTESIAN_POINT ( 'NONE',  ( -8.992715693795101828, -3.019605429927184836, 32.48692288466676814 ) ) ;
#70868=CARTESIAN_POINT ( 'NONE',  ( 0.2115384615384616196, -2.249999999999998668, 29.75000000000000355 ) ) ;
#70869=ORIENTED_EDGE ( 'NONE', *, *, #55103, .F. ) ;
#70870=CARTESIAN_POINT ( 'NONE',  ( 6.222779541268410597, -10.81320215134717344, 33.49497208177562868 ) ) ;
#70871=CARTESIAN_POINT ( 'NONE',  ( -17.29980175935171616, -7.630691491037286056, 34.74850469731152458 ) ) ;
#70872=DIRECTION ( 'NONE',  ( 0.000000000000000000, 0.8660254037844377084, -0.5000000000000015543 ) ) ;
#70873=LINE ( 'NONE', #8732, #39829 ) ;
#70874=ORIENTED_EDGE ( 'NONE', *, *, #16316, .F. ) ;
#70875=CARTESIAN_POINT ( 'NONE',  ( -17.74994558008654622, -8.346898887586322147, 34.93166121998716278 ) ) ;
#70877=LINE ( 'NONE', #51009, #81533 ) ;
#70878=CARTESIAN_POINT ( 'NONE',  ( 5.999999999999878320, -12.70778746994576025, 30.41441678777401236 ) ) ;
#70879=ORIENTED_EDGE ( 'NONE', *, *, #75334, .F. ) ;
#70880=CARTESIAN_POINT ( 'NONE',  ( -2.307692307692305711, -6.343179335718451384, 34.87096338111211935 ) ) ;
#70881=CARTESIAN_POINT ( 'NONE',  ( -12.23857555797697927, -7.369474270740069777, 34.74850911626239736 ) ) ;
#70882=CARTESIAN_POINT ( 'NONE',  ( 8.834486340506797930, -4.481592998940250538, 33.73612834413965089 ) ) ;
#70883=VERTEX_POINT ( 'NONE', #40416 ) ;
#70884=CARTESIAN_POINT ( 'NONE',  ( -10.68063560554585578, -2.506253911140460922, 30.00000000000013856 ) ) ;
#70885=EDGE_LOOP ( 'NONE', ( #35381, #56189 ) ) ;
#70887=CARTESIAN_POINT ( 'NONE',  ( 13.16168842570853670, -12.38737895849757820, 31.66785238281580206 ) ) ;
#70888=AXIS2_PLACEMENT_3D ( 'NONE', #23463, #9956, #52272 ) ;
#70889=CARTESIAN_POINT ( 'NONE',  ( 8.992243613324164997, -9.172514111537584114, 34.72667873470787470 ) ) ;
#70890=CARTESIAN_POINT ( 'NONE',  ( -8.069638770718178478, -2.612411019501189369, 31.66733052389439962 ) ) ;
#70891=EDGE_CURVE ( 'NONE', #30065, #48397, #36400, .T. ) ;
#70892=CARTESIAN_POINT ( 'NONE',  ( -14.17690049986752321, -11.71459661697925903, 32.44059661609676937 ) ) ;
#70893=CARTESIAN_POINT ( 'NONE',  ( -3.480769230769229061, -7.566082377512563184, 35.00000000000000711 ) ) ;
#70894=AXIS2_PLACEMENT_3D ( 'NONE', #68011, #34210, #41855 ) ;
#70895=EDGE_LOOP ( 'NONE', ( #32988, #33546, #6166, #21565, #19959, #44913 ) ) ;
#70896=EDGE_CURVE ( 'NONE', #70330, #31113, #30012, .T. ) ;
#70897=EDGE_LOOP ( 'NONE', ( #49267, #86001 ) ) ;
#70899=CARTESIAN_POINT ( 'NONE',  ( -16.15384615384615330, -1.129524287112498415, 32.06866353760679544 ) ) ;
#70900=CARTESIAN_POINT ( 'NONE',  ( -16.82697755857493149, -3.712312575010499494, 33.01462480002815170 ) ) ;
#70901=EDGE_CURVE ( 'NONE', #38328, #88554, #83622, .T. ) ;
#70902=CARTESIAN_POINT ( 'NONE',  ( 0.6843181305165266792, -6.717445702608402236, 34.94155399931962336 ) ) ;
#70903=CARTESIAN_POINT ( 'NONE',  ( 0.2115152373170028910, -12.45566812827425096, 31.48439005359158926 ) ) ;
#70904=FACE_OUTER_BOUND ( 'NONE', #48578, .T. ) ;
#70905=CARTESIAN_POINT ( 'NONE',  ( -17.07692307692307665, -1.466349020453238561, 30.81389545987213907 ) ) ;
#70906=EDGE_LOOP ( 'NONE', ( #17440, #64174 ) ) ;
#70907=ORIENTED_EDGE ( 'NONE', *, *, #21168, .F. ) ;
#70909=ADVANCED_FACE ( 'NONE', ( #23665 ), #10162, .F. ) ;
#70910=CARTESIAN_POINT ( 'NONE',  ( 4.403900573759605308, -4.074993327901525575, 33.72946981652012255 ) ) ;
#70912=CARTESIAN_POINT ( 'NONE',  ( -9.915792636031639518, -9.331801661448606566, 34.40259984581193464 ) ) ;
#70913=CARTESIAN_POINT ( 'NONE',  ( -8.703975197954743948, -11.48612834413965977, 32.76840700105972815 ) ) ;
#70914=VECTOR ( 'NONE', #78207, 1000.000000000000000 ) ;
#70916=EDGE_LOOP ( 'NONE', ( #17772, #56327, #18686, #30625 ) ) ;
#70917=VERTEX_POINT ( 'NONE', #22343 ) ;
#70918=CARTESIAN_POINT ( 'NONE',  ( -18.00000000000000000, -2.833524468853757305, 32.15551576947926549 ) ) ;
#70921=FACE_BOUND ( 'NONE', #41667, .T. ) ;
#70922=CARTESIAN_POINT ( 'NONE',  ( 15.10007776410167502, -9.804603061927743113, 34.18744698557895845 ) ) ;
#70923=CARTESIAN_POINT ( 'NONE',  ( -4.088590582570127197, -11.94971097300157403, 32.03036669348361443 ) ) ;
#70924=ORIENTED_EDGE ( 'NONE', *, *, #84190, .F. ) ;
#70925=CARTESIAN_POINT ( 'NONE',  ( 16.28463796167094557, -11.18335022499818621, 33.13157742990016885 ) ) ;
#70926=EDGE_CURVE ( 'NONE', #34160, #18655, #85845, .T. ) ;
#70928=CARTESIAN_POINT ( 'NONE',  ( 10.61538461538461675, -2.721908614388771852, 31.22303859784724978 ) ) ;
#70929=CARTESIAN_POINT ( 'NONE',  ( -11.76194648218548444, -5.912607949931405926, 34.49155766932282319 ) ) ;
#70931=CARTESIAN_POINT ( 'NONE',  ( -6.923076923076922462, -11.16473453929635440, 33.15142922261926373 ) ) ;
#70932=CARTESIAN_POINT ( 'NONE',  ( 3.480714749117372442, -4.336752205174647656, 33.62275283266504289 ) ) ;
#70933=FACE_OUTER_BOUND ( 'NONE', #36012, .T. ) ;
#70934=DIRECTION ( 'NONE',  ( -0.000000000000000000, 0.5000000000000011102, -0.8660254037844380415 ) ) ;
#70935=DIRECTION ( 'NONE',  ( -0.000000000000000000, 0.9396926207859093161, -0.3420201433256663259 ) ) ;
#70936=DIRECTION ( 'NONE',  ( 1.000000000000000000, 0.000000000000000000, 0.000000000000000000 ) ) ;
#70937=CARTESIAN_POINT ( 'NONE',  ( 4.403791672194295792, -12.22109172314383052, 31.39792113162168263 ) ) ;
#70938=LINE ( 'NONE', #57413, #43112 ) ;
#70939=ADVANCED_FACE ( 'NONE', ( #84500 ), #70533, .F. ) ;
#70940=CARTESIAN_POINT ( 'NONE',  ( 13.38461538461538680, -3.513871655860378418, 32.76840700105978499 ) ) ;
#70941=FACE_OUTER_BOUND ( 'NONE', #24320, .T. ) ;
#70942=CARTESIAN_POINT ( 'NONE',  ( 5.934729554039225974, -10.90142922261923886, 33.41473453929638993 ) ) ;
#70943=DIRECTION ( 'NONE',  ( -0.000000000000000000, 0.8660254037844397068, -0.4999999999999978906 ) ) ;
#70945=ORIENTED_EDGE ( 'NONE', *, *, #44932, .F. ) ;
#70948=VERTEX_POINT ( 'NONE', #57451 ) ;
#70950=CYLINDRICAL_SURFACE ( 'NONE', #11908, 0.2499999999999995559 ) ;
#70951=ORIENTED_EDGE ( 'NONE', *, *, #15660, .T. ) ;
#70953=VERTEX_POINT ( 'NONE', #71853 ) ;
#70954=CARTESIAN_POINT ( 'NONE',  ( -2.307692307692305711, -7.500000000000001776, 35.04278698407183867 ) ) ;
#70956=CARTESIAN_POINT ( 'NONE',  ( 7.622668921589514923, -8.539481045369596401, 34.89627647299170832 ) ) ;
#70957=ADVANCED_FACE ( 'NONE', ( #78172 ), #76852, .F. ) ;
#70958=CARTESIAN_POINT ( 'NONE',  ( 7.053602361310569613, -10.31582465632705237, 34.18122507451815295 ) ) ;
#70959=CARTESIAN_POINT ( 'NONE',  ( -5.076923076923197442, -5.219633306517616589, 34.19971097300220464 ) ) ;
#70960=CARTESIAN_POINT ( 'NONE',  ( 14.98079248672063990, -8.347322224742351082, 34.93158281831414769 ) ) ;
#70961=CARTESIAN_POINT ( 'NONE',  ( -8.769230769230768274, -13.78497067705608181, 32.30358669280327177 ) ) ;
#70962=CARTESIAN_POINT ( 'NONE',  ( -2.307692307692305711, -11.91647553114624181, 32.58852847137148245 ) ) ;
#70964=EDGE_CURVE ( 'NONE', #70411, #47496, #35866, .T. ) ;
#70965=EDGE_CURVE ( 'NONE', #34216, #8288, #49310, .T. ) ;
#70966=CARTESIAN_POINT ( 'NONE',  ( 1.449870955891411128, -3.300289026998475705, 32.46337939537591666 ) ) ;
#70968=EDGE_CURVE ( 'NONE', #58674, #58923, #80409, .T. ) ;
#70969=CARTESIAN_POINT ( 'NONE',  ( 10.61538461538461675, -5.471508081941601098, 34.59228464037088457 ) ) ;
#70972=CARTESIAN_POINT ( 'NONE',  ( 3.230769230769110045, -6.026961402154118908, 34.52809138561165270 ) ) ;
#70973=ORIENTED_EDGE ( 'NONE', *, *, #36483, .T. ) ;
#70975=CARTESIAN_POINT ( 'NONE',  ( 12.21151523731700550, -8.475808217655753651, 34.90892951860618609 ) ) ;
#70976=CARTESIAN_POINT ( 'NONE',  ( 9.942362003946008997, -6.567000820036036579, 34.66262288849541306 ) ) ;
#70977=CARTESIAN_POINT ( 'NONE',  ( 15.10015957556514721, -7.722926974430166069, 34.99546784045485737 ) ) ;
#70978=DIRECTION ( 'NONE',  ( 0.000000000000000000, 1.000000000000000000, 0.000000000000000000 ) ) ;
#70980=VECTOR ( 'NONE', #50742, 1000.000000000000000 ) ;
#70981=AXIS2_PLACEMENT_3D ( 'NONE', #4761, #87633, #65995 ) ;
#70982=CARTESIAN_POINT ( 'NONE',  ( -6.923076923076922462, -6.435427911321262684, 35.78748833219616898 ) ) ;
#70983=B_SPLINE_CURVE_WITH_KNOTS ( 'NONE', 3,
 ( #13937, #40544, #81086, #12175, #54928, #60795, #13497, #54031, #68009, #20697 ),
 .UNSPECIFIED., .F., .F.,
 ( 4, 2, 2, 2, 4 ),
 ( 0.000000000000000000, 0.0001954339857564075015, 0.0003908679715128150029, 0.0005863019572692224502, 0.0007817359430256300059 ),
 .UNSPECIFIED. ) ;
#70984=B_SPLINE_CURVE_WITH_KNOTS ( 'NONE', 3,
 ( #19754, #20632, #48536, #75573, #67504, #35033, #88242, #21518, #62062, #47216 ),
 .UNSPECIFIED., .F., .F.,
 ( 4, 2, 2, 2, 4 ),
 ( 0.000000000000000000, 0.0001954311564186865221, 0.0003908623128373730441, 0.0005862934692560595662, 0.0007817246256747460882 ),
 .UNSPECIFIED. ) ;
#70985=ORIENTED_EDGE ( 'NONE', *, *, #84705, .F. ) ;
#70987=VERTEX_POINT ( 'NONE', #38980 ) ;
#70988=CARTESIAN_POINT ( 'NONE',  ( -6.857821783564084228, -5.941354392334606160, 34.76329471203374055 ) ) ;
#70989=CARTESIAN_POINT ( 'NONE',  ( -8.834500769787091201, -2.379036618887870436, 30.90682066428147934 ) ) ;
#70990=FACE_OUTER_BOUND ( 'NONE', #65447, .T. ) ;
#70991=CARTESIAN_POINT ( 'NONE',  ( 17.93472999944368240, -9.528491918058357157, 34.59228464037090589 ) ) ;
#70992=EDGE_LOOP ( 'NONE', ( #8270, #61783, #22524, #70808 ) ) ;
#70993=DIRECTION ( 'NONE',  ( 0.000000000000000000, 0.9396926207859126468, 0.3420201433256571111 ) ) ;
#70994=ORIENTED_EDGE ( 'NONE', *, *, #2804, .F. ) ;
#70995=ORIENTED_EDGE ( 'NONE', *, *, #64546, .F. ) ;
#70996=VECTOR ( 'NONE', #3418, 1000.000000000000114 ) ;
#70997=CARTESIAN_POINT ( 'NONE',  ( -15.29603967673000398, -12.27809138561121394, 31.22303859784730307 ) ) ;
#70998=DIRECTION ( 'NONE',  ( -0.000000000000000000, 1.000000000000000000, -0.000000000000000000 ) ) ;
#71002=CARTESIAN_POINT ( 'NONE',  ( 4.023154687178597477, -4.118384482072085184, 33.43331474514187107 ) ) ;
#71004=ORIENTED_EDGE ( 'NONE', *, *, #49351, .F. ) ;
#71007=B_SPLINE_CURVE_WITH_KNOTS ( 'NONE', 3,
 ( #79809, #58629, #71253, #57308, #58184, #57753, #23512, #3685, #24399, #64058 ),
 .UNSPECIFIED., .F., .F.,
 ( 4, 2, 2, 2, 4 ),
 ( 0.0007817359430256320659, 0.0009771253907249987086, 0.001172514838424365460, 0.001367904286123731994, 0.001563293733823098745 ),
 .UNSPECIFIED. ) ;
#71008=VERTEX_POINT ( 'NONE', #31323 ) ;
#71009=CARTESIAN_POINT ( 'NONE',  ( -14.30769230769242917, -2.379036618888197729, 30.90682066428292885 ) ) ;
#71011=CARTESIAN_POINT ( 'NONE',  ( -7.173100160369888734, -12.43535235679832596, 30.55408501211184813 ) ) ;
#71013=CARTESIAN_POINT ( 'NONE',  ( 6.923076923076924238, -11.69971097300155272, 32.46337939537588113 ) ) ;
#71014=ORIENTED_EDGE ( 'NONE', *, *, #23573, .T. ) ;
#71015=CARTESIAN_POINT ( 'NONE',  ( -4.153846153846152411, -13.20930481340135110, 34.54067556320372745 ) ) ;
#71016=CARTESIAN_POINT ( 'NONE',  ( 4.826923076923076650, -2.249999999999998668, 29.75000000000000355 ) ) ;
#71018=FACE_BOUND ( 'NONE', #64858, .T. ) ;
#71019=DIRECTION ( 'NONE',  ( -0.000000000000000000, -1.000000000000000000, -8.673617379884033500E-16 ) ) ;
#71020=CARTESIAN_POINT ( 'NONE',  ( 17.93472999944368240, -12.70778746994557551, 30.41441678777548319 ) ) ;
#71021=ADVANCED_FACE ( 'NONE', ( #73201 ), #86286, .T. ) ;
#71022=FACE_OUTER_BOUND ( 'NONE', #33685, .T. ) ;
#71023=CARTESIAN_POINT ( 'NONE',  ( 5.749976775778544713, -12.45566812827425096, 31.48439005359158926 ) ) ;
#71024=CARTESIAN_POINT ( 'NONE',  ( 9.692307692307695177, -4.102666532097928531, 36.13435417666054406 ) ) ;
#71029=DIRECTION ( 'NONE',  ( -0.000000000000000000, -0.1736481776669307198, -0.9848077530122080203 ) ) ;
#71030=EDGE_LOOP ( 'NONE', ( #51933, #66710 ) ) ;
#71031=CARTESIAN_POINT ( 'NONE',  ( 7.145856464345333059, -2.847695495035524882, 31.58253572463339509 ) ) ;
#71032=CARTESIAN_POINT ( 'NONE',  ( -18.06608237936013595, -12.62096338111211580, 30.90682066428152908 ) ) ;
#71033=CARTESIAN_POINT ( 'NONE',  ( 16.02315555073584719, -6.369640206132551441, 34.87707690430378449 ) ) ;
#71034=CARTESIAN_POINT ( 'NONE',  ( 16.15384615384603251, -2.892918686052165622, 31.69288490824153470 ) ) ;
#71035=LINE ( 'NONE', #42690, #6855 ) ;
#71036=CARTESIAN_POINT ( 'NONE',  ( 7.596130608860880429, -8.432397168068783699, 34.66272746175022945 ) ) ;
#71037=FACE_BOUND ( 'NONE', #1127, .T. ) ;
#71038=DIRECTION ( 'NONE',  ( -0.000000000000000000, 0.9848077530122086864, -0.1736481776669273891 ) ) ;
#71039=CARTESIAN_POINT ( 'NONE',  ( -10.39242148111793895, -7.369474539155828730, 34.99858011523957657 ) ) ;
#71040=EDGE_CURVE ( 'NONE', #67434, #39096, #3393, .T. ) ;
#71041=CARTESIAN_POINT ( 'NONE',  ( -18.06608237936013239, -8.164416787775447659, 34.95778746994557906 ) ) ;
#71042=DIRECTION ( 'NONE',  ( -0.000000000000000000, -0.000000000000000000, 1.000000000000000000 ) ) ;
#71043=CARTESIAN_POINT ( 'NONE',  ( -15.09997742294444478, -6.413143153341454017, 34.63066358083362672 ) ) ;
#71044=DIRECTION ( 'NONE',  ( -0.000000000000000000, 1.000000000000000000, 3.491481338843133355E-15 ) ) ;
#71046=ORIENTED_EDGE ( 'NONE', *, *, #5336, .F. ) ;
#71047=CARTESIAN_POINT ( 'NONE',  ( -4.403869391139118683, -11.86270091957321249, 32.19358267280087915 ) ) ;
#71048=DIRECTION ( 'NONE',  ( -0.000000000000000000, 0.9848077530122085754, -0.1736481776669273613 ) ) ;
#71049=CYLINDRICAL_SURFACE ( 'NONE', #51701, 0.2500000000000009437 ) ;
#71051=CARTESIAN_POINT ( 'NONE',  ( 10.61538461538449596, -12.27809138561165270, 31.22303859784587132 ) ) ;
#71053=CARTESIAN_POINT ( 'NONE',  ( -11.31503513954675100, -7.630147987733840509, 34.99859428049665411 ) ) ;
#71055=CARTESIAN_POINT ( 'NONE',  ( -17.07692307692319744, -6.026961402154118908, 34.52809138561165270 ) ) ;
#71056=CARTESIAN_POINT ( 'NONE',  ( 13.38461538461538680, -6.343179335718451384, 34.87096338111211935 ) ) ;
#71057=CARTESIAN_POINT ( 'NONE',  ( -16.85414340794500276, -4.989023458446560255, 34.36081565061822118 ) ) ;
#71059=B_SPLINE_CURVE_WITH_KNOTS ( 'NONE', 3,
 ( #81798, #46230, #5681, #20088, #66502, #47551, #39489, #40371, #75041, #19641 ),
 .UNSPECIFIED., .F., .F.,
 ( 4, 2, 2, 2, 4 ),
 ( 0.0007817246256747452209, 0.0009771112852218887673, 0.001172497944769032531, 0.001367884604316176294, 0.001563271263863319840 ),
 .UNSPECIFIED. ) ;
#71060=EDGE_CURVE ( 'NONE', #1686, #59958, #1934, .T. ) ;
#71064=DIRECTION ( 'NONE',  ( -0.000000000000000000, 0.9848077530122085754, -0.1736481776669273613 ) ) ;
#71065=ORIENTED_EDGE ( 'NONE', *, *, #24956, .F. ) ;
#71066=CARTESIAN_POINT ( 'NONE',  ( 3.453782074862625784, -12.38742843783360748, 31.66772728687926985 ) ) ;
#71067=CARTESIAN_POINT ( 'NONE',  ( -17.14219352288385068, -2.892918686051582089, 31.69288490824015980 ) ) ;
#71070=ADVANCED_FACE ( 'NONE', ( #38074 ), #79515, .F. ) ;
#71071=CARTESIAN_POINT ( 'NONE',  ( -9.692307692307812417, -5.219633306517616589, 34.19971097300220464 ) ) ;
#71072=CARTESIAN_POINT ( 'NONE',  ( 3.480823542407543769, -11.79725096376909654, 32.30694842903960762 ) ) ;
#71073=EDGE_LOOP ( 'NONE', ( #18836, #33891 ) ) ;
#71074=CARTESIAN_POINT ( 'NONE',  ( -16.28453675695646652, -3.957541250942358424, 33.62499894934981626 ) ) ;
#71075=CARTESIAN_POINT ( 'NONE',  ( 4.153846153846154188, -5.557115091759785130, 34.35708131394839171 ) ) ;
#71076=EDGE_LOOP ( 'NONE', ( #31831, #77745 ) ) ;
#71077=CARTESIAN_POINT ( 'NONE',  ( 6.989145274079363368, -3.513871655860379306, 32.76840700105978499 ) ) ;
#71078=CARTESIAN_POINT ( 'NONE',  ( 17.30034947583786220, -7.630147987733843173, 34.99859428049665411 ) ) ;
#71079=CARTESIAN_POINT ( 'NONE',  ( 6.923076923076924238, -3.050289026998446396, 32.03036669348365706 ) ) ;
#71080=CARTESIAN_POINT ( 'NONE',  ( -15.23076923076891553, -2.255955759149395501, 30.00000000000324363 ) ) ;
#71081=EDGE_LOOP ( 'NONE', ( #4448, #38955, #4413, #46633 ) ) ;
#71082=CARTESIAN_POINT ( 'NONE',  ( 8.900021210197715860, -2.295524264805589354, 30.44142389570982488 ) ) ;
#71083=CARTESIAN_POINT ( 'NONE',  ( -11.66915214157184444, -12.35290016733513951, 31.75349464988449455 ) ) ;
#71084=LINE ( 'NONE', #57568, #26908 ) ;
#71085=VERTEX_POINT ( 'NONE', #65983 ) ;
#71086=ORIENTED_EDGE ( 'NONE', *, *, #54372, .T. ) ;
#71087=EDGE_LOOP ( 'NONE', ( #78431, #56478 ) ) ;
#71089=CARTESIAN_POINT ( 'NONE',  ( 13.51514082284903040, -3.625058011473228703, 33.29252011169590020 ) ) ;
#71090=CARTESIAN_POINT ( 'NONE',  ( -3.165514091256390827, -8.656820664281605460, 34.87096338111211224 ) ) ;
#71091=VECTOR ( 'NONE', #39035, 1000.000000000000114 ) ;
#71092=CARTESIAN_POINT ( 'NONE',  ( 15.36081439360400935, -2.504778602574659896, 29.97347330155780654 ) ) ;
#71094=ORIENTED_EDGE ( 'NONE', *, *, #85486, .F. ) ;
#71095=CARTESIAN_POINT ( 'NONE',  ( -1.384615384615383471, -2.833524468853757305, 32.15551576947925838 ) ) ;
#71096=ORIENTED_EDGE ( 'NONE', *, *, #22167, .F. ) ;
#71097=B_SPLINE_CURVE_WITH_KNOTS ( 'NONE', 3,
 ( #33887, #41537, #61346, #54593, #5987, #62240, #82088, #55486, #82971, #21253 ),
 .UNSPECIFIED., .F., .F.,
 ( 4, 2, 2, 2, 4 ),
 ( 0.0007817359430256392216, 0.0009771253907250080327, 0.001172514838424376952, 0.001367904286123745872, 0.001563293733823114791 ),
 .UNSPECIFIED. ) ;
#71098=B_SPLINE_CURVE_WITH_KNOTS ( 'NONE', 3,
 ( #38403, #65860, #88724, #81512, #46824, #34644, #12604, #26113, #40091, #19801 ),
 .UNSPECIFIED., .F., .F.,
 ( 4, 2, 2, 2, 4 ),
 ( 0.000000000000000000, 0.0001954339857564079623, 0.0003908679715128159245, 0.0005863019572692238597, 0.0007817359430256318490 ),
 .UNSPECIFIED. ) ;
#71099=CARTESIAN_POINT ( 'NONE',  ( 16.28389131668093270, -2.504778602574659896, 29.97347330155780654 ) ) ;
#71100=FACE_OUTER_BOUND ( 'NONE', #21756, .T. ) ;
#71101=DIRECTION ( 'NONE',  ( 0.000000000000000000, 0.000000000000000000, 1.000000000000000000 ) ) ;
#71102=ORIENTED_EDGE ( 'NONE', *, *, #39525, .T. ) ;
#71104=ORIENTED_EDGE ( 'NONE', *, *, #68172, .T. ) ;
#71105=CARTESIAN_POINT ( 'NONE',  ( -12.39628289026243557, -5.219633306516380244, 34.19971097300157936 ) ) ;
#71106=ORIENTED_EDGE ( 'NONE', *, *, #31612, .T. ) ;
#71107=CARTESIAN_POINT ( 'NONE',  ( -10.61538461538461320, -1.242168528481310874, 33.36296068462461051 ) ) ;
#71108=AXIS2_PLACEMENT_3D ( 'NONE', #63375, #76009, #83675 ) ;
#71109=CARTESIAN_POINT ( 'NONE',  ( -10.86540783960607293, -9.356822207818506598, 34.66110646841856635 ) ) ;
#71111=LINE ( 'NONE', #63018, #42 ) ;
#71112=CARTESIAN_POINT ( 'NONE',  ( -4.153846153845837108, -2.255955759149395501, 30.00000000000324363 ) ) ;
#71113=CARTESIAN_POINT ( 'NONE',  ( -9.019207513279360100, -12.01397095200674059, 32.43157075238190146 ) ) ;
#71114=FACE_BOUND ( 'NONE', #86405, .T. ) ;
#71115=AXIS2_PLACEMENT_3D ( 'NONE', #89073, #27349, #82303 ) ;
#71116=CARTESIAN_POINT ( 'NONE',  ( -9.469528023329623068, -4.226511098958373402, 33.85474049983370293 ) ) ;
#71117=CARTESIAN_POINT ( 'NONE',  ( -4.403822884788507253, -12.17611988154120972, 31.52148481390971213 ) ) ;
#71118=AXIS2_PLACEMENT_3D ( 'NONE', #29170, #84111, #2550 ) ;
#71119=EDGE_CURVE ( 'NONE', #76747, #88972, #45951, .T. ) ;
#71120=FACE_OUTER_BOUND ( 'NONE', #10106, .T. ) ;
#71121=CARTESIAN_POINT ( 'NONE',  ( 2.307692307692187583, -11.94971097300221174, 32.03036669348237098 ) ) ;
#71123=CARTESIAN_POINT ( 'NONE',  ( -8.069638789877792817, -3.236172620538810385, 32.36188796281390267 ) ) ;
#71124=CARTESIAN_POINT ( 'NONE',  ( 10.48523664565291647, -11.04286588640298561, 33.62463336215343901 ) ) ;
#71126=CARTESIAN_POINT ( 'NONE',  ( 14.43773991394799339, -7.723484964179501588, 34.74522123443823318 ) ) ;
#71127=EDGE_CURVE ( 'NONE', #48109, #54822, #4747, .T. ) ;
#71129=EDGE_LOOP ( 'NONE', ( #40037, #7229, #41433, #6821 ) ) ;
#71131=CARTESIAN_POINT ( 'NONE',  ( -14.30769230769230660, -4.102666532097928531, 36.13435417666054406 ) ) ;
#71132=CARTESIAN_POINT ( 'NONE',  ( 2.557746619330623083, -2.564540009722895419, 30.55348353981670684 ) ) ;
#71133=CARTESIAN_POINT ( 'NONE',  ( -14.24162395668986747, -2.721908614388772296, 31.22303859784725333 ) ) ;
#71134=CARTESIAN_POINT ( 'NONE',  ( 1.384615384615386802, -6.386643153685126251, 34.62446782046654192 ) ) ;
#71136=ORIENTED_EDGE ( 'NONE', *, *, #41435, .T. ) ;
#71137=CARTESIAN_POINT ( 'NONE',  ( 13.25446817517716980, -5.195881422630166391, 34.18770438780619259 ) ) ;
#71138=DIRECTION ( 'NONE',  ( 0.000000000000000000, 0.6427876096865373645, -0.7660444431189797898 ) ) ;
#71139=B_SPLINE_CURVE_WITH_KNOTS ( 'NONE', 3,
 ( #33696, #55287, #76003, #6659, #41792, #61151, #13858, #48081, #47198, #74690 ),
 .UNSPECIFIED., .F., .F.,
 ( 4, 2, 2, 2, 4 ),
 ( 0.0007817359430256364027, 0.0009771253907250043464, 0.001172514838424372399, 0.001367904286123740234, 0.001563293733823108286 ),
 .UNSPECIFIED. ) ;
#71140=CARTESIAN_POINT ( 'NONE',  ( -18.00000000000030553, -12.49374608885938542, 30.00000000000319744 ) ) ;
#71141=EDGE_CURVE ( 'NONE', #37467, #48549, #83627, .T. ) ;
#71142=CARTESIAN_POINT ( 'NONE',  ( -11.53846153846153655, -2.249999999999998668, 29.50000000000001421 ) ) ;
#71143=FACE_OUTER_BOUND ( 'NONE', #6782, .T. ) ;
#71146=VERTEX_POINT ( 'NONE', #11951 ) ;
#71149=VERTEX_POINT ( 'NONE', #33978 ) ;
#71150=DIRECTION ( 'NONE',  ( 0.000000000000000000, 0.8660254037844377084, 0.5000000000000015543 ) ) ;
#71151=CARTESIAN_POINT ( 'NONE',  ( 13.38461538461526423, -2.379036618888197729, 30.90682066428292885 ) ) ;
#71152=CARTESIAN_POINT ( 'NONE',  ( -6.923076923077044142, -9.442884908241554243, 34.35708131394783038 ) ) ;
#71155=DIRECTION ( 'NONE',  ( -0.000000000000000000, -0.3420201433256694346, -0.9396926207859080948 ) ) ;
#71156=ORIENTED_EDGE ( 'NONE', *, *, #77535, .T. ) ;
#71157=CARTESIAN_POINT ( 'NONE',  ( 4.088522141041845082, -7.749976730030849303, 34.74374725381503737 ) ) ;
#71158=FACE_OUTER_BOUND ( 'NONE', #35962, .T. ) ;
#71159=ORIENTED_EDGE ( 'NONE', *, *, #46070, .T. ) ;
#71160=CARTESIAN_POINT ( 'NONE',  ( 15.23076923076923173, -2.249999999999998668, 29.75000000000001776 ) ) ;
#71161=DIRECTION ( 'NONE',  ( -0.000000000000000000, 0.7660444431189791237, -0.6427876096865379196 ) ) ;
#71162=CARTESIAN_POINT ( 'NONE',  ( 6.065255139512838234, -9.528491918058460186, 34.59228464037085615 ) ) ;
#71163=CYLINDRICAL_SURFACE ( 'NONE', #50486, 0.2499999999999995559 ) ;
#71164=EDGE_CURVE ( 'NONE', #71551, #83423, #54685, .T. ) ;
#71165=CARTESIAN_POINT ( 'NONE',  ( -12.46153846153846168, -12.37446782046654192, 30.86335684631486131 ) ) ;
#71166=CARTESIAN_POINT ( 'NONE',  ( -6.923076923077044142, -5.219633306517616589, 34.19971097300220464 ) ) ;
#71167=EDGE_CURVE ( 'NONE', #9998, #37993, #47933, .T. ) ;
#71169=VERTEX_POINT ( 'NONE', #82180 ) ;
#71170=CARTESIAN_POINT ( 'NONE',  ( 5.076923076922954969, -10.21337939537710326, 33.94971097300076224 ) ) ;
#71171=DIRECTION ( 'NONE',  ( -0.000000000000000000, -0.000000000000000000, -1.000000000000000000 ) ) ;
#71173=ADVANCED_FACE ( 'NONE', ( #76292 ), #67771, .F. ) ;
#71174=CARTESIAN_POINT ( 'NONE',  ( -13.63459211555773720, -12.41269422305637171, 30.68257228309993323 ) ) ;
#71176=ADVANCED_FACE ( 'NONE', ( #67334 ), #75413, .F. ) ;
#71177=EDGE_LOOP ( 'NONE', ( #43352, #86873 ) ) ;
#71179=CARTESIAN_POINT ( 'NONE',  ( 3.007284287045282944, -9.331801661448606566, 34.40259984581193464 ) ) ;
#71180=ORIENTED_EDGE ( 'NONE', *, *, #28793, .F. ) ;
#71181=FACE_OUTER_BOUND ( 'NONE', #82542, .T. ) ;
#71182=ORIENTED_EDGE ( 'NONE', *, *, #65649, .F. ) ;
#71183=B_SPLINE_CURVE_WITH_KNOTS ( 'NONE', 3,
 ( #85239, #23958, #1929, #64062, #63626, #9566, #84361, #37028, #71257, #29849 ),
 .UNSPECIFIED., .F., .F.,
 ( 4, 2, 2, 2, 4 ),
 ( 0.0007817359430256334753, 0.0009771253907250058643, 0.001172514838424371098, 0.001367904286123736764, 0.001563293733823101998 ),
 .UNSPECIFIED. ) ;
#71184=DIRECTION ( 'NONE',  ( -0.000000000000000000, 0.5000000000000011102, -0.8660254037844380415 ) ) ;
#71185=CARTESIAN_POINT ( 'NONE',  ( 4.087762742890271639, -3.513871655860377086, 32.76840700105978499 ) ) ;
#71186=CARTESIAN_POINT ( 'NONE',  ( -1.450698795571264021, -4.098570777380720287, 33.41473453929634729 ) ) ;
#71187=CARTESIAN_POINT ( 'NONE',  ( -13.31854805126531005, -12.62096338111211757, 30.90682066428152908 ) ) ;
#71188=ORIENTED_EDGE ( 'NONE', *, *, #80871, .F. ) ;
#71189=CARTESIAN_POINT ( 'NONE',  ( -13.13466997523734037, -2.986452184633680229, 32.43230066228895225 ) ) ;
#71191=ORIENTED_EDGE ( 'NONE', *, *, #60948, .F. ) ;
#71192=CARTESIAN_POINT ( 'NONE',  ( 2.557692307692308376, -2.499999999999998668, 29.75000000000000355 ) ) ;
#71193=LINE ( 'NONE', #55908, #64200 ) ;
#71195=DIRECTION ( 'NONE',  ( -0.000000000000000000, -0.6427876096865404731, -0.7660444431189771253 ) ) ;
#71196=CARTESIAN_POINT ( 'NONE',  ( -14.55766903863466055, -10.66389620160130036, 33.62221079203477103 ) ) ;
#71197=CARTESIAN_POINT ( 'NONE',  ( -11.66915300512909326, -2.729777683071817229, 31.24903638046269450 ) ) ;
#71198=CARTESIAN_POINT ( 'NONE',  ( 2.307692307692309264, -12.29105614889573062, 35.45975837776705220 ) ) ;
#71199=DIRECTION ( 'NONE',  ( -0.000000000000000000, 1.000000000000000000, 3.491481338843133355E-15 ) ) ;
#71200=EDGE_CURVE ( 'NONE', #88652, #15863, #70679, .T. ) ;
#71201=ORIENTED_EDGE ( 'NONE', *, *, #27126, .T. ) ;
#71202=ORIENTED_EDGE ( 'NONE', *, *, #58038, .F. ) ;
#71203=FACE_BOUND ( 'NONE', #83840, .T. ) ;
#71204=ORIENTED_EDGE ( 'NONE', *, *, #54978, .F. ) ;
#71205=CARTESIAN_POINT ( 'NONE',  ( -8.703162418228332697, -4.098570777380720287, 33.41473453929635440 ) ) ;
#71206=CARTESIAN_POINT ( 'NONE',  ( 13.38461538461526601, -10.90142922262034020, 33.41473453929536674 ) ) ;
#71207=CARTESIAN_POINT ( 'NONE',  ( -14.24243673641628050, -9.442884908240273489, 34.35708131394835618 ) ) ;
#71208=EDGE_CURVE ( 'NONE', #19526, #34542, #68652, .T. ) ;
#71209=ORIENTED_EDGE ( 'NONE', *, *, #7938, .T. ) ;
#71210=EDGE_CURVE ( 'NONE', #40661, #32458, #48818, .T. ) ;
#71212=EDGE_LOOP ( 'NONE', ( #63685, #84418, #69138, #18860 ) ) ;
#71213=CARTESIAN_POINT ( 'NONE',  ( 3.230769230769231726, -4.786620604624113540, 33.94971097300155094 ) ) ;
#71214=EDGE_LOOP ( 'NONE', ( #13276, #32879, #23671, #12182 ) ) ;
#71215=B_SPLINE_CURVE_WITH_KNOTS ( 'NONE', 3,
 ( #81573, #19416, #5471, #68056, #61718, #35, #20743, #27507, #53190, #48210 ),
 .UNSPECIFIED., .F., .F.,
 ( 4, 2, 2, 2, 4 ),
 ( 0.000000000000000000, 0.0001954339857564073388, 0.0003908679715128146777, 0.0005863019572692220165, 0.0007817359430256293554 ),
 .UNSPECIFIED. ) ;
#71216=CARTESIAN_POINT ( 'NONE',  ( 2.084812790954723383, -7.630690623152302621, 34.99857592706774057 ) ) ;
#71217=CYLINDRICAL_SURFACE ( 'NONE', #41642, 0.2500000000000012212 ) ;
#71218=CARTESIAN_POINT ( 'NONE',  ( -12.21153846153845279, -2.249999999999999112, 29.81603969181031744 ) ) ;
#71219=FACE_BOUND ( 'NONE', #16581, .T. ) ;
#71220=ORIENTED_EDGE ( 'NONE', *, *, #1840, .T. ) ;
#71222=ADVANCED_FACE ( 'NONE', ( #34425 ), #27666, .F. ) ;
#71223=CARTESIAN_POINT ( 'NONE',  ( 13.38461538461538680, -13.37000171582298513, 34.34916445242398453 ) ) ;
#71224=FACE_OUTER_BOUND ( 'NONE', #26901, .T. ) ;
#71225=CARTESIAN_POINT ( 'NONE',  ( 8.900021210197715860, -6.369690395747422684, 34.87708834333098196 ) ) ;
#71226=ORIENTED_EDGE ( 'NONE', *, *, #25486, .F. ) ;
#71227=EDGE_CURVE ( 'NONE', #27467, #87554, #81296, .T. ) ;
#71228=ORIENTED_EDGE ( 'NONE', *, *, #76965, .F. ) ;
#71229=ORIENTED_EDGE ( 'NONE', *, *, #24347, .F. ) ;
#71232=CARTESIAN_POINT ( 'NONE',  ( -10.68065506134538722, -12.27809138561121394, 31.22303859784730307 ) ) ;
#71233=CARTESIAN_POINT ( 'NONE',  ( 7.846153846153846700, -10.05456864172156806, 36.03766855953608683 ) ) ;
#71234=CARTESIAN_POINT ( 'NONE',  ( 7.780070435197965928, -12.37446782046654192, 30.86335684631486487 ) ) ;
#71235=FACE_OUTER_BOUND ( 'NONE', #6550, .T. ) ;
#71236=ORIENTED_EDGE ( 'NONE', *, *, #53113, .T. ) ;
#71237=CARTESIAN_POINT ( 'NONE',  ( -3.230769230769229949, -2.538708090699994813, 30.37095296980875503 ) ) ;
#71238=CARTESIAN_POINT ( 'NONE',  ( 2.980792486720640344, -9.234221910056348293, 34.70572697212741531 ) ) ;
#71239=CARTESIAN_POINT ( 'NONE',  ( -17.20761454359064047, -11.71456829005830080, 32.44064028649416542 ) ) ;
#71241=CARTESIAN_POINT ( 'NONE',  ( 3.453782074862626228, -11.43677907613345113, 33.22367315496201456 ) ) ;
#71242=ORIENTED_EDGE ( 'NONE', *, *, #81891, .F. ) ;
#71243=LINE ( 'NONE', #4001, #75903 ) ;
#71244=EDGE_LOOP ( 'NONE', ( #69893, #36041 ) ) ;
#71245=FACE_BOUND ( 'NONE', #9358, .T. ) ;
#71246=CARTESIAN_POINT ( 'NONE',  ( -7.173053667125515176, -10.06842814019191401, 34.32929386961144758 ) ) ;
#71248=ORIENTED_EDGE ( 'NONE', *, *, #52329, .T. ) ;
#71249=VECTOR ( 'NONE', #74900, 1000.000000000000000 ) ;
#71251=CARTESIAN_POINT ( 'NONE',  ( 6.130790440966954691, -11.37503395064541678, 33.29242100308974983 ) ) ;
#71252=CARTESIAN_POINT ( 'NONE',  ( -15.23076923076922995, -9.905515769479276145, 34.41647553114623292 ) ) ;
#71253=CARTESIAN_POINT ( 'NONE',  ( -6.792551221313358312, -3.285477652293412820, 32.44071101563363158 ) ) ;
#71254=EDGE_LOOP ( 'NONE', ( #59973, #6617 ) ) ;
#71256=ORIENTED_EDGE ( 'NONE', *, *, #28936, .F. ) ;
#71257=CARTESIAN_POINT ( 'NONE',  ( 13.45068373561782771, -12.10708131394839704, 31.69288490824020954 ) ) ;
#71258=ORIENTED_EDGE ( 'NONE', *, *, #74459, .T. ) ;
#71259=CARTESIAN_POINT ( 'NONE',  ( 3.361294932532794100, -2.619367082507848998, 30.83698974864644171 ) ) ;
#71260=CARTESIAN_POINT ( 'NONE',  ( 14.98079249982688133, -2.779195860258146578, 31.39871582349836032 ) ) ;
#71261=LINE ( 'NONE', #52326, #24205 ) ;
#71262=CARTESIAN_POINT ( 'NONE',  ( 12.59206416330202494, -4.459921816937791661, 33.71989282347011851 ) ) ;
#71263=CARTESIAN_POINT ( 'NONE',  ( -7.846153846153844924, -8.973038597847269315, 34.52809138561121927 ) ) ;
#71264=ADVANCED_FACE ( 'NONE', ( #83063 ), #74980, .F. ) ;
#71265=CARTESIAN_POINT ( 'NONE',  ( 23.00000000000000000, -10.75000000000000000, 29.75000000000000355 ) ) ;
#71267=ORIENTED_EDGE ( 'NONE', *, *, #53473, .T. ) ;
#71268=B_SPLINE_CURVE_WITH_KNOTS ( 'NONE', 3,
 ( #85393, #16930, #36755, #23680, #50254, #77741, #64214, #51131, #16046, #3408 ),
 .UNSPECIFIED., .F., .F.,
 ( 4, 2, 2, 2, 4 ),
 ( 0.0007817359430256294638, 0.0009771253907249948054, 0.001172514838424360255, 0.001367904286123725489, 0.001563293733823090939 ),
 .UNSPECIFIED. ) ;
#71269=DIRECTION ( 'NONE',  ( -0.000000000000000000, -0.9396926207859093161, -0.3420201433256663259 ) ) ;
#71271=ORIENTED_EDGE ( 'NONE', *, *, #87975, .F. ) ;
#71273=VECTOR ( 'NONE', #42387, 1000.000000000000114 ) ;
#71276=EDGE_LOOP ( 'NONE', ( #51932, #62008 ) ) ;
#71277=CARTESIAN_POINT ( 'NONE',  ( 4.153846153846032507, -12.27809138561165270, 31.22303859784587132 ) ) ;
#71279=CARTESIAN_POINT ( 'NONE',  ( -17.30040802064702987, -9.331801661448606566, 34.40259984581193464 ) ) ;
#71280=VECTOR ( 'NONE', #42174, 1000.000000000000000 ) ;
#71281=CARTESIAN_POINT ( 'NONE',  ( 0.7115384615383975042, -7.565270000091922853, 34.99999999999999289 ) ) ;
#71282=CARTESIAN_POINT ( 'NONE',  ( -4.854143535654666053, -3.755027918224367767, 33.06320215134714857 ) ) ;
#71283=CARTESIAN_POINT ( 'NONE',  ( 16.15384615384603251, -3.643525952248796163, 33.31231777344771672 ) ) ;
#71284=FACE_OUTER_BOUND ( 'NONE', #13823, .T. ) ;
#71285=ORIENTED_EDGE ( 'NONE', *, *, #62910, .F. ) ;
#71286=CARTESIAN_POINT ( 'NONE',  ( -4.023054346021365468, -5.582136614379148654, 34.36778462344220486 ) ) ;
#71287=CARTESIAN_POINT ( 'NONE',  ( 9.692307692307695177, -9.780366693483667717, 34.19971097300155094 ) ) ;
#71289=EDGE_CURVE ( 'NONE', #62019, #53607, #52635, .T. ) ;
#71290=CARTESIAN_POINT ( 'NONE',  ( 8.069165197766695385, -2.758310577978207334, 31.33698337089303010 ) ) ;
#71291=ORIENTED_EDGE ( 'NONE', *, *, #67576, .T. ) ;
#71292=CARTESIAN_POINT ( 'NONE',  ( 7.715463243043538810, -2.295517848115769421, 30.44137282052136939 ) ) ;
#71293=B_SPLINE_CURVE_WITH_KNOTS ( 'NONE', 3,
 ( #33164, #34492, #20532, #14222, #74599, #26852, #25959, #60181, #68722, #6137 ),
 .UNSPECIFIED., .F., .F.,
 ( 4, 2, 2, 2, 4 ),
 ( 0.0007817359430256365111, 0.0009771253907250043464, 0.001172514838424372399, 0.001367904286123740234, 0.001563293733823108069 ),
 .UNSPECIFIED. ) ;
#71294=ORIENTED_EDGE ( 'NONE', *, *, #22493, .F. ) ;
#71295=CARTESIAN_POINT ( 'NONE',  ( 0.7114839798866020582, -9.272278438253398036, 34.42582936511637826 ) ) ;
#71297=CARTESIAN_POINT ( 'NONE',  ( 11.60371710973756265, -10.21337939537593620, 33.94971097300152252 ) ) ;
#71298=EDGE_CURVE ( 'NONE', #15704, #17995, #23123, .T. ) ;
#71299=CYLINDRICAL_SURFACE ( 'NONE', #87310, 0.2499999999999995559 ) ;
#71300=ORIENTED_EDGE ( 'NONE', *, *, #77275, .F. ) ;
#71301=DIRECTION ( 'NONE',  ( 0.000000000000000000, 0.000000000000000000, 1.000000000000000000 ) ) ;
#71302=CARTESIAN_POINT ( 'NONE',  ( 10.39245765647776309, -12.64616026154729411, 30.79003144601914244 ) ) ;
#71303=CARTESIAN_POINT ( 'NONE',  ( -12.21153846153839595, -7.434744429011176159, 34.75000000000000711 ) ) ;
#71304=CARTESIAN_POINT ( 'NONE',  ( 17.07692307692307665, -6.343179335718451384, 34.87096338111211935 ) ) ;
#71307=EDGE_LOOP ( 'NONE', ( #42518, #5277 ) ) ;
#71308=CARTESIAN_POINT ( 'NONE',  ( -1.319359813339358256, -3.835265460703683349, 33.15142922261929925 ) ) ;
#71309=ORIENTED_EDGE ( 'NONE', *, *, #13308, .F. ) ;
#71310=B_SPLINE_CURVE_WITH_KNOTS ( 'NONE', 3,
 ( #73583, #65472, #44745, #3767, #79441, #31698, #38003, #31241, #72669, #45192 ),
 .UNSPECIFIED., .F., .F.,
 ( 4, 2, 2, 2, 4 ),
 ( 0.000000000000000000, 0.0001954339857564091278, 0.0003908679715128182556, 0.0005863019572692274375, 0.0007817359430256365111 ),
 .UNSPECIFIED. ) ;
#71311=EDGE_CURVE ( 'NONE', #87033, #25963, #35273, .T. ) ;
#71312=CYLINDRICAL_SURFACE ( 'NONE', #52239, 0.2500000000000008882 ) ;
#71313=EDGE_CURVE ( 'NONE', #34697, #20749, #78065, .T. ) ;
#71316=AXIS2_PLACEMENT_3D ( 'NONE', #8889, #24157, #2552 ) ;
#71317=CARTESIAN_POINT ( 'NONE',  ( 1.134592160393929072, -8.475808217655753651, 34.90892951860618609 ) ) ;
#71318=CARTESIAN_POINT ( 'NONE',  ( -17.77722033102192967, -12.47679350104403007, 31.42216943046555855 ) ) ;
#71319=ORIENTED_EDGE ( 'NONE', *, *, #74210, .F. ) ;
#71320=EDGE_CURVE ( 'NONE', #8333, #78525, #70877, .T. ) ;
#71322=ORIENTED_EDGE ( 'NONE', *, *, #12708, .F. ) ;
#71323=EDGE_CURVE ( 'NONE', #82116, #61213, #15047, .T. ) ;
#71325=CARTESIAN_POINT ( 'NONE',  ( 11.40777093535123043, -9.084618155246140248, 34.75535874321725771 ) ) ;
#71326=CARTESIAN_POINT ( 'NONE',  ( 17.32686859527121470, -4.336752205174650321, 33.62275283266504289 ) ) ;
#71327=CARTESIAN_POINT ( 'NONE',  ( -13.13466986626724164, -5.852078868378309373, 34.47109172314383585 ) ) ;
#71328=CYLINDRICAL_SURFACE ( 'NONE', #58575, 0.2500000000000008882 ) ;
#71329=CARTESIAN_POINT ( 'NONE',  ( 5.869308533332444178, -11.71456829005830080, 32.44064028649416542 ) ) ;
#71330=CARTESIAN_POINT ( 'NONE',  ( 14.43848411551709709, -9.804649428959608670, 34.18742332936588468 ) ) ;
#71331=ORIENTED_EDGE ( 'NONE', *, *, #68557, .F. ) ;
#71332=EDGE_CURVE ( 'NONE', #4198, #47170, #9183, .T. ) ;
#71333=ORIENTED_EDGE ( 'NONE', *, *, #11829, .F. ) ;
#71334=B_SPLINE_CURVE_WITH_KNOTS ( 'NONE', 3,
 ( #10497, #17700, #66321, #32096, #4623, #58668, #11378, #37963, #19028, #59114 ),
 .UNSPECIFIED., .F., .F.,
 ( 4, 2, 2, 2, 4 ),
 ( 0.000000000000000000, 0.0001954311564186864949, 0.0003908623128373729899, 0.0005862934692560594577, 0.0007817246256747459798 ),
 .UNSPECIFIED. ) ;
#71335=AXIS2_PLACEMENT_3D ( 'NONE', #80862, #74092, #4287 ) ;
#71336=ORIENTED_EDGE ( 'NONE', *, *, #18608, .F. ) ;
#71337=CARTESIAN_POINT ( 'NONE',  ( 6.130525438233648039, -12.50538340440932217, 31.33453814440721885 ) ) ;
#71340=CARTESIAN_POINT ( 'NONE',  ( -5.326899820971668476, -12.65889640711025521, 30.72598325615533454 ) ) ;
#71341=B_SPLINE_CURVE_WITH_KNOTS ( 'NONE', 3,
 ( #68838, #7143, #34614, #62080, #390, #35501, #21084, #14339, #62948, #77805 ),
 .UNSPECIFIED., .F., .F.,
 ( 4, 2, 2, 2, 4 ),
 ( 0.000000000000000000, 0.0001954311564186871184, 0.0003908623128373742367, 0.0005862934692560614093, 0.0007817246256747484735 ),
 .UNSPECIFIED. ) ;
#71342=CARTESIAN_POINT ( 'NONE',  ( 9.019230769230832223, -7.434744429011176159, 34.75000000000000711 ) ) ;
#71344=ORIENTED_EDGE ( 'NONE', *, *, #15275, .F. ) ;
#71345=ORIENTED_EDGE ( 'NONE', *, *, #2969, .T. ) ;
#71346=CARTESIAN_POINT ( 'NONE',  ( -2.057692307692303046, -2.499999999999999556, 29.81604066197450109 ) ) ;
#71347=ORIENTED_EDGE ( 'NONE', *, *, #3112, .T. ) ;
#71348=FACE_BOUND ( 'NONE', #9927, .T. ) ;
#71349=DIRECTION ( 'NONE',  ( -0.000000000000000000, -0.5000000000000009992, -0.8660254037844380415 ) ) ;
#71350=CARTESIAN_POINT ( 'NONE',  ( -14.53117723225663838, -6.716662450894489211, 34.94144148231605840 ) ) ;
#71351=ORIENTED_EDGE ( 'NONE', *, *, #13640, .F. ) ;
#71352=CARTESIAN_POINT ( 'NONE',  ( -14.30769230769242917, -8.656820664282941280, 34.87096338111179961 ) ) ;
#71353=CARTESIAN_POINT ( 'NONE',  ( 5.076923076922953193, -8.656820664282941280, 34.87096338111179961 ) ) ;
#71354=CARTESIAN_POINT ( 'NONE',  ( 1.134592160393929738, -3.520140089381497361, 33.17453946501458262 ) ) ;
#71355=EDGE_LOOP ( 'NONE', ( #58341, #44556 ) ) ;
#71356=CARTESIAN_POINT ( 'NONE',  ( 12.33084699487090319, -4.809359713505814149, 33.96456829005828837 ) ) ;
#71357=CARTESIAN_POINT ( 'NONE',  ( -16.82697755857493149, -2.587454068350149239, 30.68340429815432557 ) ) ;
#71358=ORIENTED_EDGE ( 'NONE', *, *, #19136, .T. ) ;
#71360=DIRECTION ( 'NONE',  ( 0.000000000000000000, -1.000000000000000000, 0.000000000000000000 ) ) ;
#71361=FACE_OUTER_BOUND ( 'NONE', #69261, .T. ) ;
#71362=CARTESIAN_POINT ( 'NONE',  ( -2.557715544985270206, -2.587272538249755449, 30.68239716806877837 ) ) ;
#71364=CARTESIAN_POINT ( 'NONE',  ( -18.06608341095587633, -6.386643153685126251, 34.62446782046654903 ) ) ;
#71365=VECTOR ( 'NONE', #12685, 999.9999999999998863 ) ;
#71366=FACE_BOUND ( 'NONE', #6177, .T. ) ;
#71369=CARTESIAN_POINT ( 'NONE',  ( -0.3310130233048174109, -8.630441415882550871, 34.87705825610312615 ) ) ;
#71370=CARTESIAN_POINT ( 'NONE',  ( 4.153846153846154188, -5.471508081941601098, 34.59228464037088457 ) ) ;
#71371=CARTESIAN_POINT ( 'NONE',  ( 8.769230769230768274, -2.721908614388771852, 31.22303859784724978 ) ) ;
#71372=CARTESIAN_POINT ( 'NONE',  ( 13.60804178353017768, -7.630147987733840509, 34.99859428049665411 ) ) ;
#71376=VERTEX_POINT ( 'NONE', #63662 ) ;
#71377=EDGE_CURVE ( 'NONE', #35045, #72305, #66372, .T. ) ;
#71378=CARTESIAN_POINT ( 'NONE',  ( -9.822454901745912181, -6.001485441113819874, 34.52039167877662607 ) ) ;
#71379=ORIENTED_EDGE ( 'NONE', *, *, #27533, .T. ) ;
#71380=CARTESIAN_POINT ( 'NONE',  ( -4.153846153846273204, -11.48612834414049644, 32.76840700105863391 ) ) ;
#71381=EDGE_CURVE ( 'NONE', #23361, #25915, #30951, .T. ) ;
#71382=VECTOR ( 'NONE', #38301, 1000.000000000000114 ) ;
#71383=ORIENTED_EDGE ( 'NONE', *, *, #38756, .T. ) ;
#71384=CARTESIAN_POINT ( 'NONE',  ( -15.23076923076922995, -12.10708131394839349, 31.69288490824020244 ) ) ;
#71387=CARTESIAN_POINT ( 'NONE',  ( 6.673100192134570285, -11.28823185664190376, 33.01397839955799896 ) ) ;
#71389=CARTESIAN_POINT ( 'NONE',  ( 13.38461538461538680, -1.367168528481310208, 33.57946703557072254 ) ) ;
#71391=CARTESIAN_POINT ( 'NONE',  ( -13.60810030917971858, -8.539481045369596401, 34.89627647299170832 ) ) ;
#71392=CARTESIAN_POINT ( 'NONE',  ( -13.63459212866397507, -12.01397095200674059, 32.43157075238190146 ) ) ;
#71395=CARTESIAN_POINT ( 'NONE',  ( 1.384615384615265343, -2.892918686052166066, 31.69288490824153470 ) ) ;
#71396=CARTESIAN_POINT ( 'NONE',  ( -2.176901866725358126, -11.93129842949671726, 32.56571108434900452 ) ) ;
#71398=DIRECTION ( 'NONE',  ( -0.000000000000000000, 0.8660254037844399289, -0.4999999999999980016 ) ) ;
#71400=ORIENTED_EDGE ( 'NONE', *, *, #69152, .T. ) ;
#71401=AXIS2_PLACEMENT_3D ( 'NONE', #37733, #65199, #51670 ) ;
#71402=CARTESIAN_POINT ( 'NONE',  ( 17.07692307692295586, -12.27809138561165270, 31.22303859784587132 ) ) ;
#71403=DIRECTION ( 'NONE',  ( -0.000000000000000000, 1.000000000000000000, 3.491481338843133355E-15 ) ) ;
#71404=CARTESIAN_POINT ( 'NONE',  ( 9.823099500132483897, -6.413143153341454017, 34.63066358083362672 ) ) ;
#71405=CARTESIAN_POINT ( 'NONE',  ( 17.99999999999987566, -10.90142922262034020, 33.41473453929536674 ) ) ;
#71406=CARTESIAN_POINT ( 'NONE',  ( 3.903822929624696680, -3.520140089381497361, 33.17453946501458262 ) ) ;
#71407=CARTESIAN_POINT ( 'NONE',  ( 2.057715576749954867, -12.17611988154120972, 31.52148481390971213 ) ) ;
#71408=AXIS2_PLACEMENT_3D ( 'NONE', #76138, #14446, #69394 ) ;
#71409=ORIENTED_EDGE ( 'NONE', *, *, #68437, .F. ) ;
#71411=ORIENTED_EDGE ( 'NONE', *, *, #80185, .T. ) ;
#71413=EDGE_LOOP ( 'NONE', ( #1658, #87597, #55608, #10874 ) ) ;
#71414=DIRECTION ( 'NONE',  ( -0.000000000000000000, -0.8660254037844399289, -0.4999999999999980016 ) ) ;
#71415=DIRECTION ( 'NONE',  ( -0.000000000000000000, -0.8660254037844397068, -0.4999999999999978906 ) ) ;
#71416=DIRECTION ( 'NONE',  ( -0.000000000000000000, 0.7660444431189791237, -0.6427876096865379196 ) ) ;
#71417=CARTESIAN_POINT ( 'NONE',  ( 1.634560902963529960, -11.86320923018887719, 32.19269448109604781 ) ) ;
#71418=CARTESIAN_POINT ( 'NONE',  ( 10.61538461538461675, -9.905515769479276145, 34.41647553114623292 ) ) ;
#71419=ORIENTED_EDGE ( 'NONE', *, *, #38859, .T. ) ;
#71421=DIRECTION ( 'NONE',  ( 0.000000000000000000, 0.9396926207859126468, -0.3420201433256571111 ) ) ;
#71422=ORIENTED_EDGE ( 'NONE', *, *, #29358, .T. ) ;
#71423=VECTOR ( 'NONE', #46594, 1000.000000000000227 ) ;
#71426=ADVANCED_FACE ( 'NONE', ( #11382 ), #39313, .F. ) ;
#71427=DIRECTION ( 'NONE',  ( -0.000000000000000000, -0.000000000000000000, -1.000000000000000000 ) ) ;
#71429=CIRCLE ( 'NONE', #35519, 0.2500000000000002220 ) ;
#71430=CARTESIAN_POINT ( 'NONE',  ( -10.83886955910856464, -5.113361153441934093, 34.14387501736622710 ) ) ;
#71431=CARTESIAN_POINT ( 'NONE',  ( 11.28848479441295005, -10.82459398097509329, 33.81372124010185587 ) ) ;
#71432=LINE ( 'NONE', #37208, #36782 ) ;
#71433=VECTOR ( 'NONE', #79471, 1000.000000000000114 ) ;
#71434=AXIS2_PLACEMENT_3D ( 'NONE', #75608, #67539, #5398 ) ;
#71436=EDGE_CURVE ( 'NONE', #31351, #13749, #62058, .T. ) ;
#71437=ORIENTED_EDGE ( 'NONE', *, *, #36963, .T. ) ;
#71439=ORIENTED_EDGE ( 'NONE', *, *, #76532, .F. ) ;
#71440=CARTESIAN_POINT ( 'NONE',  ( -14.17690186672535901, -2.295524264805589354, 30.44142389570982488 ) ) ;
#71441=VERTEX_POINT ( 'NONE', #4626 ) ;
#71442=DIRECTION ( 'NONE',  ( -0.000000000000000000, -0.8660254037844397068, -0.4999999999999978906 ) ) ;
#71443=CARTESIAN_POINT ( 'NONE',  ( 4.946775867484854317, -3.817052484675422797, 33.13202310037935661 ) ) ;
#71444=EDGE_CURVE ( 'NONE', #85483, #2529, #54493, .T. ) ;
#71446=CARTESIAN_POINT ( 'NONE',  ( -3.230769230769351186, -10.21337939537710326, 33.94971097300076224 ) ) ;
#71448=CARTESIAN_POINT ( 'NONE',  ( -15.16551409125639260, -12.51329471203373700, 31.30864560766537963 ) ) ;
#71449=ORIENTED_EDGE ( 'NONE', *, *, #47027, .T. ) ;
#71450=EDGE_CURVE ( 'NONE', #72338, #78537, #86169, .T. ) ;
#71451=DIRECTION ( 'NONE',  ( 0.000000000000000000, 0.6427876096865373645, -0.7660444431189797898 ) ) ;
#71452=CARTESIAN_POINT ( 'NONE',  ( 18.00000000000000000, -12.62096338111211580, 30.90682066428153263 ) ) ;
#71453=CARTESIAN_POINT ( 'NONE',  ( 10.61538461538461675, -3.513871655860378418, 32.76840700105978499 ) ) ;
#71454=CARTESIAN_POINT ( 'NONE',  ( -0.3307480205715097044, -11.37503395064541678, 33.29242100308974983 ) ) ;
#71456=VECTOR ( 'NONE', #62765, 1000.000000000000227 ) ;
#71457=CARTESIAN_POINT ( 'NONE',  ( 16.02369894440793630, -2.619462340734461048, 30.83744416345203021 ) ) ;
#71458=CARTESIAN_POINT ( 'NONE',  ( -0.3954711281883855900, -12.62096338111211757, 30.90682066428152908 ) ) ;
#71463=VECTOR ( 'NONE', #1822, 1000.000000000000114 ) ;
#71464=CARTESIAN_POINT ( 'NONE',  ( 7.146088274689772035, -2.758310577978207778, 31.33698337089303010 ) ) ;
#71465=CARTESIAN_POINT ( 'NONE',  ( 12.21153846153846168, -2.499999999999998668, 29.75000000000000355 ) ) ;
#71467=CARTESIAN_POINT ( 'NONE',  ( 2.307692307692309264, -13.88283147151868846, 33.14645433367849847 ) ) ;
#71468=CARTESIAN_POINT ( 'NONE',  ( -10.61538461538473577, -3.083524468854526912, 32.58852847137268327 ) ) ;
#71469=DIRECTION ( 'NONE',  ( -0.000000000000000000, 0.9396926207859092051, -0.3420201433256662704 ) ) ;
#71470=FACE_BOUND ( 'NONE', #85296, .T. ) ;
#71471=CARTESIAN_POINT ( 'NONE',  ( 13.25446817517716269, -12.27039167877662251, 31.24851455888617835 ) ) ;
#71472=FACE_OUTER_BOUND ( 'NONE', #45556, .T. ) ;
#71473=AXIS2_PLACEMENT_3D ( 'NONE', #69515, #62745, #26760 ) ;
#71474=CARTESIAN_POINT ( 'NONE',  ( 16.02315468717859304, -3.062553014421049991, 32.05460306192773601 ) ) ;
#71475=DIRECTION ( 'NONE',  ( 0.000000000000000000, 0.1736481776669267785, -0.9848077530122087975 ) ) ;
#71476=CARTESIAN_POINT ( 'NONE',  ( 0.4615384615384611755, -2.900454961884010974, 35.62045528018868623 ) ) ;
#71479=B_SPLINE_CURVE_WITH_KNOTS ( 'NONE', 3,
 ( #16122, #57986, #44456, #15686, #64289, #84597, #77813, #2590, #51200, #30080 ),
 .UNSPECIFIED., .F., .F.,
 ( 4, 2, 2, 2, 4 ),
 ( 0.000000000000000000, 0.0001954311564186876876, 0.0003908623128373753751, 0.0005862934692560630356, 0.0007817246256747507503 ),
 .UNSPECIFIED. ) ;
#71480=EDGE_CURVE ( 'NONE', #28929, #24412, #16841, .T. ) ;
#71481=EDGE_LOOP ( 'NONE', ( #16420, #23351 ) ) ;
#71482=CARTESIAN_POINT ( 'NONE',  ( -7.846153846153965716, -11.48612834414049644, 32.76840700105863391 ) ) ;
#71483=DIRECTION ( 'NONE',  ( -0.000000000000000000, 0.7660444431189791237, -0.6427876096865379196 ) ) ;
#71484=CARTESIAN_POINT ( 'NONE',  ( 0.4615384615384611200, -13.53365097954675988, 30.81389545987213552 ) ) ;
#71485=CARTESIAN_POINT ( 'NONE',  ( -9.915792636031639518, -10.81261337010820256, 33.49550067578627477 ) ) ;
#71486=CARTESIAN_POINT ( 'NONE',  ( 6.857806922520604864, -12.70778746994557551, 30.41441678777548319 ) ) ;
#71487=CARTESIAN_POINT ( 'NONE',  ( -5.299788499126715458, -2.501496062324911840, 29.88072118266895671 ) ) ;
#71489=CARTESIAN_POINT ( 'NONE',  ( -1.607443482250262567, -7.369209533119137845, 34.99857337881830688 ) ) ;
#71490=CYLINDRICAL_SURFACE ( 'NONE', #76260, 0.2500000000000002220 ) ;
#71491=CARTESIAN_POINT ( 'NONE',  ( -16.94613126909829148, -5.582136614379148654, 34.36778462344220486 ) ) ;
#71492=CARTESIAN_POINT ( 'NONE',  ( 10.39189969082028675, -6.716662450894489211, 34.94144148231605840 ) ) ;
#71493=CARTESIAN_POINT ( 'NONE',  ( 2.372885295986962628, -2.255955759149235629, 29.99999999999988631 ) ) ;
#71494=CARTESIAN_POINT ( 'NONE',  ( 5.142990410273152513, -8.164416787775445883, 34.95778746994558617 ) ) ;
#71497=CARTESIAN_POINT ( 'NONE',  ( -14.24162395668986747, -3.050289026998446840, 32.03036669348366416 ) ) ;
#71498=CARTESIAN_POINT ( 'NONE',  ( 17.07692307692307665, -2.486705287966279876, 31.30864560766543647 ) ) ;
#71500=DIRECTION ( 'NONE',  ( -0.000000000000000000, -0.5000000000000009992, -0.8660254037844380415 ) ) ;
#71504=CARTESIAN_POINT ( 'NONE',  ( 7.173022332454967120, -10.92531984108285670, 33.72920026020278073 ) ) ;
#71505=CARTESIAN_POINT ( 'NONE',  ( -5.143006487878958310, -2.538708090699994813, 30.37095296980875148 ) ) ;
#71506=VERTEX_POINT ( 'NONE', #52803 ) ;
#71507=CARTESIAN_POINT ( 'NONE',  ( -16.37733107841048152, -4.225889041578354544, 33.85425143139329407 ) ) ;
#71508=CARTESIAN_POINT ( 'NONE',  ( 10.61538461538449596, -11.48612834414049644, 32.76840700105863391 ) ) ;
#71509=ORIENTED_EDGE ( 'NONE', *, *, #87428, .T. ) ;
#71511=CARTESIAN_POINT ( 'NONE',  ( 16.94631342171898680, -7.722926974430166069, 34.99546784045485737 ) ) ;
#71512=FACE_OUTER_BOUND ( 'NONE', #1931, .T. ) ;
#71513=B_SPLINE_CURVE_WITH_KNOTS ( 'NONE', 3,
 ( #6397, #14025, #67206, #5507, #7275, #32975, #27096, #62211, #81170, #33852 ),
 .UNSPECIFIED., .F., .F.,
 ( 4, 2, 2, 2, 4 ),
 ( 0.0007817246336856284103, 0.0009771112958940092897, 0.001172497958102390169, 0.001367884620310771265, 0.001563271282519152145 ),
 .UNSPECIFIED. ) ;
#71514=B_SPLINE_CURVE_WITH_KNOTS ( 'NONE', 3,
 ( #40568, #32912, #81109, #47752, #48188, #41441, #41001, #68034, #88325, #19838 ),
 .UNSPECIFIED., .F., .F.,
 ( 4, 2, 2, 2, 4 ),
 ( 0.000000000000000000, 0.0001954339857564075286, 0.0003908679715128150572, 0.0005863019572692225586, 0.0007817359430256301143 ),
 .UNSPECIFIED. ) ;
#71515=CARTESIAN_POINT ( 'NONE',  ( -13.60810032833933469, -3.236172620538810385, 32.36188796281390267 ) ) ;
#71516=EDGE_CURVE ( 'NONE', #51951, #62595, #68373, .T. ) ;
#71517=ORIENTED_EDGE ( 'NONE', *, *, #65887, .F. ) ;
#71518=B_SPLINE_CURVE_WITH_KNOTS ( 'NONE', 3,
 ( #6313, #47282, #13502, #74773, #20700, #33777, #61675, #68444, #40547, #75637 ),
 .UNSPECIFIED., .F., .F.,
 ( 4, 2, 2, 2, 4 ),
 ( 0.0007817359430256322827, 0.0009771253907249989254, 0.001172514838424365676, 0.001367904286123732428, 0.001563293733823099179 ),
 .UNSPECIFIED. ) ;
#71519=CYLINDRICAL_SURFACE ( 'NONE', #46178, 0.2499999999999986955 ) ;
#71520=B_SPLINE_CURVE_WITH_KNOTS ( 'NONE', 3,
 ( #25372, #30790, #46093, #52837, #73119, #10978, #86656, #57823, #44284, #45643 ),
 .UNSPECIFIED., .F., .F.,
 ( 4, 2, 2, 2, 4 ),
 ( 0.000000000000000000, 0.0001954311564186861968, 0.0003908623128373723936, 0.0005862934692560585904, 0.0007817246256747447872 ),
 .UNSPECIFIED. ) ;
#71521=B_SPLINE_CURVE_WITH_KNOTS ( 'NONE', 3,
 ( #88783, #60837, #73922, #6357, #61714, #13103, #33812, #27502, #60391, #20739 ),
 .UNSPECIFIED., .F., .F.,
 ( 4, 2, 2, 2, 4 ),
 ( 0.0007817246256747472808, 0.0009771112852218907189, 0.001172497944769034265, 0.001367884604316177595, 0.001563271263863321141 ),
 .UNSPECIFIED. ) ;
#71524=VERTEX_POINT ( 'NONE', #24888 ) ;
#71525=ORIENTED_EDGE ( 'NONE', *, *, #44843, .T. ) ;
#71526=EDGE_LOOP ( 'NONE', ( #38466, #37222, #37158, #87410 ) ) ;
#71527=VECTOR ( 'NONE', #7106, 1000.000000000000000 ) ;
#71528=CARTESIAN_POINT ( 'NONE',  ( -5.076923076923199218, -9.528491918059723176, 34.59228464037033035 ) ) ;
#71529=CARTESIAN_POINT ( 'NONE',  ( -3.099978789802277479, -2.845873456487966635, 32.17976146951972538 ) ) ;
#71530=ADVANCED_FACE ( 'NONE', ( #52358 ), #19907, .F. ) ;
#71533=CARTESIAN_POINT ( 'NONE',  ( 15.16549878480845948, -3.835265460703609186, 33.15142922261924241 ) ) ;
#71535=EDGE_CURVE ( 'NONE', #88762, #85190, #64054, .T. ) ;
#71536=AXIS2_PLACEMENT_3D ( 'NONE', #63428, #15699, #8941 ) ;
#71537=EDGE_LOOP ( 'NONE', ( #68933, #59446 ) ) ;
#71538=CARTESIAN_POINT ( 'NONE',  ( 4.153846153846030731, -8.656820664282941280, 34.87096338111179961 ) ) ;
#71539=ORIENTED_EDGE ( 'NONE', *, *, #8601, .T. ) ;
#71540=CARTESIAN_POINT ( 'NONE',  ( 17.29970261819148902, -5.114059244376869096, 34.14424750095245287 ) ) ;
#71541=B_SPLINE_CURVE_WITH_KNOTS ( 'NONE', 3,
 ( #71402, #16471, #85827, #44363, #37176, #2498, #30861, #50237, #38072, #84498 ),
 .UNSPECIFIED., .F., .F.,
 ( 4, 2, 2, 2, 4 ),
 ( 0.0007817359430256339090, 0.0009771253907250065148, 0.001172514838424371965, 0.001367904286123737632, 0.001563293733823103299 ),
 .UNSPECIFIED. ) ;
#71542=LINE ( 'NONE', #11184, #55131 ) ;
#71543=CARTESIAN_POINT ( 'NONE',  ( 13.38461538461526423, -10.33852847137269571, 34.16647553114546554 ) ) ;
#71545=EDGE_LOOP ( 'NONE', ( #76781, #72906 ) ) ;
#71546=CARTESIAN_POINT ( 'NONE',  ( 9.823098133274644539, -8.191423895709840863, 34.95447573519442130 ) ) ;
#71547=ORIENTED_EDGE ( 'NONE', *, *, #16946, .F. ) ;
#71548=LINE ( 'NONE', #85964, #53148 ) ;
#71549=ADVANCED_FACE ( 'NONE', ( #6413 ), #85832, .F. ) ;
#71550=CARTESIAN_POINT ( 'NONE',  ( -15.93106661257774270, -3.755027918224367767, 33.06320215134714857 ) ) ;
#71551=VERTEX_POINT ( 'NONE', #14042 ) ;
#71553=CARTESIAN_POINT ( 'NONE',  ( -7.846153846153965716, -4.481592998941358097, 33.73612834414048933 ) ) ;
#71554=CYLINDRICAL_SURFACE ( 'NONE', #52548, 0.2500000000000009437 ) ;
#71556=FACE_BOUND ( 'NONE', #38890, .T. ) ;
#71557=CARTESIAN_POINT ( 'NONE',  ( -9.469294848214294902, -4.026326845037962343, 33.68677907613344047 ) ) ;
#71558=CARTESIAN_POINT ( 'NONE',  ( 11.40831432902331954, -8.587444163452046197, 34.63053765926554206 ) ) ;
#71560=FACE_OUTER_BOUND ( 'NONE', #30013, .T. ) ;
#71561=CARTESIAN_POINT ( 'NONE',  ( 4.376858997939547358, -2.308499170217967134, 30.53291367094873721 ) ) ;
#71562=CARTESIAN_POINT ( 'NONE',  ( 8.703960768674448900, -9.528491918058357157, 34.59228464037090589 ) ) ;
#71563=DIRECTION ( 'NONE',  ( -0.000000000000000000, -0.6427876096865404731, -0.7660444431189771253 ) ) ;
#71564=ORIENTED_EDGE ( 'NONE', *, *, #60582, .T. ) ;
#71565=AXIS2_PLACEMENT_3D ( 'NONE', #11057, #87620, #65542 ) ;
#71566=CARTESIAN_POINT ( 'NONE',  ( 10.48523740594639619, -10.88202310037935661, 33.43294751532457099 ) ) ;
#71567=EDGE_LOOP ( 'NONE', ( #57447, #69393, #64970, #78859 ) ) ;
#71568=ORIENTED_EDGE ( 'NONE', *, *, #45103, .T. ) ;
#71569=CARTESIAN_POINT ( 'NONE',  ( -1.161835715637318023, -4.989023458446560255, 34.36081565061822118 ) ) ;
#71570=CARTESIAN_POINT ( 'NONE',  ( -5.933931648997562647, -12.10708131394839882, 31.69288490824020954 ) ) ;
#71571=CARTESIAN_POINT ( 'NONE',  ( 11.31553457955468645, -8.282780595021769443, 34.94152052738834868 ) ) ;
#71572=CARTESIAN_POINT ( 'NONE',  ( 14.30769230769231015, -3.937682226553329556, 33.60647404775216529 ) ) ;
#71573=DIRECTION ( 'NONE',  ( -0.000000000000000000, 0.5000000000000011102, -0.8660254037844381525 ) ) ;
#71574=CARTESIAN_POINT ( 'NONE',  ( 16.15384615384615330, -8.810774026931790459, 35.74407628777942847 ) ) ;
#71575=ORIENTED_EDGE ( 'NONE', *, *, #17249, .T. ) ;
#71576=DIRECTION ( 'NONE',  ( -1.000000000000000000, 0.000000000000000000, 0.000000000000000000 ) ) ;
#71577=CARTESIAN_POINT ( 'NONE',  ( 14.98074600654777377, -10.92453946501458795, 33.72985991061850086 ) ) ;
#71578=CARTESIAN_POINT ( 'NONE',  ( 13.38461538461570122, -2.255955759149395501, 30.00000000000324363 ) ) ;
#71580=B_SPLINE_CURVE_WITH_KNOTS ( 'NONE', 3,
 ( #6468, #27173, #74044, #61388, #88461, #54192, #14894, #67724, #88029, #82130 ),
 .UNSPECIFIED., .F., .F.,
 ( 4, 2, 2, 2, 4 ),
 ( 0.000000000000000000, 0.0001954339857564081249, 0.0003908679715128162498, 0.0005863019572692244018, 0.0007817359430256324996 ),
 .UNSPECIFIED. ) ;
#71583=ORIENTED_EDGE ( 'NONE', *, *, #12602, .T. ) ;
#71584=VERTEX_POINT ( 'NONE', #12271 ) ;
#71585=CARTESIAN_POINT ( 'NONE',  ( -7.912236225513981758, -11.35647404775217595, 33.31231777344666511 ) ) ;
#71586=VERTEX_POINT ( 'NONE', #34310 ) ;
#71587=CARTESIAN_POINT ( 'NONE',  ( -7.146003140593070846, -2.554751324335733820, 30.48935550225260727 ) ) ;
#71588=CARTESIAN_POINT ( 'NONE',  ( 18.22301135161285046, -5.667800583137506898, 34.40243808032445827 ) ) ;
#71589=CARTESIAN_POINT ( 'NONE',  ( -16.15384615384627409, -2.892918686052165622, 31.69288490824153470 ) ) ;
#71590=DIRECTION ( 'NONE',  ( 0.000000000000000000, 0.7660444431189807890, 0.6427876096865361433 ) ) ;
#71593=ORIENTED_EDGE ( 'NONE', *, *, #24163, .F. ) ;
#71595=CARTESIAN_POINT ( 'NONE',  ( -12.59168567097668401, -10.88202310037935661, 33.43294751532457099 ) ) ;
#71596=CARTESIAN_POINT ( 'NONE',  ( -1.134669866267242755, -9.272278438253398036, 34.42582936511637826 ) ) ;
#71597=EDGE_LOOP ( 'NONE', ( #46644, #42865, #42658, #67474 ) ) ;
#71598=LINE ( 'NONE', #9906, #25322 ) ;
#71599=CARTESIAN_POINT ( 'NONE',  ( -12.39547011053602432, -3.513871655860379306, 32.76840700105978499 ) ) ;
#71600=CARTESIAN_POINT ( 'NONE',  ( 15.29683656411930848, -2.833524468853757750, 32.15551576947925838 ) ) ;
#71601=CARTESIAN_POINT ( 'NONE',  ( 6.700149964170072359, -3.395401636524186362, 33.02366814457250399 ) ) ;
#71602=DIRECTION ( 'NONE',  ( 0.000000000000000000, 0.9396926207859126468, -0.3420201433256571111 ) ) ;
#71603=AXIS2_PLACEMENT_3D ( 'NONE', #29116, #22341, #34528 ) ;
#71604=CARTESIAN_POINT ( 'NONE',  ( -3.165513659493205179, -11.48612834413965977, 32.76840700105972815 ) ) ;
#71605=CARTESIAN_POINT ( 'NONE',  ( -2.980769230767794653, -7.500000000000155431, 34.75000000000007105 ) ) ;
#71607=EDGE_LOOP ( 'NONE', ( #84838, #55713, #68625, #12393 ) ) ;
#71608=CARTESIAN_POINT ( 'NONE',  ( -11.53846153846153655, -7.500000000000001776, 35.04278698407183867 ) ) ;
#71609=CARTESIAN_POINT ( 'NONE',  ( 8.834486340506792601, -11.94971097300157403, 32.03036669348361443 ) ) ;
#71610=B_SPLINE_CURVE_WITH_KNOTS ( 'NONE', 3,
 ( #37922, #3678, #58622, #73039, #38367, #78450, #86117, #24392, #16752, #18102 ),
 .UNSPECIFIED., .F., .F.,
 ( 4, 2, 2, 2, 4 ),
 ( 0.0007817246256747524850, 0.0009771112852218972241, 0.001172497944769042072, 0.001367884604316186702, 0.001563271263863331550 ),
 .UNSPECIFIED. ) ;
#71611=CARTESIAN_POINT ( 'NONE',  ( -17.07692307692307665, -4.661471528628507777, 34.16647553114623292 ) ) ;
#71613=B_SPLINE_CURVE_WITH_KNOTS ( 'NONE', 3,
 ( #35472, #54408, #27391, #82343, #81904, #13867, #78669, #43119, #9766, #30047 ),
 .UNSPECIFIED., .F., .F.,
 ( 4, 2, 2, 2, 4 ),
 ( 0.000000000000000000, 0.0001954339857564063360, 0.0003908679715128126719, 0.0005863019572692189808, 0.0007817359430256253438 ),
 .UNSPECIFIED. ) ;
#71614=CARTESIAN_POINT ( 'NONE',  ( -3.230769230769229949, -8.973038597847269315, 34.52809138561121927 ) ) ;
#71615=CARTESIAN_POINT ( 'NONE',  ( -17.14219352288385778, -2.625532179533445198, 30.86335684631481513 ) ) ;
#71616=ORIENTED_EDGE ( 'NONE', *, *, #76437, .F. ) ;
#71618=CARTESIAN_POINT ( 'NONE',  ( -1.253824943648434553, -12.35292014791297710, 31.75344720912887198 ) ) ;
#71619=ORIENTED_EDGE ( 'NONE', *, *, #36260, .T. ) ;
#71621=ORIENTED_EDGE ( 'NONE', *, *, #37373, .F. ) ;
#71622=VECTOR ( 'NONE', #80710, 1000.000000000000000 ) ;
#71623=CARTESIAN_POINT ( 'NONE',  ( 14.55774661933062752, -12.17597550085003810, 31.52189283813460463 ) ) ;
#71624=FACE_OUTER_BOUND ( 'NONE', #88836, .T. ) ;
#71625=CARTESIAN_POINT ( 'NONE',  ( -1.608100328339332030, -4.386631170607604879, 33.66268669641500111 ) ) ;
#71626=CARTESIAN_POINT ( 'NONE',  ( -14.30769230769230660, -11.69971097300155272, 32.46337939537588113 ) ) ;
#71627=ORIENTED_EDGE ( 'NONE', *, *, #45739, .F. ) ;
#71628=CARTESIAN_POINT ( 'NONE',  ( -6.700297254098854793, -6.717445702608402236, 34.94155399931962336 ) ) ;
#71630=EDGE_CURVE ( 'NONE', #23768, #37623, #27548, .T. ) ;
#71631=ORIENTED_EDGE ( 'NONE', *, *, #48973, .F. ) ;
#71632=CARTESIAN_POINT ( 'NONE',  ( 12.39545608217832573, -11.91647553114624181, 32.58852847137148245 ) ) ;
#71634=ORIENTED_EDGE ( 'NONE', *, *, #3655, .F. ) ;
#71635=AXIS2_PLACEMENT_3D ( 'NONE', #87182, #19584, #52475 ) ;
#71638=CARTESIAN_POINT ( 'NONE',  ( 16.15384615384615330, -3.886160181151819604, 36.00935417666054406 ) ) ;
#71639=FACE_OUTER_BOUND ( 'NONE', #82725, .T. ) ;
#71640=CARTESIAN_POINT ( 'NONE',  ( 0.4615384615384611200, -2.249999999999998668, 29.75000000000001776 ) ) ;
#71641=B_SPLINE_CURVE_WITH_KNOTS ( 'NONE', 3,
 ( #75577, #34600, #82799, #28738, #49446, #83236, #56201, #83691, #379, #75156 ),
 .UNSPECIFIED., .F., .F.,
 ( 4, 2, 2, 2, 4 ),
 ( 0.0007817359430256319575, 0.0009771253907249984917, 0.001172514838424365026, 0.001367904286123731343, 0.001563293733823097878 ),
 .UNSPECIFIED. ) ;
#71642=ORIENTED_EDGE ( 'NONE', *, *, #47068, .T. ) ;
#71643=ORIENTED_EDGE ( 'NONE', *, *, #49998, .F. ) ;
#71644=ADVANCED_FACE ( 'NONE', ( #67665 ), #88, .F. ) ;
#71645=FACE_BOUND ( 'NONE', #51554, .T. ) ;
#71646=ORIENTED_EDGE ( 'NONE', *, *, #66428, .F. ) ;
#71647=CARTESIAN_POINT ( 'NONE',  ( -8.069638770718176701, -5.827078755546623690, 34.72654668319379567 ) ) ;
#71648=ORIENTED_EDGE ( 'NONE', *, *, #7224, .F. ) ;
#71651=CARTESIAN_POINT ( 'NONE',  ( 13.63456090296352841, -10.76462480002816235, 33.53768742498949962 ) ) ;
#71652=CARTESIAN_POINT ( 'NONE',  ( -3.230769230769351186, -10.21337939537710326, 33.94971097300076224 ) ) ;
#71653=EDGE_LOOP ( 'NONE', ( #12976, #88614, #33039, #62761 ) ) ;
#71654=EDGE_LOOP ( 'NONE', ( #60442, #71383, #69446, #63011 ) ) ;
#71655=AXIS2_PLACEMENT_3D ( 'NONE', #3513, #23342, #34099 ) ;
#71657=CARTESIAN_POINT ( 'NONE',  ( -1.608100328339332252, -11.89387501736622710, 32.13663884655806413 ) ) ;
#71659=CARTESIAN_POINT ( 'NONE',  ( 2.373760658694747061, -4.098570777380720287, 33.41473453929635440 ) ) ;
#71660=EDGE_CURVE ( 'NONE', #72796, #38632, #65176, .T. ) ;
#71661=VECTOR ( 'NONE', #13719, 1000.000000000000227 ) ;
#71662=CARTESIAN_POINT ( 'NONE',  ( -8.069638789877794594, -2.599994579823203367, 30.74605699353653776 ) ) ;
#71663=EDGE_CURVE ( 'NONE', #86112, #47138, #54576, .T. ) ;
#71664=CARTESIAN_POINT ( 'NONE',  ( -2.437840277424004665, -12.50552854090298993, 31.33409797877408920 ) ) ;
#71665=FACE_BOUND ( 'NONE', #13924, .T. ) ;
#71667=ORIENTED_EDGE ( 'NONE', *, *, #77660, .F. ) ;
#71668=CARTESIAN_POINT ( 'NONE',  ( -1.607442077094388022, -7.369208160676172348, 34.74850200257122879 ) ) ;
#71670=CARTESIAN_POINT ( 'NONE',  ( -14.08491276642389245, -5.913360116392397892, 34.49180327182771322 ) ) ;
#71671=DIRECTION ( 'NONE',  ( 0.000000000000000000, 0.7660444431189822323, -0.6427876096865344779 ) ) ;
#71672=DIRECTION ( 'NONE',  ( 0.000000000000000000, 0.8660254037844377084, -0.5000000000000015543 ) ) ;
#71673=ORIENTED_EDGE ( 'NONE', *, *, #86940, .F. ) ;
#71674=CARTESIAN_POINT ( 'NONE',  ( -17.20707028636129721, -12.45813303252208648, 30.39737893381572675 ) ) ;
#71675=ORIENTED_EDGE ( 'NONE', *, *, #52594, .F. ) ;
#71676=EDGE_LOOP ( 'NONE', ( #3959, #49105, #33888, #72209 ) ) ;
#71677=B_SPLINE_CURVE_WITH_KNOTS ( 'NONE', 3,
 ( #52550, #11582, #74168, #53439, #67410, #18334, #80941, #12465, #81379, #80035 ),
 .UNSPECIFIED., .F., .F.,
 ( 4, 2, 2, 2, 4 ),
 ( 0.000000000000000000, 0.0001954311564186863865, 0.0003908623128373727731, 0.0005862934692560591325, 0.0007817246256747455461 ),
 .UNSPECIFIED. ) ;
#71678=CARTESIAN_POINT ( 'NONE',  ( -18.25000000000000711, -2.249999999999998668, 29.75000000000000355 ) ) ;
#71679=CARTESIAN_POINT ( 'NONE',  ( 6.000000000000001776, -3.050289026998446396, 32.03036669348365706 ) ) ;
#71680=CARTESIAN_POINT ( 'NONE',  ( 15.93036121012220541, -5.912607949931405038, 34.49155766932282319 ) ) ;
#71681=CARTESIAN_POINT ( 'NONE',  ( -4.153846153846152411, -4.098570777380720287, 33.41473453929634729 ) ) ;
#71682=CARTESIAN_POINT ( 'NONE',  ( -18.22292695890684655, -5.582147617184174848, 34.63737895849758530 ) ) ;
#71683=CARTESIAN_POINT ( 'NONE',  ( -2.557669038634660552, -9.943427161483782584, 34.11278801902876978 ) ) ;
#71684=ORIENTED_EDGE ( 'NONE', *, *, #81609, .T. ) ;
#71685=CARTESIAN_POINT ( 'NONE',  ( 17.07692307692307665, -5.557115091759785130, 34.35708131394839171 ) ) ;
#71686=CARTESIAN_POINT ( 'NONE',  ( -11.66915300512910214, -9.804603061927743113, 34.18744698557895845 ) ) ;
#71688=CARTESIAN_POINT ( 'NONE',  ( 14.37375964104238335, -2.486705287966280320, 31.30864560766543647 ) ) ;
#71689=VERTEX_POINT ( 'NONE', #39757 ) ;
#71690=AXIS2_PLACEMENT_3D ( 'NONE', #21519, #82795, #34597 ) ;
#71691=ORIENTED_EDGE ( 'NONE', *, *, #73716, .T. ) ;
#71692=FACE_BOUND ( 'NONE', #86812, .T. ) ;
#71693=ORIENTED_EDGE ( 'NONE', *, *, #35325, .T. ) ;
#71694=CARTESIAN_POINT ( 'NONE',  ( 7.622668902429900584, -2.847400154188068022, 31.58180166144859058 ) ) ;
#71695=CARTESIAN_POINT ( 'NONE',  ( -6.856907782114267214, -7.250054483168843156, 34.74374881642865631 ) ) ;
#71696=ORIENTED_EDGE ( 'NONE', *, *, #66343, .F. ) ;
#71697=CARTESIAN_POINT ( 'NONE',  ( 3.903822929624694904, -11.56360843649122216, 33.07473185843129926 ) ) ;
#71698=CARTESIAN_POINT ( 'NONE',  ( -10.68146802634049308, -6.386643153685125363, 34.62446782046654903 ) ) ;
#71699=CARTESIAN_POINT ( 'NONE',  ( 16.02369894440793630, -8.587444163452046197, 34.63053765926554206 ) ) ;
#71700=CARTESIAN_POINT ( 'NONE',  ( -1.134560964701931240, -4.074993327901524687, 33.72946981652012255 ) ) ;
#71702=CARTESIAN_POINT ( 'NONE',  ( -7.715362038329058869, -10.54018710029568595, 33.71981072465678864 ) ) ;
#71703=ORIENTED_EDGE ( 'NONE', *, *, #27948, .F. ) ;
#71706=CARTESIAN_POINT ( 'NONE',  ( -8.519176457592452678, -9.943054286541403997, 34.11300777759954883 ) ) ;
#71707=CARTESIAN_POINT ( 'NONE',  ( 15.23076923076923173, -4.661471528628507777, 34.16647553114623292 ) ) ;
#71708=CARTESIAN_POINT ( 'NONE',  ( 10.61538461538461675, -12.34228464037088635, 31.77849191805839268 ) ) ;
#71709=EDGE_CURVE ( 'NONE', #84346, #13650, #52259, .T. ) ;
#71710=CARTESIAN_POINT ( 'NONE',  ( -12.39547011053602432, -2.721908614388772296, 31.22303859784725333 ) ) ;
#71711=CARTESIAN_POINT ( 'NONE',  ( -14.37296230824862775, -8.656820664281498878, 34.87096338111211935 ) ) ;
#71712=CARTESIAN_POINT ( 'NONE',  ( 12.21151523731700550, -5.765609946408404518, 34.70566812827425451 ) ) ;
#71713=B_SPLINE_CURVE_WITH_KNOTS ( 'NONE', 3,
 ( #73031, #44199, #71686, #59063, #4571, #64925, #84785, #3231, #86106, #24381 ),
 .UNSPECIFIED., .F., .F.,
 ( 4, 2, 2, 2, 4 ),
 ( 0.000000000000000000, 0.0001954339857564090194, 0.0003908679715128180387, 0.0005863019572692270039, 0.0007817359430256360774 ),
 .UNSPECIFIED. ) ;
#71715=ORIENTED_EDGE ( 'NONE', *, *, #55855, .F. ) ;
#71716=CARTESIAN_POINT ( 'NONE',  ( 6.000000000000001776, -2.721908614388771852, 31.22303859784724978 ) ) ;
#71717=CARTESIAN_POINT ( 'NONE',  ( 6.000000000000001776, -1.129524287112498415, 32.06866353760679544 ) ) ;
#71718=VERTEX_POINT ( 'NONE', #84294 ) ;
#71719=ORIENTED_EDGE ( 'NONE', *, *, #105, .F. ) ;
#71720=CARTESIAN_POINT ( 'NONE',  ( -5.776987155906603277, -12.64618726649961289, 30.78989965857442712 ) ) ;
#71721=CARTESIAN_POINT ( 'NONE',  ( 11.31553457955469000, -4.762599654559228846, 34.23009711892697737 ) ) ;
#71722=DIRECTION ( 'NONE',  ( -0.000000000000000000, -0.3420201433256694346, -0.9396926207859080948 ) ) ;
#71723=EDGE_CURVE ( 'NONE', #31685, #27787, #6180, .T. ) ;
#71725=CARTESIAN_POINT ( 'NONE',  ( 5.076923076923075762, -1.790695186598648903, 34.54067556320373455 ) ) ;
#71726=DIRECTION ( 'NONE',  ( 0.000000000000000000, 0.9848077530122072432, -0.1736481776669354937 ) ) ;
#71727=VECTOR ( 'NONE', #22973, 1000.000000000000227 ) ;
#71728=DIRECTION ( 'NONE',  ( -0.000000000000000000, 0.1736481776669307198, -0.9848077530122080203 ) ) ;
#71729=ORIENTED_EDGE ( 'NONE', *, *, #56450, .T. ) ;
#71730=DIRECTION ( 'NONE',  ( -0.000000000000000000, 0.9396926207859092051, -0.3420201433256662704 ) ) ;
#71731=FACE_OUTER_BOUND ( 'NONE', #41680, .T. ) ;
#71732=AXIS2_PLACEMENT_3D ( 'NONE', #14771, #41352, #62489 ) ;
#71734=CARTESIAN_POINT ( 'NONE',  ( 2.177000841024748112, -3.530157926970578508, 32.79014554554150607 ) ) ;
#71735=EDGE_LOOP ( 'NONE', ( #19151, #38005, #1605, #20376 ) ) ;
#71737=EDGE_CURVE ( 'NONE', #66517, #48076, #50169, .T. ) ;
#71738=ORIENTED_EDGE ( 'NONE', *, *, #79781, .T. ) ;
#71739=CARTESIAN_POINT ( 'NONE',  ( -17.77698715590659972, -8.282913670948747864, 34.94150082978203642 ) ) ;
#71742=CARTESIAN_POINT ( 'NONE',  ( -4.153846153846274980, -12.16647553114689728, 32.15551576947799362 ) ) ;
#71744=ADVANCED_FACE ( 'NONE', ( #77079 ), #16260, .F. ) ;
#71747=CARTESIAN_POINT ( 'NONE',  ( -10.68065461594093435, -12.70778746994557551, 30.41441678777548319 ) ) ;
#71748=CARTESIAN_POINT ( 'NONE',  ( -9.442362282929646966, -3.520799739797214389, 33.17531984108286025 ) ) ;
#71749=ORIENTED_EDGE ( 'NONE', *, *, #51996, .F. ) ;
#71750=EDGE_CURVE ( 'NONE', #87879, #48963, #71193, .T. ) ;
#71751=CARTESIAN_POINT ( 'NONE',  ( -0.5916856709766827871, -8.587444163452046197, 34.63053765926554206 ) ) ;
#71752=ORIENTED_EDGE ( 'NONE', *, *, #23950, .F. ) ;
#71753=B_SPLINE_CURVE_WITH_KNOTS ( 'NONE', 3,
 ( #81599, #39730, #32962, #59537, #5937, #33410, #33843, #88374, #88815, #60872 ),
 .UNSPECIFIED., .F., .F.,
 ( 4, 2, 2, 2, 4 ),
 ( 0.0007817246256747460882, 0.0009771112852218900684, 0.001172497944769033832, 0.001367884604316177595, 0.001563271263863321575 ),
 .UNSPECIFIED. ) ;
#71755=FACE_OUTER_BOUND ( 'NONE', #1255, .T. ) ;
#71756=ADVANCED_FACE ( 'NONE', ( #50039 ), #1416, .F. ) ;
#71757=CARTESIAN_POINT ( 'NONE',  ( -16.94639763868943660, -3.625058011473227815, 33.29252011169590020 ) ) ;
#71759=EDGE_CURVE ( 'NONE', #22124, #79174, #76182, .T. ) ;
#71760=CARTESIAN_POINT ( 'NONE',  ( -9.692307692307814193, -8.656820664282941280, 34.87096338111179961 ) ) ;
#71761=CARTESIAN_POINT ( 'NONE',  ( -16.15384615384615330, -1.242168528481310874, 33.36296068462461051 ) ) ;
#71762=VERTEX_POINT ( 'NONE', #15827 ) ;
#71763=ORIENTED_EDGE ( 'NONE', *, *, #75535, .F. ) ;
#71764=ORIENTED_EDGE ( 'NONE', *, *, #15942, .F. ) ;
#71766=EDGE_CURVE ( 'NONE', #80242, #38437, #26589, .T. ) ;
#71768=CARTESIAN_POINT ( 'NONE',  ( -16.94639737515951339, -3.816742781228458448, 33.13167719472716044 ) ) ;
#71769=LINE ( 'NONE', #48959, #42474 ) ;
#71770=CYLINDRICAL_SURFACE ( 'NONE', #85402, 0.2500000000000008882 ) ;
#71771=CYLINDRICAL_SURFACE ( 'NONE', #2533, 0.2500000000000004996 ) ;
#71772=CARTESIAN_POINT ( 'NONE',  ( 0.5920641633020240491, -5.195472089885680766, 34.18748526763464923 ) ) ;
#71774=AXIS2_PLACEMENT_3D ( 'NONE', #81642, #5539, #20380 ) ;
#71775=EDGE_CURVE ( 'NONE', #50871, #85765, #56576, .T. ) ;
#71776=DIRECTION ( 'NONE',  ( 0.000000000000000000, 0.8660254037844377084, 0.5000000000000015543 ) ) ;
#71777=ADVANCED_FACE ( 'NONE', ( #45048 ), #18043, .F. ) ;
#71781=ORIENTED_EDGE ( 'NONE', *, *, #27758, .T. ) ;
#71784=ORIENTED_EDGE ( 'NONE', *, *, #27618, .T. ) ;
#71785=DIRECTION ( 'NONE',  ( -0.000000000000000000, -0.9396926207859093161, -0.3420201433256663259 ) ) ;
#71786=CARTESIAN_POINT ( 'NONE',  ( 10.61538461538449596, -9.442884908241554243, 34.35708131394783038 ) ) ;
#71787=AXIS2_PLACEMENT_3D ( 'NONE', #51104, #24096, #79502 ) ;
#71788=CARTESIAN_POINT ( 'NONE',  ( 1.450682717965462443, -4.661471528628508665, 34.16647553114624003 ) ) ;
#71789=CARTESIAN_POINT ( 'NONE',  ( -14.30769230769242739, -10.21337939537710326, 33.94971097300076224 ) ) ;
#71792=CARTESIAN_POINT ( 'NONE',  ( -17.30040800148741198, -11.60425143139329940, 33.02411095842164457 ) ) ;
#71793=VERTEX_POINT ( 'NONE', #4522 ) ;
#71794=FACE_BOUND ( 'NONE', #36444, .T. ) ;
#71795=CARTESIAN_POINT ( 'NONE',  ( 14.98079249982687777, -9.943427161483782584, 34.11278801902876978 ) ) ;
#71796=DIRECTION ( 'NONE',  ( -1.000000000000000000, 0.000000000000000000, 0.000000000000000000 ) ) ;
#71797=ORIENTED_EDGE ( 'NONE', *, *, #57702, .F. ) ;
#71798=EDGE_CURVE ( 'NONE', #26954, #57222, #47947, .T. ) ;
#71799=CARTESIAN_POINT ( 'NONE',  ( 14.30769230769231015, -2.721908614388771852, 31.22303859784724978 ) ) ;
#71800=CARTESIAN_POINT ( 'NONE',  ( 16.28437185560972011, -4.459921816937789885, 33.71989282347011851 ) ) ;
#71801=DIRECTION ( 'NONE',  ( 0.000000000000000000, -6.938893903907222067E-15, 1.000000000000000000 ) ) ;
#71802=VERTEX_POINT ( 'NONE', #23448 ) ;
#71803=CARTESIAN_POINT ( 'NONE',  ( -5.999999999999998224, -4.945431358278436385, 36.03766855953609394 ) ) ;
#71804=CARTESIAN_POINT ( 'NONE',  ( -16.85391172531022619, -2.554770724473668597, 30.48948780036025852 ) ) ;
#71805=ORIENTED_EDGE ( 'NONE', *, *, #9287, .F. ) ;
#71806=CARTESIAN_POINT ( 'NONE',  ( 8.096208266067300485, -11.47946981652013498, 33.17500667209847620 ) ) ;
#71807=CARTESIAN_POINT ( 'NONE',  ( 7.145856464345332171, -10.81320215134717344, 33.49497208177562868 ) ) ;
#71808=EDGE_LOOP ( 'NONE', ( #6455, #22464, #52242, #21476 ) ) ;
#71809=CYLINDRICAL_SURFACE ( 'NONE', #47302, 0.2499999999999979738 ) ;
#71810=CARTESIAN_POINT ( 'NONE',  ( -4.153846153846152411, -4.945431358278436385, 36.03766855953609394 ) ) ;
#71811=DIRECTION ( 'NONE',  ( 0.000000000000000000, 0.6427876096865373645, -0.7660444431189797898 ) ) ;
#71812=FACE_OUTER_BOUND ( 'NONE', #59567, .T. ) ;
#71813=CARTESIAN_POINT ( 'NONE',  ( -15.23076923076922995, -13.57706302396349152, 30.56769352161908060 ) ) ;
#71814=ADVANCED_FACE ( 'NONE', ( #51336 ), #52256, .F. ) ;
#71815=DIRECTION ( 'NONE',  ( -0.000000000000000000, 0.9848077530122085754, -0.1736481776669273613 ) ) ;
#71816=B_SPLINE_CURVE_WITH_KNOTS ( 'NONE', 3,
 ( #72535, #18048, #44156, #79751, #30660, #72987, #17147, #3187, #86519, #10845 ),
 .UNSPECIFIED., .F., .F.,
 ( 4, 2, 2, 2, 4 ),
 ( 0.0007817246256747453293, 0.0009771112852218889842, 0.001172497944769032531, 0.001367884604316176294, 0.001563271263863319840 ),
 .UNSPECIFIED. ) ;
#71818=CARTESIAN_POINT ( 'NONE',  ( 11.47270811014820779, -7.249945578846651806, 34.99404164642496795 ) ) ;
#71819=CARTESIAN_POINT ( 'NONE',  ( -16.02332045208259359, -11.93748526763465279, 32.05452791011430946 ) ) ;
#71820=LINE ( 'NONE', #60864, #61641 ) ;
#71821=CARTESIAN_POINT ( 'NONE',  ( 8.992242120843615183, -2.758310577978208666, 31.33698337089302299 ) ) ;
#71822=CARTESIAN_POINT ( 'NONE',  ( -2.557669051740897537, -5.643011162660950042, 34.66104346484419096 ) ) ;
#71825=ADVANCED_FACE ( 'NONE', ( #4061 ), #30223, .F. ) ;
#71826=CARTESIAN_POINT ( 'NONE',  ( 18.24994551834813805, -11.86320923018887541, 32.19269448109604781 ) ) ;
#71827=VERTEX_POINT ( 'NONE', #51794 ) ;
#71828=EDGE_CURVE ( 'NONE', #58400, #87066, #50902, .T. ) ;
#71830=ORIENTED_EDGE ( 'NONE', *, *, #27790, .T. ) ;
#71831=CARTESIAN_POINT ( 'NONE',  ( -13.31936024510254413, -2.379036618887895305, 30.90682066428158592 ) ) ;
#71832=EDGE_LOOP ( 'NONE', ( #13866, #60299 ) ) ;
#71833=LINE ( 'NONE', #9264, #61334 ) ;
#71835=FACE_OUTER_BOUND ( 'NONE', #40726, .T. ) ;
#71836=CARTESIAN_POINT ( 'NONE',  ( -4.853911725310227965, -2.758310577978207778, 31.33698337089303010 ) ) ;
#71837=CARTESIAN_POINT ( 'NONE',  ( 6.989144256427000990, -9.905515769479277921, 34.41647553114623292 ) ) ;
#71838=CARTESIAN_POINT ( 'NONE',  ( -18.00000000000000000, -11.16473453929635440, 33.15142922261927083 ) ) ;
#71839=EDGE_CURVE ( 'NONE', #26485, #50475, #13661, .T. ) ;
#71840=LINE ( 'NONE', #37611, #76295 ) ;
#71841=CARTESIAN_POINT ( 'NONE',  ( -7.715362038329064198, -2.729792928343270919, 31.24908615093345077 ) ) ;
#71842=CARTESIAN_POINT ( 'NONE',  ( 5.934729554039225974, -4.481592998940161721, 33.73612834413957984 ) ) ;
#71843=B_SPLINE_CURVE_WITH_KNOTS ( 'NONE', 3,
 ( #19538, #60964, #28071, #15006, #62727, #76702 ),
 .UNSPECIFIED., .F., .F.,
 ( 4, 2, 4 ),
 ( 0.0003909512603273880690, 0.0005862562993132132720, 0.0007815613382990384750 ),
 .UNSPECIFIED. ) ;
#71845=CARTESIAN_POINT ( 'NONE',  ( -11.53846153846153655, -12.78798330534102945, 29.74999999999997868 ) ) ;
#71846=CARTESIAN_POINT ( 'NONE',  ( -15.16470087976679437, -2.538708090699994813, 30.37095296980875503 ) ) ;
#71847=CARTESIAN_POINT ( 'NONE',  ( 10.48469401227430708, -5.496505350115501010, 34.60290016733514307 ) ) ;
#71850=ORIENTED_EDGE ( 'NONE', *, *, #7308, .F. ) ;
#71852=CARTESIAN_POINT ( 'NONE',  ( 11.60371710973756443, -6.026961402152789304, 34.52809138561124769 ) ) ;
#71853=CARTESIAN_POINT ( 'NONE',  ( 5.999999999999878320, -9.528491918059723176, 34.59228464037033035 ) ) ;
#71854=CARTESIAN_POINT ( 'NONE',  ( 18.13052570176355971, -10.88167719472716399, 33.43325721877153711 ) ) ;
#71855=EDGE_CURVE ( 'NONE', #85917, #31266, #29783, .T. ) ;
#71856=B_SPLINE_CURVE_WITH_KNOTS ( 'NONE', 3,
 ( #69791, #8099, #34231, #35570, #83764, #27037, #61693, #13, #27482, #64784 ),
 .UNSPECIFIED., .F., .F.,
 ( 4, 2, 2, 2, 4 ),
 ( 0.0007817246256747447872, 0.0009771112852218876831, 0.001172497944769030579, 0.001367884604316173475, 0.001563271263863316371 ),
 .UNSPECIFIED. ) ;
#71857=VECTOR ( 'NONE', #4015, 1000.000000000000000 ) ;
#71858=CARTESIAN_POINT ( 'NONE',  ( 8.638539302563211564, -11.71456829005830080, 32.44064028649416542 ) ) ;
#71859=CARTESIAN_POINT ( 'NONE',  ( 2.177000841024747224, -12.11776431015576172, 31.66791131148498906 ) ) ;
#71860=VECTOR ( 'NONE', #78933, 1000.000000000000227 ) ;
#71862=CARTESIAN_POINT ( 'NONE',  ( -10.36538461538467715, -7.565270000091922853, 34.99999999999999289 ) ) ;
#71863=ORIENTED_EDGE ( 'NONE', *, *, #44384, .T. ) ;
#71865=CARTESIAN_POINT ( 'NONE',  ( -9.442362282929646966, -2.986452184633680229, 32.43230066228895225 ) ) ;
#71866=CARTESIAN_POINT ( 'NONE',  ( -6.249976744048589161, -12.65889640711025521, 30.72598325615533454 ) ) ;
#71867=CARTESIAN_POINT ( 'NONE',  ( 16.21991450484859243, -2.721908614388772296, 31.22303859784725333 ) ) ;
#71868=CARTESIAN_POINT ( 'NONE',  ( 4.219101725122176738, -3.835265460703683349, 33.15142922261929925 ) ) ;
#71869=CARTESIAN_POINT ( 'NONE',  ( -18.00000000000000000, -13.49681301100524244, 30.80739993210377392 ) ) ;
#71870=ORIENTED_EDGE ( 'NONE', *, *, #8060, .T. ) ;
#71871=CARTESIAN_POINT ( 'NONE',  ( 8.899756470994336865, -3.816742781228458448, 33.13167719472716044 ) ) ;
#71872=ORIENTED_EDGE ( 'NONE', *, *, #9648, .F. ) ;
#71873=VERTEX_POINT ( 'NONE', #9939 ) ;
#71874=ADVANCED_FACE ( 'NONE', ( #30652 ), #58122, .F. ) ;
#71876=DIRECTION ( 'NONE',  ( 0.000000000000000000, 0.000000000000000000, 1.000000000000000000 ) ) ;
#71877=CARTESIAN_POINT ( 'NONE',  ( 16.37685750545900376, -12.39991518177334129, 30.74647679643404530 ) ) ;
#71878=B_SPLINE_CURVE_WITH_KNOTS ( 'NONE', 3,
 ( #17, #67589, #26597, #34235, #68035, #27926, #6338, #61251, #21161, #48189 ),
 .UNSPECIFIED., .F., .F.,
 ( 4, 2, 2, 2, 4 ),
 ( 0.000000000000000000, 0.0001954311564186876334, 0.0003908623128373752667, 0.0005862934692560629272, 0.0007817246256747505334 ),
 .UNSPECIFIED. ) ;
#71879=CARTESIAN_POINT ( 'NONE',  ( -13.38461538461538325, -13.75783147151868846, 33.36296068462461051 ) ) ;
#71880=EDGE_CURVE ( 'NONE', #18025, #66904, #72672, .T. ) ;
#71882=CARTESIAN_POINT ( 'NONE',  ( -16.82686876528476461, -3.136992222400443175, 32.19305428654138979 ) ) ;
#71883=ADVANCED_FACE ( 'NONE', ( #13057 ), #54029, .F. ) ;
#71884=CARTESIAN_POINT ( 'NONE',  ( -16.02305434602137169, -2.729792928343270031, 31.24908615093345432 ) ) ;
#71885=VERTEX_POINT ( 'NONE', #5417 ) ;
#71886=ORIENTED_EDGE ( 'NONE', *, *, #62086, .F. ) ;
#71888=VERTEX_POINT ( 'NONE', #5860 ) ;
#71889=CARTESIAN_POINT ( 'NONE',  ( -12.59168567097668223, -11.47017969459904130, 32.78971311882034456 ) ) ;
#71890=EDGE_LOOP ( 'NONE', ( #19436, #24164, #4992, #64304 ) ) ;
#71891=ADVANCED_FACE ( 'NONE', ( #68007 ), #35422, .F. ) ;
#71892=CYLINDRICAL_SURFACE ( 'NONE', #49309, 0.2499999999999997502 ) ;
#71893=CARTESIAN_POINT ( 'NONE',  ( 3.230769230769231726, -9.819645486525091727, 36.12317359536749706 ) ) ;
#71895=ORIENTED_EDGE ( 'NONE', *, *, #65155, .F. ) ;
#71896=EDGE_CURVE ( 'NONE', #63245, #87401, #42710, .T. ) ;
#71898=ORIENTED_EDGE ( 'NONE', *, *, #839, .T. ) ;
#71899=CARTESIAN_POINT ( 'NONE',  ( -13.38461538461538325, -11.35647404775217417, 33.31231777344666511 ) ) ;
#71900=CARTESIAN_POINT ( 'NONE',  ( 17.77707304109314634, -12.64616026154729411, 30.79003144601914244 ) ) ;
#71901=CARTESIAN_POINT ( 'NONE',  ( -15.10024379253558635, -3.068774925481847493, 32.56582465632704526 ) ) ;
#71902=DIRECTION ( 'NONE',  ( 0.000000000000000000, 0.1736481776669275834, 0.9848077530122086864 ) ) ;
#71904=CARTESIAN_POINT ( 'NONE',  ( -10.74553258511631171, -5.915902021225889484, 34.75552854090298638 ) ) ;
#71905=VECTOR ( 'NONE', #81996, 1000.000000000000114 ) ;
#71906=CARTESIAN_POINT ( 'NONE',  ( 15.90386942290380290, -2.564618984488975517, 30.55390908950641915 ) ) ;
#71907=CARTESIAN_POINT ( 'NONE',  ( -0.2387587925603949501, -12.69155399931963046, 30.53255429739158444 ) ) ;
#71908=ORIENTED_EDGE ( 'NONE', *, *, #10966, .F. ) ;
#71909=ADVANCED_FACE ( 'NONE', ( #26573 ), #42196, .F. ) ;
#71910=CARTESIAN_POINT ( 'NONE',  ( 1.384615384615386802, -13.87047571288749737, 32.06866353760679544 ) ) ;
#71911=CARTESIAN_POINT ( 'NONE',  ( 8.834486340506797930, -6.879047030191282275, 34.71129190930002295 ) ) ;
#71912=ORIENTED_EDGE ( 'NONE', *, *, #56819, .T. ) ;
#71914=CARTESIAN_POINT ( 'NONE',  ( -5.010854725920638408, -5.557115091759786019, 34.35708131394839882 ) ) ;
#71915=CARTESIAN_POINT ( 'NONE',  ( 3.480769230770666578, -7.500000000000155431, 34.75000000000007105 ) ) ;
#71917=CARTESIAN_POINT ( 'NONE',  ( 7.623227628637698317, -8.239355502252617924, 34.69524867566427417 ) ) ;
#71918=FACE_BOUND ( 'NONE', #49555, .T. ) ;
#71919=CARTESIAN_POINT ( 'NONE',  ( 12.39626846098214230, -10.33852847137145048, 34.16647553114627556 ) ) ;
#71920=CARTESIAN_POINT ( 'NONE',  ( -10.48454628489785279, -7.277220318596961057, 34.99547417642776992 ) ) ;
#71921=B_SPLINE_CURVE_WITH_KNOTS ( 'NONE', 3,
 ( #64838, #16658, #11247, #58523, #72048, #52218, #79708, #4489, #44562, #85574 ),
 .UNSPECIFIED., .F., .F.,
 ( 4, 2, 2, 2, 4 ),
 ( 0.000000000000000000, 0.0001954339857564083688, 0.0003908679715128167377, 0.0005863019572692250523, 0.0007817359430256334753 ),
 .UNSPECIFIED. ) ;
#71922=DIRECTION ( 'NONE',  ( 0.000000000000000000, 0.6427876096865368094, 0.7660444431189802339 ) ) ;
#71924=CARTESIAN_POINT ( 'NONE',  ( -11.53846153846166089, -11.06231777344772027, 33.60647404775119895 ) ) ;
#71925=CARTESIAN_POINT ( 'NONE',  ( 15.93036121012220541, -10.81261337010820256, 33.49550067578627477 ) ) ;
#71926=CARTESIAN_POINT ( 'NONE',  ( 1.384615384615701439, -2.255955759149395501, 30.00000000000324363 ) ) ;
#71928=B_SPLINE_CURVE_WITH_KNOTS ( 'NONE', 3,
 ( #87375, #18461, #61647, #45916, #61200, #19346, #11708, #53112, #39185, #74743 ),
 .UNSPECIFIED., .F., .F.,
 ( 4, 2, 2, 2, 4 ),
 ( 0.0007817246256747484735, 0.0009771112852218931041, 0.001172497944769037735, 0.001367884604316182365, 0.001563271263863326996 ),
 .UNSPECIFIED. ) ;
#71929=EDGE_CURVE ( 'NONE', #80088, #45538, #55594, .T. ) ;
#71930=VERTEX_POINT ( 'NONE', #88734 ) ;
#71931=FACE_OUTER_BOUND ( 'NONE', #60279, .T. ) ;
#71932=EDGE_CURVE ( 'NONE', #73377, #20451, #19367, .T. ) ;
#71933=CARTESIAN_POINT ( 'NONE',  ( -4.946397375159510723, -3.285477652293412820, 32.44071101563363158 ) ) ;
#71934=CYLINDRICAL_SURFACE ( 'NONE', #67569, 0.2500000000000002220 ) ;
#71936=CARTESIAN_POINT ( 'NONE',  ( -4.403822897894744237, -4.818429247618089661, 34.26397095200675125 ) ) ;
#71937=CARTESIAN_POINT ( 'NONE',  ( -16.85414340794500276, -8.540255544307068902, 34.89611431652622286 ) ) ;
#71939=DIRECTION ( 'NONE',  ( -0.000000000000000000, 0.3420201433256694346, -0.9396926207859080948 ) ) ;
#71940=DIRECTION ( 'NONE',  ( -0.000000000000000000, -0.1736481776669307198, -0.9848077530122080203 ) ) ;
#71941=EDGE_CURVE ( 'NONE', #86769, #69764, #1859, .T. ) ;
#71942=CARTESIAN_POINT ( 'NONE',  ( -7.623374177175779032, -10.23759521482555357, 34.22997729860117033 ) ) ;
#71943=CARTESIAN_POINT ( 'NONE',  ( 17.77707304109314634, -8.282780595021769443, 34.94152052738834868 ) ) ;
#71944=CARTESIAN_POINT ( 'NONE',  ( -8.769230769230768274, -9.584722331328613620, 36.20867863119891439 ) ) ;
#71945=CARTESIAN_POINT ( 'NONE',  ( 10.86538461538461675, -2.499999999999998668, 29.75000000000000355 ) ) ;
#71946=CARTESIAN_POINT ( 'NONE',  ( -6.250023224221458840, -12.07920672191015221, 32.31858351112116168 ) ) ;
#71947=EDGE_CURVE ( 'NONE', #20065, #28968, #82433, .T. ) ;
#71948=LINE ( 'NONE', #30519, #35584 ) ;
#71949=EDGE_LOOP ( 'NONE', ( #36192, #616 ) ) ;
#71951=CARTESIAN_POINT ( 'NONE',  ( -17.07692307692319744, -2.892918686052165622, 31.69288490824153470 ) ) ;
#71953=CARTESIAN_POINT ( 'NONE',  ( 0.4615384615384611200, -1.129524287112498415, 32.06866353760679544 ) ) ;
#71954=CARTESIAN_POINT ( 'NONE',  ( 3.453780582382080411, -11.76359900205217457, 32.36225158514719880 ) ) ;
#71955=ORIENTED_EDGE ( 'NONE', *, *, #81186, .T. ) ;
#71956=CARTESIAN_POINT ( 'NONE',  ( -6.792551484843277976, -10.31582465632705237, 34.18122507451815295 ) ) ;
#71957=CARTESIAN_POINT ( 'NONE',  ( -0.6844654204453104462, -12.64616026154729411, 30.79003144601913533 ) ) ;
#71958=CARTESIAN_POINT ( 'NONE',  ( 7.596130608860881317, -2.587272538249754117, 30.68239716806877837 ) ) ;
#71959=ORIENTED_EDGE ( 'NONE', *, *, #55203, .F. ) ;
#71960=CARTESIAN_POINT ( 'NONE',  ( 11.60452887181161508, -4.661471528628508665, 34.16647553114624003 ) ) ;
#71961=DIRECTION ( 'NONE',  ( -0.000000000000000000, -0.7660444431189791237, -0.6427876096865379196 ) ) ;
#71962=ADVANCED_FACE ( 'NONE', ( #52978 ), #3463, .F. ) ;
#71963=DIRECTION ( 'NONE',  ( 0.000000000000000000, -6.938893903907222067E-15, 1.000000000000000000 ) ) ;
#71964=CARTESIAN_POINT ( 'NONE',  ( -15.36132914438259434, -2.254533558242299396, 29.97296025877828285 ) ) ;
#71966=ORIENTED_EDGE ( 'NONE', *, *, #19148, .T. ) ;
#71967=B_SPLINE_CURVE_WITH_KNOTS ( 'NONE', 3,
 ( #17804, #11041, #11938, #45257, #66876, #4276, #72729, #37613, #71842, #65076 ),
 .UNSPECIFIED., .F., .F.,
 ( 4, 2, 2, 2, 4 ),
 ( 0.000000000000000000, 0.0001954339857564075828, 0.0003908679715128151656, 0.0005863019572692227755, 0.0007817359430256303312 ),
 .UNSPECIFIED. ) ;
#71968=CARTESIAN_POINT ( 'NONE',  ( -12.59222906464876957, -2.295517848115769421, 30.44137282052137294 ) ) ;
#71969=EDGE_CURVE ( 'NONE', #13360, #68144, #52095, .T. ) ;
#71970=CARTESIAN_POINT ( 'NONE',  ( 10.61538461538449418, -4.320704448113951379, 33.92786785259630022 ) ) ;
#71972=FACE_OUTER_BOUND ( 'NONE', #84083, .T. ) ;
#71973=ORIENTED_EDGE ( 'NONE', *, *, #85663, .T. ) ;
#71974=EDGE_LOOP ( 'NONE', ( #72676, #82123 ) ) ;
#71975=VERTEX_POINT ( 'NONE', #80022 ) ;
#71977=CARTESIAN_POINT ( 'NONE',  ( 3.361559671736179311, -2.295524264805589354, 30.44142389570982488 ) ) ;
#71978=CYLINDRICAL_SURFACE ( 'NONE', #71655, 0.2500000000000009437 ) ;
#71979=CARTESIAN_POINT ( 'NONE',  ( -2.980714810855777053, -8.346898887586323923, 34.93166121998716278 ) ) ;
#71980=AXIS2_PLACEMENT_3D ( 'NONE', #53896, #52554, #73284 ) ;
#71981=VECTOR ( 'NONE', #79115, 1000.000000000000227 ) ;
#71982=CARTESIAN_POINT ( 'NONE',  ( 15.23076923076923173, -3.513871655860378418, 32.76840700105978499 ) ) ;
#71984=ORIENTED_EDGE ( 'NONE', *, *, #10914, .T. ) ;
#71985=CARTESIAN_POINT ( 'NONE',  ( -1.161604033002534564, -4.887748414852792322, 34.01359900205216746 ) ) ;
#71986=VERTEX_POINT ( 'NONE', #30929 ) ;
#71987=LINE ( 'NONE', #30992, #7684 ) ;
#71988=CARTESIAN_POINT ( 'NONE',  ( -3.230769230769229949, -2.833524468853757305, 32.15551576947925838 ) ) ;
#71989=CARTESIAN_POINT ( 'NONE',  ( -13.31935981333936425, -12.46129190930001052, 30.37095296980870174 ) ) ;
#71990=ORIENTED_EDGE ( 'NONE', *, *, #58053, .T. ) ;
#71991=ORIENTED_EDGE ( 'NONE', *, *, #9770, .T. ) ;
#71992=EDGE_LOOP ( 'NONE', ( #24878, #47748 ) ) ;
#71993=CARTESIAN_POINT ( 'NONE',  ( 8.769230769230768274, -2.538708090699994813, 30.37095296980875503 ) ) ;
#71994=ORIENTED_EDGE ( 'NONE', *, *, #42981, .T. ) ;
#71996=CARTESIAN_POINT ( 'NONE',  ( -5.750054481651857508, -8.433404298154334455, 34.66254593164985920 ) ) ;
#71997=CARTESIAN_POINT ( 'NONE',  ( -5.207070286361298095, -10.19110544564092002, 33.96427741523702792 ) ) ;
#71998=VERTEX_POINT ( 'NONE', #65602 ) ;
#72000=VECTOR ( 'NONE', #6171, 1000.000000000000000 ) ;
#72001=CARTESIAN_POINT ( 'NONE',  ( 4.153846153846154188, -1.129524287112498415, 32.06866353760679544 ) ) ;
#72002=EDGE_CURVE ( 'NONE', #39482, #2976, #72367, .T. ) ;
#72003=DIRECTION ( 'NONE',  ( -0.000000000000000000, 0.1736481776669307198, -0.9848077530122080203 ) ) ;
#72004=FACE_BOUND ( 'NONE', #36929, .T. ) ;
#72005=CARTESIAN_POINT ( 'NONE',  ( -3.230769230769351186, -11.48612834414049644, 32.76840700105863391 ) ) ;
#72006=CARTESIAN_POINT ( 'NONE',  ( 9.823146110320458035, -7.277220443632450575, 34.74524770363009196 ) ) ;
#72007=LINE ( 'NONE', #84658, #69587 ) ;
#72008=CARTESIAN_POINT ( 'NONE',  ( 17.32692307692308020, -2.499999999999999556, 29.81604066197449754 ) ) ;
#72009=CARTESIAN_POINT ( 'NONE',  ( 9.822833394071258439, -3.285477652293413264, 32.44071101563363158 ) ) ;
#72010=CARTESIAN_POINT ( 'NONE',  ( 11.40777007179398161, -11.18331474514187995, 33.13161551792790505 ) ) ;
#72011=DIRECTION ( 'NONE',  ( -0.000000000000000000, 0.8660254037844397068, -0.4999999999999978906 ) ) ;
#72012=ORIENTED_EDGE ( 'NONE', *, *, #87519, .T. ) ;
#72013=CARTESIAN_POINT ( 'NONE',  ( -5.750054481651856619, -11.86320923018887541, 32.19269448109604781 ) ) ;
#72014=EDGE_LOOP ( 'NONE', ( #67498, #73125 ) ) ;
#72015=ORIENTED_EDGE ( 'NONE', *, *, #86418, .T. ) ;
#72016=DIRECTION ( 'NONE',  ( 0.000000000000000000, 0.000000000000000000, -1.000000000000000000 ) ) ;
#72017=CARTESIAN_POINT ( 'NONE',  ( 10.68063975489745232, -12.16647553114626490, 32.15551576947920864 ) ) ;
#72018=EDGE_CURVE ( 'NONE', #4532, #41328, #41578, .T. ) ;
#72019=CYLINDRICAL_SURFACE ( 'NONE', #77351, 0.2499999999999994726 ) ;
#72020=CARTESIAN_POINT ( 'NONE',  ( 2.530705151785702878, -2.308499170217967134, 30.53291367094873721 ) ) ;
#72021=CARTESIAN_POINT ( 'NONE',  ( -4.023320715612507037, -3.625058011473227815, 33.29252011169590020 ) ) ;
#72022=EDGE_LOOP ( 'NONE', ( #58250, #43988 ) ) ;
#72024=CARTESIAN_POINT ( 'NONE',  ( 6.792929713638702793, -3.817052484675422797, 33.13202310037935661 ) ) ;
#72026=AXIS2_PLACEMENT_3D ( 'NONE', #73140, #19087, #62275 ) ;
#72027=DIRECTION ( 'NONE',  ( -0.000000000000000000, 0.6427876096865404731, -0.7660444431189770143 ) ) ;
#72028=CARTESIAN_POINT ( 'NONE',  ( -14.98082382139119062, -10.92531984108285670, 33.72920026020278073 ) ) ;
#72031=EDGE_CURVE ( 'NONE', #13813, #50611, #28668, .T. ) ;
#72032=EDGE_LOOP ( 'NONE', ( #84915, #42849, #54496, #72530 ) ) ;
#72033=CARTESIAN_POINT ( 'NONE',  ( -14.53061926659915315, -4.762599654559228846, 34.23009711892697737 ) ) ;
#72034=ADVANCED_FACE ( 'NONE', ( #58853 ), #51630, .F. ) ;
#72035=ORIENTED_EDGE ( 'NONE', *, *, #75129, .T. ) ;
#72036=CARTESIAN_POINT ( 'NONE',  ( 7.846153846153846700, -6.343179335718451384, 34.87096338111211935 ) ) ;
#72037=CARTESIAN_POINT ( 'NONE',  ( -12.21159294319032362, -10.05730279482229683, 34.04704008940765902 ) ) ;
#72038=CARTESIAN_POINT ( 'NONE',  ( -16.15384615384627409, -5.219633306517616589, 34.19971097300220464 ) ) ;
#72039=CYLINDRICAL_SURFACE ( 'NONE', #44263, 0.2499999999999973355 ) ;
#72041=CARTESIAN_POINT ( 'NONE',  ( -13.60754160213153163, -8.239355502252617924, 34.69524867566427417 ) ) ;
#72042=ORIENTED_EDGE ( 'NONE', *, *, #49170, .F. ) ;
#72045=CARTESIAN_POINT ( 'NONE',  ( 5.076923076923075762, -1.466349020453238561, 30.81389545987213907 ) ) ;
#72046=EDGE_LOOP ( 'NONE', ( #62380, #57667 ) ) ;
#72048=CARTESIAN_POINT ( 'NONE',  ( 14.05771557674995265, -12.17611988154120972, 31.52148481390971213 ) ) ;
#72049=CARTESIAN_POINT ( 'NONE',  ( 2.084207363968360482, -3.236172620538810385, 32.36188796281390267 ) ) ;
#72050=CARTESIAN_POINT ( 'NONE',  ( 11.53846153846141576, -8.656820664282941280, 34.87096338111179961 ) ) ;
#72051=DIRECTION ( 'NONE',  ( -0.000000000000000000, -0.5000000000000009992, -0.8660254037844380415 ) ) ;
#72052=ADVANCED_FACE ( 'NONE', ( #86359 ), #78692, .F. ) ;
#72053=CARTESIAN_POINT ( 'NONE',  ( 7.780883845597525550, -3.643525952247789412, 33.31231777344662959 ) ) ;
#72057=B_SPLINE_CURVE_WITH_KNOTS ( 'NONE', 3,
 ( #66696, #81110, #19396, #59039, #79323, #46421, #3645, #24812, #58589, #10866 ),
 .UNSPECIFIED., .F., .F.,
 ( 4, 2, 2, 2, 4 ),
 ( 0.0007817246336856291692, 0.0009771112958940105907, 0.001172497958102391904, 0.001367884620310773434, 0.001563271282519154747 ),
 .UNSPECIFIED. ) ;
#72059=CARTESIAN_POINT ( 'NONE',  ( -13.16183571563731647, -10.23759521482555357, 34.22997729860117033 ) ) ;
#72060=CARTESIAN_POINT ( 'NONE',  ( -14.30769230769230660, -13.37000171582298513, 34.34916445242398453 ) ) ;
#72062=B_SPLINE_CURVE_WITH_KNOTS ( 'NONE', 3,
 ( #2046, #87044, #10476, #73061, #77261, #73516, #24413, #70510, #31173, #86592 ),
 .UNSPECIFIED., .F., .F.,
 ( 4, 2, 2, 2, 4 ),
 ( 0.000000000000000000, 0.0001954311564186876334, 0.0003908623128373752667, 0.0005862934692560629272, 0.0007817246256747505334 ),
 .UNSPECIFIED. ) ;
#72063=CARTESIAN_POINT ( 'NONE',  ( -13.44988583057615905, -12.46129190929999986, 30.37095296980880832 ) ) ;
#72064=CARTESIAN_POINT ( 'NONE',  ( 16.08857615328983925, -5.094484230520675894, 34.41647553114621161 ) ) ;
#72065=ORIENTED_EDGE ( 'NONE', *, *, #1363, .F. ) ;
#72067=CARTESIAN_POINT ( 'NONE',  ( -2.307692307692305711, -11.11383981884818262, 36.00935417666054406 ) ) ;
#72068=ADVANCED_FACE ( 'NONE', ( #37696 ), #61845, .F. ) ;
#72069=EDGE_LOOP ( 'NONE', ( #84725, #69901 ) ) ;
#72070=CARTESIAN_POINT ( 'NONE',  ( -3.903791733932698182, -2.544122305571457687, 31.48381861865059150 ) ) ;
#72071=ORIENTED_EDGE ( 'NONE', *, *, #19023, .T. ) ;
#72072=VECTOR ( 'NONE', #43065, 1000.000000000000000 ) ;
#72073=CARTESIAN_POINT ( 'NONE',  ( 17.86930853333243974, -6.413092428213692742, 34.63065189839063152 ) ) ;
#72075=EDGE_CURVE ( 'NONE', #23009, #30124, #56433, .T. ) ;
#72076=CARTESIAN_POINT ( 'NONE',  ( 3.930361210122202742, -3.754499324213721234, 33.06261337010820256 ) ) ;
#72077=CARTESIAN_POINT ( 'NONE',  ( -4.153846153846152411, -13.75783147151868846, 33.36296068462461051 ) ) ;
#72078=VERTEX_POINT ( 'NONE', #13670 ) ;
#72079=CARTESIAN_POINT ( 'NONE',  ( 0.4615384615384611200, -4.661471528628507777, 34.16647553114623292 ) ) ;
#72081=VERTEX_POINT ( 'NONE', #55096 ) ;
#72082=DIRECTION ( 'NONE',  ( 0.000000000000000000, 0.1736481776669275834, 0.9848077530122086864 ) ) ;
#72083=EDGE_CURVE ( 'NONE', #33177, #18739, #60882, .T. ) ;
#72084=B_SPLINE_CURVE_WITH_KNOTS ( 'NONE', 3,
 ( #21441, #89038, #27315, #12471, #74620, #68298, #13795, #5711, #40399, #54331 ),
 .UNSPECIFIED., .F., .F.,
 ( 4, 2, 2, 2, 4 ),
 ( 0.000000000000000000, 0.0001954339857564097241, 0.0003908679715128194482, 0.0005863019572692291723, 0.0007817359430256388964 ),
 .UNSPECIFIED. ) ;
#72085=ORIENTED_EDGE ( 'NONE', *, *, #74200, .F. ) ;
#72086=CARTESIAN_POINT ( 'NONE',  ( 12.21151523731700372, -12.07920672191015221, 32.31858351112116168 ) ) ;
#72087=DIRECTION ( 'NONE',  ( 0.000000000000000000, 0.9396926207859126468, -0.3420201433256571111 ) ) ;
#72088=ORIENTED_EDGE ( 'NONE', *, *, #40853, .T. ) ;
#72089=CARTESIAN_POINT ( 'NONE',  ( -11.53846153846153655, -2.900454961884010974, 35.62045528018868623 ) ) ;
#72090=CARTESIAN_POINT ( 'NONE',  ( 0.4615384615384611200, -3.886160181151819604, 36.00935417666054406 ) ) ;
#72091=CARTESIAN_POINT ( 'NONE',  ( 1.384615384615386802, -2.499999999999998668, 29.50000000000001066 ) ) ;
#72093=CARTESIAN_POINT ( 'NONE',  ( -11.53846153846166089, -3.643525952248795718, 33.31231777344771672 ) ) ;
#72094=EDGE_LOOP ( 'NONE', ( #7801, #6591, #9743, #34653, #26727, #72276 ) ) ;
#72095=ORIENTED_EDGE ( 'NONE', *, *, #3845, .F. ) ;
#72097=EDGE_LOOP ( 'NONE', ( #76137, #8156 ) ) ;
#72098=CYLINDRICAL_SURFACE ( 'NONE', #25702, 0.2500000000000002220 ) ;
#72100=CARTESIAN_POINT ( 'NONE',  ( -14.05774689831426372, -10.92531984108285670, 33.72920026020278073 ) ) ;
#72101=DIRECTION ( 'NONE',  ( -0.000000000000000000, 0.5000000000000011102, -0.8660254037844380415 ) ) ;
#72102=VERTEX_POINT ( 'NONE', #14115 ) ;
#72104=ORIENTED_EDGE ( 'NONE', *, *, #25655, .T. ) ;
#72105=VERTEX_POINT ( 'NONE', #82591 ) ;
#72106=CARTESIAN_POINT ( 'NONE',  ( -1.384615384615383471, -11.69971097300155272, 32.46337939537588113 ) ) ;
#72108=CARTESIAN_POINT ( 'NONE',  ( -10.36543909703647337, -9.272278438253398036, 34.42582936511637115 ) ) ;
#72109=DIRECTION ( 'NONE',  ( 0.000000000000000000, 0.3420201433256610524, 0.9396926207859113145 ) ) ;
#72110=CARTESIAN_POINT ( 'NONE',  ( -15.93106648486808119, -10.97394488606063589, 33.68653795673696294 ) ) ;
#72111=FACE_BOUND ( 'NONE', #26723, .T. ) ;
#72112=ORIENTED_EDGE ( 'NONE', *, *, #59124, .T. ) ;
#72113=CARTESIAN_POINT ( 'NONE',  ( 13.31934538405906387, -11.06231777344662781, 33.60647404775220082 ) ) ;
#72114=DIRECTION ( 'NONE',  ( -0.000000000000000000, 1.000000000000000000, -0.000000000000000000 ) ) ;
#72115=CARTESIAN_POINT ( 'NONE',  ( 13.38461538461538680, -8.120952969808772792, 34.71129190930000163 ) ) ;
#72116=CARTESIAN_POINT ( 'NONE',  ( 8.069165197766697162, -10.61302985866383963, 33.66295027996417843 ) ) ;
#72117=VERTEX_POINT ( 'NONE', #41587 ) ;
#72118=CARTESIAN_POINT ( 'NONE',  ( 9.692307692307695177, -2.538708090699994813, 30.37095296980875503 ) ) ;
#72119=ORIENTED_EDGE ( 'NONE', *, *, #74689, .F. ) ;
#72121=CARTESIAN_POINT ( 'NONE',  ( 10.61538461538461675, -12.37446782046654192, 30.86335684631486131 ) ) ;
#72122=CARTESIAN_POINT ( 'NONE',  ( -1.607542343522232686, -5.582147617184174848, 34.63737895849758530 ) ) ;
#72123=B_SPLINE_CURVE_WITH_KNOTS ( 'NONE', 3,
 ( #74561, #12415, #6982, #39899, #5653, #40336, #68246, #61038, #88540, #34456 ),
 .UNSPECIFIED., .F., .F.,
 ( 4, 2, 2, 2, 4 ),
 ( 0.0007817359430256333669, 0.0009771253907250056474, 0.001172514838424370881, 0.001367904286123736331, 0.001563293733823101564 ),
 .UNSPECIFIED. ) ;
#72124=VECTOR ( 'NONE', #9439, 1000.000000000000000 ) ;
#72125=CARTESIAN_POINT ( 'NONE',  ( 15.90386942290380290, -5.728515186090277211, 34.42611988154120439 ) ) ;
#72126=CARTESIAN_POINT ( 'NONE',  ( -2.242436736416282272, -12.27809138561124591, 31.22303859784720359 ) ) ;
#72127=CARTESIAN_POINT ( 'NONE',  ( 16.94644636880661537, -7.276988635370451597, 34.74523720219453793 ) ) ;
#72128=CARTESIAN_POINT ( 'NONE',  ( -12.21159294319032362, -4.336752205174649433, 33.62275283266504289 ) ) ;
#72129=VERTEX_POINT ( 'NONE', #21307 ) ;
#72131=CARTESIAN_POINT ( 'NONE',  ( -0.3962833220256234412, -3.643525952247865352, 33.31231777344670064 ) ) ;
#72132=CARTESIAN_POINT ( 'NONE',  ( 10.36536139116315880, -2.985938066672154445, 32.43141759479405550 ) ) ;
#72133=CARTESIAN_POINT ( 'NONE',  ( -4.023320452082586485, -3.816742781228458448, 33.13167719472716044 ) ) ;
#72134=VECTOR ( 'NONE', #37500, 1000.000000000000114 ) ;
#72135=EDGE_LOOP ( 'NONE', ( #68390, #69761 ) ) ;
#72137=FACE_BOUND ( 'NONE', #82679, .T. ) ;
#72138=EDGE_CURVE ( 'NONE', #1586, #40194, #27627, .T. ) ;
#72139=ORIENTED_EDGE ( 'NONE', *, *, #20394, .F. ) ;
#72140=CARTESIAN_POINT ( 'NONE',  ( 7.716006636715624367, -2.882441371585227063, 31.66841991370171527 ) ) ;
#72141=CARTESIAN_POINT ( 'NONE',  ( 4.946775107191377252, -3.069018819979302926, 32.56621877034667278 ) ) ;
#72143=CARTESIAN_POINT ( 'NONE',  ( -3.296039676730006640, -12.46129190929999986, 30.37095296980880832 ) ) ;
#72144=CARTESIAN_POINT ( 'NONE',  ( 6.673100192134569397, -10.66389620160130036, 33.62221079203477103 ) ) ;
#72146=CARTESIAN_POINT ( 'NONE',  ( -1.319360245102545681, -4.320704448112861584, 33.92786785259548310 ) ) ;
#72147=ORIENTED_EDGE ( 'NONE', *, *, #72660, .T. ) ;
#72150=CARTESIAN_POINT ( 'NONE',  ( 13.63466980452883526, -8.346898887586323923, 34.93166121998716278 ) ) ;
#72151=VERTEX_POINT ( 'NONE', #49233 ) ;
#72152=LINE ( 'NONE', #31622, #13833 ) ;
#72153=CARTESIAN_POINT ( 'NONE',  ( 9.692307692308007816, -2.255955759149395501, 30.00000000000324363 ) ) ;
#72154=CARTESIAN_POINT ( 'NONE',  ( -7.623374177175776367, -3.563462043263029067, 33.22394488606062879 ) ) ;
#72155=CARTESIAN_POINT ( 'NONE',  ( 10.48523664565292002, -12.50552854090298638, 31.33409797877408920 ) ) ;
#72156=LINE ( 'NONE', #84367, #18872 ) ;
#72157=ADVANCED_FACE ( 'NONE', ( #20866 ), #157, .F. ) ;
#72158=CARTESIAN_POINT ( 'NONE',  ( 6.130791807824786055, -2.729792928343270919, 31.24908615093345077 ) ) ;
#72161=VERTEX_POINT ( 'NONE', #69941 ) ;
#72162=CARTESIAN_POINT ( 'NONE',  ( 17.32686848630111953, -2.986452184633680229, 32.43230066228895225 ) ) ;
#72163=CARTESIAN_POINT ( 'NONE',  ( 13.45068271796546178, -12.62096338111211757, 30.90682066428152908 ) ) ;
#72164=CARTESIAN_POINT ( 'NONE',  ( -0.2114841499001463287, -4.943051570960393271, 34.04725096376908766 ) ) ;
#72165=AXIS2_PLACEMENT_3D ( 'NONE', #74134, #40358, #5232 ) ;
#72166=EDGE_LOOP ( 'NONE', ( #16947, #55031 ) ) ;
#72167=ORIENTED_EDGE ( 'NONE', *, *, #7372, .T. ) ;
#72169=CARTESIAN_POINT ( 'NONE',  ( 12.59206389977210705, -4.299079248970732792, 33.91157788607253565 ) ) ;
#72170=CARTESIAN_POINT ( 'NONE',  ( -4.946132635956126400, -12.62708834333097663, 30.88030960425257021 ) ) ;
#72171=VECTOR ( 'NONE', #2609, 1000.000000000000114 ) ;
#72172=DIRECTION ( 'NONE',  ( -0.000000000000000000, 0.9396926207859092051, -0.3420201433256662704 ) ) ;
#72173=CARTESIAN_POINT ( 'NONE',  ( 9.692307692307572609, -12.46129190930018460, 30.37095296980731973 ) ) ;
#72175=DIRECTION ( 'NONE',  ( -0.000000000000000000, 1.000000000000000000, -0.000000000000000000 ) ) ;
#72176=EDGE_LOOP ( 'NONE', ( #18371, #3846 ) ) ;
#72177=CARTESIAN_POINT ( 'NONE',  ( -4.088590582570128973, -6.026961402152789304, 34.52809138561124769 ) ) ;
#72178=EDGE_CURVE ( 'NONE', #26379, #73147, #76992, .T. ) ;
#72179=CARTESIAN_POINT ( 'NONE',  ( -1.514762594053604028, -6.852621066184267029, 34.70813303252209181 ) ) ;
#72181=CARTESIAN_POINT ( 'NONE',  ( 7.146089767170319185, -6.460100341425561332, 34.89618726649961644 ) ) ;
#72182=CARTESIAN_POINT ( 'NONE',  ( 2.057669070399343880, -3.711651800289232916, 33.01384336483936011 ) ) ;
#72183=ORIENTED_EDGE ( 'NONE', *, *, #15717, .T. ) ;
#72186=CARTESIAN_POINT ( 'NONE',  ( 12.21156171748987163, -9.234221910056348293, 34.70572697212741531 ) ) ;
#72188=CARTESIAN_POINT ( 'NONE',  ( -13.63461538461538325, -7.500000000000001776, 35.00000000000000000 ) ) ;
#72189=CARTESIAN_POINT ( 'NONE',  ( -10.61538461538461320, -3.050289026998446396, 32.03036669348365706 ) ) ;
#72190=EDGE_LOOP ( 'NONE', ( #81100, #60592, #53128, #56346 ) ) ;
#72191=CARTESIAN_POINT ( 'NONE',  ( -2.438382910802613157, -6.369640206132550553, 34.87707690430378449 ) ) ;
#72192=CARTESIAN_POINT ( 'NONE',  ( 10.39245839786846659, -3.586966769969701208, 32.86292498521069660 ) ) ;
#72195=ORIENTED_EDGE ( 'NONE', *, *, #785, .T. ) ;
#72196=FACE_OUTER_BOUND ( 'NONE', #48229, .T. ) ;
#72197=EDGE_LOOP ( 'NONE', ( #45041, #27956, #4653, #85314 ) ) ;
#72198=AXIS2_PLACEMENT_3D ( 'NONE', #51000, #57782, #58660 ) ;
#72200=DIRECTION ( 'NONE',  ( 0.000000000000000000, 0.9396926207859126468, 0.3420201433256571111 ) ) ;
#72201=CARTESIAN_POINT ( 'NONE',  ( -3.480745961711584346, -12.17611988154120972, 31.52148481390971213 ) ) ;
#72202=CARTESIAN_POINT ( 'NONE',  ( 7.846153846153846700, -12.34228464037088635, 31.77849191805839268 ) ) ;
#72203=CARTESIAN_POINT ( 'NONE',  ( -6.223484943723948781, -4.386631170607603991, 33.66268669641500111 ) ) ;
#72204=CARTESIAN_POINT ( 'NONE',  ( 12.52679403281448245, -10.21337939537593620, 33.94971097300152252 ) ) ;
#72205=EDGE_LOOP ( 'NONE', ( #77947, #30280 ) ) ;
#72206=EDGE_LOOP ( 'NONE', ( #56513, #71258, #54722, #22918 ) ) ;
#72207=VERTEX_POINT ( 'NONE', #54642 ) ;
#72209=ORIENTED_EDGE ( 'NONE', *, *, #65322, .F. ) ;
#72210=ORIENTED_EDGE ( 'NONE', *, *, #37589, .T. ) ;
#72211=CARTESIAN_POINT ( 'NONE',  ( -1.319359813339359366, -3.300289026998475705, 32.46337939537591666 ) ) ;
#72213=CARTESIAN_POINT ( 'NONE',  ( -2.057637996053991447, -3.136992222400443175, 32.19305428654138979 ) ) ;
#72214=B_SPLINE_CURVE_WITH_KNOTS ( 'NONE', 3,
 ( #80661, #3637, #52273, #66230, #73892, #32452, #18503, #45961, #38324, #73451 ),
 .UNSPECIFIED., .F., .F.,
 ( 4, 2, 2, 2, 4 ),
 ( 0.0007817359430256293554, 0.0009771253907249974075, 0.001172514838424365460, 0.001367904286123733512, 0.001563293733823094625 ),
 .UNSPECIFIED. ) ;
#72215=CARTESIAN_POINT ( 'NONE',  ( -6.923076923076615152, -2.506253911140614576, 30.00000000000323297 ) ) ;
#72216=LINE ( 'NONE', #59596, #81108 ) ;
#72217=CARTESIAN_POINT ( 'NONE',  ( 7.780071466793708979, -12.62096338111211580, 30.90682066428152197 ) ) ;
#72218=B_SPLINE_CURVE_WITH_KNOTS ( 'NONE', 3,
 ( #78490, #17695, #70871, #58217, #23984, #85708, #78940, #17238, #10493, #9172 ),
 .UNSPECIFIED., .F., .F.,
 ( 4, 2, 2, 2, 4 ),
 ( 0.000000000000000000, 0.0001954339881912783015, 0.0003908679763825566029, 0.0005863019645738348773, 0.0007817359527651132059 ),
 .UNSPECIFIED. ) ;
#72220=CARTESIAN_POINT ( 'NONE',  ( 0.4615384615383396616, -5.219633306517616589, 34.19971097300220464 ) ) ;
#72222=B_SPLINE_CURVE_WITH_KNOTS ( 'NONE', 3,
 ( #30606, #37812, #29738, #9026, #16648, #58079, #78347, #86007, #51747, #78795 ),
 .UNSPECIFIED., .F., .F.,
 ( 4, 2, 2, 2, 4 ),
 ( 0.000000000000000000, 0.0001954311564186872268, 0.0003908623128373744536, 0.0005862934692560616261, 0.0007817246256747489071 ),
 .UNSPECIFIED. ) ;
#72223=CARTESIAN_POINT ( 'NONE',  ( 4.153846153846154188, -13.87047571288749737, 32.06866353760679544 ) ) ;
#72224=DIRECTION ( 'NONE',  ( -0.000000000000000000, -0.7660444431189791237, -0.6427876096865379196 ) ) ;
#72225=CARTESIAN_POINT ( 'NONE',  ( -6.923076923076922462, -12.09954503811598769, 35.62045528018868623 ) ) ;
#72226=ORIENTED_EDGE ( 'NONE', *, *, #81810, .F. ) ;
#72228=EDGE_CURVE ( 'NONE', #23052, #60815, #20042, .T. ) ;
#72230=CARTESIAN_POINT ( 'NONE',  ( 0.3954560821783248414, -2.833524468853757305, 32.15551576947924417 ) ) ;
#72231=VERTEX_POINT ( 'NONE', #41149 ) ;
#72232=CARTESIAN_POINT ( 'NONE',  ( 6.700149964170075023, -11.43668979543635089, 33.22377378376089752 ) ) ;
#72233=CARTESIAN_POINT ( 'NONE',  ( -7.846153846153965716, -11.48612834414049644, 32.76840700105863391 ) ) ;
#72234=FACE_OUTER_BOUND ( 'NONE', #43915, .T. ) ;
#72236=EDGE_LOOP ( 'NONE', ( #81000, #47048, #70879, #15230 ) ) ;
#72238=CARTESIAN_POINT ( 'NONE',  ( -17.29985003582992320, -11.43668979543635089, 33.22377378376089752 ) ) ;
#72239=ORIENTED_EDGE ( 'NONE', *, *, #7836, .F. ) ;
#72240=FACE_BOUND ( 'NONE', #20133, .T. ) ;
#72241=DIRECTION ( 'NONE',  ( -0.000000000000000000, 1.000000000000000000, 3.491481338843133355E-15 ) ) ;
#72242=ADVANCED_FACE ( 'NONE', ( #44778 ), #72258, .F. ) ;
#72243=CARTESIAN_POINT ( 'NONE',  ( -14.37377468705243722, -6.343179335718451384, 34.87096338111212646 ) ) ;
#72245=CARTESIAN_POINT ( 'NONE',  ( 17.75002326905764605, -2.779195860258148798, 31.39871582349836743 ) ) ;
#72246=CARTESIAN_POINT ( 'NONE',  ( -4.826923076923076650, -2.499999999999998668, 29.75000000000000355 ) ) ;
#72247=CARTESIAN_POINT ( 'NONE',  ( 1.254467414883692733, -3.625366637846545448, 33.29286588640298561 ) ) ;
#72248=ORIENTED_EDGE ( 'NONE', *, *, #18820, .T. ) ;
#72249=ADVANCED_FACE ( 'NONE', ( #24071 ), #3802, .F. ) ;
#72250=CARTESIAN_POINT ( 'NONE',  ( 12.21151522424549896, -5.056417327199099532, 34.11270091957321426 ) ) ;
#72251=FACE_OUTER_BOUND ( 'NONE', #72094, .T. ) ;
#72252=ORIENTED_EDGE ( 'NONE', *, *, #11324, .F. ) ;
#72253=CARTESIAN_POINT ( 'NONE',  ( 5.777171902365124900, -7.369209533119140509, 34.99857337881830688 ) ) ;
#72254=CARTESIAN_POINT ( 'NONE',  ( -9.469528023329624844, -9.418065098278013636, 34.63729479722530158 ) ) ;
#72255=ORIENTED_EDGE ( 'NONE', *, *, #25243, .F. ) ;
#72256=CARTESIAN_POINT ( 'NONE',  ( 6.923076923076924238, -6.681629849574314051, 35.83090037661290239 ) ) ;
#72257=CARTESIAN_POINT ( 'NONE',  ( -15.23076923076922995, -2.833524468853757305, 32.15551576947925838 ) ) ;
#72258=PLANE ( 'NONE',  #39673 ) ;
#72260=FACE_OUTER_BOUND ( 'NONE', #51405, .T. ) ;
#72261=FACE_BOUND ( 'NONE', #79442, .T. ) ;
#72263=CARTESIAN_POINT ( 'NONE',  ( 2.373760658694747949, -9.780366693483667717, 34.19971097300155805 ) ) ;
#72264=B_SPLINE_CURVE_WITH_KNOTS ( 'NONE', 3,
 ( #65683, #61600, #74239, #27819, #68807, #48521, #60716, #67485, #21050, #5780 ),
 .UNSPECIFIED., .F., .F.,
 ( 4, 2, 2, 2, 4 ),
 ( 0.000000000000000000, 0.0001954311564186871184, 0.0003908623128373742367, 0.0005862934692560614093, 0.0007817246256747484735 ),
 .UNSPECIFIED. ) ;
#72265=ADVANCED_FACE ( 'NONE', ( #17320 ), #9670, .F. ) ;
#72266=CARTESIAN_POINT ( 'NONE',  ( 8.519230769230768274, -2.499999999999998668, 29.75000000000000355 ) ) ;
#72267=LINE ( 'NONE', #65053, #12724 ) ;
#72268=CARTESIAN_POINT ( 'NONE',  ( -10.61538461538461320, -8.120952969808772792, 34.71129190930000163 ) ) ;
#72270=VERTEX_POINT ( 'NONE', #3355 ) ;
#72272=ORIENTED_EDGE ( 'NONE', *, *, #75906, .F. ) ;
#72273=EDGE_CURVE ( 'NONE', #19537, #70678, #82363, .T. ) ;
#72274=EDGE_LOOP ( 'NONE', ( #70748, #70468 ) ) ;
#72276=ORIENTED_EDGE ( 'NONE', *, *, #62613, .T. ) ;
#72277=CARTESIAN_POINT ( 'NONE',  ( 1.515140822849029734, -12.15418822224088657, 32.17964115625579069 ) ) ;
#72279=FACE_OUTER_BOUND ( 'NONE', #12845, .T. ) ;
#72280=CARTESIAN_POINT ( 'NONE',  ( -16.15384615384627409, -6.879047030192662504, 34.71129190930017927 ) ) ;
#72282=DIRECTION ( 'NONE',  ( 0.000000000000000000, 0.8660254037844377084, -0.5000000000000015543 ) ) ;
#72283=CARTESIAN_POINT ( 'NONE',  ( -16.40382289789474157, -10.06842814019191401, 34.32929386961144758 ) ) ;
#72284=CARTESIAN_POINT ( 'NONE',  ( 0.5923289025054114809, -5.496552790871119143, 34.60292014791297532 ) ) ;
#72285=CARTESIAN_POINT ( 'NONE',  ( 0.4615384615383382183, -2.657715359629662544, 31.77849191805970364 ) ) ;
#72287=CARTESIAN_POINT ( 'NONE',  ( 18.13079044096695469, -11.37503395064541678, 33.29242100308974983 ) ) ;
#72289=EDGE_CURVE ( 'NONE', #36016, #86769, #86243, .T. ) ;
#72290=EDGE_CURVE ( 'NONE', #53160, #58504, #4887, .T. ) ;
#72291=FACE_OUTER_BOUND ( 'NONE', #57737, .T. ) ;
#72292=AXIS2_PLACEMENT_3D ( 'NONE', #62739, #83484, #35736 ) ;
#72295=EDGE_CURVE ( 'NONE', #57358, #68032, #39870, .T. ) ;
#72296=CARTESIAN_POINT ( 'NONE',  ( 7.846153846153846700, -1.117168528481311540, 33.14645433367849847 ) ) ;
#72297=CARTESIAN_POINT ( 'NONE',  ( 1.384615384615264011, -11.06231777344772027, 33.60647404775119895 ) ) ;
#72298=CARTESIAN_POINT ( 'NONE',  ( 16.21991348719623360, -12.34228464037088813, 31.77849191805839268 ) ) ;
#72299=CARTESIAN_POINT ( 'NONE',  ( 16.15384615384615330, -11.69971097300155272, 32.46337939537588113 ) ) ;
#72300=EDGE_CURVE ( 'NONE', #86068, #24853, #26429, .T. ) ;
#72303=CARTESIAN_POINT ( 'NONE',  ( -3.230769230769229949, -13.95598074871891292, 31.83374038241031911 ) ) ;
#72304=B_SPLINE_CURVE_WITH_KNOTS ( 'NONE', 3,
 ( #2195, #56704, #9408, #71540, #84201, #57588, #78297, #10296, #57148, #36006 ),
 .UNSPECIFIED., .F., .F.,
 ( 4, 2, 2, 2, 4 ),
 ( 0.0007817359430256285964, 0.0009771253907249948054, 0.001172514838424360906, 0.001367904286123727223, 0.001563293733823093324 ),
 .UNSPECIFIED. ) ;
#72305=VERTEX_POINT ( 'NONE', #59192 ) ;
#72306=CARTESIAN_POINT ( 'NONE',  ( 17.74997676270703550, -12.43535235679832596, 30.55408501211184813 ) ) ;
#72307=ORIENTED_EDGE ( 'NONE', *, *, #58318, .T. ) ;
#72310=CARTESIAN_POINT ( 'NONE',  ( -11.40767109749458541, -11.37503395064541678, 33.29242100308974273 ) ) ;
#72311=CARTESIAN_POINT ( 'NONE',  ( 9.823099500132485673, -12.11778462344221019, 31.66786338562085135 ) ) ;
#72312=CARTESIAN_POINT ( 'NONE',  ( 2.084766090176161324, -5.667676309546437530, 34.40238873228292249 ) ) ;
#72313=CARTESIAN_POINT ( 'NONE',  ( -13.38461538461550582, -3.300289026999228881, 32.46337939537708905 ) ) ;
#72314=EDGE_LOOP ( 'NONE', ( #15393, #26447, #52124, #30360 ) ) ;
#72315=VECTOR ( 'NONE', #47822, 1000.000000000000000 ) ;
#72317=VERTEX_POINT ( 'NONE', #87138 ) ;
#72319=VERTEX_POINT ( 'NONE', #65045 ) ;
#72320=CARTESIAN_POINT ( 'NONE',  ( 1.254468175177168909, -11.47017969459903952, 32.78971311882034456 ) ) ;
#72321=CARTESIAN_POINT ( 'NONE',  ( -0.3954711281883861451, -9.905515769479277921, 34.41647553114623292 ) ) ;
#72322=CARTESIAN_POINT ( 'NONE',  ( 8.769230769230645706, -5.941354392335915335, 34.76329471203413846 ) ) ;
#72323=B_SPLINE_CURVE_WITH_KNOTS ( 'NONE', 3,
 ( #35592, #14884, #1352, #63930, #22076, #49547, #77022, #15321, #42800, #43229 ),
 .UNSPECIFIED., .F., .F.,
 ( 4, 2, 2, 2, 4 ),
 ( 0.0007817246256747446788, 0.0009771112852218874663, 0.001172497944769030145, 0.001367884604316172825, 0.001563271263863315720 ),
 .UNSPECIFIED. ) ;
#72324=ADVANCED_FACE ( 'NONE', ( #58297 ), #85788, .F. ) ;
#72325=CARTESIAN_POINT ( 'NONE',  ( -15.09997742294444478, -3.062576670634119758, 32.05464942895959979 ) ) ;
#72326=CARTESIAN_POINT ( 'NONE',  ( -1.384615384615383471, -13.63283147151868846, 33.57946703557072254 ) ) ;
#72327=CYLINDRICAL_SURFACE ( 'NONE', #72470, 0.2499999999999986955 ) ;
#72329=VERTEX_POINT ( 'NONE', #25862 ) ;
#72331=EDGE_CURVE ( 'NONE', #88393, #34480, #73622, .T. ) ;
#72333=CARTESIAN_POINT ( 'NONE',  ( 15.29683758177167086, -5.557115091759786019, 34.35708131394839882 ) ) ;
#72334=VERTEX_POINT ( 'NONE', #47899 ) ;
#72335=CARTESIAN_POINT ( 'NONE',  ( 1.318531973659505363, -9.780366693483667717, 34.19971097300155805 ) ) ;
#72336=CARTESIAN_POINT ( 'NONE',  ( 12.59232890250541281, -8.191423895709840863, 34.95447573519442130 ) ) ;
#72338=VERTEX_POINT ( 'NONE', #75379 ) ;
#72339=CARTESIAN_POINT ( 'NONE',  ( -1.384615384615506484, -2.657715359629662544, 31.77849191805970364 ) ) ;
#72340=ORIENTED_EDGE ( 'NONE', *, *, #71516, .F. ) ;
#72341=CARTESIAN_POINT ( 'NONE',  ( -13.45069776397551742, -11.35647404775217595, 33.31231777344666511 ) ) ;
#72343=AXIS2_PLACEMENT_3D ( 'NONE', #78558, #52418, #32598 ) ;
#72344=FACE_BOUND ( 'NONE', #20045, .T. ) ;
#72345=FACE_OUTER_BOUND ( 'NONE', #39499, .T. ) ;
#72347=VECTOR ( 'NONE', #86425, 1000.000000000000227 ) ;
#72348=EDGE_CURVE ( 'NONE', #53721, #32825, #66116, .T. ) ;
#72349=CARTESIAN_POINT ( 'NONE',  ( -0.5922290646487685661, -12.35290016733513951, 31.75349464988449455 ) ) ;
#72350=DIRECTION ( 'NONE',  ( -0.000000000000000000, -0.000000000000000000, -1.000000000000000000 ) ) ;
#72351=ORIENTED_EDGE ( 'NONE', *, *, #35663, .T. ) ;
#72352=CARTESIAN_POINT ( 'NONE',  ( -10.61538461538473399, -10.21337939537710326, 33.94971097300076224 ) ) ;
#72357=CARTESIAN_POINT ( 'NONE',  ( 17.01084069756293715, -10.67929555188718460, 33.92786785259543336 ) ) ;
#72359=CARTESIAN_POINT ( 'NONE',  ( 9.692307692307695177, -7.500000000000001776, 35.04278698407183867 ) ) ;
#72361=FACE_BOUND ( 'NONE', #50531, .T. ) ;
#72362=CARTESIAN_POINT ( 'NONE',  ( 5.207448515156721136, -5.915461855592777596, 34.75538340440931506 ) ) ;
#72363=CARTESIAN_POINT ( 'NONE',  ( 9.692307692307695177, -12.78798330534102945, 29.74999999999997868 ) ) ;
#72364=CARTESIAN_POINT ( 'NONE',  ( -18.25002322422145440, -8.475808217655755428, 34.90892951860618609 ) ) ;
#72365=CARTESIAN_POINT ( 'NONE',  ( 18.06525557127602610, -11.48612834413965977, 32.76840700105972815 ) ) ;
#72366=CARTESIAN_POINT ( 'NONE',  ( 0.6845513056318558442, -2.889357225399415086, 32.26129605718031002 ) ) ;
#72367=LINE ( 'NONE', #17435, #9563 ) ;
#72368=CYLINDRICAL_SURFACE ( 'NONE', #87903, 0.2500000000000004996 ) ;
#72371=CYLINDRICAL_SURFACE ( 'NONE', #80970, 0.2499999999999986955 ) ;
#72372=CARTESIAN_POINT ( 'NONE',  ( 7.976679284387491187, -10.31582465632705237, 34.18122507451815295 ) ) ;
#72373=CARTESIAN_POINT ( 'NONE',  ( -7.596153846153844924, -2.499999999999998668, 29.75000000000000355 ) ) ;
#72374=CARTESIAN_POINT ( 'NONE',  ( -9.757578138268467427, -10.90142922261923886, 33.41473453929638993 ) ) ;
#72375=DIRECTION ( 'NONE',  ( 0.000000000000000000, 0.3420201433256610524, 0.9396926207859113145 ) ) ;
#72376=CARTESIAN_POINT ( 'NONE',  ( 5.299702745901138101, -12.11081565061823717, 32.26097654155341843 ) ) ;
#72378=CARTESIAN_POINT ( 'NONE',  ( -2.373774687052440768, -3.322132147404559976, 32.92929555188719348 ) ) ;
#72379=DIRECTION ( 'NONE',  ( -0.000000000000000000, -0.000000000000000000, -1.000000000000000000 ) ) ;
#72381=CYLINDRICAL_SURFACE ( 'NONE', #10144, 0.2500000000000008882 ) ;
#72382=CARTESIAN_POINT ( 'NONE',  ( 4.946232473812766983, -9.084618155246140248, 34.75535874321725771 ) ) ;
#72383=CARTESIAN_POINT ( 'NONE',  ( 0.3308469948709032993, -11.18331474514187995, 33.13161551792790505 ) ) ;
#72384=FACE_OUTER_BOUND ( 'NONE', #56848, .T. ) ;
#72385=CARTESIAN_POINT ( 'NONE',  ( -11.53846153846153655, -13.37000171582298513, 34.34916445242398453 ) ) ;
#72386=EDGE_CURVE ( 'NONE', #70094, #22687, #43634, .T. ) ;
#72387=CARTESIAN_POINT ( 'NONE',  ( -1.253824943648435220, -11.93129842949671726, 32.56571108434900452 ) ) ;
#72388=ORIENTED_EDGE ( 'NONE', *, *, #14711, .F. ) ;
#72390=FACE_OUTER_BOUND ( 'NONE', #22174, .T. ) ;
#72392=EDGE_CURVE ( 'NONE', #35101, #7659, #2786, .T. ) ;
#72393=B_SPLINE_CURVE_WITH_KNOTS ( 'NONE', 3,
 ( #58878, #78256, #31864, #86378, #9804, #71946, #37269, #64734, #59322, #79604 ),
 .UNSPECIFIED., .F., .F.,
 ( 4, 2, 2, 2, 4 ),
 ( 0.000000000000000000, 0.0001954311564186861697, 0.0003908623128373723394, 0.0005862934692560584820, 0.0007817246256747446788 ),
 .UNSPECIFIED. ) ;
#72394=CARTESIAN_POINT ( 'NONE',  ( 9.692307692307695177, -13.57706302396349152, 30.56769352161908060 ) ) ;
#72395=CARTESIAN_POINT ( 'NONE',  ( -17.01085574357300345, -5.471508081941601098, 34.59228464037088457 ) ) ;
#72396=ORIENTED_EDGE ( 'NONE', *, *, #32625, .F. ) ;
#72397=CARTESIAN_POINT ( 'NONE',  ( -17.74994558008654622, -6.523592122091591783, 34.90882529074906415 ) ) ;
#72399=CARTESIAN_POINT ( 'NONE',  ( -7.846153846153844924, -12.34228464037088635, 31.77849191805839268 ) ) ;
#72400=ORIENTED_EDGE ( 'NONE', *, *, #12945, .T. ) ;
#72401=CARTESIAN_POINT ( 'NONE',  ( 6.856993512121043466, -3.050289026998445951, 32.03036669348365706 ) ) ;
#72402=CARTESIAN_POINT ( 'NONE',  ( 17.01160016143089848, -7.749976743299138882, 34.99404534957040624 ) ) ;
#72403=EDGE_CURVE ( 'NONE', #55151, #25698, #7118, .T. ) ;
#72405=CARTESIAN_POINT ( 'NONE',  ( -14.24243673641628227, -11.48612834413965977, 32.76840700105972815 ) ) ;
#72407=CARTESIAN_POINT ( 'NONE',  ( 2.307692307692309264, -12.10708131394839349, 31.69288490824020244 ) ) ;
#72408=DIRECTION ( 'NONE',  ( -0.000000000000000000, 0.5000000000000011102, -0.8660254037844380415 ) ) ;
#72409=VECTOR ( 'NONE', #53491, 1000.000000000000000 ) ;
#72410=CARTESIAN_POINT ( 'NONE',  ( 15.00784227186237807, -10.01117774369187252, 34.36070679894347535 ) ) ;
#72413=EDGE_CURVE ( 'NONE', #12765, #77653, #60078, .T. ) ;
#72414=ORIENTED_EDGE ( 'NONE', *, *, #51825, .T. ) ;
#72415=VECTOR ( 'NONE', #36785, 1000.000000000000000 ) ;
#72416=LINE ( 'NONE', #17929, #47207 ) ;
#72417=CARTESIAN_POINT ( 'NONE',  ( -2.980714810855777053, -2.920487667080175154, 32.31805714834170828 ) ) ;
#72418=EDGE_CURVE ( 'NONE', #70948, #76645, #17819, .T. ) ;
#72419=CARTESIAN_POINT ( 'NONE',  ( 13.31853197365950692, -11.16473453929635440, 33.15142922261925662 ) ) ;
#72420=CARTESIAN_POINT ( 'NONE',  ( 6.923076923076924238, -2.721908614388771852, 31.22303859784724978 ) ) ;
#72422=ORIENTED_EDGE ( 'NONE', *, *, #85056, .F. ) ;
#72423=EDGE_LOOP ( 'NONE', ( #50267, #41303, #20742, #22447 ) ) ;
#72425=ORIENTED_EDGE ( 'NONE', *, *, #61694, .T. ) ;
#72426=CARTESIAN_POINT ( 'NONE',  ( -14.08467946359890988, -11.43677907613344757, 33.22367315496202167 ) ) ;
#72427=EDGE_CURVE ( 'NONE', #7245, #22506, #74770, .T. ) ;
#72428=B_SPLINE_CURVE_WITH_KNOTS ( 'NONE', 3,
 ( #61405, #16769, #28983, #78033, #15014, #50551, #1498, #43800, #22209, #63184 ),
 .UNSPECIFIED., .F., .F.,
 ( 4, 2, 2, 2, 4 ),
 ( 0.000000000000000000, 0.0001954311564186863323, 0.0003908623128373726646, 0.0005862934692560590241, 0.0007817246256747453293 ),
 .UNSPECIFIED. ) ;
#72429=DIRECTION ( 'NONE',  ( -0.000000000000000000, 0.9848077530122085754, -0.1736481776669273613 ) ) ;
#72430=CARTESIAN_POINT ( 'NONE',  ( 10.48469314871705826, -11.18331474514187995, 33.13161551792790505 ) ) ;
#72431=CARTESIAN_POINT ( 'NONE',  ( -13.38461538461538325, -12.37446782046654192, 30.86335684631486131 ) ) ;
#72432=ORIENTED_EDGE ( 'NONE', *, *, #36789, .F. ) ;
#72433=ORIENTED_EDGE ( 'NONE', *, *, #20508, .F. ) ;
#72435=VECTOR ( 'NONE', #87112, 1000.000000000000114 ) ;
#72436=ORIENTED_EDGE ( 'NONE', *, *, #73193, .T. ) ;
#72438=ORIENTED_EDGE ( 'NONE', *, *, #6361, .T. ) ;
#72439=CARTESIAN_POINT ( 'NONE',  ( -10.61538461538429878, -2.255955759149395501, 30.00000000000324363 ) ) ;
#72441=ORIENTED_EDGE ( 'NONE', *, *, #52116, .F. ) ;
#72442=EDGE_CURVE ( 'NONE', #81428, #83740, #32792, .T. ) ;
#72443=CARTESIAN_POINT ( 'NONE',  ( -13.63459211555773720, -4.236021600441997492, 33.53823185664189310 ) ) ;
#72444=CYLINDRICAL_SURFACE ( 'NONE', #65214, 0.2499999999999973355 ) ;
#72445=DIRECTION ( 'NONE',  ( 0.000000000000000000, 0.7660444431189822323, -0.6427876096865344779 ) ) ;
#72446=FACE_BOUND ( 'NONE', #2735, .T. ) ;
#72447=DIRECTION ( 'NONE',  ( 0.000000000000000000, 0.000000000000000000, 1.000000000000000000 ) ) ;
#72448=CARTESIAN_POINT ( 'NONE',  ( -4.283993363284377409, -12.27039167877662251, 31.24851455888617835 ) ) ;
#72449=CYLINDRICAL_SURFACE ( 'NONE', #48044, 0.2500000000000004996 ) ;
#72450=CARTESIAN_POINT ( 'NONE',  ( 3.480823650682684178, -3.435999193479609470, 33.07426656108011542 ) ) ;
#72451=CARTESIAN_POINT ( 'NONE',  ( 9.915087233576103998, -3.236590943229499029, 32.36255958852954251 ) ) ;
#72452=CARTESIAN_POINT ( 'NONE',  ( -7.912237257109728361, -3.050289026998445951, 32.03036669348365706 ) ) ;
#72453=CARTESIAN_POINT ( 'NONE',  ( 5.076923076922954969, -2.625532179533778709, 30.86335684631627174 ) ) ;
#72454=ORIENTED_EDGE ( 'NONE', *, *, #47288, .F. ) ;
#72455=DIRECTION ( 'NONE',  ( 0.000000000000000000, 0.1736481776669267785, -0.9848077530122087975 ) ) ;
#72456=DIRECTION ( 'NONE',  ( -0.000000000000000000, -0.5000000000000009992, -0.8660254037844380415 ) ) ;
#72457=ORIENTED_EDGE ( 'NONE', *, *, #45066, .F. ) ;
#72458=EDGE_CURVE ( 'NONE', #47909, #64420, #87702, .T. ) ;
#72459=ORIENTED_EDGE ( 'NONE', *, *, #16147, .F. ) ;
#72460=B_SPLINE_CURVE_WITH_KNOTS ( 'NONE', 3,
 ( #32531, #10937, #72629, #73079, #65864, #25784, #44700, #65430, #60448, #11832 ),
 .UNSPECIFIED., .F., .F.,
 ( 4, 2, 2, 2, 4 ),
 ( 0.000000000000000000, 0.0001954311564186861426, 0.0003908623128373722852, 0.0005862934692560583735, 0.0007817246256747445703 ),
 .UNSPECIFIED. ) ;
#72461=DIRECTION ( 'NONE',  ( 0.000000000000000000, -6.938893903907222067E-15, 1.000000000000000000 ) ) ;
#72462=CARTESIAN_POINT ( 'NONE',  ( 1.384615384615265343, -10.90142922262034020, 33.41473453929536674 ) ) ;
#72463=ADVANCED_FACE ( 'NONE', ( #50106 ), #28076, .F. ) ;
#72464=B_SPLINE_CURVE_WITH_KNOTS ( 'NONE', 3,
 ( #22905, #64323, #30112, #37750, #23345, #1308, #44050, #22468, #84631, #56259 ),
 .UNSPECIFIED., .F., .F.,
 ( 4, 2, 2, 2, 4 ),
 ( 0.0007817246256747517261, 0.0009771112852218961399, 0.001172497944769040771, 0.001367884604316185401, 0.001563271263863329815 ),
 .UNSPECIFIED. ) ;
#72465=CARTESIAN_POINT ( 'NONE',  ( 11.47237915910140416, -8.164416787775445883, 34.95778746994557906 ) ) ;
#72466=CARTESIAN_POINT ( 'NONE',  ( -1.384615384615505151, -5.219633306517616589, 34.19971097300220464 ) ) ;
#72467=CARTESIAN_POINT ( 'NONE',  ( 12.46153846153846168, -12.09954503811598769, 35.62045528018868623 ) ) ;
#72468=ORIENTED_EDGE ( 'NONE', *, *, #25569, .F. ) ;
#72469=DIRECTION ( 'NONE',  ( 0.000000000000000000, 0.6427876096865373645, -0.7660444431189797898 ) ) ;
#72470=AXIS2_PLACEMENT_3D ( 'NONE', #73685, #78645, #10637 ) ;
#72471=DIRECTION ( 'NONE',  ( -0.000000000000000000, -0.9848077530122086864, -0.1736481776669273613 ) ) ;
#72472=CARTESIAN_POINT ( 'NONE',  ( 6.857806477116148436, -3.835265460703609186, 33.15142922261924241 ) ) ;
#72473=CARTESIAN_POINT ( 'NONE',  ( -1.384615384615383471, -9.905515769479276145, 34.41647553114623292 ) ) ;
#72474=CARTESIAN_POINT ( 'NONE',  ( 24.00000000000000000, -5.499999999999981348, 27.25000000000000000 ) ) ;
#72475=CARTESIAN_POINT ( 'NONE',  ( -1.384615384615383471, -1.629998284177014645, 34.34916445242399163 ) ) ;
#72477=ORIENTED_EDGE ( 'NONE', *, *, #34818, .F. ) ;
#72478=VECTOR ( 'NONE', #72408, 1000.000000000000114 ) ;
#72479=VERTEX_POINT ( 'NONE', #20869 ) ;
#72480=AXIS2_PLACEMENT_3D ( 'NONE', #30474, #85425, #63819 ) ;
#72481=CARTESIAN_POINT ( 'NONE',  ( 9.692307692307695177, -9.058645607665452459, 34.76329471203371924 ) ) ;
#72482=CARTESIAN_POINT ( 'NONE',  ( -18.13061035962451584, -7.722926236386454590, 34.74524107206102030 ) ) ;
#72484=CARTESIAN_POINT ( 'NONE',  ( -16.21992956480203318, -4.786620604624113540, 33.94971097300155805 ) ) ;
#72485=CARTESIAN_POINT ( 'NONE',  ( -0.7115616857599200706, -12.07920672191015221, 32.31858351112116168 ) ) ;
#72488=DIRECTION ( 'NONE',  ( -0.000000000000000000, 0.3420201433256694901, -0.9396926207859082059 ) ) ;
#72489=VERTEX_POINT ( 'NONE', #83025 ) ;
#72490=FACE_OUTER_BOUND ( 'NONE', #78442, .T. ) ;
#72491=CARTESIAN_POINT ( 'NONE',  ( 5.999999999999878320, -10.33852847137269571, 34.16647553114546554 ) ) ;
#72493=CARTESIAN_POINT ( 'NONE',  ( 3.165499230212911463, -12.51329471203370325, 31.30864560766548976 ) ) ;
#72494=CARTESIAN_POINT ( 'NONE',  ( 3.230769230769110045, -2.892918686052166066, 31.69288490824153470 ) ) ;
#72495=DIRECTION ( 'NONE',  ( -0.000000000000000000, 0.5000000000000011102, -0.8660254037844380415 ) ) ;
#72496=CYLINDRICAL_SURFACE ( 'NONE', #53018, 0.2500000000000008882 ) ;
#72497=CARTESIAN_POINT ( 'NONE',  ( -15.23076923076922995, -3.669653830205710676, 35.88435417666054406 ) ) ;
#72498=CARTESIAN_POINT ( 'NONE',  ( -11.53846153846166089, -5.941354392335915335, 34.76329471203413846 ) ) ;
#72499=CARTESIAN_POINT ( 'NONE',  ( 15.29602480204525250, -11.48612834413965977, 32.76840700105972815 ) ) ;
#72500=EDGE_LOOP ( 'NONE', ( #49432, #1294 ) ) ;
#72502=CARTESIAN_POINT ( 'NONE',  ( 9.019176287578909879, -11.86320923018887719, 32.19269448109604070 ) ) ;
#72503=CARTESIAN_POINT ( 'NONE',  ( 12.46153846153846168, -12.48256725967547354, 35.29906147534542527 ) ) ;
#72505=ADVANCED_FACE ( 'NONE', ( #75813 ), #84364, .F. ) ;
#72506=CARTESIAN_POINT ( 'NONE',  ( -14.30769230769242739, -5.219633306517616589, 34.19971097300220464 ) ) ;
#72507=CARTESIAN_POINT ( 'NONE',  ( 14.05771556364371655, -4.818429247618089661, 34.26397095200675125 ) ) ;
#72508=CARTESIAN_POINT ( 'NONE',  ( -16.15384615384615330, -3.050289026998446396, 32.03036669348365706 ) ) ;
#72509=EDGE_LOOP ( 'NONE', ( #73889, #7031, #61478, #66968 ) ) ;
#72511=CARTESIAN_POINT ( 'NONE',  ( -15.48074597481782178, -4.075325502946081535, 33.72974371597206300 ) ) ;
#72512=ADVANCED_FACE ( 'NONE', ( #55986 ), #49236, .F. ) ;
#72513=VERTEX_POINT ( 'NONE', #21310 ) ;
#72515=CARTESIAN_POINT ( 'NONE',  ( -4.403869378067609475, -8.475808217655753651, 34.90892951860618609 ) ) ;
#72516=EDGE_CURVE ( 'NONE', #15199, #83533, #14616, .T. ) ;
#72517=ORIENTED_EDGE ( 'NONE', *, *, #41256, .T. ) ;
#72518=CARTESIAN_POINT ( 'NONE',  ( -3.230769230769229949, -13.78497067705608181, 32.30358669280327177 ) ) ;
#72519=CARTESIAN_POINT ( 'NONE',  ( 13.13463865367303285, -9.943427161483782584, 34.11278801902876978 ) ) ;
#72520=CARTESIAN_POINT ( 'NONE',  ( 16.94677510719138169, -6.809168938359901446, 34.95455904226513866 ) ) ;
#72521=VERTEX_POINT ( 'NONE', #72153 ) ;
#72522=CARTESIAN_POINT ( 'NONE',  ( -12.46153846153846168, -2.249999999999998668, 29.50000000000001421 ) ) ;
#72523=ORIENTED_EDGE ( 'NONE', *, *, #78078, .T. ) ;
#72524=EDGE_CURVE ( 'NONE', #55585, #46544, #48906, .T. ) ;
#72526=ORIENTED_EDGE ( 'NONE', *, *, #86170, .T. ) ;
#72527=CARTESIAN_POINT ( 'NONE',  ( -16.15384615384627409, -2.379036618888197285, 30.90682066428292885 ) ) ;
#72529=EDGE_CURVE ( 'NONE', #43520, #45617, #23227, .T. ) ;
#72530=ORIENTED_EDGE ( 'NONE', *, *, #14055, .F. ) ;
#72531=CARTESIAN_POINT ( 'NONE',  ( -5.934744428723973897, -11.48612834413965977, 32.76840700105972815 ) ) ;
#72533=LINE ( 'NONE', #38971, #50918 ) ;
#72535=CARTESIAN_POINT ( 'NONE',  ( -14.30769230769242917, -10.33852847137269571, 34.16647553114546554 ) ) ;
#72536=CARTESIAN_POINT ( 'NONE',  ( -11.40767109749458541, -3.338503747796866872, 32.95102852606553512 ) ) ;
#72537=AXIS2_PLACEMENT_3D ( 'NONE', #32569, #82555, #61359 ) ;
#72538=ORIENTED_EDGE ( 'NONE', *, *, #14071, .F. ) ;
#72539=ORIENTED_EDGE ( 'NONE', *, *, #78078, .F. ) ;
#72540=ORIENTED_EDGE ( 'NONE', *, *, #6268, .F. ) ;
#72541=CARTESIAN_POINT ( 'NONE',  ( 3.165499230212911908, -5.941354392334500467, 34.76329471203369792 ) ) ;
#72542=ORIENTED_EDGE ( 'NONE', *, *, #4802, .F. ) ;
#72543=EDGE_CURVE ( 'NONE', #24141, #44733, #20982, .T. ) ;
#72544=VECTOR ( 'NONE', #68082, 1000.000000000000000 ) ;
#72545=EDGE_CURVE ( 'NONE', #4333, #68833, #23961, .T. ) ;
#72546=DIRECTION ( 'NONE',  ( 0.000000000000000000, 0.6427876096865368094, 0.7660444431189802339 ) ) ;
#72547=CARTESIAN_POINT ( 'NONE',  ( 9.562159722575998444, -5.915902021225889484, 34.75552854090298638 ) ) ;
#72548=VERTEX_POINT ( 'NONE', #86583 ) ;
#72549=ORIENTED_EDGE ( 'NONE', *, *, #87763, .T. ) ;
#72550=CARTESIAN_POINT ( 'NONE',  ( 0.2380535369741301754, -8.539481045369598178, 34.89627647299170832 ) ) ;
#72551=VERTEX_POINT ( 'NONE', #66289 ) ;
#72552=FACE_OUTER_BOUND ( 'NONE', #53476, .T. ) ;
#72554=EDGE_CURVE ( 'NONE', #5310, #73152, #4594, .T. ) ;
#72555=CARTESIAN_POINT ( 'NONE',  ( 17.07692307692295586, -12.51329471203414379, 31.30864560766407578 ) ) ;
#72556=CARTESIAN_POINT ( 'NONE',  ( -15.90390074446811042, -10.92531984108285670, 33.72920026020278073 ) ) ;
#72557=FACE_BOUND ( 'NONE', #45751, .T. ) ;
#72558=ORIENTED_EDGE ( 'NONE', *, *, #5049, .F. ) ;
#72559=FACE_OUTER_BOUND ( 'NONE', #19224, .T. ) ;
#72561=CYLINDRICAL_SURFACE ( 'NONE', #80538, 0.2499999999999995559 ) ;
#72562=CARTESIAN_POINT ( 'NONE',  ( 2.057715563643717882, -8.347322224742351082, 34.93158281831414769 ) ) ;
#72563=CARTESIAN_POINT ( 'NONE',  ( -1.450698795571264910, -2.538708090699994813, 30.37095296980875148 ) ) ;
#72566=VERTEX_POINT ( 'NONE', #85242 ) ;
#72567=ADVANCED_FACE ( 'NONE', ( #17213 ), #17670, .F. ) ;
#72568=ORIENTED_EDGE ( 'NONE', *, *, #71709, .T. ) ;
#72569=AXIS2_PLACEMENT_3D ( 'NONE', #2243, #84693, #83810 ) ;
#72570=CARTESIAN_POINT ( 'NONE',  ( -0.4615384615385826339, -9.442884908241554243, 34.35708131394783038 ) ) ;
#72572=CARTESIAN_POINT ( 'NONE',  ( -10.83886955910856287, -12.24155766932282496, 31.33739205006857986 ) ) ;
#72573=CARTESIAN_POINT ( 'NONE',  ( -2.084680956079455694, -12.15243808032445827, 31.58219941686247978 ) ) ;
#72574=EDGE_CURVE ( 'NONE', #21910, #62783, #75869, .T. ) ;
#72575=CARTESIAN_POINT ( 'NONE',  ( 7.716006636715626144, -12.45813303252208648, 30.39737893381572675 ) ) ;
#72576=CARTESIAN_POINT ( 'NONE',  ( 17.99999999999987566, -5.094484230521993062, 34.41647553114689373 ) ) ;
#72578=EDGE_LOOP ( 'NONE', ( #58602, #41934 ) ) ;
#72579=CARTESIAN_POINT ( 'NONE',  ( -5.142193077479395136, -6.835583212224499938, 34.95778746994557906 ) ) ;
#72580=DIRECTION ( 'NONE',  ( 0.000000000000000000, 0.000000000000000000, 1.000000000000000000 ) ) ;
#72581=CARTESIAN_POINT ( 'NONE',  ( -14.17764725177253382, -2.254550872974306674, 29.97347326024527092 ) ) ;
#72582=CARTESIAN_POINT ( 'NONE',  ( 14.37294744720514572, -2.657715359629132301, 31.77849191805844242 ) ) ;
#72583=EDGE_LOOP ( 'NONE', ( #61235, #6655 ) ) ;
#72584=EDGE_CURVE ( 'NONE', #37767, #73916, #19881, .T. ) ;
#72585=ORIENTED_EDGE ( 'NONE', *, *, #85820, .F. ) ;
#72586=FACE_BOUND ( 'NONE', #8070, .T. ) ;
#72587=ORIENTED_EDGE ( 'NONE', *, *, #86541, .F. ) ;
#72588=CARTESIAN_POINT ( 'NONE',  ( 18.13083841801275753, -7.277220443632451463, 34.74524770363009196 ) ) ;
#72589=DIRECTION ( 'NONE',  ( -0.000000000000000000, 0.9848077530122085754, -0.1736481776669273613 ) ) ;
#72591=CARTESIAN_POINT ( 'NONE',  ( -7.780898274877818821, -4.481592998940249650, 33.73612834413965089 ) ) ;
#72592=CARTESIAN_POINT ( 'NONE',  ( -10.83831083290076158, -6.503392248772476236, 34.64988816332204635 ) ) ;
#72593=CARTESIAN_POINT ( 'NONE',  ( 4.826946345980722697, -2.779195860258147022, 31.39871582349836743 ) ) ;
#72594=CARTESIAN_POINT ( 'NONE',  ( 5.076923076923075762, -8.564572088678739092, 35.78748833219616898 ) ) ;
#72596=VERTEX_POINT ( 'NONE', #41048 ) ;
#72598=ORIENTED_EDGE ( 'NONE', *, *, #30986, .F. ) ;
#72599=CARTESIAN_POINT ( 'NONE',  ( 15.29602480204525605, -8.613356846314928816, 34.62446782046653482 ) ) ;
#72600=CARTESIAN_POINT ( 'NONE',  ( 4.087762742890272527, -6.386643153685125363, 34.62446782046654903 ) ) ;
#72601=FACE_OUTER_BOUND ( 'NONE', #28241, .T. ) ;
#72602=CARTESIAN_POINT ( 'NONE',  ( -10.61538461538473577, -3.643525952248795718, 33.31231777344771672 ) ) ;
#72603=CARTESIAN_POINT ( 'NONE',  ( -7.976301055592065481, -9.418419913701741919, 34.36755862841477693 ) ) ;
#72605=CARTESIAN_POINT ( 'NONE',  ( 5.142991427925514003, -12.37446782046654192, 30.86335684631486842 ) ) ;
#72606=B_SPLINE_CURVE_WITH_KNOTS ( 'NONE', 3,
 ( #2814, #30306, #72169, #23975, #46036, #10924, #57774, #4611, #79834, #32082 ),
 .UNSPECIFIED., .F., .F.,
 ( 4, 2, 2, 2, 4 ),
 ( 0.0007817246256747464135, 0.0009771112852218900684, 0.001172497944769033615, 0.001367884604316177161, 0.001563271263863320925 ),
 .UNSPECIFIED. ) ;
#72609=CARTESIAN_POINT ( 'NONE',  ( 5.076923076923075762, -11.91647553114624181, 32.58852847137148245 ) ) ;
#72610=DIRECTION ( 'NONE',  ( 0.000000000000000000, 0.6427876096865373645, -0.7660444431189797898 ) ) ;
#72611=CARTESIAN_POINT ( 'NONE',  ( 6.250000000000000888, -2.499999999999998668, 29.75000000000000355 ) ) ;
#72612=EDGE_CURVE ( 'NONE', #71888, #61379, #37086, .T. ) ;
#72613=VECTOR ( 'NONE', #54225, 999.9999999999998863 ) ;
#72614=VERTEX_POINT ( 'NONE', #87476 ) ;
#72615=ORIENTED_EDGE ( 'NONE', *, *, #87885, .F. ) ;
#72616=CARTESIAN_POINT ( 'NONE',  ( -1.515175976357303833, -2.504760397472875155, 29.97295953869789997 ) ) ;
#72617=CARTESIAN_POINT ( 'NONE',  ( -14.24162497434223340, -2.486705287966280320, 31.30864560766543647 ) ) ;
#72618=CARTESIAN_POINT ( 'NONE',  ( 13.25392391794783009, -3.530157926970578952, 32.79014554554150607 ) ) ;
#72619=DIRECTION ( 'NONE',  ( 0.000000000000000000, 0.8660254037844377084, -0.5000000000000015543 ) ) ;
#72620=DIRECTION ( 'NONE',  ( 0.000000000000000000, 0.6427876096865373645, -0.7660444431189797898 ) ) ;
#72621=FACE_OUTER_BOUND ( 'NONE', #65108, .T. ) ;
#72622=CARTESIAN_POINT ( 'NONE',  ( -12.46153846153846168, -13.95598074871891292, 31.83374038241031911 ) ) ;
#72623=ORIENTED_EDGE ( 'NONE', *, *, #30868, .T. ) ;
#72624=CARTESIAN_POINT ( 'NONE',  ( 0.4615384615384611200, -3.669653830205710676, 35.88435417666054406 ) ) ;
#72625=CARTESIAN_POINT ( 'NONE',  ( -0.3954701105360233226, -8.120952969808774569, 34.71129190929999453 ) ) ;
#72626=CARTESIAN_POINT ( 'NONE',  ( 6.988332062589762472, -6.835583212224609184, 34.95778746994559327 ) ) ;
#72627=CARTESIAN_POINT ( 'NONE',  ( -14.30769230769230660, -1.129524287112498415, 32.06866353760679544 ) ) ;
#72628=ORIENTED_EDGE ( 'NONE', *, *, #1631, .T. ) ;
#72629=CARTESIAN_POINT ( 'NONE',  ( 12.33084785842815734, -2.494641256782728966, 31.33461815524612959 ) ) ;
#72630=VERTEX_POINT ( 'NONE', #59533 ) ;
#72631=FACE_OUTER_BOUND ( 'NONE', #41746, .T. ) ;
#72633=CARTESIAN_POINT ( 'NONE',  ( -1.634592115557738090, -9.148715823498378086, 34.47080413974185120 ) ) ;
#72634=CARTESIAN_POINT ( 'NONE',  ( 5.999999999999878320, -12.16647553114689728, 32.15551576947799362 ) ) ;
#72635=ORIENTED_EDGE ( 'NONE', *, *, #80734, .F. ) ;
#72636=CARTESIAN_POINT ( 'NONE',  ( 0.4615384615383396616, -3.300289026999228881, 32.46337939537708905 ) ) ;
#72637=CARTESIAN_POINT ( 'NONE',  ( 6.000000000000001776, -9.780366693483667717, 34.19971097300155094 ) ) ;
#72638=CARTESIAN_POINT ( 'NONE',  ( 10.36536137809165226, -3.711651800289232028, 33.01384336483936011 ) ) ;
#72640=ADVANCED_FACE ( 'NONE', ( #46469 ), #87035, .F. ) ;
#72641=B_SPLINE_CURVE_WITH_KNOTS ( 'NONE', 3,
 ( #66219, #19372, #46842, #26131, #12178, #32004, #32444, #39213, #4525, #52262 ),
 .UNSPECIFIED., .F., .F.,
 ( 4, 2, 2, 2, 4 ),
 ( 0.000000000000000000, 0.0001954339857564097241, 0.0003908679715128194482, 0.0005863019572692291723, 0.0007817359430256388964 ),
 .UNSPECIFIED. ) ;
#72642=CARTESIAN_POINT ( 'NONE',  ( 9.442307692307693401, -2.499999999999998668, 29.75000000000000355 ) ) ;
#72643=FACE_OUTER_BOUND ( 'NONE', #58818, .T. ) ;
#72644=ORIENTED_EDGE ( 'NONE', *, *, #58857, .T. ) ;
#72645=CARTESIAN_POINT ( 'NONE',  ( 9.692307692307695177, -9.584722331328613620, 36.20867863119891439 ) ) ;
#72646=ORIENTED_EDGE ( 'NONE', *, *, #88572, .F. ) ;
#72648=CARTESIAN_POINT ( 'NONE',  ( 5.076923076923075762, -3.050289026998446396, 32.03036669348365706 ) ) ;
#72649=CARTESIAN_POINT ( 'NONE',  ( -6.923076923077045919, -8.656820664282941280, 34.87096338111179961 ) ) ;
#72651=EDGE_CURVE ( 'NONE', #45729, #84649, #13598, .T. ) ;
#72652=CARTESIAN_POINT ( 'NONE',  ( -9.626240358957616650, -6.343179335718452272, 34.87096338111212646 ) ) ;
#72653=CARTESIAN_POINT ( 'NONE',  ( 12.59206416330202316, -10.19071101563364756, 33.96452234770658407 ) ) ;
#72654=VERTEX_POINT ( 'NONE', #26642 ) ;
#72655=ORIENTED_EDGE ( 'NONE', *, *, #52421, .T. ) ;
#72656=ORIENTED_EDGE ( 'NONE', *, *, #82301, .T. ) ;
#72657=ORIENTED_EDGE ( 'NONE', *, *, #46026, .T. ) ;
#72658=EDGE_LOOP ( 'NONE', ( #60875, #33526, #87002, #37522 ) ) ;
#72660=EDGE_CURVE ( 'NONE', #71376, #71885, #83386, .T. ) ;
#72661=DIRECTION ( 'NONE',  ( -0.000000000000000000, 0.6427876096865404731, -0.7660444431189770143 ) ) ;
#72662=CYLINDRICAL_SURFACE ( 'NONE', #67561, 0.2499999999999995559 ) ;
#72663=CARTESIAN_POINT ( 'NONE',  ( -2.057692307690870415, -7.500000000000155431, 34.75000000000007105 ) ) ;
#72664=CARTESIAN_POINT ( 'NONE',  ( 6.000000000000001776, -6.343179335718451384, 34.87096338111211935 ) ) ;
#72665=CARTESIAN_POINT ( 'NONE',  ( 7.623226887246997485, -12.64616026154729411, 30.79003144601913533 ) ) ;
#72666=CARTESIAN_POINT ( 'NONE',  ( 3.007284287045283389, -5.912607949931405038, 34.49155766932282319 ) ) ;
#72667=CARTESIAN_POINT ( 'NONE',  ( -17.93474442872397034, -10.21337939537593797, 33.94971097300152252 ) ) ;
#72668=CARTESIAN_POINT ( 'NONE',  ( 16.94636316330970871, -2.254533558242299396, 29.97296025877827930 ) ) ;
#72669=CARTESIAN_POINT ( 'NONE',  ( -4.219116599806928214, -10.21337939537584383, 33.94971097300158647 ) ) ;
#72672=B_SPLINE_CURVE_WITH_KNOTS ( 'NONE', 3,
 ( #81525, #33334, #7956, #6307, #39657, #67563, #67119, #74767, #28217, #53593 ),
 .UNSPECIFIED., .F., .F.,
 ( 4, 2, 2, 2, 4 ),
 ( 0.0007817246256747474977, 0.0009771112852218909357, 0.001172497944769034482, 0.001367884604316178029, 0.001563271263863321575 ),
 .UNSPECIFIED. ) ;
#72673=ORIENTED_EDGE ( 'NONE', *, *, #63194, .F. ) ;
#72674=ORIENTED_EDGE ( 'NONE', *, *, #56981, .F. ) ;
#72675=CARTESIAN_POINT ( 'NONE',  ( 0.2115617174898705155, -12.01397095200673881, 32.43157075238190146 ) ) ;
#72676=ORIENTED_EDGE ( 'NONE', *, *, #55318, .T. ) ;
#72678=DIRECTION ( 'NONE',  ( 0.000000000000000000, 0.9848077530122072432, -0.1736481776669354937 ) ) ;
#72679=B_SPLINE_CURVE_WITH_KNOTS ( 'NONE', 3,
 ( #22879, #8496, #84166, #77386, #64299, #23756, #29652, #57995, #49908, #51209 ),
 .UNSPECIFIED., .F., .F.,
 ( 4, 2, 2, 2, 4 ),
 ( 0.000000000000000000, 0.0001954311564186874978, 0.0003908623128373749957, 0.0005862934692560624935, 0.0007817246256747499913 ),
 .UNSPECIFIED. ) ;
#72680=CARTESIAN_POINT ( 'NONE',  ( -1.134615384615369260, -2.249999999999999112, 29.81603969181031033 ) ) ;
#72681=EDGE_CURVE ( 'NONE', #73158, #763, #1689, .T. ) ;
#72682=CARTESIAN_POINT ( 'NONE',  ( 4.153846153846032507, -2.625532179533778709, 30.86335684631627174 ) ) ;
#72683=EDGE_CURVE ( 'NONE', #89080, #64424, #46021, .T. ) ;
#72684=FACE_BOUND ( 'NONE', #65432, .T. ) ;
#72686=ORIENTED_EDGE ( 'NONE', *, *, #68223, .T. ) ;
#72687=LINE ( 'NONE', #25395, #87436 ) ;
#72688=ORIENTED_EDGE ( 'NONE', *, *, #86332, .T. ) ;
#72689=FACE_BOUND ( 'NONE', #75625, .T. ) ;
#72690=CARTESIAN_POINT ( 'NONE',  ( -6.000000000000119904, -9.442884908241554243, 34.35708131394783038 ) ) ;
#72691=CARTESIAN_POINT ( 'NONE',  ( -3.931066612577742259, -11.89424750095246175, 32.13594075562311758 ) ) ;
#72692=ORIENTED_EDGE ( 'NONE', *, *, #57342, .T. ) ;
#72693=CARTESIAN_POINT ( 'NONE',  ( 2.084207363968360038, -8.496056993536548418, 34.65000542017679663 ) ) ;
#72695=CARTESIAN_POINT ( 'NONE',  ( 2.057669083470850424, -11.56360843649121861, 33.07473185843129926 ) ) ;
#72696=EDGE_LOOP ( 'NONE', ( #51220, #36415, #68897, #87355 ) ) ;
#72697=CARTESIAN_POINT ( 'NONE',  ( 17.75000000000000000, -7.500000000000001776, 35.00000000000000000 ) ) ;
#72698=DIRECTION ( 'NONE',  ( 0.000000000000000000, 0.000000000000000000, -1.000000000000000000 ) ) ;
#72699=ORIENTED_EDGE ( 'NONE', *, *, #25673, .T. ) ;
#72700=DIRECTION ( 'NONE',  ( -0.000000000000000000, -0.6427876096865404731, -0.7660444431189770143 ) ) ;
#72702=ORIENTED_EDGE ( 'NONE', *, *, #38823, .T. ) ;
#72703=CARTESIAN_POINT ( 'NONE',  ( 18.22301135161285046, -6.503523203565941380, 34.64991518177335195 ) ) ;
#72704=CARTESIAN_POINT ( 'NONE',  ( 13.13459214732242408, -2.587272538249754117, 30.68239716806877837 ) ) ;
#72705=CARTESIAN_POINT ( 'NONE',  ( -15.93106661257773560, -8.496831190052089866, 34.64984203495476578 ) ) ;
#72706=CARTESIAN_POINT ( 'NONE',  ( -10.48485891362104994, -6.001044277235009439, 34.52024696741798948 ) ) ;
#72707=CARTESIAN_POINT ( 'NONE',  ( 3.230769230769231726, -2.721908614388771852, 31.22303859784724978 ) ) ;
#72708=DIRECTION ( 'NONE',  ( 1.000000000000000000, 0.000000000000000000, 0.000000000000000000 ) ) ;
#72709=CARTESIAN_POINT ( 'NONE',  ( 4.376857505459003761, -12.15243808032446005, 31.58219941686247978 ) ) ;
#72710=CARTESIAN_POINT ( 'NONE',  ( -0.4615384615384611200, -11.16473453929635440, 33.15142922261926373 ) ) ;
#72711=CARTESIAN_POINT ( 'NONE',  ( 8.900022577055556994, -12.11778462344221019, 31.66786338562085135 ) ) ;
#72712=LINE ( 'NONE', #9677, #60228 ) ;
#72713=LINE ( 'NONE', #73170, #59304 ) ;
#72715=ORIENTED_EDGE ( 'NONE', *, *, #67381, .T. ) ;
#72717=VERTEX_POINT ( 'NONE', #5037 ) ;
#72718=ORIENTED_EDGE ( 'NONE', *, *, #14535, .F. ) ;
#72719=CARTESIAN_POINT ( 'NONE',  ( -7.623374177175779920, -2.612705202774698421, 31.66806509827799943 ) ) ;
#72720=ORIENTED_EDGE ( 'NONE', *, *, #56180, .F. ) ;
#72721=CARTESIAN_POINT ( 'NONE',  ( -11.53846153846166089, -9.528491918059723176, 34.59228464037033035 ) ) ;
#72723=CARTESIAN_POINT ( 'NONE',  ( 4.153846153846154188, -4.786620604624113540, 33.94971097300155094 ) ) ;
#72724=CARTESIAN_POINT ( 'NONE',  ( -15.23076923076922995, -12.34228464037088635, 31.77849191805839268 ) ) ;
#72725=CARTESIAN_POINT ( 'NONE',  ( -0.2114841499001470781, -5.728107161865378494, 34.42597550085002922 ) ) ;
#72726=CARTESIAN_POINT ( 'NONE',  ( -6.000000000000121680, -2.657715359629662988, 31.77849191805970364 ) ) ;
#72728=CARTESIAN_POINT ( 'NONE',  ( -10.61538461538473399, -4.481592998941358097, 33.73612834414048933 ) ) ;
#72729=CARTESIAN_POINT ( 'NONE',  ( 5.776515056276054771, -4.386631170607603991, 33.66268669641500111 ) ) ;
#72732=DIRECTION ( 'NONE',  ( -0.000000000000000000, 0.9396926207859093161, -0.3420201433256663259 ) ) ;
#72733=CARTESIAN_POINT ( 'NONE',  ( 4.153846153846030731, -2.379036618888197729, 30.90682066428292885 ) ) ;
#72734=CYLINDRICAL_SURFACE ( 'NONE', #10488, 0.2499999999999995559 ) ;
#72735=EDGE_LOOP ( 'NONE', ( #66265, #35102, #62223, #86052 ) ) ;
#72736=ORIENTED_EDGE ( 'NONE', *, *, #30943, .T. ) ;
#72737=CARTESIAN_POINT ( 'NONE',  ( -11.47320596718551045, -6.026961402152789304, 34.52809138561124769 ) ) ;
#72738=CARTESIAN_POINT ( 'NONE',  ( -17.20707028636129721, -8.587444163452046197, 34.63053765926554206 ) ) ;
#72739=CARTESIAN_POINT ( 'NONE',  ( 16.15384615384615330, -12.34228464037088635, 31.77849191805839268 ) ) ;
#72741=VECTOR ( 'NONE', #62044, 1000.000000000000114 ) ;
#72742=CARTESIAN_POINT ( 'NONE',  ( 17.07692307692307665, -12.34228464037088635, 31.77849191805839268 ) ) ;
#72743=CARTESIAN_POINT ( 'NONE',  ( -10.61538461538461320, -4.098570777380720287, 33.41473453929634729 ) ) ;
#72744=ADVANCED_FACE ( 'NONE', ( #5492 ), #53217, .F. ) ;
#72745=EDGE_CURVE ( 'NONE', #86745, #30027, #50025, .T. ) ;
#72746=ORIENTED_EDGE ( 'NONE', *, *, #27924, .T. ) ;
#72747=CARTESIAN_POINT ( 'NONE',  ( -10.68070753087678781, -7.749976743299138882, 34.99404534957040624 ) ) ;
#72748=ORIENTED_EDGE ( 'NONE', *, *, #24246, .T. ) ;
#72750=CARTESIAN_POINT ( 'NONE',  ( -9.692307692307814193, -3.083524468854526912, 32.58852847137268327 ) ) ;
#72751=ADVANCED_FACE ( 'NONE', ( #27528 ), #7262, .F. ) ;
#72752=CYLINDRICAL_SURFACE ( 'NONE', #61468, 0.2500000000000008882 ) ;
#72753=CIRCLE ( 'NONE', #33925, 0.2500000000000002220 ) ;
#72754=CARTESIAN_POINT ( 'NONE',  ( -9.627052121031661969, -6.879047030191282275, 34.71129190930002295 ) ) ;
#72756=CARTESIAN_POINT ( 'NONE',  ( 9.692307692307695177, -3.322132147404559976, 32.92929555188717927 ) ) ;
#72757=CARTESIAN_POINT ( 'NONE',  ( 13.25446741488368829, -8.630895178749533159, 34.87696386517710323 ) ) ;
#72759=ORIENTED_EDGE ( 'NONE', *, *, #88539, .T. ) ;
#72760=ORIENTED_EDGE ( 'NONE', *, *, #49846, .T. ) ;
#72761=ORIENTED_EDGE ( 'NONE', *, *, #19710, .F. ) ;
#72762=EDGE_CURVE ( 'NONE', #74862, #23459, #28873, .T. ) ;
#72763=CARTESIAN_POINT ( 'NONE',  ( -7.146561847641252463, -12.11044203135681840, 32.26167407432752299 ) ) ;
#72765=CARTESIAN_POINT ( 'NONE',  ( 8.992243613324164997, -5.582272713120729257, 34.63742843783360570 ) ) ;
#72767=CARTESIAN_POINT ( 'NONE',  ( -11.76194646302587010, -8.539481045369596401, 34.89627647299170832 ) ) ;
#72768=CARTESIAN_POINT ( 'NONE',  ( -16.02332045208259359, -2.882268652242223617, 31.66798894389554064 ) ) ;
#72769=ORIENTED_EDGE ( 'NONE', *, *, #74816, .F. ) ;
#72771=DIRECTION ( 'NONE',  ( -0.000000000000000000, 0.3420201433256694346, -0.9396926207859080948 ) ) ;
#72772=VERTEX_POINT ( 'NONE', #28408 ) ;
#72773=CARTESIAN_POINT ( 'NONE',  ( -5.934744428723973897, -3.300289026998475705, 32.46337939537591666 ) ) ;
#72774=ORIENTED_EDGE ( 'NONE', *, *, #6713, .F. ) ;
#72775=CARTESIAN_POINT ( 'NONE',  ( 1.384615384615265343, -10.21337939537710326, 33.94971097300076224 ) ) ;
#72776=FACE_OUTER_BOUND ( 'NONE', #14079, .T. ) ;
#72779=ADVANCED_FACE ( 'NONE', ( #48231 ), #35169, .F. ) ;
#72780=ORIENTED_EDGE ( 'NONE', *, *, #53851, .F. ) ;
#72781=EDGE_CURVE ( 'NONE', #67447, #78622, #77942, .T. ) ;
#72782=CARTESIAN_POINT ( 'NONE',  ( 8.769230769230768274, -13.53365097954675988, 30.81389545987213552 ) ) ;
#72784=CARTESIAN_POINT ( 'NONE',  ( 2.530471848960718084, -9.332535724633405749, 34.40230450496446224 ) ) ;
#72785=DIRECTION ( 'NONE',  ( -0.000000000000000000, -0.6427876096865404731, -0.7660444431189770143 ) ) ;
#72786=FACE_BOUND ( 'NONE', #51706, .T. ) ;
#72787=CARTESIAN_POINT ( 'NONE',  ( 5.076923076923075762, -4.661471528628507777, 34.16647553114623292 ) ) ;
#72788=DIRECTION ( 'NONE',  ( -0.000000000000000000, 0.1736481776669307198, -0.9848077530122080203 ) ) ;
#72789=EDGE_CURVE ( 'NONE', #30370, #56543, #8149, .T. ) ;
#72790=CARTESIAN_POINT ( 'NONE',  ( -1.607542343522233130, -3.395401636524185474, 33.02366814457250399 ) ) ;
#72791=CARTESIAN_POINT ( 'NONE',  ( -3.360917200500926239, -8.630895178749536711, 34.87696386517710323 ) ) ;
#72792=VERTEX_POINT ( 'NONE', #69404 ) ;
#72793=ADVANCED_FACE ( 'NONE', ( #1382 ), #83367, .F. ) ;
#72796=VERTEX_POINT ( 'NONE', #21207 ) ;
#72797=B_SPLINE_CURVE_WITH_KNOTS ( 'NONE', 3,
 ( #47123, #61525, #75488, #12903, #34508, #20980, #68736, #7032, #48451, #75937 ),
 .UNSPECIFIED., .F., .F.,
 ( 4, 2, 2, 2, 4 ),
 ( 0.0007817246336856289524, 0.0009771112958940099402, 0.001172497958102391036, 0.001367884620310772133, 0.001563271282519153229 ),
 .UNSPECIFIED. ) ;
#72798=CARTESIAN_POINT ( 'NONE',  ( -18.00000000000000000, -3.050289026998447284, 32.03036669348365706 ) ) ;
#72799=CARTESIAN_POINT ( 'NONE',  ( -18.25002322422145440, -12.68155406624981119, 30.59749803192733708 ) ) ;
#72800=CARTESIAN_POINT ( 'NONE',  ( 10.55011461482829738, -8.656820664281498878, 34.87096338111211935 ) ) ;
#72801=FACE_OUTER_BOUND ( 'NONE', #46304, .T. ) ;
#72802=DIRECTION ( 'NONE',  ( 1.000000000000000000, 0.000000000000000000, 0.000000000000000000 ) ) ;
#72803=FACE_BOUND ( 'NONE', #23466, .T. ) ;
#72804=LINE ( 'NONE', #37240, #61927 ) ;
#72805=DIRECTION ( 'NONE',  ( -0.000000000000000000, 0.000000000000000000, 1.000000000000000000 ) ) ;
#72806=( GEOMETRIC_REPRESENTATION_CONTEXT ( 3 ) GLOBAL_UNCERTAINTY_ASSIGNED_CONTEXT ( ( #69518 ) ) GLOBAL_UNIT_ASSIGNED_CONTEXT ( ( #80625, #26556, #18907 ) ) REPRESENTATION_CONTEXT ( 'NONE', 'WORKASPACE' ) );
#72807=CARTESIAN_POINT ( 'NONE',  ( 16.02369894440793630, -3.285722584762969856, 32.44110544564090759 ) ) ;
#72808=CARTESIAN_POINT ( 'NONE',  ( 2.980745993476266342, -4.335965774309649134, 33.62209801155881905 ) ) ;
#72809=CARTESIAN_POINT ( 'NONE',  ( -20.99999999999999645, -7.500000000000000000, 29.75000000000000355 ) ) ;
#72810=CARTESIAN_POINT ( 'NONE',  ( 15.90382291655318880, -10.76384336483936011, 33.53834819971076087 ) ) ;
#72811=CARTESIAN_POINT ( 'NONE',  ( 6.250054419913455561, -4.818054556918156095, 34.26375889529406749 ) ) ;
#72813=ORIENTED_EDGE ( 'NONE', *, *, #12915, .F. ) ;
#72814=CARTESIAN_POINT ( 'NONE',  ( -7.976845312821407852, -11.18331474514187995, 33.13161551792790505 ) ) ;
#72815=CARTESIAN_POINT ( 'NONE',  ( 7.715462379486289102, -8.999036380462719364, 34.52022231692819076 ) ) ;
#72816=CARTESIAN_POINT ( 'NONE',  ( -13.51517529822874586, -2.254533558242299396, 29.97296025877828285 ) ) ;
#72817=DIRECTION ( 'NONE',  ( -0.000000000000000000, 0.9848077530122085754, -0.1736481776669273613 ) ) ;
#72818=CARTESIAN_POINT ( 'NONE',  ( 10.74591031714818001, -12.27024696741798770, 31.24895572276497546 ) ) ;
#72819=CARTESIAN_POINT ( 'NONE',  ( -6.923076923076922462, -13.78497067705608181, 32.30358669280327177 ) ) ;
#72821=CARTESIAN_POINT ( 'NONE',  ( -8.703162418228330921, -2.721908614388772296, 31.22303859784725333 ) ) ;
#72822=CARTESIAN_POINT ( 'NONE',  ( 0.4615384615383396616, -3.835265460704628371, 33.15142922262033665 ) ) ;
#72823=AXIS2_PLACEMENT_3D ( 'NONE', #55687, #83180, #21467 ) ;
#72824=CARTESIAN_POINT ( 'NONE',  ( 11.28846153846153832, -7.500000000000001776, 35.00000000000000000 ) ) ;
#72825=CARTESIAN_POINT ( 'NONE',  ( -0.4615384615385840772, -8.656820664282941280, 34.87096338111179961 ) ) ;
#72826=CARTESIAN_POINT ( 'NONE',  ( 8.703147358274888390, -9.780366693483667717, 34.19971097300155805 ) ) ;
#72827=CARTESIAN_POINT ( 'NONE',  ( -8.992156986746916658, -9.086856451489515152, 34.49173150075333183 ) ) ;
#72828=EDGE_CURVE ( 'NONE', #85857, #49108, #57510, .T. ) ;
#72829=DIRECTION ( 'NONE',  ( 1.000000000000000000, 0.000000000000000000, 0.000000000000000000 ) ) ;
#72830=AXIS2_PLACEMENT_3D ( 'NONE', #77473, #46, #36059 ) ;
#72831=DIRECTION ( 'NONE',  ( -0.000000000000000000, -0.5000000000000009992, -0.8660254037844380415 ) ) ;
#72832=ORIENTED_EDGE ( 'NONE', *, *, #70797, .F. ) ;
#72833=B_SPLINE_CURVE_WITH_KNOTS ( 'NONE', 3,
 ( #73698, #74127, #66928, #75023, #19620, #33137 ),
 .UNSPECIFIED., .F., .F.,
 ( 4, 2, 4 ),
 ( 0.0003909512603273901832, 0.0005862562993132176088, 0.0007815613382990449802 ),
 .UNSPECIFIED. ) ;
#72834=CARTESIAN_POINT ( 'NONE',  ( 15.23076923076923173, -11.35647404775217417, 33.31231777344666511 ) ) ;
#72835=CARTESIAN_POINT ( 'NONE',  ( 8.899756470994331536, -11.46989282347013095, 32.79007818306219946 ) ) ;
#72837=B_SPLINE_CURVE_WITH_KNOTS ( 'NONE', 3,
 ( #7166, #8055, #8499, #28773, #56238, #22445, #70192, #84169, #41397, #7611 ),
 .UNSPECIFIED., .F., .F.,
 ( 4, 2, 2, 2, 4 ),
 ( 0.000000000000000000, 0.0001954311564186862781, 0.0003908623128373725562, 0.0005862934692560588072, 0.0007817246256747451124 ),
 .UNSPECIFIED. ) ;
#72838=CARTESIAN_POINT ( 'NONE',  ( 13.38461538461526601, -10.21337939537710326, 33.94971097300076224 ) ) ;
#72839=FACE_OUTER_BOUND ( 'NONE', #26123, .T. ) ;
#72840=ORIENTED_EDGE ( 'NONE', *, *, #62218, .T. ) ;
#72841=CARTESIAN_POINT ( 'NONE',  ( -18.00000000000000000, -8.973038597847269315, 34.52809138561121927 ) ) ;
#72843=CARTESIAN_POINT ( 'NONE',  ( -7.715628407920204879, -12.50538340440932394, 31.33453814440721885 ) ) ;
#72844=ORIENTED_EDGE ( 'NONE', *, *, #53872, .F. ) ;
#72845=CARTESIAN_POINT ( 'NONE',  ( -12.59222906464877134, -9.084618155246140248, 34.75535874321725771 ) ) ;
#72846=CARTESIAN_POINT ( 'NONE',  ( -1.384615384615383471, -1.951392089020283160, 34.73218667398347748 ) ) ;
#72847=CARTESIAN_POINT ( 'NONE',  ( -4.826977558574935934, -9.272278438253401589, 34.42582936511637826 ) ) ;
#72848=ADVANCED_FACE ( 'NONE', ( #42824 ), #59, .F. ) ;
#72849=DIRECTION ( 'NONE',  ( 0.000000000000000000, 0.000000000000000000, 1.000000000000000000 ) ) ;
#72850=ORIENTED_EDGE ( 'NONE', *, *, #85063, .T. ) ;
#72851=FACE_OUTER_BOUND ( 'NONE', #48497, .T. ) ;
#72852=CARTESIAN_POINT ( 'NONE',  ( -12.52680846209478460, -2.657715359629089225, 31.77849191805832874 ) ) ;
#72853=AXIS2_PLACEMENT_3D ( 'NONE', #25974, #86819, #46690 ) ;
#72854=CARTESIAN_POINT ( 'NONE',  ( -11.53846153846166089, -6.835583212225970762, 34.95778746994575670 ) ) ;
#72855=ORIENTED_EDGE ( 'NONE', *, *, #5358, .F. ) ;
#72856=VERTEX_POINT ( 'NONE', #82488 ) ;
#72857=VERTEX_POINT ( 'NONE', #20767 ) ;
#72859=CARTESIAN_POINT ( 'NONE',  ( -18.13014720943822056, -3.817052484675422352, 33.13202310037935661 ) ) ;
#72860=DIRECTION ( 'NONE',  ( 0.000000000000000000, 0.4999999999999960032, -0.8660254037844410391 ) ) ;
#72861=CIRCLE ( 'NONE', #26838, 0.2500000000000002220 ) ;
#72862=EDGE_CURVE ( 'NONE', #59563, #13845, #52765, .T. ) ;
#72863=CARTESIAN_POINT ( 'NONE',  ( 13.25446817517716447, -11.47017969459903952, 32.78971311882035167 ) ) ;
#72864=DIRECTION ( 'NONE',  ( -0.000000000000000000, 1.000000000000000000, 3.491481338843133355E-15 ) ) ;
#72865=ORIENTED_EDGE ( 'NONE', *, *, #46634, .F. ) ;
#72867=ORIENTED_EDGE ( 'NONE', *, *, #47151, .T. ) ;
#72868=CARTESIAN_POINT ( 'NONE',  ( -1.254089682851820653, -5.195472089885680766, 34.18748526763464923 ) ) ;
#72869=VERTEX_POINT ( 'NONE', #16226 ) ;
#72870=CARTESIAN_POINT ( 'NONE',  ( -16.15384615384627409, -12.51329471203414379, 31.30864560766407578 ) ) ;
#72871=B_SPLINE_CURVE_WITH_KNOTS ( 'NONE', 3,
 ( #30424, #78603, #77277, #9276, #70526, #37621, #24102, #36737, #30857, #43051 ),
 .UNSPECIFIED., .F., .F.,
 ( 4, 2, 2, 2, 4 ),
 ( 0.0007817359430256315238, 0.0009771253907249976244, 0.001172514838424363508, 0.001367904286123729392, 0.001563293733823095492 ),
 .UNSPECIFIED. ) ;
#72872=CARTESIAN_POINT ( 'NONE',  ( 8.769230769230768274, -12.78798330534102945, 29.74999999999997868 ) ) ;
#72873=EDGE_CURVE ( 'NONE', #68769, #8206, #75795, .T. ) ;
#72874=AXIS2_PLACEMENT_3D ( 'NONE', #4093, #53625, #37893 ) ;
#72875=CARTESIAN_POINT ( 'NONE',  ( 2.438484115517095319, -3.530189275343204702, 32.79018710029569661 ) ) ;
#72876=CARTESIAN_POINT ( 'NONE',  ( -7.911423846710166075, -10.33852847137145048, 34.16647553114627556 ) ) ;
#72878=EDGE_LOOP ( 'NONE', ( #57483, #15171 ) ) ;
#72879=B_SPLINE_CURVE_WITH_KNOTS ( 'NONE', 3,
 ( #72822, #44906, #65616, #17000, #24193, #37711, #23744, #65178, #79599, #3476 ),
 .UNSPECIFIED., .F., .F.,
 ( 4, 2, 2, 2, 4 ),
 ( 0.0007817359430256372700, 0.0009771253907250052138, 0.001172514838424373266, 0.001367904286123741101, 0.001563293733823109153 ),
 .UNSPECIFIED. ) ;
#72880=EDGE_LOOP ( 'NONE', ( #48840, #44636 ) ) ;
#72881=AXIS2_PLACEMENT_3D ( 'NONE', #16873, #52874, #71811 ) ;
#72882=ORIENTED_EDGE ( 'NONE', *, *, #80136, .F. ) ;
#72883=DIRECTION ( 'NONE',  ( -0.000000000000000000, -0.9848077530122085754, -0.1736481776669273613 ) ) ;
#72884=VERTEX_POINT ( 'NONE', #36505 ) ;
#72885=CARTESIAN_POINT ( 'NONE',  ( 16.94623247381277054, -5.496505350115500121, 34.60290016733514307 ) ) ;
#72886=CARTESIAN_POINT ( 'NONE',  ( 12.23805351781451378, -11.41268669641499756, 32.86336882939238535 ) ) ;
#72887=ADVANCED_FACE ( 'NONE', ( #51759 ), #65729, .F. ) ;
#72888=ORIENTED_EDGE ( 'NONE', *, *, #66045, .F. ) ;
#72889=CIRCLE ( 'NONE', #44071, 0.2500000000000002220 ) ;
#72892=DIRECTION ( 'NONE',  ( -0.000000000000000000, 0.9396926207859092051, -0.3420201433256662704 ) ) ;
#72893=FACE_BOUND ( 'NONE', #70897, .T. ) ;
#72894=CARTESIAN_POINT ( 'NONE',  ( -0.4615384615385826339, -4.481592998941358097, 33.73612834414048933 ) ) ;
#72895=CYLINDRICAL_SURFACE ( 'NONE', #57165, 0.2500000000000012212 ) ;
#72896=EDGE_CURVE ( 'NONE', #47112, #71524, #84427, .T. ) ;
#72897=CARTESIAN_POINT ( 'NONE',  ( -8.096177083446809419, -12.22074536777954989, 31.39888409691088356 ) ) ;
#72898=CYLINDRICAL_SURFACE ( 'NONE', #18744, 0.2499999999999994726 ) ;
#72899=CARTESIAN_POINT ( 'NONE',  ( 14.55763771707035303, -2.986452184633680673, 32.43230066228895225 ) ) ;
#72900=CARTESIAN_POINT ( 'NONE',  ( 8.519207545009310323, -9.356822207818506598, 34.66110646841856635 ) ) ;
#72901=CARTESIAN_POINT ( 'NONE',  ( 12.46153846153846168, -13.63283147151868846, 33.57946703557072254 ) ) ;
#72902=VERTEX_POINT ( 'NONE', #77920 ) ;
#72903=ADVANCED_FACE ( 'NONE', ( #58977 ), #43691, .F. ) ;
#72904=CARTESIAN_POINT ( 'NONE',  ( -17.32689982097166492, -5.643011162660950042, 34.66104346484419096 ) ) ;
#72905=CARTESIAN_POINT ( 'NONE',  ( -13.51530598772569469, -9.084618155246140248, 34.75535874321725771 ) ) ;
#72906=ORIENTED_EDGE ( 'NONE', *, *, #354, .T. ) ;
#72907=ORIENTED_EDGE ( 'NONE', *, *, #6852, .F. ) ;
#72908=CARTESIAN_POINT ( 'NONE',  ( -11.76194646302587010, -12.69144148231606017, 30.53333754910549303 ) ) ;
#72909=CARTESIAN_POINT ( 'NONE',  ( 1.607395053593452028, -5.827830569534415694, 34.72679350104403539 ) ) ;
#72910=B_SPLINE_CURVE_WITH_KNOTS ( 'NONE', 3,
 ( #54981, #8571, #35148, #21631, #83348, #36046, #68930, #7241, #70266, #34711 ),
 .UNSPECIFIED., .F., .F.,
 ( 4, 2, 2, 2, 4 ),
 ( 0.000000000000000000, 0.0001954339857564081791, 0.0003908679715128163582, 0.0005863019572692245102, 0.0007817359430256327164 ),
 .UNSPECIFIED. ) ;
#72911=B_SPLINE_CURVE_WITH_KNOTS ( 'NONE', 3,
 ( #62865, #34084, #1180, #69203, #61547, #53913, #34965, #62426, #81401, #89053 ),
 .UNSPECIFIED., .F., .F.,
 ( 4, 2, 2, 2, 4 ),
 ( 0.0007817359527651132059, 0.0009771254036996528287, 0.001172514854634192560, 0.001367904305568732291, 0.001563293756503272023 ),
 .UNSPECIFIED. ) ;
#72912=CARTESIAN_POINT ( 'NONE',  ( 16.28437185560972011, -2.619367082507847666, 30.83698974864643461 ) ) ;
#72913=FACE_OUTER_BOUND ( 'NONE', #55930, .T. ) ;
#72914=CYLINDRICAL_SURFACE ( 'NONE', #54811, 0.2499999999999994726 ) ;
#72915=ORIENTED_EDGE ( 'NONE', *, *, #52951, .F. ) ;
#72916=AXIS2_PLACEMENT_3D ( 'NONE', #74414, #12713, #2721 ) ;
#72918=CARTESIAN_POINT ( 'NONE',  ( 10.61538461538461675, -7.500000000000001776, 35.04278698407183867 ) ) ;
#72919=CARTESIAN_POINT ( 'NONE',  ( 5.076923076923075762, -5.557115091759785130, 34.35708131394839171 ) ) ;
#72921=CARTESIAN_POINT ( 'NONE',  ( -1.634592128663975519, -10.06842814019191401, 34.32929386961144758 ) ) ;
#72922=CARTESIAN_POINT ( 'NONE',  ( 10.61538461538461675, -4.098570777380720287, 33.41473453929634729 ) ) ;
#72923=FILL_AREA_STYLE ('',( #53535 ) ) ;
#72925=EDGE_CURVE ( 'NONE', #79557, #7925, #63984, .T. ) ;
#72926=AXIS2_PLACEMENT_3D ( 'NONE', #60349, #87860, #8962 ) ;
#72928=ORIENTED_EDGE ( 'NONE', *, *, #15405, .T. ) ;
#72929=VERTEX_POINT ( 'NONE', #84702 ) ;
#72931=EDGE_CURVE ( 'NONE', #56176, #68565, #44119, .T. ) ;
#72933=CARTESIAN_POINT ( 'NONE',  ( 12.71153846153989697, -7.500000000000155431, 34.75000000000007105 ) ) ;
#72934=CARTESIAN_POINT ( 'NONE',  ( 22.75000000000000000, -10.50000000000000000, 29.75000000000000355 ) ) ;
#72935=CARTESIAN_POINT ( 'NONE',  ( 14.43848411551708999, -2.729792928343269587, 31.24908615093345077 ) ) ;
#72936=CARTESIAN_POINT ( 'NONE',  ( 2.557692307693744560, -7.500000000000155431, 34.75000000000007105 ) ) ;
#72938=CARTESIAN_POINT ( 'NONE',  ( 8.638540166120458608, -3.957541250942358424, 33.62499894934981626 ) ) ;
#72939=CYLINDRICAL_SURFACE ( 'NONE', #11524, 0.2500000000000008882 ) ;
#72940=CARTESIAN_POINT ( 'NONE',  ( -9.019207513279360100, -12.65889640711025521, 30.72598325615533454 ) ) ;
#72941=CARTESIAN_POINT ( 'NONE',  ( -18.22337594069816902, -12.49852196912267566, 29.88021232661720461 ) ) ;
#72942=CARTESIAN_POINT ( 'NONE',  ( 9.758376043310134307, -2.721908614388771852, 31.22303859784725333 ) ) ;
#72943=CARTESIAN_POINT ( 'NONE',  ( 3.296024802045256497, -2.892918686051626498, 31.69288490824026638 ) ) ;
#72944=CARTESIAN_POINT ( 'NONE',  ( -12.71156168575991785, -8.475808217655753651, 34.90892951860618609 ) ) ;
#72945=EDGE_CURVE ( 'NONE', #66285, #53910, #71598, .T. ) ;
#72946=CARTESIAN_POINT ( 'NONE',  ( 3.930919936330004472, -12.39988816332205701, 30.74660775122750778 ) ) ;
#72947=B_SPLINE_CURVE_WITH_KNOTS ( 'NONE', 3,
 ( #55260, #82748, #49827, #7967, #56148, #77744, #21020, #762, #84520, #41312 ),
 .UNSPECIFIED., .F., .F.,
 ( 4, 2, 2, 2, 4 ),
 ( 0.000000000000000000, 0.0001954339857564078809, 0.0003908679715128157619, 0.0005863019572692236428, 0.0007817359430256315238 ),
 .UNSPECIFIED. ) ;
#72948=CARTESIAN_POINT ( 'NONE',  ( 1.384615384615264011, -9.528491918059723176, 34.59228464037033035 ) ) ;
#72949=CARTESIAN_POINT ( 'NONE',  ( 7.716005876422152632, -3.625366637846545892, 33.29286588640298561 ) ) ;
#72950=CARTESIAN_POINT ( 'NONE',  ( -16.85391023282967637, -2.889357225399416418, 32.26129605718031002 ) ) ;
#72951=VERTEX_POINT ( 'NONE', #64837 ) ;
#72953=ADVANCED_FACE ( 'NONE', ( #30616 ), #66175, .F. ) ;
#72954=CARTESIAN_POINT ( 'NONE',  ( 18.13052543823364360, -5.070358843744208421, 34.40418822224088302 ) ) ;
#72955=LINE ( 'NONE', #51770, #46239 ) ;
#72957=EDGE_CURVE ( 'NONE', #13993, #18183, #45908, .T. ) ;
#72958=CARTESIAN_POINT ( 'NONE',  ( -14.17690049986752321, -4.809403383903225304, 33.96459661697924304 ) ) ;
#72959=CARTESIAN_POINT ( 'NONE',  ( 15.93091919493930320, -4.762599654559227069, 34.23009711892697737 ) ) ;
#72960=CARTESIAN_POINT ( 'NONE',  ( 5.326868486301119532, -4.176053281294514363, 33.81426240980091791 ) ) ;
#72961=ORIENTED_EDGE ( 'NONE', *, *, #86022, .T. ) ;
#72964=EDGE_LOOP ( 'NONE', ( #40099, #14067 ) ) ;
#72965=EDGE_CURVE ( 'NONE', #22884, #85301, #60313, .T. ) ;
#72966=LINE ( 'NONE', #59455, #54350 ) ;
#72967=B_SPLINE_CURVE_WITH_KNOTS ( 'NONE', 3,
 ( #19319, #82356, #48103, #74716, #88687, #61621, #76023, #75578, #68384, #13880 ),
 .UNSPECIFIED., .F., .F.,
 ( 4, 2, 2, 2, 4 ),
 ( 0.000000000000000000, 0.0001954311564186867389, 0.0003908623128373734778, 0.0005862934692560602167, 0.0007817246256747469556 ),
 .UNSPECIFIED. ) ;
#72968=ORIENTED_EDGE ( 'NONE', *, *, #25531, .T. ) ;
#72970=CARTESIAN_POINT ( 'NONE',  ( 15.23076923076923173, -2.249999999999998668, 29.50000000000001421 ) ) ;
#72971=CARTESIAN_POINT ( 'NONE',  ( -9.469296340694846492, -2.758310577978207778, 31.33698337089302299 ) ) ;
#72973=DIRECTION ( 'NONE',  ( -0.000000000000000000, -0.1736481776669307198, -0.9848077530122080203 ) ) ;
#72974=ORIENTED_EDGE ( 'NONE', *, *, #58076, .T. ) ;
#72977=CARTESIAN_POINT ( 'NONE',  ( 11.31553532094538994, -3.586966769969701208, 32.86292498521069660 ) ) ;
#72978=VERTEX_POINT ( 'NONE', #25201 ) ;
#72979=CARTESIAN_POINT ( 'NONE',  ( -15.23076923076935252, -2.657715359629662544, 31.77849191805970364 ) ) ;
#72980=CARTESIAN_POINT ( 'NONE',  ( 2.530471848960719417, -3.236590943229497253, 32.36255958852954251 ) ) ;
#72981=EDGE_LOOP ( 'NONE', ( #11275, #44935, #33470, #2811 ) ) ;
#72982=FACE_OUTER_BOUND ( 'NONE', #39985, .T. ) ;
#72983=FACE_OUTER_BOUND ( 'NONE', #14004, .T. ) ;
#72984=EDGE_CURVE ( 'NONE', #37230, #61048, #2723, .T. ) ;
#72985=CARTESIAN_POINT ( 'NONE',  ( 0.2380535369741298979, -2.353723527008297012, 30.78948104536958397 ) ) ;
#72986=B_SPLINE_CURVE_WITH_KNOTS ( 'NONE', 3,
 ( #66785, #33003, #60468, #38428, #38877, #5085, #59578, #4188, #87081, #24451 ),
 .UNSPECIFIED., .F., .F.,
 ( 4, 2, 2, 2, 4 ),
 ( 0.0007817246256747474977, 0.0009771112852218909357, 0.001172497944769034482, 0.001367884604316178029, 0.001563271263863321575 ),
 .UNSPECIFIED. ) ;
#72987=CARTESIAN_POINT ( 'NONE',  ( -14.05763788777885637, -10.06805714834173493, 34.32951233291982618 ) ) ;
#72989=ORIENTED_EDGE ( 'NONE', *, *, #34481, .F. ) ;
#72991=ORIENTED_EDGE ( 'NONE', *, *, #80702, .T. ) ;
#72992=CARTESIAN_POINT ( 'NONE',  ( 3.296836564119306701, -12.62096338111211757, 30.90682066428152908 ) ) ;
#72993=ORIENTED_EDGE ( 'NONE', *, *, #59706, .F. ) ;
#72995=VECTOR ( 'NONE', #21550, 1000.000000000000114 ) ;
#72996=CARTESIAN_POINT ( 'NONE',  ( -8.834501215191545853, -10.21337939537584383, 33.94971097300158647 ) ) ;
#72997=LINE ( 'NONE', #11295, #56857 ) ;
#72998=VERTEX_POINT ( 'NONE', #52664 ) ;
#72999=ORIENTED_EDGE ( 'NONE', *, *, #17151, .T. ) ;
#73000=DIRECTION ( 'NONE',  ( -0.000000000000000000, 0.6427876096865404731, -0.7660444431189771253 ) ) ;
#73001=ORIENTED_EDGE ( 'NONE', *, *, #73458, .F. ) ;
#73002=CARTESIAN_POINT ( 'NONE',  ( 9.915319043920543862, -8.239487800360276282, 34.69522927552633718 ) ) ;
#73003=EDGE_CURVE ( 'NONE', #74304, #56304, #87368, .T. ) ;
#73004=CARTESIAN_POINT ( 'NONE',  ( -11.76194648218548622, -3.754499324213721234, 33.06261337010820256 ) ) ;
#73005=CARTESIAN_POINT ( 'NONE',  ( 0.3962680155776857061, -5.219633306516282545, 34.19971097300152962 ) ) ;
#73006=FACE_BOUND ( 'NONE', #13337, .T. ) ;
#73007=B_SPLINE_CURVE_WITH_KNOTS ( 'NONE', 3,
 ( #80192, #18492, #27019, #13500, #50697, #28336, #27902, #27463, #55809, #75636 ),
 .UNSPECIFIED., .F., .F.,
 ( 4, 2, 2, 2, 4 ),
 ( 0.000000000000000000, 0.0001954339857564074473, 0.0003908679715128148945, 0.0005863019572692223418, 0.0007817359430256297891 ),
 .UNSPECIFIED. ) ;
#73008=CARTESIAN_POINT ( 'NONE',  ( -6.130147209438218781, -6.001485441113818986, 34.52039167877662607 ) ) ;
#73009=CARTESIAN_POINT ( 'NONE',  ( -12.46153846153846168, -1.790695186598648903, 34.54067556320373455 ) ) ;
#73013=CARTESIAN_POINT ( 'NONE',  ( -14.17716660592874334, -6.001044277235009439, 34.52024696741798948 ) ) ;
#73014=CARTESIAN_POINT ( 'NONE',  ( 10.61538461538461675, -5.180354513474913603, 36.12317359536750416 ) ) ;
#73015=CARTESIAN_POINT ( 'NONE',  ( 7.976945653978634532, -10.54018710029568595, 33.71981072465678864 ) ) ;
#73016=ORIENTED_EDGE ( 'NONE', *, *, #28223, .F. ) ;
#73017=EDGE_CURVE ( 'NONE', #38306, #87613, #27472, .T. ) ;
#73018=FACE_OUTER_BOUND ( 'NONE', #45753, .T. ) ;
#73019=EDGE_LOOP ( 'NONE', ( #59140, #83956 ) ) ;
#73022=DIRECTION ( 'NONE',  ( -0.000000000000000000, -0.5000000000000009992, -0.8660254037844380415 ) ) ;
#73023=CARTESIAN_POINT ( 'NONE',  ( -9.442253272394237840, -8.346898887586323923, 34.93166121998716278 ) ) ;
#73024=EDGE_CURVE ( 'NONE', #63890, #33486, #67526, .T. ) ;
#73025=CARTESIAN_POINT ( 'NONE',  ( 3.165499230212911463, -3.643525952247789412, 33.31231777344662959 ) ) ;
#73029=EDGE_LOOP ( 'NONE', ( #32197, #78814, #43169, #31914 ) ) ;
#73030=CARTESIAN_POINT ( 'NONE',  ( -5.207071046654771607, -6.809168938359898782, 34.95455904226513866 ) ) ;
#73031=CARTESIAN_POINT ( 'NONE',  ( -11.53846153846153655, -9.780366693483667717, 34.19971097300155094 ) ) ;
#73032=CARTESIAN_POINT ( 'NONE',  ( -14.24249931939765546, -2.255955759149234741, 29.99999999999988631 ) ) ;
#73033=CARTESIAN_POINT ( 'NONE',  ( -4.023054346021365468, -3.530189275343204702, 32.79018710029569661 ) ) ;
#73034=ORIENTED_EDGE ( 'NONE', *, *, #29996, .F. ) ;
#73035=ADVANCED_FACE ( 'NONE', ( #32405 ), #5382, .F. ) ;
#73036=EDGE_LOOP ( 'NONE', ( #72968, #55207, #62899, #17949 ) ) ;
#73038=ORIENTED_EDGE ( 'NONE', *, *, #39418, .T. ) ;
#73039=CARTESIAN_POINT ( 'NONE',  ( 11.76124120743959978, -12.47679350104403007, 31.42216943046555855 ) ) ;
#73040=CARTESIAN_POINT ( 'NONE',  ( -5.777036865733325754, -7.369474539155828730, 34.99858011523957657 ) ) ;
#73041=EDGE_LOOP ( 'NONE', ( #81071, #44300 ) ) ;
#73042=DIRECTION ( 'NONE',  ( -0.000000000000000000, -0.7660444431189791237, -0.6427876096865379196 ) ) ;
#73043=FACE_OUTER_BOUND ( 'NONE', #25786, .T. ) ;
#73044=CARTESIAN_POINT ( 'NONE',  ( 5.076923076923075762, -2.721908614388771852, 31.22303859784724978 ) ) ;
#73045=CARTESIAN_POINT ( 'NONE',  ( -17.07692307692319744, -12.27809138561165270, 31.22303859784587132 ) ) ;
#73047=ORIENTED_EDGE ( 'NONE', *, *, #75120, .F. ) ;
#73048=CARTESIAN_POINT ( 'NONE',  ( -7.846153846153844924, -9.780366693483667717, 34.19971097300155094 ) ) ;
#73050=DIRECTION ( 'NONE',  ( 0.000000000000000000, 0.1736481776669275834, 0.9848077530122086864 ) ) ;
#73051=CARTESIAN_POINT ( 'NONE',  ( 4.153846153846032507, -6.879047030192662504, 34.71129190930017927 ) ) ;
#73052=CARTESIAN_POINT ( 'NONE',  ( -11.53846153846153655, -2.499999999999998668, 29.75000000000001421 ) ) ;
#73054=CARTESIAN_POINT ( 'NONE',  ( -5.869954944080226333, -2.254550872974306674, 29.97347326024527447 ) ) ;
#73055=B_SPLINE_CURVE_WITH_KNOTS ( 'NONE', 3,
 ( #43899, #83124, #56531, #21415, #1143, #29077, #15109, #9671, #50196, #8798 ),
 .UNSPECIFIED., .F., .F.,
 ( 4, 2, 2, 2, 4 ),
 ( 0.000000000000000000, 0.0001954311564186875520, 0.0003908623128373751041, 0.0005862934692560627103, 0.0007817246256747502082 ),
 .UNSPECIFIED. ) ;
#73056=CARTESIAN_POINT ( 'NONE',  ( 17.99999999999987566, -2.625532179533778709, 30.86335684631627174 ) ) ;
#73057=B_SPLINE_CURVE_WITH_KNOTS ( 'NONE', 3,
 ( #46237, #53878, #27730, #39937, #18770, #20094, #34493, #75476, #74600, #47558 ),
 .UNSPECIFIED., .F., .F.,
 ( 4, 2, 2, 2, 4 ),
 ( 0.000000000000000000, 0.0001954339857564063089, 0.0003908679715128126177, 0.0005863019572692189808, 0.0007817359430256252354 ),
 .UNSPECIFIED. ) ;
#73059=ORIENTED_EDGE ( 'NONE', *, *, #67055, .T. ) ;
#73060=EDGE_CURVE ( 'NONE', #55169, #60609, #88750, .T. ) ;
#73061=CARTESIAN_POINT ( 'NONE',  ( 14.08476534878545827, -2.308479472611653094, 30.53278059502174457 ) ) ;
#73062=CARTESIAN_POINT ( 'NONE',  ( 7.596153846153846700, -7.500000000000001776, 35.00000000000000000 ) ) ;
#73063=CARTESIAN_POINT ( 'NONE',  ( -0.3954701105360233782, -4.786620604624112651, 33.94971097300155094 ) ) ;
#73064=ORIENTED_EDGE ( 'NONE', *, *, #88412, .F. ) ;
#73065=ORIENTED_EDGE ( 'NONE', *, *, #50162, .T. ) ;
#73066=CARTESIAN_POINT ( 'NONE',  ( -11.60454494941741999, -10.51840700105979387, 33.73612834413961536 ) ) ;
#73067=CARTESIAN_POINT ( 'NONE',  ( -7.715363405186893786, -5.496552790871119143, 34.60292014791297532 ) ) ;
#73068=CARTESIAN_POINT ( 'NONE',  ( 17.14217821643591932, -3.643525952247864019, 33.31231777344670064 ) ) ;
#73069=CARTESIAN_POINT ( 'NONE',  ( -8.769230769230768274, -10.67929555188718282, 33.92786785259544047 ) ) ;
#73071=CARTESIAN_POINT ( 'NONE',  ( 17.93472999944368240, -12.16647553114622049, 32.15551576947930812 ) ) ;
#73072=FACE_OUTER_BOUND ( 'NONE', #41166, .T. ) ;
#73073=ORIENTED_EDGE ( 'NONE', *, *, #30444, .F. ) ;
#73075=EDGE_CURVE ( 'NONE', #12820, #72772, #15671, .T. ) ;
#73076=CARTESIAN_POINT ( 'NONE',  ( -6.065324012804307330, -7.749976730030849303, 34.74374725381503737 ) ) ;
#73077=DIRECTION ( 'NONE',  ( 0.000000000000000000, 1.000000000000000000, 0.000000000000000000 ) ) ;
#73079=CARTESIAN_POINT ( 'NONE',  ( 12.23861150263160802, -2.523278758544489797, 31.42238647778637528 ) ) ;
#73080=ORIENTED_EDGE ( 'NONE', *, *, #18308, .T. ) ;
#73081=AXIS2_PLACEMENT_3D ( 'NONE', #38380, #17671, #24857 ) ;
#73082=CARTESIAN_POINT ( 'NONE',  ( 1.515453802628148772, -7.277220443632450575, 34.74524770363009196 ) ) ;
#73084=DIRECTION ( 'NONE',  ( -0.000000000000000000, 0.7660444431189791237, -0.6427876096865379196 ) ) ;
#73085=CARTESIAN_POINT ( 'NONE',  ( 17.93472999944368240, -10.33852847137145048, 34.16647553114627556 ) ) ;
#73086=VERTEX_POINT ( 'NONE', #75175 ) ;
#73087=DIRECTION ( 'NONE',  ( -0.000000000000000000, -0.000000000000000000, -1.000000000000000000 ) ) ;
#73088=CARTESIAN_POINT ( 'NONE',  ( 13.63466980452883526, -9.233818618650603938, 34.70587769442853698 ) ) ;
#73089=EDGE_CURVE ( 'NONE', #21246, #75513, #82376, .T. ) ;
#73090=CARTESIAN_POINT ( 'NONE',  ( 17.07692307692307665, -9.905515769479276145, 34.41647553114623292 ) ) ;
#73091=AXIS2_PLACEMENT_3D ( 'NONE', #79633, #17930, #58450 ) ;
#73093=CARTESIAN_POINT ( 'NONE',  ( -2.084912638714240707, -10.97394488606064122, 33.68653795673694873 ) ) ;
#73094=EDGE_CURVE ( 'NONE', #9934, #65490, #72753, .T. ) ;
#73095=EDGE_CURVE ( 'NONE', #58120, #70789, #42467, .T. ) ;
#73096=VECTOR ( 'NONE', #59904, 1000.000000000000114 ) ;
#73097=ORIENTED_EDGE ( 'NONE', *, *, #76385, .F. ) ;
#73099=EDGE_LOOP ( 'NONE', ( #59306, #42762 ) ) ;
#73100=CARTESIAN_POINT ( 'NONE',  ( -15.10024379253558635, -6.808710257144161559, 34.95449254468098843 ) ) ;
#73101=EDGE_CURVE ( 'NONE', #4777, #80366, #835, .T. ) ;
#73102=CARTESIAN_POINT ( 'NONE',  ( -9.561781990544126586, -12.27024696741798948, 31.24895572276497546 ) ) ;
#73103=CARTESIAN_POINT ( 'NONE',  ( -13.44988583057615905, -2.892918686051582977, 31.69288490824015980 ) ) ;
#73104=DIRECTION ( 'NONE',  ( -0.000000000000000000, -0.9848077530122086864, -0.1736481776669273613 ) ) ;
#73106=CARTESIAN_POINT ( 'NONE',  ( 9.562160482869472844, -8.587444163452046197, 34.63053765926554206 ) ) ;
#73107=EDGE_LOOP ( 'NONE', ( #32878, #65124 ) ) ;
#73109=ORIENTED_EDGE ( 'NONE', *, *, #75535, .T. ) ;
#73110=ORIENTED_EDGE ( 'NONE', *, *, #16887, .T. ) ;
#73111=EDGE_LOOP ( 'NONE', ( #18667, #6819, #18156, #82176 ) ) ;
#73113=DIRECTION ( 'NONE',  ( 0.000000000000000000, 0.9848077530122072432, -0.1736481776669354937 ) ) ;
#73114=AXIS2_PLACEMENT_3D ( 'NONE', #51734, #17986, #72469 ) ;
#73115=CARTESIAN_POINT ( 'NONE',  ( -2.373016320496614817, -7.749976730030849303, 34.74374725381503737 ) ) ;
#73116=CARTESIAN_POINT ( 'NONE',  ( 6.923076923076800782, -12.16647553114689728, 32.15551576947799362 ) ) ;
#73117=CARTESIAN_POINT ( 'NONE',  ( 13.13463865367303285, -8.303909089506435137, 34.68538101551103381 ) ) ;
#73119=CARTESIAN_POINT ( 'NONE',  ( -6.249976744048591826, -2.920706130388546651, 32.31842814019191223 ) ) ;
#73122=CARTESIAN_POINT ( 'NONE',  ( 0.4615384615383396616, -3.300289026999228881, 32.46337939537708905 ) ) ;
#73123=ORIENTED_EDGE ( 'NONE', *, *, #67177, .F. ) ;
#73124=ORIENTED_EDGE ( 'NONE', *, *, #59328, .F. ) ;
#73125=ORIENTED_EDGE ( 'NONE', *, *, #61560, .T. ) ;
#73126=CARTESIAN_POINT ( 'NONE',  ( 11.66898697669518192, -2.647132371071621471, 31.75357179365171589 ) ) ;
#73127=EDGE_LOOP ( 'NONE', ( #2230, #2910 ) ) ;
#73128=CARTESIAN_POINT ( 'NONE',  ( 0.4615384615384611200, -2.499999999999998668, 29.75000000000001421 ) ) ;
#73129=CARTESIAN_POINT ( 'NONE',  ( -16.37733109757010652, -10.11188796281391511, 34.01382737946119050 ) ) ;
#73131=CARTESIAN_POINT ( 'NONE',  ( -1.161239898842963969, -2.251407671071270489, 29.88021292934942252 ) ) ;
#73132=CARTESIAN_POINT ( 'NONE',  ( -11.28851612908349722, -9.357781135181031829, 34.66075350412533851 ) ) ;
#73133=FACE_BOUND ( 'NONE', #77979, .T. ) ;
#73134=ORIENTED_EDGE ( 'NONE', *, *, #8114, .F. ) ;
#73135=ORIENTED_EDGE ( 'NONE', *, *, #51036, .T. ) ;
#73136=EDGE_CURVE ( 'NONE', #47964, #45215, #80106, .T. ) ;
#73137=DIRECTION ( 'NONE',  ( -0.000000000000000000, -0.7660444431189791237, -0.6427876096865379196 ) ) ;
#73138=ORIENTED_EDGE ( 'NONE', *, *, #8728, .T. ) ;
#73139=FACE_BOUND ( 'NONE', #51004, .T. ) ;
#73140=CARTESIAN_POINT ( 'NONE',  ( -8.769230769230768274, -1.790695186598648903, 34.54067556320373455 ) ) ;
#73141=VECTOR ( 'NONE', #26643, 1000.000000000000114 ) ;
#73142=CARTESIAN_POINT ( 'NONE',  ( -39.05038313613820122, -2.249999999999998668, 29.75000000000000355 ) ) ;
#73143=ORIENTED_EDGE ( 'NONE', *, *, #51036, .F. ) ;
#73144=CARTESIAN_POINT ( 'NONE',  ( -15.00798968950081580, -12.24180327182772388, 31.33663988360758168 ) ) ;
#73145=CARTESIAN_POINT ( 'NONE',  ( 8.638755584155049405, -7.276987145209184327, 34.99546412871779211 ) ) ;
#73146=CARTESIAN_POINT ( 'NONE',  ( -5.326923076923075762, -7.500000000000001776, 35.00000000000000000 ) ) ;
#73147=VERTEX_POINT ( 'NONE', #83259 ) ;
#73148=B_SPLINE_CURVE_WITH_KNOTS ( 'NONE', 3,
 ( #51675, #45827, #17922, #80971, #45377, #25116, #65203, #17479, #39093, #72407 ),
 .UNSPECIFIED., .F., .F.,
 ( 4, 2, 2, 2, 4 ),
 ( 0.0007817359430256332585, 0.0009771253907250054306, 0.001172514838424370664, 0.001367904286123735897, 0.001563293733823100913 ),
 .UNSPECIFIED. ) ;
#73149=CARTESIAN_POINT ( 'NONE',  ( -1.384615384615383471, -13.75783147151868846, 33.36296068462461051 ) ) ;
#73150=CARTESIAN_POINT ( 'NONE',  ( 7.173022332454967120, -5.766571408460171355, 34.70601412856602508 ) ) ;
#73151=DIRECTION ( 'NONE',  ( 1.000000000000000000, 0.000000000000000000, 0.000000000000000000 ) ) ;
#73152=VERTEX_POINT ( 'NONE', #29210 ) ;
#73154=EDGE_CURVE ( 'NONE', #58651, #39220, #69300, .T. ) ;
#73155=CARTESIAN_POINT ( 'NONE',  ( -2.438383774359863754, -11.18331474514187995, 33.13161551792790505 ) ) ;
#73156=CARTESIAN_POINT ( 'NONE',  ( -17.07692307692319744, -11.94971097300221174, 32.03036669348237098 ) ) ;
#73158=VERTEX_POINT ( 'NONE', #56662 ) ;
#73159=CARTESIAN_POINT ( 'NONE',  ( -17.07692307692307665, -12.62096338111211580, 30.90682066428153263 ) ) ;
#73160=CARTESIAN_POINT ( 'NONE',  ( -15.23076923076922995, -7.500000000000001776, 35.04278698407183867 ) ) ;
#73161=CARTESIAN_POINT ( 'NONE',  ( -15.90379184220783948, -8.303483539816726378, 34.68545999027711702 ) ) ;
#73162=CYLINDRICAL_SURFACE ( 'NONE', #64442, 0.2500000000000009437 ) ;
#73163=DIRECTION ( 'NONE',  ( -0.000000000000000000, -0.9396926207859093161, -0.3420201433256663259 ) ) ;
#73164=DIRECTION ( 'NONE',  ( 0.000000000000000000, 0.8660254037844377084, -0.5000000000000015543 ) ) ;
#73165=CARTESIAN_POINT ( 'NONE',  ( -1.634592115557738756, -4.943428324936578910, 34.04746400365624481 ) ) ;
#73166=CARTESIAN_POINT ( 'NONE',  ( 8.639082799499073317, -3.069018819979302926, 32.56621877034667278 ) ) ;
#73167=VECTOR ( 'NONE', #61451, 999.9999999999998863 ) ;
#73168=CARTESIAN_POINT ( 'NONE',  ( -16.02305434602136458, -11.71459661697925903, 32.44059661609676937 ) ) ;
#73169=CARTESIAN_POINT ( 'NONE',  ( -15.10024379253559168, -2.647132371071621471, 31.75357179365171589 ) ) ;
#73170=CARTESIAN_POINT ( 'NONE',  ( -5.999999999999998224, -1.117168528481311540, 33.14645433367849847 ) ) ;
#73173=EDGE_CURVE ( 'NONE', #32782, #44632, #14803, .T. ) ;
#73174=CARTESIAN_POINT ( 'NONE',  ( -12.71151519248081740, -8.303909089506435137, 34.68538101551103381 ) ) ;
#73175=EDGE_LOOP ( 'NONE', ( #24774, #39151 ) ) ;
#73176=ORIENTED_EDGE ( 'NONE', *, *, #68375, .T. ) ;
#73178=CYLINDRICAL_SURFACE ( 'NONE', #48398, 0.2500000000000008882 ) ;
#73179=ORIENTED_EDGE ( 'NONE', *, *, #25122, .F. ) ;
#73180=CARTESIAN_POINT ( 'NONE',  ( -15.23076923076935074, -6.026961402154118019, 34.52809138561165270 ) ) ;
#73182=CARTESIAN_POINT ( 'NONE',  ( 3.230769230769108269, -2.379036618888197285, 30.90682066428292885 ) ) ;
#73183=CARTESIAN_POINT ( 'NONE',  ( 5.934729554039225974, -11.48612834413959582, 32.76840700105983473 ) ) ;
#73184=CARTESIAN_POINT ( 'NONE',  ( -7.846153846153844924, -5.557115091759785130, 34.35708131394839171 ) ) ;
#73185=CARTESIAN_POINT ( 'NONE',  ( 9.757562831820530747, -3.083524468853784839, 32.58852847137153930 ) ) ;
#73186=CARTESIAN_POINT ( 'NONE',  ( -10.61538461538473577, -3.643525952248795718, 33.31231777344771672 ) ) ;
#73187=CARTESIAN_POINT ( 'NONE',  ( 0.5920638997721058283, -5.915461855592777596, 34.75538340440931506 ) ) ;
#73188=CARTESIAN_POINT ( 'NONE',  ( 0.5920638997721026087, -2.647132371071621471, 31.75357179365173010 ) ) ;
#73190=LINE ( 'NONE', #19132, #11783 ) ;
#73192=EDGE_CURVE ( 'NONE', #20258, #56147, #34173, .T. ) ;
#73193=EDGE_CURVE ( 'NONE', #5405, #43224, #4988, .T. ) ;
#73195=CIRCLE ( 'NONE', #70295, 0.2500000000000002220 ) ;
#73196=ORIENTED_EDGE ( 'NONE', *, *, #10725, .F. ) ;
#73197=ORIENTED_EDGE ( 'NONE', *, *, #63446, .T. ) ;
#73198=B_SPLINE_CURVE_WITH_KNOTS ( 'NONE', 3,
 ( #38840, #36287, #4602, #32075, #72162, #22321, #15571, #43037, #63744, #51419 ),
 .UNSPECIFIED., .F., .F.,
 ( 4, 2, 2, 2, 4 ),
 ( 0.0007817246256747550871, 0.0009771112852218989588, 0.001172497944769042939, 0.001367884604316186702, 0.001563271263863330682 ),
 .UNSPECIFIED. ) ;
#73199=CARTESIAN_POINT ( 'NONE',  ( -9.627052121031661969, -3.835265460703683349, 33.15142922261929925 ) ) ;
#73200=FACE_OUTER_BOUND ( 'NONE', #56209, .T. ) ;
#73201=FACE_OUTER_BOUND ( 'NONE', #51865, .T. ) ;
#73203=B_SPLINE_CURVE_WITH_KNOTS ( 'NONE', 3,
 ( #68174, #88471, #69058, #40269, #39822, #5584, #68611, #61396, #25858, #26740 ),
 .UNSPECIFIED., .F., .F.,
 ( 4, 2, 2, 2, 4 ),
 ( 0.0007817246256747442451, 0.0009771112852218870326, 0.001172497944769029929, 0.001367884604316172825, 0.001563271263863315504 ),
 .UNSPECIFIED. ) ;
#73204=CARTESIAN_POINT ( 'NONE',  ( 8.545745825506822158, -11.89387501736622710, 32.13663884655806413 ) ) ;
#73205=ADVANCED_FACE ( 'NONE', ( #36398 ), #78254, .F. ) ;
#73206=CARTESIAN_POINT ( 'NONE',  ( -16.21911659980693443, -9.442884908240170461, 34.35708131394840592 ) ) ;
#73207=EDGE_CURVE ( 'NONE', #33353, #35763, #46766, .T. ) ;
#73208=ADVANCED_FACE ( 'NONE', ( #44910 ), #31407, .F. ) ;
#73209=ORIENTED_EDGE ( 'NONE', *, *, #80267, .F. ) ;
#73210=CARTESIAN_POINT ( 'NONE',  ( 2.980792486720640344, -6.524016743844655686, 34.90889640711025521 ) ) ;
#73211=ORIENTED_EDGE ( 'NONE', *, *, #68707, .F. ) ;
#73212=VERTEX_POINT ( 'NONE', #77376 ) ;
#73213=CARTESIAN_POINT ( 'NONE',  ( 0.6843181305165279005, -12.47679350104403007, 31.42216943046555855 ) ) ;
#73214=CARTESIAN_POINT ( 'NONE',  ( 4.153846153846154188, -2.538708090699994813, 30.37095296980875503 ) ) ;
#73215=CARTESIAN_POINT ( 'NONE',  ( -4.403869378067610363, -12.68155406624981119, 30.59749803192733708 ) ) ;
#73216=CYLINDRICAL_SURFACE ( 'NONE', #70981, 0.2499999999999995559 ) ;
#73217=CARTESIAN_POINT ( 'NONE',  ( 13.13463864056679675, -5.643011162660950042, 34.66104346484419096 ) ) ;
#73218=AXIS2_PLACEMENT_3D ( 'NONE', #69123, #83087, #21374 ) ;
#73219=EDGE_LOOP ( 'NONE', ( #26319, #63143, #5442, #71229 ) ) ;
#73220=ORIENTED_EDGE ( 'NONE', *, *, #43555, .T. ) ;
#73221=ORIENTED_EDGE ( 'NONE', *, *, #45308, .F. ) ;
#73222=B_SPLINE_CURVE_WITH_KNOTS ( 'NONE', 3,
 ( #38154, #58867, #16548, #44015, #4372, #65173, #86368, #3472, #71486, #85903 ),
 .UNSPECIFIED., .F., .F.,
 ( 4, 2, 2, 2, 4 ),
 ( 0.000000000000000000, 0.0001954311564186879315, 0.0003908623128373758630, 0.0005862934692560637946, 0.0007817246256747517261 ),
 .UNSPECIFIED. ) ;
#73225=B_SPLINE_CURVE_WITH_KNOTS ( 'NONE', 3,
 ( #65489, #9656, #51060, #15984, #23611, #10101, #30376, #37567, #65030, #29938 ),
 .UNSPECIFIED., .F., .F.,
 ( 4, 2, 2, 2, 4 ),
 ( 0.000000000000000000, 0.0001954339857564075286, 0.0003908679715128150572, 0.0005863019572692225586, 0.0007817359430256301143 ),
 .UNSPECIFIED. ) ;
#73226=CARTESIAN_POINT ( 'NONE',  ( 16.28437159207980045, -5.915461855592777596, 34.75538340440931506 ) ) ;
#73227=CARTESIAN_POINT ( 'NONE',  ( 1.319344938654610777, -3.835265460703609186, 33.15142922261924241 ) ) ;
#73228=CARTESIAN_POINT ( 'NONE',  ( -4.088700374514188773, -7.750023238201980469, 34.74374492549440419 ) ) ;
#73229=CARTESIAN_POINT ( 'NONE',  ( 17.86930853333243974, -8.147922237126337563, 34.70805685702651999 ) ) ;
#73230=ORIENTED_EDGE ( 'NONE', *, *, #77019, .F. ) ;
#73231=EDGE_LOOP ( 'NONE', ( #57132, #36681 ) ) ;
#73232=CARTESIAN_POINT ( 'NONE',  ( 4.826899852701619587, -10.18141759479407327, 34.26406193332782379 ) ) ;
#73233=CARTESIAN_POINT ( 'NONE',  ( -13.38461538461538325, -5.471508081941601098, 34.59228464037088457 ) ) ;
#73234=VERTEX_POINT ( 'NONE', #8930 ) ;
#73235=CARTESIAN_POINT ( 'NONE',  ( 8.069165197766698938, -12.39991518177334129, 30.74647679643404530 ) ) ;
#73236=CARTESIAN_POINT ( 'NONE',  ( -7.053636836690285961, -2.254533558242299396, 29.97296025877828285 ) ) ;
#73237=CARTESIAN_POINT ( 'NONE',  ( -5.999999999999998224, -6.386643153685126251, 34.62446782046654192 ) ) ;
#73238=EDGE_LOOP ( 'NONE', ( #55432, #54049 ) ) ;
#73239=CYLINDRICAL_SURFACE ( 'NONE', #12387, 0.2500000000000002220 ) ;
#73240=AXIS2_PLACEMENT_3D ( 'NONE', #52877, #19545, #39390 ) ;
#73241=ORIENTED_EDGE ( 'NONE', *, *, #57726, .F. ) ;
#73243=LINE ( 'NONE', #59275, #77420 ) ;
#73244=CARTESIAN_POINT ( 'NONE',  ( 7.596177102105253987, -4.075325502946086864, 33.72974371597207721 ) ) ;
#73245=CARTESIAN_POINT ( 'NONE',  ( 14.05769230769230838, -7.500000000000001776, 35.04278698407183867 ) ) ;
#73247=CARTESIAN_POINT ( 'NONE',  ( -10.83831083290075803, -10.61292498521070549, 33.66303323003028680 ) ) ;
#73248=EDGE_LOOP ( 'NONE', ( #82153, #11355, #25425, #66813 ) ) ;
#73251=CARTESIAN_POINT ( 'NONE',  ( 20.74999999999999645, -4.499999999999999112, 29.75000000000000355 ) ) ;
#73252=ORIENTED_EDGE ( 'NONE', *, *, #45633, .F. ) ;
#73253=B_SPLINE_CURVE_WITH_KNOTS ( 'NONE', 3,
 ( #63716, #2022, #29505, #50191, #77677, #43453, #70929, #64150, #2453, #29943 ),
 .UNSPECIFIED., .F., .F.,
 ( 4, 2, 2, 2, 4 ),
 ( 0.000000000000000000, 0.0001954339857564074473, 0.0003908679715128148945, 0.0005863019572692223418, 0.0007817359430256297891 ),
 .UNSPECIFIED. ) ;
#73254=B_SPLINE_CURVE_WITH_KNOTS ( 'NONE', 3,
 ( #19809, #5411, #87854, #47270, #74759, #60340, #6300, #27009, #26119, #81966 ),
 .UNSPECIFIED., .F., .F.,
 ( 4, 2, 2, 2, 4 ),
 ( 0.000000000000000000, 0.0001954339857564092362, 0.0003908679715128184724, 0.0005863019572692276544, 0.0007817359430256369448 ),
 .UNSPECIFIED. ) ;
#73255=CARTESIAN_POINT ( 'NONE',  ( -9.626240358957616650, -4.661471528628508665, 34.16647553114624003 ) ) ;
#73256=CARTESIAN_POINT ( 'NONE',  ( -6.000000000000119904, -10.90142922262034020, 33.41473453929536674 ) ) ;
#73257=CYLINDRICAL_SURFACE ( 'NONE', #68770, 0.2500000000000008882 ) ;
#73258=DIRECTION ( 'NONE',  ( 0.000000000000000000, 0.000000000000000000, 1.000000000000000000 ) ) ;
#73259=FACE_BOUND ( 'NONE', #4520, .T. ) ;
#73260=DIRECTION ( 'NONE',  ( -0.000000000000000000, -0.000000000000000000, -1.000000000000000000 ) ) ;
#73261=CARTESIAN_POINT ( 'NONE',  ( -7.846153846153844924, -2.486705287966279876, 31.30864560766543647 ) ) ;
#73262=CARTESIAN_POINT ( 'NONE',  ( 9.915683633005873077, -2.501478030877322567, 29.88021232661721172 ) ) ;
#73263=CARTESIAN_POINT ( 'NONE',  ( -0.4615384615384611200, -5.557115091759785130, 34.35708131394839171 ) ) ;
#73264=DIRECTION ( 'NONE',  ( -0.000000000000000000, 0.6427876096865404731, -0.7660444431189770143 ) ) ;
#73265=CARTESIAN_POINT ( 'NONE',  ( 12.33139125210024112, -12.45813303252208648, 30.39737893381572675 ) ) ;
#73266=CARTESIAN_POINT ( 'NONE',  ( 13.16113046005105325, -2.612411019501189369, 31.66733052389439962 ) ) ;
#73268=DIRECTION ( 'NONE',  ( -0.000000000000000000, -0.5000000000000009992, -0.8660254037844380415 ) ) ;
#73269=ORIENTED_EDGE ( 'NONE', *, *, #6852, .T. ) ;
#73270=EDGE_CURVE ( 'NONE', #88317, #68189, #24253, .T. ) ;
#73272=AXIS2_PLACEMENT_3D ( 'NONE', #18278, #87200, #80884 ) ;
#73273=CARTESIAN_POINT ( 'NONE',  ( 12.46153846153846168, -2.499999999999998668, 29.75000000000001421 ) ) ;
#73276=CARTESIAN_POINT ( 'NONE',  ( -2.307692307692427391, -11.94971097300221174, 32.03036669348237098 ) ) ;
#73278=CARTESIAN_POINT ( 'NONE',  ( -16.94639763868943660, -2.372941743896878286, 30.88044141588253311 ) ) ;
#73279=CARTESIAN_POINT ( 'NONE',  ( 9.692307692307572609, -2.892918686052165622, 31.69288490824153470 ) ) ;
#73281=CARTESIAN_POINT ( 'NONE',  ( 14.24160889673643027, -10.51840700105979387, 33.73612834413961536 ) ) ;
#73282=CARTESIAN_POINT ( 'NONE',  ( 1.384615384615386802, -13.20930481340135110, 34.54067556320372745 ) ) ;
#73283=VECTOR ( 'NONE', #48304, 999.9999999999998863 ) ;
#73284=DIRECTION ( 'NONE',  ( 0.000000000000000000, 0.000000000000000000, 1.000000000000000000 ) ) ;
#73285=CARTESIAN_POINT ( 'NONE',  ( 4.853996118016225658, -9.172386477786396597, 34.72672124145550043 ) ) ;
#73286=CARTESIAN_POINT ( 'NONE',  ( -7.173053654019277303, -4.236021600441998380, 33.53823185664189310 ) ) ;
#73287=CARTESIAN_POINT ( 'NONE',  ( 1.384615384615264011, -10.33852847137269571, 34.16647553114546554 ) ) ;
#73288=AXIS2_PLACEMENT_3D ( 'NONE', #27212, #68639, #54669 ) ;
#73289=CARTESIAN_POINT ( 'NONE',  ( -2.057692307692306599, -2.249999999999998668, 29.75000000000000355 ) ) ;
#73291=CARTESIAN_POINT ( 'NONE',  ( -1.161835715637319133, -12.11081565061823717, 32.26097654155341843 ) ) ;
#73292=EDGE_LOOP ( 'NONE', ( #68159, #12510 ) ) ;
#73293=CARTESIAN_POINT ( 'NONE',  ( 16.37685899793954292, -4.762714258010882773, 34.23016756924214832 ) ) ;
#73294=DIRECTION ( 'NONE',  ( -0.000000000000000000, -0.8660254037844399289, -0.4999999999999980016 ) ) ;
#73296=CARTESIAN_POINT ( 'NONE',  ( 7.053867364043872712, -10.70102852606553157, 33.91149625220312913 ) ) ;
#73297=CARTESIAN_POINT ( 'NONE',  ( -1.384615384615505151, -12.27809138561165270, 31.22303859784587132 ) ) ;
#73298=ORIENTED_EDGE ( 'NONE', *, *, #16056, .F. ) ;
#73299=FACE_OUTER_BOUND ( 'NONE', #41212, .T. ) ;
#73300=CARTESIAN_POINT ( 'NONE',  ( 0.7115384615384606759, -7.500000000000001776, 35.04278698407183867 ) ) ;
#73301=CARTESIAN_POINT ( 'NONE',  ( 5.076923076923075762, -12.34228464037088635, 31.77849191805839268 ) ) ;
#73303=CARTESIAN_POINT ( 'NONE',  ( -13.13456107297707121, -11.28795663066794575, 33.01431243580653785 ) ) ;
#73304=CARTESIAN_POINT ( 'NONE',  ( 5.076923076923075762, -6.435427911321262684, 35.78748833219616898 ) ) ;
#73305=CARTESIAN_POINT ( 'NONE',  ( -8.769230769230768274, -2.538708090699994813, 30.37095296980875503 ) ) ;
#73306=DIRECTION ( 'NONE',  ( 0.000000000000000000, 0.9396926207859126468, -0.3420201433256571111 ) ) ;
#73307=ORIENTED_EDGE ( 'NONE', *, *, #48021, .T. ) ;
#73308=B_SPLINE_CURVE_WITH_KNOTS ( 'NONE', 3,
 ( #67505, #73368, #5797, #4918, #19755, #12122, #54416, #32384, #12558, #61170 ),
 .UNSPECIFIED., .F., .F.,
 ( 4, 2, 2, 2, 4 ),
 ( 0.000000000000000000, 0.0001954311564186868202, 0.0003908623128373736404, 0.0005862934692560604335, 0.0007817246256747472808 ),
 .UNSPECIFIED. ) ;
#73309=CARTESIAN_POINT ( 'NONE',  ( -10.61538461538461320, -1.215029322943914858, 32.30358669280327177 ) ) ;
#73310=CARTESIAN_POINT ( 'NONE',  ( -6.000000000000119904, -12.27809138561165270, 31.22303859784587132 ) ) ;
#73311=ADVANCED_FACE ( 'NONE', ( #72384 ), #63858, .F. ) ;
#73312=DIRECTION ( 'NONE',  ( 0.000000000000000000, 0.3420201433256610524, 0.9396926207859113145 ) ) ;
#73313=ORIENTED_EDGE ( 'NONE', *, *, #35544, .T. ) ;
#73314=ORIENTED_EDGE ( 'NONE', *, *, #33915, .T. ) ;
#73315=EDGE_CURVE ( 'NONE', #83108, #15672, #10696, .T. ) ;
#73316=ORIENTED_EDGE ( 'NONE', *, *, #96, .T. ) ;
#73317=EDGE_CURVE ( 'NONE', #36016, #38481, #71479, .T. ) ;
#73318=CARTESIAN_POINT ( 'NONE',  ( -9.915792636031637741, -2.847400154188067578, 31.58180166144859058 ) ) ;
#73319=CARTESIAN_POINT ( 'NONE',  ( -3.165514091256391271, -3.083524468853784839, 32.58852847137153930 ) ) ;
#73320=B_SPLINE_CURVE_WITH_KNOTS ( 'NONE', 3,
 ( #9046, #17118, #22111, #49582, #50453, #70744, #43701, #56774, #51312, #57224 ),
 .UNSPECIFIED., .F., .F.,
 ( 4, 2, 2, 2, 4 ),
 ( 0.0007817246256747460882, 0.0009771112852218892010, 0.001172497944769032314, 0.001367884604316175210, 0.001563271263863318323 ),
 .UNSPECIFIED. ) ;
#73321=DIRECTION ( 'NONE',  ( 0.000000000000000000, -6.938893903907222067E-15, 1.000000000000000000 ) ) ;
#73322=B_SPLINE_CURVE_WITH_KNOTS ( 'NONE', 3,
 ( #17277, #86200, #51935, #44734, #78090, #37995 ),
 .UNSPECIFIED., .F., .F.,
 ( 4, 2, 4 ),
 ( 2.823925224926892107E-17, 0.0001954756301636994555, 0.0003909512603273706676 ),
 .UNSPECIFIED. ) ;
#73323=CARTESIAN_POINT ( 'NONE',  ( 15.10007776410167502, -3.530157926970578952, 32.79014554554150607 ) ) ;
#73324=ORIENTED_EDGE ( 'NONE', *, *, #82111, .F. ) ;
#73326=CARTESIAN_POINT ( 'NONE',  ( 10.74542967130438953, -2.254550872974306674, 29.97347326024527092 ) ) ;
#73327=ORIENTED_EDGE ( 'NONE', *, *, #6377, .F. ) ;
#73328=CARTESIAN_POINT ( 'NONE',  ( -16.28399412357785536, -12.50552854090298638, 31.33409797877408920 ) ) ;
#73329=CARTESIAN_POINT ( 'NONE',  ( -3.454254155333562171, -4.988325925672468131, 34.36044203135681130 ) ) ;
#73330=VECTOR ( 'NONE', #31840, 1000.000000000000000 ) ;
#73331=AXIS2_PLACEMENT_3D ( 'NONE', #11754, #25264, #72109 ) ;
#73332=CARTESIAN_POINT ( 'NONE',  ( 10.61538461538461675, -11.16473453929635440, 33.15142922261926373 ) ) ;
#73333=CARTESIAN_POINT ( 'NONE',  ( 13.38461538461538680, -9.905515769479276145, 34.41647553114623292 ) ) ;
#73334=EDGE_LOOP ( 'NONE', ( #76011, #43889, #82546, #76548 ) ) ;
#73335=VECTOR ( 'NONE', #18797, 1000.000000000000000 ) ;
#73337=VECTOR ( 'NONE', #75995, 999.9999999999998863 ) ;
#73338=ORIENTED_EDGE ( 'NONE', *, *, #26822, .F. ) ;
#73339=CARTESIAN_POINT ( 'NONE',  ( -8.703163435880695076, -11.91647553114624358, 32.58852847137148245 ) ) ;
#73340=CARTESIAN_POINT ( 'NONE',  ( 15.23076923076911093, -2.625532179533778709, 30.86335684631627174 ) ) ;
#73341=EDGE_LOOP ( 'NONE', ( #20626, #44656 ) ) ;
#73342=CARTESIAN_POINT ( 'NONE',  ( 18.22277966897806678, -12.11081565061823717, 32.26097654155341843 ) ) ;
#73343=CARTESIAN_POINT ( 'NONE',  ( -13.60754160213153163, -6.503392248772476236, 34.64988816332204635 ) ) ;
#73344=CARTESIAN_POINT ( 'NONE',  ( 6.700211500873284542, -2.501496062324911840, 29.88072118266895671 ) ) ;
#73345=LINE ( 'NONE', #52618, #1965 ) ;
#73346=CYLINDRICAL_SURFACE ( 'NONE', #84281, 0.2500000000000002220 ) ;
#73347=FACE_BOUND ( 'NONE', #59962, .T. ) ;
#73349=CARTESIAN_POINT ( 'NONE',  ( -6.223484924564331777, -12.47654668319379567, 31.42292124445336654 ) ) ;
#73350=CARTESIAN_POINT ( 'NONE',  ( -10.36543920600657209, -10.92531984108285670, 33.72920026020278073 ) ) ;
#73351=DIRECTION ( 'NONE',  ( -0.000000000000000000, -0.5000000000000009992, -0.8660254037844380415 ) ) ;
#73352=CARTESIAN_POINT ( 'NONE',  ( 15.29683656411930848, -9.905515769479276145, 34.41647553114623292 ) ) ;
#73356=CARTESIAN_POINT ( 'NONE',  ( 11.28843830116857383, -3.202444869320336451, 32.30641848906366675 ) ) ;
#73357=CARTESIAN_POINT ( 'NONE',  ( -13.45069776397551564, -9.058645607665454236, 34.76329471203372634 ) ) ;
#73358=ORIENTED_EDGE ( 'NONE', *, *, #76449, .T. ) ;
#73359=ORIENTED_EDGE ( 'NONE', *, *, #61203, .T. ) ;
#73360=ADVANCED_FACE ( 'NONE', ( #78708 ), #38162, .F. ) ;
#73361=FACE_OUTER_BOUND ( 'NONE', #80269, .T. ) ;
#73363=DIRECTION ( 'NONE',  ( 0.000000000000000000, 0.1736481776669267785, -0.9848077530122087975 ) ) ;
#73364=CARTESIAN_POINT ( 'NONE',  ( 0.4615384615384611200, -2.486705287966279876, 31.30864560766543647 ) ) ;
#73365=LINE ( 'NONE', #52640, #53335 ) ;
#73367=CARTESIAN_POINT ( 'NONE',  ( 14.55763782604044998, -9.272278438253398036, 34.42582936511637115 ) ) ;
#73368=CARTESIAN_POINT ( 'NONE',  ( -4.219928533206288357, -9.058645607665454236, 34.76329471203372634 ) ) ;
#73369=DIRECTION ( 'NONE',  ( -0.000000000000000000, -0.9848077530122085754, -0.1736481776669273613 ) ) ;
#73370=DIRECTION ( 'NONE',  ( -0.000000000000000000, -0.000000000000000000, -1.000000000000000000 ) ) ;
#73371=LINE ( 'NONE', #18430, #70426 ) ;
#73372=CARTESIAN_POINT ( 'NONE',  ( -5.142193522883853340, -9.442884908240170461, 34.35708131394840592 ) ) ;
#73374=DIRECTION ( 'NONE',  ( 0.000000000000000000, 0.9848077530122072432, -0.1736481776669354937 ) ) ;
#73375=AXIS2_PLACEMENT_3D ( 'NONE', #28295, #55766, #19335 ) ;
#73377=VERTEX_POINT ( 'NONE', #30950 ) ;
#73378=B_SPLINE_CURVE_WITH_KNOTS ( 'NONE', 3,
 ( #56219, #78706, #1719, #71943, #30515, #64731, #85027, #10254, #62954, #85464 ),
 .UNSPECIFIED., .F., .F.,
 ( 4, 2, 2, 2, 4 ),
 ( 0.000000000000000000, 0.0001954311564186869015, 0.0003908623128373738030, 0.0005862934692560607588, 0.0007817246256747476061 ),
 .UNSPECIFIED. ) ;
#73379=ORIENTED_EDGE ( 'NONE', *, *, #17938, .T. ) ;
#73381=CARTESIAN_POINT ( 'NONE',  ( 4.853438152358743096, -10.97335522853832579, 33.68706563782419749 ) ) ;
#73382=CARTESIAN_POINT ( 'NONE',  ( 16.37662569511456567, -6.760870238392814535, 34.69528174975672385 ) ) ;
#73383=FACE_OUTER_BOUND ( 'NONE', #79334, .T. ) ;
#73384=CARTESIAN_POINT ( 'NONE',  ( -11.53846153846166089, -5.094484230521993062, 34.41647553114689373 ) ) ;
#73386=FACE_OUTER_BOUND ( 'NONE', #82219, .T. ) ;
#73389=CARTESIAN_POINT ( 'NONE',  ( 16.15384615384615330, -10.05456864172156806, 36.03766855953608683 ) ) ;
#73390=CARTESIAN_POINT ( 'NONE',  ( -5.011667937410237528, -2.379036618887895305, 30.90682066428159303 ) ) ;
#73392=CARTESIAN_POINT ( 'NONE',  ( 9.692307692307695177, -5.180354513474913603, 36.12317359536750416 ) ) ;
#73393=CYLINDRICAL_SURFACE ( 'NONE', #68834, 0.2500000000000009437 ) ;
#73396=CARTESIAN_POINT ( 'NONE',  ( -6.130147209438221445, -10.19110544564092002, 33.96427741523702792 ) ) ;
#73397=B_SPLINE_CURVE_WITH_KNOTS ( 'NONE', 3,
 ( #73159, #11455, #38939, #32174, #59636, #87136, #14903, #56757, #8141, #83811 ),
 .UNSPECIFIED., .F., .F.,
 ( 4, 2, 2, 2, 4 ),
 ( 0.000000000000000000, 0.0001954311564186880128, 0.0003908623128373760257, 0.0005862934692560640114, 0.0007817246256747520513 ),
 .UNSPECIFIED. ) ;
#73398=AXIS2_PLACEMENT_3D ( 'NONE', #31927, #3985, #85533 ) ;
#73399=ADVANCED_FACE ( 'NONE', ( #33186 ), #74622, .F. ) ;
#73400=CARTESIAN_POINT ( 'NONE',  ( -7.846153846153844924, -12.37446782046654192, 30.86335684631486131 ) ) ;
#73401=ORIENTED_EDGE ( 'NONE', *, *, #49815, .T. ) ;
#73402=CARTESIAN_POINT ( 'NONE',  ( 1.384615384615386802, -2.499999999999998668, 29.75000000000001421 ) ) ;
#73403=CARTESIAN_POINT ( 'NONE',  ( -3.296852641725110722, -3.513871655860377086, 32.76840700105978499 ) ) ;
#73406=B_SPLINE_CURVE_WITH_KNOTS ( 'NONE', 3,
 ( #27863, #55330, #40074, #12146, #82378, #13903, #47245, #54003, #21094, #62091 ),
 .UNSPECIFIED., .F., .F.,
 ( 4, 2, 2, 2, 4 ),
 ( 0.0007817246256747476061, 0.0009771112852218909357, 0.001172497944769034049, 0.001367884604316177161, 0.001563271263863320491 ),
 .UNSPECIFIED. ) ;
#73407=VECTOR ( 'NONE', #67078, 1000.000000000000000 ) ;
#73408=AXIS2_PLACEMENT_3D ( 'NONE', #23929, #73022, #18528 ) ;
#73409=EDGE_CURVE ( 'NONE', #64009, #10019, #57609, .T. ) ;
#73410=FACE_OUTER_BOUND ( 'NONE', #59515, .T. ) ;
#73411=CARTESIAN_POINT ( 'NONE',  ( -5.999999999999998224, -12.34228464037088635, 31.77849191805839268 ) ) ;
#73412=CARTESIAN_POINT ( 'NONE',  ( 9.692307692307572609, -6.879047030192662504, 34.71129190930017927 ) ) ;
#73413=EDGE_LOOP ( 'NONE', ( #12096, #27706 ) ) ;
#73415=LINE ( 'NONE', #40089, #5257 ) ;
#73417=ORIENTED_EDGE ( 'NONE', *, *, #84815, .F. ) ;
#73418=AXIS2_PLACEMENT_3D ( 'NONE', #58366, #73692, #3873 ) ;
#73419=CARTESIAN_POINT ( 'NONE',  ( -2.177166605928743337, -2.619367082507848998, 30.83698974864644171 ) ) ;
#73421=ORIENTED_EDGE ( 'NONE', *, *, #76448, .F. ) ;
#73422=DIRECTION ( 'NONE',  ( 0.000000000000000000, 0.6427876096865373645, -0.7660444431189797898 ) ) ;
#73423=CARTESIAN_POINT ( 'NONE',  ( -15.45425415533356350, -3.019605429927184836, 32.48692288466676814 ) ) ;
#73424=EDGE_CURVE ( 'NONE', #18827, #22236, #31782, .T. ) ;
#73425=CARTESIAN_POINT ( 'NONE',  ( 15.45378058238207863, -2.758310577978208666, 31.33698337089302299 ) ) ;
#73426=EDGE_LOOP ( 'NONE', ( #88357, #1119 ) ) ;
#73428=DIRECTION ( 'NONE',  ( -0.000000000000000000, 0.9848077530122086864, -0.1736481776669273891 ) ) ;
#73430=CARTESIAN_POINT ( 'NONE',  ( -5.776987155906605942, -2.308499170217967134, 30.53291367094873721 ) ) ;
#73432=CARTESIAN_POINT ( 'NONE',  ( 2.307692307692309264, -9.058645607665452459, 34.76329471203371924 ) ) ;
#73433=CARTESIAN_POINT ( 'NONE',  ( 12.52679403281448778, -12.27809138561124591, 31.22303859784720359 ) ) ;
#73434=EDGE_CURVE ( 'NONE', #70760, #35719, #37187, .T. ) ;
#73435=CARTESIAN_POINT ( 'NONE',  ( -10.39237326377176274, -6.503523203565941380, 34.64991518177335195 ) ) ;
#73436=ADVANCED_FACE ( 'NONE', ( #39958 ), #87263, .F. ) ;
#73437=DIRECTION ( 'NONE',  ( 0.000000000000000000, -6.938893903907222067E-15, 1.000000000000000000 ) ) ;
#73438=CYLINDRICAL_SURFACE ( 'NONE', #46461, 0.2499999999999986955 ) ;
#73439=CARTESIAN_POINT ( 'NONE',  ( -1.161602540521989635, -10.77377354290276301, 33.85451476688484718 ) ) ;
#73440=B_SPLINE_CURVE_WITH_KNOTS ( 'NONE', 3,
 ( #4057, #37857, #45044, #45938, #58119, #3174, #73430, #79295, #4519, #11729 ),
 .UNSPECIFIED., .F., .F.,
 ( 4, 2, 2, 2, 4 ),
 ( 0.0007817246256747516176, 0.0009771112852218965736, 0.001172497944769041421, 0.001367884604316186269, 0.001563271263863331333 ),
 .UNSPECIFIED. ) ;
#73441=B_SPLINE_CURVE_WITH_KNOTS ( 'NONE', 3,
 ( #36754, #84514, #30003, #2957, #56588, #37639, #49390, #57909, #70989, #35880 ),
 .UNSPECIFIED., .F., .F.,
 ( 4, 2, 2, 2, 4 ),
 ( 0.000000000000000000, 0.0001954311564186876063, 0.0003908623128373752125, 0.0005862934692560628188, 0.0007817246256747504250 ),
 .UNSPECIFIED. ) ;
#73442=CARTESIAN_POINT ( 'NONE',  ( 13.45068271796546178, -11.91647553114624358, 32.58852847137148245 ) ) ;
#73443=B_SPLINE_CURVE_WITH_KNOTS ( 'NONE', 3,
 ( #23302, #78245, #50760, #38603, #44014, #51191, #26865, #19659, #5703, #89030 ),
 .UNSPECIFIED., .F., .F.,
 ( 4, 2, 2, 2, 4 ),
 ( 0.000000000000000000, 0.0001954311564186865763, 0.0003908623128373731525, 0.0005862934692560596746, 0.0007817246256747463051 ),
 .UNSPECIFIED. ) ;
#73444=EDGE_LOOP ( 'NONE', ( #57398, #3866, #41424, #80459 ) ) ;
#73445=ORIENTED_EDGE ( 'NONE', *, *, #51024, .F. ) ;
#73446=EDGE_LOOP ( 'NONE', ( #1132, #30987, #37186, #33793, #23532, #31719 ) ) ;
#73447=CARTESIAN_POINT ( 'NONE',  ( 15.29683758177167086, -2.538708090699994813, 30.37095296980875503 ) ) ;
#73449=VECTOR ( 'NONE', #41059, 1000.000000000000000 ) ;
#73450=CARTESIAN_POINT ( 'NONE',  ( 10.39189967166066708, -5.113361153441934093, 34.14387501736622710 ) ) ;
#73451=CARTESIAN_POINT ( 'NONE',  ( 1.384615384615386802, -2.721908614388771852, 31.22303859784724978 ) ) ;
#73453=CARTESIAN_POINT ( 'NONE',  ( 15.48071464014727283, -9.357781135181031829, 34.66075350412533851 ) ) ;
#73454=ORIENTED_EDGE ( 'NONE', *, *, #75265, .F. ) ;
#73455=CARTESIAN_POINT ( 'NONE',  ( 17.29993592101647337, -9.172514111537580561, 34.72667873470787470 ) ) ;
#73456=ORIENTED_EDGE ( 'NONE', *, *, #6683, .T. ) ;
#73458=EDGE_CURVE ( 'NONE', #75360, #30124, #11359, .T. ) ;
#73460=CARTESIAN_POINT ( 'NONE',  ( 4.153846153846154188, -11.91647553114624181, 32.58852847137148245 ) ) ;
#73461=ADVANCED_FACE ( 'NONE', ( #32303 ), #12040, .F. ) ;
#73462=CARTESIAN_POINT ( 'NONE',  ( 3.903846153846154632, -2.249999999999998668, 29.75000000000000355 ) ) ;
#73463=FACE_BOUND ( 'NONE', #44219, .T. ) ;
#73464=CARTESIAN_POINT ( 'NONE',  ( 17.29993592101647337, -6.460100341425561332, 34.89618726649961644 ) ) ;
#73465=CARTESIAN_POINT ( 'NONE',  ( 1.450781991207027222, -7.250054591869667497, 34.99404684341514127 ) ) ;
#73466=B_SPLINE_CURVE_WITH_KNOTS ( 'NONE', 3,
 ( #85214, #3226, #64468, #71682, #30699, #30267, #23933, #57734, #44643, #18088 ),
 .UNSPECIFIED., .F., .F.,
 ( 4, 2, 2, 2, 4 ),
 ( 0.000000000000000000, 0.0001954311564186865763, 0.0003908623128373731525, 0.0005862934692560596746, 0.0007817246256747463051 ),
 .UNSPECIFIED. ) ;
#73469=EDGE_CURVE ( 'NONE', #18264, #61398, #88604, .T. ) ;
#73470=CARTESIAN_POINT ( 'NONE',  ( -1.449885385171703289, -2.379036618887870880, 30.90682066428147579 ) ) ;
#73471=CARTESIAN_POINT ( 'NONE',  ( -10.61538461538461320, -13.53365097954675988, 30.81389545987213552 ) ) ;
#73472=CARTESIAN_POINT ( 'NONE',  ( 10.36538461538461497, -7.566083408709835645, 34.74999999999999289 ) ) ;
#73473=CARTESIAN_POINT ( 'NONE',  ( 17.29993442853592711, -9.086983370893049639, 34.49168942202179267 ) ) ;
#73474=EDGE_LOOP ( 'NONE', ( #79649, #44104 ) ) ;
#73476=ORIENTED_EDGE ( 'NONE', *, *, #73987, .T. ) ;
#73477=EDGE_LOOP ( 'NONE', ( #25987, #61904 ) ) ;
#73479=CARTESIAN_POINT ( 'NONE',  ( -16.15384615384615330, -2.833524468853757305, 32.15551576947925838 ) ) ;
#73480=DIRECTION ( 'NONE',  ( -0.000000000000000000, -0.5000000000000009992, -0.8660254037844380415 ) ) ;
#73481=CYLINDRICAL_SURFACE ( 'NONE', #14031, 0.2499999999999986955 ) ;
#73482=CARTESIAN_POINT ( 'NONE',  ( -14.53117723225663482, -12.11044203135681840, 32.26167407432752299 ) ) ;
#73483=CYLINDRICAL_SURFACE ( 'NONE', #80307, 0.2499999999999995559 ) ;
#73484=CARTESIAN_POINT ( 'NONE',  ( -15.45425417449318140, -3.754499324213721234, 33.06261337010820256 ) ) ;
#73485=ORIENTED_EDGE ( 'NONE', *, *, #53172, .F. ) ;
#73486=FACE_OUTER_BOUND ( 'NONE', #42970, .T. ) ;
#73487=CARTESIAN_POINT ( 'NONE',  ( 0.4615384615384611200, -9.780366693483667717, 34.19971097300155094 ) ) ;
#73488=CARTESIAN_POINT ( 'NONE',  ( 10.39245839786846659, -3.105860786376062332, 32.13614157043599562 ) ) ;
#73489=CARTESIAN_POINT ( 'NONE',  ( 5.326923076924511946, -7.500000000000155431, 34.75000000000007105 ) ) ;
#73490=VERTEX_POINT ( 'NONE', #89040 ) ;
#73491=VERTEX_POINT ( 'NONE', #57332 ) ;
#73493=EDGE_LOOP ( 'NONE', ( #68490, #50789, #65318, #44955 ) ) ;
#73494=DIRECTION ( 'NONE',  ( 0.000000000000000000, 0.8660254037844377084, -0.5000000000000015543 ) ) ;
#73495=CARTESIAN_POINT ( 'NONE',  ( -7.715362038329061534, -4.809403383903224416, 33.96459661697924304 ) ) ;
#73497=CARTESIAN_POINT ( 'NONE',  ( 2.980769230769232170, -7.500000000000001776, 35.00000000000000000 ) ) ;
#73498=CARTESIAN_POINT ( 'NONE',  ( -5.207070286361293654, -2.882441371585227063, 31.66841991370171527 ) ) ;
#73499=CARTESIAN_POINT ( 'NONE',  ( 0.4615384615383396616, -12.27809138561165270, 31.22303859784587132 ) ) ;
#73500=EDGE_CURVE ( 'NONE', #5405, #54514, #62413, .T. ) ;
#73501=CARTESIAN_POINT ( 'NONE',  ( 14.55769230769237410, -7.434744429011176159, 34.75000000000000711 ) ) ;
#73502=DIRECTION ( 'NONE',  ( 0.000000000000000000, 0.3420201433256610524, 0.9396926207859113145 ) ) ;
#73503=ORIENTED_EDGE ( 'NONE', *, *, #84734, .F. ) ;
#73504=CARTESIAN_POINT ( 'NONE',  ( -15.45425415533355995, -12.11044203135681840, 32.26167407432752299 ) ) ;
#73505=ORIENTED_EDGE ( 'NONE', *, *, #6964, .T. ) ;
#73506=CARTESIAN_POINT ( 'NONE',  ( 15.23076923076923173, -6.681629849574314051, 35.83090037661290239 ) ) ;
#73507=CARTESIAN_POINT ( 'NONE',  ( 8.992243613324164997, -12.38742843783360748, 31.66772728687926985 ) ) ;
#73508=DIRECTION ( 'NONE',  ( -0.000000000000000000, -0.000000000000000000, -1.000000000000000000 ) ) ;
#73509=AXIS2_PLACEMENT_3D ( 'NONE', #38633, #11612, #24670 ) ;
#73510=CARTESIAN_POINT ( 'NONE',  ( 15.23076923076911093, -12.46129190930018460, 30.37095296980731973 ) ) ;
#73511=LINE ( 'NONE', #74390, #47672 ) ;
#73512=LINE ( 'NONE', #37600, #1793 ) ;
#73513=VECTOR ( 'NONE', #49211, 1000.000000000000227 ) ;
#73516=CARTESIAN_POINT ( 'NONE',  ( 14.05766908347085042, -2.341070481393819236, 30.72580821765574299 ) ) ;
#73517=CARTESIAN_POINT ( 'NONE',  ( -14.24243716817947281, -3.643525952247864463, 33.31231777344670064 ) ) ;
#73518=CARTESIAN_POINT ( 'NONE',  ( -0.3962828902624375149, -5.219633306516380244, 34.19971097300157936 ) ) ;
#73519=ORIENTED_EDGE ( 'NONE', *, *, #5551, .T. ) ;
#73520=ORIENTED_EDGE ( 'NONE', *, *, #40276, .F. ) ;
#73522=CARTESIAN_POINT ( 'NONE',  ( 3.230769230769538147, -2.506253911140615021, 30.00000000000323297 ) ) ;
#73523=CARTESIAN_POINT ( 'NONE',  ( -0.4615384615381544209, -2.506253911140615021, 30.00000000000323297 ) ) ;
#73525=CARTESIAN_POINT ( 'NONE',  ( 6.923076923076802558, -6.026961402154118908, 34.52809138561165270 ) ) ;
#73526=CARTESIAN_POINT ( 'NONE',  ( 14.30769230769231015, -13.20930481340135110, 34.54067556320372745 ) ) ;
#73527=EDGE_LOOP ( 'NONE', ( #3571, #8294 ) ) ;
#73528=CARTESIAN_POINT ( 'NONE',  ( -16.40382289789473802, -6.524016743844656574, 34.90889640711025521 ) ) ;
#73529=EDGE_CURVE ( 'NONE', #53273, #24676, #28588, .T. ) ;
#73532=CARTESIAN_POINT ( 'NONE',  ( 4.377272552760941515, -7.630147987733840509, 34.99859428049665411 ) ) ;
#73533=CARTESIAN_POINT ( 'NONE',  ( 4.023698184114458343, -8.630895178749536711, 34.87696386517710323 ) ) ;
#73535=CARTESIAN_POINT ( 'NONE',  ( 12.68431800280687227, -3.755027918224367767, 33.06320215134714857 ) ) ;
#73536=B_SPLINE_CURVE_WITH_KNOTS ( 'NONE', 3,
 ( #59434, #86486, #16664, #18013, #44124, #9911, #35455, #83661, #2104, #35904 ),
 .UNSPECIFIED., .F., .F.,
 ( 4, 2, 2, 2, 4 ),
 ( 0.000000000000000000, 0.0001954339857564074473, 0.0003908679715128148945, 0.0005863019572692223418, 0.0007817359430256297891 ),
 .UNSPECIFIED. ) ;
#73538=B_SPLINE_CURVE_WITH_KNOTS ( 'NONE', 3,
 ( #36279, #63733, #65056, #2035, #16441, #30836, #56975, #71372, #84469, #85350 ),
 .UNSPECIFIED., .F., .F.,
 ( 4, 2, 2, 2, 4 ),
 ( 0.000000000000000000, 0.0001954311584214072381, 0.0003908623168428144762, 0.0005862934752642217414, 0.0007817246336856289524 ),
 .UNSPECIFIED. ) ;
#73539=VECTOR ( 'NONE', #53631, 1000.000000000000227 ) ;
#73540=AXIS2_PLACEMENT_3D ( 'NONE', #30268, #57735, #16741 ) ;
#73541=EDGE_LOOP ( 'NONE', ( #88352, #49071 ) ) ;
#73544=CARTESIAN_POINT ( 'NONE',  ( -8.769230769230768274, -8.164416787775445883, 34.95778746994557906 ) ) ;
#73545=ORIENTED_EDGE ( 'NONE', *, *, #40173, .T. ) ;
#73546=EDGE_CURVE ( 'NONE', #62563, #28571, #34951, .T. ) ;
#73547=CARTESIAN_POINT ( 'NONE',  ( -13.25408994638174320, -5.070358843744210198, 34.40418822224088302 ) ) ;
#73548=FACE_OUTER_BOUND ( 'NONE', #9567, .T. ) ;
#73549=DIRECTION ( 'NONE',  ( -0.000000000000000000, 0.6427876096865404731, -0.7660444431189771253 ) ) ;
#73550=VECTOR ( 'NONE', #28283, 1000.000000000000227 ) ;
#73552=CARTESIAN_POINT ( 'NONE',  ( 11.53846153846153832, -2.517432740324522911, 35.29906147534542527 ) ) ;
#73553=CARTESIAN_POINT ( 'NONE',  ( -3.099977422944443450, -12.38066358083363738, 30.83685684665853444 ) ) ;
#73554=EDGE_LOOP ( 'NONE', ( #12654, #59170, #60866, #79952 ) ) ;
#73555=CARTESIAN_POINT ( 'NONE',  ( -4.087778820496075660, -12.34228464037088813, 31.77849191805839268 ) ) ;
#73556=EDGE_LOOP ( 'NONE', ( #72974, #3836 ) ) ;
#73557=CARTESIAN_POINT ( 'NONE',  ( 8.703147358274888390, -12.37446782046654192, 30.86335684631486487 ) ) ;
#73558=EDGE_CURVE ( 'NONE', #89000, #83351, #23151, .T. ) ;
#73559=CARTESIAN_POINT ( 'NONE',  ( 3.230769230769231726, -3.669653830205710676, 35.88435417666054406 ) ) ;
#73560=CARTESIAN_POINT ( 'NONE',  ( -13.63463862190835130, -2.823816976329319051, 31.52131813110795733 ) ) ;
#73562=ADVANCED_FACE ( 'NONE', ( #48914 ), #34516, .F. ) ;
#73563=CARTESIAN_POINT ( 'NONE',  ( -6.792551221313361864, -6.001044277235011215, 34.52024696741798948 ) ) ;
#73564=CARTESIAN_POINT ( 'NONE',  ( -13.38461538461538325, -2.499999999999998668, 29.75000000000001421 ) ) ;
#73565=CARTESIAN_POINT ( 'NONE',  ( 16.15384615384603251, -12.16647553114689728, 32.15551576947799362 ) ) ;
#73567=ORIENTED_EDGE ( 'NONE', *, *, #49974, .T. ) ;
#73569=VECTOR ( 'NONE', #9073, 1000.000000000000227 ) ;
#73571=B_SPLINE_CURVE_WITH_KNOTS ( 'NONE', 3,
 ( #81002, #54395, #21046, #41786, #27378, #55283, #40464, #89100, #48517, #67923 ),
 .UNSPECIFIED., .F., .F.,
 ( 4, 2, 2, 2, 4 ),
 ( 0.0007817359430256353185, 0.0009771253907250028285, 0.001172514838424370230, 0.001367904286123737632, 0.001563293733823105033 ),
 .UNSPECIFIED. ) ;
#73572=EDGE_CURVE ( 'NONE', #79986, #6875, #27754, .T. ) ;
#73573=VERTEX_POINT ( 'NONE', #20556 ) ;
#73575=CARTESIAN_POINT ( 'NONE',  ( 11.40831356872984514, -9.504002272028875709, 34.60269587691767867 ) ) ;
#73576=CARTESIAN_POINT ( 'NONE',  ( -13.38461538461538325, -2.249999999999998668, 29.75000000000001776 ) ) ;
#73577=EDGE_CURVE ( 'NONE', #83084, #63180, #48019, .T. ) ;
#73578=CARTESIAN_POINT ( 'NONE',  ( -5.934744428723973897, -5.219633306516380244, 34.19971097300157936 ) ) ;
#73579=CARTESIAN_POINT ( 'NONE',  ( 5.010840697562939816, -11.35647404775217595, 33.31231777344666511 ) ) ;
#73580=CARTESIAN_POINT ( 'NONE',  ( 8.546304551714618114, -9.086856451489515152, 34.49173150075333183 ) ) ;
#73581=CARTESIAN_POINT ( 'NONE',  ( 11.53846153846141753, -12.46129190930018460, 30.37095296980731973 ) ) ;
#73582=LINE ( 'NONE', #88431, #16409 ) ;
#73583=CARTESIAN_POINT ( 'NONE',  ( -4.153846153846152411, -9.780366693483667717, 34.19971097300155094 ) ) ;
#73584=VERTEX_POINT ( 'NONE', #68743 ) ;
#73585=ORIENTED_EDGE ( 'NONE', *, *, #88145, .T. ) ;
#73586=ORIENTED_EDGE ( 'NONE', *, *, #23145, .T. ) ;
#73587=CARTESIAN_POINT ( 'NONE',  ( -1.514762594053601585, -11.47017969459903952, 32.78971311882034456 ) ) ;
#73588=EDGE_CURVE ( 'NONE', #62974, #46529, #60804, .T. ) ;
#73589=EDGE_LOOP ( 'NONE', ( #61181, #73401, #27011, #76792 ) ) ;
#73590=CARTESIAN_POINT ( 'NONE',  ( 16.37685750545900376, -11.76359900205217457, 32.36225158514719880 ) ) ;
#73591=CARTESIAN_POINT ( 'NONE',  ( 9.692307692307695177, -3.886160181151819604, 36.00935417666054406 ) ) ;
#73592=CYLINDRICAL_SURFACE ( 'NONE', #15458, 0.2500000000000008882 ) ;
#73593=CARTESIAN_POINT ( 'NONE',  ( 4.376857505459002873, -2.554770724473668153, 30.48948780036025852 ) ) ;
#73594=FACE_BOUND ( 'NONE', #25966, .T. ) ;
#73595=EDGE_LOOP ( 'NONE', ( #5440, #52240 ) ) ;
#73596=EDGE_CURVE ( 'NONE', #75481, #44313, #82357, .T. ) ;
#73597=ORIENTED_EDGE ( 'NONE', *, *, #24046, .F. ) ;
#73598=CARTESIAN_POINT ( 'NONE',  ( 4.826946332874483936, -2.318417181685854978, 30.59732222474233865 ) ) ;
#73599=ORIENTED_EDGE ( 'NONE', *, *, #24456, .T. ) ;
#73600=FACE_BOUND ( 'NONE', #4968, .T. ) ;
#73601=CARTESIAN_POINT ( 'NONE',  ( 9.757562831820530747, -5.941354392334607049, 34.76329471203374055 ) ) ;
#73603=DIRECTION ( 'NONE',  ( -0.000000000000000000, 0.5000000000000011102, -0.8660254037844380415 ) ) ;
#73604=EDGE_LOOP ( 'NONE', ( #61119, #25335, #42979, #35202 ) ) ;
#73605=DIRECTION ( 'NONE',  ( 0.000000000000000000, 0.1736481776669267785, -0.9848077530122087975 ) ) ;
#73606=CARTESIAN_POINT ( 'NONE',  ( -6.673131513698878692, -2.341251567377310217, 30.72681386836322659 ) ) ;
#73608=ORIENTED_EDGE ( 'NONE', *, *, #20773, .T. ) ;
#73609=CARTESIAN_POINT ( 'NONE',  ( 14.30769230769231015, -11.35647404775217417, 33.31231777344666511 ) ) ;
#73610=CARTESIAN_POINT ( 'NONE',  ( -18.25002323729296450, -5.056417327199098644, 34.11270091957320716 ) ) ;
#73612=DIRECTION ( 'NONE',  ( -0.000000000000000000, 0.1736481776669307198, -0.9848077530122080203 ) ) ;
#73613=EDGE_LOOP ( 'NONE', ( #34180, #51027, #41875, #11617 ) ) ;
#73614=AXIS2_PLACEMENT_3D ( 'NONE', #2592, #85915, #57542 ) ;
#73615=EDGE_CURVE ( 'NONE', #7659, #35101, #30805, .T. ) ;
#73616=CARTESIAN_POINT ( 'NONE',  ( 2.557746727605761272, -12.41089969410671223, 31.60739465890703670 ) ) ;
#73617=CYLINDRICAL_SURFACE ( 'NONE', #80140, 0.2499999999999973355 ) ;
#73618=B_SPLINE_CURVE_WITH_KNOTS ( 'NONE', 3,
 ( #3409, #24572, #87192, #78627, #60132, #52487, #58348, #65996, #24122, #66901 ),
 .UNSPECIFIED., .F., .F.,
 ( 4, 2, 2, 2, 4 ),
 ( 0.000000000000000000, 0.0001954311564186872810, 0.0003908623128373745620, 0.0005862934692560618430, 0.0007817246256747491240 ),
 .UNSPECIFIED. ) ;
#73619=ORIENTED_EDGE ( 'NONE', *, *, #73154, .T. ) ;
#73620=CARTESIAN_POINT ( 'NONE',  ( 0.2115617305961065842, -9.148715823498378086, 34.47080413974185120 ) ) ;
#73621=FACE_OUTER_BOUND ( 'NONE', #81971, .T. ) ;
#73622=LINE ( 'NONE', #20435, #822 ) ;
#73623=CARTESIAN_POINT ( 'NONE',  ( -8.703975197954745724, -9.442884908240273489, 34.35708131394835618 ) ) ;
#73624=B_SPLINE_CURVE_WITH_KNOTS ( 'NONE', 3,
 ( #3421, #31347, #79088, #45292, #30889, #51586, #44845, #72325, #10634, #38100 ),
 .UNSPECIFIED., .F., .F.,
 ( 4, 2, 2, 2, 4 ),
 ( 0.0007817359430256322827, 0.0009771253907249989254, 0.001172514838424365676, 0.001367904286123732428, 0.001563293733823098962 ),
 .UNSPECIFIED. ) ;
#73625=CARTESIAN_POINT ( 'NONE',  ( 0.3313904918067608896, -2.647304123082327543, 31.75400227202884906 ) ) ;
#73626=CARTESIAN_POINT ( 'NONE',  ( 6.856993512121044354, -8.973038597847269315, 34.52809138561120506 ) ) ;
#73629=CARTESIAN_POINT ( 'NONE',  ( -3.454254174493178287, -2.599994579823203367, 30.74605699353653776 ) ) ;
#73630=CARTESIAN_POINT ( 'NONE',  ( -18.00000000000000000, -13.72934399251292170, 33.34651343095209342 ) ) ;
#73632=ORIENTED_EDGE ( 'NONE', *, *, #89105, .T. ) ;
#73633=CYLINDRICAL_SURFACE ( 'NONE', #50527, 0.2500000000000012212 ) ;
#73634=ORIENTED_EDGE ( 'NONE', *, *, #76110, .F. ) ;
#73635=ORIENTED_EDGE ( 'NONE', *, *, #34363, .T. ) ;
#73636=FACE_OUTER_BOUND ( 'NONE', #76245, .T. ) ;
#73637=VERTEX_POINT ( 'NONE', #58653 ) ;
#73638=CARTESIAN_POINT ( 'NONE',  ( -5.999999999999998224, -9.905515769479276145, 34.41647553114623292 ) ) ;
#73640=CARTESIAN_POINT ( 'NONE',  ( 3.165499230212911908, -2.379036618887870880, 30.90682066428147934 ) ) ;
#73641=CARTESIAN_POINT ( 'NONE',  ( 12.46153846153846168, -9.584722331328613620, 36.20867863119891439 ) ) ;
#73642=CARTESIAN_POINT ( 'NONE',  ( -3.007757879156379932, -9.086983370893047862, 34.49168942202179267 ) ) ;
#73643=CARTESIAN_POINT ( 'NONE',  ( -7.846153846153844924, -8.564572088678739092, 35.78748833219616898 ) ) ;
#73644=CARTESIAN_POINT ( 'NONE',  ( -5.143005456283213483, -3.322132147404559976, 32.92929555188719348 ) ) ;
#73645=CARTESIAN_POINT ( 'NONE',  ( -7.846153846153965716, -2.892918686052166066, 31.69288490824153470 ) ) ;
#73646=CARTESIAN_POINT ( 'NONE',  ( 1.384615384615386802, -7.500000000000001776, 35.04278698407183867 ) ) ;
#73647=VECTOR ( 'NONE', #32580, 1000.000000000000227 ) ;
#73649=CARTESIAN_POINT ( 'NONE',  ( 10.86533002476265786, -12.45601412856602686, 31.48342859153981621 ) ) ;
#73650=CARTESIAN_POINT ( 'NONE',  ( -4.377331078410482412, -12.11044203135681840, 32.26167407432752299 ) ) ;
#73651=CARTESIAN_POINT ( 'NONE',  ( 18.25000000000000000, -2.499999999999998668, 29.75000000000000355 ) ) ;
#73652=ORIENTED_EDGE ( 'NONE', *, *, #27191, .F. ) ;
#73653=ORIENTED_EDGE ( 'NONE', *, *, #71323, .F. ) ;
#73654=CARTESIAN_POINT ( 'NONE',  ( 3.164686851409094448, -10.67929555188718460, 33.92786785259543336 ) ) ;
#73655=CARTESIAN_POINT ( 'NONE',  ( 7.596177115211491859, -11.28823185664190376, 33.01397839955799896 ) ) ;
#73656=CARTESIAN_POINT ( 'NONE',  ( -2.307692307692428724, -2.379036618888197285, 30.90682066428292885 ) ) ;
#73657=CARTESIAN_POINT ( 'NONE',  ( -7.053224892808619195, -5.915902021225892149, 34.75552854090298638 ) ) ;
#73658=EDGE_CURVE ( 'NONE', #7689, #25692, #72606, .T. ) ;
#73660=CARTESIAN_POINT ( 'NONE',  ( -4.854143407945009869, -3.020022701398814569, 32.48759521482552515 ) ) ;
#73661=EDGE_CURVE ( 'NONE', #63695, #6887, #68306, .T. ) ;
#73662=ORIENTED_EDGE ( 'NONE', *, *, #4189, .T. ) ;
#73663=CARTESIAN_POINT ( 'NONE',  ( -4.826868765284763718, -12.41262288849542017, 30.68299917996395010 ) ) ;
#73666=ORIENTED_EDGE ( 'NONE', *, *, #63943, .T. ) ;
#73667=VECTOR ( 'NONE', #50420, 1000.000000000000114 ) ;
#73668=CARTESIAN_POINT ( 'NONE',  ( -14.24152316672964957, -7.250054483168843156, 34.74374881642865631 ) ) ;
#73669=VECTOR ( 'NONE', #13504, 1000.000000000000000 ) ;
#73671=CARTESIAN_POINT ( 'NONE',  ( -9.626239341305252495, -6.386643153685127139, 34.62446782046654192 ) ) ;
#73672=LINE ( 'NONE', #11965, #22050 ) ;
#73673=CARTESIAN_POINT ( 'NONE',  ( -13.13456107297707121, -3.136992222400443175, 32.19305428654138979 ) ) ;
#73674=ORIENTED_EDGE ( 'NONE', *, *, #51944, .T. ) ;
#73676=ORIENTED_EDGE ( 'NONE', *, *, #60482, .T. ) ;
#73677=ORIENTED_EDGE ( 'NONE', *, *, #36764, .F. ) ;
#73678=DIRECTION ( 'NONE',  ( -0.000000000000000000, 0.7660444431189791237, -0.6427876096865379196 ) ) ;
#73681=DIRECTION ( 'NONE',  ( -0.000000000000000000, 0.6427876096865404731, -0.7660444431189770143 ) ) ;
#73682=CARTESIAN_POINT ( 'NONE',  ( 10.61538461538449418, -5.094484230521993062, 34.41647553114689373 ) ) ;
#73684=ADVANCED_FACE ( 'NONE', ( #25770 ), #19014, .F. ) ;
#73685=CARTESIAN_POINT ( 'NONE',  ( -11.53846153846153655, -9.819645486525091727, 36.12317359536749706 ) ) ;
#73686=ORIENTED_EDGE ( 'NONE', *, *, #40180, .T. ) ;
#73687=ORIENTED_EDGE ( 'NONE', *, *, #28566, .F. ) ;
#73689=CYLINDRICAL_SURFACE ( 'NONE', #57380, 0.2499999999999994726 ) ;
#73690=ORIENTED_EDGE ( 'NONE', *, *, #32326, .F. ) ;
#73691=CARTESIAN_POINT ( 'NONE',  ( -9.692307692307814193, -10.33852847137269571, 34.16647553114546554 ) ) ;
#73692=DIRECTION ( 'NONE',  ( -0.000000000000000000, 0.7660444431189791237, -0.6427876096865379196 ) ) ;
#73693=AXIS2_PLACEMENT_3D ( 'NONE', #9554, #2344, #37018 ) ;
#73696=EDGE_CURVE ( 'NONE', #64679, #54531, #34002, .T. ) ;
#73698=CARTESIAN_POINT ( 'NONE',  ( 3.230769230769546141, -2.255955759149395501, 30.00000000000324363 ) ) ;
#73699=ORIENTED_EDGE ( 'NONE', *, *, #13912, .F. ) ;
#73700=CARTESIAN_POINT ( 'NONE',  ( -13.44988538517170440, -11.67786785259540849, 32.92929555188721480 ) ) ;
#73701=DIRECTION ( 'NONE',  ( -0.000000000000000000, -0.9396926207859093161, -0.3420201433256663259 ) ) ;
#73702=CARTESIAN_POINT ( 'NONE',  ( -12.23875892027004930, -12.44528174975671853, 30.48912976160716681 ) ) ;
#73703=B_SPLINE_CURVE_WITH_KNOTS ( 'NONE', 3,
 ( #57302, #49222, #1918, #14998, #63615, #70384, #9555, #36595, #64049, #37019 ),
 .UNSPECIFIED., .F., .F.,
 ( 4, 2, 2, 2, 4 ),
 ( 0.000000000000000000, 0.0001954339857564097241, 0.0003908679715128194482, 0.0005863019572692291723, 0.0007817359430256388964 ),
 .UNSPECIFIED. ) ;
#73704=CARTESIAN_POINT ( 'NONE',  ( -5.076923076923197442, -12.27809138561165270, 31.22303859784587132 ) ) ;
#73706=LINE ( 'NONE', #53407, #14626 ) ;
#73707=ORIENTED_EDGE ( 'NONE', *, *, #27473, .T. ) ;
#73708=CARTESIAN_POINT ( 'NONE',  ( 6.700150705560775855, -8.239355502252617924, 34.69524867566427417 ) ) ;
#73709=CARTESIAN_POINT ( 'NONE',  ( -9.019253993452228002, -4.175268141568685643, 33.81360843649122216 ) ) ;
#73710=DIRECTION ( 'NONE',  ( 0.000000000000000000, 0.7660444431189807890, 0.6427876096865361433 ) ) ;
#73711=ADVANCED_FACE ( 'NONE', ( #39741 ), #5054, .F. ) ;
#73713=CARTESIAN_POINT ( 'NONE',  ( 4.153846153846154188, -2.517432740324522911, 35.29906147534542527 ) ) ;
#73715=CARTESIAN_POINT ( 'NONE',  ( -16.28453675695647007, -11.93127051446800380, 32.56575433478200665 ) ) ;
#73716=EDGE_CURVE ( 'NONE', #42352, #66607, #79156, .T. ) ;
#73717=CARTESIAN_POINT ( 'NONE',  ( 10.39189967166066708, -11.89387501736622710, 32.13663884655806413 ) ) ;
#73719=FACE_BOUND ( 'NONE', #69199, .T. ) ;
#73720=CARTESIAN_POINT ( 'NONE',  ( 13.38461538461538680, -13.88283147151868846, 33.14645433367849847 ) ) ;
#73721=FACE_OUTER_BOUND ( 'NONE', #5772, .T. ) ;
#73722=CARTESIAN_POINT ( 'NONE',  ( -15.23076923076922995, -4.661471528628507777, 34.16647553114623292 ) ) ;
#73723=CARTESIAN_POINT ( 'NONE',  ( 1.254467414883689402, -12.70455904226513866, 30.44083106164009322 ) ) ;
#73724=CARTESIAN_POINT ( 'NONE',  ( -9.692307692307812417, -10.90142922262034020, 33.41473453929536674 ) ) ;
#73725=CARTESIAN_POINT ( 'NONE',  ( 1.449870524128224369, -3.083524468853784839, 32.58852847137153930 ) ) ;
#73726=CARTESIAN_POINT ( 'NONE',  ( 8.769230769230645706, -12.70778746994576025, 30.41441678777401236 ) ) ;
#73728=EDGE_CURVE ( 'NONE', #41702, #58570, #58723, .T. ) ;
#73729=ORIENTED_EDGE ( 'NONE', *, *, #15039, .T. ) ;
#73731=CARTESIAN_POINT ( 'NONE',  ( -12.21153846153840128, -7.434744860731433924, 35.00000000000000711 ) ) ;
#73732=ORIENTED_EDGE ( 'NONE', *, *, #42226, .T. ) ;
#73733=AXIS2_PLACEMENT_3D ( 'NONE', #22152, #35672, #16277 ) ;
#73734=CYLINDRICAL_SURFACE ( 'NONE', #65041, 0.2500000000000009437 ) ;
#73735=CARTESIAN_POINT ( 'NONE',  ( -4.088590582570128973, -12.27809138561124591, 31.22303859784720359 ) ) ;
#73736=LINE ( 'NONE', #87696, #50241 ) ;
#73738=DIRECTION ( 'NONE',  ( -0.000000000000000000, -0.8660254037844397068, -0.4999999999999978906 ) ) ;
#73739=CARTESIAN_POINT ( 'NONE',  ( 5.999999999999878320, -3.643525952248796163, 33.31231777344771672 ) ) ;
#73742=CARTESIAN_POINT ( 'NONE',  ( 14.98079248672064345, -12.01397095200674059, 32.43157075238190146 ) ) ;
#73743=CARTESIAN_POINT ( 'NONE',  ( -14.37377468705243899, -11.35647404775217595, 33.31231777344666511 ) ) ;
#73745=CARTESIAN_POINT ( 'NONE',  ( 9.692307692307570832, -4.320704448113951379, 33.92786785259630022 ) ) ;
#73746=CARTESIAN_POINT ( 'NONE',  ( 8.519207531937803779, -10.05641848906368097, 34.04755513067966177 ) ) ;
#73747=CARTESIAN_POINT ( 'NONE',  ( -11.47320596718551400, -10.21337939537593620, 33.94971097300152252 ) ) ;
#73749=B_SPLINE_CURVE_WITH_KNOTS ( 'NONE', 3,
 ( #9849, #3080, #44503, #31907, #25587, #52154, #3965, #72875, #80086, #44059 ),
 .UNSPECIFIED., .F., .F.,
 ( 4, 2, 2, 2, 4 ),
 ( 0.0007817359430256372700, 0.0009771253907250054306, 0.001172514838424373700, 0.001367904286123741969, 0.001563293733823110021 ),
 .UNSPECIFIED. ) ;
#73750=CARTESIAN_POINT ( 'NONE',  ( 2.980769230769232170, -7.500000000000001776, 35.00000000000000000 ) ) ;
#73752=B_SPLINE_CURVE_WITH_KNOTS ( 'NONE', 3,
 ( #52683, #67992, #45926, #19798, #81070, #46822, #47260, #13041, #88286, #39643 ),
 .UNSPECIFIED., .F., .F.,
 ( 4, 2, 2, 2, 4 ),
 ( 0.0007817246256747494492, 0.0009771112852218935378, 0.001172497944769037518, 0.001367884604316181498, 0.001563271263863325695 ),
 .UNSPECIFIED. ) ;
#73753=EDGE_LOOP ( 'NONE', ( #70464, #39571 ) ) ;
#73754=CARTESIAN_POINT ( 'NONE',  ( -10.61538461538461320, -13.87047571288749737, 32.06866353760679544 ) ) ;
#73755=CARTESIAN_POINT ( 'NONE',  ( 13.38461538461526601, -3.835265460704628371, 33.15142922262033665 ) ) ;
#73757=CARTESIAN_POINT ( 'NONE',  ( -15.10072417484945717, -2.254550872974306674, 29.97347326024527092 ) ) ;
#73758=CARTESIAN_POINT ( 'NONE',  ( -9.019253993452226226, -3.520140089381495585, 33.17453946501458262 ) ) ;
#73759=VERTEX_POINT ( 'NONE', #32518 ) ;
#73761=CARTESIAN_POINT ( 'NONE',  ( -12.23875879256039489, -12.69155399931963046, 30.53255429739157734 ) ) ;
#73762=CARTESIAN_POINT ( 'NONE',  ( -7.623141002060451754, -12.38742843783360748, 31.66772728687926985 ) ) ;
#73763=ORIENTED_EDGE ( 'NONE', *, *, #5798, .F. ) ;
#73764=CARTESIAN_POINT ( 'NONE',  ( -13.38461538461538325, -11.16473453929635440, 33.15142922261926373 ) ) ;
#73765=DIRECTION ( 'NONE',  ( 0.000000000000000000, 0.8660254037844377084, 0.5000000000000015543 ) ) ;
#73766=CARTESIAN_POINT ( 'NONE',  ( 4.826923076923076650, -7.500000000000001776, 35.00000000000000000 ) ) ;
#73767=CARTESIAN_POINT ( 'NONE',  ( 11.78851585009985570, -9.148310452688876993, 34.47095581063188519 ) ) ;
#73768=ORIENTED_EDGE ( 'NONE', *, *, #13592, .T. ) ;
#73769=CARTESIAN_POINT ( 'NONE',  ( 6.923076923077238654, -2.255955759149395501, 30.00000000000324363 ) ) ;
#73770=CARTESIAN_POINT ( 'NONE',  ( -15.29685161012936767, -11.35647404775217595, 33.31231777344666511 ) ) ;
#73771=CARTESIAN_POINT ( 'NONE',  ( 15.23076923076923173, -1.509761064869970415, 31.06009739812519044 ) ) ;
#73772=ORIENTED_EDGE ( 'NONE', *, *, #40423, .T. ) ;
#73773=ORIENTED_EDGE ( 'NONE', *, *, #6791, .T. ) ;
#73774=EDGE_LOOP ( 'NONE', ( #72195, #21429, #46726, #84637 ) ) ;
#73775=CARTESIAN_POINT ( 'NONE',  ( 5.142178648199101865, -12.27809138561124591, 31.22303859784720359 ) ) ;
#73777=CARTESIAN_POINT ( 'NONE',  ( 13.38461538461526601, -11.48612834414049644, 32.76840700105863391 ) ) ;
#73778=CARTESIAN_POINT ( 'NONE',  ( -17.87193355239358894, -7.274843614157066263, 34.99539393749329719 ) ) ;
#73779=VERTEX_POINT ( 'NONE', #82055 ) ;
#73780=B_SPLINE_CURVE_WITH_KNOTS ( 'NONE', 3,
 ( #17374, #44831, #30002, #58796, #57018, #23236, #77296, #72310, #10618, #50698 ),
 .UNSPECIFIED., .F., .F.,
 ( 4, 2, 2, 2, 4 ),
 ( 0.0007817246256747463051, 0.0009771112852218896347, 0.001172497944769032747, 0.001367884604316176077, 0.001563271263863319407 ),
 .UNSPECIFIED. ) ;
#73781=B_SPLINE_CURVE_WITH_KNOTS ( 'NONE', 3,
 ( #76123, #41911, #69378, #7679, #8120, #35140, #62602, #912, #55851, #83341 ),
 .UNSPECIFIED., .F., .F.,
 ( 4, 2, 2, 2, 4 ),
 ( 0.0007817246256747470640, 0.0009771112852218898515, 0.001172497944769032747, 0.001367884604316175643, 0.001563271263863318539 ),
 .UNSPECIFIED. ) ;
#73782=ORIENTED_EDGE ( 'NONE', *, *, #69711, .F. ) ;
#73783=VERTEX_POINT ( 'NONE', #6823 ) ;
#73784=LINE ( 'NONE', #48056, #60225 ) ;
#73785=ORIENTED_EDGE ( 'NONE', *, *, #65064, .F. ) ;
#73786=DIRECTION ( 'NONE',  ( 0.000000000000000000, 0.1736481776669267785, -0.9848077530122087975 ) ) ;
#73787=CARTESIAN_POINT ( 'NONE',  ( 14.98079249982687955, -3.137211980971221781, 32.19342716148376837 ) ) ;
#73788=DIRECTION ( 'NONE',  ( 0.000000000000000000, 0.3420201433256641055, -0.9396926207859100932 ) ) ;
#73789=CARTESIAN_POINT ( 'NONE',  ( -15.16551365949320562, -9.442884908240273489, 34.35708131394835618 ) ) ;
#73792=VERTEX_POINT ( 'NONE', #55020 ) ;
#73793=ORIENTED_EDGE ( 'NONE', *, *, #74782, .F. ) ;
#73794=CARTESIAN_POINT ( 'NONE',  ( -10.83886953994894675, -10.97335522853832579, 33.68706563782419749 ) ) ;
#73795=DIRECTION ( 'NONE',  ( 0.000000000000000000, 0.1736481776669267785, -0.9848077530122087975 ) ) ;
#73797=CARTESIAN_POINT ( 'NONE',  ( 2.241609928332174206, -2.486705287966279876, 31.30864560766542937 ) ) ;
#73799=EDGE_CURVE ( 'NONE', #60558, #47459, #56496, .T. ) ;
#73800=CYLINDRICAL_SURFACE ( 'NONE', #31675, 0.2499999999999994726 ) ;
#73801=CARTESIAN_POINT ( 'NONE',  ( -1.634592115557738090, -8.303909089506435137, 34.68538101551103381 ) ) ;
#73802=CARTESIAN_POINT ( 'NONE',  ( -2.177166605928745113, -11.46989282347013095, 32.79007818306219946 ) ) ;
#73803=FACE_BOUND ( 'NONE', #5869, .T. ) ;
#73805=CARTESIAN_POINT ( 'NONE',  ( -0.4615384615384611200, -12.62096338111211580, 30.90682066428153263 ) ) ;
#73806=LINE ( 'NONE', #54402, #26467 ) ;
#73807=CARTESIAN_POINT ( 'NONE',  ( -17.75000000000000711, -12.75000000000000178, 29.75000000000000355 ) ) ;
#73808=DIRECTION ( 'NONE',  ( -0.000000000000000000, -0.8660254037844399289, -0.4999999999999980016 ) ) ;
#73810=FACE_OUTER_BOUND ( 'NONE', #69132, .T. ) ;
#73812=CARTESIAN_POINT ( 'NONE',  ( -17.32694630114453105, -5.765609946408405406, 34.70566812827424741 ) ) ;
#73813=CARTESIAN_POINT ( 'NONE',  ( -13.44988538517170440, -9.528491918058357157, 34.59228464037090589 ) ) ;
#73814=ORIENTED_EDGE ( 'NONE', *, *, #41533, .T. ) ;
#73815=EDGE_LOOP ( 'NONE', ( #10010, #56862, #36239, #57329 ) ) ;
#73818=AXIS2_PLACEMENT_3D ( 'NONE', #69851, #29752, #8154 ) ;
#73820=FACE_OUTER_BOUND ( 'NONE', #34938, .T. ) ;
#73821=B_SPLINE_CURVE_WITH_KNOTS ( 'NONE', 3,
 ( #54010, #68857, #48137, #76506, #75607, #26994, #40951, #68416, #61650, #61206 ),
 .UNSPECIFIED., .F., .F.,
 ( 4, 2, 2, 2, 4 ),
 ( 0.000000000000000000, 0.0001954311564186863323, 0.0003908623128373726646, 0.0005862934692560590241, 0.0007817246256747453293 ),
 .UNSPECIFIED. ) ;
#73823=DIRECTION ( 'NONE',  ( -0.000000000000000000, -0.000000000000000000, -1.000000000000000000 ) ) ;
#73825=EDGE_CURVE ( 'NONE', #6722, #30991, #19956, .T. ) ;
#73826=CARTESIAN_POINT ( 'NONE',  ( -6.923076923077044142, -10.21337939537710326, 33.94971097300076224 ) ) ;
#73827=CARTESIAN_POINT ( 'NONE',  ( -14.43784027742400689, -4.299443229763728169, 33.91186481527756058 ) ) ;
#73828=CARTESIAN_POINT ( 'NONE',  ( 10.61538461538449596, -12.46129190930018460, 30.37095296980731973 ) ) ;
#73829=DIRECTION ( 'NONE',  ( -0.000000000000000000, 1.000000000000000000, 3.491481338843133355E-15 ) ) ;
#73830=CARTESIAN_POINT ( 'NONE',  ( -5.299849294439222369, -9.086856451489516928, 34.49173150075333183 ) ) ;
#73831=PRESENTATION_STYLE_ASSIGNMENT (( #25183 ) ) ;
#73834=VERTEX_POINT ( 'NONE', #83384 ) ;
#73835=VERTEX_POINT ( 'NONE', #49141 ) ;
#73836=CARTESIAN_POINT ( 'NONE',  ( -9.822455662039391910, -2.647304123082328875, 31.75400227202885972 ) ) ;
#73837=CARTESIAN_POINT ( 'NONE',  ( 16.37685750545900376, -6.503523203565941380, 34.64991518177335195 ) ) ;
#73838=LINE ( 'NONE', #26977, #83387 ) ;
#73839=DIRECTION ( 'NONE',  ( -0.000000000000000000, 0.7660444431189791237, -0.6427876096865379196 ) ) ;
#73840=CARTESIAN_POINT ( 'NONE',  ( -14.98082371242109190, -2.824170634883621744, 31.52227843825338738 ) ) ;
#73842=CARTESIAN_POINT ( 'NONE',  ( -1.514763354347079982, -4.299443229763728169, 33.91186481527756058 ) ) ;
#73843=FACE_OUTER_BOUND ( 'NONE', #66234, .T. ) ;
#73844=CARTESIAN_POINT ( 'NONE',  ( 15.23076923076923173, -12.78798330534103123, 29.99999999999997868 ) ) ;
#73845=CARTESIAN_POINT ( 'NONE',  ( -6.222866263063099979, -2.251424796025575770, 29.88072029997477586 ) ) ;
#73846=CARTESIAN_POINT ( 'NONE',  ( 17.99999999999987566, -10.21337939537710326, 33.94971097300076224 ) ) ;
#73847=DIRECTION ( 'NONE',  ( 0.000000000000000000, 1.000000000000000000, 0.000000000000000000 ) ) ;
#73848=DIRECTION ( 'NONE',  ( 0.000000000000000000, 0.9396926207859126468, -0.3420201433256571111 ) ) ;
#73849=DIRECTION ( 'NONE',  ( 0.000000000000000000, 0.7660444431189822323, -0.6427876096865344779 ) ) ;
#73853=B_SPLINE_CURVE_WITH_KNOTS ( 'NONE', 3,
 ( #83466, #29840, #56425, #69052, #22629, #63617, #9135, #55530, #14550, #22196 ),
 .UNSPECIFIED., .F., .F.,
 ( 4, 2, 2, 2, 4 ),
 ( 0.0007817246256747451124, 0.0009771112852218885505, 0.001172497944769032097, 0.001367884604316175427, 0.001563271263863318973 ),
 .UNSPECIFIED. ) ;
#73854=DIRECTION ( 'NONE',  ( -0.000000000000000000, -0.3420201433256694346, -0.9396926207859080948 ) ) ;
#73855=CARTESIAN_POINT ( 'NONE',  ( 8.769230769230768274, -7.500000000000001776, 35.04278698407183867 ) ) ;
#73856=CARTESIAN_POINT ( 'NONE',  ( -14.30769230769230660, -1.215029322943914858, 32.30358669280327177 ) ) ;
#73858=VECTOR ( 'NONE', #66606, 999.9999999999998863 ) ;
#73859=VECTOR ( 'NONE', #19066, 1000.000000000000227 ) ;
#73860=CARTESIAN_POINT ( 'NONE',  ( 13.60739492588379562, -5.114059244376869984, 34.14424750095245287 ) ) ;
#73861=CARTESIAN_POINT ( 'NONE',  ( 10.83834774965129455, -7.369474539155828730, 34.99858011523957657 ) ) ;
#73864=CARTESIAN_POINT ( 'NONE',  ( -14.30769230769230660, -5.471508081941601098, 34.59228464037088457 ) ) ;
#73865=ORIENTED_EDGE ( 'NONE', *, *, #52594, .T. ) ;
#73866=CARTESIAN_POINT ( 'NONE',  ( -2.057637996053991891, -2.564540009722895419, 30.55348353981670684 ) ) ;
#73867=VERTEX_POINT ( 'NONE', #14026 ) ;
#73868=CARTESIAN_POINT ( 'NONE',  ( -18.24997673094235395, -11.79746400365624481, 32.30657167506340954 ) ) ;
#73869=CARTESIAN_POINT ( 'NONE',  ( -1.608100309179712806, -12.11044203135681840, 32.26167407432752299 ) ) ;
#73870=FACE_OUTER_BOUND ( 'NONE', #26254, .T. ) ;
#73871=ORIENTED_EDGE ( 'NONE', *, *, #82126, .T. ) ;
#73872=EDGE_LOOP ( 'NONE', ( #68354, #41672, #12316, #80881 ) ) ;
#73873=ORIENTED_EDGE ( 'NONE', *, *, #19045, .T. ) ;
#73874=CARTESIAN_POINT ( 'NONE',  ( -0.5916856709766818989, -3.285722584762969856, 32.44110544564090759 ) ) ;
#73875=CARTESIAN_POINT ( 'NONE',  ( 12.46153846153846168, -12.37446782046654192, 30.86335684631486131 ) ) ;
#73876=DIRECTION ( 'NONE',  ( -0.000000000000000000, 0.5000000000000009992, -0.8660254037844380415 ) ) ;
#73877=LINE ( 'NONE', #26127, #68776 ) ;
#73878=CARTESIAN_POINT ( 'NONE',  ( 9.627037246346917598, -9.442884908240170461, 34.35708131394840592 ) ) ;
#73879=DIRECTION ( 'NONE',  ( -0.000000000000000000, -0.7660444431189791237, -0.6427876096865379196 ) ) ;
#73880=LINE ( 'NONE', #53147, #63913 ) ;
#73881=ADVANCED_FACE ( 'NONE', ( #22557 ), #2268, .F. ) ;
#73882=AXIS2_PLACEMENT_3D ( 'NONE', #70759, #16689, #23877 ) ;
#73883=CARTESIAN_POINT ( 'NONE',  ( -12.68446467905460828, -6.503392248772476236, 34.64988816332204635 ) ) ;
#73884=EDGE_CURVE ( 'NONE', #75693, #82406, #46923, .T. ) ;
#73886=ORIENTED_EDGE ( 'NONE', *, *, #1827, .T. ) ;
#73887=ORIENTED_EDGE ( 'NONE', *, *, #85591, .T. ) ;
#73888=CARTESIAN_POINT ( 'NONE',  ( -3.903900744468109973, -8.476813868363244353, 34.90874843262270133 ) ) ;
#73889=ORIENTED_EDGE ( 'NONE', *, *, #58004, .F. ) ;
#73890=EDGE_CURVE ( 'NONE', #44606, #12325, #42633, .T. ) ;
#73891=CARTESIAN_POINT ( 'NONE',  ( 10.36536137809165403, -5.056417327199099532, 34.11270091957321426 ) ) ;
#73892=CARTESIAN_POINT ( 'NONE',  ( 1.634560902963527740, -2.824170634883621744, 31.52227843825337317 ) ) ;
#73893=EDGE_CURVE ( 'NONE', #49441, #35424, #29703, .T. ) ;
#73894=ORIENTED_EDGE ( 'NONE', *, *, #81824, .T. ) ;
#73895=DIRECTION ( 'NONE',  ( -1.000000000000000000, 0.000000000000000000, 0.000000000000000000 ) ) ;
#73896=ORIENTED_EDGE ( 'NONE', *, *, #26335, .F. ) ;
#73897=CARTESIAN_POINT ( 'NONE',  ( 11.53846153846141753, -2.625532179533778709, 30.86335684631627174 ) ) ;
#73898=EDGE_LOOP ( 'NONE', ( #67993, #62794 ) ) ;
#73899=CARTESIAN_POINT ( 'NONE',  ( -9.627114704013038704, -2.255955759149236073, 29.99999999999988987 ) ) ;
#73900=B_SPLINE_CURVE_WITH_KNOTS ( 'NONE', 3,
 ( #83310, #70672, #77862, #55824, #16597, #36442 ),
 .UNSPECIFIED., .F., .F.,
 ( 4, 2, 4 ),
 ( 0.0003909512603273894243, 0.0005862562993132134888, 0.0007815613382990374992 ),
 .UNSPECIFIED. ) ;
#73902=EDGE_CURVE ( 'NONE', #76288, #54695, #63972, .T. ) ;
#73903=CARTESIAN_POINT ( 'NONE',  ( -8.834501215191545853, -5.219633306516282545, 34.19971097300152962 ) ) ;
#73904=CARTESIAN_POINT ( 'NONE',  ( -11.53846153846153655, -11.91647553114624181, 32.58852847137148245 ) ) ;
#73905=FACE_BOUND ( 'NONE', #2555, .T. ) ;
#73907=CARTESIAN_POINT ( 'NONE',  ( 2.242368294888000158, -7.749976730030849303, 34.74374725381503737 ) ) ;
#73908=CARTESIAN_POINT ( 'NONE',  ( 1.607578518882061491, -7.369474539155830506, 34.99858011523957657 ) ) ;
#73910=CARTESIAN_POINT ( 'NONE',  ( 13.51540582558233794, -4.684288915650983043, 34.18129842949671371 ) ) ;
#73911=CARTESIAN_POINT ( 'NONE',  ( 1.384615384615386802, -12.34228464037088635, 31.77849191805839268 ) ) ;
#73912=LINE ( 'NONE', #40575, #81232 ) ;
#73913=CARTESIAN_POINT ( 'NONE',  ( -9.692307692307691624, -10.89733346790207413, 36.13435417666054406 ) ) ;
#73915=CARTESIAN_POINT ( 'NONE',  ( -10.54931626438217585, -4.098570777380720287, 33.41473453929635440 ) ) ;
#73916=VERTEX_POINT ( 'NONE', #82940 ) ;
#73917=ORIENTED_EDGE ( 'NONE', *, *, #30220, .T. ) ;
#73918=CARTESIAN_POINT ( 'NONE',  ( -0.5922299282060198289, -8.999036380462717588, 34.52022231692819076 ) ) ;
#73919=CARTESIAN_POINT ( 'NONE',  ( -0.4615384615384611200, -7.500000000000001776, 35.04278698407183867 ) ) ;
#73920=B_SPLINE_CURVE_WITH_KNOTS ( 'NONE', 3,
 ( #47444, #28976, #61843, #41584, #1042, #7802, #81695, #600, #55093, #34821 ),
 .UNSPECIFIED., .F., .F.,
 ( 4, 2, 2, 2, 4 ),
 ( 0.0007817359430256221996, 0.0009771253907249863487, 0.001172514838424350498, 0.001367904286123714647, 0.001563293733823078796 ),
 .UNSPECIFIED. ) ;
#73921=CARTESIAN_POINT ( 'NONE',  ( 16.21910129335898887, -11.67786785259547777, 32.92929555188713664 ) ) ;
#73922=CARTESIAN_POINT ( 'NONE',  ( -4.023320715612507925, -9.503571793651733657, 34.60286762892837942 ) ) ;
#73924=CARTESIAN_POINT ( 'NONE',  ( -2.084680956079458358, -2.758310577978208666, 31.33698337089302299 ) ) ;
#73925=VERTEX_POINT ( 'NONE', #56348 ) ;
#73926=EDGE_CURVE ( 'NONE', #29248, #32965, #74864, .T. ) ;
#73927=CARTESIAN_POINT ( 'NONE',  ( -11.78848477575450282, -12.22074536777954989, 31.39888409691088356 ) ) ;
#73928=CARTESIAN_POINT ( 'NONE',  ( 15.16468685140909400, -3.937682226553330445, 33.60647404775217240 ) ) ;
#73929=CARTESIAN_POINT ( 'NONE',  ( 10.61538461538449418, -3.083524468854526912, 32.58852847137268327 ) ) ;
#73930=EDGE_CURVE ( 'NONE', #12523, #20467, #69861, .T. ) ;
#73931=CARTESIAN_POINT ( 'NONE',  ( -3.230769230769229949, -12.62096338111211580, 30.90682066428153263 ) ) ;
#73932=ORIENTED_EDGE ( 'NONE', *, *, #27515, .F. ) ;
#73933=ORIENTED_EDGE ( 'NONE', *, *, #78970, .F. ) ;
#73935=ORIENTED_EDGE ( 'NONE', *, *, #63148, .T. ) ;
#73936=EDGE_CURVE ( 'NONE', #2090, #30159, #81233, .T. ) ;
#73938=CARTESIAN_POINT ( 'NONE',  ( -6.249999999999997335, -7.500000000000001776, 35.00000000000000000 ) ) ;
#73939=EDGE_CURVE ( 'NONE', #7198, #69679, #57669, .T. ) ;
#73940=ORIENTED_EDGE ( 'NONE', *, *, #42215, .T. ) ;
#73942=CARTESIAN_POINT ( 'NONE',  ( -6.130147969731693181, -9.504002272028875709, 34.60269587691767867 ) ) ;
#73943=CARTESIAN_POINT ( 'NONE',  ( 3.480823650682684178, -10.06805714834173848, 34.32951233291982618 ) ) ;
#73944=CARTESIAN_POINT ( 'NONE',  ( 14.37386144865496718, -7.250054483168843156, 34.74374881642865631 ) ) ;
#73945=CARTESIAN_POINT ( 'NONE',  ( -11.47239318745910275, -8.973038597847271092, 34.52809138561121216 ) ) ;
#73947=ORIENTED_EDGE ( 'NONE', *, *, #51202, .F. ) ;
#73948=CARTESIAN_POINT ( 'NONE',  ( -15.23076923076922995, -11.91647553114624181, 32.58852847137148245 ) ) ;
#73949=ORIENTED_EDGE ( 'NONE', *, *, #23992, .F. ) ;
#73950=CARTESIAN_POINT ( 'NONE',  ( -5.076923076923199218, -2.379036618888197729, 30.90682066428292885 ) ) ;
#73951=CARTESIAN_POINT ( 'NONE',  ( 8.900021210197715860, -12.35292014791297710, 31.75344720912887198 ) ) ;
#73952=CARTESIAN_POINT ( 'NONE',  ( -13.38461538461550582, -5.219633306517616589, 34.19971097300220464 ) ) ;
#73953=CARTESIAN_POINT ( 'NONE',  ( -10.74607521849492464, -3.338472653186243644, 32.95098750199972670 ) ) ;
#73954=CARTESIAN_POINT ( 'NONE',  ( 2.372947447205147053, -2.657715359629131857, 31.77849191805844242 ) ) ;
#73955=DIRECTION ( 'NONE',  ( 0.000000000000000000, 0.9396926207859126468, 0.3420201433256571111 ) ) ;
#73956=CARTESIAN_POINT ( 'NONE',  ( -0.5922290646487671228, -2.494641256782728966, 31.33461815524612959 ) ) ;
#73958=VERTEX_POINT ( 'NONE', #30207 ) ;
#73959=CARTESIAN_POINT ( 'NONE',  ( 15.10062202133100939, -8.587444163452046197, 34.63053765926554206 ) ) ;
#73960=CARTESIAN_POINT ( 'NONE',  ( -4.153846153846152411, -13.95598074871891292, 31.83374038241031911 ) ) ;
#73961=CARTESIAN_POINT ( 'NONE',  ( -13.38461538461550582, -8.613356846316285953, 34.62446782046622218 ) ) ;
#73962=ORIENTED_EDGE ( 'NONE', *, *, #4354, .F. ) ;
#73963=CARTESIAN_POINT ( 'NONE',  ( -12.71156169883143150, -11.86270091957321249, 32.19358267280087915 ) ) ;
#73964=DIRECTION ( 'NONE',  ( 0.000000000000000000, -6.938893903907222067E-15, 1.000000000000000000 ) ) ;
#73965=CARTESIAN_POINT ( 'NONE',  ( 13.31934493865461278, -3.835265460703609186, 33.15142922261924241 ) ) ;
#73966=CYLINDRICAL_SURFACE ( 'NONE', #15742, 0.2499999999999995559 ) ;
#73968=CARTESIAN_POINT ( 'NONE',  ( 6.000000000000001776, -8.120952969808772792, 34.71129190930000163 ) ) ;
#73969=EDGE_LOOP ( 'NONE', ( #54475, #76468, #34639, #54983 ) ) ;
#73971=FACE_OUTER_BOUND ( 'NONE', #6539, .T. ) ;
#73972=AXIS2_PLACEMENT_3D ( 'NONE', #56501, #48849, #43865 ) ;
#73973=CARTESIAN_POINT ( 'NONE',  ( 15.23076923076923173, -13.63283147151868846, 33.57946703557072254 ) ) ;
#73974=CARTESIAN_POINT ( 'NONE',  ( -2.084912638714238931, -5.827830569534416583, 34.72679350104403539 ) ) ;
#73975=ORIENTED_EDGE ( 'NONE', *, *, #17901, .F. ) ;
#73976=CARTESIAN_POINT ( 'NONE',  ( 16.15384615384615330, -12.34228464037088635, 31.77849191805839268 ) ) ;
#73977=B_SPLINE_CURVE_WITH_KNOTS ( 'NONE', 3,
 ( #33883, #53263, #25354, #25804, #80761, #12286, #67239, #60469, #26243, #53713 ),
 .UNSPECIFIED., .F., .F.,
 ( 4, 2, 2, 2, 4 ),
 ( 0.0007817246256747453293, 0.0009771112852218889842, 0.001172497944769032531, 0.001367884604316176294, 0.001563271263863319840 ),
 .UNSPECIFIED. ) ;
#73978=AXIS2_PLACEMENT_3D ( 'NONE', #17039, #35997, #44489 ) ;
#73980=VERTEX_POINT ( 'NONE', #79727 ) ;
#73981=DIRECTION ( 'NONE',  ( -0.000000000000000000, -0.3420201433256694901, -0.9396926207859082059 ) ) ;
#73983=CARTESIAN_POINT ( 'NONE',  ( -20.74999999999999645, -7.500000000000000000, 29.75000000000000355 ) ) ;
#73984=ORIENTED_EDGE ( 'NONE', *, *, #87315, .F. ) ;
#73986=CARTESIAN_POINT ( 'NONE',  ( -14.43825222130567276, -2.254533558242299396, 29.97296025877828285 ) ) ;
#73987=EDGE_CURVE ( 'NONE', #45914, #7438, #44137, .T. ) ;
#73989=EDGE_CURVE ( 'NONE', #22506, #7245, #26523, .T. ) ;
#73990=CARTESIAN_POINT ( 'NONE',  ( -5.999999999999998224, -5.471508081941601098, 34.59228464037088457 ) ) ;
#73991=DIRECTION ( 'NONE',  ( -0.000000000000000000, 0.9396926207859093161, -0.3420201433256663259 ) ) ;
#73993=CARTESIAN_POINT ( 'NONE',  ( -4.023055712879203938, -12.35292014791297710, 31.75344720912887198 ) ) ;
#73994=ORIENTED_EDGE ( 'NONE', *, *, #39554, .T. ) ;
#73995=CARTESIAN_POINT ( 'NONE',  ( 8.519207531937803779, -12.43535235679832596, 30.55408501211184813 ) ) ;
#74000=CARTESIAN_POINT ( 'NONE',  ( 6.222779541268410597, -9.332535724633407526, 34.40230450496446224 ) ) ;
#74001=CARTESIAN_POINT ( 'NONE',  ( -6.673022611438608642, -5.728107161865375829, 34.42597550085002922 ) ) ;
#74002=CARTESIAN_POINT ( 'NONE',  ( 7.846153846153846700, -12.37446782046654192, 30.86335684631486131 ) ) ;
#74003=LINE ( 'NONE', #76088, #1960 ) ;
#74004=EDGE_CURVE ( 'NONE', #45628, #16932, #57601, .T. ) ;
#74005=EDGE_LOOP ( 'NONE', ( #26732, #70397 ) ) ;
#74006=VERTEX_POINT ( 'NONE', #65748 ) ;
#74007=ORIENTED_EDGE ( 'NONE', *, *, #62377, .F. ) ;
#74008=VERTEX_POINT ( 'NONE', #43708 ) ;
#74009=CARTESIAN_POINT ( 'NONE',  ( -10.36543909703647159, -11.37275283266504111, 32.91324779482534524 ) ) ;
#74010=EDGE_CURVE ( 'NONE', #16935, #67793, #48999, .T. ) ;
#74011=CARTESIAN_POINT ( 'NONE',  ( -3.454254155333561283, -6.716662450894490100, 34.94144148231605840 ) ) ;
#74012=CARTESIAN_POINT ( 'NONE',  ( 15.16549878480845770, -5.219633306516282545, 34.19971097300152962 ) ) ;
#74014=CARTESIAN_POINT ( 'NONE',  ( 3.480823650682683734, -9.233818618650603938, 34.70587769442853698 ) ) ;
#74015=CARTESIAN_POINT ( 'NONE',  ( -0.6850234052624076808, -11.89387501736623243, 32.13663884655804992 ) ) ;
#74016=CARTESIAN_POINT ( 'NONE',  ( -15.23076923076935074, -8.613356846316285953, 34.62446782046622218 ) ) ;
#74018=ORIENTED_EDGE ( 'NONE', *, *, #79220, .T. ) ;
#74019=B_SPLINE_CURVE_WITH_KNOTS ( 'NONE', 3,
 ( #13352, #47577, #33629, #27750, #19230, #34066, #41276, #69184, #54329, #82711 ),
 .UNSPECIFIED., .F., .F.,
 ( 4, 2, 2, 2, 4 ),
 ( 0.000000000000000000, 0.0001954311564186879315, 0.0003908623128373758630, 0.0005862934692560637946, 0.0007817246256747517261 ),
 .UNSPECIFIED. ) ;
#74020=ORIENTED_EDGE ( 'NONE', *, *, #12372, .T. ) ;
#74022=CARTESIAN_POINT ( 'NONE',  ( -1.608100328339331142, -11.41268669641500466, 32.86336882939237825 ) ) ;
#74024=FACE_OUTER_BOUND ( 'NONE', #80653, .T. ) ;
#74025=CARTESIAN_POINT ( 'NONE',  ( -7.623374177175779032, -9.418065098278013636, 34.63729479722530158 ) ) ;
#74027=CARTESIAN_POINT ( 'NONE',  ( -9.019253993452222673, -6.652501968072648708, 34.93155406624980941 ) ) ;
#74028=FACE_BOUND ( 'NONE', #10559, .T. ) ;
#74029=EDGE_LOOP ( 'NONE', ( #71191, #82023 ) ) ;
#74031=ADVANCED_FACE ( 'NONE', ( #85590 ), #78824, .F. ) ;
#74032=ORIENTED_EDGE ( 'NONE', *, *, #63724, .T. ) ;
#74033=CARTESIAN_POINT ( 'NONE',  ( -18.00000000000000000, -7.500000000000001776, 35.00000000000000000 ) ) ;
#74034=AXIS2_PLACEMENT_3D ( 'NONE', #56921, #77198, #9620 ) ;
#74035=ORIENTED_EDGE ( 'NONE', *, *, #49895, .T. ) ;
#74037=FACE_BOUND ( 'NONE', #65117, .T. ) ;
#74039=CARTESIAN_POINT ( 'NONE',  ( 15.00728430620490172, -6.716662450894489211, 34.94144148231605840 ) ) ;
#74040=EDGE_LOOP ( 'NONE', ( #70444, #19100, #63358, #87623 ) ) ;
#74041=CARTESIAN_POINT ( 'NONE',  ( -6.130476708116463058, -7.276988635370452485, 34.74523720219453793 ) ) ;
#74042=CARTESIAN_POINT ( 'NONE',  ( 9.019230769232187583, -7.500000000000154543, 35.00000000000007105 ) ) ;
#74043=EDGE_CURVE ( 'NONE', #84646, #19767, #74301, .T. ) ;
#74044=CARTESIAN_POINT ( 'NONE',  ( 1.253923917947826538, -3.062553014421049546, 32.05460306192773601 ) ) ;
#74045=ORIENTED_EDGE ( 'NONE', *, *, #22345, .T. ) ;
#74046=CARTESIAN_POINT ( 'NONE',  ( 14.30769230769231015, -3.322132147404559976, 32.92929555188717927 ) ) ;
#74047=CARTESIAN_POINT ( 'NONE',  ( -5.999999999999998224, -11.11383981884818262, 36.00935417666054406 ) ) ;
#74048=LINE ( 'NONE', #75372, #43309 ) ;
#74049=ORIENTED_EDGE ( 'NONE', *, *, #79035, .T. ) ;
#74050=B_SPLINE_CURVE_WITH_KNOTS ( 'NONE', 3,
 ( #39242, #37438, #86546, #10871, #32466, #32030, #23920, #50936, #51369, #79328 ),
 .UNSPECIFIED., .F., .F.,
 ( 4, 2, 2, 2, 4 ),
 ( 0.000000000000000000, 0.0001954311564186861155, 0.0003908623128373722310, 0.0005862934692560583735, 0.0007817246256747444619 ),
 .UNSPECIFIED. ) ;
#74051=CARTESIAN_POINT ( 'NONE',  ( 2.438482748659257737, -12.35292014791297710, 31.75344720912887198 ) ) ;
#74052=CARTESIAN_POINT ( 'NONE',  ( 4.153846153846154188, -9.905515769479276145, 34.41647553114623292 ) ) ;
#74053=EDGE_LOOP ( 'NONE', ( #47461, #21328 ) ) ;
#74054=CARTESIAN_POINT ( 'NONE',  ( 8.639082799499069765, -11.66186481527757302, 32.95055677023626117 ) ) ;
#74055=CYLINDRICAL_SURFACE ( 'NONE', #16661, 0.2500000000000009437 ) ;
#74056=CARTESIAN_POINT ( 'NONE',  ( 0.4615384615383382183, -11.06231777344772027, 33.60647404775119895 ) ) ;
#74057=CARTESIAN_POINT ( 'NONE',  ( 13.63466969625370240, -12.41262288849542017, 30.68299917996395010 ) ) ;
#74058=CARTESIAN_POINT ( 'NONE',  ( -15.93083480223330817, -4.187068189119696804, 33.49521262558774026 ) ) ;
#74059=LINE ( 'NONE', #26306, #65341 ) ;
#74060=CARTESIAN_POINT ( 'NONE',  ( -1.384615384615505151, -5.219633306517616589, 34.19971097300220464 ) ) ;
#74061=CARTESIAN_POINT ( 'NONE',  ( 9.692307692307695177, -4.661471528628507777, 34.16647553114623292 ) ) ;
#74062=CARTESIAN_POINT ( 'NONE',  ( 8.834486340506796154, -12.27809138561124591, 31.22303859784720359 ) ) ;
#74063=CARTESIAN_POINT ( 'NONE',  ( -6.857821351800898135, -2.892918686051625166, 31.69288490824025928 ) ) ;
#74064=EDGE_CURVE ( 'NONE', #44215, #76427, #86675, .T. ) ;
#74066=ORIENTED_EDGE ( 'NONE', *, *, #78491, .F. ) ;
#74067=CARTESIAN_POINT ( 'NONE',  ( -12.46153846153858247, -8.613356846316285953, 34.62446782046622218 ) ) ;
#74068=EDGE_LOOP ( 'NONE', ( #86327, #37424, #29661, #9125 ) ) ;
#74069=EDGE_CURVE ( 'NONE', #10994, #24465, #66224, .T. ) ;
#74070=ORIENTED_EDGE ( 'NONE', *, *, #21011, .T. ) ;
#74071=CARTESIAN_POINT ( 'NONE',  ( 5.076923076923075762, -13.53365097954675988, 30.81389545987213552 ) ) ;
#74073=CARTESIAN_POINT ( 'NONE',  ( -14.30769230769242739, -6.026961402154118019, 34.52809138561165270 ) ) ;
#74076=CARTESIAN_POINT ( 'NONE',  ( 10.61538461538461675, -2.486705287966279876, 31.30864560766543647 ) ) ;
#74077=CARTESIAN_POINT ( 'NONE',  ( -7.596208327805703320, -5.852078868378309373, 34.47109172314383585 ) ) ;
#74078=CARTESIAN_POINT ( 'NONE',  ( -5.300408001487405762, -3.562934362175799841, 33.22335522853832401 ) ) ;
#74079=DIRECTION ( 'NONE',  ( -0.000000000000000000, 0.9396926207859092051, -0.3420201433256662704 ) ) ;
#74080=DIRECTION ( 'NONE',  ( 0.000000000000000000, 0.9848077530122072432, 0.1736481776669354937 ) ) ;
#74083=CARTESIAN_POINT ( 'NONE',  ( 3.230769230769231726, -4.102666532097928531, 36.13435417666054406 ) ) ;
#74084=CARTESIAN_POINT ( 'NONE',  ( -9.692307692307691624, -1.509761064869970415, 31.06009739812519044 ) ) ;
#74085=CARTESIAN_POINT ( 'NONE',  ( -2.557669038634660108, -4.236021600441998380, 33.53823185664189310 ) ) ;
#74086=EDGE_CURVE ( 'NONE', #47342, #47846, #73752, .T. ) ;
#74087=EDGE_CURVE ( 'NONE', #37210, #50903, #73415, .T. ) ;
#74089=VERTEX_POINT ( 'NONE', #11719 ) ;
#74090=CARTESIAN_POINT ( 'NONE',  ( 14.98076923076923173, -2.499999999999998668, 29.75000000000000355 ) ) ;
#74091=CYLINDRICAL_SURFACE ( 'NONE', #46017, 0.2500000000000012212 ) ;
#74092=DIRECTION ( 'NONE',  ( -0.000000000000000000, 1.000000000000000000, 0.000000000000000000 ) ) ;
#74095=CARTESIAN_POINT ( 'NONE',  ( -0.5268089074992371446, -6.879047030191174805, 34.71129190930000163 ) ) ;
#74098=VERTEX_POINT ( 'NONE', #26110 ) ;
#74099=CARTESIAN_POINT ( 'NONE',  ( 5.999999999999878320, -11.06231777344772027, 33.60647404775119895 ) ) ;
#74101=VERTEX_POINT ( 'NONE', #80629 ) ;
#74102=CARTESIAN_POINT ( 'NONE',  ( 5.326868595271217366, -8.433404298154334455, 34.66254593164985920 ) ) ;
#74104=CARTESIAN_POINT ( 'NONE',  ( -4.377331078410484189, -12.69144148231606017, 30.53333754910549303 ) ) ;
#74105=B_SPLINE_CURVE_WITH_KNOTS ( 'NONE', 3,
 ( #74757, #88727, #6298, #47715, #41407, #68868, #67998, #40964, #54465, #28325 ),
 .UNSPECIFIED., .F., .F.,
 ( 4, 2, 2, 2, 4 ),
 ( 0.000000000000000000, 0.0001954339857564076099, 0.0003908679715128152198, 0.0005863019572692228839, 0.0007817359430256304396 ),
 .UNSPECIFIED. ) ;
#74106=VECTOR ( 'NONE', #9630, 1000.000000000000227 ) ;
#74107=CARTESIAN_POINT ( 'NONE',  ( 11.66898697669518548, -2.372941743896879174, 30.88044141588253666 ) ) ;
#74108=CARTESIAN_POINT ( 'NONE',  ( 14.30769230769231015, -7.500000000000001776, 35.04278698407183867 ) ) ;
#74109=ADVANCED_FACE ( 'NONE', ( #59890 ), #87386, .F. ) ;
#74110=ORIENTED_EDGE ( 'NONE', *, *, #38854, .F. ) ;
#74111=ORIENTED_EDGE ( 'NONE', *, *, #14499, .F. ) ;
#74112=VERTEX_POINT ( 'NONE', #27000 ) ;
#74113=CARTESIAN_POINT ( 'NONE',  ( 5.777073782483853392, -2.554751324335733820, 30.48935550225260727 ) ) ;
#74114=CARTESIAN_POINT ( 'NONE',  ( 9.942253101685738059, -2.341251567377310217, 30.72681386836322659 ) ) ;
#74115=CARTESIAN_POINT ( 'NONE',  ( 16.28463659481310799, -5.496552790871120031, 34.60292014791297532 ) ) ;
#74116=CARTESIAN_POINT ( 'NONE',  ( -16.37677311275299985, -2.308479472611653094, 30.53278059502174457 ) ) ;
#74117=LINE ( 'NONE', #68681, #26517 ) ;
#74118=ORIENTED_EDGE ( 'NONE', *, *, #88529, .F. ) ;
#74119=VERTEX_POINT ( 'NONE', #46383 ) ;
#74121=CARTESIAN_POINT ( 'NONE',  ( 11.53846153846153832, -8.973038597847269315, 34.52809138561121927 ) ) ;
#74122=EDGE_LOOP ( 'NONE', ( #83179, #88671, #49560, #78648 ) ) ;
#74123=CARTESIAN_POINT ( 'NONE',  ( 10.39189967166066708, -12.44517049084099725, 30.48991314939691932 ) ) ;
#74124=LINE ( 'NONE', #12421, #21584 ) ;
#74127=CARTESIAN_POINT ( 'NONE',  ( 3.295962219063885090, -2.255955759149235629, 29.99999999999988631 ) ) ;
#74128=VERTEX_POINT ( 'NONE', #67102 ) ;
#74129=CARTESIAN_POINT ( 'NONE',  ( 13.60739505359345181, -10.97394488606064122, 33.68653795673694873 ) ) ;
#74130=CARTESIAN_POINT ( 'NONE',  ( -3.230769230769229949, -12.78798330534102945, 29.74999999999997868 ) ) ;
#74131=EDGE_CURVE ( 'NONE', #58896, #2541, #60331, .T. ) ;
#74132=FACE_BOUND ( 'NONE', #12382, .T. ) ;
#74133=CARTESIAN_POINT ( 'NONE',  ( -5.076923076923075762, -12.10708131394839349, 31.69288490824020244 ) ) ;
#74134=CARTESIAN_POINT ( 'NONE',  ( 2.307692307692309264, -2.499999999999998668, 29.75000000000001421 ) ) ;
#74135=VERTEX_POINT ( 'NONE', #53575 ) ;
#74136=CARTESIAN_POINT ( 'NONE',  ( 6.857806477116147548, -8.613356846314824011, 34.62446782046655613 ) ) ;
#74137=EDGE_CURVE ( 'NONE', #54522, #54986, #85525, .T. ) ;
#74138=CARTESIAN_POINT ( 'NONE',  ( -14.08491276642389245, -2.600157965045224451, 30.74683119005207743 ) ) ;
#74139=B_SPLINE_CURVE_WITH_KNOTS ( 'NONE', 3,
 ( #77945, #50892, #45487, #85153, #58546, #4048, #64859, #16249, #86500, #31536 ),
 .UNSPECIFIED., .F., .F.,
 ( 4, 2, 2, 2, 4 ),
 ( 0.000000000000000000, 0.0001954311564186871184, 0.0003908623128373742367, 0.0005862934692560614093, 0.0007817246256747484735 ),
 .UNSPECIFIED. ) ;
#74140=LINE ( 'NONE', #12437, #53811 ) ;
#74142=EDGE_CURVE ( 'NONE', #85754, #1046, #65094, .T. ) ;
#74143=CARTESIAN_POINT ( 'NONE',  ( 6.923076923076924238, -1.215029322943914858, 32.30358669280327177 ) ) ;
#74144=CARTESIAN_POINT ( 'NONE',  ( 14.37375964104238513, -9.905515769479276145, 34.41647553114623292 ) ) ;
#74145=CARTESIAN_POINT ( 'NONE',  ( 4.153846153846030731, -11.67786785259630911, 32.92929555188603530 ) ) ;
#74146=LINE ( 'NONE', #19203, #60142 ) ;
#74147=CARTESIAN_POINT ( 'NONE',  ( -0.5921488211629901688, -7.722926236386453702, 34.74524107206102030 ) ) ;
#74148=AXIS2_PLACEMENT_3D ( 'NONE', #43024, #51526, #3809 ) ;
#74149=FACE_BOUND ( 'NONE', #68251, .T. ) ;
#74150=DIRECTION ( 'NONE',  ( 0.000000000000000000, 1.000000000000000000, 0.000000000000000000 ) ) ;
#74151=CARTESIAN_POINT ( 'NONE',  ( 11.53846153846153832, -13.87047571288749737, 32.06866353760679544 ) ) ;
#74152=CARTESIAN_POINT ( 'NONE',  ( 9.757501674091050958, -2.506253911140448043, 29.99999999999988631 ) ) ;
#74153=CARTESIAN_POINT ( 'NONE',  ( -8.546451227962355901, -11.89424750095246175, 32.13594075562311758 ) ) ;
#74154=CARTESIAN_POINT ( 'NONE',  ( -2.242437168179467477, -12.51329471203373700, 31.30864560766537963 ) ) ;
#74155=EDGE_CURVE ( 'NONE', #60075, #46303, #44675, .T. ) ;
#74156=CARTESIAN_POINT ( 'NONE',  ( 8.835298102580845025, -12.62096338111211757, 30.90682066428152908 ) ) ;
#74158=ORIENTED_EDGE ( 'NONE', *, *, #11073, .F. ) ;
#74159=DIRECTION ( 'NONE',  ( 0.000000000000000000, 0.6427876096865373645, -0.7660444431189797898 ) ) ;
#74160=VERTEX_POINT ( 'NONE', #1737 ) ;
#74161=FACE_OUTER_BOUND ( 'NONE', #62109, .T. ) ;
#74163=CARTESIAN_POINT ( 'NONE',  ( 2.242422307135989890, -2.379036618887870880, 30.90682066428147934 ) ) ;
#74164=CYLINDRICAL_SURFACE ( 'NONE', #61756, 0.2499999999999994726 ) ;
#74166=VERTEX_POINT ( 'NONE', #13919 ) ;
#74167=CARTESIAN_POINT ( 'NONE',  ( 3.296837581771669523, -6.386643153685127139, 34.62446782046654192 ) ) ;
#74168=CARTESIAN_POINT ( 'NONE',  ( 1.253924781505079356, -11.93127051446800024, 32.56575433478200665 ) ) ;
#74170=CARTESIAN_POINT ( 'NONE',  ( 15.10007862765893094, -11.93127051446799847, 32.56575433478202797 ) ) ;
#74171=CARTESIAN_POINT ( 'NONE',  ( 11.53846153846153832, -2.538708090699994813, 30.37095296980875503 ) ) ;
#74172=CARTESIAN_POINT ( 'NONE',  ( -4.826868657009622865, -12.01375889529407281, 32.43194544308182969 ) ) ;
#74173=CARTESIAN_POINT ( 'NONE',  ( -0.5916864312701562989, -8.630895178749536711, 34.87696386517710323 ) ) ;
#74174=CARTESIAN_POINT ( 'NONE',  ( 0.3954550505825807916, -11.16473453929635440, 33.15142922261925662 ) ) ;
#74177=CARTESIAN_POINT ( 'NONE',  ( 3.361607561255992138, -7.277220318596959281, 34.99547417642776992 ) ) ;
#74180=CYLINDRICAL_SURFACE ( 'NONE', #25458, 0.2500000000000008882 ) ;
#74181=CARTESIAN_POINT ( 'NONE',  ( 15.36155967173618286, -10.70102852606553157, 33.91149625220312913 ) ) ;
#74183=EDGE_CURVE ( 'NONE', #72329, #7620, #75717, .T. ) ;
#74185=CARTESIAN_POINT ( 'NONE',  ( -8.769230769230768274, -3.322132147404559976, 32.92929555188717927 ) ) ;
#74186=ORIENTED_EDGE ( 'NONE', *, *, #82386, .F. ) ;
#74187=CARTESIAN_POINT ( 'NONE',  ( 6.988332494352945901, -8.613356846314928816, 34.62446782046653482 ) ) ;
#74188=LINE ( 'NONE', #67432, #48839 ) ;
#74189=CARTESIAN_POINT ( 'NONE',  ( 8.068933515131908152, -2.612705202774698421, 31.66806509827799943 ) ) ;
#74190=ORIENTED_EDGE ( 'NONE', *, *, #48626, .T. ) ;
#74191=CARTESIAN_POINT ( 'NONE',  ( 11.60452988946397923, -4.786620604624113540, 33.94971097300155805 ) ) ;
#74192=LINE ( 'NONE', #12492, #82936 ) ;
#74193=CARTESIAN_POINT ( 'NONE',  ( -16.94608474643631979, -7.277220318596959281, 34.99547417642776992 ) ) ;
#74195=CARTESIAN_POINT ( 'NONE',  ( -11.76194646302587010, -2.612411019501189369, 31.66733052389439962 ) ) ;
#74196=EDGE_CURVE ( 'NONE', #765, #38908, #48583, .T. ) ;
#74198=FACE_OUTER_BOUND ( 'NONE', #34643, .T. ) ;
#74199=CYLINDRICAL_SURFACE ( 'NONE', #35069, 0.2499999999999995559 ) ;
#74200=EDGE_CURVE ( 'NONE', #87991, #85626, #84424, .T. ) ;
#74201=ADVANCED_FACE ( 'NONE', ( #41850 ), #35078, .F. ) ;
#74202=CARTESIAN_POINT ( 'NONE',  ( -13.16183571563731824, -8.540255544307065350, 34.89611431652622286 ) ) ;
#74203=ORIENTED_EDGE ( 'NONE', *, *, #46727, .T. ) ;
#74204=VERTEX_POINT ( 'NONE', #55787 ) ;
#74205=EDGE_LOOP ( 'NONE', ( #56168, #14847, #50632, #40222 ) ) ;
#74206=CARTESIAN_POINT ( 'NONE',  ( -9.822999158975248335, -2.729777683071817229, 31.24903638046269450 ) ) ;
#74207=CARTESIAN_POINT ( 'NONE',  ( -6.792551221313360976, -4.459921816937789885, 33.71989282347011851 ) ) ;
#74208=CARTESIAN_POINT ( 'NONE',  ( -8.069080805060693251, -12.64616026154729411, 30.79003144601914244 ) ) ;
#74209=CARTESIAN_POINT ( 'NONE',  ( -9.469528023329624844, -12.69155399931963046, 30.53255429739157734 ) ) ;
#74210=EDGE_CURVE ( 'NONE', #3309, #14831, #10234, .T. ) ;
#74211=CARTESIAN_POINT ( 'NONE',  ( -18.06870381900347056, -7.250491025975066783, 34.99406763069168846 ) ) ;
#74212=ORIENTED_EDGE ( 'NONE', *, *, #21829, .F. ) ;
#74213=EDGE_CURVE ( 'NONE', #24368, #49738, #51217, .T. ) ;
#74214=ADVANCED_FACE ( 'NONE', ( #24213 ), #44475, .F. ) ;
#74215=AXIS2_PLACEMENT_3D ( 'NONE', #41248, #13325, #68711 ) ;
#74216=VERTEX_POINT ( 'NONE', #58003 ) ;
#74217=EDGE_LOOP ( 'NONE', ( #53336, #32126, #62636, #51532 ) ) ;
#74218=CARTESIAN_POINT ( 'NONE',  ( -6.923076923076922462, -8.164416787775445883, 34.95778746994557906 ) ) ;
#74219=ORIENTED_EDGE ( 'NONE', *, *, #71320, .T. ) ;
#74220=CARTESIAN_POINT ( 'NONE',  ( 14.30769230769231015, -9.058645607665452459, 34.76329471203371924 ) ) ;
#74221=EDGE_CURVE ( 'NONE', #46544, #47459, #38178, .T. ) ;
#74222=CARTESIAN_POINT ( 'NONE',  ( 15.16468581981335007, -3.050289026998445951, 32.03036669348365706 ) ) ;
#74223=CARTESIAN_POINT ( 'NONE',  ( -18.00000000000000000, -1.163064389776900187, 32.05645593858272235 ) ) ;
#74224=CARTESIAN_POINT ( 'NONE',  ( 1.384615384615386802, -10.89733346790207413, 36.13435417666054406 ) ) ;
#74225=AXIS2_PLACEMENT_3D ( 'NONE', #43731, #71199, #9502 ) ;
#74226=ORIENTED_EDGE ( 'NONE', *, *, #86306, .F. ) ;
#74227=ORIENTED_EDGE ( 'NONE', *, *, #31104, .T. ) ;
#74228=ORIENTED_EDGE ( 'NONE', *, *, #46415, .T. ) ;
#74229=DIRECTION ( 'NONE',  ( -0.000000000000000000, 0.3420201433256694346, -0.9396926207859080948 ) ) ;
#74230=FACE_OUTER_BOUND ( 'NONE', #64499, .T. ) ;
#74231=ORIENTED_EDGE ( 'NONE', *, *, #28836, .T. ) ;
#74232=CARTESIAN_POINT ( 'NONE',  ( 2.084207383127975266, -2.612411019501189813, 31.66733052389439962 ) ) ;
#74234=VERTEX_POINT ( 'NONE', #30967 ) ;
#74235=CARTESIAN_POINT ( 'NONE',  ( 15.23076923076953904, -2.506253911140615021, 30.00000000000323297 ) ) ;
#74236=CARTESIAN_POINT ( 'NONE',  ( 9.692307692308007816, -2.255955759149395501, 30.00000000000324363 ) ) ;
#74238=FACE_BOUND ( 'NONE', #68578, .T. ) ;
#74239=CARTESIAN_POINT ( 'NONE',  ( -15.36145983387954139, -8.191372820521381826, 34.95448215188424967 ) ) ;
#74240=CARTESIAN_POINT ( 'NONE',  ( -6.250023224221457951, -12.45566812827425096, 31.48439005359158926 ) ) ;
#74241=EDGE_CURVE ( 'NONE', #25331, #88566, #23764, .T. ) ;
#74242=CYLINDRICAL_SURFACE ( 'NONE', #65275, 0.2499999999999979738 ) ;
#74243=CARTESIAN_POINT ( 'NONE',  ( -17.87203884117228014, -12.74539040900690701, 29.97526117654243905 ) ) ;
#74244=CYLINDRICAL_SURFACE ( 'NONE', #2971, 0.2500000000000002220 ) ;
#74246=CARTESIAN_POINT ( 'NONE',  ( -39.05038313613820122, -2.249999999999998668, 29.75000000000000355 ) ) ;
#74247=CARTESIAN_POINT ( 'NONE',  ( 11.53846153846141576, -12.51329471203414379, 31.30864560766407578 ) ) ;
#74248=VERTEX_POINT ( 'NONE', #30533 ) ;
#74250=CARTESIAN_POINT ( 'NONE',  ( -7.846153846153965716, -2.625532179533778709, 30.86335684631627174 ) ) ;
#74251=ORIENTED_EDGE ( 'NONE', *, *, #33860, .T. ) ;
#74252=ORIENTED_EDGE ( 'NONE', *, *, #32269, .F. ) ;
#74253=AXIS2_PLACEMENT_3D ( 'NONE', #19580, #82632, #14599 ) ;
#74254=CARTESIAN_POINT ( 'NONE',  ( -17.30040802064703342, -11.41268669641499756, 32.86336882939238535 ) ) ;
#74255=ADVANCED_FACE ( 'NONE', ( #63874 ), #78725, .F. ) ;
#74256=B_SPLINE_CURVE_WITH_KNOTS ( 'NONE', 3,
 ( #50197, #71364, #15996, #84462, #9246, #3804, #63725, #30390, #56966, #10119 ),
 .UNSPECIFIED., .F., .F.,
 ( 4, 2, 2, 2, 4 ),
 ( 0.000000000000000000, 0.0001954339857564075015, 0.0003908679715128150029, 0.0005863019572692224502, 0.0007817359430256300059 ),
 .UNSPECIFIED. ) ;
#74257=CARTESIAN_POINT ( 'NONE',  ( -13.51530598772569469, -4.684245665217972032, 34.18127051446801090 ) ) ;
#74259=ORIENTED_EDGE ( 'NONE', *, *, #760, .F. ) ;
#74261=CARTESIAN_POINT ( 'NONE',  ( 6.699591998512593349, -8.539481045369598178, 34.89627647299170832 ) ) ;
#74262=FACE_BOUND ( 'NONE', #13949, .T. ) ;
#74263=CARTESIAN_POINT ( 'NONE',  ( 16.15384615384615330, -7.500000000000001776, 35.04278698407183867 ) ) ;
#74264=CARTESIAN_POINT ( 'NONE',  ( 5.933917620639865831, -6.343179335718451384, 34.87096338111212646 ) ) ;
#74265=CARTESIAN_POINT ( 'NONE',  ( -8.992156986746914882, -6.503392248772476236, 34.64988816332204635 ) ) ;
#74266=FACE_OUTER_BOUND ( 'NONE', #42701, .T. ) ;
#74267=DIRECTION ( 'NONE',  ( 0.000000000000000000, 0.8660254037844377084, 0.5000000000000015543 ) ) ;
#74269=ORIENTED_EDGE ( 'NONE', *, *, #65556, .F. ) ;
#74272=CARTESIAN_POINT ( 'NONE',  ( 6.988332494352949453, -12.27809138561124591, 31.22303859784720359 ) ) ;
#74273=CARTESIAN_POINT ( 'NONE',  ( 4.403846153846156852, -2.499999999999999112, 29.81604066197450109 ) ) ;
#74274=B_SPLINE_CURVE_WITH_KNOTS ( 'NONE', 3,
 ( #4162, #4619, #67214, #5514, #59108, #86608, #39306, #32092, #19461, #32983 ),
 .UNSPECIFIED., .F., .F.,
 ( 4, 2, 2, 2, 4 ),
 ( 0.0007817246256747511840, 0.0009771112852218952725, 0.001172497944769039470, 0.001367884604316183667, 0.001563271263863327864 ),
 .UNSPECIFIED. ) ;
#74275=CARTESIAN_POINT ( 'NONE',  ( 6.923076923076924238, -12.10708131394839349, 31.69288490824020244 ) ) ;
#74276=DIRECTION ( 'NONE',  ( -0.000000000000000000, -0.9396926207859093161, -0.3420201433256663259 ) ) ;
#74278=B_SPLINE_CURVE_WITH_KNOTS ( 'NONE', 3,
 ( #81759, #80434, #18729, #20050, #41214, #47510, #68240, #6541, #33574, #34001 ),
 .UNSPECIFIED., .F., .F.,
 ( 4, 2, 2, 2, 4 ),
 ( 0.000000000000000000, 0.0001954311564186875792, 0.0003908623128373751583, 0.0005862934692560627103, 0.0007817246256747503166 ),
 .UNSPECIFIED. ) ;
#74279=DIRECTION ( 'NONE',  ( -0.000000000000000000, -0.7660444431189791237, -0.6427876096865379196 ) ) ;
#74281=ADVANCED_FACE ( 'NONE', ( #17022 ), #52130, .F. ) ;
#74282=DIRECTION ( 'NONE',  ( 0.000000000000000000, 0.8660254037844377084, -0.5000000000000015543 ) ) ;
#74283=CARTESIAN_POINT ( 'NONE',  ( 13.13459216039393240, -10.18141759479407327, 34.26406193332782379 ) ) ;
#74284=CARTESIAN_POINT ( 'NONE',  ( -9.692307692307812417, -11.48612834414049644, 32.76840700105863391 ) ) ;
#74285=CARTESIAN_POINT ( 'NONE',  ( 5.076923076923075762, -10.67929555188718282, 33.92786785259544047 ) ) ;
#74286=CARTESIAN_POINT ( 'NONE',  ( 7.053602361310568725, -3.625058011473227815, 33.29252011169590020 ) ) ;
#74287=AXIS2_PLACEMENT_3D ( 'NONE', #83939, #77608, #22222 ) ;
#74288=CARTESIAN_POINT ( 'NONE',  ( -3.296039676730006196, -8.613356846314824011, 34.62446782046655613 ) ) ;
#74289=CARTESIAN_POINT ( 'NONE',  ( -15.48079246806219267, -8.432397168068783699, 34.66272746175022945 ) ) ;
#74290=VERTEX_POINT ( 'NONE', #22886 ) ;
#74291=LINE ( 'NONE', #5831, #19731 ) ;
#74292=DIRECTION ( 'NONE',  ( -0.000000000000000000, -0.000000000000000000, -1.000000000000000000 ) ) ;
#74294=CYLINDRICAL_SURFACE ( 'NONE', #70542, 0.2499999999999986955 ) ;
#74295=DIRECTION ( 'NONE',  ( -0.000000000000000000, -0.9396926207859093161, -0.3420201433256663259 ) ) ;
#74296=CYLINDRICAL_SURFACE ( 'NONE', #68659, 0.2500000000000008882 ) ;
#74297=DIRECTION ( 'NONE',  ( -0.000000000000000000, 0.7660444431189791237, -0.6427876096865379196 ) ) ;
#74298=ORIENTED_EDGE ( 'NONE', *, *, #67545, .F. ) ;
#74300=EDGE_CURVE ( 'NONE', #17248, #67353, #79618, .T. ) ;
#74301=LINE ( 'NONE', #5843, #16751 ) ;
#74303=ADVANCED_FACE ( 'NONE', ( #64749 ), #85485, .F. ) ;
#74304=VERTEX_POINT ( 'NONE', #3498 ) ;
#74306=CARTESIAN_POINT ( 'NONE',  ( -2.241623956689867470, -2.538708090699994813, 30.37095296980875503 ) ) ;
#74307=ORIENTED_EDGE ( 'NONE', *, *, #38518, .F. ) ;
#74308=CARTESIAN_POINT ( 'NONE',  ( 3.100621261037534548, -5.070767119584671967, 34.40440758774516183 ) ) ;
#74310=EDGE_CURVE ( 'NONE', #76471, #86342, #77855, .T. ) ;
#74311=LINE ( 'NONE', #12612, #70033 ) ;
#74312=VERTEX_POINT ( 'NONE', #50785 ) ;
#74313=ORIENTED_EDGE ( 'NONE', *, *, #48574, .F. ) ;
#74314=VERTEX_POINT ( 'NONE', #84613 ) ;
#74316=DIRECTION ( 'NONE',  ( -0.000000000000000000, 0.6427876096865404731, -0.7660444431189771253 ) ) ;
#74317=B_SPLINE_CURVE_WITH_KNOTS ( 'NONE', 3,
 ( #88819, #25765, #46480, #67, #68090, #13577, #41057, #73959, #53676, #53225 ),
 .UNSPECIFIED., .F., .F.,
 ( 4, 2, 2, 2, 4 ),
 ( 0.000000000000000000, 0.0001954339857564079623, 0.0003908679715128159245, 0.0005863019572692238597, 0.0007817359430256318490 ),
 .UNSPECIFIED. ) ;
#74318=AXIS2_PLACEMENT_3D ( 'NONE', #14473, #48248, #21673 ) ;
#74319=CARTESIAN_POINT ( 'NONE',  ( -9.692307692307691624, -9.780366693483667717, 34.19971097300155094 ) ) ;
#74320=CARTESIAN_POINT ( 'NONE',  ( -1.634592128663974631, -11.47974371597208076, 33.17467449705390692 ) ) ;
#74321=CARTESIAN_POINT ( 'NONE',  ( -10.83831157429145975, -11.98009711892699514, 32.48740034544076138 ) ) ;
#74322=CARTESIAN_POINT ( 'NONE',  ( 7.146089767170319185, -8.282913670948747864, 34.94150082978203642 ) ) ;
#74324=VECTOR ( 'NONE', #2284, 1000.000000000000227 ) ;
#74325=CARTESIAN_POINT ( 'NONE',  ( 10.55011416942384450, -12.27809138561121394, 31.22303859784730307 ) ) ;
#74326=EDGE_CURVE ( 'NONE', #82738, #36760, #49937, .T. ) ;
#74327=ORIENTED_EDGE ( 'NONE', *, *, #41781, .F. ) ;
#74328=ORIENTED_EDGE ( 'NONE', *, *, #56925, .F. ) ;
#74329=VECTOR ( 'NONE', #53544, 1000.000000000000000 ) ;
#74330=ORIENTED_EDGE ( 'NONE', *, *, #57479, .T. ) ;
#74331=CARTESIAN_POINT ( 'NONE',  ( -17.29984929443921970, -9.886141570436013382, 34.14413921362392301 ) ) ;
#74332=ORIENTED_EDGE ( 'NONE', *, *, #71750, .F. ) ;
#74333=B_SPLINE_CURVE_WITH_KNOTS ( 'NONE', 3,
 ( #19667, #67857, #6158, #88602, #47579, #34069, #9271, #23654, #76382, #16460 ),
 .UNSPECIFIED., .F., .F.,
 ( 4, 2, 2, 2, 4 ),
 ( 0.000000000000000000, 0.0001954311564186875792, 0.0003908623128373751583, 0.0005862934692560627103, 0.0007817246256747503166 ),
 .UNSPECIFIED. ) ;
#74334=DIRECTION ( 'NONE',  ( 0.000000000000000000, 0.4999999999999985567, 0.8660254037844395958 ) ) ;
#74335=CARTESIAN_POINT ( 'NONE',  ( 9.562160482869472844, -5.195881422630166391, 34.18770438780619259 ) ) ;
#74336=EDGE_LOOP ( 'NONE', ( #69331, #82035, #62400, #48089 ) ) ;
#74337=CARTESIAN_POINT ( 'NONE',  ( -12.21159305216042057, -11.56426240980093745, 33.07394671870546432 ) ) ;
#74338=EDGE_LOOP ( 'NONE', ( #74186, #40111 ) ) ;
#74339=CARTESIAN_POINT ( 'NONE',  ( 14.30769230769218581, -9.528491918059723176, 34.59228464037033035 ) ) ;
#74341=DIRECTION ( 'NONE',  ( -0.000000000000000000, -0.5000000000000009992, -0.8660254037844380415 ) ) ;
#74343=B_SPLINE_CURVE_WITH_KNOTS ( 'NONE', 3,
 ( #29635, #41824, #84149, #55762, #14794, #42270, #49890, #57092, #15678, #43145 ),
 .UNSPECIFIED., .F., .F.,
 ( 4, 2, 2, 2, 4 ),
 ( 0.0007817246256747447872, 0.0009771112852218876831, 0.001172497944769030579, 0.001367884604316173475, 0.001563271263863316371 ),
 .UNSPECIFIED. ) ;
#74344=CARTESIAN_POINT ( 'NONE',  ( -0.4615384615385840772, -5.941354392335915335, 34.76329471203413846 ) ) ;
#74346=AXIS2_PLACEMENT_3D ( 'NONE', #80865, #25903, #67338 ) ;
#74347=FACE_BOUND ( 'NONE', #78974, .T. ) ;
#74348=B_SPLINE_CURVE_WITH_KNOTS ( 'NONE', 3,
 ( #48633, #70243, #61702, #63024, #22061, #15308, #27932, #21, #28367, #27489 ),
 .UNSPECIFIED., .F., .F.,
 ( 4, 2, 2, 2, 4 ),
 ( 0.000000000000000000, 0.0001954311564186876334, 0.0003908623128373752667, 0.0005862934692560629272, 0.0007817246256747505334 ),
 .UNSPECIFIED. ) ;
#74349=DIRECTION ( 'NONE',  ( -0.000000000000000000, -0.000000000000000000, -1.000000000000000000 ) ) ;
#74350=CARTESIAN_POINT ( 'NONE',  ( 16.15384615384603251, -3.643525952248796163, 33.31231777344771672 ) ) ;
#74352=CARTESIAN_POINT ( 'NONE',  ( 10.55011461482829738, -10.33852847137145048, 34.16647553114627556 ) ) ;
#74353=CARTESIAN_POINT ( 'NONE',  ( 10.83881157724618660, -7.630147231320743018, 34.74852402298682819 ) ) ;
#74354=CARTESIAN_POINT ( 'NONE',  ( -8.096130590202436750, -9.234221910056348293, 34.70572697212741531 ) ) ;
#74355=CIRCLE ( 'NONE', #77233, 5.000000000000000888 ) ;
#74356=CARTESIAN_POINT ( 'NONE',  ( -11.66860950819323328, -3.625366637846544116, 33.29286588640298561 ) ) ;
#74357=ORIENTED_EDGE ( 'NONE', *, *, #6097, .T. ) ;
#74358=ORIENTED_EDGE ( 'NONE', *, *, #52535, .F. ) ;
#74359=CARTESIAN_POINT ( 'NONE',  ( 2.057669083470851756, -2.985938066672154445, 32.43141759479405550 ) ) ;
#74360=CARTESIAN_POINT ( 'NONE',  ( -14.24162395668986747, -12.37446782046654192, 30.86335684631486842 ) ) ;
#74361=CARTESIAN_POINT ( 'NONE',  ( 15.48071464014727283, -8.476813868363244353, 34.90874843262270133 ) ) ;
#74362=CARTESIAN_POINT ( 'NONE',  ( -14.43784027742400156, -12.15440758774515473, 32.17923288041532004 ) ) ;
#74363=CARTESIAN_POINT ( 'NONE',  ( 16.85343813319912698, -8.496056993536548418, 34.65000542017679663 ) ) ;
#74364=LINE ( 'NONE', #79791, #31799 ) ;
#74366=CARTESIAN_POINT ( 'NONE',  ( 4.153846153846030731, -6.835583212225970762, 34.95778746994575670 ) ) ;
#74367=CARTESIAN_POINT ( 'NONE',  ( 0.7115927731767762721, -9.943054286541400444, 34.11300777759954883 ) ) ;
#74368=CARTESIAN_POINT ( 'NONE',  ( 17.07692307692295586, -4.320704448113951379, 33.92786785259630022 ) ) ;
#74369=CARTESIAN_POINT ( 'NONE',  ( -3.360917200500928015, -12.70455904226513866, 30.44083106164009322 ) ) ;
#74370=EDGE_LOOP ( 'NONE', ( #55922, #29867 ) ) ;
#74371=ORIENTED_EDGE ( 'NONE', *, *, #46220, .T. ) ;
#74373=ORIENTED_EDGE ( 'NONE', *, *, #58527, .F. ) ;
#74374=AXIS2_PLACEMENT_3D ( 'NONE', #59566, #65870, #66772 ) ;
#74375=CARTESIAN_POINT ( 'NONE',  ( 0.4615384615384611755, -13.57706302396349152, 30.56769352161908060 ) ) ;
#74376=ORIENTED_EDGE ( 'NONE', *, *, #46868, .F. ) ;
#74377=CARTESIAN_POINT ( 'NONE',  ( -16.15384615384627409, -5.219633306517616589, 34.19971097300220464 ) ) ;
#74378=CARTESIAN_POINT ( 'NONE',  ( -6.223484924564328225, -9.417330523894424488, 34.63758898049880486 ) ) ;
#74379=CARTESIAN_POINT ( 'NONE',  ( 3.296836564119306257, -9.905515769479277921, 34.41647553114623292 ) ) ;
#74382=VERTEX_POINT ( 'NONE', #58893 ) ;
#74383=B_SPLINE_CURVE_WITH_KNOTS ( 'NONE', 3,
 ( #225, #33576, #81761, #40778, #75881, #663, #47958, #55603, #40332, #33123 ),
 .UNSPECIFIED., .F., .F.,
 ( 4, 2, 2, 2, 4 ),
 ( 0.0007817246256747446788, 0.0009771112852218879000, 0.001172497944769031013, 0.001367884604316174126, 0.001563271263863317238 ),
 .UNSPECIFIED. ) ;
#74384=CARTESIAN_POINT ( 'NONE',  ( -0.2385256174450670896, -11.98016756924214832, 32.48728574198911190 ) ) ;
#74385=ORIENTED_EDGE ( 'NONE', *, *, #18640, .T. ) ;
#74387=CARTESIAN_POINT ( 'NONE',  ( -9.019230769230768274, -7.500000000000001776, 35.00000000000000000 ) ) ;
#74388=CARTESIAN_POINT ( 'NONE',  ( -13.38461538461538325, -4.786620604624113540, 33.94971097300155094 ) ) ;
#74389=CARTESIAN_POINT ( 'NONE',  ( 9.823099500132480344, -10.54018710029568595, 33.71981072465678864 ) ) ;
#74390=CARTESIAN_POINT ( 'NONE',  ( -39.05038313613820122, -12.75000000000000178, 29.75000000000000355 ) ) ;
#74391=VECTOR ( 'NONE', #73854, 1000.000000000000114 ) ;
#74392=CARTESIAN_POINT ( 'NONE',  ( -11.53846153846153655, -1.044019251281081972, 31.83374038241031911 ) ) ;
#74393=CARTESIAN_POINT ( 'NONE',  ( -3.230769230769229949, -6.386643153685126251, 34.62446782046654192 ) ) ;
#74395=EDGE_LOOP ( 'NONE', ( #39353, #62006, #16705, #75905 ) ) ;
#74396=CARTESIAN_POINT ( 'NONE',  ( 0.4615384615383382183, -2.657715359629662544, 31.77849191805970364 ) ) ;
#74397=CARTESIAN_POINT ( 'NONE',  ( 0.4615384615384611200, -8.164416787775445883, 34.95778746994557906 ) ) ;
#74398=EDGE_CURVE ( 'NONE', #28383, #47782, #37010, .T. ) ;
#74400=EDGE_LOOP ( 'NONE', ( #47844, #17227, #6151, #86674 ) ) ;
#74401=CARTESIAN_POINT ( 'NONE',  ( -16.40384615384615330, -7.500000000000001776, 35.00000000000000000 ) ) ;
#74402=CARTESIAN_POINT ( 'NONE',  ( 11.28848479441294828, -12.65889640711025521, 30.72598325615533454 ) ) ;
#74403=EDGE_CURVE ( 'NONE', #83400, #15837, #48827, .T. ) ;
#74404=CARTESIAN_POINT ( 'NONE',  ( -10.74607521849492642, -2.295517848115769421, 30.44137282052137294 ) ) ;
#74405=CARTESIAN_POINT ( 'NONE',  ( 7.053602624840487501, -6.001044277235011215, 34.52024696741798948 ) ) ;
#74408=AXIS2_PLACEMENT_3D ( 'NONE', #42356, #8119, #69811 ) ;
#74409=CARTESIAN_POINT ( 'NONE',  ( 9.442284455014730682, -10.76384336483936011, 33.53834819971076087 ) ) ;
#74410=EDGE_CURVE ( 'NONE', #51516, #8808, #509, .T. ) ;
#74411=CYLINDRICAL_SURFACE ( 'NONE', #84400, 0.2499999999999998890 ) ;
#74412=CARTESIAN_POINT ( 'NONE',  ( -2.241624974342230736, -5.471508081941601098, 34.59228464037088457 ) ) ;
#74413=ORIENTED_EDGE ( 'NONE', *, *, #25088, .T. ) ;
#74414=CARTESIAN_POINT ( 'NONE',  ( 17.07692307692307665, -13.53365097954675988, 30.81389545987213552 ) ) ;
#74415=ORIENTED_EDGE ( 'NONE', *, *, #18474, .F. ) ;
#74416=CARTESIAN_POINT ( 'NONE',  ( 6.923076923076924238, -5.180354513474913603, 36.12317359536750416 ) ) ;
#74418=DIRECTION ( 'NONE',  ( -0.000000000000000000, 0.7660444431189791237, -0.6427876096865379196 ) ) ;
#74419=ORIENTED_EDGE ( 'NONE', *, *, #49160, .T. ) ;
#74420=FACE_OUTER_BOUND ( 'NONE', #17046, .T. ) ;
#74421=DIRECTION ( 'NONE',  ( 0.000000000000000000, 0.9396926207859126468, 0.3420201433256571111 ) ) ;
#74422=DIRECTION ( 'NONE',  ( 1.000000000000000000, 0.000000000000000000, 0.000000000000000000 ) ) ;
#74423=CARTESIAN_POINT ( 'NONE',  ( -8.096130590202436750, -4.818429247618089661, 34.26397095200675125 ) ) ;
#74424=CARTESIAN_POINT ( 'NONE',  ( -1.450697763975519416, -10.67929555188718460, 33.92786785259543336 ) ) ;
#74425=EDGE_CURVE ( 'NONE', #55155, #23906, #74192, .T. ) ;
#74426=ORIENTED_EDGE ( 'NONE', *, *, #1700, .T. ) ;
#74427=FACE_BOUND ( 'NONE', #73341, .T. ) ;
#74428=EDGE_CURVE ( 'NONE', #69764, #86769, #53131, .T. ) ;
#74429=ORIENTED_EDGE ( 'NONE', *, *, #16276, .F. ) ;
#74430=CARTESIAN_POINT ( 'NONE',  ( -1.384615384615383471, -1.422936976036506707, 30.56769352161908415 ) ) ;
#74431=ADVANCED_FACE ( 'NONE', ( #88177 ), #66087, .F. ) ;
#74432=CARTESIAN_POINT ( 'NONE',  ( -18.00000000000000000, -9.815202283848471154, 36.11096599634342397 ) ) ;
#74434=CARTESIAN_POINT ( 'NONE',  ( 6.066068351002440906, -8.973038597847269315, 34.52809138561122637 ) ) ;
#74435=DIRECTION ( 'NONE',  ( 0.000000000000000000, 0.000000000000000000, 1.000000000000000000 ) ) ;
#74436=CARTESIAN_POINT ( 'NONE',  ( 14.30769230769231015, -8.164416787775445883, 34.95778746994557906 ) ) ;
#74437=B_SPLINE_CURVE_WITH_KNOTS ( 'NONE', 3,
 ( #66188, #10372, #80164, #4498, #66646, #45476, #58534, #52675, #31068, #45918 ),
 .UNSPECIFIED., .F., .F.,
 ( 4, 2, 2, 2, 4 ),
 ( 0.000000000000000000, 0.0001954311564186864949, 0.0003908623128373729899, 0.0005862934692560594577, 0.0007817246256747459798 ),
 .UNSPECIFIED. ) ;
#74438=B_SPLINE_CURVE_WITH_KNOTS ( 'NONE', 3,
 ( #89106, #75559, #56181, #27385, #13860, #55289, #41794, #41342, #28713, #69256 ),
 .UNSPECIFIED., .F., .F.,
 ( 4, 2, 2, 2, 4 ),
 ( 0.0007817359430256293554, 0.0009771253907249952391, 0.001172514838424361123, 0.001367904286123727007, 0.001563293733823092890 ),
 .UNSPECIFIED. ) ;
#74439=ORIENTED_EDGE ( 'NONE', *, *, #9194, .F. ) ;
#74440=ORIENTED_EDGE ( 'NONE', *, *, #69339, .F. ) ;
#74441=EDGE_LOOP ( 'NONE', ( #7604, #23365 ) ) ;
#74443=ORIENTED_EDGE ( 'NONE', *, *, #38199, .T. ) ;
#74445=CARTESIAN_POINT ( 'NONE',  ( 4.153846153846154188, -9.905515769479276145, 34.41647553114623292 ) ) ;
#74446=CARTESIAN_POINT ( 'NONE',  ( -3.903900635498011251, -9.272278438253401589, 34.42582936511637826 ) ) ;
#74447=CARTESIAN_POINT ( 'NONE',  ( 4.826946332874485712, -11.47974371597207899, 33.17467449705390692 ) ) ;
#74448=CARTESIAN_POINT ( 'NONE',  ( 3.230769230769108269, -9.528491918059723176, 34.59228464037033035 ) ) ;
#74449=CARTESIAN_POINT ( 'NONE',  ( -5.207614543590636025, -8.147922237126337563, 34.70805685702651999 ) ) ;
#74450=CARTESIAN_POINT ( 'NONE',  ( -4.826868765284762830, -4.235687564193446164, 33.53795663066793509 ) ) ;
#74451=CARTESIAN_POINT ( 'NONE',  ( 11.31497659473759043, -10.11188796281391511, 34.01382737946119050 ) ) ;
#74452=VERTEX_POINT ( 'NONE', #5289 ) ;
#74453=ORIENTED_EDGE ( 'NONE', *, *, #50155, .T. ) ;
#74454=ORIENTED_EDGE ( 'NONE', *, *, #19278, .T. ) ;
#74456=EDGE_LOOP ( 'NONE', ( #3229, #53477 ) ) ;
#74457=CARTESIAN_POINT ( 'NONE',  ( -1.384615384615506484, -2.657715359629662544, 31.77849191805970364 ) ) ;
#74458=CARTESIAN_POINT ( 'NONE',  ( -9.822998295418001291, -3.957541250942358424, 33.62499894934981626 ) ) ;
#74459=EDGE_CURVE ( 'NONE', #76451, #27137, #26452, .T. ) ;
#74460=CARTESIAN_POINT ( 'NONE',  ( -16.15384615384615330, -10.89733346790207413, 36.13435417666054406 ) ) ;
#74461=AXIS2_PLACEMENT_3D ( 'NONE', #33051, #60518, #57306 ) ;
#74462=CARTESIAN_POINT ( 'NONE',  ( -15.23076923076922995, -9.905515769479276145, 34.41647553114623292 ) ) ;
#74463=FACE_BOUND ( 'NONE', #74821, .T. ) ;
#74464=ORIENTED_EDGE ( 'NONE', *, *, #78056, .T. ) ;
#74465=DIRECTION ( 'NONE',  ( -0.000000000000000000, -0.5000000000000009992, -0.8660254037844380415 ) ) ;
#74466=EDGE_LOOP ( 'NONE', ( #63116, #40805 ) ) ;
#74467=CARTESIAN_POINT ( 'NONE',  ( 17.14217821643591932, -5.941354392334603496, 34.76329471203374055 ) ) ;
#74468=B_SPLINE_CURVE_WITH_KNOTS ( 'NONE', 3,
 ( #12838, #47056, #11516, #11067, #26358, #40322, #38997, #86300, #32230, #87191 ),
 .UNSPECIFIED., .F., .F.,
 ( 4, 2, 2, 2, 4 ),
 ( 0.0007817246256747491240, 0.0009771112852218931041, 0.001172497944769036867, 0.001367884604316180631, 0.001563271263863324611 ),
 .UNSPECIFIED. ) ;
#74469=CIRCLE ( 'NONE', #35650, 0.2500000000000002220 ) ;
#74470=ORIENTED_EDGE ( 'NONE', *, *, #71320, .F. ) ;
#74471=FACE_BOUND ( 'NONE', #4776, .T. ) ;
#74472=CARTESIAN_POINT ( 'NONE',  ( 9.915087361285760181, -5.827830569534417471, 34.72679350104403539 ) ) ;
#74473=CARTESIAN_POINT ( 'NONE',  ( 15.16549923021291058, -6.835583212224499938, 34.95778746994557906 ) ) ;
#74474=EDGE_LOOP ( 'NONE', ( #28807, #21804 ) ) ;
#74475=LINE ( 'NONE', #14103, #62166 ) ;
#74476=CYLINDRICAL_SURFACE ( 'NONE', #4483, 0.2499999999999994726 ) ;
#74477=VECTOR ( 'NONE', #76404, 1000.000000000000227 ) ;
#74478=CARTESIAN_POINT ( 'NONE',  ( 15.23076923076911093, -8.613356846316285953, 34.62446782046622218 ) ) ;
#74479=ORIENTED_EDGE ( 'NONE', *, *, #2176, .T. ) ;
#74480=CARTESIAN_POINT ( 'NONE',  ( -8.546451100252699717, -3.563462043263030399, 33.22394488606062879 ) ) ;
#74481=CARTESIAN_POINT ( 'NONE',  ( -5.076923076923075762, -8.564572088678739092, 35.78748833219616898 ) ) ;
#74482=CARTESIAN_POINT ( 'NONE',  ( -3.480792468062195777, -2.823816976329320827, 31.52131813110797154 ) ) ;
#74483=DIRECTION ( 'NONE',  ( -0.000000000000000000, -0.5000000000000009992, -0.8660254037844380415 ) ) ;
#74484=EDGE_LOOP ( 'NONE', ( #59115, #6536, #26691, #22037 ) ) ;
#74485=ADVANCED_FACE ( 'NONE', ( #6178 ), #25112, .F. ) ;
#74486=FACE_OUTER_BOUND ( 'NONE', #85785, .T. ) ;
#74487=CARTESIAN_POINT ( 'NONE',  ( -16.02305571287920571, -9.929761469519743144, 34.40412654351204225 ) ) ;
#74488=ORIENTED_EDGE ( 'NONE', *, *, #4741, .F. ) ;
#74489=CARTESIAN_POINT ( 'NONE',  ( 0.3313912521002400635, -9.418419913701741919, 34.36755862841477693 ) ) ;
#74490=CARTESIAN_POINT ( 'NONE',  ( 9.915270826574369423, -7.369474539155828730, 34.99858011523957657 ) ) ;
#74491=DIRECTION ( 'NONE',  ( -0.000000000000000000, -0.000000000000000000, -1.000000000000000000 ) ) ;
#74492=CARTESIAN_POINT ( 'NONE',  ( -5.076923076923075762, -13.63283147151868846, 33.57946703557072254 ) ) ;
#74493=CARTESIAN_POINT ( 'NONE',  ( -7.145905020711801114, -7.369209533119140509, 34.99857337881830688 ) ) ;
#74494=CARTESIAN_POINT ( 'NONE',  ( 17.01084069756293715, -4.661471528628507777, 34.16647553114621871 ) ) ;
#74496=CARTESIAN_POINT ( 'NONE',  ( 16.28463796167094557, -5.582136614379148654, 34.36778462344220486 ) ) ;
#74497=CARTESIAN_POINT ( 'NONE',  ( -12.21148414990014963, -11.28795663066794575, 33.01431243580653785 ) ) ;
#74499=ORIENTED_EDGE ( 'NONE', *, *, #74843, .T. ) ;
#74500=B_SPLINE_CURVE_WITH_KNOTS ( 'NONE', 3,
 ( #2906, #79027, #4258, #51085, #17785, #17329, #30396, #54096, #37591, #78578 ),
 .UNSPECIFIED., .F., .F.,
 ( 4, 2, 2, 2, 4 ),
 ( 0.000000000000000000, 0.0001954311584214072381, 0.0003908623168428144762, 0.0005862934752642217414, 0.0007817246336856289524 ),
 .UNSPECIFIED. ) ;
#74501=LINE ( 'NONE', #59204, #10171 ) ;
#74502=ORIENTED_EDGE ( 'NONE', *, *, #24364, .F. ) ;
#74503=ADVANCED_FACE ( 'NONE', ( #61112 ), #26891, .F. ) ;
#74504=AXIS2_PLACEMENT_3D ( 'NONE', #23072, #87346, #25621 ) ;
#74505=VERTEX_POINT ( 'NONE', #60223 ) ;
#74506=CARTESIAN_POINT ( 'NONE',  ( -8.638705330997126453, -6.808710257144161559, 34.95449254468098843 ) ) ;
#74508=CARTESIAN_POINT ( 'NONE',  ( 15.23076923076923173, -7.500000000000001776, 35.04278698407183867 ) ) ;
#74510=CARTESIAN_POINT ( 'NONE',  ( -14.08491263871423982, -3.020022701398813236, 32.48759521482552515 ) ) ;
#74511=EDGE_CURVE ( 'NONE', #58033, #70825, #16591, .T. ) ;
#74512=CARTESIAN_POINT ( 'NONE',  ( 6.923076923076924238, -9.905515769479276145, 34.41647553114623292 ) ) ;
#74513=CARTESIAN_POINT ( 'NONE',  ( -3.100243529005665799, -9.417988943895561960, 34.36773134775778260 ) ) ;
#74514=CYLINDRICAL_SURFACE ( 'NONE', #79188, 0.2499999999999979738 ) ;
#74515=CARTESIAN_POINT ( 'NONE',  ( 10.86538461538603606, -7.500000000000154543, 35.00000000000007105 ) ) ;
#74517=CARTESIAN_POINT ( 'NONE',  ( 6.792386319966619013, -12.35290016733513951, 31.75349464988449455 ) ) ;
#74518=CARTESIAN_POINT ( 'NONE',  ( 11.53846153846153832, -8.564572088678739092, 35.78748833219616898 ) ) ;
#74519=CARTESIAN_POINT ( 'NONE',  ( -10.39200912961219458, -2.251407671071268712, 29.88021292934943318 ) ) ;
#74521=EDGE_CURVE ( 'NONE', #4115, #57358, #34532, .T. ) ;
#74522=CARTESIAN_POINT ( 'NONE',  ( 18.22337594069818323, -2.501478030877322567, 29.88021232661721172 ) ) ;
#74523=B_SPLINE_CURVE_WITH_KNOTS ( 'NONE', 3,
 ( #42890, #36997, #29380, #83884, #42445, #70805, #22602, #78430, #43761, #22171 ),
 .UNSPECIFIED., .F., .F.,
 ( 4, 2, 2, 2, 4 ),
 ( 0.0007817246256747450040, 0.0009771112852218876831, 0.001172497944769030579, 0.001367884604316173258, 0.001563271263863315937 ),
 .UNSPECIFIED. ) ;
#74524=EDGE_CURVE ( 'NONE', #21466, #5024, #7045, .T. ) ;
#74525=EDGE_LOOP ( 'NONE', ( #175, #46183 ) ) ;
#74526=EDGE_LOOP ( 'NONE', ( #222, #66543, #53827, #56922 ) ) ;
#74527=CARTESIAN_POINT ( 'NONE',  ( 14.24242230713598900, -8.656820664281498878, 34.87096338111211935 ) ) ;
#74528=FACE_OUTER_BOUND ( 'NONE', #11393, .T. ) ;
#74530=CARTESIAN_POINT ( 'NONE',  ( -7.146003881983771677, -5.582147617184174848, 34.63737895849758530 ) ) ;
#74531=ADVANCED_FACE ( 'NONE', ( #76402 ), #304, .F. ) ;
#74533=DIRECTION ( 'NONE',  ( 0.000000000000000000, -0.000000000000000000, 1.000000000000000000 ) ) ;
#74534=CARTESIAN_POINT ( 'NONE',  ( -9.692307692307691624, -4.945431358278436385, 36.03766855953609394 ) ) ;
#74535=ADVANCED_FACE ( 'NONE', ( #75962 ), #69205, .F. ) ;
#74536=EDGE_LOOP ( 'NONE', ( #31372, #74499, #7966, #62304 ) ) ;
#74537=CARTESIAN_POINT ( 'NONE',  ( 2.980746006547774218, -6.652501968072646932, 34.93155406624980941 ) ) ;
#74538=EDGE_LOOP ( 'NONE', ( #26957, #26365, #21468, #10083 ) ) ;
#74540=ORIENTED_EDGE ( 'NONE', *, *, #57133, .T. ) ;
#74541=CARTESIAN_POINT ( 'NONE',  ( 16.37685899793954292, -9.172514111537580561, 34.72667873470787470 ) ) ;
#74542=LINE ( 'NONE', #40320, #16797 ) ;
#74543=EDGE_CURVE ( 'NONE', #15407, #6007, #46760, .T. ) ;
#74544=DIRECTION ( 'NONE',  ( 0.000000000000000000, 0.000000000000000000, 1.000000000000000000 ) ) ;
#74545=EDGE_CURVE ( 'NONE', #65338, #20445, #75788, .T. ) ;
#74547=DIRECTION ( 'NONE',  ( -0.000000000000000000, 1.000000000000000000, -0.000000000000000000 ) ) ;
#74548=CARTESIAN_POINT ( 'NONE',  ( 12.46153846153846168, -12.10708131394839349, 31.69288490824020244 ) ) ;
#74549=ORIENTED_EDGE ( 'NONE', *, *, #1946, .T. ) ;
#74550=ORIENTED_EDGE ( 'NONE', *, *, #83336, .F. ) ;
#74551=B_SPLINE_CURVE_WITH_KNOTS ( 'NONE', 3,
 ( #31957, #58513, #52209, #30175, #23836, #85125, #86008, #72935, #44552, #45454 ),
 .UNSPECIFIED., .F., .F.,
 ( 4, 2, 2, 2, 4 ),
 ( 0.0007817359430256294638, 0.0009771253907249941549, 0.001172514838424358954, 0.001367904286123723754, 0.001563293733823095492 ),
 .UNSPECIFIED. ) ;
#74552=ORIENTED_EDGE ( 'NONE', *, *, #52820, .F. ) ;
#74553=ORIENTED_EDGE ( 'NONE', *, *, #69022, .T. ) ;
#74554=CARTESIAN_POINT ( 'NONE',  ( -2.307692307692305711, -1.242168528481310874, 33.36296068462461051 ) ) ;
#74555=CARTESIAN_POINT ( 'NONE',  ( -2.307692307692428724, -10.33852847137269571, 34.16647553114546554 ) ) ;
#74557=CARTESIAN_POINT ( 'NONE',  ( 14.53111870660709748, -7.630147987733840509, 34.99859428049665411 ) ) ;
#74559=ADVANCED_FACE ( 'NONE', ( #83623 ), #75085, .F. ) ;
#74560=CARTESIAN_POINT ( 'NONE',  ( 17.77651505627605033, -5.113361153441931428, 34.14387501736621999 ) ) ;
#74561=CARTESIAN_POINT ( 'NONE',  ( -10.61538461538473399, -12.27809138561165270, 31.22303859784587132 ) ) ;
#74562=ORIENTED_EDGE ( 'NONE', *, *, #42770, .T. ) ;
#74563=VERTEX_POINT ( 'NONE', #21902 ) ;
#74564=ORIENTED_EDGE ( 'NONE', *, *, #13075, .T. ) ;
#74566=CARTESIAN_POINT ( 'NONE',  ( -10.36533030374629938, -11.79725096376909299, 32.30694842903960762 ) ) ;
#74567=VERTEX_POINT ( 'NONE', #49375 ) ;
#74568=DIRECTION ( 'NONE',  ( 0.000000000000000000, 0.9396926207859126468, 0.3420201433256571111 ) ) ;
#74569=CARTESIAN_POINT ( 'NONE',  ( -12.39628332202562433, -12.16647553114626490, 32.15551576947920864 ) ) ;
#74570=VECTOR ( 'NONE', #78801, 1000.000000000000114 ) ;
#74571=EDGE_CURVE ( 'NONE', #73158, #35045, #89055, .T. ) ;
#74573=ORIENTED_EDGE ( 'NONE', *, *, #44864, .T. ) ;
#74575=CARTESIAN_POINT ( 'NONE',  ( 7.976944287120798727, -3.957578996910242619, 33.62503395064540257 ) ) ;
#74576=VERTEX_POINT ( 'NONE', #48034 ) ;
#74577=EDGE_CURVE ( 'NONE', #18726, #74998, #57896, .T. ) ;
#74578=CARTESIAN_POINT ( 'NONE',  ( 2.057715576749955311, -6.567427716900047230, 34.66269422305636283 ) ) ;
#74579=FACE_BOUND ( 'NONE', #35352, .T. ) ;
#74581=EDGE_CURVE ( 'NONE', #64872, #12730, #67198, .T. ) ;
#74583=ORIENTED_EDGE ( 'NONE', *, *, #51268, .T. ) ;
#74584=CARTESIAN_POINT ( 'NONE',  ( -5.076923076923197442, -12.46129190930018460, 30.37095296980731973 ) ) ;
#74586=DIRECTION ( 'NONE',  ( -0.000000000000000000, -0.8660254037844397068, -0.4999999999999978906 ) ) ;
#74587=ORIENTED_EDGE ( 'NONE', *, *, #7546, .F. ) ;
#74588=EDGE_CURVE ( 'NONE', #60815, #23052, #87624, .T. ) ;
#74589=CARTESIAN_POINT ( 'NONE',  ( -11.53846153846153655, -2.486705287966279876, 31.30864560766543647 ) ) ;
#74590=LINE ( 'NONE', #48428, #69897 ) ;
#74591=CARTESIAN_POINT ( 'NONE',  ( -3.903791733932699959, -2.318338780012835443, 30.59689888758630261 ) ) ;
#74592=B_SPLINE_CURVE_WITH_KNOTS ( 'NONE', 3,
 ( #28536, #83488, #21770, #15021, #42495, #8268, #35740, #63191, #81710, #19994 ),
 .UNSPECIFIED., .F., .F.,
 ( 4, 2, 2, 2, 4 ),
 ( 0.000000000000000000, 0.0001954311564186878502, 0.0003908623128373757004, 0.0005862934692560635777, 0.0007817246256747514008 ),
 .UNSPECIFIED. ) ;
#74593=CARTESIAN_POINT ( 'NONE',  ( 6.000000000000001776, -13.37000171582298513, 34.34916445242398453 ) ) ;
#74594=CARTESIAN_POINT ( 'NONE',  ( 7.911409417429871027, -3.300289026998475705, 32.46337939537591666 ) ) ;
#74595=FACE_BOUND ( 'NONE', #31936, .T. ) ;
#74597=CARTESIAN_POINT ( 'NONE',  ( 14.98076923076923173, -7.500000000000001776, 35.04278698407183867 ) ) ;
#74598=CARTESIAN_POINT ( 'NONE',  ( -14.98082382139119062, -4.932303261841489928, 34.32971442181322885 ) ) ;
#74599=CARTESIAN_POINT ( 'NONE',  ( -5.750054481651858396, -10.05730279482229683, 34.04704008940765902 ) ) ;
#74600=CARTESIAN_POINT ( 'NONE',  ( 17.93472955403922242, -11.48612834413959582, 32.76840700105983473 ) ) ;
#74601=CARTESIAN_POINT ( 'NONE',  ( 5.999999999999878320, -5.094484230521993062, 34.41647553114689373 ) ) ;
#74603=ORIENTED_EDGE ( 'NONE', *, *, #886, .F. ) ;
#74604=CARTESIAN_POINT ( 'NONE',  ( -12.23857532727178921, -7.369474539155828730, 34.99858011523957657 ) ) ;
#74605=ORIENTED_EDGE ( 'NONE', *, *, #47569, .F. ) ;
#74606=CARTESIAN_POINT ( 'NONE',  ( -18.06527000055631760, -3.643525952247788524, 33.31231777344662248 ) ) ;
#74607=ORIENTED_EDGE ( 'NONE', *, *, #67586, .T. ) ;
#74608=CARTESIAN_POINT ( 'NONE',  ( 16.37662582282421653, -12.69155399931963046, 30.53255429739158444 ) ) ;
#74610=DIRECTION ( 'NONE',  ( -0.000000000000000000, -0.8660254037844399289, -0.4999999999999980016 ) ) ;
#74611=ORIENTED_EDGE ( 'NONE', *, *, #2001, .F. ) ;
#74612=CARTESIAN_POINT ( 'NONE',  ( 16.82694633287449193, -12.65889640711025521, 30.72598325615533454 ) ) ;
#74613=DIRECTION ( 'NONE',  ( -0.000000000000000000, 0.5000000000000011102, -0.8660254037844381525 ) ) ;
#74616=CARTESIAN_POINT ( 'NONE',  ( -5.076923076923075762, -13.87047571288749737, 32.06866353760679544 ) ) ;
#74617=CYLINDRICAL_SURFACE ( 'NONE', #60446, 0.2500000000000009437 ) ;
#74618=EDGE_CURVE ( 'NONE', #35110, #9301, #69246, .T. ) ;
#74619=LINE ( 'NONE', #60203, #8740 ) ;
#74620=CARTESIAN_POINT ( 'NONE',  ( 3.903869422903798458, -11.79746400365624659, 32.30657167506340954 ) ) ;
#74621=CARTESIAN_POINT ( 'NONE',  ( 2.307692307692309264, -2.721908614388771852, 31.22303859784724978 ) ) ;
#74622=CYLINDRICAL_SURFACE ( 'NONE', #38230, 0.2499999999999986955 ) ;
#74624=DIRECTION ( 'NONE',  ( -0.000000000000000000, -0.000000000000000000, -1.000000000000000000 ) ) ;
#74627=CARTESIAN_POINT ( 'NONE',  ( 7.053124358327376164, -7.723484941389743952, 34.99544897038808955 ) ) ;
#74628=CARTESIAN_POINT ( 'NONE',  ( 15.29602437028207085, -11.06231777344671130, 33.60647404775212976 ) ) ;
#74630=CARTESIAN_POINT ( 'NONE',  ( -5.999999999999998224, -2.292212530054420494, 30.41441678777542634 ) ) ;
#74631=VECTOR ( 'NONE', #32406, 999.9999999999998863 ) ;
#74632=DIRECTION ( 'NONE',  ( 0.000000000000000000, 0.000000000000000000, 1.000000000000000000 ) ) ;
#74635=DIRECTION ( 'NONE',  ( 0.000000000000000000, 0.9848077530122072432, 0.1736481776669354937 ) ) ;
#74636=CARTESIAN_POINT ( 'NONE',  ( 4.153846153846154188, -9.058645607665452459, 34.76329471203371924 ) ) ;
#74637=ORIENTED_EDGE ( 'NONE', *, *, #53826, .F. ) ;
#74638=CARTESIAN_POINT ( 'NONE',  ( 3.903822916553187472, -8.432397168068783699, 34.66272746175022945 ) ) ;
#74639=CARTESIAN_POINT ( 'NONE',  ( -15.23076923076922995, -11.91647553114624181, 32.58852847137148245 ) ) ;
#74640=AXIS2_PLACEMENT_3D ( 'NONE', #46635, #40776, #5647 ) ;
#74641=CARTESIAN_POINT ( 'NONE',  ( -16.02300782335938933, -7.277220318596959281, 34.99547417642776992 ) ) ;
#74642=ORIENTED_EDGE ( 'NONE', *, *, #69554, .F. ) ;
#74643=VECTOR ( 'NONE', #75943, 1000.000000000000114 ) ;
#74644=CARTESIAN_POINT ( 'NONE',  ( 5.076923076922954969, -4.481592998941358097, 33.73612834414048933 ) ) ;
#74645=CARTESIAN_POINT ( 'NONE',  ( -13.60754160213153163, -11.76352882383564769, 32.36236540154569497 ) ) ;
#74646=EDGE_CURVE ( 'NONE', #10442, #30860, #2410, .T. ) ;
#74647=VECTOR ( 'NONE', #64597, 1000.000000000000000 ) ;
#74648=EDGE_CURVE ( 'NONE', #13730, #21910, #9284, .T. ) ;
#74649=CARTESIAN_POINT ( 'NONE',  ( 1.254467414883687848, -3.069018819979302926, 32.56621877034667278 ) ) ;
#74650=EDGE_LOOP ( 'NONE', ( #87754, #37105 ) ) ;
#74651=ORIENTED_EDGE ( 'NONE', *, *, #45283, .F. ) ;
#74653=B_SPLINE_CURVE_WITH_KNOTS ( 'NONE', 3,
 ( #65295, #71604, #45470, #44566, #31970, #30621, #52223, #58094, #38278, #65734 ),
 .UNSPECIFIED., .F., .F.,
 ( 4, 2, 2, 2, 4 ),
 ( 0.0007817359430256262112, 0.0009771253907249911191, 0.001172514838424356136, 0.001367904286123721152, 0.001563293733823086168 ),
 .UNSPECIFIED. ) ;
#74654=EDGE_CURVE ( 'NONE', #64222, #65220, #32712, .T. ) ;
#74655=VERTEX_POINT ( 'NONE', #72299 ) ;
#74656=CARTESIAN_POINT ( 'NONE',  ( 12.68455130563185662, -10.01129605718032600, 34.36064277460058491 ) ) ;
#74657=CARTESIAN_POINT ( 'NONE',  ( -5.076923076923075762, -2.486705287966279876, 31.30864560766543647 ) ) ;
#74659=DIRECTION ( 'NONE',  ( -1.000000000000000000, 0.000000000000000000, 0.000000000000000000 ) ) ;
#74660=CARTESIAN_POINT ( 'NONE',  ( -17.32692307692307665, -7.500000000000001776, 35.00000000000000000 ) ) ;
#74661=EDGE_CURVE ( 'NONE', #70106, #88393, #82188, .T. ) ;
#74662=CARTESIAN_POINT ( 'NONE',  ( 5.326868595271218254, -5.852078868378311149, 34.47109172314383585 ) ) ;
#74663=ORIENTED_EDGE ( 'NONE', *, *, #48742, .F. ) ;
#74664=ORIENTED_EDGE ( 'NONE', *, *, #23950, .T. ) ;
#74665=ORIENTED_EDGE ( 'NONE', *, *, #18518, .T. ) ;
#74666=CARTESIAN_POINT ( 'NONE',  ( 12.46153846153846168, -5.180354513474913603, 36.12317359536750416 ) ) ;
#74668=CARTESIAN_POINT ( 'NONE',  ( 7.846153846153725020, -12.27809138561165270, 31.22303859784587132 ) ) ;
#74669=EDGE_CURVE ( 'NONE', #23762, #75680, #65984, .T. ) ;
#74670=AXIS2_PLACEMENT_3D ( 'NONE', #53646, #13988, #19418 ) ;
#74671=CARTESIAN_POINT ( 'NONE',  ( 5.776515075435670887, -12.69144148231606017, 30.53333754910549303 ) ) ;
#74672=EDGE_CURVE ( 'NONE', #36959, #86943, #39287, .T. ) ;
#74674=CARTESIAN_POINT ( 'NONE',  ( -14.98082371242109012, -9.272278438253398036, 34.42582936511637115 ) ) ;
#74676=ORIENTED_EDGE ( 'NONE', *, *, #73939, .F. ) ;
#74677=ORIENTED_EDGE ( 'NONE', *, *, #64871, .T. ) ;
#74678=CARTESIAN_POINT ( 'NONE',  ( 10.86543892702293412, -10.66356715214248752, 33.62249196103329751 ) ) ;
#74679=CARTESIAN_POINT ( 'NONE',  ( -2.438383774359863310, -2.729777683071816785, 31.24903638046268739 ) ) ;
#74680=ORIENTED_EDGE ( 'NONE', *, *, #65131, .T. ) ;
#74681=CYLINDRICAL_SURFACE ( 'NONE', #41717, 0.2499999999999995559 ) ;
#74683=CARTESIAN_POINT ( 'NONE',  ( -7.846153846153844924, -13.49023893513002648, 31.06009739812518688 ) ) ;
#74684=VERTEX_POINT ( 'NONE', #33550 ) ;
#74685=LINE ( 'NONE', #33692, #43181 ) ;
#74686=DIRECTION ( 'NONE',  ( 0.000000000000000000, -6.938893903907222067E-15, 1.000000000000000000 ) ) ;
#74687=CARTESIAN_POINT ( 'NONE',  ( 13.38461538461538680, -12.78798330534102945, 29.74999999999997868 ) ) ;
#74688=FACE_BOUND ( 'NONE', #77253, .T. ) ;
#74689=EDGE_CURVE ( 'NONE', #76970, #41347, #62856, .T. ) ;
#74690=CARTESIAN_POINT ( 'NONE',  ( 10.61538461538461675, -9.780366693483667717, 34.19971097300155094 ) ) ;
#74691=CARTESIAN_POINT ( 'NONE',  ( -12.71151519248081740, -9.148715823498378086, 34.47080413974185120 ) ) ;
#74692=CARTESIAN_POINT ( 'NONE',  ( 2.307692307692309264, -2.708943851104267164, 35.45975837776705220 ) ) ;
#74693=CARTESIAN_POINT ( 'NONE',  ( 0.4615384615383382183, -6.835583212225970762, 34.95778746994575670 ) ) ;
#74696=CARTESIAN_POINT ( 'NONE',  ( -4.946397375159511611, -10.88167719472716399, 33.43325721877153711 ) ) ;
#74698=ORIENTED_EDGE ( 'NONE', *, *, #21192, .F. ) ;
#74699=CARTESIAN_POINT ( 'NONE',  ( 2.372947878968333590, -6.879047030191282275, 34.71129190930002295 ) ) ;
#74700=CARTESIAN_POINT ( 'NONE',  ( 0.3954560821783248969, -10.67929555188718460, 33.92786785259543336 ) ) ;
#74703=AXIS2_PLACEMENT_3D ( 'NONE', #70899, #22700, #63686 ) ;
#74705=EDGE_CURVE ( 'NONE', #84371, #36979, #26349, .T. ) ;
#74707=CARTESIAN_POINT ( 'NONE',  ( 15.93091919493930320, -2.308479472611653094, 30.53278059502174457 ) ) ;
#74708=CARTESIAN_POINT ( 'NONE',  ( 9.692307692307572609, -2.892918686052165622, 31.69288490824153470 ) ) ;
#74709=ORIENTED_EDGE ( 'NONE', *, *, #480, .F. ) ;
#74710=CARTESIAN_POINT ( 'NONE',  ( 11.53846153846153832, -9.905515769479276145, 34.41647553114623292 ) ) ;
#74711=CARTESIAN_POINT ( 'NONE',  ( 6.923076923076924238, -8.164416787775445883, 34.95778746994557906 ) ) ;
#74712=FACE_BOUND ( 'NONE', #8524, .T. ) ;
#74714=CARTESIAN_POINT ( 'NONE',  ( -6.923076923076922462, -2.249999999999998668, 29.75000000000001776 ) ) ;
#74715=DIRECTION ( 'NONE',  ( -0.000000000000000000, 0.7660444431189791237, -0.6427876096865379196 ) ) ;
#74716=CARTESIAN_POINT ( 'NONE',  ( 2.084765348785460048, -6.459968553980839800, 34.89616026154728701 ) ) ;
#74717=CYLINDRICAL_SURFACE ( 'NONE', #59684, 0.2499999999999986955 ) ;
#74718=CARTESIAN_POINT ( 'NONE',  ( -10.39237177129121825, -11.43677907613344757, 33.22367315496202167 ) ) ;
#74720=ORIENTED_EDGE ( 'NONE', *, *, #86295, .F. ) ;
#74721=VERTEX_POINT ( 'NONE', #18256 ) ;
#74722=CARTESIAN_POINT ( 'NONE',  ( -12.33101302330481808, -5.915461855592780260, 34.75538340440931506 ) ) ;
#74723=CARTESIAN_POINT ( 'NONE',  ( 16.21991450484859598, -6.386643153685127139, 34.62446782046654192 ) ) ;
#74724=DIRECTION ( 'NONE',  ( -0.000000000000000000, -0.000000000000000000, -1.000000000000000000 ) ) ;
#74725=CARTESIAN_POINT ( 'NONE',  ( -0.7115384615384606759, -7.433931650972300353, 34.75000000000000711 ) ) ;
#74726=CYLINDRICAL_SURFACE ( 'NONE', #21255, 0.2499999999999986955 ) ;
#74728=ADVANCED_FACE ( 'NONE', ( #45720 ), #12386, .F. ) ;
#74729=B_SPLINE_CURVE_WITH_KNOTS ( 'NONE', 3,
 ( #49914, #42733, #34640, #42294, #56679, #70195, #76062, #48582, #62106, #62535 ),
 .UNSPECIFIED., .F., .F.,
 ( 4, 2, 2, 2, 4 ),
 ( 0.0007817246256747507503, 0.0009771112852218959231, 0.001172497944769040987, 0.001367884604316186052, 0.001563271263863331116 ),
 .UNSPECIFIED. ) ;
#74730=CARTESIAN_POINT ( 'NONE',  ( -8.769230769230892619, -10.33852847137269571, 34.16647553114546554 ) ) ;
#74731=CARTESIAN_POINT ( 'NONE',  ( -6.066082379360134169, -8.164416787775445883, 34.95778746994557906 ) ) ;
#74732=EDGE_CURVE ( 'NONE', #33999, #11687, #5938, .T. ) ;
#74733=CARTESIAN_POINT ( 'NONE',  ( 7.780883845597525550, -5.941354392334499579, 34.76329471203369792 ) ) ;
#74734=DIRECTION ( 'NONE',  ( -0.000000000000000000, -0.8660254037844397068, -0.4999999999999978906 ) ) ;
#74735=CARTESIAN_POINT ( 'NONE',  ( 9.915087233576103998, -2.847695495035523550, 31.58253572463339154 ) ) ;
#74736=CARTESIAN_POINT ( 'NONE',  ( 13.13463865367303285, -4.236021600441997492, 33.53823185664189310 ) ) ;
#74738=CARTESIAN_POINT ( 'NONE',  ( -17.07692307692307665, -11.16473453929635440, 33.15142922261926373 ) ) ;
#74739=DIRECTION ( 'NONE',  ( -0.000000000000000000, -0.7660444431189791237, -0.6427876096865379196 ) ) ;
#74741=EDGE_LOOP ( 'NONE', ( #48960, #17593 ) ) ;
#74742=AXIS2_PLACEMENT_3D ( 'NONE', #60522, #17770, #25857 ) ;
#74743=CARTESIAN_POINT ( 'NONE',  ( 8.769230769230768274, -4.661471528628507777, 34.16647553114623292 ) ) ;
#74744=CARTESIAN_POINT ( 'NONE',  ( -3.453695448285377889, -3.586966769969700763, 32.86292498521069660 ) ) ;
#74746=CARTESIAN_POINT ( 'NONE',  ( -0.2114840416250094168, -10.82426656108011720, 33.81400080652039009 ) ) ;
#74748=CARTESIAN_POINT ( 'NONE',  ( -11.53846153846166089, -5.094484230521993062, 34.41647553114689373 ) ) ;
#74749=DIRECTION ( 'NONE',  ( -0.000000000000000000, -0.6427876096865404731, -0.7660444431189770143 ) ) ;
#74750=VERTEX_POINT ( 'NONE', #4748 ) ;
#74752=CARTESIAN_POINT ( 'NONE',  ( -14.37296230824862775, -5.941354392334499579, 34.76329471203369792 ) ) ;
#74753=VERTEX_POINT ( 'NONE', #32218 ) ;
#74755=CARTESIAN_POINT ( 'NONE',  ( 0.4615384615383396616, -2.892918686052166066, 31.69288490824153470 ) ) ;
#74756=ORIENTED_EDGE ( 'NONE', *, *, #87309, .F. ) ;
#74757=CARTESIAN_POINT ( 'NONE',  ( 7.846153846153846700, -4.098570777380720287, 33.41473453929634729 ) ) ;
#74759=CARTESIAN_POINT ( 'NONE',  ( -8.096130577096202430, -3.627789207965226748, 32.91389620160131102 ) ) ;
#74761=ORIENTED_EDGE ( 'NONE', *, *, #86777, .T. ) ;
#74762=VERTEX_POINT ( 'NONE', #59679 ) ;
#74763=B_SPLINE_CURVE_WITH_KNOTS ( 'NONE', 3,
 ( #83849, #15384, #49603, #16259, #3621, #2283 ),
 .UNSPECIFIED., .F., .F.,
 ( 4, 2, 4 ),
 ( 0.0003909569690057829237, 0.0005862646681846087407, 0.0007815723673634345035 ),
 .UNSPECIFIED. ) ;
#74764=AXIS2_PLACEMENT_3D ( 'NONE', #43564, #44886, #51179 ) ;
#74765=AXIS2_PLACEMENT_3D ( 'NONE', #68786, #70998, #57923 ) ;
#74766=CARTESIAN_POINT ( 'NONE',  ( -14.98082382139118884, -4.176053281294518804, 33.81426240980091791 ) ) ;
#74767=CARTESIAN_POINT ( 'NONE',  ( 7.053867364043877153, -11.37503395064541678, 33.29242100308974983 ) ) ;
#74768=CARTESIAN_POINT ( 'NONE',  ( -10.48485891362105171, -6.852161475712352789, 34.70806712695775786 ) ) ;
#74769=CARTESIAN_POINT ( 'NONE',  ( -15.45425415533356350, -2.353723527008296568, 30.78948104536958752 ) ) ;
#74770=B_SPLINE_CURVE_WITH_KNOTS ( 'NONE', 3,
 ( #36607, #83925, #35731, #77594, #15901, #2358, #69944, #21758, #29419, #28981 ),
 .UNSPECIFIED., .F., .F.,
 ( 4, 2, 2, 2, 4 ),
 ( 0.000000000000000000, 0.0001954311564186882026, 0.0003908623128373764051, 0.0005862934692560646619, 0.0007817246256747528103 ),
 .UNSPECIFIED. ) ;
#74771=FACE_OUTER_BOUND ( 'NONE', #65437, .T. ) ;
#74772=CARTESIAN_POINT ( 'NONE',  ( -3.230769230769229949, -4.661471528628507777, 34.16647553114623292 ) ) ;
#74773=CARTESIAN_POINT ( 'NONE',  ( 13.60739492588379562, -3.236590943229499029, 32.36255958852954251 ) ) ;
#74775=AXIS2_PLACEMENT_3D ( 'NONE', #68145, #6448, #47866 ) ;
#74776=ADVANCED_FACE ( 'NONE', ( #87178 ), #52910, .F. ) ;
#74777=CARTESIAN_POINT ( 'NONE',  ( 14.30769230769231015, -3.886160181151819604, 36.00935417666054406 ) ) ;
#74778=ORIENTED_EDGE ( 'NONE', *, *, #8986, .T. ) ;
#74779=VERTEX_POINT ( 'NONE', #56022 ) ;
#74780=CARTESIAN_POINT ( 'NONE',  ( 18.06606733335007675, -9.058645607665452459, 34.76329471203371924 ) ) ;
#74781=ORIENTED_EDGE ( 'NONE', *, *, #69341, .T. ) ;
#74782=EDGE_CURVE ( 'NONE', #28433, #30133, #22036, .T. ) ;
#74783=CARTESIAN_POINT ( 'NONE',  ( 11.60452887181161508, -3.322132147404559976, 32.92929555188717927 ) ) ;
#74784=CARTESIAN_POINT ( 'NONE',  ( 11.76147289007438879, -12.15243808032445827, 31.58219941686247978 ) ) ;
#74785=EDGE_LOOP ( 'NONE', ( #16012, #20316 ) ) ;
#74787=EDGE_CURVE ( 'NONE', #86499, #54317, #88956, .T. ) ;
#74788=ORIENTED_EDGE ( 'NONE', *, *, #480, .T. ) ;
#74789=LINE ( 'NONE', #40564, #65530 ) ;
#74790=EDGE_LOOP ( 'NONE', ( #69328, #47517 ) ) ;
#74791=CARTESIAN_POINT ( 'NONE',  ( 9.915087233576098669, -8.496831190052093419, 34.64984203495476578 ) ) ;
#74792=EDGE_LOOP ( 'NONE', ( #15026, #3199 ) ) ;
#74793=CARTESIAN_POINT ( 'NONE',  ( -12.39547112818838492, -9.905515769479276145, 34.41647553114623292 ) ) ;
#74794=AXIS2_PLACEMENT_3D ( 'NONE', #81045, #66172, #5378 ) ;
#74795=CARTESIAN_POINT ( 'NONE',  ( 10.83839596699746721, -4.887748414852792322, 34.01359900205216746 ) ) ;
#74796=FACE_BOUND ( 'NONE', #84471, .T. ) ;
#74797=EDGE_CURVE ( 'NONE', #55341, #39944, #9122, .T. ) ;
#74798=CARTESIAN_POINT ( 'NONE',  ( 12.71153846153988098, -7.500000000000154543, 35.00000000000007105 ) ) ;
#74799=DIRECTION ( 'NONE',  ( -0.000000000000000000, 0.5000000000000011102, -0.8660254037844381525 ) ) ;
#74800=CARTESIAN_POINT ( 'NONE',  ( -1.608100309179714582, -2.353723527008297012, 30.78948104536958397 ) ) ;
#74801=CARTESIAN_POINT ( 'NONE',  ( -3.230769230769229949, -4.098570777380720287, 33.41473453929634729 ) ) ;
#74802=DIRECTION ( 'NONE',  ( 0.000000000000000000, 0.6427876096865368094, 0.7660444431189802339 ) ) ;
#74803=DIRECTION ( 'NONE',  ( -0.000000000000000000, 0.7660444431189791237, -0.6427876096865379196 ) ) ;
#74804=EDGE_CURVE ( 'NONE', #2166, #65829, #79948, .T. ) ;
#74805=CARTESIAN_POINT ( 'NONE',  ( -10.48459280755982626, -4.118422570099831148, 33.43335022499816489 ) ) ;
#74806=ORIENTED_EDGE ( 'NONE', *, *, #54401, .T. ) ;
#74807=ORIENTED_EDGE ( 'NONE', *, *, #69211, .T. ) ;
#74808=CARTESIAN_POINT ( 'NONE',  ( -8.769230769230890843, -11.94971097300221174, 32.03036669348237098 ) ) ;
#74810=CARTESIAN_POINT ( 'NONE',  ( -9.692307692307691624, -9.584722331328613620, 36.20867863119891439 ) ) ;
#74812=CARTESIAN_POINT ( 'NONE',  ( 8.992657168145557378, -7.630147987733840509, 34.99859428049665411 ) ) ;
#74813=CARTESIAN_POINT ( 'NONE',  ( -13.13456107297706765, -2.779044189368095275, 31.39831045268885745 ) ) ;
#74814=ORIENTED_EDGE ( 'NONE', *, *, #16168, .F. ) ;
#74815=CARTESIAN_POINT ( 'NONE',  ( -5.776987155906603277, -8.282913670948747864, 34.94150082978203642 ) ) ;
#74816=EDGE_CURVE ( 'NONE', #18683, #80371, #33979, .T. ) ;
#74817=CARTESIAN_POINT ( 'NONE',  ( -4.826977558574935045, -2.587454068350147462, 30.68340429815432202 ) ) ;
#74818=FACE_OUTER_BOUND ( 'NONE', #52948, .T. ) ;
#74819=VECTOR ( 'NONE', #9561, 1000.000000000000114 ) ;
#74820=DIRECTION ( 'NONE',  ( -0.000000000000000000, -0.5000000000000009992, -0.8660254037844380415 ) ) ;
#74821=EDGE_LOOP ( 'NONE', ( #62706, #53495 ) ) ;
#74822=B_SPLINE_CURVE_WITH_KNOTS ( 'NONE', 3,
 ( #57198, #1809, #43678, #55424, #488, #82909, #42812, #77907, #76591, #7246 ),
 .UNSPECIFIED., .F., .F.,
 ( 4, 2, 2, 2, 4 ),
 ( 0.0007817359430256326080, 0.0009771253907249993591, 0.001172514838424366327, 0.001367904286123733078, 0.001563293733823099829 ),
 .UNSPECIFIED. ) ;
#74823=ORIENTED_EDGE ( 'NONE', *, *, #61704, .T. ) ;
#74825=AXIS2_PLACEMENT_3D ( 'NONE', #34349, #83446, #575 ) ;
#74826=VERTEX_POINT ( 'NONE', #61887 ) ;
#74827=CYLINDRICAL_SURFACE ( 'NONE', #67899, 0.2499999999999995559 ) ;
#74828=ORIENTED_EDGE ( 'NONE', *, *, #6367, .T. ) ;
#74829=CARTESIAN_POINT ( 'NONE',  ( 6.923076923076924238, -1.790695186598648903, 34.54067556320373455 ) ) ;
#74830=CARTESIAN_POINT ( 'NONE',  ( -10.61538461538473399, -6.879047030192662504, 34.71129190930017927 ) ) ;
#74831=CARTESIAN_POINT ( 'NONE',  ( -5.076923076923197442, -4.481592998941358097, 33.73612834414048933 ) ) ;
#74832=CARTESIAN_POINT ( 'NONE',  ( 8.834485908743602067, -3.643525952247864463, 33.31231777344670064 ) ) ;
#74833=AXIS2_PLACEMENT_3D ( 'NONE', #3486, #2597, #52120 ) ;
#74834=EDGE_CURVE ( 'NONE', #38437, #80242, #14370, .T. ) ;
#74835=CYLINDRICAL_SURFACE ( 'NONE', #66161, 0.2499999999999995559 ) ;
#74836=ORIENTED_EDGE ( 'NONE', *, *, #64510, .T. ) ;
#74837=CARTESIAN_POINT ( 'NONE',  ( -11.78846153846154010, -7.433932668274256805, 35.00000000000000711 ) ) ;
#74838=CARTESIAN_POINT ( 'NONE',  ( -12.46153846153858247, -11.94971097300221174, 32.03036669348237098 ) ) ;
#74839=ORIENTED_EDGE ( 'NONE', *, *, #79985, .T. ) ;
#74840=CARTESIAN_POINT ( 'NONE',  ( -5.326899820971668476, -2.318417181685854978, 30.59732222474233865 ) ) ;
#74841=CARTESIAN_POINT ( 'NONE',  ( 15.90384615384614619, -2.499999999999999556, 29.81609845454691765 ) ) ;
#74842=CARTESIAN_POINT ( 'NONE',  ( 1.449761163947351328, -7.750023238201980469, 34.74374492549440419 ) ) ;
#74843=EDGE_CURVE ( 'NONE', #56000, #6801, #642, .T. ) ;
#74845=CARTESIAN_POINT ( 'NONE',  ( -2.557669051740897537, -12.65889640711025521, 30.72598325615533454 ) ) ;
#74846=CARTESIAN_POINT ( 'NONE',  ( 13.16113046005105502, -4.225889041578353655, 33.85425143139329407 ) ) ;
#74847=CARTESIAN_POINT ( 'NONE',  ( 18.22277954126840172, -2.600157965045223563, 30.74683119005207033 ) ) ;
#74850=EDGE_CURVE ( 'NONE', #74160, #85301, #47038, .T. ) ;
#74852=EDGE_CURVE ( 'NONE', #31425, #40761, #20022, .T. ) ;
#74853=CARTESIAN_POINT ( 'NONE',  ( 11.53846153846141753, -2.892918686052165622, 31.69288490824153470 ) ) ;
#74854=CARTESIAN_POINT ( 'NONE',  ( -14.08491263871424160, -3.563462043263030399, 33.22394488606062879 ) ) ;
#74857=CARTESIAN_POINT ( 'NONE',  ( -12.71151519248081740, -11.79746400365624659, 32.30657167506340954 ) ) ;
#74859=DIRECTION ( 'NONE',  ( -0.000000000000000000, 0.1736481776669307198, -0.9848077530122080203 ) ) ;
#74860=DIRECTION ( 'NONE',  ( 0.000000000000000000, 0.1736481776669275834, 0.9848077530122086864 ) ) ;
#74861=CARTESIAN_POINT ( 'NONE',  ( 14.30769230769218758, -11.48612834414049644, 32.76840700105863391 ) ) ;
#74862=VERTEX_POINT ( 'NONE', #78066 ) ;
#74863=CARTESIAN_POINT ( 'NONE',  ( 16.82694634598072625, -3.137211980971220893, 32.19342716148376837 ) ) ;
#74864=B_SPLINE_CURVE_WITH_KNOTS ( 'NONE', 3,
 ( #28890, #84723, #41953, #55895, #35639, #77064, #36084, #75721, #42403, #63536 ),
 .UNSPECIFIED., .F., .F.,
 ( 4, 2, 2, 2, 4 ),
 ( 0.000000000000000000, 0.0001954339857564081791, 0.0003908679715128163582, 0.0005863019572692245102, 0.0007817359430256327164 ),
 .UNSPECIFIED. ) ;
#74865=CARTESIAN_POINT ( 'NONE',  ( 17.29993442853592711, -5.667800583137506898, 34.40243808032445827 ) ) ;
#74866=CARTESIAN_POINT ( 'NONE',  ( 5.326868486301119532, -12.45601412856602863, 31.48342859153981621 ) ) ;
#74868=ORIENTED_EDGE ( 'NONE', *, *, #66514, .F. ) ;
#74869=CARTESIAN_POINT ( 'NONE',  ( -8.834984197544098805, -7.249945578846652694, 34.99404164642496795 ) ) ;
#74870=VERTEX_POINT ( 'NONE', #16368 ) ;
#74871=CARTESIAN_POINT ( 'NONE',  ( -16.40386939113911779, -5.851115903089112003, 34.47074536777953568 ) ) ;
#74873=CARTESIAN_POINT ( 'NONE',  ( 11.40777093535123221, -2.494641256782728966, 31.33461815524612959 ) ) ;
#74874=ORIENTED_EDGE ( 'NONE', *, *, #75834, .F. ) ;
#74876=CYLINDRICAL_SURFACE ( 'NONE', #52158, 0.2499999999999986955 ) ;
#74878=CARTESIAN_POINT ( 'NONE',  ( 13.38461538461526601, -11.94971097300221174, 32.03036669348237098 ) ) ;
#74880=EDGE_LOOP ( 'NONE', ( #70572, #57107 ) ) ;
#74881=AXIS2_PLACEMENT_3D ( 'NONE', #4792, #54288, #13315 ) ;
#74882=FACE_BOUND ( 'NONE', #35305, .T. ) ;
#74883=ORIENTED_EDGE ( 'NONE', *, *, #42146, .F. ) ;
#74884=CARTESIAN_POINT ( 'NONE',  ( 17.99999999999987566, -11.06231777344772027, 33.60647404775119895 ) ) ;
#74885=CARTESIAN_POINT ( 'NONE',  ( 5.076923076922954969, -12.46129190930018460, 30.37095296980731973 ) ) ;
#74886=AXIS2_PLACEMENT_3D ( 'NONE', #50113, #29857, #65725 ) ;
#74888=CYLINDRICAL_SURFACE ( 'NONE', #34874, 0.2499999999999998890 ) ;
#74889=CARTESIAN_POINT ( 'NONE',  ( 14.55774672760575861, -8.346898887586323923, 34.93166121998716278 ) ) ;
#74890=AXIS2_PLACEMENT_3D ( 'NONE', #63031, #21172, #34696 ) ;
#74891=ORIENTED_EDGE ( 'NONE', *, *, #5205, .F. ) ;
#74892=B_SPLINE_CURVE_WITH_KNOTS ( 'NONE', 3,
 ( #60036, #10527, #65897, #80779, #85744, #24025, #78977, #3758, #31232, #58700 ),
 .UNSPECIFIED., .F., .F.,
 ( 4, 2, 2, 2, 4 ),
 ( 0.0007817359430256330417, 0.0009771253907250000096, 0.001172514838424367194, 0.001367904286123734162, 0.001563293733823101130 ),
 .UNSPECIFIED. ) ;
#74896=VERTEX_POINT ( 'NONE', #71742 ) ;
#74897=B_SPLINE_CURVE_WITH_KNOTS ( 'NONE', 3,
 ( #57491, #43976, #77765, #57935, #63364, #35457, #22383, #85419, #77327, #43535 ),
 .UNSPECIFIED., .F., .F.,
 ( 4, 2, 2, 2, 4 ),
 ( 0.0007817246256747471724, 0.0009771112852218905021, 0.001172497944769033615, 0.001367884604316176944, 0.001563271263863320274 ),
 .UNSPECIFIED. ) ;
#74899=CARTESIAN_POINT ( 'NONE',  ( 16.28463659481310444, -10.70102852606553157, 33.91149625220312913 ) ) ;
#74900=DIRECTION ( 'NONE',  ( -0.000000000000000000, 1.000000000000000000, 3.491481338843133355E-15 ) ) ;
#74901=CARTESIAN_POINT ( 'NONE',  ( 5.076923076922953193, -11.67786785259630911, 32.92929555188603530 ) ) ;
#74902=FACE_OUTER_BOUND ( 'NONE', #6122, .T. ) ;
#74903=EDGE_CURVE ( 'NONE', #13392, #7875, #56472, .T. ) ;
#74904=CARTESIAN_POINT ( 'NONE',  ( 12.46153846153846168, -6.435427911321262684, 35.78748833219616898 ) ) ;
#74905=CARTESIAN_POINT ( 'NONE',  ( -17.93455011887488126, -12.75000000000000533, 29.49999999999997868 ) ) ;
#74908=ORIENTED_EDGE ( 'NONE', *, *, #8095, .T. ) ;
#74909=EDGE_LOOP ( 'NONE', ( #47865, #51999 ) ) ;
#74910=CARTESIAN_POINT ( 'NONE',  ( -13.60754234352223335, -12.38737895849757820, 31.66785238281580206 ) ) ;
#74911=CARTESIAN_POINT ( 'NONE',  ( -39.05038313613820122, -2.499999999999999556, 29.75000000000000355 ) ) ;
#74912=CARTESIAN_POINT ( 'NONE',  ( 6.923076923076924238, -1.629998284177014645, 34.34916445242399163 ) ) ;
#74914=CYLINDRICAL_SURFACE ( 'NONE', #16385, 0.2499999999999995559 ) ;
#74915=FACE_BOUND ( 'NONE', #1197, .T. ) ;
#74916=ORIENTED_EDGE ( 'NONE', *, *, #41553, .F. ) ;
#74917=ADVANCED_FACE ( 'NONE', ( #23997 ), #29454, .F. ) ;
#74918=CARTESIAN_POINT ( 'NONE',  ( 14.30769230769218581, -2.379036618888197729, 30.90682066428292885 ) ) ;
#74919=CARTESIAN_POINT ( 'NONE',  ( -3.165513659493205623, -6.879047030191282275, 34.71129190930002295 ) ) ;
#74920=VECTOR ( 'NONE', #86386, 1000.000000000000227 ) ;
#74921=VERTEX_POINT ( 'NONE', #50586 ) ;
#74922=CARTESIAN_POINT ( 'NONE',  ( 4.853438152358743984, -2.353723527008295680, 30.78948104536958752 ) ) ;
#74923=VERTEX_POINT ( 'NONE', #72189 ) ;
#74924=FACE_BOUND ( 'NONE', #46932, .T. ) ;
#74925=CARTESIAN_POINT ( 'NONE',  ( 7.622668902429897919, -11.89387501736622710, 32.13663884655806413 ) ) ;
#74926=B_SPLINE_CURVE_WITH_KNOTS ( 'NONE', 3,
 ( #685, #48869, #17304, #64143, #2016, #2445, #2882, #9231, #64584, #10100 ),
 .UNSPECIFIED., .F., .F.,
 ( 4, 2, 2, 2, 4 ),
 ( 0.0007817246256747455461, 0.0009771112852218883336, 0.001172497944769031230, 0.001367884604316174126, 0.001563271263863317022 ),
 .UNSPECIFIED. ) ;
#74927=CARTESIAN_POINT ( 'NONE',  ( -13.60810032833933469, -10.81261337010820256, 33.49550067578627477 ) ) ;
#74928=ORIENTED_EDGE ( 'NONE', *, *, #19082, .T. ) ;
#74929=FACE_OUTER_BOUND ( 'NONE', #6718, .T. ) ;
#74930=CARTESIAN_POINT ( 'NONE',  ( 10.61538461538449418, -5.941354392335915335, 34.76329471203413846 ) ) ;
#74931=CARTESIAN_POINT ( 'NONE',  ( 2.980792486720641232, -12.01397095200673881, 32.43157075238190146 ) ) ;
#74932=ORIENTED_EDGE ( 'NONE', *, *, #44877, .F. ) ;
#74933=B_SPLINE_CURVE_WITH_KNOTS ( 'NONE', 3,
 ( #82741, #13383, #755, #84077, #42199, #42636, #34098, #34543, #22353, #21470 ),
 .UNSPECIFIED., .F., .F.,
 ( 4, 2, 2, 2, 4 ),
 ( 0.0007817359430256322827, 0.0009771253907249989254, 0.001172514838424365676, 0.001367904286123732428, 0.001563293733823098962 ),
 .UNSPECIFIED. ) ;
#74934=CARTESIAN_POINT ( 'NONE',  ( 6.699591979352975457, -5.912607949931405038, 34.49155766932282319 ) ) ;
#74935=CARTESIAN_POINT ( 'NONE',  ( -17.07692307692307665, -1.117168528481311540, 33.14645433367849847 ) ) ;
#74936=CARTESIAN_POINT ( 'NONE',  ( 12.71148397988660150, -6.696923467548660192, 34.68552623307873972 ) ) ;
#74937=CARTESIAN_POINT ( 'NONE',  ( -17.77698715590660328, -12.64618726649961289, 30.78989965857442712 ) ) ;
#74938=EDGE_LOOP ( 'NONE', ( #82015, #28956 ) ) ;
#74939=CARTESIAN_POINT ( 'NONE',  ( -12.21159294319032185, -3.202959910592335646, 32.30730279482227019 ) ) ;
#74940=DIRECTION ( 'NONE',  ( -0.000000000000000000, -0.8660254037844399289, -0.4999999999999980016 ) ) ;
#74942=CARTESIAN_POINT ( 'NONE',  ( 9.692307692307695177, -1.215029322943914858, 32.30358669280327177 ) ) ;
#74943=CARTESIAN_POINT ( 'NONE',  ( 9.942307692309114486, -7.500000000000154543, 35.00000000000007105 ) ) ;
#74944=CARTESIAN_POINT ( 'NONE',  ( 5.869852790561781219, -9.418419913701741919, 34.36755862841477693 ) ) ;
#74945=CARTESIAN_POINT ( 'NONE',  ( -11.60373198442231590, -8.613356846314824011, 34.62446782046655613 ) ) ;
#74946=B_SPLINE_CURVE_WITH_KNOTS ( 'NONE', 3,
 ( #69310, #14813, #7608, #35071, #62529, #844, #55780, #83270, #21557, #88280 ),
 .UNSPECIFIED., .F., .F.,
 ( 4, 2, 2, 2, 4 ),
 ( 0.0007817246256747519429, 0.0009771112852218970073, 0.001172497944769042288, 0.001367884604316187353, 0.001563271263863332417 ),
 .UNSPECIFIED. ) ;
#74947=CARTESIAN_POINT ( 'NONE',  ( -13.31854703361294767, -3.513871655860379306, 32.76840700105978499 ) ) ;
#74948=ADVANCED_FACE ( 'NONE', ( #50140 ), #51010, .F. ) ;
#74949=EDGE_CURVE ( 'NONE', #45049, #25143, #81078, .T. ) ;
#74952=CARTESIAN_POINT ( 'NONE',  ( -16.15384615384627409, -8.656820664282941280, 34.87096338111179961 ) ) ;
#74953=VECTOR ( 'NONE', #75365, 1000.000000000000227 ) ;
#74954=DIRECTION ( 'NONE',  ( -0.000000000000000000, 0.1736481776669307198, -0.9848077530122080203 ) ) ;
#74956=ORIENTED_EDGE ( 'NONE', *, *, #40379, .F. ) ;
#74957=CARTESIAN_POINT ( 'NONE',  ( -15.23076923076935074, -3.835265460704628371, 33.15142922262033665 ) ) ;
#74958=ORIENTED_EDGE ( 'NONE', *, *, #27373, .F. ) ;
#74960=VERTEX_POINT ( 'NONE', #49708 ) ;
#74961=CARTESIAN_POINT ( 'NONE',  ( -8.703975629717932705, -6.835583212224610072, 34.95778746994559327 ) ) ;
#74962=EDGE_LOOP ( 'NONE', ( #44107, #6636, #63276, #46950 ) ) ;
#74963=DIRECTION ( 'NONE',  ( -0.000000000000000000, -0.1736481776669307198, -0.9848077530122080203 ) ) ;
#74965=ADVANCED_FACE ( 'NONE', ( #77625 ), #1971, .F. ) ;
#74966=CARTESIAN_POINT ( 'NONE',  ( -14.30769230769242917, -3.083524468854526912, 32.58852847137268327 ) ) ;
#74967=DIRECTION ( 'NONE',  ( -0.000000000000000000, -0.9396926207859093161, -0.3420201433256663259 ) ) ;
#74968=CARTESIAN_POINT ( 'NONE',  ( 6.249945518348143381, -3.202959910592335202, 32.30730279482227019 ) ) ;
#74969=CARTESIAN_POINT ( 'NONE',  ( -6.923076923076922462, -8.810774026931790459, 35.74407628777942847 ) ) ;
#74970=CARTESIAN_POINT ( 'NONE',  ( 9.692307692307695177, -12.34228464037088635, 31.77849191805839268 ) ) ;
#74971=DIRECTION ( 'NONE',  ( -0.000000000000000000, 1.000000000000000000, 3.491481338843133355E-15 ) ) ;
#74972=FACE_OUTER_BOUND ( 'NONE', #36797, .T. ) ;
#74973=CARTESIAN_POINT ( 'NONE',  ( 10.68145194873469173, -12.34228464037088813, 31.77849191805839268 ) ) ;
#74974=CARTESIAN_POINT ( 'NONE',  ( -13.16183584334697443, -6.760870238392817200, 34.69528174975672385 ) ) ;
#74975=CARTESIAN_POINT ( 'NONE',  ( 5.207713517890025123, -10.70102852606553157, 33.91149625220312913 ) ) ;
#74976=VERTEX_POINT ( 'NONE', #58229 ) ;
#74977=VERTEX_POINT ( 'NONE', #15492 ) ;
#74978=DIRECTION ( 'NONE',  ( -0.000000000000000000, 0.7660444431189791237, -0.6427876096865379196 ) ) ;
#74979=CARTESIAN_POINT ( 'NONE',  ( 5.207714884747862705, -8.999086150933472084, 34.52020707165672064 ) ) ;
#74980=CYLINDRICAL_SURFACE ( 'NONE', #79972, 0.2500000000000002220 ) ;
#74981=CARTESIAN_POINT ( 'NONE',  ( -11.66893824657800316, -7.276988635370452485, 34.74523720219453793 ) ) ;
#74982=LINE ( 'NONE', #25901, #26215 ) ;
#74983=CARTESIAN_POINT ( 'NONE',  ( -9.561517251340744039, -10.70102852606553157, 33.91149625220312913 ) ) ;
#74986=ORIENTED_EDGE ( 'NONE', *, *, #50912, .F. ) ;
#74987=CARTESIAN_POINT ( 'NONE',  ( -5.076923076923197442, -12.46129190930018460, 30.37095296980731973 ) ) ;
#74988=ORIENTED_EDGE ( 'NONE', *, *, #82380, .T. ) ;
#74989=VECTOR ( 'NONE', #78475, 1000.000000000000000 ) ;
#74990=B_SPLINE_CURVE_WITH_KNOTS ( 'NONE', 3,
 ( #71352, #43450, #64146, #23613, #35817, #35359, #15541, #37124, #1580, #9658 ),
 .UNSPECIFIED., .F., .F.,
 ( 4, 2, 2, 2, 4 ),
 ( 0.0007817246256747484735, 0.0009771112852218928873, 0.001172497944769037084, 0.001367884604316181498, 0.001563271263863325912 ),
 .UNSPECIFIED. ) ;
#74991=ORIENTED_EDGE ( 'NONE', *, *, #85193, .T. ) ;
#74992=CARTESIAN_POINT ( 'NONE',  ( 17.86985279056177944, -3.285722584762969856, 32.44110544564090759 ) ) ;
#74993=CARTESIAN_POINT ( 'NONE',  ( 4.023370968770434430, -7.276987145209185215, 34.99546412871779211 ) ) ;
#74994=CARTESIAN_POINT ( 'NONE',  ( 11.76124107972994537, -10.81320215134717344, 33.49497208177562868 ) ) ;
#74995=CARTESIAN_POINT ( 'NONE',  ( -11.53846153846153655, -4.102666532097928531, 36.13435417666054406 ) ) ;
#74996=DIRECTION ( 'NONE',  ( -1.000000000000000000, 0.000000000000000000, 0.000000000000000000 ) ) ;
#74997=ADVANCED_FACE ( 'NONE', ( #29890 ), #71299, .F. ) ;
#74998=VERTEX_POINT ( 'NONE', #64980 ) ;
#75000=ORIENTED_EDGE ( 'NONE', *, *, #5358, .T. ) ;
#75001=ORIENTED_EDGE ( 'NONE', *, *, #72683, .F. ) ;
#75002=AXIS2_PLACEMENT_3D ( 'NONE', #37036, #9572, #51873 ) ;
#75003=CARTESIAN_POINT ( 'NONE',  ( 18.13079044096695469, -2.295524264805589354, 30.44142389570982488 ) ) ;
#75004=CARTESIAN_POINT ( 'NONE',  ( -10.61538461538461320, -13.57706302396349152, 30.56769352161908060 ) ) ;
#75007=CARTESIAN_POINT ( 'NONE',  ( 14.05769230769230660, -7.566082377512564960, 35.00000000000000711 ) ) ;
#75008=EDGE_CURVE ( 'NONE', #67806, #38794, #19808, .T. ) ;
#75010=CARTESIAN_POINT ( 'NONE',  ( 2.307692307692309264, -5.471508081941601098, 34.59228464037088457 ) ) ;
#75011=VERTEX_POINT ( 'NONE', #15933 ) ;
#75012=EDGE_CURVE ( 'NONE', #58400, #84958, #18700, .T. ) ;
#75013=ORIENTED_EDGE ( 'NONE', *, *, #41998, .F. ) ;
#75014=VECTOR ( 'NONE', #8043, 1000.000000000000114 ) ;
#75016=CARTESIAN_POINT ( 'NONE',  ( -3.296851610129365451, -2.486705287966279876, 31.30864560766542937 ) ) ;
#75017=EDGE_LOOP ( 'NONE', ( #15261, #70779 ) ) ;
#75018=CARTESIAN_POINT ( 'NONE',  ( 9.692307692307570832, -8.656820664282941280, 34.87096338111179961 ) ) ;
#75019=CARTESIAN_POINT ( 'NONE',  ( -4.946397375159516052, -11.46989282347013095, 32.79007818306219946 ) ) ;
#75021=EDGE_LOOP ( 'NONE', ( #56607, #87022, #54949, #78473 ) ) ;
#75022=ADVANCED_FACE ( 'NONE', ( #30325 ), #38413, .F. ) ;
#75023=CARTESIAN_POINT ( 'NONE',  ( 3.454144716541651672, -2.251407671071270489, 29.88021292934942252 ) ) ;
#75024=ORIENTED_EDGE ( 'NONE', *, *, #10944, .F. ) ;
#75025=CARTESIAN_POINT ( 'NONE',  ( 8.096208157792160520, -12.17597550085003277, 31.52189283813461174 ) ) ;
#75026=FACE_BOUND ( 'NONE', #30262, .T. ) ;
#75027=DIRECTION ( 'NONE',  ( -0.000000000000000000, 0.7660444431189791237, -0.6427876096865379196 ) ) ;
#75028=EDGE_CURVE ( 'NONE', #41890, #27582, #43409, .T. ) ;
#75029=CARTESIAN_POINT ( 'NONE',  ( 9.692307692307695177, -2.249999999999998668, 29.75000000000001776 ) ) ;
#75030=VERTEX_POINT ( 'NONE', #73544 ) ;
#75031=CARTESIAN_POINT ( 'NONE',  ( 8.545745844666440050, -12.11044203135681840, 32.26167407432752299 ) ) ;
#75033=CARTESIAN_POINT ( 'NONE',  ( -0.7115384615384606759, -2.499999999999998668, 29.75000000000000355 ) ) ;
#75034=CARTESIAN_POINT ( 'NONE',  ( 0.7114839798866027243, -12.43552623307873972, 30.55307653245132826 ) ) ;
#75035=ORIENTED_EDGE ( 'NONE', *, *, #78900, .F. ) ;
#75036=VECTOR ( 'NONE', #55952, 1000.000000000000227 ) ;
#75037=CARTESIAN_POINT ( 'NONE',  ( -11.40767109749459074, -12.35292014791297710, 31.75344720912887198 ) ) ;
#75038=CARTESIAN_POINT ( 'NONE',  ( 1.161130460051055469, -4.225889041578353655, 33.85425143139329407 ) ) ;
#75039=CARTESIAN_POINT ( 'NONE',  ( -4.153846153846274980, -2.379036618888197729, 30.90682066428292885 ) ) ;
#75040=LINE ( 'NONE', #13327, #52936 ) ;
#75041=CARTESIAN_POINT ( 'NONE',  ( 8.835298102580845025, -9.905515769479276145, 34.41647553114623292 ) ) ;
#75042=EDGE_CURVE ( 'NONE', #68539, #76645, #18145, .T. ) ;
#75043=FACE_BOUND ( 'NONE', #59371, .T. ) ;
#75044=CARTESIAN_POINT ( 'NONE',  ( 5.869309396889694774, -4.684245665217972032, 34.18127051446801090 ) ) ;
#75045=CARTESIAN_POINT ( 'NONE',  ( 11.40831432902331954, -12.45813303252208648, 30.39737893381572675 ) ) ;
#75046=CARTESIAN_POINT ( 'NONE',  ( -15.23076923076935252, -5.094484230521993062, 34.41647553114689373 ) ) ;
#75047=DIRECTION ( 'NONE',  ( 0.000000000000000000, 0.3420201433256610524, 0.9396926207859113145 ) ) ;
#75048=CARTESIAN_POINT ( 'NONE',  ( -2.084912638714239819, -8.540255544307065350, 34.89611431652622286 ) ) ;
#75049=ADVANCED_FACE ( 'NONE', ( #79848 ), #61666, .F. ) ;
#75050=CARTESIAN_POINT ( 'NONE',  ( -10.61538461538461320, -6.343179335718451384, 34.87096338111211935 ) ) ;
#75052=VERTEX_POINT ( 'NONE', #4176 ) ;
#75053=CARTESIAN_POINT ( 'NONE',  ( 10.39189969082028853, -12.11044203135681840, 32.26167407432752299 ) ) ;
#75054=ORIENTED_EDGE ( 'NONE', *, *, #47084, .T. ) ;
#75055=CARTESIAN_POINT ( 'NONE',  ( 5.999999999999878320, -2.657715359629662988, 31.77849191805970364 ) ) ;
#75056=EDGE_CURVE ( 'NONE', #45617, #43520, #60624, .T. ) ;
#75057=VERTEX_POINT ( 'NONE', #86620 ) ;
#75058=ADVANCED_FACE ( 'NONE', ( #82409 ), #5071, .F. ) ;
#75059=CARTESIAN_POINT ( 'NONE',  ( -18.00000000000000000, -2.499999999999999556, 29.49999999999998579 ) ) ;
#75060=CARTESIAN_POINT ( 'NONE',  ( -1.384615384615383471, -10.51840700105979565, 33.73612834413961536 ) ) ;
#75061=CARTESIAN_POINT ( 'NONE',  ( -1.384615384615383471, -8.810774026931790459, 35.74407628777942847 ) ) ;
#75062=ORIENTED_EDGE ( 'NONE', *, *, #16516, .F. ) ;
#75063=CARTESIAN_POINT ( 'NONE',  ( -9.468880730446121774, -7.630147231320743018, 34.74852402298682819 ) ) ;
#75065=CARTESIAN_POINT ( 'NONE',  ( 4.284637961670939355, -10.54018710029568595, 33.71981072465678864 ) ) ;
#75068=CARTESIAN_POINT ( 'NONE',  ( 10.36540787133602670, -2.544273027872575366, 31.48422191005632342 ) ) ;
#75069=CARTESIAN_POINT ( 'NONE',  ( -12.33101302330481808, -8.630441415882550871, 34.87705825610312615 ) ) ;
#75070=CARTESIAN_POINT ( 'NONE',  ( -5.777220458731589403, -10.81320215134717344, 33.49497208177562868 ) ) ;
#75072=CARTESIAN_POINT ( 'NONE',  ( 14.08420736396836226, -5.912607949931405926, 34.49155766932282319 ) ) ;
#75073=ORIENTED_EDGE ( 'NONE', *, *, #6854, .T. ) ;
#75074=DIRECTION ( 'NONE',  ( 0.000000000000000000, 0.7660444431189807890, 0.6427876096865361433 ) ) ;
#75076=AXIS2_PLACEMENT_3D ( 'NONE', #78117, #31265, #58730 ) ;
#75077=CARTESIAN_POINT ( 'NONE',  ( -9.692307692307691624, -2.499999999999998668, 29.75000000000001421 ) ) ;
#75078=CARTESIAN_POINT ( 'NONE',  ( 5.326977496836529546, -6.523592122091591783, 34.90882529074906415 ) ) ;
#75079=AXIS2_PLACEMENT_3D ( 'NONE', #57362, #50602, #72200 ) ;
#75081=CARTESIAN_POINT ( 'NONE',  ( -9.692307692307691624, -13.95598074871891292, 31.83374038241031911 ) ) ;
#75082=CARTESIAN_POINT ( 'NONE',  ( -16.82697766754503377, -9.357781135181033605, 34.66075350412533851 ) ) ;
#75085=CYLINDRICAL_SURFACE ( 'NONE', #80029, 0.2500000000000012212 ) ;
#75086=CARTESIAN_POINT ( 'NONE',  ( -17.07692307692307665, -8.564572088678739092, 35.78748833219616898 ) ) ;
#75088=DIRECTION ( 'NONE',  ( -0.000000000000000000, -0.8660254037844399289, -0.4999999999999980016 ) ) ;
#75089=CARTESIAN_POINT ( 'NONE',  ( 2.242422307135989890, -4.320704448112771878, 33.92786785259540494 ) ) ;
#75090=EDGE_CURVE ( 'NONE', #46711, #19405, #48155, .T. ) ;
#75091=CARTESIAN_POINT ( 'NONE',  ( -13.60810032833933469, -11.89387501736622710, 32.13663884655806413 ) ) ;
#75092=CARTESIAN_POINT ( 'NONE',  ( -13.31854805126531005, -8.164416787775445883, 34.95778746994558617 ) ) ;
#75096=B_SPLINE_CURVE_WITH_KNOTS ( 'NONE', 3,
 ( #76462, #61604, #83674, #54855, #26948, #42240, #8002, #13862, #35021, #89108 ),
 .UNSPECIFIED., .F., .F.,
 ( 4, 2, 2, 2, 4 ),
 ( 0.0007817359430256314154, 0.0009771253907249980580, 0.001172514838424364592, 0.001367904286123731127, 0.001563293733823097661 ),
 .UNSPECIFIED. ) ;
#75097=ORIENTED_EDGE ( 'NONE', *, *, #66341, .T. ) ;
#75098=ADVANCED_FACE ( 'NONE', ( #3729 ), #27012, .F. ) ;
#75099=B_SPLINE_CURVE_WITH_KNOTS ( 'NONE', 3,
 ( #42275, #56218, #70619, #15243, #41828, #36395, #69297, #8484, #89143, #1266 ),
 .UNSPECIFIED., .F., .F.,
 ( 4, 2, 2, 2, 4 ),
 ( 0.000000000000000000, 0.0001954339857564071491, 0.0003908679715128142982, 0.0005863019572692214744, 0.0007817359430256285964 ),
 .UNSPECIFIED. ) ;
#75100=CARTESIAN_POINT ( 'NONE',  ( 12.71159288145191013, -10.06805714834173493, 34.32951233291982618 ) ) ;
#75101=CARTESIAN_POINT ( 'NONE',  ( -2.177166605928744669, -6.001044277235011215, 34.52024696741798948 ) ) ;
#75102=B_SPLINE_CURVE_WITH_KNOTS ( 'NONE', 3,
 ( #87284, #32760, #31882, #19253, #80060, #73767, #46719, #67000, #25561, #80517 ),
 .UNSPECIFIED., .F., .F.,
 ( 4, 2, 2, 2, 4 ),
 ( 0.0007817359430256294638, 0.0009771253907249950223, 0.001172514838424360472, 0.001367904286123725922, 0.001563293733823091372 ),
 .UNSPECIFIED. ) ;
#75103=DIRECTION ( 'NONE',  ( 0.000000000000000000, 0.8660254037844377084, 0.5000000000000015543 ) ) ;
#75104=CYLINDRICAL_SURFACE ( 'NONE', #71115, 0.2500000000000009437 ) ;
#75105=EDGE_CURVE ( 'NONE', #11909, #22486, #63809, .T. ) ;
#75106=CARTESIAN_POINT ( 'NONE',  ( -16.85414353565466072, -5.114059244376869096, 34.14424750095245287 ) ) ;
#75107=VECTOR ( 'NONE', #3127, 1000.000000000000227 ) ;
#75108=ORIENTED_EDGE ( 'NONE', *, *, #58552, .F. ) ;
#75110=ORIENTED_EDGE ( 'NONE', *, *, #82028, .T. ) ;
#75111=DIRECTION ( 'NONE',  ( 0.000000000000000000, 0.1736481776669267785, -0.9848077530122087975 ) ) ;
#75112=ORIENTED_EDGE ( 'NONE', *, *, #38708, .F. ) ;
#75113=CARTESIAN_POINT ( 'NONE',  ( -1.607542343522233130, -2.889293201056495786, 32.26117774369186009 ) ) ;
#75114=AXIS2_PLACEMENT_3D ( 'NONE', #3059, #35982, #53019 ) ;
#75115=CARTESIAN_POINT ( 'NONE',  ( -10.86538461538461320, -7.566083408709835645, 34.74999999999999289 ) ) ;
#75116=EDGE_CURVE ( 'NONE', #68374, #27164, #88579, .T. ) ;
#75117=CARTESIAN_POINT ( 'NONE',  ( -12.21159294319031829, -12.22109172314383052, 31.39792113162168263 ) ) ;
#75118=DIRECTION ( 'NONE',  ( -0.000000000000000000, -0.3420201433256694901, -0.9396926207859082059 ) ) ;
#75119=ORIENTED_EDGE ( 'NONE', *, *, #71210, .F. ) ;
#75120=EDGE_CURVE ( 'NONE', #19030, #35799, #35910, .T. ) ;
#75122=EDGE_LOOP ( 'NONE', ( #11662, #6570 ) ) ;
#75123=CYLINDRICAL_SURFACE ( 'NONE', #63423, 0.2499999999999986955 ) ;
#75124=DIRECTION ( 'NONE',  ( 0.000000000000000000, 0.1736481776669267785, -0.9848077530122087975 ) ) ;
#75125=ORIENTED_EDGE ( 'NONE', *, *, #52717, .F. ) ;
#75126=CARTESIAN_POINT ( 'NONE',  ( 3.230769230769231726, -1.367168528481310208, 33.57946703557072254 ) ) ;
#75127=DIRECTION ( 'NONE',  ( 0.000000000000000000, 0.9848077530122072432, 0.1736481776669354937 ) ) ;
#75129=EDGE_CURVE ( 'NONE', #86522, #2169, #21862, .T. ) ;
#75130=CARTESIAN_POINT ( 'NONE',  ( 11.53846153846141753, -11.48612834414049644, 32.76840700105863391 ) ) ;
#75131=CARTESIAN_POINT ( 'NONE',  ( 0.4615384615383382183, -9.528491918059723176, 34.59228464037033035 ) ) ;
#75132=FACE_BOUND ( 'NONE', #20548, .T. ) ;
#75133=B_SPLINE_CURVE_WITH_KNOTS ( 'NONE', 3,
 ( #27431, #82383, #7160, #405, #27869, #82827, #69306, #21099, #48571, #76052 ),
 .UNSPECIFIED., .F., .F.,
 ( 4, 2, 2, 2, 4 ),
 ( 0.0007817359430256371616, 0.0009771253907250049969, 0.001172514838424373049, 0.001367904286123741101, 0.001563293733823108937 ),
 .UNSPECIFIED. ) ;
#75134=DIRECTION ( 'NONE',  ( -0.000000000000000000, -0.9848077530122086864, -0.1736481776669273613 ) ) ;
#75135=CARTESIAN_POINT ( 'NONE',  ( -6.249976744048590938, -12.41104346484419452, 31.60698883733904196 ) ) ;
#75137=CARTESIAN_POINT ( 'NONE',  ( -2.307692307692305711, -9.584722331328613620, 36.20867863119891439 ) ) ;
#75138=CARTESIAN_POINT ( 'NONE',  ( 0.3954560821783252855, -6.343179335718452272, 34.87096338111211935 ) ) ;
#75139=CARTESIAN_POINT ( 'NONE',  ( 5.010839665967194989, -3.050289026998445951, 32.03036669348365706 ) ) ;
#75140=VECTOR ( 'NONE', #53716, 999.9999999999998863 ) ;
#75141=DIRECTION ( 'NONE',  ( -0.000000000000000000, 0.9848077530122085754, -0.1736481776669273613 ) ) ;
#75142=CARTESIAN_POINT ( 'NONE',  ( -0.5916856709766840083, -3.817052484675422797, 33.13202310037935661 ) ) ;
#75144=CARTESIAN_POINT ( 'NONE',  ( -2.557715531913761886, -4.175268141568689195, 33.81360843649122216 ) ) ;
#75145=CARTESIAN_POINT ( 'NONE',  ( 13.16178869213638336, -7.369208160676172348, 34.74850200257122879 ) ) ;
#75146=ORIENTED_EDGE ( 'NONE', *, *, #31901, .F. ) ;
#75148=CARTESIAN_POINT ( 'NONE',  ( -13.60810030917971858, -4.988325925672468131, 34.36044203135681130 ) ) ;
#75149=CARTESIAN_POINT ( 'NONE',  ( -4.283994123577846480, -3.625366637846544560, 33.29286588640298561 ) ) ;
#75150=VERTEX_POINT ( 'NONE', #21575 ) ;
#75151=DIRECTION ( 'NONE',  ( -0.000000000000000000, -0.5000000000000009992, -0.8660254037844380415 ) ) ;
#75152=CARTESIAN_POINT ( 'NONE',  ( -15.16551409125639260, -12.70778746994558439, 30.41441678777536595 ) ) ;
#75153=EDGE_CURVE ( 'NONE', #4983, #44386, #52015, .T. ) ;
#75154=FACE_BOUND ( 'NONE', #29647, .T. ) ;
#75155=CARTESIAN_POINT ( 'NONE',  ( -14.30769230769242917, -4.320704448113951379, 33.92786785259630022 ) ) ;
#75156=CARTESIAN_POINT ( 'NONE',  ( -4.153846153846152411, -8.120952969808772792, 34.71129190930000163 ) ) ;
#75157=CARTESIAN_POINT ( 'NONE',  ( 10.48469314871705826, -8.147922237126337563, 34.70805685702651999 ) ) ;
#75158=CARTESIAN_POINT ( 'NONE',  ( -3.230769230769351186, -2.892918686052166066, 31.69288490824153470 ) ) ;
#75159=CARTESIAN_POINT ( 'NONE',  ( -8.769230769230768274, -12.10708131394839349, 31.69288490824020244 ) ) ;
#75161=EDGE_LOOP ( 'NONE', ( #51836, #36348 ) ) ;
#75162=EDGE_CURVE ( 'NONE', #16008, #40783, #76753, .T. ) ;
#75163=ORIENTED_EDGE ( 'NONE', *, *, #73207, .T. ) ;
#75164=LINE ( 'NONE', #13447, #3272 ) ;
#75165=EDGE_CURVE ( 'NONE', #65590, #66285, #15499, .T. ) ;
#75166=CARTESIAN_POINT ( 'NONE',  ( -0.6850234052624077918, -2.847400154188067578, 31.58180166144859768 ) ) ;
#75167=CARTESIAN_POINT ( 'NONE',  ( 7.053915253563681986, -7.277220318596959281, 34.99547417642776992 ) ) ;
#75168=CARTESIAN_POINT ( 'NONE',  ( 17.14211606521772779, -2.255955759149236073, 29.99999999999988276 ) ) ;
#75169=CARTESIAN_POINT ( 'NONE',  ( -3.361460697436789324, -5.582088688514999397, 34.36776431015576350 ) ) ;
#75171=CARTESIAN_POINT ( 'NONE',  ( -12.68446542044531000, -4.026226216239094491, 33.68668979543634379 ) ) ;
#75172=CARTESIAN_POINT ( 'NONE',  ( 1.318533005255250856, -9.905515769479276145, 34.41647553114623292 ) ) ;
#75173=DIRECTION ( 'NONE',  ( -0.000000000000000000, 1.000000000000000000, 3.491481338843133355E-15 ) ) ;
#75174=CARTESIAN_POINT ( 'NONE',  ( -1.319470603895752214, -7.750023224968865421, 34.99404313364389907 ) ) ;
#75175=CARTESIAN_POINT ( 'NONE',  ( -4.153846153846274980, -12.51329471203414379, 31.30864560766407578 ) ) ;
#75176=CARTESIAN_POINT ( 'NONE',  ( 15.00784227186237985, -12.38737895849757820, 31.66785238281580206 ) ) ;
#75177=VECTOR ( 'NONE', #13011, 1000.000000000000227 ) ;
#75178=CARTESIAN_POINT ( 'NONE',  ( 7.173022332454968009, -3.520799739797213501, 33.17531984108286025 ) ) ;
#75179=CARTESIAN_POINT ( 'NONE',  ( -3.361460697436789324, -8.147922237126337563, 34.70805685702651999 ) ) ;
#75180=CARTESIAN_POINT ( 'NONE',  ( 12.71148397988660506, -2.824170634883621744, 31.52227843825338738 ) ) ;
#75182=VERTEX_POINT ( 'NONE', #27283 ) ;
#75183=FACE_OUTER_BOUND ( 'NONE', #59167, .T. ) ;
#75184=CARTESIAN_POINT ( 'NONE',  ( -17.20707104665477161, -6.809168938359901446, 34.95455904226513866 ) ) ;
#75187=CARTESIAN_POINT ( 'NONE',  ( -18.00000000000012079, -10.90142922262034020, 33.41473453929536674 ) ) ;
#75188=EDGE_CURVE ( 'NONE', #79961, #13301, #5752, .T. ) ;
#75189=CARTESIAN_POINT ( 'NONE',  ( -11.31544869436814338, -4.762714258010881885, 34.23016756924214832 ) ) ;
#75190=CARTESIAN_POINT ( 'NONE',  ( -9.442253380669374252, -4.943051570960394159, 34.04725096376909477 ) ) ;
#75191=ORIENTED_EDGE ( 'NONE', *, *, #15242, .T. ) ;
#75194=ORIENTED_EDGE ( 'NONE', *, *, #33479, .F. ) ;
#75195=CARTESIAN_POINT ( 'NONE',  ( 11.66898697669518548, -9.503571793651731880, 34.60286762892837942 ) ) ;
#75196=CARTESIAN_POINT ( 'NONE',  ( -10.61538461538461320, -13.37000171582298513, 34.34916445242398453 ) ) ;
#75197=ORIENTED_EDGE ( 'NONE', *, *, #30674, .F. ) ;
#75200=CARTESIAN_POINT ( 'NONE',  ( -16.40384615384615330, -7.566083408709835645, 34.74999999999999289 ) ) ;
#75201=DIRECTION ( 'NONE',  ( -1.000000000000000000, 0.000000000000000000, 0.000000000000000000 ) ) ;
#75202=ORIENTED_EDGE ( 'NONE', *, *, #53054, .T. ) ;
#75204=DIRECTION ( 'NONE',  ( -0.000000000000000000, -0.000000000000000000, -1.000000000000000000 ) ) ;
#75205=EDGE_CURVE ( 'NONE', #48154, #35110, #20086, .T. ) ;
#75206=AXIS2_PLACEMENT_3D ( 'NONE', #76467, #42245, #89114 ) ;
#75207=ORIENTED_EDGE ( 'NONE', *, *, #174, .F. ) ;
#75209=CARTESIAN_POINT ( 'NONE',  ( 7.846153846153846700, -9.058645607665452459, 34.76329471203371924 ) ) ;
#75210=CARTESIAN_POINT ( 'NONE',  ( -9.442362173959551797, -10.05730279482229683, 34.04704008940765902 ) ) ;
#75211=CARTESIAN_POINT ( 'NONE',  ( 9.562159722576001997, -9.504002272028875709, 34.60269587691767867 ) ) ;
#75212=CARTESIAN_POINT ( 'NONE',  ( -2.437839517130527156, -6.001485441113818986, 34.52039167877662607 ) ) ;
#75213=CARTESIAN_POINT ( 'NONE',  ( -0.3954711281883860896, -5.471508081941601098, 34.59228464037088457 ) ) ;
#75214=CARTESIAN_POINT ( 'NONE',  ( 4.153846153846154188, -3.886160181151819604, 36.00935417666054406 ) ) ;
#75215=EDGE_CURVE ( 'NONE', #32628, #31103, #29369, .T. ) ;
#75216=CARTESIAN_POINT ( 'NONE',  ( 10.36540788444226102, -12.17611988154120972, 31.52148481390971213 ) ) ;
#75217=ORIENTED_EDGE ( 'NONE', *, *, #21722, .T. ) ;
#75218=EDGE_CURVE ( 'NONE', #85395, #82613, #81796, .T. ) ;
#75219=ORIENTED_EDGE ( 'NONE', *, *, #40228, .T. ) ;
#75222=CARTESIAN_POINT ( 'NONE',  ( -2.307692307692305711, -13.49023893513002648, 31.06009739812518688 ) ) ;
#75223=CARTESIAN_POINT ( 'NONE',  ( 9.442330961365339448, -4.943428324936578910, 34.04746400365624481 ) ) ;
#75225=EDGE_CURVE ( 'NONE', #31195, #10433, #58370, .T. ) ;
#75226=CARTESIAN_POINT ( 'NONE',  ( 14.37375964104238513, -11.91647553114624358, 32.58852847137148245 ) ) ;
#75227=EDGE_CURVE ( 'NONE', #52135, #45323, #33674, .T. ) ;
#75230=CARTESIAN_POINT ( 'NONE',  ( -9.692307692307691624, -2.249999999999998668, 29.75000000000001776 ) ) ;
#75232=AXIS2_PLACEMENT_3D ( 'NONE', #56768, #51305, #3592 ) ;
#75233=CARTESIAN_POINT ( 'NONE',  ( -12.71156168575991785, -3.520140089381495585, 33.17453946501458262 ) ) ;
#75234=ORIENTED_EDGE ( 'NONE', *, *, #54680, .T. ) ;
#75235=CARTESIAN_POINT ( 'NONE',  ( -12.23875879256039489, -10.23759521482555357, 34.22997729860117033 ) ) ;
#75236=CARTESIAN_POINT ( 'NONE',  ( 10.68145296638705410, -4.786620604624113540, 33.94971097300155805 ) ) ;
#75237=FACE_BOUND ( 'NONE', #32659, .T. ) ;
#75238=DIRECTION ( 'NONE',  ( -0.000000000000000000, 0.9396926207859092051, -0.3420201433256662704 ) ) ;
#75239=CARTESIAN_POINT ( 'NONE',  ( 13.38461538461538680, -5.557115091759785130, 34.35708131394839171 ) ) ;
#75240=DIRECTION ( 'NONE',  ( 0.000000000000000000, -6.938893903907222067E-15, 1.000000000000000000 ) ) ;
#75241=CARTESIAN_POINT ( 'NONE',  ( 1.161688425708537808, -12.38737895849757820, 31.66785238281580206 ) ) ;
#75242=CYLINDRICAL_SURFACE ( 'NONE', #56788, 0.2499999999999997502 ) ;
#75243=CARTESIAN_POINT ( 'NONE',  ( -7.911423846710166075, -9.528491918058357157, 34.59228464037090589 ) ) ;
#75244=CARTESIAN_POINT ( 'NONE',  ( 10.54930120442873331, -9.780366693483667717, 34.19971097300155805 ) ) ;
#75245=ORIENTED_EDGE ( 'NONE', *, *, #3526, .F. ) ;
#75246=ORIENTED_EDGE ( 'NONE', *, *, #35544, .F. ) ;
#75247=CARTESIAN_POINT ( 'NONE',  ( 2.177000841024752553, -10.54014554554150607, 33.71984207302941883 ) ) ;
#75248=CARTESIAN_POINT ( 'NONE',  ( 2.372947878968333146, -10.90142922261932057, 33.41473453929631887 ) ) ;
#75249=CARTESIAN_POINT ( 'NONE',  ( -12.52762187249434156, -2.538708090699994813, 30.37095296980875148 ) ) ;
#75252=CARTESIAN_POINT ( 'NONE',  ( -9.692307692307691624, -4.786620604624113540, 33.94971097300155094 ) ) ;
#75253=VERTEX_POINT ( 'NONE', #6130 ) ;
#75254=CARTESIAN_POINT ( 'NONE',  ( 17.29993442853592001, -3.105924265160262099, 32.13625925475356127 ) ) ;
#75255=CARTESIAN_POINT ( 'NONE',  ( 14.24160889673642849, -11.16473453929635440, 33.15142922261925662 ) ) ;
#75256=LINE ( 'NONE', #43669, #70348 ) ;
#75257=CARTESIAN_POINT ( 'NONE',  ( -16.08777882049608010, -3.937682226553329556, 33.60647404775216529 ) ) ;
#75259=ORIENTED_EDGE ( 'NONE', *, *, #78997, .F. ) ;
#75260=CIRCLE ( 'NONE', #26336, 2.000000000000001776 ) ;
#75261=EDGE_CURVE ( 'NONE', #76326, #36624, #61066, .T. ) ;
#75262=VERTEX_POINT ( 'NONE', #56530 ) ;
#75264=CARTESIAN_POINT ( 'NONE',  ( 0.3957816590241516885, -7.249945686854186278, 34.74374336980224598 ) ) ;
#75265=EDGE_CURVE ( 'NONE', #28353, #57222, #35368, .T. ) ;
#75268=CARTESIAN_POINT ( 'NONE',  ( -5.326899807865429715, -2.779195860258147022, 31.39871582349836743 ) ) ;
#75269=CARTESIAN_POINT ( 'NONE',  ( 4.853996859406927378, -6.503392248772476236, 34.64988816332204635 ) ) ;
#75270=CARTESIAN_POINT ( 'NONE',  ( -17.20761368003338632, -9.084618155246140248, 34.75535874321725771 ) ) ;
#75272=EDGE_LOOP ( 'NONE', ( #6144, #33075, #83059, #3373 ) ) ;
#75274=CYLINDRICAL_SURFACE ( 'NONE', #22794, 0.2499999999999995559 ) ;
#75275=CARTESIAN_POINT ( 'NONE',  ( -16.21992956480203674, -11.69971097300155272, 32.46337939537587403 ) ) ;
#75276=ORIENTED_EDGE ( 'NONE', *, *, #76048, .T. ) ;
#75278=CARTESIAN_POINT ( 'NONE',  ( 13.38461538461538680, -12.29105614889573062, 35.45975837776705220 ) ) ;
#75279=CARTESIAN_POINT ( 'NONE',  ( 1.134615384615387468, -7.566083408709834757, 34.74999999999999289 ) ) ;
#75280=CARTESIAN_POINT ( 'NONE',  ( -16.08870137312652560, -7.750023224968867197, 34.99404313364389907 ) ) ;
#75281=CARTESIAN_POINT ( 'NONE',  ( -17.75005459062195712, -10.92531984108285670, 33.72920026020278073 ) ) ;
#75282=CARTESIAN_POINT ( 'NONE',  ( -15.23076923076922995, -3.322132147404559976, 32.92929555188717927 ) ) ;
#75284=ADVANCED_FACE ( 'NONE', ( #62822 ), #34920, .F. ) ;
#75286=EDGE_LOOP ( 'NONE', ( #71696, #20599 ) ) ;
#75287=CARTESIAN_POINT ( 'NONE',  ( 11.76147289007438346, -2.758310577978208666, 31.33698337089302299 ) ) ;
#75288=CARTESIAN_POINT ( 'NONE',  ( 12.59232890250541281, -4.684288915650983043, 34.18129842949671371 ) ) ;
#75289=CARTESIAN_POINT ( 'NONE',  ( 9.822833130541336999, -11.04252011169590020, 33.62494198852677130 ) ) ;
#75290=CARTESIAN_POINT ( 'NONE',  ( -13.13466986626724342, -8.433404298154334455, 34.66254593164985920 ) ) ;
#75292=CARTESIAN_POINT ( 'NONE',  ( -5.933931648997559982, -2.538708090699994813, 30.37095296980875503 ) ) ;
#75293=CARTESIAN_POINT ( 'NONE',  ( 11.28843831424008393, -12.68155406624981119, 30.59749803192733708 ) ) ;
#75294=CARTESIAN_POINT ( 'NONE',  ( 2.530471976670372936, -10.97394488606064122, 33.68653795673694873 ) ) ;
#75296=CARTESIAN_POINT ( 'NONE',  ( -14.30769230769230660, -6.386643153685126251, 34.62446782046654192 ) ) ;
#75298=CYLINDRICAL_SURFACE ( 'NONE', #66698, 0.2499999999999994726 ) ;
#75299=VERTEX_POINT ( 'NONE', #21856 ) ;
#75300=CARTESIAN_POINT ( 'NONE',  ( -16.21911615440247090, -6.835583212224499938, 34.95778746994557906 ) ) ;
#75301=CARTESIAN_POINT ( 'NONE',  ( 3.230769230769110045, -12.27809138561165270, 31.22303859784587132 ) ) ;
#75302=CARTESIAN_POINT ( 'NONE',  ( -14.43816749276802724, -7.276987145209185215, 34.99546412871779211 ) ) ;
#75303=ORIENTED_EDGE ( 'NONE', *, *, #63537, .F. ) ;
#75304=CARTESIAN_POINT ( 'NONE',  ( 9.442307692307693401, -7.500000000000001776, 35.00000000000000000 ) ) ;
#75305=B_SPLINE_CURVE_WITH_KNOTS ( 'NONE', 3,
 ( #76487, #388, #49009, #27852, #42267, #824, #55759, #21535, #21984, #83247 ),
 .UNSPECIFIED., .F., .F.,
 ( 4, 2, 2, 2, 4 ),
 ( 0.0007817246256747507503, 0.0009771112852218959231, 0.001172497944769040987, 0.001367884604316186052, 0.001563271263863331116 ),
 .UNSPECIFIED. ) ;
#75306=EDGE_CURVE ( 'NONE', #85662, #15420, #49765, .T. ) ;
#75307=ORIENTED_EDGE ( 'NONE', *, *, #11568, .F. ) ;
#75308=CARTESIAN_POINT ( 'NONE',  ( -2.307692307692427391, -12.27809138561165270, 31.22303859784587132 ) ) ;
#75309=CARTESIAN_POINT ( 'NONE',  ( -5.999999999999998224, -11.91647553114624181, 32.58852847137148245 ) ) ;
#75310=EDGE_LOOP ( 'NONE', ( #10521, #16893 ) ) ;
#75311=CARTESIAN_POINT ( 'NONE',  ( 7.623227628637698317, -12.15238873228292071, 31.58232369045353849 ) ) ;
#75312=CARTESIAN_POINT ( 'NONE',  ( -14.37377468705244254, -2.292212530054419606, 30.41441678777542634 ) ) ;
#75313=CARTESIAN_POINT ( 'NONE',  ( 13.31934493865461278, -6.879047030191174805, 34.71129190930000163 ) ) ;
#75314=ADVANCED_FACE ( 'NONE', ( #70933 ), #22735, .F. ) ;
#75315=DIRECTION ( 'NONE',  ( 0.000000000000000000, 0.3420201433256641055, -0.9396926207859100932 ) ) ;
#75316=CARTESIAN_POINT ( 'NONE',  ( 3.361294932532794100, -12.45806712695776319, 30.39783852428763922 ) ) ;
#75318=EDGE_LOOP ( 'NONE', ( #48226, #25895, #28202, #9514 ) ) ;
#75319=EDGE_CURVE ( 'NONE', #89081, #48963, #13263, .T. ) ;
#75320=FACE_BOUND ( 'NONE', #22154, .T. ) ;
#75321=ORIENTED_EDGE ( 'NONE', *, *, #24673, .F. ) ;
#75322=LINE ( 'NONE', #14496, #12723 ) ;
#75326=CARTESIAN_POINT ( 'NONE',  ( -6.065270445960774914, -12.27809138561121394, 31.22303859784730307 ) ) ;
#75328=B_SPLINE_CURVE_WITH_KNOTS ( 'NONE', 3,
 ( #89119, #48990, #47664, #6675, #42249, #69267, #69705, #75149, #13873, #13434 ),
 .UNSPECIFIED., .F., .F.,
 ( 4, 2, 2, 2, 4 ),
 ( 0.000000000000000000, 0.0001954311564186861155, 0.0003908623128373722310, 0.0005862934692560583735, 0.0007817246256747444619 ),
 .UNSPECIFIED. ) ;
#75329=VERTEX_POINT ( 'NONE', #43018 ) ;
#75330=VERTEX_POINT ( 'NONE', #8797 ) ;
#75331=ORIENTED_EDGE ( 'NONE', *, *, #44605, .F. ) ;
#75332=CARTESIAN_POINT ( 'NONE',  ( 6.923076923076802558, -9.442884908241554243, 34.35708131394783038 ) ) ;
#75333=EDGE_CURVE ( 'NONE', #39715, #12402, #27290, .T. ) ;
#75334=EDGE_CURVE ( 'NONE', #77192, #820, #22981, .T. ) ;
#75335=VERTEX_POINT ( 'NONE', #12202 ) ;
#75336=CARTESIAN_POINT ( 'NONE',  ( 4.219101293358989757, -10.33852847137154107, 34.16647553114620450 ) ) ;
#75337=CARTESIAN_POINT ( 'NONE',  ( -9.942307692307691624, -7.500000000000001776, 34.75000000000000000 ) ) ;
#75338=ADVANCED_FACE ( 'NONE', ( #18516 ), #86543, .F. ) ;
#75339=CYLINDRICAL_SURFACE ( 'NONE', #35677, 0.2500000000000008882 ) ;
#75340=CARTESIAN_POINT ( 'NONE',  ( 3.930980731642515380, -2.501496062324911840, 29.88072118266895671 ) ) ;
#75342=CARTESIAN_POINT ( 'NONE',  ( -4.403846153846151523, -2.249999999999998668, 29.75000000000000355 ) ) ;
#75343=CARTESIAN_POINT ( 'NONE',  ( -2.057637996053991447, -3.627508038966689163, 32.91356715214248396 ) ) ;
#75346=ORIENTED_EDGE ( 'NONE', *, *, #41781, .T. ) ;
#75347=ORIENTED_EDGE ( 'NONE', *, *, #51547, .T. ) ;
#75348=LINE ( 'NONE', #40684, #60355 ) ;
#75349=AXIS2_PLACEMENT_3D ( 'NONE', #9009, #13982, #36475 ) ;
#75350=CARTESIAN_POINT ( 'NONE',  ( -1.515305987725689363, -2.494641256782728966, 31.33461815524612959 ) ) ;
#75351=CARTESIAN_POINT ( 'NONE',  ( -7.780086512803769949, -9.058645607665452459, 34.76329471203371924 ) ) ;
#75353=CARTESIAN_POINT ( 'NONE',  ( -10.61538461538461320, -3.513871655860378418, 32.76840700105978499 ) ) ;
#75354=FACE_BOUND ( 'NONE', #23438, .T. ) ;
#75355=LINE ( 'NONE', #83452, #36054 ) ;
#75356=ORIENTED_EDGE ( 'NONE', *, *, #33341, .T. ) ;
#75359=CARTESIAN_POINT ( 'NONE',  ( 3.100622021331010725, -10.88202310037936194, 33.43294751532457099 ) ) ;
#75360=VERTEX_POINT ( 'NONE', #24362 ) ;
#75361=DIRECTION ( 'NONE',  ( -0.000000000000000000, 0.3420201433256694346, -0.9396926207859080948 ) ) ;
#75362=ORIENTED_EDGE ( 'NONE', *, *, #71381, .T. ) ;
#75363=FACE_BOUND ( 'NONE', #53462, .T. ) ;
#75364=ADVANCED_FACE ( 'NONE', ( #46865 ), #80673, .F. ) ;
#75365=DIRECTION ( 'NONE',  ( -0.000000000000000000, 0.8660254037844397068, -0.4999999999999978906 ) ) ;
#75366=CARTESIAN_POINT ( 'NONE',  ( -5.749999999998562927, -7.500000000000155431, 34.75000000000007105 ) ) ;
#75367=CARTESIAN_POINT ( 'NONE',  ( 16.82694633287448838, -12.01397095200673881, 32.43157075238190146 ) ) ;
#75368=ORIENTED_EDGE ( 'NONE', *, *, #87885, .T. ) ;
#75369=CARTESIAN_POINT ( 'NONE',  ( 6.923076923076802558, -10.21337939537710326, 33.94971097300076224 ) ) ;
#75370=LINE ( 'NONE', #150, #34214 ) ;
#75371=CARTESIAN_POINT ( 'NONE',  ( -7.846153846153844924, -2.499999999999998668, 29.50000000000001066 ) ) ;
#75372=CARTESIAN_POINT ( 'NONE',  ( 14.30769230769231015, -12.48256725967547354, 35.29906147534542527 ) ) ;
#75373=VERTEX_POINT ( 'NONE', #59934 ) ;
#75374=FACE_OUTER_BOUND ( 'NONE', #33820, .T. ) ;
#75375=CARTESIAN_POINT ( 'NONE',  ( -15.29603967673000575, -4.481592998940162609, 33.73612834413957984 ) ) ;
#75377=ORIENTED_EDGE ( 'NONE', *, *, #25033, .F. ) ;
#75378=CARTESIAN_POINT ( 'NONE',  ( -7.846153846153965716, -11.94971097300221174, 32.03036669348237098 ) ) ;
#75379=CARTESIAN_POINT ( 'NONE',  ( -5.076923076923199218, -11.67786785259630911, 32.92929555188603530 ) ) ;
#75380=CARTESIAN_POINT ( 'NONE',  ( 7.846153846153846700, -2.721908614388771852, 31.22303859784724978 ) ) ;
#75381=CARTESIAN_POINT ( 'NONE',  ( 14.08420736396836226, -9.331801661448606566, 34.40259984581193464 ) ) ;
#75382=CARTESIAN_POINT ( 'NONE',  ( 15.00784227186238162, -5.582147617184174848, 34.63737895849758530 ) ) ;
#75385=DIRECTION ( 'NONE',  ( -0.000000000000000000, -0.3420201433256694901, -0.9396926207859082059 ) ) ;
#75386=CARTESIAN_POINT ( 'NONE',  ( -12.46153846153846168, -11.16473453929635440, 33.15142922261926373 ) ) ;
#75388=ORIENTED_EDGE ( 'NONE', *, *, #50318, .F. ) ;
#75389=CARTESIAN_POINT ( 'NONE',  ( -9.692307692307691624, -1.242168528481310874, 33.36296068462461051 ) ) ;
#75390=EDGE_LOOP ( 'NONE', ( #84160, #28702 ) ) ;
#75392=ORIENTED_EDGE ( 'NONE', *, *, #56819, .F. ) ;
#75393=CARTESIAN_POINT ( 'NONE',  ( -8.519285359852727169, -6.653508905675592722, 34.93172785388651391 ) ) ;
#75394=VERTEX_POINT ( 'NONE', #39237 ) ;
#75395=CARTESIAN_POINT ( 'NONE',  ( -5.207071046654775159, -11.66186481527757479, 32.95055677023626117 ) ) ;
#75397=CARTESIAN_POINT ( 'NONE',  ( 14.43821800945587341, -11.46989282347013095, 32.79007818306219946 ) ) ;
#75398=CARTESIAN_POINT ( 'NONE',  ( 9.692307692307695177, -4.098570777380720287, 33.41473453929634729 ) ) ;
#75399=B_SPLINE_CURVE_WITH_KNOTS ( 'NONE', 3,
 ( #52492, #50708, #25025, #58352, #17836, #45742, #72763, #59255, #2967, #3858 ),
 .UNSPECIFIED., .F., .F.,
 ( 4, 2, 2, 2, 4 ),
 ( 0.000000000000000000, 0.0001954311564186861697, 0.0003908623128373723394, 0.0005862934692560584820, 0.0007817246256747446788 ),
 .UNSPECIFIED. ) ;
#75400=CARTESIAN_POINT ( 'NONE',  ( -16.02305434602136103, -5.582136614379148654, 34.36778462344220486 ) ) ;
#75401=FACE_OUTER_BOUND ( 'NONE', #18347, .T. ) ;
#75402=CARTESIAN_POINT ( 'NONE',  ( -13.44988583057615905, -2.625532179533444754, 30.86335684631481513 ) ) ;
#75403=CARTESIAN_POINT ( 'NONE',  ( 2.084207363968360038, -10.11188796281391511, 34.01382737946119050 ) ) ;
#75404=EDGE_CURVE ( 'NONE', #9579, #67350, #54162, .T. ) ;
#75407=CARTESIAN_POINT ( 'NONE',  ( -16.85414340794500276, -10.97394488606063589, 33.68653795673696294 ) ) ;
#75408=CARTESIAN_POINT ( 'NONE',  ( 7.846153846153723244, -5.941354392335915335, 34.76329471203413846 ) ) ;
#75409=EDGE_LOOP ( 'NONE', ( #18912, #78551 ) ) ;
#75411=CARTESIAN_POINT ( 'NONE',  ( 12.59232890250541281, -2.494656445102012565, 31.33466734024120015 ) ) ;
#75412=DIRECTION ( 'NONE',  ( 0.000000000000000000, 0.8660254037844377084, -0.5000000000000015543 ) ) ;
#75413=CYLINDRICAL_SURFACE ( 'NONE', #62726, 0.2499999999999997502 ) ;
#75414=CARTESIAN_POINT ( 'NONE',  ( -11.28846153846147615, -7.434744429011176159, 34.75000000000000711 ) ) ;
#75416=EDGE_CURVE ( 'NONE', #33135, #60496, #28416, .T. ) ;
#75419=AXIS2_PLACEMENT_3D ( 'NONE', #32168, #79467, #65037 ) ;
#75421=EDGE_CURVE ( 'NONE', #9134, #7438, #55199, .T. ) ;
#75422=ORIENTED_EDGE ( 'NONE', *, *, #38720, .F. ) ;
#75424=ORIENTED_EDGE ( 'NONE', *, *, #14946, .T. ) ;
#75425=DIRECTION ( 'NONE',  ( -0.000000000000000000, 1.000000000000000000, 3.491481338843133355E-15 ) ) ;
#75426=DIRECTION ( 'NONE',  ( -0.000000000000000000, 1.000000000000000000, 3.491481338843133355E-15 ) ) ;
#75427=B_SPLINE_CURVE_WITH_KNOTS ( 'NONE', 3,
 ( #84800, #16323, #78021, #44658, #66281, #3244, #64938, #43788, #78455, #37926 ),
 .UNSPECIFIED., .F., .F.,
 ( 4, 2, 2, 2, 4 ),
 ( 0.0007817359430256304396, 0.0009771253907249963233, 0.001172514838424362424, 0.001367904286123728524, 0.001563293733823094408 ),
 .UNSPECIFIED. ) ;
#75428=CARTESIAN_POINT ( 'NONE',  ( -4.219116599806928214, -4.481592998940161721, 33.73612834413957984 ) ) ;
#75429=CARTESIAN_POINT ( 'NONE',  ( -15.36146069743679199, -3.062553014421049546, 32.05460306192773601 ) ) ;
#75430=DIRECTION ( 'NONE',  ( -0.000000000000000000, 0.5000000000000011102, -0.8660254037844380415 ) ) ;
#75431=ORIENTED_EDGE ( 'NONE', *, *, #38078, .F. ) ;
#75433=EDGE_CURVE ( 'NONE', #26886, #31211, #65793, .T. ) ;
#75434=EDGE_LOOP ( 'NONE', ( #63368, #53753, #30326, #72422 ) ) ;
#75435=ORIENTED_EDGE ( 'NONE', *, *, #52633, .F. ) ;
#75436=VECTOR ( 'NONE', #39692, 1000.000000000000000 ) ;
#75437=FACE_OUTER_BOUND ( 'NONE', #17547, .T. ) ;
#75438=FACE_OUTER_BOUND ( 'NONE', #19324, .T. ) ;
#75439=CARTESIAN_POINT ( 'NONE',  ( 14.17754433796061342, -2.647304123082328875, 31.75400227202885972 ) ) ;
#75442=CARTESIAN_POINT ( 'NONE',  ( 16.21910172512217585, -10.21337939537593797, 33.94971097300152252 ) ) ;
#75443=CARTESIAN_POINT ( 'NONE',  ( -14.98071481085577972, -9.233818618650603938, 34.70587769442853698 ) ) ;
#75444=CARTESIAN_POINT ( 'NONE',  ( 14.24160889673642849, -12.37446782046654192, 30.86335684631486487 ) ) ;
#75445=VERTEX_POINT ( 'NONE', #31122 ) ;
#75446=EDGE_LOOP ( 'NONE', ( #60151, #24914, #32376, #57584 ) ) ;
#75447=EDGE_LOOP ( 'NONE', ( #66723, #27897, #87335, #71959 ) ) ;
#75448=CARTESIAN_POINT ( 'NONE',  ( -3.361459833879536507, -2.494641256782728966, 31.33461815524612959 ) ) ;
#75449=ORIENTED_EDGE ( 'NONE', *, *, #16381, .T. ) ;
#75450=CARTESIAN_POINT ( 'NONE',  ( 9.469380733400845074, -8.282780595021769443, 34.94152052738834868 ) ) ;
#75451=CARTESIAN_POINT ( 'NONE',  ( -7.846153846153844924, -8.164416787775445883, 34.95778746994557906 ) ) ;
#75453=ORIENTED_EDGE ( 'NONE', *, *, #31409, .F. ) ;
#75454=CARTESIAN_POINT ( 'NONE',  ( -10.61538461538473399, -5.219633306517616589, 34.19971097300220464 ) ) ;
#75457=FACE_BOUND ( 'NONE', #81943, .T. ) ;
#75458=CARTESIAN_POINT ( 'NONE',  ( -1.134615384615380806, -2.499999999999999556, 29.81604066197450109 ) ) ;
#75459=CARTESIAN_POINT ( 'NONE',  ( 8.546304551714619890, -4.887634598454295265, 34.01352882383564946 ) ) ;
#75461=CARTESIAN_POINT ( 'NONE',  ( 0.7115384615398965273, -7.500000000000155431, 34.75000000000007105 ) ) ;
#75462=CARTESIAN_POINT ( 'NONE',  ( 16.40390046548447245, -2.564540009722896752, 30.55348353981672105 ) ) ;
#75463=CARTESIAN_POINT ( 'NONE',  ( 0.5923302693632465088, -12.38066358083363738, 30.83685684665853444 ) ) ;
#75466=CARTESIAN_POINT ( 'NONE',  ( -12.21148404162501144, -2.318338780012835443, 30.59689888758630261 ) ) ;
#75467=CARTESIAN_POINT ( 'NONE',  ( 1.449870955891410240, -8.613356846314930593, 34.62446782046653482 ) ) ;
#75468=CARTESIAN_POINT ( 'NONE',  ( 4.284636594813105326, -11.37503395064541678, 33.29242100308974983 ) ) ;
#75469=CARTESIAN_POINT ( 'NONE',  ( 11.53846153846153832, -2.249999999999998668, 29.75000000000001776 ) ) ;
#75470=CARTESIAN_POINT ( 'NONE',  ( -0.2115384615370257404, -7.500000000000155431, 34.75000000000007105 ) ) ;
#75471=FACE_BOUND ( 'NONE', #110, .T. ) ;
#75472=CARTESIAN_POINT ( 'NONE',  ( -6.923076923076922462, -12.34228464037088635, 31.77849191805839268 ) ) ;
#75473=CARTESIAN_POINT ( 'NONE',  ( 17.01165307636676260, -3.083524468853725775, 32.58852847137143272 ) ) ;
#75474=CARTESIAN_POINT ( 'NONE',  ( -14.53117723225663660, -3.562934362175800285, 33.22335522853832401 ) ) ;
#75475=CARTESIAN_POINT ( 'NONE',  ( -18.06527000055631760, -2.379036618887871324, 30.90682066428148644 ) ) ;
#75476=CARTESIAN_POINT ( 'NONE',  ( 17.86985279056177589, -11.47017969459903952, 32.78971311882035167 ) ) ;
#75477=CARTESIAN_POINT ( 'NONE',  ( 10.61538461538449596, -3.300289026999228881, 32.46337939537708905 ) ) ;
#75479=EDGE_LOOP ( 'NONE', ( #3971, #64176 ) ) ;
#75480=CARTESIAN_POINT ( 'NONE',  ( 1.161689167099241082, -12.15238873228291538, 31.58232369045354915 ) ) ;
#75481=VERTEX_POINT ( 'NONE', #17631 ) ;
#75482=CARTESIAN_POINT ( 'NONE',  ( -13.13466997523734037, -9.357781135181031829, 34.66075350412533851 ) ) ;
#75483=ORIENTED_EDGE ( 'NONE', *, *, #47773, .F. ) ;
#75484=DIRECTION ( 'NONE',  ( 0.000000000000000000, 0.9848077530122072432, 0.1736481776669354937 ) ) ;
#75485=DIRECTION ( 'NONE',  ( 0.000000000000000000, 0.1736481776669275834, 0.9848077530122086864 ) ) ;
#75486=LINE ( 'NONE', #16343, #16504 ) ;
#75487=ORIENTED_EDGE ( 'NONE', *, *, #68083, .T. ) ;
#75488=CARTESIAN_POINT ( 'NONE',  ( 18.22296313426667780, -7.369474539155830506, 34.99858011523957657 ) ) ;
#75490=CARTESIAN_POINT ( 'NONE',  ( 12.46153846153846168, -9.905515769479276145, 34.41647553114623292 ) ) ;
#75491=B_SPLINE_CURVE_WITH_KNOTS ( 'NONE', 3,
 ( #56144, #37192, #64656, #23237, #10176, #28681, #83637, #8405, #70546, #30441 ),
 .UNSPECIFIED., .F., .F.,
 ( 4, 2, 2, 2, 4 ),
 ( 0.000000000000000000, 0.0001954311564186863323, 0.0003908623128373726646, 0.0005862934692560590241, 0.0007817246256747453293 ),
 .UNSPECIFIED. ) ;
#75492=CARTESIAN_POINT ( 'NONE',  ( -8.769230769230768274, -8.120952969808772792, 34.71129190930000163 ) ) ;
#75493=CARTESIAN_POINT ( 'NONE',  ( 16.82689983963011926, -12.43535235679832596, 30.55408501211184813 ) ) ;
#75495=CARTESIAN_POINT ( 'NONE',  ( 2.438218009455870749, -2.882268652242222284, 31.66798894389554064 ) ) ;
#75499=B_SPLINE_CURVE_WITH_KNOTS ( 'NONE', 3,
 ( #30132, #64344, #29263, #9418, #36453, #49526, #63905, #71997, #37771, #22489 ),
 .UNSPECIFIED., .F., .F.,
 ( 4, 2, 2, 2, 4 ),
 ( 0.000000000000000000, 0.0001954339857564091278, 0.0003908679715128182556, 0.0005863019572692274375, 0.0007817359430256365111 ),
 .UNSPECIFIED. ) ;
#75501=CARTESIAN_POINT ( 'NONE',  ( -5.999999999999998224, -2.249999999999998668, 29.75000000000001776 ) ) ;
#75502=ORIENTED_EDGE ( 'NONE', *, *, #13570, .F. ) ;
#75505=VECTOR ( 'NONE', #53628, 1000.000000000000227 ) ;
#75506=ADVANCED_FACE ( 'NONE', ( #72559 ), #10869, .F. ) ;
#75507=CARTESIAN_POINT ( 'NONE',  ( 2.084207383127977486, -4.988325925672468131, 34.36044203135681130 ) ) ;
#75509=ORIENTED_EDGE ( 'NONE', *, *, #70350, .T. ) ;
#75510=CARTESIAN_POINT ( 'NONE',  ( 1.449870524128225258, -8.656820664281605460, 34.87096338111211224 ) ) ;
#75511=CARTESIAN_POINT ( 'NONE',  ( 3.007843013253082454, -3.586966769969700763, 32.86292498521069660 ) ) ;
#75513=VERTEX_POINT ( 'NONE', #59042 ) ;
#75514=CARTESIAN_POINT ( 'NONE',  ( -5.207614543590636913, -5.582088688514999397, 34.36776431015576350 ) ) ;
#75515=AXIS2_PLACEMENT_3D ( 'NONE', #86530, #59480, #87419 ) ;
#75516=EDGE_CURVE ( 'NONE', #72654, #8229, #78810, .T. ) ;
#75517=DIRECTION ( 'NONE',  ( -0.000000000000000000, 0.1736481776669307198, -0.9848077530122080203 ) ) ;
#75518=CARTESIAN_POINT ( 'NONE',  ( -10.39237177129122003, -9.172514111537584114, 34.72667873470787470 ) ) ;
#75519=CARTESIAN_POINT ( 'NONE',  ( 4.853996859406927378, -4.186968288167446595, 33.49512374952580274 ) ) ;
#75520=CARTESIAN_POINT ( 'NONE',  ( -18.25002323729296450, -12.22074536777955345, 31.39888409691088356 ) ) ;
#75521=ADVANCED_FACE ( 'NONE', ( #48631 ), #82883, .F. ) ;
#75522=ORIENTED_EDGE ( 'NONE', *, *, #33390, .T. ) ;
#75523=ORIENTED_EDGE ( 'NONE', *, *, #71298, .F. ) ;
#75524=ORIENTED_EDGE ( 'NONE', *, *, #34494, .T. ) ;
#75525=CARTESIAN_POINT ( 'NONE',  ( -16.28399412357784826, -3.625366637846545448, 33.29286588640298561 ) ) ;
#75526=CARTESIAN_POINT ( 'NONE',  ( 0.4615384615383396616, -2.625532179533779154, 30.86335684631627174 ) ) ;
#75527=CARTESIAN_POINT ( 'NONE',  ( -13.25382357679059986, -12.11778462344220841, 31.66786338562085135 ) ) ;
#75528=CYLINDRICAL_SURFACE ( 'NONE', #78313, 0.2499999999999986955 ) ;
#75529=CARTESIAN_POINT ( 'NONE',  ( -17.75010451963438030, -7.431206910972181667, 35.00000000000000000 ) ) ;
#75530=ORIENTED_EDGE ( 'NONE', *, *, #53291, .F. ) ;
#75533=VERTEX_POINT ( 'NONE', #68466 ) ;
#75534=CARTESIAN_POINT ( 'NONE',  ( -6.988346923633241836, -2.657715359629089225, 31.77849191805834295 ) ) ;
#75535=EDGE_CURVE ( 'NONE', #85648, #43445, #36854, .T. ) ;
#75537=CARTESIAN_POINT ( 'NONE',  ( 6.000000000000001776, -5.471508081941601098, 34.59228464037088457 ) ) ;
#75540=ADVANCED_FACE ( 'NONE', ( #82446 ), #68909, .F. ) ;
#75541=CARTESIAN_POINT ( 'NONE',  ( -14.30769230769199218, -2.255955759149395501, 30.00000000000324363 ) ) ;
#75542=CARTESIAN_POINT ( 'NONE',  ( -6.000000000000119904, -4.481592998941358097, 33.73612834414048933 ) ) ;
#75543=ORIENTED_EDGE ( 'NONE', *, *, #69711, .T. ) ;
#75544=ORIENTED_EDGE ( 'NONE', *, *, #73572, .T. ) ;
#75545=EDGE_LOOP ( 'NONE', ( #59649, #34941 ) ) ;
#75547=DIRECTION ( 'NONE',  ( 1.000000000000000000, 0.000000000000000000, 0.000000000000000000 ) ) ;
#75548=ORIENTED_EDGE ( 'NONE', *, *, #11397, .F. ) ;
#75549=CARTESIAN_POINT ( 'NONE',  ( -2.242436736416282272, -8.613356846314928816, 34.62446782046653482 ) ) ;
#75550=AXIS2_PLACEMENT_3D ( 'NONE', #31386, #44004, #71922 ) ;
#75551=CARTESIAN_POINT ( 'NONE',  ( -14.55771554498527287, -2.587272538249755893, 30.68239716806877837 ) ) ;
#75552=ORIENTED_EDGE ( 'NONE', *, *, #76047, .F. ) ;
#75553=CARTESIAN_POINT ( 'NONE',  ( 8.769230769230647482, -12.46129190930018460, 30.37095296980731973 ) ) ;
#75554=CARTESIAN_POINT ( 'NONE',  ( 0.3308478584281524526, -9.084618155246140248, 34.75535874321725771 ) ) ;
#75555=VERTEX_POINT ( 'NONE', #47755 ) ;
#75556=FACE_BOUND ( 'NONE', #65957, .T. ) ;
#75559=CARTESIAN_POINT ( 'NONE',  ( 3.296024802045254720, -9.442884908240271713, 34.35708131394835618 ) ) ;
#75560=CARTESIAN_POINT ( 'NONE',  ( -12.46153846153858247, -2.625532179533778709, 30.86335684631627174 ) ) ;
#75562=CARTESIAN_POINT ( 'NONE',  ( -3.099978789802278811, -3.338503747796865984, 32.95102852606552801 ) ) ;
#75563=CARTESIAN_POINT ( 'NONE',  ( 12.52760579488854020, -2.833524468853757750, 32.15551576947925838 ) ) ;
#75564=ORIENTED_EDGE ( 'NONE', *, *, #57587, .T. ) ;
#75565=CYLINDRICAL_SURFACE ( 'NONE', #66256, 0.2499999999999997502 ) ;
#75567=FACE_OUTER_BOUND ( 'NONE', #12590, .T. ) ;
#75568=ORIENTED_EDGE ( 'NONE', *, *, #59866, .F. ) ;
#75570=CARTESIAN_POINT ( 'NONE',  ( 9.561616225640140243, -2.729777683071817229, 31.24903638046269450 ) ) ;
#75571=ORIENTED_EDGE ( 'NONE', *, *, #86831, .F. ) ;
#75572=EDGE_CURVE ( 'NONE', #41905, #51992, #75664, .T. ) ;
#75573=CARTESIAN_POINT ( 'NONE',  ( -9.915234651214538175, -9.172386477786396597, 34.72672124145550043 ) ) ;
#75574=CARTESIAN_POINT ( 'NONE',  ( 4.153846153846154188, -9.780366693483667717, 34.19971097300155094 ) ) ;
#75575=FACE_BOUND ( 'NONE', #28305, .T. ) ;
#75576=CARTESIAN_POINT ( 'NONE',  ( -15.29685264172511161, -5.557115091759785130, 34.35708131394839171 ) ) ;
#75577=CARTESIAN_POINT ( 'NONE',  ( -4.153846153846273204, -8.613356846316285953, 34.62446782046622218 ) ) ;
#75578=CARTESIAN_POINT ( 'NONE',  ( 2.177544337960613863, -6.809168938359898782, 34.95455904226513866 ) ) ;
#75579=CARTESIAN_POINT ( 'NONE',  ( 12.33139049180676494, -12.50552854090298638, 31.33409797877408920 ) ) ;
#75580=CARTESIAN_POINT ( 'NONE',  ( 2.241609928332172874, -10.67929555188718460, 33.92786785259543336 ) ) ;
#75581=LINE ( 'NONE', #13885, #14504 ) ;
#75583=EDGE_LOOP ( 'NONE', ( #45037, #56196 ) ) ;
#75584=ORIENTED_EDGE ( 'NONE', *, *, #47431, .T. ) ;
#75585=CARTESIAN_POINT ( 'NONE',  ( 5.326977388561388693, -6.567000820036038355, 34.66262288849541306 ) ) ;
#75586=CARTESIAN_POINT ( 'NONE',  ( -10.61538461538473577, -8.656820664282941280, 34.87096338111179961 ) ) ;
#75587=CARTESIAN_POINT ( 'NONE',  ( 18.00000000000000000, -2.708943851104267164, 35.45975837776705220 ) ) ;
#75588=CARTESIAN_POINT ( 'NONE',  ( 10.68145194873469173, -2.833524468853757750, 32.15551576947925838 ) ) ;
#75589=CARTESIAN_POINT ( 'NONE',  ( 3.230769230769231726, -11.16473453929635440, 33.15142922261926373 ) ) ;
#75591=ADVANCED_FACE ( 'NONE', ( #81999 ), #898, .F. ) ;
#75592=CARTESIAN_POINT ( 'NONE',  ( 6.923076923076924238, -2.292212530054420494, 30.41441678777542634 ) ) ;
#75593=CARTESIAN_POINT ( 'NONE',  ( 2.057692307692288392, -2.249999999999999112, 29.81609741502488120 ) ) ;
#75594=AXIS2_PLACEMENT_3D ( 'NONE', #67416, #26874, #40835 ) ;
#75595=CARTESIAN_POINT ( 'NONE',  ( -5.076923076923075762, -10.51840700105979565, 33.73612834413961536 ) ) ;
#75598=CARTESIAN_POINT ( 'NONE',  ( 5.207448515156721136, -8.630441415882550871, 34.87705825610312615 ) ) ;
#75599=CARTESIAN_POINT ( 'NONE',  ( -3.230769230769352962, -4.320704448113951379, 33.92786785259630022 ) ) ;
#75600=CARTESIAN_POINT ( 'NONE',  ( -3.230769230769351186, -8.613356846316285953, 34.62446782046622218 ) ) ;
#75601=LINE ( 'NONE', #20232, #39900 ) ;
#75602=ORIENTED_EDGE ( 'NONE', *, *, #14044, .F. ) ;
#75603=CARTESIAN_POINT ( 'NONE',  ( -14.43783951713053249, -3.817052484675422797, 33.13202310037935661 ) ) ;
#75606=EDGE_CURVE ( 'NONE', #84846, #60694, #48191, .T. ) ;
#75607=CARTESIAN_POINT ( 'NONE',  ( -9.942284436356281674, -10.82459398097509329, 33.81372124010185587 ) ) ;
#75608=CARTESIAN_POINT ( 'NONE',  ( -11.53846153846153655, -6.435427911321262684, 35.78748833219616898 ) ) ;
#75609=CARTESIAN_POINT ( 'NONE',  ( 10.36538461538461675, -2.499999999999998668, 29.75000000000000355 ) ) ;
#75610=CARTESIAN_POINT ( 'NONE',  ( -6.130609655204078301, -7.722926974430166069, 34.99546784045485737 ) ) ;
#75611=EDGE_LOOP ( 'NONE', ( #37113, #88111 ) ) ;
#75613=CARTESIAN_POINT ( 'NONE',  ( -9.469294848214294902, -5.582272713120729257, 34.63742843783360570 ) ) ;
#75614=ADVANCED_FACE ( 'NONE', ( #62586 ), #41895, .F. ) ;
#75615=ORIENTED_EDGE ( 'NONE', *, *, #2645, .F. ) ;
#75616=FACE_OUTER_BOUND ( 'NONE', #23422, .T. ) ;
#75618=ORIENTED_EDGE ( 'NONE', *, *, #11918, .F. ) ;
#75619=B_SPLINE_CURVE_WITH_KNOTS ( 'NONE', 3,
 ( #56004, #21779, #54226, #20457, #49254, #76725, #81721, #20006, #47470, #13255 ),
 .UNSPECIFIED., .F., .F.,
 ( 4, 2, 2, 2, 4 ),
 ( 0.0007817359430256306564, 0.0009771253907249969738, 0.001172514838424363291, 0.001367904286123729826, 0.001563293733823096143 ),
 .UNSPECIFIED. ) ;
#75620=CARTESIAN_POINT ( 'NONE',  ( -15.23076923076922995, -11.91647553114624181, 32.58852847137148245 ) ) ;
#75623=CARTESIAN_POINT ( 'NONE',  ( -14.98071491913091791, -12.41262288849542017, 30.68299917996395010 ) ) ;
#75624=ADVANCED_FACE ( 'NONE', ( #41444 ), #19841, .F. ) ;
#75625=EDGE_LOOP ( 'NONE', ( #45540, #15020 ) ) ;
#75626=VERTEX_POINT ( 'NONE', #74798 ) ;
#75627=DIRECTION ( 'NONE',  ( 0.000000000000000000, -6.938893903907222067E-15, 1.000000000000000000 ) ) ;
#75628=ORIENTED_EDGE ( 'NONE', *, *, #19522, .T. ) ;
#75629=EDGE_CURVE ( 'NONE', #36678, #79882, #38947, .T. ) ;
#75630=CARTESIAN_POINT ( 'NONE',  ( 7.780883845597524662, -9.528491918058357157, 34.59228464037090589 ) ) ;
#75631=DIRECTION ( 'NONE',  ( 0.000000000000000000, 0.6427876096865368094, 0.7660444431189802339 ) ) ;
#75632=CARTESIAN_POINT ( 'NONE',  ( -15.23076923076922995, -2.292212530054420494, 30.41441678777542634 ) ) ;
#75633=EDGE_CURVE ( 'NONE', #13761, #27959, #43647, .T. ) ;
#75634=AXIS2_PLACEMENT_3D ( 'NONE', #50482, #41979, #42423 ) ;
#75635=CARTESIAN_POINT ( 'NONE',  ( -10.61538461538461320, -5.180354513474913603, 36.12317359536750416 ) ) ;
#75636=CARTESIAN_POINT ( 'NONE',  ( 15.23076923076911093, -6.879047030192662504, 34.71129190930017927 ) ) ;
#75637=CARTESIAN_POINT ( 'NONE',  ( 13.38461538461538680, -3.050289026998446396, 32.03036669348365706 ) ) ;
#75638=DIRECTION ( 'NONE',  ( -0.000000000000000000, 0.9396926207859092051, -0.3420201433256662704 ) ) ;
#75639=EDGE_CURVE ( 'NONE', #79975, #35909, #8953, .T. ) ;
#75641=ORIENTED_EDGE ( 'NONE', *, *, #1432, .F. ) ;
#75642=CARTESIAN_POINT ( 'NONE',  ( -17.20761454359064047, -9.804603061927743113, 34.18744698557895845 ) ) ;
#75644=EDGE_CURVE ( 'NONE', #40637, #29464, #22800, .T. ) ;
#75645=CARTESIAN_POINT ( 'NONE',  ( -5.299850035829926753, -4.762599654559228846, 34.23009711892697737 ) ) ;
#75647=VECTOR ( 'NONE', #49468, 999.9999999999998863 ) ;
#75649=CARTESIAN_POINT ( 'NONE',  ( -8.546451100252703270, -10.97394488606064122, 33.68653795673694873 ) ) ;
#75650=CARTESIAN_POINT ( 'NONE',  ( 12.46153846153846168, -4.945431358278436385, 36.03766855953609394 ) ) ;
#75651=ORIENTED_EDGE ( 'NONE', *, *, #29051, .T. ) ;
#75652=CARTESIAN_POINT ( 'NONE',  ( 7.846153846153725020, -8.613356846316285953, 34.62446782046622218 ) ) ;
#75653=B_SPLINE_CURVE_WITH_KNOTS ( 'NONE', 3,
 ( #47867, #20838, #41119, #75779, #76220, #6449, #33909, #6880, #14526, #54614 ),
 .UNSPECIFIED., .F., .F.,
 ( 4, 2, 2, 2, 4 ),
 ( 0.0007817359430256285964, 0.0009771253907249943717, 0.001172514838424360255, 0.001367904286123726139, 0.001563293733823092023 ),
 .UNSPECIFIED. ) ;
#75656=EDGE_LOOP ( 'NONE', ( #18631, #72746, #25584, #37122 ) ) ;
#75658=B_SPLINE_CURVE_WITH_KNOTS ( 'NONE', 3,
 ( #58149, #51828, #4550, #17632, #44626, #58594, #43757, #51367, #3649, #32027 ),
 .UNSPECIFIED., .F., .F.,
 ( 4, 2, 2, 2, 4 ),
 ( 0.0007817359430256297891, 0.0009771253907249958896, 0.001172514838424362207, 0.001367904286123728524, 0.001563293733823094625 ),
 .UNSPECIFIED. ) ;
#75659=EDGE_LOOP ( 'NONE', ( #17290, #37568, #87898, #34549 ) ) ;
#75660=CARTESIAN_POINT ( 'NONE',  ( -4.403869378067609475, -4.175268141568689195, 33.81360843649122216 ) ) ;
#75662=CARTESIAN_POINT ( 'NONE',  ( -8.769230769230768274, -2.721908614388771852, 31.22303859784724978 ) ) ;
#75663=FACE_BOUND ( 'NONE', #87248, .T. ) ;
#75664=LINE ( 'NONE', #33362, #81580 ) ;
#75665=CARTESIAN_POINT ( 'NONE',  ( -17.77698864838715309, -12.15243808032446005, 31.58219941686247978 ) ) ;
#75666=DIRECTION ( 'NONE',  ( -0.000000000000000000, -0.1736481776669307198, -0.9848077530122080203 ) ) ;
#75667=CARTESIAN_POINT ( 'NONE',  ( -3.361460697436786660, -4.118384482072085184, 33.43331474514187107 ) ) ;
#75668=EDGE_CURVE ( 'NONE', #18655, #34160, #9885, .T. ) ;
#75670=CARTESIAN_POINT ( 'NONE',  ( -4.403822884788506364, -11.28823185664190376, 33.01397839955799896 ) ) ;
#75671=CARTESIAN_POINT ( 'NONE',  ( 14.55774672760575861, -6.523592122091592671, 34.90882529074906415 ) ) ;
#75672=ORIENTED_EDGE ( 'NONE', *, *, #67216, .F. ) ;
#75674=CARTESIAN_POINT ( 'NONE',  ( -16.85391172531022619, -9.886259254753566594, 34.14407573483972413 ) ) ;
#75675=CARTESIAN_POINT ( 'NONE',  ( -3.453696189676078276, -5.582147617184174848, 34.63737895849758530 ) ) ;
#75676=CARTESIAN_POINT ( 'NONE',  ( -12.68446467905460473, -2.554751324335734708, 30.48935550225260727 ) ) ;
#75678=CARTESIAN_POINT ( 'NONE',  ( 1.450682717965462221, -10.67929555188718282, 33.92786785259544757 ) ) ;
#75679=CARTESIAN_POINT ( 'NONE',  ( 6.923076923076924238, -2.499999999999998668, 29.75000000000001421 ) ) ;
#75680=VERTEX_POINT ( 'NONE', #16182 ) ;
#75681=EDGE_CURVE ( 'NONE', #48663, #39220, #14198, .T. ) ;
#75683=FACE_OUTER_BOUND ( 'NONE', #1855, .T. ) ;
#75684=CARTESIAN_POINT ( 'NONE',  ( -5.999999999999998224, -6.386643153685126251, 34.62446782046654192 ) ) ;
#75685=CARTESIAN_POINT ( 'NONE',  ( 16.82694633287448838, -4.075325502946085976, 33.72974371597207721 ) ) ;
#75686=CARTESIAN_POINT ( 'NONE',  ( -15.90390074446811042, -4.176053281294517028, 33.81426240980091791 ) ) ;
#75687=VERTEX_POINT ( 'NONE', #36025 ) ;
#75688=EDGE_CURVE ( 'NONE', #13392, #5310, #45469, .T. ) ;
#75689=VERTEX_POINT ( 'NONE', #72005 ) ;
#75692=CARTESIAN_POINT ( 'NONE',  ( 0.7115384615385245137, -7.434744429011175271, 34.75000000000000711 ) ) ;
#75693=VERTEX_POINT ( 'NONE', #58934 ) ;
#75694=AXIS2_PLACEMENT_3D ( 'NONE', #42847, #2277, #35646 ) ;
#75695=CARTESIAN_POINT ( 'NONE',  ( -1.161835843346973984, -8.496831190052093419, 34.64984203495476578 ) ) ;
#75696=CARTESIAN_POINT ( 'NONE',  ( -17.32694631421604115, -3.202444869320336895, 32.30641848906366675 ) ) ;
#75697=CARTESIAN_POINT ( 'NONE',  ( 4.153846153846154188, -13.37000171582298513, 34.34916445242398453 ) ) ;
#75698=CARTESIAN_POINT ( 'NONE',  ( 11.53846153846141753, -12.27809138561165270, 31.22303859784587132 ) ) ;
#75700=CARTESIAN_POINT ( 'NONE',  ( 9.942253210655836781, -5.852078868378309373, 34.47109172314383585 ) ) ;
#75701=ORIENTED_EDGE ( 'NONE', *, *, #3545, .T. ) ;
#75702=CARTESIAN_POINT ( 'NONE',  ( 6.000000000000001776, -8.120952969808772792, 34.71129190930000163 ) ) ;
#75703=CARTESIAN_POINT ( 'NONE',  ( -12.39628289026243912, -11.94971097300157403, 32.03036669348361443 ) ) ;
#75704=EDGE_LOOP ( 'NONE', ( #27102, #34329, #3177, #55345 ) ) ;
#75705=DIRECTION ( 'NONE',  ( -0.000000000000000000, 0.7660444431189791237, -0.6427876096865379196 ) ) ;
#75706=DIRECTION ( 'NONE',  ( -0.000000000000000000, 1.000000000000000000, 3.491481338843133355E-15 ) ) ;
#75708=CARTESIAN_POINT ( 'NONE',  ( 9.019176178608811156, -12.07971442181322352, 32.31769673815850297 ) ) ;
#75710=CARTESIAN_POINT ( 'NONE',  ( 17.32692307692301270, -7.565270445406050648, 34.75000000000000000 ) ) ;
#75711=CARTESIAN_POINT ( 'NONE',  ( -3.230769230769351186, -6.879047030192662504, 34.71129190930017927 ) ) ;
#75713=EDGE_LOOP ( 'NONE', ( #67279, #6392 ) ) ;
#75714=CARTESIAN_POINT ( 'NONE',  ( -3.007756386675836779, -6.460100341425561332, 34.89618726649961644 ) ) ;
#75715=CARTESIAN_POINT ( 'NONE',  ( 0.4615384615384611200, -3.050289026998446396, 32.03036669348365706 ) ) ;
#75716=DIRECTION ( 'NONE',  ( 0.000000000000000000, 0.4999999999999985567, 0.8660254037844395958 ) ) ;
#75717=CIRCLE ( 'NONE', #13863, 2.999999999999999112 ) ;
#75719=EDGE_LOOP ( 'NONE', ( #23120, #31789, #15070, #5750 ) ) ;
#75720=DIRECTION ( 'NONE',  ( -0.000000000000000000, -0.6427876096865404731, -0.7660444431189771253 ) ) ;
#75721=CARTESIAN_POINT ( 'NONE',  ( -2.437839517130526712, -3.285722584762969856, 32.44110544564090759 ) ) ;
#75722=EDGE_CURVE ( 'NONE', #79737, #81272, #53059, .T. ) ;
#75723=VECTOR ( 'NONE', #44890, 1000.000000000000114 ) ;
#75724=CARTESIAN_POINT ( 'NONE',  ( 10.86533002476265786, -4.932303261841489928, 34.32971442181322885 ) ) ;
#75725=CARTESIAN_POINT ( 'NONE',  ( -4.153846153846152411, -1.466349020453238561, 30.81389545987213907 ) ) ;
#75726=CARTESIAN_POINT ( 'NONE',  ( 17.07692307692295586, -3.300289026999228437, 32.46337939537709616 ) ) ;
#75729=CARTESIAN_POINT ( 'NONE',  ( 16.85343813319912343, -3.236172620538810385, 32.36188796281390267 ) ) ;
#75730=AXIS2_PLACEMENT_3D ( 'NONE', #61520, #40824, #82257 ) ;
#75732=CARTESIAN_POINT ( 'NONE',  ( 18.06525513951284267, -12.51329471203373345, 31.30864560766537963 ) ) ;
#75733=EDGE_LOOP ( 'NONE', ( #85388, #30285 ) ) ;
#75734=CARTESIAN_POINT ( 'NONE',  ( -16.85391023282967993, -11.98016756924215187, 32.48728574198911190 ) ) ;
#75735=ORIENTED_EDGE ( 'NONE', *, *, #50572, .F. ) ;
#75736=CARTESIAN_POINT ( 'NONE',  ( -16.21911659980693443, -6.026961402152685388, 34.52809138561120506 ) ) ;
#75737=DIRECTION ( 'NONE',  ( -0.000000000000000000, -0.7660444431189791237, -0.6427876096865379196 ) ) ;
#75738=ORIENTED_EDGE ( 'NONE', *, *, #31634, .T. ) ;
#75739=DIRECTION ( 'NONE',  ( -0.000000000000000000, 0.5000000000000011102, -0.8660254037844381525 ) ) ;
#75740=DIRECTION ( 'NONE',  ( -1.000000000000000000, 0.000000000000000000, 0.000000000000000000 ) ) ;
#75741=CARTESIAN_POINT ( 'NONE',  ( -10.83831083290076158, -5.667676309546437530, 34.40238873228292249 ) ) ;
#75742=CARTESIAN_POINT ( 'NONE',  ( 7.173022332454968009, -12.45601412856602863, 31.48342859153981621 ) ) ;
#75746=ORIENTED_EDGE ( 'NONE', *, *, #14841, .T. ) ;
#75747=FACE_BOUND ( 'NONE', #59370, .T. ) ;
#75748=VERTEX_POINT ( 'NONE', #12105 ) ;
#75749=LINE ( 'NONE', #7751, #15609 ) ;
#75751=B_SPLINE_CURVE_WITH_KNOTS ( 'NONE', 3,
 ( #16284, #43750, #71216, #81497, #26988, #34178, #87372, #46810, #81939, #54446 ),
 .UNSPECIFIED., .F., .F.,
 ( 4, 2, 2, 2, 4 ),
 ( 0.000000000000000000, 0.0001954311584214071026, 0.0003908623168428142051, 0.0005862934752642213077, 0.0007817246336856284103 ),
 .UNSPECIFIED. ) ;
#75752=DIRECTION ( 'NONE',  ( -0.000000000000000000, 0.8660254037844397068, -0.4999999999999978906 ) ) ;
#75753=EDGE_CURVE ( 'NONE', #36504, #74762, #77687, .T. ) ;
#75755=CARTESIAN_POINT ( 'NONE',  ( -7.846153846153844924, -9.819645486525091727, 36.12317359536749706 ) ) ;
#75756=DIRECTION ( 'NONE',  ( -0.000000000000000000, -0.6427876096865404731, -0.7660444431189770143 ) ) ;
#75757=ORIENTED_EDGE ( 'NONE', *, *, #4130, .T. ) ;
#75758=VERTEX_POINT ( 'NONE', #4899 ) ;
#75761=CARTESIAN_POINT ( 'NONE',  ( 13.51466299087107004, -7.723484964179501588, 34.74522123443823318 ) ) ;
#75762=ORIENTED_EDGE ( 'NONE', *, *, #21935, .F. ) ;
#75763=CARTESIAN_POINT ( 'NONE',  ( 4.284371592079798674, -10.31582465632705237, 34.18122507451815295 ) ) ;
#75764=EDGE_CURVE ( 'NONE', #16707, #71873, #76582, .T. ) ;
#75766=CARTESIAN_POINT ( 'NONE',  ( -17.07692307692307665, -2.833524468853757305, 32.15551576947925838 ) ) ;
#75767=B_SPLINE_CURVE_WITH_KNOTS ( 'NONE', 3,
 ( #14914, #63074, #1385, #28876, #56332, #15797, #43263, #29751, #44564, #44122 ),
 .UNSPECIFIED., .F., .F.,
 ( 4, 2, 2, 2, 4 ),
 ( 0.0007817246256747516176, 0.0009771112852218965736, 0.001172497944769041638, 0.001367884604316186702, 0.001563271263863331550 ),
 .UNSPECIFIED. ) ;
#75768=CARTESIAN_POINT ( 'NONE',  ( 8.703960323269994248, -9.442884908240170461, 34.35708131394840592 ) ) ;
#75769=CARTESIAN_POINT ( 'NONE',  ( 11.76183747915971800, -2.501478030877322567, 29.88021232661721172 ) ) ;
#75771=CARTESIAN_POINT ( 'NONE',  ( 15.48082354240754555, -9.148310452688876993, 34.47095581063188519 ) ) ;
#75772=DIRECTION ( 'NONE',  ( -0.000000000000000000, -0.5000000000000011102, -0.8660254037844380415 ) ) ;
#75773=CARTESIAN_POINT ( 'NONE',  ( 11.47237812750565666, -9.780366693483667717, 34.19971097300155805 ) ) ;
#75774=EDGE_LOOP ( 'NONE', ( #50564, #59041, #66367, #63227, #61970, #70669 ) ) ;
#75775=ORIENTED_EDGE ( 'NONE', *, *, #13716, .F. ) ;
#75776=AXIS2_PLACEMENT_3D ( 'NONE', #47449, #82144, #88042 ) ;
#75777=ORIENTED_EDGE ( 'NONE', *, *, #47564, .F. ) ;
#75779=CARTESIAN_POINT ( 'NONE',  ( 1.607394925883794068, -5.913360116392399668, 34.49180327182771322 ) ) ;
#75780=CARTESIAN_POINT ( 'NONE',  ( -9.692307692307691624, -3.937682226553329556, 33.60647404775216529 ) ) ;
#75782=CARTESIAN_POINT ( 'NONE',  ( 4.153846153846154188, -11.35647404775217417, 33.31231777344666511 ) ) ;
#75783=FACE_BOUND ( 'NONE', #83998, .T. ) ;
#75784=CARTESIAN_POINT ( 'NONE',  ( 7.846153846153846700, -11.16473453929635440, 33.15142922261926373 ) ) ;
#75786=CARTESIAN_POINT ( 'NONE',  ( -5.076923076923075762, -2.249999999999998668, 29.50000000000001421 ) ) ;
#75787=CARTESIAN_POINT ( 'NONE',  ( -0.3954701105360237112, -8.973038597847269315, 34.52809138561122637 ) ) ;
#75788=B_SPLINE_CURVE_WITH_KNOTS ( 'NONE', 3,
 ( #29119, #42188, #69641, #7949, #35414, #62866, #28667, #56132, #84065, #22344 ),
 .UNSPECIFIED., .F., .F.,
 ( 4, 2, 2, 2, 4 ),
 ( 0.000000000000000000, 0.0001954339857564097241, 0.0003908679715128194482, 0.0005863019572692291723, 0.0007817359430256388964 ),
 .UNSPECIFIED. ) ;
#75790=CARTESIAN_POINT ( 'NONE',  ( -3.360917200500924906, -3.625366637846545448, 33.29286588640298561 ) ) ;
#75791=ORIENTED_EDGE ( 'NONE', *, *, #15954, .T. ) ;
#75792=CARTESIAN_POINT ( 'NONE',  ( 1.384615384615386802, -10.67929555188718282, 33.92786785259544047 ) ) ;
#75793=EDGE_CURVE ( 'NONE', #53433, #31330, #23912, .T. ) ;
#75794=ORIENTED_EDGE ( 'NONE', *, *, #20600, .F. ) ;
#75795=B_SPLINE_CURVE_WITH_KNOTS ( 'NONE', 3,
 ( #36930, #63957, #2252, #50872, #78358, #52216, #17106, #29748, #72493, #24298 ),
 .UNSPECIFIED., .F., .F.,
 ( 4, 2, 2, 2, 4 ),
 ( 0.000000000000000000, 0.0001954311564186882026, 0.0003908623128373764051, 0.0005862934692560646619, 0.0007817246256747528103 ),
 .UNSPECIFIED. ) ;
#75796=FACE_BOUND ( 'NONE', #62813, .T. ) ;
#75797=CARTESIAN_POINT ( 'NONE',  ( 9.469381474791543241, -5.667676309546437530, 34.40238873228292249 ) ) ;
#75798=EDGE_CURVE ( 'NONE', #83778, #14363, #60025, .T. ) ;
#75799=CARTESIAN_POINT ( 'NONE',  ( 18.00000000000000000, -13.75783147151868846, 33.36296068462461051 ) ) ;
#75801=ORIENTED_EDGE ( 'NONE', *, *, #43478, .T. ) ;
#75802=CARTESIAN_POINT ( 'NONE',  ( 5.299934428535923558, -3.105924265160262543, 32.13625925475356127 ) ) ;
#75803=CARTESIAN_POINT ( 'NONE',  ( -17.86920955903305597, -3.957578996910244395, 33.62503395064540257 ) ) ;
#75804=CARTESIAN_POINT ( 'NONE',  ( 18.13079044096694759, -10.70102852606553157, 33.91149625220312913 ) ) ;
#75805=CARTESIAN_POINT ( 'NONE',  ( 6.065255571276024327, -3.835265460703683349, 33.15142922261929925 ) ) ;
#75807=EDGE_CURVE ( 'NONE', #16242, #29311, #72264, .T. ) ;
#75808=CARTESIAN_POINT ( 'NONE',  ( -12.46153846153846168, -3.050289026998446396, 32.03036669348365706 ) ) ;
#75809=CARTESIAN_POINT ( 'NONE',  ( -16.15384615384615330, -9.905515769479276145, 34.41647553114623292 ) ) ;
#75810=CARTESIAN_POINT ( 'NONE',  ( -8.769230769230768274, -10.05456864172156806, 36.03766855953608683 ) ) ;
#75811=ORIENTED_EDGE ( 'NONE', *, *, #53356, .T. ) ;
#75812=CARTESIAN_POINT ( 'NONE',  ( -18.00000000000012079, -3.643525952248793498, 33.31231777344770961 ) ) ;
#75813=FACE_OUTER_BOUND ( 'NONE', #5845, .T. ) ;
#75815=CARTESIAN_POINT ( 'NONE',  ( -10.36543909703647159, -2.587454068350147018, 30.68340429815432202 ) ) ;
#75816=VECTOR ( 'NONE', #56792, 1000.000000000000227 ) ;
#75817=CARTESIAN_POINT ( 'NONE',  ( 3.230769230769110045, -3.835265460704628371, 33.15142922262033665 ) ) ;
#75818=CARTESIAN_POINT ( 'NONE',  ( -7.846153846153844924, -10.51840700105979565, 33.73612834413961536 ) ) ;
#75819=CARTESIAN_POINT ( 'NONE',  ( -16.40382289789473802, -8.347322224742351082, 34.93158281831414058 ) ) ;
#75820=EDGE_CURVE ( 'NONE', #33682, #13888, #54851, .T. ) ;
#75821=CARTESIAN_POINT ( 'NONE',  ( 6.000000000000001776, -4.661471528628507777, 34.16647553114623292 ) ) ;
#75825=CARTESIAN_POINT ( 'NONE',  ( -17.74994568836168440, -9.148310452688869887, 34.47095581063188519 ) ) ;
#75826=EDGE_LOOP ( 'NONE', ( #80685, #37769, #38723, #19603 ) ) ;
#75827=VERTEX_POINT ( 'NONE', #33256 ) ;
#75828=CARTESIAN_POINT ( 'NONE',  ( -11.53846153846153655, -2.292212530054420494, 30.41441678777542634 ) ) ;
#75829=VECTOR ( 'NONE', #89172, 1000.000000000000114 ) ;
#75830=EDGE_LOOP ( 'NONE', ( #44087, #56417 ) ) ;
#75831=CARTESIAN_POINT ( 'NONE',  ( 1.384615384615386802, -11.91647553114624181, 32.58852847137148245 ) ) ;
#75833=CARTESIAN_POINT ( 'NONE',  ( 13.51540719244017197, -2.729792928343269587, 31.24908615093345077 ) ) ;
#75834=EDGE_CURVE ( 'NONE', #2122, #53843, #60464, .T. ) ;
#75836=CARTESIAN_POINT ( 'NONE',  ( -16.15384615384627409, -6.026961402154118908, 34.52809138561165270 ) ) ;
#75837=B_SPLINE_CURVE_WITH_KNOTS ( 'NONE', 3,
 ( #16781, #64078, #28996, #29435, #22659, #77164, #44234, #50566, #16347, #21778 ),
 .UNSPECIFIED., .F., .F.,
 ( 4, 2, 2, 2, 4 ),
 ( 0.000000000000000000, 0.0001954339857564063089, 0.0003908679715128126177, 0.0005863019572692189808, 0.0007817359430256252354 ),
 .UNSPECIFIED. ) ;
#75838=CARTESIAN_POINT ( 'NONE',  ( -6.989159302437058408, -9.058645607665454236, 34.76329471203372634 ) ) ;
#75839=CARTESIAN_POINT ( 'NONE',  ( -14.55769230769230660, -7.500000000000001776, 35.04278698407183867 ) ) ;
#75840=CARTESIAN_POINT ( 'NONE',  ( 2.530703659305157949, -11.24521262558773671, 33.06293181088029343 ) ) ;
#75842=B_SPLINE_CURVE_WITH_KNOTS ( 'NONE', 3,
 ( #31677, #24455, #79861, #67240, #17721, #73560, #45173, #65450, #73103, #66344 ),
 .UNSPECIFIED., .F., .F.,
 ( 4, 2, 2, 2, 4 ),
 ( 0.000000000000000000, 0.0001954339857564073388, 0.0003908679715128146777, 0.0005863019572692220165, 0.0007817359430256293554 ),
 .UNSPECIFIED. ) ;
#75844=EDGE_CURVE ( 'NONE', #673, #23399, #68361, .T. ) ;
#75846=CARTESIAN_POINT ( 'NONE',  ( 13.38461538461538680, -4.102666532097928531, 36.13435417666054406 ) ) ;
#75847=CARTESIAN_POINT ( 'NONE',  ( 6.000000000000001776, -1.509761064869970415, 31.06009739812519044 ) ) ;
#75848=CARTESIAN_POINT ( 'NONE',  ( -8.096177083446809419, -8.432397168068783699, 34.66272746175022945 ) ) ;
#75849=EDGE_CURVE ( 'NONE', #72929, #13144, #71139, .T. ) ;
#75850=ORIENTED_EDGE ( 'NONE', *, *, #60693, .T. ) ;
#75851=ORIENTED_EDGE ( 'NONE', *, *, #88682, .F. ) ;
#75852=CARTESIAN_POINT ( 'NONE',  ( -18.22348492456433178, -2.612411019501190701, 31.66733052389439962 ) ) ;
#75853=CYLINDRICAL_SURFACE ( 'NONE', #17402, 0.2500000000000002220 ) ;
#75854=DIRECTION ( 'NONE',  ( -0.000000000000000000, 0.5000000000000011102, -0.8660254037844380415 ) ) ;
#75855=CARTESIAN_POINT ( 'NONE',  ( -11.60421834097584970, -7.249945686854186278, 34.74374336980224598 ) ) ;
#75856=DIRECTION ( 'NONE',  ( -0.000000000000000000, 0.1736481776669307198, -0.9848077530122080203 ) ) ;
#75857=CARTESIAN_POINT ( 'NONE',  ( -9.442253272394237840, -10.82426656108012075, 33.81400080652039009 ) ) ;
#75859=EDGE_LOOP ( 'NONE', ( #79309, #10824 ) ) ;
#75860=CARTESIAN_POINT ( 'NONE',  ( -0.4615384615384611200, -8.120952969808772792, 34.71129190930000163 ) ) ;
#75861=ORIENTED_EDGE ( 'NONE', *, *, #68016, .T. ) ;
#75864=B_SPLINE_CURVE_WITH_KNOTS ( 'NONE', 3,
 ( #39046, #31383, #24624, #79581, #52533, #80017, #18318, #45781, #2566, #30493 ),
 .UNSPECIFIED., .F., .F.,
 ( 4, 2, 2, 2, 4 ),
 ( 0.000000000000000000, 0.0001954339857564080707, 0.0003908679715128161414, 0.0005863019572692241849, 0.0007817359430256322827 ),
 .UNSPECIFIED. ) ;
#75865=DIRECTION ( 'NONE',  ( -0.000000000000000000, 0.3420201433256694901, -0.9396926207859082059 ) ) ;
#75866=CARTESIAN_POINT ( 'NONE',  ( 14.08476609017615644, -4.887634598454295265, 34.01352882383564946 ) ) ;
#75867=B_SPLINE_CURVE_WITH_KNOTS ( 'NONE', 3,
 ( #67302, #80381, #18676, #46141, #81265, #45687, #73629, #59198, #17784, #5597 ),
 .UNSPECIFIED., .F., .F.,
 ( 4, 2, 2, 2, 4 ),
 ( 0.000000000000000000, 0.0001954339857564100222, 0.0003908679715128200445, 0.0005863019572692300396, 0.0007817359430256400890 ),
 .UNSPECIFIED. ) ;
#75868=CARTESIAN_POINT ( 'NONE',  ( -15.36091644020745051, -3.285722584762969856, 32.44110544564090759 ) ) ;
#75869=B_SPLINE_CURVE_WITH_KNOTS ( 'NONE', 3,
 ( #65833, #50975, #16334, #43798, #71260, #37031, #64493, #2800, #30291, #44221 ),
 .UNSPECIFIED., .F., .F.,
 ( 4, 2, 2, 2, 4 ),
 ( 0.000000000000000000, 0.0001954339857564073659, 0.0003908679715128147319, 0.0005863019572692221250, 0.0007817359430256294638 ),
 .UNSPECIFIED. ) ;
#75870=CARTESIAN_POINT ( 'NONE',  ( -13.51530598772569114, -2.494641256782728966, 31.33461815524612959 ) ) ;
#75871=VERTEX_POINT ( 'NONE', #40467 ) ;
#75872=EDGE_CURVE ( 'NONE', #13156, #4768, #63655, .T. ) ;
#75873=ORIENTED_EDGE ( 'NONE', *, *, #43840, .T. ) ;
#75874=VECTOR ( 'NONE', #40687, 1000.000000000000114 ) ;
#75875=ORIENTED_EDGE ( 'NONE', *, *, #84629, .T. ) ;
#75876=ORIENTED_EDGE ( 'NONE', *, *, #15560, .F. ) ;
#75877=CARTESIAN_POINT ( 'NONE',  ( -3.480769230769250822, -2.249999999999999112, 29.81609741502488120 ) ) ;
#75878=CARTESIAN_POINT ( 'NONE',  ( 5.076923076922954969, -10.90142922262034020, 33.41473453929536674 ) ) ;
#75879=ADVANCED_FACE ( 'NONE', ( #12538 ), #54399, .F. ) ;
#75881=CARTESIAN_POINT ( 'NONE',  ( 4.403791563224196182, -12.07971442181322352, 32.31769673815850297 ) ) ;
#75882=CARTESIAN_POINT ( 'NONE',  ( 14.24236939220013554, -7.749976743299138882, 34.99404534957040624 ) ) ;
#75883=CARTESIAN_POINT ( 'NONE',  ( 8.096153846153910649, -7.434744860731433924, 35.00000000000000711 ) ) ;
#75886=VERTEX_POINT ( 'NONE', #82333 ) ;
#75887=VERTEX_POINT ( 'NONE', #20616 ) ;
#75888=ORIENTED_EDGE ( 'NONE', *, *, #40449, .F. ) ;
#75890=LINE ( 'NONE', #13302, #7061 ) ;
#75891=ORIENTED_EDGE ( 'NONE', *, *, #53979, .T. ) ;
#75892=CARTESIAN_POINT ( 'NONE',  ( -4.153846153846152411, -2.721908614388771852, 31.22303859784724978 ) ) ;
#75893=DIRECTION ( 'NONE',  ( -0.000000000000000000, -0.5000000000000009992, -0.8660254037844380415 ) ) ;
#75896=B_SPLINE_CURVE_WITH_KNOTS ( 'NONE', 3,
 ( #86188, #51925, #58246, #64994, #38883, #3301, #79423, #45174, #30773, #59582 ),
 .UNSPECIFIED., .F., .F.,
 ( 4, 2, 2, 2, 4 ),
 ( 0.0007817246256747445703, 0.0009771112852218872494, 0.001172497944769030145, 0.001367884604316172825, 0.001563271263863315504 ),
 .UNSPECIFIED. ) ;
#75897=VERTEX_POINT ( 'NONE', #84986 ) ;
#75899=EDGE_CURVE ( 'NONE', #80426, #57743, #15202, .T. ) ;
#75900=ORIENTED_EDGE ( 'NONE', *, *, #25624, .F. ) ;
#75901=FACE_BOUND ( 'NONE', #31935, .T. ) ;
#75902=CYLINDRICAL_SURFACE ( 'NONE', #70495, 0.2500000000000008882 ) ;
#75903=VECTOR ( 'NONE', #73823, 1000.000000000000000 ) ;
#75904=CARTESIAN_POINT ( 'NONE',  ( 10.61538461538461675, -7.500000000000001776, 35.04278698407183867 ) ) ;
#75905=ORIENTED_EDGE ( 'NONE', *, *, #31558, .F. ) ;
#75906=EDGE_CURVE ( 'NONE', #79014, #64930, #56151, .T. ) ;
#75907=DIRECTION ( 'NONE',  ( -0.000000000000000000, -0.000000000000000000, -1.000000000000000000 ) ) ;
#75909=CYLINDRICAL_SURFACE ( 'NONE', #51411, 0.2500000000000008882 ) ;
#75910=CARTESIAN_POINT ( 'NONE',  ( -3.480792454990687013, -9.356822207818506598, 34.66110646841856635 ) ) ;
#75911=VERTEX_POINT ( 'NONE', #50726 ) ;
#75912=AXIS2_PLACEMENT_3D ( 'NONE', #19541, #46570, #60525 ) ;
#75913=CARTESIAN_POINT ( 'NONE',  ( 16.08808935133184903, -7.249945686854186278, 34.74374336980224598 ) ) ;
#75914=CARTESIAN_POINT ( 'NONE',  ( -4.153846153846274980, -10.33852847137269571, 34.16647553114546554 ) ) ;
#75915=CARTESIAN_POINT ( 'NONE',  ( -3.903900744468109529, -2.341251567377310217, 30.72681386836322659 ) ) ;
#75916=DIRECTION ( 'NONE',  ( -0.000000000000000000, -0.1736481776669307198, -0.9848077530122080203 ) ) ;
#75917=CARTESIAN_POINT ( 'NONE',  ( -17.07692307692307665, -11.33034616979429110, 35.88435417666054406 ) ) ;
#75918=FACE_BOUND ( 'NONE', #73426, .T. ) ;
#75919=CARTESIAN_POINT ( 'NONE',  ( 13.13463865367303463, -11.79746400365624659, 32.30657167506340954 ) ) ;
#75920=CARTESIAN_POINT ( 'NONE',  ( -6.130147969731693181, -10.31621877034669588, 34.18098118002070152 ) ) ;
#75921=ADVANCED_FACE ( 'NONE', ( #42236 ), #76899, .F. ) ;
#75922=VECTOR ( 'NONE', #50901, 1000.000000000000000 ) ;
#75923=CARTESIAN_POINT ( 'NONE',  ( 11.53846153846141576, -12.16647553114689728, 32.15551576947799362 ) ) ;
#75924=CARTESIAN_POINT ( 'NONE',  ( -8.638438961405983108, -11.71459661697925903, 32.44059661609676937 ) ) ;
#75926=CARTESIAN_POINT ( 'NONE',  ( -8.096177070375304652, -4.175268141568685643, 33.81360843649122216 ) ) ;
#75928=ORIENTED_EDGE ( 'NONE', *, *, #12062, .F. ) ;
#75929=B_SPLINE_CURVE_WITH_KNOTS ( 'NONE', 3,
 ( #68392, #61629, #74722, #20215, #89134, #53543, #81038, #27411, #5812, #88694 ),
 .UNSPECIFIED., .F., .F.,
 ( 4, 2, 2, 2, 4 ),
 ( 0.0007817246256747451124, 0.0009771112852218881168, 0.001172497944769031230, 0.001367884604316174126, 0.001563271263863317238 ),
 .UNSPECIFIED. ) ;
#75931=ORIENTED_EDGE ( 'NONE', *, *, #71164, .T. ) ;
#75932=DIRECTION ( 'NONE',  ( -1.000000000000000000, 0.000000000000000000, 0.000000000000000000 ) ) ;
#75933=ORIENTED_EDGE ( 'NONE', *, *, #3699, .T. ) ;
#75934=CARTESIAN_POINT ( 'NONE',  ( -11.31544869436814338, -6.460100341425560444, 34.89618726649961644 ) ) ;
#75935=CARTESIAN_POINT ( 'NONE',  ( -8.069638789877792817, -10.11188796281391511, 34.01382737946119050 ) ) ;
#75936=VERTEX_POINT ( 'NONE', #56178 ) ;
#75937=CARTESIAN_POINT ( 'NONE',  ( 17.75000000000000000, -7.500000000000001776, 35.00000000000000000 ) ) ;
#75939=EDGE_CURVE ( 'NONE', #85149, #45673, #66853, .T. ) ;
#75940=CARTESIAN_POINT ( 'NONE',  ( -15.45369618967607828, -9.172386477786396597, 34.72672124145550043 ) ) ;
#75942=CARTESIAN_POINT ( 'NONE',  ( -3.230769230768915534, -2.255955759149395501, 30.00000000000324363 ) ) ;
#75943=DIRECTION ( 'NONE',  ( -0.000000000000000000, 0.5000000000000011102, -0.8660254037844380415 ) ) ;
#75944=CARTESIAN_POINT ( 'NONE',  ( -1.319360245102545459, -6.835583212224609184, 34.95778746994559327 ) ) ;
#75947=CIRCLE ( 'NONE', #37090, 0.2500000000000002220 ) ;
#75948=EDGE_CURVE ( 'NONE', #80983, #36772, #8885, .T. ) ;
#75949=EDGE_CURVE ( 'NONE', #29571, #55482, #5397, .T. ) ;
#75950=CARTESIAN_POINT ( 'NONE',  ( 17.07692307692295586, -5.094484230521993062, 34.41647553114689373 ) ) ;
#75951=DIRECTION ( 'NONE',  ( -0.000000000000000000, 1.000000000000000000, 3.491481338843133355E-15 ) ) ;
#75952=EDGE_LOOP ( 'NONE', ( #64703, #80236 ) ) ;
#75953=CARTESIAN_POINT ( 'NONE',  ( 12.46153846153846168, -11.16473453929635440, 33.15142922261926373 ) ) ;
#75956=CARTESIAN_POINT ( 'NONE',  ( 0.4615384615384611200, -2.517432740324522911, 35.29906147534542527 ) ) ;
#75957=ORIENTED_EDGE ( 'NONE', *, *, #24851, .T. ) ;
#75958=CARTESIAN_POINT ( 'NONE',  ( 14.30769230769218758, -2.625532179533778709, 30.86335684631627174 ) ) ;
#75959=DIRECTION ( 'NONE',  ( -0.000000000000000000, 0.1736481776669307198, -0.9848077530122080203 ) ) ;
#75960=LINE ( 'NONE', #14705, #44020 ) ;
#75961=ORIENTED_EDGE ( 'NONE', *, *, #10056, .F. ) ;
#75962=FACE_OUTER_BOUND ( 'NONE', #571, .T. ) ;
#75964=CARTESIAN_POINT ( 'NONE',  ( -1.384615384615505151, -10.90142922262034020, 33.41473453929536674 ) ) ;
#75965=DIRECTION ( 'NONE',  ( 0.000000000000000000, 0.4999999999999960032, -0.8660254037844410391 ) ) ;
#75966=CARTESIAN_POINT ( 'NONE',  ( -9.561782254074051579, -2.647132371071621471, 31.75357179365171589 ) ) ;
#75967=CARTESIAN_POINT ( 'NONE',  ( -15.36091720050093201, -11.66186481527757302, 32.95055677023626117 ) ) ;
#75969=EDGE_LOOP ( 'NONE', ( #72523, #23233, #9263, #9840 ) ) ;
#75970=ORIENTED_EDGE ( 'NONE', *, *, #53331, .F. ) ;
#75971=CARTESIAN_POINT ( 'NONE',  ( -13.38461538461550582, -3.835265460704628371, 33.15142922262033665 ) ) ;
#75973=DIRECTION ( 'NONE',  ( -0.000000000000000000, 0.1736481776669307198, -0.9848077530122080203 ) ) ;
#75974=CARTESIAN_POINT ( 'NONE',  ( -16.82692307692314415, -7.565270000091922853, 34.99999999999999289 ) ) ;
#75975=CIRCLE ( 'NONE', #73091, 0.2500000000000002220 ) ;
#75976=ORIENTED_EDGE ( 'NONE', *, *, #42720, .F. ) ;
#75977=FACE_OUTER_BOUND ( 'NONE', #16346, .T. ) ;
#75978=ORIENTED_EDGE ( 'NONE', *, *, #35874, .T. ) ;
#75979=VERTEX_POINT ( 'NONE', #56623 ) ;
#75981=EDGE_LOOP ( 'NONE', ( #42155, #38004, #82407, #73324 ) ) ;
#75982=CARTESIAN_POINT ( 'NONE',  ( -15.45369544828537833, -12.15238873228292071, 31.58232369045353849 ) ) ;
#75984=CARTESIAN_POINT ( 'NONE',  ( -0.5276218724943415594, -4.786620604624113540, 33.94971097300155805 ) ) ;
#75985=CARTESIAN_POINT ( 'NONE',  ( -13.38461538461538325, -12.29105614889573062, 35.45975837776705220 ) ) ;
#75986=CARTESIAN_POINT ( 'NONE',  ( 4.023698944407932743, -4.460286881179643004, 33.72017969459903242 ) ) ;
#75987=CARTESIAN_POINT ( 'NONE',  ( -4.088591014333315066, -6.835583212224609184, 34.95778746994559327 ) ) ;
#75988=VERTEX_POINT ( 'NONE', #49854 ) ;
#75990=B_SPLINE_CURVE_WITH_KNOTS ( 'NONE', 3,
 ( #73739, #11127, #45797, #31855, #12032, #88154, #38605, #25536, #66970, #5264 ),
 .UNSPECIFIED., .F., .F.,
 ( 4, 2, 2, 2, 4 ),
 ( 0.0007817246256747444619, 0.0009771112852218868158, 0.001172497944769029061, 0.001367884604316171523, 0.001563271263863313769 ),
 .UNSPECIFIED. ) ;
#75991=ORIENTED_EDGE ( 'NONE', *, *, #42850, .F. ) ;
#75994=ORIENTED_EDGE ( 'NONE', *, *, #46138, .T. ) ;
#75995=DIRECTION ( 'NONE',  ( -0.000000000000000000, -0.9848077530122086864, -0.1736481776669273613 ) ) ;
#75996=CARTESIAN_POINT ( 'NONE',  ( -17.07692307692307665, -3.322132147404559976, 32.92929555188717927 ) ) ;
#75997=EDGE_LOOP ( 'NONE', ( #10391, #65456, #55826, #46746 ) ) ;
#75998=FACE_OUTER_BOUND ( 'NONE', #20539, .T. ) ;
#75999=CARTESIAN_POINT ( 'NONE',  ( 12.59206389977210705, -9.503571793651731880, 34.60286762892837942 ) ) ;
#76000=AXIS2_PLACEMENT_3D ( 'NONE', #807, #8015, #14323 ) ;
#76001=ORIENTED_EDGE ( 'NONE', *, *, #1512, .F. ) ;
#76002=FACE_BOUND ( 'NONE', #29695, .T. ) ;
#76003=CARTESIAN_POINT ( 'NONE',  ( 10.74591031714818001, -10.19071101563364756, 33.96452234770658407 ) ) ;
#76004=CARTESIAN_POINT ( 'NONE',  ( 15.93036122928182330, -2.612411019501191589, 31.66733052389440672 ) ) ;
#76005=EDGE_CURVE ( 'NONE', #65429, #69108, #19619, .T. ) ;
#76006=CARTESIAN_POINT ( 'NONE',  ( 12.33084785842815378, -6.369640206132551441, 34.87707690430378449 ) ) ;
#76007=CARTESIAN_POINT ( 'NONE',  ( 17.99999999999987566, -3.083524468854526912, 32.58852847137268327 ) ) ;
#76008=DIRECTION ( 'NONE',  ( -0.000000000000000000, -0.000000000000000000, -1.000000000000000000 ) ) ;
#76009=DIRECTION ( 'NONE',  ( -0.000000000000000000, -0.8660254037844399289, -0.4999999999999980016 ) ) ;
#76011=ORIENTED_EDGE ( 'NONE', *, *, #64216, .F. ) ;
#76012=FACE_OUTER_BOUND ( 'NONE', #37929, .T. ) ;
#76014=ORIENTED_EDGE ( 'NONE', *, *, #15951, .T. ) ;
#76015=CARTESIAN_POINT ( 'NONE',  ( 14.08420736396836226, -10.11188796281391511, 34.01382737946119050 ) ) ;
#76017=ORIENTED_EDGE ( 'NONE', *, *, #86259, .T. ) ;
#76018=CARTESIAN_POINT ( 'NONE',  ( 17.86930853333243618, -5.582088688514999397, 34.36776431015576350 ) ) ;
#76019=CYLINDRICAL_SURFACE ( 'NONE', #55888, 0.2499999999999986955 ) ;
#76020=FACE_BOUND ( 'NONE', #27969, .T. ) ;
#76021=CARTESIAN_POINT ( 'NONE',  ( 6.923076923076924238, -3.937682226553329556, 33.60647404775216529 ) ) ;
#76022=CARTESIAN_POINT ( 'NONE',  ( 4.023698184114455678, -12.50552854090298993, 31.33409797877408920 ) ) ;
#76023=CARTESIAN_POINT ( 'NONE',  ( 2.084207383127978375, -6.716662450894490100, 34.94144148231605840 ) ) ;
#76024=EDGE_CURVE ( 'NONE', #47623, #1510, #43234, .T. ) ;
#76025=CARTESIAN_POINT ( 'NONE',  ( -1.384615384615076605, -2.506253911140615021, 30.00000000000323297 ) ) ;
#76028=CARTESIAN_POINT ( 'NONE',  ( -17.86947429823644029, -5.195472089885680766, 34.18748526763464923 ) ) ;
#76031=ORIENTED_EDGE ( 'NONE', *, *, #24615, .F. ) ;
#76032=VECTOR ( 'NONE', #51098, 999.9999999999998863 ) ;
#76033=CARTESIAN_POINT ( 'NONE',  ( -9.626239341305252495, -11.69971097300155272, 32.46337939537588113 ) ) ;
#76034=CARTESIAN_POINT ( 'NONE',  ( -0.6844646790546086157, -2.758268499246657068, 31.33685645148949561 ) ) ;
#76035=CARTESIAN_POINT ( 'NONE',  ( 1.634560793993430128, -9.357781135181031829, 34.66075350412533851 ) ) ;
#76036=CARTESIAN_POINT ( 'NONE',  ( -16.82697755857493149, -11.37275283266504111, 32.91324779482534524 ) ) ;
#76037=CARTESIAN_POINT ( 'NONE',  ( 3.164685819813350953, -11.16473453929635440, 33.15142922261925662 ) ) ;
#76039=CARTESIAN_POINT ( 'NONE',  ( 0.7115928814519132395, -4.074993327901524687, 33.72946981652012255 ) ) ;
#76040=FACE_OUTER_BOUND ( 'NONE', #67235, .T. ) ;
#76042=CARTESIAN_POINT ( 'NONE',  ( -18.00000000000012079, -11.06231777344772027, 33.60647404775119895 ) ) ;
#76044=CARTESIAN_POINT ( 'NONE',  ( 14.30769230769231015, -1.367168528481310208, 33.57946703557072254 ) ) ;
#76045=CARTESIAN_POINT ( 'NONE',  ( 5.076923076922953193, -8.656820664282941280, 34.87096338111179961 ) ) ;
#76046=CARTESIAN_POINT ( 'NONE',  ( -5.777220331021932331, -11.60474049983371003, 33.02348890104160262 ) ) ;
#76047=EDGE_CURVE ( 'NONE', #70917, #2073, #35464, .T. ) ;
#76048=EDGE_CURVE ( 'NONE', #68235, #70953, #44331, .T. ) ;
#76049=CARTESIAN_POINT ( 'NONE',  ( -14.17716660592874689, -3.285477652293413264, 32.44071101563363158 ) ) ;
#76051=ORIENTED_EDGE ( 'NONE', *, *, #10786, .F. ) ;
#76052=CARTESIAN_POINT ( 'NONE',  ( -0.4615384615384611200, -3.513871655860378418, 32.76840700105978499 ) ) ;
#76053=FACE_OUTER_BOUND ( 'NONE', #58731, .T. ) ;
#76055=EDGE_CURVE ( 'NONE', #34772, #64564, #57942, .T. ) ;
#76056=CARTESIAN_POINT ( 'NONE',  ( -0.2385256174450670896, -10.77377354290276301, 33.85451476688484718 ) ) ;
#76059=DIRECTION ( 'NONE',  ( 0.000000000000000000, 0.1736481776669275834, 0.9848077530122086864 ) ) ;
#76060=CARTESIAN_POINT ( 'NONE',  ( -9.692307692307812417, -5.219633306517616589, 34.19971097300220464 ) ) ;
#76061=ORIENTED_EDGE ( 'NONE', *, *, #22450, .F. ) ;
#76062=CARTESIAN_POINT ( 'NONE',  ( 9.915320536401090123, -12.64618726649961289, 30.78989965857442712 ) ) ;
#76063=CARTESIAN_POINT ( 'NONE',  ( -9.627052552794856055, -5.941354392334607049, 34.76329471203374055 ) ) ;
#76064=ORIENTED_EDGE ( 'NONE', *, *, #85476, .F. ) ;
#76065=CARTESIAN_POINT ( 'NONE',  ( 11.53846153846153832, -9.058645607665452459, 34.76329471203371924 ) ) ;
#76066=CARTESIAN_POINT ( 'NONE',  ( 7.780829833349539371, -7.749976730030849303, 34.74374725381503737 ) ) ;
#76067=ORIENTED_EDGE ( 'NONE', *, *, #38703, .T. ) ;
#76068=CARTESIAN_POINT ( 'NONE',  ( 14.05766907039934210, -2.587272538249754117, 30.68239716806877837 ) ) ;
#76069=CARTESIAN_POINT ( 'NONE',  ( 8.769230769230645706, -6.835583212225970762, 34.95778746994575670 ) ) ;
#76070=DIRECTION ( 'NONE',  ( -0.000000000000000000, -0.1736481776669307198, -0.9848077530122080203 ) ) ;
#76071=VERTEX_POINT ( 'NONE', #66024 ) ;
#76072=B_SPLINE_CURVE_WITH_KNOTS ( 'NONE', 3,
 ( #15652, #35925, #57509, #84997, #70590, #15212, #9768, #57954, #77343, #43552 ),
 .UNSPECIFIED., .F., .F.,
 ( 4, 2, 2, 2, 4 ),
 ( 0.000000000000000000, 0.0001954311564186868473, 0.0003908623128373736946, 0.0005862934692560605419, 0.0007817246256747473893 ),
 .UNSPECIFIED. ) ;
#76074=CARTESIAN_POINT ( 'NONE',  ( 15.48071474911737333, -10.76462480002816235, 33.53768742498949962 ) ) ;
#76075=CIRCLE ( 'NONE', #53040, 0.2500000000000002220 ) ;
#76076=ORIENTED_EDGE ( 'NONE', *, *, #68016, .F. ) ;
#76077=CARTESIAN_POINT ( 'NONE',  ( -11.53846153846153655, -2.499999999999998668, 29.50000000000001066 ) ) ;
#76078=CARTESIAN_POINT ( 'NONE',  ( -5.326946301144532825, -9.356822207818506598, 34.66110646841856635 ) ) ;
#76080=DIRECTION ( 'NONE',  ( -0.000000000000000000, 0.9848077530122085754, -0.1736481776669273613 ) ) ;
#76081=CARTESIAN_POINT ( 'NONE',  ( -4.284537620513710010, -6.413092428213692742, 34.63065189839063152 ) ) ;
#76082=DIRECTION ( 'NONE',  ( -0.000000000000000000, -0.9396926207859092051, -0.3420201433256662704 ) ) ;
#76083=CARTESIAN_POINT ( 'NONE',  ( 6.923076923076800782, -2.379036618888197729, 30.90682066428292885 ) ) ;
#76084=ORIENTED_EDGE ( 'NONE', *, *, #49182, .F. ) ;
#76085=EDGE_LOOP ( 'NONE', ( #21929, #1189 ) ) ;
#76086=CARTESIAN_POINT ( 'NONE',  ( 6.989144256427000101, -12.62096338111211757, 30.90682066428152908 ) ) ;
#76087=ORIENTED_EDGE ( 'NONE', *, *, #58679, .F. ) ;
#76088=CARTESIAN_POINT ( 'NONE',  ( 11.53846153846153832, -8.810774026931790459, 35.74407628777942847 ) ) ;
#76089=ORIENTED_EDGE ( 'NONE', *, *, #47617, .F. ) ;
#76090=B_SPLINE_CURVE_WITH_KNOTS ( 'NONE', 3,
 ( #54965, #69371, #906, #56734, #7672, #62160, #13534, #20733, #35134, #70249 ),
 .UNSPECIFIED., .F., .F.,
 ( 4, 2, 2, 2, 4 ),
 ( 0.0007817359430256369448, 0.0009771253907250049969, 0.001172514838424373049, 0.001367904286123741101, 0.001563293733823109153 ),
 .UNSPECIFIED. ) ;
#76092=CARTESIAN_POINT ( 'NONE',  ( 11.78851595837499566, -3.435999193479609914, 33.07426656108010832 ) ) ;
#76093=CARTESIAN_POINT ( 'NONE',  ( 5.326977388561388693, -3.627508038966690496, 32.91356715214248396 ) ) ;
#76094=ORIENTED_EDGE ( 'NONE', *, *, #2613, .F. ) ;
#76096=EDGE_CURVE ( 'NONE', #10551, #535, #69089, .T. ) ;
#76098=VERTEX_POINT ( 'NONE', #4334 ) ;
#76099=B_SPLINE_CURVE_WITH_KNOTS ( 'NONE', 3,
 ( #58616, #9989, #10447, #23939, #44202, #31143, #24384, #18096, #37916, #64474 ),
 .UNSPECIFIED., .F., .F.,
 ( 4, 2, 2, 2, 4 ),
 ( 0.000000000000000000, 0.0001954311564186876876, 0.0003908623128373753751, 0.0005862934692560630356, 0.0007817246256747507503 ),
 .UNSPECIFIED. ) ;
#76100=EDGE_LOOP ( 'NONE', ( #43845, #66559 ) ) ;
#76101=B_SPLINE_CURVE_WITH_KNOTS ( 'NONE', 3,
 ( #73301, #39972, #32319, #66994, #4393, #11605, #32753, #86842, #39085, #46714 ),
 .UNSPECIFIED., .F., .F.,
 ( 4, 2, 2, 2, 4 ),
 ( 0.000000000000000000, 0.0001954311564186879857, 0.0003908623128373759715, 0.0005862934692560640114, 0.0007817246256747519429 ),
 .UNSPECIFIED. ) ;
#76103=EDGE_LOOP ( 'NONE', ( #11638, #61922 ) ) ;
#76105=CARTESIAN_POINT ( 'NONE',  ( 16.02369894440793630, -12.45813303252208648, 30.39737893381572675 ) ) ;
#76106=CARTESIAN_POINT ( 'NONE',  ( 17.07692307692295586, -2.892918686052165622, 31.69288490824153470 ) ) ;
#76107=FACE_BOUND ( 'NONE', #56473, .T. ) ;
#76108=CARTESIAN_POINT ( 'NONE',  ( -14.37296230824862775, -9.528491918058357157, 34.59228464037090589 ) ) ;
#76109=DIRECTION ( 'NONE',  ( -0.000000000000000000, -0.000000000000000000, -1.000000000000000000 ) ) ;
#76110=EDGE_CURVE ( 'NONE', #75887, #66983, #51819, .T. ) ;
#76111=CARTESIAN_POINT ( 'NONE',  ( 9.627037691751372250, -11.67786785259540849, 32.92929555188721480 ) ) ;
#76112=CARTESIAN_POINT ( 'NONE',  ( -0.3310130233048200754, -3.068774925481847937, 32.56582465632704526 ) ) ;
#76113=CARTESIAN_POINT ( 'NONE',  ( 5.207714884747860928, -10.54018710029568595, 33.71981072465678864 ) ) ;
#76114=CARTESIAN_POINT ( 'NONE',  ( -9.942307692307704059, -2.249999999999999556, 29.81609741502489541 ) ) ;
#76115=ORIENTED_EDGE ( 'NONE', *, *, #52025, .T. ) ;
#76116=DIRECTION ( 'NONE',  ( 0.000000000000000000, -6.938893903907222067E-15, 1.000000000000000000 ) ) ;
#76119=ORIENTED_EDGE ( 'NONE', *, *, #28146, .F. ) ;
#76120=CARTESIAN_POINT ( 'NONE',  ( 2.057715576749954867, -10.66389620160130036, 33.62221079203477103 ) ) ;
#76121=FACE_OUTER_BOUND ( 'NONE', #29670, .T. ) ;
#76122=CARTESIAN_POINT ( 'NONE',  ( 6.989145274079363368, -6.386643153685127139, 34.62446782046654192 ) ) ;
#76123=CARTESIAN_POINT ( 'NONE',  ( -17.07692307692319744, -10.33852847137269571, 34.16647553114546554 ) ) ;
#76124=CARTESIAN_POINT ( 'NONE',  ( 15.29683758177167086, -3.513871655860379306, 32.76840700105978499 ) ) ;
#76125=CARTESIAN_POINT ( 'NONE',  ( -12.23852561744506673, -4.762714258010881885, 34.23016756924214832 ) ) ;
#76126=EDGE_LOOP ( 'NONE', ( #9657, #67666, #76263, #3086 ) ) ;
#76128=CARTESIAN_POINT ( 'NONE',  ( -14.37377468705243722, -9.905515769479276145, 34.41647553114623292 ) ) ;
#76129=CARTESIAN_POINT ( 'NONE',  ( -14.08467946359890988, -12.38742843783360748, 31.66772728687926985 ) ) ;
#76130=EDGE_CURVE ( 'NONE', #13183, #83315, #59346, .T. ) ;
#76131=CARTESIAN_POINT ( 'NONE',  ( 15.29683656411930848, -12.34228464037088813, 31.77849191805839268 ) ) ;
#76132=ORIENTED_EDGE ( 'NONE', *, *, #32880, .F. ) ;
#76133=ORIENTED_EDGE ( 'NONE', *, *, #30600, .T. ) ;
#76134=ORIENTED_EDGE ( 'NONE', *, *, #23262, .F. ) ;
#76136=LINE ( 'NONE', #55867, #79410 ) ;
#76137=ORIENTED_EDGE ( 'NONE', *, *, #22291, .T. ) ;
#76138=CARTESIAN_POINT ( 'NONE',  ( -6.923076923076922462, -11.11383981884818262, 36.00935417666054406 ) ) ;
#76140=CARTESIAN_POINT ( 'NONE',  ( 1.384615384615386802, -6.681629849574314051, 35.83090037661290239 ) ) ;
#76141=CARTESIAN_POINT ( 'NONE',  ( -2.177166605928743337, -5.195472089885680766, 34.18748526763464923 ) ) ;
#76142=CARTESIAN_POINT ( 'NONE',  ( -11.47239318745910097, -6.386643153685127139, 34.62446782046654192 ) ) ;
#76144=DIRECTION ( 'NONE',  ( -0.000000000000000000, 0.1736481776669307198, -0.9848077530122080203 ) ) ;
#76145=CARTESIAN_POINT ( 'NONE',  ( -11.53846153846153655, -12.09954503811598769, 35.62045528018868623 ) ) ;
#76146=VERTEX_POINT ( 'NONE', #51607 ) ;
#76147=CARTESIAN_POINT ( 'NONE',  ( 3.230769230769231726, -13.57706302396349152, 30.56769352161908060 ) ) ;
#76148=DIRECTION ( 'NONE',  ( 0.000000000000000000, 0.9848077530122072432, 0.1736481776669354937 ) ) ;
#76149=CARTESIAN_POINT ( 'NONE',  ( 17.32697738856138869, -11.28795663066794575, 33.01431243580653785 ) ) ;
#76150=CARTESIAN_POINT ( 'NONE',  ( 8.834485908743603844, -12.16647553114626490, 32.15551576947920864 ) ) ;
#76151=CARTESIAN_POINT ( 'NONE',  ( -12.46153846153858247, -2.892918686052166066, 31.69288490824153470 ) ) ;
#76152=ADVANCED_FACE ( 'NONE', ( #4787 ), #79103, .F. ) ;
#76153=CARTESIAN_POINT ( 'NONE',  ( 16.94631271729854660, -7.722926236386454590, 34.74524107206102030 ) ) ;
#76154=CARTESIAN_POINT ( 'NONE',  ( -3.480769230769229061, -7.500000000000001776, 35.00000000000000000 ) ) ;
#76157=ORIENTED_EDGE ( 'NONE', *, *, #52960, .F. ) ;
#76158=CARTESIAN_POINT ( 'NONE',  ( -17.01085472592064107, -10.51840700105979565, 33.73612834413962247 ) ) ;
#76160=VECTOR ( 'NONE', #77568, 1000.000000000000227 ) ;
#76161=AXIS2_PLACEMENT_3D ( 'NONE', #53832, #17385, #38098 ) ;
#76162=EDGE_CURVE ( 'NONE', #43657, #56137, #60293, .T. ) ;
#76163=CYLINDRICAL_SURFACE ( 'NONE', #34605, 0.2499999999999973355 ) ;
#76164=CARTESIAN_POINT ( 'NONE',  ( 9.469380733400843297, -6.459968553980841577, 34.89616026154728701 ) ) ;
#76167=DIRECTION ( 'NONE',  ( -0.000000000000000000, 0.1736481776669307198, -0.9848077530122080203 ) ) ;
#76168=CARTESIAN_POINT ( 'NONE',  ( -5.076923076923197442, -6.879047030192662504, 34.71129190930017927 ) ) ;
#76169=AXIS2_PLACEMENT_3D ( 'NONE', #34505, #14681, #40825 ) ;
#76170=VECTOR ( 'NONE', #74341, 1000.000000000000000 ) ;
#76171=LINE ( 'NONE', #76621, #37317 ) ;
#76172=CARTESIAN_POINT ( 'NONE',  ( -17.07692307692319744, -3.835265460704628815, 33.15142922262033665 ) ) ;
#76173=AXIS2_PLACEMENT_3D ( 'NONE', #71725, #18133, #72620 ) ;
#76175=CARTESIAN_POINT ( 'NONE',  ( 12.21153846153844569, -2.249999999999998668, 29.81609741502487765 ) ) ;
#76177=CARTESIAN_POINT ( 'NONE',  ( 18.22277966897806678, -12.47679350104403007, 31.42216943046555855 ) ) ;
#76178=ORIENTED_EDGE ( 'NONE', *, *, #48774, .F. ) ;
#76180=ORIENTED_EDGE ( 'NONE', *, *, #53870, .F. ) ;
#76182=LINE ( 'NONE', #77516, #74324 ) ;
#76183=ORIENTED_EDGE ( 'NONE', *, *, #48133, .T. ) ;
#76184=CARTESIAN_POINT ( 'NONE',  ( -18.00000000000012079, -10.33852847137269926, 34.16647553114546554 ) ) ;
#76185=CARTESIAN_POINT ( 'NONE',  ( -14.30769230769230660, -5.180354513474913603, 36.12317359536750416 ) ) ;
#76186=CARTESIAN_POINT ( 'NONE',  ( -6.923076923076922462, -12.34228464037088635, 31.77849191805839268 ) ) ;
#76187=DIRECTION ( 'NONE',  ( -0.000000000000000000, -0.9396926207859093161, -0.3420201433256663259 ) ) ;
#76188=CARTESIAN_POINT ( 'NONE',  ( -0.5276208408985976206, -11.35647404775217595, 33.31231777344666511 ) ) ;
#76190=ORIENTED_EDGE ( 'NONE', *, *, #57622, .F. ) ;
#76191=FACE_BOUND ( 'NONE', #72176, .T. ) ;
#76192=ORIENTED_EDGE ( 'NONE', *, *, #56011, .F. ) ;
#76193=CARTESIAN_POINT ( 'NONE',  ( 5.076923076923075762, -9.058645607665452459, 34.76329471203371924 ) ) ;
#76196=EDGE_CURVE ( 'NONE', #49301, #3368, #61930, .T. ) ;
#76197=CARTESIAN_POINT ( 'NONE',  ( 4.284637961670941131, -11.71459661697925903, 32.44059661609676937 ) ) ;
#76198=DIRECTION ( 'NONE',  ( 0.000000000000000000, 0.9396926207859126468, 0.3420201433256571111 ) ) ;
#76200=ORIENTED_EDGE ( 'NONE', *, *, #70633, .F. ) ;
#76201=EDGE_CURVE ( 'NONE', #79352, #54551, #85032, .T. ) ;
#76202=ORIENTED_EDGE ( 'NONE', *, *, #84194, .T. ) ;
#76203=EDGE_LOOP ( 'NONE', ( #35304, #16788, #82346, #220 ) ) ;
#76204=CARTESIAN_POINT ( 'NONE',  ( -14.30769230769230660, -1.044019251281081972, 31.83374038241031911 ) ) ;
#76205=VERTEX_POINT ( 'NONE', #68696 ) ;
#76206=AXIS2_PLACEMENT_3D ( 'NONE', #86577, #31156, #3246 ) ;
#76207=CARTESIAN_POINT ( 'NONE',  ( -11.53846153846153655, -13.75783147151868846, 33.36296068462461051 ) ) ;
#76208=CARTESIAN_POINT ( 'NONE',  ( -9.942307692307693401, -7.433931650972299465, 34.75000000000000711 ) ) ;
#76209=CARTESIAN_POINT ( 'NONE',  ( -7.846153846153967493, -8.656820664282941280, 34.87096338111179961 ) ) ;
#76210=CARTESIAN_POINT ( 'NONE',  ( -1.134615384613947953, -7.500000000000155431, 34.75000000000007105 ) ) ;
#76211=AXIS2_PLACEMENT_3D ( 'NONE', #70601, #85445, #51626 ) ;
#76212=DIRECTION ( 'NONE',  ( 0.000000000000000000, 0.4999999999999960032, -0.8660254037844410391 ) ) ;
#76213=CARTESIAN_POINT ( 'NONE',  ( -18.25000000000000711, -7.569194476968191587, 35.00000000000000000 ) ) ;
#76214=CARTESIAN_POINT ( 'NONE',  ( 17.32686859527121825, -2.587454068350149239, 30.68340429815432557 ) ) ;
#76215=VERTEX_POINT ( 'NONE', #47087 ) ;
#76216=EDGE_CURVE ( 'NONE', #18497, #66197, #13312, .T. ) ;
#76217=EDGE_LOOP ( 'NONE', ( #48336, #17714, #79716, #58711 ) ) ;
#76219=CARTESIAN_POINT ( 'NONE',  ( -4.088590582570128973, -10.21337939537593620, 33.94971097300152252 ) ) ;
#76220=CARTESIAN_POINT ( 'NONE',  ( 1.634560902963528850, -5.852078868378310261, 34.47109172314383585 ) ) ;
#76221=LINE ( 'NONE', #29822, #43404 ) ;
#76222=AXIS2_PLACEMENT_3D ( 'NONE', #20470, #13268, #75412 ) ;
#76223=CARTESIAN_POINT ( 'NONE',  ( -17.77722033102192967, -5.827830569534416583, 34.72679350104403539 ) ) ;
#76224=CARTESIAN_POINT ( 'NONE',  ( 12.71159288145191013, -12.65882529074907126, 30.72640787790839312 ) ) ;
#76225=FACE_BOUND ( 'NONE', #82666, .T. ) ;
#76226=CARTESIAN_POINT ( 'NONE',  ( 8.638540166120462160, -10.70098750199973203, 33.91152734681376302 ) ) ;
#76227=ORIENTED_EDGE ( 'NONE', *, *, #26707, .T. ) ;
#76229=B_SPLINE_CURVE_WITH_KNOTS ( 'NONE', 3,
 ( #22103, #2253, #42388, #56765, #1383, #1823, #63520, #21208, #28874, #83820 ),
 .UNSPECIFIED., .F., .F.,
 ( 4, 2, 2, 2, 4 ),
 ( 0.000000000000000000, 0.0001954311564186869015, 0.0003908623128373738030, 0.0005862934692560607588, 0.0007817246256747476061 ),
 .UNSPECIFIED. ) ;
#76231=FACE_OUTER_BOUND ( 'NONE', #46652, .T. ) ;
#76232=CARTESIAN_POINT ( 'NONE',  ( 3.480714640147274164, -11.56426240980093567, 33.07394671870546432 ) ) ;
#76233=ORIENTED_EDGE ( 'NONE', *, *, #53761, .T. ) ;
#76234=CARTESIAN_POINT ( 'NONE',  ( 18.00000000000000000, -12.37446782046654192, 30.86335684631486131 ) ) ;
#76235=ORIENTED_EDGE ( 'NONE', *, *, #45508, .F. ) ;
#76236=FACE_BOUND ( 'NONE', #29196, .T. ) ;
#76237=CARTESIAN_POINT ( 'NONE',  ( -17.32689982097166848, -4.075325502946085976, 33.72974371597207721 ) ) ;
#76238=CARTESIAN_POINT ( 'NONE',  ( 3.230769230769231726, -13.87047571288749737, 32.06866353760679544 ) ) ;
#76239=CARTESIAN_POINT ( 'NONE',  ( 17.07692307692295586, -12.16647553114689728, 32.15551576947799362 ) ) ;
#76241=CARTESIAN_POINT ( 'NONE',  ( 0.4615384615383396616, -10.90142922262034020, 33.41473453929536674 ) ) ;
#76242=CARTESIAN_POINT ( 'NONE',  ( 20.74999999999999645, -12.50000000000000000, 29.75000000000000355 ) ) ;
#76243=CARTESIAN_POINT ( 'NONE',  ( 8.519207545009313876, -8.475808217655753651, 34.90892951860618609 ) ) ;
#76244=CARTESIAN_POINT ( 'NONE',  ( -7.146003140593069070, -10.61292498521070549, 33.66303323003028680 ) ) ;
#76245=EDGE_LOOP ( 'NONE', ( #50707, #79073, #37598, #54461 ) ) ;
#76246=CARTESIAN_POINT ( 'NONE',  ( -4.946132635956127288, -4.684288915650984819, 34.18129842949671371 ) ) ;
#76247=ORIENTED_EDGE ( 'NONE', *, *, #9308, .T. ) ;
#76249=ORIENTED_EDGE ( 'NONE', *, *, #54149, .T. ) ;
#76250=CARTESIAN_POINT ( 'NONE',  ( 9.627037246346921151, -3.835265460703609186, 33.15142922261924241 ) ) ;
#76251=CARTESIAN_POINT ( 'NONE',  ( -4.376772371362299019, -2.758268499246657957, 31.33685645148948140 ) ) ;
#76252=DIRECTION ( 'NONE',  ( 0.000000000000000000, 0.3420201433256641055, -0.9396926207859100932 ) ) ;
#76253=CARTESIAN_POINT ( 'NONE',  ( 14.05771557674995442, -9.148715823498378086, 34.47080413974185120 ) ) ;
#76254=CARTESIAN_POINT ( 'NONE',  ( 9.942253210655836781, -9.272278438253398036, 34.42582936511637115 ) ) ;
#76255=CARTESIAN_POINT ( 'NONE',  ( 13.63466969625370062, -5.728107161865378494, 34.42597550085002922 ) ) ;
#76256=CARTESIAN_POINT ( 'NONE',  ( 13.38461538461538680, -5.180354513474913603, 36.12317359536750416 ) ) ;
#76257=ADVANCED_FACE ( 'NONE', ( #27707 ), #40351, .F. ) ;
#76258=ADVANCED_FACE ( 'NONE', ( #88995 ), #6118, .F. ) ;
#76259=DIRECTION ( 'NONE',  ( -0.000000000000000000, 0.9848077530122085754, -0.1736481776669273613 ) ) ;
#76260=AXIS2_PLACEMENT_3D ( 'NONE', #57537, #42712, #8035 ) ;
#76263=ORIENTED_EDGE ( 'NONE', *, *, #78246, .T. ) ;
#76264=CARTESIAN_POINT ( 'NONE',  ( 17.93472955403921887, -4.481592998940161721, 33.73612834413957984 ) ) ;
#76265=ORIENTED_EDGE ( 'NONE', *, *, #19530, .T. ) ;
#76268=CARTESIAN_POINT ( 'NONE',  ( 3.100622021331010725, -5.195881422630167279, 34.18770438780618548 ) ) ;
#76271=CARTESIAN_POINT ( 'NONE',  ( -4.283994123577852697, -2.647304123082328875, 31.75400227202885262 ) ) ;
#76272=CARTESIAN_POINT ( 'NONE',  ( -11.47320639894870276, -10.33852847137154107, 34.16647553114620450 ) ) ;
#76273=CARTESIAN_POINT ( 'NONE',  ( -15.90390063549801347, -5.852078868378312038, 34.47109172314383585 ) ) ;
#76274=DIRECTION ( 'NONE',  ( 0.000000000000000000, 0.9848077530122072432, 0.1736481776669354937 ) ) ;
#76276=CARTESIAN_POINT ( 'NONE',  ( -8.992715693795103604, -2.612411019501189369, 31.66733052389439962 ) ) ;
#76277=B_SPLINE_CURVE_WITH_KNOTS ( 'NONE', 3,
 ( #1891, #63588, #84327, #70804, #9106, #36569, #22601, #34786, #76213, #62253 ),
 .UNSPECIFIED., .F., .F.,
 ( 4, 2, 2, 2, 4 ),
 ( 0.5000000000000000000, 0.6250000000000000000, 0.7500000000000000000, 0.8750000000000000000, 1.000000000000000000 ),
 .UNSPECIFIED. ) ;
#76278=LINE ( 'NONE', #29874, #55692 ) ;
#76280=B_SPLINE_CURVE_WITH_KNOTS ( 'NONE', 3,
 ( #72508, #21783, #21336, #55561, #64083, #49694, #1069, #22663, #15479, #36200 ),
 .UNSPECIFIED., .F., .F.,
 ( 4, 2, 2, 2, 4 ),
 ( 0.000000000000000000, 0.0001954339857564078809, 0.0003908679715128157619, 0.0005863019572692236428, 0.0007817359430256315238 ),
 .UNSPECIFIED. ) ;
#76281=CARTESIAN_POINT ( 'NONE',  ( 10.61538461538449596, -2.625532179533778709, 30.86335684631627174 ) ) ;
#76282=CARTESIAN_POINT ( 'NONE',  ( -2.242437168179467477, -3.083524468853784839, 32.58852847137153930 ) ) ;
#76283=AXIS2_PLACEMENT_3D ( 'NONE', #62050, #28259, #63820 ) ;
#76284=ADVANCED_FACE ( 'NONE', ( #80904 ), #61051, .F. ) ;
#76285=CARTESIAN_POINT ( 'NONE',  ( -11.78846153846153832, -2.499999999999998668, 29.75000000000000355 ) ) ;
#76286=CARTESIAN_POINT ( 'NONE',  ( -0.2115384615384616196, -2.499999999999998668, 29.75000000000000355 ) ) ;
#76288=VERTEX_POINT ( 'NONE', #32689 ) ;
#76289=ORIENTED_EDGE ( 'NONE', *, *, #59473, .T. ) ;
#76290=CARTESIAN_POINT ( 'NONE',  ( 2.980746006547773330, -10.92453946501458439, 33.72985991061850086 ) ) ;
#76291=CARTESIAN_POINT ( 'NONE',  ( 15.48071464014727283, -12.07971442181322352, 32.31769673815850297 ) ) ;
#76292=FACE_OUTER_BOUND ( 'NONE', #53369, .T. ) ;
#76293=EDGE_CURVE ( 'NONE', #37810, #8955, #36686, .T. ) ;
#76294=CARTESIAN_POINT ( 'NONE',  ( 0.3308478584281519530, -9.929715669179216775, 34.40415004197138416 ) ) ;
#76295=VECTOR ( 'NONE', #9270, 1000.000000000000000 ) ;
#76296=CARTESIAN_POINT ( 'NONE',  ( 9.915320536401090123, -11.43677907613344757, 33.22367315496202167 ) ) ;
#76298=CARTESIAN_POINT ( 'NONE',  ( -9.627052552794850726, -11.06231777344671130, 33.60647404775212976 ) ) ;
#76299=CARTESIAN_POINT ( 'NONE',  ( -5.999999999999683808, -2.255955759149395501, 30.00000000000324363 ) ) ;
#76300=ADVANCED_FACE ( 'NONE', ( #55617 ), #23169, .F. ) ;
#76301=EDGE_LOOP ( 'NONE', ( #70307, #18637 ) ) ;
#76302=CARTESIAN_POINT ( 'NONE',  ( -13.63459211555773720, -9.943427161483782584, 34.11278801902876978 ) ) ;
#76303=ORIENTED_EDGE ( 'NONE', *, *, #68513, .F. ) ;
#76304=EDGE_CURVE ( 'NONE', #44682, #21602, #8777, .T. ) ;
#76305=CARTESIAN_POINT ( 'NONE',  ( -18.00000000000000000, -1.973681607567911556, 34.71348354719103924 ) ) ;
#76306=CARTESIAN_POINT ( 'NONE',  ( 15.29683656411930848, -3.322132147404559976, 32.92929555188717927 ) ) ;
#76307=CARTESIAN_POINT ( 'NONE',  ( -6.857932142357289429, -7.750023224968867197, 34.99404313364389907 ) ) ;
#76308=CARTESIAN_POINT ( 'NONE',  ( 3.903822929624695792, -6.652501968072646932, 34.93155406624980941 ) ) ;
#76309=FACE_OUTER_BOUND ( 'NONE', #87194, .T. ) ;
#76310=ORIENTED_EDGE ( 'NONE', *, *, #19738, .T. ) ;
#76311=ADVANCED_FACE ( 'NONE', ( #69142 ), #29494, .F. ) ;
#76312=ORIENTED_EDGE ( 'NONE', *, *, #20312, .F. ) ;
#76313=ORIENTED_EDGE ( 'NONE', *, *, #7407, .T. ) ;
#76314=VERTEX_POINT ( 'NONE', #14644 ) ;
#76315=ADVANCED_FACE ( 'NONE', ( #76793 ), #7449, .F. ) ;
#76316=CARTESIAN_POINT ( 'NONE',  ( -10.61538461538461320, -12.34228464037088635, 31.77849191805839268 ) ) ;
#76317=CARTESIAN_POINT ( 'NONE',  ( -16.08777882049607655, -9.058645607665452459, 34.76329471203371924 ) ) ;
#76318=AXIS2_PLACEMENT_3D ( 'NONE', #53119, #45028, #33313 ) ;
#76319=CARTESIAN_POINT ( 'NONE',  ( -13.38461538461538325, -11.33034616979429110, 35.88435417666054406 ) ) ;
#76320=CARTESIAN_POINT ( 'NONE',  ( 11.31497659473759043, -12.24155766932282496, 31.33739205006857986 ) ) ;
#76323=ORIENTED_EDGE ( 'NONE', *, *, #71896, .T. ) ;
#76324=EDGE_CURVE ( 'NONE', #25936, #80774, #64578, .T. ) ;
#76325=ORIENTED_EDGE ( 'NONE', *, *, #45480, .F. ) ;
#76326=VERTEX_POINT ( 'NONE', #9227 ) ;
#76328=ORIENTED_EDGE ( 'NONE', *, *, #7796, .T. ) ;
#76329=EDGE_CURVE ( 'NONE', #43687, #10616, #76409, .T. ) ;
#76330=DIRECTION ( 'NONE',  ( 0.000000000000000000, 0.9848077530122072432, 0.1736481776669354937 ) ) ;
#76331=CARTESIAN_POINT ( 'NONE',  ( 14.43848274865925774, -4.684288915650983043, 34.18129842949671371 ) ) ;
#76332=CARTESIAN_POINT ( 'NONE',  ( -5.076923076923075762, -11.16473453929635440, 33.15142922261926373 ) ) ;
#76334=ORIENTED_EDGE ( 'NONE', *, *, #88271, .F. ) ;
#76336=VERTEX_POINT ( 'NONE', #70476 ) ;
#76337=CARTESIAN_POINT ( 'NONE',  ( -17.75005459062195712, -2.986452184633680229, 32.43230066228895225 ) ) ;
#76339=FACE_BOUND ( 'NONE', #81754, .T. ) ;
#76340=CARTESIAN_POINT ( 'NONE',  ( -5.749945580086545327, -2.920487667080175154, 32.31805714834170828 ) ) ;
#76345=CARTESIAN_POINT ( 'NONE',  ( 8.546303810323918171, -11.98009711892699514, 32.48740034544076138 ) ) ;
#76346=CARTESIAN_POINT ( 'NONE',  ( 10.48469314871706182, -2.729777683071817229, 31.24903638046269450 ) ) ;
#76347=CARTESIAN_POINT ( 'NONE',  ( 0.7114839798866029463, -6.696923467548660192, 34.68552623307873972 ) ) ;
#76348=CARTESIAN_POINT ( 'NONE',  ( 14.17754433796061875, -9.504002272028875709, 34.60269587691767867 ) ) ;
#76349=ORIENTED_EDGE ( 'NONE', *, *, #68657, .F. ) ;
#76350=VECTOR ( 'NONE', #3679, 1000.000000000000114 ) ;
#76351=DIRECTION ( 'NONE',  ( 0.000000000000000000, 0.7660444431189822323, -0.6427876096865344779 ) ) ;
#76352=CARTESIAN_POINT ( 'NONE',  ( -12.21159305216042057, -2.341251567377310217, 30.72681386836322659 ) ) ;
#76353=CARTESIAN_POINT ( 'NONE',  ( 1.515141086378950730, -8.586989748646450593, 34.63063291749215011 ) ) ;
#76354=CARTESIAN_POINT ( 'NONE',  ( 0.2380535178145146147, -11.89387501736623420, 32.13663884655804992 ) ) ;
#76356=DIRECTION ( 'NONE',  ( -0.000000000000000000, -0.6427876096865404731, -0.7660444431189770143 ) ) ;
#76357=FACE_BOUND ( 'NONE', #35164, .T. ) ;
#76358=CARTESIAN_POINT ( 'NONE',  ( -6.700297254098854793, -12.69155399931963046, 30.53255429739158444 ) ) ;
#76359=CARTESIAN_POINT ( 'NONE',  ( -6.222926958906846551, -10.01117774369187252, 34.36070679894347535 ) ) ;
#76360=CARTESIAN_POINT ( 'NONE',  ( 5.326977496836529546, -2.318338780012835443, 30.59689888758630261 ) ) ;
#76361=CARTESIAN_POINT ( 'NONE',  ( 3.930919194939304973, -5.582147617184174848, 34.63737895849758530 ) ) ;
#76362=CARTESIAN_POINT ( 'NONE',  ( -6.223484943723947893, -5.113361153441932316, 34.14387501736621999 ) ) ;
#76363=CARTESIAN_POINT ( 'NONE',  ( -10.86536135943320502, -6.524016743844655686, 34.90889640711025521 ) ) ;
#76365=EDGE_LOOP ( 'NONE', ( #59991, #21559 ) ) ;
#76366=CARTESIAN_POINT ( 'NONE',  ( 12.59206416330202671, -2.619367082507849442, 30.83698974864643461 ) ) ;
#76367=ORIENTED_EDGE ( 'NONE', *, *, #57901, .T. ) ;
#76368=EDGE_CURVE ( 'NONE', #9598, #65911, #48484, .T. ) ;
#76369=CARTESIAN_POINT ( 'NONE',  ( -13.38461538461538325, -10.67929555188718282, 33.92786785259544047 ) ) ;
#76370=B_SPLINE_CURVE_WITH_KNOTS ( 'NONE', 3,
 ( #78922, #24863, #52333, #17678, #38388, #46030, #8815, #79375, #45135, #29529 ),
 .UNSPECIFIED., .F., .F.,
 ( 4, 2, 2, 2, 4 ),
 ( 0.000000000000000000, 0.0001954339857564081791, 0.0003908679715128163582, 0.0005863019572692245102, 0.0007817359430256327164 ),
 .UNSPECIFIED. ) ;
#76372=DIRECTION ( 'NONE',  ( 0.000000000000000000, 0.9848077530122072432, 0.1736481776669354937 ) ) ;
#76373=EDGE_CURVE ( 'NONE', #6248, #41990, #58220, .T. ) ;
#76374=DIRECTION ( 'NONE',  ( -0.000000000000000000, 0.9848077530122086864, -0.1736481776669273891 ) ) ;
#76375=EDGE_LOOP ( 'NONE', ( #41877, #77047 ) ) ;
#76376=FACE_OUTER_BOUND ( 'NONE', #67258, .T. ) ;
#76378=B_SPLINE_CURVE_WITH_KNOTS ( 'NONE', 3,
 ( #23979, #17689, #2818, #4615, #79837, #37053, #18134, #45145, #3713, #85261 ),
 .UNSPECIFIED., .F., .F.,
 ( 4, 2, 2, 2, 4 ),
 ( 0.000000000000000000, 0.0001954339857564097241, 0.0003908679715128194482, 0.0005863019572692291723, 0.0007817359430256388964 ),
 .UNSPECIFIED. ) ;
#76380=CARTESIAN_POINT ( 'NONE',  ( -5.326899807865431491, -4.943428324936578910, 34.04746400365624481 ) ) ;
#76381=CARTESIAN_POINT ( 'NONE',  ( 16.85343813319912698, -12.44517049084099725, 30.48991314939691932 ) ) ;
#76382=CARTESIAN_POINT ( 'NONE',  ( 1.319345384059066761, -5.094484230520674117, 34.41647553114621161 ) ) ;
#76383=CARTESIAN_POINT ( 'NONE',  ( 4.826946345980720920, -8.303909089506435137, 34.68538101551103381 ) ) ;
#76384=DIRECTION ( 'NONE',  ( -0.000000000000000000, 0.9848077530122085754, -0.1736481776669273613 ) ) ;
#76385=EDGE_CURVE ( 'NONE', #59397, #27552, #79896, .T. ) ;
#76386=AXIS2_PLACEMENT_3D ( 'NONE', #49606, #83405, #8631 ) ;
#76388=CARTESIAN_POINT ( 'NONE',  ( -10.39237326377176629, -2.758310577978207778, 31.33698337089302299 ) ) ;
#76389=CARTESIAN_POINT ( 'NONE',  ( -5.999999999999998224, -3.322132147404559976, 32.92929555188717927 ) ) ;
#76390=ORIENTED_EDGE ( 'NONE', *, *, #23837, .F. ) ;
#76392=ADVANCED_FACE ( 'NONE', ( #44301 ), #37561, .F. ) ;
#76395=LINE ( 'NONE', #36739, #15960 ) ;
#76396=CARTESIAN_POINT ( 'NONE',  ( -8.992715693795100051, -3.562934362175800285, 33.22335522853832401 ) ) ;
#76397=ORIENTED_EDGE ( 'NONE', *, *, #16464, .F. ) ;
#76398=CARTESIAN_POINT ( 'NONE',  ( 6.857752910272615132, -7.749976730030849303, 34.74374725381503737 ) ) ;
#76399=CARTESIAN_POINT ( 'NONE',  ( -0.2114841499001461067, -9.943054286541405773, 34.11300777759955594 ) ) ;
#76400=CARTESIAN_POINT ( 'NONE',  ( 2.307692307692309264, -2.721908614388771852, 31.22303859784724978 ) ) ;
#76401=ORIENTED_EDGE ( 'NONE', *, *, #5089, .F. ) ;
#76402=FACE_OUTER_BOUND ( 'NONE', #68521, .T. ) ;
#76404=DIRECTION ( 'NONE',  ( -0.000000000000000000, 0.6427876096865404731, -0.7660444431189771253 ) ) ;
#76406=FACE_OUTER_BOUND ( 'NONE', #60654, .T. ) ;
#76407=CARTESIAN_POINT ( 'NONE',  ( 0.4615384615384611200, -12.34228464037088635, 31.77849191805839268 ) ) ;
#76408=B_SPLINE_CURVE_WITH_KNOTS ( 'NONE', 3,
 ( #44739, #43860, #16834, #65007, #71327, #85306, #57821, #3317, #66359, #52836 ),
 .UNSPECIFIED., .F., .F.,
 ( 4, 2, 2, 2, 4 ),
 ( 0.0007817359430256297891, 0.0009771253907249961065, 0.001172514838424362424, 0.001367904286123728741, 0.001563293733823095059 ),
 .UNSPECIFIED. ) ;
#76409=B_SPLINE_CURVE_WITH_KNOTS ( 'NONE', 3,
 ( #34904, #28149, #8335, #7887, #62805, #35811, #36689, #35353, #28606, #43003 ),
 .UNSPECIFIED., .F., .F.,
 ( 4, 2, 2, 2, 4 ),
 ( 0.000000000000000000, 0.0001954311564186868473, 0.0003908623128373736946, 0.0005862934692560605419, 0.0007817246256747473893 ),
 .UNSPECIFIED. ) ;
#76410=CIRCLE ( 'NONE', #87962, 0.2500000000000002220 ) ;
#76411=VERTEX_POINT ( 'NONE', #78550 ) ;
#76412=CARTESIAN_POINT ( 'NONE',  ( -0.3310127597748971362, -10.88167719472716399, 33.43325721877153711 ) ) ;
#76414=B_SPLINE_CURVE_WITH_KNOTS ( 'NONE', 3,
 ( #50734, #43987, #30479, #71907, #78219, #16521, #51164, #85429, #71458, #17865 ),
 .UNSPECIFIED., .F., .F.,
 ( 4, 2, 2, 2, 4 ),
 ( 0.0007817246256747514008, 0.0009771112852218959231, 0.001172497944769040337, 0.001367884604316184751, 0.001563271263863329165 ),
 .UNSPECIFIED. ) ;
#76415=B_SPLINE_CURVE_WITH_KNOTS ( 'NONE', 3,
 ( #83041, #623, #21327, #54660, #55999, #20881, #88488, #76268, #48796, #35287 ),
 .UNSPECIFIED., .F., .F.,
 ( 4, 2, 2, 2, 4 ),
 ( 0.000000000000000000, 0.0001954339857564070949, 0.0003908679715128141898, 0.0005863019572692212576, 0.0007817359430256283796 ),
 .UNSPECIFIED. ) ;
#76417=ORIENTED_EDGE ( 'NONE', *, *, #39554, .F. ) ;
#76418=AXIS2_PLACEMENT_3D ( 'NONE', #26703, #33469, #55063 ) ;
#76419=CARTESIAN_POINT ( 'NONE',  ( -13.38461538461538325, -3.513871655860378418, 32.76840700105978499 ) ) ;
#76422=CARTESIAN_POINT ( 'NONE',  ( -14.30769230769230660, -10.05456864172156806, 36.03766855953608683 ) ) ;
#76423=DIRECTION ( 'NONE',  ( -0.000000000000000000, 1.000000000000000000, 3.491481338843133355E-15 ) ) ;
#76426=VERTEX_POINT ( 'NONE', #16855 ) ;
#76427=VERTEX_POINT ( 'NONE', #17755 ) ;
#76428=EDGE_CURVE ( 'NONE', #47964, #30991, #72687, .T. ) ;
#76429=ORIENTED_EDGE ( 'NONE', *, *, #72178, .T. ) ;
#76430=CARTESIAN_POINT ( 'NONE',  ( 4.403791563224197070, -12.45601412856602863, 31.48342859153981621 ) ) ;
#76431=EDGE_LOOP ( 'NONE', ( #87972, #9832, #73896, #44598 ) ) ;
#76432=CARTESIAN_POINT ( 'NONE',  ( -0.5922299282060200509, -4.809359713505814149, 33.96456829005828837 ) ) ;
#76433=CARTESIAN_POINT ( 'NONE',  ( 5.750023255951410839, -12.65889640711025521, 30.72598325615533454 ) ) ;
#76434=CARTESIAN_POINT ( 'NONE',  ( -3.007757879156381264, -4.187068189119697692, 33.49521262558774026 ) ) ;
#76435=DIRECTION ( 'NONE',  ( -0.000000000000000000, 0.7660444431189791237, -0.6427876096865379196 ) ) ;
#76436=VERTEX_POINT ( 'NONE', #3336 ) ;
#76437=EDGE_CURVE ( 'NONE', #7171, #68701, #65026, .T. ) ;
#76438=ORIENTED_EDGE ( 'NONE', *, *, #20596, .F. ) ;
#76439=B_SPLINE_CURVE_WITH_KNOTS ( 'NONE', 3,
 ( #31137, #37453, #23063, #24377, #10883, #51845, #37910, #50521, #65808, #79341 ),
 .UNSPECIFIED., .F., .F.,
 ( 4, 2, 2, 2, 4 ),
 ( 0.000000000000000000, 0.0001954311564186860071, 0.0003908623128373720141, 0.0005862934692560580483, 0.0007817246256747440282 ),
 .UNSPECIFIED. ) ;
#76442=CARTESIAN_POINT ( 'NONE',  ( 1.161689167099238640, -8.239355502252617924, 34.69524867566427417 ) ) ;
#76443=VERTEX_POINT ( 'NONE', #10995 ) ;
#76444=B_SPLINE_CURVE_WITH_KNOTS ( 'NONE', 3,
 ( #67112, #25674, #10829, #53130, #53581, #80638, #18917, #37851, #59005, #3613 ),
 .UNSPECIFIED., .F., .F.,
 ( 4, 2, 2, 2, 4 ),
 ( 0.0007817359430256388964, 0.0009771253907250069485, 0.001172514838424375001, 0.001367904286123743270, 0.001563293733823111322 ),
 .UNSPECIFIED. ) ;
#76445=CARTESIAN_POINT ( 'NONE',  ( 13.13461538461538680, -2.499999999999998668, 29.75000000000000355 ) ) ;
#76447=B_SPLINE_CURVE_WITH_KNOTS ( 'NONE', 3,
 ( #22896, #50360, #85058, #72410, #66557, #24674, #25119, #3506, #10278, #79180 ),
 .UNSPECIFIED., .F., .F.,
 ( 4, 2, 2, 2, 4 ),
 ( 0.000000000000000000, 0.0001954311564186863052, 0.0003908623128373726104, 0.0005862934692560589156, 0.0007817246256747452209 ),
 .UNSPECIFIED. ) ;
#76448=EDGE_CURVE ( 'NONE', #47862, #27365, #31255, .T. ) ;
#76449=EDGE_CURVE ( 'NONE', #75373, #38598, #65707, .T. ) ;
#76450=CARTESIAN_POINT ( 'NONE',  ( 14.30769230769231015, -3.322132147404559976, 32.92929555188717927 ) ) ;
#76451=VERTEX_POINT ( 'NONE', #4231 ) ;
#76452=AXIS2_PLACEMENT_3D ( 'NONE', #46031, #58647, #72610 ) ;
#76455=VERTEX_POINT ( 'NONE', #86677 ) ;
#76456=FACE_BOUND ( 'NONE', #46129, .T. ) ;
#76457=EDGE_CURVE ( 'NONE', #42886, #36014, #28082, .T. ) ;
#76458=CARTESIAN_POINT ( 'NONE',  ( 11.40777007179398161, -4.809359713505814149, 33.96456829005828837 ) ) ;
#76461=CARTESIAN_POINT ( 'NONE',  ( 18.25005441991345378, -2.920487667080175154, 32.31805714834170828 ) ) ;
#76462=CARTESIAN_POINT ( 'NONE',  ( 17.99999999999987566, -4.481592998941358097, 33.73612834414048933 ) ) ;
#76463=CARTESIAN_POINT ( 'NONE',  ( -3.230769230769229949, -3.322132147404559976, 32.92929555188717927 ) ) ;
#76464=CARTESIAN_POINT ( 'NONE',  ( 18.24994551834814160, -2.824170634883622633, 31.52227843825338738 ) ) ;
#76466=CARTESIAN_POINT ( 'NONE',  ( -2.557669051740898425, -4.075325502946086864, 33.72974371597207721 ) ) ;
#76467=CARTESIAN_POINT ( 'NONE',  ( -9.692307692307691624, -13.20930481340135110, 34.54067556320372745 ) ) ;
#76468=ORIENTED_EDGE ( 'NONE', *, *, #27888, .T. ) ;
#76469=CARTESIAN_POINT ( 'NONE',  ( 8.546304551714618114, -3.105860786376062332, 32.13614157043599562 ) ) ;
#76470=DIRECTION ( 'NONE',  ( -0.000000000000000000, -0.9848077530122086864, -0.1736481776669273891 ) ) ;
#76471=VERTEX_POINT ( 'NONE', #85323 ) ;
#76472=CARTESIAN_POINT ( 'NONE',  ( -6.923076923076922462, -3.886160181151819604, 36.00935417666054406 ) ) ;
#76473=FACE_OUTER_BOUND ( 'NONE', #51681, .T. ) ;
#76474=FACE_BOUND ( 'NONE', #74466, .T. ) ;
#76475=CARTESIAN_POINT ( 'NONE',  ( -2.372962753653081958, -6.879047030191174805, 34.71129190930000163 ) ) ;
#76476=CARTESIAN_POINT ( 'NONE',  ( -17.07692307692307665, -12.37446782046654192, 30.86335684631486131 ) ) ;
#76477=CARTESIAN_POINT ( 'NONE',  ( 3.230769230769108269, -6.835583212225970762, 34.95778746994575670 ) ) ;
#76478=CARTESIAN_POINT ( 'NONE',  ( -15.45369544828537833, -9.086856451489515152, 34.49173150075333183 ) ) ;
#76479=CARTESIAN_POINT ( 'NONE',  ( -18.00000000000012079, -11.48612834414049644, 32.76840700105863391 ) ) ;
#76480=CYLINDRICAL_SURFACE ( 'NONE', #66450, 0.2499999999999979738 ) ;
#76481=CARTESIAN_POINT ( 'NONE',  ( -18.00000000000000000, -8.809628690132287332, 35.73758076001107042 ) ) ;
#76483=ORIENTED_EDGE ( 'NONE', *, *, #31901, .T. ) ;
#76485=ORIENTED_EDGE ( 'NONE', *, *, #70181, .F. ) ;
#76487=CARTESIAN_POINT ( 'NONE',  ( 14.30769230769218581, -12.70778746994576025, 30.41441678777401236 ) ) ;
#76488=CARTESIAN_POINT ( 'NONE',  ( 14.55774672760575861, -9.233818618650603938, 34.70587769442853698 ) ) ;
#76489=CARTESIAN_POINT ( 'NONE',  ( 8.703980837456683162, -2.255955759149247619, 30.00000000000013856 ) ) ;
#76490=CARTESIAN_POINT ( 'NONE',  ( -16.82686876528476105, -6.567000820036036579, 34.66262288849541306 ) ) ;
#76493=FACE_OUTER_BOUND ( 'NONE', #49492, .T. ) ;
#76494=CARTESIAN_POINT ( 'NONE',  ( 18.06606835100243558, -3.050289026998446840, 32.03036669348366416 ) ) ;
#76495=CARTESIAN_POINT ( 'NONE',  ( 6.223012844093396723, -4.026326845037961455, 33.68677907613344047 ) ) ;
#76496=CARTESIAN_POINT ( 'NONE',  ( 7.622668921589517588, -5.827078755546624578, 34.72654668319379567 ) ) ;
#76497=CARTESIAN_POINT ( 'NONE',  ( -1.134615384613964384, -7.500000000000154543, 35.00000000000007105 ) ) ;
#76498=CARTESIAN_POINT ( 'NONE',  ( -11.53846153846153655, -1.509761064869970415, 31.06009739812519044 ) ) ;
#76499=CARTESIAN_POINT ( 'NONE',  ( -5.999999999999998224, -11.35647404775217417, 33.31231777344666511 ) ) ;
#76501=DIRECTION ( 'NONE',  ( -0.000000000000000000, -0.8660254037844397068, -0.4999999999999978906 ) ) ;
#76502=ORIENTED_EDGE ( 'NONE', *, *, #2941, .T. ) ;
#76503=CARTESIAN_POINT ( 'NONE',  ( 12.33139049180676672, -4.299443229763728169, 33.91186481527756058 ) ) ;
#76504=DIRECTION ( 'NONE',  ( -0.000000000000000000, -0.3420201433256694346, -0.9396926207859080948 ) ) ;
#76506=CARTESIAN_POINT ( 'NONE',  ( -9.915234651214539952, -10.77366814457252175, 33.85459836347579454 ) ) ;
#76507=CARTESIAN_POINT ( 'NONE',  ( 16.82689985270161870, -11.56360843649121861, 33.07473185843129926 ) ) ;
#76508=ORIENTED_EDGE ( 'NONE', *, *, #10287, .T. ) ;
#76509=CARTESIAN_POINT ( 'NONE',  ( -6.988346923633242724, -3.083524468853724443, 32.58852847137143272 ) ) ;
#76511=ORIENTED_EDGE ( 'NONE', *, *, #658, .T. ) ;
#76512=CARTESIAN_POINT ( 'NONE',  ( 6.923076923076924238, -3.513871655860378418, 32.76840700105978499 ) ) ;
#76513=CARTESIAN_POINT ( 'NONE',  ( 16.94623247381276698, -2.494641256782728966, 31.33461815524612959 ) ) ;
#76514=B_SPLINE_CURVE_WITH_KNOTS ( 'NONE', 3,
 ( #53275, #5996, #46531, #87996, #13189, #46087, #5546, #46956, #21599, #26255 ),
 .UNSPECIFIED., .F., .F.,
 ( 4, 2, 2, 2, 4 ),
 ( 0.000000000000000000, 0.0001954339857564070949, 0.0003908679715128141898, 0.0005863019572692212576, 0.0007817359430256283796 ),
 .UNSPECIFIED. ) ;
#76516=CARTESIAN_POINT ( 'NONE',  ( 17.07692307692295586, -2.657715359629662544, 31.77849191805970364 ) ) ;
#76517=CARTESIAN_POINT ( 'NONE',  ( 10.68145194873469173, -10.67929555188718282, 33.92786785259544757 ) ) ;
#76519=ORIENTED_EDGE ( 'NONE', *, *, #78866, .T. ) ;
#76520=VECTOR ( 'NONE', #56955, 1000.000000000000000 ) ;
#76521=CARTESIAN_POINT ( 'NONE',  ( 16.85399685940693004, -11.24512374952581872, 33.06303171183252942 ) ) ;
#76522=CARTESIAN_POINT ( 'NONE',  ( -18.25000000000000355, -12.50000000000000000, 29.75000000000000355 ) ) ;
#76523=CARTESIAN_POINT ( 'NONE',  ( 9.692307692307695177, -6.343179335718451384, 34.87096338111211935 ) ) ;
#76524=VERTEX_POINT ( 'NONE', #67716 ) ;
#76527=CARTESIAN_POINT ( 'NONE',  ( 3.230769230769108269, -3.083524468854526912, 32.58852847137268327 ) ) ;
#76528=ORIENTED_EDGE ( 'NONE', *, *, #2404, .T. ) ;
#76529=DIRECTION ( 'NONE',  ( 0.000000000000000000, 0.1736481776669275834, 0.9848077530122086864 ) ) ;
#76530=CARTESIAN_POINT ( 'NONE',  ( -6.989159302437059296, -2.292212530054419606, 30.41441678777542634 ) ) ;
#76531=CARTESIAN_POINT ( 'NONE',  ( -16.15384615384615330, -3.937682226553329556, 33.60647404775216529 ) ) ;
#76532=EDGE_CURVE ( 'NONE', #57723, #58055, #39367, .T. ) ;
#76533=CARTESIAN_POINT ( 'NONE',  ( -6.857821783564084228, -11.67786785259547777, 32.92929555188713664 ) ) ;
#76534=CARTESIAN_POINT ( 'NONE',  ( -0.3962833220256230526, -5.941354392334606160, 34.76329471203374055 ) ) ;
#76535=CARTESIAN_POINT ( 'NONE',  ( 0.2387103639035820235, -7.369209533119137845, 34.99857337881830688 ) ) ;
#76536=CARTESIAN_POINT ( 'NONE',  ( 10.61538461538461675, -13.87047571288749737, 32.06866353760679544 ) ) ;
#76537=ORIENTED_EDGE ( 'NONE', *, *, #50247, .F. ) ;
#76538=EDGE_CURVE ( 'NONE', #49681, #43177, #27165, .T. ) ;
#76539=ORIENTED_EDGE ( 'NONE', *, *, #76055, .F. ) ;
#76540=CARTESIAN_POINT ( 'NONE',  ( 18.00000000000000000, -12.29105614889573062, 35.45975837776705220 ) ) ;
#76541=ORIENTED_EDGE ( 'NONE', *, *, #70964, .T. ) ;
#76543=VECTOR ( 'NONE', #10338, 1000.000000000000000 ) ;
#76544=VERTEX_POINT ( 'NONE', #47427 ) ;
#76545=B_SPLINE_CURVE_WITH_KNOTS ( 'NONE', 3,
 ( #7699, #20756, #14901, #54988, #36060, #28860, #34718, #21642, #69395, #15784 ),
 .UNSPECIFIED., .F., .F.,
 ( 4, 2, 2, 2, 4 ),
 ( 0.0007817359430256297891, 0.0009771253907249958896, 0.001172514838424361990, 0.001367904286123728091, 0.001563293733823094191 ),
 .UNSPECIFIED. ) ;
#76546=DIRECTION ( 'NONE',  ( -0.000000000000000000, -0.5000000000000009992, -0.8660254037844380415 ) ) ;
#76547=CARTESIAN_POINT ( 'NONE',  ( 5.207714884747862705, -3.530189275343204702, 32.79018710029569661 ) ) ;
#76548=ORIENTED_EDGE ( 'NONE', *, *, #33309, .F. ) ;
#76549=CARTESIAN_POINT ( 'NONE',  ( 8.769230769230645706, -12.70778746994576025, 30.41441678777401236 ) ) ;
#76551=ORIENTED_EDGE ( 'NONE', *, *, #15532, .T. ) ;
#76552=CARTESIAN_POINT ( 'NONE',  ( -6.700065571464073777, -11.24521262558773671, 33.06293181088029343 ) ) ;
#76553=ORIENTED_EDGE ( 'NONE', *, *, #79717, .F. ) ;
#76554=FACE_OUTER_BOUND ( 'NONE', #50181, .T. ) ;
#76555=EDGE_CURVE ( 'NONE', #57, #11273, #86159, .T. ) ;
#76556=EDGE_CURVE ( 'NONE', #30991, #6722, #49615, .T. ) ;
#76557=EDGE_LOOP ( 'NONE', ( #47210, #40819, #30645, #54471 ) ) ;
#76558=DIRECTION ( 'NONE',  ( -0.000000000000000000, 0.7660444431189791237, -0.6427876096865379196 ) ) ;
#76559=CARTESIAN_POINT ( 'NONE',  ( -9.019253993452226226, -12.07920672191015221, 32.31858351112116168 ) ) ;
#76560=FACE_BOUND ( 'NONE', #71307, .T. ) ;
#76561=B_SPLINE_CURVE_WITH_KNOTS ( 'NONE', 3,
 ( #41829, #69298, #68402, #8038, #33736, #35508, #76496, #47239, #74733, #13900 ),
 .UNSPECIFIED., .F., .F.,
 ( 4, 2, 2, 2, 4 ),
 ( 0.000000000000000000, 0.0001954311564186863323, 0.0003908623128373726646, 0.0005862934692560590241, 0.0007817246256747453293 ),
 .UNSPECIFIED. ) ;
#76562=CARTESIAN_POINT ( 'NONE',  ( 1.515141086378949398, -12.45806712695776319, 30.39783852428763922 ) ) ;
#76563=CARTESIAN_POINT ( 'NONE',  ( -20.74999999999999645, -10.50000000000000000, 29.75000000000000355 ) ) ;
#76564=CARTESIAN_POINT ( 'NONE',  ( -1.384615384615383471, -6.681629849574314051, 35.83090037661290239 ) ) ;
#76566=CARTESIAN_POINT ( 'NONE',  ( -17.30040800148741198, -8.539481045369598178, 34.89627647299170832 ) ) ;
#76567=CARTESIAN_POINT ( 'NONE',  ( -9.692307692307377209, -2.255955759149395501, 30.00000000000324363 ) ) ;
#76568=ORIENTED_EDGE ( 'NONE', *, *, #14841, .F. ) ;
#76569=CARTESIAN_POINT ( 'NONE',  ( 14.30769230769231015, -6.343179335718451384, 34.87096338111211935 ) ) ;
#76570=ORIENTED_EDGE ( 'NONE', *, *, #15717, .F. ) ;
#76571=ORIENTED_EDGE ( 'NONE', *, *, #15343, .F. ) ;
#76574=VECTOR ( 'NONE', #82365, 1000.000000000000227 ) ;
#76575=CARTESIAN_POINT ( 'NONE',  ( -9.469528023329626620, -12.47679350104403007, 31.42216943046555855 ) ) ;
#76576=LINE ( 'NONE', #28840, #12092 ) ;
#76577=DIRECTION ( 'NONE',  ( -0.000000000000000000, -0.7660444431189791237, -0.6427876096865379196 ) ) ;
#76578=CARTESIAN_POINT ( 'NONE',  ( 13.51540719244017374, -11.18335022499818621, 33.13157742990016885 ) ) ;
#76579=ORIENTED_EDGE ( 'NONE', *, *, #38331, .T. ) ;
#76580=CARTESIAN_POINT ( 'NONE',  ( 11.28843831424008570, -3.520140089381495585, 33.17453946501458262 ) ) ;
#76581=CARTESIAN_POINT ( 'NONE',  ( -14.30769230769242917, -10.33852847137269571, 34.16647553114546554 ) ) ;
#76582=B_SPLINE_CURVE_WITH_KNOTS ( 'NONE', 3,
 ( #11654, #66597, #31924, #3982, #4438, #37778, #67041, #18405, #5337, #72894 ),
 .UNSPECIFIED., .F., .F.,
 ( 4, 2, 2, 2, 4 ),
 ( 0.000000000000000000, 0.0001954339857564075557, 0.0003908679715128151114, 0.0005863019572692226671, 0.0007817359430256302227 ),
 .UNSPECIFIED. ) ;
#76583=DIRECTION ( 'NONE',  ( -0.000000000000000000, 0.9848077530122085754, -0.1736481776669273613 ) ) ;
#76584=CARTESIAN_POINT ( 'NONE',  ( -8.769230769230768274, -11.35647404775217417, 33.31231777344666511 ) ) ;
#76585=CARTESIAN_POINT ( 'NONE',  ( -11.60371252862278091, -2.506253911140460922, 30.00000000000013856 ) ) ;
#76586=EDGE_LOOP ( 'NONE', ( #784, #23752 ) ) ;
#76588=ORIENTED_EDGE ( 'NONE', *, *, #31408, .T. ) ;
#76590=ORIENTED_EDGE ( 'NONE', *, *, #7427, .T. ) ;
#76591=CARTESIAN_POINT ( 'NONE',  ( -9.626239341305252495, -12.37446782046654192, 30.86335684631486842 ) ) ;
#76593=FACE_OUTER_BOUND ( 'NONE', #63239, .T. ) ;
#76594=CARTESIAN_POINT ( 'NONE',  ( 15.36129466900287888, -4.299079248970732792, 33.91157788607253565 ) ) ;
#76595=CARTESIAN_POINT ( 'NONE',  ( 14.17754433796061875, -10.31621877034669588, 34.18098118002070152 ) ) ;
#76596=CARTESIAN_POINT ( 'NONE',  ( -39.05038313613820122, -2.499999999999999556, 29.75000000000000355 ) ) ;
#76597=CARTESIAN_POINT ( 'NONE',  ( -17.14219307747939425, -9.528491918058357157, 34.59228464037090589 ) ) ;
#76598=CARTESIAN_POINT ( 'NONE',  ( 8.703147358274890166, -6.386643153685125363, 34.62446782046654903 ) ) ;
#76599=ORIENTED_EDGE ( 'NONE', *, *, #33933, .T. ) ;
#76600=CARTESIAN_POINT ( 'NONE',  ( -5.076923076923075762, -1.790695186598648903, 34.54067556320373455 ) ) ;
#76601=DIRECTION ( 'NONE',  ( -0.000000000000000000, -0.000000000000000000, -1.000000000000000000 ) ) ;
#76603=DIRECTION ( 'NONE',  ( 1.000000000000000000, 0.000000000000000000, 0.000000000000000000 ) ) ;
#76604=CARTESIAN_POINT ( 'NONE',  ( -8.639183333980316348, -7.723484941389743952, 34.99544897038808955 ) ) ;
#76605=CARTESIAN_POINT ( 'NONE',  ( -17.29985003582992320, -11.98009711892700224, 32.48740034544074007 ) ) ;
#76606=CARTESIAN_POINT ( 'NONE',  ( 6.066067333350077639, -9.058645607665452459, 34.76329471203371924 ) ) ;
#76607=CARTESIAN_POINT ( 'NONE',  ( 18.00000000000000000, -4.102666532097928531, 36.13435417666054406 ) ) ;
#76608=CARTESIAN_POINT ( 'NONE',  ( 9.442330961365339448, -9.943427161483782584, 34.11278801902876978 ) ) ;
#76609=DIRECTION ( 'NONE',  ( -0.000000000000000000, -0.8660254037844397068, -0.4999999999999978906 ) ) ;
#76611=EDGE_LOOP ( 'NONE', ( #68494, #3424, #60236, #34355 ) ) ;
#76612=CARTESIAN_POINT ( 'NONE',  ( -1.384615384615505151, -11.48612834414049644, 32.76840700105863391 ) ) ;
#76613=CARTESIAN_POINT ( 'NONE',  ( 12.52679360105129902, -5.094484230520773593, 34.41647553114626845 ) ) ;
#76614=CARTESIAN_POINT ( 'NONE',  ( 8.769230769230645706, -11.06231777344772027, 33.60647404775119895 ) ) ;
#76615=DIRECTION ( 'NONE',  ( -0.000000000000000000, 0.1736481776669307198, -0.9848077530122080203 ) ) ;
#76616=VERTEX_POINT ( 'NONE', #5568 ) ;
#76617=CARTESIAN_POINT ( 'NONE',  ( -5.999999999999998224, -13.49023893513002648, 31.06009739812518688 ) ) ;
#76618=CARTESIAN_POINT ( 'NONE',  ( 11.47319153790521717, -4.320704448112771878, 33.92786785259540494 ) ) ;
#76619=AXIS2_PLACEMENT_3D ( 'NONE', #24336, #23451, #2289 ) ;
#76620=EDGE_CURVE ( 'NONE', #75262, #64231, #29213, .T. ) ;
#76621=CARTESIAN_POINT ( 'NONE',  ( 7.846153846153846700, -8.810774026931790459, 35.74407628777942847 ) ) ;
#76622=CARTESIAN_POINT ( 'NONE',  ( -4.153846153846273204, -10.90142922262034020, 33.41473453929536674 ) ) ;
#76623=B_SPLINE_CURVE_WITH_KNOTS ( 'NONE', 3,
 ( #65453, #78521, #4650, #32122, #44727, #10961, #58248, #17724, #10519, #73565 ),
 .UNSPECIFIED., .F., .F.,
 ( 4, 2, 2, 2, 4 ),
 ( 0.000000000000000000, 0.0001954311564186867389, 0.0003908623128373734778, 0.0005862934692560602167, 0.0007817246256747469556 ),
 .UNSPECIFIED. ) ;
#76624=ADVANCED_FACE ( 'NONE', ( #40694 ), #19520, .F. ) ;
#76625=ORIENTED_EDGE ( 'NONE', *, *, #12587, .F. ) ;
#76626=B_SPLINE_CURVE_WITH_KNOTS ( 'NONE', 3,
 ( #4842, #81838, #20128, #87722, #47594, #75078, #13364, #60661, #25994, #19244 ),
 .UNSPECIFIED., .F., .F.,
 ( 4, 2, 2, 2, 4 ),
 ( 0.0007817246256747484735, 0.0009771112852218920199, 0.001172497944769035783, 0.001367884604316179330, 0.001563271263863322876 ),
 .UNSPECIFIED. ) ;
#76627=CARTESIAN_POINT ( 'NONE',  ( 6.130791807824788719, -5.582136614379148654, 34.36778462344220486 ) ) ;
#76628=CARTESIAN_POINT ( 'NONE',  ( -8.703975629717930929, -5.941354392334607049, 34.76329471203374055 ) ) ;
#76629=CARTESIAN_POINT ( 'NONE',  ( -14.37344573600563891, -7.249945578846652694, 34.99404164642496795 ) ) ;
#76630=VERTEX_POINT ( 'NONE', #11891 ) ;
#76631=CARTESIAN_POINT ( 'NONE',  ( 1.384615384615265343, -2.892918686052166066, 31.69288490824153470 ) ) ;
#76632=EDGE_CURVE ( 'NONE', #85159, #32456, #57105, .T. ) ;
#76633=VERTEX_POINT ( 'NONE', #54182 ) ;
#76634=CARTESIAN_POINT ( 'NONE',  ( -16.28399336328437386, -6.001485441113818986, 34.52039167877662607 ) ) ;
#76635=CARTESIAN_POINT ( 'NONE',  ( 0.4615384615384611200, -9.905515769479276145, 34.41647553114623292 ) ) ;
#76638=DIRECTION ( 'NONE',  ( 0.000000000000000000, 0.1736481776669275834, 0.9848077530122086864 ) ) ;
#76639=CARTESIAN_POINT ( 'NONE',  ( -14.43838291080261627, -2.295517848115769421, 30.44137282052137294 ) ) ;
#76640=CARTESIAN_POINT ( 'NONE',  ( 0.3308469948709044095, -4.118384482072084296, 33.43331474514187107 ) ) ;
#76641=AXIS2_PLACEMENT_3D ( 'NONE', #64189, #57000, #44812 ) ;
#76643=CARTESIAN_POINT ( 'NONE',  ( -11.53846153846166089, -5.941354392335915335, 34.76329471203413846 ) ) ;
#76644=LINE ( 'NONE', #2733, #38294 ) ;
#76645=VERTEX_POINT ( 'NONE', #6892 ) ;
#76646=ORIENTED_EDGE ( 'NONE', *, *, #7069, .F. ) ;
#76647=ADVANCED_FACE ( 'NONE', ( #61831 ), #32589, .F. ) ;
#76648=FACE_BOUND ( 'NONE', #25394, .T. ) ;
#76649=ORIENTED_EDGE ( 'NONE', *, *, #39114, .F. ) ;
#76650=CARTESIAN_POINT ( 'NONE',  ( 15.10007776410167502, -12.38065189839062263, 30.83690757178629482 ) ) ;
#76652=CARTESIAN_POINT ( 'NONE',  ( 6.000000000000001776, -5.471508081941601098, 34.59228464037088457 ) ) ;
#76653=CARTESIAN_POINT ( 'NONE',  ( 5.299702618191484582, -4.387253974876676565, 33.66317474335728832 ) ) ;
#76654=ORIENTED_EDGE ( 'NONE', *, *, #54085, .T. ) ;
#76655=ORIENTED_EDGE ( 'NONE', *, *, #64670, .F. ) ;
#76656=EDGE_LOOP ( 'NONE', ( #62435, #89090 ) ) ;
#76657=B_SPLINE_CURVE_WITH_KNOTS ( 'NONE', 3,
 ( #1022, #69920, #29395, #22614, #1469, #49209, #9120, #50082, #14536, #35704 ),
 .UNSPECIFIED., .F., .F.,
 ( 4, 2, 2, 2, 4 ),
 ( 0.0007817359430256221996, 0.0009771253907249863487, 0.001172514838424350498, 0.001367904286123714647, 0.001563293733823078796 ),
 .UNSPECIFIED. ) ;
#76658=DIRECTION ( 'NONE',  ( -0.000000000000000000, -0.7660444431189791237, -0.6427876096865379196 ) ) ;
#76659=ORIENTED_EDGE ( 'NONE', *, *, #68050, .F. ) ;
#76660=EDGE_CURVE ( 'NONE', #44876, #58562, #37801, .T. ) ;
#76661=CARTESIAN_POINT ( 'NONE',  ( 3.230769230769231726, -2.721908614388771852, 31.22303859784724978 ) ) ;
#76663=CARTESIAN_POINT ( 'NONE',  ( -16.82692307692307310, -2.499999999999999112, 29.81604066197449754 ) ) ;
#76664=CARTESIAN_POINT ( 'NONE',  ( -17.20707104665477161, -3.069018819979305146, 32.56621877034667278 ) ) ;
#76665=ORIENTED_EDGE ( 'NONE', *, *, #62567, .F. ) ;
#76668=ADVANCED_FACE ( 'NONE', ( #55963 ), #62712, .F. ) ;
#76669=CARTESIAN_POINT ( 'NONE',  ( 0.5923302693632469529, -11.71459661697925903, 32.44059661609676937 ) ) ;
#76671=DIRECTION ( 'NONE',  ( 0.000000000000000000, -6.938893903907222067E-15, 1.000000000000000000 ) ) ;
#76672=DIRECTION ( 'NONE',  ( -0.000000000000000000, 0.7660444431189791237, -0.6427876096865379196 ) ) ;
#76674=ORIENTED_EDGE ( 'NONE', *, *, #970, .T. ) ;
#76675=AXIS2_PLACEMENT_3D ( 'NONE', #50481, #980, #49609 ) ;
#76676=VERTEX_POINT ( 'NONE', #42024 ) ;
#76677=CARTESIAN_POINT ( 'NONE',  ( 4.088576153289833925, -3.083524468853724443, 32.58852847137143272 ) ) ;
#76679=CARTESIAN_POINT ( 'NONE',  ( 10.83816415665302557, -6.760870238392817200, 34.69528174975672385 ) ) ;
#76680=CARTESIAN_POINT ( 'NONE',  ( 11.47237915910140238, -2.292212530054419606, 30.41441678777542634 ) ) ;
#76682=FACE_BOUND ( 'NONE', #6366, .T. ) ;
#76683=CARTESIAN_POINT ( 'NONE',  ( 8.069165197766695385, -11.24521262558773493, 33.06293181088029343 ) ) ;
#76684=ORIENTED_EDGE ( 'NONE', *, *, #88513, .F. ) ;
#76685=CARTESIAN_POINT ( 'NONE',  ( -7.596153846152425615, -7.500000000000154543, 35.00000000000007105 ) ) ;
#76687=CARTESIAN_POINT ( 'NONE',  ( -1.384615384615505151, -2.892918686052166066, 31.69288490824153470 ) ) ;
#76689=ORIENTED_EDGE ( 'NONE', *, *, #53029, .F. ) ;
#76690=CARTESIAN_POINT ( 'NONE',  ( 4.853438152358743984, -12.69144148231606017, 30.53333754910549303 ) ) ;
#76691=ORIENTED_EDGE ( 'NONE', *, *, #35459, .T. ) ;
#76692=FACE_BOUND ( 'NONE', #71974, .T. ) ;
#76693=CARTESIAN_POINT ( 'NONE',  ( 9.442330961365341224, -5.728515186090277211, 34.42611988154120439 ) ) ;
#76694=CARTESIAN_POINT ( 'NONE',  ( 4.376625822824218304, -2.612705202774697533, 31.66806509827799943 ) ) ;
#76695=CARTESIAN_POINT ( 'NONE',  ( -11.28851602011339672, -11.86320923018887541, 32.19269448109604781 ) ) ;
#76697=CARTESIAN_POINT ( 'NONE',  ( -14.53117725141625627, -12.44517049084099725, 30.48991314939691932 ) ) ;
#76698=CARTESIAN_POINT ( 'NONE',  ( -14.30769230769230660, -4.098570777380720287, 33.41473453929634729 ) ) ;
#76699=CARTESIAN_POINT ( 'NONE',  ( 10.61538461538461675, -6.343179335718451384, 34.87096338111211935 ) ) ;
#76700=CARTESIAN_POINT ( 'NONE',  ( 6.066068351002440906, -3.513871655860379306, 32.76840700105978499 ) ) ;
#76701=ORIENTED_EDGE ( 'NONE', *, *, #30257, .F. ) ;
#76702=CARTESIAN_POINT ( 'NONE',  ( 12.71153846153846168, -2.249999999999998668, 29.75000000000000355 ) ) ;
#76703=VECTOR ( 'NONE', #35908, 1000.000000000000114 ) ;
#76704=EDGE_LOOP ( 'NONE', ( #80694, #72071 ) ) ;
#76705=CARTESIAN_POINT ( 'NONE',  ( 15.90384615384615330, -7.433932668274255917, 35.00000000000000711 ) ) ;
#76706=AXIS2_PLACEMENT_3D ( 'NONE', #57465, #30879, #58347 ) ;
#76707=ORIENTED_EDGE ( 'NONE', *, *, #64191, .T. ) ;
#76708=DIRECTION ( 'NONE',  ( 0.000000000000000000, 0.9396926207859126468, 0.3420201433256571111 ) ) ;
#76709=DIRECTION ( 'NONE',  ( 0.000000000000000000, 0.8660254037844377084, 0.5000000000000015543 ) ) ;
#76711=CARTESIAN_POINT ( 'NONE',  ( 0.4615384615383382183, -3.643525952248795718, 33.31231777344771672 ) ) ;
#76712=EDGE_CURVE ( 'NONE', #83905, #83971, #63472, .T. ) ;
#76713=CARTESIAN_POINT ( 'NONE',  ( 12.46153846153846168, -4.098570777380720287, 33.41473453929634729 ) ) ;
#76714=CARTESIAN_POINT ( 'NONE',  ( -7.911424292114620727, -10.90142922261923886, 33.41473453929638993 ) ) ;
#76716=CARTESIAN_POINT ( 'NONE',  ( -20.99999999999999645, -2.249999999999999556, 29.75000000000000355 ) ) ;
#76718=ORIENTED_EDGE ( 'NONE', *, *, #77554, .T. ) ;
#76720=ORIENTED_EDGE ( 'NONE', *, *, #20692, .F. ) ;
#76721=ORIENTED_EDGE ( 'NONE', *, *, #36483, .F. ) ;
#76722=CARTESIAN_POINT ( 'NONE',  ( -4.153846153846152411, -4.786620604624113540, 33.94971097300155094 ) ) ;
#76723=ORIENTED_EDGE ( 'NONE', *, *, #33807, .T. ) ;
#76724=CARTESIAN_POINT ( 'NONE',  ( -5.869474561766354626, -12.70449254468099198, 30.44128974285582956 ) ) ;
#76725=CARTESIAN_POINT ( 'NONE',  ( -2.057637996053991447, -6.567000820036038355, 34.66262288849541306 ) ) ;
#76726=EDGE_CURVE ( 'NONE', #4768, #13156, #4463, .T. ) ;
#76727=FACE_OUTER_BOUND ( 'NONE', #17951, .T. ) ;
#76728=CARTESIAN_POINT ( 'NONE',  ( -5.076923076923075762, -8.564572088678739092, 35.78748833219616898 ) ) ;
#76729=CARTESIAN_POINT ( 'NONE',  ( 8.545745825506822158, -11.41268669641499756, 32.86336882939238535 ) ) ;
#76731=CARTESIAN_POINT ( 'NONE',  ( -4.219116599806928214, -3.835265460703609186, 33.15142922261924241 ) ) ;
#76732=CARTESIAN_POINT ( 'NONE',  ( 6.673053698855465399, -10.18141759479407327, 34.26406193332782379 ) ) ;
#76733=FACE_OUTER_BOUND ( 'NONE', #26462, .T. ) ;
#76735=CARTESIAN_POINT ( 'NONE',  ( 5.869309396889694774, -11.37499894934982514, 33.29245874905763003 ) ) ;
#76736=CARTESIAN_POINT ( 'NONE',  ( 7.596130621932389637, -2.341070481393819236, 30.72580821765574299 ) ) ;
#76737=B_SPLINE_CURVE_WITH_KNOTS ( 'NONE', 3,
 ( #81051, #31515, #58980, #28740, #62938, #36379, #37243, #8021, #84576, #8908 ),
 .UNSPECIFIED., .F., .F.,
 ( 4, 2, 2, 2, 4 ),
 ( 0.0007817359430256392216, 0.0009771253907250073822, 0.001172514838424375651, 0.001367904286123743920, 0.001563293733823112189 ),
 .UNSPECIFIED. ) ;
#76739=VECTOR ( 'NONE', #83211, 1000.000000000000000 ) ;
#76740=EDGE_CURVE ( 'NONE', #83846, #13509, #26008, .T. ) ;
#76741=EDGE_LOOP ( 'NONE', ( #14609, #43945, #68563, #87302 ) ) ;
#76743=CARTESIAN_POINT ( 'NONE',  ( 12.59206389977210350, -2.647132371071621471, 31.75357179365171589 ) ) ;
#76745=CARTESIAN_POINT ( 'NONE',  ( 11.66925334628632882, -9.804649428959608670, 34.18742332936588468 ) ) ;
#76746=DIRECTION ( 'NONE',  ( -0.000000000000000000, 0.3420201433256694901, -0.9396926207859082059 ) ) ;
#76747=VERTEX_POINT ( 'NONE', #75792 ) ;
#76748=EDGE_CURVE ( 'NONE', #33072, #85360, #78635, .T. ) ;
#76749=CYLINDRICAL_SURFACE ( 'NONE', #11879, 0.2499999999999997502 ) ;
#76750=CARTESIAN_POINT ( 'NONE',  ( -12.68436515401747045, -7.369208160676171460, 34.74850200257122879 ) ) ;
#76751=CARTESIAN_POINT ( 'NONE',  ( -12.33101275977489841, -10.88167719472716399, 33.43325721877153711 ) ) ;
#76752=ORIENTED_EDGE ( 'NONE', *, *, #15670, .T. ) ;
#76753=B_SPLINE_CURVE_WITH_KNOTS ( 'NONE', 3,
 ( #42309, #8072, #34654, #62988, #62122, #425, #1301, #28790, #89010, #46669 ),
 .UNSPECIFIED., .F., .F.,
 ( 4, 2, 2, 2, 4 ),
 ( 0.0007817246256747504250, 0.0009771112852218954894, 0.001172497944769040554, 0.001367884604316185401, 0.001563271263863330466 ),
 .UNSPECIFIED. ) ;
#76754=EDGE_CURVE ( 'NONE', #64026, #5201, #53921, .T. ) ;
#76755=CARTESIAN_POINT ( 'NONE',  ( 0.4615384615383396616, -6.026961402154118908, 34.52809138561165270 ) ) ;
#76756=ORIENTED_EDGE ( 'NONE', *, *, #37875, .F. ) ;
#76757=B_SPLINE_CURVE_WITH_KNOTS ( 'NONE', 3,
 ( #27084, #76150, #53670, #41488, #75708, #34730, #13134, #69406, #61742, #46904 ),
 .UNSPECIFIED., .F., .F.,
 ( 4, 2, 2, 2, 4 ),
 ( 0.0007817246256747448956, 0.0009771112852218876831, 0.001172497944769030579, 0.001367884604316173475, 0.001563271263863316371 ),
 .UNSPECIFIED. ) ;
#76758=CARTESIAN_POINT ( 'NONE',  ( 13.31853300525524908, -12.34228464037088280, 31.77849191805838558 ) ) ;
#76760=CARTESIAN_POINT ( 'NONE',  ( 15.48082365068267841, -3.435999193479609914, 33.07426656108010832 ) ) ;
#76761=CARTESIAN_POINT ( 'NONE',  ( -6.223484943723947893, -2.599994579823202923, 30.74605699353653776 ) ) ;
#76763=CARTESIAN_POINT ( 'NONE',  ( 2.980792486720640344, -8.347322224742351082, 34.93158281831414769 ) ) ;
#76764=FACE_OUTER_BOUND ( 'NONE', #77015, .T. ) ;
#76765=ORIENTED_EDGE ( 'NONE', *, *, #36781, .T. ) ;
#76766=VERTEX_POINT ( 'NONE', #67060 ) ;
#76767=ORIENTED_EDGE ( 'NONE', *, *, #77635, .T. ) ;
#76768=VERTEX_POINT ( 'NONE', #11674 ) ;
#76770=CARTESIAN_POINT ( 'NONE',  ( -17.30040802064702987, -10.81261337010820256, 33.49550067578627477 ) ) ;
#76771=LINE ( 'NONE', #15072, #33022 ) ;
#76773=EDGE_CURVE ( 'NONE', #24104, #30718, #66153, .T. ) ;
#76774=CARTESIAN_POINT ( 'NONE',  ( 11.53846153846153832, -12.10708131394839349, 31.69288490824020244 ) ) ;
#76775=CARTESIAN_POINT ( 'NONE',  ( -7.780898706641009355, -4.320704448112861584, 33.92786785259548310 ) ) ;
#76776=EDGE_CURVE ( 'NONE', #88899, #29433, #52642, .T. ) ;
#76777=CARTESIAN_POINT ( 'NONE',  ( 14.37294787896833270, -10.21337939537593620, 33.94971097300152252 ) ) ;
#76778=ORIENTED_EDGE ( 'NONE', *, *, #56930, .F. ) ;
#76779=EDGE_LOOP ( 'NONE', ( #9824, #78971 ) ) ;
#76780=B_SPLINE_CURVE_WITH_KNOTS ( 'NONE', 3,
 ( #32473, #45542, #86098, #80230, #11317, #32037, #59946, #59503, #52739, #72121 ),
 .UNSPECIFIED., .F., .F.,
 ( 4, 2, 2, 2, 4 ),
 ( 0.0007817359430256324996, 0.0009771253907249993591, 0.001172514838424366110, 0.001367904286123732861, 0.001563293733823099829 ),
 .UNSPECIFIED. ) ;
#76781=ORIENTED_EDGE ( 'NONE', *, *, #52088, .T. ) ;
#76782=CARTESIAN_POINT ( 'NONE',  ( 12.68454981315131214, -8.239487800360276282, 34.69522927552633718 ) ) ;
#76784=CARTESIAN_POINT ( 'NONE',  ( -11.40767109749458541, -3.957578996910242619, 33.62503395064540257 ) ) ;
#76786=CARTESIAN_POINT ( 'NONE',  ( -2.176900499867519212, -8.999086150933472084, 34.52020707165672064 ) ) ;
#76787=B_SPLINE_CURVE_WITH_KNOTS ( 'NONE', 3,
 ( #1484, #2349, #37023, #56427, #69935, #76243, #15448, #43355, #7799, #42922 ),
 .UNSPECIFIED., .F., .F.,
 ( 4, 2, 2, 2, 4 ),
 ( 0.000000000000000000, 0.0001954311564186870913, 0.0003908623128373741825, 0.0005862934692560613009, 0.0007817246256747483650 ),
 .UNSPECIFIED. ) ;
#76788=CARTESIAN_POINT ( 'NONE',  ( -10.86536134632696715, -11.79746400365624659, 32.30657167506340954 ) ) ;
#76789=ORIENTED_EDGE ( 'NONE', *, *, #78069, .F. ) ;
#76790=AXIS2_PLACEMENT_3D ( 'NONE', #8621, #77507, #23006 ) ;
#76792=ORIENTED_EDGE ( 'NONE', *, *, #88944, .F. ) ;
#76793=FACE_OUTER_BOUND ( 'NONE', #47036, .T. ) ;
#76794=VECTOR ( 'NONE', #74422, 1000.000000000000000 ) ;
#76795=EDGE_LOOP ( 'NONE', ( #46434, #45634 ) ) ;
#76796=FACE_BOUND ( 'NONE', #44937, .T. ) ;
#76797=DIRECTION ( 'NONE',  ( 0.000000000000000000, 0.9848077530122072432, 0.1736481776669354937 ) ) ;
#76798=AXIS2_PLACEMENT_3D ( 'NONE', #3100, #37780, #3547 ) ;
#76799=CARTESIAN_POINT ( 'NONE',  ( -4.377331078410483300, -10.23692288466677880, 34.23039457007281072 ) ) ;
#76802=CARTESIAN_POINT ( 'NONE',  ( 15.29693583736087348, -7.250054591869670162, 34.99404684341514127 ) ) ;
#76803=CARTESIAN_POINT ( 'NONE',  ( 3.230769230769231726, -3.050289026998446396, 32.03036669348365706 ) ) ;
#76804=CARTESIAN_POINT ( 'NONE',  ( 10.48523740594639797, -2.882441371585227508, 31.66841991370172238 ) ) ;
#76805=CARTESIAN_POINT ( 'NONE',  ( -15.48079246806219267, -6.695914987888146541, 34.68535235679833306 ) ) ;
#76806=CARTESIAN_POINT ( 'NONE',  ( -13.38461538461550582, -11.94971097300221174, 32.03036669348237098 ) ) ;
#76807=VERTEX_POINT ( 'NONE', #80584 ) ;
#76808=CARTESIAN_POINT ( 'NONE',  ( -11.31544869436814338, -12.38742843783360748, 31.66772728687926985 ) ) ;
#76809=CARTESIAN_POINT ( 'NONE',  ( -7.912236225513981758, -11.91647553114624181, 32.58852847137148245 ) ) ;
#76810=CARTESIAN_POINT ( 'NONE',  ( 0.3313912521002448930, -11.93770438780619259, 32.05411857736982029 ) ) ;
#76811=CARTESIAN_POINT ( 'NONE',  ( 15.93036122928181975, -10.97335522853832934, 33.68706563782419749 ) ) ;
#76812=CARTESIAN_POINT ( 'NONE',  ( -15.23076923076922995, -11.69971097300155272, 32.46337939537588113 ) ) ;
#76813=EDGE_CURVE ( 'NONE', #60361, #83509, #22645, .T. ) ;
#76814=FACE_BOUND ( 'NONE', #47792, .T. ) ;
#76815=CARTESIAN_POINT ( 'NONE',  ( -6.923076923077045919, -12.70778746994576025, 30.41441678777401236 ) ) ;
#76818=CARTESIAN_POINT ( 'NONE',  ( 3.903822929624695792, -5.765609946408404518, 34.70566812827425451 ) ) ;
#76819=CARTESIAN_POINT ( 'NONE',  ( -18.22292695890684655, -2.889293201056496674, 32.26117774369185298 ) ) ;
#76820=CARTESIAN_POINT ( 'NONE',  ( -10.74553258511630993, -6.809168938359901446, 34.95455904226513866 ) ) ;
#76822=ORIENTED_EDGE ( 'NONE', *, *, #7897, .F. ) ;
#76823=ADVANCED_FACE ( 'NONE', ( #32383 ), #59848, .F. ) ;
#76824=CARTESIAN_POINT ( 'NONE',  ( -8.834987571745077872, -7.249945686854186278, 34.74374336980224598 ) ) ;
#76826=ADVANCED_FACE ( 'NONE', ( #50529 ), #46337, .F. ) ;
#76827=CARTESIAN_POINT ( 'NONE',  ( -13.38461538461538325, -3.322132147404559976, 32.92929555188717927 ) ) ;
#76828=ORIENTED_EDGE ( 'NONE', *, *, #65838, .T. ) ;
#76829=B_SPLINE_CURVE_WITH_KNOTS ( 'NONE', 3,
 ( #52084, #25951, #53415, #4350, #66500, #87234, #80917, #46668, #74144, #88130 ),
 .UNSPECIFIED., .F., .F.,
 ( 4, 2, 2, 2, 4 ),
 ( 0.0007817246256747452209, 0.0009771112852218887673, 0.001172497944769032531, 0.001367884604316176294, 0.001563271263863319840 ),
 .UNSPECIFIED. ) ;
#76830=FACE_OUTER_BOUND ( 'NONE', #50413, .T. ) ;
#76831=CARTESIAN_POINT ( 'NONE',  ( -8.096130577096200653, -9.943427161483782584, 34.11278801902876978 ) ) ;
#76832=ORIENTED_EDGE ( 'NONE', *, *, #44181, .T. ) ;
#76833=CARTESIAN_POINT ( 'NONE',  ( 5.776515075435669111, -10.97335522853832579, 33.68706563782419749 ) ) ;
#76835=CARTESIAN_POINT ( 'NONE',  ( 17.32686859527121470, -8.433404298154332679, 34.66254593164985920 ) ) ;
#76836=CARTESIAN_POINT ( 'NONE',  ( 3.903869422903799347, -9.148715823498378086, 34.47080413974185120 ) ) ;
#76837=CARTESIAN_POINT ( 'NONE',  ( 6.923076923076802558, -9.442884908241554243, 34.35708131394783038 ) ) ;
#76838=EDGE_CURVE ( 'NONE', #65911, #80616, #71243, .T. ) ;
#76839=CARTESIAN_POINT ( 'NONE',  ( -3.165576242474575253, -2.255955759149235629, 29.99999999999988631 ) ) ;
#76841=CARTESIAN_POINT ( 'NONE',  ( -14.05774689831426372, -4.932303261841489928, 34.32971442181322885 ) ) ;
#76843=B_SPLINE_CURVE_WITH_KNOTS ( 'NONE', 3,
 ( #88380, #28423, #82934, #68518, #34737, #62205, #6816, #61750, #48243, #75715 ),
 .UNSPECIFIED., .F., .F.,
 ( 4, 2, 2, 2, 4 ),
 ( 0.0007817359430256327164, 0.0009771253907249995759, 0.001172514838424366327, 0.001367904286123733078, 0.001563293733823099829 ),
 .UNSPECIFIED. ) ;
#76845=CARTESIAN_POINT ( 'NONE',  ( -5.076923076923075762, -4.098570777380720287, 33.41473453929634729 ) ) ;
#76848=CARTESIAN_POINT ( 'NONE',  ( -10.61538461538473577, -5.941354392335915335, 34.76329471203413846 ) ) ;
#76849=ORIENTED_EDGE ( 'NONE', *, *, #18087, .T. ) ;
#76850=DIRECTION ( 'NONE',  ( 0.000000000000000000, 0.1736481776669275834, 0.9848077530122086864 ) ) ;
#76851=CARTESIAN_POINT ( 'NONE',  ( 12.39626846098214230, -8.656820664281498878, 34.87096338111211935 ) ) ;
#76852=CYLINDRICAL_SURFACE ( 'NONE', #15294, 0.2499999999999979738 ) ;
#76853=CARTESIAN_POINT ( 'NONE',  ( -5.207070286361298095, -6.001485441113818986, 34.52039167877662607 ) ) ;
#76855=CARTESIAN_POINT ( 'NONE',  ( -1.634638621908348632, -10.76384336483936011, 33.53834819971076087 ) ) ;
#76856=CARTESIAN_POINT ( 'NONE',  ( 15.90386942290380290, -9.148715823498378086, 34.47080413974185120 ) ) ;
#76857=CARTESIAN_POINT ( 'NONE',  ( 8.703147358274888390, -10.51840700105979387, 33.73612834413961536 ) ) ;
#76859=VECTOR ( 'NONE', #83544, 1000.000000000000114 ) ;
#76862=ORIENTED_EDGE ( 'NONE', *, *, #69158, .T. ) ;
#76864=CARTESIAN_POINT ( 'NONE',  ( 5.326868595271218254, -11.86320923018887541, 32.19269448109604781 ) ) ;
#76865=CARTESIAN_POINT ( 'NONE',  ( -6.673022611438608642, -4.235687564193446164, 33.53795663066793509 ) ) ;
#76867=FACE_OUTER_BOUND ( 'NONE', #14570, .T. ) ;
#76868=CARTESIAN_POINT ( 'NONE',  ( 12.71153846153846168, -7.500000000000001776, 35.04278698407183867 ) ) ;
#76869=ORIENTED_EDGE ( 'NONE', *, *, #84287, .F. ) ;
#76870=CARTESIAN_POINT ( 'NONE',  ( -17.07692307692307665, -4.102666532097928531, 36.13435417666054406 ) ) ;
#76871=ORIENTED_EDGE ( 'NONE', *, *, #37652, .T. ) ;
#76873=ORIENTED_EDGE ( 'NONE', *, *, #2586, .F. ) ;
#76874=CARTESIAN_POINT ( 'NONE',  ( 8.519207545009310323, -12.45566812827425451, 31.48439005359158926 ) ) ;
#76876=CARTESIAN_POINT ( 'NONE',  ( 4.284371855609715674, -6.001044277235011215, 34.52024696741798948 ) ) ;
#76877=CARTESIAN_POINT ( 'NONE',  ( -2.307692307692305711, -4.786620604624113540, 33.94971097300155094 ) ) ;
#76878=ADVANCED_FACE ( 'NONE', ( #67947 ), #48097, .F. ) ;
#76879=CARTESIAN_POINT ( 'NONE',  ( -2.307692307692305711, -9.780366693483667717, 34.19971097300155094 ) ) ;
#76881=ADVANCED_FACE ( 'NONE', ( #40914 ), #806, .F. ) ;
#76882=ORIENTED_EDGE ( 'NONE', *, *, #48604, .F. ) ;
#76883=EDGE_LOOP ( 'NONE', ( #85981, #51530, #63105, #17288 ) ) ;
#76885=ORIENTED_EDGE ( 'NONE', *, *, #59045, .F. ) ;
#76886=CARTESIAN_POINT ( 'NONE',  ( -2.057746898314262829, -3.520799739797214389, 33.17531984108286025 ) ) ;
#76888=EDGE_LOOP ( 'NONE', ( #42320, #83043, #68447, #41777 ) ) ;
#76889=ADVANCED_FACE ( 'NONE', ( #69269 ), #21067, .F. ) ;
#76890=CARTESIAN_POINT ( 'NONE',  ( 16.15384615384615330, -7.500000000000001776, 35.04278698407183867 ) ) ;
#76892=CARTESIAN_POINT ( 'NONE',  ( -0.2387587925603953110, -9.418065098278011860, 34.63729479722530158 ) ) ;
#76893=EDGE_LOOP ( 'NONE', ( #30022, #64233 ) ) ;
#76894=CARTESIAN_POINT ( 'NONE',  ( 15.10007776410167502, -10.54014554554150607, 33.71984207302941883 ) ) ;
#76895=EDGE_CURVE ( 'NONE', #77995, #30802, #52616, .T. ) ;
#76896=DIRECTION ( 'NONE',  ( -0.000000000000000000, 0.6427876096865404731, -0.7660444431189771253 ) ) ;
#76898=FACE_BOUND ( 'NONE', #8870, .T. ) ;
#76899=CYLINDRICAL_SURFACE ( 'NONE', #34113, 0.2499999999999998890 ) ;
#76900=DIRECTION ( 'NONE',  ( -0.000000000000000000, 0.3420201433256694901, -0.9396926207859082059 ) ) ;
#76901=CARTESIAN_POINT ( 'NONE',  ( 20.74999999999999645, -10.50000000000000000, 29.75000000000000355 ) ) ;
#76902=CARTESIAN_POINT ( 'NONE',  ( -6.988400935881231568, -7.749976730030849303, 34.74374725381503737 ) ) ;
#76903=CARTESIAN_POINT ( 'NONE',  ( -0.6850234052624116776, -12.24155766932282496, 31.33739205006857986 ) ) ;
#76904=CARTESIAN_POINT ( 'NONE',  ( 8.769230769230645706, -6.835583212225970762, 34.95778746994575670 ) ) ;
#76905=CARTESIAN_POINT ( 'NONE',  ( -4.153846153846152411, -10.67929555188718282, 33.92786785259544047 ) ) ;
#76906=VERTEX_POINT ( 'NONE', #14774 ) ;
#76907=CARTESIAN_POINT ( 'NONE',  ( 11.53846153846141753, -3.300289026999228881, 32.46337939537708905 ) ) ;
#76908=DIRECTION ( 'NONE',  ( -0.000000000000000000, 0.1736481776669307198, -0.9848077530122080203 ) ) ;
#76909=VERTEX_POINT ( 'NONE', #82351 ) ;
#76910=CARTESIAN_POINT ( 'NONE',  ( -14.24243716817946925, -9.528491918058460186, 34.59228464037086326 ) ) ;
#76911=CARTESIAN_POINT ( 'NONE',  ( -4.088590582570128973, -2.625532179533470512, 30.86335684631491105 ) ) ;
#76912=CARTESIAN_POINT ( 'NONE',  ( 8.769230769230768274, -11.91647553114624181, 32.58852847137148245 ) ) ;
#76914=CARTESIAN_POINT ( 'NONE',  ( -10.39237177129122003, -2.889357225399414197, 32.26129605718031002 ) ) ;
#76915=DIRECTION ( 'NONE',  ( -0.000000000000000000, -0.3420201433256694901, -0.9396926207859082059 ) ) ;
#76917=FACE_BOUND ( 'NONE', #73099, .T. ) ;
#76918=CARTESIAN_POINT ( 'NONE',  ( 13.38461538461538680, -2.292212530054420494, 30.41441678777542634 ) ) ;
#76920=CARTESIAN_POINT ( 'NONE',  ( -16.08777780284371417, -2.538708090699994813, 30.37095296980875503 ) ) ;
#76921=CARTESIAN_POINT ( 'NONE',  ( -17.93474442872397034, -11.48612834413965800, 32.76840700105972815 ) ) ;
#76922=CARTESIAN_POINT ( 'NONE',  ( 7.146088274689773812, -12.39991518177334129, 30.74647679643404530 ) ) ;
#76923=CARTESIAN_POINT ( 'NONE',  ( -17.75005448165186195, -5.057305518903949526, 34.11320923018887896 ) ) ;
#76925=ORIENTED_EDGE ( 'NONE', *, *, #5351, .T. ) ;
#76926=EDGE_CURVE ( 'NONE', #14877, #12525, #70984, .T. ) ;
#76928=AXIS2_PLACEMENT_3D ( 'NONE', #13529, #28828, #75240 ) ;
#76929=CARTESIAN_POINT ( 'NONE',  ( 16.02315555073584363, -9.084618155246140248, 34.75535874321725771 ) ) ;
#76930=CARTESIAN_POINT ( 'NONE',  ( -0.7115151924808159611, -2.779195860258148798, 31.39871582349836743 ) ) ;
#76931=DIRECTION ( 'NONE',  ( 0.000000000000000000, 0.3420201433256610524, 0.9396926207859113145 ) ) ;
#76932=DIRECTION ( 'NONE',  ( -0.000000000000000000, 0.9848077530122086864, -0.1736481776669273891 ) ) ;
#76933=DIRECTION ( 'NONE',  ( -0.000000000000000000, -0.000000000000000000, -1.000000000000000000 ) ) ;
#76935=CARTESIAN_POINT ( 'NONE',  ( 4.088089351331844590, -7.249945686854186278, 34.74374336980224598 ) ) ;
#76936=CARTESIAN_POINT ( 'NONE',  ( 17.99999999999987566, -3.300289026999228437, 32.46337939537709616 ) ) ;
#76937=EDGE_CURVE ( 'NONE', #15866, #31594, #66679, .T. ) ;
#76938=CARTESIAN_POINT ( 'NONE',  ( 15.45354877203763877, -11.89424750095246175, 32.13594075562310337 ) ) ;
#76939=CARTESIAN_POINT ( 'NONE',  ( -2.980714810855777053, -12.01375889529407637, 32.43194544308182969 ) ) ;
#76940=CARTESIAN_POINT ( 'NONE',  ( -3.296851610129365007, -3.937682226553329556, 33.60647404775217240 ) ) ;
#76941=CARTESIAN_POINT ( 'NONE',  ( 16.28463796167094557, -4.809403383903225304, 33.96459661697925014 ) ) ;
#76942=CARTESIAN_POINT ( 'NONE',  ( 1.384615384615386802, -6.386643153685126251, 34.62446782046654192 ) ) ;
#76943=EDGE_CURVE ( 'NONE', #28117, #63575, #53977, .T. ) ;
#76944=CARTESIAN_POINT ( 'NONE',  ( -0.4615384615384611200, -9.780366693483667717, 34.19971097300155094 ) ) ;
#76945=VERTEX_POINT ( 'NONE', #68821 ) ;
#76946=CARTESIAN_POINT ( 'NONE',  ( 12.23861150263161157, -4.026226216239094491, 33.68668979543634379 ) ) ;
#76947=DIRECTION ( 'NONE',  ( 0.000000000000000000, 0.3420201433256610524, 0.9396926207859113145 ) ) ;
#76950=LINE ( 'NONE', #49481, #48948 ) ;
#76952=CARTESIAN_POINT ( 'NONE',  ( 13.38461538461538680, -11.69971097300155272, 32.46337939537588113 ) ) ;
#76953=CARTESIAN_POINT ( 'NONE',  ( -5.869952564749547186, -7.723484941389743952, 34.99544897038808955 ) ) ;
#76955=DIRECTION ( 'NONE',  ( -0.000000000000000000, 0.5000000000000011102, -0.8660254037844380415 ) ) ;
#76956=CARTESIAN_POINT ( 'NONE',  ( -2.307692307692428724, -11.06231777344772027, 33.60647404775119895 ) ) ;
#76957=ADVANCED_FACE ( 'NONE', ( #12997 ), #88680, .F. ) ;
#76958=ORIENTED_EDGE ( 'NONE', *, *, #81061, .T. ) ;
#76959=CARTESIAN_POINT ( 'NONE',  ( -5.300408020647027207, -12.24155766932282496, 31.33739205006857986 ) ) ;
#76960=B_SPLINE_CURVE_WITH_KNOTS ( 'NONE', 3,
 ( #52932, #19167, #46636, #4770, #32239, #86759, #79978, #86308, #72321, #80435 ),
 .UNSPECIFIED., .F., .F.,
 ( 4, 2, 2, 2, 4 ),
 ( 0.0007817246256747457630, 0.0009771112852218887673, 0.001172497944769031663, 0.001367884604316174559, 0.001563271263863317672 ),
 .UNSPECIFIED. ) ;
#76962=CARTESIAN_POINT ( 'NONE',  ( 8.069580808015416551, -7.630147231320743018, 34.74852402298682819 ) ) ;
#76963=ORIENTED_EDGE ( 'NONE', *, *, #25774, .T. ) ;
#76964=CARTESIAN_POINT ( 'NONE',  ( -12.68446542044531000, -2.308479472611653094, 30.53278059502174457 ) ) ;
#76965=EDGE_CURVE ( 'NONE', #75827, #85310, #21523, .T. ) ;
#76966=ADVANCED_FACE ( 'NONE', ( #78230 ), #64263, .F. ) ;
#76967=CARTESIAN_POINT ( 'NONE',  ( 5.076923076923391065, -2.255955759149395501, 30.00000000000324363 ) ) ;
#76968=CARTESIAN_POINT ( 'NONE',  ( 12.71159288145191368, -12.01375889529407281, 32.43194544308182969 ) ) ;
#76969=ORIENTED_EDGE ( 'NONE', *, *, #51201, .T. ) ;
#76970=VERTEX_POINT ( 'NONE', #57074 ) ;
#76971=CARTESIAN_POINT ( 'NONE',  ( 15.48082354240754555, -10.66356715214248752, 33.62249196103329751 ) ) ;
#76972=EDGE_CURVE ( 'NONE', #11752, #48440, #87115, .T. ) ;
#76974=CARTESIAN_POINT ( 'NONE',  ( -1.318547033612944341, -2.538708090699994813, 30.37095296980875503 ) ) ;
#76975=CARTESIAN_POINT ( 'NONE',  ( 13.44987052412822237, -3.643525952247864463, 33.31231777344670064 ) ) ;
#76976=CARTESIAN_POINT ( 'NONE',  ( 16.15384615384615330, -13.53365097954675988, 30.81389545987213552 ) ) ;
#76977=DIRECTION ( 'NONE',  ( 1.000000000000000000, 0.000000000000000000, 0.000000000000000000 ) ) ;
#76978=AXIS2_PLACEMENT_3D ( 'NONE', #19320, #66621, #54422 ) ;
#76980=ORIENTED_EDGE ( 'NONE', *, *, #56798, .T. ) ;
#76981=CARTESIAN_POINT ( 'NONE',  ( 6.923076923076924238, -2.249999999999998668, 29.75000000000001776 ) ) ;
#76982=ORIENTED_EDGE ( 'NONE', *, *, #42274, .T. ) ;
#76983=EDGE_CURVE ( 'NONE', #46529, #62974, #78469, .T. ) ;
#76984=CARTESIAN_POINT ( 'NONE',  ( 7.846153846153723244, -2.657715359629662544, 31.77849191805970364 ) ) ;
#76986=B_SPLINE_CURVE_WITH_KNOTS ( 'NONE', 3,
 ( #78575, #2901, #79024, #44327, #70937, #37587, #72709, #9249, #78132, #43905 ),
 .UNSPECIFIED., .F., .F.,
 ( 4, 2, 2, 2, 4 ),
 ( 0.0007817359430256326080, 0.0009771253907250047801, 0.001172514838424369796, 0.001367904286123735030, 0.001563293733823100046 ),
 .UNSPECIFIED. ) ;
#76987=B_SPLINE_CURVE_WITH_KNOTS ( 'NONE', 3,
 ( #31841, #18768, #26410, #39935, #13332, #46235, #88137, #67393, #45783, #86803 ),
 .UNSPECIFIED., .F., .F.,
 ( 4, 2, 2, 2, 4 ),
 ( 0.0007817246256747447872, 0.0009771112852218876831, 0.001172497944769030579, 0.001367884604316173475, 0.001563271263863316371 ),
 .UNSPECIFIED. ) ;
#76988=CARTESIAN_POINT ( 'NONE',  ( 7.596130621932386973, -12.07920672191015221, 32.31858351112116168 ) ) ;
#76990=VECTOR ( 'NONE', #17733, 1000.000000000000227 ) ;
#76991=VERTEX_POINT ( 'NONE', #84569 ) ;
#76992=B_SPLINE_CURVE_WITH_KNOTS ( 'NONE', 3,
 ( #48335, #8254, #42041, #68613, #77147, #28521, #83474, #61397, #34823, #27184 ),
 .UNSPECIFIED., .F., .F.,
 ( 4, 2, 2, 2, 4 ),
 ( 0.000000000000000000, 0.0001954339857564092362, 0.0003908679715128184724, 0.0005863019572692276544, 0.0007817359430256369448 ),
 .UNSPECIFIED. ) ;
#76993=CARTESIAN_POINT ( 'NONE',  ( -12.23852710992561299, -5.667800583137506010, 34.40243808032445827 ) ) ;
#76994=ORIENTED_EDGE ( 'NONE', *, *, #71060, .T. ) ;
#76995=CARTESIAN_POINT ( 'NONE',  ( -8.638438961405983108, -8.147973898785416225, 34.70805048591653730 ) ) ;
#76996=ORIENTED_EDGE ( 'NONE', *, *, #54235, .F. ) ;
#76997=EDGE_CURVE ( 'NONE', #4299, #33013, #22843, .T. ) ;
#76998=CARTESIAN_POINT ( 'NONE',  ( -12.52680846209478283, -3.643525952247789412, 33.31231777344662959 ) ) ;
#76999=B_SPLINE_CURVE_WITH_KNOTS ( 'NONE', 3,
 ( #58104, #70746, #22113, #29322, #85586, #63532, #50020, #18467, #10816, #51773 ),
 .UNSPECIFIED., .F., .F.,
 ( 4, 2, 2, 2, 4 ),
 ( 0.000000000000000000, 0.0001954311564186865221, 0.0003908623128373730441, 0.0005862934692560595662, 0.0007817246256747460882 ),
 .UNSPECIFIED. ) ;
#77000=CARTESIAN_POINT ( 'NONE',  ( 14.30769230769231015, -5.471508081941601098, 34.59228464037088457 ) ) ;
#77001=VERTEX_POINT ( 'NONE', #35934 ) ;
#77002=FACE_OUTER_BOUND ( 'NONE', #50773, .T. ) ;
#77004=CARTESIAN_POINT ( 'NONE',  ( -8.834500769787091201, -12.16647553114622049, 32.15551576947930812 ) ) ;
#77005=FACE_BOUND ( 'NONE', #68916, .T. ) ;
#77006=CARTESIAN_POINT ( 'NONE',  ( 1.450683735617825487, -12.37446782046654192, 30.86335684631486842 ) ) ;
#77007=CARTESIAN_POINT ( 'NONE',  ( -39.05038313613820122, -2.499999999999999556, 29.75000000000000355 ) ) ;
#77008=CARTESIAN_POINT ( 'NONE',  ( -15.90390074446811042, -4.932303261841488151, 34.32971442181322885 ) ) ;
#77009=CARTESIAN_POINT ( 'NONE',  ( -16.94639763868943660, -12.50538340440932394, 31.33453814440721885 ) ) ;
#77011=DIRECTION ( 'NONE',  ( -0.000000000000000000, 0.5000000000000011102, -0.8660254037844381525 ) ) ;
#77012=ORIENTED_EDGE ( 'NONE', *, *, #27109, .T. ) ;
#77013=CARTESIAN_POINT ( 'NONE',  ( 10.39245839786846837, -9.886141570436013382, 34.14413921362392301 ) ) ;
#77015=EDGE_LOOP ( 'NONE', ( #23015, #82209, #3623, #40327 ) ) ;
#77016=AXIS2_PLACEMENT_3D ( 'NONE', #54012, #74749, #87383 ) ;
#77017=CARTESIAN_POINT ( 'NONE',  ( -1.254089946381740095, -5.070358843744210198, 34.40418822224088302 ) ) ;
#77018=CARTESIAN_POINT ( 'NONE',  ( 7.846153846153725020, -10.21337939537710326, 33.94971097300076224 ) ) ;
#77019=EDGE_CURVE ( 'NONE', #27342, #15876, #16099, .T. ) ;
#77020=CARTESIAN_POINT ( 'NONE',  ( -9.442253272394237840, -12.41089969410671223, 31.60739465890703670 ) ) ;
#77022=CARTESIAN_POINT ( 'NONE',  ( -12.23852561744506495, -2.523321265292115534, 31.42251411153756990 ) ) ;
#77024=ORIENTED_EDGE ( 'NONE', *, *, #78746, .F. ) ;
#77025=CARTESIAN_POINT ( 'NONE',  ( -18.22292621751614305, -5.667676309546435753, 34.40238873228292249 ) ) ;
#77026=CARTESIAN_POINT ( 'NONE',  ( -6.130147209438218781, -6.852621066184267029, 34.70813303252209181 ) ) ;
#77027=CARTESIAN_POINT ( 'NONE',  ( -10.39260507411620438, -10.11255958852956027, 34.01340905677048454 ) ) ;
#77028=CARTESIAN_POINT ( 'NONE',  ( 15.23076923076910916, -12.51329471203414379, 31.30864560766407578 ) ) ;
#77029=CARTESIAN_POINT ( 'NONE',  ( -11.78846153846154010, -2.499999999999999556, 29.81609845454691765 ) ) ;
#77032=EDGE_LOOP ( 'NONE', ( #26455, #74227 ) ) ;
#77033=ORIENTED_EDGE ( 'NONE', *, *, #88013, .T. ) ;
#77034=DIRECTION ( 'NONE',  ( -0.000000000000000000, 0.8660254037844399289, -0.4999999999999980016 ) ) ;
#77035=EDGE_CURVE ( 'NONE', #74290, #25133, #71035, .T. ) ;
#77036=ORIENTED_EDGE ( 'NONE', *, *, #74732, .F. ) ;
#77037=CARTESIAN_POINT ( 'NONE',  ( -1.384615384615383471, -8.120952969808772792, 34.71129190930000163 ) ) ;
#77038=CARTESIAN_POINT ( 'NONE',  ( -1.319360245102545681, -10.33852847137154107, 34.16647553114620450 ) ) ;
#77039=CARTESIAN_POINT ( 'NONE',  ( -14.30769230769242739, -6.879047030192662504, 34.71129190930017927 ) ) ;
#77041=CARTESIAN_POINT ( 'NONE',  ( -2.084912766423897335, -5.114059244376869984, 34.14424750095245287 ) ) ;
#77042=ADVANCED_FACE ( 'NONE', ( #22407 ), #30489, .F. ) ;
#77044=ORIENTED_EDGE ( 'NONE', *, *, #50345, .F. ) ;
#77045=CARTESIAN_POINT ( 'NONE',  ( -11.53846153846166089, -8.656820664282941280, 34.87096338111179961 ) ) ;
#77046=LINE ( 'NONE', #42822, #68337 ) ;
#77047=ORIENTED_EDGE ( 'NONE', *, *, #17546, .F. ) ;
#77048=CARTESIAN_POINT ( 'NONE',  ( -9.469528151039281028, -4.387253974876679230, 33.66317474335728832 ) ) ;
#77049=DIRECTION ( 'NONE',  ( 0.000000000000000000, 0.1736481776669275834, 0.9848077530122086864 ) ) ;
#77050=DIRECTION ( 'NONE',  ( -1.000000000000000000, 0.000000000000000000, 0.000000000000000000 ) ) ;
#77051=CARTESIAN_POINT ( 'NONE',  ( -2.531177232256638376, -12.69144148231606017, 30.53333754910549303 ) ) ;
#77052=CARTESIAN_POINT ( 'NONE',  ( -9.942330916529147800, -12.45566812827425451, 31.48439005359158926 ) ) ;
#77054=EDGE_CURVE ( 'NONE', #66983, #75887, #4296, .T. ) ;
#77055=FACE_OUTER_BOUND ( 'NONE', #82833, .T. ) ;
#77057=VERTEX_POINT ( 'NONE', #5242 ) ;
#77059=CARTESIAN_POINT ( 'NONE',  ( -1.634638621908349299, -12.22074536777954989, 31.39888409691088356 ) ) ;
#77060=CARTESIAN_POINT ( 'NONE',  ( -16.15384615384627409, -11.67786785259630911, 32.92929555188603530 ) ) ;
#77061=CARTESIAN_POINT ( 'NONE',  ( -13.38461538461538325, -8.564572088678739092, 35.78748833219616898 ) ) ;
#77062=EDGE_LOOP ( 'NONE', ( #86715, #25933 ) ) ;
#77063=CARTESIAN_POINT ( 'NONE',  ( 0.3308478584281516199, -3.957541250942360644, 33.62499894934982336 ) ) ;
#77064=CARTESIAN_POINT ( 'NONE',  ( -2.557715544985271983, -3.202444869320336451, 32.30641848906366675 ) ) ;
#77067=CARTESIAN_POINT ( 'NONE',  ( 1.134638653673032405, -9.148715823498378086, 34.47080413974185120 ) ) ;
#77068=CARTESIAN_POINT ( 'NONE',  ( 16.15384615384615330, -5.180354513474913603, 36.12317359536750416 ) ) ;
#77069=ORIENTED_EDGE ( 'NONE', *, *, #49745, .F. ) ;
#77072=CYLINDRICAL_SURFACE ( 'NONE', #17835, 0.2500000000000002220 ) ;
#77073=CARTESIAN_POINT ( 'NONE',  ( 8.068933387422255521, -5.913360116392399668, 34.49180327182771322 ) ) ;
#77074=CARTESIAN_POINT ( 'NONE',  ( -4.377331078410484189, -11.60425143139329940, 33.02411095842164457 ) ) ;
#77076=CARTESIAN_POINT ( 'NONE',  ( -13.25382494364843389, -2.845873456487965747, 32.17976146951972538 ) ) ;
#77079=FACE_OUTER_BOUND ( 'NONE', #22282, .T. ) ;
#77080=VERTEX_POINT ( 'NONE', #25068 ) ;
#77081=LINE ( 'NONE', #48712, #20335 ) ;
#77082=LINE ( 'NONE', #15388, #4750 ) ;
#77083=CARTESIAN_POINT ( 'NONE',  ( -4.088652172062795742, -2.506253911140448487, 29.99999999999988631 ) ) ;
#77084=VECTOR ( 'NONE', #52995, 1000.000000000000114 ) ;
#77085=CYLINDRICAL_SURFACE ( 'NONE', #13403, 0.2500000000000008882 ) ;
#77086=DIRECTION ( 'NONE',  ( 0.000000000000000000, 0.1736481776669267785, -0.9848077530122087975 ) ) ;
#77087=B_SPLINE_CURVE_WITH_KNOTS ( 'NONE', 3,
 ( #85550, #24276, #16203, #23824, #43668, #71577, #79686, #50849, #44540, #17540 ),
 .UNSPECIFIED., .F., .F.,
 ( 4, 2, 2, 2, 4 ),
 ( 0.000000000000000000, 0.0001954311564186862781, 0.0003908623128373725562, 0.0005862934692560588072, 0.0007817246256747451124 ),
 .UNSPECIFIED. ) ;
#77090=FACE_BOUND ( 'NONE', #64662, .T. ) ;
#77091=VERTEX_POINT ( 'NONE', #59740 ) ;
#77092=CARTESIAN_POINT ( 'NONE',  ( 15.36129493253279854, -2.619367082507849442, 30.83698974864643461 ) ) ;
#77093=CARTESIAN_POINT ( 'NONE',  ( -18.13014796973169851, -11.04286588640299094, 33.62463336215343901 ) ) ;
#77094=DIRECTION ( 'NONE',  ( -0.000000000000000000, -0.8660254037844398178, -0.4999999999999980571 ) ) ;
#77096=VERTEX_POINT ( 'NONE', #86351 ) ;
#77097=ORIENTED_EDGE ( 'NONE', *, *, #886, .T. ) ;
#77098=EDGE_LOOP ( 'NONE', ( #61488, #75811, #5775, #57651 ) ) ;
#77099=CARTESIAN_POINT ( 'NONE',  ( -10.74607521849492464, -8.191372820521381826, 34.95448215188424967 ) ) ;
#77100=ORIENTED_EDGE ( 'NONE', *, *, #22899, .T. ) ;
#77102=CARTESIAN_POINT ( 'NONE',  ( -5.999999999999998224, -13.88283147151868846, 33.14645433367849847 ) ) ;
#77103=CARTESIAN_POINT ( 'NONE',  ( 17.07692307692295586, -3.643525952248796163, 33.31231777344771672 ) ) ;
#77104=CARTESIAN_POINT ( 'NONE',  ( -17.14300545628321615, -2.833524468853757305, 32.15551576947924417 ) ) ;
#77105=ORIENTED_EDGE ( 'NONE', *, *, #54701, .F. ) ;
#77106=CARTESIAN_POINT ( 'NONE',  ( 13.16168916709924197, -10.61292498521070549, 33.66303323003028680 ) ) ;
#77107=DIRECTION ( 'NONE',  ( -0.000000000000000000, -0.8660254037844399289, -0.4999999999999980016 ) ) ;
#77108=CARTESIAN_POINT ( 'NONE',  ( 9.692307692307695177, -12.78798330534102945, 29.74999999999997868 ) ) ;
#77109=CARTESIAN_POINT ( 'NONE',  ( -9.692307692307812417, -3.835265460704628371, 33.15142922262033665 ) ) ;
#77110=VERTEX_POINT ( 'NONE', #52970 ) ;
#77111=B_SPLINE_CURVE_WITH_KNOTS ( 'NONE', 3,
 ( #61820, #26714, #20404, #47868, #87556, #66818, #6012, #33478, #14085, #19077 ),
 .UNSPECIFIED., .F., .F.,
 ( 4, 2, 2, 2, 4 ),
 ( 0.0007817359430256372700, 0.0009771253907250052138, 0.001172514838424373266, 0.001367904286123741101, 0.001563293733823109153 ),
 .UNSPECIFIED. ) ;
#77112=AXIS2_PLACEMENT_3D ( 'NONE', #31664, #44712, #10950 ) ;
#77113=ORIENTED_EDGE ( 'NONE', *, *, #47555, .F. ) ;
#77114=ORIENTED_EDGE ( 'NONE', *, *, #50500, .F. ) ;
#77115=CARTESIAN_POINT ( 'NONE',  ( -4.023054346021365468, -9.804649428959608670, 34.18742332936588468 ) ) ;
#77116=B_SPLINE_CURVE_WITH_KNOTS ( 'NONE', 3,
 ( #67904, #46740, #67017, #54823, #26476, #68343, #19714, #33676, #75534, #80984 ),
 .UNSPECIFIED., .F., .F.,
 ( 4, 2, 2, 2, 4 ),
 ( 0.000000000000000000, 0.0001954311564186864407, 0.0003908623128373728815, 0.0005862934692560593493, 0.0007817246256747457630 ),
 .UNSPECIFIED. ) ;
#77117=CARTESIAN_POINT ( 'NONE',  ( -7.911424292114620727, -6.879047030191174805, 34.71129190930000163 ) ) ;
#77118=CARTESIAN_POINT ( 'NONE',  ( -13.45069879557126313, -5.557115091759785130, 34.35708131394839171 ) ) ;
#77119=CARTESIAN_POINT ( 'NONE',  ( 11.53846153846141576, -2.379036618888197729, 30.90682066428292885 ) ) ;
#77121=FACE_BOUND ( 'NONE', #88895, .T. ) ;
#77122=CARTESIAN_POINT ( 'NONE',  ( -7.053767526187231240, -3.338472653186242756, 32.95098750199972670 ) ) ;
#77123=ORIENTED_EDGE ( 'NONE', *, *, #72965, .T. ) ;
#77124=CARTESIAN_POINT ( 'NONE',  ( -3.165513659493205623, -2.625532179533470512, 30.86335684631491105 ) ) ;
#77125=CARTESIAN_POINT ( 'NONE',  ( 2.057692307692309708, -2.499999999999998668, 29.75000000000000355 ) ) ;
#77126=CARTESIAN_POINT ( 'NONE',  ( -1.450698795571264466, -3.513871655860377086, 32.76840700105978499 ) ) ;
#77127=CARTESIAN_POINT ( 'NONE',  ( 7.173131342990376247, -9.233818618650603938, 34.70587769442853698 ) ) ;
#77128=ORIENTED_EDGE ( 'NONE', *, *, #56462, .T. ) ;
#77129=CARTESIAN_POINT ( 'NONE',  ( 5.011653076366756387, -12.70778746994557551, 30.41441678777548319 ) ) ;
#77130=EDGE_LOOP ( 'NONE', ( #56163, #10936 ) ) ;
#77131=FACE_BOUND ( 'NONE', #47804, .T. ) ;
#77132=CARTESIAN_POINT ( 'NONE',  ( 4.853996859406926490, -5.667676309546437530, 34.40238873228292249 ) ) ;
#77133=ADVANCED_FACE ( 'NONE', ( #18763 ), #87235, .F. ) ;
#77135=CYLINDRICAL_SURFACE ( 'NONE', #80849, 0.2500000000000002220 ) ;
#77136=CARTESIAN_POINT ( 'NONE',  ( -11.40766973063674961, -11.71459661697925903, 32.44059661609676937 ) ) ;
#77137=ORIENTED_EDGE ( 'NONE', *, *, #58953, .T. ) ;
#77140=CARTESIAN_POINT ( 'NONE',  ( -14.53117725141625627, -4.386631170607603991, 33.66268669641500111 ) ) ;
#77141=CARTESIAN_POINT ( 'NONE',  ( -15.09997878980228059, -9.929761469519743144, 34.40412654351204225 ) ) ;
#77144=VECTOR ( 'NONE', #47488, 1000.000000000000227 ) ;
#77145=CARTESIAN_POINT ( 'NONE',  ( -4.023054346021365468, -6.413143153341454017, 34.63066358083362672 ) ) ;
#77147=CARTESIAN_POINT ( 'NONE',  ( -9.019207500173124004, -3.627789207965226748, 32.91389620160131102 ) ) ;
#77148=ORIENTED_EDGE ( 'NONE', *, *, #80910, .F. ) ;
#77149=CARTESIAN_POINT ( 'NONE',  ( 3.230769230769231726, -2.538708090699994813, 30.37095296980875503 ) ) ;
#77150=CARTESIAN_POINT ( 'NONE',  ( -6.792285115252137295, -11.71459661697925903, 32.44059661609676937 ) ) ;
#77151=CARTESIAN_POINT ( 'NONE',  ( 13.38461538461538680, -8.973038597847269315, 34.52809138561121927 ) ) ;
#77152=CARTESIAN_POINT ( 'NONE',  ( 12.52679403281448600, -4.481592998940250538, 33.73612834413965089 ) ) ;
#77153=CARTESIAN_POINT ( 'NONE',  ( 16.15384615384615330, -2.538708090699994813, 30.37095296980875503 ) ) ;
#77155=EDGE_CURVE ( 'NONE', #51245, #75182, #81674, .T. ) ;
#77156=LINE ( 'NONE', #42935, #53589 ) ;
#77158=ORIENTED_EDGE ( 'NONE', *, *, #12658, .T. ) ;
#77159=CARTESIAN_POINT ( 'NONE',  ( -0.5922299282060208281, -5.582088688514999397, 34.36776431015576350 ) ) ;
#77160=CARTESIAN_POINT ( 'NONE',  ( -9.626240358957616650, -11.35647404775217595, 33.31231777344666511 ) ) ;
#77161=VERTEX_POINT ( 'NONE', #45328 ) ;
#77164=CARTESIAN_POINT ( 'NONE',  ( -10.86540785267757592, -11.37209801155882971, 32.91403422569032955 ) ) ;
#77165=CARTESIAN_POINT ( 'NONE',  ( -17.32694631421604115, -9.271318131107980420, 34.42618302367067429 ) ) ;
#77166=CARTESIAN_POINT ( 'NONE',  ( -15.23076923076922995, -13.78497067705608181, 32.30358669280327177 ) ) ;
#77167=CARTESIAN_POINT ( 'NONE',  ( -15.23076923076935074, -5.219633306517616589, 34.19971097300220464 ) ) ;
#77169=CARTESIAN_POINT ( 'NONE',  ( -8.769230769230892619, -3.083524468854526912, 32.58852847137268327 ) ) ;
#77170=CARTESIAN_POINT ( 'NONE',  ( 0.2386721984753616965, -2.251424796025575770, 29.88072029997477586 ) ) ;
#77172=DIRECTION ( 'NONE',  ( -0.000000000000000000, 0.5000000000000011102, -0.8660254037844380415 ) ) ;
#77173=CARTESIAN_POINT ( 'NONE',  ( 17.86930853333243974, -11.71456829005830080, 32.44064028649416542 ) ) ;
#77174=ADVANCED_FACE ( 'NONE', ( #72801 ), #73257, .F. ) ;
#77175=CARTESIAN_POINT ( 'NONE',  ( 12.33084699487090496, -11.71456829005830080, 32.44064028649416542 ) ) ;
#77176=DIRECTION ( 'NONE',  ( -0.000000000000000000, -0.9848077530122086864, -0.1736481776669273613 ) ) ;
#77178=EDGE_LOOP ( 'NONE', ( #7442, #80627, #80594, #6859 ) ) ;
#77181=LINE ( 'NONE', #55134, #31362 ) ;
#77182=CARTESIAN_POINT ( 'NONE',  ( -16.82692307692307665, -7.500000000000001776, 35.04278698407183867 ) ) ;
#77183=DIRECTION ( 'NONE',  ( -0.000000000000000000, 0.5000000000000011102, -0.8660254037844381525 ) ) ;
#77184=EDGE_LOOP ( 'NONE', ( #34459, #84011, #47732, #7103 ) ) ;
#77185=VECTOR ( 'NONE', #88391, 999.9999999999998863 ) ;
#77186=CARTESIAN_POINT ( 'NONE',  ( -15.93083330975275658, -8.282913670948747864, 34.94150082978203642 ) ) ;
#77187=CARTESIAN_POINT ( 'NONE',  ( -12.39536932057580643, -7.250054483168843156, 34.74374881642865631 ) ) ;
#77188=CARTESIAN_POINT ( 'NONE',  ( -8.899921372341079717, -9.084618155246140248, 34.75535874321725771 ) ) ;
#77189=B_SPLINE_CURVE_WITH_KNOTS ( 'NONE', 3,
 ( #54999, #67636, #82041, #80720, #5038, #46903, #59978, #47348, #27529, #5932 ),
 .UNSPECIFIED., .F., .F.,
 ( 4, 2, 2, 2, 4 ),
 ( 0.000000000000000000, 0.0001954311564186863323, 0.0003908623128373726646, 0.0005862934692560590241, 0.0007817246256747453293 ),
 .UNSPECIFIED. ) ;
#77190=ORIENTED_EDGE ( 'NONE', *, *, #22625, .F. ) ;
#77191=LINE ( 'NONE', #8748, #71661 ) ;
#77192=VERTEX_POINT ( 'NONE', #44427 ) ;
#77193=CARTESIAN_POINT ( 'NONE',  ( 13.13463864056679675, -12.41104346484419452, 31.60698883733904196 ) ) ;
#77194=CARTESIAN_POINT ( 'NONE',  ( -3.480792468062195333, -12.22074536777954989, 31.39888409691088356 ) ) ;
#77197=CARTESIAN_POINT ( 'NONE',  ( -9.758390071667827570, -8.164416787775445883, 34.95778746994557906 ) ) ;
#77198=DIRECTION ( 'NONE',  ( 0.000000000000000000, 1.000000000000000000, 0.000000000000000000 ) ) ;
#77202=VERTEX_POINT ( 'NONE', #25953 ) ;
#77203=ORIENTED_EDGE ( 'NONE', *, *, #39907, .T. ) ;
#77204=CARTESIAN_POINT ( 'NONE',  ( 13.13459214732242408, -3.202444869320336451, 32.30641848906366675 ) ) ;
#77205=CARTESIAN_POINT ( 'NONE',  ( 13.38461538461526601, -10.21337939537710326, 33.94971097300076224 ) ) ;
#77207=CARTESIAN_POINT ( 'NONE',  ( -2.057637887778853258, -11.47946981652013498, 33.17500667209846910 ) ) ;
#77208=CARTESIAN_POINT ( 'NONE',  ( 4.153846153846154188, -6.386643153685126251, 34.62446782046654192 ) ) ;
#77211=ORIENTED_EDGE ( 'NONE', *, *, #83334, .T. ) ;
#77212=B_SPLINE_CURVE_WITH_KNOTS ( 'NONE', 3,
 ( #46321, #82337, #40027, #67488, #76902, #83219, #55730, #8888, #57060, #7559 ),
 .UNSPECIFIED., .F., .F.,
 ( 4, 2, 2, 2, 4 ),
 ( 0.000000000000000000, 0.0001954339881912772715, 0.0003908679763825545429, 0.0005863019645738318415, 0.0007817359527651090859 ),
 .UNSPECIFIED. ) ;
#77213=EDGE_CURVE ( 'NONE', #37064, #59376, #68748, .T. ) ;
#77214=ORIENTED_EDGE ( 'NONE', *, *, #3219, .F. ) ;
#77215=CARTESIAN_POINT ( 'NONE',  ( 4.153846153846030731, -4.320704448113951379, 33.92786785259630022 ) ) ;
#77217=CARTESIAN_POINT ( 'NONE',  ( 8.992010310499175318, -8.496831190052093419, 34.64984203495476578 ) ) ;
#77218=CARTESIAN_POINT ( 'NONE',  ( 14.37294744720514750, -5.094484230520773593, 34.41647553114626845 ) ) ;
#77221=EDGE_LOOP ( 'NONE', ( #53110, #28484, #9731, #76720 ) ) ;
#77222=ORIENTED_EDGE ( 'NONE', *, *, #16516, .T. ) ;
#77223=CARTESIAN_POINT ( 'NONE',  ( 13.63461538461538858, -2.499999999999999556, 29.81604066197449754 ) ) ;
#77226=FACE_BOUND ( 'NONE', #30542, .T. ) ;
#77228=ADVANCED_FACE ( 'NONE', ( #3455 ), #30921, .F. ) ;
#77229=LINE ( 'NONE', #15539, #1707 ) ;
#77231=CARTESIAN_POINT ( 'NONE',  ( 2.241608896736428047, -8.120952969808774569, 34.71129190930000163 ) ) ;
#77233=AXIS2_PLACEMENT_3D ( 'NONE', #60785, #75201, #41410 ) ;
#77234=CARTESIAN_POINT ( 'NONE',  ( -39.05038313613820122, -2.499999999999999556, 27.25000000000000000 ) ) ;
#77235=EDGE_CURVE ( 'NONE', #60559, #49728, #9812, .T. ) ;
#77236=CARTESIAN_POINT ( 'NONE',  ( 7.846153846153723244, -4.320704448113951379, 33.92786785259630022 ) ) ;
#77237=CARTESIAN_POINT ( 'NONE',  ( 0.4615384615384611200, -12.37446782046654192, 30.86335684631486131 ) ) ;
#77238=EDGE_LOOP ( 'NONE', ( #36989, #55695 ) ) ;
#77239=CARTESIAN_POINT ( 'NONE',  ( 8.638540166120462160, -11.37499894934982692, 33.29245874905763003 ) ) ;
#77240=CARTESIAN_POINT ( 'NONE',  ( 2.057669083470850424, -12.07920672191015221, 32.31858351112116168 ) ) ;
#77241=DIRECTION ( 'NONE',  ( -0.000000000000000000, -0.6427876096865404731, -0.7660444431189771253 ) ) ;
#77242=DIRECTION ( 'NONE',  ( 0.000000000000000000, 0.4999999999999985567, 0.8660254037844395958 ) ) ;
#77244=CARTESIAN_POINT ( 'NONE',  ( 6.130525701763563262, -10.19071101563364756, 33.96452234770658407 ) ) ;
#77245=CARTESIAN_POINT ( 'NONE',  ( -8.899791360972686860, -2.504760397472875155, 29.97295953869789997 ) ) ;
#77246=CARTESIAN_POINT ( 'NONE',  ( 11.78840705680968171, -4.336752205174649433, 33.62275283266504289 ) ) ;
#77247=ADVANCED_FACE ( 'NONE', ( #60619 ), #699, .F. ) ;
#77248=CYLINDRICAL_SURFACE ( 'NONE', #54023, 0.2499999999999986955 ) ;
#77249=LINE ( 'NONE', #35832, #40071 ) ;
#77250=CARTESIAN_POINT ( 'NONE',  ( 2.530705151785703322, -6.460100341425561332, 34.89618726649961644 ) ) ;
#77251=DIRECTION ( 'NONE',  ( -0.000000000000000000, -0.7660444431189791237, -0.6427876096865379196 ) ) ;
#77253=EDGE_LOOP ( 'NONE', ( #30735, #37472 ) ) ;
#77255=EDGE_LOOP ( 'NONE', ( #26108, #12116, #65809, #49661 ) ) ;
#77256=EDGE_CURVE ( 'NONE', #77110, #53903, #88132, .T. ) ;
#77257=LINE ( 'NONE', #42598, #37739 ) ;
#77258=AXIS2_PLACEMENT_3D ( 'NONE', #10652, #65579, #3879 ) ;
#77259=ORIENTED_EDGE ( 'NONE', *, *, #55992, .T. ) ;
#77260=CARTESIAN_POINT ( 'NONE',  ( -4.153846153846152411, -2.499999999999998668, 29.75000000000001421 ) ) ;
#77261=CARTESIAN_POINT ( 'NONE',  ( 14.05771556364371833, -2.318417181685855422, 30.59732222474233865 ) ) ;
#77263=ORIENTED_EDGE ( 'NONE', *, *, #58838, .T. ) ;
#77264=CARTESIAN_POINT ( 'NONE',  ( -18.13014720943822056, -12.45813303252208648, 30.39737893381572675 ) ) ;
#77266=CARTESIAN_POINT ( 'NONE',  ( 17.32697738856138869, -8.303483539816726378, 34.68545999027711702 ) ) ;
#77267=CARTESIAN_POINT ( 'NONE',  ( 7.173131342990376247, -10.06805714834173848, 34.32951233291982618 ) ) ;
#77268=CARTESIAN_POINT ( 'NONE',  ( -5.143006487878955646, -4.786620604624113540, 33.94971097300155805 ) ) ;
#77269=FACE_OUTER_BOUND ( 'NONE', #63986, .T. ) ;
#77271=CARTESIAN_POINT ( 'NONE',  ( 5.076923076922954969, -8.613356846316285953, 34.62446782046622218 ) ) ;
#77273=CARTESIAN_POINT ( 'NONE',  ( -39.05038313613820122, -2.249999999999998668, 29.75000000000000355 ) ) ;
#77274=CYLINDRICAL_SURFACE ( 'NONE', #47743, 0.2499999999999973355 ) ;
#77275=EDGE_CURVE ( 'NONE', #75030, #10587, #74146, .T. ) ;
#77276=AXIS2_PLACEMENT_3D ( 'NONE', #38617, #39522, #53002 ) ;
#77277=CARTESIAN_POINT ( 'NONE',  ( 13.51514108637895006, -4.459921816937791661, 33.71989282347011851 ) ) ;
#77279=DIRECTION ( 'NONE',  ( 1.000000000000000000, 0.000000000000000000, 0.000000000000000000 ) ) ;
#77280=ORIENTED_EDGE ( 'NONE', *, *, #3163, .F. ) ;
#77281=EDGE_CURVE ( 'NONE', #67532, #43517, #6574, .T. ) ;
#77282=CARTESIAN_POINT ( 'NONE',  ( 7.146503884938495865, -7.630147231320743018, 34.74852402298682819 ) ) ;
#77283=CARTESIAN_POINT ( 'NONE',  ( -11.28851602011339672, -8.433404298154334455, 34.66254593164985920 ) ) ;
#77284=DIRECTION ( 'NONE',  ( 0.000000000000000000, 0.1736481776669275834, 0.9848077530122086864 ) ) ;
#77285=CARTESIAN_POINT ( 'NONE',  ( 5.326977388561391358, -2.779044189368096163, 31.39831045268886456 ) ) ;
#77286=EDGE_CURVE ( 'NONE', #68899, #20422, #45130, .T. ) ;
#77288=CARTESIAN_POINT ( 'NONE',  ( -14.17690186672535901, -3.957578996910242619, 33.62503395064540257 ) ) ;
#77289=B_SPLINE_CURVE_WITH_KNOTS ( 'NONE', 3,
 ( #60022, #87526, #25801, #26242, #53709, #3742, #86182, #79419, #86634, #28015 ),
 .UNSPECIFIED., .F., .F.,
 ( 4, 2, 2, 2, 4 ),
 ( 0.000000000000000000, 0.0001954311564186863865, 0.0003908623128373727731, 0.0005862934692560591325, 0.0007817246256747455461 ),
 .UNSPECIFIED. ) ;
#77292=ORIENTED_EDGE ( 'NONE', *, *, #56700, .T. ) ;
#77294=AXIS2_PLACEMENT_3D ( 'NONE', #49068, #8535, #448 ) ;
#77295=ORIENTED_EDGE ( 'NONE', *, *, #29377, .T. ) ;
#77296=CARTESIAN_POINT ( 'NONE',  ( -11.31544869436814160, -11.43677907613344757, 33.22367315496202167 ) ) ;
#77297=CARTESIAN_POINT ( 'NONE',  ( 6.792385456409365752, -2.729777683071817229, 31.24903638046268739 ) ) ;
#77298=CARTESIAN_POINT ( 'NONE',  ( 2.307692307692187583, -11.48612834414049644, 32.76840700105863391 ) ) ;
#77300=CARTESIAN_POINT ( 'NONE',  ( 3.230769230769108269, -9.528491918059723176, 34.59228464037033035 ) ) ;
#77301=CARTESIAN_POINT ( 'NONE',  ( 17.77707304109314634, -9.172386477786394821, 34.72672124145550043 ) ) ;
#77302=EDGE_CURVE ( 'NONE', #48730, #88631, #89011, .T. ) ;
#77303=ORIENTED_EDGE ( 'NONE', *, *, #81964, .F. ) ;
#77304=CARTESIAN_POINT ( 'NONE',  ( 16.15384615384603251, -5.219633306517616589, 34.19971097300220464 ) ) ;
#77306=ADVANCED_FACE ( 'NONE', ( #68272 ), #88571, .F. ) ;
#77307=VERTEX_POINT ( 'NONE', #82238 ) ;
#77308=CARTESIAN_POINT ( 'NONE',  ( -9.942307692307691624, -2.249999999999998668, 29.75000000000000355 ) ) ;
#77311=EDGE_CURVE ( 'NONE', #15474, #47909, #67387, .T. ) ;
#77312=ADVANCED_FACE ( 'NONE', ( #19640 ), #26846, .F. ) ;
#77313=B_SPLINE_CURVE_WITH_KNOTS ( 'NONE', 3,
 ( #42859, #75312, #76639, #34758, #35658, #62228, #36104, #28447, #13605, #22138 ),
 .UNSPECIFIED., .F., .F.,
 ( 4, 2, 2, 2, 4 ),
 ( 0.000000000000000000, 0.0001954311564186876063, 0.0003908623128373752125, 0.0005862934692560628188, 0.0007817246256747504250 ),
 .UNSPECIFIED. ) ;
#77314=CARTESIAN_POINT ( 'NONE',  ( -10.83831083290076158, -4.887634598454295265, 34.01352882383564946 ) ) ;
#77315=EDGE_CURVE ( 'NONE', #29230, #74248, #18345, .T. ) ;
#77317=CARTESIAN_POINT ( 'NONE',  ( 8.069166690247241647, -12.64618726649961289, 30.78989965857442712 ) ) ;
#77318=EDGE_LOOP ( 'NONE', ( #6559, #1979, #21792, #48350 ) ) ;
#77319=ORIENTED_EDGE ( 'NONE', *, *, #60449, .F. ) ;
#77320=ADVANCED_FACE ( 'NONE', ( #7466 ), #34921, .F. ) ;
#77322=CARTESIAN_POINT ( 'NONE',  ( -6.700064078983525739, -2.889357225399416862, 32.26129605718031002 ) ) ;
#77323=CARTESIAN_POINT ( 'NONE',  ( -14.05763788777885637, -2.318338780012835443, 30.59689888758630261 ) ) ;
#77324=ORIENTED_EDGE ( 'NONE', *, *, #21888, .T. ) ;
#77325=CARTESIAN_POINT ( 'NONE',  ( -39.05038313613820122, -2.499999999999999556, 29.75000000000000355 ) ) ;
#77326=CARTESIAN_POINT ( 'NONE',  ( 5.010839665967194989, -3.513871655860377086, 32.76840700105978499 ) ) ;
#77327=CARTESIAN_POINT ( 'NONE',  ( 2.373759641042385127, -9.058645607665452459, 34.76329471203371924 ) ) ;
#77329=VECTOR ( 'NONE', #22008, 1000.000000000000000 ) ;
#77330=CARTESIAN_POINT ( 'NONE',  ( 11.53846153846153832, -5.180354513474913603, 36.12317359536750416 ) ) ;
#77332=EDGE_LOOP ( 'NONE', ( #67675, #56150 ) ) ;
#77333=FACE_BOUND ( 'NONE', #66926, .T. ) ;
#77334=CARTESIAN_POINT ( 'NONE',  ( 11.47237812750566022, -4.786620604624113540, 33.94971097300155805 ) ) ;
#77336=CARTESIAN_POINT ( 'NONE',  ( 2.084765348785459604, -12.38737895849757820, 31.66785238281580206 ) ) ;
#77337=CARTESIAN_POINT ( 'NONE',  ( 8.068933515131908152, -10.97394488606064122, 33.68653795673694873 ) ) ;
#77338=CARTESIAN_POINT ( 'NONE',  ( -6.673022611438608642, -2.564540009722896752, 30.55348353981670684 ) ) ;
#77339=CARTESIAN_POINT ( 'NONE',  ( 16.08776274289027697, -2.538708090699995257, 30.37095296980875148 ) ) ;
#77341=ORIENTED_EDGE ( 'NONE', *, *, #50607, .T. ) ;
#77342=CARTESIAN_POINT ( 'NONE',  ( 10.61538461538461675, -6.435427911321262684, 35.78748833219616898 ) ) ;
#77343=CARTESIAN_POINT ( 'NONE',  ( 5.011653076366756387, -4.320704448112771878, 33.92786785259540494 ) ) ;
#77344=EDGE_CURVE ( 'NONE', #40637, #79352, #75040, .T. ) ;
#77345=EDGE_LOOP ( 'NONE', ( #49927, #27983 ) ) ;
#77347=CARTESIAN_POINT ( 'NONE',  ( 7.846153846153723244, -5.094484230521993062, 34.41647553114689373 ) ) ;
#77349=CARTESIAN_POINT ( 'NONE',  ( 16.15384615384615330, -6.343179335718451384, 34.87096338111211935 ) ) ;
#77351=AXIS2_PLACEMENT_3D ( 'NONE', #81791, #14207, #39148 ) ;
#77352=CARTESIAN_POINT ( 'NONE',  ( 6.000000000000001776, -13.75783147151868846, 33.36296068462461051 ) ) ;
#77353=CYLINDRICAL_SURFACE ( 'NONE', #1226, 0.2500000000000002220 ) ;
#77354=FACE_BOUND ( 'NONE', #58109, .T. ) ;
#77355=CYLINDRICAL_SURFACE ( 'NONE', #56226, 0.2499999999999979738 ) ;
#77356=FACE_OUTER_BOUND ( 'NONE', #69381, .T. ) ;
#77357=CARTESIAN_POINT ( 'NONE',  ( -15.93083480223330817, -2.554770724473668597, 30.48948780036025852 ) ) ;
#77358=CARTESIAN_POINT ( 'NONE',  ( -5.076923076923075762, -3.937682226553329556, 33.60647404775216529 ) ) ;
#77359=CARTESIAN_POINT ( 'NONE',  ( -12.71151519248081740, -4.236021600441997492, 33.53823185664189310 ) ) ;
#77360=CARTESIAN_POINT ( 'NONE',  ( 1.134615384615387246, -2.249999999999998668, 29.75000000000000355 ) ) ;
#77361=VECTOR ( 'NONE', #64456, 1000.000000000000114 ) ;
#77363=ORIENTED_EDGE ( 'NONE', *, *, #77400, .T. ) ;
#77364=ORIENTED_EDGE ( 'NONE', *, *, #39240, .F. ) ;
#77365=CYLINDRICAL_SURFACE ( 'NONE', #60761, 0.2500000000000008882 ) ;
#77367=CARTESIAN_POINT ( 'NONE',  ( -0.5916864312701554107, -3.625366637846545448, 33.29286588640298561 ) ) ;
#77368=CARTESIAN_POINT ( 'NONE',  ( -17.01166750564705055, -11.48612834413965977, 32.76840700105972815 ) ) ;
#77369=CARTESIAN_POINT ( 'NONE',  ( -17.01166750564705055, -6.879047030191284051, 34.71129190930002295 ) ) ;
#77371=CARTESIAN_POINT ( 'NONE',  ( 3.931019461367150303, -7.369208160676172348, 34.74850200257122879 ) ) ;
#77372=CARTESIAN_POINT ( 'NONE',  ( 18.25005431163831560, -3.136992222400443175, 32.19305428654138979 ) ) ;
#77373=CARTESIAN_POINT ( 'NONE',  ( 15.23076923076911093, -11.94971097300221174, 32.03036669348237098 ) ) ;
#77374=CARTESIAN_POINT ( 'NONE',  ( -1.607541602131531633, -12.39988816332205701, 30.74660775122750778 ) ) ;
#77375=CARTESIAN_POINT ( 'NONE',  ( -17.01166793741023042, -5.094484230520771817, 34.41647553114626845 ) ) ;
#77376=CARTESIAN_POINT ( 'NONE',  ( 6.000000000000001776, -2.499999999999998668, 29.50000000000001066 ) ) ;
#77377=CARTESIAN_POINT ( 'NONE',  ( 9.692307692307695177, -1.242168528481310874, 33.36296068462461051 ) ) ;
#77378=EDGE_CURVE ( 'NONE', #40578, #53938, #50554, .T. ) ;
#77379=EDGE_CURVE ( 'NONE', #16174, #19274, #29036, .T. ) ;
#77383=CARTESIAN_POINT ( 'NONE',  ( 0.6845498131513096940, -2.554770724473668153, 30.48948780036025852 ) ) ;
#77386=CARTESIAN_POINT ( 'NONE',  ( -2.530619266599154926, -4.762599654559228846, 34.23009711892697737 ) ) ;
#77387=CARTESIAN_POINT ( 'NONE',  ( -16.08777882049607655, -2.486705287966280320, 31.30864560766543647 ) ) ;
#77388=ORIENTED_EDGE ( 'NONE', *, *, #44423, .T. ) ;
#77389=CYLINDRICAL_SURFACE ( 'NONE', #71536, 0.2499999999999986955 ) ;
#77390=CARTESIAN_POINT ( 'NONE',  ( -7.846153846153967493, -12.51329471203414379, 31.30864560766407578 ) ) ;
#77391=EDGE_LOOP ( 'NONE', ( #39438, #52392, #82104, #14184 ) ) ;
#77392=LINE ( 'NONE', #22011, #983 ) ;
#77393=CARTESIAN_POINT ( 'NONE',  ( -4.853911725310227077, -9.886259254753566594, 34.14407573483972413 ) ) ;
#77395=VERTEX_POINT ( 'NONE', #55633 ) ;
#77396=B_SPLINE_CURVE_WITH_KNOTS ( 'NONE', 3,
 ( #11341, #73501, #39720, #18552, #73944, #19434, #87931, #4588, #88804, #66283 ),
 .UNSPECIFIED., .F., .F.,
 ( 4, 2, 2, 2, 4 ),
 ( 0.0007817359527651101701, 0.0009771254036996489256, 0.001172514854634187790, 0.001367904305568726653, 0.001563293756503265517 ),
 .UNSPECIFIED. ) ;
#77397=CARTESIAN_POINT ( 'NONE',  ( -13.31854703361294590, -2.538708090699994813, 30.37095296980875503 ) ) ;
#77398=VECTOR ( 'NONE', #34544, 1000.000000000000114 ) ;
#77400=EDGE_CURVE ( 'NONE', #75052, #4668, #73055, .T. ) ;
#77401=ORIENTED_EDGE ( 'NONE', *, *, #47617, .T. ) ;
#77402=B_SPLINE_CURVE_WITH_KNOTS ( 'NONE', 3,
 ( #82168, #19567, #47921, #68205, #12811, #12375, #75840, #48361, #33083, #46601 ),
 .UNSPECIFIED., .F., .F.,
 ( 4, 2, 2, 2, 4 ),
 ( 0.0007817359430256262112, 0.0009771253907249911191, 0.001172514838424356136, 0.001367904286123721152, 0.001563293733823086168 ),
 .UNSPECIFIED. ) ;
#77404=DIRECTION ( 'NONE',  ( -0.000000000000000000, 0.7660444431189791237, -0.6427876096865379196 ) ) ;
#77406=ORIENTED_EDGE ( 'NONE', *, *, #81900, .T. ) ;
#77407=ORIENTED_EDGE ( 'NONE', *, *, #12658, .F. ) ;
#77408=ADVANCED_FACE ( 'NONE', ( #56086 ), #48882, .F. ) ;
#77409=ORIENTED_EDGE ( 'NONE', *, *, #39271, .T. ) ;
#77410=CARTESIAN_POINT ( 'NONE',  ( -5.143005456283209931, -9.058645607665454236, 34.76329471203372634 ) ) ;
#77411=CARTESIAN_POINT ( 'NONE',  ( -14.55766903863466055, -3.137211980971221781, 32.19342716148376837 ) ) ;
#77414=CARTESIAN_POINT ( 'NONE',  ( 2.980792486720640344, -10.06842814019191401, 34.32929386961144758 ) ) ;
#77415=EDGE_CURVE ( 'NONE', #49885, #14228, #15995, .T. ) ;
#77418=CARTESIAN_POINT ( 'NONE',  ( 20.99999999999999645, -4.249999999999998224, 27.25000000000000000 ) ) ;
#77419=ORIENTED_EDGE ( 'NONE', *, *, #66571, .T. ) ;
#77420=VECTOR ( 'NONE', #59726, 1000.000000000000227 ) ;
#77421=EDGE_CURVE ( 'NONE', #6352, #62909, #9717, .T. ) ;
#77422=CARTESIAN_POINT ( 'NONE',  ( 9.915319043920547415, -12.39991518177334129, 30.74647679643404530 ) ) ;
#77425=CARTESIAN_POINT ( 'NONE',  ( 7.911409417429871027, -5.219633306516380244, 34.19971097300157936 ) ) ;
#77426=ORIENTED_EDGE ( 'NONE', *, *, #30767, .T. ) ;
#77427=EDGE_CURVE ( 'NONE', #30124, #75360, #12916, .T. ) ;
#77428=ORIENTED_EDGE ( 'NONE', *, *, #34973, .T. ) ;
#77429=CARTESIAN_POINT ( 'NONE',  ( 9.757562831820530747, -8.656820664281605460, 34.87096338111211224 ) ) ;
#77430=EDGE_LOOP ( 'NONE', ( #50122, #42663, #70220, #10209 ) ) ;
#77431=DIRECTION ( 'NONE',  ( 0.000000000000000000, 0.1736481776669267785, -0.9848077530122087975 ) ) ;
#77432=CARTESIAN_POINT ( 'NONE',  ( -15.93083480223330817, -3.587049720035815348, 32.86302985866382897 ) ) ;
#77433=EDGE_LOOP ( 'NONE', ( #87788, #40042, #48426, #57648 ) ) ;
#77435=CARTESIAN_POINT ( 'NONE',  ( 15.23076923076923173, -2.292212530054420494, 30.41441678777542634 ) ) ;
#77436=CARTESIAN_POINT ( 'NONE',  ( 5.142178648199100977, -11.48612834413965977, 32.76840700105972815 ) ) ;
#77437=CARTESIAN_POINT ( 'NONE',  ( 6.792928953345228393, -5.915902021225892149, 34.75552854090298638 ) ) ;
#77438=FACE_BOUND ( 'NONE', #24450, .T. ) ;
#77439=CARTESIAN_POINT ( 'NONE',  ( 7.912221179503920787, -12.34228464037088813, 31.77849191805839268 ) ) ;
#77440=CARTESIAN_POINT ( 'NONE',  ( 8.769230769230645706, -10.33852847137269571, 34.16647553114546554 ) ) ;
#77441=CARTESIAN_POINT ( 'NONE',  ( 13.38461538461538680, -12.62096338111211580, 30.90682066428153263 ) ) ;
#77442=CARTESIAN_POINT ( 'NONE',  ( -0.2387587925603975592, -3.020022701398815013, 32.48759521482552515 ) ) ;
#77443=CARTESIAN_POINT ( 'NONE',  ( -5.869208192175213945, -2.729792928343270919, 31.24908615093345077 ) ) ;
#77444=AXIS2_PLACEMENT_3D ( 'NONE', #33739, #54444, #12583 ) ;
#77445=CARTESIAN_POINT ( 'NONE',  ( -11.28840722682322628, -3.136992222400443175, 32.19305428654138979 ) ) ;
#77446=CARTESIAN_POINT ( 'NONE',  ( -16.37733107841048863, -2.612411019501189813, 31.66733052389439962 ) ) ;
#77447=ORIENTED_EDGE ( 'NONE', *, *, #21717, .T. ) ;
#77448=CARTESIAN_POINT ( 'NONE',  ( -5.749945688361685292, -11.79725096376909299, 32.30694842903960762 ) ) ;
#77449=ORIENTED_EDGE ( 'NONE', *, *, #65466, .T. ) ;
#77450=EDGE_CURVE ( 'NONE', #26582, #48512, #45230, .T. ) ;
#77451=ORIENTED_EDGE ( 'NONE', *, *, #67055, .F. ) ;
#77452=VECTOR ( 'NONE', #71427, 1000.000000000000000 ) ;
#77453=CARTESIAN_POINT ( 'NONE',  ( 14.37294787896833625, -3.835265460703683349, 33.15142922261929925 ) ) ;
#77454=CARTESIAN_POINT ( 'NONE',  ( 15.16468581981335007, -12.10708131394839349, 31.69288490824020244 ) ) ;
#77455=EDGE_CURVE ( 'NONE', #58277, #83191, #86245, .T. ) ;
#77456=AXIS2_PLACEMENT_3D ( 'NONE', #2466, #29958, #57416 ) ;
#77457=CARTESIAN_POINT ( 'NONE',  ( -5.869474298236438514, -6.852161475712352789, 34.70806712695775786 ) ) ;
#77458=CARTESIAN_POINT ( 'NONE',  ( 7.846153846153846700, -3.322132147404559976, 32.92929555188717927 ) ) ;
#77459=CARTESIAN_POINT ( 'NONE',  ( 1.384615384615386802, -10.67929555188718282, 33.92786785259544047 ) ) ;
#77460=CARTESIAN_POINT ( 'NONE',  ( 14.30769230769231015, -11.35647404775217417, 33.31231777344666511 ) ) ;
#77461=ORIENTED_EDGE ( 'NONE', *, *, #77768, .F. ) ;
#77462=CARTESIAN_POINT ( 'NONE',  ( -18.24997673094235395, -5.728515186090276323, 34.42611988154120439 ) ) ;
#77464=DIRECTION ( 'NONE',  ( -0.000000000000000000, 0.9396926207859092051, -0.3420201433256662704 ) ) ;
#77465=CARTESIAN_POINT ( 'NONE',  ( -10.61538461538461320, -9.780366693483667717, 34.19971097300155094 ) ) ;
#77466=CARTESIAN_POINT ( 'NONE',  ( -0.4615384615384611200, -12.29105614889573062, 35.45975837776705220 ) ) ;
#77469=EDGE_LOOP ( 'NONE', ( #56685, #9742 ) ) ;
#77471=CARTESIAN_POINT ( 'NONE',  ( -6.066082379360133281, -3.937682226553329556, 33.60647404775217240 ) ) ;
#77472=ORIENTED_EDGE ( 'NONE', *, *, #47490, .T. ) ;
#77473=CARTESIAN_POINT ( 'NONE',  ( -10.61538461538461320, -12.78798330534102945, 29.74999999999997868 ) ) ;
#77474=CARTESIAN_POINT ( 'NONE',  ( -1.318548051265308496, -9.905515769479277921, 34.41647553114623292 ) ) ;
#77475=CARTESIAN_POINT ( 'NONE',  ( 14.08420738312797837, -10.23692288466677880, 34.23039457007281072 ) ) ;
#77476=CARTESIAN_POINT ( 'NONE',  ( -7.846153846153965716, -5.219633306517616589, 34.19971097300220464 ) ) ;
#77478=CARTESIAN_POINT ( 'NONE',  ( 13.38461538461538680, -12.29105614889573062, 35.45975837776705220 ) ) ;
#77479=ORIENTED_EDGE ( 'NONE', *, *, #82274, .F. ) ;
#77480=LINE ( 'NONE', #22536, #41524 ) ;
#77481=LINE ( 'NONE', #86016, #28096 ) ;
#77483=CARTESIAN_POINT ( 'NONE',  ( -8.519230769229348965, -7.500000000000154543, 35.00000000000007105 ) ) ;
#77484=CARTESIAN_POINT ( 'NONE',  ( 17.07692307692295586, -3.835265460704628815, 33.15142922262033665 ) ) ;
#77485=CARTESIAN_POINT ( 'NONE',  ( -3.480745961711584791, -4.943428324936578910, 34.04746400365624481 ) ) ;
#77486=DIRECTION ( 'NONE',  ( -0.000000000000000000, 0.1736481776669307198, -0.9848077530122080203 ) ) ;
#77487=DIRECTION ( 'NONE',  ( 0.000000000000000000, 0.4999999999999985567, 0.8660254037844395958 ) ) ;
#77488=CARTESIAN_POINT ( 'NONE',  ( -11.47239420511146513, -2.833524468853757305, 32.15551576947925838 ) ) ;
#77490=ORIENTED_EDGE ( 'NONE', *, *, #64204, .T. ) ;
#77491=B_SPLINE_CURVE_WITH_KNOTS ( 'NONE', 3,
 ( #60925, #55496, #88869, #117, #82978, #1004, #41999, #7763, #35226, #41107 ),
 .UNSPECIFIED., .F., .F.,
 ( 4, 2, 2, 2, 4 ),
 ( 0.000000000000000000, 0.0001954311564186862781, 0.0003908623128373725562, 0.0005862934692560588072, 0.0007817246256747451124 ),
 .UNSPECIFIED. ) ;
#77492=CARTESIAN_POINT ( 'NONE',  ( -15.23076923076922995, -6.343179335718451384, 34.87096338111211935 ) ) ;
#77493=DIRECTION ( 'NONE',  ( -1.000000000000000000, 0.000000000000000000, 0.000000000000000000 ) ) ;
#77495=CARTESIAN_POINT ( 'NONE',  ( -15.90379173393269596, -11.47946981652013498, 33.17500667209846910 ) ) ;
#77496=DIRECTION ( 'NONE',  ( -0.000000000000000000, -0.3420201433256695456, -0.9396926207859082059 ) ) ;
#77497=VERTEX_POINT ( 'NONE', #11458 ) ;
#77501=B_SPLINE_CURVE_WITH_KNOTS ( 'NONE', 3,
 ( #46999, #6907, #33507, #62288, #12343, #60523, #33939, #74487, #53316, #75809 ),
 .UNSPECIFIED., .F., .F.,
 ( 4, 2, 2, 2, 4 ),
 ( 0.0007817246256747470640, 0.0009771112852218898515, 0.001172497944769032747, 0.001367884604316175643, 0.001563271263863318539 ),
 .UNSPECIFIED. ) ;
#77502=ORIENTED_EDGE ( 'NONE', *, *, #28431, .T. ) ;
#77503=CARTESIAN_POINT ( 'NONE',  ( -0.4615384615384611200, -10.67929555188718282, 33.92786785259544047 ) ) ;
#77504=EDGE_CURVE ( 'NONE', #36033, #15004, #38489, .T. ) ;
#77505=ORIENTED_EDGE ( 'NONE', *, *, #84082, .F. ) ;
#77506=CARTESIAN_POINT ( 'NONE',  ( 18.00000000000000000, -6.386643153685126251, 34.62446782046654192 ) ) ;
#77507=DIRECTION ( 'NONE',  ( -0.000000000000000000, 0.1736481776669307198, -0.9848077530122080203 ) ) ;
#77508=CARTESIAN_POINT ( 'NONE',  ( -12.46153846153846168, -9.905515769479276145, 34.41647553114623292 ) ) ;
#77509=CARTESIAN_POINT ( 'NONE',  ( -5.999999999999998224, -6.343179335718451384, 34.87096338111211935 ) ) ;
#77510=ORIENTED_EDGE ( 'NONE', *, *, #32084, .F. ) ;
#77511=EDGE_CURVE ( 'NONE', #26741, #18183, #29982, .T. ) ;
#77512=CARTESIAN_POINT ( 'NONE',  ( -6.792286482109971324, -6.369690395747422684, 34.87708834333098196 ) ) ;
#77513=EDGE_LOOP ( 'NONE', ( #49816, #51711, #77407, #8323 ) ) ;
#77514=VECTOR ( 'NONE', #59246, 1000.000000000000000 ) ;
#77515=CARTESIAN_POINT ( 'NONE',  ( 12.39626846098214230, -12.16647553114622049, 32.15551576947930812 ) ) ;
#77516=CARTESIAN_POINT ( 'NONE',  ( 11.53846153846153832, -13.04860791097971706, 34.73218667398347037 ) ) ;
#77517=ORIENTED_EDGE ( 'NONE', *, *, #58722, .T. ) ;
#77518=CARTESIAN_POINT ( 'NONE',  ( 8.638540166120458608, -4.684245665217972032, 34.18127051446801090 ) ) ;
#77519=CARTESIAN_POINT ( 'NONE',  ( 10.86543892702293057, -3.136992222400443175, 32.19305428654138979 ) ) ;
#77522=EDGE_CURVE ( 'NONE', #29486, #79207, #3167, .T. ) ;
#77523=VECTOR ( 'NONE', #46804, 1000.000000000000114 ) ;
#77524=FACE_OUTER_BOUND ( 'NONE', #62035, .T. ) ;
#77525=DIRECTION ( 'NONE',  ( -0.000000000000000000, -0.9848077530122085754, -0.1736481776669273613 ) ) ;
#77526=ORIENTED_EDGE ( 'NONE', *, *, #1788, .F. ) ;
#77527=ORIENTED_EDGE ( 'NONE', *, *, #81845, .T. ) ;
#77528=B_SPLINE_CURVE_WITH_KNOTS ( 'NONE', 3,
 ( #38604, #16113, #10247, #9365, #71936, #11126, #86818, #30508, #51641, #57976 ),
 .UNSPECIFIED., .F., .F.,
 ( 4, 2, 2, 2, 4 ),
 ( 0.000000000000000000, 0.0001954311564186875792, 0.0003908623128373751583, 0.0005862934692560627103, 0.0007817246256747503166 ),
 .UNSPECIFIED. ) ;
#77529=FACE_BOUND ( 'NONE', #46952, .T. ) ;
#77530=EDGE_LOOP ( 'NONE', ( #72239, #39304, #47327, #35642, #16384, #926 ) ) ;
#77531=CARTESIAN_POINT ( 'NONE',  ( 15.00784301325308157, -12.39988816332205701, 30.74660775122750778 ) ) ;
#77532=B_SPLINE_CURVE_WITH_KNOTS ( 'NONE', 3,
 ( #4014, #31044, #16215, #3129, #51289, #17997, #58511, #17096, #85123, #22966 ),
 .UNSPECIFIED., .F., .F.,
 ( 4, 2, 2, 2, 4 ),
 ( 0.0007817246256747476061, 0.0009771112852218896347, 0.001172497944769031880, 0.001367884604316173909, 0.001563271263863315937 ),
 .UNSPECIFIED. ) ;
#77533=ADVANCED_FACE ( 'NONE', ( #71812 ), #73162, .F. ) ;
#77535=EDGE_CURVE ( 'NONE', #65895, #29819, #33162, .T. ) ;
#77536=CARTESIAN_POINT ( 'NONE',  ( 17.86985203026830504, -5.915902021225892149, 34.75552854090298638 ) ) ;
#77537=CARTESIAN_POINT ( 'NONE',  ( -16.15384615384627409, -2.892918686052165622, 31.69288490824153470 ) ) ;
#77538=VERTEX_POINT ( 'NONE', #26304 ) ;
#77539=ORIENTED_EDGE ( 'NONE', *, *, #74618, .F. ) ;
#77542=EDGE_CURVE ( 'NONE', #12672, #57246, #88918, .T. ) ;
#77543=FACE_OUTER_BOUND ( 'NONE', #25188, .T. ) ;
#77544=AXIS2_PLACEMENT_3D ( 'NONE', #25700, #18945, #73895 ) ;
#77545=CARTESIAN_POINT ( 'NONE',  ( 14.17754433796061697, -12.15440758774515473, 32.17923288041532004 ) ) ;
#77546=CARTESIAN_POINT ( 'NONE',  ( -18.00000000000000000, -6.343179335718452272, 34.87096338111211935 ) ) ;
#77547=EDGE_LOOP ( 'NONE', ( #68794, #62325 ) ) ;
#77548=CARTESIAN_POINT ( 'NONE',  ( 13.38461538461526601, -10.90142922262034020, 33.41473453929536674 ) ) ;
#77549=CARTESIAN_POINT ( 'NONE',  ( -15.16551409125639260, -3.643525952247864463, 33.31231777344670064 ) ) ;
#77550=CARTESIAN_POINT ( 'NONE',  ( 16.15384615384615330, -5.471508081941601098, 34.59228464037088457 ) ) ;
#77551=CARTESIAN_POINT ( 'NONE',  ( 8.834485908743603844, -6.835583212224610072, 34.95778746994559327 ) ) ;
#77552=EDGE_LOOP ( 'NONE', ( #71539, #72438, #28444, #83560 ) ) ;
#77553=ORIENTED_EDGE ( 'NONE', *, *, #86524, .F. ) ;
#77554=EDGE_CURVE ( 'NONE', #22118, #33835, #35403, .T. ) ;
#77555=B_SPLINE_CURVE_WITH_KNOTS ( 'NONE', 3,
 ( #1136, #57403, #70035, #22730, #21409, #78122, #84016, #69593, #29069, #56958 ),
 .UNSPECIFIED., .F., .F.,
 ( 4, 2, 2, 2, 4 ),
 ( 0.000000000000000000, 0.0001954339857564064444, 0.0003908679715128128888, 0.0005863019572692193060, 0.0007817359430256257775 ),
 .UNSPECIFIED. ) ;
#77556=ORIENTED_EDGE ( 'NONE', *, *, #69341, .F. ) ;
#77557=CARTESIAN_POINT ( 'NONE',  ( 12.39545505058258179, -6.386643153685125363, 34.62446782046654903 ) ) ;
#77558=CARTESIAN_POINT ( 'NONE',  ( -9.627052552794856055, -8.656820664281605460, 34.87096338111211224 ) ) ;
#77559=B_SPLINE_CURVE_WITH_KNOTS ( 'NONE', 3,
 ( #63093, #22126, #1850, #17129, #36093, #78830 ),
 .UNSPECIFIED., .F., .F.,
 ( 4, 2, 4 ),
 ( 0.0003909569690057842790, 0.0005862646681846108007, 0.0007815723673634373224 ),
 .UNSPECIFIED. ) ;
#77560=CARTESIAN_POINT ( 'NONE',  ( 11.47319153790521717, -2.379036618887870436, 30.90682066428147934 ) ) ;
#77561=CARTESIAN_POINT ( 'NONE',  ( -2.057637887778851926, -2.544122305571458575, 31.48381861865057729 ) ) ;
#77562=EDGE_CURVE ( 'NONE', #13779, #798, #9544, .T. ) ;
#77563=FACE_BOUND ( 'NONE', #86678, .T. ) ;
#77564=CARTESIAN_POINT ( 'NONE',  ( -11.60373153901785948, -2.379036618887870436, 30.90682066428147934 ) ) ;
#77566=ORIENTED_EDGE ( 'NONE', *, *, #69781, .T. ) ;
#77568=DIRECTION ( 'NONE',  ( -0.000000000000000000, -0.7660444431189791237, -0.6427876096865379196 ) ) ;
#77569=CARTESIAN_POINT ( 'NONE',  ( 11.78846153846160227, -7.434744429011176159, 34.75000000000000711 ) ) ;
#77571=ORIENTED_EDGE ( 'NONE', *, *, #38932, .T. ) ;
#77572=EDGE_CURVE ( 'NONE', #6788, #61316, #55840, .T. ) ;
#77573=CARTESIAN_POINT ( 'NONE',  ( 4.826946332874485712, -12.65889640711025521, 30.72598325615533454 ) ) ;
#77576=FACE_BOUND ( 'NONE', #55348, .T. ) ;
#77577=CYLINDRICAL_SURFACE ( 'NONE', #70554, 0.2500000000000008882 ) ;
#77578=VECTOR ( 'NONE', #79076, 1000.000000000000114 ) ;
#77579=CARTESIAN_POINT ( 'NONE',  ( 16.82689983963011215, -11.86270091957321071, 32.19358267280088626 ) ) ;
#77580=CARTESIAN_POINT ( 'NONE',  ( 12.46153846153846168, -12.10708131394839349, 31.69288490824020244 ) ) ;
#77581=VERTEX_POINT ( 'NONE', #5146 ) ;
#77582=CARTESIAN_POINT ( 'NONE',  ( 0.3962680155776849289, -10.90142922261923886, 33.41473453929638993 ) ) ;
#77583=CARTESIAN_POINT ( 'NONE',  ( 5.207761494935837732, -7.277220443632450575, 34.74524770363009196 ) ) ;
#77584=CARTESIAN_POINT ( 'NONE',  ( -9.822999158975251888, -3.062553014421049546, 32.05460306192773601 ) ) ;
#77585=FACE_OUTER_BOUND ( 'NONE', #22260, .T. ) ;
#77586=VERTEX_POINT ( 'NONE', #75380 ) ;
#77587=AXIS2_PLACEMENT_3D ( 'NONE', #20175, #48511, #75124 ) ;
#77588=CARTESIAN_POINT ( 'NONE',  ( -7.846153846153844924, -2.833524468853757305, 32.15551576947925838 ) ) ;
#77589=EDGE_LOOP ( 'NONE', ( #78201, #777, #48057, #208 ) ) ;
#77590=VECTOR ( 'NONE', #5510, 1000.000000000000000 ) ;
#77592=VERTEX_POINT ( 'NONE', #26745 ) ;
#77593=CARTESIAN_POINT ( 'NONE',  ( 11.66925334628632882, -6.413143153341454017, 34.63066358083362672 ) ) ;
#77594=CARTESIAN_POINT ( 'NONE',  ( -1.607542343522232242, -12.38737895849757820, 31.66785238281580206 ) ) ;
#77595=CYLINDRICAL_SURFACE ( 'NONE', #50052, 0.2499999999999998890 ) ;
#77596=DIRECTION ( 'NONE',  ( 0.000000000000000000, 0.9396926207859126468, -0.3420201433256571111 ) ) ;
#77598=CARTESIAN_POINT ( 'NONE',  ( 0.2115384615384615363, -7.566083408709834757, 34.74999999999999289 ) ) ;
#77599=CARTESIAN_POINT ( 'NONE',  ( 4.153846153846154188, -5.180354513474913603, 36.12317359536750416 ) ) ;
#77601=ORIENTED_EDGE ( 'NONE', *, *, #76838, .F. ) ;
#77602=FACE_OUTER_BOUND ( 'NONE', #34215, .T. ) ;
#77603=CARTESIAN_POINT ( 'NONE',  ( 13.25414019953966971, -7.276987145209184327, 34.99546412871779211 ) ) ;
#77605=B_SPLINE_CURVE_WITH_KNOTS ( 'NONE', 3,
 ( #52082, #71032, #57516, #23283, #88129, #72799, #39039, #61064, #52968, #46667 ),
 .UNSPECIFIED., .F., .F.,
 ( 4, 2, 2, 2, 4 ),
 ( 0.000000000000000000, 0.0001954311564186879315, 0.0003908623128373758630, 0.0005862934692560637946, 0.0007817246256747517261 ),
 .UNSPECIFIED. ) ;
#77606=EDGE_LOOP ( 'NONE', ( #80205, #81246, #30777, #67222 ) ) ;
#77607=ORIENTED_EDGE ( 'NONE', *, *, #10167, .F. ) ;
#77608=DIRECTION ( 'NONE',  ( -0.000000000000000000, -0.000000000000000000, -1.000000000000000000 ) ) ;
#77609=CARTESIAN_POINT ( 'NONE',  ( 3.230769230769231726, -9.780366693483667717, 34.19971097300155094 ) ) ;
#77611=CARTESIAN_POINT ( 'NONE',  ( -5.011667505647053211, -3.835265460703683349, 33.15142922261929925 ) ) ;
#77612=CARTESIAN_POINT ( 'NONE',  ( 12.21156173059610595, -10.66389620160130036, 33.62221079203477103 ) ) ;
#77613=CARTESIAN_POINT ( 'NONE',  ( -8.834500769787089425, -3.083524468853724443, 32.58852847137143272 ) ) ;
#77614=PLANE ( 'NONE',  #81062 ) ;
#77615=B_SPLINE_CURVE_WITH_KNOTS ( 'NONE', 3,
 ( #41357, #83233, #69708, #7573, #56639, #84131, #83688, #15659, #48098, #43130 ),
 .UNSPECIFIED., .F., .F.,
 ( 4, 2, 2, 2, 4 ),
 ( 0.000000000000000000, 0.0001954311564186879044, 0.0003908623128373758088, 0.0005862934692560636861, 0.0007817246256747516176 ),
 .UNSPECIFIED. ) ;
#77616=CARTESIAN_POINT ( 'NONE',  ( -3.931066612577743147, -5.913360116392399668, 34.49180327182771322 ) ) ;
#77617=CARTESIAN_POINT ( 'NONE',  ( -17.20761454359064047, -12.11776431015576172, 31.66791131148498906 ) ) ;
#77618=CARTESIAN_POINT ( 'NONE',  ( 12.39545505058257824, -11.69971097300155272, 32.46337939537587403 ) ) ;
#77620=CARTESIAN_POINT ( 'NONE',  ( 7.596177102105253987, -2.318417181685854533, 30.59732222474233865 ) ) ;
#77621=ORIENTED_EDGE ( 'NONE', *, *, #28763, .T. ) ;
#77622=CARTESIAN_POINT ( 'NONE',  ( 15.16468581981335184, -11.16473453929635440, 33.15142922261925662 ) ) ;
#77624=CARTESIAN_POINT ( 'NONE',  ( 11.60452988946397923, -9.780366693483667717, 34.19971097300155805 ) ) ;
#77625=FACE_OUTER_BOUND ( 'NONE', #39781, .T. ) ;
#77626=VERTEX_POINT ( 'NONE', #81701 ) ;
#77627=CARTESIAN_POINT ( 'NONE',  ( 9.942253101685738059, -11.56426240980093745, 33.07394671870546432 ) ) ;
#77628=B_SPLINE_CURVE_WITH_KNOTS ( 'NONE', 3,
 ( #57059, #84988, #50729, #43544, #78215, #85869, #16517, #16965, #44413, #43983 ),
 .UNSPECIFIED., .F., .F.,
 ( 4, 2, 2, 2, 4 ),
 ( 0.0007817246256747493408, 0.0009771112852218920199, 0.001172497944769034699, 0.001367884604316177378, 0.001563271263863320057 ),
 .UNSPECIFIED. ) ;
#77629=CARTESIAN_POINT ( 'NONE',  ( 9.561617089197383734, -2.845849958028613624, 32.17971566917920967 ) ) ;
#77630=DIRECTION ( 'NONE',  ( -0.000000000000000000, 1.000000000000000000, 3.491481338843133355E-15 ) ) ;
#77631=ORIENTED_EDGE ( 'NONE', *, *, #11838, .T. ) ;
#77632=CARTESIAN_POINT ( 'NONE',  ( -10.86538461538461320, -2.499999999999998668, 29.75000000000000355 ) ) ;
#77633=ORIENTED_EDGE ( 'NONE', *, *, #89047, .F. ) ;
#77634=CARTESIAN_POINT ( 'NONE',  ( 16.21991348719623360, -9.058645607665452459, 34.76329471203371924 ) ) ;
#77635=EDGE_CURVE ( 'NONE', #14097, #1750, #41784, .T. ) ;
#77637=CYLINDRICAL_SURFACE ( 'NONE', #87353, 0.2499999999999986955 ) ;
#77638=CARTESIAN_POINT ( 'NONE',  ( -8.096130590202433197, -2.544273027872575366, 31.48422191005632342 ) ) ;
#77639=CARTESIAN_POINT ( 'NONE',  ( 1.318533005255250856, -8.164416787775445883, 34.95778746994557906 ) ) ;
#77640=CARTESIAN_POINT ( 'NONE',  ( 18.22301284409340028, -8.282913670948747864, 34.94150082978203642 ) ) ;
#77641=VECTOR ( 'NONE', #34895, 1000.000000000000227 ) ;
#77642=EDGE_LOOP ( 'NONE', ( #18230, #31560 ) ) ;
#77644=ORIENTED_EDGE ( 'NONE', *, *, #22904, .F. ) ;
#77645=EDGE_LOOP ( 'NONE', ( #74464, #70104 ) ) ;
#77646=EDGE_CURVE ( 'NONE', #54695, #18976, #13852, .T. ) ;
#77647=CARTESIAN_POINT ( 'NONE',  ( 6.923076923076924238, -10.05456864172156806, 36.03766855953608683 ) ) ;
#77648=CARTESIAN_POINT ( 'NONE',  ( -17.01166750564705410, -3.835265460703683349, 33.15142922261929925 ) ) ;
#77649=CARTESIAN_POINT ( 'NONE',  ( -4.403822897894743349, -12.41104346484419452, 31.60698883733904196 ) ) ;
#77651=CARTESIAN_POINT ( 'NONE',  ( -7.715628407920200438, -4.299079248970732792, 33.91157788607253565 ) ) ;
#77652=CARTESIAN_POINT ( 'NONE',  ( 5.142178648199099200, -10.21337939537593620, 33.94971097300152252 ) ) ;
#77653=VERTEX_POINT ( 'NONE', #60528 ) ;
#77654=ORIENTED_EDGE ( 'NONE', *, *, #21337, .F. ) ;
#77655=ORIENTED_EDGE ( 'NONE', *, *, #32021, .F. ) ;
#77656=CARTESIAN_POINT ( 'NONE',  ( 4.403791563224197070, -4.176053281294514363, 33.81426240980091791 ) ) ;
#77657=ORIENTED_EDGE ( 'NONE', *, *, #82442, .F. ) ;
#77658=CARTESIAN_POINT ( 'NONE',  ( 0.5923302693632471749, -8.147973898785416225, 34.70805048591653730 ) ) ;
#77659=CARTESIAN_POINT ( 'NONE',  ( 14.37375964104238513, -4.661471528628508665, 34.16647553114624003 ) ) ;
#77660=EDGE_CURVE ( 'NONE', #79299, #13992, #53771, .T. ) ;
#77662=ADVANCED_FACE ( 'NONE', ( #6043 ), #42046, .F. ) ;
#77663=VERTEX_POINT ( 'NONE', #36608 ) ;
#77664=VECTOR ( 'NONE', #79704, 1000.000000000000114 ) ;
#77665=ORIENTED_EDGE ( 'NONE', *, *, #5164, .T. ) ;
#77666=CARTESIAN_POINT ( 'NONE',  ( -17.77722033102192967, -3.020022701398814124, 32.48759521482552515 ) ) ;
#77667=VERTEX_POINT ( 'NONE', #48785 ) ;
#77668=FACE_BOUND ( 'NONE', #32453, .T. ) ;
#77669=CARTESIAN_POINT ( 'NONE',  ( -6.250023237292964495, -9.271318131107980420, 34.42618302367067429 ) ) ;
#77673=CARTESIAN_POINT ( 'NONE',  ( -15.16551365949320562, -5.219633306516380244, 34.19971097300157936 ) ) ;
#77674=CARTESIAN_POINT ( 'NONE',  ( 1.384615384615386802, -2.249999999999998668, 29.75000000000001776 ) ) ;
#77675=CARTESIAN_POINT ( 'NONE',  ( -4.153846153846152411, -12.09954503811598769, 35.62045528018868623 ) ) ;
#77676=ADVANCED_FACE ( 'NONE', ( #50550 ), #21759, .F. ) ;
#77677=CARTESIAN_POINT ( 'NONE',  ( -11.78843826940389050, -5.728515186090277211, 34.42611988154120439 ) ) ;
#77678=CARTESIAN_POINT ( 'NONE',  ( -13.38461538461538325, -11.69971097300155272, 32.46337939537588113 ) ) ;
#77679=CARTESIAN_POINT ( 'NONE',  ( 6.923076923076800782, -2.657715359629662988, 31.77849191805970364 ) ) ;
#77680=CARTESIAN_POINT ( 'NONE',  ( -7.846153846153844924, -6.386643153685126251, 34.62446782046654192 ) ) ;
#77681=CARTESIAN_POINT ( 'NONE',  ( -6.066083410955878108, -5.557115091759785130, 34.35708131394839171 ) ) ;
#77683=CYLINDRICAL_SURFACE ( 'NONE', #34415, 0.2499999999999995559 ) ;
#77684=FACE_BOUND ( 'NONE', #1558, .T. ) ;
#77685=CARTESIAN_POINT ( 'NONE',  ( 17.14217864819909920, -3.835265460703683349, 33.15142922261929925 ) ) ;
#77686=CARTESIAN_POINT ( 'NONE',  ( 6.989145274079362480, -3.050289026998446840, 32.03036669348366416 ) ) ;
#77687=B_SPLINE_CURVE_WITH_KNOTS ( 'NONE', 3,
 ( #32364, #79218, #59385, #52621, #80104, #39130, #39582, #46316, #44968, #38224 ),
 .UNSPECIFIED., .F., .F.,
 ( 4, 2, 2, 2, 4 ),
 ( 0.000000000000000000, 0.0001954311564186865221, 0.0003908623128373730441, 0.0005862934692560595662, 0.0007817246256747460882 ),
 .UNSPECIFIED. ) ;
#77689=FACE_OUTER_BOUND ( 'NONE', #15445, .T. ) ;
#77691=CARTESIAN_POINT ( 'NONE',  ( 6.000000000000001776, -10.51840700105979565, 33.73612834413961536 ) ) ;
#77692=FACE_OUTER_BOUND ( 'NONE', #32124, .T. ) ;
#77693=B_SPLINE_CURVE_WITH_KNOTS ( 'NONE', 3,
 ( #28370, #36030, #9432, #55843, #42787, #84665, #77446, #63483, #57173, #83330 ),
 .UNSPECIFIED., .F., .F.,
 ( 4, 2, 2, 2, 4 ),
 ( 0.000000000000000000, 0.0001954311564186867389, 0.0003908623128373734778, 0.0005862934692560602167, 0.0007817246256747469556 ),
 .UNSPECIFIED. ) ;
#77695=VERTEX_POINT ( 'NONE', #16335 ) ;
#77696=B_SPLINE_CURVE_WITH_KNOTS ( 'NONE', 3,
 ( #14348, #37608, #83713, #69302, #65071, #10593, #58319, #51541, #836, #8042 ),
 .UNSPECIFIED., .F., .F.,
 ( 4, 2, 2, 2, 4 ),
 ( 0.000000000000000000, 0.0001954311564186876876, 0.0003908623128373753751, 0.0005862934692560630356, 0.0007817246256747507503 ),
 .UNSPECIFIED. ) ;
#77698=ORIENTED_EDGE ( 'NONE', *, *, #52203, .T. ) ;
#77699=AXIS2_PLACEMENT_3D ( 'NONE', #65072, #50670, #63750 ) ;
#77700=VECTOR ( 'NONE', #46102, 1000.000000000000114 ) ;
#77701=CARTESIAN_POINT ( 'NONE',  ( -9.019230769230768274, -2.499999999999998668, 29.75000000000000355 ) ) ;
#77702=ORIENTED_EDGE ( 'NONE', *, *, #86764, .F. ) ;
#77703=CARTESIAN_POINT ( 'NONE',  ( -3.903900635498010807, -11.37275283266503756, 32.91324779482534524 ) ) ;
#77704=VERTEX_POINT ( 'NONE', #56437 ) ;
#77705=CARTESIAN_POINT ( 'NONE',  ( 5.750023255951410839, -10.82459398097509684, 33.81372124010185587 ) ) ;
#77707=CARTESIAN_POINT ( 'NONE',  ( -17.74994558008654622, -9.233818618650598609, 34.70587769442853698 ) ) ;
#77709=CARTESIAN_POINT ( 'NONE',  ( -5.750054481651858396, -9.272278438253401589, 34.42582936511637826 ) ) ;
#77710=CARTESIAN_POINT ( 'NONE',  ( 7.053602624840488389, -9.417988943895561960, 34.36773134775778260 ) ) ;
#77711=LINE ( 'NONE', #16018, #46078 ) ;
#77713=CARTESIAN_POINT ( 'NONE',  ( 4.853996859406927378, -8.239355502252617924, 34.69524867566427417 ) ) ;
#77716=CARTESIAN_POINT ( 'NONE',  ( 1.161689167099239306, -2.758268499246656624, 31.33685645148948140 ) ) ;
#77717=CARTESIAN_POINT ( 'NONE',  ( 14.43848411551709177, -10.54018710029568595, 33.71981072465678864 ) ) ;
#77718=CARTESIAN_POINT ( 'NONE',  ( -2.373775718648186928, -4.098570777380720287, 33.41473453929634729 ) ) ;
#77720=FACE_OUTER_BOUND ( 'NONE', #48852, .T. ) ;
#77721=ORIENTED_EDGE ( 'NONE', *, *, #20498, .F. ) ;
#77722=DIRECTION ( 'NONE',  ( -0.000000000000000000, 1.000000000000000000, 3.491481338843133355E-15 ) ) ;
#77723=DIRECTION ( 'NONE',  ( 0.000000000000000000, 0.9396926207859126468, 0.3420201433256571111 ) ) ;
#77724=CARTESIAN_POINT ( 'NONE',  ( 9.692307692307695177, -6.386643153685126251, 34.62446782046654192 ) ) ;
#77725=CARTESIAN_POINT ( 'NONE',  ( 16.28389358909660345, -7.723484941389743952, 34.99544897038808955 ) ) ;
#77726=DIRECTION ( 'NONE',  ( -0.000000000000000000, 0.6427876096865404731, -0.7660444431189771253 ) ) ;
#77727=EDGE_CURVE ( 'NONE', #38500, #27545, #78292, .T. ) ;
#77728=LINE ( 'NONE', #72303, #48618 ) ;
#77729=B_SPLINE_CURVE_WITH_KNOTS ( 'NONE', 3,
 ( #34112, #13840, #40448, #1209, #69233, #61579, #81872, #61134, #7535, #7976 ),
 .UNSPECIFIED., .F., .F.,
 ( 4, 2, 2, 2, 4 ),
 ( 0.000000000000000000, 0.0001954311564186862781, 0.0003908623128373725562, 0.0005862934692560588072, 0.0007817246256747451124 ),
 .UNSPECIFIED. ) ;
#77730=DIRECTION ( 'NONE',  ( -0.000000000000000000, -0.5000000000000009992, -0.8660254037844380415 ) ) ;
#77731=B_SPLINE_CURVE_WITH_KNOTS ( 'NONE', 3,
 ( #53889, #33623, #81375, #12900, #88593, #81818 ),
 .UNSPECIFIED., .F., .F.,
 ( 4, 2, 4 ),
 ( 0.000000000000000000, 0.0001954784845028888327, 0.0003909569690057776653 ),
 .UNSPECIFIED. ) ;
#77733=ORIENTED_EDGE ( 'NONE', *, *, #75722, .T. ) ;
#77735=ORIENTED_EDGE ( 'NONE', *, *, #50814, .T. ) ;
#77736=EDGE_CURVE ( 'NONE', #48033, #70194, #51475, .T. ) ;
#77737=CARTESIAN_POINT ( 'NONE',  ( -6.000000000000121680, -12.70778746994576025, 30.41441678777401236 ) ) ;
#77738=CARTESIAN_POINT ( 'NONE',  ( -3.930834802233304170, -3.105924265160262543, 32.13625925475356127 ) ) ;
#77739=DIRECTION ( 'NONE',  ( -0.000000000000000000, -0.9396926207859092051, -0.3420201433256662704 ) ) ;
#77740=EDGE_CURVE ( 'NONE', #45665, #20258, #44945, .T. ) ;
#77741=CARTESIAN_POINT ( 'NONE',  ( -13.13456107297706588, -9.148310452688876993, 34.47095581063188519 ) ) ;
#77742=FACE_OUTER_BOUND ( 'NONE', #53359, .T. ) ;
#77743=EDGE_LOOP ( 'NONE', ( #39861, #13681 ) ) ;
#77744=CARTESIAN_POINT ( 'NONE',  ( -17.32694631421604115, -4.335965774309648246, 33.62209801155881905 ) ) ;
#77745=ORIENTED_EDGE ( 'NONE', *, *, #14784, .F. ) ;
#77746=ORIENTED_EDGE ( 'NONE', *, *, #63582, .F. ) ;
#77748=EDGE_CURVE ( 'NONE', #12325, #56029, #84814, .T. ) ;
#77749=CARTESIAN_POINT ( 'NONE',  ( 8.769230769230768274, -12.34228464037088635, 31.77849191805839268 ) ) ;
#77750=CARTESIAN_POINT ( 'NONE',  ( 8.519207531937800226, -2.823816976329317274, 31.52131813110795733 ) ) ;
#77753=AXIS2_PLACEMENT_3D ( 'NONE', #1348, #49091, #28837 ) ;
#77754=EDGE_CURVE ( 'NONE', #4010, #55482, #7808, .T. ) ;
#77755=CARTESIAN_POINT ( 'NONE',  ( 0.4615384615383382183, -11.67786785259630911, 32.92929555188603530 ) ) ;
#77760=VERTEX_POINT ( 'NONE', #15012 ) ;
#77761=CARTESIAN_POINT ( 'NONE',  ( 1.134592147322421418, -8.432397168068783699, 34.66272746175022945 ) ) ;
#77762=EDGE_LOOP ( 'NONE', ( #29375, #21013, #25723, #43720 ) ) ;
#77764=CARTESIAN_POINT ( 'NONE',  ( 6.065255571276025215, -12.46129190930001052, 30.37095296980870174 ) ) ;
#77765=CARTESIAN_POINT ( 'NONE',  ( 2.438217745925954194, -9.503571793651733657, 34.60286762892837942 ) ) ;
#77766=ADVANCED_FACE ( 'NONE', ( #35732 ), #63630, .F. ) ;
#77767=ORIENTED_EDGE ( 'NONE', *, *, #50429, .T. ) ;
#77768=EDGE_CURVE ( 'NONE', #83601, #83807, #1496, .T. ) ;
#77769=CARTESIAN_POINT ( 'NONE',  ( 15.23076923076923173, -10.51840700105979565, 33.73612834413961536 ) ) ;
#77770=CARTESIAN_POINT ( 'NONE',  ( 14.30769230769231015, -2.292212530054420494, 30.41441678777542634 ) ) ;
#77772=FACE_BOUND ( 'NONE', #73527, .T. ) ;
#77773=CARTESIAN_POINT ( 'NONE',  ( -11.60373153901786125, -11.67786785259540849, 32.92929555188721480 ) ) ;
#77775=CARTESIAN_POINT ( 'NONE',  ( 2.057669083470850424, -12.45566812827425096, 31.48439005359158926 ) ) ;
#77776=CARTESIAN_POINT ( 'NONE',  ( -0.3310130233048187987, -11.66157788607254275, 32.95092075102925833 ) ) ;
#77777=FACE_OUTER_BOUND ( 'NONE', #63118, .T. ) ;
#77778=ADVANCED_FACE ( 'NONE', ( #50107 ), #77595, .F. ) ;
#77779=CARTESIAN_POINT ( 'NONE',  ( -0.4615384615385840772, -12.51329471203414379, 31.30864560766407578 ) ) ;
#77780=CARTESIAN_POINT ( 'NONE',  ( -4.403869378067610363, -10.92453946501458439, 33.72985991061850086 ) ) ;
#77782=ADVANCED_FACE ( 'NONE', ( #86584 ), #66290, .F. ) ;
#77783=DIRECTION ( 'NONE',  ( -0.000000000000000000, -0.1736481776669307198, -0.9848077530122080203 ) ) ;
#77784=ORIENTED_EDGE ( 'NONE', *, *, #10359, .F. ) ;
#77785=CARTESIAN_POINT ( 'NONE',  ( 7.173022441425066731, -2.824170634883622188, 31.52227843825338738 ) ) ;
#77786=VECTOR ( 'NONE', #78276, 1000.000000000000114 ) ;
#77788=CARTESIAN_POINT ( 'NONE',  ( -15.90379184220783948, -10.66356715214248574, 33.62249196103329751 ) ) ;
#77789=CARTESIAN_POINT ( 'NONE',  ( -5.142193522883853340, -11.94971097300153140, 32.03036669348370680 ) ) ;
#77790=CARTESIAN_POINT ( 'NONE',  ( -10.48459417441766561, -2.845873456487965747, 32.17976146951972538 ) ) ;
#77791=CARTESIAN_POINT ( 'NONE',  ( -8.899377978668987055, -6.001485441113819874, 34.52039167877662607 ) ) ;
#77792=FACE_BOUND ( 'NONE', #82061, .T. ) ;
#77793=DIRECTION ( 'NONE',  ( -0.000000000000000000, -0.7660444431189791237, -0.6427876096865379196 ) ) ;
#77794=CARTESIAN_POINT ( 'NONE',  ( 1.384615384615265343, -2.625532179533778709, 30.86335684631627174 ) ) ;
#77795=CARTESIAN_POINT ( 'NONE',  ( -18.00000000000012079, -8.656820664282943056, 34.87096338111179961 ) ) ;
#77796=CARTESIAN_POINT ( 'NONE',  ( -7.623374177175779032, -12.69155399931963046, 30.53255429739157734 ) ) ;
#77797=FACE_OUTER_BOUND ( 'NONE', #16502, .T. ) ;
#77798=CIRCLE ( 'NONE', #57679, 0.2500000000000002220 ) ;
#77799=CARTESIAN_POINT ( 'NONE',  ( 4.153846153846032507, -11.94971097300221174, 32.03036669348237098 ) ) ;
#77801=ORIENTED_EDGE ( 'NONE', *, *, #64760, .T. ) ;
#77802=CARTESIAN_POINT ( 'NONE',  ( -4.284537620513710010, -11.71456829005830080, 32.44064028649416542 ) ) ;
#77803=CARTESIAN_POINT ( 'NONE',  ( -5.010854725920637520, -3.050289026998446840, 32.03036669348366416 ) ) ;
#77804=CARTESIAN_POINT ( 'NONE',  ( -7.596153846153843148, -2.499999999999999112, 29.81604066197450109 ) ) ;
#77805=CARTESIAN_POINT ( 'NONE',  ( -8.769230769230892619, -8.656820664282941280, 34.87096338111179961 ) ) ;
#77806=CARTESIAN_POINT ( 'NONE',  ( 10.74617642320940369, -12.11778462344221019, 31.66786338562085135 ) ) ;
#77808=CARTESIAN_POINT ( 'NONE',  ( -15.36091720050093024, -12.70455904226513866, 30.44083106164009322 ) ) ;
#77809=CARTESIAN_POINT ( 'NONE',  ( 18.13079180782478161, -3.062576670634119758, 32.05464942895959979 ) ) ;
#77810=CARTESIAN_POINT ( 'NONE',  ( -7.976301815885546098, -3.069018819979302926, 32.56621877034667278 ) ) ;
#77811=CARTESIAN_POINT ( 'NONE',  ( 0.4615384615384611200, -2.833524468853757305, 32.15551576947925838 ) ) ;
#77812=CARTESIAN_POINT ( 'NONE',  ( -16.94613263595612906, -4.684288915650984819, 34.18129842949671371 ) ) ;
#77813=CARTESIAN_POINT ( 'NONE',  ( 12.23805353697412812, -12.69144148231606017, 30.53333754910549303 ) ) ;
#77814=EDGE_CURVE ( 'NONE', #53071, #14607, #21357, .T. ) ;
#77815=CARTESIAN_POINT ( 'NONE',  ( 5.076923076923075762, -5.180354513474913603, 36.12317359536750416 ) ) ;
#77817=CARTESIAN_POINT ( 'NONE',  ( 17.14217821643591932, -2.657715359629131857, 31.77849191805844242 ) ) ;
#77818=ORIENTED_EDGE ( 'NONE', *, *, #55318, .F. ) ;
#77819=DIRECTION ( 'NONE',  ( 0.000000000000000000, 0.8660254037844377084, -0.5000000000000015543 ) ) ;
#77820=CARTESIAN_POINT ( 'NONE',  ( -17.32694631421604115, -2.823816976329320827, 31.52131813110797154 ) ) ;
#77822=AXIS2_PLACEMENT_3D ( 'NONE', #29275, #56732, #84226 ) ;
#77823=VECTOR ( 'NONE', #41022, 1000.000000000000114 ) ;
#77824=CARTESIAN_POINT ( 'NONE',  ( 5.076923076922953193, -2.379036618888197729, 30.90682066428292885 ) ) ;
#77825=DIRECTION ( 'NONE',  ( -0.000000000000000000, -0.5000000000000009992, -0.8660254037844380415 ) ) ;
#77826=ORIENTED_EDGE ( 'NONE', *, *, #75012, .T. ) ;
#77828=CARTESIAN_POINT ( 'NONE',  ( -7.846153846153844924, -12.78798330534102945, 29.74999999999997868 ) ) ;
#77829=EDGE_LOOP ( 'NONE', ( #85560, #80463 ) ) ;
#77830=CARTESIAN_POINT ( 'NONE',  ( 11.60371667797437567, -5.094484230520773593, 34.41647553114626845 ) ) ;
#77831=CARTESIAN_POINT ( 'NONE',  ( 4.087762742890272527, -8.120952969808774569, 34.71129190930000163 ) ) ;
#77832=ADVANCED_FACE ( 'NONE', ( #2801 ), #16767, .F. ) ;
#77833=ORIENTED_EDGE ( 'NONE', *, *, #83071, .F. ) ;
#77834=CARTESIAN_POINT ( 'NONE',  ( -5.142193522883852452, -11.48612834413959582, 32.76840700105983473 ) ) ;
#77835=VECTOR ( 'NONE', #42699, 1000.000000000000000 ) ;
#77836=EDGE_CURVE ( 'NONE', #69004, #79311, #71261, .T. ) ;
#77837=CARTESIAN_POINT ( 'NONE',  ( 9.019176287578908102, -5.057305518903948638, 34.11320923018887896 ) ) ;
#77838=ORIENTED_EDGE ( 'NONE', *, *, #13519, .T. ) ;
#77839=CARTESIAN_POINT ( 'NONE',  ( 9.019285189144222059, -2.318338780012835443, 30.59689888758630261 ) ) ;
#77840=CARTESIAN_POINT ( 'NONE',  ( -11.78846153846153832, -2.249999999999998668, 29.75000000000000355 ) ) ;
#77842=ORIENTED_EDGE ( 'NONE', *, *, #50937, .F. ) ;
#77843=EDGE_LOOP ( 'NONE', ( #23199, #40558 ) ) ;
#77844=B_SPLINE_CURVE_WITH_KNOTS ( 'NONE', 3,
 ( #33948, #8262, #35734, #69066, #63632, #164 ),
 .UNSPECIFIED., .F., .F.,
 ( 4, 2, 4 ),
 ( 0.0003909512603273815096, 0.0005862562993132049236, 0.0007815613382990282835 ),
 .UNSPECIFIED. ) ;
#77845=ORIENTED_EDGE ( 'NONE', *, *, #69309, .F. ) ;
#77846=EDGE_CURVE ( 'NONE', #18112, #70194, #64948, .T. ) ;
#77847=CARTESIAN_POINT ( 'NONE',  ( -7.173076923076921574, -7.500000000000001776, 35.00000000000000000 ) ) ;
#77848=CARTESIAN_POINT ( 'NONE',  ( -5.776987155906605942, -5.582272713120727481, 34.63742843783360570 ) ) ;
#77849=ADVANCED_FACE ( 'NONE', ( #72601 ), #45574, .F. ) ;
#77850=CARTESIAN_POINT ( 'NONE',  ( -3.007989561791164501, -8.540255544307065350, 34.89611431652622286 ) ) ;
#77851=CARTESIAN_POINT ( 'NONE',  ( 14.05769230769230838, -7.500000000000001776, 34.75000000000000000 ) ) ;
#77852=B_SPLINE_CURVE_WITH_KNOTS ( 'NONE', 3,
 ( #67315, #88063, #19127, #65967, #26325, #11482, #53791, #79939, #66423, #81280 ),
 .UNSPECIFIED., .F., .F.,
 ( 4, 2, 2, 2, 4 ),
 ( 0.0007817246256747459798, 0.0009771112852218896347, 0.001172497944769033398, 0.001367884604316177161, 0.001563271263863320708 ),
 .UNSPECIFIED. ) ;
#77853=VECTOR ( 'NONE', #27901, 1000.000000000000114 ) ;
#77854=ORIENTED_EDGE ( 'NONE', *, *, #76196, .F. ) ;
#77855=B_SPLINE_CURVE_WITH_KNOTS ( 'NONE', 3,
 ( #85050, #23327, #10272, #58434, #85930, #29660, #44038, #36417, #2607, #57120 ),
 .UNSPECIFIED., .F., .F.,
 ( 4, 2, 2, 2, 4 ),
 ( 0.0007817359430256360774, 0.0009771253907250041296, 0.001172514838424371965, 0.001367904286123740017, 0.001563293733823108069 ),
 .UNSPECIFIED. ) ;
#77856=EDGE_CURVE ( 'NONE', #44707, #64904, #70316, .T. ) ;
#77857=VERTEX_POINT ( 'NONE', #30292 ) ;
#77858=CARTESIAN_POINT ( 'NONE',  ( 4.376858997939548246, -8.282913670948747864, 34.94150082978203642 ) ) ;
#77859=ORIENTED_EDGE ( 'NONE', *, *, #28412, .F. ) ;
#77860=B_SPLINE_CURVE_WITH_KNOTS ( 'NONE', 3,
 ( #54388, #80995, #39573, #88653, #67030, #32796, #60705, #19284, #54836, #4890 ),
 .UNSPECIFIED., .F., .F.,
 ( 4, 2, 2, 2, 4 ),
 ( 0.0007817246256747451124, 0.0009771112852218885505, 0.001172497944769032097, 0.001367884604316175427, 0.001563271263863318973 ),
 .UNSPECIFIED. ) ;
#77861=CARTESIAN_POINT ( 'NONE',  ( 16.40390057375960708, -8.346898887586322147, 34.93166121998716278 ) ) ;
#77862=CARTESIAN_POINT ( 'NONE',  ( 15.36081428668900628, -2.254550872974306230, 29.97347326024527092 ) ) ;
#77864=EDGE_LOOP ( 'NONE', ( #25246, #88198, #8189, #4311 ) ) ;
#77865=ORIENTED_EDGE ( 'NONE', *, *, #24357, .F. ) ;
#77866=FACE_OUTER_BOUND ( 'NONE', #12846, .T. ) ;
#77867=ORIENTED_EDGE ( 'NONE', *, *, #25664, .F. ) ;
#77868=FACE_OUTER_BOUND ( 'NONE', #19980, .T. ) ;
#77869=DIRECTION ( 'NONE',  ( -0.000000000000000000, 0.3420201433256694346, -0.9396926207859080948 ) ) ;
#77870=EDGE_CURVE ( 'NONE', #17339, #28781, #57761, .T. ) ;
#77871=EDGE_LOOP ( 'NONE', ( #42209, #52466 ) ) ;
#77872=CARTESIAN_POINT ( 'NONE',  ( 15.90382291655318880, -12.43535235679832596, 30.55408501211184813 ) ) ;
#77874=CARTESIAN_POINT ( 'NONE',  ( -8.769230769230892619, -12.16647553114689728, 32.15551576947799362 ) ) ;
#77875=FACE_BOUND ( 'NONE', #82962, .T. ) ;
#77876=CARTESIAN_POINT ( 'NONE',  ( -9.561782254074048026, -4.299079248970732792, 33.91157788607253565 ) ) ;
#77877=DIRECTION ( 'NONE',  ( -0.000000000000000000, -0.9396926207859093161, -0.3420201433256663259 ) ) ;
#77878=EDGE_CURVE ( 'NONE', #10589, #27949, #54488, .T. ) ;
#77879=AXIS2_PLACEMENT_3D ( 'NONE', #46115, #66830, #921 ) ;
#77880=CARTESIAN_POINT ( 'NONE',  ( 13.13459216039392885, -12.68155406624981119, 30.59749803192733708 ) ) ;
#77881=CARTESIAN_POINT ( 'NONE',  ( -16.82686865700962286, -12.41089969410671223, 31.60739465890703670 ) ) ;
#77882=CARTESIAN_POINT ( 'NONE',  ( 6.700150705560777631, -11.76352882383564769, 32.36236540154569497 ) ) ;
#77883=CARTESIAN_POINT ( 'NONE',  ( 11.31553532094539172, -11.24512374952581872, 33.06303171183252942 ) ) ;
#77884=CARTESIAN_POINT ( 'NONE',  ( 12.46153846153846168, -3.937682226553329556, 33.60647404775216529 ) ) ;
#77885=VERTEX_POINT ( 'NONE', #65834 ) ;
#77886=EDGE_CURVE ( 'NONE', #57358, #27949, #37190, .T. ) ;
#77887=CARTESIAN_POINT ( 'NONE',  ( 10.55011416942384095, -10.90142922261923886, 33.41473453929638993 ) ) ;
#77888=VERTEX_POINT ( 'NONE', #71708 ) ;
#77889=EDGE_LOOP ( 'NONE', ( #39739, #55173 ) ) ;
#77890=B_SPLINE_CURVE_WITH_KNOTS ( 'NONE', 3,
 ( #14147, #39536, #41183, #61878, #53463, #73303, #62322, #39087, #87280, #73764 ),
 .UNSPECIFIED., .F., .F.,
 ( 4, 2, 2, 2, 4 ),
 ( 0.0007817359430256252354, 0.0009771253907249898181, 0.001172514838424354401, 0.001367904286123718983, 0.001563293733823083566 ),
 .UNSPECIFIED. ) ;
#77891=DIRECTION ( 'NONE',  ( -0.000000000000000000, 0.1736481776669307198, -0.9848077530122080203 ) ) ;
#77892=CARTESIAN_POINT ( 'NONE',  ( 10.68063975489745232, -12.70778746994558439, 30.41441678777536595 ) ) ;
#77893=CARTESIAN_POINT ( 'NONE',  ( 2.372947878968333590, -2.625532179533470512, 30.86335684631491105 ) ) ;
#77894=DIRECTION ( 'NONE',  ( -0.000000000000000000, 0.3420201433256694346, -0.9396926207859080948 ) ) ;
#77895=CARTESIAN_POINT ( 'NONE',  ( 2.438482748659257293, -2.295524264805589354, 30.44142389570982488 ) ) ;
#77896=CARTESIAN_POINT ( 'NONE',  ( -2.438382910802614933, -11.37499894934982514, 33.29245874905763003 ) ) ;
#77897=VERTEX_POINT ( 'NONE', #10014 ) ;
#77898=CARTESIAN_POINT ( 'NONE',  ( -18.13014720943822056, -6.001485441113818986, 34.52039167877662607 ) ) ;
#77899=CARTESIAN_POINT ( 'NONE',  ( 0.2386115026316116827, -12.64616026154729411, 30.79003144601913533 ) ) ;
#77900=CARTESIAN_POINT ( 'NONE',  ( 17.29970261819148902, -6.760870238392814535, 34.69528174975672385 ) ) ;
#77901=CARTESIAN_POINT ( 'NONE',  ( 1.384615384615386802, -12.29105614889573062, 35.45975837776705220 ) ) ;
#77902=LINE ( 'NONE', #64817, #73667 ) ;
#77903=EDGE_CURVE ( 'NONE', #58240, #60125, #4137, .T. ) ;
#77905=VERTEX_POINT ( 'NONE', #31624 ) ;
#77906=ORIENTED_EDGE ( 'NONE', *, *, #80852, .F. ) ;
#77907=CARTESIAN_POINT ( 'NONE',  ( -9.561515884482908234, -12.38066358083363738, 30.83685684665853444 ) ) ;
#77908=EDGE_CURVE ( 'NONE', #81137, #13624, #30726, .T. ) ;
#77910=CARTESIAN_POINT ( 'NONE',  ( -7.173053654019278191, -2.564618984488975961, 30.55390908950641915 ) ) ;
#77911=CARTESIAN_POINT ( 'NONE',  ( 9.915087233576100445, -10.11255958852956027, 34.01340905677048454 ) ) ;
#77912=CARTESIAN_POINT ( 'NONE',  ( 2.307692307692309264, -3.937682226553329556, 33.60647404775216529 ) ) ;
#77913=CARTESIAN_POINT ( 'NONE',  ( -4.826868657009624641, -3.435999193479609914, 33.07426656108010832 ) ) ;
#77916=ORIENTED_EDGE ( 'NONE', *, *, #50582, .T. ) ;
#77917=CARTESIAN_POINT ( 'NONE',  ( 5.076923076923075762, -4.945431358278436385, 36.03766855953609394 ) ) ;
#77918=CARTESIAN_POINT ( 'NONE',  ( -2.242437168179467477, -12.70778746994558439, 30.41441678777536595 ) ) ;
#77919=ORIENTED_EDGE ( 'NONE', *, *, #23165, .F. ) ;
#77920=CARTESIAN_POINT ( 'NONE',  ( 0.4615384615384611755, -2.249999999999998668, 29.50000000000001421 ) ) ;
#77921=CARTESIAN_POINT ( 'NONE',  ( -9.692307692307691624, -12.10708131394839349, 31.69288490824020244 ) ) ;
#77922=VECTOR ( 'NONE', #78437, 1000.000000000000000 ) ;
#77923=FACE_OUTER_BOUND ( 'NONE', #16415, .T. ) ;
#77924=EDGE_CURVE ( 'NONE', #24060, #21693, #17214, .T. ) ;
#77926=FACE_OUTER_BOUND ( 'NONE', #86028, .T. ) ;
#77928=AXIS2_PLACEMENT_3D ( 'NONE', #1171, #28194, #290 ) ;
#77930=EDGE_LOOP ( 'NONE', ( #45731, #61710 ) ) ;
#77931=ADVANCED_FACE ( 'NONE', ( #37937 ), #65400, .F. ) ;
#77933=CARTESIAN_POINT ( 'NONE',  ( -5.076923076923075762, -7.500000000000001776, 35.04278698407183867 ) ) ;
#77935=B_SPLINE_CURVE_WITH_KNOTS ( 'NONE', 3,
 ( #61670, #19813, #62125, #41864, #74766, #428, #13056, #40541, #61224, #27898 ),
 .UNSPECIFIED., .F., .F.,
 ( 4, 2, 2, 2, 4 ),
 ( 0.0007817246256747465219, 0.0009771112852218900684, 0.001172497944769033615, 0.001367884604316177378, 0.001563271263863320925 ),
 .UNSPECIFIED. ) ;
#77936=EDGE_CURVE ( 'NONE', #77001, #61355, #12687, .T. ) ;
#77937=CARTESIAN_POINT ( 'NONE',  ( -3.230769230769351186, -9.442884908241554243, 34.35708131394783038 ) ) ;
#77938=CARTESIAN_POINT ( 'NONE',  ( -3.165514091256390827, -11.06231777344671130, 33.60647404775212976 ) ) ;
#77940=CARTESIAN_POINT ( 'NONE',  ( 9.692307692307695177, -8.810774026931790459, 35.74407628777942847 ) ) ;
#77941=DIRECTION ( 'NONE',  ( -0.000000000000000000, -0.000000000000000000, -1.000000000000000000 ) ) ;
#77942=B_SPLINE_CURVE_WITH_KNOTS ( 'NONE', 3,
 ( #61740, #34727, #15794, #62194, #8593, #55438, #69843, #56329, #43259, #41936 ),
 .UNSPECIFIED., .F., .F.,
 ( 4, 2, 2, 2, 4 ),
 ( 0.0007817359430256369448, 0.0009771253907250049969, 0.001172514838424373049, 0.001367904286123741101, 0.001563293733823109153 ),
 .UNSPECIFIED. ) ;
#77943=VERTEX_POINT ( 'NONE', #40171 ) ;
#77944=EDGE_CURVE ( 'NONE', #28039, #18683, #77189, .T. ) ;
#77945=CARTESIAN_POINT ( 'NONE',  ( 6.923076923076924238, -6.343179335718451384, 34.87096338111211935 ) ) ;
#77947=ORIENTED_EDGE ( 'NONE', *, *, #85260, .F. ) ;
#77949=CARTESIAN_POINT ( 'NONE',  ( 16.82692307692307665, -2.499999999999998668, 29.75000000000000355 ) ) ;
#77950=EDGE_CURVE ( 'NONE', #76645, #70948, #66506, .T. ) ;
#77951=CARTESIAN_POINT ( 'NONE',  ( -12.52680846209478283, -10.33852847137145048, 34.16647553114627556 ) ) ;
#77952=CARTESIAN_POINT ( 'NONE',  ( 1.384615384615386802, -13.63283147151868846, 33.57946703557072254 ) ) ;
#77953=ORIENTED_EDGE ( 'NONE', *, *, #18951, .T. ) ;
#77954=CARTESIAN_POINT ( 'NONE',  ( -13.25408994638174320, -3.068774925481847493, 32.56582465632704526 ) ) ;
#77955=CIRCLE ( 'NONE', #23296, 0.2500000000000002220 ) ;
#77957=VECTOR ( 'NONE', #62560, 1000.000000000000000 ) ;
#77958=CARTESIAN_POINT ( 'NONE',  ( 2.531068248390492492, -2.501478030877322567, 29.88021232661720816 ) ) ;
#77959=CARTESIAN_POINT ( 'NONE',  ( -4.403846153846151523, -7.500000000000001776, 34.75000000000000000 ) ) ;
#77960=ORIENTED_EDGE ( 'NONE', *, *, #14640, .F. ) ;
#77961=CARTESIAN_POINT ( 'NONE',  ( 8.519254025182176449, -4.818429247618089661, 34.26397095200675125 ) ) ;
#77962=CARTESIAN_POINT ( 'NONE',  ( -12.68446467905460473, -5.667676309546437530, 34.40238873228292249 ) ) ;
#77963=ADVANCED_FACE ( 'NONE', ( #81595 ), #19882, .F. ) ;
#77965=AXIS2_PLACEMENT_3D ( 'NONE', #75501, #7044, #28654 ) ;
#77966=CARTESIAN_POINT ( 'NONE',  ( 13.51540582558233794, -11.93129842949671726, 32.56571108434900452 ) ) ;
#77967=CARTESIAN_POINT ( 'NONE',  ( -21.00000000000000000, -12.75000000000000178, 29.75000000000000355 ) ) ;
#77968=VERTEX_POINT ( 'NONE', #32504 ) ;
#77969=ORIENTED_EDGE ( 'NONE', *, *, #43610, .F. ) ;
#77970=FACE_BOUND ( 'NONE', #74029, .T. ) ;
#77971=VERTEX_POINT ( 'NONE', #87477 ) ;
#77973=B_SPLINE_CURVE_WITH_KNOTS ( 'NONE', 3,
 ( #78110, #9645, #37112, #49311, #76788, #15088, #1567, #42560, #38014, #4226 ),
 .UNSPECIFIED., .F., .F.,
 ( 4, 2, 2, 2, 4 ),
 ( 0.000000000000000000, 0.0001954339857564097241, 0.0003908679715128194482, 0.0005863019572692291723, 0.0007817359430256388964 ),
 .UNSPECIFIED. ) ;
#77974=CARTESIAN_POINT ( 'NONE',  ( 9.692307692307572609, -12.27809138561165270, 31.22303859784587132 ) ) ;
#77975=CARTESIAN_POINT ( 'NONE',  ( 0.5276057948885368720, -12.62096338111211757, 30.90682066428152908 ) ) ;
#77977=VERTEX_POINT ( 'NONE', #61295 ) ;
#77978=CARTESIAN_POINT ( 'NONE',  ( 0.4615384615384611200, -8.164416787775445883, 34.95778746994557906 ) ) ;
#77979=EDGE_LOOP ( 'NONE', ( #11531, #85601 ) ) ;
#77980=CARTESIAN_POINT ( 'NONE',  ( -0.4615384615385826339, -10.21337939537710326, 33.94971097300076224 ) ) ;
#77981=CARTESIAN_POINT ( 'NONE',  ( -5.076923076923075762, -4.786620604624113540, 33.94971097300155094 ) ) ;
#77982=AXIS2_PLACEMENT_3D ( 'NONE', #70982, #9289, #14712 ) ;
#77983=CARTESIAN_POINT ( 'NONE',  ( 14.24160992833217065, -11.91647553114624181, 32.58852847137148245 ) ) ;
#77984=B_SPLINE_CURVE_WITH_KNOTS ( 'NONE', 3,
 ( #19219, #46683, #53885, #81371, #19654, #68287, #47116, #6590, #74606, #12895 ),
 .UNSPECIFIED., .F., .F.,
 ( 4, 2, 2, 2, 4 ),
 ( 0.000000000000000000, 0.0001954311564186864949, 0.0003908623128373729899, 0.0005862934692560594577, 0.0007817246256747459798 ),
 .UNSPECIFIED. ) ;
#77985=FACE_BOUND ( 'NONE', #36478, .T. ) ;
#77986=VERTEX_POINT ( 'NONE', #46470 ) ;
#77987=CARTESIAN_POINT ( 'NONE',  ( 10.61538461538461675, -10.89733346790207413, 36.13435417666054406 ) ) ;
#77988=EDGE_CURVE ( 'NONE', #14831, #74248, #68081, .T. ) ;
#77989=B_SPLINE_CURVE_WITH_KNOTS ( 'NONE', 3,
 ( #3017, #3904, #63843, #51185, #37697, #44437, #85450, #30930, #78693, #8910 ),
 .UNSPECIFIED., .F., .F.,
 ( 4, 2, 2, 2, 4 ),
 ( 0.0007817359430256216575, 0.0009771253907249856981, 0.001172514838424349630, 0.001367904286123713779, 0.001563293733823077711 ),
 .UNSPECIFIED. ) ;
#77991=CARTESIAN_POINT ( 'NONE',  ( -14.55766903863466055, -9.148715823498378086, 34.47080413974185120 ) ) ;
#77992=CARTESIAN_POINT ( 'NONE',  ( 9.019176178608811156, -6.653508905675592722, 34.93172785388651391 ) ) ;
#77993=ORIENTED_EDGE ( 'NONE', *, *, #57544, .T. ) ;
#77994=EDGE_CURVE ( 'NONE', #86865, #44484, #39727, .T. ) ;
#77995=VERTEX_POINT ( 'NONE', #5493 ) ;
#77996=EDGE_LOOP ( 'NONE', ( #14417, #54047, #15452, #82849 ) ) ;
#77997=CARTESIAN_POINT ( 'NONE',  ( -8.096177083446809419, -6.695914987888146541, 34.68535235679833306 ) ) ;
#77998=DIRECTION ( 'NONE',  ( -0.000000000000000000, -0.8660254037844397068, -0.4999999999999978906 ) ) ;
#77999=EDGE_CURVE ( 'NONE', #25231, #64217, #14987, .T. ) ;
#78000=CARTESIAN_POINT ( 'NONE',  ( -10.74607608205217346, -12.11776431015576172, 31.66791131148498906 ) ) ;
#78001=CARTESIAN_POINT ( 'NONE',  ( -2.307692307692428724, -2.657715359629662544, 31.77849191805970364 ) ) ;
#78002=DIRECTION ( 'NONE',  ( 0.000000000000000000, 0.8660254037844377084, -0.5000000000000015543 ) ) ;
#78003=CARTESIAN_POINT ( 'NONE',  ( -11.66915214157184622, -2.295517848115769421, 30.44137282052137294 ) ) ;
#78004=ORIENTED_EDGE ( 'NONE', *, *, #18969, .T. ) ;
#78006=CARTESIAN_POINT ( 'NONE',  ( 11.53846153846153832, -11.35647404775217417, 33.31231777344666511 ) ) ;
#78007=CARTESIAN_POINT ( 'NONE',  ( 14.30769230769231015, -12.09954503811598769, 35.62045528018868623 ) ) ;
#78008=CARTESIAN_POINT ( 'NONE',  ( -15.23076923076922995, -2.708943851104267164, 35.45975837776705220 ) ) ;
#78010=EDGE_CURVE ( 'NONE', #38500, #12730, #19441, .T. ) ;
#78011=CARTESIAN_POINT ( 'NONE',  ( -14.30769230769230660, -8.564572088678739092, 35.78748833219616898 ) ) ;
#78012=VERTEX_POINT ( 'NONE', #54101 ) ;
#78013=FACE_BOUND ( 'NONE', #38990, .T. ) ;
#78014=CARTESIAN_POINT ( 'NONE',  ( 11.66925197942849479, -2.845873456487966635, 32.17976146951972538 ) ) ;
#78016=CIRCLE ( 'NONE', #85164, 0.2500000000000002220 ) ;
#78018=CARTESIAN_POINT ( 'NONE',  ( 12.33084699487089964, -12.11776431015576172, 31.66791131148498906 ) ) ;
#78019=ORIENTED_EDGE ( 'NONE', *, *, #71663, .T. ) ;
#78020=CARTESIAN_POINT ( 'NONE',  ( -3.454254174493178287, -12.44517049084099725, 30.48991314939691932 ) ) ;
#78021=CARTESIAN_POINT ( 'NONE',  ( -2.177166605928742449, -4.459921816937789885, 33.71989282347011851 ) ) ;
#78022=CARTESIAN_POINT ( 'NONE',  ( -15.00798956179115962, -10.23759521482555357, 34.22997729860117033 ) ) ;
#78023=CARTESIAN_POINT ( 'NONE',  ( -1.134669975237340367, -4.176053281294515251, 33.81426240980091791 ) ) ;
#78026=CARTESIAN_POINT ( 'NONE',  ( -9.758390071667825794, -2.833524468853757305, 32.15551576947924417 ) ) ;
#78027=ORIENTED_EDGE ( 'NONE', *, *, #69778, .F. ) ;
#78028=CARTESIAN_POINT ( 'NONE',  ( 13.38461538461538680, -8.164416787775445883, 34.95778746994557906 ) ) ;
#78029=VERTEX_POINT ( 'NONE', #40612 ) ;
#78030=LINE ( 'NONE', #23089, #64159 ) ;
#78031=CARTESIAN_POINT ( 'NONE',  ( 15.10062126103753855, -5.070767119584671079, 34.40440758774516183 ) ) ;
#78033=CARTESIAN_POINT ( 'NONE',  ( -12.68446542044531000, -10.77366814457252175, 33.85459836347579454 ) ) ;
#78034=CARTESIAN_POINT ( 'NONE',  ( -7.846153846153965716, -9.442884908241554243, 34.35708131394783038 ) ) ;
#78035=CARTESIAN_POINT ( 'NONE',  ( -9.692307692307814193, -12.16647553114689728, 32.15551576947799362 ) ) ;
#78037=EDGE_LOOP ( 'NONE', ( #2333, #17503, #13745, #2518 ) ) ;
#78038=ADVANCED_FACE ( 'NONE', ( #6386 ), #33838, .F. ) ;
#78039=CARTESIAN_POINT ( 'NONE',  ( 9.692307692308000711, -2.506253911140615021, 30.00000000000323297 ) ) ;
#78040=DIRECTION ( 'NONE',  ( -0.000000000000000000, -0.9396926207859093161, -0.3420201433256663259 ) ) ;
#78042=ORIENTED_EDGE ( 'NONE', *, *, #21370, .F. ) ;
#78043=ORIENTED_EDGE ( 'NONE', *, *, #23659, .T. ) ;
#78044=CARTESIAN_POINT ( 'NONE',  ( 3.903822916553188804, -12.22074536777954989, 31.39888409691088356 ) ) ;
#78045=CARTESIAN_POINT ( 'NONE',  ( 11.53846153846141753, -3.835265460704628371, 33.15142922262033665 ) ) ;
#78046=CARTESIAN_POINT ( 'NONE',  ( -1.384615384615383471, -4.945431358278436385, 36.03766855953609394 ) ) ;
#78048=CARTESIAN_POINT ( 'NONE',  ( 9.019176178608811156, -11.56426240980093745, 33.07394671870546432 ) ) ;
#78049=ADVANCED_FACE ( 'NONE', ( #34281 ), #50006, .F. ) ;
#78050=CARTESIAN_POINT ( 'NONE',  ( 8.769230769230645706, -3.083524468854526912, 32.58852847137268327 ) ) ;
#78051=AXIS2_PLACEMENT_3D ( 'NONE', #31850, #64720, #3020 ) ;
#78052=CARTESIAN_POINT ( 'NONE',  ( 0.3309785479250964002, -2.254533558242299396, 29.97296025877828285 ) ) ;
#78053=ORIENTED_EDGE ( 'NONE', *, *, #16703, .T. ) ;
#78054=LINE ( 'NONE', #44693, #4575 ) ;
#78055=CARTESIAN_POINT ( 'NONE',  ( -17.32694631421604115, -12.22074536777955345, 31.39888409691088356 ) ) ;
#78056=EDGE_CURVE ( 'NONE', #48096, #44924, #81517, .T. ) ;
#78057=EDGE_CURVE ( 'NONE', #49839, #32338, #76229, .T. ) ;
#78058=CARTESIAN_POINT ( 'NONE',  ( -8.992715693795100051, -11.60425143139329940, 33.02411095842164457 ) ) ;
#78059=DIRECTION ( 'NONE',  ( -0.000000000000000000, 1.000000000000000000, -0.000000000000000000 ) ) ;
#78060=EDGE_LOOP ( 'NONE', ( #57492, #86839 ) ) ;
#78063=CARTESIAN_POINT ( 'NONE',  ( 0.5920641633020254924, -9.417988943895561960, 34.36773134775778260 ) ) ;
#78065=LINE ( 'NONE', #77182, #23953 ) ;
#78066=CARTESIAN_POINT ( 'NONE',  ( -15.23076923076935252, -5.941354392335915335, 34.76329471203413846 ) ) ;
#78067=ORIENTED_EDGE ( 'NONE', *, *, #50036, .T. ) ;
#78068=CARTESIAN_POINT ( 'NONE',  ( -2.557715531913763218, -6.652501968072646932, 34.93155406624980941 ) ) ;
#78069=EDGE_CURVE ( 'NONE', #18634, #67793, #28409, .T. ) ;
#78070=CARTESIAN_POINT ( 'NONE',  ( 9.469380733400843297, -2.889293201056495786, 32.26117774369186009 ) ) ;
#78071=B_SPLINE_CURVE_WITH_KNOTS ( 'NONE', 3,
 ( #50159, #77648, #71768, #42544, #70900, #70003, #9206, #36669, #2423, #29917 ),
 .UNSPECIFIED., .F., .F.,
 ( 4, 2, 2, 2, 4 ),
 ( 0.0007817359430256371616, 0.0009771253907250049969, 0.001172514838424373049, 0.001367904286123741101, 0.001563293733823108937 ),
 .UNSPECIFIED. ) ;
#78072=CARTESIAN_POINT ( 'NONE',  ( -8.992157728137616601, -9.172386477786396597, 34.72672124145550043 ) ) ;
#78073=ADVANCED_FACE ( 'NONE', ( #22540 ), #69844, .F. ) ;
#78076=CARTESIAN_POINT ( 'NONE',  ( 16.37662582282421653, -10.23759521482555357, 34.22997729860117033 ) ) ;
#78077=EDGE_LOOP ( 'NONE', ( #73016, #44399 ) ) ;
#78078=EDGE_CURVE ( 'NONE', #61129, #11362, #17042, .T. ) ;
#78079=AXIS2_PLACEMENT_3D ( 'NONE', #78222, #71029, #42682 ) ;
#78080=CYLINDRICAL_SURFACE ( 'NONE', #65149, 0.2499999999999986955 ) ;
#78081=AXIS2_PLACEMENT_3D ( 'NONE', #2962, #43957, #71421 ) ;
#78083=CARTESIAN_POINT ( 'NONE',  ( -14.30769230769230660, -2.249999999999998668, 29.75000000000001776 ) ) ;
#78084=CARTESIAN_POINT ( 'NONE',  ( -14.05763799605399278, -9.943054286541403997, 34.11300777759954883 ) ) ;
#78086=VECTOR ( 'NONE', #52261, 1000.000000000000000 ) ;
#78087=ORIENTED_EDGE ( 'NONE', *, *, #72554, .F. ) ;
#78088=EDGE_LOOP ( 'NONE', ( #57902, #24979 ) ) ;
#78089=VERTEX_POINT ( 'NONE', #27972 ) ;
#78090=CARTESIAN_POINT ( 'NONE',  ( -12.52678839331254679, -2.255955759149247619, 30.00000000000013856 ) ) ;
#78091=CARTESIAN_POINT ( 'NONE',  ( -16.40384615384615330, -2.249999999999998668, 29.75000000000000355 ) ) ;
#78093=EDGE_CURVE ( 'NONE', #2602, #80357, #24548, .T. ) ;
#78094=DIRECTION ( 'NONE',  ( 0.000000000000000000, 0.7660444431189822323, -0.6427876096865344779 ) ) ;
#78095=B_SPLINE_CURVE_WITH_KNOTS ( 'NONE', 3,
 ( #73186, #25883, #67317, #46599, #32635, #52007, #45255, #66874, #11484, #4730 ),
 .UNSPECIFIED., .F., .F.,
 ( 4, 2, 2, 2, 4 ),
 ( 0.0007817246256747434861, 0.0009771112852218859484, 0.001172497944769028411, 0.001367884604316171090, 0.001563271263863313552 ),
 .UNSPECIFIED. ) ;
#78096=CARTESIAN_POINT ( 'NONE',  ( 5.777073782483853392, -11.76352882383564769, 32.36236540154569497 ) ) ;
#78097=CARTESIAN_POINT ( 'NONE',  ( -5.999999999999998224, -12.37446782046654192, 30.86335684631486131 ) ) ;
#78098=B_SPLINE_CURVE_WITH_KNOTS ( 'NONE', 3,
 ( #48889, #49772, #49340, #27728, #265, #705, #22308, #68721, #28171, #20531 ),
 .UNSPECIFIED., .F., .F.,
 ( 4, 2, 2, 2, 4 ),
 ( 0.0007817246256747472808, 0.0009771112852218907189, 0.001172497944769034265, 0.001367884604316177595, 0.001563271263863321141 ),
 .UNSPECIFIED. ) ;
#78099=ORIENTED_EDGE ( 'NONE', *, *, #53723, .T. ) ;
#78100=ORIENTED_EDGE ( 'NONE', *, *, #67985, .T. ) ;
#78102=CARTESIAN_POINT ( 'NONE',  ( 11.53846153846141576, -2.657715359629662544, 31.77849191805970364 ) ) ;
#78103=ORIENTED_EDGE ( 'NONE', *, *, #37646, .F. ) ;
#78104=AXIS2_PLACEMENT_3D ( 'NONE', #29007, #79842, #53241 ) ;
#78105=CARTESIAN_POINT ( 'NONE',  ( 0.6845498131513104711, -8.239487800360276282, 34.69522927552633718 ) ) ;
#78106=CARTESIAN_POINT ( 'NONE',  ( -8.546219417617921366, -11.24521262558773493, 33.06293181088029343 ) ) ;
#78108=B_SPLINE_CURVE_WITH_KNOTS ( 'NONE', 3,
 ( #71614, #15361, #3602, #9920, #2704, #31071, #63968, #23430, #50455, #77937 ),
 .UNSPECIFIED., .F., .F.,
 ( 4, 2, 2, 2, 4 ),
 ( 0.000000000000000000, 0.0001954339857564073388, 0.0003908679715128146777, 0.0005863019572692220165, 0.0007817359430256293554 ),
 .UNSPECIFIED. ) ;
#78109=CARTESIAN_POINT ( 'NONE',  ( 1.607628228708780860, -4.762714258010882773, 34.23016756924214832 ) ) ;
#78110=CARTESIAN_POINT ( 'NONE',  ( -10.61538461538461320, -11.69971097300155272, 32.46337939537588113 ) ) ;
#78111=ORIENTED_EDGE ( 'NONE', *, *, #29686, .F. ) ;
#78113=CARTESIAN_POINT ( 'NONE',  ( -17.20707104665477161, -11.66186481527757479, 32.95055677023626117 ) ) ;
#78114=EDGE_LOOP ( 'NONE', ( #19326, #37855, #55820, #63349 ) ) ;
#78115=FACE_BOUND ( 'NONE', #68093, .T. ) ;
#78116=CARTESIAN_POINT ( 'NONE',  ( 15.23076923076911093, -10.21337939537710326, 33.94971097300076224 ) ) ;
#78117=CARTESIAN_POINT ( 'NONE',  ( -9.692307692307691624, -3.886160181151819604, 36.00935417666054406 ) ) ;
#78118=VERTEX_POINT ( 'NONE', #41937 ) ;
#78119=CARTESIAN_POINT ( 'NONE',  ( -15.10024352900566669, -5.195472089885680766, 34.18748526763464923 ) ) ;
#78120=CARTESIAN_POINT ( 'NONE',  ( 16.28463796167094557, -4.118422570099827595, 33.43335022499816489 ) ) ;
#78122=CARTESIAN_POINT ( 'NONE',  ( 3.903822916553187472, -11.37209801155882971, 32.91403422569032955 ) ) ;
#78123=CARTESIAN_POINT ( 'NONE',  ( -5.076923076923075762, -1.466349020453238561, 30.81389545987213907 ) ) ;
#78125=CARTESIAN_POINT ( 'NONE',  ( 7.976944287120798727, -11.37503395064541678, 33.29242100308974273 ) ) ;
#78127=CARTESIAN_POINT ( 'NONE',  ( 2.057715563643717882, -12.01397095200673881, 32.43157075238190146 ) ) ;
#78129=CARTESIAN_POINT ( 'NONE',  ( 13.63456079399343146, -2.341251567377310217, 30.72681386836322659 ) ) ;
#78130=DIRECTION ( 'NONE',  ( 0.000000000000000000, 0.000000000000000000, 1.000000000000000000 ) ) ;
#78131=CARTESIAN_POINT ( 'NONE',  ( -13.25382494364843389, -12.35292014791297710, 31.75344720912887198 ) ) ;
#78132=CARTESIAN_POINT ( 'NONE',  ( 4.219914504848593317, -12.10708131394839882, 31.69288490824020954 ) ) ;
#78134=FACE_OUTER_BOUND ( 'NONE', #48710, .T. ) ;
#78135=B_SPLINE_CURVE_WITH_KNOTS ( 'NONE', 3,
 ( #9692, #8819, #16015, #37161, #76835, #77266, #22758, #50221, #43483, #23647 ),
 .UNSPECIFIED., .F., .F.,
 ( 4, 2, 2, 2, 4 ),
 ( 0.0007817359430256320659, 0.0009771253907249987086, 0.001172514838424365460, 0.001367904286123732211, 0.001563293733823098962 ),
 .UNSPECIFIED. ) ;
#78136=CARTESIAN_POINT ( 'NONE',  ( -1.253824943648432777, -9.084667340241226796, 34.75534355489798344 ) ) ;
#78137=CARTESIAN_POINT ( 'NONE',  ( -11.53846153846153655, -11.16473453929635440, 33.15142922261926373 ) ) ;
#78138=CARTESIAN_POINT ( 'NONE',  ( -15.23076923076935252, -12.51329471203414379, 31.30864560766407578 ) ) ;
#78139=LINE ( 'NONE', #9680, #14580 ) ;
#78141=EDGE_LOOP ( 'NONE', ( #35945, #8578, #67823, #39819 ) ) ;
#78146=ORIENTED_EDGE ( 'NONE', *, *, #9178, .F. ) ;
#78147=ADVANCED_FACE ( 'NONE', ( #62195 ), #502, .F. ) ;
#78148=CARTESIAN_POINT ( 'NONE',  ( -4.087777802843714170, -11.16473453929635440, 33.15142922261926373 ) ) ;
#78149=EDGE_LOOP ( 'NONE', ( #4248, #35167, #3820, #12046 ) ) ;
#78152=CARTESIAN_POINT ( 'NONE',  ( 7.715463243043540587, -8.191372820521381826, 34.95448215188423546 ) ) ;
#78153=ADVANCED_FACE ( 'NONE', ( #37822 ), #45463, .F. ) ;
#78154=FACE_OUTER_BOUND ( 'NONE', #30404, .T. ) ;
#78155=CARTESIAN_POINT ( 'NONE',  ( 6.923076923076924238, -9.905515769479276145, 34.41647553114623292 ) ) ;
#78156=CARTESIAN_POINT ( 'NONE',  ( -5.326899820971668476, -2.920706130388546651, 32.31842814019191223 ) ) ;
#78157=LINE ( 'NONE', #22761, #83516 ) ;
#78158=DIRECTION ( 'NONE',  ( -0.000000000000000000, -0.9396926207859092051, -0.3420201433256662704 ) ) ;
#78159=FACE_OUTER_BOUND ( 'NONE', #66687, .T. ) ;
#78161=CARTESIAN_POINT ( 'NONE',  ( 1.384615384615386802, -3.050289026998446396, 32.03036669348365706 ) ) ;
#78162=CARTESIAN_POINT ( 'NONE',  ( -15.23076923076922995, -2.538708090699994813, 30.37095296980875503 ) ) ;
#78163=EDGE_CURVE ( 'NONE', #683, #60694, #71921, .T. ) ;
#78166=B_SPLINE_CURVE_WITH_KNOTS ( 'NONE', 3,
 ( #17978, #3111, #45431, #72909, #86453, #16629, #23818, #24727, #11215, #14651 ),
 .UNSPECIFIED., .F., .F.,
 ( 4, 2, 2, 2, 4 ),
 ( 0.0007817246256747465219, 0.0009771112852218898515, 0.001172497944769033181, 0.001367884604316176294, 0.001563271263863319624 ),
 .UNSPECIFIED. ) ;
#78167=B_SPLINE_CURVE_WITH_KNOTS ( 'NONE', 3,
 ( #2999, #43989, #16971, #24161, #1687, #84995, #56631, #57508, #58382, #17419 ),
 .UNSPECIFIED., .F., .F.,
 ( 4, 2, 2, 2, 4 ),
 ( 0.0007817359430256333669, 0.0009771253907250056474, 0.001172514838424370881, 0.001367904286123736331, 0.001563293733823101564 ),
 .UNSPECIFIED. ) ;
#78171=CARTESIAN_POINT ( 'NONE',  ( 12.33139049180676672, -8.630895178749533159, 34.87696386517710323 ) ) ;
#78172=FACE_OUTER_BOUND ( 'NONE', #20811, .T. ) ;
#78173=CARTESIAN_POINT ( 'NONE',  ( 15.36081666601968720, -7.723484941389743952, 34.99544897038808955 ) ) ;
#78174=CARTESIAN_POINT ( 'NONE',  ( 17.32686848630112308, -12.45601412856602686, 31.48342859153981621 ) ) ;
#78175=CARTESIAN_POINT ( 'NONE',  ( -14.17716686945866300, -4.299079248970732792, 33.91157788607253565 ) ) ;
#78176=B_SPLINE_CURVE_WITH_KNOTS ( 'NONE', 3,
 ( #4923, #6256, #47222, #73830, #60295, #32831, #61176, #18431, #73372, #19760 ),
 .UNSPECIFIED., .F., .F.,
 ( 4, 2, 2, 2, 4 ),
 ( 0.000000000000000000, 0.0001954339857564073659, 0.0003908679715128147319, 0.0005863019572692221250, 0.0007817359430256294638 ),
 .UNSPECIFIED. ) ;
#78178=ADVANCED_FACE ( 'NONE', ( #10357 ), #2693, .F. ) ;
#78180=CARTESIAN_POINT ( 'NONE',  ( -1.318547033612944563, -9.780366693483669494, 34.19971097300155805 ) ) ;
#78181=ORIENTED_EDGE ( 'NONE', *, *, #22807, .F. ) ;
#78184=CARTESIAN_POINT ( 'NONE',  ( -6.130147969731695845, -12.70455904226513866, 30.44083106164009322 ) ) ;
#78185=DIRECTION ( 'NONE',  ( -0.000000000000000000, 0.9848077530122086864, -0.1736481776669273891 ) ) ;
#78186=CARTESIAN_POINT ( 'NONE',  ( 4.153846153846032507, -3.835265460704628371, 33.15142922262033665 ) ) ;
#78187=CARTESIAN_POINT ( 'NONE',  ( 17.75002326905764960, -9.148715823498378086, 34.47080413974185120 ) ) ;
#78188=ORIENTED_EDGE ( 'NONE', *, *, #67177, .T. ) ;
#78189=CARTESIAN_POINT ( 'NONE',  ( -14.24162395668987102, -12.10708131394839882, 31.69288490824020954 ) ) ;
#78190=ORIENTED_EDGE ( 'NONE', *, *, #48845, .F. ) ;
#78191=B_SPLINE_CURVE_WITH_KNOTS ( 'NONE', 3,
 ( #39258, #88349, #41026, #47324, #74817, #18537, #45994, #11779, #66719, #59955 ),
 .UNSPECIFIED., .F., .F.,
 ( 4, 2, 2, 2, 4 ),
 ( 0.0007817359430256399806, 0.0009771253907250089001, 0.001172514838424378036, 0.001367904286123746956, 0.001563293733823115875 ),
 .UNSPECIFIED. ) ;
#78192=EDGE_LOOP ( 'NONE', ( #27444, #84104 ) ) ;
#78193=AXIS2_PLACEMENT_3D ( 'NONE', #57820, #30352, #69564 ) ;
#78194=CARTESIAN_POINT ( 'NONE',  ( 13.38461538461526423, -5.094484230521993062, 34.41647553114689373 ) ) ;
#78198=VECTOR ( 'NONE', #43104, 999.9999999999998863 ) ;
#78199=CARTESIAN_POINT ( 'NONE',  ( -3.903846153844716671, -7.500000000000155431, 34.75000000000007105 ) ) ;
#78200=DIRECTION ( 'NONE',  ( -0.000000000000000000, 0.8660254037844397068, -0.4999999999999978906 ) ) ;
#78201=ORIENTED_EDGE ( 'NONE', *, *, #64105, .T. ) ;
#78202=ORIENTED_EDGE ( 'NONE', *, *, #12571, .T. ) ;
#78205=CARTESIAN_POINT ( 'NONE',  ( 11.53846153846153832, -5.471508081941601098, 34.59228464037088457 ) ) ;
#78206=EDGE_LOOP ( 'NONE', ( #17485, #65221 ) ) ;
#78207=DIRECTION ( 'NONE',  ( 1.000000000000000000, 0.000000000000000000, 0.000000000000000000 ) ) ;
#78208=CARTESIAN_POINT ( 'NONE',  ( 4.826899839630112155, -3.711651800289232916, 33.01384336483936011 ) ) ;
#78209=DIRECTION ( 'NONE',  ( -0.000000000000000000, 0.3420201433256694346, -0.9396926207859080948 ) ) ;
#78210=ORIENTED_EDGE ( 'NONE', *, *, #21139, .T. ) ;
#78212=VERTEX_POINT ( 'NONE', #10803 ) ;
#78213=CARTESIAN_POINT ( 'NONE',  ( -24.00000000000000000, -5.499999999999981348, 27.75000000000000000 ) ) ;
#78214=CARTESIAN_POINT ( 'NONE',  ( 10.68064018666064108, -9.442884908240273489, 34.35708131394835618 ) ) ;
#78215=CARTESIAN_POINT ( 'NONE',  ( -17.75005459062195712, -2.589246495874658383, 31.60778113518102828 ) ) ;
#78216=CARTESIAN_POINT ( 'NONE',  ( 10.86538461538468248, -7.434744429011176159, 34.75000000000000711 ) ) ;
#78217=CARTESIAN_POINT ( 'NONE',  ( -10.68146699474474914, -5.471508081941602875, 34.59228464037088457 ) ) ;
#78218=CARTESIAN_POINT ( 'NONE',  ( 16.15384615384615330, -2.538708090699994813, 30.37095296980875503 ) ) ;
#78219=CARTESIAN_POINT ( 'NONE',  ( -0.2115930521604179049, -12.68172785388650681, 30.59649109432439573 ) ) ;
#78220=ORIENTED_EDGE ( 'NONE', *, *, #24347, .T. ) ;
#78222=CARTESIAN_POINT ( 'NONE',  ( -7.846153846153844924, -6.435427911321262684, 35.78748833219616898 ) ) ;
#78223=B_SPLINE_CURVE_WITH_KNOTS ( 'NONE', 3,
 ( #34573, #75549, #82767, #7547, #33689, #54391, #1220, #56171, #62468, #47644 ),
 .UNSPECIFIED., .F., .F.,
 ( 4, 2, 2, 2, 4 ),
 ( 0.0007817359430256317406, 0.0009771253907249982749, 0.001172514838424365026, 0.001367904286123731560, 0.001563293733823098094 ),
 .UNSPECIFIED. ) ;
#78224=ORIENTED_EDGE ( 'NONE', *, *, #37629, .T. ) ;
#78225=VECTOR ( 'NONE', #9538, 1000.000000000000227 ) ;
#78226=CARTESIAN_POINT ( 'NONE',  ( 7.053868730901709405, -2.729792928343270919, 31.24908615093345077 ) ) ;
#78227=CARTESIAN_POINT ( 'NONE',  ( 12.39628747137721909, -2.506253911140460922, 30.00000000000013856 ) ) ;
#78228=LINE ( 'NONE', #43558, #22382 ) ;
#78229=CARTESIAN_POINT ( 'NONE',  ( 2.057715563643717438, -5.643011162660950042, 34.66104346484419096 ) ) ;
#78230=FACE_OUTER_BOUND ( 'NONE', #50695, .T. ) ;
#78231=CARTESIAN_POINT ( 'NONE',  ( 12.33139125210024112, -4.460286881179643004, 33.72017969459903242 ) ) ;
#78232=FACE_BOUND ( 'NONE', #39909, .T. ) ;
#78233=CARTESIAN_POINT ( 'NONE',  ( 13.38461538461538680, -7.500000000000001776, 35.04278698407183867 ) ) ;
#78234=FACE_OUTER_BOUND ( 'NONE', #2371, .T. ) ;
#78235=CARTESIAN_POINT ( 'NONE',  ( -6.857821351800898135, -10.90142922261932057, 33.41473453929631887 ) ) ;
#78236=CARTESIAN_POINT ( 'NONE',  ( -4.826868657009623753, -10.06805714834173848, 34.32951233291982618 ) ) ;
#78238=CARTESIAN_POINT ( 'NONE',  ( -7.846153846153844924, -1.790695186598648903, 34.54067556320373455 ) ) ;
#78240=ORIENTED_EDGE ( 'NONE', *, *, #16152, .F. ) ;
#78241=EDGE_CURVE ( 'NONE', #44632, #8069, #6389, .T. ) ;
#78242=CYLINDRICAL_SURFACE ( 'NONE', #27703, 0.2499999999999979738 ) ;
#78245=CARTESIAN_POINT ( 'NONE',  ( -10.68146699474474914, -11.35647404775217595, 33.31231777344666511 ) ) ;
#78246=EDGE_CURVE ( 'NONE', #11323, #45031, #38272, .T. ) ;
#78247=CARTESIAN_POINT ( 'NONE',  ( 13.38461538461526423, -10.33852847137269571, 34.16647553114546554 ) ) ;
#78249=CARTESIAN_POINT ( 'NONE',  ( -8.769230769230768274, -2.721908614388771852, 31.22303859784724978 ) ) ;
#78250=CARTESIAN_POINT ( 'NONE',  ( -12.46153846153846168, -5.180354513474913603, 36.12317359536750416 ) ) ;
#78251=FACE_OUTER_BOUND ( 'NONE', #33494, .T. ) ;
#78252=CARTESIAN_POINT ( 'NONE',  ( -12.46153846153846168, -13.75783147151868846, 33.36296068462461051 ) ) ;
#78253=CARTESIAN_POINT ( 'NONE',  ( -3.230769230769229949, -3.937682226553329556, 33.60647404775216529 ) ) ;
#78254=CYLINDRICAL_SURFACE ( 'NONE', #84295, 0.2500000000000008882 ) ;
#78256=CARTESIAN_POINT ( 'NONE',  ( -6.066082379360133281, -11.91647553114624181, 32.58852847137148245 ) ) ;
#78257=EDGE_CURVE ( 'NONE', #86451, #23528, #26619, .T. ) ;
#78258=DIRECTION ( 'NONE',  ( 0.000000000000000000, -6.938893903907222067E-15, 1.000000000000000000 ) ) ;
#78259=ORIENTED_EDGE ( 'NONE', *, *, #53622, .T. ) ;
#78260=CARTESIAN_POINT ( 'NONE',  ( 17.29993592101647337, -12.64618726649961289, 30.78989965857442712 ) ) ;
#78261=CARTESIAN_POINT ( 'NONE',  ( -5.777220331021934108, -2.612705202774697533, 31.66806509827799943 ) ) ;
#78263=B_SPLINE_CURVE_WITH_KNOTS ( 'NONE', 3,
 ( #48122, #35057, #48561, #13899, #55767, #69733, #34620, #28756, #82373, #27420 ),
 .UNSPECIFIED., .F., .F.,
 ( 4, 2, 2, 2, 4 ),
 ( 0.000000000000000000, 0.0001954311564186862781, 0.0003908623128373725562, 0.0005862934692560588072, 0.0007817246256747451124 ),
 .UNSPECIFIED. ) ;
#78264=CARTESIAN_POINT ( 'NONE',  ( 0.5267936010512989098, -3.643525952247864463, 33.31231777344670064 ) ) ;
#78265=CARTESIAN_POINT ( 'NONE',  ( 9.692307692307695177, -10.67929555188718282, 33.92786785259544047 ) ) ;
#78267=CARTESIAN_POINT ( 'NONE',  ( 1.634560902963528184, -4.336752205174647656, 33.62275283266504289 ) ) ;
#78268=CARTESIAN_POINT ( 'NONE',  ( 12.46153846153833911, -6.026961402154118019, 34.52809138561165270 ) ) ;
#78269=EDGE_LOOP ( 'NONE', ( #744, #46909, #79693, #40759 ) ) ;
#78270=CARTESIAN_POINT ( 'NONE',  ( 6.673100192134571174, -3.137211980971221781, 32.19342716148376837 ) ) ;
#78271=CARTESIAN_POINT ( 'NONE',  ( 7.846153846153846700, -1.422936976036506707, 30.56769352161908415 ) ) ;
#78272=B_SPLINE_CURVE_WITH_KNOTS ( 'NONE', 3,
 ( #14836, #42313, #34657, #35547, #62126, #1304, #429, #49502, #76974, #22465 ),
 .UNSPECIFIED., .F., .F.,
 ( 4, 2, 2, 2, 4 ),
 ( 0.0007817359430256398721, 0.0009771253907250089001, 0.001172514838424377820, 0.001367904286123746739, 0.001563293733823115659 ),
 .UNSPECIFIED. ) ;
#78273=CARTESIAN_POINT ( 'NONE',  ( 8.769230769230645706, -5.094484230521993062, 34.41647553114689373 ) ) ;
#78274=CARTESIAN_POINT ( 'NONE',  ( -13.63463862190834952, -3.202444869320336451, 32.30641848906366675 ) ) ;
#78275=ORIENTED_EDGE ( 'NONE', *, *, #9591, .F. ) ;
#78276=DIRECTION ( 'NONE',  ( -0.000000000000000000, -0.3420201433256694346, -0.9396926207859080948 ) ) ;
#78278=EDGE_CURVE ( 'NONE', #76411, #13379, #21184, .T. ) ;
#78279=LINE ( 'NONE', #80066, #47020 ) ;
#78280=ORIENTED_EDGE ( 'NONE', *, *, #14158, .F. ) ;
#78281=ADVANCED_FACE ( 'NONE', ( #45013 ), #43692, .F. ) ;
#78282=ORIENTED_EDGE ( 'NONE', *, *, #22253, .F. ) ;
#78283=B_SPLINE_CURVE_WITH_KNOTS ( 'NONE', 3,
 ( #41189, #62329, #198, #83062, #82631, #28109, #55573, #21351, #23558, #1968 ),
 .UNSPECIFIED., .F., .F.,
 ( 4, 2, 2, 2, 4 ),
 ( 0.0007817246256747445703, 0.0009771112852218870326, 0.001172497944769029495, 0.001367884604316171957, 0.001563271263863314419 ),
 .UNSPECIFIED. ) ;
#78284=ORIENTED_EDGE ( 'NONE', *, *, #86637, .T. ) ;
#78285=EDGE_CURVE ( 'NONE', #8200, #58928, #36931, .T. ) ;
#78286=CARTESIAN_POINT ( 'NONE',  ( -18.13069146666756026, -3.530157926970575399, 32.79014554554149896 ) ) ;
#78287=CARTESIAN_POINT ( 'NONE',  ( -8.638705067467206788, -3.285477652293413264, 32.44071101563363158 ) ) ;
#78288=EDGE_CURVE ( 'NONE', #62161, #74008, #25695, .T. ) ;
#78289=CARTESIAN_POINT ( 'NONE',  ( -7.779984705191187899, -7.250054483168840491, 34.74374881642864921 ) ) ;
#78290=CARTESIAN_POINT ( 'NONE',  ( 5.999999999999878320, -4.320704448113951379, 33.92786785259630022 ) ) ;
#78291=ORIENTED_EDGE ( 'NONE', *, *, #38260, .T. ) ;
#78292=B_SPLINE_CURVE_WITH_KNOTS ( 'NONE', 3,
 ( #23091, #35274, #69063, #42487, #36178, #7370, #9149, #43364, #62294, #83026 ),
 .UNSPECIFIED., .F., .F.,
 ( 4, 2, 2, 2, 4 ),
 ( 0.000000000000000000, 0.0001954311564186864407, 0.0003908623128373728815, 0.0005862934692560593493, 0.0007817246256747457630 ),
 .UNSPECIFIED. ) ;
#78294=CARTESIAN_POINT ( 'NONE',  ( 9.442284455014730682, -4.335965774309649134, 33.62209801155881905 ) ) ;
#78296=B_SPLINE_CURVE_WITH_KNOTS ( 'NONE', 3,
 ( #20896, #69091, #35759, #48809, #7398, #13704, #40744, #74975, #35302, #82626 ),
 .UNSPECIFIED., .F., .F.,
 ( 4, 2, 2, 2, 4 ),
 ( 0.0007817246256747461966, 0.0009771112852218892010, 0.001172497944769032314, 0.001367884604316175427, 0.001563271263863318323 ),
 .UNSPECIFIED. ) ;
#78297=CARTESIAN_POINT ( 'NONE',  ( 17.29993442853592711, -4.887748414852792322, 34.01359900205217457 ) ) ;
#78298=DIRECTION ( 'NONE',  ( -0.000000000000000000, 1.000000000000000000, 3.491481338843133355E-15 ) ) ;
#78299=DIRECTION ( 'NONE',  ( 0.000000000000000000, 1.000000000000000000, 0.000000000000000000 ) ) ;
#78300=EDGE_LOOP ( 'NONE', ( #31898, #3906, #68282, #42550 ) ) ;
#78302=CARTESIAN_POINT ( 'NONE',  ( -12.21159294319032362, -5.057305518903948638, 34.11320923018887896 ) ) ;
#78303=ORIENTED_EDGE ( 'NONE', *, *, #82296, .T. ) ;
#78304=FACE_OUTER_BOUND ( 'NONE', #7632, .T. ) ;
#78305=ADVANCED_FACE ( 'NONE', ( #18893 ), #5383, .F. ) ;
#78307=CARTESIAN_POINT ( 'NONE',  ( -16.15384615384615330, -9.819645486525091727, 36.12317359536749706 ) ) ;
#78308=ORIENTED_EDGE ( 'NONE', *, *, #75844, .F. ) ;
#78309=CARTESIAN_POINT ( 'NONE',  ( -9.019207500173124004, -10.66389620160130036, 33.62221079203477103 ) ) ;
#78311=CARTESIAN_POINT ( 'NONE',  ( 10.86543892702293057, -3.627508038966690496, 32.91356715214248396 ) ) ;
#78312=FACE_BOUND ( 'NONE', #70588, .T. ) ;
#78313=AXIS2_PLACEMENT_3D ( 'NONE', #62445, #81864, #33225 ) ;
#78314=CARTESIAN_POINT ( 'NONE',  ( -9.627052552794857831, -4.320704448112861584, 33.92786785259548310 ) ) ;
#78315=CARTESIAN_POINT ( 'NONE',  ( 3.903869409797562806, -2.318417181685854978, 30.59732222474233865 ) ) ;
#78316=AXIS2_PLACEMENT_3D ( 'NONE', #43693, #64395, #51761 ) ;
#78317=CARTESIAN_POINT ( 'NONE',  ( 8.703960323269994248, -2.625532179533445198, 30.86335684631481513 ) ) ;
#78319=CARTESIAN_POINT ( 'NONE',  ( -16.02305571287920216, -2.845873456487966635, 32.17976146951972538 ) ) ;
#78320=CARTESIAN_POINT ( 'NONE',  ( 11.53846153846153832, -11.16473453929635440, 33.15142922261926373 ) ) ;
#78323=DIRECTION ( 'NONE',  ( -0.000000000000000000, -0.9848077530122085754, -0.1736481776669273613 ) ) ;
#78325=ORIENTED_EDGE ( 'NONE', *, *, #88877, .F. ) ;
#78326=EDGE_CURVE ( 'NONE', #56176, #47929, #88979, .T. ) ;
#78327=CARTESIAN_POINT ( 'NONE',  ( 14.43821800945587697, -3.816742781228458448, 33.13167719472716044 ) ) ;
#78328=CARTESIAN_POINT ( 'NONE',  ( 15.16549923021291058, -3.083524468853724443, 32.58852847137143272 ) ) ;
#78329=B_SPLINE_CURVE_WITH_KNOTS ( 'NONE', 3,
 ( #15310, #903, #48196, #49084, #466, #21612, #76566, #14873, #69368, #21169 ),
 .UNSPECIFIED., .F., .F.,
 ( 4, 2, 2, 2, 4 ),
 ( 0.000000000000000000, 0.0001954311564186869286, 0.0003908623128373738573, 0.0005862934692560607588, 0.0007817246256747477145 ),
 .UNSPECIFIED. ) ;
#78330=CARTESIAN_POINT ( 'NONE',  ( 13.25392478150507891, -11.37499894934982692, 33.29245874905763003 ) ) ;
#78331=CARTESIAN_POINT ( 'NONE',  ( -14.24243673641628405, -2.892918686051626498, 31.69288490824026638 ) ) ;
#78332=CYLINDRICAL_SURFACE ( 'NONE', #83263, 0.2499999999999994726 ) ;
#78333=CARTESIAN_POINT ( 'NONE',  ( -2.372962308248626417, -11.67786785259541027, 32.92929555188721480 ) ) ;
#78334=EDGE_LOOP ( 'NONE', ( #39793, #83083 ) ) ;
#78335=CARTESIAN_POINT ( 'NONE',  ( -1.384615384615383471, -13.78497067705608181, 32.30358669280327177 ) ) ;
#78336=CARTESIAN_POINT ( 'NONE',  ( -14.98082371242109012, -10.05730279482229683, 34.04704008940765902 ) ) ;
#78337=CARTESIAN_POINT ( 'NONE',  ( -12.46153846153846168, -11.35647404775217417, 33.31231777344666511 ) ) ;
#78338=LINE ( 'NONE', #16640, #2189 ) ;
#78341=VERTEX_POINT ( 'NONE', #59430 ) ;
#78342=ORIENTED_EDGE ( 'NONE', *, *, #32713, .F. ) ;
#78343=EDGE_CURVE ( 'NONE', #14645, #40586, #6202, .T. ) ;
#78345=EDGE_LOOP ( 'NONE', ( #68237, #41079 ) ) ;
#78346=DIRECTION ( 'NONE',  ( -0.000000000000000000, 0.5000000000000011102, -0.8660254037844381525 ) ) ;
#78347=CARTESIAN_POINT ( 'NONE',  ( 17.77651507543566822, -11.60425143139329940, 33.02411095842164457 ) ) ;
#78348=CARTESIAN_POINT ( 'NONE',  ( -16.37733109757010297, -2.847400154188068910, 31.58180166144859768 ) ) ;
#78349=EDGE_CURVE ( 'NONE', #70251, #87090, #18011, .T. ) ;
#78350=CARTESIAN_POINT ( 'NONE',  ( -15.16551365949320918, -2.892918686051626498, 31.69288490824026638 ) ) ;
#78352=FACE_OUTER_BOUND ( 'NONE', #77391, .T. ) ;
#78354=VERTEX_POINT ( 'NONE', #74285 ) ;
#78356=LINE ( 'NONE', #64391, #42503 ) ;
#78357=ORIENTED_EDGE ( 'NONE', *, *, #86033, .T. ) ;
#78358=CARTESIAN_POINT ( 'NONE',  ( 2.980792486720640788, -12.41104346484419452, 31.60698883733904196 ) ) ;
#78359=CARTESIAN_POINT ( 'NONE',  ( -13.38461538461538325, -9.584722331328613620, 36.20867863119891439 ) ) ;
#78360=CARTESIAN_POINT ( 'NONE',  ( -3.296039676730006196, -5.219633306516282545, 34.19971097300152252 ) ) ;
#78362=CARTESIAN_POINT ( 'NONE',  ( -5.999999999999998224, -4.661471528628507777, 34.16647553114623292 ) ) ;
#78363=EDGE_CURVE ( 'NONE', #33880, #38977, #83586, .T. ) ;
#78364=CARTESIAN_POINT ( 'NONE',  ( 9.561617089197383734, -4.684245665217972032, 34.18127051446801090 ) ) ;
#78365=CARTESIAN_POINT ( 'NONE',  ( -12.46153846153846168, -6.435427911321262684, 35.78748833219616898 ) ) ;
#78368=CARTESIAN_POINT ( 'NONE',  ( -16.40386937806761125, -9.356822207818511927, 34.66110646841856635 ) ) ;
#78369=CARTESIAN_POINT ( 'NONE',  ( 1.134592147322421196, -5.851115903089112003, 34.47074536777953568 ) ) ;
#78370=CARTESIAN_POINT ( 'NONE',  ( -13.38461538461550582, -9.442884908241554243, 34.35708131394783038 ) ) ;
#78373=CARTESIAN_POINT ( 'NONE',  ( 7.846153846153846700, -3.669653830205710676, 35.88435417666054406 ) ) ;
#78374=CARTESIAN_POINT ( 'NONE',  ( 8.703960768674448900, -10.33852847137145048, 34.16647553114627556 ) ) ;
#78375=ORIENTED_EDGE ( 'NONE', *, *, #51684, .T. ) ;
#78377=CARTESIAN_POINT ( 'NONE',  ( -15.23076923076935252, -4.320704448113951379, 33.92786785259630022 ) ) ;
#78378=ADVANCED_FACE ( 'NONE', ( #60760 ), #73393, .F. ) ;
#78380=DIRECTION ( 'NONE',  ( -0.000000000000000000, 0.9848077530122086864, -0.1736481776669273891 ) ) ;
#78381=EDGE_LOOP ( 'NONE', ( #61664, #57368, #73763, #69214 ) ) ;
#78382=CARTESIAN_POINT ( 'NONE',  ( 14.43821800945587519, -12.27024696741798770, 31.24895572276497546 ) ) ;
#78383=CARTESIAN_POINT ( 'NONE',  ( 3.100621261037534548, -4.299443229763728169, 33.91186481527756058 ) ) ;
#78384=EDGE_CURVE ( 'NONE', #45298, #55677, #20252, .T. ) ;
#78385=CARTESIAN_POINT ( 'NONE',  ( -0.4615384615384611200, -9.905515769479276145, 34.41647553114623292 ) ) ;
#78386=CARTESIAN_POINT ( 'NONE',  ( -13.38461538461538325, -12.62096338111211580, 30.90682066428153263 ) ) ;
#78388=DIRECTION ( 'NONE',  ( -0.000000000000000000, -0.9396926207859093161, -0.3420201433256663259 ) ) ;
#78390=ORIENTED_EDGE ( 'NONE', *, *, #33364, .T. ) ;
#78391=CARTESIAN_POINT ( 'NONE',  ( -17.93474486048716088, -12.16647553114626845, 32.15551576947920864 ) ) ;
#78392=CARTESIAN_POINT ( 'NONE',  ( 2.372947878968334479, -3.300289026998474817, 32.46337939537591666 ) ) ;
#78394=EDGE_CURVE ( 'NONE', #71169, #84435, #43842, .T. ) ;
#78395=B_SPLINE_CURVE_WITH_KNOTS ( 'NONE', 3,
 ( #56249, #83733, #63437, #9825, #1744, #77839, #23334, #71082, #43174, #29231 ),
 .UNSPECIFIED., .F., .F.,
 ( 4, 2, 2, 2, 4 ),
 ( 0.0007817246256747505334, 0.0009771112852218954894, 0.001172497944769040554, 0.001367884604316185618, 0.001563271263863330682 ),
 .UNSPECIFIED. ) ;
#78396=VECTOR ( 'NONE', #53493, 1000.000000000000114 ) ;
#78398=CARTESIAN_POINT ( 'NONE',  ( 11.53846153846153832, -8.318370150425687726, 35.83090037661290239 ) ) ;
#78399=B_SPLINE_CURVE_WITH_KNOTS ( 'NONE', 3,
 ( #83099, #35344, #15526, #1118, #22277, #49741, #22710, #674, #50172, #28140 ),
 .UNSPECIFIED., .F., .F.,
 ( 4, 2, 2, 2, 4 ),
 ( 0.000000000000000000, 0.0001954339857564126514, 0.0003908679715128183098, 0.0005863019572692239681, 0.0007817359430256294638 ),
 .UNSPECIFIED. ) ;
#78400=CYLINDRICAL_SURFACE ( 'NONE', #20725, 0.2500000000000012212 ) ;
#78401=DIRECTION ( 'NONE',  ( -0.000000000000000000, 0.8660254037844397068, -0.4999999999999978906 ) ) ;
#78402=CARTESIAN_POINT ( 'NONE',  ( -16.15384615384615330, -2.833524468853757305, 32.15551576947925838 ) ) ;
#78403=ORIENTED_EDGE ( 'NONE', *, *, #3064, .F. ) ;
#78404=EDGE_LOOP ( 'NONE', ( #7138, #6960 ) ) ;
#78405=FACE_BOUND ( 'NONE', #50173, .T. ) ;
#78406=ORIENTED_EDGE ( 'NONE', *, *, #40324, .T. ) ;
#78407=CARTESIAN_POINT ( 'NONE',  ( -7.976844449264153702, -5.496505350115501010, 34.60290016733514307 ) ) ;
#78409=CARTESIAN_POINT ( 'NONE',  ( 17.77651507543566822, -5.827078755546626354, 34.72654668319379567 ) ) ;
#78410=DIRECTION ( 'NONE',  ( 0.000000000000000000, 0.8660254037844377084, 0.5000000000000015543 ) ) ;
#78411=ORIENTED_EDGE ( 'NONE', *, *, #54732, .F. ) ;
#78412=VERTEX_POINT ( 'NONE', #84927 ) ;
#78413=AXIS2_PLACEMENT_3D ( 'NONE', #25598, #24244, #25148 ) ;
#78414=VERTEX_POINT ( 'NONE', #16896 ) ;
#78415=CARTESIAN_POINT ( 'NONE',  ( 3.480823542407546434, -4.943051570960395047, 34.04725096376909477 ) ) ;
#78416=ORIENTED_EDGE ( 'NONE', *, *, #6820, .F. ) ;
#78417=CARTESIAN_POINT ( 'NONE',  ( 16.15384615384603251, -10.21337939537710326, 33.94971097300076224 ) ) ;
#78418=EDGE_CURVE ( 'NONE', #19767, #42964, #78135, .T. ) ;
#78419=CARTESIAN_POINT ( 'NONE',  ( -15.23076923076935074, -6.879047030192662504, 34.71129190930017927 ) ) ;
#78420=B_SPLINE_CURVE_WITH_KNOTS ( 'NONE', 3,
 ( #69458, #47852, #55055, #14070, #6438, #21264, #26698, #41545, #76208, #75337 ),
 .UNSPECIFIED., .F., .F.,
 ( 4, 2, 2, 2, 4 ),
 ( 0.0007817359527651104954, 0.0009771254036996493593, 0.001172514854634188223, 0.001367904305568727087, 0.001563293756503265951 ),
 .UNSPECIFIED. ) ;
#78421=DIRECTION ( 'NONE',  ( 0.000000000000000000, 0.9848077530122072432, -0.1736481776669354937 ) ) ;
#78422=EDGE_CURVE ( 'NONE', #38805, #31074, #38424, .T. ) ;
#78423=FACE_BOUND ( 'NONE', #72578, .T. ) ;
#78424=VERTEX_POINT ( 'NONE', #1164 ) ;
#78425=B_SPLINE_CURVE_WITH_KNOTS ( 'NONE', 3,
 ( #26795, #12834, #47500, #54699, #18720, #67343, #13279, #74992, #87628, #32660 ),
 .UNSPECIFIED., .F., .F.,
 ( 4, 2, 2, 2, 4 ),
 ( 0.000000000000000000, 0.0001954339857564079352, 0.0003908679715128158703, 0.0005863019572692237513, 0.0007817359430256317406 ),
 .UNSPECIFIED. ) ;
#78426=CARTESIAN_POINT ( 'NONE',  ( 13.25446741488368829, -11.04286588640298561, 33.62463336215343901 ) ) ;
#78427=EDGE_CURVE ( 'NONE', #46262, #26954, #30413, .T. ) ;
#78428=CARTESIAN_POINT ( 'NONE',  ( -14.05763799605399278, -5.728107161865378494, 34.42597550085002922 ) ) ;
#78429=CARTESIAN_POINT ( 'NONE',  ( -11.53846153846153655, -2.833524468853757305, 32.15551576947925838 ) ) ;
#78430=CARTESIAN_POINT ( 'NONE',  ( -1.253824943648434109, -2.845873456487965747, 32.17976146951972538 ) ) ;
#78431=ORIENTED_EDGE ( 'NONE', *, *, #84734, .T. ) ;
#78433=ORIENTED_EDGE ( 'NONE', *, *, #20139, .F. ) ;
#78434=ORIENTED_EDGE ( 'NONE', *, *, #20750, .F. ) ;
#78435=EDGE_CURVE ( 'NONE', #25168, #67178, #15132, .T. ) ;
#78437=DIRECTION ( 'NONE',  ( -0.000000000000000000, -0.1736481776669307198, -0.9848077530122080203 ) ) ;
#78438=CYLINDRICAL_SURFACE ( 'NONE', #6828, 0.2500000000000002220 ) ;
#78439=CARTESIAN_POINT ( 'NONE',  ( -3.930834802233302394, -4.187068189119697692, 33.49521262558774026 ) ) ;
#78440=CARTESIAN_POINT ( 'NONE',  ( 17.29988598048456439, -7.369474270740072441, 34.74850911626239736 ) ) ;
#78441=CYLINDRICAL_SURFACE ( 'NONE', #73540, 0.2499999999999973355 ) ;
#78442=EDGE_LOOP ( 'NONE', ( #55154, #55042, #63266, #36665 ) ) ;
#78443=CARTESIAN_POINT ( 'NONE',  ( 6.792386319966619013, -2.494641256782728966, 31.33461815524612959 ) ) ;
#78444=CARTESIAN_POINT ( 'NONE',  ( 17.99999999999987566, -3.643525952248796163, 33.31231777344771672 ) ) ;
#78445=CARTESIAN_POINT ( 'NONE',  ( -0.4615384615384611200, -4.945431358278436385, 36.03766855953609394 ) ) ;
#78446=CARTESIAN_POINT ( 'NONE',  ( 14.53047197667036805, -2.612705202774698421, 31.66806509827799943 ) ) ;
#78447=VERTEX_POINT ( 'NONE', #28646 ) ;
#78448=VERTEX_POINT ( 'NONE', #64179 ) ;
#78449=FACE_BOUND ( 'NONE', #50116, .T. ) ;
#78450=CARTESIAN_POINT ( 'NONE',  ( 11.78851595837499211, -12.41089969410671223, 31.60739465890703670 ) ) ;
#78451=CARTESIAN_POINT ( 'NONE',  ( -11.31568199719312773, -11.89424750095246175, 32.13594075562311758 ) ) ;
#78452=EDGE_LOOP ( 'NONE', ( #33688, #54657, #77148, #84479 ) ) ;
#78454=CARTESIAN_POINT ( 'NONE',  ( 9.692307692307695177, -1.044019251281081972, 31.83374038241031911 ) ) ;
#78455=CARTESIAN_POINT ( 'NONE',  ( -2.241623956689868358, -4.098570777380720287, 33.41473453929635440 ) ) ;
#78456=FACE_OUTER_BOUND ( 'NONE', #2981, .T. ) ;
#78457=EDGE_CURVE ( 'NONE', #5283, #32510, #55638, .T. ) ;
#78458=CARTESIAN_POINT ( 'NONE',  ( -0.4615384615384611200, -2.249999999999998668, 29.75000000000001776 ) ) ;
#78459=VERTEX_POINT ( 'NONE', #49358 ) ;
#78460=CARTESIAN_POINT ( 'NONE',  ( -7.596099534515528440, -10.66356715214248752, 33.62249196103329751 ) ) ;
#78461=ORIENTED_EDGE ( 'NONE', *, *, #5763, .T. ) ;
#78462=CARTESIAN_POINT ( 'NONE',  ( 13.60762822870878352, -8.282913670948747864, 34.94150082978203642 ) ) ;
#78463=EDGE_LOOP ( 'NONE', ( #67900, #17275 ) ) ;
#78464=CARTESIAN_POINT ( 'NONE',  ( 15.48082354240754555, -8.303483539816731707, 34.68545999027711702 ) ) ;
#78465=CARTESIAN_POINT ( 'NONE',  ( 15.00728430620490172, -4.988325925672468131, 34.36044203135681130 ) ) ;
#78466=DIRECTION ( 'NONE',  ( 1.000000000000000000, 0.000000000000000000, 0.000000000000000000 ) ) ;
#78467=CARTESIAN_POINT ( 'NONE',  ( -14.98076923076781064, -7.500000000000154543, 35.00000000000007105 ) ) ;
#78469=B_SPLINE_CURVE_WITH_KNOTS ( 'NONE', 3,
 ( #30054, #57519, #83686, #8461, #51175, #69707, #29618, #23286, #15658, #78681 ),
 .UNSPECIFIED., .F., .F.,
 ( 4, 2, 2, 2, 4 ),
 ( 0.0007817246256747476061, 0.0009771112852218911526, 0.001172497944769034916, 0.001367884604316178462, 0.001563271263863322009 ),
 .UNSPECIFIED. ) ;
#78470=CARTESIAN_POINT ( 'NONE',  ( -1.384615384615383471, -12.37446782046654192, 30.86335684631486131 ) ) ;
#78471=B_SPLINE_CURVE_WITH_KNOTS ( 'NONE', 3,
 ( #61957, #12018, #88582, #75048, #81363, #13774, #47997, #6138, #25960, #80474 ),
 .UNSPECIFIED., .F., .F.,
 ( 4, 2, 2, 2, 4 ),
 ( 0.0007817246256747494492, 0.0009771112852218935378, 0.001172497944769037518, 0.001367884604316181498, 0.001563271263863325695 ),
 .UNSPECIFIED. ) ;
#78473=ORIENTED_EDGE ( 'NONE', *, *, #59061, .F. ) ;
#78474=B_SPLINE_CURVE_WITH_KNOTS ( 'NONE', 3,
 ( #3021, #22856, #71933, #15675, #43142, #16545, #57973, #10244, #77803, #64721 ),
 .UNSPECIFIED., .F., .F.,
 ( 4, 2, 2, 2, 4 ),
 ( 0.0007817359430256320659, 0.0009771253907249987086, 0.001172514838424365460, 0.001367904286123731994, 0.001563293733823098745 ),
 .UNSPECIFIED. ) ;
#78475=DIRECTION ( 'NONE',  ( -0.000000000000000000, 0.1736481776669307198, -0.9848077530122080203 ) ) ;
#78476=CARTESIAN_POINT ( 'NONE',  ( -3.230769230769352962, -12.51329471203414379, 31.30864560766407578 ) ) ;
#78477=VECTOR ( 'NONE', #10117, 1000.000000000000114 ) ;
#78479=ORIENTED_EDGE ( 'NONE', *, *, #75807, .T. ) ;
#78480=CARTESIAN_POINT ( 'NONE',  ( 10.61538461538461675, -8.164416787775445883, 34.95778746994557906 ) ) ;
#78482=CARTESIAN_POINT ( 'NONE',  ( 6.066068351002440906, -11.16473453929635440, 33.15142922261926373 ) ) ;
#78483=AXIS2_PLACEMENT_3D ( 'NONE', #41175, #20010, #6938 ) ;
#78484=CARTESIAN_POINT ( 'NONE',  ( 0.5266832422580927098, -7.750023224968865421, 34.99404313364389907 ) ) ;
#78485=CARTESIAN_POINT ( 'NONE',  ( 10.55011416942384272, -4.481592998940162609, 33.73612834413957984 ) ) ;
#78487=CARTESIAN_POINT ( 'NONE',  ( -7.846153846153844924, -1.422936976036506707, 30.56769352161908415 ) ) ;
#78488=ORIENTED_EDGE ( 'NONE', *, *, #38199, .F. ) ;
#78489=CARTESIAN_POINT ( 'NONE',  ( 6.000000000000001776, -10.51840700105979565, 33.73612834413961536 ) ) ;
#78490=CARTESIAN_POINT ( 'NONE',  ( -17.32692307692307665, -7.500000000000001776, 34.75000000000000000 ) ) ;
#78491=EDGE_CURVE ( 'NONE', #50611, #83181, #8374, .T. ) ;
#78492=CARTESIAN_POINT ( 'NONE',  ( -3.230769230769229949, -2.486705287966279876, 31.30864560766543647 ) ) ;
#78494=EDGE_LOOP ( 'NONE', ( #85494, #84075, #30892, #72587 ) ) ;
#78496=ADVANCED_FACE ( 'NONE', ( #1613 ), #29101, .F. ) ;
#78497=ORIENTED_EDGE ( 'NONE', *, *, #57673, .F. ) ;
#78498=CARTESIAN_POINT ( 'NONE',  ( 12.21151523731700372, -9.356822207818506598, 34.66110646841856635 ) ) ;
#78499=CARTESIAN_POINT ( 'NONE',  ( -3.230769230769229949, -2.721908614388771852, 31.22303859784724978 ) ) ;
#78500=CARTESIAN_POINT ( 'NONE',  ( 6.000000000000001776, -12.62096338111211580, 30.90682066428153263 ) ) ;
#78501=EDGE_LOOP ( 'NONE', ( #12631, #23132 ) ) ;
#78502=EDGE_CURVE ( 'NONE', #20537, #18188, #9393, .T. ) ;
#78504=CARTESIAN_POINT ( 'NONE',  ( -10.61538461538461320, -10.51840700105979565, 33.73612834413961536 ) ) ;
#78505=B_SPLINE_CURVE_WITH_KNOTS ( 'NONE', 3,
 ( #54197, #13229, #53762, #46123, #5136, #80365, #25407, #33934, #19536, #60071 ),
 .UNSPECIFIED., .F., .F.,
 ( 4, 2, 2, 2, 4 ),
 ( 0.0007817359430256392216, 0.0009771253907250080327, 0.001172514838424376952, 0.001367904286123745872, 0.001563293733823114791 ),
 .UNSPECIFIED. ) ;
#78506=DIRECTION ( 'NONE',  ( -0.000000000000000000, 0.1736481776669307198, -0.9848077530122080203 ) ) ;
#78507=EDGE_CURVE ( 'NONE', #51867, #18418, #7319, .T. ) ;
#78508=B_SPLINE_CURVE_WITH_KNOTS ( 'NONE', 3,
 ( #229, #26815, #34008, #53840, #61473, #41661, #69129, #33126, #87647, #25924 ),
 .UNSPECIFIED., .F., .F.,
 ( 4, 2, 2, 2, 4 ),
 ( 0.000000000000000000, 0.0001954311564186861697, 0.0003908623128373723394, 0.0005862934692560584820, 0.0007817246256747446788 ),
 .UNSPECIFIED. ) ;
#78509=B_SPLINE_CURVE_WITH_KNOTS ( 'NONE', 3,
 ( #25209, #87373, #81498, #53109, #52671, #87829, #32855, #19344, #80615, #5828 ),
 .UNSPECIFIED., .F., .F.,
 ( 4, 2, 2, 2, 4 ),
 ( 0.000000000000000000, 0.0001954339857564090194, 0.0003908679715128180387, 0.0005863019572692270039, 0.0007817359430256360774 ),
 .UNSPECIFIED. ) ;
#78510=CARTESIAN_POINT ( 'NONE',  ( -9.469294848214296678, -3.395485233115139057, 33.02377354290275946 ) ) ;
#78511=B_SPLINE_CURVE_WITH_KNOTS ( 'NONE', 3,
 ( #46805, #86934, #5822, #24752, #33300, #74283, #25200, #25647, #67525, #18891 ),
 .UNSPECIFIED., .F., .F.,
 ( 4, 2, 2, 2, 4 ),
 ( 0.000000000000000000, 0.0001954311564186863052, 0.0003908623128373726104, 0.0005862934692560589156, 0.0007817246256747452209 ),
 .UNSPECIFIED. ) ;
#78512=VERTEX_POINT ( 'NONE', #66421 ) ;
#78513=CARTESIAN_POINT ( 'NONE',  ( -14.30769230769230660, -13.75783147151868846, 33.36296068462461051 ) ) ;
#78515=ADVANCED_FACE ( 'NONE', ( #72279 ), #10592, .F. ) ;
#78517=CARTESIAN_POINT ( 'NONE',  ( -16.15384615384615330, -11.16473453929635440, 33.15142922261926373 ) ) ;
#78518=DIRECTION ( 'NONE',  ( -0.000000000000000000, 1.000000000000000000, 3.491481338843133355E-15 ) ) ;
#78519=VECTOR ( 'NONE', #95, 1000.000000000000227 ) ;
#78520=CARTESIAN_POINT ( 'NONE',  ( -9.942284436356283450, -8.347322224742351082, 34.93158281831414058 ) ) ;
#78521=CARTESIAN_POINT ( 'NONE',  ( 16.08776377448601025, -11.91647553114624181, 32.58852847137148245 ) ) ;
#78522=ORIENTED_EDGE ( 'NONE', *, *, #84019, .T. ) ;
#78523=ORIENTED_EDGE ( 'NONE', *, *, #61888, .F. ) ;
#78524=VERTEX_POINT ( 'NONE', #65522 ) ;
#78525=VERTEX_POINT ( 'NONE', #79937 ) ;
#78526=CARTESIAN_POINT ( 'NONE',  ( -10.61538461538461320, -8.120952969808772792, 34.71129190930000163 ) ) ;
#78528=CARTESIAN_POINT ( 'NONE',  ( -15.23076923076922995, -8.973038597847269315, 34.52809138561121927 ) ) ;
#78529=ADVANCED_FACE ( 'NONE', ( #71835 ), #65964, .F. ) ;
#78530=CARTESIAN_POINT ( 'NONE',  ( -4.283994123577850921, -12.50552854090298993, 31.33409797877408920 ) ) ;
#78531=CARTESIAN_POINT ( 'NONE',  ( -13.51476335434707821, -3.625366637846544116, 33.29286588640298561 ) ) ;
#78532=CARTESIAN_POINT ( 'NONE',  ( 3.007843013253083786, -5.667676309546437530, 34.40238873228292249 ) ) ;
#78533=ADVANCED_FACE ( 'NONE', ( #30847 ), #85810, .F. ) ;
#78534=CARTESIAN_POINT ( 'NONE',  ( -17.77722045873158763, -10.11255958852956027, 34.01340905677048454 ) ) ;
#78535=CARTESIAN_POINT ( 'NONE',  ( -5.142173008697161762, -2.255955759149247619, 30.00000000000013856 ) ) ;
#78536=ORIENTED_EDGE ( 'NONE', *, *, #39496, .F. ) ;
#78537=VERTEX_POINT ( 'NONE', #79496 ) ;
#78539=ORIENTED_EDGE ( 'NONE', *, *, #15160, .T. ) ;
#78540=CARTESIAN_POINT ( 'NONE',  ( 11.53846153846153832, -2.486705287966279876, 31.30864560766543647 ) ) ;
#78542=ORIENTED_EDGE ( 'NONE', *, *, #79821, .T. ) ;
#78543=CARTESIAN_POINT ( 'NONE',  ( 0.7115927731767760500, -8.303483539816728154, 34.68545999027711702 ) ) ;
#78544=CARTESIAN_POINT ( 'NONE',  ( -17.77698715590659972, -11.43677907613344757, 33.22367315496203588 ) ) ;
#78545=DIRECTION ( 'NONE',  ( 0.000000000000000000, 0.8660254037844377084, -0.5000000000000015543 ) ) ;
#78546=CARTESIAN_POINT ( 'NONE',  ( 4.284371855609715674, -2.619367082507848554, 30.83698974864644171 ) ) ;
#78548=EDGE_CURVE ( 'NONE', #80310, #45473, #34107, .T. ) ;
#78549=ORIENTED_EDGE ( 'NONE', *, *, #68012, .F. ) ;
#78550=CARTESIAN_POINT ( 'NONE',  ( -9.692307692307691624, -12.10708131394839349, 31.69288490824020244 ) ) ;
#78551=ORIENTED_EDGE ( 'NONE', *, *, #5225, .T. ) ;
#78552=FACE_BOUND ( 'NONE', #59925, .T. ) ;
#78553=CARTESIAN_POINT ( 'NONE',  ( 13.44987052412822059, -12.51329471203373345, 31.30864560766537963 ) ) ;
#78554=CARTESIAN_POINT ( 'NONE',  ( -14.43838291080261627, -6.369640206132551441, 34.87707690430378449 ) ) ;
#78555=VERTEX_POINT ( 'NONE', #72723 ) ;
#78556=CARTESIAN_POINT ( 'NONE',  ( -0.2115384615384616196, -2.249999999999998668, 29.75000000000000355 ) ) ;
#78557=CARTESIAN_POINT ( 'NONE',  ( 11.47237915910140771, -6.343179335718451384, 34.87096338111212646 ) ) ;
#78558=CARTESIAN_POINT ( 'NONE',  ( -9.692307692307691624, -2.708943851104267164, 35.45975837776705220 ) ) ;
#78559=VERTEX_POINT ( 'NONE', #4726 ) ;
#78560=CARTESIAN_POINT ( 'NONE',  ( -5.076923076923075762, -1.466349020453238561, 30.81389545987213907 ) ) ;
#78561=CARTESIAN_POINT ( 'NONE',  ( 1.607395053593451140, -2.612705202774697533, 31.66806509827799943 ) ) ;
#78563=ORIENTED_EDGE ( 'NONE', *, *, #21103, .T. ) ;
#78564=B_SPLINE_CURVE_WITH_KNOTS ( 'NONE', 3,
 ( #32562, #60035, #87541, #25817, #74009, #19059, #12300, #67249, #56711, #16603 ),
 .UNSPECIFIED., .F., .F.,
 ( 4, 2, 2, 2, 4 ),
 ( 0.0007817359430256252354, 0.0009771253907249898181, 0.001172514838424354401, 0.001367904286123718983, 0.001563293733823083566 ),
 .UNSPECIFIED. ) ;
#78565=EDGE_CURVE ( 'NONE', #75626, #16317, #63128, .T. ) ;
#78566=CARTESIAN_POINT ( 'NONE',  ( 3.480823542407546434, -8.303483539816728154, 34.68545999027711702 ) ) ;
#78567=CARTESIAN_POINT ( 'NONE',  ( -9.627052552794857831, -9.528491918058460186, 34.59228464037086326 ) ) ;
#78568=CARTESIAN_POINT ( 'NONE',  ( 24.00000000000000000, -5.499999999999981348, 27.75000000000000000 ) ) ;
#78569=CARTESIAN_POINT ( 'NONE',  ( -7.623142494540996239, -6.503523203565941380, 34.64991518177335195 ) ) ;
#78570=CARTESIAN_POINT ( 'NONE',  ( -16.08777780284371772, -8.120952969808772792, 34.71129190929999453 ) ) ;
#78571=CARTESIAN_POINT ( 'NONE',  ( -10.61538461538461320, -5.557115091759785130, 34.35708131394839171 ) ) ;
#78572=CYLINDRICAL_SURFACE ( 'NONE', #4190, 0.2499999999999979738 ) ;
#78573=EDGE_CURVE ( 'NONE', #76766, #58189, #35223, .T. ) ;
#78574=CARTESIAN_POINT ( 'NONE',  ( 7.846153846153846700, -2.833524468853757305, 32.15551576947925838 ) ) ;
#78575=CARTESIAN_POINT ( 'NONE',  ( 4.153846153846032507, -12.27809138561165270, 31.22303859784587132 ) ) ;
#78576=CARTESIAN_POINT ( 'NONE',  ( 17.07692307692307665, -3.937682226553329556, 33.60647404775216529 ) ) ;
#78577=CARTESIAN_POINT ( 'NONE',  ( 1.634560902963529738, -11.37275283266503756, 32.91324779482534524 ) ) ;
#78578=CARTESIAN_POINT ( 'NONE',  ( 12.71153846153988098, -7.500000000000154543, 35.00000000000007105 ) ) ;
#78579=CARTESIAN_POINT ( 'NONE',  ( -10.74607608205217346, -8.147922237126337563, 34.70805685702651999 ) ) ;
#78580=CARTESIAN_POINT ( 'NONE',  ( -2.437840277424001112, -5.915902021225892149, 34.75552854090298638 ) ) ;
#78583=ORIENTED_EDGE ( 'NONE', *, *, #6917, .T. ) ;
#78586=CARTESIAN_POINT ( 'NONE',  ( -5.076923076923197442, -10.90142922262034020, 33.41473453929536674 ) ) ;
#78587=ORIENTED_EDGE ( 'NONE', *, *, #2709, .T. ) ;
#78588=CARTESIAN_POINT ( 'NONE',  ( -4.023320452082591814, -11.46989282347013095, 32.79007818306219946 ) ) ;
#78589=VECTOR ( 'NONE', #80507, 1000.000000000000114 ) ;
#78590=ORIENTED_EDGE ( 'NONE', *, *, #57181, .T. ) ;
#78591=CARTESIAN_POINT ( 'NONE',  ( 5.777073041093149897, -10.77366814457252175, 33.85459836347579454 ) ) ;
#78594=CARTESIAN_POINT ( 'NONE',  ( 9.757563263583717728, -11.48612834413965977, 32.76840700105972815 ) ) ;
#78595=CARTESIAN_POINT ( 'NONE',  ( 7.053867364043872712, -9.929761469519744921, 34.40412654351204225 ) ) ;
#78596=DIRECTION ( 'NONE',  ( -0.000000000000000000, 0.8660254037844399289, -0.4999999999999980016 ) ) ;
#78598=CARTESIAN_POINT ( 'NONE',  ( -7.780085495151407571, -2.721908614388772296, 31.22303859784725333 ) ) ;
#78599=CARTESIAN_POINT ( 'NONE',  ( 0.6845513056318561773, -2.523321265292116422, 31.42251411153756990 ) ) ;
#78601=CARTESIAN_POINT ( 'NONE',  ( 18.25005441991345378, -11.47946981652013498, 33.17500667209846910 ) ) ;
#78602=CARTESIAN_POINT ( 'NONE',  ( 7.846153846153846700, -12.10708131394839349, 31.69288490824020244 ) ) ;
#78603=CARTESIAN_POINT ( 'NONE',  ( 13.44987095589141468, -4.481592998940250538, 33.73612834413965089 ) ) ;
#78604=B_SPLINE_CURVE_WITH_KNOTS ( 'NONE', 3,
 ( #46949, #47395, #35215, #82540, #88860, #74889, #7755, #14060, #553, #74436 ),
 .UNSPECIFIED., .F., .F.,
 ( 4, 2, 2, 2, 4 ),
 ( 0.0007817246256747483650, 0.0009771112852218926705, 0.001172497944769037084, 0.001367884604316181498, 0.001563271263863325695 ),
 .UNSPECIFIED. ) ;
#78606=B_SPLINE_CURVE_WITH_KNOTS ( 'NONE', 3,
 ( #27445, #47263, #75195, #13922, #40528, #20247, #68865, #6723, #81959, #76065 ),
 .UNSPECIFIED., .F., .F.,
 ( 4, 2, 2, 2, 4 ),
 ( 0.0007817246256747459798, 0.0009771112852218896347, 0.001172497944769033398, 0.001367884604316177161, 0.001563271263863320708 ),
 .UNSPECIFIED. ) ;
#78608=B_SPLINE_CURVE_WITH_KNOTS ( 'NONE', 3,
 ( #277, #82705, #20976, #35390, #76831, #48449, #75935, #41709, #69179, #34940 ),
 .UNSPECIFIED., .F., .F.,
 ( 4, 2, 2, 2, 4 ),
 ( 0.000000000000000000, 0.0001954339857564090194, 0.0003908679715128180387, 0.0005863019572692270039, 0.0007817359430256360774 ),
 .UNSPECIFIED. ) ;
#78609=DIRECTION ( 'NONE',  ( -0.000000000000000000, -0.000000000000000000, -1.000000000000000000 ) ) ;
#78610=CARTESIAN_POINT ( 'NONE',  ( 11.66898724022510514, -6.001044277235009439, 34.52024696741798948 ) ) ;
#78611=DIRECTION ( 'NONE',  ( -0.000000000000000000, -0.7660444431189791237, -0.6427876096865379196 ) ) ;
#78612=CARTESIAN_POINT ( 'NONE',  ( 15.93096663710857186, -7.630690623152299956, 34.99857592706774057 ) ) ;
#78614=AXIS2_PLACEMENT_3D ( 'NONE', #5966, #75737, #46500 ) ;
#78615=CARTESIAN_POINT ( 'NONE',  ( -14.24162497434223340, -3.937682226553329556, 33.60647404775216529 ) ) ;
#78618=ORIENTED_EDGE ( 'NONE', *, *, #75633, .F. ) ;
#78619=CARTESIAN_POINT ( 'NONE',  ( -10.36538461538319389, -7.500000000000154543, 35.00000000000007105 ) ) ;
#78621=EDGE_CURVE ( 'NONE', #29336, #72117, #52462, .T. ) ;
#78622=VERTEX_POINT ( 'NONE', #81278 ) ;
#78623=CARTESIAN_POINT ( 'NONE',  ( 7.623226887246995709, -10.77366814457251998, 33.85459836347579454 ) ) ;
#78624=CARTESIAN_POINT ( 'NONE',  ( 18.25000000000000000, -2.249999999999998668, 29.75000000000000355 ) ) ;
#78625=DIRECTION ( 'NONE',  ( 0.000000000000000000, 0.1736481776669275834, 0.9848077530122086864 ) ) ;
#78626=CARTESIAN_POINT ( 'NONE',  ( 2.307692307692187583, -6.026961402154118908, 34.52809138561165270 ) ) ;
#78627=CARTESIAN_POINT ( 'NONE',  ( -5.299850035829924089, -8.282780595021769443, 34.94152052738834868 ) ) ;
#78629=EDGE_CURVE ( 'NONE', #23503, #82006, #15941, .T. ) ;
#78631=ORIENTED_EDGE ( 'NONE', *, *, #54144, .T. ) ;
#78633=VERTEX_POINT ( 'NONE', #26322 ) ;
#78634=B_SPLINE_CURVE_WITH_KNOTS ( 'NONE', 3,
 ( #51940, #11414, #17735, #37999, #3761, #86204, #79876, #78531, #58705, #45187 ),
 .UNSPECIFIED., .F., .F.,
 ( 4, 2, 2, 2, 4 ),
 ( 0.000000000000000000, 0.0001954311564186858715, 0.0003908623128373717431, 0.0005862934692560576146, 0.0007817246256747434861 ),
 .UNSPECIFIED. ) ;
#78635=B_SPLINE_CURVE_WITH_KNOTS ( 'NONE', 3,
 ( #41569, #55521, #7350, #83007, #34805, #62272, #588, #21289, #48763, #76234 ),
 .UNSPECIFIED., .F., .F.,
 ( 4, 2, 2, 2, 4 ),
 ( 0.0007817359430256323911, 0.0009771253907249991422, 0.001172514838424365893, 0.001367904286123732644, 0.001563293733823099396 ),
 .UNSPECIFIED. ) ;
#78636=CARTESIAN_POINT ( 'NONE',  ( 18.13052543823364360, -2.372941743896878286, 30.88044141588253311 ) ) ;
#78637=FACE_OUTER_BOUND ( 'NONE', #65554, .T. ) ;
#78638=B_SPLINE_CURVE_WITH_KNOTS ( 'NONE', 3,
 ( #6238, #32814, #68368, #48088, #6667, #61606, #89111, #13865, #18856, #41346 ),
 .UNSPECIFIED., .F., .F.,
 ( 4, 2, 2, 2, 4 ),
 ( 0.0007817246256747474977, 0.0009771112852218909357, 0.001172497944769034482, 0.001367884604316178029, 0.001563271263863321575 ),
 .UNSPECIFIED. ) ;
#78639=AXIS2_PLACEMENT_3D ( 'NONE', #54365, #4407, #66101 ) ;
#78641=CYLINDRICAL_SURFACE ( 'NONE', #12066, 0.2500000000000009437 ) ;
#78642=DIRECTION ( 'NONE',  ( 0.000000000000000000, 0.000000000000000000, -1.000000000000000000 ) ) ;
#78644=EDGE_CURVE ( 'NONE', #13666, #5455, #5080, .T. ) ;
#78645=DIRECTION ( 'NONE',  ( -0.000000000000000000, 0.3420201433256694346, -0.9396926207859080948 ) ) ;
#78646=AXIS2_PLACEMENT_3D ( 'NONE', #42306, #35538, #69759 ) ;
#78648=ORIENTED_EDGE ( 'NONE', *, *, #80548, .F. ) ;
#78651=LINE ( 'NONE', #32251, #84743 ) ;
#78652=ORIENTED_EDGE ( 'NONE', *, *, #24124, .F. ) ;
#78653=CARTESIAN_POINT ( 'NONE',  ( 12.46153846153846168, -13.20930481340135110, 34.54067556320372745 ) ) ;
#78655=CARTESIAN_POINT ( 'NONE',  ( 6.000000000000001776, -6.681629849574314051, 35.83090037661290239 ) ) ;
#78656=EDGE_LOOP ( 'NONE', ( #48829, #65847, #37744, #82196 ) ) ;
#78657=EDGE_CURVE ( 'NONE', #31669, #15410, #64238, .T. ) ;
#78658=CARTESIAN_POINT ( 'NONE',  ( -14.55771553191376100, -12.45566812827425451, 31.48439005359158926 ) ) ;
#78659=EDGE_LOOP ( 'NONE', ( #74991, #12798, #88026, #87670 ) ) ;
#78660=CARTESIAN_POINT ( 'NONE',  ( -9.019207513279361876, -4.818429247618089661, 34.26397095200675125 ) ) ;
#78662=FACE_OUTER_BOUND ( 'NONE', #82362, .T. ) ;
#78663=CARTESIAN_POINT ( 'NONE',  ( 6.000000000000001776, -12.34228464037088635, 31.77849191805839268 ) ) ;
#78666=CARTESIAN_POINT ( 'NONE',  ( 5.010839665967194989, -2.538708090699994813, 30.37095296980875148 ) ) ;
#78667=CARTESIAN_POINT ( 'NONE',  ( 17.07692307692307665, -2.292212530054420494, 30.41441678777542634 ) ) ;
#78668=ORIENTED_EDGE ( 'NONE', *, *, #54075, .F. ) ;
#78669=CARTESIAN_POINT ( 'NONE',  ( -18.22348494372394967, -10.81261337010820256, 33.49550067578627477 ) ) ;
#78671=EDGE_CURVE ( 'NONE', #12765, #8388, #32045, .T. ) ;
#78672=ORIENTED_EDGE ( 'NONE', *, *, #52098, .T. ) ;
#78673=B_SPLINE_CURVE_WITH_KNOTS ( 'NONE', 3,
 ( #11322, #66263, #4567, #59508, #87012, #25284, #73484, #11776, #80693, #18975 ),
 .UNSPECIFIED., .F., .F.,
 ( 4, 2, 2, 2, 4 ),
 ( 0.000000000000000000, 0.0001954339857564092362, 0.0003908679715128184724, 0.0005863019572692276544, 0.0007817359430256369448 ),
 .UNSPECIFIED. ) ;
#78675=B_SPLINE_CURVE_WITH_KNOTS ( 'NONE', 3,
 ( #65467, #73578, #86653, #85747, #18176, #52835, #24922, #51939, #44282, #45186 ),
 .UNSPECIFIED., .F., .F.,
 ( 4, 2, 2, 2, 4 ),
 ( 0.0007817359430256282712, 0.0009771253907249945886, 0.001172514838424360689, 0.001367904286123726790, 0.001563293733823093107 ),
 .UNSPECIFIED. ) ;
#78676=CARTESIAN_POINT ( 'NONE',  ( 6.989145274079363368, -2.721908614388772296, 31.22303859784725333 ) ) ;
#78677=DIRECTION ( 'NONE',  ( -0.000000000000000000, -0.9396926207859092051, -0.3420201433256662704 ) ) ;
#78678=CARTESIAN_POINT ( 'NONE',  ( -4.153846153846152411, -2.538708090699994813, 30.37095296980875503 ) ) ;
#78679=CARTESIAN_POINT ( 'NONE',  ( -39.05038313613820122, -2.249999999999998668, 29.75000000000000355 ) ) ;
#78680=B_SPLINE_CURVE_WITH_KNOTS ( 'NONE', 3,
 ( #59095, #3261, #45137, #85692, #38390, #72611 ),
 .UNSPECIFIED., .F., .F.,
 ( 4, 2, 4 ),
 ( 0.0003909569690057869895, 0.0005862646681846149206, 0.0007815723673634428518 ),
 .UNSPECIFIED. ) ;
#78681=CARTESIAN_POINT ( 'NONE',  ( 7.846153846153846700, -6.343179335718451384, 34.87096338111211935 ) ) ;
#78683=CARTESIAN_POINT ( 'NONE',  ( 12.39626801557768943, -4.481592998940162609, 33.73612834413957984 ) ) ;
#78684=EDGE_CURVE ( 'NONE', #29891, #8133, #84708, .T. ) ;
#78685=FACE_BOUND ( 'NONE', #12700, .T. ) ;
#78686=CARTESIAN_POINT ( 'NONE',  ( 5.076923076922953193, -5.941354392335915335, 34.76329471203413846 ) ) ;
#78688=VECTOR ( 'NONE', #24201, 1000.000000000000227 ) ;
#78689=CARTESIAN_POINT ( 'NONE',  ( 15.90382291655318880, -3.202444869320336451, 32.30641848906366675 ) ) ;
#78690=CARTESIAN_POINT ( 'NONE',  ( -10.61538461538461320, -13.87047571288749737, 32.06866353760679544 ) ) ;
#78692=CYLINDRICAL_SURFACE ( 'NONE', #5323, 0.2499999999999995559 ) ;
#78693=CARTESIAN_POINT ( 'NONE',  ( 8.835299120233207404, -10.51840700105979565, 33.73612834413962247 ) ) ;
#78695=VERTEX_POINT ( 'NONE', #31786 ) ;
#78696=CARTESIAN_POINT ( 'NONE',  ( -4.283993363284374745, -11.93770438780619259, 32.05411857736982029 ) ) ;
#78697=CARTESIAN_POINT ( 'NONE',  ( -4.153846153846273204, -3.300289026999228881, 32.46337939537708905 ) ) ;
#78698=CARTESIAN_POINT ( 'NONE',  ( -9.692307692307691624, -8.973038597847269315, 34.52809138561121927 ) ) ;
#78699=CARTESIAN_POINT ( 'NONE',  ( 16.85343815235874132, -8.539481045369598178, 34.89627647299170832 ) ) ;
#78700=CARTESIAN_POINT ( 'NONE',  ( 7.846153846153846700, -4.786620604624113540, 33.94971097300155094 ) ) ;
#78701=CARTESIAN_POINT ( 'NONE',  ( -5.326923076923085532, -2.499999999999999556, 29.81609845454692120 ) ) ;
#78703=CARTESIAN_POINT ( 'NONE',  ( -16.28453675695646652, -5.496505350115500121, 34.60290016733514307 ) ) ;
#78704=DIRECTION ( 'NONE',  ( 0.000000000000000000, 0.000000000000000000, 1.000000000000000000 ) ) ;
#78705=CARTESIAN_POINT ( 'NONE',  ( 10.61538461538449418, -4.320704448113951379, 33.92786785259630022 ) ) ;
#78706=CARTESIAN_POINT ( 'NONE',  ( 17.93391762063986050, -8.164416787775445883, 34.95778746994557906 ) ) ;
#78707=CARTESIAN_POINT ( 'NONE',  ( -3.230769230769352962, -4.320704448113951379, 33.92786785259630022 ) ) ;
#78708=FACE_OUTER_BOUND ( 'NONE', #3704, .T. ) ;
#78709=VECTOR ( 'NONE', #87557, 1000.000000000000114 ) ;
#78710=CARTESIAN_POINT ( 'NONE',  ( 20.99999999999999645, -4.249999999999998224, 29.75000000000000355 ) ) ;
#78712=VERTEX_POINT ( 'NONE', #87632 ) ;
#78713=CARTESIAN_POINT ( 'NONE',  ( 1.384615384615693667, -2.506253911140615021, 30.00000000000323297 ) ) ;
#78714=DIRECTION ( 'NONE',  ( -0.000000000000000000, 1.000000000000000000, 3.491481338843133355E-15 ) ) ;
#78717=DIRECTION ( 'NONE',  ( -0.000000000000000000, -0.9396926207859093161, -0.3420201433256663259 ) ) ;
#78718=CYLINDRICAL_SURFACE ( 'NONE', #82912, 0.2500000000000008882 ) ;
#78719=ORIENTED_EDGE ( 'NONE', *, *, #22668, .F. ) ;
#78721=LINE ( 'NONE', #62214, #58877 ) ;
#78722=CARTESIAN_POINT ( 'NONE',  ( 12.21156173059610772, -5.728515186090277211, 34.42611988154120439 ) ) ;
#78723=EDGE_LOOP ( 'NONE', ( #37214, #10735 ) ) ;
#78724=CARTESIAN_POINT ( 'NONE',  ( -13.38461538461538325, -9.905515769479276145, 34.41647553114623292 ) ) ;
#78725=CYLINDRICAL_SURFACE ( 'NONE', #55590, 0.2499999999999994726 ) ;
#78726=AXIS2_PLACEMENT_3D ( 'NONE', #87266, #72831, #38615 ) ;
#78727=CARTESIAN_POINT ( 'NONE',  ( 5.076923076923075762, -11.11383981884818262, 36.00935417666054406 ) ) ;
#78728=CARTESIAN_POINT ( 'NONE',  ( -14.30769230769230660, -2.249999999999998668, 29.50000000000001421 ) ) ;
#78729=ORIENTED_EDGE ( 'NONE', *, *, #77378, .T. ) ;
#78731=CARTESIAN_POINT ( 'NONE',  ( 10.83839745947801170, -4.026326845037962343, 33.68677907613344047 ) ) ;
#78733=VERTEX_POINT ( 'NONE', #10619 ) ;
#78734=ORIENTED_EDGE ( 'NONE', *, *, #29362, .T. ) ;
#78735=ORIENTED_EDGE ( 'NONE', *, *, #74310, .F. ) ;
#78736=DIRECTION ( 'NONE',  ( -0.000000000000000000, -0.8660254037844399289, -0.4999999999999980016 ) ) ;
#78737=LINE ( 'NONE', #31441, #9822 ) ;
#78738=B_SPLINE_CURVE_WITH_KNOTS ( 'NONE', 3,
 ( #87167, #66431, #88500, #33086, #53354, #52459, #11490, #12378, #32210, #40742 ),
 .UNSPECIFIED., .F., .F.,
 ( 4, 2, 2, 2, 4 ),
 ( 0.0007817246256747530271, 0.0009771112852218974409, 0.001172497944769041638, 0.001367884604316185835, 0.001563271263863330249 ),
 .UNSPECIFIED. ) ;
#78739=CYLINDRICAL_SURFACE ( 'NONE', #73978, 0.2499999999999993616 ) ;
#78740=LINE ( 'NONE', #65219, #57824 ) ;
#78742=VERTEX_POINT ( 'NONE', #25467 ) ;
#78743=CARTESIAN_POINT ( 'NONE',  ( 10.83876010115703536, -2.251407671071270489, 29.88021292934942963 ) ) ;
#78744=ORIENTED_EDGE ( 'NONE', *, *, #48550, .T. ) ;
#78745=CARTESIAN_POINT ( 'NONE',  ( 12.52679360105129902, -11.67786785259547777, 32.92929555188713664 ) ) ;
#78746=EDGE_CURVE ( 'NONE', #67493, #39653, #11628, .T. ) ;
#78747=CARTESIAN_POINT ( 'NONE',  ( -8.638705067467206788, -12.45806712695776319, 30.39783852428763922 ) ) ;
#78749=ORIENTED_EDGE ( 'NONE', *, *, #77836, .F. ) ;
#78750=ORIENTED_EDGE ( 'NONE', *, *, #57147, .T. ) ;
#78751=ORIENTED_EDGE ( 'NONE', *, *, #4798, .T. ) ;
#78754=CARTESIAN_POINT ( 'NONE',  ( -5.076923076923075762, -5.180354513474913603, 36.12317359536750416 ) ) ;
#78756=CARTESIAN_POINT ( 'NONE',  ( -10.74607521849492464, -9.084618155246140248, 34.75535874321725771 ) ) ;
#78758=EDGE_CURVE ( 'NONE', #29939, #61361, #65100, .T. ) ;
#78759=CARTESIAN_POINT ( 'NONE',  ( 6.792516331335002988, -2.504760397472873823, 29.97295953869789997 ) ) ;
#78760=CARTESIAN_POINT ( 'NONE',  ( -1.607541602131531189, -8.239355502252617924, 34.69524867566427417 ) ) ;
#78761=CARTESIAN_POINT ( 'NONE',  ( 8.992010310499177095, -5.913360116392397892, 34.49180327182771322 ) ) ;
#78763=FACE_BOUND ( 'NONE', #53803, .T. ) ;
#78764=CARTESIAN_POINT ( 'NONE',  ( 14.98074599347626368, -5.851115903089112003, 34.47074536777953568 ) ) ;
#78765=CARTESIAN_POINT ( 'NONE',  ( 9.942307692307759126, -7.434744429011176159, 34.75000000000000711 ) ) ;
#78766=CARTESIAN_POINT ( 'NONE',  ( -15.16470087976679615, -10.51840700105979565, 33.73612834413962247 ) ) ;
#78767=CARTESIAN_POINT ( 'NONE',  ( 16.40390057375960708, -4.074993327901525575, 33.72946981652012255 ) ) ;
#78768=DIRECTION ( 'NONE',  ( -0.000000000000000000, 0.5000000000000011102, -0.8660254037844381525 ) ) ;
#78769=DIRECTION ( 'NONE',  ( -0.000000000000000000, 0.9396926207859092051, -0.3420201433256662704 ) ) ;
#78770=CARTESIAN_POINT ( 'NONE',  ( 5.326977388561387805, -2.564540009722896752, 30.55348353981670684 ) ) ;
#78771=VERTEX_POINT ( 'NONE', #17375 ) ;
#78772=CARTESIAN_POINT ( 'NONE',  ( -15.93106648486808119, -3.563462043263029955, 33.22394488606062879 ) ) ;
#78773=ORIENTED_EDGE ( 'NONE', *, *, #12075, .T. ) ;
#78774=ORIENTED_EDGE ( 'NONE', *, *, #44070, .F. ) ;
#78775=CARTESIAN_POINT ( 'NONE',  ( -11.78848476268299628, -12.68155406624981119, 30.59749803192733708 ) ) ;
#78776=CARTESIAN_POINT ( 'NONE',  ( 1.254468175177166689, -10.88202310037936194, 33.43294751532457099 ) ) ;
#78777=CARTESIAN_POINT ( 'NONE',  ( 11.47319153790521717, -8.656820664281498878, 34.87096338111211935 ) ) ;
#78778=CARTESIAN_POINT ( 'NONE',  ( 2.372947447205147053, -2.379036618887895305, 30.90682066428159303 ) ) ;
#78779=CARTESIAN_POINT ( 'NONE',  ( 17.99999999999987566, -12.51329471203414379, 31.30864560766407578 ) ) ;
#78780=ORIENTED_EDGE ( 'NONE', *, *, #44442, .T. ) ;
#78781=EDGE_CURVE ( 'NONE', #83912, #5662, #52484, .T. ) ;
#78782=EDGE_CURVE ( 'NONE', #45673, #21173, #86299, .T. ) ;
#78783=CARTESIAN_POINT ( 'NONE',  ( 18.06525513951284267, -2.657715359629131857, 31.77849191805844242 ) ) ;
#78784=CARTESIAN_POINT ( 'NONE',  ( 0.2115617174898698494, -12.65889640711025521, 30.72598325615533454 ) ) ;
#78785=CARTESIAN_POINT ( 'NONE',  ( -10.61538461538461320, -8.564572088678739092, 35.78748833219616898 ) ) ;
#78786=DIRECTION ( 'NONE',  ( 0.000000000000000000, 0.000000000000000000, 1.000000000000000000 ) ) ;
#78787=CARTESIAN_POINT ( 'NONE',  ( -17.01085574357300345, -2.486705287966280320, 31.30864560766543647 ) ) ;
#78791=EDGE_CURVE ( 'NONE', #30670, #71085, #30903, .T. ) ;
#78793=ORIENTED_EDGE ( 'NONE', *, *, #38894, .T. ) ;
#78794=CYLINDRICAL_SURFACE ( 'NONE', #39803, 0.2500000000000002220 ) ;
#78795=CARTESIAN_POINT ( 'NONE',  ( 17.99999999999987566, -11.67786785259630911, 32.92929555188603530 ) ) ;
#78796=CARTESIAN_POINT ( 'NONE',  ( -14.05763799605399278, -6.567000820036036579, 34.66262288849541306 ) ) ;
#78797=CARTESIAN_POINT ( 'NONE',  ( 2.241935505177999222, -7.249945686854185389, 34.74374336980224598 ) ) ;
#78799=CARTESIAN_POINT ( 'NONE',  ( 14.05771556364371655, -6.524016743844655686, 34.90889640711025521 ) ) ;
#78801=DIRECTION ( 'NONE',  ( -0.000000000000000000, 0.9396926207859092051, -0.3420201433256662704 ) ) ;
#78802=CARTESIAN_POINT ( 'NONE',  ( -2.307692307692305711, -12.62096338111211580, 30.90682066428153263 ) ) ;
#78804=CARTESIAN_POINT ( 'NONE',  ( -9.942307692307691624, -7.566082377512564960, 35.00000000000000711 ) ) ;
#78805=CARTESIAN_POINT ( 'NONE',  ( -12.21148414990014963, -3.627508038966690496, 32.91356715214248396 ) ) ;
#78806=B_SPLINE_CURVE_WITH_KNOTS ( 'NONE', 3,
 ( #73523, #31640, #24873, #32519, #59994, #45142 ),
 .UNSPECIFIED., .F., .F.,
 ( 4, 2, 4 ),
 ( 0.0003909569690057875316, 0.0005862646681846158964, 0.0007815723673634442613 ),
 .UNSPECIFIED. ) ;
#78807=DIRECTION ( 'NONE',  ( 0.000000000000000000, 0.3420201433256641055, -0.9396926207859100932 ) ) ;
#78808=CARTESIAN_POINT ( 'NONE',  ( 0.5920641633020229389, -2.882268652242222728, 31.66798894389554064 ) ) ;
#78809=LINE ( 'NONE', #17110, #59452 ) ;
#78810=B_SPLINE_CURVE_WITH_KNOTS ( 'NONE', 3,
 ( #18071, #19, #21607, #55396, #13087, #34238 ),
 .UNSPECIFIED., .F., .F.,
 ( 4, 2, 4 ),
 ( 0.0003909569690057545718, 0.0005862646681845668905, 0.0007815723673633792092 ),
 .UNSPECIFIED. ) ;
#78811=CARTESIAN_POINT ( 'NONE',  ( -12.46153846153858424, -3.643525952248795718, 33.31231777344771672 ) ) ;
#78812=CARTESIAN_POINT ( 'NONE',  ( 15.45354877203763522, -11.41317474335729543, 32.86274602512330034 ) ) ;
#78814=ORIENTED_EDGE ( 'NONE', *, *, #7069, .T. ) ;
#78815=CARTESIAN_POINT ( 'NONE',  ( -15.93106648486808119, -6.717445702608400460, 34.94155399931962336 ) ) ;
#78816=CARTESIAN_POINT ( 'NONE',  ( 8.899756470994335089, -11.93748526763465279, 32.05452791011430946 ) ) ;
#78817=CARTESIAN_POINT ( 'NONE',  ( -17.20761368003338632, -4.684245665217972032, 34.18127051446801090 ) ) ;
#78819=B_SPLINE_CURVE_WITH_KNOTS ( 'NONE', 3,
 ( #27046, #40134, #60380, #5003, #4552, #66247, #26602, #73910, #32917, #54509 ),
 .UNSPECIFIED., .F., .F.,
 ( 4, 2, 2, 2, 4 ),
 ( 0.0007817246256747484735, 0.0009771112852218931041, 0.001172497944769037735, 0.001367884604316182365, 0.001563271263863326996 ),
 .UNSPECIFIED. ) ;
#78820=CARTESIAN_POINT ( 'NONE',  ( 0.2386122440223122643, -3.586966769969700763, 32.86292498521069660 ) ) ;
#78821=DIRECTION ( 'NONE',  ( 0.000000000000000000, 0.000000000000000000, 1.000000000000000000 ) ) ;
#78822=VERTEX_POINT ( 'NONE', #21365 ) ;
#78824=CYLINDRICAL_SURFACE ( 'NONE', #22479, 0.2499999999999994726 ) ;
#78825=ORIENTED_EDGE ( 'NONE', *, *, #58004, .T. ) ;
#78826=CARTESIAN_POINT ( 'NONE',  ( -18.22348492456433178, -4.988325925672469019, 34.36044203135681130 ) ) ;
#78827=ORIENTED_EDGE ( 'NONE', *, *, #82568, .F. ) ;
#78829=CARTESIAN_POINT ( 'NONE',  ( 6.989144256426998325, -3.937682226553329556, 33.60647404775216529 ) ) ;
#78830=CARTESIAN_POINT ( 'NONE',  ( -5.749999999999999112, -2.499999999999998668, 29.75000000000000355 ) ) ;
#78831=CYLINDRICAL_SURFACE ( 'NONE', #9607, 0.2500000000000009437 ) ;
#78832=ORIENTED_EDGE ( 'NONE', *, *, #3609, .F. ) ;
#78833=CARTESIAN_POINT ( 'NONE',  ( -1.384615384615383471, -1.790695186598648903, 34.54067556320373455 ) ) ;
#78834=ORIENTED_EDGE ( 'NONE', *, *, #72612, .T. ) ;
#78835=CARTESIAN_POINT ( 'NONE',  ( 13.38461538461526601, -4.481592998941358097, 33.73612834414048933 ) ) ;
#78836=EDGE_LOOP ( 'NONE', ( #14080, #87425 ) ) ;
#78837=CYLINDRICAL_SURFACE ( 'NONE', #2542, 0.2499999999999986955 ) ;
#78838=DIRECTION ( 'NONE',  ( -0.000000000000000000, 0.9396926207859093161, -0.3420201433256663259 ) ) ;
#78839=VERTEX_POINT ( 'NONE', #40321 ) ;
#78841=PLANE ( 'NONE',  #1844 ) ;
#78842=CARTESIAN_POINT ( 'NONE',  ( -5.076923076923199218, -12.51329471203414379, 31.30864560766407578 ) ) ;
#78843=EDGE_CURVE ( 'NONE', #39886, #62997, #13701, .T. ) ;
#78844=CARTESIAN_POINT ( 'NONE',  ( 4.853438133199127869, -9.331801661448606566, 34.40259984581193464 ) ) ;
#78845=CARTESIAN_POINT ( 'NONE',  ( -11.31544869436814160, -3.395485233115139057, 33.02377354290275946 ) ) ;
#78846=B_SPLINE_CURVE_WITH_KNOTS ( 'NONE', 3,
 ( #88224, #26054, #26497, #81006, #18406, #54400, #6233, #60717, #5781, #86890 ),
 .UNSPECIFIED., .F., .F.,
 ( 4, 2, 2, 2, 4 ),
 ( 0.0007817359430256391132, 0.0009771253907250075990, 0.001172514838424375868, 0.001367904286123744354, 0.001563293733823112840 ),
 .UNSPECIFIED. ) ;
#78847=B_SPLINE_CURVE_WITH_KNOTS ( 'NONE', 3,
 ( #74275, #26978, #32842, #48117, #33730, #81041, #66629, #61185, #6694, #33293 ),
 .UNSPECIFIED., .F., .F.,
 ( 4, 2, 2, 2, 4 ),
 ( 0.000000000000000000, 0.0001954339857564081520, 0.0003908679715128163040, 0.0005863019572692244018, 0.0007817359430256326080 ),
 .UNSPECIFIED. ) ;
#78851=CARTESIAN_POINT ( 'NONE',  ( 3.164686851409095336, -5.471508081941601986, 34.59228464037088457 ) ) ;
#78852=ORIENTED_EDGE ( 'NONE', *, *, #87296, .F. ) ;
#78853=EDGE_CURVE ( 'NONE', #4262, #62614, #69529, .T. ) ;
#78854=VECTOR ( 'NONE', #1049, 1000.000000000000000 ) ;
#78855=DIRECTION ( 'NONE',  ( 0.000000000000000000, -3.469446951953611033E-15, -1.000000000000000000 ) ) ;
#78858=EDGE_LOOP ( 'NONE', ( #82476, #62245, #60855, #54766 ) ) ;
#78859=ORIENTED_EDGE ( 'NONE', *, *, #39545, .F. ) ;
#78860=ORIENTED_EDGE ( 'NONE', *, *, #847, .F. ) ;
#78861=CARTESIAN_POINT ( 'NONE',  ( 3.361294932532794988, -5.195472089885680766, 34.18748526763464923 ) ) ;
#78862=ORIENTED_EDGE ( 'NONE', *, *, #59762, .T. ) ;
#78864=DIRECTION ( 'NONE',  ( -0.000000000000000000, 0.9396926207859093161, -0.3420201433256663259 ) ) ;
#78865=AXIS2_PLACEMENT_3D ( 'NONE', #79857, #26682, #54139 ) ;
#78866=EDGE_CURVE ( 'NONE', #58471, #81511, #87630, .T. ) ;
#78867=CARTESIAN_POINT ( 'NONE',  ( 3.903869409797562806, -12.65889640711025521, 30.72598325615533454 ) ) ;
#78868=CARTESIAN_POINT ( 'NONE',  ( 12.23861224402230619, -2.554751324335735152, 30.48935550225260727 ) ) ;
#78869=FACE_BOUND ( 'NONE', #30094, .T. ) ;
#78870=ORIENTED_EDGE ( 'NONE', *, *, #46540, .T. ) ;
#78871=CARTESIAN_POINT ( 'NONE',  ( 13.16113046005105502, -10.97335522853832579, 33.68706563782419749 ) ) ;
#78872=B_SPLINE_CURVE_WITH_KNOTS ( 'NONE', 3,
 ( #40146, #68481, #67607, #67162, #6358, #19412, #54974, #6780, #47771, #26171 ),
 .UNSPECIFIED., .F., .F.,
 ( 4, 2, 2, 2, 4 ),
 ( 0.000000000000000000, 0.0001954311564186881484, 0.0003908623128373762967, 0.0005862934692560644451, 0.0007817246256747525934 ),
 .UNSPECIFIED. ) ;
#78873=EDGE_CURVE ( 'NONE', #8529, #11982, #52377, .T. ) ;
#78874=LINE ( 'NONE', #52289, #1443 ) ;
#78875=CARTESIAN_POINT ( 'NONE',  ( 4.153846153846154188, -12.10708131394839349, 31.69288490824020244 ) ) ;
#78876=CARTESIAN_POINT ( 'NONE',  ( 10.61538461538461675, -2.721908614388771852, 31.22303859784724978 ) ) ;
#78877=EDGE_LOOP ( 'NONE', ( #39403, #85422 ) ) ;
#78878=CARTESIAN_POINT ( 'NONE',  ( 9.442284455014730682, -2.587272538249754117, 30.68239716806877837 ) ) ;
#78879=ORIENTED_EDGE ( 'NONE', *, *, #80515, .F. ) ;
#78880=ORIENTED_EDGE ( 'NONE', *, *, #11177, .T. ) ;
#78881=LINE ( 'NONE', #25725, #84918 ) ;
#78882=LINE ( 'NONE', #38350, #34776 ) ;
#78883=B_SPLINE_CURVE_WITH_KNOTS ( 'NONE', 3,
 ( #67306, #17790, #66412, #25426, #73174, #45242, #81269, #53332, #33071, #74067 ),
 .UNSPECIFIED., .F., .F.,
 ( 4, 2, 2, 2, 4 ),
 ( 0.000000000000000000, 0.0001954339857564078809, 0.0003908679715128157619, 0.0005863019572692236428, 0.0007817359430256315238 ),
 .UNSPECIFIED. ) ;
#78884=DIRECTION ( 'NONE',  ( 0.000000000000000000, 0.9848077530122072432, -0.1736481776669354937 ) ) ;
#78885=DIRECTION ( 'NONE',  ( -0.000000000000000000, 0.8660254037844399289, -0.4999999999999980016 ) ) ;
#78886=DIRECTION ( 'NONE',  ( 0.000000000000000000, 0.8660254037844377084, -0.5000000000000015543 ) ) ;
#78887=CARTESIAN_POINT ( 'NONE',  ( -2.557715544985271983, -10.05641848906368097, 34.04755513067966177 ) ) ;
#78889=EDGE_CURVE ( 'NONE', #53607, #52583, #1320, .T. ) ;
#78890=FACE_OUTER_BOUND ( 'NONE', #88218, .T. ) ;
#78891=CARTESIAN_POINT ( 'NONE',  ( -0.2387587925603949779, -3.563462043263031287, 33.22394488606064300 ) ) ;
#78892=CARTESIAN_POINT ( 'NONE',  ( -18.00000000000000000, -2.499999999999999556, 29.74999999999998579 ) ) ;
#78893=EDGE_CURVE ( 'NONE', #32458, #14846, #20066, .T. ) ;
#78894=CARTESIAN_POINT ( 'NONE',  ( 14.55763771707035126, -2.589246495874658383, 31.60778113518102828 ) ) ;
#78895=VERTEX_POINT ( 'NONE', #61456 ) ;
#78896=VECTOR ( 'NONE', #60620, 1000.000000000000000 ) ;
#78897=ORIENTED_EDGE ( 'NONE', *, *, #75416, .F. ) ;
#78898=FACE_BOUND ( 'NONE', #16255, .T. ) ;
#78899=ORIENTED_EDGE ( 'NONE', *, *, #49325, .T. ) ;
#78900=EDGE_CURVE ( 'NONE', #17581, #3390, #2929, .T. ) ;
#78901=CYLINDRICAL_SURFACE ( 'NONE', #56386, 0.2499999999999994726 ) ;
#78902=CARTESIAN_POINT ( 'NONE',  ( -1.254089946381738763, -2.372941743896878286, 30.88044141588254377 ) ) ;
#78903=EDGE_CURVE ( 'NONE', #22888, #25656, #48066, .T. ) ;
#78904=EDGE_LOOP ( 'NONE', ( #58682, #76982 ) ) ;
#78906=CARTESIAN_POINT ( 'NONE',  ( -10.68065506134538545, -6.879047030191174805, 34.71129190930000163 ) ) ;
#78907=CARTESIAN_POINT ( 'NONE',  ( 16.15384615384615330, -8.120952969808772792, 34.71129190930000163 ) ) ;
#78908=CARTESIAN_POINT ( 'NONE',  ( 6.923076923076924238, -3.513871655860378418, 32.76840700105978499 ) ) ;
#78909=ORIENTED_EDGE ( 'NONE', *, *, #61363, .F. ) ;
#78910=CARTESIAN_POINT ( 'NONE',  ( -10.61538461538461320, -12.29105614889573062, 35.45975837776705220 ) ) ;
#78911=VERTEX_POINT ( 'NONE', #30338 ) ;
#78912=CARTESIAN_POINT ( 'NONE',  ( 17.01165263096229907, -10.90142922261923886, 33.41473453929638993 ) ) ;
#78913=EDGE_LOOP ( 'NONE', ( #61657, #18923, #36140, #52271 ) ) ;
#78915=CARTESIAN_POINT ( 'NONE',  ( -8.769230769230768274, -1.422936976036506707, 30.56769352161908415 ) ) ;
#78916=DIRECTION ( 'NONE',  ( 0.000000000000000000, 0.9848077530122072432, 0.1736481776669354937 ) ) ;
#78917=CARTESIAN_POINT ( 'NONE',  ( -10.83886953994894675, -3.562934362175800285, 33.22335522853832401 ) ) ;
#78919=CARTESIAN_POINT ( 'NONE',  ( -9.942330916529147800, -12.07920672191015221, 32.31858351112116168 ) ) ;
#78921=ORIENTED_EDGE ( 'NONE', *, *, #27191, .T. ) ;
#78922=CARTESIAN_POINT ( 'NONE',  ( -3.230769230769229949, -3.050289026998446396, 32.03036669348365706 ) ) ;
#78923=CARTESIAN_POINT ( 'NONE',  ( -15.00798968950081935, -3.755027918224367323, 33.06320215134714857 ) ) ;
#78924=CARTESIAN_POINT ( 'NONE',  ( 14.30769230769231015, -9.819645486525091727, 36.12317359536749706 ) ) ;
#78925=VECTOR ( 'NONE', #53218, 999.9999999999998863 ) ;
#78927=VERTEX_POINT ( 'NONE', #22255 ) ;
#78928=DIRECTION ( 'NONE',  ( -0.000000000000000000, 0.9848077530122086864, -0.1736481776669273891 ) ) ;
#78929=CARTESIAN_POINT ( 'NONE',  ( -7.846153846153844924, -5.471508081941601098, 34.59228464037088457 ) ) ;
#78930=FACE_OUTER_BOUND ( 'NONE', #60115, .T. ) ;
#78931=AXIS2_PLACEMENT_3D ( 'NONE', #40112, #88748, #48612 ) ;
#78933=DIRECTION ( 'NONE',  ( -0.000000000000000000, -0.6427876096865404731, -0.7660444431189771253 ) ) ;
#78934=CARTESIAN_POINT ( 'NONE',  ( 16.40390057375960708, -3.435999193479609026, 33.07426656108011542 ) ) ;
#78936=CARTESIAN_POINT ( 'NONE',  ( 16.15384615384615330, -6.435427911321262684, 35.78748833219616898 ) ) ;
#78937=VERTEX_POINT ( 'NONE', #29030 ) ;
#78938=EDGE_CURVE ( 'NONE', #70481, #3368, #38675, .T. ) ;
#78939=CARTESIAN_POINT ( 'NONE',  ( 6.130791807824786943, -10.54018710029568595, 33.71981072465678864 ) ) ;
#78940=CARTESIAN_POINT ( 'NONE',  ( -16.94687547066739697, -7.723484964179501588, 34.74522123443823318 ) ) ;
#78943=DIRECTION ( 'NONE',  ( 0.000000000000000000, 0.4999999999999960032, -0.8660254037844410391 ) ) ;
#78944=LINE ( 'NONE', #85710, #36394 ) ;
#78946=VERTEX_POINT ( 'NONE', #9618 ) ;
#78947=CARTESIAN_POINT ( 'NONE',  ( -7.846153846153965716, -3.835265460704628371, 33.15142922262033665 ) ) ;
#78948=B_SPLINE_CURVE_WITH_KNOTS ( 'NONE', 3,
 ( #46366, #19343, #75179, #13464, #40944, #60317, #68407, #48128, #74288, #75600 ),
 .UNSPECIFIED., .F., .F.,
 ( 4, 2, 2, 2, 4 ),
 ( 0.000000000000000000, 0.0001954339857564079352, 0.0003908679715128158703, 0.0005863019572692237513, 0.0007817359430256317406 ),
 .UNSPECIFIED. ) ;
#78949=ADVANCED_FACE ( 'NONE', ( #56037 ), #1543, .F. ) ;
#78950=EDGE_LOOP ( 'NONE', ( #54612, #4892 ) ) ;
#78951=CARTESIAN_POINT ( 'NONE',  ( -18.00000000000000000, -8.164416787775447659, 34.95778746994557906 ) ) ;
#78952=CARTESIAN_POINT ( 'NONE',  ( -13.31947060389575199, -7.750023224968867197, 34.99404313364389907 ) ) ;
#78953=CARTESIAN_POINT ( 'NONE',  ( 4.153846153846154188, -3.886160181151819604, 36.00935417666054406 ) ) ;
#78954=EDGE_LOOP ( 'NONE', ( #85401, #30466, #14822, #21574 ) ) ;
#78955=CARTESIAN_POINT ( 'NONE',  ( 8.769230769230768274, -2.249999999999998668, 29.75000000000001776 ) ) ;
#78956=CARTESIAN_POINT ( 'NONE',  ( -5.999999999999998224, -4.098570777380720287, 33.41473453929634729 ) ) ;
#78957=EDGE_CURVE ( 'NONE', #47875, #73916, #88851, .T. ) ;
#78958=DIRECTION ( 'NONE',  ( 0.000000000000000000, 0.4999999999999960032, -0.8660254037844410391 ) ) ;
#78959=DIRECTION ( 'NONE',  ( 0.000000000000000000, 0.9396926207859126468, 0.3420201433256571111 ) ) ;
#78960=ORIENTED_EDGE ( 'NONE', *, *, #20753, .T. ) ;
#78961=CARTESIAN_POINT ( 'NONE',  ( -1.384615384615505151, -3.835265460704628371, 33.15142922262033665 ) ) ;
#78962=ORIENTED_EDGE ( 'NONE', *, *, #43278, .T. ) ;
#78964=DIRECTION ( 'NONE',  ( -0.000000000000000000, -0.1736481776669307198, -0.9848077530122080203 ) ) ;
#78965=CARTESIAN_POINT ( 'NONE',  ( -16.40386939113911779, -11.37209801155882793, 32.91403422569033665 ) ) ;
#78966=EDGE_CURVE ( 'NONE', #30322, #28852, #18952, .T. ) ;
#78967=CARTESIAN_POINT ( 'NONE',  ( 7.780883845597527326, -12.51329471203370325, 31.30864560766548976 ) ) ;
#78968=CARTESIAN_POINT ( 'NONE',  ( -14.05774678934416322, -11.86320923018887541, 32.19269448109604781 ) ) ;
#78969=CARTESIAN_POINT ( 'NONE',  ( 15.10062202133101472, -11.93770438780619259, 32.05411857736982029 ) ) ;
#78970=EDGE_CURVE ( 'NONE', #30665, #82411, #62778, .T. ) ;
#78971=ORIENTED_EDGE ( 'NONE', *, *, #75028, .F. ) ;
#78973=EDGE_LOOP ( 'NONE', ( #55249, #17677 ) ) ;
#78974=EDGE_LOOP ( 'NONE', ( #54073, #46831 ) ) ;
#78975=ORIENTED_EDGE ( 'NONE', *, *, #47708, .T. ) ;
#78976=CARTESIAN_POINT ( 'NONE',  ( 12.71159277317677549, -11.79725096376909654, 32.30694842903959341 ) ) ;
#78977=CARTESIAN_POINT ( 'NONE',  ( -1.161604033002534786, -12.39991518177334129, 30.74647679643404530 ) ) ;
#78978=CARTESIAN_POINT ( 'NONE',  ( 14.55769230769372946, -7.500000000000154543, 35.00000000000007105 ) ) ;
#78979=DIRECTION ( 'NONE',  ( -0.000000000000000000, -0.1736481776669307198, -0.9848077530122080203 ) ) ;
#78980=DIRECTION ( 'NONE',  ( 0.000000000000000000, -6.938893903907222067E-15, 1.000000000000000000 ) ) ;
#78981=CARTESIAN_POINT ( 'NONE',  ( 3.165498784808455923, -6.026961402152685388, 34.52809138561120506 ) ) ;
#78982=AXIS2_PLACEMENT_3D ( 'NONE', #63568, #41986, #22586 ) ;
#78983=CARTESIAN_POINT ( 'NONE',  ( -17.77698864838715309, -9.886259254753570147, 34.14407573483972413 ) ) ;
#78984=CARTESIAN_POINT ( 'NONE',  ( 9.562159722576001997, -10.31621877034669588, 34.18098118002070152 ) ) ;
#78985=CARTESIAN_POINT ( 'NONE',  ( 7.976944287120795174, -4.684288915650983043, 34.18129842949671371 ) ) ;
#78986=VERTEX_POINT ( 'NONE', #15504 ) ;
#78987=ORIENTED_EDGE ( 'NONE', *, *, #50607, .F. ) ;
#78988=ORIENTED_EDGE ( 'NONE', *, *, #33223, .T. ) ;
#78989=DIRECTION ( 'NONE',  ( -0.000000000000000000, -0.8660254037844399289, -0.4999999999999980016 ) ) ;
#78990=ORIENTED_EDGE ( 'NONE', *, *, #49668, .T. ) ;
#78991=CARTESIAN_POINT ( 'NONE',  ( -9.822454901745912181, -9.418419913701741919, 34.36755862841477693 ) ) ;
#78992=CARTESIAN_POINT ( 'NONE',  ( -16.28453762051371712, -9.804603061927743113, 34.18744698557895845 ) ) ;
#78994=CARTESIAN_POINT ( 'NONE',  ( 8.703473966716462229, -7.249945686854186278, 34.74374336980224598 ) ) ;
#78995=CARTESIAN_POINT ( 'NONE',  ( 6.988332494352946789, -2.625532179533470512, 30.86335684631491105 ) ) ;
#78997=EDGE_CURVE ( 'NONE', #44583, #71986, #42975, .T. ) ;
#78998=ADVANCED_FACE ( 'NONE', ( #29467 ), #56917, .F. ) ;
#78999=EDGE_LOOP ( 'NONE', ( #1190, #41032, #42497, #4321 ) ) ;
#79000=CARTESIAN_POINT ( 'NONE',  ( -17.14300545628321260, -11.35647404775217595, 33.31231777344666511 ) ) ;
#79001=ORIENTED_EDGE ( 'NONE', *, *, #29668, .T. ) ;
#79002=EDGE_CURVE ( 'NONE', #42943, #72270, #37984, .T. ) ;
#79003=FACE_BOUND ( 'NONE', #52918, .T. ) ;
#79005=CARTESIAN_POINT ( 'NONE',  ( 5.076923076922953193, -3.643525952248796163, 33.31231777344771672 ) ) ;
#79006=EDGE_LOOP ( 'NONE', ( #14976, #7383 ) ) ;
#79007=CARTESIAN_POINT ( 'NONE',  ( -1.134560964701930796, -5.642605341092957083, 34.66089969410670335 ) ) ;
#79009=EDGE_CURVE ( 'NONE', #74008, #65490, #32118, .T. ) ;
#79010=DIRECTION ( 'NONE',  ( 0.000000000000000000, 0.7660444431189822323, -0.6427876096865344779 ) ) ;
#79011=VERTEX_POINT ( 'NONE', #86639 ) ;
#79012=CARTESIAN_POINT ( 'NONE',  ( -14.55769230769230660, -2.499999999999998668, 29.75000000000000355 ) ) ;
#79013=CARTESIAN_POINT ( 'NONE',  ( -14.37377571864818293, -5.557115091759785130, 34.35708131394839171 ) ) ;
#79014=VERTEX_POINT ( 'NONE', #5090 ) ;
#79015=CARTESIAN_POINT ( 'NONE',  ( 5.934246571686668581, -7.249945578846651806, 34.99404164642496795 ) ) ;
#79016=CARTESIAN_POINT ( 'NONE',  ( -2.307692307692427391, -10.21337939537710326, 33.94971097300076224 ) ) ;
#79017=ORIENTED_EDGE ( 'NONE', *, *, #31894, .T. ) ;
#79019=CARTESIAN_POINT ( 'NONE',  ( -10.36533030374629583, -4.943051570960394159, 34.04725096376909477 ) ) ;
#79021=CARTESIAN_POINT ( 'NONE',  ( 16.15384615384603251, -11.06231777344772027, 33.60647404775119895 ) ) ;
#79022=DIRECTION ( 'NONE',  ( -0.000000000000000000, -0.6427876096865404731, -0.7660444431189770143 ) ) ;
#79023=CARTESIAN_POINT ( 'NONE',  ( 9.019285189144223835, -4.074993327901527351, 33.72946981652012255 ) ) ;
#79024=CARTESIAN_POINT ( 'NONE',  ( 4.284371855609719226, -12.27024696741798770, 31.24895572276497546 ) ) ;
#79025=CARTESIAN_POINT ( 'NONE',  ( 11.78846153846160583, -7.434744860731433924, 35.00000000000000711 ) ) ;
#79026=CARTESIAN_POINT ( 'NONE',  ( -1.384615384615506484, -9.528491918059723176, 34.59228464037033035 ) ) ;
#79027=CARTESIAN_POINT ( 'NONE',  ( 12.21153846153846168, -7.566082377512564960, 35.00000000000000711 ) ) ;
#79028=CARTESIAN_POINT ( 'NONE',  ( 8.835299120233207404, -2.721908614388771852, 31.22303859784725333 ) ) ;
#79030=CIRCLE ( 'NONE', #56015, 0.2500000000000002220 ) ;
#79032=VERTEX_POINT ( 'NONE', #44724 ) ;
#79033=CARTESIAN_POINT ( 'NONE',  ( 0.3954550505825799589, -12.37446782046654192, 30.86335684631486487 ) ) ;
#79035=EDGE_CURVE ( 'NONE', #29464, #40637, #80213, .T. ) ;
#79036=ORIENTED_EDGE ( 'NONE', *, *, #78384, .F. ) ;
#79037=CARTESIAN_POINT ( 'NONE',  ( -8.769230769230768274, -11.69971097300155272, 32.46337939537588113 ) ) ;
#79038=ORIENTED_EDGE ( 'NONE', *, *, #22625, .T. ) ;
#79039=CARTESIAN_POINT ( 'NONE',  ( -5.776987155906605942, -10.01129605718032778, 34.36064277460058491 ) ) ;
#79041=CARTESIAN_POINT ( 'NONE',  ( 3.007842271862382066, -2.308479472611653094, 30.53278059502174457 ) ) ;
#79042=CARTESIAN_POINT ( 'NONE',  ( -5.749945580086544439, -11.47946981652013498, 33.17500667209846910 ) ) ;
#79044=CARTESIAN_POINT ( 'NONE',  ( -3.230769230769229949, -8.318370150425687726, 35.83090037661290239 ) ) ;
#79046=CARTESIAN_POINT ( 'NONE',  ( 0.6845513056318558442, -5.582272713120728369, 34.63742843783360570 ) ) ;
#79047=CARTESIAN_POINT ( 'NONE',  ( -7.596208327805703320, -12.22109172314383052, 31.39792113162168263 ) ) ;
#79050=CARTESIAN_POINT ( 'NONE',  ( 1.515407192440172190, -3.062576670634119758, 32.05464942895959979 ) ) ;
#79052=CARTESIAN_POINT ( 'NONE',  ( 10.48523664565292002, -5.915902021225889484, 34.75552854090298638 ) ) ;
#79053=ADVANCED_FACE ( 'NONE', ( #31678 ), #24457, .F. ) ;
#79054=B_SPLINE_CURVE_WITH_KNOTS ( 'NONE', 3,
 ( #51905, #64099, #2393, #23121, #72186, #78498, #2832, #43395, #24437, #3727 ),
 .UNSPECIFIED., .F., .F.,
 ( 4, 2, 2, 2, 4 ),
 ( 0.000000000000000000, 0.0001954311564186864949, 0.0003908623128373729899, 0.0005862934692560594577, 0.0007817246256747459798 ),
 .UNSPECIFIED. ) ;
#79055=VECTOR ( 'NONE', #48211, 1000.000000000000227 ) ;
#79056=AXIS2_PLACEMENT_3D ( 'NONE', #15959, #30349, #29038 ) ;
#79057=VERTEX_POINT ( 'NONE', #17264 ) ;
#79059=CARTESIAN_POINT ( 'NONE',  ( 7.715462379486289990, -11.18331474514187995, 33.13161551792790505 ) ) ;
#79060=CARTESIAN_POINT ( 'NONE',  ( -2.530619266599154038, -2.308479472611653094, 30.53278059502174457 ) ) ;
#79061=CARTESIAN_POINT ( 'NONE',  ( 3.903846153846154632, -7.500000000000001776, 35.04278698407183867 ) ) ;
#79062=B_SPLINE_CURVE_WITH_KNOTS ( 'NONE', 3,
 ( #77349, #64707, #71033, #16976, #21968, #43127, #23718, #10227, #85003, #84127 ),
 .UNSPECIFIED., .F., .F.,
 ( 4, 2, 2, 2, 4 ),
 ( 0.000000000000000000, 0.0001954311564186871726, 0.0003908623128373743452, 0.0005862934692560615177, 0.0007817246256747486903 ),
 .UNSPECIFIED. ) ;
#79064=CARTESIAN_POINT ( 'NONE',  ( 15.00794253829022828, -7.369208160676172348, 34.74850200257122879 ) ) ;
#79065=CARTESIAN_POINT ( 'NONE',  ( 9.468822748583745508, -11.41268669641499756, 32.86336882939238535 ) ) ;
#79066=EDGE_CURVE ( 'NONE', #29866, #45581, #80314, .T. ) ;
#79067=VECTOR ( 'NONE', #71403, 1000.000000000000000 ) ;
#79068=B_SPLINE_CURVE_WITH_KNOTS ( 'NONE', 3,
 ( #38170, #45363, #58426, #39529, #3930, #58884, #19243, #46709, #18354, #17909 ),
 .UNSPECIFIED., .F., .F.,
 ( 4, 2, 2, 2, 4 ),
 ( 0.000000000000000000, 0.0001954311564186861697, 0.0003908623128373723394, 0.0005862934692560584820, 0.0007817246256747446788 ),
 .UNSPECIFIED. ) ;
#79069=EDGE_CURVE ( 'NONE', #43756, #74204, #75896, .T. ) ;
#79070=ORIENTED_EDGE ( 'NONE', *, *, #40521, .F. ) ;
#79071=CARTESIAN_POINT ( 'NONE',  ( 17.77707378248385339, -12.39988816332205701, 30.74660775122750778 ) ) ;
#79072=ORIENTED_EDGE ( 'NONE', *, *, #82288, .T. ) ;
#79073=ORIENTED_EDGE ( 'NONE', *, *, #53029, .T. ) ;
#79074=CARTESIAN_POINT ( 'NONE',  ( 0.6845513056318554002, -12.38742843783360748, 31.66772728687926985 ) ) ;
#79075=CARTESIAN_POINT ( 'NONE',  ( 3.296837581771669523, -5.557115091759786019, 34.35708131394839882 ) ) ;
#79076=DIRECTION ( 'NONE',  ( -0.000000000000000000, 0.9396926207859092051, -0.3420201433256662704 ) ) ;
#79077=CARTESIAN_POINT ( 'NONE',  ( 1.384615384615386802, -11.69971097300155272, 32.46337939537588113 ) ) ;
#79078=CYLINDRICAL_SURFACE ( 'NONE', #42342, 0.2500000000000009437 ) ;
#79082=ORIENTED_EDGE ( 'NONE', *, *, #73409, .F. ) ;
#79083=VERTEX_POINT ( 'NONE', #87084 ) ;
#79084=CARTESIAN_POINT ( 'NONE',  ( 12.59158362437324108, -2.504778602574659896, 29.97347330155780654 ) ) ;
#79085=B_SPLINE_CURVE_WITH_KNOTS ( 'NONE', 3,
 ( #77840, #51676, #38186, #51222, #38634, #44480 ),
 .UNSPECIFIED., .F., .F.,
 ( 4, 2, 4 ),
 ( 3.165870343657672947E-17, 0.0001954756301637038194, 0.0003909512603273759801 ),
 .UNSPECIFIED. ) ;
#79087=CARTESIAN_POINT ( 'NONE',  ( 8.899756207464417201, -5.915461855592780260, 34.75538340440931506 ) ) ;
#79088=CARTESIAN_POINT ( 'NONE',  ( -15.10024352900566846, -3.285477652293413264, 32.44071101563363158 ) ) ;
#79089=CYLINDRICAL_SURFACE ( 'NONE', #29238, 0.2499999999999994726 ) ;
#79090=DIRECTION ( 'NONE',  ( -0.000000000000000000, 0.6427876096865404731, -0.7660444431189771253 ) ) ;
#79091=ORIENTED_EDGE ( 'NONE', *, *, #3311, .F. ) ;
#79092=VERTEX_POINT ( 'NONE', #46073 ) ;
#79094=ORIENTED_EDGE ( 'NONE', *, *, #80267, .T. ) ;
#79095=CARTESIAN_POINT ( 'NONE',  ( -10.55012904410859242, -11.94971097300157403, 32.03036669348361443 ) ) ;
#79096=ORIENTED_EDGE ( 'NONE', *, *, #436, .F. ) ;
#79097=DIRECTION ( 'NONE',  ( 0.000000000000000000, 0.8660254037844377084, -0.5000000000000015543 ) ) ;
#79098=FACE_OUTER_BOUND ( 'NONE', #78114, .T. ) ;
#79100=ORIENTED_EDGE ( 'NONE', *, *, #68391, .F. ) ;
#79101=CARTESIAN_POINT ( 'NONE',  ( -13.63459211555773720, -12.17611988154120972, 31.52148481390971213 ) ) ;
#79102=ORIENTED_EDGE ( 'NONE', *, *, #22774, .F. ) ;
#79103=CYLINDRICAL_SURFACE ( 'NONE', #77258, 0.2500000000000009437 ) ;
#79104=B_SPLINE_CURVE_WITH_KNOTS ( 'NONE', 3,
 ( #88255, #54430, #26081, #19768, #87357, #25636, #80596, #73836, #5369, #40929 ),
 .UNSPECIFIED., .F., .F.,
 ( 4, 2, 2, 2, 4 ),
 ( 0.000000000000000000, 0.0001954311564186861697, 0.0003908623128373723394, 0.0005862934692560584820, 0.0007817246256747446788 ),
 .UNSPECIFIED. ) ;
#79105=DIRECTION ( 'NONE',  ( -0.000000000000000000, -0.1736481776669307198, -0.9848077530122080203 ) ) ;
#79107=CARTESIAN_POINT ( 'NONE',  ( -15.00798956179116317, -3.020022701398813236, 32.48759521482552515 ) ) ;
#79108=CARTESIAN_POINT ( 'NONE',  ( 10.68155375634727378, -7.250054483168843156, 34.74374881642865631 ) ) ;
#79109=VECTOR ( 'NONE', #18675, 1000.000000000000000 ) ;
#79110=CARTESIAN_POINT ( 'NONE',  ( -6.792551221313363641, -2.619367082507848554, 30.83698974864644171 ) ) ;
#79111=AXIS2_PLACEMENT_3D ( 'NONE', #19732, #32358, #76330 ) ;
#79112=CARTESIAN_POINT ( 'NONE',  ( 15.93036121012220541, -2.599994579823202923, 30.74605699353653776 ) ) ;
#79113=CARTESIAN_POINT ( 'NONE',  ( 18.22301135161285046, -2.758310577978207778, 31.33698337089302299 ) ) ;
#79114=VERTEX_POINT ( 'NONE', #11858 ) ;
#79115=DIRECTION ( 'NONE',  ( -0.000000000000000000, 0.8660254037844397068, -0.4999999999999978906 ) ) ;
#79116=EDGE_CURVE ( 'NONE', #26024, #31319, #55582, .T. ) ;
#79117=CARTESIAN_POINT ( 'NONE',  ( -8.834500769787091201, -4.320704448112771878, 33.92786785259540494 ) ) ;
#79119=ORIENTED_EDGE ( 'NONE', *, *, #21251, .T. ) ;
#79120=AXIS2_PLACEMENT_3D ( 'NONE', #42122, #677, #69575 ) ;
#79124=CARTESIAN_POINT ( 'NONE',  ( -4.946131269098287930, -5.582136614379148654, 34.36778462344220486 ) ) ;
#79125=DIRECTION ( 'NONE',  ( -0.000000000000000000, 0.5000000000000011102, -0.8660254037844381525 ) ) ;
#79126=DIRECTION ( 'NONE',  ( 0.000000000000000000, 0.9848077530122072432, 0.1736481776669354937 ) ) ;
#79127=CARTESIAN_POINT ( 'NONE',  ( 12.39545505058258001, -4.098570777380720287, 33.41473453929634729 ) ) ;
#79128=FACE_BOUND ( 'NONE', #5415, .T. ) ;
#79129=CARTESIAN_POINT ( 'NONE',  ( 13.25392391794782654, -12.11776431015576172, 31.66791131148498906 ) ) ;
#79130=CARTESIAN_POINT ( 'NONE',  ( -10.83821271301949629, -7.369209533119140509, 34.99857337881830688 ) ) ;
#79131=CARTESIAN_POINT ( 'NONE',  ( -6.923076923076922462, -10.51840700105979565, 33.73612834413961536 ) ) ;
#79132=CARTESIAN_POINT ( 'NONE',  ( -1.253823576790597416, -12.11778462344221019, 31.66786338562085135 ) ) ;
#79133=DIRECTION ( 'NONE',  ( 0.000000000000000000, 0.9396926207859126468, -0.3420201433256571111 ) ) ;
#79134=CARTESIAN_POINT ( 'NONE',  ( 12.46153846153833911, -12.46129190930018460, 30.37095296980731973 ) ) ;
#79135=ADVANCED_FACE ( 'NONE', ( #6856 ), #39775, .F. ) ;
#79138=ORIENTED_EDGE ( 'NONE', *, *, #2106, .T. ) ;
#79139=DIRECTION ( 'NONE',  ( 0.000000000000000000, -6.938893903907222067E-15, 1.000000000000000000 ) ) ;
#79140=EDGE_CURVE ( 'NONE', #25943, #80428, #52280, .T. ) ;
#79141=DIRECTION ( 'NONE',  ( 0.000000000000000000, 0.1736481776669267785, -0.9848077530122087975 ) ) ;
#79142=CARTESIAN_POINT ( 'NONE',  ( -7.622777905455662584, -2.501478030877322567, 29.88021232661720816 ) ) ;
#79143=DIRECTION ( 'NONE',  ( 0.000000000000000000, -0.000000000000000000, -1.000000000000000000 ) ) ;
#79145=CARTESIAN_POINT ( 'NONE',  ( -17.01166793741023042, -8.656820664281605460, 34.87096338111211224 ) ) ;
#79147=CARTESIAN_POINT ( 'NONE',  ( -2.557669051740898425, -3.436278759898155233, 33.07459398097509506 ) ) ;
#79148=CARTESIAN_POINT ( 'NONE',  ( -2.176901866725357237, -6.369690395747422684, 34.87708834333098196 ) ) ;
#79149=ADVANCED_FACE ( 'NONE', ( #41093 ), #41535, .F. ) ;
#79150=CARTESIAN_POINT ( 'NONE',  ( 3.296024370282070404, -4.320704448112861584, 33.92786785259548310 ) ) ;
#79151=CARTESIAN_POINT ( 'NONE',  ( -0.5276208408985972875, -8.164416787775445883, 34.95778746994557906 ) ) ;
#79152=CARTESIAN_POINT ( 'NONE',  ( 6.923076923076802558, -4.481592998941358097, 33.73612834414048933 ) ) ;
#79153=CARTESIAN_POINT ( 'NONE',  ( 5.326977496836529546, -8.346898887586323923, 34.93166121998716278 ) ) ;
#79154=CARTESIAN_POINT ( 'NONE',  ( -18.06608341095587633, -2.721908614388772296, 31.22303859784724978 ) ) ;
#79155=CARTESIAN_POINT ( 'NONE',  ( -23.00000000000000000, -5.499999999999981348, 27.75000000000000000 ) ) ;
#79156=B_SPLINE_CURVE_WITH_KNOTS ( 'NONE', 3,
 ( #60881, #88383, #74, #59993, #47362, #26657, #82504, #27097, #12254, #5951 ),
 .UNSPECIFIED., .F., .F.,
 ( 4, 2, 2, 2, 4 ),
 ( 0.0007817359430256283796, 0.0009771253907249941549, 0.001172514838424359822, 0.001367904286123725489, 0.001563293733823091156 ),
 .UNSPECIFIED. ) ;
#79157=ORIENTED_EDGE ( 'NONE', *, *, #75116, .F. ) ;
#79158=LINE ( 'NONE', #51206, #16829 ) ;
#79159=DIRECTION ( 'NONE',  ( 0.000000000000000000, -6.938893903907222067E-15, 1.000000000000000000 ) ) ;
#79161=EDGE_CURVE ( 'NONE', #66561, #43361, #53265, .T. ) ;
#79163=CARTESIAN_POINT ( 'NONE',  ( 12.46153846153846168, -13.87047571288749737, 32.06866353760679544 ) ) ;
#79164=ORIENTED_EDGE ( 'NONE', *, *, #8657, .F. ) ;
#79165=CARTESIAN_POINT ( 'NONE',  ( -18.00000000000012079, -6.835583212225971650, 34.95778746994575670 ) ) ;
#79166=DIRECTION ( 'NONE',  ( -0.000000000000000000, -0.9396926207859093161, -0.3420201433256663259 ) ) ;
#79167=CARTESIAN_POINT ( 'NONE',  ( 7.976679284387489410, -2.647132371071621471, 31.75357179365171589 ) ) ;
#79168=ORIENTED_EDGE ( 'NONE', *, *, #50980, .T. ) ;
#79169=CARTESIAN_POINT ( 'NONE',  ( -4.153846153846273204, -5.219633306517616589, 34.19971097300220464 ) ) ;
#79170=EDGE_CURVE ( 'NONE', #38474, #54624, #37292, .T. ) ;
#79171=CARTESIAN_POINT ( 'NONE',  ( 16.82692307692307665, -7.500000000000001776, 35.00000000000000000 ) ) ;
#79172=CARTESIAN_POINT ( 'NONE',  ( -5.010854725920638408, -8.973038597847269315, 34.52809138561122637 ) ) ;
#79173=CARTESIAN_POINT ( 'NONE',  ( -15.45363549383233170, -2.251424796025575326, 29.88072029997477586 ) ) ;
#79174=VERTEX_POINT ( 'NONE', #80764 ) ;
#79176=LINE ( 'NONE', #85936, #72478 ) ;
#79177=EDGE_CURVE ( 'NONE', #32825, #53721, #32999, .T. ) ;
#79178=EDGE_CURVE ( 'NONE', #82187, #42382, #7153, .T. ) ;
#79179=AXIS2_PLACEMENT_3D ( 'NONE', #3882, #58831, #85870 ) ;
#79180=CARTESIAN_POINT ( 'NONE',  ( 15.23076923076910916, -10.33852847137269571, 34.16647553114546554 ) ) ;
#79181=EDGE_LOOP ( 'NONE', ( #74158, #64933, #32530, #11550 ) ) ;
#79182=ORIENTED_EDGE ( 'NONE', *, *, #70060, .F. ) ;
#79183=ORIENTED_EDGE ( 'NONE', *, *, #32103, .T. ) ;
#79185=CARTESIAN_POINT ( 'NONE',  ( -9.757578138268467427, -10.21337939537584383, 33.94971097300158647 ) ) ;
#79186=CARTESIAN_POINT ( 'NONE',  ( 6.223012844093394946, -2.308499170217967134, 30.53291367094873721 ) ) ;
#79187=CARTESIAN_POINT ( 'NONE',  ( 13.13463865367303285, -11.28823185664190376, 33.01397839955799896 ) ) ;
#79188=AXIS2_PLACEMENT_3D ( 'NONE', #26326, #6061, #79941 ) ;
#79189=EDGE_CURVE ( 'NONE', #53330, #32867, #69887, .T. ) ;
#79191=B_SPLINE_CURVE_WITH_KNOTS ( 'NONE', 3,
 ( #67852, #33626, #51096, #78591, #77705, #56554, #76833, #64619, #36289, #85361 ),
 .UNSPECIFIED., .F., .F.,
 ( 4, 2, 2, 2, 4 ),
 ( 0.000000000000000000, 0.0001954311564186865492, 0.0003908623128373730983, 0.0005862934692560596746, 0.0007817246256747461966 ),
 .UNSPECIFIED. ) ;
#79193=DIRECTION ( 'NONE',  ( -0.000000000000000000, -0.1736481776669307198, -0.9848077530122080203 ) ) ;
#79195=ADVANCED_FACE ( 'NONE', ( #17497 ), #29359, .F. ) ;
#79196=ORIENTED_EDGE ( 'NONE', *, *, #37618, .F. ) ;
#79197=VERTEX_POINT ( 'NONE', #58458 ) ;
#79198=CARTESIAN_POINT ( 'NONE',  ( -1.134561072977068541, -4.943051570960395047, 34.04725096376909477 ) ) ;
#79200=CARTESIAN_POINT ( 'NONE',  ( -14.05774689831426372, -11.56426240980093745, 33.07394671870546432 ) ) ;
#79202=CARTESIAN_POINT ( 'NONE',  ( 16.15384615384615330, -8.164416787775445883, 34.95778746994557906 ) ) ;
#79203=CARTESIAN_POINT ( 'NONE',  ( 1.634669696253701288, -10.66356715214248396, 33.62249196103329751 ) ) ;
#79204=CARTESIAN_POINT ( 'NONE',  ( -1.319360245102545681, -12.70778746994558439, 30.41441678777537305 ) ) ;
#79205=ORIENTED_EDGE ( 'NONE', *, *, #73884, .F. ) ;
#79206=ORIENTED_EDGE ( 'NONE', *, *, #46074, .T. ) ;
#79207=VERTEX_POINT ( 'NONE', #51695 ) ;
#79208=CARTESIAN_POINT ( 'NONE',  ( -3.230769230769352962, -8.656820664282941280, 34.87096338111179961 ) ) ;
#79209=ORIENTED_EDGE ( 'NONE', *, *, #17387, .T. ) ;
#79210=CARTESIAN_POINT ( 'NONE',  ( -15.23076923076922995, -10.89733346790207413, 36.13435417666054406 ) ) ;
#79211=CARTESIAN_POINT ( 'NONE',  ( 18.06525513951284267, -5.941354392334603496, 34.76329471203374055 ) ) ;
#79213=CARTESIAN_POINT ( 'NONE',  ( 5.076923076923383071, -2.506253911140614576, 30.00000000000323297 ) ) ;
#79215=CARTESIAN_POINT ( 'NONE',  ( 12.46153846153833911, -5.941354392335915335, 34.76329471203413846 ) ) ;
#79216=CARTESIAN_POINT ( 'NONE',  ( -5.869474561766353737, -3.625058011473227815, 33.29252011169590020 ) ) ;
#79217=FACE_BOUND ( 'NONE', #1818, .T. ) ;
#79218=CARTESIAN_POINT ( 'NONE',  ( -5.143005456283212595, -9.905515769479276145, 34.41647553114623292 ) ) ;
#79219=CARTESIAN_POINT ( 'NONE',  ( 2.438484115517094875, -8.147973898785416225, 34.70805048591653730 ) ) ;
#79220=EDGE_CURVE ( 'NONE', #23012, #23399, #28688, .T. ) ;
#79221=CARTESIAN_POINT ( 'NONE',  ( -15.00798968950081758, -10.81320215134717344, 33.49497208177562868 ) ) ;
#79223=CARTESIAN_POINT ( 'NONE',  ( 9.758376043310132530, -3.050289026998446840, 32.03036669348366416 ) ) ;
#79224=B_SPLINE_CURVE_WITH_KNOTS ( 'NONE', 3,
 ( #72919, #29403, #86911, #77132, #70827, #38694, #1915, #86460, #29836, #70380 ),
 .UNSPECIFIED., .F., .F.,
 ( 4, 2, 2, 2, 4 ),
 ( 0.000000000000000000, 0.0001954339857564070678, 0.0003908679715128141356, 0.0005863019572692211492, 0.0007817359430256282712 ),
 .UNSPECIFIED. ) ;
#79227=VERTEX_POINT ( 'NONE', #1873 ) ;
#79228=CARTESIAN_POINT ( 'NONE',  ( 10.36536137809165403, -10.76384336483936011, 33.53834819971076087 ) ) ;
#79229=LINE ( 'NONE', #79671, #23477 ) ;
#79230=ORIENTED_EDGE ( 'NONE', *, *, #13401, .T. ) ;
#79232=CARTESIAN_POINT ( 'NONE',  ( -6.923076923077044142, -8.613356846316285953, 34.62446782046622218 ) ) ;
#79233=CARTESIAN_POINT ( 'NONE',  ( 10.83839745947800992, -11.98016756924215009, 32.48728574198911190 ) ) ;
#79234=CARTESIAN_POINT ( 'NONE',  ( 13.31853300525524908, -11.35647404775217595, 33.31231777344666511 ) ) ;
#79235=DIRECTION ( 'NONE',  ( 0.000000000000000000, 0.8660254037844377084, 0.5000000000000015543 ) ) ;
#79236=CARTESIAN_POINT ( 'NONE',  ( 14.53070515178570510, -11.43677907613344757, 33.22367315496202167 ) ) ;
#79237=VERTEX_POINT ( 'NONE', #15400 ) ;
#79238=CARTESIAN_POINT ( 'NONE',  ( 17.99999999999987566, -2.657715359629662544, 31.77849191805970364 ) ) ;
#79239=CARTESIAN_POINT ( 'NONE',  ( -15.00775787915638126, -9.886259254753566594, 34.14407573483972413 ) ) ;
#79240=LINE ( 'NONE', #39158, #41673 ) ;
#79241=CARTESIAN_POINT ( 'NONE',  ( 10.74591031714818179, -4.459921816937791661, 33.71989282347011851 ) ) ;
#79242=CARTESIAN_POINT ( 'NONE',  ( 2.307692307692309264, -5.471508081941601098, 34.59228464037088457 ) ) ;
#79244=EDGE_LOOP ( 'NONE', ( #4559, #64958, #67572, #83888 ) ) ;
#79246=AXIS2_PLACEMENT_3D ( 'NONE', #75679, #47772, #34254 ) ;
#79247=ORIENTED_EDGE ( 'NONE', *, *, #50345, .T. ) ;
#79248=CARTESIAN_POINT ( 'NONE',  ( -8.096177070375304652, -11.56360843649121684, 33.07473185843129926 ) ) ;
#79250=CARTESIAN_POINT ( 'NONE',  ( -12.46153846153846168, -2.249999999999998668, 29.75000000000001776 ) ) ;
#79251=CARTESIAN_POINT ( 'NONE',  ( 9.822833394071256663, -10.19071101563364756, 33.96452234770658407 ) ) ;
#79253=CARTESIAN_POINT ( 'NONE',  ( 2.057692307692309708, -7.433931650972300353, 34.75000000000000711 ) ) ;
#79256=DIRECTION ( 'NONE',  ( -0.000000000000000000, -0.3420201433256694901, -0.9396926207859082059 ) ) ;
#79257=CARTESIAN_POINT ( 'NONE',  ( 12.46153846153846168, -4.098570777380720287, 33.41473453929634729 ) ) ;
#79258=VERTEX_POINT ( 'NONE', #70784 ) ;
#79259=EDGE_CURVE ( 'NONE', #57187, #24353, #56595, .T. ) ;
#79260=LINE ( 'NONE', #26091, #27183 ) ;
#79261=CARTESIAN_POINT ( 'NONE',  ( -6.130559913613361722, -2.254533558242299396, 29.97296025877828285 ) ) ;
#79262=ORIENTED_EDGE ( 'NONE', *, *, #6205, .T. ) ;
#79263=DIRECTION ( 'NONE',  ( 0.000000000000000000, 0.8660254037844377084, 0.5000000000000015543 ) ) ;
#79264=CARTESIAN_POINT ( 'NONE',  ( -12.46153846153858247, -3.835265460704628371, 33.15142922262033665 ) ) ;
#79265=CARTESIAN_POINT ( 'NONE',  ( 2.057715576749955311, -3.137211980971222669, 32.19342716148376837 ) ) ;
#79266=CARTESIAN_POINT ( 'NONE',  ( 11.66925197942848769, -8.191423895709840863, 34.95447573519442130 ) ) ;
#79267=CARTESIAN_POINT ( 'NONE',  ( -6.130691466667558487, -9.804603061927743113, 34.18744698557895845 ) ) ;
#79268=CARTESIAN_POINT ( 'NONE',  ( 9.442284468086239002, -4.931416488878822335, 34.32920672191015399 ) ) ;
#79269=CARTESIAN_POINT ( 'NONE',  ( -11.53846153846166089, -3.083524468854526912, 32.58852847137268327 ) ) ;
#79271=EDGE_LOOP ( 'NONE', ( #79096, #57428, #84308, #64782 ) ) ;
#79272=CARTESIAN_POINT ( 'NONE',  ( 11.78840705680968171, -11.86320923018887719, 32.19269448109604070 ) ) ;
#79273=DIRECTION ( 'NONE',  ( -0.000000000000000000, 0.8660254037844397068, -0.4999999999999978906 ) ) ;
#79274=CARTESIAN_POINT ( 'NONE',  ( 14.30769230769231015, -2.249999999999998668, 29.50000000000001421 ) ) ;
#79276=CARTESIAN_POINT ( 'NONE',  ( -14.05774678934416499, -5.057305518903948638, 34.11320923018887896 ) ) ;
#79277=CARTESIAN_POINT ( 'NONE',  ( 7.846153846153725020, -6.879047030192662504, 34.71129190930017927 ) ) ;
#79278=FACE_OUTER_BOUND ( 'NONE', #9613, .T. ) ;
#79279=ORIENTED_EDGE ( 'NONE', *, *, #4545, .F. ) ;
#79281=EDGE_CURVE ( 'NONE', #53257, #84227, #84523, .T. ) ;
#79283=VERTEX_POINT ( 'NONE', #70336 ) ;
#79284=DIRECTION ( 'NONE',  ( 0.000000000000000000, 0.1736481776669267785, -0.9848077530122087975 ) ) ;
#79285=ORIENTED_EDGE ( 'NONE', *, *, #85045, .F. ) ;
#79286=VECTOR ( 'NONE', #68986, 1000.000000000000000 ) ;
#79287=CYLINDRICAL_SURFACE ( 'NONE', #19043, 0.2500000000000009437 ) ;
#79288=CARTESIAN_POINT ( 'NONE',  ( -9.561515884482908234, -2.729792928343269587, 31.24908615093345077 ) ) ;
#79289=ADVANCED_FACE ( 'NONE', ( #49171 ), #8643, .F. ) ;
#79290=CARTESIAN_POINT ( 'NONE',  ( 17.01084069756293715, -6.343179335718451384, 34.87096338111212646 ) ) ;
#79291=EDGE_LOOP ( 'NONE', ( #41046, #15715, #51044, #21126 ) ) ;
#79294=ORIENTED_EDGE ( 'NONE', *, *, #13712, .T. ) ;
#79295=CARTESIAN_POINT ( 'NONE',  ( -5.869209559033048862, -2.295524264805589354, 30.44142389570982488 ) ) ;
#79296=ORIENTED_EDGE ( 'NONE', *, *, #65014, .F. ) ;
#79297=CARTESIAN_POINT ( 'NONE',  ( 13.38461538461526601, -11.94971097300221174, 32.03036669348237098 ) ) ;
#79299=VERTEX_POINT ( 'NONE', #69449 ) ;
#79300=CARTESIAN_POINT ( 'NONE',  ( 3.230769230769108269, -11.67786785259630911, 32.92929555188603530 ) ) ;
#79301=CARTESIAN_POINT ( 'NONE',  ( 10.61538461538449596, -3.300289026999228881, 32.46337939537708905 ) ) ;
#79302=CARTESIAN_POINT ( 'NONE',  ( 23.00000000000000000, -4.249999999999998224, 29.75000000000000355 ) ) ;
#79303=DIRECTION ( 'NONE',  ( -0.000000000000000000, 0.9396926207859092051, -0.3420201433256662704 ) ) ;
#79304=CARTESIAN_POINT ( 'NONE',  ( 3.230769230769231726, -7.500000000000001776, 35.04278698407183867 ) ) ;
#79309=ORIENTED_EDGE ( 'NONE', *, *, #42981, .F. ) ;
#79310=CARTESIAN_POINT ( 'NONE',  ( 3.230769230769108269, -12.70778746994576025, 30.41441678777401236 ) ) ;
#79311=VERTEX_POINT ( 'NONE', #80543 ) ;
#79312=CIRCLE ( 'NONE', #40495, 2.000000000000001776 ) ;
#79313=CARTESIAN_POINT ( 'NONE',  ( -17.07692307692319744, -8.656820664282941280, 34.87096338111179961 ) ) ;
#79314=CARTESIAN_POINT ( 'NONE',  ( -10.74607608205217346, -8.999036380462717588, 34.52022231692819076 ) ) ;
#79315=ORIENTED_EDGE ( 'NONE', *, *, #34419, .F. ) ;
#79316=VECTOR ( 'NONE', #5251, 1000.000000000000227 ) ;
#79317=EDGE_LOOP ( 'NONE', ( #68950, #26, #43207, #67673 ) ) ;
#79318=EDGE_LOOP ( 'NONE', ( #39325, #17886 ) ) ;
#79319=CARTESIAN_POINT ( 'NONE',  ( 3.480714749117372442, -5.057305518903949526, 34.11320923018887896 ) ) ;
#79320=ORIENTED_EDGE ( 'NONE', *, *, #20692, .T. ) ;
#79321=DIRECTION ( 'NONE',  ( 0.000000000000000000, 0.3420201433256610524, 0.9396926207859113145 ) ) ;
#79323=CARTESIAN_POINT ( 'NONE',  ( -9.626141085716049872, -7.250054591869670162, 34.99404684341514127 ) ) ;
#79324=FACE_BOUND ( 'NONE', #44210, .T. ) ;
#79325=EDGE_LOOP ( 'NONE', ( #27110, #69702, #16089, #12022 ) ) ;
#79326=CARTESIAN_POINT ( 'NONE',  ( 17.32686848630112308, -6.653508905675593610, 34.93172785388651391 ) ) ;
#79327=CARTESIAN_POINT ( 'NONE',  ( 13.45068373561782415, -8.973038597847271092, 34.52809138561121216 ) ) ;
#79328=CARTESIAN_POINT ( 'NONE',  ( 5.076923076922953193, -3.643525952248796163, 33.31231777344771672 ) ) ;
#79329=CARTESIAN_POINT ( 'NONE',  ( -14.37377571864818648, -8.973038597847271092, 34.52809138561120506 ) ) ;
#79330=CARTESIAN_POINT ( 'NONE',  ( -1.607541602131532077, -2.554751324335734264, 30.48935550225260727 ) ) ;
#79331=ORIENTED_EDGE ( 'NONE', *, *, #32617, .T. ) ;
#79333=VERTEX_POINT ( 'NONE', #39110 ) ;
#79334=EDGE_LOOP ( 'NONE', ( #70429, #64576, #44978, #8498 ) ) ;
#79336=DIRECTION ( 'NONE',  ( 0.000000000000000000, -6.938893903907222067E-15, 1.000000000000000000 ) ) ;
#79338=CARTESIAN_POINT ( 'NONE',  ( -10.61538461538473399, -12.27809138561165270, 31.22303859784587132 ) ) ;
#79339=CARTESIAN_POINT ( 'NONE',  ( -13.60810030917971858, -3.019605429927184836, 32.48692288466676814 ) ) ;
#79340=CARTESIAN_POINT ( 'NONE',  ( 1.607394925883793846, -10.11255958852956027, 34.01340905677048454 ) ) ;
#79341=CARTESIAN_POINT ( 'NONE',  ( 14.30769230769218581, -3.083524468854526912, 32.58852847137268327 ) ) ;
#79343=FACE_OUTER_BOUND ( 'NONE', #73029, .T. ) ;
#79344=CARTESIAN_POINT ( 'NONE',  ( 2.980746006547774218, -9.356822207818506598, 34.66110646841856635 ) ) ;
#79346=CARTESIAN_POINT ( 'NONE',  ( 10.61538461538449596, -11.94971097300221174, 32.03036669348237098 ) ) ;
#79347=AXIS2_PLACEMENT_3D ( 'NONE', #71845, #65531, #10600 ) ;
#79348=ORIENTED_EDGE ( 'NONE', *, *, #30674, .T. ) ;
#79349=ORIENTED_EDGE ( 'NONE', *, *, #11494, .T. ) ;
#79350=FACE_BOUND ( 'NONE', #57459, .T. ) ;
#79352=VERTEX_POINT ( 'NONE', #74668 ) ;
#79354=LINE ( 'NONE', #83240, #66333 ) ;
#79355=EDGE_LOOP ( 'NONE', ( #5943, #3285, #75346, #75483 ) ) ;
#79356=CARTESIAN_POINT ( 'NONE',  ( -16.21911615440247445, -11.67786785259541027, 32.92929555188721480 ) ) ;
#79357=CARTESIAN_POINT ( 'NONE',  ( -10.86536134632696715, -6.567427716900048118, 34.66269422305636283 ) ) ;
#79358=CARTESIAN_POINT ( 'NONE',  ( -8.546219417617917813, -6.503523203565941380, 34.64991518177335195 ) ) ;
#79359=LINE ( 'NONE', #84802, #80746 ) ;
#79360=B_SPLINE_CURVE_WITH_KNOTS ( 'NONE', 3,
 ( #43639, #85083, #30566, #85519, #71996, #51708, #1772, #23797, #29262, #2640 ),
 .UNSPECIFIED., .F., .F.,
 ( 4, 2, 2, 2, 4 ),
 ( 0.0007817359430256319575, 0.0009771253907249984917, 0.001172514838424365026, 0.001367904286123731343, 0.001563293733823097878 ),
 .UNSPECIFIED. ) ;
#79361=CARTESIAN_POINT ( 'NONE',  ( 6.000000000000001776, -1.422936976036506707, 30.56769352161908415 ) ) ;
#79362=ORIENTED_EDGE ( 'NONE', *, *, #35371, .T. ) ;
#79363=ADVANCED_FACE ( 'NONE', ( #60695 ), #67463, .F. ) ;
#79366=FACE_OUTER_BOUND ( 'NONE', #61626, .T. ) ;
#79367=EDGE_CURVE ( 'NONE', #70883, #4654, #85632, .T. ) ;
#79369=CARTESIAN_POINT ( 'NONE',  ( 13.38461538461538680, -10.05456864172156806, 36.03766855953608683 ) ) ;
#79370=CARTESIAN_POINT ( 'NONE',  ( -10.86540783960607293, -3.520140089381495585, 33.17453946501458262 ) ) ;
#79371=CARTESIAN_POINT ( 'NONE',  ( -8.069638789877792817, -9.331801661448606566, 34.40259984581193464 ) ) ;
#79372=LINE ( 'NONE', #24860, #66515 ) ;
#79374=ORIENTED_EDGE ( 'NONE', *, *, #86772, .T. ) ;
#79375=CARTESIAN_POINT ( 'NONE',  ( -3.360916440207450506, -3.285722584762969856, 32.44110544564090759 ) ) ;
#79376=CARTESIAN_POINT ( 'NONE',  ( 2.530705151785705098, -4.026326845037965008, 33.68677907613344047 ) ) ;
#79378=ADVANCED_FACE ( 'NONE', ( #46298 ), #40447, .F. ) ;
#79379=CIRCLE ( 'NONE', #54942, 0.2500000000000002220 ) ;
#79380=EDGE_LOOP ( 'NONE', ( #86531, #31654, #4383, #81123 ) ) ;
#79381=EDGE_LOOP ( 'NONE', ( #71684, #59960, #88118, #71667 ) ) ;
#79382=CARTESIAN_POINT ( 'NONE',  ( 9.822833130541342328, -3.625058011473228703, 33.29252011169590020 ) ) ;
#79384=EDGE_CURVE ( 'NONE', #66553, #30965, #31985, .T. ) ;
#79385=DIRECTION ( 'NONE',  ( 0.000000000000000000, 0.4999999999999985567, 0.8660254037844395958 ) ) ;
#79386=AXIS2_PLACEMENT_3D ( 'NONE', #49262, #68643, #13700 ) ;
#79387=CARTESIAN_POINT ( 'NONE',  ( 10.39245839786846659, -5.667676309546437530, 34.40238873228292249 ) ) ;
#79388=CARTESIAN_POINT ( 'NONE',  ( 10.39189967166066708, -4.386631170607603991, 33.66268669641500111 ) ) ;
#79389=CARTESIAN_POINT ( 'NONE',  ( -16.94639763868943660, -11.66157788607254275, 32.95092075102925833 ) ) ;
#79391=VERTEX_POINT ( 'NONE', #26031 ) ;
#79392=CARTESIAN_POINT ( 'NONE',  ( 3.230769230769231726, -6.386643153685126251, 34.62446782046654192 ) ) ;
#79395=CARTESIAN_POINT ( 'NONE',  ( -5.934854220668035474, -7.750023238201980469, 34.74374492549440419 ) ) ;
#79396=CARTESIAN_POINT ( 'NONE',  ( 17.01083966596719321, -8.973038597847269315, 34.52809138561120506 ) ) ;
#79397=EDGE_LOOP ( 'NONE', ( #1043, #17994, #3753, #82628 ) ) ;
#79398=CARTESIAN_POINT ( 'NONE',  ( 13.51540719244017374, -6.413143153341454017, 34.63066358083362672 ) ) ;
#79399=B_SPLINE_CURVE_WITH_KNOTS ( 'NONE', 3,
 ( #58526, #52669, #31060, #86023, #38277, #18012, #31517, #4492, #11704, #78362 ),
 .UNSPECIFIED., .F., .F.,
 ( 4, 2, 2, 2, 4 ),
 ( 0.0007817246256747503166, 0.0009771112852218946220, 0.001172497944769039036, 0.001367884604316183233, 0.001563271263863327647 ),
 .UNSPECIFIED. ) ;
#79400=ORIENTED_EDGE ( 'NONE', *, *, #37766, .T. ) ;
#79401=B_SPLINE_CURVE_WITH_KNOTS ( 'NONE', 3,
 ( #71055, #30514, #44453, #9369, #65180, #84594, #57538, #71491, #64730, #16553 ),
 .UNSPECIFIED., .F., .F.,
 ( 4, 2, 2, 2, 4 ),
 ( 0.0007817359430256300059, 0.0009771253907249963233, 0.001172514838424362858, 0.001367904286123729392, 0.001563293733823095709 ),
 .UNSPECIFIED. ) ;
#79402=CARTESIAN_POINT ( 'NONE',  ( -17.14219307747939069, -2.657715359629089669, 31.77849191805834295 ) ) ;
#79404=CARTESIAN_POINT ( 'NONE',  ( -1.450698795571263577, -8.973038597847271092, 34.52809138561120506 ) ) ;
#79405=CARTESIAN_POINT ( 'NONE',  ( 6.065255139512838234, -12.16647553114626490, 32.15551576947920864 ) ) ;
#79406=ORIENTED_EDGE ( 'NONE', *, *, #65892, .F. ) ;
#79407=CARTESIAN_POINT ( 'NONE',  ( -4.153846153846273204, -6.026961402154118908, 34.52809138561165270 ) ) ;
#79408=CARTESIAN_POINT ( 'NONE',  ( -1.608100309179715914, -12.69144148231606017, 30.53333754910549303 ) ) ;
#79409=CARTESIAN_POINT ( 'NONE',  ( -10.61538461538473399, -10.90142922262034020, 33.41473453929536674 ) ) ;
#79410=VECTOR ( 'NONE', #14442, 1000.000000000000114 ) ;
#79412=CARTESIAN_POINT ( 'NONE',  ( 3.453548899747294953, -3.020022701398814124, 32.48759521482552515 ) ) ;
#79413=EDGE_CURVE ( 'NONE', #47764, #27494, #43767, .T. ) ;
#79415=CARTESIAN_POINT ( 'NONE',  ( -10.86538461538461675, -2.499999999999999556, 29.81609845454691765 ) ) ;
#79416=EDGE_CURVE ( 'NONE', #79083, #85360, #59363, .T. ) ;
#79417=ORIENTED_EDGE ( 'NONE', *, *, #27727, .T. ) ;
#79418=VECTOR ( 'NONE', #70308, 1000.000000000000000 ) ;
#79419=CARTESIAN_POINT ( 'NONE',  ( -2.437840277424006885, -2.647304123082328875, 31.75400227202885262 ) ) ;
#79420=CARTESIAN_POINT ( 'NONE',  ( 5.076923076923075762, -12.10708131394839349, 31.69288490824020244 ) ) ;
#79423=CARTESIAN_POINT ( 'NONE',  ( 9.915320536401091900, -2.523321265292115534, 31.42251411153756990 ) ) ;
#79426=CARTESIAN_POINT ( 'NONE',  ( 12.68431800280687050, -10.11255958852956027, 34.01340905677048454 ) ) ;
#79427=ORIENTED_EDGE ( 'NONE', *, *, #78349, .T. ) ;
#79428=VERTEX_POINT ( 'NONE', #19275 ) ;
#79432=CARTESIAN_POINT ( 'NONE',  ( -10.55012904410859065, -8.613356846314928816, 34.62446782046653482 ) ) ;
#79433=CARTESIAN_POINT ( 'NONE',  ( -3.480792454990687013, -6.652501968072646932, 34.93155406624980941 ) ) ;
#79434=CARTESIAN_POINT ( 'NONE',  ( -2.177644701436622476, -7.723484964179500700, 34.74522123443823318 ) ) ;
#79435=B_SPLINE_CURVE_WITH_KNOTS ( 'NONE', 3,
 ( #38726, #35744, #18017, #28994, #79272, #15025, #51768, #56449, #45023, #22220 ),
 .UNSPECIFIED., .F., .F.,
 ( 4, 2, 2, 2, 4 ),
 ( 0.0007817359430256388964, 0.0009771253907250073822, 0.001172514838424375868, 0.001367904286123744571, 0.001563293733823113056 ),
 .UNSPECIFIED. ) ;
#79437=CARTESIAN_POINT ( 'NONE',  ( -16.28399336328437386, -2.619462340734462380, 30.83744416345203021 ) ) ;
#79438=CARTESIAN_POINT ( 'NONE',  ( 0.5923302693632468419, -4.809403383903225304, 33.96459661697924304 ) ) ;
#79439=DIRECTION ( 'NONE',  ( 0.000000000000000000, 0.4999999999999985567, 0.8660254037844395958 ) ) ;
#79440=LINE ( 'NONE', #85309, #61030 ) ;
#79441=CARTESIAN_POINT ( 'NONE',  ( -4.403822884788507253, -9.943427161483782584, 34.11278801902876978 ) ) ;
#79442=EDGE_LOOP ( 'NONE', ( #73220, #26063 ) ) ;
#79443=VERTEX_POINT ( 'NONE', #74220 ) ;
#79444=VECTOR ( 'NONE', #53809, 1000.000000000000000 ) ;
#79445=VERTEX_POINT ( 'NONE', #62454 ) ;
#79446=DIRECTION ( 'NONE',  ( 0.000000000000000000, 1.000000000000000000, 0.000000000000000000 ) ) ;
#79447=ORIENTED_EDGE ( 'NONE', *, *, #22450, .T. ) ;
#79448=CARTESIAN_POINT ( 'NONE',  ( 7.780883400193070898, -3.300289026998414865, 32.46337939537583139 ) ) ;
#79449=CARTESIAN_POINT ( 'NONE',  ( -16.21992956480203318, -9.780366693483667717, 34.19971097300155805 ) ) ;
#79450=EDGE_CURVE ( 'NONE', #27477, #75533, #39394, .T. ) ;
#79451=CARTESIAN_POINT ( 'NONE',  ( 12.46153846153846168, -9.819645486525091727, 36.12317359536749706 ) ) ;
#79452=CARTESIAN_POINT ( 'NONE',  ( 7.173022441425066731, -2.587454068350147462, 30.68340429815432202 ) ) ;
#79453=FACE_BOUND ( 'NONE', #81832, .T. ) ;
#79454=VERTEX_POINT ( 'NONE', #69667 ) ;
#79455=EDGE_LOOP ( 'NONE', ( #87797, #28724, #26895, #61028 ) ) ;
#79456=DIRECTION ( 'NONE',  ( -0.000000000000000000, -0.3420201433256694901, -0.9396926207859082059 ) ) ;
#79457=ORIENTED_EDGE ( 'NONE', *, *, #28223, .T. ) ;
#79458=FACE_BOUND ( 'NONE', #17557, .T. ) ;
#79459=LINE ( 'NONE', #17758, #28918 ) ;
#79460=CYLINDRICAL_SURFACE ( 'NONE', #86595, 0.2499999999999997502 ) ;
#79461=VERTEX_POINT ( 'NONE', #75537 ) ;
#79462=CARTESIAN_POINT ( 'NONE',  ( -15.16470087976679970, -12.10708131394839882, 31.69288490824020954 ) ) ;
#79463=CARTESIAN_POINT ( 'NONE',  ( -1.384615384615383471, -8.164416787775445883, 34.95778746994557906 ) ) ;
#79464=CARTESIAN_POINT ( 'NONE',  ( 14.30769230769231015, -13.53365097954675988, 30.81389545987213552 ) ) ;
#79465=ORIENTED_EDGE ( 'NONE', *, *, #86960, .F. ) ;
#79466=CYLINDRICAL_SURFACE ( 'NONE', #12626, 0.2500000000000009437 ) ;
#79467=DIRECTION ( 'NONE',  ( -0.000000000000000000, -0.8660254037844399289, -0.4999999999999980016 ) ) ;
#79468=ORIENTED_EDGE ( 'NONE', *, *, #21445, .F. ) ;
#79470=CARTESIAN_POINT ( 'NONE',  ( 2.057692307692309708, -7.500000000000001776, 34.75000000000000000 ) ) ;
#79471=DIRECTION ( 'NONE',  ( -0.000000000000000000, 0.9396926207859092051, -0.3420201433256662704 ) ) ;
#79473=ORIENTED_EDGE ( 'NONE', *, *, #67323, .T. ) ;
#79474=CARTESIAN_POINT ( 'NONE',  ( 3.230769230769108269, -6.835583212225970762, 34.95778746994575670 ) ) ;
#79475=CARTESIAN_POINT ( 'NONE',  ( 13.31934493865461278, -2.625532179533445198, 30.86335684631481513 ) ) ;
#79476=CARTESIAN_POINT ( 'NONE',  ( 16.02315555073584008, -2.845849958028613624, 32.17971566917920967 ) ) ;
#79477=B_SPLINE_CURVE_WITH_KNOTS ( 'NONE', 3,
 ( #4502, #67541, #73861, #31980, #5840, #81067, #19351, #4041, #59445, #47257 ),
 .UNSPECIFIED., .F., .F.,
 ( 4, 2, 2, 2, 4 ),
 ( 0.0007817246336856289524, 0.0009771112958940101571, 0.001172497958102391253, 0.001367884620310772350, 0.001563271282519153446 ),
 .UNSPECIFIED. ) ;
#79479=CARTESIAN_POINT ( 'NONE',  ( 9.442284468086237226, -12.45566812827425451, 31.48439005359158926 ) ) ;
#79480=CARTESIAN_POINT ( 'NONE',  ( -0.2381629757660416458, -2.251407671071270489, 29.88021292934942963 ) ) ;
#79481=CARTESIAN_POINT ( 'NONE',  ( -1.634638621908350631, -2.823816976329317718, 31.52131813110795733 ) ) ;
#79483=CARTESIAN_POINT ( 'NONE',  ( 8.992010310499175318, -12.24180327182771855, 31.33663988360758879 ) ) ;
#79484=CARTESIAN_POINT ( 'NONE',  ( 3.230769230769538147, -2.506253911140615021, 30.00000000000323297 ) ) ;
#79485=CARTESIAN_POINT ( 'NONE',  ( -10.83831083290076158, -8.239355502252617924, 34.69524867566427417 ) ) ;
#79488=DIRECTION ( 'NONE',  ( -0.000000000000000000, 0.3420201433256694901, -0.9396926207859082059 ) ) ;
#79489=ORIENTED_EDGE ( 'NONE', *, *, #33618, .F. ) ;
#79490=EDGE_CURVE ( 'NONE', #30370, #11900, #2823, .T. ) ;
#79491=EDGE_LOOP ( 'NONE', ( #39531, #2769 ) ) ;
#79492=CARTESIAN_POINT ( 'NONE',  ( -1.384615384615383471, -1.466349020453238561, 30.81389545987213907 ) ) ;
#79494=CARTESIAN_POINT ( 'NONE',  ( -18.00000000000012079, -12.46129190930018460, 30.37095296980731973 ) ) ;
#79496=CARTESIAN_POINT ( 'NONE',  ( -5.076923076923197442, -11.48612834414049644, 32.76840700105863391 ) ) ;
#79497=EDGE_CURVE ( 'NONE', #20943, #1690, #62893, .T. ) ;
#79498=CARTESIAN_POINT ( 'NONE',  ( 5.999999999999880096, -11.48612834414049644, 32.76840700105863391 ) ) ;
#79500=CARTESIAN_POINT ( 'NONE',  ( -12.33101302330481985, -4.299079248970732792, 33.91157788607253565 ) ) ;
#79501=CARTESIAN_POINT ( 'NONE',  ( 1.384615384615386802, -12.78798330534102767, 29.49999999999997868 ) ) ;
#79502=DIRECTION ( 'NONE',  ( 0.000000000000000000, 0.9396926207859126468, 0.3420201433256571111 ) ) ;
#79503=DIRECTION ( 'NONE',  ( -1.000000000000000000, 0.000000000000000000, 0.000000000000000000 ) ) ;
#79505=DIRECTION ( 'NONE',  ( 0.000000000000000000, 0.3420201433256610524, 0.9396926207859113145 ) ) ;
#79506=CARTESIAN_POINT ( 'NONE',  ( -15.00798968950081758, -2.600157965045224451, 30.74683119005207743 ) ) ;
#79507=EDGE_CURVE ( 'NONE', #76524, #22606, #1207, .T. ) ;
#79508=DIRECTION ( 'NONE',  ( -0.000000000000000000, 0.5000000000000011102, -0.8660254037844380415 ) ) ;
#79509=VECTOR ( 'NONE', #87591, 1000.000000000000000 ) ;
#79510=EDGE_CURVE ( 'NONE', #61245, #28895, #88644, .T. ) ;
#79511=ORIENTED_EDGE ( 'NONE', *, *, #43828, .F. ) ;
#79512=ORIENTED_EDGE ( 'NONE', *, *, #58103, .T. ) ;
#79513=CARTESIAN_POINT ( 'NONE',  ( -2.307692307692305711, -12.78798330534103123, 29.99999999999997868 ) ) ;
#79514=CARTESIAN_POINT ( 'NONE',  ( -17.07692307692307665, -8.120952969808772792, 34.71129190930000163 ) ) ;
#79515=CYLINDRICAL_SURFACE ( 'NONE', #16700, 0.2500000000000008882 ) ;
#79518=CARTESIAN_POINT ( 'NONE',  ( 3.930919194939304084, -3.395401636524186362, 33.02366814457250399 ) ) ;
#79519=AXIS2_PLACEMENT_3D ( 'NONE', #76185, #21687, #55037 ) ;
#79521=EDGE_CURVE ( 'NONE', #49031, #15672, #28619, .T. ) ;
#79522=ORIENTED_EDGE ( 'NONE', *, *, #52518, .T. ) ;
#79523=CARTESIAN_POINT ( 'NONE',  ( 17.77651505627605033, -12.44517049084099725, 30.48991314939691932 ) ) ;
#79525=EDGE_CURVE ( 'NONE', #25295, #2963, #769, .T. ) ;
#79526=ORIENTED_EDGE ( 'NONE', *, *, #74241, .T. ) ;
#79527=CARTESIAN_POINT ( 'NONE',  ( 10.61538461538461675, -12.48256725967547354, 35.29906147534542527 ) ) ;
#79528=CARTESIAN_POINT ( 'NONE',  ( 6.066169140962657913, -7.250054483168843156, 34.74374881642865631 ) ) ;
#79529=CARTESIAN_POINT ( 'NONE',  ( -0.3953718549468210330, -7.250054591869666609, 34.99404684341514127 ) ) ;
#79530=EDGE_CURVE ( 'NONE', #48470, #70777, #32926, .T. ) ;
#79531=B_SPLINE_CURVE_WITH_KNOTS ( 'NONE', 3,
 ( #3503, #26456, #48038, #41743, #53919, #21009, #47156, #13818, #6622, #61116 ),
 .UNSPECIFIED., .F., .F.,
 ( 4, 2, 2, 2, 4 ),
 ( 0.000000000000000000, 0.0001954311564186863865, 0.0003908623128373727731, 0.0005862934692560591325, 0.0007817246256747455461 ),
 .UNSPECIFIED. ) ;
#79534=ORIENTED_EDGE ( 'NONE', *, *, #13780, .T. ) ;
#79536=AXIS2_PLACEMENT_3D ( 'NONE', #50447, #42394, #83373 ) ;
#79538=ORIENTED_EDGE ( 'NONE', *, *, #58844, .T. ) ;
#79539=CARTESIAN_POINT ( 'NONE',  ( -4.087778820496075660, -11.91647553114624358, 32.58852847137148245 ) ) ;
#79541=EDGE_CURVE ( 'NONE', #30860, #88554, #86281, .T. ) ;
#79542=CARTESIAN_POINT ( 'NONE',  ( -6.923076923076922462, -8.318370150425687726, 35.83090037661290239 ) ) ;
#79543=CARTESIAN_POINT ( 'NONE',  ( 10.61538461538449596, -10.90142922262034020, 33.41473453929536674 ) ) ;
#79544=EDGE_CURVE ( 'NONE', #87443, #24897, #10186, .T. ) ;
#79548=ORIENTED_EDGE ( 'NONE', *, *, #59227, .T. ) ;
#79551=CARTESIAN_POINT ( 'NONE',  ( -13.44988538517170440, -5.941354392334499579, 34.76329471203369792 ) ) ;
#79552=EDGE_LOOP ( 'NONE', ( #35260, #42401 ) ) ;
#79553=CARTESIAN_POINT ( 'NONE',  ( 1.319344938654610555, -10.21337939537584205, 33.94971097300158647 ) ) ;
#79554=CARTESIAN_POINT ( 'NONE',  ( 12.52760579488853665, -8.164416787775445883, 34.95778746994558617 ) ) ;
#79555=EDGE_CURVE ( 'NONE', #62627, #79057, #81281, .T. ) ;
#79557=VERTEX_POINT ( 'NONE', #84090 ) ;
#79558=CARTESIAN_POINT ( 'NONE',  ( 10.68063975489745232, -2.379036618887895305, 30.90682066428158592 ) ) ;
#79559=VERTEX_POINT ( 'NONE', #51584 ) ;
#79561=CARTESIAN_POINT ( 'NONE',  ( 5.776515075435672664, -9.417330523894424488, 34.63758898049880486 ) ) ;
#79562=CARTESIAN_POINT ( 'NONE',  ( -6.923076923076922462, -2.721908614388771852, 31.22303859784724978 ) ) ;
#79563=DIRECTION ( 'NONE',  ( 0.000000000000000000, 0.1736481776669267785, -0.9848077530122087975 ) ) ;
#79564=CARTESIAN_POINT ( 'NONE',  ( -0.4615384615385840772, -11.67786785259630911, 32.92929555188603530 ) ) ;
#79565=CARTESIAN_POINT ( 'NONE',  ( 7.846153846153723244, -2.379036618888197729, 30.90682066428292885 ) ) ;
#79566=EDGE_CURVE ( 'NONE', #47342, #19850, #85404, .T. ) ;
#79569=DIRECTION ( 'NONE',  ( -1.000000000000000000, 0.000000000000000000, 0.000000000000000000 ) ) ;
#79570=ORIENTED_EDGE ( 'NONE', *, *, #2524, .T. ) ;
#79571=CARTESIAN_POINT ( 'NONE',  ( -11.47320639894870276, -8.656820664281605460, 34.87096338111211224 ) ) ;
#79572=CARTESIAN_POINT ( 'NONE',  ( 3.230769230769110045, -4.481592998941358097, 33.73612834414048933 ) ) ;
#79575=CARTESIAN_POINT ( 'NONE',  ( 2.307692307692309264, -10.51840700105979565, 33.73612834413961536 ) ) ;
#79576=DIRECTION ( 'NONE',  ( -0.000000000000000000, 0.3420201433256694901, -0.9396926207859082059 ) ) ;
#79577=CARTESIAN_POINT ( 'NONE',  ( -6.130147209438218781, -10.88202310037935661, 33.43294751532457099 ) ) ;
#79578=CARTESIAN_POINT ( 'NONE',  ( 11.53846153846153832, -5.557115091759785130, 34.35708131394839171 ) ) ;
#79579=CARTESIAN_POINT ( 'NONE',  ( 7.780070435197965928, -8.120952969808774569, 34.71129190930000163 ) ) ;
#79580=FACE_BOUND ( 'NONE', #68597, .T. ) ;
#79581=CARTESIAN_POINT ( 'NONE',  ( 12.23861224402230619, -3.105860786376062332, 32.13614157043599562 ) ) ;
#79582=DIRECTION ( 'NONE',  ( -0.000000000000000000, 0.9848077530122086864, -0.1736481776669273891 ) ) ;
#79584=CARTESIAN_POINT ( 'NONE',  ( -1.384615384615505151, -12.27809138561165270, 31.22303859784587132 ) ) ;
#79585=CARTESIAN_POINT ( 'NONE',  ( 14.08420738312797660, -10.97335522853832579, 33.68706563782419749 ) ) ;
#79586=DIRECTION ( 'NONE',  ( 0.000000000000000000, 0.4999999999999960032, -0.8660254037844410391 ) ) ;
#79589=ORIENTED_EDGE ( 'NONE', *, *, #38338, .F. ) ;
#79591=CARTESIAN_POINT ( 'NONE',  ( 16.21910129335899597, -12.70778746994558439, 30.41441678777537305 ) ) ;
#79592=CARTESIAN_POINT ( 'NONE',  ( 11.53846153846153832, -6.189225973068211317, 35.74407628777942847 ) ) ;
#79593=CARTESIAN_POINT ( 'NONE',  ( -13.13461538461538325, -2.499999999999998668, 29.75000000000000355 ) ) ;
#79595=CARTESIAN_POINT ( 'NONE',  ( -12.52762084089859407, -6.343179335718451384, 34.87096338111212646 ) ) ;
#79597=ADVANCED_FACE ( 'NONE', ( #43084 ), #51139, .F. ) ;
#79598=CARTESIAN_POINT ( 'NONE',  ( -15.45425415533356350, -12.69144148231606017, 30.53333754910549303 ) ) ;
#79599=CARTESIAN_POINT ( 'NONE',  ( 0.5276068125408995835, -3.513871655860379306, 32.76840700105978499 ) ) ;
#79601=DIRECTION ( 'NONE',  ( -0.000000000000000000, 1.000000000000000000, 3.491481338843133355E-15 ) ) ;
#79602=CARTESIAN_POINT ( 'NONE',  ( -7.053768389744480061, -4.118384482072085184, 33.43331474514187107 ) ) ;
#79603=DIRECTION ( 'NONE',  ( 0.000000000000000000, 0.4999999999999985567, 0.8660254037844395958 ) ) ;
#79604=CARTESIAN_POINT ( 'NONE',  ( -6.000000000000121680, -12.16647553114689728, 32.15551576947799362 ) ) ;
#79606=EDGE_LOOP ( 'NONE', ( #83425, #23166 ) ) ;
#79607=CARTESIAN_POINT ( 'NONE',  ( 17.20744851515672025, -12.70449254468099198, 30.44128974285582956 ) ) ;
#79608=CARTESIAN_POINT ( 'NONE',  ( 6.923076923076802558, -5.219633306517616589, 34.19971097300220464 ) ) ;
#79610=CARTESIAN_POINT ( 'NONE',  ( 2.084207363968360038, -4.386631170607603991, 33.66268669641500111 ) ) ;
#79611=CARTESIAN_POINT ( 'NONE',  ( 6.923076923076800782, -4.320704448113951379, 33.92786785259630022 ) ) ;
#79612=ORIENTED_EDGE ( 'NONE', *, *, #10063, .T. ) ;
#79613=CARTESIAN_POINT ( 'NONE',  ( -18.00000000000012079, -9.442884908241554243, 34.35708131394783038 ) ) ;
#79616=ORIENTED_EDGE ( 'NONE', *, *, #53356, .F. ) ;
#79618=LINE ( 'NONE', #72846, #32567 ) ;
#79620=CARTESIAN_POINT ( 'NONE',  ( -11.78843828251013015, -2.544273027872575366, 31.48422191005632342 ) ) ;
#79621=EDGE_LOOP ( 'NONE', ( #76873, #80244, #31688, #79285 ) ) ;
#79622=LINE ( 'NONE', #73309, #23141 ) ;
#79623=CARTESIAN_POINT ( 'NONE',  ( 10.61538461538461675, -3.937682226553329556, 33.60647404775216529 ) ) ;
#79624=AXIS2_PLACEMENT_3D ( 'NONE', #27911, #20709, #53268 ) ;
#79625=ADVANCED_FACE ( 'NONE', ( #2522 ), #63350, .F. ) ;
#79626=CARTESIAN_POINT ( 'NONE',  ( -1.134561072977069651, -5.728107161865378494, 34.42597550085002922 ) ) ;
#79629=ADVANCED_FACE ( 'NONE', ( #78637 ), #64666, .F. ) ;
#79631=AXIS2_PLACEMENT_3D ( 'NONE', #26787, #35314, #646 ) ;
#79632=CARTESIAN_POINT ( 'NONE',  ( -9.822454901745912181, -10.19110544564092002, 33.96427741523702792 ) ) ;
#79633=CARTESIAN_POINT ( 'NONE',  ( 16.15384615384615330, -2.499999999999998668, 29.75000000000001421 ) ) ;
#79634=EDGE_CURVE ( 'NONE', #62369, #63637, #63063, .T. ) ;
#79635=FACE_OUTER_BOUND ( 'NONE', #73446, .T. ) ;
#79636=EDGE_CURVE ( 'NONE', #73637, #67905, #36334, .T. ) ;
#79637=CARTESIAN_POINT ( 'NONE',  ( 15.23076923076911093, -3.835265460704628371, 33.15142922262033665 ) ) ;
#79638=B_SPLINE_CURVE_WITH_KNOTS ( 'NONE', 3,
 ( #48124, #7150, #14346, #399, #67969, #21092, #27861, #6272, #62517, #14802 ),
 .UNSPECIFIED., .F., .F.,
 ( 4, 2, 2, 2, 4 ),
 ( 0.0007817359430256252354, 0.0009771253907249898181, 0.001172514838424354401, 0.001367904286123718983, 0.001563293733823083566 ),
 .UNSPECIFIED. ) ;
#79639=ORIENTED_EDGE ( 'NONE', *, *, #52696, .T. ) ;
#79640=EDGE_LOOP ( 'NONE', ( #13073, #18288, #66793, #35115 ) ) ;
#79641=CARTESIAN_POINT ( 'NONE',  ( 4.219101293358989757, -5.941354392334606160, 34.76329471203374055 ) ) ;
#79642=ORIENTED_EDGE ( 'NONE', *, *, #80772, .T. ) ;
#79643=CARTESIAN_POINT ( 'NONE',  ( -16.15384615384615330, -12.34228464037088635, 31.77849191805839268 ) ) ;
#79645=CARTESIAN_POINT ( 'NONE',  ( -3.453696189676079609, -4.762599654559228846, 34.23009711892697737 ) ) ;
#79646=CARTESIAN_POINT ( 'NONE',  ( 1.607626736228235931, -10.61302985866383963, 33.66295027996417843 ) ) ;
#79648=ORIENTED_EDGE ( 'NONE', *, *, #39023, .T. ) ;
#79649=ORIENTED_EDGE ( 'NONE', *, *, #62675, .F. ) ;
#79650=AXIS2_PLACEMENT_3D ( 'NONE', #3663, #78885, #38802 ) ;
#79651=ORIENTED_EDGE ( 'NONE', *, *, #37866, .F. ) ;
#79653=VERTEX_POINT ( 'NONE', #16055 ) ;
#79654=CARTESIAN_POINT ( 'NONE',  ( 18.06606733335007675, -11.91647553114624358, 32.58852847137148245 ) ) ;
#79657=CARTESIAN_POINT ( 'NONE',  ( 15.23076923076923173, -13.53365097954675988, 30.81389545987213552 ) ) ;
#79658=LINE ( 'NONE', #59382, #58017 ) ;
#79659=LINE ( 'NONE', #45413, #13787 ) ;
#79660=FACE_BOUND ( 'NONE', #42438, .T. ) ;
#79663=CARTESIAN_POINT ( 'NONE',  ( -6.673022503163470454, -9.233818618650603938, 34.70587769442853698 ) ) ;
#79664=CARTESIAN_POINT ( 'NONE',  ( -8.069080063669993308, -12.15238873228292071, 31.58232369045353849 ) ) ;
#79665=CARTESIAN_POINT ( 'NONE',  ( 16.21910129335899597, -4.320704448112858032, 33.92786785259548310 ) ) ;
#79666=CARTESIAN_POINT ( 'NONE',  ( -8.546217925137376881, -11.98016756924215009, 32.48728574198911190 ) ) ;
#79667=CARTESIAN_POINT ( 'NONE',  ( -8.096130577096198877, -3.137211980971221781, 32.19342716148376837 ) ) ;
#79668=LINE ( 'NONE', #72901, #69215 ) ;
#79669=ORIENTED_EDGE ( 'NONE', *, *, #37773, .T. ) ;
#79670=CARTESIAN_POINT ( 'NONE',  ( 2.530703659305158837, -6.503523203565942268, 34.64991518177335195 ) ) ;
#79671=CARTESIAN_POINT ( 'NONE',  ( -17.07692307692307665, -10.05456864172156806, 36.03766855953608683 ) ) ;
#79672=ORIENTED_EDGE ( 'NONE', *, *, #86418, .F. ) ;
#79673=ORIENTED_EDGE ( 'NONE', *, *, #45752, .T. ) ;
#79674=CARTESIAN_POINT ( 'NONE',  ( -6.857008572074484221, -8.120952969808772792, 34.71129190929999453 ) ) ;
#79675=CARTESIAN_POINT ( 'NONE',  ( -5.869474298236433185, -12.27024696741798770, 31.24895572276497546 ) ) ;
#79676=EDGE_CURVE ( 'NONE', #10584, #49301, #20102, .T. ) ;
#79677=CARTESIAN_POINT ( 'NONE',  ( -13.51522574423990974, -7.722926236386453702, 34.74524107206102030 ) ) ;
#79678=DIRECTION ( 'NONE',  ( -0.000000000000000000, 0.9396926207859093161, -0.3420201433256663259 ) ) ;
#79679=CARTESIAN_POINT ( 'NONE',  ( 12.21151523731700550, -10.92453946501458795, 33.72985991061850086 ) ) ;
#79680=VERTEX_POINT ( 'NONE', #52047 ) ;
#79681=CARTESIAN_POINT ( 'NONE',  ( -6.923076923076922462, -12.48256725967547354, 35.29906147534542527 ) ) ;
#79682=CARTESIAN_POINT ( 'NONE',  ( 4.284371592079797786, -5.070358843744210198, 34.40418822224088302 ) ) ;
#79683=VECTOR ( 'NONE', #37098, 1000.000000000000114 ) ;
#79685=DIRECTION ( 'NONE',  ( 0.000000000000000000, 0.4999999999999985567, 0.8660254037844395958 ) ) ;
#79686=CARTESIAN_POINT ( 'NONE',  ( 15.00728430620490172, -10.97335522853832579, 33.68706563782419749 ) ) ;
#79687=CARTESIAN_POINT ( 'NONE',  ( 7.846153846153846700, -5.557115091759785130, 34.35708131394839171 ) ) ;
#79688=CARTESIAN_POINT ( 'NONE',  ( 10.74617642320940725, -4.118422570099828484, 33.43335022499816489 ) ) ;
#79689=CARTESIAN_POINT ( 'NONE',  ( -14.98071481085577972, -10.82426656108012075, 33.81400080652039009 ) ) ;
#79691=VERTEX_POINT ( 'NONE', #52493 ) ;
#79693=ORIENTED_EDGE ( 'NONE', *, *, #52998, .T. ) ;
#79694=AXIS2_PLACEMENT_3D ( 'NONE', #48523, #82336, #81896 ) ;
#79695=CARTESIAN_POINT ( 'NONE',  ( -8.069638770718174925, -11.60425143139329940, 33.02411095842164457 ) ) ;
#79696=CARTESIAN_POINT ( 'NONE',  ( -7.053768389744483613, -2.541943142973490666, 30.39792223712631980 ) ) ;
#79697=CARTESIAN_POINT ( 'NONE',  ( 9.942253210655836781, -10.05730279482229683, 34.04704008940765902 ) ) ;
#79698=CYLINDRICAL_SURFACE ( 'NONE', #59662, 0.2500000000000008882 ) ;
#79699=CARTESIAN_POINT ( 'NONE',  ( 16.94644789184735956, -7.276987145209182550, 34.99546412871779211 ) ) ;
#79701=EDGE_CURVE ( 'NONE', #22384, #41958, #76960, .T. ) ;
#79702=B_SPLINE_CURVE_WITH_KNOTS ( 'NONE', 3,
 ( #3087, #28815, #84645, #84209, #9415, #63465, #76552, #50819, #56275, #1329 ),
 .UNSPECIFIED., .F., .F.,
 ( 4, 2, 2, 2, 4 ),
 ( 0.0007817359430256257775, 0.0009771253907249911191, 0.001172514838424356352, 0.001367904286123721586, 0.001563293733823086819 ),
 .UNSPECIFIED. ) ;
#79703=CARTESIAN_POINT ( 'NONE',  ( 8.545745844666436497, -4.225889041578353655, 33.85425143139329407 ) ) ;
#79704=DIRECTION ( 'NONE',  ( -0.000000000000000000, 0.9396926207859092051, -0.3420201433256662704 ) ) ;
#79705=CARTESIAN_POINT ( 'NONE',  ( 7.846153846153846700, -1.044019251281081972, 31.83374038241031911 ) ) ;
#79706=DIRECTION ( 'NONE',  ( -0.000000000000000000, -0.9396926207859093161, -0.3420201433256663259 ) ) ;
#79708=CARTESIAN_POINT ( 'NONE',  ( 14.08420736396836048, -12.24155766932282496, 31.33739205006857986 ) ) ;
#79711=LINE ( 'NONE', #44563, #53836 ) ;
#79712=CARTESIAN_POINT ( 'NONE',  ( 7.145856592054988354, -2.353885683473779800, 30.79025554430704759 ) ) ;
#79713=CARTESIAN_POINT ( 'NONE',  ( 10.68145296638705588, -2.721908614388771852, 31.22303859784725333 ) ) ;
#79714=CARTESIAN_POINT ( 'NONE',  ( 7.596130621932389637, -3.520140089381496473, 33.17453946501458262 ) ) ;
#79715=CARTESIAN_POINT ( 'NONE',  ( -7.596208327805704208, -12.43552623307873972, 30.55307653245132826 ) ) ;
#79716=ORIENTED_EDGE ( 'NONE', *, *, #44342, .F. ) ;
#79717=EDGE_CURVE ( 'NONE', #41880, #77905, #46195, .T. ) ;
#79719=CARTESIAN_POINT ( 'NONE',  ( -5.299751174557954414, -7.369209533119140509, 34.99857337881830688 ) ) ;
#79720=CARTESIAN_POINT ( 'NONE',  ( 5.777073041093152561, -2.523278758544489797, 31.42238647778637528 ) ) ;
#79722=CARTESIAN_POINT ( 'NONE',  ( -18.24999999999999645, -2.499999999999999556, 29.81609845454691410 ) ) ;
#79723=CARTESIAN_POINT ( 'NONE',  ( 16.15384615384615330, -4.661471528628507777, 34.16647553114623292 ) ) ;
#79724=CARTESIAN_POINT ( 'NONE',  ( -0.4615384615384611200, -2.538708090699994813, 30.37095296980875503 ) ) ;
#79725=EDGE_LOOP ( 'NONE', ( #36470, #53648, #48764, #49292 ) ) ;
#79727=CARTESIAN_POINT ( 'NONE',  ( -7.846153846153844924, -11.35647404775217417, 33.31231777344666511 ) ) ;
#79729=AXIS2_PLACEMENT_3D ( 'NONE', #492, #63060, #84252 ) ;
#79730=LINE ( 'NONE', #18030, #70167 ) ;
#79731=ORIENTED_EDGE ( 'NONE', *, *, #26011, .F. ) ;
#79732=CARTESIAN_POINT ( 'NONE',  ( 2.980792486720639900, -4.818429247618089661, 34.26397095200675125 ) ) ;
#79733=DIRECTION ( 'NONE',  ( -0.000000000000000000, -0.000000000000000000, -1.000000000000000000 ) ) ;
#79734=DIRECTION ( 'NONE',  ( -0.000000000000000000, -0.000000000000000000, -1.000000000000000000 ) ) ;
#79735=VERTEX_POINT ( 'NONE', #25920 ) ;
#79736=CARTESIAN_POINT ( 'NONE',  ( 11.47237915910140771, -11.91647553114624181, 32.58852847137148245 ) ) ;
#79737=VERTEX_POINT ( 'NONE', #3859 ) ;
#79738=CARTESIAN_POINT ( 'NONE',  ( 11.40777007179397984, -3.530157926970578952, 32.79014554554150607 ) ) ;
#79739=B_SPLINE_CURVE_WITH_KNOTS ( 'NONE', 3,
 ( #68023, #5436, #60811, #88316, #32899, #20711, #60365, #48175, #54045, #54490 ),
 .UNSPECIFIED., .F., .F.,
 ( 4, 2, 2, 2, 4 ),
 ( 0.0007817359430256322827, 0.0009771253907249989254, 0.001172514838424365676, 0.001367904286123732428, 0.001563293733823099179 ),
 .UNSPECIFIED. ) ;
#79740=B_SPLINE_CURVE_WITH_KNOTS ( 'NONE', 3,
 ( #28552, #7397, #8282, #14144, #8727, #35301, #47926, #56461, #15038, #6942 ),
 .UNSPECIFIED., .F., .F.,
 ( 4, 2, 2, 2, 4 ),
 ( 0.000000000000000000, 0.0001954311564186864949, 0.0003908623128373729899, 0.0005862934692560594577, 0.0007817246256747459798 ),
 .UNSPECIFIED. ) ;
#79742=ORIENTED_EDGE ( 'NONE', *, *, #6285, .T. ) ;
#79743=CARTESIAN_POINT ( 'NONE',  ( 13.51514108637895184, -11.93748526763465279, 32.05452791011430946 ) ) ;
#79744=DIRECTION ( 'NONE',  ( -0.000000000000000000, 0.9848077530122085754, -0.1736481776669273613 ) ) ;
#79745=B_SPLINE_CURVE_WITH_KNOTS ( 'NONE', 3,
 ( #86926, #39615, #81040, #18442, #74273, #4478 ),
 .UNSPECIFIED., .F., .F.,
 ( 4, 2, 4 ),
 ( 0.0003909569690057842790, 0.0005862646681846108007, 0.0007815723673634373224 ),
 .UNSPECIFIED. ) ;
#79746=VERTEX_POINT ( 'NONE', #4313 ) ;
#79747=CYLINDRICAL_SURFACE ( 'NONE', #49055, 0.2500000000000004996 ) ;
#79748=DIRECTION ( 'NONE',  ( -0.000000000000000000, 0.6427876096865404731, -0.7660444431189770143 ) ) ;
#79749=CARTESIAN_POINT ( 'NONE',  ( 0.3954560821783241198, -2.292212530054419606, 30.41441678777542634 ) ) ;
#79750=EDGE_CURVE ( 'NONE', #67601, #51593, #86723, .T. ) ;
#79751=CARTESIAN_POINT ( 'NONE',  ( -14.08491263871423982, -10.23759521482555357, 34.22997729860117033 ) ) ;
#79752=CARTESIAN_POINT ( 'NONE',  ( 16.15384615384615330, -10.89733346790207413, 36.13435417666054406 ) ) ;
#79753=VECTOR ( 'NONE', #58598, 1000.000000000000000 ) ;
#79755=ORIENTED_EDGE ( 'NONE', *, *, #44155, .T. ) ;
#79756=ORIENTED_EDGE ( 'NONE', *, *, #61807, .T. ) ;
#79757=FACE_OUTER_BOUND ( 'NONE', #44274, .T. ) ;
#79758=EDGE_LOOP ( 'NONE', ( #6553, #13835, #82455, #81673 ) ) ;
#79759=EDGE_CURVE ( 'NONE', #47629, #8176, #29742, .T. ) ;
#79760=AXIS2_PLACEMENT_3D ( 'NONE', #4870, #19267, #60240 ) ;
#79761=VECTOR ( 'NONE', #71815, 1000.000000000000114 ) ;
#79762=CARTESIAN_POINT ( 'NONE',  ( 10.48523740594639619, -5.195881422630166391, 34.18770438780619259 ) ) ;
#79763=CARTESIAN_POINT ( 'NONE',  ( -10.74553182482283198, -9.418419913701741919, 34.36755862841477693 ) ) ;
#79764=ORIENTED_EDGE ( 'NONE', *, *, #85385, .F. ) ;
#79765=ADVANCED_FACE ( 'NONE', ( #88103 ), #26368, .F. ) ;
#79766=EDGE_LOOP ( 'NONE', ( #5044, #18381 ) ) ;
#79767=CARTESIAN_POINT ( 'NONE',  ( 3.453548772037639214, -5.114059244376869984, 34.14424750095245287 ) ) ;
#79768=EDGE_LOOP ( 'NONE', ( #34360, #44406, #2691, #38917 ) ) ;
#79769=CARTESIAN_POINT ( 'NONE',  ( -12.39639368081883042, -7.750023224968867197, 34.99404313364389907 ) ) ;
#79770=CARTESIAN_POINT ( 'NONE',  ( 16.85343815235874132, -12.47654668319379567, 31.42292124445336654 ) ) ;
#79771=B_SPLINE_CURVE_WITH_KNOTS ( 'NONE', 3,
 ( #48197, #26605, #33803, #82004, #74354, #24, #33368, #26162, #75243, #88773 ),
 .UNSPECIFIED., .F., .F.,
 ( 4, 2, 2, 2, 4 ),
 ( 0.000000000000000000, 0.0001954311564186865221, 0.0003908623128373730441, 0.0005862934692560595662, 0.0007817246256747460882 ),
 .UNSPECIFIED. ) ;
#79772=CARTESIAN_POINT ( 'NONE',  ( 0.2115617305961060846, -4.943428324936578910, 34.04746400365624481 ) ) ;
#79773=FACE_BOUND ( 'NONE', #16189, .T. ) ;
#79774=B_SPLINE_CURVE_WITH_KNOTS ( 'NONE', 3,
 ( #64825, #60749, #12135, #87359, #67961, #38705, #52654, #80141, #6263, #5814 ),
 .UNSPECIFIED., .F., .F.,
 ( 4, 2, 2, 2, 4 ),
 ( 0.000000000000000000, 0.0001954339857564080707, 0.0003908679715128161414, 0.0005863019572692241849, 0.0007817359430256322827 ),
 .UNSPECIFIED. ) ;
#79775=CARTESIAN_POINT ( 'NONE',  ( 17.20744851515672025, -6.808710257144159783, 34.95449254468098843 ) ) ;
#79776=CARTESIAN_POINT ( 'NONE',  ( 13.60739492588379562, -9.332535724633409302, 34.40230450496446934 ) ) ;
#79777=DIRECTION ( 'NONE',  ( -0.000000000000000000, -0.9848077530122086864, -0.1736481776669273613 ) ) ;
#79778=CARTESIAN_POINT ( 'NONE',  ( 2.242422307135989890, -8.656820664281497102, 34.87096338111211935 ) ) ;
#79780=ORIENTED_EDGE ( 'NONE', *, *, #83505, .F. ) ;
#79781=EDGE_CURVE ( 'NONE', #71793, #45833, #70568, .T. ) ;
#79782=CARTESIAN_POINT ( 'NONE',  ( -17.07692307692319744, -12.46129190930018460, 30.37095296980731973 ) ) ;
#79783=ORIENTED_EDGE ( 'NONE', *, *, #88185, .F. ) ;
#79784=EDGE_LOOP ( 'NONE', ( #57274, #67790 ) ) ;
#79785=VECTOR ( 'NONE', #932, 1000.000000000000114 ) ;
#79786=CARTESIAN_POINT ( 'NONE',  ( -7.053224892808619195, -4.299443229763728169, 33.91186481527756058 ) ) ;
#79787=CARTESIAN_POINT ( 'NONE',  ( 10.74591031714818357, -6.001044277235009439, 34.52024696741798948 ) ) ;
#79788=CYLINDRICAL_SURFACE ( 'NONE', #9714, 0.2499999999999986955 ) ;
#79789=CARTESIAN_POINT ( 'NONE',  ( -2.084912766423895558, -12.24180327182771855, 31.33663988360758168 ) ) ;
#79790=CARTESIAN_POINT ( 'NONE',  ( 7.596130608860880429, -12.43535235679832596, 30.55408501211184813 ) ) ;
#79791=CARTESIAN_POINT ( 'NONE',  ( -2.307692307692305711, -10.05456864172156806, 36.03766855953608683 ) ) ;
#79792=ORIENTED_EDGE ( 'NONE', *, *, #80413, .T. ) ;
#79793=CARTESIAN_POINT ( 'NONE',  ( 6.792928953345223064, -2.647304123082328875, 31.75400227202885262 ) ) ;
#79794=ADVANCED_FACE ( 'NONE', ( #61032 ), #62787, .F. ) ;
#79795=CARTESIAN_POINT ( 'NONE',  ( 3.100078627658923391, -9.084618155246140248, 34.75535874321725771 ) ) ;
#79796=CARTESIAN_POINT ( 'NONE',  ( 2.307692307692309264, -12.62096338111211580, 30.90682066428153263 ) ) ;
#79797=EDGE_CURVE ( 'NONE', #57707, #79832, #17934, .T. ) ;
#79798=CARTESIAN_POINT ( 'NONE',  ( -3.931066612577740482, -3.755027918224367767, 33.06320215134714857 ) ) ;
#79799=ORIENTED_EDGE ( 'NONE', *, *, #52252, .T. ) ;
#79800=EDGE_LOOP ( 'NONE', ( #67782, #12996 ) ) ;
#79803=CYLINDRICAL_SURFACE ( 'NONE', #39178, 0.2499999999999986955 ) ;
#79804=CARTESIAN_POINT ( 'NONE',  ( -6.249999999999997335, -7.433932668274256805, 35.00000000000000711 ) ) ;
#79805=ORIENTED_EDGE ( 'NONE', *, *, #27451, .T. ) ;
#79806=CARTESIAN_POINT ( 'NONE',  ( -16.37733107841048508, -11.60425143139329940, 33.02411095842164457 ) ) ;
#79807=CARTESIAN_POINT ( 'NONE',  ( 6.000000000000001776, -11.35647404775217417, 33.31231777344666511 ) ) ;
#79808=CARTESIAN_POINT ( 'NONE',  ( -8.546451227962359454, -6.760870238392817200, 34.69528174975672385 ) ) ;
#79809=CARTESIAN_POINT ( 'NONE',  ( -6.923076923077044142, -3.300289026999228881, 32.46337939537708905 ) ) ;
#79810=ADVANCED_FACE ( 'NONE', ( #75438 ), #54265, .F. ) ;
#79811=B_SPLINE_CURVE_WITH_KNOTS ( 'NONE', 3,
 ( #53182, #44638, #73918, #11771, #65368, #39249, #66711, #31132, #24824, #72570 ),
 .UNSPECIFIED., .F., .F.,
 ( 4, 2, 2, 2, 4 ),
 ( 0.000000000000000000, 0.0001954339857564073659, 0.0003908679715128147319, 0.0005863019572692221250, 0.0007817359430256294638 ),
 .UNSPECIFIED. ) ;
#79812=CARTESIAN_POINT ( 'NONE',  ( -11.40766973063674605, -8.999086150933475636, 34.52020707165672775 ) ) ;
#79813=EDGE_LOOP ( 'NONE', ( #42325, #34346 ) ) ;
#79814=CARTESIAN_POINT ( 'NONE',  ( -7.715362038329057981, -9.804649428959608670, 34.18742332936588468 ) ) ;
#79816=CARTESIAN_POINT ( 'NONE',  ( 3.230769230769110045, -5.219633306517616589, 34.19971097300220464 ) ) ;
#79817=CARTESIAN_POINT ( 'NONE',  ( -12.59222906464877134, -2.845849958028613624, 32.17971566917920967 ) ) ;
#79818=CARTESIAN_POINT ( 'NONE',  ( -7.596208436775803818, -3.520799739797213945, 33.17531984108286025 ) ) ;
#79819=B_SPLINE_CURVE_WITH_KNOTS ( 'NONE', 3,
 ( #75301, #6830, #14035, #61765, #27555, #41511, #68978, #7283, #34748, #62219 ),
 .UNSPECIFIED., .F., .F.,
 ( 4, 2, 2, 2, 4 ),
 ( 0.0007817359430256332585, 0.0009771253907250054306, 0.001172514838424370664, 0.001367904286123735897, 0.001563293733823100913 ),
 .UNSPECIFIED. ) ;
#79820=B_SPLINE_CURVE_WITH_KNOTS ( 'NONE', 3,
 ( #32064, #40167, #53665, #60865, #59529, #46899, #74384, #67632, #87032, #25306 ),
 .UNSPECIFIED., .F., .F.,
 ( 4, 2, 2, 2, 4 ),
 ( 0.0007817246256747453293, 0.0009771112852218883336, 0.001172497944769031230, 0.001367884604316174126, 0.001563271263863317238 ),
 .UNSPECIFIED. ) ;
#79821=EDGE_CURVE ( 'NONE', #19611, #64420, #20051, .T. ) ;
#79823=CARTESIAN_POINT ( 'NONE',  ( -8.519176349317316266, -8.346898887586323923, 34.93166121998716278 ) ) ;
#79824=CARTESIAN_POINT ( 'NONE',  ( 6.223011351612849573, -2.758310577978207778, 31.33698337089303010 ) ) ;
#79826=ORIENTED_EDGE ( 'NONE', *, *, #36306, .T. ) ;
#79827=CARTESIAN_POINT ( 'NONE',  ( -4.153846153846152411, -10.67929555188718282, 33.92786785259544047 ) ) ;
#79828=DIRECTION ( 'NONE',  ( -0.000000000000000000, -0.5000000000000009992, -0.8660254037844380415 ) ) ;
#79829=DIRECTION ( 'NONE',  ( -0.000000000000000000, 0.3420201433256694346, -0.9396926207859080948 ) ) ;
#79830=AXIS2_PLACEMENT_3D ( 'NONE', #64937, #3243, #10457 ) ;
#79832=VERTEX_POINT ( 'NONE', #74555 ) ;
#79833=CARTESIAN_POINT ( 'NONE',  ( 9.942362112221147186, -3.435999193479609914, 33.07426656108010832 ) ) ;
#79834=CARTESIAN_POINT ( 'NONE',  ( 12.52760579488853665, -3.937682226553329556, 33.60647404775216529 ) ) ;
#79835=CARTESIAN_POINT ( 'NONE',  ( 17.14299041027315695, -3.322132147404559532, 32.92929555188717927 ) ) ;
#79836=CARTESIAN_POINT ( 'NONE',  ( 13.31934538405906565, -3.083524468853724443, 32.58852847137143272 ) ) ;
#79837=CARTESIAN_POINT ( 'NONE',  ( -9.019207500173124004, -11.79746400365624659, 32.30657167506340954 ) ) ;
#79838=CARTESIAN_POINT ( 'NONE',  ( 5.933916589044120116, -8.120952969808774569, 34.71129190930000163 ) ) ;
#79839=ORIENTED_EDGE ( 'NONE', *, *, #10295, .F. ) ;
#79840=FACE_OUTER_BOUND ( 'NONE', #64206, .T. ) ;
#79841=CARTESIAN_POINT ( 'NONE',  ( -5.749999999998562927, -7.500000000000155431, 34.75000000000007105 ) ) ;
#79842=DIRECTION ( 'NONE',  ( -0.000000000000000000, 0.7660444431189791237, -0.6427876096865379196 ) ) ;
#79843=ORIENTED_EDGE ( 'NONE', *, *, #35329, .T. ) ;
#79844=CARTESIAN_POINT ( 'NONE',  ( 13.60739492588379562, -6.760870238392817200, 34.69528174975672385 ) ) ;
#79845=ORIENTED_EDGE ( 'NONE', *, *, #48726, .T. ) ;
#79846=FACE_OUTER_BOUND ( 'NONE', #40, .T. ) ;
#79847=CARTESIAN_POINT ( 'NONE',  ( 10.39189969082028675, -3.562934362175799841, 33.22335522853832401 ) ) ;
#79848=FACE_OUTER_BOUND ( 'NONE', #17221, .T. ) ;
#79849=ORIENTED_EDGE ( 'NONE', *, *, #4095, .F. ) ;
#79851=CARTESIAN_POINT ( 'NONE',  ( -11.40793583669797506, -12.45806712695776319, 30.39783852428763922 ) ) ;
#79855=CARTESIAN_POINT ( 'NONE',  ( -2.242437168179467477, -11.06231777344671130, 33.60647404775212976 ) ) ;
#79856=ORIENTED_EDGE ( 'NONE', *, *, #75948, .T. ) ;
#79857=CARTESIAN_POINT ( 'NONE',  ( -1.384615384615383471, -13.87047571288749737, 32.06866353760679544 ) ) ;
#79859=CARTESIAN_POINT ( 'NONE',  ( -15.00798956179116317, -6.717445702608402236, 34.94155399931962336 ) ) ;
#79860=CARTESIAN_POINT ( 'NONE',  ( -10.36538461538461320, -2.499999999999998668, 29.75000000000000355 ) ) ;
#79861=CARTESIAN_POINT ( 'NONE',  ( -13.51530685128294174, -2.729777683071817229, 31.24903638046269450 ) ) ;
#79862=DIRECTION ( 'NONE',  ( -0.000000000000000000, 0.9848077530122085754, -0.1736481776669273613 ) ) ;
#79863=CARTESIAN_POINT ( 'NONE',  ( -6.066083410955878108, -4.098570777380720287, 33.41473453929634729 ) ) ;
#79864=CARTESIAN_POINT ( 'NONE',  ( -6.700064078983529292, -2.523321265292115090, 31.42251411153756280 ) ) ;
#79865=B_SPLINE_CURVE_WITH_KNOTS ( 'NONE', 3,
 ( #18852, #59388, #31471, #79664, #45418, #72897, #60270, #45866, #12540, #11202 ),
 .UNSPECIFIED., .F., .F.,
 ( 4, 2, 2, 2, 4 ),
 ( 0.000000000000000000, 0.0001954339857564083417, 0.0003908679715128166835, 0.0005863019572692250523, 0.0007817359430256333669 ),
 .UNSPECIFIED. ) ;
#79866=EDGE_LOOP ( 'NONE', ( #65799, #73379, #21258, #36351, #10466, #42524 ) ) ;
#79867=VERTEX_POINT ( 'NONE', #55602 ) ;
#79868=EDGE_LOOP ( 'NONE', ( #6538, #18419 ) ) ;
#79869=ORIENTED_EDGE ( 'NONE', *, *, #72781, .T. ) ;
#79870=ORIENTED_EDGE ( 'NONE', *, *, #9653, .T. ) ;
#79871=VECTOR ( 'NONE', #55309, 1000.000000000000000 ) ;
#79872=LINE ( 'NONE', #18172, #81907 ) ;
#79873=CARTESIAN_POINT ( 'NONE',  ( -11.53846153846153655, -8.973038597847269315, 34.52809138561121927 ) ) ;
#79874=CARTESIAN_POINT ( 'NONE',  ( 15.00728428704528561, -5.113361153441934093, 34.14387501736622710 ) ) ;
#79875=CARTESIAN_POINT ( 'NONE',  ( 17.07692307692307665, -5.471508081941601098, 34.59228464037088457 ) ) ;
#79876=CARTESIAN_POINT ( 'NONE',  ( -13.60810030917971680, -3.562934362175800285, 33.22335522853832401 ) ) ;
#79877=CARTESIAN_POINT ( 'NONE',  ( 2.980792499826877773, -5.728515186090277211, 34.42611988154120439 ) ) ;
#79878=EDGE_CURVE ( 'NONE', #33346, #56271, #50144, .T. ) ;
#79879=CARTESIAN_POINT ( 'NONE',  ( 5.776515056276054771, -11.89387501736622710, 32.13663884655806413 ) ) ;
#79880=CARTESIAN_POINT ( 'NONE',  ( -4.088590582570127197, -10.90142922261932057, 33.41473453929631887 ) ) ;
#79882=VERTEX_POINT ( 'NONE', #20491 ) ;
#79884=EDGE_LOOP ( 'NONE', ( #84376, #3216 ) ) ;
#79885=ORIENTED_EDGE ( 'NONE', *, *, #63567, .T. ) ;
#79886=CYLINDRICAL_SURFACE ( 'NONE', #83388, 0.2500000000000012212 ) ;
#79887=VERTEX_POINT ( 'NONE', #40330 ) ;
#79888=CARTESIAN_POINT ( 'NONE',  ( -15.90390063549801347, -6.696923467548659303, 34.68552623307873972 ) ) ;
#79890=CARTESIAN_POINT ( 'NONE',  ( 8.519230769230768274, -7.433931650972300353, 34.75000000000000711 ) ) ;
#79891=CARTESIAN_POINT ( 'NONE',  ( 4.219101725122177626, -2.625532179533470512, 30.86335684631491105 ) ) ;
#79892=FACE_BOUND ( 'NONE', #65578, .T. ) ;
#79893=EDGE_LOOP ( 'NONE', ( #30116, #29935 ) ) ;
#79894=EDGE_CURVE ( 'NONE', #44547, #26565, #82398, .T. ) ;
#79895=ORIENTED_EDGE ( 'NONE', *, *, #70211, .F. ) ;
#79896=LINE ( 'NONE', #18198, #80222 ) ;
#79898=FACE_BOUND ( 'NONE', #31828, .T. ) ;
#79899=CARTESIAN_POINT ( 'NONE',  ( -8.769230769230768274, -2.486705287966279876, 31.30864560766543647 ) ) ;
#79900=CARTESIAN_POINT ( 'NONE',  ( 14.98079248672063990, -6.524016743844655686, 34.90889640711025521 ) ) ;
#79902=CARTESIAN_POINT ( 'NONE',  ( 17.99999999999987566, -2.892918686052165622, 31.69288490824153470 ) ) ;
#79903=DIRECTION ( 'NONE',  ( -0.000000000000000000, -0.8660254037844399289, -0.4999999999999980016 ) ) ;
#79904=CARTESIAN_POINT ( 'NONE',  ( -18.22292695890684655, -4.026226216239095379, 33.68668979543632958 ) ) ;
#79905=EDGE_LOOP ( 'NONE', ( #46492, #54820 ) ) ;
#79906=CARTESIAN_POINT ( 'NONE',  ( 17.77712048326241145, -7.630690623152299956, 34.99857592706774057 ) ) ;
#79907=CARTESIAN_POINT ( 'NONE',  ( 3.007843013253082010, -12.15238873228292071, 31.58232369045353849 ) ) ;
#79910=CARTESIAN_POINT ( 'NONE',  ( -10.61538461538473399, -8.613356846316285953, 34.62446782046622218 ) ) ;
#79911=DIRECTION ( 'NONE',  ( -0.000000000000000000, 0.8660254037844399289, -0.4999999999999980016 ) ) ;
#79912=ORIENTED_EDGE ( 'NONE', *, *, #83287, .F. ) ;
#79913=CARTESIAN_POINT ( 'NONE',  ( 18.06606835100243913, -6.386643153685127139, 34.62446782046654192 ) ) ;
#79914=DIRECTION ( 'NONE',  ( -0.000000000000000000, -0.3420201433256694346, -0.9396926207859080948 ) ) ;
#79915=CARTESIAN_POINT ( 'NONE',  ( -2.530618525208454539, -2.554751324335734264, 30.48935550225260727 ) ) ;
#79916=CARTESIAN_POINT ( 'NONE',  ( 14.98079248672064345, -12.65889640711025521, 30.72598325615533454 ) ) ;
#79917=CARTESIAN_POINT ( 'NONE',  ( -6.673076923075503153, -7.500000000000154543, 35.00000000000007105 ) ) ;
#79918=EDGE_CURVE ( 'NONE', #76443, #85803, #21117, .T. ) ;
#79919=CARTESIAN_POINT ( 'NONE',  ( 17.14299041027315695, -4.661471528628508665, 34.16647553114624003 ) ) ;
#79920=CARTESIAN_POINT ( 'NONE',  ( 14.05769230769230127, -2.499999999999999556, 29.81609845454692120 ) ) ;
#79921=DIRECTION ( 'NONE',  ( 0.000000000000000000, 0.9848077530122072432, -0.1736481776669354937 ) ) ;
#79922=CARTESIAN_POINT ( 'NONE',  ( 9.019285080869083870, -12.17597550085003810, 31.52189283813460463 ) ) ;
#79923=DIRECTION ( 'NONE',  ( -0.000000000000000000, -0.3420201433256695456, -0.9396926207859082059 ) ) ;
#79924=CARTESIAN_POINT ( 'NONE',  ( 12.21151523731700550, -4.931416488878822335, 34.32920672191015399 ) ) ;
#79926=ORIENTED_EDGE ( 'NONE', *, *, #680, .F. ) ;
#79927=ADVANCED_FACE ( 'NONE', ( #64120 ), #3313, .F. ) ;
#79928=B_SPLINE_CURVE_WITH_KNOTS ( 'NONE', 3,
 ( #53877, #68278, #6583, #74153, #60626, #48436, #33611, #75924, #39936, #34048 ),
 .UNSPECIFIED., .F., .F.,
 ( 4, 2, 2, 2, 4 ),
 ( 0.0007817359430256388964, 0.0009771253907250075990, 0.001172514838424376085, 0.001367904286123744571, 0.001563293733823113273 ),
 .UNSPECIFIED. ) ;
#79930=ORIENTED_EDGE ( 'NONE', *, *, #7387, .F. ) ;
#79933=CARTESIAN_POINT ( 'NONE',  ( -17.01085574357299990, -3.937682226553329556, 33.60647404775216529 ) ) ;
#79934=ORIENTED_EDGE ( 'NONE', *, *, #8723, .T. ) ;
#79935=CARTESIAN_POINT ( 'NONE',  ( -15.00775787915638126, -5.667800583137506010, 34.40243808032445827 ) ) ;
#79937=CARTESIAN_POINT ( 'NONE',  ( -15.23076923076935074, -2.625532179533778709, 30.86335684631627174 ) ) ;
#79938=CARTESIAN_POINT ( 'NONE',  ( -1.384615384615383471, -2.292212530054420494, 30.41441678777542634 ) ) ;
#79939=CARTESIAN_POINT ( 'NONE',  ( 9.823098133274644539, -9.084667340241226796, 34.75534355489798344 ) ) ;
#79940=CARTESIAN_POINT ( 'NONE',  ( -12.33074802057151409, -3.957578996910242619, 33.62503395064540257 ) ) ;
#79941=DIRECTION ( 'NONE',  ( 0.000000000000000000, 0.7660444431189822323, -0.6427876096865344779 ) ) ;
#79942=CARTESIAN_POINT ( 'NONE',  ( 0.4615384615384611200, -5.471508081941601098, 34.59228464037088457 ) ) ;
#79943=DIRECTION ( 'NONE',  ( -0.000000000000000000, 0.6427876096865404731, -0.7660444431189771253 ) ) ;
#79946=CARTESIAN_POINT ( 'NONE',  ( 5.299935921016473372, -2.889357225399416862, 32.26129605718031002 ) ) ;
#79947=CARTESIAN_POINT ( 'NONE',  ( -18.00000000000000000, -2.292212530054419606, 30.41441678777542990 ) ) ;
#79948=B_SPLINE_CURVE_WITH_KNOTS ( 'NONE', 3,
 ( #35309, #81738, #13270, #55137, #20472, #47934, #82633, #83512, #13710, #34426 ),
 .UNSPECIFIED., .F., .F.,
 ( 4, 2, 2, 2, 4 ),
 ( 0.000000000000000000, 0.0001954339857564070678, 0.0003908679715128141356, 0.0005863019572692211492, 0.0007817359430256282712 ),
 .UNSPECIFIED. ) ;
#79949=CARTESIAN_POINT ( 'NONE',  ( 5.869309396889692998, -3.338472653186242756, 32.95098750199972670 ) ) ;
#79950=B_SPLINE_CURVE_WITH_KNOTS ( 'NONE', 3,
 ( #40011, #26929, #46306, #47184, #87317, #12094, #73794, #40456, #53049, #12970 ),
 .UNSPECIFIED., .F., .F.,
 ( 4, 2, 2, 2, 4 ),
 ( 0.000000000000000000, 0.0001954311564186863323, 0.0003908623128373726646, 0.0005862934692560590241, 0.0007817246256747453293 ),
 .UNSPECIFIED. ) ;
#79951=EDGE_LOOP ( 'NONE', ( #65783, #59592 ) ) ;
#79952=ORIENTED_EDGE ( 'NONE', *, *, #14646, .F. ) ;
#79954=CARTESIAN_POINT ( 'NONE',  ( 7.716006636715626144, -11.47017969459903952, 32.78971311882034456 ) ) ;
#79955=CARTESIAN_POINT ( 'NONE',  ( 1.319345384059066317, -11.06231777344662781, 33.60647404775220082 ) ) ;
#79956=CARTESIAN_POINT ( 'NONE',  ( 6.130045055919775443, -2.254550872974306674, 29.97347326024527447 ) ) ;
#79957=AXIS2_PLACEMENT_3D ( 'NONE', #44177, #64016, #70798 ) ;
#79958=CARTESIAN_POINT ( 'NONE',  ( 4.088576153289834814, -3.643525952247789412, 33.31231777344662959 ) ) ;
#79959=CARTESIAN_POINT ( 'NONE',  ( -4.946132635956124624, -2.845873456487966635, 32.17976146951972538 ) ) ;
#79960=EDGE_CURVE ( 'NONE', #33331, #66936, #45838, .T. ) ;
#79961=VERTEX_POINT ( 'NONE', #78091 ) ;
#79962=CARTESIAN_POINT ( 'NONE',  ( 17.99999999999987566, -12.46129190930018460, 30.37095296980731973 ) ) ;
#79963=EDGE_LOOP ( 'NONE', ( #44041, #3755, #36173, #10159 ) ) ;
#79965=CARTESIAN_POINT ( 'NONE',  ( 7.780071466793709867, -10.67929555188718460, 33.92786785259543336 ) ) ;
#79966=CARTESIAN_POINT ( 'NONE',  ( 4.153846153846032507, -2.625532179533778709, 30.86335684631627174 ) ) ;
#79967=AXIS2_PLACEMENT_3D ( 'NONE', #73392, #5823, #33301 ) ;
#79968=CARTESIAN_POINT ( 'NONE',  ( 11.60371710973756443, -10.90142922261932057, 33.41473453929631887 ) ) ;
#79970=CARTESIAN_POINT ( 'NONE',  ( 13.38461538461538680, -5.471508081941601098, 34.59228464037088457 ) ) ;
#79971=ADVANCED_FACE ( 'NONE', ( #8315 ), #1995, .F. ) ;
#79972=AXIS2_PLACEMENT_3D ( 'NONE', #5624, #62330, #21352 ) ;
#79973=EDGE_LOOP ( 'NONE', ( #27795, #36605 ) ) ;
#79974=B_SPLINE_CURVE_WITH_KNOTS ( 'NONE', 3,
 ( #80423, #18724, #51572, #46189, #27681, #67789, #13284, #654, #88527, #40767 ),
 .UNSPECIFIED., .F., .F.,
 ( 4, 2, 2, 2, 4 ),
 ( 0.000000000000000000, 0.0001954339857564126514, 0.0003908679715128183098, 0.0005863019572692239681, 0.0007817359430256294638 ),
 .UNSPECIFIED. ) ;
#79975=VERTEX_POINT ( 'NONE', #23147 ) ;
#79978=CARTESIAN_POINT ( 'NONE',  ( -0.2385256174450668676, -10.01129605718032778, 34.36064277460058491 ) ) ;
#79979=DIRECTION ( 'NONE',  ( 0.000000000000000000, 0.7660444431189807890, 0.6427876096865361433 ) ) ;
#79980=CARTESIAN_POINT ( 'NONE',  ( 10.36536139116316235, -4.931416488878822335, 34.32920672191015399 ) ) ;
#79982=CARTESIAN_POINT ( 'NONE',  ( -4.403846153846151523, -7.500000000000001776, 34.75000000000000000 ) ) ;
#79983=CARTESIAN_POINT ( 'NONE',  ( 5.749976762707035505, -12.43535235679832596, 30.55408501211184813 ) ) ;
#79984=EDGE_LOOP ( 'NONE', ( #32080, #44422, #24689, #82870 ) ) ;
#79985=EDGE_CURVE ( 'NONE', #11337, #1879, #25440, .T. ) ;
#79986=VERTEX_POINT ( 'NONE', #22701 ) ;
#79987=CARTESIAN_POINT ( 'NONE',  ( 11.60365552024489766, -2.506253911140448043, 29.99999999999988631 ) ) ;
#79988=CARTESIAN_POINT ( 'NONE',  ( -6.000000000000119904, -3.300289026999228881, 32.46337939537708905 ) ) ;
#79989=ORIENTED_EDGE ( 'NONE', *, *, #38703, .F. ) ;
#79990=CARTESIAN_POINT ( 'NONE',  ( -9.915792616872021625, -10.23692288466677880, 34.23039457007281072 ) ) ;
#79991=CARTESIAN_POINT ( 'NONE',  ( 12.46153846153833911, -8.656820664282941280, 34.87096338111179961 ) ) ;
#79993=ORIENTED_EDGE ( 'NONE', *, *, #18602, .T. ) ;
#79994=EDGE_CURVE ( 'NONE', #14985, #29486, #76771, .T. ) ;
#79995=CARTESIAN_POINT ( 'NONE',  ( 10.83839745947800992, -2.308499170217967134, 30.53291367094873721 ) ) ;
#79998=CARTESIAN_POINT ( 'NONE',  ( 0.3954560821783245639, -11.35647404775217595, 33.31231777344667222 ) ) ;
#79999=CARTESIAN_POINT ( 'NONE',  ( -12.33101275977490197, -12.45806712695776319, 30.39783852428763922 ) ) ;
#80000=LINE ( 'NONE', #80907, #63346 ) ;
#80002=EDGE_CURVE ( 'NONE', #2976, #63180, #78071, .T. ) ;
#80005=ORIENTED_EDGE ( 'NONE', *, *, #80160, .F. ) ;
#80006=CARTESIAN_POINT ( 'NONE',  ( -11.47239420511146513, -8.164416787775445883, 34.95778746994558617 ) ) ;
#80008=CARTESIAN_POINT ( 'NONE',  ( 14.98074599347626368, -4.335965774309649134, 33.62209801155881905 ) ) ;
#80010=ORIENTED_EDGE ( 'NONE', *, *, #18601, .F. ) ;
#80011=LINE ( 'NONE', #87233, #27195 ) ;
#80012=CARTESIAN_POINT ( 'NONE',  ( 10.54930223602447903, -8.164416787775445883, 34.95778746994557906 ) ) ;
#80014=CARTESIAN_POINT ( 'NONE',  ( 16.15384615384615330, -12.78798330534102767, 29.49999999999997868 ) ) ;
#80015=EDGE_CURVE ( 'NONE', #18617, #48928, #694, .T. ) ;
#80016=FACE_BOUND ( 'NONE', #82471, .T. ) ;
#80017=CARTESIAN_POINT ( 'NONE',  ( 12.21151522424549896, -3.202444869320336451, 32.30641848906366675 ) ) ;
#80018=CARTESIAN_POINT ( 'NONE',  ( 4.376625822824220080, -12.69155399931963046, 30.53255429739158444 ) ) ;
#80019=CARTESIAN_POINT ( 'NONE',  ( 2.307692307692309264, -9.905515769479276145, 34.41647553114623292 ) ) ;
#80020=CARTESIAN_POINT ( 'NONE',  ( 1.134638640566795864, -12.65889640711025521, 30.72598325615533454 ) ) ;
#80021=CARTESIAN_POINT ( 'NONE',  ( -11.40793610022789828, -11.04252011169590020, 33.62494198852677130 ) ) ;
#80022=CARTESIAN_POINT ( 'NONE',  ( -9.692307692307691624, -2.499999999999998668, 29.50000000000001066 ) ) ;
#80023=CARTESIAN_POINT ( 'NONE',  ( 8.899756207464411872, -12.70449254468099198, 30.44128974285582956 ) ) ;
#80025=CARTESIAN_POINT ( 'NONE',  ( -12.33070013105169771, -7.277220318596961057, 34.99547417642776992 ) ) ;
#80026=ORIENTED_EDGE ( 'NONE', *, *, #18684, .F. ) ;
#80027=CYLINDRICAL_SURFACE ( 'NONE', #14729, 0.2500000000000012212 ) ;
#80028=ADVANCED_FACE ( 'NONE', ( #25368 ), #72662, .F. ) ;
#80029=AXIS2_PLACEMENT_3D ( 'NONE', #6618, #34086, #20570 ) ;
#80030=EDGE_CURVE ( 'NONE', #52889, #68628, #46951, .T. ) ;
#80032=CARTESIAN_POINT ( 'NONE',  ( -13.63461538461539213, -2.250000000000000000, 29.81609741502490252 ) ) ;
#80033=DIRECTION ( 'NONE',  ( 0.000000000000000000, 0.8660254037844377084, -0.5000000000000015543 ) ) ;
#80034=CARTESIAN_POINT ( 'NONE',  ( 17.01165307636676260, -12.70778746994557551, 30.41441678777548319 ) ) ;
#80035=CARTESIAN_POINT ( 'NONE',  ( 1.384615384615264011, -12.16647553114689728, 32.15551576947799362 ) ) ;
#80037=DIRECTION ( 'NONE',  ( 0.000000000000000000, 0.9848077530122072432, -0.1736481776669354937 ) ) ;
#80038=CARTESIAN_POINT ( 'NONE',  ( 16.40384615384615330, -7.500000000000001776, 35.04278698407183867 ) ) ;
#80041=CARTESIAN_POINT ( 'NONE',  ( 9.469380733400845074, -4.026226216239094491, 33.68668979543634379 ) ) ;
#80042=CARTESIAN_POINT ( 'NONE',  ( 7.145856464345333059, -4.387253974876676565, 33.66317474335728832 ) ) ;
#80043=CARTESIAN_POINT ( 'NONE',  ( -8.769230769230890843, -9.442884908241554243, 34.35708131394783038 ) ) ;
#80044=CARTESIAN_POINT ( 'NONE',  ( -2.177647251772534265, -2.254550872974306674, 29.97347326024527447 ) ) ;
#80045=CARTESIAN_POINT ( 'NONE',  ( -11.47320596718551045, -10.90142922261932057, 33.41473453929631887 ) ) ;
#80046=ORIENTED_EDGE ( 'NONE', *, *, #76385, .T. ) ;
#80047=CARTESIAN_POINT ( 'NONE',  ( -7.846153846153965716, -3.835265460704628371, 33.15142922262033665 ) ) ;
#80048=CARTESIAN_POINT ( 'NONE',  ( 15.48082365068268018, -10.82426656108012075, 33.81400080652039009 ) ) ;
#80050=CARTESIAN_POINT ( 'NONE',  ( -17.07692307692319744, -12.16647553114689728, 32.15551576947799362 ) ) ;
#80051=CYLINDRICAL_SURFACE ( 'NONE', #65652, 0.2499999999999986955 ) ;
#80052=ORIENTED_EDGE ( 'NONE', *, *, #88439, .T. ) ;
#80053=CARTESIAN_POINT ( 'NONE',  ( 16.15384615384615330, -12.78798330534102945, 29.74999999999997868 ) ) ;
#80054=CARTESIAN_POINT ( 'NONE',  ( 1.634615384616805889, -7.500000000000154543, 35.00000000000007105 ) ) ;
#80055=CARTESIAN_POINT ( 'NONE',  ( -11.53846153846165912, -10.21337939537710326, 33.94971097300076224 ) ) ;
#80056=EDGE_LOOP ( 'NONE', ( #27793, #21635, #70994, #28058, #1396, #83281 ) ) ;
#80057=LINE ( 'NONE', #86844, #13961 ) ;
#80058=CARTESIAN_POINT ( 'NONE',  ( 3.930361210122204518, -8.496056993536548418, 34.65000542017679663 ) ) ;
#80059=DIRECTION ( 'NONE',  ( -0.000000000000000000, 1.000000000000000000, 3.491481338843133355E-15 ) ) ;
#80060=CARTESIAN_POINT ( 'NONE',  ( 11.78840705680968171, -9.272278438253398036, 34.42582936511637115 ) ) ;
#80062=FACE_OUTER_BOUND ( 'NONE', #49420, .T. ) ;
#80063=EDGE_CURVE ( 'NONE', #32965, #29248, #53346, .T. ) ;
#80066=CARTESIAN_POINT ( 'NONE',  ( -2.307692307692305711, -13.63283147151868846, 33.57946703557072254 ) ) ;
#80067=ORIENTED_EDGE ( 'NONE', *, *, #50711, .F. ) ;
#80068=EDGE_LOOP ( 'NONE', ( #18828, #70674, #28496, #81952 ) ) ;
#80070=EDGE_CURVE ( 'NONE', #8934, #37210, #6127, .T. ) ;
#80071=EDGE_LOOP ( 'NONE', ( #85588, #26188, #6302, #65979 ) ) ;
#80072=EDGE_CURVE ( 'NONE', #5830, #25778, #18621, .T. ) ;
#80073=CARTESIAN_POINT ( 'NONE',  ( 0.3308469948709019115, -8.147922237126337563, 34.70805685702651999 ) ) ;
#80074=CARTESIAN_POINT ( 'NONE',  ( 6.000000000000001776, -2.292212530054420494, 30.41441678777542634 ) ) ;
#80075=AXIS2_PLACEMENT_3D ( 'NONE', #62101, #409, #82832 ) ;
#80076=CYLINDRICAL_SURFACE ( 'NONE', #16483, 0.2500000000000002220 ) ;
#80077=EDGE_CURVE ( 'NONE', #1531, #27912, #74892, .T. ) ;
#80078=CARTESIAN_POINT ( 'NONE',  ( -10.36538461538461320, -2.249999999999998668, 29.75000000000000355 ) ) ;
#80079=ORIENTED_EDGE ( 'NONE', *, *, #32437, .F. ) ;
#80080=VERTEX_POINT ( 'NONE', #86201 ) ;
#80081=CARTESIAN_POINT ( 'NONE',  ( 15.45378058238208219, -4.887748414852792322, 34.01359900205216746 ) ) ;
#80083=CARTESIAN_POINT ( 'NONE',  ( -6.673022503163469565, -4.074993327901525575, 33.72946981652012255 ) ) ;
#80084=CARTESIAN_POINT ( 'NONE',  ( 3.230769230769231726, -2.249999999999998668, 29.50000000000001421 ) ) ;
#80085=AXIS2_PLACEMENT_3D ( 'NONE', #51448, #44706, #64101 ) ;
#80086=CARTESIAN_POINT ( 'NONE',  ( 2.373760658694747061, -3.513871655860379306, 32.76840700105978499 ) ) ;
#80087=CARTESIAN_POINT ( 'NONE',  ( 17.07692307692295586, -8.613356846316285953, 34.62446782046622218 ) ) ;
#80088=VERTEX_POINT ( 'NONE', #17732 ) ;
#80089=ADVANCED_FACE ( 'NONE', ( #45184 ), #4205, .F. ) ;
#80090=ORIENTED_EDGE ( 'NONE', *, *, #76943, .T. ) ;
#80091=AXIS2_PLACEMENT_3D ( 'NONE', #6806, #49573, #82923 ) ;
#80092=VERTEX_POINT ( 'NONE', #13625 ) ;
#80093=CARTESIAN_POINT ( 'NONE',  ( 2.307692307692309264, -12.37446782046654192, 30.86335684631486131 ) ) ;
#80095=CARTESIAN_POINT ( 'NONE',  ( 17.07692307692307665, -5.471508081941601098, 34.59228464037088457 ) ) ;
#80096=B_SPLINE_CURVE_WITH_KNOTS ( 'NONE', 3,
 ( #69950, #77598, #35735, #28985, #56440, #26089, #6697, #12578, #59867, #81044 ),
 .UNSPECIFIED., .F., .F.,
 ( 4, 2, 2, 2, 4 ),
 ( 0.000000000000000000, 0.0001954339881912774612, 0.0003908679763825549224, 0.0005863019645738323836, 0.0007817359527651098448 ),
 .UNSPECIFIED. ) ;
#80097=CARTESIAN_POINT ( 'NONE',  ( 12.46153846153833911, -11.48612834414049644, 32.76840700105863391 ) ) ;
#80098=EDGE_LOOP ( 'NONE', ( #69358, #79526, #71634, #38857 ) ) ;
#80099=AXIS2_PLACEMENT_3D ( 'NONE', #6709, #60321, #25657 ) ;
#80100=CARTESIAN_POINT ( 'NONE',  ( -13.60810032833933469, -4.386631170607603991, 33.66268669641500111 ) ) ;
#80101=CYLINDRICAL_SURFACE ( 'NONE', #3369, 0.2499999999999995559 ) ;
#80102=DIRECTION ( 'NONE',  ( -0.000000000000000000, 1.000000000000000000, 3.491481338843133355E-15 ) ) ;
#80103=FACE_BOUND ( 'NONE', #71030, .T. ) ;
#80104=CARTESIAN_POINT ( 'NONE',  ( -5.326899820971668476, -10.06842814019191401, 34.32929386961144758 ) ) ;
#80105=CARTESIAN_POINT ( 'NONE',  ( -6.000000000000121680, -12.51329471203414379, 31.30864560766407578 ) ) ;
#80106=B_SPLINE_CURVE_WITH_KNOTS ( 'NONE', 3,
 ( #400, #8487, #13457, #48564, #35959, #63413, #27862, #40941, #27423, #82820 ),
 .UNSPECIFIED., .F., .F.,
 ( 4, 2, 2, 2, 4 ),
 ( 0.0007817246256747484735, 0.0009771112852218920199, 0.001172497944769035783, 0.001367884604316179330, 0.001563271263863322876 ),
 .UNSPECIFIED. ) ;
#80107=CARTESIAN_POINT ( 'NONE',  ( -9.019207500173124004, -4.236021600441997492, 33.53823185664189310 ) ) ;
#80108=CARTESIAN_POINT ( 'NONE',  ( 17.32692307692307665, -2.499999999999998668, 29.75000000000000355 ) ) ;
#80109=CARTESIAN_POINT ( 'NONE',  ( 14.55774672760576394, -2.920487667080175598, 32.31805714834170828 ) ) ;
#80110=CARTESIAN_POINT ( 'NONE',  ( -10.36538461538317790, -7.500000000000155431, 34.75000000000007105 ) ) ;
#80112=EDGE_LOOP ( 'NONE', ( #13230, #74988, #59544, #43422 ) ) ;
#80113=CARTESIAN_POINT ( 'NONE',  ( 11.53846153846153832, -3.050289026998446396, 32.03036669348365706 ) ) ;
#80114=CARTESIAN_POINT ( 'NONE',  ( -13.60754234352223335, -9.172386477786396597, 34.72672124145550043 ) ) ;
#80115=ORIENTED_EDGE ( 'NONE', *, *, #43751, .T. ) ;
#80116=VERTEX_POINT ( 'NONE', #62246 ) ;
#80117=CARTESIAN_POINT ( 'NONE',  ( 5.750023269057647823, -6.567427716900047230, 34.66269422305636283 ) ) ;
#80119=CARTESIAN_POINT ( 'NONE',  ( 6.923076923076924238, -11.16473453929635440, 33.15142922261926373 ) ) ;
#80120=CARTESIAN_POINT ( 'NONE',  ( 16.08776274289027342, -3.513871655860377086, 32.76840700105978499 ) ) ;
#80121=DIRECTION ( 'NONE',  ( -0.000000000000000000, 0.5000000000000011102, -0.8660254037844380415 ) ) ;
#80122=ORIENTED_EDGE ( 'NONE', *, *, #41385, .T. ) ;
#80125=CARTESIAN_POINT ( 'NONE',  ( 4.376858997939547358, -4.762714258010880997, 34.23016756924214832 ) ) ;
#80126=EDGE_CURVE ( 'NONE', #40124, #42322, #51071, .T. ) ;
#80127=EDGE_CURVE ( 'NONE', #40782, #30954, #11388, .T. ) ;
#80128=DIRECTION ( 'NONE',  ( -0.000000000000000000, 0.8660254037844399289, -0.4999999999999980016 ) ) ;
#80129=CARTESIAN_POINT ( 'NONE',  ( -11.78846153846153832, -7.500000000000001776, 35.04278698407183867 ) ) ;
#80130=CARTESIAN_POINT ( 'NONE',  ( -1.515305987725692694, -9.929715669179220328, 34.40415004197138416 ) ) ;
#80131=CARTESIAN_POINT ( 'NONE',  ( 2.530471848960717640, -5.114059244376869984, 34.14424750095245287 ) ) ;
#80132=FACE_OUTER_BOUND ( 'NONE', #9925, .T. ) ;
#80135=ORIENTED_EDGE ( 'NONE', *, *, #81305, .T. ) ;
#80136=EDGE_CURVE ( 'NONE', #87474, #12672, #59711, .T. ) ;
#80138=DIRECTION ( 'NONE',  ( 0.000000000000000000, 1.000000000000000000, -0.000000000000000000 ) ) ;
#80139=ADVANCED_FACE ( 'NONE', ( #14069 ), #41544, .F. ) ;
#80140=AXIS2_PLACEMENT_3D ( 'NONE', #18214, #65938, #51515 ) ;
#80141=CARTESIAN_POINT ( 'NONE',  ( -4.283993363284372080, -12.45813303252208648, 30.39737893381572675 ) ) ;
#80143=DIRECTION ( 'NONE',  ( 0.000000000000000000, 0.3420201433256641055, -0.9396926207859100932 ) ) ;
#80144=CYLINDRICAL_SURFACE ( 'NONE', #64577, 0.2499999999999997502 ) ;
#80146=B_SPLINE_CURVE_WITH_KNOTS ( 'NONE', 3,
 ( #23534, #28542, #1511, #50990, #56882, #23104, #36194, #63643, #30305, #15915 ),
 .UNSPECIFIED., .F., .F.,
 ( 4, 2, 2, 2, 4 ),
 ( 0.000000000000000000, 0.0001954339857564071491, 0.0003908679715128142982, 0.0005863019572692214744, 0.0007817359430256285964 ),
 .UNSPECIFIED. ) ;
#80147=CARTESIAN_POINT ( 'NONE',  ( -1.384615384615506484, -4.320704448113951379, 33.92786785259630022 ) ) ;
#80148=DIRECTION ( 'NONE',  ( 0.000000000000000000, 0.3420201433256610524, 0.9396926207859113145 ) ) ;
#80149=EDGE_CURVE ( 'NONE', #33117, #10201, #37050, .T. ) ;
#80150=FACE_OUTER_BOUND ( 'NONE', #37175, .T. ) ;
#80151=CARTESIAN_POINT ( 'NONE',  ( -12.46153846153858247, -12.46129190930018460, 30.37095296980731973 ) ) ;
#80153=B_SPLINE_CURVE_WITH_KNOTS ( 'NONE', 3,
 ( #31094, #44601, #71197, #16699, #50478, #58566, #9943, #29786, #70770, #23891 ),
 .UNSPECIFIED., .F., .F.,
 ( 4, 2, 2, 2, 4 ),
 ( 0.000000000000000000, 0.0001954339857564073388, 0.0003908679715128146777, 0.0005863019572692220165, 0.0007817359430256293554 ),
 .UNSPECIFIED. ) ;
#80154=CARTESIAN_POINT ( 'NONE',  ( 15.23076923076910916, -12.51329471203414379, 31.30864560766407578 ) ) ;
#80155=B_SPLINE_CURVE_WITH_KNOTS ( 'NONE', 3,
 ( #5088, #3746, #32552, #60024, #87528, #25805, #19047, #31216, #24304, #71605 ),
 .UNSPECIFIED., .F., .F.,
 ( 4, 2, 2, 2, 4 ),
 ( 0.000000000000000000, 0.0001954339881912774070, 0.0003908679763825548140, 0.0005863019645738322752, 0.0007817359527651096280 ),
 .UNSPECIFIED. ) ;
#80156=CARTESIAN_POINT ( 'NONE',  ( -0.4615384615384611200, -1.242168528481310874, 33.36296068462461051 ) ) ;
#80157=CARTESIAN_POINT ( 'NONE',  ( 4.023698944407933631, -12.45813303252208648, 30.39737893381572675 ) ) ;
#80158=CARTESIAN_POINT ( 'NONE',  ( -0.4615384615384611200, -11.16473453929635440, 33.15142922261926373 ) ) ;
#80159=CARTESIAN_POINT ( 'NONE',  ( -16.94613263595612551, -2.845873456487966635, 32.17976146951972538 ) ) ;
#80160=EDGE_CURVE ( 'NONE', #62909, #6352, #61778, .T. ) ;
#80161=ORIENTED_EDGE ( 'NONE', *, *, #174, .T. ) ;
#80162=DIRECTION ( 'NONE',  ( 0.000000000000000000, 1.000000000000000000, 0.000000000000000000 ) ) ;
#80163=CARTESIAN_POINT ( 'NONE',  ( 18.00000000000000000, -4.661471528628507777, 34.16647553114623292 ) ) ;
#80164=CARTESIAN_POINT ( 'NONE',  ( -4.284536756956461190, -5.496505350115500121, 34.60290016733514307 ) ) ;
#80166=CARTESIAN_POINT ( 'NONE',  ( 5.142178216435913107, -10.33852847137154107, 34.16647553114620450 ) ) ;
#80168=CARTESIAN_POINT ( 'NONE',  ( 15.90382292962469180, -4.931416488878822335, 34.32920672191015399 ) ) ;
#80169=EDGE_CURVE ( 'NONE', #36938, #87581, #88778, .T. ) ;
#80170=CARTESIAN_POINT ( 'NONE',  ( -0.2114841499001470504, -2.564540009722895419, 30.55348353981670684 ) ) ;
#80175=FACE_OUTER_BOUND ( 'NONE', #8501, .T. ) ;
#80176=VERTEX_POINT ( 'NONE', #43752 ) ;
#80177=CARTESIAN_POINT ( 'NONE',  ( -18.00000000000000000, -11.69971097300155449, 32.46337939537587403 ) ) ;
#80178=ADVANCED_FACE ( 'NONE', ( #77543 ), #71217, .F. ) ;
#80179=CARTESIAN_POINT ( 'NONE',  ( 13.13459214732242408, -10.05641848906368097, 34.04755513067966177 ) ) ;
#80180=CARTESIAN_POINT ( 'NONE',  ( 15.48082354240754732, -2.779044189368095719, 31.39831045268885745 ) ) ;
#80182=CARTESIAN_POINT ( 'NONE',  ( 0.3308478584281521195, -4.684245665217972032, 34.18127051446801090 ) ) ;
#80183=ORIENTED_EDGE ( 'NONE', *, *, #2486, .F. ) ;
#80184=CARTESIAN_POINT ( 'NONE',  ( 13.38461538461570122, -2.255955759149395501, 30.00000000000324363 ) ) ;
#80185=EDGE_CURVE ( 'NONE', #8069, #44632, #43605, .T. ) ;
#80186=ORIENTED_EDGE ( 'NONE', *, *, #65789, .F. ) ;
#80187=CARTESIAN_POINT ( 'NONE',  ( -0.7115616988314276137, -3.202444869320336451, 32.30641848906366675 ) ) ;
#80188=CARTESIAN_POINT ( 'NONE',  ( 2.557637826040450868, -3.202959910592335202, 32.30730279482227019 ) ) ;
#80189=CARTESIAN_POINT ( 'NONE',  ( -10.39260507411620438, -6.760870238392817200, 34.69528174975672385 ) ) ;
#80190=B_SPLINE_CURVE_WITH_KNOTS ( 'NONE', 3,
 ( #87241, #74152, #46675, #73262, #87683, #25073 ),
 .UNSPECIFIED., .F., .F.,
 ( 4, 2, 4 ),
 ( 0.0003909569690057805385, 0.0005862646681846044039, 0.0007815723673634283235 ),
 .UNSPECIFIED. ) ;
#80191=CARTESIAN_POINT ( 'NONE',  ( -10.68146699474474914, -11.91647553114624181, 32.58852847137148245 ) ) ;
#80192=CARTESIAN_POINT ( 'NONE',  ( 15.23076923076923173, -6.386643153685126251, 34.62446782046654192 ) ) ;
#80194=ADVANCED_FACE ( 'NONE', ( #8652 ), #22160, .F. ) ;
#80195=CARTESIAN_POINT ( 'NONE',  ( 4.853996859406927378, -9.086856451489516928, 34.49173150075333183 ) ) ;
#80196=VERTEX_POINT ( 'NONE', #78419 ) ;
#80197=VERTEX_POINT ( 'NONE', #36129 ) ;
#80198=ADVANCED_FACE ( 'NONE', ( #42439 ), #29371, .F. ) ;
#80199=VERTEX_POINT ( 'NONE', #8208 ) ;
#80200=DIRECTION ( 'NONE',  ( 1.000000000000000000, 0.000000000000000000, 0.000000000000000000 ) ) ;
#80201=ORIENTED_EDGE ( 'NONE', *, *, #52490, .F. ) ;
#80202=AXIS2_PLACEMENT_3D ( 'NONE', #57990, #57106, #1725 ) ;
#80203=LINE ( 'NONE', #59029, #65082 ) ;
#80204=CARTESIAN_POINT ( 'NONE',  ( 9.692307692307695177, -5.471508081941601098, 34.59228464037088457 ) ) ;
#80205=ORIENTED_EDGE ( 'NONE', *, *, #87641, .T. ) ;
#80206=EDGE_CURVE ( 'NONE', #58189, #76766, #42502, .T. ) ;
#80207=CARTESIAN_POINT ( 'NONE',  ( -14.24243673641627872, -4.481592998940250538, 33.73612834413965089 ) ) ;
#80208=EDGE_CURVE ( 'NONE', #72796, #17639, #50502, .T. ) ;
#80209=ORIENTED_EDGE ( 'NONE', *, *, #71880, .F. ) ;
#80210=CYLINDRICAL_SURFACE ( 'NONE', #48290, 0.2499999999999986955 ) ;
#80211=EDGE_LOOP ( 'NONE', ( #68684, #73662, #13010, #4134 ) ) ;
#80212=CARTESIAN_POINT ( 'NONE',  ( 7.846153846153846700, -8.318370150425687726, 35.83090037661290239 ) ) ;
#80213=B_SPLINE_CURVE_WITH_KNOTS ( 'NONE', 3,
 ( #72202, #65451, #4193, #52373, #59136, #16820, #31218, #87529, #78967, #25806 ),
 .UNSPECIFIED., .F., .F.,
 ( 4, 2, 2, 2, 4 ),
 ( 0.000000000000000000, 0.0001954311564186882026, 0.0003908623128373764051, 0.0005862934692560646619, 0.0007817246256747528103 ),
 .UNSPECIFIED. ) ;
#80214=DIRECTION ( 'NONE',  ( -0.000000000000000000, 0.6427876096865404731, -0.7660444431189771253 ) ) ;
#80215=B_SPLINE_CURVE_WITH_KNOTS ( 'NONE', 3,
 ( #38680, #73357, #72905, #80114, #86898, #26062, #53519, #32818, #73813, #58486 ),
 .UNSPECIFIED., .F., .F.,
 ( 4, 2, 2, 2, 4 ),
 ( 0.000000000000000000, 0.0001954311564186865221, 0.0003908623128373730441, 0.0005862934692560595662, 0.0007817246256747460882 ),
 .UNSPECIFIED. ) ;
#80216=DIRECTION ( 'NONE',  ( 0.000000000000000000, 0.9848077530122072432, -0.1736481776669354937 ) ) ;
#80217=FACE_BOUND ( 'NONE', #84534, .T. ) ;
#80218=CARTESIAN_POINT ( 'NONE',  ( 17.29970274590113632, -6.717445702608400460, 34.94155399931962336 ) ) ;
#80220=CARTESIAN_POINT ( 'NONE',  ( 6.000000000000001776, -11.69971097300155272, 32.46337939537588113 ) ) ;
#80221=FACE_OUTER_BOUND ( 'NONE', #28115, .T. ) ;
#80222=VECTOR ( 'NONE', #73137, 1000.000000000000227 ) ;
#80224=CARTESIAN_POINT ( 'NONE',  ( -7.846153846153965716, -12.46129190930018460, 30.37095296980731973 ) ) ;
#80225=EDGE_LOOP ( 'NONE', ( #74228, #935 ) ) ;
#80226=DIRECTION ( 'NONE',  ( 0.000000000000000000, 0.7660444431189822323, -0.6427876096865344779 ) ) ;
#80228=ORIENTED_EDGE ( 'NONE', *, *, #44813, .F. ) ;
#80229=AXIS2_PLACEMENT_3D ( 'NONE', #50864, #9899, #52657 ) ;
#80230=CARTESIAN_POINT ( 'NONE',  ( 10.83816415665302557, -12.44528174975671853, 30.48912976160716681 ) ) ;
#80231=CARTESIAN_POINT ( 'NONE',  ( 2.530703659305157949, -10.61302985866383963, 33.66295027996417843 ) ) ;
#80232=CARTESIAN_POINT ( 'NONE',  ( -4.284455809050233377, -7.722926974430166069, 34.99546784045485737 ) ) ;
#80233=CARTESIAN_POINT ( 'NONE',  ( -13.51476335434708353, -3.069018819979302926, 32.56621877034667278 ) ) ;
#80234=CARTESIAN_POINT ( 'NONE',  ( 16.94623161025552704, -8.147922237126337563, 34.70805685702651999 ) ) ;
#80235=CARTESIAN_POINT ( 'NONE',  ( -13.13466986626724520, -2.824170634883621744, 31.52227843825338738 ) ) ;
#80236=ORIENTED_EDGE ( 'NONE', *, *, #13075, .F. ) ;
#80239=CARTESIAN_POINT ( 'NONE',  ( 15.10007862765892206, -3.957541250942358424, 33.62499894934981626 ) ) ;
#80240=CARTESIAN_POINT ( 'NONE',  ( 10.39189967166066708, -3.236172620538810385, 32.36188796281390267 ) ) ;
#80241=CARTESIAN_POINT ( 'NONE',  ( 4.826923076923076650, -7.566083408709834757, 34.74999999999999289 ) ) ;
#80242=VERTEX_POINT ( 'NONE', #62684 ) ;
#80243=B_SPLINE_CURVE_WITH_KNOTS ( 'NONE', 3,
 ( #31501, #58966, #44548, #72033, #86923, #10343, #25189, #37809, #52205, #65276 ),
 .UNSPECIFIED., .F., .F.,
 ( 4, 2, 2, 2, 4 ),
 ( 0.000000000000000000, 0.0001954311564186871184, 0.0003908623128373742367, 0.0005862934692560614093, 0.0007817246256747484735 ),
 .UNSPECIFIED. ) ;
#80244=ORIENTED_EDGE ( 'NONE', *, *, #45005, .T. ) ;
#80246=ORIENTED_EDGE ( 'NONE', *, *, #8060, .F. ) ;
#80248=CARTESIAN_POINT ( 'NONE',  ( 4.853438152358743096, -3.019605429927184836, 32.48692288466676814 ) ) ;
#80250=VERTEX_POINT ( 'NONE', #55935 ) ;
#80251=CARTESIAN_POINT ( 'NONE',  ( 3.165499230212912352, -12.70778746994557551, 30.41441678777548319 ) ) ;
#80252=DIRECTION ( 'NONE',  ( -0.000000000000000000, 0.6427876096865404731, -0.7660444431189771253 ) ) ;
#80253=DIRECTION ( 'NONE',  ( -0.000000000000000000, 0.9848077530122086864, -0.1736481776669273891 ) ) ;
#80256=ORIENTED_EDGE ( 'NONE', *, *, #54701, .T. ) ;
#80258=CARTESIAN_POINT ( 'NONE',  ( 0.3962680155776850954, -10.21337939537584383, 33.94971097300158647 ) ) ;
#80261=CARTESIAN_POINT ( 'NONE',  ( -2.980714810855776609, -2.544122305571458575, 31.48381861865057729 ) ) ;
#80262=CARTESIAN_POINT ( 'NONE',  ( -7.780086512803770837, -3.322132147404559976, 32.92929555188717927 ) ) ;
#80263=CARTESIAN_POINT ( 'NONE',  ( 10.61538461538449418, -12.51329471203414379, 31.30864560766407578 ) ) ;
#80264=CARTESIAN_POINT ( 'NONE',  ( -4.023320715612508813, -5.070358843744210198, 34.40418822224088302 ) ) ;
#80265=DIRECTION ( 'NONE',  ( -0.000000000000000000, 0.1736481776669307198, -0.9848077530122080203 ) ) ;
#80266=CARTESIAN_POINT ( 'NONE',  ( 15.23076923076923173, -3.669653830205710676, 35.88435417666054406 ) ) ;
#80267=EDGE_CURVE ( 'NONE', #38598, #45177, #83875, .T. ) ;
#80269=EDGE_LOOP ( 'NONE', ( #72538, #28979, #51657, #8713, #62367, #63642 ) ) ;
#80270=AXIS2_PLACEMENT_3D ( 'NONE', #46442, #82465, #34257 ) ;
#80271=CARTESIAN_POINT ( 'NONE',  ( -7.846153846153844924, -6.189225973068211317, 35.74407628777942847 ) ) ;
#80274=ORIENTED_EDGE ( 'NONE', *, *, #7835, .F. ) ;
#80275=AXIS2_PLACEMENT_3D ( 'NONE', #44928, #64751, #30535 ) ;
#80276=ORIENTED_EDGE ( 'NONE', *, *, #72762, .T. ) ;
#80278=CARTESIAN_POINT ( 'NONE',  ( 7.780883845597525550, -6.835583212224499050, 34.95778746994557906 ) ) ;
#80279=CARTESIAN_POINT ( 'NONE',  ( -0.5276208408985972875, -9.058645607665454236, 34.76329471203372634 ) ) ;
#80280=CARTESIAN_POINT ( 'NONE',  ( 10.48523740594639442, -4.460286881179643004, 33.72017969459903242 ) ) ;
#80281=EDGE_CURVE ( 'NONE', #21202, #48918, #70347, .T. ) ;
#80282=CARTESIAN_POINT ( 'NONE',  ( 7.173131234715237170, -5.728107161865375829, 34.42597550085002922 ) ) ;
#80283=CARTESIAN_POINT ( 'NONE',  ( -15.09997878980228059, -8.191423895709840863, 34.95447573519442130 ) ) ;
#80284=ORIENTED_EDGE ( 'NONE', *, *, #33007, .F. ) ;
#80285=B_SPLINE_CURVE_WITH_KNOTS ( 'NONE', 3,
 ( #77794, #37241, #2134, #43133, #65158, #16098, #3459, #63839, #30059, #57523 ),
 .UNSPECIFIED., .F., .F.,
 ( 4, 2, 2, 2, 4 ),
 ( 0.0007817359430256398721, 0.0009771253907250089001, 0.001172514838424377820, 0.001367904286123746739, 0.001563293733823115659 ),
 .UNSPECIFIED. ) ;
#80287=CYLINDRICAL_SURFACE ( 'NONE', #54146, 0.2500000000000009437 ) ;
#80288=CARTESIAN_POINT ( 'NONE',  ( 3.930361229281822855, -8.539481045369598178, 34.89627647299170832 ) ) ;
#80289=ORIENTED_EDGE ( 'NONE', *, *, #33112, .F. ) ;
#80290=CARTESIAN_POINT ( 'NONE',  ( -7.780898274877819709, -3.835265460703683349, 33.15142922261929925 ) ) ;
#80291=ADVANCED_FACE ( 'NONE', ( #28474 ), #83427, .F. ) ;
#80292=ORIENTED_EDGE ( 'NONE', *, *, #55866, .F. ) ;
#80294=CARTESIAN_POINT ( 'NONE',  ( 1.254138676498922411, -7.276988635370452485, 34.74523720219453793 ) ) ;
#80297=CARTESIAN_POINT ( 'NONE',  ( 6.130790440966950250, -11.93129842949671726, 32.56571108434900452 ) ) ;
#80299=ADVANCED_FACE ( 'NONE', ( #3644 ), #32460, .F. ) ;
#80300=CARTESIAN_POINT ( 'NONE',  ( -13.31936024510254413, -5.094484230520773593, 34.41647553114626845 ) ) ;
#80301=CARTESIAN_POINT ( 'NONE',  ( 13.60739505359345181, -9.418065098278013636, 34.63729479722530158 ) ) ;
#80302=DIRECTION ( 'NONE',  ( -0.000000000000000000, 0.9396926207859092051, -0.3420201433256662704 ) ) ;
#80304=DIRECTION ( 'NONE',  ( -0.000000000000000000, 0.1736481776669307198, -0.9848077530122080203 ) ) ;
#80305=FACE_OUTER_BOUND ( 'NONE', #59252, .T. ) ;
#80307=AXIS2_PLACEMENT_3D ( 'NONE', #34253, #12661, #82013 ) ;
#80309=CYLINDRICAL_SURFACE ( 'NONE', #1202, 0.2499999999999998890 ) ;
#80310=VERTEX_POINT ( 'NONE', #45529 ) ;
#80312=CARTESIAN_POINT ( 'NONE',  ( -12.46153846153858424, -3.083524468854526912, 32.58852847137268327 ) ) ;
#80313=CARTESIAN_POINT ( 'NONE',  ( -0.2115930521604195702, -2.589246495874657938, 31.60778113518102828 ) ) ;
#80314=LINE ( 'NONE', #58689, #9937 ) ;
#80315=B_SPLINE_CURVE_WITH_KNOTS ( 'NONE', 3,
 ( #82457, #77454, #83338, #1349, #62164, #82895, #473, #41909, #35589, #63036 ),
 .UNSPECIFIED., .F., .F.,
 ( 4, 2, 2, 2, 4 ),
 ( 0.000000000000000000, 0.0001954339857564083688, 0.0003908679715128167377, 0.0005863019572692250523, 0.0007817359430256334753 ),
 .UNSPECIFIED. ) ;
#80316=CARTESIAN_POINT ( 'NONE',  ( -2.307692307692305711, -8.810774026931790459, 35.74407628777942847 ) ) ;
#80317=CARTESIAN_POINT ( 'NONE',  ( -6.250023237292963607, -4.335965774309649134, 33.62209801155881905 ) ) ;
#80318=CARTESIAN_POINT ( 'NONE',  ( 12.68454981315131214, -9.886259254753566594, 34.14407573483972413 ) ) ;
#80319=EDGE_CURVE ( 'NONE', #23856, #13098, #68336, .T. ) ;
#80321=ORIENTED_EDGE ( 'NONE', *, *, #64871, .F. ) ;
#80322=EDGE_LOOP ( 'NONE', ( #19421, #5586, #51970, #38616 ) ) ;
#80323=EDGE_CURVE ( 'NONE', #51403, #18589, #87651, .T. ) ;
#80324=ADVANCED_FACE ( 'NONE', ( #18512 ), #31117, .F. ) ;
#80326=ORIENTED_EDGE ( 'NONE', *, *, #55001, .F. ) ;
#80327=CARTESIAN_POINT ( 'NONE',  ( -16.15384615384627409, -3.835265460704628815, 33.15142922262033665 ) ) ;
#80328=CARTESIAN_POINT ( 'NONE',  ( -2.057746789344164107, -3.202959910592335202, 32.30730279482227019 ) ) ;
#80329=VECTOR ( 'NONE', #14216, 1000.000000000000114 ) ;
#80330=CARTESIAN_POINT ( 'NONE',  ( -3.930834802233302394, -9.086983370893049639, 34.49168942202179267 ) ) ;
#80331=EDGE_CURVE ( 'NONE', #61132, #79227, #70416, .T. ) ;
#80333=CARTESIAN_POINT ( 'NONE',  ( 0.4615384615384611755, -5.415277668671390821, 36.20867863119892149 ) ) ;
#80334=CARTESIAN_POINT ( 'NONE',  ( 8.638539302563213340, -8.999036380462717588, 34.52022231692819076 ) ) ;
#80335=CARTESIAN_POINT ( 'NONE',  ( -14.30769230769230660, -13.78497067705608181, 32.30358669280327177 ) ) ;
#80336=CARTESIAN_POINT ( 'NONE',  ( 16.85405681385997667, -2.251424796025574881, 29.88072029997477586 ) ) ;
#80338=ORIENTED_EDGE ( 'NONE', *, *, #9138, .T. ) ;
#80339=VERTEX_POINT ( 'NONE', #65354 ) ;
#80340=ORIENTED_EDGE ( 'NONE', *, *, #22052, .T. ) ;
#80341=CARTESIAN_POINT ( 'NONE',  ( -13.38461538461538325, -12.34228464037088635, 31.77849191805839268 ) ) ;
#80342=ORIENTED_EDGE ( 'NONE', *, *, #88754, .F. ) ;
#80343=CARTESIAN_POINT ( 'NONE',  ( 6.792386319966616348, -11.37499894934982514, 33.29245874905763003 ) ) ;
#80344=CARTESIAN_POINT ( 'NONE',  ( -18.00000000000012079, -11.67786785259630733, 32.92929555188604240 ) ) ;
#80345=CARTESIAN_POINT ( 'NONE',  ( 16.40384615384608935, -7.565270445406050648, 34.75000000000000000 ) ) ;
#80347=FACE_BOUND ( 'NONE', #83206, .T. ) ;
#80348=ORIENTED_EDGE ( 'NONE', *, *, #40878, .F. ) ;
#80349=B_SPLINE_CURVE_WITH_KNOTS ( 'NONE', 3,
 ( #32543, #46062, #59572, #85725, #24006, #3735, #39323, #31208, #18152, #11847 ),
 .UNSPECIFIED., .F., .F.,
 ( 4, 2, 2, 2, 4 ),
 ( 0.0007817246256747461966, 0.0009771112852218892010, 0.001172497944769032314, 0.001367884604316175427, 0.001563271263863318323 ),
 .UNSPECIFIED. ) ;
#80350=EDGE_LOOP ( 'NONE', ( #15600, #27735, #82662, #53860 ) ) ;
#80351=CARTESIAN_POINT ( 'NONE',  ( -4.853911725310227077, -6.503523203565942268, 34.64991518177335195 ) ) ;
#80352=EDGE_LOOP ( 'NONE', ( #64677, #46748, #25721, #75523 ) ) ;
#80353=FACE_BOUND ( 'NONE', #25741, .T. ) ;
#80354=CARTESIAN_POINT ( 'NONE',  ( -9.627052552794857831, -2.379036618887895305, 30.90682066428158592 ) ) ;
#80355=B_SPLINE_CURVE_WITH_KNOTS ( 'NONE', 3,
 ( #4461, #31945, #11225, #24734, #25625, #52195, #11676, #78014, #17539, #64045 ),
 .UNSPECIFIED., .F., .F.,
 ( 4, 2, 2, 2, 4 ),
 ( 0.0007817246256747440282, 0.0009771112852218863821, 0.001172497944769028844, 0.001367884604316171307, 0.001563271263863313769 ),
 .UNSPECIFIED. ) ;
#80356=CARTESIAN_POINT ( 'NONE',  ( 18.06525557127601900, -5.219633306516380244, 34.19971097300157936 ) ) ;
#80357=VERTEX_POINT ( 'NONE', #51821 ) ;
#80358=FACE_OUTER_BOUND ( 'NONE', #62579, .T. ) ;
#80359=CARTESIAN_POINT ( 'NONE',  ( -6.700064078983529292, -2.308499170217967134, 30.53291367094873721 ) ) ;
#80360=CARTESIAN_POINT ( 'NONE',  ( 1.319345384059066983, -3.643525952247789412, 33.31231777344662959 ) ) ;
#80362=B_SPLINE_CURVE_WITH_KNOTS ( 'NONE', 3,
 ( #15495, #42966, #63220, #15051, #36646, #44261, #51014, #36215, #71747, #1535 ),
 .UNSPECIFIED., .F., .F.,
 ( 4, 2, 2, 2, 4 ),
 ( 0.000000000000000000, 0.0001954311564186876876, 0.0003908623128373753751, 0.0005862934692560630356, 0.0007817246256747507503 ),
 .UNSPECIFIED. ) ;
#80363=CARTESIAN_POINT ( 'NONE',  ( 18.06514478071962415, -7.750023224968865421, 34.99404313364389907 ) ) ;
#80364=CARTESIAN_POINT ( 'NONE',  ( 7.053867364043872712, -5.496552790871117367, 34.60292014791297532 ) ) ;
#80365=CARTESIAN_POINT ( 'NONE',  ( -9.442253380669379581, -2.564540009722895419, 30.55348353981670684 ) ) ;
#80366=VERTEX_POINT ( 'NONE', #86083 ) ;
#80367=AXIS2_PLACEMENT_3D ( 'NONE', #56702, #8084, #28343 ) ;
#80368=CARTESIAN_POINT ( 'NONE',  ( -2.530618525208451874, -11.24512374952581872, 33.06303171183252942 ) ) ;
#80369=CARTESIAN_POINT ( 'NONE',  ( -16.82686876528476816, -11.79725096376909299, 32.30694842903960762 ) ) ;
#80370=VECTOR ( 'NONE', #2689, 1000.000000000000114 ) ;
#80371=VERTEX_POINT ( 'NONE', #39233 ) ;
#80372=CARTESIAN_POINT ( 'NONE',  ( 0.3308469948709026887, -8.999036380462717588, 34.52022231692819076 ) ) ;
#80373=CARTESIAN_POINT ( 'NONE',  ( 14.53047184896071542, -8.496831190052093419, 34.64984203495476578 ) ) ;
#80374=DIRECTION ( 'NONE',  ( 0.000000000000000000, 0.000000000000000000, -1.000000000000000000 ) ) ;
#80375=CARTESIAN_POINT ( 'NONE',  ( 18.00000000000000000, -13.53365097954675988, 30.81389545987213552 ) ) ;
#80376=CARTESIAN_POINT ( 'NONE',  ( -10.61538461538473399, -2.625532179533778709, 30.86335684631627174 ) ) ;
#80377=CARTESIAN_POINT ( 'NONE',  ( 10.61538461538461675, -11.16473453929635440, 33.15142922261926373 ) ) ;
#80379=LINE ( 'NONE', #39393, #79109 ) ;
#80380=VECTOR ( 'NONE', #65372, 999.9999999999998863 ) ;
#80381=CARTESIAN_POINT ( 'NONE',  ( -3.296852641725110722, -2.538708090699994813, 30.37095296980875148 ) ) ;
#80382=CARTESIAN_POINT ( 'NONE',  ( -12.39628289026243735, -11.48612834413965977, 32.76840700105972815 ) ) ;
#80384=ORIENTED_EDGE ( 'NONE', *, *, #13533, .T. ) ;
#80386=EDGE_LOOP ( 'NONE', ( #13743, #55217 ) ) ;
#80388=CYLINDRICAL_SURFACE ( 'NONE', #41287, 0.2500000000000009437 ) ;
#80389=EDGE_LOOP ( 'NONE', ( #70639, #3125, #28858, #249 ) ) ;
#80390=CARTESIAN_POINT ( 'NONE',  ( 3.361294932532794100, -10.19071101563364401, 33.96452234770658407 ) ) ;
#80392=DIRECTION ( 'NONE',  ( 0.000000000000000000, 0.4999999999999960032, -0.8660254037844410391 ) ) ;
#80393=CARTESIAN_POINT ( 'NONE',  ( -15.29685161012936767, -12.34228464037088280, 31.77849191805838558 ) ) ;
#80394=CARTESIAN_POINT ( 'NONE',  ( -3.230769230769229949, -8.973038597847269315, 34.52809138561121927 ) ) ;
#80395=CARTESIAN_POINT ( 'NONE',  ( 9.692307692307570832, -3.083524468854526912, 32.58852847137268327 ) ) ;
#80396=CARTESIAN_POINT ( 'NONE',  ( -5.011667937410240192, -2.657715359629131857, 31.77849191805844242 ) ) ;
#80398=CARTESIAN_POINT ( 'NONE',  ( -1.384615384615383471, -12.09954503811598769, 35.62045528018868623 ) ) ;
#80400=DIRECTION ( 'NONE',  ( 0.000000000000000000, 0.9848077530122072432, 0.1736481776669354937 ) ) ;
#80401=CARTESIAN_POINT ( 'NONE',  ( -14.55769230769230660, -2.499999999999999556, 29.81609845454691765 ) ) ;
#80402=B_SPLINE_CURVE_WITH_KNOTS ( 'NONE', 3,
 ( #68816, #74700, #53970, #81905, #33267, #27392, #40476, #67940, #20195, #54409 ),
 .UNSPECIFIED., .F., .F.,
 ( 4, 2, 2, 2, 4 ),
 ( 0.000000000000000000, 0.0001954311564186865492, 0.0003908623128373730983, 0.0005862934692560596746, 0.0007817246256747461966 ),
 .UNSPECIFIED. ) ;
#80403=DIRECTION ( 'NONE',  ( -0.000000000000000000, 0.1736481776669307198, -0.9848077530122080203 ) ) ;
#80404=EDGE_CURVE ( 'NONE', #30732, #23776, #23183, .T. ) ;
#80405=ORIENTED_EDGE ( 'NONE', *, *, #87751, .T. ) ;
#80406=ORIENTED_EDGE ( 'NONE', *, *, #77522, .F. ) ;
#80407=CARTESIAN_POINT ( 'NONE',  ( -8.992715712954719720, -12.44517049084099725, 30.48991314939691932 ) ) ;
#80408=CARTESIAN_POINT ( 'NONE',  ( 15.23076923076923173, -1.117168528481311540, 33.14645433367849847 ) ) ;
#80409=LINE ( 'NONE', #3840, #5199 ) ;
#80411=DIRECTION ( 'NONE',  ( -0.000000000000000000, 0.9848077530122086864, -0.1736481776669273891 ) ) ;
#80412=CARTESIAN_POINT ( 'NONE',  ( -16.15384615384627409, -9.442884908241554243, 34.35708131394783038 ) ) ;
#80413=EDGE_CURVE ( 'NONE', #81993, #35424, #4546, .T. ) ;
#80414=VERTEX_POINT ( 'NONE', #73460 ) ;
#80415=CARTESIAN_POINT ( 'NONE',  ( -4.946131269098290595, -12.38066358083363738, 30.83685684665853444 ) ) ;
#80416=ORIENTED_EDGE ( 'NONE', *, *, #44589, .F. ) ;
#80417=EDGE_LOOP ( 'NONE', ( #70682, #82515 ) ) ;
#80418=CARTESIAN_POINT ( 'NONE',  ( 0.5923289025054097046, -12.35292014791297710, 31.75344720912887198 ) ) ;
#80419=B_SPLINE_CURVE_WITH_KNOTS ( 'NONE', 3,
 ( #80113, #18416, #11663, #26061, #45873, #73356, #39140, #18858, #28267, #76907 ),
 .UNSPECIFIED., .F., .F.,
 ( 4, 2, 2, 2, 4 ),
 ( 0.000000000000000000, 0.0001954339857564080707, 0.0003908679715128161414, 0.0005863019572692241849, 0.0007817359430256322827 ),
 .UNSPECIFIED. ) ;
#80420=CARTESIAN_POINT ( 'NONE',  ( -14.17716686945866655, -6.808710257144161559, 34.95449254468098843 ) ) ;
#80421=CARTESIAN_POINT ( 'NONE',  ( -4.376773112753000738, -12.64616026154729411, 30.79003144601913533 ) ) ;
#80422=CARTESIAN_POINT ( 'NONE',  ( 1.384615384615386802, -11.35647404775217417, 33.31231777344666511 ) ) ;
#80423=CARTESIAN_POINT ( 'NONE',  ( 6.000000000000001776, -2.721908614388771852, 31.22303859784724978 ) ) ;
#80424=B_SPLINE_CURVE_WITH_KNOTS ( 'NONE', 3,
 ( #79564, #57501, #77776, #11097, #86784, #38574, #43984, #71454, #9761, #66028 ),
 .UNSPECIFIED., .F., .F.,
 ( 4, 2, 2, 2, 4 ),
 ( 0.0007817246256747477145, 0.0009771112852218913694, 0.001172497944769034916, 0.001367884604316178462, 0.001563271263863322009 ),
 .UNSPECIFIED. ) ;
#80425=AXIS2_PLACEMENT_3D ( 'NONE', #5215, #12418, #88545 ) ;
#80426=VERTEX_POINT ( 'NONE', #6760 ) ;
#80427=VECTOR ( 'NONE', #29977, 1000.000000000000114 ) ;
#80428=VERTEX_POINT ( 'NONE', #457 ) ;
#80429=B_SPLINE_CURVE_WITH_KNOTS ( 'NONE', 3,
 ( #77390, #16134, #72843, #11150, #44923, #38625, #73762, #33201, #66084, #72399 ),
 .UNSPECIFIED., .F., .F.,
 ( 4, 2, 2, 2, 4 ),
 ( 0.0007817246256747516176, 0.0009771112852218970073, 0.001172497944769042288, 0.001367884604316187570, 0.001563271263863332851 ),
 .UNSPECIFIED. ) ;
#80431=EDGE_CURVE ( 'NONE', #77897, #72081, #5974, .T. ) ;
#80433=ORIENTED_EDGE ( 'NONE', *, *, #8922, .F. ) ;
#80434=CARTESIAN_POINT ( 'NONE',  ( -6.066082379360133281, -4.661471528628507777, 34.16647553114621871 ) ) ;
#80435=CARTESIAN_POINT ( 'NONE',  ( -0.4615384615384611200, -9.905515769479276145, 34.41647553114623292 ) ) ;
#80436=CARTESIAN_POINT ( 'NONE',  ( 16.40379156322419973, -5.766571408460170467, 34.70601412856602508 ) ) ;
#80437=CARTESIAN_POINT ( 'NONE',  ( 10.61538461538461675, -4.661471528628507777, 34.16647553114623292 ) ) ;
#80438=EDGE_CURVE ( 'NONE', #38767, #65096, #25255, .T. ) ;
#80439=CARTESIAN_POINT ( 'NONE',  ( -16.85391172531022974, -3.105924265160262099, 32.13625925475356127 ) ) ;
#80440=CARTESIAN_POINT ( 'NONE',  ( 17.99999999999987566, -8.613356846316285953, 34.62446782046622218 ) ) ;
#80441=ORIENTED_EDGE ( 'NONE', *, *, #11863, .T. ) ;
#80442=ORIENTED_EDGE ( 'NONE', *, *, #39622, .T. ) ;
#80443=CARTESIAN_POINT ( 'NONE',  ( 11.78846153846154188, -2.499999999999999556, 29.81604066197449754 ) ) ;
#80444=CARTESIAN_POINT ( 'NONE',  ( -12.46153846153846168, -11.16473453929635440, 33.15142922261926373 ) ) ;
#80445=VERTEX_POINT ( 'NONE', #74344 ) ;
#80447=CARTESIAN_POINT ( 'NONE',  ( 12.59206389977210705, -8.630441415882550871, 34.87705825610312615 ) ) ;
#80449=VERTEX_POINT ( 'NONE', #81551 ) ;
#80450=CARTESIAN_POINT ( 'NONE',  ( 6.923076923076924238, -12.78798330534102945, 29.74999999999997868 ) ) ;
#80451=AXIS2_PLACEMENT_3D ( 'NONE', #35147, #12667, #482 ) ;
#80453=CARTESIAN_POINT ( 'NONE',  ( -13.51476335434708353, -11.66186481527757302, 32.95055677023626117 ) ) ;
#80454=CARTESIAN_POINT ( 'NONE',  ( 0.2115152373170025857, -11.56360843649121861, 33.07473185843129926 ) ) ;
#80455=CARTESIAN_POINT ( 'NONE',  ( 1.384615384615386802, -1.466349020453238561, 30.81389545987213907 ) ) ;
#80456=DIRECTION ( 'NONE',  ( 0.000000000000000000, 0.7660444431189822323, -0.6427876096865344779 ) ) ;
#80457=DIRECTION ( 'NONE',  ( -0.000000000000000000, 1.000000000000000000, 3.491481338843133355E-15 ) ) ;
#80458=LINE ( 'NONE', #39918, #69283 ) ;
#80459=ORIENTED_EDGE ( 'NONE', *, *, #16422, .F. ) ;
#80460=CARTESIAN_POINT ( 'NONE',  ( 6.923076923076924238, -8.120952969808772792, 34.71129190930000163 ) ) ;
#80461=CARTESIAN_POINT ( 'NONE',  ( -8.899921372341079717, -3.957541250942358424, 33.62499894934981626 ) ) ;
#80462=CARTESIAN_POINT ( 'NONE',  ( -11.53846153846153655, -1.422936976036506707, 30.56769352161908415 ) ) ;
#80463=ORIENTED_EDGE ( 'NONE', *, *, #54978, .T. ) ;
#80464=B_SPLINE_CURVE_WITH_KNOTS ( 'NONE', 3,
 ( #61395, #42481, #14113, #35267, #35725, #14555, #88911, #55981, #69057, #47892 ),
 .UNSPECIFIED., .F., .F.,
 ( 4, 2, 2, 2, 4 ),
 ( 0.000000000000000000, 0.0001954339857564074473, 0.0003908679715128148945, 0.0005863019572692223418, 0.0007817359430256297891 ),
 .UNSPECIFIED. ) ;
#80465=DIRECTION ( 'NONE',  ( -0.000000000000000000, -0.9396926207859092051, -0.3420201433256662704 ) ) ;
#80466=DIRECTION ( 'NONE',  ( -0.000000000000000000, 0.3420201433256694346, -0.9396926207859080948 ) ) ;
#80467=CARTESIAN_POINT ( 'NONE',  ( -18.00000000000000000, -1.503186988994757778, 30.80739993210377747 ) ) ;
#80468=CARTESIAN_POINT ( 'NONE',  ( 7.912222197156284054, -3.050289026998446840, 32.03036669348366416 ) ) ;
#80469=FACE_BOUND ( 'NONE', #57832, .T. ) ;
#80472=CARTESIAN_POINT ( 'NONE',  ( -15.16470189741915675, -4.661471528628508665, 34.16647553114624003 ) ) ;
#80473=CARTESIAN_POINT ( 'NONE',  ( -1.254089682851818210, -12.27024696741798770, 31.24895572276497546 ) ) ;
#80474=CARTESIAN_POINT ( 'NONE',  ( -2.307692307692305711, -8.164416787775445883, 34.95778746994557906 ) ) ;
#80476=LINE ( 'NONE', #66956, #59186 ) ;
#80478=CARTESIAN_POINT ( 'NONE',  ( 10.36536139116315525, -12.07920672191015221, 32.31858351112116168 ) ) ;
#80479=VERTEX_POINT ( 'NONE', #13963 ) ;
#80480=VECTOR ( 'NONE', #42020, 1000.000000000000000 ) ;
#80481=VECTOR ( 'NONE', #33678, 1000.000000000000114 ) ;
#80482=CARTESIAN_POINT ( 'NONE',  ( 0.2115617305961066674, -6.567427716900047230, 34.66269422305636283 ) ) ;
#80483=CARTESIAN_POINT ( 'NONE',  ( 16.40379156322419973, -12.68172785388650681, 30.59649109432439573 ) ) ;
#80485=CARTESIAN_POINT ( 'NONE',  ( -7.846153846153844924, -9.058645607665452459, 34.76329471203371924 ) ) ;
#80486=CARTESIAN_POINT ( 'NONE',  ( 17.07692307692295586, -12.70778746994576025, 30.41441678777401236 ) ) ;
#80487=CARTESIAN_POINT ( 'NONE',  ( -12.59168643127016196, -6.809168938359901446, 34.95455904226513866 ) ) ;
#80490=EDGE_CURVE ( 'NONE', #79832, #1945, #20721, .T. ) ;
#80491=CARTESIAN_POINT ( 'NONE',  ( 4.219914504848590653, -10.51840700105979565, 33.73612834413962247 ) ) ;
#80492=CARTESIAN_POINT ( 'NONE',  ( 8.546303810323916395, -2.523278758544489797, 31.42238647778637528 ) ) ;
#80494=CARTESIAN_POINT ( 'NONE',  ( -4.826977667545033768, -12.07971442181322352, 32.31769673815850297 ) ) ;
#80495=CARTESIAN_POINT ( 'NONE',  ( -0.5268084620947810492, -8.656820664281497102, 34.87096338111211935 ) ) ;
#80496=CARTESIAN_POINT ( 'NONE',  ( -7.053224132515142131, -4.460286881179643004, 33.72017969459903242 ) ) ;
#80497=CARTESIAN_POINT ( 'NONE',  ( -9.019207500173124004, -9.148715823498378086, 34.47080413974185120 ) ) ;
#80499=CARTESIAN_POINT ( 'NONE',  ( 3.453732365035905971, -7.369474539155830506, 34.99858011523957657 ) ) ;
#80500=CARTESIAN_POINT ( 'NONE',  ( 8.068933515131908152, -9.418065098278013636, 34.63729479722530158 ) ) ;
#80501=EDGE_LOOP ( 'NONE', ( #48055, #5095, #19198, #9851 ) ) ;
#80503=CARTESIAN_POINT ( 'NONE',  ( -2.307692307692305711, -10.89733346790207413, 36.13435417666054406 ) ) ;
#80505=EDGE_CURVE ( 'NONE', #42562, #72489, #66089, .T. ) ;
#80506=CARTESIAN_POINT ( 'NONE',  ( 16.15384615384615330, -13.57706302396349152, 30.56769352161908060 ) ) ;
#80507=DIRECTION ( 'NONE',  ( -0.000000000000000000, -0.9396926207859092051, -0.3420201433256662704 ) ) ;
#80509=LINE ( 'NONE', #75081, #19807 ) ;
#80510=CARTESIAN_POINT ( 'NONE',  ( 9.469380733400845074, -12.64616026154729411, 30.79003144601914244 ) ) ;
#80511=CARTESIAN_POINT ( 'NONE',  ( 11.47319153790521717, -3.083524468853724443, 32.58852847137143272 ) ) ;
#80512=EDGE_LOOP ( 'NONE', ( #46274, #55294 ) ) ;
#80513=CARTESIAN_POINT ( 'NONE',  ( -9.942284436356281674, -11.47974371597208076, 33.17467449705390692 ) ) ;
#80514=CARTESIAN_POINT ( 'NONE',  ( -2.980714919130916574, -3.627508038966689163, 32.91356715214248396 ) ) ;
#80515=EDGE_CURVE ( 'NONE', #15626, #62076, #71514, .T. ) ;
#80516=CARTESIAN_POINT ( 'NONE',  ( 2.177545098254089151, -12.45813303252208648, 30.39737893381572675 ) ) ;
#80517=CARTESIAN_POINT ( 'NONE',  ( 11.53846153846153832, -8.973038597847269315, 34.52809138561121927 ) ) ;
#80518=ORIENTED_EDGE ( 'NONE', *, *, #17584, .T. ) ;
#80522=EDGE_CURVE ( 'NONE', #82892, #54013, #54274, .T. ) ;
#80524=ORIENTED_EDGE ( 'NONE', *, *, #1988, .T. ) ;
#80525=B_SPLINE_CURVE_WITH_KNOTS ( 'NONE', 3,
 ( #73462, #80671, #11755, #59931, #25713, #53168 ),
 .UNSPECIFIED., .F., .F.,
 ( 4, 2, 4 ),
 ( 4.220987180333913997E-17, 0.0001954756301637163962, 0.0003909512603273906169 ),
 .UNSPECIFIED. ) ;
#80526=VECTOR ( 'NONE', #56746, 1000.000000000000114 ) ;
#80528=EDGE_CURVE ( 'NONE', #76451, #76314, #26376, .T. ) ;
#80529=B_SPLINE_CURVE_WITH_KNOTS ( 'NONE', 3,
 ( #64574, #23162, #86671, #24937, #51494, #2873, #78109, #10990, #71788, #24485 ),
 .UNSPECIFIED., .F., .F.,
 ( 4, 2, 2, 2, 4 ),
 ( 0.0007817246256747503166, 0.0009771112852218944052, 0.001172497944769038602, 0.001367884604316182799, 0.001563271263863326996 ),
 .UNSPECIFIED. ) ;
#80530=CARTESIAN_POINT ( 'NONE',  ( -15.23076923076922995, -2.249999999999998668, 29.75000000000001776 ) ) ;
#80532=B_SPLINE_CURVE_WITH_KNOTS ( 'NONE', 3,
 ( #27773, #40855, #49379, #83625, #54352, #41741, #35417, #308, #1184, #28670 ),
 .UNSPECIFIED., .F., .F.,
 ( 4, 2, 2, 2, 4 ),
 ( 0.0007817246256747446788, 0.0009771112852218879000, 0.001172497944769031013, 0.001367884604316174126, 0.001563271263863317238 ),
 .UNSPECIFIED. ) ;
#80533=CARTESIAN_POINT ( 'NONE',  ( -9.626240358957616650, -12.62096338111211757, 30.90682066428152908 ) ) ;
#80534=CYLINDRICAL_SURFACE ( 'NONE', #30502, 0.2500000000000008882 ) ;
#80535=EDGE_LOOP ( 'NONE', ( #65374, #86567 ) ) ;
#80536=EDGE_CURVE ( 'NONE', #26904, #60833, #39321, .T. ) ;
#80537=VERTEX_POINT ( 'NONE', #55833 ) ;
#80538=AXIS2_PLACEMENT_3D ( 'NONE', #45086, #18074, #65361 ) ;
#80539=VERTEX_POINT ( 'NONE', #82880 ) ;
#80541=EDGE_CURVE ( 'NONE', #33660, #58760, #61806, .T. ) ;
#80542=ORIENTED_EDGE ( 'NONE', *, *, #35160, .F. ) ;
#80543=CARTESIAN_POINT ( 'NONE',  ( -2.307692307692427391, -3.835265460704628371, 33.15142922262033665 ) ) ;
#80544=B_SPLINE_CURVE_WITH_KNOTS ( 'NONE', 3,
 ( #25898, #38525, #66439, #31773, #4746, #59231, #52908, #44817, #80861, #30862 ),
 .UNSPECIFIED., .F., .F.,
 ( 4, 2, 2, 2, 4 ),
 ( 0.0007817359430256315238, 0.0009771253907249980580, 0.001172514838424364592, 0.001367904286123730910, 0.001563293733823097444 ),
 .UNSPECIFIED. ) ;
#80545=CARTESIAN_POINT ( 'NONE',  ( 15.00728428704528561, -3.236172620538810385, 32.36188796281390267 ) ) ;
#80546=AXIS2_PLACEMENT_3D ( 'NONE', #32616, #11917, #60085 ) ;
#80547=VECTOR ( 'NONE', #76558, 1000.000000000000227 ) ;
#80548=EDGE_CURVE ( 'NONE', #73980, #34740, #43208, .T. ) ;
#80549=EDGE_CURVE ( 'NONE', #77001, #86079, #49971, .T. ) ;
#80550=DIRECTION ( 'NONE',  ( 0.000000000000000000, 1.000000000000000000, 0.000000000000000000 ) ) ;
#80551=CARTESIAN_POINT ( 'NONE',  ( -13.31854703361294767, -12.37446782046654192, 30.86335684631486842 ) ) ;
#80553=ORIENTED_EDGE ( 'NONE', *, *, #9098, .T. ) ;
#80554=VECTOR ( 'NONE', #66125, 999.9999999999998863 ) ;
#80555=ORIENTED_EDGE ( 'NONE', *, *, #53146, .T. ) ;
#80556=CARTESIAN_POINT ( 'NONE',  ( 6.923076923076924238, -13.04860791097971706, 34.73218667398347037 ) ) ;
#80557=CARTESIAN_POINT ( 'NONE',  ( 5.299934428535925335, -4.887748414852792322, 34.01359900205216746 ) ) ;
#80558=EDGE_LOOP ( 'NONE', ( #52805, #83598 ) ) ;
#80560=CARTESIAN_POINT ( 'NONE',  ( 17.01084069756293715, -5.471508081941601986, 34.59228464037088457 ) ) ;
#80561=CARTESIAN_POINT ( 'NONE',  ( -0.3962833220256226641, -5.094484230520773593, 34.41647553114626845 ) ) ;
#80562=DIRECTION ( 'NONE',  ( -0.000000000000000000, 0.5000000000000011102, -0.8660254037844381525 ) ) ;
#80563=B_SPLINE_CURVE_WITH_KNOTS ( 'NONE', 3,
 ( #73724, #13334, #39495, #68279, #12450, #19647, #66955, #26412, #12888, #60627 ),
 .UNSPECIFIED., .F., .F.,
 ( 4, 2, 2, 2, 4 ),
 ( 0.0007817359430256216575, 0.0009771253907249856981, 0.001172514838424349847, 0.001367904286123713779, 0.001563293733823077928 ),
 .UNSPECIFIED. ) ;
#80564=CARTESIAN_POINT ( 'NONE',  ( -13.63461538461539035, -2.499999999999999556, 29.81609845454691765 ) ) ;
#80565=CARTESIAN_POINT ( 'NONE',  ( 9.019285080869080318, -5.728107161865378494, 34.42597550085002922 ) ) ;
#80566=FACE_BOUND ( 'NONE', #77469, .T. ) ;
#80568=CARTESIAN_POINT ( 'NONE',  ( -12.59222992820601839, -8.999036380462717588, 34.52022231692819076 ) ) ;
#80569=CYLINDRICAL_SURFACE ( 'NONE', #59562, 0.2499999999999979738 ) ;
#80571=CARTESIAN_POINT ( 'NONE',  ( -5.076923076923197442, -3.300289026999228881, 32.46337939537708905 ) ) ;
#80573=CARTESIAN_POINT ( 'NONE',  ( 3.230769230769231726, -10.67929555188718282, 33.92786785259544047 ) ) ;
#80575=CARTESIAN_POINT ( 'NONE',  ( -17.20707104665477161, -5.915902021225892149, 34.75552854090298638 ) ) ;
#80576=CARTESIAN_POINT ( 'NONE',  ( 12.52760579488853665, -3.322132147404559976, 32.92929555188717927 ) ) ;
#80577=ORIENTED_EDGE ( 'NONE', *, *, #41178, .F. ) ;
#80578=ORIENTED_EDGE ( 'NONE', *, *, #17135, .T. ) ;
#80579=CARTESIAN_POINT ( 'NONE',  ( -17.07692307692319744, -11.48612834414049644, 32.76840700105863391 ) ) ;
#80580=CARTESIAN_POINT ( 'NONE',  ( -15.48079246806219267, -2.587272538249755893, 30.68239716806877837 ) ) ;
#80581=CARTESIAN_POINT ( 'NONE',  ( 12.23861150263161157, -10.77366814457252175, 33.85459836347579454 ) ) ;
#80583=EDGE_CURVE ( 'NONE', #51136, #27202, #71111, .T. ) ;
#80584=CARTESIAN_POINT ( 'NONE',  ( -6.000000000000119904, -8.613356846316285953, 34.62446782046622218 ) ) ;
#80585=CARTESIAN_POINT ( 'NONE',  ( 14.30769230769218758, -3.300289026999228881, 32.46337939537708905 ) ) ;
#80586=CARTESIAN_POINT ( 'NONE',  ( -18.00000000000000000, -3.050289026998447284, 32.03036669348365706 ) ) ;
#80587=CARTESIAN_POINT ( 'NONE',  ( -0.4615384615385826339, -3.835265460704628371, 33.15142922262033665 ) ) ;
#80588=CARTESIAN_POINT ( 'NONE',  ( -12.68502340526241312, -5.113361153441934093, 34.14387501736622710 ) ) ;
#80589=CARTESIAN_POINT ( 'NONE',  ( -9.442307692307691624, -2.249999999999998668, 29.75000000000000355 ) ) ;
#80592=VECTOR ( 'NONE', #71155, 1000.000000000000114 ) ;
#80594=ORIENTED_EDGE ( 'NONE', *, *, #15087, .T. ) ;
#80596=CARTESIAN_POINT ( 'NONE',  ( -9.915792616872025178, -2.612411019501189369, 31.66733052389439962 ) ) ;
#80597=CARTESIAN_POINT ( 'NONE',  ( 7.053868730901711182, -12.11778462344220841, 31.66786338562085135 ) ) ;
#80598=CYLINDRICAL_SURFACE ( 'NONE', #33028, 0.2500000000000012212 ) ;
#80599=LINE ( 'NONE', #18884, #22246 ) ;
#80600=CARTESIAN_POINT ( 'NONE',  ( -15.23076923076922995, -2.721908614388771852, 31.22303859784724978 ) ) ;
#80602=ADVANCED_FACE ( 'NONE', ( #77002 ), #48628, .F. ) ;
#80603=EDGE_CURVE ( 'NONE', #63637, #62369, #15706, .T. ) ;
#80604=CARTESIAN_POINT ( 'NONE',  ( -7.623374304885435215, -8.496831190052096971, 34.64984203495476578 ) ) ;
#80605=CARTESIAN_POINT ( 'NONE',  ( 1.384615384615265343, -5.219633306517616589, 34.19971097300220464 ) ) ;
#80607=B_SPLINE_CURVE_WITH_KNOTS ( 'NONE', 3,
 ( #23, #20731, #27934, #43218, #62158, #15755, #63027, #70246, #49537, #62591 ),
 .UNSPECIFIED., .F., .F.,
 ( 4, 2, 2, 2, 4 ),
 ( 0.0007817359430256327164, 0.0009771253907249993591, 0.001172514838424366110, 0.001367904286123732861, 0.001563293733823099396 ),
 .UNSPECIFIED. ) ;
#80608=LINE ( 'NONE', #53102, #38106 ) ;
#80609=CARTESIAN_POINT ( 'NONE',  ( -9.822999158975251888, -11.18331474514187995, 33.13161551792790505 ) ) ;
#80610=CARTESIAN_POINT ( 'NONE',  ( 13.63456079399342791, -2.589246495874658383, 31.60778113518102828 ) ) ;
#80611=DIRECTION ( 'NONE',  ( -0.000000000000000000, 1.000000000000000000, -0.000000000000000000 ) ) ;
#80612=CARTESIAN_POINT ( 'NONE',  ( 7.911408985666682270, -8.656820664281605460, 34.87096338111211224 ) ) ;
#80614=VECTOR ( 'NONE', #60720, 999.9999999999998863 ) ;
#80615=CARTESIAN_POINT ( 'NONE',  ( -15.29603967673000575, -10.21337939537584383, 33.94971097300158647 ) ) ;
#80616=VERTEX_POINT ( 'NONE', #14866 ) ;
#80617=CARTESIAN_POINT ( 'NONE',  ( -5.011667505647051435, -11.94971097300157403, 32.03036669348361443 ) ) ;
#80618=CARTESIAN_POINT ( 'NONE',  ( -3.360916440207453615, -3.817052484675422797, 33.13202310037935661 ) ) ;
#80619=CARTESIAN_POINT ( 'NONE',  ( 5.869309396889695662, -2.494641256782728966, 31.33461815524612959 ) ) ;
#80621=AXIS2_PLACEMENT_3D ( 'NONE', #20551, #7034, #48013 ) ;
#80623=EDGE_CURVE ( 'NONE', #9301, #35110, #16626, .T. ) ;
#80624=CARTESIAN_POINT ( 'NONE',  ( -14.05763799605399278, -4.943051570960394159, 34.04725096376909477 ) ) ;
#80625=( LENGTH_UNIT ( ) NAMED_UNIT ( * ) SI_UNIT ( .MILLI., .METRE. ) );
#80626=CARTESIAN_POINT ( 'NONE',  ( -18.25000000000000711, -2.249999999999998668, 29.75000000000000355 ) ) ;
#80627=ORIENTED_EDGE ( 'NONE', *, *, #51307, .T. ) ;
#80629=CARTESIAN_POINT ( 'NONE',  ( -9.692307692307691624, -11.69971097300155272, 32.46337939537588113 ) ) ;
#80630=EDGE_CURVE ( 'NONE', #54915, #78412, #67231, .T. ) ;
#80633=VECTOR ( 'NONE', #12872, 1000.000000000000000 ) ;
#80634=CARTESIAN_POINT ( 'NONE',  ( -7.053224892808620083, -11.66186481527757479, 32.95055677023626117 ) ) ;
#80636=ORIENTED_EDGE ( 'NONE', *, *, #41708, .T. ) ;
#80637=CARTESIAN_POINT ( 'NONE',  ( 3.100078627658922947, -4.684245665217971144, 34.18127051446801090 ) ) ;
#80638=CARTESIAN_POINT ( 'NONE',  ( -7.596099534515528440, -11.79725096376909654, 32.30694842903960762 ) ) ;
#80640=ADVANCED_FACE ( 'NONE', ( #85968 ), #45411, .F. ) ;
#80641=ORIENTED_EDGE ( 'NONE', *, *, #57231, .F. ) ;
#80642=CARTESIAN_POINT ( 'NONE',  ( 0.4615384615383382183, -5.094484230521993062, 34.41647553114689373 ) ) ;
#80644=EDGE_LOOP ( 'NONE', ( #39594, #67791 ) ) ;
#80646=DIRECTION ( 'NONE',  ( 0.000000000000000000, -0.000000000000000000, 1.000000000000000000 ) ) ;
#80647=CARTESIAN_POINT ( 'NONE',  ( 18.00000000000000000, -9.905515769479276145, 34.41647553114623292 ) ) ;
#80648=CARTESIAN_POINT ( 'NONE',  ( -14.30769230769230660, -1.790695186598648903, 34.54067556320373455 ) ) ;
#80649=CARTESIAN_POINT ( 'NONE',  ( -5.076923076923075762, -1.629998284177014645, 34.34916445242399163 ) ) ;
#80650=CARTESIAN_POINT ( 'NONE',  ( 12.46153846153846168, -4.786620604624113540, 33.94971097300155094 ) ) ;
#80651=CARTESIAN_POINT ( 'NONE',  ( 10.61538461538449596, -12.27809138561165270, 31.22303859784587132 ) ) ;
#80653=EDGE_LOOP ( 'NONE', ( #81319, #84306, #87945, #40823 ) ) ;
#80655=ORIENTED_EDGE ( 'NONE', *, *, #39434, .T. ) ;
#80656=LINE ( 'NONE', #17615, #4154 ) ;
#80657=ORIENTED_EDGE ( 'NONE', *, *, #504, .T. ) ;
#80658=EDGE_CURVE ( 'NONE', #32515, #76205, #47918, .T. ) ;
#80660=CARTESIAN_POINT ( 'NONE',  ( -14.17690186672535901, -10.70102852606553157, 33.91149625220312913 ) ) ;
#80661=CARTESIAN_POINT ( 'NONE',  ( 1.384615384615265343, -2.892918686052166066, 31.69288490824153470 ) ) ;
#80663=CARTESIAN_POINT ( 'NONE',  ( 14.53070515178570332, -11.98016756924215009, 32.48728574198911190 ) ) ;
#80664=EDGE_LOOP ( 'NONE', ( #4503, #79315 ) ) ;
#80665=CARTESIAN_POINT ( 'NONE',  ( 17.01083966596719321, -9.780366693483667717, 34.19971097300155805 ) ) ;
#80666=ORIENTED_EDGE ( 'NONE', *, *, #5296, .F. ) ;
#80667=DIRECTION ( 'NONE',  ( 0.000000000000000000, 0.000000000000000000, 1.000000000000000000 ) ) ;
#80669=CARTESIAN_POINT ( 'NONE',  ( -11.60373198442231235, -3.835265460703609186, 33.15142922261924241 ) ) ;
#80671=CARTESIAN_POINT ( 'NONE',  ( 3.903846153846132871, -2.249999999999999112, 29.81609741502488120 ) ) ;
#80672=FACE_BOUND ( 'NONE', #85959, .T. ) ;
#80673=CYLINDRICAL_SURFACE ( 'NONE', #65665, 0.2499999999999993616 ) ;
#80674=CARTESIAN_POINT ( 'NONE',  ( 16.02315555073584363, -3.338472653186243200, 32.95098750199972670 ) ) ;
#80675=AXIS2_PLACEMENT_3D ( 'NONE', #18241, #11037, #25437 ) ;
#80676=VECTOR ( 'NONE', #4454, 1000.000000000000114 ) ;
#80678=CARTESIAN_POINT ( 'NONE',  ( -3.454254174493179175, -4.386631170607603991, 33.66268669641500111 ) ) ;
#80679=ADVANCED_FACE ( 'NONE', ( #11195 ), #31920, .F. ) ;
#80680=CARTESIAN_POINT ( 'NONE',  ( -8.769230769230768274, -13.20930481340135110, 34.54067556320372745 ) ) ;
#80681=CYLINDRICAL_SURFACE ( 'NONE', #51964, 0.2499999999999998890 ) ;
#80682=ORIENTED_EDGE ( 'NONE', *, *, #67216, .T. ) ;
#80683=CARTESIAN_POINT ( 'NONE',  ( -13.38461538461507594, -2.506253911140614576, 30.00000000000323297 ) ) ;
#80684=ORIENTED_EDGE ( 'NONE', *, *, #28922, .T. ) ;
#80685=ORIENTED_EDGE ( 'NONE', *, *, #20280, .T. ) ;
#80687=CARTESIAN_POINT ( 'NONE',  ( -7.053767526187233905, -3.957541250942359756, 33.62499894934981626 ) ) ;
#80688=LINE ( 'NONE', #41018, #256 ) ;
#80690=CARTESIAN_POINT ( 'NONE',  ( -11.53846153846153655, -8.564572088678739092, 35.78748833219616898 ) ) ;
#80691=CARTESIAN_POINT ( 'NONE',  ( -13.38461538461550582, -2.892918686052166066, 31.69288490824153470 ) ) ;
#80693=CARTESIAN_POINT ( 'NONE',  ( -15.29603967673000398, -3.835265460703609186, 33.15142922261924241 ) ) ;
#80694=ORIENTED_EDGE ( 'NONE', *, *, #66179, .T. ) ;
#80695=EDGE_CURVE ( 'NONE', #34591, #43471, #62883, .T. ) ;
#80696=CARTESIAN_POINT ( 'NONE',  ( -5.933932666649924137, -8.164416787775445883, 34.95778746994558617 ) ) ;
#80697=CARTESIAN_POINT ( 'NONE',  ( 14.24242186173153435, -11.48612834413959582, 32.76840700105983473 ) ) ;
#80698=CARTESIAN_POINT ( 'NONE',  ( -14.55766903863466055, -8.303909089506435137, 34.68538101551103381 ) ) ;
#80700=EDGE_LOOP ( 'NONE', ( #60019, #81097, #77818, #21872 ) ) ;
#80701=B_SPLINE_CURVE_WITH_KNOTS ( 'NONE', 3,
 ( #82550, #14513, #40671, #48292, #68135, #83428, #20391, #55938, #69011, #69899 ),
 .UNSPECIFIED., .F., .F.,
 ( 4, 2, 2, 2, 4 ),
 ( 0.0007817359430256371616, 0.0009771253907250052138, 0.001172514838424373266, 0.001367904286123741318, 0.001563293733823109370 ),
 .UNSPECIFIED. ) ;
#80702=EDGE_CURVE ( 'NONE', #86919, #8179, #58991, .T. ) ;
#80703=EDGE_LOOP ( 'NONE', ( #67422, #68669, #59145, #66081 ) ) ;
#80706=CARTESIAN_POINT ( 'NONE',  ( 15.48071474911737333, -6.696923467548660192, 34.68552623307873972 ) ) ;
#80707=CARTESIAN_POINT ( 'NONE',  ( -7.780898274877819709, -5.219633306516380244, 34.19971097300157936 ) ) ;
#80708=VERTEX_POINT ( 'NONE', #79213 ) ;
#80709=DIRECTION ( 'NONE',  ( 0.000000000000000000, 0.7660444431189822323, -0.6427876096865344779 ) ) ;
#80710=DIRECTION ( 'NONE',  ( -0.000000000000000000, -0.5000000000000009992, -0.8660254037844380415 ) ) ;
#80711=CARTESIAN_POINT ( 'NONE',  ( 3.230769230769108269, -5.941354392335915335, 34.76329471203413846 ) ) ;
#80712=DIRECTION ( 'NONE',  ( -0.000000000000000000, -0.9396926207859092051, -0.3420201433256662704 ) ) ;
#80713=EDGE_CURVE ( 'NONE', #74576, #673, #60672, .T. ) ;
#80714=CARTESIAN_POINT ( 'NONE',  ( -11.53846153846153655, -8.973038597847269315, 34.52809138561121927 ) ) ;
#80715=ORIENTED_EDGE ( 'NONE', *, *, #88611, .F. ) ;
#80717=ORIENTED_EDGE ( 'NONE', *, *, #79066, .F. ) ;
#80720=CARTESIAN_POINT ( 'NONE',  ( -11.76138849736838488, -10.77366814457252175, 33.85459836347579454 ) ) ;
#80721=AXIS2_PLACEMENT_3D ( 'NONE', #27564, #41974, #76638 ) ;
#80722=CARTESIAN_POINT ( 'NONE',  ( 15.29602480204525605, -12.46129190930001052, 30.37095296980870174 ) ) ;
#80723=CARTESIAN_POINT ( 'NONE',  ( 15.23076923076910916, -2.379036618888197729, 30.90682066428292885 ) ) ;
#80724=DIRECTION ( 'NONE',  ( 0.000000000000000000, 0.9848077530122072432, 0.1736481776669354937 ) ) ;
#80725=AXIS2_PLACEMENT_3D ( 'NONE', #88612, #60660, #88170 ) ;
#80727=ORIENTED_EDGE ( 'NONE', *, *, #20923, .T. ) ;
#80728=CYLINDRICAL_SURFACE ( 'NONE', #31764, 0.2500000000000009437 ) ;
#80729=CARTESIAN_POINT ( 'NONE',  ( 7.623274329416259931, -7.630690623152301733, 34.99857592706772635 ) ) ;
#80731=ORIENTED_EDGE ( 'NONE', *, *, #23573, .F. ) ;
#80732=CARTESIAN_POINT ( 'NONE',  ( -8.835313148590904220, -5.471508081941602875, 34.59228464037088457 ) ) ;
#80733=DIRECTION ( 'NONE',  ( 0.000000000000000000, 0.6427876096865373645, -0.7660444431189797898 ) ) ;
#80734=EDGE_CURVE ( 'NONE', #67131, #1344, #39145, .T. ) ;
#80735=CARTESIAN_POINT ( 'NONE',  ( 13.13463865367303463, -3.627789207965226748, 32.91389620160131102 ) ) ;
#80736=CARTESIAN_POINT ( 'NONE',  ( -7.053224132515142131, -6.001485441113818986, 34.52039167877662607 ) ) ;
#80737=CARTESIAN_POINT ( 'NONE',  ( 6.923076923076802558, -3.300289026999228881, 32.46337939537708905 ) ) ;
#80738=DIRECTION ( 'NONE',  ( 0.000000000000000000, 0.9848077530122072432, -0.1736481776669354937 ) ) ;
#80739=ORIENTED_EDGE ( 'NONE', *, *, #65921, .F. ) ;
#80740=CARTESIAN_POINT ( 'NONE',  ( 9.692307692307572609, -10.90142922262034020, 33.41473453929536674 ) ) ;
#80741=B_SPLINE_CURVE_WITH_KNOTS ( 'NONE', 3,
 ( #87254, #45796, #73278, #25085, #19225, #88596, #25973, #12464, #32294, #39949 ),
 .UNSPECIFIED., .F., .F.,
 ( 4, 2, 2, 2, 4 ),
 ( 0.0007817246256747528103, 0.0009771112852218970073, 0.001172497944769041421, 0.001367884604316185835, 0.001563271263863330032 ),
 .UNSPECIFIED. ) ;
#80742=CARTESIAN_POINT ( 'NONE',  ( -14.30769230769230660, -2.721908614388771852, 31.22303859784724978 ) ) ;
#80743=CARTESIAN_POINT ( 'NONE',  ( -2.242437168179467033, -5.941354392334606160, 34.76329471203374055 ) ) ;
#80744=ORIENTED_EDGE ( 'NONE', *, *, #36085, .T. ) ;
#80745=CARTESIAN_POINT ( 'NONE',  ( -7.846153846153844924, -3.513871655860378418, 32.76840700105978499 ) ) ;
#80746=VECTOR ( 'NONE', #17664, 1000.000000000000000 ) ;
#80747=ORIENTED_EDGE ( 'NONE', *, *, #18060, .T. ) ;
#80748=CARTESIAN_POINT ( 'NONE',  ( 13.38461538461526601, -3.835265460704628371, 33.15142922262033665 ) ) ;
#80752=CARTESIAN_POINT ( 'NONE',  ( 13.51514082284903040, -9.503571793651731880, 34.60286762892837942 ) ) ;
#80753=CARTESIAN_POINT ( 'NONE',  ( 1.384615384615386802, -5.471508081941601098, 34.59228464037088457 ) ) ;
#80754=AXIS2_PLACEMENT_3D ( 'NONE', #29645, #35960, #57102 ) ;
#80755=LINE ( 'NONE', #10506, #620 ) ;
#80756=CARTESIAN_POINT ( 'NONE',  ( -4.853910232829680815, -8.282913670948747864, 34.94150082978203642 ) ) ;
#80757=VERTEX_POINT ( 'NONE', #47191 ) ;
#80759=ORIENTED_EDGE ( 'NONE', *, *, #74648, .F. ) ;
#80761=CARTESIAN_POINT ( 'NONE',  ( -10.36543920600657032, -10.18230066228895758, 34.26354781536631577 ) ) ;
#80763=CARTESIAN_POINT ( 'NONE',  ( -0.3307480205715097599, -2.494656445102013453, 31.33466734024120015 ) ) ;
#80764=CARTESIAN_POINT ( 'NONE',  ( 11.53846153846153832, -11.16473453929635440, 33.15142922261926373 ) ) ;
#80766=FACE_OUTER_BOUND ( 'NONE', #28250, .T. ) ;
#80767=CARTESIAN_POINT ( 'NONE',  ( -9.469294848214296678, -6.460100341425560444, 34.89618726649961644 ) ) ;
#80768=CARTESIAN_POINT ( 'NONE',  ( 7.596177102105256651, -2.544273027872575366, 31.48422191005632342 ) ) ;
#80769=B_SPLINE_CURVE_WITH_KNOTS ( 'NONE', 3,
 ( #50539, #71698, #31154, #72592, #79357, #37469, #23510, #3683, #78906, #17202 ),
 .UNSPECIFIED., .F., .F.,
 ( 4, 2, 2, 2, 4 ),
 ( 0.000000000000000000, 0.0001954339857564074473, 0.0003908679715128148945, 0.0005863019572692223418, 0.0007817359430256297891 ),
 .UNSPECIFIED. ) ;
#80771=ORIENTED_EDGE ( 'NONE', *, *, #40423, .F. ) ;
#80772=EDGE_CURVE ( 'NONE', #3349, #79887, #67036, .T. ) ;
#80773=B_SPLINE_CURVE_WITH_KNOTS ( 'NONE', 3,
 ( #27690, #55159, #68242, #81324, #7430, #34888, #47513, #75439, #6102, #82203 ),
 .UNSPECIFIED., .F., .F.,
 ( 4, 2, 2, 2, 4 ),
 ( 0.000000000000000000, 0.0001954311564186861426, 0.0003908623128373722852, 0.0005862934692560583735, 0.0007817246256747445703 ),
 .UNSPECIFIED. ) ;
#80774=VERTEX_POINT ( 'NONE', #53055 ) ;
#80775=AXIS2_PLACEMENT_3D ( 'NONE', #88882, #67705, #80794 ) ;
#80776=B_SPLINE_CURVE_WITH_KNOTS ( 'NONE', 3,
 ( #27453, #54920, #82405, #20688, #48152, #75623, #68870, #422, #1746, #41859 ),
 .UNSPECIFIED., .F., .F.,
 ( 4, 2, 2, 2, 4 ),
 ( 0.0007817359430256326080, 0.0009771253907249993591, 0.001172514838424366327, 0.001367904286123733078, 0.001563293733823099829 ),
 .UNSPECIFIED. ) ;
#80777=ORIENTED_EDGE ( 'NONE', *, *, #73546, .T. ) ;
#80778=CARTESIAN_POINT ( 'NONE',  ( -5.076923076923075762, -3.937682226553329556, 33.60647404775216529 ) ) ;
#80779=CARTESIAN_POINT ( 'NONE',  ( -1.161835843346975095, -12.44528174975671853, 30.48912976160716681 ) ) ;
#80780=AXIS2_PLACEMENT_3D ( 'NONE', #45025, #86946, #4950 ) ;
#80781=ADVANCED_FACE ( 'NONE', ( #5776 ), #6227, .F. ) ;
#80782=CARTESIAN_POINT ( 'NONE',  ( -15.23076923076922995, -10.51840700105979565, 33.73612834413961536 ) ) ;
#80783=CARTESIAN_POINT ( 'NONE',  ( 6.223011351612852238, -12.15243808032446005, 31.58219941686247978 ) ) ;
#80784=CARTESIAN_POINT ( 'NONE',  ( 11.40777007179397984, -2.541943142973491554, 30.39792223712631980 ) ) ;
#80785=CARTESIAN_POINT ( 'NONE',  ( -0.5916856709766776801, -11.93770438780619259, 32.05411857736982029 ) ) ;
#80786=DIRECTION ( 'NONE',  ( -0.000000000000000000, 0.9848077530122085754, -0.1736481776669273613 ) ) ;
#80787=CARTESIAN_POINT ( 'NONE',  ( 14.30769230769231015, -2.708943851104267164, 35.45975837776705220 ) ) ;
#80788=ORIENTED_EDGE ( 'NONE', *, *, #30162, .T. ) ;
#80789=ORIENTED_EDGE ( 'NONE', *, *, #85997, .T. ) ;
#80790=EDGE_LOOP ( 'NONE', ( #51366, #24660, #70360, #37315, #11991, #65476 ) ) ;
#80791=CARTESIAN_POINT ( 'NONE',  ( -1.384615384615383471, -11.16473453929635440, 33.15142922261926373 ) ) ;
#80792=ORIENTED_EDGE ( 'NONE', *, *, #22235, .T. ) ;
#80793=DIRECTION ( 'NONE',  ( -0.000000000000000000, -0.3420201433256694346, -0.9396926207859080948 ) ) ;
#80794=DIRECTION ( 'NONE',  ( 0.000000000000000000, 0.7660444431189807890, 0.6427876096865361433 ) ) ;
#80796=CARTESIAN_POINT ( 'NONE',  ( -9.019207513279361876, -6.524016743844655686, 34.90889640711025521 ) ) ;
#80797=FACE_BOUND ( 'NONE', #12079, .T. ) ;
#80798=ORIENTED_EDGE ( 'NONE', *, *, #52044, .T. ) ;
#80800=CARTESIAN_POINT ( 'NONE',  ( 18.00000000000000000, -13.88283147151868846, 33.14645433367849847 ) ) ;
#80801=ADVANCED_FACE ( 'NONE', ( #46759 ), #26937, .F. ) ;
#80802=ORIENTED_EDGE ( 'NONE', *, *, #11411, .F. ) ;
#80803=FACE_BOUND ( 'NONE', #39272, .T. ) ;
#80805=VECTOR ( 'NONE', #73603, 1000.000000000000114 ) ;
#80806=CARTESIAN_POINT ( 'NONE',  ( 15.00784227186237807, -6.459968553980841577, 34.89616026154728701 ) ) ;
#80807=VERTEX_POINT ( 'NONE', #74235 ) ;
#80808=CARTESIAN_POINT ( 'NONE',  ( 2.177545098254087375, -8.587444163452046197, 34.63053765926554206 ) ) ;
#80811=ORIENTED_EDGE ( 'NONE', *, *, #82859, .F. ) ;
#80813=CYLINDRICAL_SURFACE ( 'NONE', #86956, 0.2499999999999994726 ) ;
#80814=CARTESIAN_POINT ( 'NONE',  ( -7.976301055592065481, -2.882441371585227952, 31.66841991370172238 ) ) ;
#80816=VECTOR ( 'NONE', #55665, 1000.000000000000227 ) ;
#80817=ADVANCED_FACE ( 'NONE', ( #88660 ), #73800, .F. ) ;
#80818=CARTESIAN_POINT ( 'NONE',  ( -1.634638621908349521, -5.851115903089112003, 34.47074536777953568 ) ) ;
#80819=CARTESIAN_POINT ( 'NONE',  ( -15.48074596171158390, -4.236021600441997492, 33.53823185664189310 ) ) ;
#80820=ORIENTED_EDGE ( 'NONE', *, *, #42842, .F. ) ;
#80821=CARTESIAN_POINT ( 'NONE',  ( 3.296836564119306257, -6.343179335718452272, 34.87096338111212646 ) ) ;
#80822=DIRECTION ( 'NONE',  ( -0.000000000000000000, 0.9848077530122086864, -0.1736481776669273891 ) ) ;
#80823=CARTESIAN_POINT ( 'NONE',  ( 5.749976762707035505, -9.271318131107980420, 34.42618302367067429 ) ) ;
#80824=CARTESIAN_POINT ( 'NONE',  ( 13.60739492588379562, -12.44528174975671853, 30.48912976160716681 ) ) ;
#80825=CARTESIAN_POINT ( 'NONE',  ( -16.15384615384615330, -4.098570777380720287, 33.41473453929634729 ) ) ;
#80826=CARTESIAN_POINT ( 'NONE',  ( 6.923076923076924238, -8.973038597847269315, 34.52809138561121927 ) ) ;
#80827=CARTESIAN_POINT ( 'NONE',  ( 0.4615384615384611200, -11.35647404775217417, 33.31231777344666511 ) ) ;
#80828=CARTESIAN_POINT ( 'NONE',  ( 9.942362112221147186, -4.818054556918156983, 34.26375889529406749 ) ) ;
#80829=EDGE_CURVE ( 'NONE', #55479, #4302, #56368, .T. ) ;
#80830=EDGE_CURVE ( 'NONE', #85285, #27220, #74685, .T. ) ;
#80831=CARTESIAN_POINT ( 'NONE',  ( 8.769230769230647482, -12.27809138561165270, 31.22303859784587132 ) ) ;
#80832=CARTESIAN_POINT ( 'NONE',  ( -6.923076923077044142, -2.892918686052165622, 31.69288490824153470 ) ) ;
#80834=ORIENTED_EDGE ( 'NONE', *, *, #80583, .F. ) ;
#80835=CARTESIAN_POINT ( 'NONE',  ( 4.853438152358743984, -6.716662450894490100, 34.94144148231605840 ) ) ;
#80838=CARTESIAN_POINT ( 'NONE',  ( -2.242436736416281828, -12.46129190930001052, 30.37095296980870174 ) ) ;
#80839=EDGE_LOOP ( 'NONE', ( #9466, #51295, #18101, #69636 ) ) ;
#80840=CARTESIAN_POINT ( 'NONE',  ( 3.480714749117371998, -10.05730279482229683, 34.04704008940765902 ) ) ;
#80842=CARTESIAN_POINT ( 'NONE',  ( 3.230769230769231726, -2.292212530054420494, 30.41441678777542634 ) ) ;
#80843=EDGE_CURVE ( 'NONE', #80176, #36938, #21391, .T. ) ;
#80844=CARTESIAN_POINT ( 'NONE',  ( 10.68145194873469173, -2.486705287966280320, 31.30864560766543647 ) ) ;
#80845=DIRECTION ( 'NONE',  ( -0.000000000000000000, -0.000000000000000000, -1.000000000000000000 ) ) ;
#80846=CARTESIAN_POINT ( 'NONE',  ( -3.230769230769229949, -12.34228464037088635, 31.77849191805839268 ) ) ;
#80847=CARTESIAN_POINT ( 'NONE',  ( -13.38461538461538325, -2.538708090699994813, 30.37095296980875503 ) ) ;
#80848=CARTESIAN_POINT ( 'NONE',  ( -11.53846153846165912, -5.219633306517616589, 34.19971097300220464 ) ) ;
#80849=AXIS2_PLACEMENT_3D ( 'NONE', #22626, #50093, #15443 ) ;
#80851=EDGE_CURVE ( 'NONE', #14278, #48006, #69294, .T. ) ;
#80852=EDGE_CURVE ( 'NONE', #14768, #21373, #23598, .T. ) ;
#80853=CARTESIAN_POINT ( 'NONE',  ( -0.4615384615384611200, -2.538708090699994813, 30.37095296980875503 ) ) ;
#80854=CARTESIAN_POINT ( 'NONE',  ( -13.16160403300253634, -6.503523203565941380, 34.64991518177335195 ) ) ;
#80855=VECTOR ( 'NONE', #85372, 1000.000000000000000 ) ;
#80856=DIRECTION ( 'NONE',  ( 0.000000000000000000, 0.1736481776669275834, 0.9848077530122086864 ) ) ;
#80857=ADVANCED_FACE ( 'NONE', ( #50174 ), #44751, .F. ) ;
#80858=ORIENTED_EDGE ( 'NONE', *, *, #78427, .T. ) ;
#80860=DIRECTION ( 'NONE',  ( 0.000000000000000000, 0.6427876096865368094, 0.7660444431189802339 ) ) ;
#80861=CARTESIAN_POINT ( 'NONE',  ( -14.24162395668986747, -8.120952969808772792, 34.71129190929999453 ) ) ;
#80862=CARTESIAN_POINT ( 'NONE',  ( -39.05038313613820122, -2.249999999999999556, 27.25000000000000000 ) ) ;
#80864=DIRECTION ( 'NONE',  ( 0.000000000000000000, 1.000000000000000000, 0.000000000000000000 ) ) ;
#80865=CARTESIAN_POINT ( 'NONE',  ( -10.61538461538461320, -9.819645486525091727, 36.12317359536749706 ) ) ;
#80867=CARTESIAN_POINT ( 'NONE',  ( 3.100078627658924280, -6.369640206132550553, 34.87707690430378449 ) ) ;
#80868=ORIENTED_EDGE ( 'NONE', *, *, #16338, .T. ) ;
#80869=B_SPLINE_CURVE_WITH_KNOTS ( 'NONE', 3,
 ( #70673, #77425, #84642, #69783, #15734, #8091, #23356, #8533, #63898, #83311 ),
 .UNSPECIFIED., .F., .F.,
 ( 4, 2, 2, 2, 4 ),
 ( 0.0007817359430256288133, 0.0009771253907249945886, 0.001172514838424360255, 0.001367904286123725922, 0.001563293733823091589 ),
 .UNSPECIFIED. ) ;
#80870=ORIENTED_EDGE ( 'NONE', *, *, #88682, .T. ) ;
#80871=EDGE_CURVE ( 'NONE', #31146, #31749, #40267, .T. ) ;
#80872=CARTESIAN_POINT ( 'NONE',  ( -8.638440328263820689, -4.684288915650983043, 34.18129842949671371 ) ) ;
#80873=AXIS2_PLACEMENT_3D ( 'NONE', #15611, #42204, #21921 ) ;
#80874=CARTESIAN_POINT ( 'NONE',  ( 3.903822916553189248, -2.587272538249754117, 30.68239716806877837 ) ) ;
#80875=CARTESIAN_POINT ( 'NONE',  ( 9.692307692307695177, -12.10708131394839349, 31.69288490824020244 ) ) ;
#80876=CARTESIAN_POINT ( 'NONE',  ( 1.161130460051055691, -11.60425143139329940, 33.02411095842164457 ) ) ;
#80877=CARTESIAN_POINT ( 'NONE',  ( -13.63463860883684120, -2.588893531581426988, 31.60682220781847818 ) ) ;
#80878=AXIS2_PLACEMENT_3D ( 'NONE', #39430, #47935, #27227 ) ;
#80879=ORIENTED_EDGE ( 'NONE', *, *, #66787, .F. ) ;
#80880=EDGE_CURVE ( 'NONE', #33560, #86342, #16404, .T. ) ;
#80881=ORIENTED_EDGE ( 'NONE', *, *, #43858, .F. ) ;
#80882=ORIENTED_EDGE ( 'NONE', *, *, #55386, .F. ) ;
#80883=CARTESIAN_POINT ( 'NONE',  ( -4.153846153846152411, -2.486705287966279876, 31.30864560766543647 ) ) ;
#80884=DIRECTION ( 'NONE',  ( 0.000000000000000000, 0.000000000000000000, 1.000000000000000000 ) ) ;
#80886=CARTESIAN_POINT ( 'NONE',  ( 16.15384615384603251, -5.941354392335915335, 34.76329471203413846 ) ) ;
#80887=B_SPLINE_CURVE_WITH_KNOTS ( 'NONE', 3,
 ( #5380, #32403, #32847, #60311, #52214, #59869, #25646, #53101, #39623, #81046 ),
 .UNSPECIFIED., .F., .F.,
 ( 4, 2, 2, 2, 4 ),
 ( 0.0007817359527651104954, 0.0009771254036996493593, 0.001172514854634188223, 0.001367904305568727087, 0.001563293756503265951 ),
 .UNSPECIFIED. ) ;
#80888=CARTESIAN_POINT ( 'NONE',  ( -15.45425417449317784, -11.41268669641500466, 32.86336882939237825 ) ) ;
#80889=CARTESIAN_POINT ( 'NONE',  ( -15.90384615384473399, -7.500000000000154543, 35.00000000000007105 ) ) ;
#80890=DIRECTION ( 'NONE',  ( -0.000000000000000000, -0.1736481776669307198, -0.9848077530122080203 ) ) ;
#80891=EDGE_LOOP ( 'NONE', ( #84509, #35693, #88516, #34911 ) ) ;
#80892=ORIENTED_EDGE ( 'NONE', *, *, #40172, .F. ) ;
#80893=ADVANCED_FACE ( 'NONE', ( #17293 ), #85316, .F. ) ;
#80894=CARTESIAN_POINT ( 'NONE',  ( 17.20744877868663281, -12.45806712695776319, 30.39783852428763566 ) ) ;
#80895=ORIENTED_EDGE ( 'NONE', *, *, #25088, .F. ) ;
#80896=CARTESIAN_POINT ( 'NONE',  ( -9.942284423250047354, -4.943428324936578910, 34.04746400365624481 ) ) ;
#80897=CARTESIAN_POINT ( 'NONE',  ( 7.911347827937202482, -2.506253911140448487, 29.99999999999988631 ) ) ;
#80898=AXIS2_PLACEMENT_3D ( 'NONE', #81581, #13117, #47333 ) ;
#80902=CARTESIAN_POINT ( 'NONE',  ( -1.134669975237340811, -11.56426240980093567, 33.07394671870546432 ) ) ;
#80903=ORIENTED_EDGE ( 'NONE', *, *, #16386, .F. ) ;
#80904=FACE_OUTER_BOUND ( 'NONE', #6493, .T. ) ;
#80905=DIRECTION ( 'NONE',  ( -0.000000000000000000, 1.000000000000000000, 3.491481338843133355E-15 ) ) ;
#80906=FACE_BOUND ( 'NONE', #83487, .T. ) ;
#80907=CARTESIAN_POINT ( 'NONE',  ( 12.46153846153846168, -13.37000171582298513, 34.34916445242398453 ) ) ;
#80908=CARTESIAN_POINT ( 'NONE',  ( -14.17764714485753075, -2.504778602574660340, 29.97347330155780654 ) ) ;
#80909=EDGE_LOOP ( 'NONE', ( #54805, #41981, #28026, #47215 ) ) ;
#80910=EDGE_CURVE ( 'NONE', #37595, #58918, #2584, .T. ) ;
#80911=CARTESIAN_POINT ( 'NONE',  ( 11.47237915910140416, -11.35647404775217595, 33.31231777344666511 ) ) ;
#80914=DIRECTION ( 'NONE',  ( 0.000000000000000000, -6.938893903907222067E-15, 1.000000000000000000 ) ) ;
#80915=ORIENTED_EDGE ( 'NONE', *, *, #77035, .F. ) ;
#80916=LINE ( 'NONE', #74143, #11374 ) ;
#80917=CARTESIAN_POINT ( 'NONE',  ( 14.53070515178570332, -10.01129605718032600, 34.36064277460058491 ) ) ;
#80918=CARTESIAN_POINT ( 'NONE',  ( 17.20771488474786537, -9.804649428959608670, 34.18742332936588468 ) ) ;
#80920=CARTESIAN_POINT ( 'NONE',  ( 10.39245839786846659, -11.76352882383564769, 32.36236540154569497 ) ) ;
#80921=FACE_BOUND ( 'NONE', #23581, .T. ) ;
#80922=CARTESIAN_POINT ( 'NONE',  ( 13.31934538405906743, -12.16647553114622049, 32.15551576947930812 ) ) ;
#80923=CYLINDRICAL_SURFACE ( 'NONE', #22990, 0.2500000000000008882 ) ;
#80924=EDGE_CURVE ( 'NONE', #73759, #85253, #47744, .T. ) ;
#80925=CYLINDRICAL_SURFACE ( 'NONE', #41104, 0.2500000000000004996 ) ;
#80926=CYLINDRICAL_SURFACE ( 'NONE', #15612, 0.2499999999999995559 ) ;
#80927=CARTESIAN_POINT ( 'NONE',  ( 15.48082354240754555, -9.943054286541403997, 34.11300777759954883 ) ) ;
#80928=CARTESIAN_POINT ( 'NONE',  ( -4.153846153846152411, -9.819645486525091727, 36.12317359536749706 ) ) ;
#80930=ORIENTED_EDGE ( 'NONE', *, *, #77344, .T. ) ;
#80931=DIRECTION ( 'NONE',  ( -0.000000000000000000, 0.9396926207859092051, -0.3420201433256662704 ) ) ;
#80933=AXIS2_PLACEMENT_3D ( 'NONE', #46411, #59479, #31106 ) ;
#80934=CARTESIAN_POINT ( 'NONE',  ( -14.30769230769230660, -10.67929555188718282, 33.92786785259544047 ) ) ;
#80936=CARTESIAN_POINT ( 'NONE',  ( 7.596130608860880429, -9.271318131107980420, 34.42618302367067429 ) ) ;
#80937=CARTESIAN_POINT ( 'NONE',  ( -11.53846153846153655, -1.215029322943914858, 32.30358669280327177 ) ) ;
#80939=EDGE_LOOP ( 'NONE', ( #29393, #49144, #53032, #52829 ) ) ;
#80940=CARTESIAN_POINT ( 'NONE',  ( 3.361561038594018225, -6.413143153341454017, 34.63066358083362672 ) ) ;
#80941=CARTESIAN_POINT ( 'NONE',  ( 1.161130460051058133, -12.11044203135681840, 32.26167407432752299 ) ) ;
#80943=CARTESIAN_POINT ( 'NONE',  ( 2.084207363968360038, -11.89387501736622710, 32.13663884655806413 ) ) ;
#80944=CARTESIAN_POINT ( 'NONE',  ( 5.076923076923075762, -4.786620604624113540, 33.94971097300155094 ) ) ;
#80945=CARTESIAN_POINT ( 'NONE',  ( -5.011667937410240192, -12.16647553114626490, 32.15551576947920864 ) ) ;
#80948=CARTESIAN_POINT ( 'NONE',  ( -8.835314180186646382, -8.973038597847271092, 34.52809138561120506 ) ) ;
#80949=B_SPLINE_CURVE_WITH_KNOTS ( 'NONE', 3,
 ( #50812, #37306, #43628, #65225, #37758, #85075, #77422, #16596, #85954, #44056 ),
 .UNSPECIFIED., .F., .F.,
 ( 4, 2, 2, 2, 4 ),
 ( 0.0007817359430256324996, 0.0009771253907249993591, 0.001172514838424366110, 0.001367904286123732861, 0.001563293733823099829 ),
 .UNSPECIFIED. ) ;
#80951=EDGE_CURVE ( 'NONE', #64799, #33151, #24040, .T. ) ;
#80952=CARTESIAN_POINT ( 'NONE',  ( 5.299702745901138989, -2.612705202774697533, 31.66806509827799943 ) ) ;
#80953=CARTESIAN_POINT ( 'NONE',  ( -1.384615384615383471, -11.91647553114624181, 32.58852847137148245 ) ) ;
#80954=EDGE_LOOP ( 'NONE', ( #46926, #38498, #26030, #19120 ) ) ;
#80955=CARTESIAN_POINT ( 'NONE',  ( 17.29970261819148902, -2.847695495035524882, 31.58253572463339154 ) ) ;
#80956=CARTESIAN_POINT ( 'NONE',  ( 9.692307692307695177, -5.471508081941601098, 34.59228464037088457 ) ) ;
#80958=CARTESIAN_POINT ( 'NONE',  ( 2.242421861731532573, -4.481592998940161721, 33.73612834413957984 ) ) ;
#80959=DIRECTION ( 'NONE',  ( 0.000000000000000000, 0.8660254037844377084, -0.5000000000000015543 ) ) ;
#80960=VERTEX_POINT ( 'NONE', #64132 ) ;
#80961=DIRECTION ( 'NONE',  ( -0.000000000000000000, -0.8660254037844397068, -0.4999999999999978906 ) ) ;
#80962=CARTESIAN_POINT ( 'NONE',  ( -12.23852561744506851, -12.64618726649961289, 30.78989965857442712 ) ) ;
#80963=CARTESIAN_POINT ( 'NONE',  ( 11.53846153846141576, -3.083524468854526912, 32.58852847137268327 ) ) ;
#80964=ORIENTED_EDGE ( 'NONE', *, *, #45093, .F. ) ;
#80965=CARTESIAN_POINT ( 'NONE',  ( -8.069080063669991532, -8.239355502252617924, 34.69524867566427417 ) ) ;
#80966=CARTESIAN_POINT ( 'NONE',  ( 3.903869422903798458, -8.303909089506435137, 34.68538101551103381 ) ) ;
#80967=CARTESIAN_POINT ( 'NONE',  ( 15.45378207486262667, -5.582272713120729257, 34.63742843783360570 ) ) ;
#80968=CARTESIAN_POINT ( 'NONE',  ( -14.30769230769230660, -11.16473453929635440, 33.15142922261926373 ) ) ;
#80969=VERTEX_POINT ( 'NONE', #84436 ) ;
#80970=AXIS2_PLACEMENT_3D ( 'NONE', #38149, #30503, #50320 ) ;
#80971=CARTESIAN_POINT ( 'NONE',  ( 2.530471848960718084, -12.24180327182771855, 31.33663988360758168 ) ) ;
#80972=DIRECTION ( 'NONE',  ( -0.000000000000000000, -0.000000000000000000, -1.000000000000000000 ) ) ;
#80973=CARTESIAN_POINT ( 'NONE',  ( 1.384615384615264011, -3.083524468854526912, 32.58852847137268327 ) ) ;
#80974=ORIENTED_EDGE ( 'NONE', *, *, #75668, .F. ) ;
#80975=ORIENTED_EDGE ( 'NONE', *, *, #64696, .T. ) ;
#80976=EDGE_LOOP ( 'NONE', ( #3705, #14100 ) ) ;
#80977=DIRECTION ( 'NONE',  ( -0.000000000000000000, -0.1736481776669307198, -0.9848077530122080203 ) ) ;
#80978=CARTESIAN_POINT ( 'NONE',  ( -2.307692307692305711, -8.564572088678739092, 35.78748833219616898 ) ) ;
#80979=CARTESIAN_POINT ( 'NONE',  ( -9.692307692307691624, -12.62096338111211580, 30.90682066428153263 ) ) ;
#80980=CARTESIAN_POINT ( 'NONE',  ( 5.076923076922954969, -6.026961402154118908, 34.52809138561165270 ) ) ;
#80981=VERTEX_POINT ( 'NONE', #22712 ) ;
#80982=VERTEX_POINT ( 'NONE', #64570 ) ;
#80983=VERTEX_POINT ( 'NONE', #29927 ) ;
#80984=CARTESIAN_POINT ( 'NONE',  ( -6.923076923077045919, -2.657715359629662988, 31.77849191805970364 ) ) ;
#80985=ORIENTED_EDGE ( 'NONE', *, *, #35473, .F. ) ;
#80987=FACE_OUTER_BOUND ( 'NONE', #86013, .T. ) ;
#80988=AXIS2_PLACEMENT_3D ( 'NONE', #50265, #48505, #7978 ) ;
#80990=CARTESIAN_POINT ( 'NONE',  ( 6.923076923076802558, -11.94971097300221174, 32.03036669348237098 ) ) ;
#80991=VERTEX_POINT ( 'NONE', #44293 ) ;
#80992=VECTOR ( 'NONE', #43950, 1000.000000000000114 ) ;
#80993=ORIENTED_EDGE ( 'NONE', *, *, #16349, .F. ) ;
#80994=ORIENTED_EDGE ( 'NONE', *, *, #45920, .F. ) ;
#80995=CARTESIAN_POINT ( 'NONE',  ( 14.37294744720514750, -11.06231777344671130, 33.60647404775212976 ) ) ;
#80996=CARTESIAN_POINT ( 'NONE',  ( -10.54931728203453822, -2.486705287966280320, 31.30864560766543647 ) ) ;
#80999=CARTESIAN_POINT ( 'NONE',  ( 12.39545505058258179, -11.16473453929635440, 33.15142922261925662 ) ) ;
#81000=ORIENTED_EDGE ( 'NONE', *, *, #60659, .T. ) ;
#81001=DIRECTION ( 'NONE',  ( -0.000000000000000000, 0.7660444431189791237, -0.6427876096865379196 ) ) ;
#81002=CARTESIAN_POINT ( 'NONE',  ( -18.00000000000012079, -2.625532179533778709, 30.86335684631627174 ) ) ;
#81004=FACE_BOUND ( 'NONE', #12264, .T. ) ;
#81005=CARTESIAN_POINT ( 'NONE',  ( -17.93393164899756087, -8.120952969808772792, 34.71129190929999453 ) ) ;
#81006=CARTESIAN_POINT ( 'NONE',  ( -1.161835843346972874, -11.89424750095246175, 32.13594075562311758 ) ) ;
#81007=EDGE_CURVE ( 'NONE', #67341, #74655, #64964, .T. ) ;
#81008=CARTESIAN_POINT ( 'NONE',  ( -10.39237177129122003, -10.77377354290276124, 33.85451476688484718 ) ) ;
#81009=DIRECTION ( 'NONE',  ( 0.000000000000000000, 0.000000000000000000, -1.000000000000000000 ) ) ;
#81010=CARTESIAN_POINT ( 'NONE',  ( -5.207070286361298095, -3.285722584762969856, 32.44110544564090759 ) ) ;
#81012=CARTESIAN_POINT ( 'NONE',  ( 17.99999999999987566, -6.835583212225970762, 34.95778746994575670 ) ) ;
#81013=VERTEX_POINT ( 'NONE', #32149 ) ;
#81015=EDGE_CURVE ( 'NONE', #24114, #51057, #38458, .T. ) ;
#81016=CYLINDRICAL_SURFACE ( 'NONE', #33592, 0.2499999999999994726 ) ;
#81018=ORIENTED_EDGE ( 'NONE', *, *, #21597, .F. ) ;
#81021=AXIS2_PLACEMENT_3D ( 'NONE', #83638, #75973, #15166 ) ;
#81022=CARTESIAN_POINT ( 'NONE',  ( -13.45069776397551564, -4.661471528628507777, 34.16647553114621871 ) ) ;
#81023=LINE ( 'NONE', #87796, #67749 ) ;
#81025=CARTESIAN_POINT ( 'NONE',  ( 14.55774661933062575, -9.148310452688876993, 34.47095581063188519 ) ) ;
#81026=DIRECTION ( 'NONE',  ( -0.000000000000000000, 1.000000000000000000, 3.491481338843133355E-15 ) ) ;
#81027=FACE_BOUND ( 'NONE', #65893, .T. ) ;
#81028=LINE ( 'NONE', #19317, #82081 ) ;
#81029=CARTESIAN_POINT ( 'NONE',  ( 5.869309396889695662, -6.369640206132550553, 34.87707690430378449 ) ) ;
#81030=DIRECTION ( 'NONE',  ( -0.000000000000000000, 0.6427876096865404731, -0.7660444431189771253 ) ) ;
#81032=FACE_OUTER_BOUND ( 'NONE', #84882, .T. ) ;
#81033=( LENGTH_UNIT ( ) NAMED_UNIT ( * ) SI_UNIT ( .MILLI., .METRE. ) );
#81034=CARTESIAN_POINT ( 'NONE',  ( 0.3962680155776852620, -6.026961402152685388, 34.52809138561120506 ) ) ;
#81036=ORIENTED_EDGE ( 'NONE', *, *, #74850, .F. ) ;
#81038=CARTESIAN_POINT ( 'NONE',  ( -12.23852561744506495, -5.582272713120729257, 34.63742843783360570 ) ) ;
#81039=FACE_OUTER_BOUND ( 'NONE', #82672, .T. ) ;
#81040=CARTESIAN_POINT ( 'NONE',  ( 4.283891316680932704, -2.504778602574660340, 29.97347330155780298 ) ) ;
#81041=CARTESIAN_POINT ( 'NONE',  ( 6.673053685783957967, -12.22074536777954989, 31.39888409691088356 ) ) ;
#81042=CARTESIAN_POINT ( 'NONE',  ( 5.326977496836529546, -3.435999193479609914, 33.07426656108010832 ) ) ;
#81044=CARTESIAN_POINT ( 'NONE',  ( 0.7115384615398965273, -7.500000000000155431, 34.75000000000007105 ) ) ;
#81045=CARTESIAN_POINT ( 'NONE',  ( 16.15384615384615330, -1.129524287112498415, 32.06866353760679544 ) ) ;
#81046=CARTESIAN_POINT ( 'NONE',  ( -13.63461538461538325, -7.500000000000001776, 34.75000000000000000 ) ) ;
#81047=DIRECTION ( 'NONE',  ( -0.000000000000000000, -0.3420201433256694346, -0.9396926207859080948 ) ) ;
#81048=CARTESIAN_POINT ( 'NONE',  ( 9.692307692307572609, -2.892918686052165622, 31.69288490824153470 ) ) ;
#81049=CARTESIAN_POINT ( 'NONE',  ( 8.519254038288416098, -12.17611988154120972, 31.52148481390971213 ) ) ;
#81051=CARTESIAN_POINT ( 'NONE',  ( -3.230769230769351186, -11.94971097300221174, 32.03036669348237098 ) ) ;
#81052=EDGE_CURVE ( 'NONE', #47795, #11542, #17747, .T. ) ;
#81054=CARTESIAN_POINT ( 'NONE',  ( -8.519285359852727169, -11.56426240980093745, 33.07394671870546432 ) ) ;
#81055=CARTESIAN_POINT ( 'NONE',  ( -15.48074596171158390, -8.303909089506435137, 34.68538101551103381 ) ) ;
#81057=ORIENTED_EDGE ( 'NONE', *, *, #16207, .T. ) ;
#81058=CARTESIAN_POINT ( 'NONE',  ( -0.4615384615384611200, -2.721908614388771852, 31.22303859784724978 ) ) ;
#81059=CARTESIAN_POINT ( 'NONE',  ( 18.25005441991345734, -4.818054556918155207, 34.26375889529406749 ) ) ;
#81061=EDGE_CURVE ( 'NONE', #66904, #18025, #43435, .T. ) ;
#81062=AXIS2_PLACEMENT_3D ( 'NONE', #36632, #64085, #64969 ) ;
#81063=ADVANCED_FACE ( 'NONE', ( #25834 ), #11428, .F. ) ;
#81064=CARTESIAN_POINT ( 'NONE',  ( 14.30769230769231015, -6.343179335718451384, 34.87096338111211935 ) ) ;
#81065=DIRECTION ( 'NONE',  ( 0.000000000000000000, 0.3420201433256641055, -0.9396926207859100932 ) ) ;
#81066=CARTESIAN_POINT ( 'NONE',  ( -10.61538461538461320, -3.886160181151819604, 36.00935417666054406 ) ) ;
#81067=CARTESIAN_POINT ( 'NONE',  ( 10.54963118707128622, -7.249945578846651806, 34.99404164642496795 ) ) ;
#81068=ORIENTED_EDGE ( 'NONE', *, *, #6347, .F. ) ;
#81070=CARTESIAN_POINT ( 'NONE',  ( 3.480714640147273720, -8.476813868363244353, 34.90874843262270133 ) ) ;
#81071=ORIENTED_EDGE ( 'NONE', *, *, #53635, .F. ) ;
#81072=CARTESIAN_POINT ( 'NONE',  ( 1.384615384615386802, -13.75783147151868846, 33.36296068462461051 ) ) ;
#81073=CARTESIAN_POINT ( 'NONE',  ( 18.25005431163831204, -9.148310452688871663, 34.47095581063188519 ) ) ;
#81074=ORIENTED_EDGE ( 'NONE', *, *, #4166, .T. ) ;
#81075=B_SPLINE_CURVE_WITH_KNOTS ( 'NONE', 3,
 ( #32203, #67757, #74513, #87604, #52894, #25882, #73642, #6060, #33080, #80394 ),
 .UNSPECIFIED., .F., .F.,
 ( 4, 2, 2, 2, 4 ),
 ( 0.0007817359430256293554, 0.0009771253907249952391, 0.001172514838424361123, 0.001367904286123727007, 0.001563293733823092890 ),
 .UNSPECIFIED. ) ;
#81077=CARTESIAN_POINT ( 'NONE',  ( -13.38461538461550582, -2.625532179533778709, 30.86335684631627174 ) ) ;
#81078=B_SPLINE_CURVE_WITH_KNOTS ( 'NONE', 3,
 ( #63216, #84398, #83961, #22239, #10046, #23124, #63663, #57792, #43833, #9605 ),
 .UNSPECIFIED., .F., .F.,
 ( 4, 2, 2, 2, 4 ),
 ( 0.0007817359430256216575, 0.0009771253907249856981, 0.001172514838424349630, 0.001367904286123713779, 0.001563293733823077711 ),
 .UNSPECIFIED. ) ;
#81079=CARTESIAN_POINT ( 'NONE',  ( -17.07692307692319744, -12.27809138561165270, 31.22303859784587132 ) ) ;
#81080=ORIENTED_EDGE ( 'NONE', *, *, #82259, .F. ) ;
#81081=ORIENTED_EDGE ( 'NONE', *, *, #2083, .T. ) ;
#81082=ORIENTED_EDGE ( 'NONE', *, *, #19101, .T. ) ;
#81084=CARTESIAN_POINT ( 'NONE',  ( 12.21151522424549896, -12.43535235679832596, 30.55408501211184813 ) ) ;
#81085=CARTESIAN_POINT ( 'NONE',  ( -9.561781990544133691, -10.19071101563364756, 33.96452234770658407 ) ) ;
#81086=CARTESIAN_POINT ( 'NONE',  ( -17.20761454359064047, -5.582088688514999397, 34.36776431015576350 ) ) ;
#81087=CARTESIAN_POINT ( 'NONE',  ( 9.469381474791543241, -9.086856451489515152, 34.49173150075333183 ) ) ;
#81088=DIRECTION ( 'NONE',  ( 0.000000000000000000, 0.9396926207859126468, 0.3420201433256571111 ) ) ;
#81089=DIRECTION ( 'NONE',  ( -0.000000000000000000, -0.1736481776669307198, -0.9848077530122080203 ) ) ;
#81091=CARTESIAN_POINT ( 'NONE',  ( -6.249999999999997335, -7.500000000000001776, 35.04278698407183867 ) ) ;
#81092=EDGE_CURVE ( 'NONE', #20954, #11611, #10542, .T. ) ;
#81093=ORIENTED_EDGE ( 'NONE', *, *, #69069, .T. ) ;
#81094=ORIENTED_EDGE ( 'NONE', *, *, #21251, .F. ) ;
#81095=EDGE_LOOP ( 'NONE', ( #57024, #87792 ) ) ;
#81096=CARTESIAN_POINT ( 'NONE',  ( 18.24994540937804643, -9.357781135181033605, 34.66075350412533851 ) ) ;
#81097=ORIENTED_EDGE ( 'NONE', *, *, #15057, .T. ) ;
#81098=CARTESIAN_POINT ( 'NONE',  ( -8.519176349317316266, -10.82426656108012075, 33.81400080652039009 ) ) ;
#81099=CARTESIAN_POINT ( 'NONE',  ( -39.05038313613820122, -2.249999999999999556, 27.25000000000000000 ) ) ;
#81100=ORIENTED_EDGE ( 'NONE', *, *, #39369, .F. ) ;
#81101=CARTESIAN_POINT ( 'NONE',  ( 15.45354889974729318, -9.418065098278013636, 34.63729479722530158 ) ) ;
#81102=EDGE_CURVE ( 'NONE', #62076, #15626, #34820, .T. ) ;
#81103=EDGE_LOOP ( 'NONE', ( #51908, #87019 ) ) ;
#81104=DIRECTION ( 'NONE',  ( -0.000000000000000000, -0.3420201433256694901, -0.9396926207859082059 ) ) ;
#81106=B_SPLINE_CURVE_WITH_KNOTS ( 'NONE', 3,
 ( #69993, #22258, #8307, #84859, #50606, #2414, #77640, #35783, #8755, #15506 ),
 .UNSPECIFIED., .F., .F.,
 ( 4, 2, 2, 2, 4 ),
 ( 0.0007817246256747476061, 0.0009771112852218902852, 0.001172497944769033181, 0.001367884604316175860, 0.001563271263863318539 ),
 .UNSPECIFIED. ) ;
#81107=CARTESIAN_POINT ( 'NONE',  ( 6.923076923076924238, -4.102666532097928531, 36.13435417666054406 ) ) ;
#81108=VECTOR ( 'NONE', #10529, 1000.000000000000227 ) ;
#81109=CARTESIAN_POINT ( 'NONE',  ( -16.28453762051371356, -6.413092428213692742, 34.63065189839063152 ) ) ;
#81110=CARTESIAN_POINT ( 'NONE',  ( -9.442307692307627676, -7.434744860731433924, 35.00000000000000711 ) ) ;
#81111=FACE_BOUND ( 'NONE', #88191, .T. ) ;
#81112=VECTOR ( 'NONE', #73549, 1000.000000000000227 ) ;
#81114=CARTESIAN_POINT ( 'NONE',  ( 1.134615384615387246, -7.433932668274255029, 35.00000000000000711 ) ) ;
#81115=EDGE_CURVE ( 'NONE', #65326, #31209, #28451, .T. ) ;
#81116=DIRECTION ( 'NONE',  ( 0.000000000000000000, 0.4999999999999960032, -0.8660254037844410391 ) ) ;
#81117=CARTESIAN_POINT ( 'NONE',  ( 4.284637961670941131, -8.147973898785416225, 34.70805048591653730 ) ) ;
#81118=CYLINDRICAL_SURFACE ( 'NONE', #20719, 0.2499999999999973355 ) ;
#81119=CARTESIAN_POINT ( 'NONE',  ( -12.46153846153846168, -5.557115091759785130, 34.35708131394839171 ) ) ;
#81120=CARTESIAN_POINT ( 'NONE',  ( -11.53846153846153655, -3.322132147404559976, 32.92929555188717927 ) ) ;
#81121=EDGE_CURVE ( 'NONE', #8179, #61168, #60404, .T. ) ;
#81122=ORIENTED_EDGE ( 'NONE', *, *, #46203, .F. ) ;
#81123=ORIENTED_EDGE ( 'NONE', *, *, #61704, .F. ) ;
#81124=DIRECTION ( 'NONE',  ( 0.000000000000000000, 0.8660254037844377084, 0.5000000000000015543 ) ) ;
#81125=CYLINDRICAL_SURFACE ( 'NONE', #18915, 0.2499999999999995837 ) ;
#81126=CARTESIAN_POINT ( 'NONE',  ( 15.45354889974729318, -8.540255544307065350, 34.89611431652622286 ) ) ;
#81127=CARTESIAN_POINT ( 'NONE',  ( 8.769230769230768274, -8.973038597847269315, 34.52809138561121927 ) ) ;
#81128=CARTESIAN_POINT ( 'NONE',  ( 8.703907853738597211, -7.749976743299138882, 34.99404534957040624 ) ) ;
#81129=CARTESIAN_POINT ( 'NONE',  ( -2.307692307692305711, -2.721908614388771852, 31.22303859784724978 ) ) ;
#81130=ORIENTED_EDGE ( 'NONE', *, *, #65431, .T. ) ;
#81131=LINE ( 'NONE', #60843, #64422 ) ;
#81132=CARTESIAN_POINT ( 'NONE',  ( 11.66850914471722689, -7.723484964179501588, 34.74522123443823318 ) ) ;
#81133=CARTESIAN_POINT ( 'NONE',  ( -14.05763788777885637, -12.41089969410671223, 31.60739465890703670 ) ) ;
#81134=ADVANCED_FACE ( 'NONE', ( #74024 ), #12319, .F. ) ;
#81135=CARTESIAN_POINT ( 'NONE',  ( -3.454254155333562171, -12.69144148231606017, 30.53333754910549303 ) ) ;
#81136=ORIENTED_EDGE ( 'NONE', *, *, #69196, .F. ) ;
#81137=VERTEX_POINT ( 'NONE', #35238 ) ;
#81138=SHAPE_DEFINITION_REPRESENTATION ( #26805, #36256 ) ;
#81139=EDGE_LOOP ( 'NONE', ( #17942, #65713, #62819, #38258 ) ) ;
#81140=EDGE_CURVE ( 'NONE', #57134, #572, #55068, .T. ) ;
#81141=CARTESIAN_POINT ( 'NONE',  ( 15.36156103859402222, -6.413143153341454017, 34.63066358083362672 ) ) ;
#81142=CARTESIAN_POINT ( 'NONE',  ( -14.30769230769230660, -5.471508081941601098, 34.59228464037088457 ) ) ;
#81144=EDGE_CURVE ( 'NONE', #58206, #37680, #35954, .T. ) ;
#81146=CARTESIAN_POINT ( 'NONE',  ( 14.98079249982687777, -9.148715823498378086, 34.47080413974185120 ) ) ;
#81147=CARTESIAN_POINT ( 'NONE',  ( -10.61538461538461320, -9.819645486525091727, 36.12317359536749706 ) ) ;
#81149=CARTESIAN_POINT ( 'NONE',  ( -0.5922299282060190517, -11.18331474514187995, 33.13161551792790505 ) ) ;
#81152=CARTESIAN_POINT ( 'NONE',  ( -15.16470189741915320, -2.292212530054420494, 30.41441678777542990 ) ) ;
#81153=ORIENTED_EDGE ( 'NONE', *, *, #46220, .F. ) ;
#81155=CARTESIAN_POINT ( 'NONE',  ( -2.557669038634660108, -9.148715823498378086, 34.47080413974185120 ) ) ;
#81156=CARTESIAN_POINT ( 'NONE',  ( 1.634615384616822320, -7.500000000000155431, 34.75000000000007105 ) ) ;
#81157=DIRECTION ( 'NONE',  ( -0.000000000000000000, -0.8660254037844397068, -0.4999999999999980016 ) ) ;
#81158=CARTESIAN_POINT ( 'NONE',  ( -8.703975629717930929, -8.656820664281605460, 34.87096338111211224 ) ) ;
#81159=EDGE_CURVE ( 'NONE', #59485, #15487, #24454, .T. ) ;
#81161=CARTESIAN_POINT ( 'NONE',  ( 12.59206416330202316, -11.46989282347013095, 32.79007818306219946 ) ) ;
#81163=EDGE_LOOP ( 'NONE', ( #48696, #64569, #17197, #74637 ) ) ;
#81164=LINE ( 'NONE', #81603, #28801 ) ;
#81165=CARTESIAN_POINT ( 'NONE',  ( -10.61538461538461320, -13.75783147151868846, 33.36296068462461051 ) ) ;
#81166=EDGE_CURVE ( 'NONE', #78029, #47861, #46628, .T. ) ;
#81167=VERTEX_POINT ( 'NONE', #88441 ) ;
#81168=ADVANCED_FACE ( 'NONE', ( #47415 ), #26713, .F. ) ;
#81169=ORIENTED_EDGE ( 'NONE', *, *, #241, .T. ) ;
#81170=CARTESIAN_POINT ( 'NONE',  ( 2.057692307692309264, -7.433932668274255029, 35.00000000000000711 ) ) ;
#81171=CARTESIAN_POINT ( 'NONE',  ( 2.980769230769232170, -2.499999999999998668, 29.75000000000000355 ) ) ;
#81172=CARTESIAN_POINT ( 'NONE',  ( -6.989160334032800570, -5.557115091759785130, 34.35708131394839171 ) ) ;
#81173=DIRECTION ( 'NONE',  ( -0.000000000000000000, 0.8660254037844399289, -0.4999999999999980016 ) ) ;
#81174=CARTESIAN_POINT ( 'NONE',  ( 0.7114838709165044461, -2.341251567377310217, 30.72681386836322659 ) ) ;
#81175=EDGE_LOOP ( 'NONE', ( #56243, #58266 ) ) ;
#81177=AXIS2_PLACEMENT_3D ( 'NONE', #68576, #12311, #27148 ) ;
#81178=CARTESIAN_POINT ( 'NONE',  ( 17.14217864819909920, -6.026961402152790193, 34.52809138561124769 ) ) ;
#81179=CARTESIAN_POINT ( 'NONE',  ( -2.057637887778852814, -5.642605341092957083, 34.66089969410670335 ) ) ;
#81180=ORIENTED_EDGE ( 'NONE', *, *, #48318, .T. ) ;
#81181=CARTESIAN_POINT ( 'NONE',  ( -16.85414340794500276, -12.11081565061823717, 32.26097654155341843 ) ) ;
#81182=AXIS2_PLACEMENT_3D ( 'NONE', #23848, #65731, #78807 ) ;
#81183=ORIENTED_EDGE ( 'NONE', *, *, #21011, .F. ) ;
#81184=DIRECTION ( 'NONE',  ( 0.000000000000000000, 0.9848077530122072432, -0.1736481776669354937 ) ) ;
#81185=DIRECTION ( 'NONE',  ( 0.000000000000000000, 0.000000000000000000, 1.000000000000000000 ) ) ;
#81186=EDGE_CURVE ( 'NONE', #12296, #33660, #47482, .T. ) ;
#81187=ORIENTED_EDGE ( 'NONE', *, *, #11590, .F. ) ;
#81188=CARTESIAN_POINT ( 'NONE',  ( -5.076923076923075762, -10.05456864172156806, 36.03766855953608683 ) ) ;
#81189=CARTESIAN_POINT ( 'NONE',  ( -11.31568199719312773, -12.44528174975671853, 30.48912976160716681 ) ) ;
#81191=CARTESIAN_POINT ( 'NONE',  ( 11.40831356872984514, -12.50552854090298638, 31.33409797877408920 ) ) ;
#81192=CARTESIAN_POINT ( 'NONE',  ( -1.384615384615383471, -10.67929555188718282, 33.92786785259544047 ) ) ;
#81193=EDGE_CURVE ( 'NONE', #80774, #58760, #27155, .T. ) ;
#81195=FACE_BOUND ( 'NONE', #68171, .T. ) ;
#81196=VERTEX_POINT ( 'NONE', #68147 ) ;
#81197=CARTESIAN_POINT ( 'NONE',  ( -5.999999999999998224, -2.538708090699994813, 30.37095296980875503 ) ) ;
#81199=CARTESIAN_POINT ( 'NONE',  ( -15.23076923076922995, -1.790695186598648903, 34.54067556320373455 ) ) ;
#81200=B_SPLINE_CURVE_WITH_KNOTS ( 'NONE', 3,
 ( #56854, #28967, #23506, #78451, #76695, #56423, #84796, #77136, #50536, #85227 ),
 .UNSPECIFIED., .F., .F.,
 ( 4, 2, 2, 2, 4 ),
 ( 0.0007817359430256388964, 0.0009771253907250075990, 0.001172514838424376085, 0.001367904286123744571, 0.001563293733823113273 ),
 .UNSPECIFIED. ) ;
#81201=EDGE_CURVE ( 'NONE', #41602, #87319, #75653, .T. ) ;
#81202=CARTESIAN_POINT ( 'NONE',  ( 18.22277954126840527, -12.24180327182771855, 31.33663988360758168 ) ) ;
#81203=CARTESIAN_POINT ( 'NONE',  ( -2.307692307692305711, -2.721908614388771852, 31.22303859784724978 ) ) ;
#81204=CARTESIAN_POINT ( 'NONE',  ( -5.999999999999998224, -12.10708131394839349, 31.69288490824020244 ) ) ;
#81206=ADVANCED_FACE ( 'NONE', ( #34792 ), #62260, .F. ) ;
#81207=AXIS2_PLACEMENT_3D ( 'NONE', #81147, #53208, #88360 ) ;
#81209=ORIENTED_EDGE ( 'NONE', *, *, #31031, .F. ) ;
#81210=VERTEX_POINT ( 'NONE', #27596 ) ;
#81211=CARTESIAN_POINT ( 'NONE',  ( -5.326946301144535489, -4.175268141568689195, 33.81360843649122216 ) ) ;
#81212=CARTESIAN_POINT ( 'NONE',  ( -17.20761368003338987, -9.929715669179216775, 34.40415004197138416 ) ) ;
#81213=CARTESIAN_POINT ( 'NONE',  ( -10.39237177129122003, -4.762714258010881885, 34.23016756924214832 ) ) ;
#81214=CYLINDRICAL_SURFACE ( 'NONE', #47168, 0.2499999999999994726 ) ;
#81215=CARTESIAN_POINT ( 'NONE',  ( -5.143006487878956534, -10.51840700105979387, 33.73612834413961536 ) ) ;
#81216=DIRECTION ( 'NONE',  ( 0.000000000000000000, 0.000000000000000000, 1.000000000000000000 ) ) ;
#81217=CARTESIAN_POINT ( 'NONE',  ( -5.076923076923197442, -4.481592998941358097, 33.73612834414048933 ) ) ;
#81218=CARTESIAN_POINT ( 'NONE',  ( 17.07692307692307665, -2.538708090699994813, 30.37095296980875503 ) ) ;
#81219=ORIENTED_EDGE ( 'NONE', *, *, #13032, .F. ) ;
#81221=ORIENTED_EDGE ( 'NONE', *, *, #33618, .T. ) ;
#81223=CARTESIAN_POINT ( 'NONE',  ( 2.307692307692187583, -2.625532179533779154, 30.86335684631627174 ) ) ;
#81225=ADVANCED_FACE ( 'NONE', ( #56836 ), #9979, .F. ) ;
#81227=LINE ( 'NONE', #74912, #73647 ) ;
#81229=CARTESIAN_POINT ( 'NONE',  ( -9.757578138268465651, -6.879047030191174805, 34.71129190930000163 ) ) ;
#81230=FACE_BOUND ( 'NONE', #85312, .T. ) ;
#81231=EDGE_LOOP ( 'NONE', ( #71991, #76588 ) ) ;
#81232=VECTOR ( 'NONE', #68042, 1000.000000000000227 ) ;
#81233=B_SPLINE_CURVE_WITH_KNOTS ( 'NONE', 3,
 ( #56780, #64857, #4505, #23434, #31983, #86498, #23866, #3607, #24773, #2708 ),
 .UNSPECIFIED., .F., .F.,
 ( 4, 2, 2, 2, 4 ),
 ( 0.000000000000000000, 0.0001954339857564091549, 0.0003908679715128183098, 0.0005863019572692274375, 0.0007817359430256366195 ),
 .UNSPECIFIED. ) ;
#81235=CARTESIAN_POINT ( 'NONE',  ( -5.076923076923075762, -6.386643153685126251, 34.62446782046654192 ) ) ;
#81237=ORIENTED_EDGE ( 'NONE', *, *, #55980, .T. ) ;
#81238=FACE_BOUND ( 'NONE', #44790, .T. ) ;
#81239=CARTESIAN_POINT ( 'NONE',  ( -9.469528023329624844, -2.353885683473779800, 30.79025554430704403 ) ) ;
#81241=CARTESIAN_POINT ( 'NONE',  ( -13.38461538461538325, -10.51840700105979565, 33.73612834413961536 ) ) ;
#81242=VERTEX_POINT ( 'NONE', #36577 ) ;
#81243=DIRECTION ( 'NONE',  ( -0.000000000000000000, 0.7660444431189791237, -0.6427876096865379196 ) ) ;
#81245=CARTESIAN_POINT ( 'NONE',  ( -1.384615384615506484, -9.528491918059723176, 34.59228464037033035 ) ) ;
#81246=ORIENTED_EDGE ( 'NONE', *, *, #52524, .T. ) ;
#81247=DIRECTION ( 'NONE',  ( -0.000000000000000000, 1.000000000000000000, -0.000000000000000000 ) ) ;
#81248=CARTESIAN_POINT ( 'NONE',  ( -7.623141002060451754, -8.282913670948747864, 34.94150082978203642 ) ) ;
#81249=CARTESIAN_POINT ( 'NONE',  ( 6.673100192134570285, -12.41269422305637171, 30.68257228309993323 ) ) ;
#81250=CARTESIAN_POINT ( 'NONE',  ( -17.86947456176635640, -12.70449254468099198, 30.44128974285582956 ) ) ;
#81252=CARTESIAN_POINT ( 'NONE',  ( -14.30769230769230660, -1.129524287112498415, 32.06866353760679544 ) ) ;
#81253=CARTESIAN_POINT ( 'NONE',  ( -5.076923076923197442, -3.300289026999228881, 32.46337939537708905 ) ) ;
#81254=ORIENTED_EDGE ( 'NONE', *, *, #38343, .F. ) ;
#81255=CARTESIAN_POINT ( 'NONE',  ( 3.361294669002876212, -6.808710257144159783, 34.95449254468098843 ) ) ;
#81257=CARTESIAN_POINT ( 'NONE',  ( -7.846153846153967493, -12.51329471203414379, 31.30864560766407578 ) ) ;
#81258=CARTESIAN_POINT ( 'NONE',  ( 16.40379156322419973, -12.07971442181321997, 32.31769673815850297 ) ) ;
#81259=CARTESIAN_POINT ( 'NONE',  ( -16.08777780284371772, -4.098570777380720287, 33.41473453929635440 ) ) ;
#81260=CARTESIAN_POINT ( 'NONE',  ( 17.32697749683652688, -4.818054556918155207, 34.26375889529406749 ) ) ;
#81261=CARTESIAN_POINT ( 'NONE',  ( 6.130525701763568591, -11.93748526763465279, 32.05452791011430946 ) ) ;
#81262=CARTESIAN_POINT ( 'NONE',  ( 8.519254025182176449, -2.920706130388546651, 32.31842814019191223 ) ) ;
#81263=EDGE_CURVE ( 'NONE', #84497, #78448, #50945, .T. ) ;
#81265=CARTESIAN_POINT ( 'NONE',  ( -3.480745961711584791, -2.564618984488975961, 30.55390908950641915 ) ) ;
#81266=CARTESIAN_POINT ( 'NONE',  ( -12.33074665371367473, -11.18335022499818621, 33.13157742990016885 ) ) ;
#81268=ORIENTED_EDGE ( 'NONE', *, *, #31105, .F. ) ;
#81269=CARTESIAN_POINT ( 'NONE',  ( -12.68502340526241312, -8.496056993536548418, 34.65000542017679663 ) ) ;
#81270=ORIENTED_EDGE ( 'NONE', *, *, #16924, .F. ) ;
#81272=VERTEX_POINT ( 'NONE', #42450 ) ;
#81273=DIRECTION ( 'NONE',  ( 0.000000000000000000, 0.8660254037844377084, -0.5000000000000015543 ) ) ;
#81275=ORIENTED_EDGE ( 'NONE', *, *, #87379, .F. ) ;
#81276=CARTESIAN_POINT ( 'NONE',  ( 1.607395053593450918, -12.11081565061823717, 32.26097654155341843 ) ) ;
#81278=CARTESIAN_POINT ( 'NONE',  ( -10.61538461538461320, -3.513871655860378418, 32.76840700105978499 ) ) ;
#81279=CARTESIAN_POINT ( 'NONE',  ( -8.899377978668987055, -3.285722584762969856, 32.44110544564090759 ) ) ;
#81280=CARTESIAN_POINT ( 'NONE',  ( 9.692307692307695177, -9.058645607665452459, 34.76329471203371924 ) ) ;
#81281=B_SPLINE_CURVE_WITH_KNOTS ( 'NONE', 3,
 ( #49832, #84526, #9307, #58353, #2091, #77750, #30450, #30887, #24130, #35891 ),
 .UNSPECIFIED., .F., .F.,
 ( 4, 2, 2, 2, 4 ),
 ( 0.000000000000000000, 0.0001954339857564073659, 0.0003908679715128147319, 0.0005863019572692221250, 0.0007817359430256294638 ),
 .UNSPECIFIED. ) ;
#81282=AXIS2_PLACEMENT_3D ( 'NONE', #88258, #39616, #13450 ) ;
#81283=CARTESIAN_POINT ( 'NONE',  ( -11.53846153846153655, -11.91647553114624181, 32.58852847137148245 ) ) ;
#81286=EDGE_CURVE ( 'NONE', #76991, #8812, #1488, .T. ) ;
#81287=DIRECTION ( 'NONE',  ( 0.000000000000000000, 0.9848077530122072432, 0.1736481776669354937 ) ) ;
#81288=CARTESIAN_POINT ( 'NONE',  ( 10.74617505635156789, -12.35292014791297710, 31.75344720912887198 ) ) ;
#81289=CARTESIAN_POINT ( 'NONE',  ( 12.46153846153877609, -2.255955759149395501, 30.00000000000324363 ) ) ;
#81290=EDGE_CURVE ( 'NONE', #33107, #77986, #15524, .T. ) ;
#81291=CARTESIAN_POINT ( 'NONE',  ( 18.13004516283478296, -2.504778602574659896, 29.97347330155780654 ) ) ;
#81292=ORIENTED_EDGE ( 'NONE', *, *, #11645, .T. ) ;
#81293=EDGE_LOOP ( 'NONE', ( #62349, #3135 ) ) ;
#81294=CARTESIAN_POINT ( 'NONE',  ( 14.30769230769231015, -8.164416787775445883, 34.95778746994557906 ) ) ;
#81295=CARTESIAN_POINT ( 'NONE',  ( 5.142178648199100088, -9.442884908240271713, 34.35708131394835618 ) ) ;
#81296=LINE ( 'NONE', #14153, #58413 ) ;
#81300=CARTESIAN_POINT ( 'NONE',  ( -9.915234651214539952, -6.459968553980841577, 34.89616026154728701 ) ) ;
#81301=DIRECTION ( 'NONE',  ( 0.000000000000000000, 0.9396926207859126468, -0.3420201433256571111 ) ) ;
#81302=ORIENTED_EDGE ( 'NONE', *, *, #96, .F. ) ;
#81304=ORIENTED_EDGE ( 'NONE', *, *, #30119, .T. ) ;
#81305=EDGE_CURVE ( 'NONE', #70228, #52302, #44531, .T. ) ;
#81306=ORIENTED_EDGE ( 'NONE', *, *, #23831, .T. ) ;
#81307=DIRECTION ( 'NONE',  ( -0.000000000000000000, 0.6427876096865404731, -0.7660444431189770143 ) ) ;
#81308=B_SPLINE_CURVE_WITH_KNOTS ( 'NONE', 3,
 ( #65084, #11050, #2942, #30427, #16031, #23223, #3391, #24105, #51555, #36741 ),
 .UNSPECIFIED., .F., .F.,
 ( 4, 2, 2, 2, 4 ),
 ( 0.000000000000000000, 0.0001954311564186868744, 0.0003908623128373737488, 0.0005862934692560606504, 0.0007817246256747474977 ),
 .UNSPECIFIED. ) ;
#81309=B_SPLINE_CURVE_WITH_KNOTS ( 'NONE', 3,
 ( #76918, #15222, #1698, #17430, #50749, #17877, #58848, #86801, #58392, #44430 ),
 .UNSPECIFIED., .F., .F.,
 ( 4, 2, 2, 2, 4 ),
 ( 0.000000000000000000, 0.0001954311564186876334, 0.0003908623128373752667, 0.0005862934692560629272, 0.0007817246256747505334 ),
 .UNSPECIFIED. ) ;
#81310=CARTESIAN_POINT ( 'NONE',  ( 3.930919936330005360, -2.554751324335733820, 30.48935550225260727 ) ) ;
#81311=CARTESIAN_POINT ( 'NONE',  ( 11.76147289007438523, -10.61302985866384141, 33.66295027996417843 ) ) ;
#81315=EDGE_LOOP ( 'NONE', ( #76001, #34433, #20591, #8695 ) ) ;
#81316=ADVANCED_FACE ( 'NONE', ( #8669 ), #70810, .F. ) ;
#81317=VERTEX_POINT ( 'NONE', #43769 ) ;
#81318=B_SPLINE_CURVE_WITH_KNOTS ( 'NONE', 3,
 ( #2599, #63425, #29219, #56673, #57552, #85042 ),
 .UNSPECIFIED., .F., .F.,
 ( 4, 2, 4 ),
 ( 0.0003909569690057776653, 0.0005862646681846002839, 0.0007815723673634227941 ),
 .UNSPECIFIED. ) ;
#81319=ORIENTED_EDGE ( 'NONE', *, *, #78435, .F. ) ;
#81320=ORIENTED_EDGE ( 'NONE', *, *, #56700, .F. ) ;
#81322=CARTESIAN_POINT ( 'NONE',  ( 5.999999999999880096, -2.625532179533778709, 30.86335684631627174 ) ) ;
#81323=DIRECTION ( 'NONE',  ( -0.000000000000000000, -0.9848077530122085754, -0.1736481776669273613 ) ) ;
#81324=CARTESIAN_POINT ( 'NONE',  ( 14.08476534878545827, -2.523278758544489797, 31.42238647778637528 ) ) ;
#81325=CARTESIAN_POINT ( 'NONE',  ( 16.15384615384615330, -9.780366693483667717, 34.19971097300155094 ) ) ;
#81326=CARTESIAN_POINT ( 'NONE',  ( 8.519230769230768274, -7.500000000000001776, 34.75000000000000000 ) ) ;
#81328=EDGE_CURVE ( 'NONE', #22454, #2963, #76780, .T. ) ;
#81329=ORIENTED_EDGE ( 'NONE', *, *, #23985, .F. ) ;
#81330=VECTOR ( 'NONE', #35166, 1000.000000000000227 ) ;
#81331=CARTESIAN_POINT ( 'NONE',  ( -10.39260507411620083, -11.89424750095246175, 32.13594075562311758 ) ) ;
#81332=ORIENTED_EDGE ( 'NONE', *, *, #47975, .F. ) ;
#81333=ADVANCED_FACE ( 'NONE', ( #58605 ), #5462, .F. ) ;
#81334=CARTESIAN_POINT ( 'NONE',  ( -9.692307692307812417, -5.219633306517616589, 34.19971097300220464 ) ) ;
#81335=CARTESIAN_POINT ( 'NONE',  ( -4.946131269098287930, -11.18335022499818621, 33.13157742990016885 ) ) ;
#81336=EDGE_CURVE ( 'NONE', #30954, #10997, #18970, .T. ) ;
#81338=VERTEX_POINT ( 'NONE', #38797 ) ;
#81339=B_SPLINE_CURVE_WITH_KNOTS ( 'NONE', 3,
 ( #31271, #39377, #25403, #79904, #5132, #11005, #58285, #38477, #31722, #59181 ),
 .UNSPECIFIED., .F., .F.,
 ( 4, 2, 2, 2, 4 ),
 ( 0.000000000000000000, 0.0001954311564186876334, 0.0003908623128373752667, 0.0005862934692560629272, 0.0007817246256747505334 ),
 .UNSPECIFIED. ) ;
#81340=CARTESIAN_POINT ( 'NONE',  ( -1.318548051265307608, -11.35647404775217595, 33.31231777344667222 ) ) ;
#81342=CARTESIAN_POINT ( 'NONE',  ( 2.307692307692187583, -6.879047030192662504, 34.71129190930017927 ) ) ;
#81343=CARTESIAN_POINT ( 'NONE',  ( -17.07692307692307665, -1.790695186598648903, 34.54067556320373455 ) ) ;
#81344=CARTESIAN_POINT ( 'NONE',  ( -12.23852710992561299, -12.39991518177334129, 30.74647679643404530 ) ) ;
#81345=CARTESIAN_POINT ( 'NONE',  ( -7.173100160369886957, -3.711651800289232916, 33.01384336483936011 ) ) ;
#81346=CARTESIAN_POINT ( 'NONE',  ( 8.545745825506822158, -5.113361153441934093, 34.14387501736622710 ) ) ;
#81347=ORIENTED_EDGE ( 'NONE', *, *, #45959, .T. ) ;
#81348=CARTESIAN_POINT ( 'NONE',  ( -18.00000000000000000, -13.34771219727535474, 34.33046132563154629 ) ) ;
#81349=CARTESIAN_POINT ( 'NONE',  ( 8.900021210197715860, -8.191423895709840863, 34.95447573519442130 ) ) ;
#81350=CARTESIAN_POINT ( 'NONE',  ( 14.05766908347085220, -9.356822207818506598, 34.66110646841856635 ) ) ;
#81351=ORIENTED_EDGE ( 'NONE', *, *, #68822, .F. ) ;
#81352=CARTESIAN_POINT ( 'NONE',  ( -9.692307692307691624, -4.661471528628507777, 34.16647553114623292 ) ) ;
#81353=CARTESIAN_POINT ( 'NONE',  ( -7.780898274877820597, -11.48612834413965977, 32.76840700105972815 ) ) ;
#81354=CARTESIAN_POINT ( 'NONE',  ( 17.14217864819910275, -10.21337939537593797, 33.94971097300152252 ) ) ;
#81355=CARTESIAN_POINT ( 'NONE',  ( -2.084679463598910765, -9.172514111537584114, 34.72667873470787470 ) ) ;
#81356=CARTESIAN_POINT ( 'NONE',  ( 14.30769230769218581, -11.67786785259630911, 32.92929555188603530 ) ) ;
#81358=FACE_BOUND ( 'NONE', #39561, .T. ) ;
#81359=CARTESIAN_POINT ( 'NONE',  ( 1.449760165335018725, -7.750023224968865421, 34.99404313364389907 ) ) ;
#81360=DIRECTION ( 'NONE',  ( -0.000000000000000000, 0.9396926207859093161, -0.3420201433256663259 ) ) ;
#81361=CARTESIAN_POINT ( 'NONE',  ( -15.00775638667583678, -4.762714258010881885, 34.23016756924214832 ) ) ;
#81362=CARTESIAN_POINT ( 'NONE',  ( 3.100158871144702122, -7.722926236386453702, 34.74524107206102030 ) ) ;
#81363=CARTESIAN_POINT ( 'NONE',  ( -2.057746898314263717, -8.476813868363244353, 34.90874843262270133 ) ) ;
#81364=CARTESIAN_POINT ( 'NONE',  ( 13.16168842570853670, -2.523278758544489797, 31.42238647778637528 ) ) ;
#81366=VERTEX_POINT ( 'NONE', #45095 ) ;
#81367=B_SPLINE_CURVE_WITH_KNOTS ( 'NONE', 3,
 ( #12228, #68066, #33824, #40596, #34267, #19427, #18987, #46453, #46891, #6371 ),
 .UNSPECIFIED., .F., .F.,
 ( 4, 2, 2, 2, 4 ),
 ( 0.000000000000000000, 0.0001954311564186866034, 0.0003908623128373732067, 0.0005862934692560597830, 0.0007817246256747464135 ),
 .UNSPECIFIED. ) ;
#81368=CARTESIAN_POINT ( 'NONE',  ( 10.54930223602448258, -11.91647553114624181, 32.58852847137148245 ) ) ;
#81369=ORIENTED_EDGE ( 'NONE', *, *, #8394, .F. ) ;
#81370=B_SPLINE_CURVE_WITH_KNOTS ( 'NONE', 3,
 ( #74042, #60515, #25402, #24057, #44766, #17309, #73145, #51506, #31721, #59179 ),
 .UNSPECIFIED., .F., .F.,
 ( 4, 2, 2, 2, 4 ),
 ( 0.0007817246336856289524, 0.0009771112958940101571, 0.001172497958102391253, 0.001367884620310772350, 0.001563271282519153446 ),
 .UNSPECIFIED. ) ;
#81371=CARTESIAN_POINT ( 'NONE',  ( -18.22292695890684655, -3.395401636524181477, 33.02366814457251110 ) ) ;
#81373=CARTESIAN_POINT ( 'NONE',  ( 2.084207383127978375, -2.353723527008296568, 30.78948104536958752 ) ) ;
#81375=CARTESIAN_POINT ( 'NONE',  ( 15.00790380856559025, -2.501496062324912284, 29.88072118266895671 ) ) ;
#81376=VECTOR ( 'NONE', #58042, 1000.000000000000227 ) ;
#81377=VERTEX_POINT ( 'NONE', #10436 ) ;
#81378=CARTESIAN_POINT ( 'NONE',  ( -10.55012947587177763, -12.16647553114626490, 32.15551576947920864 ) ) ;
#81379=CARTESIAN_POINT ( 'NONE',  ( 1.319345384059066317, -12.16647553114622049, 32.15551576947930812 ) ) ;
#81381=FACE_OUTER_BOUND ( 'NONE', #4927, .T. ) ;
#81382=CARTESIAN_POINT ( 'NONE',  ( 8.769230769230645706, -2.657715359629662544, 31.77849191805970364 ) ) ;
#81383=CARTESIAN_POINT ( 'NONE',  ( -12.21148404162501144, -9.233818618650603938, 34.70587769442853698 ) ) ;
#81384=CARTESIAN_POINT ( 'NONE',  ( -18.00000000000000000, -1.248569425608316630, 32.29137909377919868 ) ) ;
#81385=CARTESIAN_POINT ( 'NONE',  ( -0.2387589202700519386, -4.387253974876676565, 33.66317474335728832 ) ) ;
#81386=CARTESIAN_POINT ( 'NONE',  ( 1.607628228708781304, -10.01129605718032778, 34.36064277460058491 ) ) ;
#81387=EDGE_CURVE ( 'NONE', #27582, #41890, #13286, .T. ) ;
#81389=CARTESIAN_POINT ( 'NONE',  ( 14.05771557674995265, -5.728515186090277211, 34.42611988154120439 ) ) ;
#81391=ORIENTED_EDGE ( 'NONE', *, *, #52044, .F. ) ;
#81393=CYLINDRICAL_SURFACE ( 'NONE', #11114, 0.2500000000000009437 ) ;
#81394=DIRECTION ( 'NONE',  ( -0.000000000000000000, 0.5000000000000011102, -0.8660254037844380415 ) ) ;
#81396=CARTESIAN_POINT ( 'NONE',  ( -18.00000000000000000, -12.37446782046654192, 30.86335684631486131 ) ) ;
#81397=CARTESIAN_POINT ( 'NONE',  ( -16.15384615384627409, -11.06231777344772027, 33.60647404775119895 ) ) ;
#81398=ORIENTED_EDGE ( 'NONE', *, *, #87812, .T. ) ;
#81399=CARTESIAN_POINT ( 'NONE',  ( 1.384615384615386802, -13.49023893513002648, 31.06009739812518688 ) ) ;
#81400=CARTESIAN_POINT ( 'NONE',  ( -14.37296275365308418, -11.48612834413959582, 32.76840700105983473 ) ) ;
#81401=CARTESIAN_POINT ( 'NONE',  ( -17.32692307692307665, -7.433931650972299465, 34.75000000000000711 ) ) ;
#81402=ORIENTED_EDGE ( 'NONE', *, *, #207, .T. ) ;
#81404=CARTESIAN_POINT ( 'NONE',  ( 2.057669070399344768, -12.43535235679832596, 30.55408501211184813 ) ) ;
#81405=CARTESIAN_POINT ( 'NONE',  ( -12.68446542044531178, -4.762599654559228846, 34.23009711892697737 ) ) ;
#81406=EDGE_CURVE ( 'NONE', #14199, #56137, #25279, .T. ) ;
#81408=CARTESIAN_POINT ( 'NONE',  ( -9.626240358957616650, -2.486705287966280320, 31.30864560766543647 ) ) ;
#81409=CARTESIAN_POINT ( 'NONE',  ( -15.23076923076935252, -11.67786785259630911, 32.92929555188603530 ) ) ;
#81411=VERTEX_POINT ( 'NONE', #73479 ) ;
#81412=ORIENTED_EDGE ( 'NONE', *, *, #70751, .T. ) ;
#81413=ORIENTED_EDGE ( 'NONE', *, *, #21764, .T. ) ;
#81414=EDGE_CURVE ( 'NONE', #29059, #31685, #78881, .T. ) ;
#81415=ORIENTED_EDGE ( 'NONE', *, *, #28972, .T. ) ;
#81416=CARTESIAN_POINT ( 'NONE',  ( 12.59232890250541281, -9.929761469519743144, 34.40412654351204225 ) ) ;
#81417=CARTESIAN_POINT ( 'NONE',  ( -6.923076923077044142, -3.300289026999228881, 32.46337939537708905 ) ) ;
#81418=EDGE_CURVE ( 'NONE', #25833, #77581, #79811, .T. ) ;
#81419=CARTESIAN_POINT ( 'NONE',  ( -7.846153846153967493, -12.70778746994576025, 30.41441678777401236 ) ) ;
#81421=CARTESIAN_POINT ( 'NONE',  ( -17.01166750564705055, -5.219633306516380244, 34.19971097300157936 ) ) ;
#81422=ORIENTED_EDGE ( 'NONE', *, *, #68753, .T. ) ;
#81424=VERTEX_POINT ( 'NONE', #10878 ) ;
#81425=EDGE_CURVE ( 'NONE', #30965, #66553, #48692, .T. ) ;
#81426=EDGE_LOOP ( 'NONE', ( #53503, #57314 ) ) ;
#81427=CARTESIAN_POINT ( 'NONE',  ( -3.100724067934452322, -2.504778602574659896, 29.97347330155780298 ) ) ;
#81428=VERTEX_POINT ( 'NONE', #18082 ) ;
#81429=CARTESIAN_POINT ( 'NONE',  ( -6.700297254098854793, -4.226511098958374291, 33.85474049983370293 ) ) ;
#81430=CARTESIAN_POINT ( 'NONE',  ( 6.130790440966952026, -2.494656445102013453, 31.33466734024120015 ) ) ;
#81434=ORIENTED_EDGE ( 'NONE', *, *, #45999, .F. ) ;
#81436=VERTEX_POINT ( 'NONE', #69374 ) ;
#81437=B_SPLINE_CURVE_WITH_KNOTS ( 'NONE', 3,
 ( #5313, #12514, #60246, #87753, #88200, #53487, #40000, #83194, #41764, #16054 ),
 .UNSPECIFIED., .F., .F.,
 ( 4, 2, 2, 2, 4 ),
 ( 0.000000000000000000, 0.0001954339857564070678, 0.0003908679715128141356, 0.0005863019572692211492, 0.0007817359430256282712 ),
 .UNSPECIFIED. ) ;
#81439=CARTESIAN_POINT ( 'NONE',  ( 10.74591031714818357, -10.88167719472716399, 33.43325721877153711 ) ) ;
#81440=CARTESIAN_POINT ( 'NONE',  ( -2.373775718648187372, -2.721908614388772296, 31.22303859784724622 ) ) ;
#81441=ORIENTED_EDGE ( 'NONE', *, *, #37397, .F. ) ;
#81442=LINE ( 'NONE', #87773, #80554 ) ;
#81443=EDGE_CURVE ( 'NONE', #65658, #51461, #8979, .T. ) ;
#81444=ADVANCED_FACE ( 'NONE', ( #33809 ), #61711, .F. ) ;
#81445=CARTESIAN_POINT ( 'NONE',  ( -14.43838377435986686, -2.541943142973491554, 30.39792223712631980 ) ) ;
#81446=ORIENTED_EDGE ( 'NONE', *, *, #12795, .F. ) ;
#81447=DIRECTION ( 'NONE',  ( 0.000000000000000000, 0.8660254037844377084, 0.5000000000000015543 ) ) ;
#81449=CARTESIAN_POINT ( 'NONE',  ( 4.284637961670938466, -2.729792928343270919, 31.24908615093345077 ) ) ;
#81450=FACE_BOUND ( 'NONE', #84329, .T. ) ;
#81451=EDGE_CURVE ( 'NONE', #34858, #4333, #68048, .T. ) ;
#81452=CARTESIAN_POINT ( 'NONE',  ( -0.6850234052624104564, -10.11188796281391511, 34.01382737946119050 ) ) ;
#81454=DIRECTION ( 'NONE',  ( 0.000000000000000000, 0.7660444431189822323, -0.6427876096865344779 ) ) ;
#81455=CARTESIAN_POINT ( 'NONE',  ( 0.4615384615384611200, -6.343179335718451384, 34.87096338111211935 ) ) ;
#81456=CARTESIAN_POINT ( 'NONE',  ( 6.923076923076924238, -10.67929555188718282, 33.92786785259544047 ) ) ;
#81457=CARTESIAN_POINT ( 'NONE',  ( -5.011667505647053211, -10.90142922261932057, 33.41473453929631887 ) ) ;
#81458=DIRECTION ( 'NONE',  ( -0.000000000000000000, -0.000000000000000000, -1.000000000000000000 ) ) ;
#81460=CARTESIAN_POINT ( 'NONE',  ( 2.530471848960718084, -6.760870238392817200, 34.69528174975672385 ) ) ;
#81461=CARTESIAN_POINT ( 'NONE',  ( 14.30769230769218758, -10.21337939537710326, 33.94971097300076224 ) ) ;
#81462=EDGE_LOOP ( 'NONE', ( #45964, #9012, #4854, #77842 ) ) ;
#81463=EDGE_LOOP ( 'NONE', ( #28328, #5192, #36448, #74440 ) ) ;
#81464=AXIS2_PLACEMENT_3D ( 'NONE', #77828, #85927, #63871 ) ;
#81466=CARTESIAN_POINT ( 'NONE',  ( -14.37377571864818293, -4.786620604624113540, 33.94971097300155805 ) ) ;
#81467=CARTESIAN_POINT ( 'NONE',  ( 12.39626846098214052, -11.06231777344662781, 33.60647404775220082 ) ) ;
#81469=CARTESIAN_POINT ( 'NONE',  ( -15.23076923076922995, -1.629998284177014645, 34.34916445242399163 ) ) ;
#81470=DIRECTION ( 'NONE',  ( 0.000000000000000000, 0.1736481776669275834, 0.9848077530122086864 ) ) ;
#81471=FACE_BOUND ( 'NONE', #74792, .T. ) ;
#81472=CARTESIAN_POINT ( 'NONE',  ( -16.94613126909829148, -4.118422570099827595, 33.43335022499816489 ) ) ;
#81473=CYLINDRICAL_SURFACE ( 'NONE', #43053, 0.2499999999999997502 ) ;
#81474=CARTESIAN_POINT ( 'NONE',  ( 10.54930120442873687, -8.120952969808774569, 34.71129190930000163 ) ) ;
#81475=CARTESIAN_POINT ( 'NONE',  ( 2.307692307692309264, -4.786620604624113540, 33.94971097300155094 ) ) ;
#81477=LINE ( 'NONE', #34157, #10390 ) ;
#81479=ORIENTED_EDGE ( 'NONE', *, *, #68033, .F. ) ;
#81480=ORIENTED_EDGE ( 'NONE', *, *, #57046, .T. ) ;
#81481=B_SPLINE_CURVE_WITH_KNOTS ( 'NONE', 3,
 ( #17001, #24194, #10693, #71942, #37712, #30946, #38159, #3918, #58873, #86373 ),
 .UNSPECIFIED., .F., .F.,
 ( 4, 2, 2, 2, 4 ),
 ( 0.0007817246256747453293, 0.0009771112852218889842, 0.001172497944769032747, 0.001367884604316176294, 0.001563271263863320057 ),
 .UNSPECIFIED. ) ;
#81483=CARTESIAN_POINT ( 'NONE',  ( 12.59237687955122453, -7.277220443632450575, 34.74524770363009196 ) ) ;
#81484=CARTESIAN_POINT ( 'NONE',  ( -10.61538461538473399, -12.27809138561165270, 31.22303859784587132 ) ) ;
#81485=CARTESIAN_POINT ( 'NONE',  ( 17.20696813284285298, -2.254550872974305786, 29.97347326024527092 ) ) ;
#81486=B_SPLINE_CURVE_WITH_KNOTS ( 'NONE', 3,
 ( #7851, #21355, #20474, #82635, #7409, #35312, #41193, #27228, #20907, #33983 ),
 .UNSPECIFIED., .F., .F.,
 ( 4, 2, 2, 2, 4 ),
 ( 0.0007817246256747464135, 0.0009771112852218900684, 0.001172497944769033615, 0.001367884604316177161, 0.001563271263863320925 ),
 .UNSPECIFIED. ) ;
#81487=CARTESIAN_POINT ( 'NONE',  ( 17.07692307692307665, -11.11383981884818262, 36.00935417666054406 ) ) ;
#81489=CARTESIAN_POINT ( 'NONE',  ( -8.835313148590904220, -9.905515769479276145, 34.41647553114623292 ) ) ;
#81490=CARTESIAN_POINT ( 'NONE',  ( 5.777073041093149897, -2.889293201056495786, 32.26117774369186009 ) ) ;
#81491=CARTESIAN_POINT ( 'NONE',  ( -15.48076923076922995, -2.249999999999998668, 29.75000000000000355 ) ) ;
#81492=CARTESIAN_POINT ( 'NONE',  ( 10.74617505635156789, -3.338503747796866872, 32.95102852606553512 ) ) ;
#81493=CARTESIAN_POINT ( 'NONE',  ( -6.249976730942353065, -2.779195860258147022, 31.39871582349836743 ) ) ;
#81495=CARTESIAN_POINT ( 'NONE',  ( -3.454254155333559950, -10.23692288466677880, 34.23039457007281072 ) ) ;
#81496=VECTOR ( 'NONE', #56328, 1000.000000000000227 ) ;
#81497=CARTESIAN_POINT ( 'NONE',  ( 2.177082652488226078, -7.722926974430166069, 34.99546784045485737 ) ) ;
#81498=CARTESIAN_POINT ( 'NONE',  ( -15.36146069743678844, -9.804603061927743113, 34.18744698557895845 ) ) ;
#81503=CARTESIAN_POINT ( 'NONE',  ( -0.3954711281883860341, -10.67929555188718282, 33.92786785259544757 ) ) ;
#81504=CARTESIAN_POINT ( 'NONE',  ( -8.769230769230768274, -13.53365097954675988, 30.81389545987213552 ) ) ;
#81505=CYLINDRICAL_SURFACE ( 'NONE', #1091, 0.2500000000000008882 ) ;
#81506=CARTESIAN_POINT ( 'NONE',  ( -0.3962828902624367933, -2.625532179533470067, 30.86335684631491105 ) ) ;
#81507=ORIENTED_EDGE ( 'NONE', *, *, #24065, .F. ) ;
#81511=VERTEX_POINT ( 'NONE', #20736 ) ;
#81512=CARTESIAN_POINT ( 'NONE',  ( 8.546304551714619890, -8.239355502252617924, 34.69524867566427417 ) ) ;
#81513=CARTESIAN_POINT ( 'NONE',  ( 18.13052570176356681, -9.417988943895561960, 34.36773134775778260 ) ) ;
#81514=ORIENTED_EDGE ( 'NONE', *, *, #58838, .F. ) ;
#81515=CARTESIAN_POINT ( 'NONE',  ( -10.61538461538461320, -5.471508081941601098, 34.59228464037088457 ) ) ;
#81516=CARTESIAN_POINT ( 'NONE',  ( -14.98076923076781064, -7.500000000000154543, 35.00000000000007105 ) ) ;
#81517=B_SPLINE_CURVE_WITH_KNOTS ( 'NONE', 3,
 ( #35170, #82924, #48676, #69405, #56330, #942, #84261, #15795, #63071, #77484 ),
 .UNSPECIFIED., .F., .F.,
 ( 4, 2, 2, 2, 4 ),
 ( 0.000000000000000000, 0.0001954339857564093717, 0.0003908679715128187434, 0.0005863019572692280881, 0.0007817359430256374869 ),
 .UNSPECIFIED. ) ;
#81519=ORIENTED_EDGE ( 'NONE', *, *, #8956, .F. ) ;
#81520=VECTOR ( 'NONE', #36411, 1000.000000000000227 ) ;
#81521=ORIENTED_EDGE ( 'NONE', *, *, #67195, .F. ) ;
#81522=EDGE_CURVE ( 'NONE', #16211, #63956, #47576, .T. ) ;
#81523=ORIENTED_EDGE ( 'NONE', *, *, #57599, .T. ) ;
#81524=CARTESIAN_POINT ( 'NONE',  ( 3.480823650682685511, -12.01375889529407637, 32.43194544308182969 ) ) ;
#81525=CARTESIAN_POINT ( 'NONE',  ( 6.923076923076800782, -11.67786785259630911, 32.92929555188603530 ) ) ;
#81527=CARTESIAN_POINT ( 'NONE',  ( -10.55012904410858532, -6.879047030191282275, 34.71129190930002295 ) ) ;
#81528=CARTESIAN_POINT ( 'NONE',  ( -1.608100309179715026, -11.60425143139329940, 33.02411095842164457 ) ) ;
#81529=B_SPLINE_CURVE_WITH_KNOTS ( 'NONE', 3,
 ( #70728, #3134, #85567, #23841, #78799, #67079, #25644, #39620, #10796, #25197 ),
 .UNSPECIFIED., .F., .F.,
 ( 4, 2, 2, 2, 4 ),
 ( 0.000000000000000000, 0.0001954311564186868473, 0.0003908623128373736946, 0.0005862934692560605419, 0.0007817246256747473893 ),
 .UNSPECIFIED. ) ;
#81530=DIRECTION ( 'NONE',  ( -0.000000000000000000, -0.7660444431189791237, -0.6427876096865379196 ) ) ;
#81531=CARTESIAN_POINT ( 'NONE',  ( 9.758375025657770152, -9.905515769479276145, 34.41647553114623292 ) ) ;
#81532=CYLINDRICAL_SURFACE ( 'NONE', #52408, 0.2499999999999994726 ) ;
#81533=VECTOR ( 'NONE', #83511, 999.9999999999998863 ) ;
#81534=CARTESIAN_POINT ( 'NONE',  ( -7.846153846153844924, -1.951392089020283160, 34.73218667398347748 ) ) ;
#81535=ORIENTED_EDGE ( 'NONE', *, *, #24687, .T. ) ;
#81536=EDGE_CURVE ( 'NONE', #44047, #41209, #61263, .T. ) ;
#81537=EDGE_LOOP ( 'NONE', ( #27150, #80005 ) ) ;
#81538=CARTESIAN_POINT ( 'NONE',  ( -0.2387589202700515223, -12.24180327182771855, 31.33663988360758168 ) ) ;
#81539=ORIENTED_EDGE ( 'NONE', *, *, #4229, .T. ) ;
#81540=B_SPLINE_CURVE_WITH_KNOTS ( 'NONE', 3,
 ( #58054, #2656, #24261, #36468, #57616, #85538, #71126, #51724, #29715, #85099 ),
 .UNSPECIFIED., .F., .F.,
 ( 4, 2, 2, 2, 4 ),
 ( 0.000000000000000000, 0.0001954339881912775425, 0.0003908679763825550850, 0.0005863019645738326005, 0.0007817359527651101701 ),
 .UNSPECIFIED. ) ;
#81541=DIRECTION ( 'NONE',  ( 0.000000000000000000, 0.000000000000000000, 1.000000000000000000 ) ) ;
#81542=CARTESIAN_POINT ( 'NONE',  ( 11.66898724022510336, -12.27024696741798770, 31.24895572276497546 ) ) ;
#81543=ORIENTED_EDGE ( 'NONE', *, *, #46223, .T. ) ;
#81544=CARTESIAN_POINT ( 'NONE',  ( -8.769230769230892619, -4.320704448113951379, 33.92786785259630022 ) ) ;
#81545=ORIENTED_EDGE ( 'NONE', *, *, #5963, .F. ) ;
#81546=CARTESIAN_POINT ( 'NONE',  ( 11.76124107972994537, -2.600157965045224895, 30.74683119005207743 ) ) ;
#81547=ORIENTED_EDGE ( 'NONE', *, *, #20221, .F. ) ;
#81548=CARTESIAN_POINT ( 'NONE',  ( -12.68441797827604667, -7.630690623152299956, 34.99857592706774057 ) ) ;
#81549=EDGE_CURVE ( 'NONE', #28353, #46262, #49810, .T. ) ;
#81550=ADVANCED_FACE ( 'NONE', ( #14421 ), #26166, .F. ) ;
#81551=CARTESIAN_POINT ( 'NONE',  ( 4.153846153846154188, -10.67929555188718282, 33.92786785259544047 ) ) ;
#81552=CARTESIAN_POINT ( 'NONE',  ( -9.019254006523736322, -2.823816976329319051, 31.52131813110795733 ) ) ;
#81554=FACE_BOUND ( 'NONE', #70906, .T. ) ;
#81555=DIRECTION ( 'NONE',  ( -0.000000000000000000, -0.000000000000000000, -1.000000000000000000 ) ) ;
#81556=CARTESIAN_POINT ( 'NONE',  ( -2.307692307692428724, -4.320704448113951379, 33.92786785259630022 ) ) ;
#81557=CARTESIAN_POINT ( 'NONE',  ( -8.769230769230768274, -1.242168528481310874, 33.36296068462461051 ) ) ;
#81559=CARTESIAN_POINT ( 'NONE',  ( -13.38461538461538325, -9.905515769479276145, 34.41647553114623292 ) ) ;
#81560=CARTESIAN_POINT ( 'NONE',  ( 16.02315468717859304, -4.118384482072086072, 33.43331474514187107 ) ) ;
#81561=AXIS2_PLACEMENT_3D ( 'NONE', #24509, #79911, #87134 ) ;
#81562=CARTESIAN_POINT ( 'NONE',  ( -10.48485891362105171, -4.459921816937791661, 33.71989282347011851 ) ) ;
#81563=EDGE_CURVE ( 'NONE', #71146, #64437, #19408, .T. ) ;
#81564=VERTEX_POINT ( 'NONE', #5901 ) ;
#81565=ORIENTED_EDGE ( 'NONE', *, *, #87763, .F. ) ;
#81566=CARTESIAN_POINT ( 'NONE',  ( -5.143005456283213483, -11.91647553114624181, 32.58852847137148245 ) ) ;
#81567=CARTESIAN_POINT ( 'NONE',  ( -14.05763799605399278, -12.41262288849542017, 30.68299917996395010 ) ) ;
#81568=CARTESIAN_POINT ( 'NONE',  ( -4.219169069338327915, -7.749976743299137993, 34.99404534957040624 ) ) ;
#81570=CARTESIAN_POINT ( 'NONE',  ( 8.546351252493185058, -7.630690623152299956, 34.99857592706774057 ) ) ;
#81571=LINE ( 'NONE', #12662, #64821 ) ;
#81572=ORIENTED_EDGE ( 'NONE', *, *, #45014, .F. ) ;
#81573=CARTESIAN_POINT ( 'NONE',  ( 2.307692307692309264, -8.973038597847269315, 34.52809138561121927 ) ) ;
#81576=DIRECTION ( 'NONE',  ( 0.000000000000000000, 0.9396926207859126468, -0.3420201433256571111 ) ) ;
#81577=ORIENTED_EDGE ( 'NONE', *, *, #87121, .F. ) ;
#81579=ORIENTED_EDGE ( 'NONE', *, *, #85476, .T. ) ;
#81580=VECTOR ( 'NONE', #14411, 1000.000000000000114 ) ;
#81581=CARTESIAN_POINT ( 'NONE',  ( -17.07692307692307665, -1.129524287112498415, 32.06866353760679544 ) ) ;
#81582=VERTEX_POINT ( 'NONE', #74808 ) ;
#81583=CARTESIAN_POINT ( 'NONE',  ( 15.23076923076911093, -2.892918686052165622, 31.69288490824153470 ) ) ;
#81584=CARTESIAN_POINT ( 'NONE',  ( 14.53070515178570510, -5.582272713120729257, 34.63742843783360570 ) ) ;
#81585=CARTESIAN_POINT ( 'NONE',  ( 3.480714640147273720, -5.766571408460171355, 34.70601412856602508 ) ) ;
#81586=CARTESIAN_POINT ( 'NONE',  ( -2.373775718648186928, -8.120952969808774569, 34.71129190930000163 ) ) ;
#81587=CARTESIAN_POINT ( 'NONE',  ( 9.758376043310132530, -5.557115091759786019, 34.35708131394839882 ) ) ;
#81588=ORIENTED_EDGE ( 'NONE', *, *, #81159, .F. ) ;
#81589=CARTESIAN_POINT ( 'NONE',  ( -15.09997878980228059, -2.494656445102012565, 31.33466734024120015 ) ) ;
#81590=CARTESIAN_POINT ( 'NONE',  ( -15.23076923076935252, -2.379036618888197729, 30.90682066428292885 ) ) ;
#81591=VERTEX_POINT ( 'NONE', #33374 ) ;
#81592=DIRECTION ( 'NONE',  ( -0.000000000000000000, 0.3420201433256694346, -0.9396926207859080948 ) ) ;
#81593=CARTESIAN_POINT ( 'NONE',  ( -2.438383774359864642, -8.999036380462717588, 34.52022231692819076 ) ) ;
#81594=B_SPLINE_CURVE_WITH_KNOTS ( 'NONE', 3,
 ( #11780, #86563, #11327, #73488, #32939, #5020, #80240, #39259, #37915, #24382 ),
 .UNSPECIFIED., .F., .F.,
 ( 4, 2, 2, 2, 4 ),
 ( 0.000000000000000000, 0.0001954339857564080707, 0.0003908679715128161414, 0.0005863019572692241849, 0.0007817359430256322827 ),
 .UNSPECIFIED. ) ;
#81595=FACE_OUTER_BOUND ( 'NONE', #10660, .T. ) ;
#81596=CARTESIAN_POINT ( 'NONE',  ( -2.373774687052442545, -12.62096338111211580, 30.90682066428152197 ) ) ;
#81597=CYLINDRICAL_SURFACE ( 'NONE', #41891, 0.2500000000000009437 ) ;
#81598=VECTOR ( 'NONE', #43158, 1000.000000000000114 ) ;
#81599=CARTESIAN_POINT ( 'NONE',  ( -8.769230769230892619, -9.528491918059723176, 34.59228464037033035 ) ) ;
#81600=CARTESIAN_POINT ( 'NONE',  ( 12.59233026936325039, -11.18335022499818621, 33.13157742990016885 ) ) ;
#81602=VERTEX_POINT ( 'NONE', #26611 ) ;
#81603=CARTESIAN_POINT ( 'NONE',  ( 14.30769230769231015, -13.57706302396349152, 30.56769352161908060 ) ) ;
#81604=CYLINDRICAL_SURFACE ( 'NONE', #51937, 0.2500000000000012212 ) ;
#81605=CARTESIAN_POINT ( 'NONE',  ( -9.692307692307691624, -5.557115091759785130, 34.35708131394839171 ) ) ;
#81606=ORIENTED_EDGE ( 'NONE', *, *, #30369, .T. ) ;
#81607=CARTESIAN_POINT ( 'NONE',  ( -5.776988648387150427, -2.554770724473668153, 30.48948780036025852 ) ) ;
#81608=CARTESIAN_POINT ( 'NONE',  ( 3.100208639027310475, -2.504760397472875155, 29.97295953869789997 ) ) ;
#81609=EDGE_CURVE ( 'NONE', #79299, #57617, #34664, .T. ) ;
#81610=CARTESIAN_POINT ( 'NONE',  ( 6.923076923076924238, -12.09954503811598769, 35.62045528018868623 ) ) ;
#81611=CARTESIAN_POINT ( 'NONE',  ( 14.30769230769231015, -13.20930481340135110, 34.54067556320372745 ) ) ;
#81612=CARTESIAN_POINT ( 'NONE',  ( 17.74997677577853850, -2.588893531581426100, 31.60682220781849239 ) ) ;
#81613=EDGE_LOOP ( 'NONE', ( #7693, #58118 ) ) ;
#81615=CARTESIAN_POINT ( 'NONE',  ( -16.21992853320628569, -6.343179335718451384, 34.87096338111212646 ) ) ;
#81616=CARTESIAN_POINT ( 'NONE',  ( -14.43838377435986331, -2.729777683071817229, 31.24903638046269450 ) ) ;
#81617=CARTESIAN_POINT ( 'NONE',  ( 7.846153846153725020, -10.21337939537710326, 33.94971097300076224 ) ) ;
#81618=VERTEX_POINT ( 'NONE', #42353 ) ;
#81619=CARTESIAN_POINT ( 'NONE',  ( -8.638392438744007862, -7.277220318596961057, 34.99547417642776992 ) ) ;
#81622=VERTEX_POINT ( 'NONE', #70700 ) ;
#81625=CARTESIAN_POINT ( 'NONE',  ( -5.777220331021932331, -12.11081565061823717, 32.26097654155341843 ) ) ;
#81626=ORIENTED_EDGE ( 'NONE', *, *, #17742, .F. ) ;
#81627=VECTOR ( 'NONE', #9167, 1000.000000000000227 ) ;
#81628=ADVANCED_FACE ( 'NONE', ( #84670 ), #8561, .F. ) ;
#81629=CARTESIAN_POINT ( 'NONE',  ( -13.38461538461538325, -4.661471528628507777, 34.16647553114623292 ) ) ;
#81630=LINE ( 'NONE', #60458, #21966 ) ;
#81631=CARTESIAN_POINT ( 'NONE',  ( -7.846153846153844924, -1.242168528481310874, 33.36296068462461051 ) ) ;
#81632=CARTESIAN_POINT ( 'NONE',  ( -9.692307692307814193, -11.67786785259630911, 32.92929555188603530 ) ) ;
#81633=CYLINDRICAL_SURFACE ( 'NONE', #51168, 0.2499999999999986955 ) ;
#81636=CARTESIAN_POINT ( 'NONE',  ( 13.38461538461538680, -2.249999999999998668, 29.75000000000001776 ) ) ;
#81638=DIRECTION ( 'NONE',  ( 0.000000000000000000, 0.7660444431189807890, 0.6427876096865361433 ) ) ;
#81639=FACE_OUTER_BOUND ( 'NONE', #3582, .T. ) ;
#81640=EDGE_CURVE ( 'NONE', #79746, #86676, #368, .T. ) ;
#81642=CARTESIAN_POINT ( 'NONE',  ( 1.384615384615386802, -2.708943851104267164, 35.45975837776705220 ) ) ;
#81643=CARTESIAN_POINT ( 'NONE',  ( -10.61538461538461320, -1.242168528481310874, 33.36296068462461051 ) ) ;
#81644=CARTESIAN_POINT ( 'NONE',  ( 16.82689983963011926, -2.587272538249754117, 30.68239716806877837 ) ) ;
#81645=ORIENTED_EDGE ( 'NONE', *, *, #70443, .T. ) ;
#81646=ORIENTED_EDGE ( 'NONE', *, *, #43589, .F. ) ;
#81648=ORIENTED_EDGE ( 'NONE', *, *, #67420, .F. ) ;
#81649=EDGE_CURVE ( 'NONE', #19083, #292, #14239, .T. ) ;
#81650=AXIS2_PLACEMENT_3D ( 'NONE', #81724, #13256, #40737 ) ;
#81651=CARTESIAN_POINT ( 'NONE',  ( -4.283993363284373856, -6.001485441113818986, 34.52039167877662607 ) ) ;
#81652=CARTESIAN_POINT ( 'NONE',  ( 16.37685899793954292, -10.77377354290276301, 33.85451476688484718 ) ) ;
#81653=EDGE_CURVE ( 'NONE', #603, #59888, #22507, .T. ) ;
#81654=DIRECTION ( 'NONE',  ( 0.000000000000000000, 0.9396926207859126468, 0.3420201433256571111 ) ) ;
#81655=FACE_OUTER_BOUND ( 'NONE', #22924, .T. ) ;
#81656=CARTESIAN_POINT ( 'NONE',  ( -5.326946314216042033, -10.76384336483936011, 33.53834819971076087 ) ) ;
#81657=EDGE_CURVE ( 'NONE', #57345, #72521, #82057, .T. ) ;
#81658=CARTESIAN_POINT ( 'NONE',  ( 2.307692307692309264, -2.721908614388771852, 31.22303859784724978 ) ) ;
#81659=ADVANCED_FACE ( 'NONE', ( #63035 ), #57620, .F. ) ;
#81660=CARTESIAN_POINT ( 'NONE',  ( 16.15384615384603251, -3.300289026999228437, 32.46337939537709616 ) ) ;
#81661=CARTESIAN_POINT ( 'NONE',  ( 1.134615384615387246, -7.500000000000001776, 34.75000000000000000 ) ) ;
#81662=VERTEX_POINT ( 'NONE', #29718 ) ;
#81663=ORIENTED_EDGE ( 'NONE', *, *, #52831, .F. ) ;
#81664=ORIENTED_EDGE ( 'NONE', *, *, #16401, .F. ) ;
#81665=CARTESIAN_POINT ( 'NONE',  ( -12.46153846153858247, -10.90142922262034020, 33.41473453929536674 ) ) ;
#81666=ORIENTED_EDGE ( 'NONE', *, *, #50810, .F. ) ;
#81667=DIRECTION ( 'NONE',  ( -0.000000000000000000, -0.5000000000000009992, -0.8660254037844380415 ) ) ;
#81668=CYLINDRICAL_SURFACE ( 'NONE', #80775, 0.2499999999999973355 ) ;
#81669=CARTESIAN_POINT ( 'NONE',  ( 18.00000000000000000, -1.466349020453238561, 30.81389545987213907 ) ) ;
#81671=CARTESIAN_POINT ( 'NONE',  ( -15.29603923132555110, -10.33852847137145048, 34.16647553114627556 ) ) ;
#81672=FACE_BOUND ( 'NONE', #28246, .T. ) ;
#81673=ORIENTED_EDGE ( 'NONE', *, *, #81336, .F. ) ;
#81674=B_SPLINE_CURVE_WITH_KNOTS ( 'NONE', 3,
 ( #79578, #31836, #11563, #39488, #66501, #38136, #65594, #32706, #87678, #17874 ),
 .UNSPECIFIED., .F., .F.,
 ( 4, 2, 2, 2, 4 ),
 ( 0.000000000000000000, 0.0001954339857564074473, 0.0003908679715128148945, 0.0005863019572692223418, 0.0007817359430256297891 ),
 .UNSPECIFIED. ) ;
#81675=CARTESIAN_POINT ( 'NONE',  ( -8.769230769230768274, -2.499999999999998668, 29.50000000000001066 ) ) ;
#81676=CARTESIAN_POINT ( 'NONE',  ( -1.449885385171703511, -3.643525952247789412, 33.31231777344662959 ) ) ;
#81677=ORIENTED_EDGE ( 'NONE', *, *, #78278, .T. ) ;
#81678=CARTESIAN_POINT ( 'NONE',  ( -8.519230769230766498, -2.499999999999999556, 29.81604066197449754 ) ) ;
#81679=VECTOR ( 'NONE', #46765, 999.9999999999998863 ) ;
#81680=ORIENTED_EDGE ( 'NONE', *, *, #81788, .T. ) ;
#81681=FACE_BOUND ( 'NONE', #27300, .T. ) ;
#81682=CARTESIAN_POINT ( 'NONE',  ( -9.442362282929646966, -2.341251567377310217, 30.72681386836322659 ) ) ;
#81683=CARTESIAN_POINT ( 'NONE',  ( 8.069529331926265314, -2.251407671071270489, 29.88021292934943318 ) ) ;
#81685=CARTESIAN_POINT ( 'NONE',  ( -12.21159294319032362, -8.433404298154334455, 34.66254593164985920 ) ) ;
#81686=DIRECTION ( 'NONE',  ( -0.000000000000000000, -0.5000000000000009992, -0.8660254037844380415 ) ) ;
#81687=AXIS2_PLACEMENT_3D ( 'NONE', #75725, #41507, #85593 ) ;
#81688=FACE_OUTER_BOUND ( 'NONE', #80350, .T. ) ;
#81689=ORIENTED_EDGE ( 'NONE', *, *, #76895, .F. ) ;
#81690=CARTESIAN_POINT ( 'NONE',  ( -8.546217925137373328, -3.395485233115139057, 33.02377354290275946 ) ) ;
#81691=DIRECTION ( 'NONE',  ( -0.000000000000000000, -0.8660254037844397068, -0.4999999999999978906 ) ) ;
#81692=CARTESIAN_POINT ( 'NONE',  ( 18.06525513951284267, -11.06231777344670952, 33.60647404775212266 ) ) ;
#81693=LINE ( 'NONE', #66838, #4473 ) ;
#81694=ORIENTED_EDGE ( 'NONE', *, *, #40386, .F. ) ;
#81695=CARTESIAN_POINT ( 'NONE',  ( 16.37685750545900376, -10.61302985866384141, 33.66295027996417843 ) ) ;
#81697=ORIENTED_EDGE ( 'NONE', *, *, #42512, .T. ) ;
#81700=CARTESIAN_POINT ( 'NONE',  ( -13.16183584334697265, -5.114059244376869984, 34.14424750095245287 ) ) ;
#81701=CARTESIAN_POINT ( 'NONE',  ( 10.86538461538605205, -7.500000000000155431, 34.75000000000007105 ) ) ;
#81702=LINE ( 'NONE', #11017, #7085 ) ;
#81703=EDGE_CURVE ( 'NONE', #66105, #45448, #63680, .T. ) ;
#81704=CARTESIAN_POINT ( 'NONE',  ( 15.10062126103753322, -5.915902021225889484, 34.75552854090298638 ) ) ;
#81707=CARTESIAN_POINT ( 'NONE',  ( 14.30769230769231015, -3.513871655860378418, 32.76840700105978499 ) ) ;
#81709=ORIENTED_EDGE ( 'NONE', *, *, #76201, .T. ) ;
#81710=CARTESIAN_POINT ( 'NONE',  ( -16.21911615440246734, -5.094484230520675894, 34.41647553114621161 ) ) ;
#81711=ORIENTED_EDGE ( 'NONE', *, *, #39545, .T. ) ;
#81712=EDGE_CURVE ( 'NONE', #16973, #44052, #38240, .T. ) ;
#81714=EDGE_LOOP ( 'NONE', ( #10831, #42877 ) ) ;
#81715=DIRECTION ( 'NONE',  ( -0.000000000000000000, -0.5000000000000009992, -0.8660254037844380415 ) ) ;
#81716=ORIENTED_EDGE ( 'NONE', *, *, #25486, .T. ) ;
#81717=CARTESIAN_POINT ( 'NONE',  ( 1.634669804528839698, -12.01375889529407281, 32.43194544308182969 ) ) ;
#81719=CARTESIAN_POINT ( 'NONE',  ( 17.86985203026830149, -5.070767119584671079, 34.40440758774516183 ) ) ;
#81720=CARTESIAN_POINT ( 'NONE',  ( -11.28840711854808632, -10.06805714834173493, 34.32951233291982618 ) ) ;
#81721=CARTESIAN_POINT ( 'NONE',  ( -2.084680956079456582, -6.503523203565942268, 34.64991518177335195 ) ) ;
#81722=EDGE_CURVE ( 'NONE', #58791, #58630, #45506, .T. ) ;
#81723=VECTOR ( 'NONE', #88870, 1000.000000000000114 ) ;
#81724=CARTESIAN_POINT ( 'NONE',  ( 3.230769230769231726, -1.242168528481310874, 33.36296068462461051 ) ) ;
#81725=CARTESIAN_POINT ( 'NONE',  ( -13.51476259405360203, -2.619462340734462380, 30.83744416345203021 ) ) ;
#81728=CARTESIAN_POINT ( 'NONE',  ( 10.68063975489745587, -12.51329471203373345, 31.30864560766537963 ) ) ;
#81729=CARTESIAN_POINT ( 'NONE',  ( 10.61538461538461675, -2.249999999999998668, 29.75000000000001776 ) ) ;
#81730=VECTOR ( 'NONE', #78609, 1000.000000000000000 ) ;
#81731=FACE_OUTER_BOUND ( 'NONE', #4767, .T. ) ;
#81732=EDGE_CURVE ( 'NONE', #21879, #74312, #66147, .T. ) ;
#81733=VERTEX_POINT ( 'NONE', #58057 ) ;
#81734=ORIENTED_EDGE ( 'NONE', *, *, #52028, .T. ) ;
#81735=CARTESIAN_POINT ( 'NONE',  ( -11.47239318745910097, -5.557115091759786019, 34.35708131394839882 ) ) ;
#81736=CARTESIAN_POINT ( 'NONE',  ( 5.207448778686640800, -9.417988943895561960, 34.36773134775778260 ) ) ;
#81737=DIRECTION ( 'NONE',  ( 0.000000000000000000, 0.000000000000000000, 1.000000000000000000 ) ) ;
#81738=CARTESIAN_POINT ( 'NONE',  ( 5.933916589044121892, -5.557115091759785130, 34.35708131394839171 ) ) ;
#81739=ADVANCED_FACE ( 'NONE', ( #38685 ), #17977, .F. ) ;
#81740=CARTESIAN_POINT ( 'NONE',  ( 6.222779541268409709, -5.114059244376869984, 34.14424750095245287 ) ) ;
#81741=CARTESIAN_POINT ( 'NONE',  ( -13.63459212866397507, -10.82459398097509329, 33.81372124010185587 ) ) ;
#81742=CARTESIAN_POINT ( 'NONE',  ( -2.557669051740897537, -8.347322224742351082, 34.93158281831414769 ) ) ;
#81744=CARTESIAN_POINT ( 'NONE',  ( -10.61538461538461320, -5.415277668671390821, 36.20867863119892149 ) ) ;
#81745=ORIENTED_EDGE ( 'NONE', *, *, #86026, .T. ) ;
#81746=AXIS2_PLACEMENT_3D ( 'NONE', #74130, #80905, #33140 ) ;
#81748=CARTESIAN_POINT ( 'NONE',  ( 16.40379156322419973, -9.357781135181033605, 34.66075350412533851 ) ) ;
#81749=CARTESIAN_POINT ( 'NONE',  ( 4.403846153846215472, -7.434744860731433924, 35.00000000000000711 ) ) ;
#81750=CARTESIAN_POINT ( 'NONE',  ( -0.2385271099256117411, -6.503523203565942268, 34.64991518177335195 ) ) ;
#81753=ORIENTED_EDGE ( 'NONE', *, *, #81653, .F. ) ;
#81754=EDGE_LOOP ( 'NONE', ( #43438, #50081 ) ) ;
#81755=B_SPLINE_CURVE_WITH_KNOTS ( 'NONE', 3,
 ( #49652, #15879, #71239, #8233, #15436, #57740, #16312, #85660, #43778, #64039 ),
 .UNSPECIFIED., .F., .F.,
 ( 4, 2, 2, 2, 4 ),
 ( 0.000000000000000000, 0.0001954339857564096157, 0.0003908679715128192313, 0.0005863019572692288470, 0.0007817359430256384627 ),
 .UNSPECIFIED. ) ;
#81756=ORIENTED_EDGE ( 'NONE', *, *, #87040, .T. ) ;
#81757=ORIENTED_EDGE ( 'NONE', *, *, #62702, .F. ) ;
#81758=EDGE_CURVE ( 'NONE', #2169, #86522, #50741, .T. ) ;
#81759=CARTESIAN_POINT ( 'NONE',  ( -5.999999999999998224, -4.661471528628507777, 34.16647553114623292 ) ) ;
#81760=CARTESIAN_POINT ( 'NONE',  ( -2.373774687052442545, -9.905515769479276145, 34.41647553114623292 ) ) ;
#81761=CARTESIAN_POINT ( 'NONE',  ( 4.284371592079796898, -12.15418822224088657, 32.17964115625579069 ) ) ;
#81762=ADVANCED_FACE ( 'NONE', ( #73361 ), #37790, .F. ) ;
#81763=CARTESIAN_POINT ( 'NONE',  ( 14.43773974294276208, -7.723484941389743952, 34.99544897038808955 ) ) ;
#81764=AXIS2_PLACEMENT_3D ( 'NONE', #1935, #29420, #63183 ) ;
#81765=CARTESIAN_POINT ( 'NONE',  ( -17.07692307692307665, -3.050289026998446396, 32.03036669348365706 ) ) ;
#81766=EDGE_CURVE ( 'NONE', #20268, #49865, #4671, .T. ) ;
#81767=CARTESIAN_POINT ( 'NONE',  ( 14.05766907039934210, -12.43535235679832596, 30.55408501211184813 ) ) ;
#81768=VERTEX_POINT ( 'NONE', #37337 ) ;
#81770=EDGE_LOOP ( 'NONE', ( #54727, #77137 ) ) ;
#81772=CARTESIAN_POINT ( 'NONE',  ( -3.230769230769352962, -2.657715359629662544, 31.77849191805970364 ) ) ;
#81773=ORIENTED_EDGE ( 'NONE', *, *, #77450, .F. ) ;
#81774=CARTESIAN_POINT ( 'NONE',  ( 12.46153846153846168, -2.249999999999998668, 29.75000000000001776 ) ) ;
#81775=DIRECTION ( 'NONE',  ( -0.000000000000000000, 0.7660444431189791237, -0.6427876096865379196 ) ) ;
#81776=VECTOR ( 'NONE', #85348, 1000.000000000000000 ) ;
#81778=ORIENTED_EDGE ( 'NONE', *, *, #52444, .T. ) ;
#81779=VECTOR ( 'NONE', #57287, 1000.000000000000227 ) ;
#81780=EDGE_CURVE ( 'NONE', #64954, #56376, #3110, .T. ) ;
#81781=CARTESIAN_POINT ( 'NONE',  ( -1.253824943648432333, -2.494656445102013453, 31.33466734024120015 ) ) ;
#81782=EDGE_LOOP ( 'NONE', ( #18838, #43675, #35358, #54807 ) ) ;
#81783=DIRECTION ( 'NONE',  ( -0.000000000000000000, 1.000000000000000000, 3.491481338843133355E-15 ) ) ;
#81784=FACE_BOUND ( 'NONE', #2535, .T. ) ;
#81785=CARTESIAN_POINT ( 'NONE',  ( -4.946397375159510723, -12.27024696741798770, 31.24895572276497546 ) ) ;
#81788=EDGE_CURVE ( 'NONE', #31874, #58385, #44532, .T. ) ;
#81789=CARTESIAN_POINT ( 'NONE',  ( 8.638540166120465713, -11.93127051446799847, 32.56575433478202797 ) ) ;
#81790=CARTESIAN_POINT ( 'NONE',  ( -15.23076923076922995, -1.117168528481311540, 33.14645433367849847 ) ) ;
#81791=CARTESIAN_POINT ( 'NONE',  ( -18.00000000000000000, -3.895656007487076078, 35.99290692298802696 ) ) ;
#81792=CARTESIAN_POINT ( 'NONE',  ( -3.230769230769352962, -9.528491918059723176, 34.59228464037033035 ) ) ;
#81794=DIRECTION ( 'NONE',  ( -0.000000000000000000, -0.9396926207859093161, -0.3420201433256663259 ) ) ;
#81795=FACE_OUTER_BOUND ( 'NONE', #61679, .T. ) ;
#81796=LINE ( 'NONE', #19639, #42677 ) ;
#81797=CARTESIAN_POINT ( 'NONE',  ( -2.242437168179467033, -9.528491918058460186, 34.59228464037085615 ) ) ;
#81798=CARTESIAN_POINT ( 'NONE',  ( 8.769230769230645706, -10.33852847137269571, 34.16647553114546554 ) ) ;
#81799=EDGE_CURVE ( 'NONE', #45833, #52906, #29565, .T. ) ;
#81800=FACE_BOUND ( 'NONE', #14674, .T. ) ;
#81801=CARTESIAN_POINT ( 'NONE',  ( 1.608041783530174129, -7.630147987733843173, 34.99859428049665411 ) ) ;
#81802=CARTESIAN_POINT ( 'NONE',  ( -8.769230769230768274, -4.945431358278436385, 36.03766855953609394 ) ) ;
#81803=CARTESIAN_POINT ( 'NONE',  ( -15.00798956179116317, -4.989023458446560255, 34.36081565061822118 ) ) ;
#81804=CARTESIAN_POINT ( 'NONE',  ( -16.15384615384627409, -4.320704448113951379, 33.92786785259630022 ) ) ;
#81809=VERTEX_POINT ( 'NONE', #9298 ) ;
#81810=EDGE_CURVE ( 'NONE', #75748, #77695, #75491, .T. ) ;
#81811=B_SPLINE_CURVE_WITH_KNOTS ( 'NONE', 3,
 ( #24558, #86741, #71858, #31325, #52474, #37630, #73204, #58336, #31776, #11504 ),
 .UNSPECIFIED., .F., .F.,
 ( 4, 2, 2, 2, 4 ),
 ( 0.000000000000000000, 0.0001954339857564097241, 0.0003908679715128194482, 0.0005863019572692291723, 0.0007817359430256388964 ),
 .UNSPECIFIED. ) ;
#81812=CARTESIAN_POINT ( 'NONE',  ( -8.638438961405983108, -5.582136614379148654, 34.36778462344220486 ) ) ;
#81813=VERTEX_POINT ( 'NONE', #36324 ) ;
#81814=LINE ( 'NONE', #67845, #39230 ) ;
#81815=ORIENTED_EDGE ( 'NONE', *, *, #1622, .T. ) ;
#81816=CARTESIAN_POINT ( 'NONE',  ( 4.153846153846154188, -8.564572088678739092, 35.78748833219616898 ) ) ;
#81817=CARTESIAN_POINT ( 'NONE',  ( -7.846153846153844924, -13.53365097954675988, 30.81389545987213552 ) ) ;
#81818=CARTESIAN_POINT ( 'NONE',  ( 15.23076923076953904, -2.506253911140615021, 30.00000000000323297 ) ) ;
#81820=CARTESIAN_POINT ( 'NONE',  ( 1.384615384615386802, -4.661471528628507777, 34.16647553114623292 ) ) ;
#81822=CYLINDRICAL_SURFACE ( 'NONE', #36053, 0.2500000000000004996 ) ;
#81823=DIRECTION ( 'NONE',  ( -0.000000000000000000, 0.8660254037844399289, -0.4999999999999980016 ) ) ;
#81824=EDGE_CURVE ( 'NONE', #5310, #13392, #73441, .T. ) ;
#81825=CARTESIAN_POINT ( 'NONE',  ( -12.21159305216042057, -9.357781135181031829, 34.66075350412533851 ) ) ;
#81826=LINE ( 'NONE', #34949, #61692 ) ;
#81827=CARTESIAN_POINT ( 'NONE',  ( -1.384615384615383471, -6.343179335718451384, 34.87096338111211935 ) ) ;
#81828=CARTESIAN_POINT ( 'NONE',  ( 11.60371710973756620, -3.835265460703683349, 33.15142922261929925 ) ) ;
#81830=CARTESIAN_POINT ( 'NONE',  ( 5.142990410273150736, -2.486705287966279876, 31.30864560766543647 ) ) ;
#81832=EDGE_LOOP ( 'NONE', ( #83492, #34636 ) ) ;
#81835=B_SPLINE_CURVE_WITH_KNOTS ( 'NONE', 3,
 ( #16352, #56006, #28098, #23108, #55560, #35750, #62751, #83049, #21335, #9165 ),
 .UNSPECIFIED., .F., .F.,
 ( 4, 2, 2, 2, 4 ),
 ( 0.0007817359430256399806, 0.0009771253907250089001, 0.001172514838424378036, 0.001367904286123746956, 0.001563293733823115875 ),
 .UNSPECIFIED. ) ;
#81836=CARTESIAN_POINT ( 'NONE',  ( -17.86920819217521483, -12.38066358083363738, 30.83685684665853444 ) ) ;
#81837=VECTOR ( 'NONE', #85683, 1000.000000000000227 ) ;
#81838=CARTESIAN_POINT ( 'NONE',  ( 5.142178216435913107, -6.835583212224609184, 34.95778746994559327 ) ) ;
#81839=VERTEX_POINT ( 'NONE', #77298 ) ;
#81840=DIRECTION ( 'NONE',  ( -0.000000000000000000, 0.8660254037844399289, -0.4999999999999980016 ) ) ;
#81841=CARTESIAN_POINT ( 'NONE',  ( -0.2387589202700533542, -10.11255958852955850, 34.01340905677049165 ) ) ;
#81843=EDGE_LOOP ( 'NONE', ( #19955, #58016, #39201, #22278, #37552, #16470 ) ) ;
#81844=CARTESIAN_POINT ( 'NONE',  ( -3.099977422944444783, -3.530189275343204702, 32.79018710029569661 ) ) ;
#81845=EDGE_CURVE ( 'NONE', #5354, #20560, #1193, .T. ) ;
#81846=DIRECTION ( 'NONE',  ( -0.000000000000000000, -0.5000000000000009992, -0.8660254037844380415 ) ) ;
#81848=CARTESIAN_POINT ( 'NONE',  ( -10.39260494640654819, -9.418065098278013636, 34.63729479722530158 ) ) ;
#81849=ADVANCED_FACE ( 'NONE', ( #16045 ), #15605, .F. ) ;
#81850=ORIENTED_EDGE ( 'NONE', *, *, #44696, .F. ) ;
#81852=CARTESIAN_POINT ( 'NONE',  ( 15.23076923076911093, -10.21337939537710326, 33.94971097300076224 ) ) ;
#81853=CARTESIAN_POINT ( 'NONE',  ( 12.21153846153846168, -7.500000000000001776, 35.04278698407183867 ) ) ;
#81854=VECTOR ( 'NONE', #82792, 1000.000000000000227 ) ;
#81855=CARTESIAN_POINT ( 'NONE',  ( 1.319345384059066539, -3.083524468853724443, 32.58852847137143272 ) ) ;
#81856=ORIENTED_EDGE ( 'NONE', *, *, #40334, .T. ) ;
#81857=ORIENTED_EDGE ( 'NONE', *, *, #32410, .F. ) ;
#81858=ORIENTED_EDGE ( 'NONE', *, *, #76972, .T. ) ;
#81859=B_SPLINE_CURVE_WITH_KNOTS ( 'NONE', 3,
 ( #27825, #69697, #15648, #63376, #7563, #21057, #62483, #55733, #8004, #14311 ),
 .UNSPECIFIED., .F., .F.,
 ( 4, 2, 2, 2, 4 ),
 ( 0.000000000000000000, 0.0001954339857564093175, 0.0003908679715128186350, 0.0005863019572692279796, 0.0007817359430256372700 ),
 .UNSPECIFIED. ) ;
#81860=EDGE_LOOP ( 'NONE', ( #24702, #80052, #44086, #65815 ) ) ;
#81861=CARTESIAN_POINT ( 'NONE',  ( 5.207448778686641688, -12.27024696741798770, 31.24895572276497546 ) ) ;
#81862=DIRECTION ( 'NONE',  ( 0.000000000000000000, 0.4999999999999960032, -0.8660254037844410391 ) ) ;
#81863=CARTESIAN_POINT ( 'NONE',  ( 9.692307692307572609, -5.219633306517616589, 34.19971097300220464 ) ) ;
#81864=DIRECTION ( 'NONE',  ( -0.000000000000000000, -0.3420201433256694901, -0.9396926207859082059 ) ) ;
#81865=CARTESIAN_POINT ( 'NONE',  ( 16.02315468717859659, -4.809359713505814149, 33.96456829005828837 ) ) ;
#81866=ORIENTED_EDGE ( 'NONE', *, *, #51108, .T. ) ;
#81867=EDGE_LOOP ( 'NONE', ( #69322, #56785, #37731, #19493, #15623, #13490 ) ) ;
#81868=EDGE_LOOP ( 'NONE', ( #69760, #80186 ) ) ;
#81869=CYLINDRICAL_SURFACE ( 'NONE', #51574, 0.2499999999999986955 ) ;
#81871=CARTESIAN_POINT ( 'NONE',  ( -4.946132635956127288, -12.35292014791297710, 31.75344720912887198 ) ) ;
#81872=CARTESIAN_POINT ( 'NONE',  ( -3.454254155333559062, -12.11044203135681840, 32.26167407432752299 ) ) ;
#81873=EDGE_CURVE ( 'NONE', #82763, #12084, #32574, .T. ) ;
#81874=CARTESIAN_POINT ( 'NONE',  ( 7.145856592054990131, -4.989023458446560255, 34.36081565061822118 ) ) ;
#81875=CARTESIAN_POINT ( 'NONE',  ( 11.53846153846153832, -6.386643153685126251, 34.62446782046654192 ) ) ;
#81876=ADVANCED_FACE ( 'NONE', ( #57020 ), #43514, .F. ) ;
#81877=EDGE_LOOP ( 'NONE', ( #81391, #32232 ) ) ;
#81878=EDGE_LOOP ( 'NONE', ( #40987, #47083 ) ) ;
#81879=B_SPLINE_CURVE_WITH_KNOTS ( 'NONE', 3,
 ( #49226, #15001, #70387, #1483, #29841, #62721, #42921, #56426, #62282, #41580 ),
 .UNSPECIFIED., .F., .F.,
 ( 4, 2, 2, 2, 4 ),
 ( 0.000000000000000000, 0.0001954311564186879044, 0.0003908623128373758088, 0.0005862934692560636861, 0.0007817246256747516176 ),
 .UNSPECIFIED. ) ;
#81880=B_SPLINE_CURVE_WITH_KNOTS ( 'NONE', 3,
 ( #27060, #61269, #69814, #55413, #6781, #914, #76125, #41913, #8122, #56303 ),
 .UNSPECIFIED., .F., .F.,
 ( 4, 2, 2, 2, 4 ),
 ( 0.0007817246256747484735, 0.0009771112852218922368, 0.001172497944769036217, 0.001367884604316180197, 0.001563271263863323960 ),
 .UNSPECIFIED. ) ;
#81883=CARTESIAN_POINT ( 'NONE',  ( -10.36543920600657565, -2.589246495874658383, 31.60778113518102828 ) ) ;
#81884=EDGE_LOOP ( 'NONE', ( #80284, #51566, #28835, #46793 ) ) ;
#81885=EDGE_CURVE ( 'NONE', #58249, #27791, #28270, .T. ) ;
#81886=CARTESIAN_POINT ( 'NONE',  ( -4.153846153846152411, -6.435427911321262684, 35.78748833219616898 ) ) ;
#81887=CARTESIAN_POINT ( 'NONE',  ( -14.37296275365308063, -2.625532179533444754, 30.86335684631481513 ) ) ;
#81888=ORIENTED_EDGE ( 'NONE', *, *, #80331, .T. ) ;
#81889=DIRECTION ( 'NONE',  ( -0.000000000000000000, -0.9396926207859093161, -0.3420201433256663259 ) ) ;
#81890=CARTESIAN_POINT ( 'NONE',  ( 9.915683178080113791, -2.251407671071270489, 29.88021292934942963 ) ) ;
#81891=EDGE_CURVE ( 'NONE', #22506, #720, #14533, .T. ) ;
#81892=CARTESIAN_POINT ( 'NONE',  ( -0.4615384615384611200, -11.11383981884818262, 36.00935417666054406 ) ) ;
#81893=FACE_BOUND ( 'NONE', #28148, .T. ) ;
#81894=CARTESIAN_POINT ( 'NONE',  ( -0.6844646790546099480, -9.886141570436013382, 34.14413921362392301 ) ) ;
#81895=LINE ( 'NONE', #4900, #70159 ) ;
#81896=DIRECTION ( 'NONE',  ( 0.000000000000000000, 0.9848077530122072432, -0.1736481776669354937 ) ) ;
#81897=LINE ( 'NONE', #6663, #80614 ) ;
#81900=EDGE_CURVE ( 'NONE', #33320, #73867, #88436, .T. ) ;
#81901=CARTESIAN_POINT ( 'NONE',  ( -4.023007823359388446, -7.277220318596959281, 34.99547417642776992 ) ) ;
#81902=DIRECTION ( 'NONE',  ( -1.000000000000000000, 0.000000000000000000, 0.000000000000000000 ) ) ;
#81903=ORIENTED_EDGE ( 'NONE', *, *, #7098, .F. ) ;
#81904=CARTESIAN_POINT ( 'NONE',  ( -18.24997673094235395, -10.66389620160130036, 33.62221079203477103 ) ) ;
#81905=CARTESIAN_POINT ( 'NONE',  ( 0.2386115026316120435, -10.77366814457252175, 33.85459836347579454 ) ) ;
#81907=VECTOR ( 'NONE', #31231, 1000.000000000000227 ) ;
#81909=CARTESIAN_POINT ( 'NONE',  ( -15.29685264172511161, -2.538708090699994813, 30.37095296980875148 ) ) ;
#81910=CARTESIAN_POINT ( 'NONE',  ( -14.30769230769230660, -4.098570777380720287, 33.41473453929634729 ) ) ;
#81912=CARTESIAN_POINT ( 'NONE',  ( -15.90390063549801347, -11.37275283266504111, 32.91324779482534524 ) ) ;
#81913=CARTESIAN_POINT ( 'NONE',  ( -14.98071481085577972, -12.65882529074907126, 30.72640787790839312 ) ) ;
#81914=FACE_BOUND ( 'NONE', #86179, .T. ) ;
#81915=CARTESIAN_POINT ( 'NONE',  ( -17.07692307692307665, -4.098570777380720287, 33.41473453929634729 ) ) ;
#81916=CARTESIAN_POINT ( 'NONE',  ( -16.94687802100330742, -2.254550872974305342, 29.97347326024527092 ) ) ;
#81917=CARTESIAN_POINT ( 'NONE',  ( -8.899922235898330314, -6.413092428213692742, 34.63065189839063152 ) ) ;
#81918=CARTESIAN_POINT ( 'NONE',  ( 16.15384615384615330, -12.29105614889573062, 35.45975837776705220 ) ) ;
#81919=CARTESIAN_POINT ( 'NONE',  ( 2.084207383127975710, -10.97335522853832579, 33.68706563782419749 ) ) ;
#81922=EDGE_CURVE ( 'NONE', #25790, #74135, #56191, .T. ) ;
#81923=B_SPLINE_CURVE_WITH_KNOTS ( 'NONE', 3,
 ( #17981, #66150, #9879, #58493, #23820, #22952 ),
 .UNSPECIFIED., .F., .F.,
 ( 4, 2, 4 ),
 ( 0.0003909512603273947911, 0.0005862562993132216203, 0.0007815613382990483412 ),
 .UNSPECIFIED. ) ;
#81924=ORIENTED_EDGE ( 'NONE', *, *, #72931, .F. ) ;
#81925=CARTESIAN_POINT ( 'NONE',  ( 4.946775107191377252, -11.04286588640298561, 33.62463336215343901 ) ) ;
#81926=CARTESIAN_POINT ( 'NONE',  ( 16.40379167219429490, -6.696923467548659303, 34.68552623307873972 ) ) ;
#81927=CARTESIAN_POINT ( 'NONE',  ( -0.4615384615385840772, -6.835583212225970762, 34.95778746994575670 ) ) ;
#81928=CARTESIAN_POINT ( 'NONE',  ( -13.38461538461538325, -8.810774026931790459, 35.74407628777942847 ) ) ;
#81929=CARTESIAN_POINT ( 'NONE',  ( -3.230769230769229949, -5.557115091759785130, 34.35708131394839171 ) ) ;
#81931=LINE ( 'NONE', #32401, #8658 ) ;
#81932=CARTESIAN_POINT ( 'NONE',  ( 6.000000000000001776, -2.833524468853757305, 32.15551576947925838 ) ) ;
#81933=EDGE_CURVE ( 'NONE', #1002, #78695, #59373, .T. ) ;
#81934=CARTESIAN_POINT ( 'NONE',  ( 17.99999999999987566, -4.320704448113951379, 33.92786785259630022 ) ) ;
#81935=CARTESIAN_POINT ( 'NONE',  ( -7.846153846153844924, -8.973038597847269315, 34.52809138561121927 ) ) ;
#81936=CARTESIAN_POINT ( 'NONE',  ( -6.130691466667555822, -2.729777683071817229, 31.24903638046268739 ) ) ;
#81937=CARTESIAN_POINT ( 'NONE',  ( 15.23076923076923173, -12.34228464037088635, 31.77849191805839268 ) ) ;
#81938=CARTESIAN_POINT ( 'NONE',  ( 6.923076923076924238, -3.322132147404559976, 32.92929555188717927 ) ) ;
#81939=CARTESIAN_POINT ( 'NONE',  ( 2.557692307692246203, -7.565270000091922853, 34.99999999999999289 ) ) ;
#81940=ADVANCED_FACE ( 'NONE', ( #14984 ), #55514, .F. ) ;
#81941=EDGE_CURVE ( 'NONE', #74006, #72884, #7342, .T. ) ;
#81942=CARTESIAN_POINT ( 'NONE',  ( 12.59233026936324329, -2.729792928343269587, 31.24908615093345077 ) ) ;
#81943=EDGE_LOOP ( 'NONE', ( #28427, #25293 ) ) ;
#81944=VECTOR ( 'NONE', #73829, 1000.000000000000000 ) ;
#81945=LINE ( 'NONE', #68412, #81598 ) ;
#81946=LINE ( 'NONE', #68413, #51779 ) ;
#81948=CARTESIAN_POINT ( 'NONE',  ( -0.4615384615385840772, -11.06231777344772027, 33.60647404775119895 ) ) ;
#81952=ORIENTED_EDGE ( 'NONE', *, *, #67116, .F. ) ;
#81954=CARTESIAN_POINT ( 'NONE',  ( 17.93391658904412012, -3.513871655860377086, 32.76840700105978499 ) ) ;
#81955=B_SPLINE_CURVE_WITH_KNOTS ( 'NONE', 3,
 ( #11710, #38728, #39187, #58988, #27320, #31976, #39634, #17575, #38285, #59439 ),
 .UNSPECIFIED., .F., .F.,
 ( 4, 2, 2, 2, 4 ),
 ( 0.000000000000000000, 0.0001954311564186868473, 0.0003908623128373736946, 0.0005862934692560605419, 0.0007817246256747473893 ),
 .UNSPECIFIED. ) ;
#81956=EDGE_CURVE ( 'NONE', #5991, #79867, #31455, .T. ) ;
#81957=B_SPLINE_CURVE_WITH_KNOTS ( 'NONE', 3,
 ( #77441, #17066, #10315, #50398, #22937, #77880, #23807, #65246, #44521, #50830 ),
 .UNSPECIFIED., .F., .F.,
 ( 4, 2, 2, 2, 4 ),
 ( 0.000000000000000000, 0.0001954311564186876876, 0.0003908623128373753751, 0.0005862934692560630356, 0.0007817246256747507503 ),
 .UNSPECIFIED. ) ;
#81958=ORIENTED_EDGE ( 'NONE', *, *, #67465, .F. ) ;
#81959=CARTESIAN_POINT ( 'NONE',  ( 11.60452887181161508, -9.058645607665452459, 34.76329471203371924 ) ) ;
#81960=CARTESIAN_POINT ( 'NONE',  ( -7.053767526187231240, -11.37499894934982514, 33.29245874905763003 ) ) ;
#81961=VERTEX_POINT ( 'NONE', #29392 ) ;
#81962=CARTESIAN_POINT ( 'NONE',  ( 16.85343813319912343, -11.41268669641499756, 32.86336882939238535 ) ) ;
#81963=EDGE_CURVE ( 'NONE', #83460, #28375, #75355, .T. ) ;
#81964=EDGE_CURVE ( 'NONE', #53, #7171, #7703, .T. ) ;
#81966=CARTESIAN_POINT ( 'NONE',  ( -7.846153846153965716, -3.835265460704628371, 33.15142922262033665 ) ) ;
#81967=EDGE_LOOP ( 'NONE', ( #72999, #7089, #7078, #29408 ) ) ;
#81969=CARTESIAN_POINT ( 'NONE',  ( 6.066067333350078528, -11.91647553114624358, 32.58852847137148245 ) ) ;
#81970=EDGE_CURVE ( 'NONE', #72319, #363, #45100, .T. ) ;
#81971=EDGE_LOOP ( 'NONE', ( #80771, #49838, #8772, #10087 ) ) ;
#81974=CARTESIAN_POINT ( 'NONE',  ( 3.361294669002874436, -12.15418822224088657, 32.17964115625579069 ) ) ;
#81975=CARTESIAN_POINT ( 'NONE',  ( -9.692307692307812417, -10.21337939537710326, 33.94971097300076224 ) ) ;
#81976=CARTESIAN_POINT ( 'NONE',  ( 9.442284468086235449, -9.356822207818506598, 34.66110646841856635 ) ) ;
#81977=LINE ( 'NONE', #20263, #77853 ) ;
#81978=DIRECTION ( 'NONE',  ( -0.000000000000000000, -0.8660254037844399289, -0.4999999999999980016 ) ) ;
#81980=VECTOR ( 'NONE', #13892, 1000.000000000000227 ) ;
#81981=CARTESIAN_POINT ( 'NONE',  ( -17.07692307692319744, -6.879047030192662504, 34.71129190930017927 ) ) ;
#81982=ORIENTED_EDGE ( 'NONE', *, *, #18388, .F. ) ;
#81983=ORIENTED_EDGE ( 'NONE', *, *, #8845, .T. ) ;
#81985=ORIENTED_EDGE ( 'NONE', *, *, #87906, .T. ) ;
#81986=ADVANCED_FACE ( 'NONE', ( #3665 ), #57288, .F. ) ;
#81987=DIRECTION ( 'NONE',  ( 1.000000000000000000, 0.000000000000000000, 0.000000000000000000 ) ) ;
#81988=CYLINDRICAL_SURFACE ( 'NONE', #746, 0.2500000000000009437 ) ;
#81989=ORIENTED_EDGE ( 'NONE', *, *, #33112, .T. ) ;
#81990=CARTESIAN_POINT ( 'NONE',  ( 15.23076923076923173, -9.058645607665452459, 34.76329471203371924 ) ) ;
#81991=VERTEX_POINT ( 'NONE', #23495 ) ;
#81992=CARTESIAN_POINT ( 'NONE',  ( 11.60452988946397745, -2.538708090699994813, 30.37095296980875503 ) ) ;
#81993=VERTEX_POINT ( 'NONE', #38355 ) ;
#81994=DIRECTION ( 'NONE',  ( -0.000000000000000000, 1.000000000000000000, 3.491481338843133355E-15 ) ) ;
#81995=ORIENTED_EDGE ( 'NONE', *, *, #11342, .F. ) ;
#81996=DIRECTION ( 'NONE',  ( -0.000000000000000000, 0.5000000000000011102, -0.8660254037844380415 ) ) ;
#81997=CARTESIAN_POINT ( 'NONE',  ( 10.74591031714818357, -5.195472089885680766, 34.18748526763464923 ) ) ;
#81998=FACE_BOUND ( 'NONE', #18920, .T. ) ;
#81999=FACE_OUTER_BOUND ( 'NONE', #39758, .T. ) ;
#82000=FACE_OUTER_BOUND ( 'NONE', #27906, .T. ) ;
#82001=CARTESIAN_POINT ( 'NONE',  ( 9.561617089197390840, -11.37499894934982692, 33.29245874905763003 ) ) ;
#82002=CARTESIAN_POINT ( 'NONE',  ( 4.376625695114563008, -8.496831190052096971, 34.64984203495476578 ) ) ;
#82003=CARTESIAN_POINT ( 'NONE',  ( 4.153846153846030731, -9.528491918059723176, 34.59228464037033035 ) ) ;
#82004=CARTESIAN_POINT ( 'NONE',  ( -8.069080805060693251, -9.172386477786396597, 34.72672124145550043 ) ) ;
#82005=CYLINDRICAL_SURFACE ( 'NONE', #44584, 0.2500000000000004996 ) ;
#82006=VERTEX_POINT ( 'NONE', #72576 ) ;
#82007=ORIENTED_EDGE ( 'NONE', *, *, #2107, .F. ) ;
#82008=CARTESIAN_POINT ( 'NONE',  ( -5.326946301144535489, -12.07920672191015221, 32.31858351112116168 ) ) ;
#82009=CARTESIAN_POINT ( 'NONE',  ( -18.13014796973170206, -10.31621877034669588, 34.18098118002070152 ) ) ;
#82010=EDGE_CURVE ( 'NONE', #28117, #81424, #8821, .T. ) ;
#82011=CARTESIAN_POINT ( 'NONE',  ( -9.561782254074046250, -12.50538340440932394, 31.33453814440721885 ) ) ;
#82012=CARTESIAN_POINT ( 'NONE',  ( 3.361294932532796764, -10.88167719472716399, 33.43325721877153711 ) ) ;
#82013=DIRECTION ( 'NONE',  ( 0.000000000000000000, 0.9848077530122072432, 0.1736481776669354937 ) ) ;
#82014=CARTESIAN_POINT ( 'NONE',  ( 13.38461538461538680, -11.16473453929635440, 33.15142922261926373 ) ) ;
#82015=ORIENTED_EDGE ( 'NONE', *, *, #34225, .T. ) ;
#82016=CARTESIAN_POINT ( 'NONE',  ( 17.07692307692295586, -3.300289026999228437, 32.46337939537709616 ) ) ;
#82017=B_SPLINE_CURVE_WITH_KNOTS ( 'NONE', 3,
 ( #56321, #82142, #22532, #35612, #60967, #77913, #63949, #42377, #2244, #70279 ),
 .UNSPECIFIED., .F., .F.,
 ( 4, 2, 2, 2, 4 ),
 ( 0.0007817246256747444619, 0.0009771112852218868158, 0.001172497944769029061, 0.001367884604316171523, 0.001563271263863313769 ),
 .UNSPECIFIED. ) ;
#82018=CARTESIAN_POINT ( 'NONE',  ( 0.7114839798866018361, -10.05730279482229683, 34.04704008940765902 ) ) ;
#82019=CARTESIAN_POINT ( 'NONE',  ( -9.019207500173124004, -12.17611988154120972, 31.52148481390971213 ) ) ;
#82021=CARTESIAN_POINT ( 'NONE',  ( -7.053767526187231240, -6.369640206132550553, 34.87707690430378449 ) ) ;
#82022=EDGE_LOOP ( 'NONE', ( #35608, #51508 ) ) ;
#82023=ORIENTED_EDGE ( 'NONE', *, *, #80695, .F. ) ;
#82024=AXIS2_PLACEMENT_3D ( 'NONE', #49014, #70173, #27417 ) ;
#82025=AXIS2_PLACEMENT_3D ( 'NONE', #8102, #49528, #35573 ) ;
#82026=ORIENTED_EDGE ( 'NONE', *, *, #61695, .T. ) ;
#82027=CARTESIAN_POINT ( 'NONE',  ( 0.7114839798866025022, -10.76462480002816235, 33.53768742498949962 ) ) ;
#82028=EDGE_CURVE ( 'NONE', #44956, #69684, #76439, .T. ) ;
#82029=ORIENTED_EDGE ( 'NONE', *, *, #56336, .T. ) ;
#82030=CARTESIAN_POINT ( 'NONE',  ( -16.02332045208259359, -5.195472089885680766, 34.18748526763464923 ) ) ;
#82031=CARTESIAN_POINT ( 'NONE',  ( 14.30769230769231015, -5.471508081941601098, 34.59228464037088457 ) ) ;
#82032=CARTESIAN_POINT ( 'NONE',  ( 3.361294669002876656, -5.915461855592777596, 34.75538340440931506 ) ) ;
#82034=DIRECTION ( 'NONE',  ( -0.000000000000000000, -0.3420201433256694901, -0.9396926207859082059 ) ) ;
#82035=ORIENTED_EDGE ( 'NONE', *, *, #3225, .T. ) ;
#82036=CARTESIAN_POINT ( 'NONE',  ( 4.284371855609718338, -4.459921816937789885, 33.71989282347011851 ) ) ;
#82037=CARTESIAN_POINT ( 'NONE',  ( -13.38461538461538325, -4.098570777380720287, 33.41473453929634729 ) ) ;
#82038=ORIENTED_EDGE ( 'NONE', *, *, #28365, .F. ) ;
#82039=FACE_OUTER_BOUND ( 'NONE', #77430, .T. ) ;
#82040=DIRECTION ( 'NONE',  ( -0.000000000000000000, 0.7660444431189791237, -0.6427876096865379196 ) ) ;
#82041=CARTESIAN_POINT ( 'NONE',  ( -11.66915214157184444, -10.70098750199973203, 33.91152734681376302 ) ) ;
#82042=CARTESIAN_POINT ( 'NONE',  ( 11.60452887181161508, -9.905515769479276145, 34.41647553114623292 ) ) ;
#82043=CARTESIAN_POINT ( 'NONE',  ( -12.52680890749923570, -2.892918686051582977, 31.69288490824015980 ) ) ;
#82044=EDGE_CURVE ( 'NONE', #14505, #58651, #41040, .T. ) ;
#82046=CARTESIAN_POINT ( 'NONE',  ( -0.4615384615384611200, -13.87047571288749737, 32.06866353760679544 ) ) ;
#82048=ORIENTED_EDGE ( 'NONE', *, *, #86880, .T. ) ;
#82049=DIRECTION ( 'NONE',  ( -0.000000000000000000, -0.000000000000000000, -1.000000000000000000 ) ) ;
#82050=LINE ( 'NONE', #14021, #39052 ) ;
#82051=CARTESIAN_POINT ( 'NONE',  ( 9.942253101685738059, -10.92531984108285670, 33.72920026020278073 ) ) ;
#82053=ORIENTED_EDGE ( 'NONE', *, *, #70270, .F. ) ;
#82055=CARTESIAN_POINT ( 'NONE',  ( -7.846153846153844924, -10.51840700105979565, 33.73612834413961536 ) ) ;
#82056=B_SPLINE_CURVE_WITH_KNOTS ( 'NONE', 3,
 ( #68585, #34351, #14086, #34794, #14981, #35699, #8223, #577, #82995, #42453 ),
 .UNSPECIFIED., .F., .F.,
 ( 4, 2, 2, 2, 4 ),
 ( 0.0007817246256747528103, 0.0009771112852218978746, 0.001172497944769042939, 0.001367884604316188003, 0.001563271263863333068 ),
 .UNSPECIFIED. ) ;
#82057=B_SPLINE_CURVE_WITH_KNOTS ( 'NONE', 3,
 ( #29280, #30152, #50839, #83337, #21619, #8116 ),
 .UNSPECIFIED., .F., .F.,
 ( 4, 2, 4 ),
 ( 4.563551064100006665E-17, 0.0001954756301637168570, 0.0003909512603273880690 ),
 .UNSPECIFIED. ) ;
#82058=CARTESIAN_POINT ( 'NONE',  ( 2.307692307692186251, -11.06231777344772027, 33.60647404775119895 ) ) ;
#82059=LINE ( 'NONE', #47365, #42789 ) ;
#82060=CARTESIAN_POINT ( 'NONE',  ( 17.86930939688968678, -2.494641256782728966, 31.33461815524612959 ) ) ;
#82061=EDGE_LOOP ( 'NONE', ( #17300, #25167 ) ) ;
#82062=B_SPLINE_CURVE_WITH_KNOTS ( 'NONE', 3,
 ( #13893, #14793, #28290, #21537, #48555, #49889, #84148, #69288, #55761, #22858 ),
 .UNSPECIFIED., .F., .F.,
 ( 4, 2, 2, 2, 4 ),
 ( 0.000000000000000000, 0.0001954339857564081249, 0.0003908679715128162498, 0.0005863019572692244018, 0.0007817359430256324996 ),
 .UNSPECIFIED. ) ;
#82063=DIRECTION ( 'NONE',  ( 1.000000000000000000, 0.000000000000000000, 0.000000000000000000 ) ) ;
#82064=ADVANCED_FACE ( 'NONE', ( #71235 ), #78441, .F. ) ;
#82065=EDGE_CURVE ( 'NONE', #59177, #1945, #13123, .T. ) ;
#82066=LINE ( 'NONE', #67657, #77185 ) ;
#82067=CARTESIAN_POINT ( 'NONE',  ( 5.299935921016468932, -12.38742843783360748, 31.66772728687926985 ) ) ;
#82068=AXIS2_PLACEMENT_3D ( 'NONE', #33182, #60202, #19665 ) ;
#82070=CYLINDRICAL_SURFACE ( 'NONE', #60001, 0.2499999999999986955 ) ;
#82071=ORIENTED_EDGE ( 'NONE', *, *, #56091, .F. ) ;
#82073=CARTESIAN_POINT ( 'NONE',  ( -23.00000000000000000, -12.50000000000000000, 27.25000000000000000 ) ) ;
#82074=ORIENTED_EDGE ( 'NONE', *, *, #23659, .F. ) ;
#82075=CARTESIAN_POINT ( 'NONE',  ( -1.384615384615383471, -5.557115091759785130, 34.35708131394839171 ) ) ;
#82076=CARTESIAN_POINT ( 'NONE',  ( 4.284371592079798674, -9.503571793651733657, 34.60286762892837942 ) ) ;
#82077=CARTESIAN_POINT ( 'NONE',  ( 1.161689167099239750, -4.186968288167446595, 33.49512374952580274 ) ) ;
#82078=FACE_OUTER_BOUND ( 'NONE', #22590, .T. ) ;
#82080=ORIENTED_EDGE ( 'NONE', *, *, #74521, .F. ) ;
#82081=VECTOR ( 'NONE', #54871, 1000.000000000000000 ) ;
#82082=FACE_BOUND ( 'NONE', #6411, .T. ) ;
#82083=ORIENTED_EDGE ( 'NONE', *, *, #37975, .T. ) ;
#82084=DIRECTION ( 'NONE',  ( -0.000000000000000000, -0.9396926207859092051, -0.3420201433256662704 ) ) ;
#82086=CARTESIAN_POINT ( 'NONE',  ( 4.946231610255519051, -11.71456829005830080, 32.44064028649416542 ) ) ;
#82087=CARTESIAN_POINT ( 'NONE',  ( 6.130790440966950250, -5.496552790871117367, 34.60292014791297532 ) ) ;
#82088=CARTESIAN_POINT ( 'NONE',  ( -11.31545018684868964, -2.554770724473667265, 30.48948780036025852 ) ) ;
#82090=ORIENTED_EDGE ( 'NONE', *, *, #3949, .F. ) ;
#82092=ORIENTED_EDGE ( 'NONE', *, *, #42281, .F. ) ;
#82094=CARTESIAN_POINT ( 'NONE',  ( -0.4615384615384611200, -3.050289026998446396, 32.03036669348365706 ) ) ;
#82095=EDGE_LOOP ( 'NONE', ( #24021, #18535 ) ) ;
#82096=CARTESIAN_POINT ( 'NONE',  ( -17.14300545628320904, -9.905515769479276145, 34.41647553114623292 ) ) ;
#82097=CARTESIAN_POINT ( 'NONE',  ( -5.076923076923075762, -12.78798330534102767, 29.49999999999997868 ) ) ;
#82098=FACE_OUTER_BOUND ( 'NONE', #70647, .T. ) ;
#82099=CARTESIAN_POINT ( 'NONE',  ( 17.86930853333243618, -9.804603061927743113, 34.18744698557895845 ) ) ;
#82100=CARTESIAN_POINT ( 'NONE',  ( 5.011653076366756387, -10.33852847137145048, 34.16647553114627556 ) ) ;
#82101=LINE ( 'NONE', #80335, #62324 ) ;
#82102=DIRECTION ( 'NONE',  ( 0.000000000000000000, 0.7660444431189807890, 0.6427876096865361433 ) ) ;
#82103=CARTESIAN_POINT ( 'NONE',  ( 11.47319109250076430, -10.21337939537584383, 33.94971097300158647 ) ) ;
#82104=ORIENTED_EDGE ( 'NONE', *, *, #26002, .T. ) ;
#82105=ORIENTED_EDGE ( 'NONE', *, *, #3536, .F. ) ;
#82106=ORIENTED_EDGE ( 'NONE', *, *, #69996, .F. ) ;
#82107=CARTESIAN_POINT ( 'NONE',  ( -13.51530598772569114, -12.35290016733513951, 31.75349464988449455 ) ) ;
#82109=CARTESIAN_POINT ( 'NONE',  ( -7.846153846153844924, -4.098570777380720287, 33.41473453929634729 ) ) ;
#82110=EDGE_CURVE ( 'NONE', #83962, #30445, #35614, .T. ) ;
#82111=EDGE_CURVE ( 'NONE', #47411, #2090, #81571, .T. ) ;
#82113=FACE_OUTER_BOUND ( 'NONE', #63459, .T. ) ;
#82114=FACE_BOUND ( 'NONE', #59068, .T. ) ;
#82115=CARTESIAN_POINT ( 'NONE',  ( -12.46153846153846168, -12.78798330534103123, 29.99999999999997868 ) ) ;
#82116=VERTEX_POINT ( 'NONE', #39703 ) ;
#82118=DIRECTION ( 'NONE',  ( -0.000000000000000000, 0.6427876096865404731, -0.7660444431189770143 ) ) ;
#82119=CARTESIAN_POINT ( 'NONE',  ( 3.007284287045282500, -10.81261337010820256, 33.49550067578627477 ) ) ;
#82120=VECTOR ( 'NONE', #80931, 1000.000000000000114 ) ;
#82121=ORIENTED_EDGE ( 'NONE', *, *, #10359, .T. ) ;
#82123=ORIENTED_EDGE ( 'NONE', *, *, #49931, .T. ) ;
#82124=FACE_BOUND ( 'NONE', #86570, .T. ) ;
#82125=CARTESIAN_POINT ( 'NONE',  ( 9.468822748583747284, -5.912607949931405926, 34.49155766932282319 ) ) ;
#82126=EDGE_CURVE ( 'NONE', #66604, #33483, #26039, .T. ) ;
#82127=ORIENTED_EDGE ( 'NONE', *, *, #2527, .F. ) ;
#82128=CARTESIAN_POINT ( 'NONE',  ( -8.096153846153855582, -2.249999999999999112, 29.81609741502487765 ) ) ;
#82130=CARTESIAN_POINT ( 'NONE',  ( 1.384615384615265343, -3.300289026999228881, 32.46337939537708905 ) ) ;
#82131=ORIENTED_EDGE ( 'NONE', *, *, #4194, .F. ) ;
#82134=CARTESIAN_POINT ( 'NONE',  ( 14.17754433796061164, -11.66186481527757302, 32.95055677023626117 ) ) ;
#82135=CARTESIAN_POINT ( 'NONE',  ( -16.40382288478850725, -12.41269422305637171, 30.68257228309993323 ) ) ;
#82136=FACE_OUTER_BOUND ( 'NONE', #73493, .T. ) ;
#82137=ORIENTED_EDGE ( 'NONE', *, *, #69009, .F. ) ;
#82138=CARTESIAN_POINT ( 'NONE',  ( -12.46153846153846168, -10.89733346790207413, 36.13435417666054406 ) ) ;
#82139=CARTESIAN_POINT ( 'NONE',  ( 3.903822929624696236, -10.18141759479407327, 34.26406193332782379 ) ) ;
#82140=CARTESIAN_POINT ( 'NONE',  ( 16.08809272553282099, -7.249945578846654470, 34.99404164642496795 ) ) ;
#82141=ORIENTED_EDGE ( 'NONE', *, *, #6305, .F. ) ;
#82142=CARTESIAN_POINT ( 'NONE',  ( -5.011667937410238416, -3.643525952247864463, 33.31231777344670064 ) ) ;
#82143=CARTESIAN_POINT ( 'NONE',  ( 9.442307692307693401, -7.500000000000001776, 35.00000000000000000 ) ) ;
#82144=DIRECTION ( 'NONE',  ( -0.000000000000000000, 0.9396926207859093161, -0.3420201433256663259 ) ) ;
#82145=CARTESIAN_POINT ( 'NONE',  ( 16.15384615384603251, -12.16647553114689728, 32.15551576947799362 ) ) ;
#82146=DIRECTION ( 'NONE',  ( -0.000000000000000000, -0.1736481776669307198, -0.9848077530122080203 ) ) ;
#82147=CARTESIAN_POINT ( 'NONE',  ( 9.915319043920545639, -9.086983370893049639, 34.49168942202179267 ) ) ;
#82149=CARTESIAN_POINT ( 'NONE',  ( -16.21911615440247090, -8.656820664281497102, 34.87096338111211935 ) ) ;
#82151=CARTESIAN_POINT ( 'NONE',  ( -6.857008572074485997, -2.721908614388772296, 31.22303859784725333 ) ) ;
#82153=ORIENTED_EDGE ( 'NONE', *, *, #2696, .T. ) ;
#82154=CARTESIAN_POINT ( 'NONE',  ( -18.00000000000012079, -9.442884908241554243, 34.35708131394783038 ) ) ;
#82155=VERTEX_POINT ( 'NONE', #86559 ) ;
#82156=VECTOR ( 'NONE', #35030, 1000.000000000000000 ) ;
#82157=VERTEX_POINT ( 'NONE', #24829 ) ;
#82158=CARTESIAN_POINT ( 'NONE',  ( 2.307692307692309264, -12.10708131394839349, 31.69288490824020244 ) ) ;
#82159=VERTEX_POINT ( 'NONE', #40147 ) ;
#82160=CARTESIAN_POINT ( 'NONE',  ( 14.08420736396836226, -8.496056993536548418, 34.65000542017679663 ) ) ;
#82162=CARTESIAN_POINT ( 'NONE',  ( 14.53070365930516061, -11.24521262558773493, 33.06293181088029343 ) ) ;
#82163=CARTESIAN_POINT ( 'NONE',  ( -7.912236225513981758, -8.164416787775445883, 34.95778746994557906 ) ) ;
#82164=CARTESIAN_POINT ( 'NONE',  ( 7.780903914379759811, -2.255955759149247619, 30.00000000000013856 ) ) ;
#82165=AXIS2_PLACEMENT_3D ( 'NONE', #5576, #79903, #25850 ) ;
#82166=DIRECTION ( 'NONE',  ( 0.000000000000000000, 0.000000000000000000, 1.000000000000000000 ) ) ;
#82167=CARTESIAN_POINT ( 'NONE',  ( 9.758375025657770152, -12.34228464037088813, 31.77849191805839268 ) ) ;
#82168=CARTESIAN_POINT ( 'NONE',  ( 2.307692307692187583, -11.48612834414049644, 32.76840700105863391 ) ) ;
#82169=CARTESIAN_POINT ( 'NONE',  ( 6.700149964170073247, -12.38737895849757820, 31.66785238281580206 ) ) ;
#82170=CARTESIAN_POINT ( 'NONE',  ( 10.36536137809165403, -2.587272538249754117, 30.68239716806877837 ) ) ;
#82171=CARTESIAN_POINT ( 'NONE',  ( -16.94639763868943660, -11.04252011169590020, 33.62494198852677840 ) ) ;
#82172=EDGE_CURVE ( 'NONE', #76768, #83657, #26172, .T. ) ;
#82173=EDGE_CURVE ( 'NONE', #46391, #58385, #62559, .T. ) ;
#82174=DIRECTION ( 'NONE',  ( 0.000000000000000000, 0.3420201433256610524, 0.9396926207859113145 ) ) ;
#82176=ORIENTED_EDGE ( 'NONE', *, *, #78621, .F. ) ;
#82177=EDGE_CURVE ( 'NONE', #46513, #15704, #21724, .T. ) ;
#82178=CARTESIAN_POINT ( 'NONE',  ( -18.00000000000012079, -2.657715359629662988, 31.77849191805970364 ) ) ;
#82179=CYLINDRICAL_SURFACE ( 'NONE', #7194, 0.2500000000000009437 ) ;
#82180=CARTESIAN_POINT ( 'NONE',  ( -18.00000000000012079, -9.528491918059723176, 34.59228464037033035 ) ) ;
#82181=CARTESIAN_POINT ( 'NONE',  ( -11.28846153846010303, -7.500000000000155431, 34.75000000000007105 ) ) ;
#82182=EDGE_CURVE ( 'NONE', #68899, #71885, #74364, .T. ) ;
#82183=LINE ( 'NONE', #87619, #14709 ) ;
#82186=CYLINDRICAL_SURFACE ( 'NONE', #16364, 0.2499999999999994726 ) ;
#82187=VERTEX_POINT ( 'NONE', #53188 ) ;
#82188=B_SPLINE_CURVE_WITH_KNOTS ( 'NONE', 3,
 ( #84501, #16034, #43504, #70977, #36744, #84945, #78173, #16474, #39429, #46175 ),
 .UNSPECIFIED., .F., .F.,
 ( 4, 2, 2, 2, 4 ),
 ( 0.000000000000000000, 0.0001954311584214072381, 0.0003908623168428144762, 0.0005862934752642217414, 0.0007817246336856289524 ),
 .UNSPECIFIED. ) ;
#82189=CARTESIAN_POINT ( 'NONE',  ( 3.164686851409094892, -6.343179335718451384, 34.87096338111212646 ) ) ;
#82190=ORIENTED_EDGE ( 'NONE', *, *, #67069, .F. ) ;
#82191=CARTESIAN_POINT ( 'NONE',  ( -8.638705330997126453, -5.070358843744210198, 34.40418822224088302 ) ) ;
#82192=LINE ( 'NONE', #14167, #22651 ) ;
#82194=CYLINDRICAL_SURFACE ( 'NONE', #47951, 0.2499999999999995559 ) ;
#82195=CARTESIAN_POINT ( 'NONE',  ( -13.63459212866397507, -2.544273027872575366, 31.48422191005632342 ) ) ;
#82196=ORIENTED_EDGE ( 'NONE', *, *, #38467, .F. ) ;
#82197=ORIENTED_EDGE ( 'NONE', *, *, #30189, .F. ) ;
#82198=EDGE_CURVE ( 'NONE', #63575, #20877, #78673, .T. ) ;
#82199=EDGE_LOOP ( 'NONE', ( #54181, #6608 ) ) ;
#82200=EDGE_LOOP ( 'NONE', ( #79091, #77012, #35837, #58547 ) ) ;
#82201=CARTESIAN_POINT ( 'NONE',  ( -13.38461538461550582, -6.879047030192662504, 34.71129190930017927 ) ) ;
#82202=CARTESIAN_POINT ( 'NONE',  ( -2.557715531913763662, -10.18141759479407327, 34.26406193332782379 ) ) ;
#82203=CARTESIAN_POINT ( 'NONE',  ( 14.30769230769218581, -2.657715359629662544, 31.77849191805970364 ) ) ;
#82204=VECTOR ( 'NONE', #88025, 1000.000000000000000 ) ;
#82206=CARTESIAN_POINT ( 'NONE',  ( 17.86930939688968678, -2.845849958028613624, 32.17971566917920967 ) ) ;
#82207=CARTESIAN_POINT ( 'NONE',  ( 12.33139049180676494, -3.069018819979302926, 32.56621877034667278 ) ) ;
#82208=ORIENTED_EDGE ( 'NONE', *, *, #15042, .T. ) ;
#82209=ORIENTED_EDGE ( 'NONE', *, *, #41968, .T. ) ;
#82210=AXIS2_PLACEMENT_3D ( 'NONE', #82545, #20821, #29366 ) ;
#82211=EDGE_CURVE ( 'NONE', #37942, #84770, #1309, .T. ) ;
#82212=B_SPLINE_CURVE_WITH_KNOTS ( 'NONE', 3,
 ( #51216, #72401, #85049, #23326, #78270, #16573, #44037, #23763, #30532, #85484 ),
 .UNSPECIFIED., .F., .F.,
 ( 4, 2, 2, 2, 4 ),
 ( 0.000000000000000000, 0.0001954339857564080165, 0.0003908679715128160329, 0.0005863019572692240765, 0.0007817359430256320659 ),
 .UNSPECIFIED. ) ;
#82213=ORIENTED_EDGE ( 'NONE', *, *, #35388, .T. ) ;
#82214=CARTESIAN_POINT ( 'NONE',  ( -3.230769230769229949, -2.486705287966279876, 31.30864560766543647 ) ) ;
#82215=ORIENTED_EDGE ( 'NONE', *, *, #52831, .T. ) ;
#82216=FACE_OUTER_BOUND ( 'NONE', #7209, .T. ) ;
#82217=CARTESIAN_POINT ( 'NONE',  ( -16.15384615384615330, -13.20930481340135110, 34.54067556320372745 ) ) ;
#82219=EDGE_LOOP ( 'NONE', ( #49413, #66449, #67173, #24700 ) ) ;
#82220=CARTESIAN_POINT ( 'NONE',  ( -1.161602540521988747, -2.523321265292116422, 31.42251411153756990 ) ) ;
#82222=CARTESIAN_POINT ( 'NONE',  ( 2.084766090176162212, -6.503392248772476236, 34.64988816332204635 ) ) ;
#82223=FACE_BOUND ( 'NONE', #3338, .T. ) ;
#82224=FACE_OUTER_BOUND ( 'NONE', #75272, .T. ) ;
#82225=ADVANCED_FACE ( 'NONE', ( #48650 ), #477, .F. ) ;
#82226=DIRECTION ( 'NONE',  ( -0.000000000000000000, -0.6427876096865404731, -0.7660444431189770143 ) ) ;
#82227=ORIENTED_EDGE ( 'NONE', *, *, #65816, .T. ) ;
#82230=EDGE_CURVE ( 'NONE', #58112, #60787, #81880, .T. ) ;
#82231=CARTESIAN_POINT ( 'NONE',  ( 16.40390057375961064, -6.523592122091590895, 34.90882529074906415 ) ) ;
#82232=FACE_OUTER_BOUND ( 'NONE', #28273, .T. ) ;
#82233=EDGE_LOOP ( 'NONE', ( #453, #85843 ) ) ;
#82234=VECTOR ( 'NONE', #31706, 1000.000000000000114 ) ;
#82236=DIRECTION ( 'NONE',  ( -0.000000000000000000, -0.000000000000000000, -1.000000000000000000 ) ) ;
#82237=CARTESIAN_POINT ( 'NONE',  ( 17.32686859527121825, -10.05730279482229683, 34.04704008940765902 ) ) ;
#82238=CARTESIAN_POINT ( 'NONE',  ( -10.61538461538473577, -8.656820664282941280, 34.87096338111179961 ) ) ;
#82239=DIRECTION ( 'NONE',  ( 1.000000000000000000, 0.000000000000000000, 0.000000000000000000 ) ) ;
#82240=FACE_BOUND ( 'NONE', #53614, .T. ) ;
#82241=CARTESIAN_POINT ( 'NONE',  ( 13.31853300525524908, -11.91647553114624181, 32.58852847137148245 ) ) ;
#82242=CARTESIAN_POINT ( 'NONE',  ( 16.85343815235874132, -3.019605429927187501, 32.48692288466676814 ) ) ;
#82244=CARTESIAN_POINT ( 'NONE',  ( -6.988347369037699153, -12.27809138561121394, 31.22303859784730307 ) ) ;
#82245=CARTESIAN_POINT ( 'NONE',  ( 3.007890548340584225, -7.630691491037286056, 34.74850469731152458 ) ) ;
#82248=CARTESIAN_POINT ( 'NONE',  ( -8.069638770718176701, -4.225889041578353655, 33.85425143139329407 ) ) ;
#82251=CARTESIAN_POINT ( 'NONE',  ( 1.319344938654611221, -12.27809138561121394, 31.22303859784730307 ) ) ;
#82252=VERTEX_POINT ( 'NONE', #88785 ) ;
#82253=B_SPLINE_CURVE_WITH_KNOTS ( 'NONE', 3,
 ( #65868, #4173, #86618, #73082, #66325, #4625, #80294, #6837, #55467, #34308 ),
 .UNSPECIFIED., .F., .F.,
 ( 4, 2, 2, 2, 4 ),
 ( 0.0007817359527651098448, 0.0009771254036996487088, 0.001172514854634187573, 0.001367904305568726220, 0.001563293756503265084 ),
 .UNSPECIFIED. ) ;
#82255=CARTESIAN_POINT ( 'NONE',  ( -15.10024352900566846, -4.459921816937791661, 33.71989282347011851 ) ) ;
#82257=DIRECTION ( 'NONE',  ( 0.000000000000000000, 0.1736481776669275834, 0.9848077530122086864 ) ) ;
#82258=CARTESIAN_POINT ( 'NONE',  ( 14.08476534878545827, -4.026226216239094491, 33.68668979543634379 ) ) ;
#82259=EDGE_CURVE ( 'NONE', #47287, #67226, #49096, .T. ) ;
#82260=DIRECTION ( 'NONE',  ( -0.000000000000000000, -0.8660254037844397068, -0.4999999999999978906 ) ) ;
#82261=ORIENTED_EDGE ( 'NONE', *, *, #51056, .F. ) ;
#82262=CARTESIAN_POINT ( 'NONE',  ( 5.076923076923075762, -11.91647553114624181, 32.58852847137148245 ) ) ;
#82264=CARTESIAN_POINT ( 'NONE',  ( -15.29685161012936589, -9.058645607665454236, 34.76329471203372634 ) ) ;
#82267=DIRECTION ( 'NONE',  ( -0.000000000000000000, -0.8660254037844397068, -0.4999999999999978906 ) ) ;
#82268=CARTESIAN_POINT ( 'NONE',  ( -1.254089946381739651, -6.808710257144161559, 34.95449254468098843 ) ) ;
#82269=CARTESIAN_POINT ( 'NONE',  ( 11.53846153846153832, -3.513871655860378418, 32.76840700105978499 ) ) ;
#82271=B_SPLINE_CURVE_WITH_KNOTS ( 'NONE', 3,
 ( #13339, #73731, #74604, #80025, #53883, #19217, #25965, #33170, #60632, #4366 ),
 .UNSPECIFIED., .F., .F.,
 ( 4, 2, 2, 2, 4 ),
 ( 0.0007817246336856291692, 0.0009771112958940105907, 0.001172497958102391904, 0.001367884620310773434, 0.001563271282519154747 ),
 .UNSPECIFIED. ) ;
#82272=DIRECTION ( 'NONE',  ( -0.000000000000000000, -0.9848077530122086864, -0.1736481776669273613 ) ) ;
#82273=CARTESIAN_POINT ( 'NONE',  ( -4.403869378067608586, -2.985938066672154445, 32.43141759479405550 ) ) ;
#82274=EDGE_CURVE ( 'NONE', #62624, #75979, #4507, .T. ) ;
#82275=ORIENTED_EDGE ( 'NONE', *, *, #22673, .T. ) ;
#82276=LINE ( 'NONE', #54786, #32086 ) ;
#82280=DIRECTION ( 'NONE',  ( -0.000000000000000000, -0.6427876096865404731, -0.7660444431189771253 ) ) ;
#82282=ORIENTED_EDGE ( 'NONE', *, *, #67981, .F. ) ;
#82283=CARTESIAN_POINT ( 'NONE',  ( -17.07692307692307665, -5.415277668671390821, 36.20867863119892149 ) ) ;
#82284=CARTESIAN_POINT ( 'NONE',  ( 3.164685819813350953, -3.513871655860377086, 32.76840700105978499 ) ) ;
#82285=CYLINDRICAL_SURFACE ( 'NONE', #13816, 0.2499999999999986955 ) ;
#82286=EDGE_LOOP ( 'NONE', ( #12616, #58167, #51394, #9557 ) ) ;
#82287=CARTESIAN_POINT ( 'NONE',  ( 8.639082799499069765, -5.915902021225889484, 34.75552854090298638 ) ) ;
#82288=EDGE_CURVE ( 'NONE', #77995, #25963, #82462, .T. ) ;
#82289=CARTESIAN_POINT ( 'NONE',  ( -16.82692307692300915, -7.434744860731433924, 35.00000000000000711 ) ) ;
#82291=CARTESIAN_POINT ( 'NONE',  ( 13.38461538461538680, -12.78798330534102767, 29.49999999999997868 ) ) ;
#82292=CARTESIAN_POINT ( 'NONE',  ( -9.469294848214296678, -2.523321265292115534, 31.42251411153756990 ) ) ;
#82293=CARTESIAN_POINT ( 'NONE',  ( -15.45425415533356173, -11.60425143139329940, 33.02411095842164457 ) ) ;
#82294=ORIENTED_EDGE ( 'NONE', *, *, #58679, .T. ) ;
#82295=B_SPLINE_CURVE_WITH_KNOTS ( 'NONE', 3,
 ( #81516, #26567, #54467, #6299, #7624, #62118, #54022, #89169, #48151, #62545 ),
 .UNSPECIFIED., .F., .F.,
 ( 4, 2, 2, 2, 4 ),
 ( 0.0007817246336856291692, 0.0009771112958940105907, 0.001172497958102391904, 0.001367884620310773434, 0.001563271282519154747 ),
 .UNSPECIFIED. ) ;
#82296=EDGE_CURVE ( 'NONE', #76455, #88588, #41842, .T. ) ;
#82297=VERTEX_POINT ( 'NONE', #75252 ) ;
#82298=ORIENTED_EDGE ( 'NONE', *, *, #11451, .F. ) ;
#82300=CARTESIAN_POINT ( 'NONE',  ( 0.2386122440223120422, -2.554751324335733820, 30.48935550225260727 ) ) ;
#82301=EDGE_CURVE ( 'NONE', #83936, #77943, #13984, .T. ) ;
#82302=CARTESIAN_POINT ( 'NONE',  ( -13.31935981333935892, -12.27809138561124591, 31.22303859784720359 ) ) ;
#82303=DIRECTION ( 'NONE',  ( 0.000000000000000000, 0.4999999999999985567, 0.8660254037844395958 ) ) ;
#82304=DIRECTION ( 'NONE',  ( 0.000000000000000000, 0.3420201433256610524, 0.9396926207859113145 ) ) ;
#82305=VECTOR ( 'NONE', #17094, 1000.000000000000227 ) ;
#82306=ORIENTED_EDGE ( 'NONE', *, *, #74588, .T. ) ;
#82307=EDGE_CURVE ( 'NONE', #2112, #71085, #61716, .T. ) ;
#82308=ORIENTED_EDGE ( 'NONE', *, *, #2639, .T. ) ;
#82309=ORIENTED_EDGE ( 'NONE', *, *, #65973, .F. ) ;
#82310=CARTESIAN_POINT ( 'NONE',  ( -6.988346923633242724, -8.656820664281497102, 34.87096338111211935 ) ) ;
#82311=VERTEX_POINT ( 'NONE', #41462 ) ;
#82312=CARTESIAN_POINT ( 'NONE',  ( -1.384615384615506484, -3.083524468854526912, 32.58852847137268327 ) ) ;
#82313=VECTOR ( 'NONE', #58438, 999.9999999999998863 ) ;
#82314=EDGE_CURVE ( 'NONE', #86754, #67131, #68923, .T. ) ;
#82316=EDGE_CURVE ( 'NONE', #7820, #88099, #61446, .T. ) ;
#82318=CARTESIAN_POINT ( 'NONE',  ( 15.23076923076923173, -12.37446782046654192, 30.86335684631486131 ) ) ;
#82319=ORIENTED_EDGE ( 'NONE', *, *, #76997, .T. ) ;
#82320=EDGE_LOOP ( 'NONE', ( #65104, #75424, #14575, #48495 ) ) ;
#82321=EDGE_CURVE ( 'NONE', #67169, #54354, #15184, .T. ) ;
#82322=ORIENTED_EDGE ( 'NONE', *, *, #63659, .F. ) ;
#82323=CARTESIAN_POINT ( 'NONE',  ( 10.86533013373275836, -10.76462480002816235, 33.53768742498949962 ) ) ;
#82324=CARTESIAN_POINT ( 'NONE',  ( -11.53846153846153655, -10.89733346790207413, 36.13435417666054406 ) ) ;
#82325=ORIENTED_EDGE ( 'NONE', *, *, #77908, .T. ) ;
#82328=EDGE_LOOP ( 'NONE', ( #77702, #25343, #15789, #1455 ) ) ;
#82331=EDGE_LOOP ( 'NONE', ( #22017, #43359, #13740, #14320 ) ) ;
#82332=FACE_BOUND ( 'NONE', #60072, .T. ) ;
#82333=CARTESIAN_POINT ( 'NONE',  ( 1.384615384615386802, -3.322132147404559976, 32.92929555188717927 ) ) ;
#82336=DIRECTION ( 'NONE',  ( -0.000000000000000000, -0.1736481776669307198, -0.9848077530122080203 ) ) ;
#82337=CARTESIAN_POINT ( 'NONE',  ( -7.173076923076920686, -7.566083408709834757, 34.74999999999999289 ) ) ;
#82338=CARTESIAN_POINT ( 'NONE',  ( 4.826946345980721809, -9.943427161483782584, 34.11278801902876978 ) ) ;
#82339=VECTOR ( 'NONE', #88742, 1000.000000000000227 ) ;
#82340=CARTESIAN_POINT ( 'NONE',  ( -3.931066612577743147, -2.847695495035524882, 31.58253572463339509 ) ) ;
#82341=CARTESIAN_POINT ( 'NONE',  ( 13.38461538461538680, -12.09954503811598769, 35.62045528018868623 ) ) ;
#82343=CARTESIAN_POINT ( 'NONE',  ( -18.22292621751614305, -10.61292498521070549, 33.66303323003028680 ) ) ;
#82344=CYLINDRICAL_SURFACE ( 'NONE', #11945, 0.2500000000000009437 ) ;
#82345=EDGE_CURVE ( 'NONE', #53520, #23339, #46463, .T. ) ;
#82346=ORIENTED_EDGE ( 'NONE', *, *, #78343, .F. ) ;
#82347=VECTOR ( 'NONE', #81846, 1000.000000000000000 ) ;
#82348=CARTESIAN_POINT ( 'NONE',  ( -14.17716686945866655, -9.503571793651731880, 34.60286762892837942 ) ) ;
#82350=VERTEX_POINT ( 'NONE', #16634 ) ;
#82351=CARTESIAN_POINT ( 'NONE',  ( -9.692307692307814193, -2.657715359629662544, 31.77849191805970364 ) ) ;
#82352=CARTESIAN_POINT ( 'NONE',  ( 6.856994543716785628, -8.164416787775445883, 34.95778746994557906 ) ) ;
#82353=FACE_BOUND ( 'NONE', #68423, .T. ) ;
#82354=DIRECTION ( 'NONE',  ( -1.000000000000000000, 0.000000000000000000, 0.000000000000000000 ) ) ;
#82355=CARTESIAN_POINT ( 'NONE',  ( -16.82686876528476105, -12.41262288849542017, 30.68299917996395010 ) ) ;
#82356=CARTESIAN_POINT ( 'NONE',  ( 2.241609928332172874, -6.343179335718451384, 34.87096338111212646 ) ) ;
#82357=B_SPLINE_CURVE_WITH_KNOTS ( 'NONE', 3,
 ( #4151, #52339, #3707, #85256, #44235, #45141, #11364, #73067, #18574, #78929 ),
 .UNSPECIFIED., .F., .F.,
 ( 4, 2, 2, 2, 4 ),
 ( 0.0007817246256747451124, 0.0009771112852218883336, 0.001172497944769031663, 0.001367884604316174993, 0.001563271263863318323 ),
 .UNSPECIFIED. ) ;
#82358=CARTESIAN_POINT ( 'NONE',  ( 1.384615384615264011, -12.70778746994576025, 30.41441678777401236 ) ) ;
#82360=CARTESIAN_POINT ( 'NONE',  ( 2.057715563643718326, -10.82459398097509684, 33.81372124010185587 ) ) ;
#82362=EDGE_LOOP ( 'NONE', ( #68369, #73038, #45695, #56909 ) ) ;
#82363=B_SPLINE_CURVE_WITH_KNOTS ( 'NONE', 3,
 ( #58748, #86696, #79476, #43898, #11457, #64599, #32176, #38488, #85340, #17775 ),
 .UNSPECIFIED., .F., .F.,
 ( 4, 2, 2, 2, 4 ),
 ( 0.000000000000000000, 0.0001954311564186887718, 0.0003908623128373775435, 0.0005862934692560662882, 0.0007817246256747550871 ),
 .UNSPECIFIED. ) ;
#82365=DIRECTION ( 'NONE',  ( -0.000000000000000000, 0.8660254037844397068, -0.4999999999999978906 ) ) ;
#82366=DIRECTION ( 'NONE',  ( 0.000000000000000000, -6.938893903907222067E-15, 1.000000000000000000 ) ) ;
#82367=CARTESIAN_POINT ( 'NONE',  ( 1.449870524128225036, -9.528491918058460186, 34.59228464037085615 ) ) ;
#82368=CARTESIAN_POINT ( 'NONE',  ( 8.769230769230768274, -11.35647404775217417, 33.31231777344666511 ) ) ;
#82369=CARTESIAN_POINT ( 'NONE',  ( -14.98071491913091613, -2.779044189368095275, 31.39831045268885745 ) ) ;
#82371=FACE_OUTER_BOUND ( 'NONE', #49165, .T. ) ;
#82372=CARTESIAN_POINT ( 'NONE',  ( 1.134638640566794754, -10.06842814019191401, 34.32929386961144758 ) ) ;
#82373=CARTESIAN_POINT ( 'NONE',  ( 9.627037691751372250, -11.06231777344662781, 33.60647404775220082 ) ) ;
#82376=LINE ( 'NONE', #35060, #75647 ) ;
#82378=CARTESIAN_POINT ( 'NONE',  ( -0.2115930521604180437, -4.176053281294514363, 33.81426240980091791 ) ) ;
#82379=CYLINDRICAL_SURFACE ( 'NONE', #46278, 0.2499999999999998890 ) ;
#82380=EDGE_CURVE ( 'NONE', #126, #14193, #24912, .T. ) ;
#82381=CARTESIAN_POINT ( 'NONE',  ( -3.230769230769229949, -9.780366693483667717, 34.19971097300155094 ) ) ;
#82382=ORIENTED_EDGE ( 'NONE', *, *, #78422, .F. ) ;
#82383=CARTESIAN_POINT ( 'NONE',  ( -0.3962828902624361826, -3.835265460703683349, 33.15142922261929925 ) ) ;
#82384=CARTESIAN_POINT ( 'NONE',  ( 0.5276068125409003606, -2.538708090699994813, 30.37095296980875503 ) ) ;
#82386=EDGE_CURVE ( 'NONE', #82533, #74234, #83964, .T. ) ;
#82387=DIRECTION ( 'NONE',  ( -0.000000000000000000, -0.6427876096865404731, -0.7660444431189771253 ) ) ;
#82388=DIRECTION ( 'NONE',  ( -0.000000000000000000, 0.3420201433256694346, -0.9396926207859080948 ) ) ;
#82389=DIRECTION ( 'NONE',  ( -0.000000000000000000, -0.5000000000000009992, -0.8660254037844380415 ) ) ;
#82390=CARTESIAN_POINT ( 'NONE',  ( -14.05769230769230660, -2.249999999999998668, 29.75000000000000355 ) ) ;
#82391=ORIENTED_EDGE ( 'NONE', *, *, #3436, .T. ) ;
#82393=CARTESIAN_POINT ( 'NONE',  ( 16.85343815235874132, -2.612411019501191589, 31.66733052389440672 ) ) ;
#82395=ORIENTED_EDGE ( 'NONE', *, *, #13097, .F. ) ;
#82396=CARTESIAN_POINT ( 'NONE',  ( -15.93106661257773915, -10.11255958852955672, 34.01340905677048454 ) ) ;
#82397=B_SPLINE_CURVE_WITH_KNOTS ( 'NONE', 3,
 ( #73180, #52000, #86716, #24982, #25433, #11477, #79935, #45698, #17340, #87600 ),
 .UNSPECIFIED., .F., .F.,
 ( 4, 2, 2, 2, 4 ),
 ( 0.0007817359430256297891, 0.0009771253907249961065, 0.001172514838424362424, 0.001367904286123728741, 0.001563293733823095059 ),
 .UNSPECIFIED. ) ;
#82398=B_SPLINE_CURVE_WITH_KNOTS ( 'NONE', 3,
 ( #47957, #14176, #69124, #62352, #28130, #224, #13735, #42108, #67797, #68675 ),
 .UNSPECIFIED., .F., .F.,
 ( 4, 2, 2, 2, 4 ),
 ( 0.000000000000000000, 0.0001954339857564093175, 0.0003908679715128186350, 0.0005863019572692279796, 0.0007817359430256372700 ),
 .UNSPECIFIED. ) ;
#82399=CARTESIAN_POINT ( 'NONE',  ( -2.307692307692305711, -10.67929555188718282, 33.92786785259544047 ) ) ;
#82400=EDGE_CURVE ( 'NONE', #88629, #38816, #58062, .T. ) ;
#82401=VERTEX_POINT ( 'NONE', #78779 ) ;
#82403=B_SPLINE_CURVE_WITH_KNOTS ( 'NONE', 3,
 ( #70486, #51068, #1137, #84017, #22296, #84896, #70036, #49760, #63717, #29506 ),
 .UNSPECIFIED., .F., .F.,
 ( 4, 2, 2, 2, 4 ),
 ( 0.0007817359430256320659, 0.0009771253907249987086, 0.001172514838424365460, 0.001367904286123731994, 0.001563293733823098745 ),
 .UNSPECIFIED. ) ;
#82405=CARTESIAN_POINT ( 'NONE',  ( -15.10024352900566846, -12.45806712695776319, 30.39783852428763922 ) ) ;
#82406=VERTEX_POINT ( 'NONE', #31029 ) ;
#82407=ORIENTED_EDGE ( 'NONE', *, *, #73936, .F. ) ;
#82408=EDGE_CURVE ( 'NONE', #57426, #54624, #63931, .T. ) ;
#82409=FACE_OUTER_BOUND ( 'NONE', #1328, .T. ) ;
#82411=VERTEX_POINT ( 'NONE', #10774 ) ;
#82412=AXIS2_PLACEMENT_3D ( 'NONE', #883, #1323, #29254 ) ;
#82413=CARTESIAN_POINT ( 'NONE',  ( 7.596177102105253987, -9.234221910056348293, 34.70572697212741531 ) ) ;
#82414=CARTESIAN_POINT ( 'NONE',  ( 5.076923076923075762, -4.661471528628507777, 34.16647553114623292 ) ) ;
#82415=CARTESIAN_POINT ( 'NONE',  ( -10.83831083290076158, -2.554751324335734708, 30.48935550225260727 ) ) ;
#82416=CYLINDRICAL_SURFACE ( 'NONE', #4510, 0.2499999999999986955 ) ;
#82417=LINE ( 'NONE', #9724, #7639 ) ;
#82418=DIRECTION ( 'NONE',  ( -0.000000000000000000, -0.7660444431189791237, -0.6427876096865379196 ) ) ;
#82420=CARTESIAN_POINT ( 'NONE',  ( 16.15384615384603251, -12.70778746994576025, 30.41441678777401236 ) ) ;
#82421=EDGE_LOOP ( 'NONE', ( #51882, #40747 ) ) ;
#82423=CARTESIAN_POINT ( 'NONE',  ( 12.46153846153833911, -12.16647553114689728, 32.15551576947799362 ) ) ;
#82424=ORIENTED_EDGE ( 'NONE', *, *, #56783, .F. ) ;
#82425=EDGE_CURVE ( 'NONE', #4955, #42964, #81023, .T. ) ;
#82426=CYLINDRICAL_SURFACE ( 'NONE', #79624, 0.2500000000000012212 ) ;
#82427=B_SPLINE_CURVE_WITH_KNOTS ( 'NONE', 3,
 ( #58772, #2930, #3381, #24540, #70960, #36295, #63752, #43926, #36728, #2054 ),
 .UNSPECIFIED., .F., .F.,
 ( 4, 2, 2, 2, 4 ),
 ( 0.000000000000000000, 0.0001954311564186870913, 0.0003908623128373741825, 0.0005862934692560613009, 0.0007817246256747483650 ),
 .UNSPECIFIED. ) ;
#82428=B_SPLINE_CURVE_WITH_KNOTS ( 'NONE', 3,
 ( #30811, #58728, #85327, #16417, #29498, #77669, #85771, #23172, #45212, #72690 ),
 .UNSPECIFIED., .F., .F.,
 ( 4, 2, 2, 2, 4 ),
 ( 0.000000000000000000, 0.0001954339857564073659, 0.0003908679715128147319, 0.0005863019572692221250, 0.0007817359430256294638 ),
 .UNSPECIFIED. ) ;
#82429=B_SPLINE_CURVE_WITH_KNOTS ( 'NONE', 3,
 ( #51987, #38045, #71369, #24519, #43465, #85797, #9251, #58303, #37143, #2465 ),
 .UNSPECIFIED., .F., .F.,
 ( 4, 2, 2, 2, 4 ),
 ( 0.0007817246256747493408, 0.0009771112852218933210, 0.001172497944769037301, 0.001367884604316181281, 0.001563271263863325261 ),
 .UNSPECIFIED. ) ;
#82430=CARTESIAN_POINT ( 'NONE',  ( -10.61538461538473399, -4.481592998941358097, 33.73612834414048933 ) ) ;
#82431=FACE_BOUND ( 'NONE', #54968, .T. ) ;
#82432=ORIENTED_EDGE ( 'NONE', *, *, #37501, .T. ) ;
#82433=B_SPLINE_CURVE_WITH_KNOTS ( 'NONE', 3,
 ( #45337, #18324, #11572, #66049, #38144, #72810, #71925, #39051, #11118, #66510 ),
 .UNSPECIFIED., .F., .F.,
 ( 4, 2, 2, 2, 4 ),
 ( 0.000000000000000000, 0.0001954339857564055499, 0.0003908679715128110998, 0.0005863019572692165955, 0.0007817359430256221996 ),
 .UNSPECIFIED. ) ;
#82434=CYLINDRICAL_SURFACE ( 'NONE', #32672, 0.2500000000000008882 ) ;
#82435=EDGE_CURVE ( 'NONE', #36751, #30821, #3379, .T. ) ;
#82440=CARTESIAN_POINT ( 'NONE',  ( -12.52762084089859407, -3.322132147404559532, 32.92929555188719348 ) ) ;
#82441=ORIENTED_EDGE ( 'NONE', *, *, #20514, .T. ) ;
#82442=EDGE_CURVE ( 'NONE', #18050, #45619, #39150, .T. ) ;
#82443=CARTESIAN_POINT ( 'NONE',  ( -4.403822897894744237, -4.075325502946086864, 33.72974371597207721 ) ) ;
#82444=CARTESIAN_POINT ( 'NONE',  ( -4.219928533206288357, -6.343179335718451384, 34.87096338111212646 ) ) ;
#82445=FACE_BOUND ( 'NONE', #88809, .T. ) ;
#82446=FACE_OUTER_BOUND ( 'NONE', #77606, .T. ) ;
#82447=CARTESIAN_POINT ( 'NONE',  ( -17.75005448165185840, -12.22109172314383052, 31.39792113162168263 ) ) ;
#82448=CARTESIAN_POINT ( 'NONE',  ( 15.29602437028207085, -2.657715359629132301, 31.77849191805844242 ) ) ;
#82449=DIRECTION ( 'NONE',  ( -0.000000000000000000, 0.9396926207859092051, -0.3420201433256662704 ) ) ;
#82451=CARTESIAN_POINT ( 'NONE',  ( -4.153846153846152411, -11.16473453929635440, 33.15142922261926373 ) ) ;
#82452=CARTESIAN_POINT ( 'NONE',  ( -6.222865422203639696, -2.501496062324911840, 29.88072118266895671 ) ) ;
#82454=EDGE_CURVE ( 'NONE', #81338, #25143, #12555, .T. ) ;
#82455=ORIENTED_EDGE ( 'NONE', *, *, #1700, .F. ) ;
#82456=CARTESIAN_POINT ( 'NONE',  ( -16.94639737515951694, -10.19071101563364401, 33.96452234770658407 ) ) ;
#82457=CARTESIAN_POINT ( 'NONE',  ( 15.23076923076923173, -12.10708131394839349, 31.69288490824020244 ) ) ;
#82458=CARTESIAN_POINT ( 'NONE',  ( -18.00000000000000000, -4.098570777380720287, 33.41473453929634729 ) ) ;
#82459=CARTESIAN_POINT ( 'NONE',  ( 8.769230769230768274, -13.63283147151868846, 33.57946703557072254 ) ) ;
#82461=CARTESIAN_POINT ( 'NONE',  ( -13.38461538461538325, -5.471508081941601098, 34.59228464037088457 ) ) ;
#82462=LINE ( 'NONE', #68482, #33219 ) ;
#82463=EDGE_CURVE ( 'NONE', #14282, #34190, #37846, .T. ) ;
#82464=ORIENTED_EDGE ( 'NONE', *, *, #12308, .T. ) ;
#82465=DIRECTION ( 'NONE',  ( -0.000000000000000000, -0.5000000000000009992, -0.8660254037844380415 ) ) ;
#82466=CARTESIAN_POINT ( 'NONE',  ( -14.30769230769230660, -2.721908614388771852, 31.22303859784724978 ) ) ;
#82467=CARTESIAN_POINT ( 'NONE',  ( -8.769230769230768274, -12.10708131394839349, 31.69288490824020244 ) ) ;
#82468=CARTESIAN_POINT ( 'NONE',  ( -15.93083330975275302, -4.026326845037968560, 33.68677907613345468 ) ) ;
#82469=VERTEX_POINT ( 'NONE', #87343 ) ;
#82470=EDGE_CURVE ( 'NONE', #47021, #11337, #73365, .T. ) ;
#82471=EDGE_LOOP ( 'NONE', ( #43500, #24385 ) ) ;
#82472=CIRCLE ( 'NONE', #43615, 0.2500000000000002220 ) ;
#82473=VERTEX_POINT ( 'NONE', #26067 ) ;
#82474=AXIS2_PLACEMENT_3D ( 'NONE', #2633, #30122, #57589 ) ;
#82475=CARTESIAN_POINT ( 'NONE',  ( 0.6845498131513105822, -10.61302985866383963, 33.66295027996417843 ) ) ;
#82476=ORIENTED_EDGE ( 'NONE', *, *, #31584, .T. ) ;
#82477=CARTESIAN_POINT ( 'NONE',  ( -9.915792636031639518, -12.44517049084099725, 30.48991314939691932 ) ) ;
#82478=DIRECTION ( 'NONE',  ( -0.000000000000000000, 0.8660254037844397068, -0.4999999999999978906 ) ) ;
#82479=LINE ( 'NONE', #75697, #85502 ) ;
#82480=CARTESIAN_POINT ( 'NONE',  ( 11.53846153846153832, -3.513871655860378418, 32.76840700105978499 ) ) ;
#82481=VECTOR ( 'NONE', #51304, 1000.000000000000000 ) ;
#82482=CARTESIAN_POINT ( 'NONE',  ( 2.307692307692309264, -5.180354513474913603, 36.12317359536750416 ) ) ;
#82483=VERTEX_POINT ( 'NONE', #38689 ) ;
#82484=CARTESIAN_POINT ( 'NONE',  ( -11.28846153846147438, -7.434744860731433924, 35.00000000000000711 ) ) ;
#82485=CARTESIAN_POINT ( 'NONE',  ( 7.846153846153846700, -2.249999999999998668, 29.75000000000001776 ) ) ;
#82486=ORIENTED_EDGE ( 'NONE', *, *, #16962, .F. ) ;
#82488=CARTESIAN_POINT ( 'NONE',  ( 15.23076923076910916, -2.657715359629662544, 31.77849191805970364 ) ) ;
#82489=CARTESIAN_POINT ( 'NONE',  ( 17.20744877868663281, -11.46989282347013095, 32.79007818306219946 ) ) ;
#82490=CARTESIAN_POINT ( 'NONE',  ( -16.37672567058374185, -7.630690623152299956, 34.99857592706774057 ) ) ;
#82491=CARTESIAN_POINT ( 'NONE',  ( 3.230769230769231726, -5.180354513474913603, 36.12317359536750416 ) ) ;
#82496=FACE_OUTER_BOUND ( 'NONE', #78269, .T. ) ;
#82497=DIRECTION ( 'NONE',  ( -0.000000000000000000, 0.3420201433256694901, -0.9396926207859082059 ) ) ;
#82498=EDGE_CURVE ( 'NONE', #81338, #42788, #52659, .T. ) ;
#82499=B_SPLINE_CURVE_WITH_KNOTS ( 'NONE', 3,
 ( #57400, #63714, #37125, #37570, #2020, #29941, #84013, #43887, #15099, #76803 ),
 .UNSPECIFIED., .F., .F.,
 ( 4, 2, 2, 2, 4 ),
 ( 0.0007817359430256327164, 0.0009771253907249993591, 0.001172514838424366110, 0.001367904286123732861, 0.001563293733823099396 ),
 .UNSPECIFIED. ) ;
#82501=CARTESIAN_POINT ( 'NONE',  ( -13.16160403300253634, -8.239487800360276282, 34.69522927552633718 ) ) ;
#82503=CARTESIAN_POINT ( 'NONE',  ( 14.30769230769231015, -3.886160181151819604, 36.00935417666054406 ) ) ;
#82504=CARTESIAN_POINT ( 'NONE',  ( -3.007757879156380820, -5.667800583137508674, 34.40243808032445827 ) ) ;
#82506=AXIS2_PLACEMENT_3D ( 'NONE', #88463, #6901, #26733 ) ;
#82507=CARTESIAN_POINT ( 'NONE',  ( -0.5922290646487686772, -10.70098750199973203, 33.91152734681376302 ) ) ;
#82508=EDGE_CURVE ( 'NONE', #79011, #35777, #46335, .T. ) ;
#82510=CARTESIAN_POINT ( 'NONE',  ( 17.07692307692307665, -2.517432740324522911, 35.29906147534542527 ) ) ;
#82511=ORIENTED_EDGE ( 'NONE', *, *, #24338, .T. ) ;
#82512=CARTESIAN_POINT ( 'NONE',  ( -12.33074665371366940, -8.999086150933475636, 34.52020707165672775 ) ) ;
#82513=CARTESIAN_POINT ( 'NONE',  ( -5.999999999999998224, -1.790695186598648903, 34.54067556320373455 ) ) ;
#82514=CARTESIAN_POINT ( 'NONE',  ( 5.326977496836529546, -12.41089969410671223, 31.60739465890703670 ) ) ;
#82515=ORIENTED_EDGE ( 'NONE', *, *, #33726, .F. ) ;
#82516=ADVANCED_FACE ( 'NONE', ( #73820 ), #72914, .F. ) ;
#82517=DIRECTION ( 'NONE',  ( -0.000000000000000000, -0.7660444431189791237, -0.6427876096865379196 ) ) ;
#82518=ORIENTED_EDGE ( 'NONE', *, *, #77814, .T. ) ;
#82519=LINE ( 'NONE', #43723, #75922 ) ;
#82520=CARTESIAN_POINT ( 'NONE',  ( -5.869474561766356402, -12.15418822224088657, 32.17964115625579069 ) ) ;
#82522=CARTESIAN_POINT ( 'NONE',  ( 7.596130608860881317, -12.22074536777954989, 31.39888409691088356 ) ) ;
#82523=FACE_OUTER_BOUND ( 'NONE', #72190, .T. ) ;
#82524=CARTESIAN_POINT ( 'NONE',  ( -6.673022503163469565, -12.41089969410671223, 31.60739465890703670 ) ) ;
#82526=CARTESIAN_POINT ( 'NONE',  ( -7.976301815885541657, -5.070767119584671079, 34.40440758774516183 ) ) ;
#82527=CARTESIAN_POINT ( 'NONE',  ( -1.634592128663974853, -10.82459398097509684, 33.81372124010185587 ) ) ;
#82528=B_SPLINE_CURVE_WITH_KNOTS ( 'NONE', 3,
 ( #1683, #84990, #56627, #84113, #22394, #36360 ),
 .UNSPECIFIED., .F., .F.,
 ( 4, 2, 4 ),
 ( 4.593128804320400861E-17, 0.0001954756301637176972, 0.0003909512603273894243 ),
 .UNSPECIFIED. ) ;
#82530=VECTOR ( 'NONE', #24472, 1000.000000000000114 ) ;
#82531=ORIENTED_EDGE ( 'NONE', *, *, #70751, .F. ) ;
#82532=FACE_BOUND ( 'NONE', #15067, .T. ) ;
#82533=VERTEX_POINT ( 'NONE', #60284 ) ;
#82535=EDGE_CURVE ( 'NONE', #4425, #61846, #48095, .T. ) ;
#82536=VECTOR ( 'NONE', #66758, 1000.000000000000227 ) ;
#82537=CARTESIAN_POINT ( 'NONE',  ( 18.24994540937804643, -6.653508905675593610, 34.93172785388651391 ) ) ;
#82538=ADVANCED_FACE ( 'NONE', ( #61167 ), #40911, .F. ) ;
#82539=CARTESIAN_POINT ( 'NONE',  ( 8.769230769230768274, -3.513871655860378418, 32.76840700105978499 ) ) ;
#82540=CARTESIAN_POINT ( 'NONE',  ( 14.53047197667037338, -8.540255544307065350, 34.89611431652622286 ) ) ;
#82541=ORIENTED_EDGE ( 'NONE', *, *, #20266, .F. ) ;
#82542=EDGE_LOOP ( 'NONE', ( #63262, #71347, #71285, #20666 ) ) ;
#82543=EDGE_LOOP ( 'NONE', ( #28686, #6515, #66418, #70019 ) ) ;
#82544=B_SPLINE_CURVE_WITH_KNOTS ( 'NONE', 3,
 ( #65498, #48998, #35486, #64596, #812, #78566, #2894, #23622, #30385, #43895 ),
 .UNSPECIFIED., .F., .F.,
 ( 4, 2, 2, 2, 4 ),
 ( 0.0007817359430256317406, 0.0009771253907249982749, 0.001172514838424365026, 0.001367904286123731560, 0.001563293733823098094 ),
 .UNSPECIFIED. ) ;
#82545=CARTESIAN_POINT ( 'NONE',  ( -15.23076923076922995, -8.564572088678739092, 35.78748833219616898 ) ) ;
#82546=ORIENTED_EDGE ( 'NONE', *, *, #74787, .T. ) ;
#82547=EDGE_CURVE ( 'NONE', #16511, #6173, #21516, .T. ) ;
#82548=EDGE_CURVE ( 'NONE', #61048, #37230, #50590, .T. ) ;
#82549=CARTESIAN_POINT ( 'NONE',  ( 14.98074600654777377, -3.520140089381495585, 33.17453946501458262 ) ) ;
#82550=CARTESIAN_POINT ( 'NONE',  ( 1.384615384615265343, -3.835265460704628371, 33.15142922262033665 ) ) ;
#82551=CARTESIAN_POINT ( 'NONE',  ( 18.00000000000000000, -8.164416787775445883, 34.95778746994557906 ) ) ;
#82552=CARTESIAN_POINT ( 'NONE',  ( 3.296024370282069960, -9.528491918058460186, 34.59228464037085615 ) ) ;
#82554=CARTESIAN_POINT ( 'NONE',  ( 15.36129493253279499, -9.417988943895561960, 34.36773134775777550 ) ) ;
#82555=DIRECTION ( 'NONE',  ( -0.000000000000000000, -0.6427876096865404731, -0.7660444431189770143 ) ) ;
#82556=CARTESIAN_POINT ( 'NONE',  ( -5.142193522883852452, -3.835265460703609186, 33.15142922261924241 ) ) ;
#82557=VERTEX_POINT ( 'NONE', #88678 ) ;
#82558=B_SPLINE_CURVE_WITH_KNOTS ( 'NONE', 3,
 ( #82992, #84333, #57284, #69029, #28489, #43332, #35239, #14527, #1462, #49642 ),
 .UNSPECIFIED., .F., .F.,
 ( 4, 2, 2, 2, 4 ),
 ( 0.0007817246256747477145, 0.0009771112852218909357, 0.001172497944769034265, 0.001367884604316177595, 0.001563271263863320708 ),
 .UNSPECIFIED. ) ;
#82559=ORIENTED_EDGE ( 'NONE', *, *, #23589, .T. ) ;
#82560=EDGE_CURVE ( 'NONE', #8100, #79207, #21064, .T. ) ;
#82561=EDGE_LOOP ( 'NONE', ( #64489, #5349 ) ) ;
#82562=CARTESIAN_POINT ( 'NONE',  ( 3.930361229281820190, -3.019605429927184836, 32.48692288466676814 ) ) ;
#82563=B_SPLINE_CURVE_WITH_KNOTS ( 'NONE', 3,
 ( #32449, #24345, #59916, #46408, #73888, #51807, #67132, #37873, #5429, #32894 ),
 .UNSPECIFIED., .F., .F.,
 ( 4, 2, 2, 2, 4 ),
 ( 0.0007817246256747491240, 0.0009771112852218931041, 0.001172497944769036867, 0.001367884604316180631, 0.001563271263863324611 ),
 .UNSPECIFIED. ) ;
#82564=CARTESIAN_POINT ( 'NONE',  ( 14.30769230769231015, -2.499999999999998668, 29.75000000000001421 ) ) ;
#82565=CARTESIAN_POINT ( 'NONE',  ( -9.942330916529147800, -4.175268141568685643, 33.81360843649122216 ) ) ;
#82566=FACE_OUTER_BOUND ( 'NONE', #49245, .T. ) ;
#82567=CARTESIAN_POINT ( 'NONE',  ( -9.915233909823838232, -6.503392248772476236, 34.64988816332204635 ) ) ;
#82568=EDGE_CURVE ( 'NONE', #56880, #2574, #5459, .T. ) ;
#82569=FACE_BOUND ( 'NONE', #85695, .T. ) ;
#82570=CARTESIAN_POINT ( 'NONE',  ( 16.37662569511456567, -3.236590943229497697, 32.36255958852954251 ) ) ;
#82572=ORIENTED_EDGE ( 'NONE', *, *, #82826, .T. ) ;
#82573=LINE ( 'NONE', #44869, #57445 ) ;
#82574=FACE_OUTER_BOUND ( 'NONE', #12007, .T. ) ;
#82575=CYLINDRICAL_SURFACE ( 'NONE', #52476, 0.2499999999999986955 ) ;
#82576=ORIENTED_EDGE ( 'NONE', *, *, #46169, .F. ) ;
#82577=CARTESIAN_POINT ( 'NONE',  ( 4.946232473812767871, -12.62707690430377383, 30.88035979386743435 ) ) ;
#82578=ORIENTED_EDGE ( 'NONE', *, *, #60133, .T. ) ;
#82579=FACE_BOUND ( 'NONE', #38865, .T. ) ;
#82580=CARTESIAN_POINT ( 'NONE',  ( -12.46153846153846168, -13.63283147151868846, 33.57946703557072254 ) ) ;
#82581=DIRECTION ( 'NONE',  ( -0.000000000000000000, 0.8660254037844399289, -0.4999999999999980016 ) ) ;
#82582=CARTESIAN_POINT ( 'NONE',  ( 16.85343815235874132, -12.11044203135681840, 32.26167407432752299 ) ) ;
#82585=CARTESIAN_POINT ( 'NONE',  ( 14.30769230769218758, -8.613356846316285953, 34.62446782046622218 ) ) ;
#82587=CARTESIAN_POINT ( 'NONE',  ( 5.999999999999880096, -3.835265460704628371, 33.15142922262033665 ) ) ;
#82589=CARTESIAN_POINT ( 'NONE',  ( -12.39547011053602432, -3.050289026998446840, 32.03036669348366416 ) ) ;
#82591=CARTESIAN_POINT ( 'NONE',  ( -15.23076923076922995, -2.292212530054420494, 30.41441678777542634 ) ) ;
#82592=EDGE_LOOP ( 'NONE', ( #71180, #82707, #19481, #17302 ) ) ;
#82593=LINE ( 'NONE', #19982, #45466 ) ;
#82595=CARTESIAN_POINT ( 'NONE',  ( -4.826977558574935934, -8.433404298154334455, 34.66254593164985920 ) ) ;
#82596=CARTESIAN_POINT ( 'NONE',  ( -8.769230769230890843, -11.48612834414049644, 32.76840700105863391 ) ) ;
#82597=CARTESIAN_POINT ( 'NONE',  ( 9.823099500132483897, -8.999086150933475636, 34.52020707165672775 ) ) ;
#82598=CARTESIAN_POINT ( 'NONE',  ( -5.776987155906603277, -6.460100341425561332, 34.89618726649961644 ) ) ;
#82599=VECTOR ( 'NONE', #25483, 1000.000000000000114 ) ;
#82600=CARTESIAN_POINT ( 'NONE',  ( -2.438252899434225629, -2.504760397472875155, 29.97295953869789997 ) ) ;
#82601=CARTESIAN_POINT ( 'NONE',  ( -10.61538461538473399, -2.892918686052166066, 31.69288490824153470 ) ) ;
#82602=B_SPLINE_CURVE_WITH_KNOTS ( 'NONE', 3,
 ( #29603, #78217, #70585, #51162, #15645, #43985, #16519, #71904, #57061, #43113 ),
 .UNSPECIFIED., .F., .F.,
 ( 4, 2, 2, 2, 4 ),
 ( 0.000000000000000000, 0.0001954311564186862781, 0.0003908623128373725562, 0.0005862934692560588072, 0.0007817246256747451124 ),
 .UNSPECIFIED. ) ;
#82605=ORIENTED_EDGE ( 'NONE', *, *, #17590, .F. ) ;
#82606=B_SPLINE_CURVE_WITH_KNOTS ( 'NONE', 3,
 ( #212, #66895, #61019, #47053, #81748, #27676, #74541, #49719, #77634, #62774 ),
 .UNSPECIFIED., .F., .F.,
 ( 4, 2, 2, 2, 4 ),
 ( 0.0007817246256747484735, 0.0009771112852218915863, 0.001172497944769034916, 0.001367884604316178029, 0.001563271263863321141 ),
 .UNSPECIFIED. ) ;
#82609=EDGE_LOOP ( 'NONE', ( #58572, #77767 ) ) ;
#82610=AXIS2_PLACEMENT_3D ( 'NONE', #44078, #9864, #64353 ) ;
#82611=ORIENTED_EDGE ( 'NONE', *, *, #72300, .T. ) ;
#82612=CARTESIAN_POINT ( 'NONE',  ( -11.40793610022789828, -2.372941743896879174, 30.88044141588253666 ) ) ;
#82613=VERTEX_POINT ( 'NONE', #48534 ) ;
#82614=CARTESIAN_POINT ( 'NONE',  ( -4.376773112753000738, -2.523278758544489797, 31.42238647778637528 ) ) ;
#82616=CARTESIAN_POINT ( 'NONE',  ( 12.39578503322513114, -7.249945578846651806, 34.99404164642496795 ) ) ;
#82617=B_SPLINE_CURVE_WITH_KNOTS ( 'NONE', 3,
 ( #12933, #33207, #52578, #26454, #79620, #18365, #74195, #4398, #67439, #59787 ),
 .UNSPECIFIED., .F., .F.,
 ( 4, 2, 2, 2, 4 ),
 ( 0.000000000000000000, 0.0001954311564186861697, 0.0003908623128373723394, 0.0005862934692560584820, 0.0007817246256747446788 ),
 .UNSPECIFIED. ) ;
#82618=CYLINDRICAL_SURFACE ( 'NONE', #66896, 0.2500000000000012212 ) ;
#82619=CARTESIAN_POINT ( 'NONE',  ( 3.100622021331010281, -8.587444163452046197, 34.63053765926554206 ) ) ;
#82620=LINE ( 'NONE', #55122, #1532 ) ;
#82621=CARTESIAN_POINT ( 'NONE',  ( -15.45425415533356350, -4.988325925672468131, 34.36044203135681130 ) ) ;
#82622=CARTESIAN_POINT ( 'NONE',  ( -11.78843826940389583, -4.943428324936578910, 34.04746400365624481 ) ) ;
#82623=CARTESIAN_POINT ( 'NONE',  ( -4.153846153846152411, -3.513871655860378418, 32.76840700105978499 ) ) ;
#82624=DIRECTION ( 'NONE',  ( 0.000000000000000000, 0.9848077530122072432, -0.1736481776669354937 ) ) ;
#82625=LINE ( 'NONE', #75846, #67878 ) ;
#82626=CARTESIAN_POINT ( 'NONE',  ( 5.076923076923075762, -10.67929555188718282, 33.92786785259544047 ) ) ;
#82627=CARTESIAN_POINT ( 'NONE',  ( -9.915234651214539952, -11.43668979543635089, 33.22377378376089752 ) ) ;
#82628=ORIENTED_EDGE ( 'NONE', *, *, #52930, .F. ) ;
#82629=EDGE_LOOP ( 'NONE', ( #19651, #54794, #60447, #22572 ) ) ;
#82630=CARTESIAN_POINT ( 'NONE',  ( -15.23076923076922995, -8.120952969808772792, 34.71129190930000163 ) ) ;
#82631=CARTESIAN_POINT ( 'NONE',  ( 1.634560793993429906, -3.520799739797214389, 33.17531984108286025 ) ) ;
#82632=DIRECTION ( 'NONE',  ( -0.000000000000000000, -0.1736481776669307198, -0.9848077530122080203 ) ) ;
#82633=CARTESIAN_POINT ( 'NONE',  ( 5.776515056276054771, -5.912607949931405038, 34.49155766932282319 ) ) ;
#82634=CARTESIAN_POINT ( 'NONE',  ( -16.15384615384627409, -8.656820664282941280, 34.87096338111179961 ) ) ;
#82635=CARTESIAN_POINT ( 'NONE',  ( 11.76124120743960333, -4.226511098958373402, 33.85474049983370293 ) ) ;
#82636=VECTOR ( 'NONE', #27717, 999.9999999999998863 ) ;
#82639=CARTESIAN_POINT ( 'NONE',  ( -14.30769230769242917, -12.70778746994576025, 30.41441678777401236 ) ) ;
#82640=EDGE_LOOP ( 'NONE', ( #10724, #85205, #23125, #19479 ) ) ;
#82641=B_SPLINE_CURVE_WITH_KNOTS ( 'NONE', 3,
 ( #67303, #80382, #6489, #33950, #46581, #74497, #32619, #81266, #39834, #75386 ),
 .UNSPECIFIED., .F., .F.,
 ( 4, 2, 2, 2, 4 ),
 ( 0.0007817359430256252354, 0.0009771253907249898181, 0.001172514838424354401, 0.001367904286123718983, 0.001563293733823083566 ),
 .UNSPECIFIED. ) ;
#82644=CARTESIAN_POINT ( 'NONE',  ( 8.899756207464411872, -9.503571793651731880, 34.60286762892837942 ) ) ;
#82645=DIRECTION ( 'NONE',  ( -0.000000000000000000, 1.000000000000000000, -0.000000000000000000 ) ) ;
#82646=DIRECTION ( 'NONE',  ( -0.000000000000000000, 0.1736481776669307198, -0.9848077530122080203 ) ) ;
#82647=DIRECTION ( 'NONE',  ( -0.000000000000000000, -0.000000000000000000, -1.000000000000000000 ) ) ;
#82648=ORIENTED_EDGE ( 'NONE', *, *, #255, .F. ) ;
#82649=VERTEX_POINT ( 'NONE', #81910 ) ;
#82650=ORIENTED_EDGE ( 'NONE', *, *, #36649, .T. ) ;
#82652=VECTOR ( 'NONE', #75141, 1000.000000000000114 ) ;
#82653=EDGE_CURVE ( 'NONE', #14193, #126, #75328, .T. ) ;
#82654=CARTESIAN_POINT ( 'NONE',  ( 13.16113044089144068, -3.236172620538810385, 32.36188796281390267 ) ) ;
#82655=DIRECTION ( 'NONE',  ( -0.000000000000000000, 0.9848077530122085754, -0.1736481776669273613 ) ) ;
#82657=AXIS2_PLACEMENT_3D ( 'NONE', #30006, #63782, #57466 ) ;
#82659=CARTESIAN_POINT ( 'NONE',  ( -14.30769230769230660, -2.833524468853757305, 32.15551576947925838 ) ) ;
#82660=CARTESIAN_POINT ( 'NONE',  ( -17.86947429823644029, -4.459921816937791661, 33.71989282347011851 ) ) ;
#82661=CARTESIAN_POINT ( 'NONE',  ( 14.17754509825408960, -12.45813303252208648, 30.39737893381572675 ) ) ;
#82662=ORIENTED_EDGE ( 'NONE', *, *, #82535, .T. ) ;
#82663=EDGE_LOOP ( 'NONE', ( #71642, #13520, #34322, #65109 ) ) ;
#82664=VERTEX_POINT ( 'NONE', #68819 ) ;
#82665=CARTESIAN_POINT ( 'NONE',  ( 16.15384615384615330, -12.29105614889573062, 35.45975837776705220 ) ) ;
#82666=EDGE_LOOP ( 'NONE', ( #58465, #55285 ) ) ;
#82667=B_SPLINE_CURVE_WITH_KNOTS ( 'NONE', 3,
 ( #33262, #5343, #39137, #54405, #66602, #4905, #32369, #39589, #47204, #25609 ),
 .UNSPECIFIED., .F., .F.,
 ( 4, 2, 2, 2, 4 ),
 ( 0.000000000000000000, 0.0001954339857564058752, 0.0003908679715128117503, 0.0005863019572692176797, 0.0007817359430256235007 ),
 .UNSPECIFIED. ) ;
#82668=CARTESIAN_POINT ( 'NONE',  ( 9.627037691751372250, -8.656820664281498878, 34.87096338111211935 ) ) ;
#82669=CYLINDRICAL_SURFACE ( 'NONE', #18712, 0.2499999999999997502 ) ;
#82672=EDGE_LOOP ( 'NONE', ( #55550, #38103, #27513, #16572 ) ) ;
#82675=FACE_BOUND ( 'NONE', #6008, .T. ) ;
#82676=CARTESIAN_POINT ( 'NONE',  ( -5.777220331021934996, -3.020022701398814569, 32.48759521482552515 ) ) ;
#82677=EDGE_CURVE ( 'NONE', #41163, #83846, #57073, .T. ) ;
#82679=EDGE_LOOP ( 'NONE', ( #83119, #1438 ) ) ;
#82680=LINE ( 'NONE', #7003, #51839 ) ;
#82681=LINE ( 'NONE', #20951, #55057 ) ;
#82682=CYLINDRICAL_SURFACE ( 'NONE', #38533, 0.2499999999999986955 ) ;
#82684=ORIENTED_EDGE ( 'NONE', *, *, #50036, .F. ) ;
#82686=CARTESIAN_POINT ( 'NONE',  ( -11.47320639894870276, -12.51329471203373700, 31.30864560766537963 ) ) ;
#82687=CARTESIAN_POINT ( 'NONE',  ( 1.384615384615265343, -8.613356846316285953, 34.62446782046622218 ) ) ;
#82688=CARTESIAN_POINT ( 'NONE',  ( -12.46153846153846168, -12.10708131394839349, 31.69288490824020244 ) ) ;
#82690=CARTESIAN_POINT ( 'NONE',  ( 7.846153846153846700, -6.189225973068211317, 35.74407628777942847 ) ) ;
#82691=FACE_BOUND ( 'NONE', #85837, .T. ) ;
#82692=DIRECTION ( 'NONE',  ( -0.000000000000000000, 0.5000000000000011102, -0.8660254037844380415 ) ) ;
#82693=CYLINDRICAL_SURFACE ( 'NONE', #41703, 0.2500000000000002220 ) ;
#82694=CARTESIAN_POINT ( 'NONE',  ( 11.60452887181161508, -11.91647553114624358, 32.58852847137148245 ) ) ;
#82696=CARTESIAN_POINT ( 'NONE',  ( 5.749976762707035505, -10.76384336483936011, 33.53834819971076087 ) ) ;
#82697=CARTESIAN_POINT ( 'NONE',  ( -10.74607521849492464, -6.369640206132551441, 34.87707690430378449 ) ) ;
#82699=EDGE_LOOP ( 'NONE', ( #59380, #55717, #5262, #7943, #12324, #60633, #17161, #9581 ) ) ;
#82700=CARTESIAN_POINT ( 'NONE',  ( 12.68454981315131036, -2.554770724473668153, 30.48948780036025852 ) ) ;
#82701=EDGE_LOOP ( 'NONE', ( #21508, #2018 ) ) ;
#82702=CARTESIAN_POINT ( 'NONE',  ( -13.16160254052199008, -10.77377354290276124, 33.85451476688484718 ) ) ;
#82703=EDGE_LOOP ( 'NONE', ( #28605, #67115, #51053, #19355, #7200, #18496 ) ) ;
#82704=CYLINDRICAL_SURFACE ( 'NONE', #38383, 0.2499999999999995559 ) ;
#82705=CARTESIAN_POINT ( 'NONE',  ( -7.912237257109724808, -9.780366693483667717, 34.19971097300155805 ) ) ;
#82707=ORIENTED_EDGE ( 'NONE', *, *, #31916, .T. ) ;
#82708=CARTESIAN_POINT ( 'NONE',  ( -15.23076923076935252, -10.33852847137269571, 34.16647553114546554 ) ) ;
#82710=CARTESIAN_POINT ( 'NONE',  ( 0.4615384615384611200, -1.790695186598648903, 34.54067556320373455 ) ) ;
#82711=CARTESIAN_POINT ( 'NONE',  ( -6.923076923077045919, -12.70778746994576025, 30.41441678777401236 ) ) ;
#82712=CARTESIAN_POINT ( 'NONE',  ( 12.23805351781451556, -2.847400154188068022, 31.58180166144859058 ) ) ;
#82713=CARTESIAN_POINT ( 'NONE',  ( 10.61538461538449418, -2.657715359629662544, 31.77849191805970364 ) ) ;
#82714=LINE ( 'NONE', #48913, #49691 ) ;
#82717=CARTESIAN_POINT ( 'NONE',  ( -10.39260507411620438, -2.847695495035523550, 31.58253572463339154 ) ) ;
#82718=CARTESIAN_POINT ( 'NONE',  ( -6.000000000000121680, -3.643525952248796163, 33.31231777344771672 ) ) ;
#82719=ORIENTED_EDGE ( 'NONE', *, *, #20068, .T. ) ;
#82722=AXIS2_PLACEMENT_3D ( 'NONE', #45562, #73042, #11338 ) ;
#82723=DIRECTION ( 'NONE',  ( -0.000000000000000000, 0.7660444431189791237, -0.6427876096865379196 ) ) ;
#82725=EDGE_LOOP ( 'NONE', ( #87830, #25245, #18718, #24977 ) ) ;
#82726=CARTESIAN_POINT ( 'NONE',  ( 1.634560793993429906, -8.476813868363244353, 34.90874843262270133 ) ) ;
#82728=CARTESIAN_POINT ( 'NONE',  ( 2.084207363968362259, -2.847400154188067578, 31.58180166144859768 ) ) ;
#82729=VERTEX_POINT ( 'NONE', #15657 ) ;
#82730=CARTESIAN_POINT ( 'NONE',  ( -5.300408020647025431, -5.912607949931405038, 34.49155766932282319 ) ) ;
#82731=B_SPLINE_CURVE_WITH_KNOTS ( 'NONE', 3,
 ( #78102, #45650, #73126, #37551, #66368, #16402, #43870, #9639, #37107, #78540 ),
 .UNSPECIFIED., .F., .F.,
 ( 4, 2, 2, 2, 4 ),
 ( 0.0007817246256747445703, 0.0009771112852218872494, 0.001172497944769030145, 0.001367884604316172825, 0.001563271263863315504 ),
 .UNSPECIFIED. ) ;
#82732=CARTESIAN_POINT ( 'NONE',  ( -17.32692307692307665, -7.500000000000001776, 35.00000000000000000 ) ) ;
#82733=EDGE_CURVE ( 'NONE', #49839, #16707, #21969, .T. ) ;
#82734=CARTESIAN_POINT ( 'NONE',  ( -10.48485917715097138, -9.503571793651731880, 34.60286762892837942 ) ) ;
#82735=CARTESIAN_POINT ( 'NONE',  ( -16.94613126909829504, -2.729792928343270031, 31.24908615093345432 ) ) ;
#82736=LINE ( 'NONE', #21010, #27928 ) ;
#82738=VERTEX_POINT ( 'NONE', #2129 ) ;
#82739=ORIENTED_EDGE ( 'NONE', *, *, #43998, .F. ) ;
#82740=EDGE_CURVE ( 'NONE', #54936, #74567, #9774, .T. ) ;
#82741=CARTESIAN_POINT ( 'NONE',  ( -9.692307692307812417, -3.300289026999228881, 32.46337939537708905 ) ) ;
#82743=EDGE_CURVE ( 'NONE', #22897, #58039, #27002, .T. ) ;
#82744=CARTESIAN_POINT ( 'NONE',  ( 9.915319043920545639, -4.887748414852792322, 34.01359900205216746 ) ) ;
#82745=CARTESIAN_POINT ( 'NONE',  ( -8.096130590202434973, -10.82459398097509329, 33.81372124010185587 ) ) ;
#82746=VECTOR ( 'NONE', #56220, 1000.000000000000227 ) ;
#82747=ORIENTED_EDGE ( 'NONE', *, *, #41131, .T. ) ;
#82748=CARTESIAN_POINT ( 'NONE',  ( -17.14300648787895653, -4.098570777380720287, 33.41473453929634729 ) ) ;
#82749=EDGE_LOOP ( 'NONE', ( #9830, #69417, #35345, #28689 ) ) ;
#82750=ORIENTED_EDGE ( 'NONE', *, *, #20600, .T. ) ;
#82752=VERTEX_POINT ( 'NONE', #70595 ) ;
#82753=DIRECTION ( 'NONE',  ( 0.000000000000000000, 0.8660254037844377084, -0.5000000000000015543 ) ) ;
#82754=ORIENTED_EDGE ( 'NONE', *, *, #34977, .T. ) ;
#82756=B_SPLINE_CURVE_WITH_KNOTS ( 'NONE', 3,
 ( #82858, #35096, #76081, #49052, #56258, #33776, #55366, #88738, #62130, #1307 ),
 .UNSPECIFIED., .F., .F.,
 ( 4, 2, 2, 2, 4 ),
 ( 0.000000000000000000, 0.0001954339857564077183, 0.0003908679715128154366, 0.0005863019572692231007, 0.0007817359430256308733 ),
 .UNSPECIFIED. ) ;
#82757=CARTESIAN_POINT ( 'NONE',  ( 5.777073041093152561, -12.64616026154729411, 30.79003144601913533 ) ) ;
#82758=ADVANCED_FACE ( 'NONE', ( #57518 ), #85004, .F. ) ;
#82759=CARTESIAN_POINT ( 'NONE',  ( -9.822454901745912181, -8.587444163452046197, 34.63053765926554206 ) ) ;
#82760=CARTESIAN_POINT ( 'NONE',  ( -3.903791733932699515, -6.523592122091591783, 34.90882529074906415 ) ) ;
#82761=VERTEX_POINT ( 'NONE', #76912 ) ;
#82763=VERTEX_POINT ( 'NONE', #71034 ) ;
#82764=LINE ( 'NONE', #8427, #53334 ) ;
#82765=DIRECTION ( 'NONE',  ( -1.000000000000000000, 0.000000000000000000, 0.000000000000000000 ) ) ;
#82766=EDGE_LOOP ( 'NONE', ( #25247, #13551, #49705, #81514 ) ) ;
#82767=CARTESIAN_POINT ( 'NONE',  ( -2.177166605928743781, -8.586989748646452369, 34.63063291749215011 ) ) ;
#82768=VECTOR ( 'NONE', #32714, 999.9999999999998863 ) ;
#82769=CARTESIAN_POINT ( 'NONE',  ( -0.5916864312701572981, -6.809168938359898782, 34.95455904226513866 ) ) ;
#82770=EDGE_CURVE ( 'NONE', #60559, #48169, #30053, .T. ) ;
#82771=ORIENTED_EDGE ( 'NONE', *, *, #41527, .F. ) ;
#82772=EDGE_CURVE ( 'NONE', #13992, #54951, #37659, .T. ) ;
#82773=CARTESIAN_POINT ( 'NONE',  ( 13.38461538461538680, -4.786620604624113540, 33.94971097300155094 ) ) ;
#82774=DIRECTION ( 'NONE',  ( 0.000000000000000000, 0.8660254037844377084, 0.5000000000000015543 ) ) ;
#82775=ORIENTED_EDGE ( 'NONE', *, *, #27727, .F. ) ;
#82776=FACE_BOUND ( 'NONE', #64455, .T. ) ;
#82777=B_SPLINE_CURVE_WITH_KNOTS ( 'NONE', 3,
 ( #65632, #53460, #25997, #73761, #12055, #32318, #80962, #59780, #25555, #25108 ),
 .UNSPECIFIED., .F., .F.,
 ( 4, 2, 2, 2, 4 ),
 ( 0.0007817246256747507503, 0.0009771112852218957062, 0.001172497944769040771, 0.001367884604316185835, 0.001563271263863330682 ),
 .UNSPECIFIED. ) ;
#82779=LINE ( 'NONE', #42237, #48546 ) ;
#82780=DIRECTION ( 'NONE',  ( -0.000000000000000000, 0.5000000000000011102, -0.8660254037844381525 ) ) ;
#82781=CARTESIAN_POINT ( 'NONE',  ( 10.86538461538605205, -7.500000000000155431, 34.75000000000007105 ) ) ;
#82782=CARTESIAN_POINT ( 'NONE',  ( -0.5916856709766853406, -12.27039167877662251, 31.24851455888617835 ) ) ;
#82784=CARTESIAN_POINT ( 'NONE',  ( -10.61538461538461320, -1.790695186598648903, 34.54067556320373455 ) ) ;
#82785=CARTESIAN_POINT ( 'NONE',  ( -4.153846153846274980, -11.06231777344772027, 33.60647404775119895 ) ) ;
#82786=VERTEX_POINT ( 'NONE', #36804 ) ;
#82787=EDGE_CURVE ( 'NONE', #14363, #35493, #50745, .T. ) ;
#82790=DIRECTION ( 'NONE',  ( -0.000000000000000000, 0.9848077530122086864, -0.1736481776669273891 ) ) ;
#82792=DIRECTION ( 'NONE',  ( -0.000000000000000000, 0.6427876096865404731, -0.7660444431189771253 ) ) ;
#82794=CARTESIAN_POINT ( 'NONE',  ( 11.31497661389721010, -10.23692288466677880, 34.23039457007281072 ) ) ;
#82795=DIRECTION ( 'NONE',  ( -0.000000000000000000, -0.7660444431189791237, -0.6427876096865379196 ) ) ;
#82796=FACE_BOUND ( 'NONE', #26138, .T. ) ;
#82797=B_SPLINE_CURVE_WITH_KNOTS ( 'NONE', 3,
 ( #56392, #8654, #49631, #35688, #2314, #48294, #69900, #42000, #7764, #69459 ),
 .UNSPECIFIED., .F., .F.,
 ( 4, 2, 2, 2, 4 ),
 ( 0.000000000000000000, 0.0001954339857564089651, 0.0003908679715128179303, 0.0005863019572692268954, 0.0007817359430256358606 ),
 .UNSPECIFIED. ) ;
#82798=DIRECTION ( 'NONE',  ( -0.000000000000000000, -0.6427876096865404731, -0.7660444431189770143 ) ) ;
#82799=CARTESIAN_POINT ( 'NONE',  ( -4.023320452082589149, -8.586989748646452369, 34.63063291749215011 ) ) ;
#82801=CARTESIAN_POINT ( 'NONE',  ( 17.99999999999987566, -10.90142922262034020, 33.41473453929536674 ) ) ;
#82803=DIRECTION ( 'NONE',  ( -0.000000000000000000, 0.7660444431189791237, -0.6427876096865379196 ) ) ;
#82804=CARTESIAN_POINT ( 'NONE',  ( -14.05774689831426372, -5.766571408460171355, 34.70601412856602508 ) ) ;
#82806=ORIENTED_EDGE ( 'NONE', *, *, #22369, .F. ) ;
#82807=B_SPLINE_CURVE_WITH_KNOTS ( 'NONE', 3,
 ( #14233, #42600, #69178, #55214, #718, #7922, #75934, #21876, #27304, #88591 ),
 .UNSPECIFIED., .F., .F.,
 ( 4, 2, 2, 2, 4 ),
 ( 0.0007817246256747474977, 0.0009771112852218911526, 0.001172497944769034699, 0.001367884604316178462, 0.001563271263863322009 ),
 .UNSPECIFIED. ) ;
#82809=CARTESIAN_POINT ( 'NONE',  ( -9.692307692307691624, -11.69971097300155272, 32.46337939537588113 ) ) ;
#82810=DIRECTION ( 'NONE',  ( -0.000000000000000000, 1.000000000000000000, 3.491481338843133355E-15 ) ) ;
#82811=CARTESIAN_POINT ( 'NONE',  ( 6.673076923076926015, -7.433932668274256805, 35.00000000000000711 ) ) ;
#82812=CARTESIAN_POINT ( 'NONE',  ( 18.00000000000000000, -11.33034616979429110, 35.88435417666054406 ) ) ;
#82813=CARTESIAN_POINT ( 'NONE',  ( -16.15384615384615330, -12.10708131394839349, 31.69288490824020244 ) ) ;
#82815=CARTESIAN_POINT ( 'NONE',  ( -16.15384615384627409, -5.941354392335915335, 34.76329471203413846 ) ) ;
#82816=CARTESIAN_POINT ( 'NONE',  ( 2.307692307692309264, -6.435427911321262684, 35.78748833219616898 ) ) ;
#82817=CARTESIAN_POINT ( 'NONE',  ( 15.29683758177167086, -11.69971097300155272, 32.46337939537588113 ) ) ;
#82818=DIRECTION ( 'NONE',  ( -0.000000000000000000, 0.9848077530122085754, -0.1736481776669273613 ) ) ;
#82820=CARTESIAN_POINT ( 'NONE',  ( -5.076923076923075762, -6.343179335718451384, 34.87096338111211935 ) ) ;
#82821=CARTESIAN_POINT ( 'NONE',  ( 5.869852790561778555, -12.27039167877662251, 31.24851455888617835 ) ) ;
#82822=EDGE_CURVE ( 'NONE', #32882, #78424, #82840, .T. ) ;
#82823=CARTESIAN_POINT ( 'NONE',  ( -13.38461538461550759, -9.528491918059723176, 34.59228464037033035 ) ) ;
#82824=CARTESIAN_POINT ( 'NONE',  ( 12.46153846153846168, -2.721908614388771852, 31.22303859784724978 ) ) ;
#82825=ORIENTED_EDGE ( 'NONE', *, *, #17038, .T. ) ;
#82826=EDGE_CURVE ( 'NONE', #59207, #33581, #57960, .T. ) ;
#82827=CARTESIAN_POINT ( 'NONE',  ( -0.2114841499001472724, -3.627508038966690496, 32.91356715214248396 ) ) ;
#82828=CARTESIAN_POINT ( 'NONE',  ( -3.230769230769351186, -12.46129190930018460, 30.37095296980731973 ) ) ;
#82830=ADVANCED_FACE ( 'NONE', ( #82136 ), #6473, .F. ) ;
#82831=CARTESIAN_POINT ( 'NONE',  ( -18.00000000000000000, -2.916148748677405145, 35.60175215339625510 ) ) ;
#82832=DIRECTION ( 'NONE',  ( 0.000000000000000000, 0.9396926207859126468, -0.3420201433256571111 ) ) ;
#82833=EDGE_LOOP ( 'NONE', ( #81903, #20824, #20754, #6193 ) ) ;
#82834=FACE_OUTER_BOUND ( 'NONE', #40895, .T. ) ;
#82835=CARTESIAN_POINT ( 'NONE',  ( -6.249999999999996447, -7.566082377512563184, 35.00000000000000711 ) ) ;
#82836=EDGE_LOOP ( 'NONE', ( #80433, #38523 ) ) ;
#82837=CARTESIAN_POINT ( 'NONE',  ( 7.911409417429874580, -3.835265460703683349, 33.15142922261929925 ) ) ;
#82839=EDGE_LOOP ( 'NONE', ( #47643, #51851 ) ) ;
#82840=B_SPLINE_CURVE_WITH_KNOTS ( 'NONE', 3,
 ( #63386, #8901, #1694, #36371, #78229, #43996, #16093, #63833, #37236, #3007 ),
 .UNSPECIFIED., .F., .F.,
 ( 4, 2, 2, 2, 4 ),
 ( 0.000000000000000000, 0.0001954311564186864678, 0.0003908623128373729357, 0.0005862934692560594577, 0.0007817246256747458714 ),
 .UNSPECIFIED. ) ;
#82841=DIRECTION ( 'NONE',  ( -0.000000000000000000, 0.9848077530122085754, -0.1736481776669273613 ) ) ;
#82842=EDGE_CURVE ( 'NONE', #7785, #85805, #78505, .T. ) ;
#82843=DIRECTION ( 'NONE',  ( -0.000000000000000000, 0.7660444431189791237, -0.6427876096865379196 ) ) ;
#82844=ORIENTED_EDGE ( 'NONE', *, *, #40950, .T. ) ;
#82845=CARTESIAN_POINT ( 'NONE',  ( -10.68146699474474914, -3.937682226553330445, 33.60647404775217240 ) ) ;
#82846=DIRECTION ( 'NONE',  ( -0.000000000000000000, 0.8660254037844397068, -0.4999999999999978906 ) ) ;
#82847=AXIS2_PLACEMENT_3D ( 'NONE', #39725, #75705, #40169 ) ;
#82848=DIRECTION ( 'NONE',  ( 0.000000000000000000, 0.9396926207859126468, -0.3420201433256571111 ) ) ;
#82849=ORIENTED_EDGE ( 'NONE', *, *, #25762, .F. ) ;
#82851=CARTESIAN_POINT ( 'NONE',  ( 5.999999999999880096, -6.879047030192662504, 34.71129190930017927 ) ) ;
#82852=ORIENTED_EDGE ( 'NONE', *, *, #69139, .F. ) ;
#82854=CARTESIAN_POINT ( 'NONE',  ( -5.076923076923075762, -9.058645607665452459, 34.76329471203371924 ) ) ;
#82855=CARTESIAN_POINT ( 'NONE',  ( 2.307692307692309264, -11.35647404775217417, 33.31231777344666511 ) ) ;
#82857=CARTESIAN_POINT ( 'NONE',  ( -6.923076923077045919, -11.67786785259630911, 32.92929555188603530 ) ) ;
#82858=CARTESIAN_POINT ( 'NONE',  ( -4.153846153846152411, -6.386643153685126251, 34.62446782046654192 ) ) ;
#82859=EDGE_CURVE ( 'NONE', #46262, #28353, #9745, .T. ) ;
#82860=LINE ( 'NONE', #69770, #664 ) ;
#82861=CARTESIAN_POINT ( 'NONE',  ( 3.007284306204901281, -10.23692288466677880, 34.23039457007281072 ) ) ;
#82862=ORIENTED_EDGE ( 'NONE', *, *, #77846, .F. ) ;
#82863=EDGE_LOOP ( 'NONE', ( #56833, #74553 ) ) ;
#82864=CARTESIAN_POINT ( 'NONE',  ( 7.053867364043876265, -12.62708834333097663, 30.88030960425257021 ) ) ;
#82865=ORIENTED_EDGE ( 'NONE', *, *, #59933, .T. ) ;
#82866=CARTESIAN_POINT ( 'NONE',  ( -5.326946301144535489, -4.931416488878822335, 34.32920672191015399 ) ) ;
#82867=ORIENTED_EDGE ( 'NONE', *, *, #76457, .F. ) ;
#82868=DIRECTION ( 'NONE',  ( -0.000000000000000000, 1.000000000000000000, -0.000000000000000000 ) ) ;
#82869=CARTESIAN_POINT ( 'NONE',  ( 5.299702618191484582, -3.755027918224367767, 33.06320215134714857 ) ) ;
#82870=ORIENTED_EDGE ( 'NONE', *, *, #701, .F. ) ;
#82871=CARTESIAN_POINT ( 'NONE',  ( -9.757558682468932432, -2.506253911140460922, 30.00000000000013856 ) ) ;
#82873=VERTEX_POINT ( 'NONE', #46996 ) ;
#82874=ORIENTED_EDGE ( 'NONE', *, *, #1596, .T. ) ;
#82875=B_SPLINE_CURVE_WITH_KNOTS ( 'NONE', 3,
 ( #59741, #54304, #25069, #80920, #18316, #33158, #73717, #67832, #45779, #25954 ),
 .UNSPECIFIED., .F., .F.,
 ( 4, 2, 2, 2, 4 ),
 ( 0.000000000000000000, 0.0001954339857564097241, 0.0003908679715128194482, 0.0005863019572692291723, 0.0007817359430256388964 ),
 .UNSPECIFIED. ) ;
#82877=EDGE_CURVE ( 'NONE', #4743, #50820, #27939, .T. ) ;
#82879=EDGE_CURVE ( 'NONE', #66653, #78771, #74048, .T. ) ;
#82880=CARTESIAN_POINT ( 'NONE',  ( -1.384615384615505151, -2.625532179533778709, 30.86335684631627174 ) ) ;
#82881=CARTESIAN_POINT ( 'NONE',  ( 17.01083966596719677, -2.721908614388770964, 31.22303859784723912 ) ) ;
#82882=FACE_BOUND ( 'NONE', #72166, .T. ) ;
#82883=CYLINDRICAL_SURFACE ( 'NONE', #25504, 0.2500000000000012212 ) ;
#82884=CARTESIAN_POINT ( 'NONE',  ( -6.923076923077044142, -12.27809138561165270, 31.22303859784587132 ) ) ;
#82885=EDGE_CURVE ( 'NONE', #63695, #79014, #81693, .T. ) ;
#82886=CARTESIAN_POINT ( 'NONE',  ( 15.48071464014727283, -2.589246495874658383, 31.60778113518102828 ) ) ;
#82887=CARTESIAN_POINT ( 'NONE',  ( -0.3962833220256232192, -3.083524468853785283, 32.58852847137153930 ) ) ;
#82888=CARTESIAN_POINT ( 'NONE',  ( 5.076923076922954969, -10.90142922262034020, 33.41473453929536674 ) ) ;
#82890=ADVANCED_FACE ( 'NONE', ( #18662 ), #40264, .F. ) ;
#82891=FACE_OUTER_BOUND ( 'NONE', #22183, .T. ) ;
#82892=VERTEX_POINT ( 'NONE', #6904 ) ;
#82894=CARTESIAN_POINT ( 'NONE',  ( 2.242422307135989890, -3.083524468853724443, 32.58852847137143272 ) ) ;
#82895=CARTESIAN_POINT ( 'NONE',  ( 14.98074599347626545, -12.22074536777954989, 31.39888409691088356 ) ) ;
#82896=CARTESIAN_POINT ( 'NONE',  ( 7.145856464345331283, -6.760870238392817200, 34.69528174975672385 ) ) ;
#82897=CYLINDRICAL_SURFACE ( 'NONE', #60937, 0.2499999999999994726 ) ;
#82898=CARTESIAN_POINT ( 'NONE',  ( -10.61538461538473577, -12.51329471203414379, 31.30864560766407578 ) ) ;
#82899=CARTESIAN_POINT ( 'NONE',  ( 9.758376043310134307, -2.538708090699994813, 30.37095296980875503 ) ) ;
#82900=ORIENTED_EDGE ( 'NONE', *, *, #63489, .T. ) ;
#82902=CARTESIAN_POINT ( 'NONE',  ( -39.05038313613820122, -2.249999999999998668, 29.75000000000000355 ) ) ;
#82903=CARTESIAN_POINT ( 'NONE',  ( 16.94677510719138169, -4.299443229763728169, 33.91186481527756058 ) ) ;
#82904=DIRECTION ( 'NONE',  ( 0.000000000000000000, 0.7660444431189822323, -0.6427876096865344779 ) ) ;
#82905=ORIENTED_EDGE ( 'NONE', *, *, #20204, .T. ) ;
#82906=ADVANCED_FACE ( 'NONE', ( #59630 ), #87131, .F. ) ;
#82907=EDGE_LOOP ( 'NONE', ( #68019, #25494 ) ) ;
#82908=VERTEX_POINT ( 'NONE', #32603 ) ;
#82909=CARTESIAN_POINT ( 'NONE',  ( -9.442253380669379581, -12.41262288849542017, 30.68299917996395010 ) ) ;
#82910=EDGE_CURVE ( 'NONE', #79986, #765, #69890, .T. ) ;
#82911=ORIENTED_EDGE ( 'NONE', *, *, #85675, .T. ) ;
#82912=AXIS2_PLACEMENT_3D ( 'NONE', #31420, #86387, #17910 ) ;
#82913=CYLINDRICAL_SURFACE ( 'NONE', #72830, 0.2500000000000002220 ) ;
#82914=CARTESIAN_POINT ( 'NONE',  ( 1.384615384615264011, -3.643525952248795718, 33.31231777344771672 ) ) ;
#82915=CARTESIAN_POINT ( 'NONE',  ( 14.24160992833217065, -9.905515769479276145, 34.41647553114623292 ) ) ;
#82917=CARTESIAN_POINT ( 'NONE',  ( -11.28851602011339672, -6.696923467548660192, 34.68552623307873972 ) ) ;
#82918=ORIENTED_EDGE ( 'NONE', *, *, #23175, .F. ) ;
#82919=CARTESIAN_POINT ( 'NONE',  ( 11.31559611625790041, -2.501496062324912284, 29.88072118266895671 ) ) ;
#82920=DIRECTION ( 'NONE',  ( -0.000000000000000000, 0.3420201433256694346, -0.9396926207859080948 ) ) ;
#82921=ORIENTED_EDGE ( 'NONE', *, *, #14433, .T. ) ;
#82922=LINE ( 'NONE', #51193, #81496 ) ;
#82923=DIRECTION ( 'NONE',  ( 0.000000000000000000, 0.7660444431189822323, -0.6427876096865344779 ) ) ;
#82924=CARTESIAN_POINT ( 'NONE',  ( 17.01083966596719321, -3.513871655860377086, 32.76840700105978499 ) ) ;
#82925=CARTESIAN_POINT ( 'NONE',  ( 11.66898697669518548, -10.31582465632705237, 34.18122507451815295 ) ) ;
#82926=EDGE_CURVE ( 'NONE', #64675, #7863, #28069, .T. ) ;
#82927=LINE ( 'NONE', #76607, #8846 ) ;
#82928=CARTESIAN_POINT ( 'NONE',  ( -3.360917200500928459, -11.04286588640298561, 33.62463336215343901 ) ) ;
#82929=CARTESIAN_POINT ( 'NONE',  ( -3.164602624177589529, -7.250054591869667497, 34.99404684341514127 ) ) ;
#82931=ORIENTED_EDGE ( 'NONE', *, *, #9095, .F. ) ;
#82933=CARTESIAN_POINT ( 'NONE',  ( -2.980714810855777053, -6.523592122091589118, 34.90882529074906415 ) ) ;
#82934=CARTESIAN_POINT ( 'NONE',  ( 0.5920641633020263805, -3.285477652293412820, 32.44071101563363158 ) ) ;
#82935=CYLINDRICAL_SURFACE ( 'NONE', #83485, 0.2499999999999998890 ) ;
#82936=VECTOR ( 'NONE', #67876, 1000.000000000000000 ) ;
#82938=ORIENTED_EDGE ( 'NONE', *, *, #72002, .T. ) ;
#82939=CARTESIAN_POINT ( 'NONE',  ( 7.976679284387489410, -12.15418822224088657, 32.17964115625579069 ) ) ;
#82940=CARTESIAN_POINT ( 'NONE',  ( -6.000000000000119904, -2.625532179533778709, 30.86335684631627174 ) ) ;
#82941=CARTESIAN_POINT ( 'NONE',  ( -0.7115152055870523906, -12.65889640711025521, 30.72598325615533454 ) ) ;
#82942=EDGE_CURVE ( 'NONE', #84330, #71586, #29412, .T. ) ;
#82943=CARTESIAN_POINT ( 'NONE',  ( 9.469428175570110184, -7.630690623152299956, 34.99857592706774057 ) ) ;
#82944=ORIENTED_EDGE ( 'NONE', *, *, #4901, .T. ) ;
#82945=LINE ( 'NONE', #63092, #70740 ) ;
#82946=EDGE_CURVE ( 'NONE', #30896, #29433, #68775, .T. ) ;
#82947=CARTESIAN_POINT ( 'NONE',  ( 17.32686859527121470, -5.852078868378311149, 34.47109172314383585 ) ) ;
#82948=DIRECTION ( 'NONE',  ( -0.000000000000000000, -0.5000000000000009992, -0.8660254037844380415 ) ) ;
#82949=ORIENTED_EDGE ( 'NONE', *, *, #32242, .T. ) ;
#82950=FACE_OUTER_BOUND ( 'NONE', #42776, .T. ) ;
#82951=EDGE_LOOP ( 'NONE', ( #86874, #55828, #77517, #65646 ) ) ;
#82953=CARTESIAN_POINT ( 'NONE',  ( 0.6843181305165274564, -10.23759521482555357, 34.22997729860117033 ) ) ;
#82957=ADVANCED_FACE ( 'NONE', ( #28516 ), #152, .F. ) ;
#82958=CARTESIAN_POINT ( 'NONE',  ( -10.68065506134539078, -6.026961402152685388, 34.52809138561120506 ) ) ;
#82960=CARTESIAN_POINT ( 'NONE',  ( 11.47237915910140238, -12.34228464037088280, 31.77849191805838558 ) ) ;
#82962=EDGE_LOOP ( 'NONE', ( #24466, #79182 ) ) ;
#82963=FACE_BOUND ( 'NONE', #43423, .T. ) ;
#82964=ORIENTED_EDGE ( 'NONE', *, *, #2420, .F. ) ;
#82965=LINE ( 'NONE', #74430, #8410 ) ;
#82967=B_SPLINE_CURVE_WITH_KNOTS ( 'NONE', 3,
 ( #75586, #68393, #8029, #62946, #41373, #6692, #34164, #14791, #56211, #35498 ),
 .UNSPECIFIED., .F., .F.,
 ( 4, 2, 2, 2, 4 ),
 ( 0.0007817246256747484735, 0.0009771112852218928873, 0.001172497944769037084, 0.001367884604316181498, 0.001563271263863325912 ),
 .UNSPECIFIED. ) ;
#82968=CARTESIAN_POINT ( 'NONE',  ( 6.857826991302839126, -2.255955759149247619, 30.00000000000013856 ) ) ;
#82969=CIRCLE ( 'NONE', #16863, 0.2500000000000002220 ) ;
#82970=CARTESIAN_POINT ( 'NONE',  ( 3.100621261037533660, -11.66186481527757479, 32.95055677023626117 ) ) ;
#82971=CARTESIAN_POINT ( 'NONE',  ( -11.47239318745910097, -2.538708090699994813, 30.37095296980875503 ) ) ;
#82974=ORIENTED_EDGE ( 'NONE', *, *, #7975, .F. ) ;
#82975=LINE ( 'NONE', #76204, #47685 ) ;
#82976=ORIENTED_EDGE ( 'NONE', *, *, #23064, .F. ) ;
#82977=CARTESIAN_POINT ( 'NONE',  ( 4.284636594813102661, -9.929761469519744921, 34.40412654351204225 ) ) ;
#82978=CARTESIAN_POINT ( 'NONE',  ( -11.78843828251013015, -5.643011162660950042, 34.66104346484419096 ) ) ;
#82979=CARTESIAN_POINT ( 'NONE',  ( -5.076923076923075762, -3.513871655860378418, 32.76840700105978499 ) ) ;
#82980=CARTESIAN_POINT ( 'NONE',  ( 16.21991348719623360, -2.292212530054420050, 30.41441678777542990 ) ) ;
#82981=EDGE_CURVE ( 'NONE', #45693, #4584, #41989, .T. ) ;
#82982=CARTESIAN_POINT ( 'NONE',  ( 16.15384615384615330, -9.819645486525091727, 36.12317359536749706 ) ) ;
#82984=CARTESIAN_POINT ( 'NONE',  ( -4.946132635956124624, -11.37503395064541678, 33.29242100308974983 ) ) ;
#82985=ORIENTED_EDGE ( 'NONE', *, *, #30943, .F. ) ;
#82986=EDGE_CURVE ( 'NONE', #27220, #19422, #16139, .T. ) ;
#82988=B_SPLINE_CURVE_WITH_KNOTS ( 'NONE', 3,
 ( #26840, #88563, #47542, #20519, #45432, #66149, #20952, #89004, #34478, #61940 ),
 .UNSPECIFIED., .F., .F.,
 ( 4, 2, 2, 2, 4 ),
 ( 0.0007817246256747520513, 0.0009771112852218959231, 0.001172497944769039903, 0.001367884604316183883, 0.001563271263863327864 ),
 .UNSPECIFIED. ) ;
#82989=ORIENTED_EDGE ( 'NONE', *, *, #19555, .F. ) ;
#82990=CARTESIAN_POINT ( 'NONE',  ( -5.076923076923075762, -10.67929555188718282, 33.92786785259544047 ) ) ;
#82991=CARTESIAN_POINT ( 'NONE',  ( -1.608100309179717025, -2.612411019501189813, 31.66733052389439962 ) ) ;
#82992=CARTESIAN_POINT ( 'NONE',  ( 1.384615384615264011, -11.67786785259630911, 32.92929555188603530 ) ) ;
#82993=ADVANCED_FACE ( 'NONE', ( #77585 ), #35723, .F. ) ;
#82994=B_SPLINE_CURVE_WITH_KNOTS ( 'NONE', 3,
 ( #59542, #73518, #10478, #25321, #24866, #72164, #52783, #45584, #73063, #30734 ),
 .UNSPECIFIED., .F., .F.,
 ( 4, 2, 2, 2, 4 ),
 ( 0.0007817359430256287049, 0.0009771253907249945886, 0.001172514838424360255, 0.001367904286123725922, 0.001563293733823091589 ),
 .UNSPECIFIED. ) ;
#82995=CARTESIAN_POINT ( 'NONE',  ( 1.450682717965462887, -12.34228464037088813, 31.77849191805839268 ) ) ;
#82996=CARTESIAN_POINT ( 'NONE',  ( 14.30769230769231015, -12.78798330534102767, 29.49999999999997868 ) ) ;
#82997=FACE_BOUND ( 'NONE', #29363, .T. ) ;
#82998=CARTESIAN_POINT ( 'NONE',  ( 8.703148389870634105, -10.67929555188718460, 33.92786785259543336 ) ) ;
#82999=VERTEX_POINT ( 'NONE', #49666 ) ;
#83000=CARTESIAN_POINT ( 'NONE',  ( 14.53047197667037338, -12.47679350104403007, 31.42216943046555855 ) ) ;
#83002=CARTESIAN_POINT ( 'NONE',  ( -14.30769230769230660, -1.117168528481311540, 33.14645433367849847 ) ) ;
#83003=DIRECTION ( 'NONE',  ( 0.000000000000000000, 0.000000000000000000, -1.000000000000000000 ) ) ;
#83004=CARTESIAN_POINT ( 'NONE',  ( 7.053867364043876265, -9.084667340241226796, 34.75534355489798344 ) ) ;
#83006=ADVANCED_FACE ( 'NONE', ( #28973 ), #7361, .F. ) ;
#83007=CARTESIAN_POINT ( 'NONE',  ( 18.22277954126840172, -12.44528174975671853, 30.48912976160715615 ) ) ;
#83008=ORIENTED_EDGE ( 'NONE', *, *, #24246, .F. ) ;
#83009=FACE_BOUND ( 'NONE', #60257, .T. ) ;
#83011=LINE ( 'NONE', #63614, #24755 ) ;
#83012=CARTESIAN_POINT ( 'NONE',  ( 16.94623247381276343, -11.93127051446800380, 32.56575433478200665 ) ) ;
#83013=ORIENTED_EDGE ( 'NONE', *, *, #44942, .F. ) ;
#83014=CARTESIAN_POINT ( 'NONE',  ( 0.2115617305961065842, -10.66389620160130036, 33.62221079203477103 ) ) ;
#83015=CARTESIAN_POINT ( 'NONE',  ( -14.30769230769242739, -4.481592998941358097, 33.73612834414048933 ) ) ;
#83016=CARTESIAN_POINT ( 'NONE',  ( 12.68454981315131391, -6.503523203565941380, 34.64991518177335195 ) ) ;
#83017=DIRECTION ( 'NONE',  ( -0.000000000000000000, -0.6427876096865404731, -0.7660444431189770143 ) ) ;
#83018=ORIENTED_EDGE ( 'NONE', *, *, #14725, .F. ) ;
#83019=EDGE_CURVE ( 'NONE', #67105, #38304, #16325, .T. ) ;
#83020=CARTESIAN_POINT ( 'NONE',  ( -5.011667937410239304, -5.094484230520773593, 34.41647553114626845 ) ) ;
#83021=ORIENTED_EDGE ( 'NONE', *, *, #10622, .F. ) ;
#83022=CARTESIAN_POINT ( 'NONE',  ( 16.40384615384757439, -7.500000000000154543, 35.00000000000007105 ) ) ;
#83023=EDGE_LOOP ( 'NONE', ( #76313, #76183, #15126, #16884 ) ) ;
#83024=CARTESIAN_POINT ( 'NONE',  ( 3.480714749117373774, -2.587454068350147907, 30.68340429815432202 ) ) ;
#83025=CARTESIAN_POINT ( 'NONE',  ( -8.769230769230890843, -5.219633306517616589, 34.19971097300220464 ) ) ;
#83026=CARTESIAN_POINT ( 'NONE',  ( 5.076923076922953193, -2.657715359629662988, 31.77849191805970364 ) ) ;
#83027=CARTESIAN_POINT ( 'NONE',  ( 14.30769230769218758, -9.442884908241554243, 34.35708131394783038 ) ) ;
#83028=AXIS2_PLACEMENT_3D ( 'NONE', #14472, #62642, #57668 ) ;
#83029=CARTESIAN_POINT ( 'NONE',  ( -13.31936024510254768, -3.643525952247864463, 33.31231777344670064 ) ) ;
#83030=CARTESIAN_POINT ( 'NONE',  ( 13.51514108637895184, -6.001044277235009439, 34.52024696741798948 ) ) ;
#83031=CYLINDRICAL_SURFACE ( 'NONE', #44628, 0.2499999999999986955 ) ;
#83032=CARTESIAN_POINT ( 'NONE',  ( 1.384615384615386802, -4.102666532097928531, 36.13435417666054406 ) ) ;
#83034=ORIENTED_EDGE ( 'NONE', *, *, #13521, .T. ) ;
#83035=VECTOR ( 'NONE', #35335, 1000.000000000000114 ) ;
#83036=ADVANCED_FACE ( 'NONE', ( #51862 ), #43791, .F. ) ;
#83037=DIRECTION ( 'NONE',  ( -0.000000000000000000, -0.7660444431189791237, -0.6427876096865379196 ) ) ;
#83038=ORIENTED_EDGE ( 'NONE', *, *, #34466, .T. ) ;
#83039=ORIENTED_EDGE ( 'NONE', *, *, #68476, .T. ) ;
#83040=EDGE_CURVE ( 'NONE', #7083, #3322, #33372, .T. ) ;
#83041=CARTESIAN_POINT ( 'NONE',  ( 3.230769230769231726, -4.786620604624113540, 33.94971097300155094 ) ) ;
#83042=AXIS2_PLACEMENT_3D ( 'NONE', #16124, #30084, #78258 ) ;
#83043=ORIENTED_EDGE ( 'NONE', *, *, #41608, .T. ) ;
#83044=CYLINDRICAL_SURFACE ( 'NONE', #87288, 0.2500000000000008882 ) ;
#83046=CARTESIAN_POINT ( 'NONE',  ( -8.096130590202434973, -8.347322224742351082, 34.93158281831414058 ) ) ;
#83047=CARTESIAN_POINT ( 'NONE',  ( 6.222779541268410597, -3.236590943229499029, 32.36255958852954251 ) ) ;
#83048=CARTESIAN_POINT ( 'NONE',  ( -11.53846153846153655, -11.16473453929635440, 33.15142922261926373 ) ) ;
#83049=CARTESIAN_POINT ( 'NONE',  ( 6.130791807824788719, -2.541949514083464479, 30.39797389878540557 ) ) ;
#83050=CARTESIAN_POINT ( 'NONE',  ( 8.703147358274890166, -11.16473453929635440, 33.15142922261925662 ) ) ;
#83051=CARTESIAN_POINT ( 'NONE',  ( 15.93091993633000847, -11.76352882383564769, 32.36236540154569497 ) ) ;
#83053=CARTESIAN_POINT ( 'NONE',  ( -0.6844646790546100590, -2.554751324335733820, 30.48935550225260727 ) ) ;
#83054=CARTESIAN_POINT ( 'NONE',  ( 17.77651505627605033, -11.89387501736623420, 32.13663884655804992 ) ) ;
#83055=EDGE_CURVE ( 'NONE', #47762, #60409, #71007, .T. ) ;
#83056=CARTESIAN_POINT ( 'NONE',  ( 14.30769230769261569, -2.506253911140615021, 30.00000000000323297 ) ) ;
#83057=CARTESIAN_POINT ( 'NONE',  ( 11.53846153846153832, -4.786620604624113540, 33.94971097300155094 ) ) ;
#83058=VERTEX_POINT ( 'NONE', #2350 ) ;
#83059=ORIENTED_EDGE ( 'NONE', *, *, #82425, .T. ) ;
#83060=VECTOR ( 'NONE', #32915, 999.9999999999998863 ) ;
#83061=CARTESIAN_POINT ( 'NONE',  ( -17.93474900983876452, -12.49374608885954352, 30.00000000000010658 ) ) ;
#83062=CARTESIAN_POINT ( 'NONE',  ( 1.607395053593452916, -3.563462043263030399, 33.22394488606062879 ) ) ;
#83063=FACE_OUTER_BOUND ( 'NONE', #34446, .T. ) ;
#83064=CARTESIAN_POINT ( 'NONE',  ( 0.4615384615383382183, -10.33852847137269571, 34.16647553114546554 ) ) ;
#83065=B_SPLINE_CURVE_WITH_KNOTS ( 'NONE', 3,
 ( #28653, #56122, #14247, #62415, #42613, #8382, #13800, #70524, #35855, #7043 ),
 .UNSPECIFIED., .F., .F.,
 ( 4, 2, 2, 2, 4 ),
 ( 0.000000000000000000, 0.0001954311564186881213, 0.0003908623128373762425, 0.0005862934692560643367, 0.0007817246256747524850 ),
 .UNSPECIFIED. ) ;
#83066=CARTESIAN_POINT ( 'NONE',  ( -16.08859101433330707, -8.656820664281605460, 34.87096338111211224 ) ) ;
#83067=EDGE_CURVE ( 'NONE', #64445, #59172, #79359, .T. ) ;
#83068=B_SPLINE_CURVE_WITH_KNOTS ( 'NONE', 3,
 ( #20618, #34583, #76006, #6234, #14306, #27821, #35019, #42238, #13420, #54853 ),
 .UNSPECIFIED., .F., .F.,
 ( 4, 2, 2, 2, 4 ),
 ( 0.000000000000000000, 0.0001954311564186868473, 0.0003908623128373736946, 0.0005862934692560605419, 0.0007817246256747473893 ),
 .UNSPECIFIED. ) ;
#83069=CYLINDRICAL_SURFACE ( 'NONE', #22585, 0.2500000000000009437 ) ;
#83070=CARTESIAN_POINT ( 'NONE',  ( -2.557715531913763662, -8.475808217655753651, 34.90892951860618609 ) ) ;
#83071=EDGE_CURVE ( 'NONE', #29011, #18655, #9139, .T. ) ;
#83073=AXIS2_PLACEMENT_3D ( 'NONE', #12487, #81840, #87276 ) ;
#83074=ORIENTED_EDGE ( 'NONE', *, *, #19496, .T. ) ;
#83075=LINE ( 'NONE', #648, #65949 ) ;
#83077=ADVANCED_FACE ( 'NONE', ( #37471 ), #17204, .F. ) ;
#83080=CARTESIAN_POINT ( 'NONE',  ( 12.39545505058258179, -8.120952969808774569, 34.71129190930000163 ) ) ;
#83082=CARTESIAN_POINT ( 'NONE',  ( -3.100721795518779356, -7.723484941389743952, 34.99544897038808955 ) ) ;
#83083=ORIENTED_EDGE ( 'NONE', *, *, #25287, .F. ) ;
#83084=VERTEX_POINT ( 'NONE', #23951 ) ;
#83085=VERTEX_POINT ( 'NONE', #78908 ) ;
#83086=EDGE_LOOP ( 'NONE', ( #11852, #50060, #15196, #82576 ) ) ;
#83087=DIRECTION ( 'NONE',  ( -0.000000000000000000, -0.6427876096865404731, -0.7660444431189770143 ) ) ;
#83088=CARTESIAN_POINT ( 'NONE',  ( -15.90379173393269951, -9.233818618650598609, 34.70587769442853698 ) ) ;
#83089=B_SPLINE_CURVE_WITH_KNOTS ( 'NONE', 3,
 ( #44380, #63781, #85841, #65551, #38091, #16489, #29566, #84955, #70547, #2959 ),
 .UNSPECIFIED., .F., .F.,
 ( 4, 2, 2, 2, 4 ),
 ( 0.000000000000000000, 0.0001954339857564080165, 0.0003908679715128160329, 0.0005863019572692240765, 0.0007817359430256320659 ),
 .UNSPECIFIED. ) ;
#83091=B_SPLINE_CURVE_WITH_KNOTS ( 'NONE', 3,
 ( #87264, #6164, #34073, #26878, #47585, #33635, #25544, #39960, #52999, #12476 ),
 .UNSPECIFIED., .F., .F.,
 ( 4, 2, 2, 2, 4 ),
 ( 0.000000000000000000, 0.0001954339881912775425, 0.0003908679763825550850, 0.0005863019645738326005, 0.0007817359527651101701 ),
 .UNSPECIFIED. ) ;
#83092=CARTESIAN_POINT ( 'NONE',  ( -2.084912638714241151, -11.60474049983370648, 33.02348890104160262 ) ) ;
#83093=DIRECTION ( 'NONE',  ( -0.000000000000000000, -0.6427876096865404731, -0.7660444431189771253 ) ) ;
#83094=DIRECTION ( 'NONE',  ( 0.000000000000000000, 0.1736481776669267785, -0.9848077530122087975 ) ) ;
#83096=ORIENTED_EDGE ( 'NONE', *, *, #60439, .F. ) ;
#83098=ORIENTED_EDGE ( 'NONE', *, *, #61097, .F. ) ;
#83099=CARTESIAN_POINT ( 'NONE',  ( 4.153846153846154188, -2.721908614388771852, 31.22303859784724978 ) ) ;
#83100=EDGE_LOOP ( 'NONE', ( #20765, #46912, #31444, #36187 ) ) ;
#83101=CARTESIAN_POINT ( 'NONE',  ( -10.36533019547116119, -6.523592122091592671, 34.90882529074906415 ) ) ;
#83104=EDGE_LOOP ( 'NONE', ( #10952, #38202, #64699, #23693 ) ) ;
#83105=ORIENTED_EDGE ( 'NONE', *, *, #22317, .T. ) ;
#83106=CARTESIAN_POINT ( 'NONE',  ( 13.44980936639873903, -2.506253911140448043, 29.99999999999988631 ) ) ;
#83107=B_SPLINE_CURVE_WITH_KNOTS ( 'NONE', 3,
 ( #32715, #30927, #59747, #65160, #45335, #17433, #59297, #24627, #51182, #17881 ),
 .UNSPECIFIED., .F., .F.,
 ( 4, 2, 2, 2, 4 ),
 ( 0.000000000000000000, 0.0001954339881912776238, 0.0003908679763825552477, 0.0005863019645738329257, 0.0007817359527651104954 ),
 .UNSPECIFIED. ) ;
#83108=VERTEX_POINT ( 'NONE', #50967 ) ;
#83109=FACE_BOUND ( 'NONE', #27200, .T. ) ;
#83110=CARTESIAN_POINT ( 'NONE',  ( -5.750054590621957118, -2.986452184633680673, 32.43230066228895225 ) ) ;
#83111=AXIS2_PLACEMENT_3D ( 'NONE', #84003, #56068, #56515 ) ;
#83113=ORIENTED_EDGE ( 'NONE', *, *, #42903, .F. ) ;
#83114=DIRECTION ( 'NONE',  ( -0.000000000000000000, -0.9848077530122085754, -0.1736481776669273613 ) ) ;
#83115=CARTESIAN_POINT ( 'NONE',  ( -15.90379173393269951, -12.65882529074907126, 30.72640787790838601 ) ) ;
#83118=DIRECTION ( 'NONE',  ( -0.000000000000000000, -0.9848077530122086864, -0.1736481776669273613 ) ) ;
#83119=ORIENTED_EDGE ( 'NONE', *, *, #26011, .T. ) ;
#83121=CARTESIAN_POINT ( 'NONE',  ( 6.249945518348142492, -8.433404298154334455, 34.66254593164985920 ) ) ;
#83122=FACE_OUTER_BOUND ( 'NONE', #37219, .T. ) ;
#83123=CARTESIAN_POINT ( 'NONE',  ( 16.40379167219429846, -9.272278438253401589, 34.42582936511637826 ) ) ;
#83124=CARTESIAN_POINT ( 'NONE',  ( -0.5276208408985973985, -4.661471528628507777, 34.16647553114621871 ) ) ;
#83125=CARTESIAN_POINT ( 'NONE',  ( -15.09997742294444478, -11.71459661697925903, 32.44059661609676937 ) ) ;
#83126=FACE_BOUND ( 'NONE', #66100, .T. ) ;
#83127=CARTESIAN_POINT ( 'NONE',  ( 13.38461538461538680, -11.69971097300155272, 32.46337939537588113 ) ) ;
#83128=CARTESIAN_POINT ( 'NONE',  ( -6.000000000000121680, -10.33852847137269571, 34.16647553114546554 ) ) ;
#83130=CARTESIAN_POINT ( 'NONE',  ( 5.076923076923075762, -2.292212530054420494, 30.41441678777542634 ) ) ;
#83131=LINE ( 'NONE', #62391, #68849 ) ;
#83132=CARTESIAN_POINT ( 'NONE',  ( -6.250023237292964495, -5.056417327199099532, 34.11270091957320716 ) ) ;
#83133=CARTESIAN_POINT ( 'NONE',  ( -18.13014720943822056, -10.19110544564092358, 33.96427741523702792 ) ) ;
#83134=B_SPLINE_CURVE_WITH_KNOTS ( 'NONE', 3,
 ( #48510, #62902, #83658, #70119, #57043, #35901, #84537, #1665, #69240, #21488 ),
 .UNSPECIFIED., .F., .F.,
 ( 4, 2, 2, 2, 4 ),
 ( 0.000000000000000000, 0.0001954339881912776238, 0.0003908679763825552477, 0.0005863019645738329257, 0.0007817359527651104954 ),
 .UNSPECIFIED. ) ;
#83136=ORIENTED_EDGE ( 'NONE', *, *, #51424, .F. ) ;
#83137=B_SPLINE_CURVE_WITH_KNOTS ( 'NONE', 3,
 ( #18240, #38964, #6059, #52003, #33533, #46156, #60992, #39411, #73183, #79498 ),
 .UNSPECIFIED., .F., .F.,
 ( 4, 2, 2, 2, 4 ),
 ( 0.000000000000000000, 0.0001954339857564064444, 0.0003908679715128128888, 0.0005863019572692193060, 0.0007817359430256257775 ),
 .UNSPECIFIED. ) ;
#83139=ORIENTED_EDGE ( 'NONE', *, *, #41599, .F. ) ;
#83140=CARTESIAN_POINT ( 'NONE',  ( -14.98082371242109012, -4.336752205174649433, 33.62275283266504289 ) ) ;
#83141=EDGE_LOOP ( 'NONE', ( #85411, #69720 ) ) ;
#83143=CARTESIAN_POINT ( 'NONE',  ( -18.22348494372394967, -2.599994579823202479, 30.74605699353653776 ) ) ;
#83144=EDGE_LOOP ( 'NONE', ( #52786, #58116 ) ) ;
#83147=CARTESIAN_POINT ( 'NONE',  ( -4.023801097926381409, -2.254550872974306674, 29.97347326024527447 ) ) ;
#83148=CARTESIAN_POINT ( 'NONE',  ( -12.46153846153846168, -11.11383981884818262, 36.00935417666054406 ) ) ;
#83149=CARTESIAN_POINT ( 'NONE',  ( -2.980769230769230393, -2.249999999999998668, 29.75000000000000355 ) ) ;
#83150=CARTESIAN_POINT ( 'NONE',  ( 10.36536139116315525, -2.588893531581426988, 31.60682220781847818 ) ) ;
#83151=FACE_OUTER_BOUND ( 'NONE', #31039, .T. ) ;
#83152=CARTESIAN_POINT ( 'NONE',  ( 11.76147289007438523, -3.587049720035815348, 32.86302985866382897 ) ) ;
#83155=CARTESIAN_POINT ( 'NONE',  ( -10.48485891362105171, -2.882268652242222284, 31.66798894389554064 ) ) ;
#83156=CARTESIAN_POINT ( 'NONE',  ( -6.066082379360134169, -3.322132147404559976, 32.92929555188719348 ) ) ;
#83157=EDGE_CURVE ( 'NONE', #16191, #43656, #33088, .T. ) ;
#83160=AXIS2_PLACEMENT_3D ( 'NONE', #18748, #72785, #25938 ) ;
#83163=CARTESIAN_POINT ( 'NONE',  ( -9.442362173959550020, -11.37275283266504111, 32.91324779482534524 ) ) ;
#83164=ORIENTED_EDGE ( 'NONE', *, *, #4330, .F. ) ;
#83165=CARTESIAN_POINT ( 'NONE',  ( 7.173076923078359535, -7.500000000000155431, 34.75000000000007105 ) ) ;
#83166=CARTESIAN_POINT ( 'NONE',  ( -14.43783951713052716, -11.47017969459904130, 32.78971311882034456 ) ) ;
#83167=CARTESIAN_POINT ( 'NONE',  ( 2.057669070399344324, -2.823816976329320827, 31.52131813110797154 ) ) ;
#83168=ORIENTED_EDGE ( 'NONE', *, *, #84696, .F. ) ;
#83169=CARTESIAN_POINT ( 'NONE',  ( -7.911477858958151366, -7.749976730030849303, 34.74374725381503737 ) ) ;
#83171=DIRECTION ( 'NONE',  ( 0.000000000000000000, 0.000000000000000000, 1.000000000000000000 ) ) ;
#83172=B_SPLINE_CURVE_WITH_KNOTS ( 'NONE', 3,
 ( #43721, #42851, #43290, #28903, #70761, #83847, #9066, #70313, #84733, #63983 ),
 .UNSPECIFIED., .F., .F.,
 ( 4, 2, 2, 2, 4 ),
 ( 0.0007817246256747516176, 0.0009771112852218965736, 0.001172497944769041638, 0.001367884604316186702, 0.001563271263863331550 ),
 .UNSPECIFIED. ) ;
#83173=CARTESIAN_POINT ( 'NONE',  ( 5.076923076922954969, -6.026961402154118908, 34.52809138561165270 ) ) ;
#83174=CARTESIAN_POINT ( 'NONE',  ( -16.85391172531022264, -2.758310577978207334, 31.33698337089302299 ) ) ;
#83176=LINE ( 'NONE', #32541, #549 ) ;
#83178=EDGE_CURVE ( 'NONE', #63622, #69827, #8646, .T. ) ;
#83179=ORIENTED_EDGE ( 'NONE', *, *, #16938, .T. ) ;
#83180=DIRECTION ( 'NONE',  ( -0.000000000000000000, 0.5000000000000011102, -0.8660254037844381525 ) ) ;
#83181=VERTEX_POINT ( 'NONE', #12234 ) ;
#83183=CARTESIAN_POINT ( 'NONE',  ( -4.153846153846274980, -11.06231777344772027, 33.60647404775119895 ) ) ;
#83184=CARTESIAN_POINT ( 'NONE',  ( 6.923076923076924238, -2.721908614388771852, 31.22303859784724978 ) ) ;
#83185=DIRECTION ( 'NONE',  ( -0.000000000000000000, 1.000000000000000000, 3.491481338843133355E-15 ) ) ;
#83186=CARTESIAN_POINT ( 'NONE',  ( -16.82692307692165556, -7.500000000000154543, 35.00000000000007105 ) ) ;
#83188=ORIENTED_EDGE ( 'NONE', *, *, #78349, .F. ) ;
#83189=DIRECTION ( 'NONE',  ( -0.000000000000000000, 0.9848077530122085754, -0.1736481776669273613 ) ) ;
#83190=ORIENTED_EDGE ( 'NONE', *, *, #23569, .F. ) ;
#83191=VERTEX_POINT ( 'NONE', #19874 ) ;
#83192=AXIS2_PLACEMENT_3D ( 'NONE', #50520, #51382, #78886 ) ;
#83193=ORIENTED_EDGE ( 'NONE', *, *, #52421, .F. ) ;
#83194=CARTESIAN_POINT ( 'NONE',  ( -7.976301055592065481, -5.195881422630166391, 34.18770438780619259 ) ) ;
#83195=VERTEX_POINT ( 'NONE', #25302 ) ;
#83196=CARTESIAN_POINT ( 'NONE',  ( 4.376857505459002873, -5.667800583137508674, 34.40243808032445827 ) ) ;
#83197=CARTESIAN_POINT ( 'NONE',  ( -8.769230769230768274, -13.20930481340135110, 34.54067556320372745 ) ) ;
#83198=B_SPLINE_CURVE_WITH_KNOTS ( 'NONE', 3,
 ( #24449, #2405, #16813, #64988, #4186, #44266, #9614, #50147, #57359, #3293 ),
 .UNSPECIFIED., .F., .F.,
 ( 4, 2, 2, 2, 4 ),
 ( 0.000000000000000000, 0.0001954311564186866576, 0.0003908623128373733152, 0.0005862934692560599998, 0.0007817246256747466303 ),
 .UNSPECIFIED. ) ;
#83199=CARTESIAN_POINT ( 'NONE',  ( 4.153846153846154188, -4.098570777380720287, 33.41473453929634729 ) ) ;
#83200=CARTESIAN_POINT ( 'NONE',  ( 14.08486421005743061, -7.369209533119137845, 34.99857337881830688 ) ) ;
#83201=ORIENTED_EDGE ( 'NONE', *, *, #23145, .F. ) ;
#83203=EDGE_LOOP ( 'NONE', ( #81122, #33952 ) ) ;
#83205=CARTESIAN_POINT ( 'NONE',  ( -14.17716686945866655, -2.372941743896879174, 30.88044141588253666 ) ) ;
#83206=EDGE_LOOP ( 'NONE', ( #52445, #69250 ) ) ;
#83207=CARTESIAN_POINT ( 'NONE',  ( 9.468822748583747284, -11.89387501736622710, 32.13663884655806413 ) ) ;
#83208=B_SPLINE_CURVE_WITH_KNOTS ( 'NONE', 3,
 ( #43472, #43032, #70503, #29963, #84916, #31745, #25873, #4263, #19118, #26315 ),
 .UNSPECIFIED., .F., .F.,
 ( 4, 2, 2, 2, 4 ),
 ( 0.0007817246256747459798, 0.0009771112852218896347, 0.001172497944769033181, 0.001367884604316176728, 0.001563271263863320274 ),
 .UNSPECIFIED. ) ;
#83209=DIRECTION ( 'NONE',  ( -1.000000000000000000, -0.000000000000000000, -0.000000000000000000 ) ) ;
#83210=ORIENTED_EDGE ( 'NONE', *, *, #34538, .F. ) ;
#83211=DIRECTION ( 'NONE',  ( -0.000000000000000000, 0.1736481776669307198, -0.9848077530122080203 ) ) ;
#83212=CARTESIAN_POINT ( 'NONE',  ( -15.09997878980228414, -12.35292014791297710, 31.75344720912887198 ) ) ;
#83213=AXIS2_PLACEMENT_3D ( 'NONE', #39155, #11675, #81470 ) ;
#83215=FACE_BOUND ( 'NONE', #48976, .T. ) ;
#83216=CARTESIAN_POINT ( 'NONE',  ( 15.48082365068267841, -11.47946981652013498, 33.17500667209847620 ) ) ;
#83217=CYLINDRICAL_SURFACE ( 'NONE', #25549, 0.2499999999999998890 ) ;
#83218=DIRECTION ( 'NONE',  ( -1.000000000000000000, 0.000000000000000000, 0.000000000000000000 ) ) ;
#83219=CARTESIAN_POINT ( 'NONE',  ( -6.857931143744957936, -7.750023238201980469, 34.74374492549440419 ) ) ;
#83220=CARTESIAN_POINT ( 'NONE',  ( -0.4615384615384611200, -12.10708131394839349, 31.69288490824020244 ) ) ;
#83221=CARTESIAN_POINT ( 'NONE',  ( -2.980823821391187067, -3.520799739797214389, 33.17531984108286025 ) ) ;
#83222=LINE ( 'NONE', #43549, #29041 ) ;
#83223=VERTEX_POINT ( 'NONE', #47340 ) ;
#83224=CARTESIAN_POINT ( 'NONE',  ( 14.30769230769218758, -12.46129190930018460, 30.37095296980731973 ) ) ;
#83226=EDGE_LOOP ( 'NONE', ( #9706, #32948 ) ) ;
#83227=EDGE_CURVE ( 'NONE', #5662, #57710, #77396, .T. ) ;
#83228=EDGE_CURVE ( 'NONE', #71718, #85122, #84897, .T. ) ;
#83232=CARTESIAN_POINT ( 'NONE',  ( 11.31553457955469000, -10.01117774369187252, 34.36070679894347535 ) ) ;
#83233=CARTESIAN_POINT ( 'NONE',  ( -4.219928533206290133, -2.292212530054419606, 30.41441678777542634 ) ) ;
#83234=FACE_BOUND ( 'NONE', #47190, .T. ) ;
#83235=CARTESIAN_POINT ( 'NONE',  ( 6.792928953345226617, -4.299443229763728169, 33.91186481527756058 ) ) ;
#83236=CARTESIAN_POINT ( 'NONE',  ( -3.903791842207837259, -8.303483539816728154, 34.68545999027711702 ) ) ;
#83237=CARTESIAN_POINT ( 'NONE',  ( 7.976679284387491187, -11.66157788607254098, 32.95092075102925833 ) ) ;
#83238=CARTESIAN_POINT ( 'NONE',  ( -5.999999999999998224, -13.53365097954675988, 30.81389545987213552 ) ) ;
#83239=CARTESIAN_POINT ( 'NONE',  ( 6.923076923076802558, -12.27809138561165270, 31.22303859784587132 ) ) ;
#83240=CARTESIAN_POINT ( 'NONE',  ( -3.230769230769229949, -9.584722331328613620, 36.20867863119891439 ) ) ;
#83242=ORIENTED_EDGE ( 'NONE', *, *, #65395, .F. ) ;
#83244=EDGE_CURVE ( 'NONE', #20327, #29327, #22680, .T. ) ;
#83245=AXIS2_PLACEMENT_3D ( 'NONE', #14010, #70734, #77050 ) ;
#83246=CARTESIAN_POINT ( 'NONE',  ( -9.442362173959548244, -11.86320923018887541, 32.19269448109604781 ) ) ;
#83247=CARTESIAN_POINT ( 'NONE',  ( 14.30769230769231015, -12.62096338111211580, 30.90682066428153263 ) ) ;
#83248=CARTESIAN_POINT ( 'NONE',  ( 4.153846153846154188, -8.564572088678739092, 35.78748833219616898 ) ) ;
#83249=CARTESIAN_POINT ( 'NONE',  ( 8.769230769230647482, -4.481592998941358097, 33.73612834414048933 ) ) ;
#83251=CARTESIAN_POINT ( 'NONE',  ( -16.85391172531022619, -6.503523203565941380, 34.64991518177335195 ) ) ;
#83253=CARTESIAN_POINT ( 'NONE',  ( 6.857806922520603976, -2.379036618887870436, 30.90682066428147934 ) ) ;
#83254=CARTESIAN_POINT ( 'NONE',  ( 18.00000000000000000, -2.249999999999998668, 29.75000000000001776 ) ) ;
#83256=CARTESIAN_POINT ( 'NONE',  ( -10.61538461538461320, -2.900454961884010974, 35.62045528018868623 ) ) ;
#83258=CARTESIAN_POINT ( 'NONE',  ( 10.83839745947801170, -3.395485233115139057, 33.02377354290275946 ) ) ;
#83259=CARTESIAN_POINT ( 'NONE',  ( -8.769230769230890843, -3.835265460704628371, 33.15142922262033665 ) ) ;
#83261=DIRECTION ( 'NONE',  ( -0.000000000000000000, 0.5000000000000011102, -0.8660254037844380415 ) ) ;
#83262=CARTESIAN_POINT ( 'NONE',  ( 12.71148387091650278, -2.341251567377310217, 30.72681386836322659 ) ) ;
#83263=AXIS2_PLACEMENT_3D ( 'NONE', #37342, #71573, #79235 ) ;
#83264=EDGE_CURVE ( 'NONE', #60387, #44924, #5031, .T. ) ;
#83265=CARTESIAN_POINT ( 'NONE',  ( 18.00000000000000000, -13.57706302396349152, 30.56769352161908060 ) ) ;
#83267=CARTESIAN_POINT ( 'NONE',  ( 12.46153846153833911, -4.320704448113951379, 33.92786785259630022 ) ) ;
#83268=CARTESIAN_POINT ( 'NONE',  ( 8.769230769230768274, -5.415277668671390821, 36.20867863119892149 ) ) ;
#83270=CARTESIAN_POINT ( 'NONE',  ( -5.869209559033048862, -12.35292014791297710, 31.75344720912887198 ) ) ;
#83271=DIRECTION ( 'NONE',  ( -0.000000000000000000, 0.7660444431189791237, -0.6427876096865379196 ) ) ;
#83272=ORIENTED_EDGE ( 'NONE', *, *, #4966, .F. ) ;
#83273=CARTESIAN_POINT ( 'NONE',  ( 2.980769230769232170, -7.500000000000001776, 34.75000000000000000 ) ) ;
#83274=CARTESIAN_POINT ( 'NONE',  ( -9.469528151039281028, -5.114059244376869984, 34.14424750095245287 ) ) ;
#83275=ORIENTED_EDGE ( 'NONE', *, *, #56694, .F. ) ;
#83276=CARTESIAN_POINT ( 'NONE',  ( 9.692307692308000711, -2.506253911140615021, 30.00000000000323297 ) ) ;
#83277=CARTESIAN_POINT ( 'NONE',  ( -2.307692307692305711, -10.67929555188718282, 33.92786785259544047 ) ) ;
#83278=VERTEX_POINT ( 'NONE', #38824 ) ;
#83279=CARTESIAN_POINT ( 'NONE',  ( -5.142193522883852452, -12.27809138561121394, 31.22303859784730307 ) ) ;
#83280=CARTESIAN_POINT ( 'NONE',  ( -6.923076923077045919, -11.67786785259630911, 32.92929555188603530 ) ) ;
#83281=ORIENTED_EDGE ( 'NONE', *, *, #29137, .T. ) ;
#83283=CARTESIAN_POINT ( 'NONE',  ( -16.40384615384615330, -7.500000000000001776, 34.75000000000000000 ) ) ;
#83285=CARTESIAN_POINT ( 'NONE',  ( 9.942253101685738059, -6.653508905675592722, 34.93172785388651391 ) ) ;
#83286=EDGE_LOOP ( 'NONE', ( #1610, #32261 ) ) ;
#83287=EDGE_CURVE ( 'NONE', #84018, #2381, #34315, .T. ) ;
#83288=EDGE_LOOP ( 'NONE', ( #3352, #2878, #10931, #81577 ) ) ;
#83289=CARTESIAN_POINT ( 'NONE',  ( 6.000000000000001776, -6.386643153685126251, 34.62446782046654192 ) ) ;
#83292=CARTESIAN_POINT ( 'NONE',  ( 7.716005876422150855, -9.504002272028873932, 34.60269587691767867 ) ) ;
#83293=EDGE_CURVE ( 'NONE', #37623, #76098, #33399, .T. ) ;
#83294=CARTESIAN_POINT ( 'NONE',  ( 15.45378207486262667, -12.64618726649961289, 30.78989965857442712 ) ) ;
#83295=CARTESIAN_POINT ( 'NONE',  ( 2.307692307692186251, -11.67786785259630911, 32.92929555188603530 ) ) ;
#83296=EDGE_CURVE ( 'NONE', #1437, #20693, #86988, .T. ) ;
#83297=CARTESIAN_POINT ( 'NONE',  ( -6.673022503163469565, -11.47946981652013498, 33.17500667209846910 ) ) ;
#83298=DIRECTION ( 'NONE',  ( -0.000000000000000000, 0.8660254037844399289, -0.4999999999999980016 ) ) ;
#83301=EDGE_LOOP ( 'NONE', ( #63056, #36876 ) ) ;
#83302=VERTEX_POINT ( 'NONE', #49565 ) ;
#83303=CARTESIAN_POINT ( 'NONE',  ( 5.076923076922954969, -9.442884908241554243, 34.35708131394783038 ) ) ;
#83304=ORIENTED_EDGE ( 'NONE', *, *, #31409, .T. ) ;
#83305=B_SPLINE_CURVE_WITH_KNOTS ( 'NONE', 3,
 ( #42929, #63181, #1494, #56435, #70398, #8700, #63628, #77593, #50974, #51408 ),
 .UNSPECIFIED., .F., .F.,
 ( 4, 2, 2, 2, 4 ),
 ( 0.0007817359430256297891, 0.0009771253907249958896, 0.001172514838424361990, 0.001367904286123728091, 0.001563293733823094191 ),
 .UNSPECIFIED. ) ;
#83309=VECTOR ( 'NONE', #78518, 1000.000000000000000 ) ;
#83310=CARTESIAN_POINT ( 'NONE',  ( 15.23076923076954614, -2.255955759149395501, 30.00000000000324363 ) ) ;
#83311=CARTESIAN_POINT ( 'NONE',  ( 7.846153846153846700, -4.786620604624113540, 33.94971097300155094 ) ) ;
#83312=VERTEX_POINT ( 'NONE', #48668 ) ;
#83313=DIRECTION ( 'NONE',  ( -0.000000000000000000, 0.5000000000000011102, -0.8660254037844380415 ) ) ;
#83314=AXIS2_PLACEMENT_3D ( 'NONE', #12857, #40341, #87652 ) ;
#83315=VERTEX_POINT ( 'NONE', #34720 ) ;
#83316=CARTESIAN_POINT ( 'NONE',  ( -16.28399336328437386, -3.817052484675422797, 33.13202310037935661 ) ) ;
#83317=ORIENTED_EDGE ( 'NONE', *, *, #85558, .F. ) ;
#83318=VECTOR ( 'NONE', #74079, 1000.000000000000114 ) ;
#83319=CARTESIAN_POINT ( 'NONE',  ( -10.36538461538317790, -7.500000000000155431, 34.75000000000007105 ) ) ;
#83321=ORIENTED_EDGE ( 'NONE', *, *, #25992, .F. ) ;
#83322=CARTESIAN_POINT ( 'NONE',  ( -6.673022503163469565, -4.818054556918156095, 34.26375889529406749 ) ) ;
#83324=FACE_BOUND ( 'NONE', #82839, .T. ) ;
#83325=CARTESIAN_POINT ( 'NONE',  ( 5.869852030268306819, -2.373036134822904319, 30.88089517874952250 ) ) ;
#83326=DIRECTION ( 'NONE',  ( -0.000000000000000000, -0.5000000000000011102, -0.8660254037844381525 ) ) ;
#83327=CYLINDRICAL_SURFACE ( 'NONE', #76928, 0.2500000000000002220 ) ;
#83329=CARTESIAN_POINT ( 'NONE',  ( -14.30769230769242739, -10.21337939537710326, 33.94971097300076224 ) ) ;
#83330=CARTESIAN_POINT ( 'NONE',  ( -16.15384615384627409, -2.657715359629662988, 31.77849191805970364 ) ) ;
#83332=CARTESIAN_POINT ( 'NONE',  ( 14.55763771707034948, -6.653508905675592722, 34.93172785388651391 ) ) ;
#83333=ORIENTED_EDGE ( 'NONE', *, *, #59061, .T. ) ;
#83334=EDGE_CURVE ( 'NONE', #69894, #31984, #5290, .T. ) ;
#83335=VERTEX_POINT ( 'NONE', #75698 ) ;
#83336=EDGE_CURVE ( 'NONE', #43893, #922, #18212, .T. ) ;
#83337=CARTESIAN_POINT ( 'NONE',  ( 9.561747778694329014, -2.254533558242299396, 29.97296025877828285 ) ) ;
#83338=CARTESIAN_POINT ( 'NONE',  ( 15.10007776410167324, -12.11776431015576172, 31.66791131148498906 ) ) ;
#83339=B_SPLINE_CURVE_WITH_KNOTS ( 'NONE', 3,
 ( #13607, #35205, #62663, #75741, #88847, #14943, #42421, #55038, #82958, #41082 ),
 .UNSPECIFIED., .F., .F.,
 ( 4, 2, 2, 2, 4 ),
 ( 0.000000000000000000, 0.0001954339857564074473, 0.0003908679715128148945, 0.0005863019572692223418, 0.0007817359430256297891 ),
 .UNSPECIFIED. ) ;
#83340=CARTESIAN_POINT ( 'NONE',  ( -11.53846153846153655, -11.69971097300155272, 32.46337939537588113 ) ) ;
#83341=CARTESIAN_POINT ( 'NONE',  ( -17.07692307692307665, -9.905515769479276145, 34.41647553114623292 ) ) ;
#83342=DIRECTION ( 'NONE',  ( -0.000000000000000000, -0.3420201433256694901, -0.9396926207859082059 ) ) ;
#83343=CARTESIAN_POINT ( 'NONE',  ( 13.63466969625370062, -11.28795663066794575, 33.01431243580653785 ) ) ;
#83344=ORIENTED_EDGE ( 'NONE', *, *, #30761, .F. ) ;
#83345=CARTESIAN_POINT ( 'NONE',  ( 11.31497661389721010, -3.562934362175799841, 33.22335522853832401 ) ) ;
#83346=CYLINDRICAL_SURFACE ( 'NONE', #20033, 0.2499999999999997502 ) ;
#83347=CARTESIAN_POINT ( 'NONE',  ( -10.61538461538473399, -10.21337939537710326, 33.94971097300076224 ) ) ;
#83348=CARTESIAN_POINT ( 'NONE',  ( 2.980792499826878217, -3.137211980971222669, 32.19342716148376837 ) ) ;
#83349=CARTESIAN_POINT ( 'NONE',  ( -11.66902213020345513, -2.504760397472875155, 29.97295953869789997 ) ) ;
#83350=ORIENTED_EDGE ( 'NONE', *, *, #8544, .F. ) ;
#83351=VERTEX_POINT ( 'NONE', #82480 ) ;
#83352=ORIENTED_EDGE ( 'NONE', *, *, #51684, .F. ) ;
#83354=CARTESIAN_POINT ( 'NONE',  ( -6.249976744048591826, -4.075325502946086864, 33.72974371597207721 ) ) ;
#83355=EDGE_LOOP ( 'NONE', ( #32604, #84296 ) ) ;
#83356=CARTESIAN_POINT ( 'NONE',  ( -17.07692307692307665, -13.88283147151868846, 33.14645433367849847 ) ) ;
#83357=CARTESIAN_POINT ( 'NONE',  ( -17.20761454359064047, -3.062553014421049991, 32.05460306192773601 ) ) ;
#83358=CARTESIAN_POINT ( 'NONE',  ( -2.057692307690870415, -7.500000000000155431, 34.75000000000007105 ) ) ;
#83359=ADVANCED_FACE ( 'NONE', ( #35613 ), #42378, .F. ) ;
#83361=CARTESIAN_POINT ( 'NONE',  ( -11.47320596718551400, -6.879047030191282275, 34.71129190930002295 ) ) ;
#83362=ORIENTED_EDGE ( 'NONE', *, *, #65556, .T. ) ;
#83363=CARTESIAN_POINT ( 'NONE',  ( -10.61538461538473577, -4.320704448113951379, 33.92786785259630022 ) ) ;
#83364=CARTESIAN_POINT ( 'NONE',  ( -12.33101275977489841, -11.93748526763465279, 32.05452791011430946 ) ) ;
#83366=DIRECTION ( 'NONE',  ( -0.000000000000000000, -0.9848077530122086864, -0.1736481776669273613 ) ) ;
#83367=CYLINDRICAL_SURFACE ( 'NONE', #80091, 0.2499999999999979738 ) ;
#83368=CARTESIAN_POINT ( 'NONE',  ( 17.07692307692295586, -11.48612834414049644, 32.76840700105863391 ) ) ;
#83369=CARTESIAN_POINT ( 'NONE',  ( 15.29602437028207085, -3.083524468853784839, 32.58852847137153930 ) ) ;
#83371=CARTESIAN_POINT ( 'NONE',  ( 9.562160482869472844, -10.19110544564092002, 33.96427741523702792 ) ) ;
#83373=DIRECTION ( 'NONE',  ( 0.000000000000000000, 0.1736481776669267785, -0.9848077530122087975 ) ) ;
#83375=VERTEX_POINT ( 'NONE', #565 ) ;
#83376=CARTESIAN_POINT ( 'NONE',  ( -15.48079245499068612, -6.652501968072648708, 34.93155406624980941 ) ) ;
#83377=CARTESIAN_POINT ( 'NONE',  ( -14.08467946359890988, -3.395485233115139057, 33.02377354290275946 ) ) ;
#83378=B_SPLINE_CURVE_WITH_KNOTS ( 'NONE', 3,
 ( #35306, #21350, #15489, #61440, #83061, #61884 ),
 .UNSPECIFIED., .F., .F.,
 ( 4, 2, 4 ),
 ( 0.000000000000000000, 0.0001954784845028707536, 0.0003909569690057415072 ),
 .UNSPECIFIED. ) ;
#83379=B_SPLINE_CURVE_WITH_KNOTS ( 'NONE', 3,
 ( #11112, #37691, #79129, #30924, #44885, #85888, #52090, #71471, #31839, #85008 ),
 .UNSPECIFIED., .F., .F.,
 ( 4, 2, 2, 2, 4 ),
 ( 0.000000000000000000, 0.0001954339857564083688, 0.0003908679715128167377, 0.0005863019572692250523, 0.0007817359430256334753 ),
 .UNSPECIFIED. ) ;
#83380=CARTESIAN_POINT ( 'NONE',  ( 9.019176178608812933, -10.92531984108285670, 33.72920026020278073 ) ) ;
#83382=B_SPLINE_CURVE_WITH_KNOTS ( 'NONE', 3,
 ( #69167, #55200, #14668, #20964, #61510, #76360, #84028, #42150, #15114, #83130 ),
 .UNSPECIFIED., .F., .F.,
 ( 4, 2, 2, 2, 4 ),
 ( 0.0007817246256747516176, 0.0009771112852218965736, 0.001172497944769041421, 0.001367884604316186269, 0.001563271263863331333 ),
 .UNSPECIFIED. ) ;
#83383=ORIENTED_EDGE ( 'NONE', *, *, #27913, .F. ) ;
#83384=CARTESIAN_POINT ( 'NONE',  ( 3.230769230769110045, -11.94971097300221174, 32.03036669348237098 ) ) ;
#83385=EDGE_CURVE ( 'NONE', #85101, #58822, #65417, .T. ) ;
#83386=B_SPLINE_CURVE_WITH_KNOTS ( 'NONE', 3,
 ( #60422, #11803, #81593, #32067, #81155, #33837, #5931, #40611, #68080, #25756 ),
 .UNSPECIFIED., .F., .F.,
 ( 4, 2, 2, 2, 4 ),
 ( 0.000000000000000000, 0.0001954339857564073388, 0.0003908679715128146777, 0.0005863019572692220165, 0.0007817359430256293554 ),
 .UNSPECIFIED. ) ;
#83387=VECTOR ( 'NONE', #54432, 1000.000000000000114 ) ;
#83388=AXIS2_PLACEMENT_3D ( 'NONE', #87107, #18187, #3324 ) ;
#83389=CARTESIAN_POINT ( 'NONE',  ( -1.319359813339359366, -6.879047030191282275, 34.71129190930002295 ) ) ;
#83390=FACE_OUTER_BOUND ( 'NONE', #87489, .T. ) ;
#83392=ORIENTED_EDGE ( 'NONE', *, *, #63579, .T. ) ;
#83393=CARTESIAN_POINT ( 'NONE',  ( -16.15384615384627409, -6.835583212225970762, 34.95778746994575670 ) ) ;
#83394=EDGE_CURVE ( 'NONE', #30224, #52884, #33204, .T. ) ;
#83395=CYLINDRICAL_SURFACE ( 'NONE', #75694, 0.2500000000000008882 ) ;
#83397=EDGE_LOOP ( 'NONE', ( #6962, #23035 ) ) ;
#83398=CARTESIAN_POINT ( 'NONE',  ( -2.557669051740896649, -12.01397095200673881, 32.43157075238190146 ) ) ;
#83399=ADVANCED_FACE ( 'NONE', ( #13629 ), #66012, .F. ) ;
#83400=VERTEX_POINT ( 'NONE', #11532 ) ;
#83401=CARTESIAN_POINT ( 'NONE',  ( 12.71159288145191013, -12.41089969410671223, 31.60739465890703670 ) ) ;
#83402=CARTESIAN_POINT ( 'NONE',  ( 13.38461538461538680, -8.564572088678739092, 35.78748833219616898 ) ) ;
#83403=ORIENTED_EDGE ( 'NONE', *, *, #36992, .F. ) ;
#83404=ADVANCED_FACE ( 'NONE', ( #55501 ), #39015, .F. ) ;
#83405=DIRECTION ( 'NONE',  ( -0.000000000000000000, -0.7660444431189791237, -0.6427876096865379196 ) ) ;
#83406=CARTESIAN_POINT ( 'NONE',  ( 4.219913487196229163, -9.058645607665452459, 34.76329471203371924 ) ) ;
#83407=DIRECTION ( 'NONE',  ( 0.000000000000000000, 0.9396926207859126468, 0.3420201433256571111 ) ) ;
#83408=CARTESIAN_POINT ( 'NONE',  ( 1.254467414883690735, -6.809168938359898782, 34.95455904226513866 ) ) ;
#83409=CARTESIAN_POINT ( 'NONE',  ( -4.023055712879200385, -3.957578996910242619, 33.62503395064540257 ) ) ;
#83411=EDGE_LOOP ( 'NONE', ( #31002, #52708, #85336, #6649 ) ) ;
#83412=FACE_BOUND ( 'NONE', #76085, .T. ) ;
#83413=ORIENTED_EDGE ( 'NONE', *, *, #79797, .T. ) ;
#83414=B_SPLINE_CURVE_WITH_KNOTS ( 'NONE', 3,
 ( #25565, #73770, #12065, #39544, #67004, #46723, #82293, #75967, #88626, #81409 ),
 .UNSPECIFIED., .F., .F.,
 ( 4, 2, 2, 2, 4 ),
 ( 0.000000000000000000, 0.0001954311564186865763, 0.0003908623128373731525, 0.0005862934692560596746, 0.0007817246256747463051 ),
 .UNSPECIFIED. ) ;
#83415=CARTESIAN_POINT ( 'NONE',  ( -4.153846153846152411, -10.05456864172156806, 36.03766855953608683 ) ) ;
#83416=EDGE_CURVE ( 'NONE', #48963, #89081, #44979, .T. ) ;
#83417=DIRECTION ( 'NONE',  ( -0.000000000000000000, -0.000000000000000000, -1.000000000000000000 ) ) ;
#83418=EDGE_CURVE ( 'NONE', #81424, #28117, #8480, .T. ) ;
#83419=CARTESIAN_POINT ( 'NONE',  ( 6.066067333350077639, -2.833524468853757750, 32.15551576947925838 ) ) ;
#83420=CARTESIAN_POINT ( 'NONE',  ( 0.6845513056318558442, -12.64618726649961289, 30.78989965857442712 ) ) ;
#83421=ORIENTED_EDGE ( 'NONE', *, *, #27039, .T. ) ;
#83423=VERTEX_POINT ( 'NONE', #43324 ) ;
#83424=CARTESIAN_POINT ( 'NONE',  ( -0.2115929431903189328, -3.202959910592335202, 32.30730279482227019 ) ) ;
#83425=ORIENTED_EDGE ( 'NONE', *, *, #60193, .T. ) ;
#83426=ADVANCED_FACE ( 'NONE', ( #35229 ), #28941, .F. ) ;
#83427=CYLINDRICAL_SURFACE ( 'NONE', #17261, 0.2499999999999998890 ) ;
#83428=CARTESIAN_POINT ( 'NONE',  ( 1.634669696253700621, -3.627508038966689163, 32.91356715214248396 ) ) ;
#83429=ADVANCED_FACE ( 'NONE', ( #8660 ), #36568, .F. ) ;
#83430=B_SPLINE_CURVE_WITH_KNOTS ( 'NONE', 3,
 ( #2679, #38259, #86004, #30171, #85559, #65717, #9455, #45450, #37355, #64823 ),
 .UNSPECIFIED., .F., .F.,
 ( 4, 2, 2, 2, 4 ),
 ( 0.000000000000000000, 0.0001954311564186881213, 0.0003908623128373762425, 0.0005862934692560643367, 0.0007817246256747524850 ),
 .UNSPECIFIED. ) ;
#83431=CARTESIAN_POINT ( 'NONE',  ( -18.13069060311030611, -6.369640206132552329, 34.87707690430378449 ) ) ;
#83432=EDGE_LOOP ( 'NONE', ( #28687, #52336 ) ) ;
#83433=CARTESIAN_POINT ( 'NONE',  ( 8.769230769230647482, -9.442884908241554243, 34.35708131394783038 ) ) ;
#83434=EDGE_CURVE ( 'NONE', #65345, #82786, #63341, .T. ) ;
#83435=CARTESIAN_POINT ( 'NONE',  ( 14.30769230769231015, -8.973038597847269315, 34.52809138561121927 ) ) ;
#83436=CARTESIAN_POINT ( 'NONE',  ( 16.82692307692307665, -7.500000000000001776, 35.04278698407183867 ) ) ;
#83437=CARTESIAN_POINT ( 'NONE',  ( -11.76138775597768671, -3.105860786376062332, 32.13614157043599562 ) ) ;
#83438=ORIENTED_EDGE ( 'NONE', *, *, #80072, .T. ) ;
#83439=EDGE_LOOP ( 'NONE', ( #64779, #52681 ) ) ;
#83440=AXIS2_PLACEMENT_3D ( 'NONE', #73855, #74292, #39633 ) ;
#83441=VERTEX_POINT ( 'NONE', #83882 ) ;
#83443=CARTESIAN_POINT ( 'NONE',  ( -3.930834802233302394, -9.886259254753566594, 34.14407573483972413 ) ) ;
#83444=ADVANCED_FACE ( 'NONE', ( #22168 ), #50510, .F. ) ;
#83445=UNCERTAINTY_MEASURE_WITH_UNIT (LENGTH_MEASURE( 1.000000000000000082E-05 ), #81033, 'distance_accuracy_value', 'NONE');
#83446=DIRECTION ( 'NONE',  ( 0.000000000000000000, 1.000000000000000000, 0.000000000000000000 ) ) ;
#83447=CARTESIAN_POINT ( 'NONE',  ( -13.63459211555773720, -5.728515186090277211, 34.42611988154120439 ) ) ;
#83448=AXIS2_PLACEMENT_3D ( 'NONE', #62763, #83959, #35307 ) ;
#83449=CYLINDRICAL_SURFACE ( 'NONE', #37034, 0.2499999999999998890 ) ;
#83450=CARTESIAN_POINT ( 'NONE',  ( 14.30769230769231015, -4.102666532097928531, 36.13435417666054406 ) ) ;
#83451=CARTESIAN_POINT ( 'NONE',  ( -11.53846153846153655, -3.886160181151819604, 36.00935417666054406 ) ) ;
#83452=CARTESIAN_POINT ( 'NONE',  ( 3.230769230769231726, -2.900454961884010974, 35.62045528018868623 ) ) ;
#83453=ORIENTED_EDGE ( 'NONE', *, *, #7328, .F. ) ;
#83454=CARTESIAN_POINT ( 'NONE',  ( -7.781009065434213667, -7.750023224968868085, 34.99404313364389907 ) ) ;
#83455=CARTESIAN_POINT ( 'NONE',  ( 10.61538461538449418, -10.33852847137269571, 34.16647553114546554 ) ) ;
#83456=DIRECTION ( 'NONE',  ( -0.000000000000000000, -0.000000000000000000, -1.000000000000000000 ) ) ;
#83458=ORIENTED_EDGE ( 'NONE', *, *, #42653, .T. ) ;
#83460=VERTEX_POINT ( 'NONE', #85202 ) ;
#83461=FACE_BOUND ( 'NONE', #45310, .T. ) ;
#83462=CARTESIAN_POINT ( 'NONE',  ( -18.00000000000000000, -2.486705287966279876, 31.30864560766543647 ) ) ;
#83463=DIRECTION ( 'NONE',  ( -0.000000000000000000, -0.9396926207859092051, -0.3420201433256662704 ) ) ;
#83464=LINE ( 'NONE', #22194, #67758 ) ;
#83465=ORIENTED_EDGE ( 'NONE', *, *, #35482, .T. ) ;
#83466=CARTESIAN_POINT ( 'NONE',  ( 11.53846153846141576, -11.06231777344772027, 33.60647404775119895 ) ) ;
#83467=CARTESIAN_POINT ( 'NONE',  ( 15.45354889974729318, -2.353885683473779800, 30.79025554430704403 ) ) ;
#83468=CARTESIAN_POINT ( 'NONE',  ( -15.10024379253558457, -10.31582465632705237, 34.18122507451815295 ) ) ;
#83470=CARTESIAN_POINT ( 'NONE',  ( 6.130791807824788719, -3.530189275343204702, 32.79018710029569661 ) ) ;
#83472=DIRECTION ( 'NONE',  ( 0.000000000000000000, 0.7660444431189822323, -0.6427876096865344779 ) ) ;
#83473=ORIENTED_EDGE ( 'NONE', *, *, #53870, .T. ) ;
#83474=CARTESIAN_POINT ( 'NONE',  ( -8.992715712954719720, -3.754499324213721234, 33.06261337010820256 ) ) ;
#83475=VERTEX_POINT ( 'NONE', #1890 ) ;
#83476=CARTESIAN_POINT ( 'NONE',  ( 7.622668902429898807, -10.81261337010820256, 33.49550067578627477 ) ) ;
#83477=CARTESIAN_POINT ( 'NONE',  ( -6.923076923077044142, -11.94971097300221174, 32.03036669348237098 ) ) ;
#83478=CARTESIAN_POINT ( 'NONE',  ( -6.923076923076922462, -1.129524287112498415, 32.06866353760679544 ) ) ;
#83479=CARTESIAN_POINT ( 'NONE',  ( -13.38461538461538325, -9.058645607665452459, 34.76329471203371924 ) ) ;
#83480=CARTESIAN_POINT ( 'NONE',  ( 16.82689985270161515, -4.931416488878822335, 34.32920672191015399 ) ) ;
#83481=B_SPLINE_CURVE_WITH_KNOTS ( 'NONE', 3,
 ( #36872, #83756, #22042, #50815, #84641, #76988, #64335, #22916, #15290, #70226 ),
 .UNSPECIFIED., .F., .F.,
 ( 4, 2, 2, 2, 4 ),
 ( 0.000000000000000000, 0.0001954311564186861697, 0.0003908623128373723394, 0.0005862934692560584820, 0.0007817246256747446788 ),
 .UNSPECIFIED. ) ;
#83482=CARTESIAN_POINT ( 'NONE',  ( -5.999999999999998224, -6.343179335718451384, 34.87096338111211935 ) ) ;
#83483=CARTESIAN_POINT ( 'NONE',  ( 16.37685750545900376, -5.667800583137506898, 34.40243808032445827 ) ) ;
#83484=DIRECTION ( 'NONE',  ( 0.000000000000000000, -1.000000000000000000, 0.000000000000000000 ) ) ;
#83485=AXIS2_PLACEMENT_3D ( 'NONE', #35182, #62639, #21668 ) ;
#83487=EDGE_LOOP ( 'NONE', ( #4329, #88532 ) ) ;
#83488=CARTESIAN_POINT ( 'NONE',  ( -16.21992853320628925, -4.661471528628507777, 34.16647553114621871 ) ) ;
#83491=CARTESIAN_POINT ( 'NONE',  ( -8.769230769230892619, -6.835583212225970762, 34.95778746994575670 ) ) ;
#83492=ORIENTED_EDGE ( 'NONE', *, *, #30241, .F. ) ;
#83493=CARTESIAN_POINT ( 'NONE',  ( 10.68063975489745232, -8.656820664281605460, 34.87096338111211224 ) ) ;
#83494=CARTESIAN_POINT ( 'NONE',  ( 3.230769230769110045, -8.613356846316285953, 34.62446782046622218 ) ) ;
#83495=CARTESIAN_POINT ( 'NONE',  ( -6.923076923077045919, -9.528491918059723176, 34.59228464037033035 ) ) ;
#83496=CARTESIAN_POINT ( 'NONE',  ( -4.853911725310227077, -3.587049720035815348, 32.86302985866382897 ) ) ;
#83497=CARTESIAN_POINT ( 'NONE',  ( 12.23861224402231684, -10.61292498521070549, 33.66303323003028680 ) ) ;
#83498=CARTESIAN_POINT ( 'NONE',  ( -8.992157728137618378, -2.889293201056495786, 32.26117774369186009 ) ) ;
#83499=CARTESIAN_POINT ( 'NONE',  ( -10.61538461538461320, -2.486705287966279876, 31.30864560766543647 ) ) ;
#83501=CARTESIAN_POINT ( 'NONE',  ( 6.923076923076924238, -13.49023893513002648, 31.06009739812518688 ) ) ;
#83503=CARTESIAN_POINT ( 'NONE',  ( 5.869852030268305931, -11.66186481527757479, 32.95055677023626117 ) ) ;
#83504=CARTESIAN_POINT ( 'NONE',  ( -9.757577692864012775, -3.643525952247789412, 33.31231777344662959 ) ) ;
#83505=EDGE_CURVE ( 'NONE', #78089, #62624, #29378, .T. ) ;
#83508=ORIENTED_EDGE ( 'NONE', *, *, #8332, .T. ) ;
#83509=VERTEX_POINT ( 'NONE', #83435 ) ;
#83510=CARTESIAN_POINT ( 'NONE',  ( -18.25002322422145440, -2.588893531581426544, 31.60682220781847818 ) ) ;
#83511=DIRECTION ( 'NONE',  ( -0.000000000000000000, -0.9848077530122086864, -0.1736481776669273613 ) ) ;
#83512=CARTESIAN_POINT ( 'NONE',  ( 5.869852790561781219, -6.001485441113818986, 34.52039167877662607 ) ) ;
#83513=ORIENTED_EDGE ( 'NONE', *, *, #85740, .T. ) ;
#83515=B_SPLINE_CURVE_WITH_KNOTS ( 'NONE', 3,
 ( #15318, #42795, #20737, #75675, #70254, #48203, #84233, #63927, #13980, #41458 ),
 .UNSPECIFIED., .F., .F.,
 ( 4, 2, 2, 2, 4 ),
 ( 0.000000000000000000, 0.0001954311564186864678, 0.0003908623128373729357, 0.0005862934692560594577, 0.0007817246256747458714 ),
 .UNSPECIFIED. ) ;
#83516=VECTOR ( 'NONE', #57882, 1000.000000000000000 ) ;
#83517=CARTESIAN_POINT ( 'NONE',  ( 9.692307692307695177, -11.35647404775217417, 33.31231777344666511 ) ) ;
#83519=PLANE ( 'NONE',  #19700 ) ;
#83520=EDGE_CURVE ( 'NONE', #68189, #54936, #41694, .T. ) ;
#83522=LINE ( 'NONE', #9190, #32243 ) ;
#83524=CARTESIAN_POINT ( 'NONE',  ( 14.30769230769231015, -2.833524468853757305, 32.15551576947925838 ) ) ;
#83525=EDGE_LOOP ( 'NONE', ( #14524, #20447, #61709, #25596 ) ) ;
#83526=ADVANCED_FACE ( 'NONE', ( #62688 ), #45976, .F. ) ;
#83529=DIRECTION ( 'NONE',  ( 1.000000000000000000, 0.000000000000000000, 0.000000000000000000 ) ) ;
#83531=CARTESIAN_POINT ( 'NONE',  ( -6.673131513698880468, -2.589246495874657938, 31.60778113518102828 ) ) ;
#83532=EDGE_LOOP ( 'NONE', ( #85321, #82026, #47078, #63091 ) ) ;
#83533=VERTEX_POINT ( 'NONE', #37895 ) ;
#83534=ORIENTED_EDGE ( 'NONE', *, *, #35727, .T. ) ;
#83535=ORIENTED_EDGE ( 'NONE', *, *, #54929, .F. ) ;
#83536=CARTESIAN_POINT ( 'NONE',  ( -17.14219352288385778, -10.90142922261923886, 33.41473453929638993 ) ) ;
#83537=CARTESIAN_POINT ( 'NONE',  ( 13.63466969625370417, -9.943054286541403997, 34.11300777759954883 ) ) ;
#83539=ADVANCED_FACE ( 'NONE', ( #80221 ), #9971, .F. ) ;
#83541=CARTESIAN_POINT ( 'NONE',  ( 11.40831432902331599, -12.27039167877662251, 31.24851455888617835 ) ) ;
#83542=B_SPLINE_CURVE_WITH_KNOTS ( 'NONE', 3,
 ( #39808, #73601, #67276, #74472, #19524, #66381, #5571, #60511, #88023, #26283 ),
 .UNSPECIFIED., .F., .F.,
 ( 4, 2, 2, 2, 4 ),
 ( 0.0007817246256747450040, 0.0009771112852218881168, 0.001172497944769031230, 0.001367884604316174342, 0.001563271263863317455 ),
 .UNSPECIFIED. ) ;
#83543=CARTESIAN_POINT ( 'NONE',  ( 4.376857505459002873, -6.503523203565942268, 34.64991518177335195 ) ) ;
#83544=DIRECTION ( 'NONE',  ( -0.000000000000000000, 0.5000000000000011102, -0.8660254037844380415 ) ) ;
#83545=ORIENTED_EDGE ( 'NONE', *, *, #354, .F. ) ;
#83546=B_SPLINE_CURVE_WITH_KNOTS ( 'NONE', 3,
 ( #21578, #7187, #63448, #35092, #55363, #49049, #83741, #49929, #62553, #54927 ),
 .UNSPECIFIED., .F., .F.,
 ( 4, 2, 2, 2, 4 ),
 ( 0.0007817359430256294638, 0.0009771253907249950223, 0.001172514838424360472, 0.001367904286123725922, 0.001563293733823091372 ),
 .UNSPECIFIED. ) ;
#83547=EDGE_LOOP ( 'NONE', ( #48153, #58484, #58951, #82806 ) ) ;
#83548=ORIENTED_EDGE ( 'NONE', *, *, #54341, .F. ) ;
#83549=CARTESIAN_POINT ( 'NONE',  ( 12.46153846153833911, -8.613356846316285953, 34.62446782046622218 ) ) ;
#83552=DIRECTION ( 'NONE',  ( -0.000000000000000000, -0.7660444431189791237, -0.6427876096865379196 ) ) ;
#83553=CARTESIAN_POINT ( 'NONE',  ( -5.300408001487407539, -12.69144148231606017, 30.53333754910549303 ) ) ;
#83556=ORIENTED_EDGE ( 'NONE', *, *, #46754, .T. ) ;
#83557=EDGE_CURVE ( 'NONE', #65490, #12295, #18878, .T. ) ;
#83558=EDGE_CURVE ( 'NONE', #41513, #26582, #74050, .T. ) ;
#83560=ORIENTED_EDGE ( 'NONE', *, *, #2273, .F. ) ;
#83561=CARTESIAN_POINT ( 'NONE',  ( 13.51466054745016621, -2.504778602574659896, 29.97347330155780654 ) ) ;
#83562=VERTEX_POINT ( 'NONE', #10426 ) ;
#83563=FACE_BOUND ( 'NONE', #59606, .T. ) ;
#83564=CARTESIAN_POINT ( 'NONE',  ( -1.319421402832027912, -2.506253911140448043, 29.99999999999988631 ) ) ;
#83565=VECTOR ( 'NONE', #42661, 1000.000000000000000 ) ;
#83566=VECTOR ( 'NONE', #34594, 1000.000000000000114 ) ;
#83567=CARTESIAN_POINT ( 'NONE',  ( -8.769230769230768274, -11.33034616979429110, 35.88435417666054406 ) ) ;
#83568=EDGE_LOOP ( 'NONE', ( #36086, #48394 ) ) ;
#83569=CARTESIAN_POINT ( 'NONE',  ( 15.36160756125598681, -7.277220318596961057, 34.99547417642776992 ) ) ;
#83570=CYLINDRICAL_SURFACE ( 'NONE', #1534, 0.2499999999999993616 ) ;
#83571=CARTESIAN_POINT ( 'NONE',  ( 10.39189967166067063, -2.847400154188068022, 31.58180166144859058 ) ) ;
#83573=DIRECTION ( 'NONE',  ( -0.000000000000000000, 0.5000000000000011102, -0.8660254037844380415 ) ) ;
#83574=ADVANCED_FACE ( 'NONE', ( #5004 ), #59046, .F. ) ;
#83575=EDGE_LOOP ( 'NONE', ( #71319, #29716 ) ) ;
#83576=CARTESIAN_POINT ( 'NONE',  ( -11.28840711854808632, -12.41089969410671223, 31.60739465890703670 ) ) ;
#83577=CARTESIAN_POINT ( 'NONE',  ( 14.30769230769231015, -2.900454961884010974, 35.62045528018868623 ) ) ;
#83578=CARTESIAN_POINT ( 'NONE',  ( 2.307692307692309264, -1.117168528481311540, 33.14645433367849847 ) ) ;
#83580=ADVANCED_FACE ( 'NONE', ( #3213 ), #72561, .F. ) ;
#83581=DIRECTION ( 'NONE',  ( -0.000000000000000000, -0.000000000000000000, -1.000000000000000000 ) ) ;
#83582=EDGE_CURVE ( 'NONE', #52308, #3410, #78874, .T. ) ;
#83583=FACE_BOUND ( 'NONE', #21573, .T. ) ;
#83584=CARTESIAN_POINT ( 'NONE',  ( -6.673022503163470454, -12.65882529074907126, 30.72640787790839312 ) ) ;
#83585=CARTESIAN_POINT ( 'NONE',  ( -6.130690603110309667, -9.929715669179216775, 34.40415004197138416 ) ) ;
#83586=B_SPLINE_CURVE_WITH_KNOTS ( 'NONE', 3,
 ( #18453, #5824, #19339, #40942, #74736, #87369, #33302, #13022, #47691, #6274 ),
 .UNSPECIFIED., .F., .F.,
 ( 4, 2, 2, 2, 4 ),
 ( 0.000000000000000000, 0.0001954339857564078809, 0.0003908679715128157619, 0.0005863019572692236428, 0.0007817359430256315238 ),
 .UNSPECIFIED. ) ;
#83587=CARTESIAN_POINT ( 'NONE',  ( -7.053768389744485390, -12.11776431015576172, 31.66791131148498906 ) ) ;
#83588=CARTESIAN_POINT ( 'NONE',  ( 4.088576153289833925, -5.941354392334500467, 34.76329471203369792 ) ) ;
#83589=CARTESIAN_POINT ( 'NONE',  ( -6.065270445960775803, -5.219633306516282545, 34.19971097300152252 ) ) ;
#83590=B_SPLINE_CURVE_WITH_KNOTS ( 'NONE', 3,
 ( #52523, #37682, #45773, #66496, #24162, #4799 ),
 .UNSPECIFIED., .F., .F.,
 ( 4, 2, 4 ),
 ( 4.563551064100006665E-17, 0.0001954756301637168570, 0.0003909512603273880690 ),
 .UNSPECIFIED. ) ;
#83591=CARTESIAN_POINT ( 'NONE',  ( -0.4615384615385826339, -11.94971097300221174, 32.03036669348237098 ) ) ;
#83593=EDGE_CURVE ( 'NONE', #37632, #84179, #54719, .T. ) ;
#83594=ORIENTED_EDGE ( 'NONE', *, *, #79985, .F. ) ;
#83596=ORIENTED_EDGE ( 'NONE', *, *, #77740, .T. ) ;
#83597=CARTESIAN_POINT ( 'NONE',  ( -13.16160254052199008, -9.172514111537584114, 34.72667873470787470 ) ) ;
#83598=ORIENTED_EDGE ( 'NONE', *, *, #80169, .T. ) ;
#83599=CARTESIAN_POINT ( 'NONE',  ( -11.28851602011339850, -2.824170634883621744, 31.52227843825338738 ) ) ;
#83600=CARTESIAN_POINT ( 'NONE',  ( -15.93083330975275658, -11.98016756924215187, 32.48728574198911190 ) ) ;
#83601=VERTEX_POINT ( 'NONE', #4096 ) ;
#83602=DIRECTION ( 'NONE',  ( -0.000000000000000000, -0.8660254037844397068, -0.4999999999999978906 ) ) ;
#83604=CARTESIAN_POINT ( 'NONE',  ( -17.93393266664992325, -9.058645607665452459, 34.76329471203371924 ) ) ;
#83605=DIRECTION ( 'NONE',  ( 0.000000000000000000, 0.000000000000000000, 1.000000000000000000 ) ) ;
#83606=CARTESIAN_POINT ( 'NONE',  ( -5.326946301144534601, -2.985938066672154445, 32.43141759479405550 ) ) ;
#83607=CARTESIAN_POINT ( 'NONE',  ( -5.299849294439222369, -12.39988816332205701, 30.74660775122750778 ) ) ;
#83609=CARTESIAN_POINT ( 'NONE',  ( 5.076923076923075762, -8.120952969808772792, 34.71129190930000163 ) ) ;
#83612=CARTESIAN_POINT ( 'NONE',  ( -6.249976744048591826, -3.436278759898155677, 33.07459398097509506 ) ) ;
#83613=VECTOR ( 'NONE', #41162, 1000.000000000000000 ) ;
#83614=CARTESIAN_POINT ( 'NONE',  ( 8.769230769230768274, -9.780366693483667717, 34.19971097300155094 ) ) ;
#83616=ADVANCED_FACE ( 'NONE', ( #59937 ), #66704, .F. ) ;
#83617=B_SPLINE_CURVE_WITH_KNOTS ( 'NONE', 3,
 ( #7444, #74569, #61483, #40788, #40344, #34016, #68253, #14190, #6992, #41228 ),
 .UNSPECIFIED., .F., .F.,
 ( 4, 2, 2, 2, 4 ),
 ( 0.0007817246256747447872, 0.0009771112852218876831, 0.001172497944769030579, 0.001367884604316173475, 0.001563271263863316371 ),
 .UNSPECIFIED. ) ;
#83618=CARTESIAN_POINT ( 'NONE',  ( -10.39237177129121825, -5.582272713120729257, 34.63742843783360570 ) ) ;
#83619=ORIENTED_EDGE ( 'NONE', *, *, #46070, .F. ) ;
#83620=DIRECTION ( 'NONE',  ( -0.000000000000000000, 0.9848077530122086864, -0.1736481776669273891 ) ) ;
#83621=CARTESIAN_POINT ( 'NONE',  ( 15.90386942290380290, -12.17611988154120795, 31.52148481390971213 ) ) ;
#83622=LINE ( 'NONE', #30429, #54116 ) ;
#83623=FACE_OUTER_BOUND ( 'NONE', #52491, .T. ) ;
#83624=CARTESIAN_POINT ( 'NONE',  ( 13.38461538461538680, -2.538708090699994813, 30.37095296980875503 ) ) ;
#83625=CARTESIAN_POINT ( 'NONE',  ( 7.145856592054987466, -12.11081565061823717, 32.26097654155341843 ) ) ;
#83626=ADVANCED_FACE ( 'NONE', ( #31124 ), #44182, .F. ) ;
#83627=B_SPLINE_CURVE_WITH_KNOTS ( 'NONE', 3,
 ( #51557, #32217, #87177, #79060, #45719, #17361, #25453, #52909, #46174, #73656 ),
 .UNSPECIFIED., .F., .F.,
 ( 4, 2, 2, 2, 4 ),
 ( 0.000000000000000000, 0.0001954311564186879044, 0.0003908623128373758088, 0.0005862934692560636861, 0.0007817246256747516176 ),
 .UNSPECIFIED. ) ;
#83629=CARTESIAN_POINT ( 'NONE',  ( 10.54930120442873331, -3.513871655860377086, 32.76840700105978499 ) ) ;
#83630=VECTOR ( 'NONE', #64603, 1000.000000000000000 ) ;
#83631=EDGE_LOOP ( 'NONE', ( #55667, #22555, #61724, #43421 ) ) ;
#83632=ORIENTED_EDGE ( 'NONE', *, *, #65973, .T. ) ;
#83633=EDGE_CURVE ( 'NONE', #47782, #28383, #46125, .T. ) ;
#83634=ORIENTED_EDGE ( 'NONE', *, *, #11129, .T. ) ;
#83635=CARTESIAN_POINT ( 'NONE',  ( 5.142178648199100088, -11.94971097300157403, 32.03036669348361443 ) ) ;
#83636=CARTESIAN_POINT ( 'NONE',  ( -4.023054346021367245, -3.062576670634119758, 32.05464942895959979 ) ) ;
#83637=CARTESIAN_POINT ( 'NONE',  ( -15.45425415533356350, -10.97335522853832579, 33.68706563782419749 ) ) ;
#83638=CARTESIAN_POINT ( 'NONE',  ( 13.38461538461538680, -8.564572088678739092, 35.78748833219616898 ) ) ;
#83640=EDGE_LOOP ( 'NONE', ( #88211, #21614 ) ) ;
#83642=FACE_OUTER_BOUND ( 'NONE', #34837, .T. ) ;
#83644=B_SPLINE_CURVE_WITH_KNOTS ( 'NONE', 3,
 ( #17040, #25130, #85068, #38646, #51233, #59356, #44051, #9837, #85947, #44943 ),
 .UNSPECIFIED., .F., .F.,
 ( 4, 2, 2, 2, 4 ),
 ( 0.0007817359430256322827, 0.0009771253907249989254, 0.001172514838424365676, 0.001367904286123732428, 0.001563293733823098962 ),
 .UNSPECIFIED. ) ;
#83645=ORIENTED_EDGE ( 'NONE', *, *, #49102, .T. ) ;
#83646=ORIENTED_EDGE ( 'NONE', *, *, #38404, .T. ) ;
#83647=DIRECTION ( 'NONE',  ( -0.000000000000000000, -0.6427876096865404731, -0.7660444431189771253 ) ) ;
#83648=ORIENTED_EDGE ( 'NONE', *, *, #35172, .F. ) ;
#83650=CARTESIAN_POINT ( 'NONE',  ( -16.40382288478850725, -4.236021600441997492, 33.53823185664189310 ) ) ;
#83651=CARTESIAN_POINT ( 'NONE',  ( 2.242441317531067568, -2.506253911140460922, 30.00000000000013856 ) ) ;
#83653=LINE ( 'NONE', #35001, #74106 ) ;
#83656=ORIENTED_EDGE ( 'NONE', *, *, #49111, .F. ) ;
#83657=VERTEX_POINT ( 'NONE', #67150 ) ;
#83658=CARTESIAN_POINT ( 'NONE',  ( -14.53057099012095499, -7.630691491037285168, 34.74850469731152458 ) ) ;
#83660=EDGE_LOOP ( 'NONE', ( #54866, #87172, #60254, #87674 ) ) ;
#83661=CARTESIAN_POINT ( 'NONE',  ( 11.40831432902331954, -6.852621066184266141, 34.70813303252209181 ) ) ;
#83662=CARTESIAN_POINT ( 'NONE',  ( 6.000000000000001776, -12.37446782046654192, 30.86335684631486131 ) ) ;
#83663=CARTESIAN_POINT ( 'NONE',  ( -0.2115930521604181269, -9.357781135181031829, 34.66075350412533851 ) ) ;
#83664=ORIENTED_EDGE ( 'NONE', *, *, #77542, .F. ) ;
#83665=EDGE_CURVE ( 'NONE', #23792, #22049, #37494, .T. ) ;
#83666=CARTESIAN_POINT ( 'NONE',  ( 10.61538461538461675, -2.708943851104267164, 35.45975837776705220 ) ) ;
#83667=LINE ( 'NONE', #787, #43941 ) ;
#83668=EDGE_LOOP ( 'NONE', ( #50796, #26666, #52504, #8182 ) ) ;
#83669=FACE_BOUND ( 'NONE', #26640, .T. ) ;
#83670=CARTESIAN_POINT ( 'NONE',  ( -10.74607521849492464, -4.684245665217972032, 34.18127051446801090 ) ) ;
#83671=DIRECTION ( 'NONE',  ( 0.000000000000000000, 0.6427876096865373645, -0.7660444431189797898 ) ) ;
#83672=CARTESIAN_POINT ( 'NONE',  ( -16.15384615384615330, -12.78798330534102767, 29.49999999999997868 ) ) ;
#83673=LINE ( 'NONE', #56182, #7240 ) ;
#83674=CARTESIAN_POINT ( 'NONE',  ( 18.13052570176355971, -4.459921816937789885, 33.71989282347011851 ) ) ;
#83675=DIRECTION ( 'NONE',  ( 0.000000000000000000, 0.4999999999999960032, -0.8660254037844410391 ) ) ;
#83676=CARTESIAN_POINT ( 'NONE',  ( -4.284536756956459413, -10.70098750199973203, 33.91152734681376302 ) ) ;
#83677=ORIENTED_EDGE ( 'NONE', *, *, #87837, .F. ) ;
#83678=CARTESIAN_POINT ( 'NONE',  ( 14.37294787896833270, -12.46129190930001052, 30.37095296980870174 ) ) ;
#83680=ORIENTED_EDGE ( 'NONE', *, *, #13716, .T. ) ;
#83681=B_SPLINE_CURVE_WITH_KNOTS ( 'NONE', 3,
 ( #75187, #88717, #25663, #54453, #53120, #20240, #13476, #61651, #35072, #62530 ),
 .UNSPECIFIED., .F., .F.,
 ( 4, 2, 2, 2, 4 ),
 ( 0.0007817359430256253438, 0.0009771253907249904686, 0.001172514838424355485, 0.001367904286123720501, 0.001563293733823085518 ),
 .UNSPECIFIED. ) ;
#83683=CARTESIAN_POINT ( 'NONE',  ( -10.86538461538461320, -7.500000000000001776, 35.04278698407183867 ) ) ;
#83684=CARTESIAN_POINT ( 'NONE',  ( -7.596099426240392027, -10.82426656108011720, 33.81400080652039009 ) ) ;
#83685=ORIENTED_EDGE ( 'NONE', *, *, #30658, .F. ) ;
#83686=CARTESIAN_POINT ( 'NONE',  ( 7.976679284387489410, -6.808710257144161559, 34.95449254468098843 ) ) ;
#83688=CARTESIAN_POINT ( 'NONE',  ( -4.377331078410484189, -2.353723527008295680, 30.78948104536958752 ) ) ;
#83689=FACE_BOUND ( 'NONE', #24245, .T. ) ;
#83691=CARTESIAN_POINT ( 'NONE',  ( -4.023054346021365468, -8.147973898785416225, 34.70805048591653730 ) ) ;
#83692=DIRECTION ( 'NONE',  ( 0.000000000000000000, 0.1736481776669275834, 0.9848077530122086864 ) ) ;
#83693=CARTESIAN_POINT ( 'NONE',  ( -7.596099426240392027, -12.65882529074907126, 30.72640787790839312 ) ) ;
#83694=CARTESIAN_POINT ( 'NONE',  ( -14.98082371242109012, -6.696923467548660192, 34.68552623307873972 ) ) ;
#83697=ORIENTED_EDGE ( 'NONE', *, *, #56345, .F. ) ;
#83700=CARTESIAN_POINT ( 'NONE',  ( -2.307692307692305711, -13.88283147151868846, 33.14645433367849847 ) ) ;
#83701=CARTESIAN_POINT ( 'NONE',  ( -15.45425415533356350, -5.827078755546623690, 34.72654668319379567 ) ) ;
#83702=FACE_OUTER_BOUND ( 'NONE', #42843, .T. ) ;
#83703=CYLINDRICAL_SURFACE ( 'NONE', #2099, 0.2500000000000012212 ) ;
#83706=VECTOR ( 'NONE', #47476, 999.9999999999998863 ) ;
#83707=CARTESIAN_POINT ( 'NONE',  ( 0.6843181305165271233, -4.226511098958374291, 33.85474049983370293 ) ) ;
#83708=DIRECTION ( 'NONE',  ( 1.000000000000000000, 0.000000000000000000, 0.000000000000000000 ) ) ;
#83709=DIRECTION ( 'NONE',  ( 0.000000000000000000, 1.000000000000000000, 0.000000000000000000 ) ) ;
#83710=CARTESIAN_POINT ( 'NONE',  ( -3.230769230769352962, -12.16647553114689728, 32.15551576947799362 ) ) ;
#83712=CARTESIAN_POINT ( 'NONE',  ( 18.00000000000000000, -9.780366693483667717, 34.19971097300155094 ) ) ;
#83713=CARTESIAN_POINT ( 'NONE',  ( -9.822998295417995962, -12.62707690430377383, 30.88035979386743435 ) ) ;
#83714=CARTESIAN_POINT ( 'NONE',  ( 10.39250509864703176, -7.630690623152299956, 34.99857592706774057 ) ) ;
#83715=CARTESIAN_POINT ( 'NONE',  ( 7.846153846153846700, -13.87047571288749737, 32.06866353760679544 ) ) ;
#83717=CARTESIAN_POINT ( 'NONE',  ( 3.930361210122205406, -5.113361153441933205, 34.14387501736621999 ) ) ;
#83718=LINE ( 'NONE', #83268, #12965 ) ;
#83720=CARTESIAN_POINT ( 'NONE',  ( 0.5276057948885353177, -3.322132147404559976, 32.92929555188717927 ) ) ;
#83721=CARTESIAN_POINT ( 'NONE',  ( 16.94677510719138525, -11.66186481527757479, 32.95055677023626117 ) ) ;
#83722=ORIENTED_EDGE ( 'NONE', *, *, #46955, .T. ) ;
#83723=CARTESIAN_POINT ( 'NONE',  ( -7.173100147298380413, -2.985938066672154445, 32.43141759479405550 ) ) ;
#83724=LINE ( 'NONE', #49033, #32520 ) ;
#83725=EDGE_LOOP ( 'NONE', ( #74307, #74212 ) ) ;
#83727=CARTESIAN_POINT ( 'NONE',  ( -2.531177232256639265, -10.97335522853832579, 33.68706563782419749 ) ) ;
#83728=ORIENTED_EDGE ( 'NONE', *, *, #57704, .F. ) ;
#83729=PLANE ( 'NONE',  #23305 ) ;
#83731=ORIENTED_EDGE ( 'NONE', *, *, #47071, .T. ) ;
#83732=AXIS2_PLACEMENT_3D ( 'NONE', #30278, #1033, #55971 ) ;
#83733=CARTESIAN_POINT ( 'NONE',  ( 8.834485908743603844, -2.379036618887895305, 30.90682066428158592 ) ) ;
#83737=ORIENTED_EDGE ( 'NONE', *, *, #2420, .T. ) ;
#83738=CARTESIAN_POINT ( 'NONE',  ( 15.36129493253280032, -10.88167719472716399, 33.43325721877153711 ) ) ;
#83740=VERTEX_POINT ( 'NONE', #33366 ) ;
#83741=CARTESIAN_POINT ( 'NONE',  ( 12.68454981315131214, -9.086983370893049639, 34.49168942202179267 ) ) ;
#83742=CARTESIAN_POINT ( 'NONE',  ( -14.30769230769242739, -3.300289026999228881, 32.46337939537708905 ) ) ;
#83743=CARTESIAN_POINT ( 'NONE',  ( -0.2114840416250085009, -5.642605341092957083, 34.66089969410670335 ) ) ;
#83744=CARTESIAN_POINT ( 'NONE',  ( -7.623190942592358965, -7.369474270740069777, 34.74850911626239025 ) ) ;
#83747=VERTEX_POINT ( 'NONE', #61257 ) ;
#83748=CARTESIAN_POINT ( 'NONE',  ( 4.219913487196229163, -8.164416787775445883, 34.95778746994558617 ) ) ;
#83749=EDGE_LOOP ( 'NONE', ( #54879, #78631, #43241, #20715 ) ) ;
#83750=B_SPLINE_CURVE_WITH_KNOTS ( 'NONE', 3,
 ( #44334, #52439, #18228, #23196, #3363, #79924, #11467, #30835, #66409, #30397 ),
 .UNSPECIFIED., .F., .F.,
 ( 4, 2, 2, 2, 4 ),
 ( 0.000000000000000000, 0.0001954311564186871184, 0.0003908623128373742367, 0.0005862934692560614093, 0.0007817246256747484735 ),
 .UNSPECIFIED. ) ;
#83753=EDGE_CURVE ( 'NONE', #44409, #24035, #23620, .T. ) ;
#83754=ORIENTED_EDGE ( 'NONE', *, *, #65297, .F. ) ;
#83755=AXIS2_PLACEMENT_3D ( 'NONE', #66676, #31556, #32445 ) ;
#83756=CARTESIAN_POINT ( 'NONE',  ( 7.780071466793708979, -11.91647553114624181, 32.58852847137148245 ) ) ;
#83757=CARTESIAN_POINT ( 'NONE',  ( 6.923076923076800782, -9.528491918059723176, 34.59228464037033035 ) ) ;
#83759=CARTESIAN_POINT ( 'NONE',  ( -1.384615384615383471, -11.33034616979429110, 35.88435417666054406 ) ) ;
#83760=CIRCLE ( 'NONE', #44904, 0.2500000000000002220 ) ;
#83761=EDGE_LOOP ( 'NONE', ( #43083, #25634, #79196, #23142 ) ) ;
#83762=CARTESIAN_POINT ( 'NONE',  ( -12.21148414990014963, -4.943051570960394159, 34.04725096376909477 ) ) ;
#83763=ORIENTED_EDGE ( 'NONE', *, *, #38338, .T. ) ;
#83764=CARTESIAN_POINT ( 'NONE',  ( -14.05774689831426372, -12.07971442181322175, 32.31769673815850297 ) ) ;
#83766=ORIENTED_EDGE ( 'NONE', *, *, #7963, .F. ) ;
#83767=EDGE_CURVE ( 'NONE', #79227, #72161, #53174, .T. ) ;
#83768=CARTESIAN_POINT ( 'NONE',  ( 17.99999999999987566, -10.90142922262034020, 33.41473453929536674 ) ) ;
#83769=CARTESIAN_POINT ( 'NONE',  ( -8.769230769230768274, -11.91647553114624181, 32.58852847137148245 ) ) ;
#83771=FACE_BOUND ( 'NONE', #35286, .T. ) ;
#83772=CARTESIAN_POINT ( 'NONE',  ( -11.66860874789975533, -2.619462340734462380, 30.83744416345203021 ) ) ;
#83773=CARTESIAN_POINT ( 'NONE',  ( -6.792285115252138183, -12.11778462344220841, 31.66786338562085135 ) ) ;
#83774=CARTESIAN_POINT ( 'NONE',  ( 15.45378207486262667, -2.523321265292115534, 31.42251411153756990 ) ) ;
#83775=CARTESIAN_POINT ( 'NONE',  ( 0.7115384615384606759, -2.249999999999998668, 29.75000000000000355 ) ) ;
#83777=DIRECTION ( 'NONE',  ( 0.000000000000000000, 0.6427876096865368094, 0.7660444431189802339 ) ) ;
#83778=VERTEX_POINT ( 'NONE', #60827 ) ;
#83779=CARTESIAN_POINT ( 'NONE',  ( 10.36536137809165403, -10.05641848906368097, 34.04755513067966177 ) ) ;
#83781=B_SPLINE_CURVE_WITH_KNOTS ( 'NONE', 3,
 ( #23374, #65686, #44079, #9865, #45419, #72450, #17068, #30144, #52624, #3101 ),
 .UNSPECIFIED., .F., .F.,
 ( 4, 2, 2, 2, 4 ),
 ( 0.0007817246256747442451, 0.0009771112852218870326, 0.001172497944769029929, 0.001367884604316172825, 0.001563271263863315504 ),
 .UNSPECIFIED. ) ;
#83782=ORIENTED_EDGE ( 'NONE', *, *, #38635, .F. ) ;
#83783=CARTESIAN_POINT ( 'NONE',  ( 7.846153846153846700, -6.386643153685126251, 34.62446782046654192 ) ) ;
#83784=CARTESIAN_POINT ( 'NONE',  ( 7.912222197156284054, -9.780366693483667717, 34.19971097300155805 ) ) ;
#83785=B_SPLINE_CURVE_WITH_KNOTS ( 'NONE', 3,
 ( #78320, #58482, #72010, #77883, #57172, #85096, #36465, #58050, #16619, #85979 ),
 .UNSPECIFIED., .F., .F.,
 ( 4, 2, 2, 2, 4 ),
 ( 0.000000000000000000, 0.0001954339857564063360, 0.0003908679715128126719, 0.0005863019572692189808, 0.0007817359430256253438 ),
 .UNSPECIFIED. ) ;
#83787=B_SPLINE_CURVE_WITH_KNOTS ( 'NONE', 3,
 ( #39957, #75944, #82268, #88603, #69187, #5712, #60648, #54332, #34070, #81827 ),
 .UNSPECIFIED., .F., .F.,
 ( 4, 2, 2, 2, 4 ),
 ( 0.0007817246256747471724, 0.0009771112852218905021, 0.001172497944769033615, 0.001367884604316176944, 0.001563271263863320274 ),
 .UNSPECIFIED. ) ;
#83788=CARTESIAN_POINT ( 'NONE',  ( 6.923076923076802558, -6.879047030192662504, 34.71129190930017927 ) ) ;
#83789=CYLINDRICAL_SURFACE ( 'NONE', #19282, 0.2499999999999997502 ) ;
#83790=CARTESIAN_POINT ( 'NONE',  ( 15.36129493253280032, -3.816742781228458448, 33.13167719472716044 ) ) ;
#83791=CARTESIAN_POINT ( 'NONE',  ( 13.44987095589141113, -11.48612834413965977, 32.76840700105972815 ) ) ;
#83792=ORIENTED_EDGE ( 'NONE', *, *, #51658, .T. ) ;
#83793=EDGE_CURVE ( 'NONE', #79114, #70013, #62230, .T. ) ;
#83794=CARTESIAN_POINT ( 'NONE',  ( -2.307692307692305711, -12.78798330534102945, 29.74999999999997868 ) ) ;
#83795=CARTESIAN_POINT ( 'NONE',  ( -14.30769230769230660, -9.905515769479276145, 34.41647553114623292 ) ) ;
#83796=CARTESIAN_POINT ( 'NONE',  ( 13.38461538461538680, -11.35647404775217417, 33.31231777344666511 ) ) ;
#83797=EDGE_CURVE ( 'NONE', #67310, #3936, #35429, .T. ) ;
#83798=CARTESIAN_POINT ( 'NONE',  ( -8.769230769230768274, -2.486705287966279876, 31.30864560766543647 ) ) ;
#83799=CARTESIAN_POINT ( 'NONE',  ( 2.530705151785704654, -5.582272713120728369, 34.63742843783360570 ) ) ;
#83800=EDGE_LOOP ( 'NONE', ( #48000, #40912, #59708, #84678 ) ) ;
#83801=CARTESIAN_POINT ( 'NONE',  ( -0.4615384615385840772, -2.379036618888197285, 30.90682066428292885 ) ) ;
#83802=ORIENTED_EDGE ( 'NONE', *, *, #47942, .T. ) ;
#83804=ORIENTED_EDGE ( 'NONE', *, *, #59107, .T. ) ;
#83805=EDGE_CURVE ( 'NONE', #76443, #38647, #63481, .T. ) ;
#83806=CARTESIAN_POINT ( 'NONE',  ( 3.480769230770666578, -7.500000000000155431, 34.75000000000007105 ) ) ;
#83807=VERTEX_POINT ( 'NONE', #41900 ) ;
#83809=CARTESIAN_POINT ( 'NONE',  ( -17.07692307692319744, -3.300289026999228437, 32.46337939537709616 ) ) ;
#83810=DIRECTION ( 'NONE',  ( 0.000000000000000000, 0.4999999999999960032, -0.8660254037844410391 ) ) ;
#83811=CARTESIAN_POINT ( 'NONE',  ( -17.07692307692319744, -12.70778746994576025, 30.41441678777401236 ) ) ;
#83812=CARTESIAN_POINT ( 'NONE',  ( -16.82686876528476461, -12.17597550085003633, 31.52189283813461884 ) ) ;
#83813=CARTESIAN_POINT ( 'NONE',  ( 0.5267936010512993539, -9.528491918058460186, 34.59228464037085615 ) ) ;
#83814=EDGE_LOOP ( 'NONE', ( #52510, #53944, #65382, #84977 ) ) ;
#83815=CARTESIAN_POINT ( 'NONE',  ( 4.219101725122177626, -4.481592998940251427, 33.73612834413965089 ) ) ;
#83816=CARTESIAN_POINT ( 'NONE',  ( -0.7115616857599188494, -5.765609946408404518, 34.70566812827425451 ) ) ;
#83818=LINE ( 'NONE', #55437, #51223 ) ;
#83819=CARTESIAN_POINT ( 'NONE',  ( 3.164685819813350065, -12.37446782046654192, 30.86335684631486487 ) ) ;
#83820=CARTESIAN_POINT ( 'NONE',  ( -0.4615384615385840772, -4.320704448113951379, 33.92786785259630022 ) ) ;
#83821=CARTESIAN_POINT ( 'NONE',  ( -17.74994568836168440, -11.79725096376909654, 32.30694842903960762 ) ) ;
#83822=CYLINDRICAL_SURFACE ( 'NONE', #66315, 0.2500000000000004996 ) ;
#83823=CARTESIAN_POINT ( 'NONE',  ( -11.53846153846153655, -10.67929555188718282, 33.92786785259544047 ) ) ;
#83826=VERTEX_POINT ( 'NONE', #70691 ) ;
#83827=CARTESIAN_POINT ( 'NONE',  ( -16.82686876528476105, -10.66356715214248574, 33.62249196103329751 ) ) ;
#83828=CYLINDRICAL_SURFACE ( 'NONE', #7415, 0.2499999999999993616 ) ;
#83829=AXIS2_PLACEMENT_3D ( 'NONE', #12796, #46142, #67743 ) ;
#83830=CARTESIAN_POINT ( 'NONE',  ( 9.019285189144222059, -10.82426656108012075, 33.81400080652039009 ) ) ;
#83832=ORIENTED_EDGE ( 'NONE', *, *, #74428, .T. ) ;
#83834=CARTESIAN_POINT ( 'NONE',  ( -16.15384615384615330, -12.10708131394839349, 31.69288490824020244 ) ) ;
#83835=AXIS2_PLACEMENT_3D ( 'NONE', #86974, #25241, #52702 ) ;
#83836=ORIENTED_EDGE ( 'NONE', *, *, #44096, .T. ) ;
#83837=CARTESIAN_POINT ( 'NONE',  ( 14.24244237591822859, -2.255955759149247619, 30.00000000000013856 ) ) ;
#83838=CARTESIAN_POINT ( 'NONE',  ( 14.24242186173153435, -3.300289026998414865, 32.46337939537583139 ) ) ;
#83839=B_SPLINE_CURVE_WITH_KNOTS ( 'NONE', 3,
 ( #83347, #1801, #21628, #77027, #9886, #84241, #1358, #69820, #70265, #77465 ),
 .UNSPECIFIED., .F., .F.,
 ( 4, 2, 2, 2, 4 ),
 ( 0.0007817359430256360774, 0.0009771253907250041296, 0.001172514838424371965, 0.001367904286123740017, 0.001563293733823108069 ),
 .UNSPECIFIED. ) ;
#83840=EDGE_LOOP ( 'NONE', ( #57802, #24068 ) ) ;
#83841=ADVANCED_FACE ( 'NONE', ( #36463 ), #21611, .F. ) ;
#83842=CARTESIAN_POINT ( 'NONE',  ( -15.45425417449317784, -2.847400154188067578, 31.58180166144859058 ) ) ;
#83843=CARTESIAN_POINT ( 'NONE',  ( 17.07692307692295586, -10.21337939537710326, 33.94971097300076224 ) ) ;
#83844=CARTESIAN_POINT ( 'NONE',  ( 9.692307692307570832, -10.33852847137269571, 34.16647553114546554 ) ) ;
#83845=FACE_OUTER_BOUND ( 'NONE', #41799, .T. ) ;
#83846=VERTEX_POINT ( 'NONE', #71121 ) ;
#83847=CARTESIAN_POINT ( 'NONE',  ( -2.980714810855778829, -2.318338780012835443, 30.59689888758630261 ) ) ;
#83849=CARTESIAN_POINT ( 'NONE',  ( -6.923076923076615152, -2.506253911140614576, 30.00000000000323297 ) ) ;
#83850=CARTESIAN_POINT ( 'NONE',  ( -10.74607608205216991, -2.729777683071817229, 31.24903638046269450 ) ) ;
#83851=ORIENTED_EDGE ( 'NONE', *, *, #35133, .T. ) ;
#83852=CARTESIAN_POINT ( 'NONE',  ( 10.74617505635156789, -11.37503395064541678, 33.29242100308974273 ) ) ;
#83853=CARTESIAN_POINT ( 'NONE',  ( -16.15384615384615330, -7.500000000000001776, 35.04278698407183867 ) ) ;
#83854=CARTESIAN_POINT ( 'NONE',  ( -6.857009589726846599, -12.34228464037088813, 31.77849191805839268 ) ) ;
#83858=CARTESIAN_POINT ( 'NONE',  ( -18.13014720943822056, -4.460286881179643892, 33.72017969459903242 ) ) ;
#83859=VERTEX_POINT ( 'NONE', #8996 ) ;
#83861=FACE_BOUND ( 'NONE', #51575, .T. ) ;
#83863=CARTESIAN_POINT ( 'NONE',  ( 8.703960323269996024, -3.835265460703609186, 33.15142922261924241 ) ) ;
#83865=CARTESIAN_POINT ( 'NONE',  ( 4.153846153846032507, -11.94971097300221174, 32.03036669348237098 ) ) ;
#83866=CARTESIAN_POINT ( 'NONE',  ( 15.23076923076923173, -6.343179335718451384, 34.87096338111211935 ) ) ;
#83867=CARTESIAN_POINT ( 'NONE',  ( 5.326868595271218254, -4.336752205174647656, 33.62275283266504289 ) ) ;
#83868=EDGE_CURVE ( 'NONE', #25396, #81013, #51512, .T. ) ;
#83870=ORIENTED_EDGE ( 'NONE', *, *, #5063, .T. ) ;
#83872=CARTESIAN_POINT ( 'NONE',  ( 13.63461538461682210, -7.500000000000155431, 34.75000000000007105 ) ) ;
#83873=ORIENTED_EDGE ( 'NONE', *, *, #55803, .T. ) ;
#83874=EDGE_CURVE ( 'NONE', #87089, #24060, #25701, .T. ) ;
#83875=LINE ( 'NONE', #42883, #84794 ) ;
#83876=CARTESIAN_POINT ( 'NONE',  ( 7.846153846153846700, -10.89733346790207413, 36.13435417666054406 ) ) ;
#83877=CARTESIAN_POINT ( 'NONE',  ( -16.15384615384627409, -11.06231777344772027, 33.60647404775119895 ) ) ;
#83878=EDGE_LOOP ( 'NONE', ( #66075, #78053 ) ) ;
#83879=CARTESIAN_POINT ( 'NONE',  ( 16.15384615384603251, -2.379036618888197729, 30.90682066428292885 ) ) ;
#83880=EDGE_CURVE ( 'NONE', #74779, #26040, #57913, .T. ) ;
#83881=AXIS2_PLACEMENT_3D ( 'NONE', #24696, #80550, #23789 ) ;
#83882=CARTESIAN_POINT ( 'NONE',  ( -1.384615384615506484, -12.70778746994576025, 30.41441678777401236 ) ) ;
#83883=CARTESIAN_POINT ( 'NONE',  ( 4.087763774486019130, -2.486705287966279432, 31.30864560766542937 ) ) ;
#83884=CARTESIAN_POINT ( 'NONE',  ( -1.161835715637320465, -3.020022701398814124, 32.48759521482552515 ) ) ;
#83886=EDGE_CURVE ( 'NONE', #60602, #87727, #21384, .T. ) ;
#83887=B_SPLINE_CURVE_WITH_KNOTS ( 'NONE', 3,
 ( #73525, #32978, #74405, #53235, #26660, #80282, #33856, #19457, #6825, #5954 ),
 .UNSPECIFIED., .F., .F.,
 ( 4, 2, 2, 2, 4 ),
 ( 0.0007817359430256282712, 0.0009771253907249941549, 0.001172514838424359822, 0.001367904286123725489, 0.001563293733823091372 ),
 .UNSPECIFIED. ) ;
#83888=ORIENTED_EDGE ( 'NONE', *, *, #29051, .F. ) ;
#83889=ORIENTED_EDGE ( 'NONE', *, *, #17043, .T. ) ;
#83890=CARTESIAN_POINT ( 'NONE',  ( 3.903822929624696236, -2.985938066672154445, 32.43141759479405550 ) ) ;
#83891=CARTESIAN_POINT ( 'NONE',  ( -18.12796115882773051, -2.254609590993097878, 29.97526117654244970 ) ) ;
#83892=DIRECTION ( 'NONE',  ( -0.000000000000000000, 0.8660254037844397068, -0.4999999999999978906 ) ) ;
#83893=CARTESIAN_POINT ( 'NONE',  ( 9.692307692307695177, -11.35647404775217417, 33.31231777344666511 ) ) ;
#83894=CARTESIAN_POINT ( 'NONE',  ( -3.230769230769351186, -11.48612834414049644, 32.76840700105863391 ) ) ;
#83895=CARTESIAN_POINT ( 'NONE',  ( -39.05038313613820122, -7.500000000000000000, 29.75000000000000355 ) ) ;
#83896=CARTESIAN_POINT ( 'NONE',  ( 9.823099500132480344, -3.530189275343204702, 32.79018710029569661 ) ) ;
#83897=ORIENTED_EDGE ( 'NONE', *, *, #66158, .T. ) ;
#83898=EDGE_CURVE ( 'NONE', #60046, #14768, #53612, .T. ) ;
#83899=LINE ( 'NONE', #48758, #32806 ) ;
#83900=CARTESIAN_POINT ( 'NONE',  ( 16.15384615384603251, -12.16647553114689728, 32.15551576947799362 ) ) ;
#83901=CARTESIAN_POINT ( 'NONE',  ( 11.60463067942419535, -7.250054483168843156, 34.74374881642865631 ) ) ;
#83902=CARTESIAN_POINT ( 'NONE',  ( -2.307692307692305711, -3.937682226553329556, 33.60647404775216529 ) ) ;
#83903=EDGE_LOOP ( 'NONE', ( #73782, #76832, #85518, #75194 ) ) ;
#83905=VERTEX_POINT ( 'NONE', #64354 ) ;
#83906=FACE_BOUND ( 'NONE', #82421, .T. ) ;
#83908=ADVANCED_FACE ( 'NONE', ( #64795 ), #72898, .F. ) ;
#83910=CARTESIAN_POINT ( 'NONE',  ( -7.173076923076921574, -7.433931650972300353, 34.75000000000000711 ) ) ;
#83911=EDGE_CURVE ( 'NONE', #18264, #40036, #83781, .T. ) ;
#83912=VERTEX_POINT ( 'NONE', #10316 ) ;
#83914=CARTESIAN_POINT ( 'NONE',  ( -5.933932666649924137, -9.058645607665452459, 34.76329471203371924 ) ) ;
#83915=CARTESIAN_POINT ( 'NONE',  ( -15.16470189741915675, -9.905515769479276145, 34.41647553114623292 ) ) ;
#83916=CARTESIAN_POINT ( 'NONE',  ( 6.000000000000001776, -3.513871655860378418, 32.76840700105978499 ) ) ;
#83917=ORIENTED_EDGE ( 'NONE', *, *, #68219, .T. ) ;
#83918=CARTESIAN_POINT ( 'NONE',  ( -9.942330916529147800, -2.985938066672154445, 32.43141759479405550 ) ) ;
#83919=VECTOR ( 'NONE', #51154, 1000.000000000000000 ) ;
#83920=EDGE_LOOP ( 'NONE', ( #8092, #55356 ) ) ;
#83924=FACE_OUTER_BOUND ( 'NONE', #21640, .T. ) ;
#83925=CARTESIAN_POINT ( 'NONE',  ( -1.450697763975520083, -12.34228464037088280, 31.77849191805838558 ) ) ;
#83926=CARTESIAN_POINT ( 'NONE',  ( 7.715463243043537034, -9.929715669179220328, 34.40415004197138416 ) ) ;
#83927=DIRECTION ( 'NONE',  ( 0.000000000000000000, 0.6427876096865373645, -0.7660444431189797898 ) ) ;
#83929=DIRECTION ( 'NONE',  ( -0.000000000000000000, -0.000000000000000000, -1.000000000000000000 ) ) ;
#83930=CARTESIAN_POINT ( 'NONE',  ( 14.05771557674995265, -3.627789207965226748, 32.91389620160131102 ) ) ;
#83931=B_SPLINE_CURVE_WITH_KNOTS ( 'NONE', 3,
 ( #52414, #67720, #53304, #80806, #79900, #46557, #74039, #5573, #74473, #12769 ),
 .UNSPECIFIED., .F., .F.,
 ( 4, 2, 2, 2, 4 ),
 ( 0.000000000000000000, 0.0001954311564186868473, 0.0003908623128373736946, 0.0005862934692560605419, 0.0007817246256747473893 ),
 .UNSPECIFIED. ) ;
#83933=VERTEX_POINT ( 'NONE', #37781 ) ;
#83934=CARTESIAN_POINT ( 'NONE',  ( -0.5276218724943415594, -5.557115091759785130, 34.35708131394839171 ) ) ;
#83935=ORIENTED_EDGE ( 'NONE', *, *, #27286, .F. ) ;
#83936=VERTEX_POINT ( 'NONE', #51261 ) ;
#83938=ORIENTED_EDGE ( 'NONE', *, *, #71947, .T. ) ;
#83939=CARTESIAN_POINT ( 'NONE',  ( -13.38461538461538325, -7.500000000000001776, 35.04278698407183867 ) ) ;
#83940=CARTESIAN_POINT ( 'NONE',  ( 6.130791807824788719, -11.18335022499818621, 33.13157742990016885 ) ) ;
#83942=CARTESIAN_POINT ( 'NONE',  ( -4.946131269098287930, -3.530189275343204702, 32.79018710029569661 ) ) ;
#83943=CARTESIAN_POINT ( 'NONE',  ( -13.16160254052199008, -6.460100341425560444, 34.89618726649961644 ) ) ;
#83944=LINE ( 'NONE', #63648, #6840 ) ;
#83945=CARTESIAN_POINT ( 'NONE',  ( -4.283993363284374745, -3.817052484675422797, 33.13202310037935661 ) ) ;
#83946=EDGE_CURVE ( 'NONE', #78414, #10638, #15030, .T. ) ;
#83947=CYLINDRICAL_SURFACE ( 'NONE', #56337, 0.2500000000000008882 ) ;
#83948=CARTESIAN_POINT ( 'NONE',  ( 11.40777007179398161, -10.54014554554150607, 33.71984207302941883 ) ) ;
#83949=VECTOR ( 'NONE', #72429, 1000.000000000000114 ) ;
#83950=DIRECTION ( 'NONE',  ( -0.000000000000000000, -0.3420201433256694901, -0.9396926207859082059 ) ) ;
#83951=CARTESIAN_POINT ( 'NONE',  ( -17.14217300869715643, -2.255955759149247175, 30.00000000000014211 ) ) ;
#83952=ADVANCED_FACE ( 'NONE', ( #71560 ), #30576, .F. ) ;
#83956=ORIENTED_EDGE ( 'NONE', *, *, #22328, .T. ) ;
#83957=EDGE_LOOP ( 'NONE', ( #11476, #68327, #17335, #50460 ) ) ;
#83958=DIRECTION ( 'NONE',  ( -0.000000000000000000, -0.1736481776669307198, -0.9848077530122080203 ) ) ;
#83959=DIRECTION ( 'NONE',  ( 0.000000000000000000, 0.000000000000000000, 1.000000000000000000 ) ) ;
#83960=CARTESIAN_POINT ( 'NONE',  ( -3.164700879766792152, -2.721908614388771852, 31.22303859784725333 ) ) ;
#83961=CARTESIAN_POINT ( 'NONE',  ( 12.59206416330202671, -10.88167719472716399, 33.43325721877153711 ) ) ;
#83962=VERTEX_POINT ( 'NONE', #3548 ) ;
#83963=CARTESIAN_POINT ( 'NONE',  ( -8.769230769230768274, -1.951392089020283160, 34.73218667398347748 ) ) ;
#83964=B_SPLINE_CURVE_WITH_KNOTS ( 'NONE', 3,
 ( #30158, #9011, #77896, #3561, #51275, #36477, #49978, #23389, #78333, #50844 ),
 .UNSPECIFIED., .F., .F.,
 ( 4, 2, 2, 2, 4 ),
 ( 0.000000000000000000, 0.0001954311564186869557, 0.0003908623128373739115, 0.0005862934692560608672, 0.0007817246256747478229 ),
 .UNSPECIFIED. ) ;
#83965=CARTESIAN_POINT ( 'NONE',  ( -17.32689980786543060, -3.627789207965226304, 32.91389620160131102 ) ) ;
#83967=B_SPLINE_CURVE_WITH_KNOTS ( 'NONE', 3,
 ( #45645, #64563, #80336, #72668, #16838, #51945 ),
 .UNSPECIFIED., .F., .F.,
 ( 4, 2, 4 ),
 ( 4.906730591320636874E-17, 0.0001954756301637213293, 0.0003909512603273935984 ),
 .UNSPECIFIED. ) ;
#83968=CARTESIAN_POINT ( 'NONE',  ( -3.230769230769229949, -12.10708131394839349, 31.69288490824020244 ) ) ;
#83969=ORIENTED_EDGE ( 'NONE', *, *, #17863, .F. ) ;
#83970=CARTESIAN_POINT ( 'NONE',  ( 0.5276068125408989173, -5.557115091759786019, 34.35708131394839882 ) ) ;
#83971=VERTEX_POINT ( 'NONE', #44522 ) ;
#83972=CARTESIAN_POINT ( 'NONE',  ( 9.942362003946010773, -11.79725096376909654, 32.30694842903959341 ) ) ;
#83973=CARTESIAN_POINT ( 'NONE',  ( -3.361460697436791989, -12.11776431015576172, 31.66791131148498906 ) ) ;
#83974=CARTESIAN_POINT ( 'NONE',  ( -1.384615384615506484, -9.528491918059723176, 34.59228464037033035 ) ) ;
#83975=CARTESIAN_POINT ( 'NONE',  ( -9.627052552794857831, -6.835583212224610072, 34.95778746994559327 ) ) ;
#83976=CYLINDRICAL_SURFACE ( 'NONE', #45076, 0.2500000000000008882 ) ;
#83977=EDGE_CURVE ( 'NONE', #37879, #86398, #31109, .T. ) ;
#83978=VERTEX_POINT ( 'NONE', #24255 ) ;
#83981=ORIENTED_EDGE ( 'NONE', *, *, #21192, .T. ) ;
#83983=CARTESIAN_POINT ( 'NONE',  ( 13.31853197365950692, -3.050289026998445951, 32.03036669348365706 ) ) ;
#83984=CARTESIAN_POINT ( 'NONE',  ( 15.90382292962469535, -5.765609946408405406, 34.70566812827424741 ) ) ;
#83985=LINE ( 'NONE', #64557, #79683 ) ;
#83986=CARTESIAN_POINT ( 'NONE',  ( 16.82689985270161870, -10.18141759479407327, 34.26406193332782379 ) ) ;
#83987=CARTESIAN_POINT ( 'NONE',  ( 4.219101725122176738, -6.879047030191282275, 34.71129190930002295 ) ) ;
#83989=ORIENTED_EDGE ( 'NONE', *, *, #9308, .F. ) ;
#83990=EDGE_LOOP ( 'NONE', ( #19532, #49057 ) ) ;
#83992=CARTESIAN_POINT ( 'NONE',  ( -3.099977422944443894, -10.54018710029568595, 33.71981072465678864 ) ) ;
#83993=ORIENTED_EDGE ( 'NONE', *, *, #36130, .F. ) ;
#83994=CARTESIAN_POINT ( 'NONE',  ( 0.4615384615384611200, -8.120952969808772792, 34.71129190930000163 ) ) ;
#83995=CARTESIAN_POINT ( 'NONE',  ( 13.51540582558234149, -3.957578996910242619, 33.62503395064540257 ) ) ;
#83996=B_SPLINE_CURVE_WITH_KNOTS ( 'NONE', 3,
 ( #62063, #29187, #14775, #42252, #70598, #62493, #27839, #28275, #55302, #55745 ),
 .UNSPECIFIED., .F., .F.,
 ( 4, 2, 2, 2, 4 ),
 ( 0.0007817246256747499913, 0.0009771112852218944052, 0.001172497944769038819, 0.001367884604316183016, 0.001563271263863327430 ),
 .UNSPECIFIED. ) ;
#83998=EDGE_LOOP ( 'NONE', ( #86566, #50880 ) ) ;
#83999=VECTOR ( 'NONE', #18034, 1000.000000000000227 ) ;
#84000=EDGE_CURVE ( 'NONE', #63608, #30358, #40470, .T. ) ;
#84001=EDGE_CURVE ( 'NONE', #88762, #5458, #20619, .T. ) ;
#84002=ORIENTED_EDGE ( 'NONE', *, *, #87785, .T. ) ;
#84003=CARTESIAN_POINT ( 'NONE',  ( -18.00000000000000000, -1.270656007487078965, 33.34651343095210052 ) ) ;
#84005=EDGE_LOOP ( 'NONE', ( #79102, #54252, #3769, #78146 ) ) ;
#84006=ADVANCED_FACE ( 'NONE', ( #32811 ), #54403, .F. ) ;
#84007=FACE_BOUND ( 'NONE', #81103, .T. ) ;
#84008=CARTESIAN_POINT ( 'NONE',  ( 6.923076923076802558, -4.481592998941358097, 33.73612834414048933 ) ) ;
#84011=ORIENTED_EDGE ( 'NONE', *, *, #9799, .T. ) ;
#84012=CARTESIAN_POINT ( 'NONE',  ( 2.307692307692309264, -8.120952969808772792, 34.71129190930000163 ) ) ;
#84013=CARTESIAN_POINT ( 'NONE',  ( 3.453780582382079523, -3.105924265160262543, 32.13625925475356127 ) ) ;
#84014=EDGE_CURVE ( 'NONE', #78118, #65478, #81897, .T. ) ;
#84016=CARTESIAN_POINT ( 'NONE',  ( 3.930361210122207183, -11.41268669641500466, 32.86336882939237825 ) ) ;
#84017=CARTESIAN_POINT ( 'NONE',  ( 4.376625695114563008, -3.236590943229499029, 32.36255958852954251 ) ) ;
#84018=VERTEX_POINT ( 'NONE', #12984 ) ;
#84019=EDGE_CURVE ( 'NONE', #6434, #13761, #4153, .T. ) ;
#84020=CARTESIAN_POINT ( 'NONE',  ( -0.5921481167425443060, -7.722926974430166069, 34.99546784045485737 ) ) ;
#84021=CARTESIAN_POINT ( 'NONE',  ( 3.361561038594018225, -4.118422570099827595, 33.43335022499816489 ) ) ;
#84023=CARTESIAN_POINT ( 'NONE',  ( 5.750023269057646047, -4.943428324936578910, 34.04746400365624481 ) ) ;
#84024=CARTESIAN_POINT ( 'NONE',  ( -10.61538461538461320, -13.04860791097971706, 34.73218667398347037 ) ) ;
#84025=CARTESIAN_POINT ( 'NONE',  ( -13.31936024510254413, -12.51329471203373700, 31.30864560766537963 ) ) ;
#84026=CARTESIAN_POINT ( 'NONE',  ( -6.857009589726848375, -12.62096338111211757, 30.90682066428152908 ) ) ;
#84027=CARTESIAN_POINT ( 'NONE',  ( 11.31563344082666411, -7.369209533119137845, 34.99857337881830688 ) ) ;
#84028=CARTESIAN_POINT ( 'NONE',  ( 5.299935921016468932, -2.308499170217967134, 30.53291367094873721 ) ) ;
#84030=CARTESIAN_POINT ( 'NONE',  ( 2.557746727605761272, -6.523592122091589118, 34.90882529074906415 ) ) ;
#84031=ADVANCED_FACE ( 'NONE', ( #66600 ), #67931, .F. ) ;
#84032=CARTESIAN_POINT ( 'NONE',  ( 17.07692307692307665, -2.249999999999998668, 29.50000000000001421 ) ) ;
#84034=VERTEX_POINT ( 'NONE', #25607 ) ;
#84037=CARTESIAN_POINT ( 'NONE',  ( -6.000000000000119904, -11.94971097300221174, 32.03036669348237098 ) ) ;
#84039=ORIENTED_EDGE ( 'NONE', *, *, #25171, .T. ) ;
#84040=CARTESIAN_POINT ( 'NONE',  ( 8.769230769230768274, -2.499999999999998668, 29.50000000000001066 ) ) ;
#84041=FACE_OUTER_BOUND ( 'NONE', #11576, .T. ) ;
#84042=ORIENTED_EDGE ( 'NONE', *, *, #15238, .T. ) ;
#84043=CARTESIAN_POINT ( 'NONE',  ( -18.25002323729296450, -12.43535235679832596, 30.55408501211184813 ) ) ;
#84045=DIRECTION ( 'NONE',  ( -0.000000000000000000, -0.1736481776669307198, -0.9848077530122080203 ) ) ;
#84046=CARTESIAN_POINT ( 'NONE',  ( -3.903846153846152855, -2.249999999999998668, 29.75000000000000355 ) ) ;
#84047=CARTESIAN_POINT ( 'NONE',  ( 6.988332494352947677, -9.442884908240271713, 34.35708131394835618 ) ) ;
#84048=AXIS2_PLACEMENT_3D ( 'NONE', #86236, #72698, #25406 ) ;
#84049=CARTESIAN_POINT ( 'NONE',  ( -5.326946314216043810, -12.43535235679832596, 30.55408501211184813 ) ) ;
#84050=CARTESIAN_POINT ( 'NONE',  ( 11.53846153846153832, -2.721908614388771852, 31.22303859784724978 ) ) ;
#84051=CARTESIAN_POINT ( 'NONE',  ( -13.60754234352223158, -11.98009711892699514, 32.48740034544076138 ) ) ;
#84053=EDGE_CURVE ( 'NONE', #30988, #18603, #36391, .T. ) ;
#84054=CARTESIAN_POINT ( 'NONE',  ( -18.00000000000000000, -2.533126527117917082, 35.28035834855298702 ) ) ;
#84055=CARTESIAN_POINT ( 'NONE',  ( -6.250023224221457063, -3.520140089381497361, 33.17453946501458262 ) ) ;
#84057=B_SPLINE_CURVE_WITH_KNOTS ( 'NONE', 3,
 ( #1764, #15291, #22481, #884, #49065, #56707, #1324, #50382, #28811, #83757 ),
 .UNSPECIFIED., .F., .F.,
 ( 4, 2, 2, 2, 4 ),
 ( 0.000000000000000000, 0.0001954311564186868202, 0.0003908623128373736404, 0.0005862934692560604335, 0.0007817246256747472808 ),
 .UNSPECIFIED. ) ;
#84060=DIRECTION ( 'NONE',  ( 0.000000000000000000, 1.000000000000000000, 0.000000000000000000 ) ) ;
#84061=VERTEX_POINT ( 'NONE', #68365 ) ;
#84062=CARTESIAN_POINT ( 'NONE',  ( 14.43821800945587697, -2.619367082507849442, 30.83698974864643461 ) ) ;
#84063=DIRECTION ( 'NONE',  ( 0.000000000000000000, 0.1736481776669267785, -0.9848077530122087975 ) ) ;
#84064=CARTESIAN_POINT ( 'NONE',  ( -8.899377978668987055, -11.47017969459904130, 32.78971311882034456 ) ) ;
#84065=CARTESIAN_POINT ( 'NONE',  ( -14.37296275365308418, -11.94971097300153140, 32.03036669348370680 ) ) ;
#84066=CARTESIAN_POINT ( 'NONE',  ( 13.63456090296352841, -2.587454068350148351, 30.68340429815432202 ) ) ;
#84067=CARTESIAN_POINT ( 'NONE',  ( -14.24243716817946925, -4.320704448112861584, 33.92786785259548310 ) ) ;
#84069=CYLINDRICAL_SURFACE ( 'NONE', #14529, 0.2499999999999994726 ) ;
#84070=EDGE_CURVE ( 'NONE', #29793, #4115, #24574, .T. ) ;
#84071=ORIENTED_EDGE ( 'NONE', *, *, #27358, .F. ) ;
#84073=B_SPLINE_CURVE_WITH_KNOTS ( 'NONE', 3,
 ( #18227, #45688, #73169, #11466, #38950, #66408, #5927, #81589, #6802, #55 ),
 .UNSPECIFIED., .F., .F.,
 ( 4, 2, 2, 2, 4 ),
 ( 0.0007817246256747446788, 0.0009771112852218874663, 0.001172497944769030145, 0.001367884604316172825, 0.001563271263863315720 ),
 .UNSPECIFIED. ) ;
#84074=VECTOR ( 'NONE', #57579, 1000.000000000000114 ) ;
#84075=ORIENTED_EDGE ( 'NONE', *, *, #15382, .T. ) ;
#84077=CARTESIAN_POINT ( 'NONE',  ( -9.469528151039281028, -3.236590943229499029, 32.36255958852954251 ) ) ;
#84078=CARTESIAN_POINT ( 'NONE',  ( 8.769230769230768274, -12.37446782046654192, 30.86335684631486131 ) ) ;
#84079=CARTESIAN_POINT ( 'NONE',  ( 6.857806922520603976, -3.083524468853724443, 32.58852847137143272 ) ) ;
#84080=LINE ( 'NONE', #9728, #26363 ) ;
#84081=CARTESIAN_POINT ( 'NONE',  ( 17.93391658904412012, -8.973038597847269315, 34.52809138561120506 ) ) ;
#84082=EDGE_CURVE ( 'NONE', #49317, #27628, #77212, .T. ) ;
#84083=EDGE_LOOP ( 'NONE', ( #23033, #13732, #21037, #80067 ) ) ;
#84084=EDGE_CURVE ( 'NONE', #31229, #4299, #15967, .T. ) ;
#84086=EDGE_LOOP ( 'NONE', ( #69180, #53747 ) ) ;
#84087=ORIENTED_EDGE ( 'NONE', *, *, #54957, .F. ) ;
#84088=CARTESIAN_POINT ( 'NONE',  ( 4.403900573759605308, -12.41089969410671223, 31.60739465890703670 ) ) ;
#84089=ORIENTED_EDGE ( 'NONE', *, *, #47485, .F. ) ;
#84090=CARTESIAN_POINT ( 'NONE',  ( -13.38461538461538325, -11.16473453929635440, 33.15142922261926373 ) ) ;
#84091=B_SPLINE_CURVE_WITH_KNOTS ( 'NONE', 3,
 ( #48745, #88004, #68577, #124, #76214, #41551, #7330, #7768, #26265, #81218 ),
 .UNSPECIFIED., .F., .F.,
 ( 4, 2, 2, 2, 4 ),
 ( 0.0007817359430256392216, 0.0009771253907250078159, 0.001172514838424376302, 0.001367904286123745004, 0.001563293733823113490 ),
 .UNSPECIFIED. ) ;
#84092=CARTESIAN_POINT ( 'NONE',  ( -10.74607608205217346, -4.809359713505814149, 33.96456829005828837 ) ) ;
#84093=CARTESIAN_POINT ( 'NONE',  ( -21.00000000000000355, -2.249999999999999556, 27.25000000000000000 ) ) ;
#84094=CARTESIAN_POINT ( 'NONE',  ( -15.90379173393269596, -5.642605341092955307, 34.66089969410670335 ) ) ;
#84095=VERTEX_POINT ( 'NONE', #48524 ) ;
#84096=ORIENTED_EDGE ( 'NONE', *, *, #73270, .T. ) ;
#84097=ORIENTED_EDGE ( 'NONE', *, *, #54725, .T. ) ;
#84098=CARTESIAN_POINT ( 'NONE',  ( -6.923076923077045919, -3.083524468854526912, 32.58852847137268327 ) ) ;
#84099=CARTESIAN_POINT ( 'NONE',  ( 11.66898697669518725, -5.915461855592780260, 34.75538340440931506 ) ) ;
#84100=ORIENTED_EDGE ( 'NONE', *, *, #52499, .T. ) ;
#84101=CARTESIAN_POINT ( 'NONE',  ( -8.769230769230768274, -1.367168528481310208, 33.57946703557072254 ) ) ;
#84103=CARTESIAN_POINT ( 'NONE',  ( -3.164700879766790820, -9.780366693483667717, 34.19971097300155805 ) ) ;
#84104=ORIENTED_EDGE ( 'NONE', *, *, #9178, .T. ) ;
#84105=CARTESIAN_POINT ( 'NONE',  ( -11.53846153846153655, -4.786620604624113540, 33.94971097300155094 ) ) ;
#84107=VERTEX_POINT ( 'NONE', #41795 ) ;
#84108=FACE_BOUND ( 'NONE', #9580, .T. ) ;
#84109=CARTESIAN_POINT ( 'NONE',  ( -11.53846153846153655, -11.35647404775217417, 33.31231777344666511 ) ) ;
#84110=CARTESIAN_POINT ( 'NONE',  ( 13.51514082284903040, -6.808710257144161559, 34.95449254468098843 ) ) ;
#84111=DIRECTION ( 'NONE',  ( -0.000000000000000000, 0.7660444431189791237, -0.6427876096865379196 ) ) ;
#84112=CARTESIAN_POINT ( 'NONE',  ( 7.846153846153723244, -11.06231777344772027, 33.60647404775119895 ) ) ;
#84113=CARTESIAN_POINT ( 'NONE',  ( 15.10020931715586556, -2.254533558242299396, 29.97296025877828285 ) ) ;
#84114=DIRECTION ( 'NONE',  ( 0.000000000000000000, 0.3420201433256610524, 0.9396926207859113145 ) ) ;
#84115=CARTESIAN_POINT ( 'NONE',  ( 14.55774672760575861, -2.318338780012835443, 30.59689888758630261 ) ) ;
#84116=VERTEX_POINT ( 'NONE', #41343 ) ;
#84117=CARTESIAN_POINT ( 'NONE',  ( -4.153846153846274980, -2.379036618888197729, 30.90682066428292885 ) ) ;
#84118=EDGE_CURVE ( 'NONE', #85950, #25790, #15205, .T. ) ;
#84119=CARTESIAN_POINT ( 'NONE',  ( -6.066082379360133281, -11.35647404775217595, 33.31231777344666511 ) ) ;
#84120=ORIENTED_EDGE ( 'NONE', *, *, #29686, .T. ) ;
#84121=B_SPLINE_CURVE_WITH_KNOTS ( 'NONE', 3,
 ( #24953, #65932, #24505, #9664, #65036, #86235, #3347, #51509, #85780, #31724 ),
 .UNSPECIFIED., .F., .F.,
 ( 4, 2, 2, 2, 4 ),
 ( 0.000000000000000000, 0.0001954311564186871184, 0.0003908623128373742367, 0.0005862934692560614093, 0.0007817246256747484735 ),
 .UNSPECIFIED. ) ;
#84122=EDGE_CURVE ( 'NONE', #67157, #44863, #62919, .T. ) ;
#84123=B_SPLINE_CURVE_WITH_KNOTS ( 'NONE', 3,
 ( #64225, #10189, #57478, #37204, #83650, #15619, #21931, #23248, #49405, #23688 ),
 .UNSPECIFIED., .F., .F.,
 ( 4, 2, 2, 2, 4 ),
 ( 0.000000000000000000, 0.0001954339857564078809, 0.0003908679715128157619, 0.0005863019572692236428, 0.0007817359430256315238 ),
 .UNSPECIFIED. ) ;
#84124=CARTESIAN_POINT ( 'NONE',  ( -2.307692307692305711, -1.242168528481310874, 33.36296068462461051 ) ) ;
#84125=B_SPLINE_CURVE_WITH_KNOTS ( 'NONE', 3,
 ( #39530, #18355, #87274, #61543, #67429, #59776, #66989, #47143, #66542, #81397 ),
 .UNSPECIFIED., .F., .F.,
 ( 4, 2, 2, 2, 4 ),
 ( 0.000000000000000000, 0.0001954311564186870371, 0.0003908623128373740741, 0.0005862934692560610840, 0.0007817246256747481482 ),
 .UNSPECIFIED. ) ;
#84126=DIRECTION ( 'NONE',  ( -0.000000000000000000, 0.9848077530122085754, -0.1736481776669273613 ) ) ;
#84127=CARTESIAN_POINT ( 'NONE',  ( 16.15384615384603251, -6.835583212225970762, 34.95778746994575670 ) ) ;
#84128=CARTESIAN_POINT ( 'NONE',  ( -7.846153846153967493, -11.06231777344772027, 33.60647404775119895 ) ) ;
#84129=B_SPLINE_CURVE_WITH_KNOTS ( 'NONE', 3,
 ( #77000, #84648, #8987, #2206, #56717, #58037, #85522, #49952, #29699, #15300 ),
 .UNSPECIFIED., .F., .F.,
 ( 4, 2, 2, 2, 4 ),
 ( 0.000000000000000000, 0.0001954311564186862510, 0.0003908623128373725020, 0.0005862934692560588072, 0.0007817246256747450040 ),
 .UNSPECIFIED. ) ;
#84130=CARTESIAN_POINT ( 'NONE',  ( -0.2115929431903194047, -12.43552623307873972, 30.55307653245132826 ) ) ;
#84131=CARTESIAN_POINT ( 'NONE',  ( -4.403869378067608586, -2.341070481393820124, 30.72580821765574299 ) ) ;
#84132=AXIS2_PLACEMENT_3D ( 'NONE', #26161, #6348, #5453 ) ;
#84133=FACE_BOUND ( 'NONE', #22490, .T. ) ;
#84134=CARTESIAN_POINT ( 'NONE',  ( -2.438383774359863754, -6.413092428213692742, 34.63065189839063152 ) ) ;
#84136=CARTESIAN_POINT ( 'NONE',  ( -15.90390063549801347, -2.587454068350149239, 30.68340429815432557 ) ) ;
#84137=CARTESIAN_POINT ( 'NONE',  ( -17.77722045873158763, -11.41317474335729543, 32.86274602512330034 ) ) ;
#84138=DIRECTION ( 'NONE',  ( 0.000000000000000000, 0.7660444431189822323, -0.6427876096865344779 ) ) ;
#84140=DIRECTION ( 'NONE',  ( -0.000000000000000000, -0.8660254037844399289, -0.4999999999999980016 ) ) ;
#84142=VERTEX_POINT ( 'NONE', #69694 ) ;
#84143=EDGE_LOOP ( 'NONE', ( #24152, #69319, #30115, #40392 ) ) ;
#84144=AXIS2_PLACEMENT_3D ( 'NONE', #57879, #21546, #85364 ) ;
#84145=CARTESIAN_POINT ( 'NONE',  ( -9.469296340694842939, -11.76359900205217457, 32.36225158514719880 ) ) ;
#84146=CARTESIAN_POINT ( 'NONE',  ( -15.48074597481782178, -5.643011162660950042, 34.66104346484419096 ) ) ;
#84147=CYLINDRICAL_SURFACE ( 'NONE', #56040, 0.2499999999999979738 ) ;
#84148=CARTESIAN_POINT ( 'NONE',  ( -1.608100328339332696, -3.236172620538810385, 32.36188796281390267 ) ) ;
#84149=CARTESIAN_POINT ( 'NONE',  ( -4.023320715612510590, -3.068774925481847493, 32.56582465632704526 ) ) ;
#84151=CARTESIAN_POINT ( 'NONE',  ( -12.68502338610279523, -4.225889041578353655, 33.85425143139329407 ) ) ;
#84152=CARTESIAN_POINT ( 'NONE',  ( 17.99999999999987566, -3.300289026999228437, 32.46337939537709616 ) ) ;
#84153=ADVANCED_FACE ( 'NONE', ( #35918 ), #22830, .F. ) ;
#84154=CARTESIAN_POINT ( 'NONE',  ( -0.4615384615384611200, -3.322132147404559976, 32.92929555188717927 ) ) ;
#84155=CARTESIAN_POINT ( 'NONE',  ( -1.384615384615383471, -12.37446782046654192, 30.86335684631486131 ) ) ;
#84156=CYLINDRICAL_SURFACE ( 'NONE', #29570, 0.2499999999999986955 ) ;
#84157=DIRECTION ( 'NONE',  ( -0.000000000000000000, -0.7660444431189791237, -0.6427876096865379196 ) ) ;
#84158=CARTESIAN_POINT ( 'NONE',  ( 12.46153846153833911, -2.379036618888197729, 30.90682066428292885 ) ) ;
#84159=CARTESIAN_POINT ( 'NONE',  ( 7.976679547917409963, -6.852161475712352789, 34.70806712695775786 ) ) ;
#84160=ORIENTED_EDGE ( 'NONE', *, *, #82044, .F. ) ;
#84161=CARTESIAN_POINT ( 'NONE',  ( 12.39545608217832395, -3.937682226553330445, 33.60647404775217240 ) ) ;
#84162=CARTESIAN_POINT ( 'NONE',  ( 0.6843180028068690524, -2.600157965045226227, 30.74683119005207743 ) ) ;
#84165=B_SPLINE_CURVE_WITH_KNOTS ( 'NONE', 3,
 ( #71465, #17872, #58841, #10667, #78227, #65592 ),
 .UNSPECIFIED., .F., .F.,
 ( 4, 2, 4 ),
 ( 0.000000000000000000, 0.0001954784845028902692, 0.0003909569690057805385 ),
 .UNSPECIFIED. ) ;
#84166=CARTESIAN_POINT ( 'NONE',  ( -2.438382910802614933, -4.684245665217971144, 34.18127051446801090 ) ) ;
#84167=CARTESIAN_POINT ( 'NONE',  ( -16.02332071561251325, -2.647132371071621471, 31.75357179365173010 ) ) ;
#84169=CARTESIAN_POINT ( 'NONE',  ( -9.822455662039390134, -5.915902021225889484, 34.75552854090298638 ) ) ;
#84170=CARTESIAN_POINT ( 'NONE',  ( -16.15384615384615330, -10.51840700105979565, 33.73612834413961536 ) ) ;
#84172=CARTESIAN_POINT ( 'NONE',  ( 7.146088274689773812, -3.587049720035815348, 32.86302985866382897 ) ) ;
#84173=EDGE_CURVE ( 'NONE', #75262, #85639, #56626, .T. ) ;
#84174=CARTESIAN_POINT ( 'NONE',  ( -5.076923076923197442, -10.21337939537710326, 33.94971097300076224 ) ) ;
#84175=VERTEX_POINT ( 'NONE', #75560 ) ;
#84176=LINE ( 'NONE', #22889, #10324 ) ;
#84177=VECTOR ( 'NONE', #8039, 1000.000000000000000 ) ;
#84178=CARTESIAN_POINT ( 'NONE',  ( 6.923076923076800782, -5.941354392335915335, 34.76329471203413846 ) ) ;
#84179=VERTEX_POINT ( 'NONE', #34584 ) ;
#84180=CARTESIAN_POINT ( 'NONE',  ( -4.153846153846152411, -1.466349020453238561, 30.81389545987213907 ) ) ;
#84181=CARTESIAN_POINT ( 'NONE',  ( -16.08777780284371772, -3.050289026998446840, 32.03036669348366416 ) ) ;
#84182=ADVANCED_FACE ( 'NONE', ( #49428 ), #28714, .F. ) ;
#84183=CARTESIAN_POINT ( 'NONE',  ( 12.52760579488853665, -11.91647553114624358, 32.58852847137148245 ) ) ;
#84184=ORIENTED_EDGE ( 'NONE', *, *, #16463, .F. ) ;
#84185=EDGE_LOOP ( 'NONE', ( #32109, #5311, #39058, #28265 ) ) ;
#84186=ORIENTED_EDGE ( 'NONE', *, *, #31459, .T. ) ;
#84187=CARTESIAN_POINT ( 'NONE',  ( -7.173053667125516952, -2.318417181685854978, 30.59732222474233865 ) ) ;
#84189=CARTESIAN_POINT ( 'NONE',  ( 15.23076923076923173, -9.058645607665452459, 34.76329471203371924 ) ) ;
#84190=EDGE_CURVE ( 'NONE', #34444, #45063, #83673, .T. ) ;
#84191=B_SPLINE_CURVE_WITH_KNOTS ( 'NONE', 3,
 ( #51610, #36792, #71901, #79107, #24155, #57945, #2117, #17412, #23706, #50286 ),
 .UNSPECIFIED., .F., .F.,
 ( 4, 2, 2, 2, 4 ),
 ( 0.0007817246256747442451, 0.0009771112852218865989, 0.001172497944769029061, 0.001367884604316171523, 0.001563271263863313986 ),
 .UNSPECIFIED. ) ;
#84192=LINE ( 'NONE', #49054, #88092 ) ;
#84193=EDGE_CURVE ( 'NONE', #10767, #73377, #40710, .T. ) ;
#84194=EDGE_CURVE ( 'NONE', #77626, #34382, #20279, .T. ) ;
#84197=DIRECTION ( 'NONE',  ( -0.000000000000000000, 0.6427876096865404731, -0.7660444431189770143 ) ) ;
#84198=ORIENTED_EDGE ( 'NONE', *, *, #87629, .F. ) ;
#84199=EDGE_CURVE ( 'NONE', #30802, #87033, #16082, .T. ) ;
#84200=EDGE_CURVE ( 'NONE', #20277, #17317, #10214, .T. ) ;
#84201=CARTESIAN_POINT ( 'NONE',  ( 17.32686859527121470, -5.057305518903949526, 34.11320923018887896 ) ) ;
#84202=ORIENTED_EDGE ( 'NONE', *, *, #76748, .F. ) ;
#84205=VECTOR ( 'NONE', #7088, 1000.000000000000227 ) ;
#84206=ORIENTED_EDGE ( 'NONE', *, *, #69441, .T. ) ;
#84207=CARTESIAN_POINT ( 'NONE',  ( 5.999999999999878320, -6.835583212225970762, 34.95778746994575670 ) ) ;
#84208=ORIENTED_EDGE ( 'NONE', *, *, #70263, .T. ) ;
#84209=CARTESIAN_POINT ( 'NONE',  ( -6.700297381808513641, -11.41317474335729187, 32.86274602512330034 ) ) ;
#84210=ORIENTED_EDGE ( 'NONE', *, *, #20076, .F. ) ;
#84211=CARTESIAN_POINT ( 'NONE',  ( -0.7115151924808159611, -10.66389620160130036, 33.62221079203477103 ) ) ;
#84213=EDGE_LOOP ( 'NONE', ( #23579, #32173 ) ) ;
#84214=DIRECTION ( 'NONE',  ( 0.000000000000000000, 0.4999999999999985567, 0.8660254037844395958 ) ) ;
#84215=CARTESIAN_POINT ( 'NONE',  ( -8.769230769230890843, -8.613356846316285953, 34.62446782046622218 ) ) ;
#84216=DIRECTION ( 'NONE',  ( -0.000000000000000000, 0.5000000000000011102, -0.8660254037844380415 ) ) ;
#84217=B_SPLINE_CURVE_WITH_KNOTS ( 'NONE', 3,
 ( #50274, #37216, #51151, #69680, #30462, #71011, #9320, #63362, #62905, #49844 ),
 .UNSPECIFIED., .F., .F.,
 ( 4, 2, 2, 2, 4 ),
 ( 0.000000000000000000, 0.0001954339857564080707, 0.0003908679715128161414, 0.0005863019572692241849, 0.0007817359430256322827 ),
 .UNSPECIFIED. ) ;
#84218=FACE_BOUND ( 'NONE', #37808, .T. ) ;
#84219=CARTESIAN_POINT ( 'NONE',  ( -9.561517251340742263, -3.957578996910242619, 33.62503395064540257 ) ) ;
#84220=CARTESIAN_POINT ( 'NONE',  ( -18.00000000000000000, -2.538708090699994813, 30.37095296980875858 ) ) ;
#84221=B_SPLINE_CURVE_WITH_KNOTS ( 'NONE', 3,
 ( #33087, #53355, #32211, #74519, #59668, #87168 ),
 .UNSPECIFIED., .F., .F.,
 ( 4, 2, 4 ),
 ( 0.0003909512603273747875, 0.0005862562993132002616, 0.0007815613382990257898 ),
 .UNSPECIFIED. ) ;
#84222=CARTESIAN_POINT ( 'NONE',  ( 8.769230769230647482, -2.625532179533778709, 30.86335684631627174 ) ) ;
#84224=CARTESIAN_POINT ( 'NONE',  ( -5.750054481651858396, -2.824170634883622188, 31.52227843825338738 ) ) ;
#84225=CARTESIAN_POINT ( 'NONE',  ( -11.31568199719312773, -3.236590943229499029, 32.36255958852954251 ) ) ;
#84226=DIRECTION ( 'NONE',  ( 0.000000000000000000, 0.9848077530122072432, 0.1736481776669354937 ) ) ;
#84227=VERTEX_POINT ( 'NONE', #50287 ) ;
#84228=CARTESIAN_POINT ( 'NONE',  ( -6.065250990161240807, -2.506253911140460477, 30.00000000000013856 ) ) ;
#84229=ORIENTED_EDGE ( 'NONE', *, *, #36555, .F. ) ;
#84231=AXIS2_PLACEMENT_3D ( 'NONE', #18024, #74297, #86495 ) ;
#84232=CARTESIAN_POINT ( 'NONE',  ( 14.53070365930516061, -3.587049720035815348, 32.86302985866382897 ) ) ;
#84233=CARTESIAN_POINT ( 'NONE',  ( -3.454254155333559950, -5.827078755546623690, 34.72654668319379567 ) ) ;
#84234=CARTESIAN_POINT ( 'NONE',  ( 16.15384615384603251, -9.442884908241554243, 34.35708131394783038 ) ) ;
#84235=LINE ( 'NONE', #62168, #23580 ) ;
#84236=DIRECTION ( 'NONE',  ( -0.000000000000000000, 0.1736481776669307198, -0.9848077530122080203 ) ) ;
#84237=CARTESIAN_POINT ( 'NONE',  ( -3.903900744468109973, -3.520799739797214389, 33.17531984108286025 ) ) ;
#84238=VERTEX_POINT ( 'NONE', #65138 ) ;
#84239=CARTESIAN_POINT ( 'NONE',  ( 11.47237915910140771, -3.322132147404559532, 32.92929555188719348 ) ) ;
#84240=DIRECTION ( 'NONE',  ( 0.000000000000000000, 0.6427876096865368094, 0.7660444431189802339 ) ) ;
#84241=CARTESIAN_POINT ( 'NONE',  ( -10.36533030374629583, -9.943054286541403997, 34.11300777759954883 ) ) ;
#84242=CARTESIAN_POINT ( 'NONE',  ( 15.45354889974729318, -12.47679350104403007, 31.42216943046555855 ) ) ;
#84243=CARTESIAN_POINT ( 'NONE',  ( 2.557637717070351258, -5.766571408460171355, 34.70601412856602508 ) ) ;
#84245=VERTEX_POINT ( 'NONE', #2994 ) ;
#84246=B_SPLINE_CURVE_WITH_KNOTS ( 'NONE', 3,
 ( #89017, #19646, #20093, #46676, #7017, #88138, #20965, #40815, #75475, #7473 ),
 .UNSPECIFIED., .F., .F.,
 ( 4, 2, 2, 2, 4 ),
 ( 0.000000000000000000, 0.0001954311564186872539, 0.0003908623128373745078, 0.0005862934692560617346, 0.0007817246256747490156 ),
 .UNSPECIFIED. ) ;
#84248=DIRECTION ( 'NONE',  ( 0.000000000000000000, 0.4999999999999985567, 0.8660254037844395958 ) ) ;
#84249=EDGE_LOOP ( 'NONE', ( #72655, #45369, #70841, #74269 ) ) ;
#84250=CARTESIAN_POINT ( 'NONE',  ( -9.942330929600657896, -12.43535235679832596, 30.55408501211184813 ) ) ;
#84251=CARTESIAN_POINT ( 'NONE',  ( -1.134560964701931240, -10.06805714834173848, 34.32951233291982618 ) ) ;
#84252=DIRECTION ( 'NONE',  ( 0.000000000000000000, 0.9396926207859126468, -0.3420201433256571111 ) ) ;
#84253=CARTESIAN_POINT ( 'NONE',  ( 2.530471976670375600, -10.23759521482555357, 34.22997729860117033 ) ) ;
#84254=CARTESIAN_POINT ( 'NONE',  ( -2.176900499867520988, -4.809403383903226192, 33.96459661697924304 ) ) ;
#84258=CARTESIAN_POINT ( 'NONE',  ( -2.057746789344164551, -10.76462480002816235, 33.53768742498949962 ) ) ;
#84259=EDGE_LOOP ( 'NONE', ( #23244, #63419, #48611, #56896, #56045, #17753 ) ) ;
#84260=CARTESIAN_POINT ( 'NONE',  ( 3.230769230769110045, -12.46129190930018460, 30.37095296980731973 ) ) ;
#84261=CARTESIAN_POINT ( 'NONE',  ( 16.85343813319912698, -3.754499324213721234, 33.06261337010820256 ) ) ;
#84262=B_SPLINE_CURVE_WITH_KNOTS ( 'NONE', 3,
 ( #70692, #84661, #2216, #23809, #8997, #58049, #85095, #78319, #10317, #64355 ),
 .UNSPECIFIED., .F., .F.,
 ( 4, 2, 2, 2, 4 ),
 ( 0.0007817246256747554124, 0.0009771112852218991757, 0.001172497944769043156, 0.001367884604316187136, 0.001563271263863330899 ),
 .UNSPECIFIED. ) ;
#84263=CARTESIAN_POINT ( 'NONE',  ( 15.45378207486263200, -2.889357225399416418, 32.26129605718031002 ) ) ;
#84264=B_SPLINE_CURVE_WITH_KNOTS ( 'NONE', 3,
 ( #50145, #49712, #77188, #78072, #29460, #16374, #43841, #56907, #15940, #43405 ),
 .UNSPECIFIED., .F., .F.,
 ( 4, 2, 2, 2, 4 ),
 ( 0.000000000000000000, 0.0001954311564186865221, 0.0003908623128373730441, 0.0005862934692560595662, 0.0007817246256747460882 ),
 .UNSPECIFIED. ) ;
#84265=FACE_OUTER_BOUND ( 'NONE', #4404, .T. ) ;
#84266=CYLINDRICAL_SURFACE ( 'NONE', #66611, 0.2499999999999995559 ) ;
#84267=CARTESIAN_POINT ( 'NONE',  ( -8.096177083446809419, -12.43535235679832596, 30.55408501211184813 ) ) ;
#84269=ORIENTED_EDGE ( 'NONE', *, *, #4580, .F. ) ;
#84270=B_SPLINE_CURVE_WITH_KNOTS ( 'NONE', 3,
 ( #88213, #32351, #40890, #68352, #6650, #59818, #34120, #61586, #12526, #53498 ),
 .UNSPECIFIED., .F., .F.,
 ( 4, 2, 2, 2, 4 ),
 ( 0.000000000000000000, 0.0001954339881912772715, 0.0003908679763825545429, 0.0005863019645738318415, 0.0007817359527651090859 ),
 .UNSPECIFIED. ) ;
#84271=CARTESIAN_POINT ( 'NONE',  ( -39.05038313613820122, -2.249999999999998668, 29.75000000000000355 ) ) ;
#84272=CARTESIAN_POINT ( 'NONE',  ( -17.14300545628321260, -4.661471528628507777, 34.16647553114621871 ) ) ;
#84274=B_SPLINE_CURVE_WITH_KNOTS ( 'NONE', 3,
 ( #14913, #50009, #1825, #28875, #56331, #83821, #36507, #42827, #50445, #85136 ),
 .UNSPECIFIED., .F., .F.,
 ( 4, 2, 2, 2, 4 ),
 ( 0.0007817359430256270785, 0.0009771253907249926370, 0.001172514838424358087, 0.001367904286123723754, 0.001563293733823089204 ),
 .UNSPECIFIED. ) ;
#84275=ADVANCED_FACE ( 'NONE', ( #72345 ), #2551, .F. ) ;
#84276=CARTESIAN_POINT ( 'NONE',  ( -16.15384615384615330, -11.35647404775217417, 33.31231777344666511 ) ) ;
#84277=CARTESIAN_POINT ( 'NONE',  ( -7.596099426240392027, -2.920487667080175154, 32.31805714834172960 ) ) ;
#84278=ORIENTED_EDGE ( 'NONE', *, *, #47063, .T. ) ;
#84280=CARTESIAN_POINT ( 'NONE',  ( -5.300408020647025431, -6.760086850603068243, 34.69517049084099369 ) ) ;
#84281=AXIS2_PLACEMENT_3D ( 'NONE', #65681, #80102, #17514 ) ;
#84282=ORIENTED_EDGE ( 'NONE', *, *, #88088, .T. ) ;
#84283=CARTESIAN_POINT ( 'NONE',  ( 9.822355127558148880, -7.723484941389743952, 34.99544897038808955 ) ) ;
#84284=VERTEX_POINT ( 'NONE', #51161 ) ;
#84286=FACE_OUTER_BOUND ( 'NONE', #48498, .T. ) ;
#84287=EDGE_CURVE ( 'NONE', #70953, #32825, #10655, .T. ) ;
#84288=CARTESIAN_POINT ( 'NONE',  ( -0.4615384615385840772, -10.33852847137269571, 34.16647553114546554 ) ) ;
#84289=CARTESIAN_POINT ( 'NONE',  ( -12.21148404162501144, -10.82426656108012075, 33.81400080652039009 ) ) ;
#84290=EDGE_LOOP ( 'NONE', ( #86469, #35666 ) ) ;
#84291=CYLINDRICAL_SURFACE ( 'NONE', #23982, 0.2500000000000012212 ) ;
#84292=ORIENTED_EDGE ( 'NONE', *, *, #55478, .F. ) ;
#84293=DIRECTION ( 'NONE',  ( 0.000000000000000000, 0.9396926207859126468, 0.3420201433256571111 ) ) ;
#84294=CARTESIAN_POINT ( 'NONE',  ( 8.769230769230645706, -3.643525952248795718, 33.31231777344771672 ) ) ;
#84295=AXIS2_PLACEMENT_3D ( 'NONE', #44024, #17004, #10256 ) ;
#84296=ORIENTED_EDGE ( 'NONE', *, *, #13081, .F. ) ;
#84297=CARTESIAN_POINT ( 'NONE',  ( -6.130690603110307002, -10.70098750199973203, 33.91152734681376302 ) ) ;
#84298=CARTESIAN_POINT ( 'NONE',  ( -12.71151519248081740, -5.728515186090277211, 34.42611988154120439 ) ) ;
#84299=CARTESIAN_POINT ( 'NONE',  ( -11.66915214157184622, -2.845849958028613624, 32.17971566917920967 ) ) ;
#84300=CARTESIAN_POINT ( 'NONE',  ( 13.38461538461538680, -6.681629849574314051, 35.83090037661290239 ) ) ;
#84302=B_SPLINE_CURVE_WITH_KNOTS ( 'NONE', 3,
 ( #77039, #15340, #42816, #36061, #30607, #78796, #45899, #10792, #23405, #66168 ),
 .UNSPECIFIED., .F., .F.,
 ( 4, 2, 2, 2, 4 ),
 ( 0.0007817359430256297891, 0.0009771253907249958896, 0.001172514838424361990, 0.001367904286123728091, 0.001563293733823094191 ),
 .UNSPECIFIED. ) ;
#84303=EDGE_CURVE ( 'NONE', #13360, #87648, #48179, .T. ) ;
#84304=ADVANCED_FACE ( 'NONE', ( #43545 ), #44414, .F. ) ;
#84305=VERTEX_POINT ( 'NONE', #50730 ) ;
#84306=ORIENTED_EDGE ( 'NONE', *, *, #21829, .T. ) ;
#84307=FACE_BOUND ( 'NONE', #21227, .T. ) ;
#84308=ORIENTED_EDGE ( 'NONE', *, *, #71298, .T. ) ;
#84309=CARTESIAN_POINT ( 'NONE',  ( 6.923076923076800782, -10.33852847137269571, 34.16647553114546554 ) ) ;
#84311=CARTESIAN_POINT ( 'NONE',  ( 6.249945409378047323, -2.986452184633680673, 32.43230066228895225 ) ) ;
#84312=CARTESIAN_POINT ( 'NONE',  ( 0.5920638997721064944, -12.70449254468099198, 30.44128974285582956 ) ) ;
#84313=EDGE_CURVE ( 'NONE', #34976, #28470, #64692, .T. ) ;
#84314=ORIENTED_EDGE ( 'NONE', *, *, #26088, .T. ) ;
#84315=ORIENTED_EDGE ( 'NONE', *, *, #53817, .F. ) ;
#84317=CARTESIAN_POINT ( 'NONE',  ( 11.66898724022509981, -11.46989282347013095, 32.79007818306219946 ) ) ;
#84318=EDGE_LOOP ( 'NONE', ( #46617, #46244, #20808, #14279 ) ) ;
#84320=DIRECTION ( 'NONE',  ( -0.000000000000000000, 0.9396926207859093161, -0.3420201433256663259 ) ) ;
#84321=DIRECTION ( 'NONE',  ( -0.000000000000000000, 0.5000000000000011102, -0.8660254037844380415 ) ) ;
#84323=ORIENTED_EDGE ( 'NONE', *, *, #29907, .T. ) ;
#84324=CARTESIAN_POINT ( 'NONE',  ( -8.638705330997126453, -4.299079248970732792, 33.91157788607253565 ) ) ;
#84325=B_SPLINE_CURVE_WITH_KNOTS ( 'NONE', 3,
 ( #54476, #33333, #33769, #88733, #88301, #47725, #42312, #13495, #14381, #54028 ),
 .UNSPECIFIED., .F., .F.,
 ( 4, 2, 2, 2, 4 ),
 ( 0.0007817246256747505334, 0.0009771112852218939715, 0.001172497944769037518, 0.001367884604316181064, 0.001563271263863324611 ),
 .UNSPECIFIED. ) ;
#84326=CARTESIAN_POINT ( 'NONE',  ( 0.5276068125408999165, -11.69971097300155272, 32.46337939537588113 ) ) ;
#84327=CARTESIAN_POINT ( 'NONE',  ( -17.77479207347668932, -7.628180278152856708, 34.99865929289143196 ) ) ;
#84329=EDGE_LOOP ( 'NONE', ( #61558, #36005 ) ) ;
#84330=VERTEX_POINT ( 'NONE', #72787 ) ;
#84333=CARTESIAN_POINT ( 'NONE',  ( 1.449870524128224814, -11.67786785259547777, 32.92929555188713664 ) ) ;
#84334=B_SPLINE_CURVE_WITH_KNOTS ( 'NONE', 3,
 ( #26652, #951, #55890, #5946, #54109, #63529, #37380, #50883, #64403, #1391 ),
 .UNSPECIFIED., .F., .F.,
 ( 4, 2, 2, 2, 4 ),
 ( 0.0007817246256747445703, 0.0009771112852218870326, 0.001172497944769029495, 0.001367884604316171957, 0.001563271263863314419 ),
 .UNSPECIFIED. ) ;
#84335=CARTESIAN_POINT ( 'NONE',  ( 9.692307692307695177, -4.661471528628507777, 34.16647553114623292 ) ) ;
#84336=LINE ( 'NONE', #71233, #59527 ) ;
#84337=FACE_BOUND ( 'NONE', #41125, .T. ) ;
#84338=CARTESIAN_POINT ( 'NONE',  ( -9.692307692307691624, -13.75783147151868846, 33.36296068462461051 ) ) ;
#84339=VERTEX_POINT ( 'NONE', #24606 ) ;
#84340=DIRECTION ( 'NONE',  ( -0.000000000000000000, 0.9848077530122086864, -0.1736481776669273891 ) ) ;
#84341=LINE ( 'NONE', #83002, #28715 ) ;
#84342=CARTESIAN_POINT ( 'NONE',  ( 14.30769230769231015, -4.786620604624113540, 33.94971097300155094 ) ) ;
#84343=CARTESIAN_POINT ( 'NONE',  ( -11.31568199719312240, -3.755027918224367323, 33.06320215134714857 ) ) ;
#84344=ORIENTED_EDGE ( 'NONE', *, *, #61810, .T. ) ;
#84345=CARTESIAN_POINT ( 'NONE',  ( 6.222779668978065004, -10.97394488606064122, 33.68653795673694873 ) ) ;
#84346=VERTEX_POINT ( 'NONE', #52072 ) ;
#84347=FACE_BOUND ( 'NONE', #16513, .T. ) ;
#84348=CARTESIAN_POINT ( 'NONE',  ( 18.22301135161285046, -3.587049720035815348, 32.86302985866382897 ) ) ;
#84349=AXIS2_PLACEMENT_3D ( 'NONE', #52574, #54349, #66997 ) ;
#84350=CARTESIAN_POINT ( 'NONE',  ( -6.923076923076922462, -11.35647404775217417, 33.31231777344666511 ) ) ;
#84351=CARTESIAN_POINT ( 'NONE',  ( -3.100243529005668019, -8.586989748646452369, 34.63063291749215011 ) ) ;
#84352=ORIENTED_EDGE ( 'NONE', *, *, #59134, .T. ) ;
#84353=CARTESIAN_POINT ( 'NONE',  ( 12.46153846153846168, -12.29105614889573062, 35.45975837776705220 ) ) ;
#84354=CARTESIAN_POINT ( 'NONE',  ( 5.299885980484561721, -7.369474270740069777, 34.74850911626239736 ) ) ;
#84355=CARTESIAN_POINT ( 'NONE',  ( 8.703148389870632329, -2.292212530054419606, 30.41441678777542634 ) ) ;
#84356=CARTESIAN_POINT ( 'NONE',  ( 6.250054311638314708, -3.627508038966690496, 32.91356715214248396 ) ) ;
#84357=EDGE_LOOP ( 'NONE', ( #54218, #39245, #56582, #83096 ) ) ;
#84358=EDGE_CURVE ( 'NONE', #27674, #60953, #80424, .T. ) ;
#84359=DIRECTION ( 'NONE',  ( 0.000000000000000000, 0.6427876096865373645, -0.7660444431189797898 ) ) ;
#84360=ORIENTED_EDGE ( 'NONE', *, *, #18647, .F. ) ;
#84361=CARTESIAN_POINT ( 'NONE',  ( 13.60762673622823726, -12.15243808032445827, 31.58219941686247978 ) ) ;
#84362=ORIENTED_EDGE ( 'NONE', *, *, #68677, .F. ) ;
#84363=CARTESIAN_POINT ( 'NONE',  ( -8.899841128855296546, -7.722926236386453702, 34.74524107206102030 ) ) ;
#84364=CYLINDRICAL_SURFACE ( 'NONE', #21137, 0.2499999999999993616 ) ;
#84365=DIRECTION ( 'NONE',  ( -0.000000000000000000, 0.9848077530122085754, -0.1736481776669273613 ) ) ;
#84366=CARTESIAN_POINT ( 'NONE',  ( -12.46153846153846168, -13.20930481340135110, 34.54067556320372745 ) ) ;
#84367=CARTESIAN_POINT ( 'NONE',  ( -12.46153846153846168, -8.810774026931790459, 35.74407628777942847 ) ) ;
#84369=CARTESIAN_POINT ( 'NONE',  ( 12.59158606779414491, -7.723484964179501588, 34.74522123443823318 ) ) ;
#84371=VERTEX_POINT ( 'NONE', #4337 ) ;
#84372=CARTESIAN_POINT ( 'NONE',  ( 4.153846153846154188, -1.242168528481310874, 33.36296068462461051 ) ) ;
#84373=LINE ( 'NONE', #15911, #48147 ) ;
#84374=ORIENTED_EDGE ( 'NONE', *, *, #66327, .F. ) ;
#84375=EDGE_CURVE ( 'NONE', #41758, #60114, #59995, .T. ) ;
#84376=ORIENTED_EDGE ( 'NONE', *, *, #70715, .F. ) ;
#84377=ORIENTED_EDGE ( 'NONE', *, *, #73075, .F. ) ;
#84378=CARTESIAN_POINT ( 'NONE',  ( 10.74617505635156789, -8.191423895709840863, 34.95447573519442130 ) ) ;
#84380=CARTESIAN_POINT ( 'NONE',  ( -17.20707028636129721, -9.418419913701741919, 34.36755862841477693 ) ) ;
#84381=DIRECTION ( 'NONE',  ( -0.000000000000000000, 0.8660254037844397068, -0.4999999999999978906 ) ) ;
#84383=CARTESIAN_POINT ( 'NONE',  ( 12.46153846153846168, -6.386643153685126251, 34.62446782046654192 ) ) ;
#84385=DIRECTION ( 'NONE',  ( -1.000000000000000000, 0.000000000000000000, 0.000000000000000000 ) ) ;
#84386=VECTOR ( 'NONE', #18130, 1000.000000000000000 ) ;
#84387=DIRECTION ( 'NONE',  ( -0.000000000000000000, -0.1736481776669307198, -0.9848077530122080203 ) ) ;
#84388=CARTESIAN_POINT ( 'NONE',  ( -1.384615384615383471, -6.386643153685126251, 34.62446782046654192 ) ) ;
#84389=EDGE_CURVE ( 'NONE', #41035, #57710, #33594, .T. ) ;
#84392=B_SPLINE_CURVE_WITH_KNOTS ( 'NONE', 3,
 ( #25297, #45113, #73040, #11791, #65821, #18103, #39270, #59520, #79804, #73938 ),
 .UNSPECIFIED., .F., .F.,
 ( 4, 2, 2, 2, 4 ),
 ( 0.0007817246336856291692, 0.0009771112958940103739, 0.001172497958102391470, 0.001367884620310772566, 0.001563271282519153879 ),
 .UNSPECIFIED. ) ;
#84393=ADVANCED_FACE ( 'NONE', ( #88122 ), #39474, .F. ) ;
#84395=CARTESIAN_POINT ( 'NONE',  ( 0.4615384615383396616, -9.442884908241554243, 34.35708131394783038 ) ) ;
#84396=CARTESIAN_POINT ( 'NONE',  ( -16.02380109792638407, -2.254550872974305342, 29.97347326024527092 ) ) ;
#84398=CARTESIAN_POINT ( 'NONE',  ( 12.52679403281448423, -10.90142922261932057, 33.41473453929631887 ) ) ;
#84399=ORIENTED_EDGE ( 'NONE', *, *, #33523, .F. ) ;
#84400=AXIS2_PLACEMENT_3D ( 'NONE', #82513, #13593, #40196 ) ;
#84401=CARTESIAN_POINT ( 'NONE',  ( 6.130791807824786943, -4.809403383903225304, 33.96459661697924304 ) ) ;
#84402=CARTESIAN_POINT ( 'NONE',  ( 9.692307692307695177, -2.833524468853757305, 32.15551576947925838 ) ) ;
#84403=CARTESIAN_POINT ( 'NONE',  ( -9.561782254074046250, -3.625058011473228703, 33.29252011169590020 ) ) ;
#84404=EDGE_CURVE ( 'NONE', #59603, #68701, #41573, .T. ) ;
#84405=ORIENTED_EDGE ( 'NONE', *, *, #66124, .T. ) ;
#84406=CARTESIAN_POINT ( 'NONE',  ( 16.28437159207980045, -10.31582465632704704, 34.18122507451815295 ) ) ;
#84408=ORIENTED_EDGE ( 'NONE', *, *, #60193, .F. ) ;
#84409=B_SPLINE_CURVE_WITH_KNOTS ( 'NONE', 3,
 ( #14462, #7714, #14012, #35174, #75281, #28413, #55883, #21657, #49128, #20770 ),
 .UNSPECIFIED., .F., .F.,
 ( 4, 2, 2, 2, 4 ),
 ( 0.0007817246256747416430, 0.0009771112852218831295, 0.001172497944769024508, 0.001367884604316165886, 0.001563271263863307481 ),
 .UNSPECIFIED. ) ;
#84410=CARTESIAN_POINT ( 'NONE',  ( 9.692307692307572609, -11.94971097300221174, 32.03036669348237098 ) ) ;
#84411=CARTESIAN_POINT ( 'NONE',  ( -17.01166793741023042, -3.643525952247864019, 33.31231777344670064 ) ) ;
#84414=CARTESIAN_POINT ( 'NONE',  ( -1.449885385171703733, -9.528491918058357157, 34.59228464037090589 ) ) ;
#84415=EDGE_CURVE ( 'NONE', #52853, #46179, #80000, .T. ) ;
#84416=CARTESIAN_POINT ( 'NONE',  ( -9.822998295417999515, -8.191372820521381826, 34.95448215188424967 ) ) ;
#84417=CARTESIAN_POINT ( 'NONE',  ( -11.53846153846153655, -9.058645607665452459, 34.76329471203371924 ) ) ;
#84418=ORIENTED_EDGE ( 'NONE', *, *, #62086, .T. ) ;
#84419=ORIENTED_EDGE ( 'NONE', *, *, #31385, .T. ) ;
#84420=B_SPLINE_CURVE_WITH_KNOTS ( 'NONE', 3,
 ( #75553, #12978, #12534, #40018, #13854, #41334, #33253, #60713, #88220, #62042 ),
 .UNSPECIFIED., .F., .F.,
 ( 4, 2, 2, 2, 4 ),
 ( 0.0007817359430256324996, 0.0009771253907249993591, 0.001172514838424366110, 0.001367904286123732861, 0.001563293733823099829 ),
 .UNSPECIFIED. ) ;
#84421=ORIENTED_EDGE ( 'NONE', *, *, #12493, .T. ) ;
#84422=AXIS2_PLACEMENT_3D ( 'NONE', #47463, #13249, #40730 ) ;
#84423=CARTESIAN_POINT ( 'NONE',  ( -10.74607521849491754, -12.35290016733513951, 31.75349464988449455 ) ) ;
#84424=B_SPLINE_CURVE_WITH_KNOTS ( 'NONE', 3,
 ( #20679, #76063, #48143, #22449, #852, #69751, #75613, #41401, #14362, #49036 ),
 .UNSPECIFIED., .F., .F.,
 ( 4, 2, 2, 2, 4 ),
 ( 0.0007817246256747451124, 0.0009771112852218881168, 0.001172497944769031230, 0.001367884604316174126, 0.001563271263863317238 ),
 .UNSPECIFIED. ) ;
#84425=CARTESIAN_POINT ( 'NONE',  ( -12.46153846153858424, -12.70778746994576025, 30.41441678777401236 ) ) ;
#84426=CYLINDRICAL_SURFACE ( 'NONE', #78193, 0.2499999999999979738 ) ;
#84427=B_SPLINE_CURVE_WITH_KNOTS ( 'NONE', 3,
 ( #45012, #78804, #17561, #38271, #64393, #44561, #37821, #65290, #86018, #31511 ),
 .UNSPECIFIED., .F., .F.,
 ( 4, 2, 2, 2, 4 ),
 ( 0.000000000000000000, 0.0001954311584214072923, 0.0003908623168428145846, 0.0005862934752642218498, 0.0007817246336856291692 ),
 .UNSPECIFIED. ) ;
#84429=CARTESIAN_POINT ( 'NONE',  ( -18.00000000000000000, -4.098570777380720287, 33.41473453929634729 ) ) ;
#84430=DIRECTION ( 'NONE',  ( -0.000000000000000000, 1.000000000000000000, 3.491481338843133355E-15 ) ) ;
#84431=VERTEX_POINT ( 'NONE', #26834 ) ;
#84432=EDGE_LOOP ( 'NONE', ( #39117, #84206, #77502, #23222, #16828, #7095 ) ) ;
#84433=ORIENTED_EDGE ( 'NONE', *, *, #63760, .F. ) ;
#84434=DIRECTION ( 'NONE',  ( -0.000000000000000000, -0.3420201433256694346, -0.9396926207859080948 ) ) ;
#84435=VERTEX_POINT ( 'NONE', #40796 ) ;
#84436=CARTESIAN_POINT ( 'NONE',  ( 9.019230769232187583, -7.500000000000154543, 35.00000000000007105 ) ) ;
#84437=CARTESIAN_POINT ( 'NONE',  ( 13.38461538461538680, -3.937682226553329556, 33.60647404775216529 ) ) ;
#84438=ADVANCED_FACE ( 'NONE', ( #66491 ), #6120, .F. ) ;
#84441=EDGE_LOOP ( 'NONE', ( #65013, #86496 ) ) ;
#84443=CARTESIAN_POINT ( 'NONE',  ( 5.300349475837862201, -7.630147987733840509, 34.99859428049665411 ) ) ;
#84445=ORIENTED_EDGE ( 'NONE', *, *, #52394, .F. ) ;
#84446=FACE_BOUND ( 'NONE', #27781, .T. ) ;
#84447=CARTESIAN_POINT ( 'NONE',  ( 13.51514082284903040, -12.50538340440932394, 31.33453814440721885 ) ) ;
#84448=CARTESIAN_POINT ( 'NONE',  ( 7.976679284387491187, -5.915461855592780260, 34.75538340440931506 ) ) ;
#84449=ORIENTED_EDGE ( 'NONE', *, *, #88796, .T. ) ;
#84450=CARTESIAN_POINT ( 'NONE',  ( 16.15384615384603251, -11.48612834414049644, 32.76840700105863391 ) ) ;
#84451=CARTESIAN_POINT ( 'NONE',  ( 16.15384615384615330, -4.098570777380720287, 33.41473453929634729 ) ) ;
#84452=AXIS2_PLACEMENT_3D ( 'NONE', #31887, #23771, #73312 ) ;
#84453=LINE ( 'NONE', #70034, #46449 ) ;
#84455=CARTESIAN_POINT ( 'NONE',  ( 1.384615384615386802, -11.69971097300155272, 32.46337939537588113 ) ) ;
#84456=ADVANCED_FACE ( 'NONE', ( #40354 ), #12868, .F. ) ;
#84457=B_SPLINE_CURVE_WITH_KNOTS ( 'NONE', 3,
 ( #86147, #24870, #79382, #53230, #3264, #79833, #66307, #10923, #24418, #45587 ),
 .UNSPECIFIED., .F., .F.,
 ( 4, 2, 2, 2, 4 ),
 ( 0.0007817246256747434861, 0.0009771112852218861652, 0.001172497944769028844, 0.001367884604316171740, 0.001563271263863314419 ),
 .UNSPECIFIED. ) ;
#84458=CARTESIAN_POINT ( 'NONE',  ( -7.146003140593069958, -11.24512374952581872, 33.06303171183252942 ) ) ;
#84459=CARTESIAN_POINT ( 'NONE',  ( -8.096130590202434973, -12.01397095200674059, 32.43157075238190146 ) ) ;
#84460=CARTESIAN_POINT ( 'NONE',  ( -5.999999999999998224, -5.557115091759785130, 34.35708131394839171 ) ) ;
#84461=CARTESIAN_POINT ( 'NONE',  ( 5.776515056276054771, -5.113361153441932316, 34.14387501736621999 ) ) ;
#84462=CARTESIAN_POINT ( 'NONE',  ( -18.22292621751613950, -6.503392248772476236, 34.64988816332204635 ) ) ;
#84463=CARTESIAN_POINT ( 'NONE',  ( -1.384615384615383471, -5.471508081941601098, 34.59228464037088457 ) ) ;
#84464=CARTESIAN_POINT ( 'NONE',  ( 13.31934493865461100, -11.94971097300153140, 32.03036669348370680 ) ) ;
#84465=CARTESIAN_POINT ( 'NONE',  ( -2.307692307692305711, -2.708943851104267164, 35.45975837776705220 ) ) ;
#84466=CARTESIAN_POINT ( 'NONE',  ( -16.15384615384627409, -11.94971097300221174, 32.03036669348237098 ) ) ;
#84467=CARTESIAN_POINT ( 'NONE',  ( -11.47239318745910275, -11.16473453929635440, 33.15142922261926373 ) ) ;
#84468=CARTESIAN_POINT ( 'NONE',  ( 5.750023269057646935, -10.66389620160130036, 33.62221079203477103 ) ) ;
#84469=CARTESIAN_POINT ( 'NONE',  ( 13.63461538461532641, -7.565270000091922853, 34.99999999999999289 ) ) ;
#84471=EDGE_LOOP ( 'NONE', ( #10904, #62682 ) ) ;
#84475=EDGE_CURVE ( 'NONE', #56543, #77704, #5050, .T. ) ;
#84476=VECTOR ( 'NONE', #12866, 1000.000000000000114 ) ;
#84477=ORIENTED_EDGE ( 'NONE', *, *, #24772, .F. ) ;
#84478=CARTESIAN_POINT ( 'NONE',  ( 16.02369894440793274, -11.47017969459903952, 32.78971311882035167 ) ) ;
#84479=ORIENTED_EDGE ( 'NONE', *, *, #39423, .F. ) ;
#84480=CARTESIAN_POINT ( 'NONE',  ( -7.846153846153844924, -5.557115091759785130, 34.35708131394839171 ) ) ;
#84482=CARTESIAN_POINT ( 'NONE',  ( -17.86920955903305597, -9.084667340241228572, 34.75534355489798344 ) ) ;
#84483=EDGE_CURVE ( 'NONE', #26289, #21025, #50163, .T. ) ;
#84484=CARTESIAN_POINT ( 'NONE',  ( 13.45068271796546533, -2.833524468853757750, 32.15551576947925838 ) ) ;
#84485=CARTESIAN_POINT ( 'NONE',  ( 17.86930939688969033, -2.295517848115769421, 30.44137282052136939 ) ) ;
#84486=CARTESIAN_POINT ( 'NONE',  ( -7.846153846153844924, -13.53365097954675988, 30.81389545987213552 ) ) ;
#84487=CARTESIAN_POINT ( 'NONE',  ( -13.38461538461538325, -8.164416787775445883, 34.95778746994557906 ) ) ;
#84488=CARTESIAN_POINT ( 'NONE',  ( -13.38461538461538325, -11.91647553114624181, 32.58852847137148245 ) ) ;
#84490=CARTESIAN_POINT ( 'NONE',  ( -1.384615384615383471, -12.62096338111211580, 30.90682066428153263 ) ) ;
#84491=CARTESIAN_POINT ( 'NONE',  ( 6.923076923076924238, -12.29105614889573062, 35.45975837776705220 ) ) ;
#84492=ADVANCED_FACE ( 'NONE', ( #70479 ), #75902, .F. ) ;
#84493=CARTESIAN_POINT ( 'NONE',  ( 10.39189969082028675, -5.827078755546623690, 34.72654668319379567 ) ) ;
#84495=B_SPLINE_CURVE_WITH_KNOTS ( 'NONE', 3,
 ( #40307, #45717, #67769, #54240, #32215, #59676, #80407, #52907, #25451, #18705 ),
 .UNSPECIFIED., .F., .F.,
 ( 4, 2, 2, 2, 4 ),
 ( 0.000000000000000000, 0.0001954339857564081520, 0.0003908679715128163040, 0.0005863019572692244018, 0.0007817359430256326080 ),
 .UNSPECIFIED. ) ;
#84496=CARTESIAN_POINT ( 'NONE',  ( -10.48485917715096782, -5.915461855592780260, 34.75538340440931506 ) ) ;
#84497=VERTEX_POINT ( 'NONE', #63268 ) ;
#84498=CARTESIAN_POINT ( 'NONE',  ( 17.07692307692307665, -12.10708131394839349, 31.69288490824020244 ) ) ;
#84499=CARTESIAN_POINT ( 'NONE',  ( 12.23805353697412812, -8.539481045369596401, 34.89627647299170832 ) ) ;
#84500=FACE_OUTER_BOUND ( 'NONE', #59700, .T. ) ;
#84501=CARTESIAN_POINT ( 'NONE',  ( 14.98076923076923173, -7.500000000000001776, 35.00000000000000000 ) ) ;
#84502=LINE ( 'NONE', #50242, #46402 ) ;
#84503=CARTESIAN_POINT ( 'NONE',  ( 9.469381474791545017, -11.24512374952581872, 33.06303171183252942 ) ) ;
#84504=FACE_OUTER_BOUND ( 'NONE', #31177, .T. ) ;
#84505=B_SPLINE_CURVE_WITH_KNOTS ( 'NONE', 3,
 ( #9051, #23862, #15809, #56776, #71174, #30203, #44576, #1838, #72063, #36520 ),
 .UNSPECIFIED., .F., .F.,
 ( 4, 2, 2, 2, 4 ),
 ( 0.000000000000000000, 0.0001954339857564081520, 0.0003908679715128163040, 0.0005863019572692244018, 0.0007817359430256326080 ),
 .UNSPECIFIED. ) ;
#84507=EDGE_CURVE ( 'NONE', #35065, #45495, #51263, .T. ) ;
#84508=ORIENTED_EDGE ( 'NONE', *, *, #51063, .T. ) ;
#84509=ORIENTED_EDGE ( 'NONE', *, *, #57571, .F. ) ;
#84510=EDGE_CURVE ( 'NONE', #16561, #36288, #28609, .T. ) ;
#84511=ORIENTED_EDGE ( 'NONE', *, *, #68219, .F. ) ;
#84513=CARTESIAN_POINT ( 'NONE',  ( -4.153846153846273204, -3.300289026999228881, 32.46337939537708905 ) ) ;
#84514=CARTESIAN_POINT ( 'NONE',  ( -8.835313148590907772, -2.292212530054419606, 30.41441678777542634 ) ) ;
#84515=EDGE_CURVE ( 'NONE', #363, #13588, #84662, .T. ) ;
#84516=VECTOR ( 'NONE', #34744, 1000.000000000000000 ) ;
#84517=CARTESIAN_POINT ( 'NONE',  ( 4.284371855609720114, -3.816742781228458448, 33.13167719472716044 ) ) ;
#84518=CARTESIAN_POINT ( 'NONE',  ( 17.86985279056177944, -9.418419913701741919, 34.36755862841477693 ) ) ;
#84519=VERTEX_POINT ( 'NONE', #68699 ) ;
#84520=CARTESIAN_POINT ( 'NONE',  ( -17.14219352288385778, -4.481592998940161721, 33.73612834413957984 ) ) ;
#84521=ORIENTED_EDGE ( 'NONE', *, *, #48641, .F. ) ;
#84522=ORIENTED_EDGE ( 'NONE', *, *, #25118, .F. ) ;
#84523=B_SPLINE_CURVE_WITH_KNOTS ( 'NONE', 3,
 ( #83865, #14957, #28923, #22151, #991, #28017, #55925, #76197, #49619, #14500 ),
 .UNSPECIFIED., .F., .F.,
 ( 4, 2, 2, 2, 4 ),
 ( 0.0007817359430256388964, 0.0009771253907250073822, 0.001172514838424375868, 0.001367904286123744354, 0.001563293733823112840 ),
 .UNSPECIFIED. ) ;
#84524=CARTESIAN_POINT ( 'NONE',  ( 4.153846153846030731, -12.51329471203414379, 31.30864560766407578 ) ) ;
#84525=EDGE_LOOP ( 'NONE', ( #15718, #85117, #42161, #24675 ) ) ;
#84526=CARTESIAN_POINT ( 'NONE',  ( 8.703147358274886614, -2.721908614388770964, 31.22303859784723912 ) ) ;
#84527=EDGE_CURVE ( 'NONE', #84330, #4777, #46986, .T. ) ;
#84528=CARTESIAN_POINT ( 'NONE',  ( -10.86540785267757947, -5.056417327199099532, 34.11270091957321426 ) ) ;
#84529=AXIS2_PLACEMENT_3D ( 'NONE', #72359, #66040, #10669 ) ;
#84531=CARTESIAN_POINT ( 'NONE',  ( -9.758391103263569732, -8.120952969808774569, 34.71129190930000163 ) ) ;
#84532=CARTESIAN_POINT ( 'NONE',  ( -12.23816252084027845, -2.501478030877323455, 29.88021232661721172 ) ) ;
#84533=ORIENTED_EDGE ( 'NONE', *, *, #43902, .F. ) ;
#84534=EDGE_LOOP ( 'NONE', ( #3865, #35408 ) ) ;
#84536=ORIENTED_EDGE ( 'NONE', *, *, #53291, .T. ) ;
#84537=CARTESIAN_POINT ( 'NONE',  ( -14.17764470143662336, -7.723484964179501588, 34.74522123443823318 ) ) ;
#84538=CARTESIAN_POINT ( 'NONE',  ( 1.161130440891438242, -8.496056993536548418, 34.65000542017679663 ) ) ;
#84539=ORIENTED_EDGE ( 'NONE', *, *, #66246, .F. ) ;
#84540=DIRECTION ( 'NONE',  ( -0.000000000000000000, -0.8660254037844397068, -0.4999999999999978906 ) ) ;
#84542=EDGE_CURVE ( 'NONE', #17855, #456, #57684, .T. ) ;
#84543=DIRECTION ( 'NONE',  ( -0.000000000000000000, -0.8660254037844397068, -0.4999999999999978906 ) ) ;
#84544=ORIENTED_EDGE ( 'NONE', *, *, #50247, .T. ) ;
#84546=DIRECTION ( 'NONE',  ( -0.000000000000000000, -0.7660444431189791237, -0.6427876096865379196 ) ) ;
#84547=CARTESIAN_POINT ( 'NONE',  ( -15.00775638667583678, -12.38742843783360748, 31.66772728687926985 ) ) ;
#84548=ORIENTED_EDGE ( 'NONE', *, *, #80208, .T. ) ;
#84549=FACE_BOUND ( 'NONE', #14201, .T. ) ;
#84550=ADVANCED_FACE ( 'NONE', ( #82224 ), #20513, .F. ) ;
#84551=CARTESIAN_POINT ( 'NONE',  ( -10.83886953994894675, -4.988325925672468131, 34.36044203135681130 ) ) ;
#84552=DIRECTION ( 'NONE',  ( -0.000000000000000000, 0.3420201433256694346, -0.9396926207859080948 ) ) ;
#84553=CARTESIAN_POINT ( 'NONE',  ( 2.241609928332171986, -12.34228464037088280, 31.77849191805838558 ) ) ;
#84554=B_SPLINE_CURVE_WITH_KNOTS ( 'NONE', 3,
 ( #19194, #80911, #38579, #86343, #58836, #65587, #32270, #87227, #52078, #39033 ),
 .UNSPECIFIED., .F., .F.,
 ( 4, 2, 2, 2, 4 ),
 ( 0.000000000000000000, 0.0001954311564186865763, 0.0003908623128373731525, 0.0005862934692560596746, 0.0007817246256747463051 ),
 .UNSPECIFIED. ) ;
#84556=DIRECTION ( 'NONE',  ( 0.000000000000000000, 0.9848077530122072432, -0.1736481776669354937 ) ) ;
#84557=CARTESIAN_POINT ( 'NONE',  ( -3.296851610129364563, -3.322132147404559976, 32.92929555188719348 ) ) ;
#84558=DIRECTION ( 'NONE',  ( -0.000000000000000000, -0.9848077530122085754, -0.1736481776669273613 ) ) ;
#84559=ORIENTED_EDGE ( 'NONE', *, *, #68157, .T. ) ;
#84560=LINE ( 'NONE', #22835, #17346 ) ;
#84561=DIRECTION ( 'NONE',  ( -0.000000000000000000, 0.9396926207859093161, -0.3420201433256663259 ) ) ;
#84562=ORIENTED_EDGE ( 'NONE', *, *, #47317, .T. ) ;
#84563=EDGE_CURVE ( 'NONE', #32782, #35007, #74926, .T. ) ;
#84564=CARTESIAN_POINT ( 'NONE',  ( -16.28453675695646652, -12.62707690430377383, 30.88035979386743435 ) ) ;
#84565=CARTESIAN_POINT ( 'NONE',  ( 10.39189967166066708, -6.760086850603066466, 34.69517049084099369 ) ) ;
#84566=CARTESIAN_POINT ( 'NONE',  ( 2.980769230769232170, -7.500000000000001776, 34.75000000000000000 ) ) ;
#84567=CARTESIAN_POINT ( 'NONE',  ( -5.326899807865431491, -11.79746400365624659, 32.30657167506340954 ) ) ;
#84568=VECTOR ( 'NONE', #85671, 1000.000000000000227 ) ;
#84569=CARTESIAN_POINT ( 'NONE',  ( -18.00000000000000711, -2.252971138473345292, 29.99985851721553942 ) ) ;
#84570=CARTESIAN_POINT ( 'NONE',  ( -8.992156986746916658, -5.667676309546437530, 34.40238873228292249 ) ) ;
#84571=FACE_BOUND ( 'NONE', #72135, .T. ) ;
#84572=EDGE_CURVE ( 'NONE', #20155, #22078, #44305, .T. ) ;
#84573=CARTESIAN_POINT ( 'NONE',  ( -2.557715544985271094, -6.695914987888143877, 34.68535235679833306 ) ) ;
#84574=DIRECTION ( 'NONE',  ( -0.000000000000000000, -0.1736481776669307198, -0.9848077530122080203 ) ) ;
#84575=CARTESIAN_POINT ( 'NONE',  ( -18.06527000055631760, -8.656820664281497102, 34.87096338111211935 ) ) ;
#84576=CARTESIAN_POINT ( 'NONE',  ( -3.164700879766790820, -11.69971097300155272, 32.46337939537588113 ) ) ;
#84577=CARTESIAN_POINT ( 'NONE',  ( -15.00798968950081758, -6.760870238392817200, 34.69528174975672385 ) ) ;
#84578=CYLINDRICAL_SURFACE ( 'NONE', #36120, 0.2499999999999998890 ) ;
#84579=AXIS2_PLACEMENT_3D ( 'NONE', #73009, #11307, #25269 ) ;
#84581=VERTEX_POINT ( 'NONE', #36692 ) ;
#84582=EDGE_LOOP ( 'NONE', ( #23583, #81057, #12843, #77633 ) ) ;
#84583=DIRECTION ( 'NONE',  ( -0.000000000000000000, -0.5000000000000009992, -0.8660254037844380415 ) ) ;
#84584=AXIS2_PLACEMENT_3D ( 'NONE', #57672, #57233, #79284 ) ;
#84585=CARTESIAN_POINT ( 'NONE',  ( -4.376772371362300795, -3.105860786376062332, 32.13614157043599562 ) ) ;
#84586=CARTESIAN_POINT ( 'NONE',  ( -0.5268084620947812713, -3.643525952247789412, 33.31231777344662959 ) ) ;
#84587=CARTESIAN_POINT ( 'NONE',  ( -16.82686876528476105, -11.28795663066794575, 33.01431243580653785 ) ) ;
#84588=CARTESIAN_POINT ( 'NONE',  ( -16.37677237136229991, -12.15238873228291716, 31.58232369045353849 ) ) ;
#84591=CARTESIAN_POINT ( 'NONE',  ( -8.546451227962359454, -2.847695495035523550, 31.58253572463339154 ) ) ;
#84592=CARTESIAN_POINT ( 'NONE',  ( 3.930361229281823743, -12.11044203135681840, 32.26167407432752299 ) ) ;
#84593=EDGE_CURVE ( 'NONE', #48918, #81272, #82428, .T. ) ;
#84594=CARTESIAN_POINT ( 'NONE',  ( -16.82686876528476105, -5.728107161865375829, 34.42597550085002922 ) ) ;
#84595=CYLINDRICAL_SURFACE ( 'NONE', #18580, 0.2500000000000009437 ) ;
#84596=CARTESIAN_POINT ( 'NONE',  ( -16.82697766754503377, -4.932303261841488151, 34.32971442181322885 ) ) ;
#84597=CARTESIAN_POINT ( 'NONE',  ( 12.21151523731700550, -12.68155406624981119, 30.59749803192733708 ) ) ;
#84598=B_SPLINE_CURVE_WITH_KNOTS ( 'NONE', 3,
 ( #17155, #87418, #45960, #10411, #86529, #73891, #73450, #79762, #23902, #18056 ),
 .UNSPECIFIED., .F., .F.,
 ( 4, 2, 2, 2, 4 ),
 ( 0.000000000000000000, 0.0001954339857564072033, 0.0003908679715128144066, 0.0005863019572692215828, 0.0007817359430256288133 ),
 .UNSPECIFIED. ) ;
#84599=CYLINDRICAL_SURFACE ( 'NONE', #50569, 0.2499999999999986955 ) ;
#84600=CARTESIAN_POINT ( 'NONE',  ( 8.069165197766697162, -6.503523203565941380, 34.64991518177335195 ) ) ;
#84602=FACE_OUTER_BOUND ( 'NONE', #44027, .T. ) ;
#84603=CARTESIAN_POINT ( 'NONE',  ( 7.173131234715239835, -4.943051570960391494, 34.04725096376909477 ) ) ;
#84605=CARTESIAN_POINT ( 'NONE',  ( 0.7115928814519133505, -3.435999193479609026, 33.07426656108010832 ) ) ;
#84608=ORIENTED_EDGE ( 'NONE', *, *, #17809, .F. ) ;
#84609=CARTESIAN_POINT ( 'NONE',  ( -16.28440674558808254, -2.504760397472873823, 29.97295953869789997 ) ) ;
#84610=CARTESIAN_POINT ( 'NONE',  ( 12.21151522424549896, -5.851115903089112003, 34.47074536777953568 ) ) ;
#84611=ORIENTED_EDGE ( 'NONE', *, *, #85566, .F. ) ;
#84612=CARTESIAN_POINT ( 'NONE',  ( 9.442307692307693401, -2.499999999999998668, 29.75000000000000355 ) ) ;
#84613=CARTESIAN_POINT ( 'NONE',  ( -12.46153846153846168, -6.343179335718451384, 34.87096338111211935 ) ) ;
#84615=CARTESIAN_POINT ( 'NONE',  ( -13.25382357679060519, -2.541949514083464479, 30.39797389878540557 ) ) ;
#84617=DIRECTION ( 'NONE',  ( 0.000000000000000000, 0.3420201433256610524, 0.9396926207859113145 ) ) ;
#84618=EDGE_LOOP ( 'NONE', ( #71764, #12503 ) ) ;
#84619=FACE_OUTER_BOUND ( 'NONE', #19876, .T. ) ;
#84620=CARTESIAN_POINT ( 'NONE',  ( -11.76138849736838488, -12.38737895849757820, 31.66785238281580206 ) ) ;
#84622=CARTESIAN_POINT ( 'NONE',  ( 12.68431813051652846, -12.11081565061823717, 32.26097654155341843 ) ) ;
#84623=EDGE_LOOP ( 'NONE', ( #17187, #85594 ) ) ;
#84624=ORIENTED_EDGE ( 'NONE', *, *, #49464, .F. ) ;
#84625=EDGE_CURVE ( 'NONE', #85495, #74166, #53375, .T. ) ;
#84627=CARTESIAN_POINT ( 'NONE',  ( -18.06608341095587988, -3.513871655860376197, 32.76840700105978499 ) ) ;
#84628=CARTESIAN_POINT ( 'NONE',  ( -6.000000000000121680, -5.941354392335915335, 34.76329471203413846 ) ) ;
#84629=EDGE_CURVE ( 'NONE', #51377, #27221, #44762, .T. ) ;
#84630=B_SPLINE_CURVE_WITH_KNOTS ( 'NONE', 3,
 ( #87008, #17182, #44639, #72122, #10437, #38798, #37905, #59504, #4105, #65369 ),
 .UNSPECIFIED., .F., .F.,
 ( 4, 2, 2, 2, 4 ),
 ( 0.000000000000000000, 0.0001954311564186866305, 0.0003908623128373732609, 0.0005862934692560598914, 0.0007817246256747465219 ),
 .UNSPECIFIED. ) ;
#84631=CARTESIAN_POINT ( 'NONE',  ( -4.087778820496076548, -12.62096338111211757, 30.90682066428152908 ) ) ;
#84633=CARTESIAN_POINT ( 'NONE',  ( 17.99999999999987566, -12.16647553114689728, 32.15551576947799362 ) ) ;
#84634=ORIENTED_EDGE ( 'NONE', *, *, #52920, .F. ) ;
#84635=ORIENTED_EDGE ( 'NONE', *, *, #28725, .F. ) ;
#84636=CARTESIAN_POINT ( 'NONE',  ( 9.468822748583747284, -4.386631170607603991, 33.66268669641500111 ) ) ;
#84637=ORIENTED_EDGE ( 'NONE', *, *, #18625, .F. ) ;
#84640=ORIENTED_EDGE ( 'NONE', *, *, #24065, .T. ) ;
#84641=CARTESIAN_POINT ( 'NONE',  ( 7.596177102105255763, -12.01397095200673881, 32.43157075238190146 ) ) ;
#84642=CARTESIAN_POINT ( 'NONE',  ( 7.976679547917409963, -5.195472089885680766, 34.18748526763464923 ) ) ;
#84643=EDGE_LOOP ( 'NONE', ( #4399, #53412, #53205, #13756 ) ) ;
#84644=ORIENTED_EDGE ( 'NONE', *, *, #23992, .T. ) ;
#84645=CARTESIAN_POINT ( 'NONE',  ( -6.792551221313363641, -11.46989282347013095, 32.79007818306219946 ) ) ;
#84646=VERTEX_POINT ( 'NONE', #38023 ) ;
#84647=CARTESIAN_POINT ( 'NONE',  ( 4.284637961670938466, -4.809403383903226192, 33.96459661697924304 ) ) ;
#84648=CARTESIAN_POINT ( 'NONE',  ( 14.24160992833217065, -5.471508081941602875, 34.59228464037088457 ) ) ;
#84649=VERTEX_POINT ( 'NONE', #16858 ) ;
#84650=CARTESIAN_POINT ( 'NONE',  ( 15.00784227186238162, -2.308479472611653094, 30.53278059502174457 ) ) ;
#84651=B_SPLINE_CURVE_WITH_KNOTS ( 'NONE', 3,
 ( #20375, #14050, #75316, #68549, #6845, #41526, #68991, #7300, #34762, #63114 ),
 .UNSPECIFIED., .F., .F.,
 ( 4, 2, 2, 2, 4 ),
 ( 0.0007817359430256328248, 0.0009771253907249995759, 0.001172514838424366327, 0.001367904286123733078, 0.001563293733823099829 ),
 .UNSPECIFIED. ) ;
#84652=CARTESIAN_POINT ( 'NONE',  ( 5.299934428535925335, -11.24521262558773671, 33.06293181088029343 ) ) ;
#84653=FACE_OUTER_BOUND ( 'NONE', #65544, .T. ) ;
#84654=FACE_BOUND ( 'NONE', #58437, .T. ) ;
#84655=EDGE_CURVE ( 'NONE', #58130, #14228, #39528, .T. ) ;
#84657=CARTESIAN_POINT ( 'NONE',  ( 2.557746619330623528, -8.303483539816728154, 34.68545999027711702 ) ) ;
#84658=CARTESIAN_POINT ( 'NONE',  ( 6.000000000000001776, -12.78798330534102767, 29.49999999999997868 ) ) ;
#84659=B_SPLINE_CURVE_WITH_KNOTS ( 'NONE', 3,
 ( #31422, #85925, #17467, #25107, #78267, #30962, #58429, #9815, #44469, #4391 ),
 .UNSPECIFIED., .F., .F.,
 ( 4, 2, 2, 2, 4 ),
 ( 0.0007817359430256302227, 0.0009771253907249963233, 0.001172514838424362424, 0.001367904286123728524, 0.001563293733823094625 ),
 .UNSPECIFIED. ) ;
#84660=CARTESIAN_POINT ( 'NONE',  ( 0.6849139473108805110, -2.251407671071270489, 29.88021292934942252 ) ) ;
#84661=CARTESIAN_POINT ( 'NONE',  ( -16.08859101433331062, -3.083524468853783951, 32.58852847137153930 ) ) ;
#84662=B_SPLINE_CURVE_WITH_KNOTS ( 'NONE', 3,
 ( #13754, #28152, #41236, #1575, #29063, #7890, #69146, #35356, #56518, #84008 ),
 .UNSPECIFIED., .F., .F.,
 ( 4, 2, 2, 2, 4 ),
 ( 0.000000000000000000, 0.0001954339857564075828, 0.0003908679715128151656, 0.0005863019572692227755, 0.0007817359430256303312 ),
 .UNSPECIFIED. ) ;
#84663=VECTOR ( 'NONE', #23962, 1000.000000000000114 ) ;
#84664=CARTESIAN_POINT ( 'NONE',  ( 8.546303810323914618, -9.172386477786396597, 34.72672124145550043 ) ) ;
#84665=CARTESIAN_POINT ( 'NONE',  ( -16.40386937806761836, -2.588893531581426544, 31.60682220781847818 ) ) ;
#84666=EDGE_LOOP ( 'NONE', ( #33288, #18211, #4703, #32450, #86867, #42385 ) ) ;
#84667=DIRECTION ( 'NONE',  ( -0.000000000000000000, -0.5000000000000009992, -0.8660254037844380415 ) ) ;
#84668=ORIENTED_EDGE ( 'NONE', *, *, #59632, .F. ) ;
#84670=FACE_OUTER_BOUND ( 'NONE', #6019, .T. ) ;
#84671=CARTESIAN_POINT ( 'NONE',  ( 10.74617505635156789, -11.93129842949671726, 32.56571108434900452 ) ) ;
#84672=EDGE_CURVE ( 'NONE', #80991, #41728, #79459, .T. ) ;
#84673=AXIS2_PLACEMENT_3D ( 'NONE', #76600, #14907, #69839 ) ;
#84674=CARTESIAN_POINT ( 'NONE',  ( -6.673022611438608642, -6.567000820036038355, 34.66262288849541306 ) ) ;
#84675=DIRECTION ( 'NONE',  ( -0.000000000000000000, 0.5000000000000011102, -0.8660254037844381525 ) ) ;
#84677=CARTESIAN_POINT ( 'NONE',  ( 14.37294744720514750, -11.67786785259547777, 32.92929555188713664 ) ) ;
#84678=ORIENTED_EDGE ( 'NONE', *, *, #56273, .F. ) ;
#84679=DIRECTION ( 'NONE',  ( 0.000000000000000000, -6.938893903907222067E-15, 1.000000000000000000 ) ) ;
#84680=ADVANCED_FACE ( 'NONE', ( #9655 ), #37119, .F. ) ;
#84682=CARTESIAN_POINT ( 'NONE',  ( 14.24242230713598900, -12.70778746994557551, 30.41441678777548319 ) ) ;
#84683=CARTESIAN_POINT ( 'NONE',  ( 2.307692307692309264, -5.180354513474913603, 36.12317359536750416 ) ) ;
#84684=CARTESIAN_POINT ( 'NONE',  ( -8.638440328263817136, -2.494656445102012565, 31.33466734024120015 ) ) ;
#84688=VERTEX_POINT ( 'NONE', #32160 ) ;
#84689=CARTESIAN_POINT ( 'NONE',  ( -7.715363405186896451, -11.93129842949671726, 32.56571108434900452 ) ) ;
#84690=VERTEX_POINT ( 'NONE', #12767 ) ;
#84691=DIRECTION ( 'NONE',  ( -1.000000000000000000, 0.000000000000000000, 0.000000000000000000 ) ) ;
#84692=CARTESIAN_POINT ( 'NONE',  ( 10.83816415665302380, -2.600157965045224895, 30.74683119005207743 ) ) ;
#84693=DIRECTION ( 'NONE',  ( -0.000000000000000000, -0.8660254037844399289, -0.4999999999999980016 ) ) ;
#84694=CARTESIAN_POINT ( 'NONE',  ( -0.6844654204453088919, -11.98009711892699691, 32.48740034544075428 ) ) ;
#84696=EDGE_CURVE ( 'NONE', #48440, #11752, #87875, .T. ) ;
#84697=CARTESIAN_POINT ( 'NONE',  ( 4.153846153846154188, -5.415277668671390821, 36.20867863119892149 ) ) ;
#84698=ORIENTED_EDGE ( 'NONE', *, *, #78288, .F. ) ;
#84700=CARTESIAN_POINT ( 'NONE',  ( 17.93475006822591666, -2.255955759149247619, 30.00000000000014566 ) ) ;
#84702=CARTESIAN_POINT ( 'NONE',  ( 10.61538461538449596, -10.21337939537710326, 33.94971097300076224 ) ) ;
#84703=CARTESIAN_POINT ( 'NONE',  ( -12.39628289026243202, -3.835265460703683349, 33.15142922261929925 ) ) ;
#84705=EDGE_CURVE ( 'NONE', #72630, #58556, #5126, .T. ) ;
#84706=CARTESIAN_POINT ( 'NONE',  ( 15.23076923076923173, -2.833524468853757305, 32.15551576947925838 ) ) ;
#84707=CARTESIAN_POINT ( 'NONE',  ( 11.66898697669518725, -8.630441415882550871, 34.87705825610312615 ) ) ;
#84708=B_SPLINE_CURVE_WITH_KNOTS ( 'NONE', 3,
 ( #38542, #72754, #46625, #11515, #51570, #65550, #87190, #66454, #73671, #5195 ),
 .UNSPECIFIED., .F., .F.,
 ( 4, 2, 2, 2, 4 ),
 ( 0.0007817359430256297891, 0.0009771253907249958896, 0.001172514838424361990, 0.001367904286123728091, 0.001563293733823094191 ),
 .UNSPECIFIED. ) ;
#84709=CARTESIAN_POINT ( 'NONE',  ( -2.307692307692305711, -13.75783147151868846, 33.36296068462461051 ) ) ;
#84710=CARTESIAN_POINT ( 'NONE',  ( -11.53846153846153655, -2.833524468853757305, 32.15551576947925838 ) ) ;
#84711=B_SPLINE_CURVE_WITH_KNOTS ( 'NONE', 3,
 ( #70928, #64589, #76346, #36262, #14654, #42137, #83571, #76804, #49326, #42573 ),
 .UNSPECIFIED., .F., .F.,
 ( 4, 2, 2, 2, 4 ),
 ( 0.000000000000000000, 0.0001954339857564073659, 0.0003908679715128147319, 0.0005863019572692221250, 0.0007817359430256294638 ),
 .UNSPECIFIED. ) ;
#84713=EDGE_LOOP ( 'NONE', ( #77601, #56046, #21685, #14391 ) ) ;
#84715=EDGE_CURVE ( 'NONE', #35784, #42127, #83542, .T. ) ;
#84716=CARTESIAN_POINT ( 'NONE',  ( -1.253823576790596528, -11.18335022499818621, 33.13157742990016885 ) ) ;
#84717=FACE_OUTER_BOUND ( 'NONE', #34011, .T. ) ;
#84719=CARTESIAN_POINT ( 'NONE',  ( 0.3308469948708994690, -3.530157926970578508, 32.79014554554150607 ) ) ;
#84720=CARTESIAN_POINT ( 'NONE',  ( -7.623141002060447313, -2.889357225399416862, 32.26129605718031712 ) ) ;
#84721=ORIENTED_EDGE ( 'NONE', *, *, #48667, .T. ) ;
#84723=CARTESIAN_POINT ( 'NONE',  ( -2.373775718648186484, -3.050289026998445951, 32.03036669348365706 ) ) ;
#84724=B_SPLINE_CURVE_WITH_KNOTS ( 'NONE', 3,
 ( #80605, #44555, #31961, #87819, #39173, #53552, #24749, #86932, #45905, #58517 ),
 .UNSPECIFIED., .F., .F.,
 ( 4, 2, 2, 2, 4 ),
 ( 0.0007817359430256284880, 0.0009771253907249941549, 0.001172514838424359822, 0.001367904286123725489, 0.001563293733823091156 ),
 .UNSPECIFIED. ) ;
#84725=ORIENTED_EDGE ( 'NONE', *, *, #47187, .T. ) ;
#84726=CARTESIAN_POINT ( 'NONE',  ( -4.219928533206287469, -8.164416787775445883, 34.95778746994557906 ) ) ;
#84729=CARTESIAN_POINT ( 'NONE',  ( 3.164686851409095780, -3.937682226553329556, 33.60647404775217240 ) ) ;
#84730=CARTESIAN_POINT ( 'NONE',  ( -0.5916864312701569650, -10.31621877034669588, 34.18098118002070152 ) ) ;
#84731=CARTESIAN_POINT ( 'NONE',  ( -6.923076923077045919, -2.379036618888197729, 30.90682066428292885 ) ) ;
#84733=CARTESIAN_POINT ( 'NONE',  ( -3.164701897419153642, -2.292212530054420494, 30.41441678777542990 ) ) ;
#84734=EDGE_CURVE ( 'NONE', #49519, #19405, #25465, .T. ) ;
#84735=EDGE_LOOP ( 'NONE', ( #49346, #58224, #55164, #63845 ) ) ;
#84737=LINE ( 'NONE', #50473, #65878 ) ;
#84738=CARTESIAN_POINT ( 'NONE',  ( -10.68146802634049308, -2.721908614388770964, 31.22303859784723912 ) ) ;
#84739=VERTEX_POINT ( 'NONE', #79899 ) ;
#84740=CARTESIAN_POINT ( 'NONE',  ( -0.4615384615384611200, -6.386643153685126251, 34.62446782046654192 ) ) ;
#84741=DIRECTION ( 'NONE',  ( -0.000000000000000000, -0.7660444431189791237, -0.6427876096865379196 ) ) ;
#84742=CARTESIAN_POINT ( 'NONE',  ( -4.153846153845845102, -2.506253911140614576, 30.00000000000323297 ) ) ;
#84743=VECTOR ( 'NONE', #25489, 1000.000000000000000 ) ;
#84744=AXIS2_PLACEMENT_3D ( 'NONE', #4378, #79601, #3478 ) ;
#84745=CARTESIAN_POINT ( 'NONE',  ( 9.442307692307693401, -2.249999999999998668, 29.75000000000000355 ) ) ;
#84746=CARTESIAN_POINT ( 'NONE',  ( -4.153846153846152411, -3.937682226553329556, 33.60647404775216529 ) ) ;
#84747=AXIS2_PLACEMENT_3D ( 'NONE', #65698, #11218, #50411 ) ;
#84748=ORIENTED_EDGE ( 'NONE', *, *, #21257, .F. ) ;
#84749=ORIENTED_EDGE ( 'NONE', *, *, #49248, .T. ) ;
#84750=FACE_BOUND ( 'NONE', #83920, .T. ) ;
#84751=ORIENTED_EDGE ( 'NONE', *, *, #50952, .F. ) ;
#84752=CARTESIAN_POINT ( 'NONE',  ( -5.011730088628421065, -2.255955759149235629, 29.99999999999988631 ) ) ;
#84753=CARTESIAN_POINT ( 'NONE',  ( 17.93472999944368240, -5.941354392334501355, 34.76329471203369792 ) ) ;
#84754=CARTESIAN_POINT ( 'NONE',  ( -18.00000000000000000, -3.937682226553330445, 33.60647404775216529 ) ) ;
#84756=EDGE_CURVE ( 'NONE', #1870, #69237, #64210, .T. ) ;
#84757=ORIENTED_EDGE ( 'NONE', *, *, #9409, .F. ) ;
#84758=CARTESIAN_POINT ( 'NONE',  ( -15.23076923076922995, -2.517432740324522911, 35.29906147534542527 ) ) ;
#84760=CARTESIAN_POINT ( 'NONE',  ( -10.61538461538473399, -9.442884908241554243, 34.35708131394783038 ) ) ;
#84761=CARTESIAN_POINT ( 'NONE',  ( 3.007284287045284721, -2.847400154188067578, 31.58180166144859768 ) ) ;
#84762=AXIS2_PLACEMENT_3D ( 'NONE', #9672, #86246, #23189 ) ;
#84763=CARTESIAN_POINT ( 'NONE',  ( -14.30769230769230660, -6.435427911321262684, 35.78748833219616898 ) ) ;
#84764=FACE_BOUND ( 'NONE', #86466, .T. ) ;
#84765=ORIENTED_EDGE ( 'NONE', *, *, #64791, .T. ) ;
#84766=CARTESIAN_POINT ( 'NONE',  ( -5.207070286361298095, -10.88202310037935661, 33.43294751532457099 ) ) ;
#84767=CARTESIAN_POINT ( 'NONE',  ( -6.249976744048591826, -6.524016743844655686, 34.90889640711025521 ) ) ;
#84768=CARTESIAN_POINT ( 'NONE',  ( 14.30769230769218758, -6.879047030192662504, 34.71129190930017927 ) ) ;
#84769=FACE_OUTER_BOUND ( 'NONE', #41541, .T. ) ;
#84770=VERTEX_POINT ( 'NONE', #52411 ) ;
#84772=EDGE_LOOP ( 'NONE', ( #78774, #83802, #34812, #73652 ) ) ;
#84773=ADVANCED_FACE ( 'NONE', ( #18201 ), #45663, .F. ) ;
#84775=CARTESIAN_POINT ( 'NONE',  ( -8.096130577096200653, -6.567427716900048118, 34.66269422305636283 ) ) ;
#84777=B_SPLINE_CURVE_WITH_KNOTS ( 'NONE', 3,
 ( #30719, #58186, #23955, #10463, #65393, #3687, #56431, #77145, #15451, #42925 ),
 .UNSPECIFIED., .F., .F.,
 ( 4, 2, 2, 2, 4 ),
 ( 0.0007817359430256308733, 0.0009771253907249971907, 0.001172514838424363725, 0.001367904286123730259, 0.001563293733823096577 ),
 .UNSPECIFIED. ) ;
#84778=CARTESIAN_POINT ( 'NONE',  ( -8.703163435880695076, -12.34228464037088813, 31.77849191805839268 ) ) ;
#84779=CARTESIAN_POINT ( 'NONE',  ( -2.307692307692305711, -2.486705287966279876, 31.30864560766543647 ) ) ;
#84780=FACE_BOUND ( 'NONE', #39082, .T. ) ;
#84781=DIRECTION ( 'NONE',  ( -0.000000000000000000, 0.8660254037844399289, -0.4999999999999980016 ) ) ;
#84782=EDGE_LOOP ( 'NONE', ( #49485, #85098 ) ) ;
#84783=DIRECTION ( 'NONE',  ( 0.000000000000000000, 0.1736481776669275834, 0.9848077530122086864 ) ) ;
#84784=EDGE_CURVE ( 'NONE', #85662, #54661, #21147, .T. ) ;
#84785=CARTESIAN_POINT ( 'NONE',  ( -11.76194648218548622, -10.11188796281391511, 34.01382737946119050 ) ) ;
#84786=LINE ( 'NONE', #23068, #89085 ) ;
#84787=DIRECTION ( 'NONE',  ( 0.000000000000000000, 0.7660444431189807890, 0.6427876096865361433 ) ) ;
#84788=ORIENTED_EDGE ( 'NONE', *, *, #24631, .T. ) ;
#84789=CARTESIAN_POINT ( 'NONE',  ( 8.769230769230645706, -12.70778746994576025, 30.41441678777401236 ) ) ;
#84790=EDGE_LOOP ( 'NONE', ( #54284, #83098 ) ) ;
#84791=FACE_BOUND ( 'NONE', #16326, .T. ) ;
#84794=VECTOR ( 'NONE', #64452, 1000.000000000000227 ) ;
#84795=CARTESIAN_POINT ( 'NONE',  ( 4.284371592079796010, -2.647132371071621471, 31.75357179365173010 ) ) ;
#84796=CARTESIAN_POINT ( 'NONE',  ( -11.31545018684868786, -11.76359900205217457, 32.36225158514719880 ) ) ;
#84797=ORIENTED_EDGE ( 'NONE', *, *, #7455, .F. ) ;
#84798=B_SPLINE_CURVE_WITH_KNOTS ( 'NONE', 3,
 ( #55365, #48605, #47728, #88112, #80896, #20939, #54278, #88988, #67366, #81334 ),
 .UNSPECIFIED., .F., .F.,
 ( 4, 2, 2, 2, 4 ),
 ( 0.000000000000000000, 0.0001954339857564071762, 0.0003908679715128143524, 0.0005863019572692215828, 0.0007817359430256287049 ),
 .UNSPECIFIED. ) ;
#84799=CARTESIAN_POINT ( 'NONE',  ( -16.21992853320628925, -11.35647404775217595, 33.31231777344666511 ) ) ;
#84800=CARTESIAN_POINT ( 'NONE',  ( -2.307692307692427391, -4.481592998941358097, 33.73612834414048933 ) ) ;
#84801=CARTESIAN_POINT ( 'NONE',  ( -9.822454901745912181, -3.285722584762969856, 32.44110544564090759 ) ) ;
#84802=CARTESIAN_POINT ( 'NONE',  ( 10.61538461538461675, -6.681629849574314051, 35.83090037661290239 ) ) ;
#84803=ORIENTED_EDGE ( 'NONE', *, *, #27668, .T. ) ;
#84804=B_SPLINE_CURVE_WITH_KNOTS ( 'NONE', 3,
 ( #80341, #19073, #82107, #74910, #88880, #68581, #53287, #27154, #46972, #25832 ),
 .UNSPECIFIED., .F., .F.,
 ( 4, 2, 2, 2, 4 ),
 ( 0.000000000000000000, 0.0001954311564186882568, 0.0003908623128373765136, 0.0005862934692560647703, 0.0007817246256747530271 ),
 .UNSPECIFIED. ) ;
#84805=VECTOR ( 'NONE', #12028, 1000.000000000000000 ) ;
#84807=CARTESIAN_POINT ( 'NONE',  ( -9.692307692307691624, -2.833524468853757305, 32.15551576947925838 ) ) ;
#84808=ORIENTED_EDGE ( 'NONE', *, *, #76024, .T. ) ;
#84810=CARTESIAN_POINT ( 'NONE',  ( 18.06606733335007675, -5.471508081941601098, 34.59228464037088457 ) ) ;
#84811=ORIENTED_EDGE ( 'NONE', *, *, #63330, .F. ) ;
#84812=CARTESIAN_POINT ( 'NONE',  ( -8.992109451659418440, -7.630691491037285168, 34.74850469731152458 ) ) ;
#84813=CARTESIAN_POINT ( 'NONE',  ( 15.16468685140909400, -4.661471528628507777, 34.16647553114621871 ) ) ;
#84814=LINE ( 'NONE', #14561, #88929 ) ;
#84815=EDGE_CURVE ( 'NONE', #54586, #59185, #737, .T. ) ;
#84816=CARTESIAN_POINT ( 'NONE',  ( -15.16562445004959692, -7.750023224968867197, 34.99404313364389907 ) ) ;
#84817=CARTESIAN_POINT ( 'NONE',  ( -8.096130577096198877, -9.148715823498378086, 34.47080413974185120 ) ) ;
#84820=ORIENTED_EDGE ( 'NONE', *, *, #8394, .T. ) ;
#84821=CARTESIAN_POINT ( 'NONE',  ( -15.23076923076922995, -3.513871655860378418, 32.76840700105978499 ) ) ;
#84822=CARTESIAN_POINT ( 'NONE',  ( 5.869852030268307708, -8.630895178749536711, 34.87696386517710323 ) ) ;
#84823=VERTEX_POINT ( 'NONE', #40698 ) ;
#84824=ORIENTED_EDGE ( 'NONE', *, *, #4475, .F. ) ;
#84825=ORIENTED_EDGE ( 'NONE', *, *, #54341, .T. ) ;
#84826=LINE ( 'NONE', #36625, #23911 ) ;
#84827=DIRECTION ( 'NONE',  ( -0.000000000000000000, -0.7660444431189791237, -0.6427876096865379196 ) ) ;
#84828=DIRECTION ( 'NONE',  ( -0.000000000000000000, 0.6427876096865404731, -0.7660444431189770143 ) ) ;
#84830=CARTESIAN_POINT ( 'NONE',  ( -5.076923076923075762, -3.513871655860378418, 32.76840700105978499 ) ) ;
#84831=CARTESIAN_POINT ( 'NONE',  ( -16.85391023282967637, -11.43677907613345113, 33.22367315496201456 ) ) ;
#84832=CARTESIAN_POINT ( 'NONE',  ( 13.60799087038780542, -2.251407671071270489, 29.88021292934943318 ) ) ;
#84833=ORIENTED_EDGE ( 'NONE', *, *, #13592, .F. ) ;
#84834=CARTESIAN_POINT ( 'NONE',  ( 2.980745993476265898, -6.695914987888143877, 34.68535235679833306 ) ) ;
#84835=CARTESIAN_POINT ( 'NONE',  ( -1.515306851282941292, -6.413092428213692742, 34.63065189839063152 ) ) ;
#84836=CARTESIAN_POINT ( 'NONE',  ( 3.230769230769231726, -2.249999999999998668, 29.75000000000001776 ) ) ;
#84837=DIRECTION ( 'NONE',  ( -0.000000000000000000, -0.5000000000000009992, -0.8660254037844380415 ) ) ;
#84838=ORIENTED_EDGE ( 'NONE', *, *, #11352, .T. ) ;
#84840=VERTEX_POINT ( 'NONE', #83462 ) ;
#84841=B_SPLINE_CURVE_WITH_KNOTS ( 'NONE', 3,
 ( #7720, #950, #35180, #62637, #31524, #16235, #86945, #79719, #44571, #4035 ),
 .UNSPECIFIED., .F., .F.,
 ( 4, 2, 2, 2, 4 ),
 ( 0.0007817246336856291692, 0.0009771112958940103739, 0.001172497958102391470, 0.001367884620310772566, 0.001563271282519153879 ),
 .UNSPECIFIED. ) ;
#84842=CARTESIAN_POINT ( 'NONE',  ( 15.23076923076911093, -11.48612834414049644, 32.76840700105863391 ) ) ;
#84843=FACE_OUTER_BOUND ( 'NONE', #70698, .T. ) ;
#84844=CARTESIAN_POINT ( 'NONE',  ( 11.78840705680968171, -10.05730279482229683, 34.04704008940765902 ) ) ;
#84845=CARTESIAN_POINT ( 'NONE',  ( 6.249945409378045547, -12.68172785388650681, 30.59649109432439573 ) ) ;
#84846=VERTEX_POINT ( 'NONE', #27611 ) ;
#84847=CARTESIAN_POINT ( 'NONE',  ( -16.15384615384615330, -13.75783147151868846, 33.36296068462461051 ) ) ;
#84848=CARTESIAN_POINT ( 'NONE',  ( 9.692307692307695177, -2.499999999999998668, 29.75000000000001421 ) ) ;
#84849=CARTESIAN_POINT ( 'NONE',  ( 8.992242120843618736, -4.187068189119697692, 33.49521262558774026 ) ) ;
#84850=ORIENTED_EDGE ( 'NONE', *, *, #4646, .F. ) ;
#84851=AXIS2_PLACEMENT_3D ( 'NONE', #73471, #24365, #17633 ) ;
#84852=CARTESIAN_POINT ( 'NONE',  ( 16.15384615384615330, -9.905515769479276145, 34.41647553114623292 ) ) ;
#84853=VERTEX_POINT ( 'NONE', #13655 ) ;
#84854=B_SPLINE_CURVE_WITH_KNOTS ( 'NONE', 3,
 ( #7507, #61994, #6615, #81841, #34083, #76399, #13811, #42185, #55237, #20131 ),
 .UNSPECIFIED., .F., .F.,
 ( 4, 2, 2, 2, 4 ),
 ( 0.0007817359430256365111, 0.0009771253907250043464, 0.001172514838424372399, 0.001367904286123740234, 0.001563293733823107852 ),
 .UNSPECIFIED. ) ;
#84855=CARTESIAN_POINT ( 'NONE',  ( -9.692307692307691624, -12.10708131394839349, 31.69288490824020244 ) ) ;
#84856=CARTESIAN_POINT ( 'NONE',  ( -16.82686865700962642, -3.435999193479609026, 33.07426656108011542 ) ) ;
#84857=CARTESIAN_POINT ( 'NONE',  ( -7.976844449264150150, -2.494641256782728966, 31.33461815524612959 ) ) ;
#84858=CARTESIAN_POINT ( 'NONE',  ( -14.08491276642389600, -10.11255958852956027, 34.01340905677048454 ) ) ;
#84859=CARTESIAN_POINT ( 'NONE',  ( 18.22277966897806678, -8.540255544307068902, 34.89611431652622286 ) ) ;
#84860=VECTOR ( 'NONE', #44754, 1000.000000000000114 ) ;
#84861=ORIENTED_EDGE ( 'NONE', *, *, #81290, .T. ) ;
#84862=VECTOR ( 'NONE', #38979, 999.9999999999998863 ) ;
#84863=ORIENTED_EDGE ( 'NONE', *, *, #71127, .F. ) ;
#84864=EDGE_LOOP ( 'NONE', ( #55316, #29527, #45043, #18054 ) ) ;
#84865=CARTESIAN_POINT ( 'NONE',  ( -1.254089682851817988, -3.285477652293412820, 32.44071101563363158 ) ) ;
#84867=CARTESIAN_POINT ( 'NONE',  ( -12.39628332202562255, -12.51329471203373700, 31.30864560766537963 ) ) ;
#84868=DIRECTION ( 'NONE',  ( -0.000000000000000000, -0.6427876096865404731, -0.7660444431189770143 ) ) ;
#84870=FACE_OUTER_BOUND ( 'NONE', #40446, .T. ) ;
#84871=CARTESIAN_POINT ( 'NONE',  ( 5.207714884747862705, -9.804649428959608670, 34.18742332936588468 ) ) ;
#84872=ORIENTED_EDGE ( 'NONE', *, *, #12518, .T. ) ;
#84874=ORIENTED_EDGE ( 'NONE', *, *, #6426, .T. ) ;
#84877=ORIENTED_EDGE ( 'NONE', *, *, #315, .T. ) ;
#84878=CARTESIAN_POINT ( 'NONE',  ( 16.15384615384615330, -2.517432740324522911, 35.29906147534542527 ) ) ;
#84879=CARTESIAN_POINT ( 'NONE',  ( 16.15384615384615330, -4.945431358278436385, 36.03766855953609394 ) ) ;
#84880=CARTESIAN_POINT ( 'NONE',  ( 8.992193672792254233, -7.369474270740069777, 34.74850911626239736 ) ) ;
#84881=CARTESIAN_POINT ( 'NONE',  ( 13.63456090296352841, -8.433404298154334455, 34.66254593164985920 ) ) ;
#84882=EDGE_LOOP ( 'NONE', ( #49826, #15914, #64475, #50780 ) ) ;
#84883=EDGE_CURVE ( 'NONE', #42856, #49110, #33923, .T. ) ;
#84884=AXIS2_PLACEMENT_3D ( 'NONE', #78250, #30075, #56217 ) ;
#84885=EDGE_LOOP ( 'NONE', ( #75735, #84352, #12513, #1299 ) ) ;
#84886=CARTESIAN_POINT ( 'NONE',  ( 13.45068271796546178, -10.67929555188718282, 33.92786785259544757 ) ) ;
#84887=ORIENTED_EDGE ( 'NONE', *, *, #42085, .T. ) ;
#84888=FACE_BOUND ( 'NONE', #68603, .T. ) ;
#84889=DIRECTION ( 'NONE',  ( -0.000000000000000000, -0.5000000000000009992, -0.8660254037844380415 ) ) ;
#84890=CARTESIAN_POINT ( 'NONE',  ( -4.153846153846152411, -9.819645486525091727, 36.12317359536749706 ) ) ;
#84891=ORIENTED_EDGE ( 'NONE', *, *, #23600, .T. ) ;
#84893=CARTESIAN_POINT ( 'NONE',  ( 4.826946332874483936, -8.347322224742351082, 34.93158281831414769 ) ) ;
#84894=CARTESIAN_POINT ( 'NONE',  ( 1.161688425708536920, -3.395401636524185474, 33.02366814457250399 ) ) ;
#84896=CARTESIAN_POINT ( 'NONE',  ( 4.403900465484466231, -3.136992222400443175, 32.19305428654138979 ) ) ;
#84897=B_SPLINE_CURVE_WITH_KNOTS ( 'NONE', 3,
 ( #54537, #74832, #13122, #32061, #87029, #67182, #11797, #32497, #40602, #54093 ),
 .UNSPECIFIED., .F., .F.,
 ( 4, 2, 2, 2, 4 ),
 ( 0.0007817246256747434861, 0.0009771112852218861652, 0.001172497944769028844, 0.001367884604316171740, 0.001563271263863314419 ),
 .UNSPECIFIED. ) ;
#84898=CARTESIAN_POINT ( 'NONE',  ( 8.096099255531887806, -11.56426240980093745, 33.07394671870546432 ) ) ;
#84899=CARTESIAN_POINT ( 'NONE',  ( -9.692307692307691624, -2.708943851104267164, 35.45975837776705220 ) ) ;
#84900=CARTESIAN_POINT ( 'NONE',  ( 23.00000000000000000, -7.500000000000000000, 29.75000000000000355 ) ) ;
#84901=CARTESIAN_POINT ( 'NONE',  ( -6.249976730942353065, -5.728515186090277211, 34.42611988154120439 ) ) ;
#84902=B_SPLINE_CURVE_WITH_KNOTS ( 'NONE', 3,
 ( #88283, #38734, #12598, #46380, #72960, #40086, #26107, #53572, #65745, #66196 ),
 .UNSPECIFIED., .F., .F.,
 ( 4, 2, 2, 2, 4 ),
 ( 0.0007817246256747473893, 0.0009771112852218905021, 0.001172497944769033615, 0.001367884604316176944, 0.001563271263863320057 ),
 .UNSPECIFIED. ) ;
#84903=CARTESIAN_POINT ( 'NONE',  ( 16.08776377448601735, -10.67929555188718460, 33.92786785259543336 ) ) ;
#84904=DIRECTION ( 'NONE',  ( 0.000000000000000000, 0.9848077530122072432, 0.1736481776669354937 ) ) ;
#84905=ADVANCED_FACE ( 'NONE', ( #61834 ), #49217, .F. ) ;
#84906=FACE_BOUND ( 'NONE', #26627, .T. ) ;
#84908=CARTESIAN_POINT ( 'NONE',  ( 11.66898724022510159, -4.459921816937791661, 33.71989282347011851 ) ) ;
#84909=CARTESIAN_POINT ( 'NONE',  ( 12.46153846153846168, -5.415277668671390821, 36.20867863119892149 ) ) ;
#84911=CARTESIAN_POINT ( 'NONE',  ( 4.153846153846154188, -2.249999999999998668, 29.75000000000001776 ) ) ;
#84912=EDGE_CURVE ( 'NONE', #29932, #57265, #14789, .T. ) ;
#84915=ORIENTED_EDGE ( 'NONE', *, *, #3994, .T. ) ;
#84916=CARTESIAN_POINT ( 'NONE',  ( -3.903900744468109973, -5.766571408460172243, 34.70601412856602508 ) ) ;
#84917=ORIENTED_EDGE ( 'NONE', *, *, #29287, .T. ) ;
#84918=VECTOR ( 'NONE', #37904, 1000.000000000000114 ) ;
#84919=CARTESIAN_POINT ( 'NONE',  ( -9.942284423250045577, -5.728515186090277211, 34.42611988154120439 ) ) ;
#84921=VERTEX_POINT ( 'NONE', #69929 ) ;
#84922=EDGE_CURVE ( 'NONE', #10416, #40235, #20853, .T. ) ;
#84923=CARTESIAN_POINT ( 'NONE',  ( 13.38461538461538680, -3.886160181151819604, 36.00935417666054406 ) ) ;
#84924=ORIENTED_EDGE ( 'NONE', *, *, #62029, .T. ) ;
#84925=CARTESIAN_POINT ( 'NONE',  ( -6.250023237292964495, -11.86270091957321249, 32.19358267280087915 ) ) ;
#84927=CARTESIAN_POINT ( 'NONE',  ( -8.769230769230890843, -10.90142922262034020, 33.41473453929536674 ) ) ;
#84928=VECTOR ( 'NONE', #20117, 1000.000000000000000 ) ;
#84929=CARTESIAN_POINT ( 'NONE',  ( 7.173022332454967120, -10.18230066228895758, 34.26354781536631577 ) ) ;
#84930=CARTESIAN_POINT ( 'NONE',  ( -5.076923076923075762, -2.833524468853757305, 32.15551576947925838 ) ) ;
#84931=CARTESIAN_POINT ( 'NONE',  ( -17.77425180499407276, -2.249999999999999556, 29.62260770777999497 ) ) ;
#84932=CARTESIAN_POINT ( 'NONE',  ( 15.48076923076916955, -7.565270445406050648, 34.75000000000000000 ) ) ;
#84933=CARTESIAN_POINT ( 'NONE',  ( -14.30769230769230660, -3.322132147404559976, 32.92929555188717927 ) ) ;
#84936=CARTESIAN_POINT ( 'NONE',  ( -11.40793610022789828, -2.647132371071621471, 31.75357179365171589 ) ) ;
#84937=CARTESIAN_POINT ( 'NONE',  ( -14.98071491913091791, -2.564540009722895419, 30.55348353981670684 ) ) ;
#84938=CARTESIAN_POINT ( 'NONE',  ( -8.769230769230768274, -1.129524287112498415, 32.06866353760679544 ) ) ;
#84940=DIRECTION ( 'NONE',  ( -0.000000000000000000, 0.9848077530122085754, -0.1736481776669273613 ) ) ;
#84941=VERTEX_POINT ( 'NONE', #48322 ) ;
#84942=CARTESIAN_POINT ( 'NONE',  ( 4.153846153846154188, -2.249999999999998668, 29.75000000000001776 ) ) ;
#84943=CARTESIAN_POINT ( 'NONE',  ( 15.90384615384615330, -2.249999999999998668, 29.75000000000000355 ) ) ;
#84944=CARTESIAN_POINT ( 'NONE',  ( 1.134592160393929072, -5.765609946408405406, 34.70566812827424741 ) ) ;
#84945=CARTESIAN_POINT ( 'NONE',  ( 15.29591401148886121, -7.750023224968867197, 34.99404313364389907 ) ) ;
#84946=CARTESIAN_POINT ( 'NONE',  ( 14.98076923076923173, -7.433931650972300353, 34.75000000000000711 ) ) ;
#84947=CARTESIAN_POINT ( 'NONE',  ( -8.899922235898330314, -8.147922237126337563, 34.70805685702651999 ) ) ;
#84950=DIRECTION ( 'NONE',  ( -0.000000000000000000, 0.9396926207859093161, -0.3420201433256663259 ) ) ;
#84951=ORIENTED_EDGE ( 'NONE', *, *, #86903, .F. ) ;
#84952=ORIENTED_EDGE ( 'NONE', *, *, #36171, .F. ) ;
#84954=CARTESIAN_POINT ( 'NONE',  ( 16.37662569511456567, -2.847695495035524882, 31.58253572463339154 ) ) ;
#84955=CARTESIAN_POINT ( 'NONE',  ( -6.130147209438218781, -3.285722584762969856, 32.44110544564090759 ) ) ;
#84956=CARTESIAN_POINT ( 'NONE',  ( 10.83816428436268353, -10.23759521482555357, 34.22997729860117033 ) ) ;
#84958=VERTEX_POINT ( 'NONE', #1478 ) ;
#84959=CARTESIAN_POINT ( 'NONE',  ( -6.792285115252135519, -5.582136614379148654, 34.36778462344220486 ) ) ;
#84960=VERTEX_POINT ( 'NONE', #56419 ) ;
#84961=ORIENTED_EDGE ( 'NONE', *, *, #6162, .T. ) ;
#84962=AXIS2_PLACEMENT_3D ( 'NONE', #88898, #1032, #68599 ) ;
#84963=CARTESIAN_POINT ( 'NONE',  ( -15.23076923076922995, -12.10708131394839349, 31.69288490824020244 ) ) ;
#84964=DIRECTION ( 'NONE',  ( -0.000000000000000000, -0.7660444431189791237, -0.6427876096865379196 ) ) ;
#84965=CARTESIAN_POINT ( 'NONE',  ( -18.00000000000000000, -1.395656007487078076, 33.56301978189821256 ) ) ;
#84967=EDGE_CURVE ( 'NONE', #62470, #62488, #80355, .T. ) ;
#84969=CARTESIAN_POINT ( 'NONE',  ( 13.38461538461538680, -1.790695186598648903, 34.54067556320373455 ) ) ;
#84971=EDGE_CURVE ( 'NONE', #46562, #3642, #79224, .T. ) ;
#84974=AXIS2_PLACEMENT_3D ( 'NONE', #28833, #78323, #72455 ) ;
#84976=CARTESIAN_POINT ( 'NONE',  ( -14.30769230769230660, -2.292212530054420494, 30.41441678777542634 ) ) ;
#84977=ORIENTED_EDGE ( 'NONE', *, *, #34582, .F. ) ;
#84978=CARTESIAN_POINT ( 'NONE',  ( 1.607626736228236819, -9.086983370893047862, 34.49168942202179267 ) ) ;
#84980=FACE_OUTER_BOUND ( 'NONE', #12803, .T. ) ;
#84981=ORIENTED_EDGE ( 'NONE', *, *, #85130, .F. ) ;
#84982=EDGE_CURVE ( 'NONE', #75555, #15629, #56852, .T. ) ;
#84983=CARTESIAN_POINT ( 'NONE',  ( -7.846153846153844924, -1.790695186598648903, 34.54067556320373455 ) ) ;
#84984=ORIENTED_EDGE ( 'NONE', *, *, #3225, .F. ) ;
#84985=FACE_BOUND ( 'NONE', #70643, .T. ) ;
#84986=CARTESIAN_POINT ( 'NONE',  ( 15.23076923076923173, -4.786620604624113540, 33.94971097300155094 ) ) ;
#84987=CARTESIAN_POINT ( 'NONE',  ( -7.173100160369892286, -2.823816976329319495, 31.52131813110795733 ) ) ;
#84988=CARTESIAN_POINT ( 'NONE',  ( -17.93474486048716088, -2.657715359629131857, 31.77849191805843532 ) ) ;
#84989=CARTESIAN_POINT ( 'NONE',  ( 5.933917620639864055, -12.34228464037088280, 31.77849191805838558 ) ) ;
#84990=CARTESIAN_POINT ( 'NONE',  ( 14.98076923076921574, -2.249999999999998668, 29.81609741502487410 ) ) ;
#84992=DIRECTION ( 'NONE',  ( -0.000000000000000000, -0.7660444431189791237, -0.6427876096865379196 ) ) ;
#84993=CARTESIAN_POINT ( 'NONE',  ( -12.46153846153846168, -7.500000000000001776, 35.04278698407183867 ) ) ;
#84995=CARTESIAN_POINT ( 'NONE',  ( -11.28840722682322628, -12.17597550085003633, 31.52189283813461884 ) ) ;
#84996=ADVANCED_FACE ( 'NONE', ( #50534 ), #50092, .F. ) ;
#84997=CARTESIAN_POINT ( 'NONE',  ( 4.853996118016224770, -4.026226216239095379, 33.68668979543632958 ) ) ;
#84998=B_SPLINE_CURVE_WITH_KNOTS ( 'NONE', 3,
 ( #29646, #29214, #84159, #9374, #36833, #37719, #84600, #22872, #57545, #50334 ),
 .UNSPECIFIED., .F., .F.,
 ( 4, 2, 2, 2, 4 ),
 ( 0.0007817359430256307648, 0.0009771253907249971907, 0.001172514838424363725, 0.001367904286123730259, 0.001563293733823096577 ),
 .UNSPECIFIED. ) ;
#85000=CARTESIAN_POINT ( 'NONE',  ( -17.07692307692307665, -2.249999999999998668, 29.50000000000001421 ) ) ;
#85001=VECTOR ( 'NONE', #34536, 1000.000000000000227 ) ;
#85002=CARTESIAN_POINT ( 'NONE',  ( 18.00000000000000000, -1.215029322943914858, 32.30358669280327177 ) ) ;
#85003=CARTESIAN_POINT ( 'NONE',  ( 16.08857615328984281, -6.835583212224500826, 34.95778746994557906 ) ) ;
#85004=CYLINDRICAL_SURFACE ( 'NONE', #34633, 0.2499999999999986955 ) ;
#85005=CARTESIAN_POINT ( 'NONE',  ( -10.39260494640654819, -3.020022701398813236, 32.48759521482552515 ) ) ;
#85007=FACE_BOUND ( 'NONE', #60478, .T. ) ;
#85008=CARTESIAN_POINT ( 'NONE',  ( 13.38461538461526601, -12.27809138561165270, 31.22303859784587132 ) ) ;
#85009=CARTESIAN_POINT ( 'NONE',  ( 17.93391762063986050, -10.67929555188718460, 33.92786785259543336 ) ) ;
#85011=CARTESIAN_POINT ( 'NONE',  ( -7.715363405186896451, -12.62708834333097663, 30.88030960425257021 ) ) ;
#85012=CARTESIAN_POINT ( 'NONE',  ( 7.623288423950207893, -2.501496062324912284, 29.88072118266895671 ) ) ;
#85014=CARTESIAN_POINT ( 'NONE',  ( -14.30769230769230660, -1.242168528481310874, 33.36296068462461051 ) ) ;
#85017=FACE_OUTER_BOUND ( 'NONE', #2430, .T. ) ;
#85018=EDGE_CURVE ( 'NONE', #67601, #37942, #87348, .T. ) ;
#85020=CARTESIAN_POINT ( 'NONE',  ( -0.6850233861027922311, -3.562934362175799841, 33.22335522853832401 ) ) ;
#85021=CARTESIAN_POINT ( 'NONE',  ( 16.82689985270161870, -8.475808217655753651, 34.90892951860618609 ) ) ;
#85022=DIRECTION ( 'NONE',  ( -0.000000000000000000, 0.9396926207859093161, -0.3420201433256663259 ) ) ;
#85024=CARTESIAN_POINT ( 'NONE',  ( -11.40841410321108640, -7.723484941389743952, 34.99544897038808955 ) ) ;
#85025=FACE_OUTER_BOUND ( 'NONE', #77552, .T. ) ;
#85026=CARTESIAN_POINT ( 'NONE',  ( 11.47313862296936549, -7.749976743299138882, 34.99404534957040624 ) ) ;
#85027=CARTESIAN_POINT ( 'NONE',  ( 17.77651507543566822, -8.539481045369598178, 34.89627647299170832 ) ) ;
#85028=CARTESIAN_POINT ( 'NONE',  ( -10.61538461538461320, -1.117168528481311540, 33.14645433367849847 ) ) ;
#85029=CARTESIAN_POINT ( 'NONE',  ( -15.23076923076922995, -1.790695186598648903, 34.54067556320373455 ) ) ;
#85030=CYLINDRICAL_SURFACE ( 'NONE', #62083, 0.2499999999999973355 ) ;
#85031=B_SPLINE_CURVE_WITH_KNOTS ( 'NONE', 3,
 ( #66969, #60198, #32729, #87699, #17281, #24029, #86654, #79437, #31694, #16394 ),
 .UNSPECIFIED., .F., .F.,
 ( 4, 2, 2, 2, 4 ),
 ( 0.000000000000000000, 0.0001954339857564098867, 0.0003908679715128197734, 0.0005863019572692296059, 0.0007817359430256395469 ),
 .UNSPECIFIED. ) ;
#85032=B_SPLINE_CURVE_WITH_KNOTS ( 'NONE', 3,
 ( #41233, #47530, #47974, #20511, #67373, #75025, #68258, #34024, #27269, #244 ),
 .UNSPECIFIED., .F., .F.,
 ( 4, 2, 2, 2, 4 ),
 ( 0.0007817359430256329332, 0.0009771253907249995759, 0.001172514838424366327, 0.001367904286123732861, 0.001563293733823099612 ),
 .UNSPECIFIED. ) ;
#85033=CARTESIAN_POINT ( 'NONE',  ( 15.23076923076923173, -9.584722331328613620, 36.20867863119891439 ) ) ;
#85034=ADVANCED_FACE ( 'NONE', ( #45888 ), #77577, .F. ) ;
#85036=B_SPLINE_CURVE_WITH_KNOTS ( 'NONE', 3,
 ( #16085, #56629, #21507, #36796, #35470, #84115, #48527, #36362, #14764, #21961 ),
 .UNSPECIFIED., .F., .F.,
 ( 4, 2, 2, 2, 4 ),
 ( 0.0007817246256747505334, 0.0009771112852218954894, 0.001172497944769040554, 0.001367884604316185618, 0.001563271263863330682 ),
 .UNSPECIFIED. ) ;
#85037=CARTESIAN_POINT ( 'NONE',  ( 15.23076923076910916, -11.67786785259630911, 32.92929555188603530 ) ) ;
#85040=AXIS2_PLACEMENT_3D ( 'NONE', #70247, #29713, #83777 ) ;
#85041=AXIS2_PLACEMENT_3D ( 'NONE', #42443, #1451, #49634 ) ;
#85042=CARTESIAN_POINT ( 'NONE',  ( 9.019230769230768274, -2.499999999999998668, 29.75000000000000355 ) ) ;
#85043=CARTESIAN_POINT ( 'NONE',  ( -16.85391023282967637, -5.582272713120730145, 34.63742843783360570 ) ) ;
#85045=EDGE_CURVE ( 'NONE', #76427, #44215, #3908, .T. ) ;
#85046=CARTESIAN_POINT ( 'NONE',  ( -18.24997673094235395, -9.148715823498378086, 34.47080413974185120 ) ) ;
#85047=LINE ( 'NONE', #56677, #55535 ) ;
#85048=ORIENTED_EDGE ( 'NONE', *, *, #22328, .F. ) ;
#85049=CARTESIAN_POINT ( 'NONE',  ( 6.792385456409363087, -3.062553014421049546, 32.05460306192773601 ) ) ;
#85050=CARTESIAN_POINT ( 'NONE',  ( -13.38461538461550582, -10.21337939537710326, 33.94971097300076224 ) ) ;
#85051=FACE_OUTER_BOUND ( 'NONE', #31343, .T. ) ;
#85052=VECTOR ( 'NONE', #71044, 1000.000000000000000 ) ;
#85053=CARTESIAN_POINT ( 'NONE',  ( -13.38461538461550582, -3.300289026999228881, 32.46337939537708905 ) ) ;
#85055=DIRECTION ( 'NONE',  ( -0.000000000000000000, -0.3420201433256694901, -0.9396926207859082059 ) ) ;
#85056=EDGE_CURVE ( 'NONE', #69076, #15420, #49063, .T. ) ;
#85057=CARTESIAN_POINT ( 'NONE',  ( -10.61538461538461320, -12.78798330534102767, 29.49999999999997868 ) ) ;
#85058=CARTESIAN_POINT ( 'NONE',  ( 15.10007862765892206, -9.929715669179220328, 34.40415004197138416 ) ) ;
#85059=ORIENTED_EDGE ( 'NONE', *, *, #22242, .T. ) ;
#85060=ORIENTED_EDGE ( 'NONE', *, *, #67277, .T. ) ;
#85061=EDGE_CURVE ( 'NONE', #66369, #17845, #67062, .T. ) ;
#85062=EDGE_LOOP ( 'NONE', ( #68902, #6747, #69268, #60096 ) ) ;
#85063=EDGE_CURVE ( 'NONE', #73584, #44052, #31739, .T. ) ;
#85064=CARTESIAN_POINT ( 'NONE',  ( -18.00000000000000000, -3.513871655860376197, 32.76840700105977788 ) ) ;
#85066=CARTESIAN_POINT ( 'NONE',  ( -3.164701897419154530, -8.164416787775445883, 34.95778746994558617 ) ) ;
#85067=EDGE_CURVE ( 'NONE', #18168, #49352, #15926, .T. ) ;
#85068=CARTESIAN_POINT ( 'NONE',  ( -10.48485891362105171, -3.285477652293413264, 32.44071101563363158 ) ) ;
#85070=VERTEX_POINT ( 'NONE', #26072 ) ;
#85071=ORIENTED_EDGE ( 'NONE', *, *, #27613, .T. ) ;
#85072=CARTESIAN_POINT ( 'NONE',  ( -2.057692307692243538, -7.434744860731434812, 35.00000000000000711 ) ) ;
#85074=AXIS2_PLACEMENT_3D ( 'NONE', #43807, #71269, #64073 ) ;
#85075=CARTESIAN_POINT ( 'NONE',  ( 9.942362003946010773, -12.41262288849542017, 30.68299917996395010 ) ) ;
#85076=CARTESIAN_POINT ( 'NONE',  ( -17.86947429823644029, -3.285477652293416817, 32.44071101563363158 ) ) ;
#85077=CARTESIAN_POINT ( 'NONE',  ( -8.703163435880695076, -12.62096338111211757, 30.90682066428152908 ) ) ;
#85078=ORIENTED_EDGE ( 'NONE', *, *, #58844, .F. ) ;
#85080=ORIENTED_EDGE ( 'NONE', *, *, #38422, .F. ) ;
#85081=CARTESIAN_POINT ( 'NONE',  ( 9.915320536401090123, -8.282913670948747864, 34.94150082978203642 ) ) ;
#85083=CARTESIAN_POINT ( 'NONE',  ( -5.934744428723974785, -8.613356846314928816, 34.62446782046653482 ) ) ;
#85084=CARTESIAN_POINT ( 'NONE',  ( -14.30769230769242739, -9.442884908241554243, 34.35708131394783038 ) ) ;
#85085=ORIENTED_EDGE ( 'NONE', *, *, #16386, .T. ) ;
#85086=CARTESIAN_POINT ( 'NONE',  ( 12.59206389977210705, -6.808710257144161559, 34.95449254468098843 ) ) ;
#85087=CARTESIAN_POINT ( 'NONE',  ( 8.769230769230647482, -6.879047030192662504, 34.71129190930017927 ) ) ;
#85088=CARTESIAN_POINT ( 'NONE',  ( 6.700149964170073247, -5.582147617184174848, 34.63737895849758530 ) ) ;
#85089=FACE_BOUND ( 'NONE', #61120, .T. ) ;
#85091=CARTESIAN_POINT ( 'NONE',  ( -6.792286482109971324, -9.084667340241226796, 34.75534355489798344 ) ) ;
#85093=DIRECTION ( 'NONE',  ( -0.000000000000000000, 0.6427876096865404731, -0.7660444431189771253 ) ) ;
#85094=CARTESIAN_POINT ( 'NONE',  ( -3.230769230769229949, -3.886160181151819604, 36.00935417666054406 ) ) ;
#85095=CARTESIAN_POINT ( 'NONE',  ( -15.93083330975275658, -2.889357225399416418, 32.26129605718031002 ) ) ;
#85096=CARTESIAN_POINT ( 'NONE',  ( 11.28843830116857383, -11.37209801155882793, 32.91403422569033665 ) ) ;
#85097=FACE_OUTER_BOUND ( 'NONE', #87453, .T. ) ;
#85098=ORIENTED_EDGE ( 'NONE', *, *, #52947, .T. ) ;
#85099=CARTESIAN_POINT ( 'NONE',  ( 14.55769230769374367, -7.500000000000155431, 34.75000000000007105 ) ) ;
#85100=ORIENTED_EDGE ( 'NONE', *, *, #85615, .T. ) ;
#85101=VERTEX_POINT ( 'NONE', #6253 ) ;
#85102=CARTESIAN_POINT ( 'NONE',  ( 14.30769230769218758, -3.835265460704628371, 33.15142922262033665 ) ) ;
#85103=CARTESIAN_POINT ( 'NONE',  ( 15.10007862765892206, -2.845849958028613624, 32.17971566917920967 ) ) ;
#85104=B_SPLINE_CURVE_WITH_KNOTS ( 'NONE', 3,
 ( #31944, #59408, #38692, #23823, #24733, #58497, #23391, #52194, #16636, #44097 ),
 .UNSPECIFIED., .F., .F.,
 ( 4, 2, 2, 2, 4 ),
 ( 0.0007817246256747476061, 0.0009771112852218896347, 0.001172497944769031880, 0.001367884604316173909, 0.001563271263863315937 ),
 .UNSPECIFIED. ) ;
#85106=CARTESIAN_POINT ( 'NONE',  ( 14.55763771707034948, -4.176053281294518804, 33.81426240980091791 ) ) ;
#85107=CARTESIAN_POINT ( 'NONE',  ( 1.254468175177166689, -6.852621066184267029, 34.70813303252209181 ) ) ;
#85108=CARTESIAN_POINT ( 'NONE',  ( 1.161689167099238640, -11.76352882383564769, 32.36236540154569497 ) ) ;
#85109=ORIENTED_EDGE ( 'NONE', *, *, #82842, .F. ) ;
#85111=EDGE_CURVE ( 'NONE', #41186, #62418, #14611, .T. ) ;
#85112=CARTESIAN_POINT ( 'NONE',  ( -15.10024352900566846, -10.19071101563364756, 33.96452234770658407 ) ) ;
#85113=CARTESIAN_POINT ( 'NONE',  ( 10.61538461538449418, -8.656820664282941280, 34.87096338111179961 ) ) ;
#85114=DIRECTION ( 'NONE',  ( 0.000000000000000000, 0.7660444431189807890, 0.6427876096865361433 ) ) ;
#85115=CARTESIAN_POINT ( 'NONE',  ( 13.63456079399342791, -5.766571408460171355, 34.70601412856602508 ) ) ;
#85117=ORIENTED_EDGE ( 'NONE', *, *, #55943, .T. ) ;
#85118=EDGE_CURVE ( 'NONE', #46284, #23459, #20034, .T. ) ;
#85119=ORIENTED_EDGE ( 'NONE', *, *, #63653, .F. ) ;
#85122=VERTEX_POINT ( 'NONE', #41359 ) ;
#85123=CARTESIAN_POINT ( 'NONE',  ( 17.14299041027315340, -3.937682226553329556, 33.60647404775216529 ) ) ;
#85124=CARTESIAN_POINT ( 'NONE',  ( 10.74591031714818357, -2.619367082507849442, 30.83698974864643461 ) ) ;
#85125=CARTESIAN_POINT ( 'NONE',  ( 14.55774661933062575, -2.779044189368095719, 31.39831045268885745 ) ) ;
#85126=CARTESIAN_POINT ( 'NONE',  ( 6.000000000000317080, -2.255955759149395501, 30.00000000000324363 ) ) ;
#85130=EDGE_CURVE ( 'NONE', #49988, #74119, #81028, .T. ) ;
#85132=DIRECTION ( 'NONE',  ( -0.000000000000000000, -0.9848077530122085754, -0.1736481776669273613 ) ) ;
#85133=EDGE_LOOP ( 'NONE', ( #30782, #21940 ) ) ;
#85135=CARTESIAN_POINT ( 'NONE',  ( -9.915233909823841785, -12.15238873228292071, 31.58232369045353849 ) ) ;
#85136=CARTESIAN_POINT ( 'NONE',  ( -18.00000000000000000, -11.69971097300155449, 32.46337939537587403 ) ) ;
#85137=CARTESIAN_POINT ( 'NONE',  ( 6.673100179028331524, -3.436278759898155677, 33.07459398097509506 ) ) ;
#85138=FACE_OUTER_BOUND ( 'NONE', #14747, .T. ) ;
#85140=VECTOR ( 'NONE', #51892, 1000.000000000000114 ) ;
#85141=EDGE_CURVE ( 'NONE', #53125, #18436, #40918, .T. ) ;
#85143=ORIENTED_EDGE ( 'NONE', *, *, #26654, .T. ) ;
#85144=CARTESIAN_POINT ( 'NONE',  ( -12.21153846153702638, -7.500000000000155431, 34.75000000000007105 ) ) ;
#85145=FACE_OUTER_BOUND ( 'NONE', #55712, .T. ) ;
#85147=CARTESIAN_POINT ( 'NONE',  ( 4.403846153847572609, -7.500000000000154543, 35.00000000000007105 ) ) ;
#85148=CARTESIAN_POINT ( 'NONE',  ( 2.373759641042384683, -11.91647553114624358, 32.58852847137148245 ) ) ;
#85149=VERTEX_POINT ( 'NONE', #53531 ) ;
#85152=ORIENTED_EDGE ( 'NONE', *, *, #70719, .F. ) ;
#85153=CARTESIAN_POINT ( 'NONE',  ( 6.700149964170072359, -6.459968553980839800, 34.89616026154728701 ) ) ;
#85154=ORIENTED_EDGE ( 'NONE', *, *, #61553, .F. ) ;
#85157=DIRECTION ( 'NONE',  ( -0.000000000000000000, 1.000000000000000000, 3.491481338843133355E-15 ) ) ;
#85158=CARTESIAN_POINT ( 'NONE',  ( -12.46153846153858424, -11.06231777344772027, 33.60647404775119895 ) ) ;
#85159=VERTEX_POINT ( 'NONE', #88685 ) ;
#85160=CARTESIAN_POINT ( 'NONE',  ( -9.019230769230784261, -2.249999999999999556, 29.81609741502488120 ) ) ;
#85161=ADVANCED_FACE ( 'NONE', ( #6680 ), #378, .F. ) ;
#85162=VECTOR ( 'NONE', #65710, 1000.000000000000227 ) ;
#85163=ORIENTED_EDGE ( 'NONE', *, *, #11310, .F. ) ;
#85164=AXIS2_PLACEMENT_3D ( 'NONE', #58128, #37868, #4978 ) ;
#85166=CARTESIAN_POINT ( 'NONE',  ( 4.946775107191380805, -5.915902021225892149, 34.75552854090298638 ) ) ;
#85167=EDGE_CURVE ( 'NONE', #65648, #30667, #87803, .T. ) ;
#85168=B_SPLINE_CURVE_WITH_KNOTS ( 'NONE', 3,
 ( #57751, #4586, #45563, #44212, #58181, #64483, #30282, #71251, #52316, #79807 ),
 .UNSPECIFIED., .F., .F.,
 ( 4, 2, 2, 2, 4 ),
 ( 0.0007817246256747474977, 0.0009771112852218909357, 0.001172497944769034482, 0.001367884604316178029, 0.001563271263863321575 ),
 .UNSPECIFIED. ) ;
#85169=EDGE_LOOP ( 'NONE', ( #51601, #4079, #34307, #81757 ) ) ;
#85170=CARTESIAN_POINT ( 'NONE',  ( 8.769230769230768274, -4.661471528628507777, 34.16647553114623292 ) ) ;
#85171=CARTESIAN_POINT ( 'NONE',  ( -17.07692307692307665, -2.721908614388771852, 31.22303859784724978 ) ) ;
#85174=ADVANCED_FACE ( 'NONE', ( #70600 ), #56641, .F. ) ;
#85175=CARTESIAN_POINT ( 'NONE',  ( 1.253924781505079356, -6.369640206132550553, 34.87707690430378449 ) ) ;
#85177=ORIENTED_EDGE ( 'NONE', *, *, #12571, .F. ) ;
#85178=ORIENTED_EDGE ( 'NONE', *, *, #55007, .T. ) ;
#85179=ADVANCED_FACE ( 'NONE', ( #29189 ), #77355, .F. ) ;
#85180=FACE_BOUND ( 'NONE', #23446, .T. ) ;
#85182=CARTESIAN_POINT ( 'NONE',  ( -4.853547591150658036, -2.251407671071270489, 29.88021292934942252 ) ) ;
#85183=CARTESIAN_POINT ( 'NONE',  ( 6.066067333350078528, -5.471508081941601098, 34.59228464037088457 ) ) ;
#85184=FACE_OUTER_BOUND ( 'NONE', #14235, .T. ) ;
#85185=EDGE_LOOP ( 'NONE', ( #26013, #28581 ) ) ;
#85186=EDGE_CURVE ( 'NONE', #72319, #530, #43630, .T. ) ;
#85188=ORIENTED_EDGE ( 'NONE', *, *, #45844, .F. ) ;
#85190=VERTEX_POINT ( 'NONE', #63838 ) ;
#85192=CARTESIAN_POINT ( 'NONE',  ( 15.90382291655318880, -10.05641848906368097, 34.04755513067966177 ) ) ;
#85193=EDGE_CURVE ( 'NONE', #33270, #85539, #64046, .T. ) ;
#85194=EDGE_CURVE ( 'NONE', #19723, #56760, #2780, .T. ) ;
#85195=CARTESIAN_POINT ( 'NONE',  ( 3.007843013253083786, -2.758268499246657068, 31.33685645148949561 ) ) ;
#85197=FACE_OUTER_BOUND ( 'NONE', #3555, .T. ) ;
#85199=FACE_BOUND ( 'NONE', #31020, .T. ) ;
#85200=ORIENTED_EDGE ( 'NONE', *, *, #24997, .F. ) ;
#85201=CYLINDRICAL_SURFACE ( 'NONE', #42852, 0.2499999999999973355 ) ;
#85202=CARTESIAN_POINT ( 'NONE',  ( 3.230769230769108269, -4.320704448113951379, 33.92786785259630022 ) ) ;
#85203=DIRECTION ( 'NONE',  ( -0.000000000000000000, -0.6427876096865404731, -0.7660444431189770143 ) ) ;
#85204=CARTESIAN_POINT ( 'NONE',  ( 11.78840705680968171, -8.433404298154334455, 34.66254593164985920 ) ) ;
#85205=ORIENTED_EDGE ( 'NONE', *, *, #71766, .T. ) ;
#85207=CARTESIAN_POINT ( 'NONE',  ( -2.057746789344164551, -9.272278438253398036, 34.42582936511637826 ) ) ;
#85208=ORIENTED_EDGE ( 'NONE', *, *, #12945, .F. ) ;
#85212=CARTESIAN_POINT ( 'NONE',  ( 6.923076923076924238, -6.435427911321262684, 35.78748833219616898 ) ) ;
#85214=CARTESIAN_POINT ( 'NONE',  ( -18.00000000000000000, -5.471508081941599322, 34.59228464037088457 ) ) ;
#85215=DIRECTION ( 'NONE',  ( 0.000000000000000000, 0.4999999999999985567, 0.8660254037844395958 ) ) ;
#85216=EDGE_LOOP ( 'NONE', ( #30484, #68917 ) ) ;
#85218=CARTESIAN_POINT ( 'NONE',  ( 17.93391762063986761, -3.322132147404559976, 32.92929555188719348 ) ) ;
#85219=CARTESIAN_POINT ( 'NONE',  ( 4.284371855609718338, -9.417988943895561960, 34.36773134775778260 ) ) ;
#85220=CARTESIAN_POINT ( 'NONE',  ( 10.83839596699746721, -11.76359900205217635, 32.36225158514719880 ) ) ;
#85221=ORIENTED_EDGE ( 'NONE', *, *, #65265, .T. ) ;
#85222=EDGE_LOOP ( 'NONE', ( #24552, #25021, #38751, #20921 ) ) ;
#85223=FACE_BOUND ( 'NONE', #43971, .T. ) ;
#85224=ADVANCED_FACE ( 'NONE', ( #49876 ), #70153, .F. ) ;
#85226=CARTESIAN_POINT ( 'NONE',  ( 17.86952329188353872, -7.276988635370451597, 34.74523720219453793 ) ) ;
#85227=CARTESIAN_POINT ( 'NONE',  ( -11.53846153846153655, -11.69971097300155272, 32.46337939537588113 ) ) ;
#85229=CARTESIAN_POINT ( 'NONE',  ( -16.40386937806761125, -11.56360843649121861, 33.07473185843129926 ) ) ;
#85230=CARTESIAN_POINT ( 'NONE',  ( 6.792385456409368416, -10.54014554554150607, 33.71984207302941883 ) ) ;
#85231=CARTESIAN_POINT ( 'NONE',  ( -9.915233909823841785, -3.105860786376062332, 32.13614157043599562 ) ) ;
#85232=CARTESIAN_POINT ( 'NONE',  ( 4.284371592079798674, -6.808710257144159783, 34.95449254468098843 ) ) ;
#85233=VERTEX_POINT ( 'NONE', #8017 ) ;
#85234=VECTOR ( 'NONE', #80864, 1000.000000000000000 ) ;
#85235=B_SPLINE_CURVE_WITH_KNOTS ( 'NONE', 3,
 ( #11773, #46437, #61266, #32039, #45545, #18085, #18972, #19854, #73025, #39251 ),
 .UNSPECIFIED., .F., .F.,
 ( 4, 2, 2, 2, 4 ),
 ( 0.000000000000000000, 0.0001954311564186860613, 0.0003908623128373721225, 0.0005862934692560581567, 0.0007817246256747442451 ),
 .UNSPECIFIED. ) ;
#85237=VERTEX_POINT ( 'NONE', #35484 ) ;
#85239=CARTESIAN_POINT ( 'NONE',  ( 13.38461538461526601, -12.27809138561165270, 31.22303859784587132 ) ) ;
#85240=ORIENTED_EDGE ( 'NONE', *, *, #23867, .F. ) ;
#85241=CYLINDRICAL_SURFACE ( 'NONE', #51153, 0.2499999999999986955 ) ;
#85242=CARTESIAN_POINT ( 'NONE',  ( -14.05769230769088729, -7.500000000000154543, 35.00000000000007105 ) ) ;
#85243=DIRECTION ( 'NONE',  ( -0.000000000000000000, -0.8660254037844397068, -0.4999999999999978906 ) ) ;
#85244=B_SPLINE_CURVE_WITH_KNOTS ( 'NONE', 3,
 ( #5515, #18138, #46044, #45597, #25333, #66316, #4620, #5064, #32528, #32093 ),
 .UNSPECIFIED., .F., .F.,
 ( 4, 2, 2, 2, 4 ),
 ( 0.0007817359430256361858, 0.0009771253907250041296, 0.001172514838424372182, 0.001367904286123740234, 0.001563293733823108286 ),
 .UNSPECIFIED. ) ;
#85245=CARTESIAN_POINT ( 'NONE',  ( 12.68431800280687050, -4.387253974876679230, 33.66317474335728832 ) ) ;
#85246=CARTESIAN_POINT ( 'NONE',  ( 14.30769230769231015, -10.67929555188718282, 33.92786785259544047 ) ) ;
#85247=CARTESIAN_POINT ( 'NONE',  ( 6.250000000000000888, -7.500000000000001776, 35.04278698407183867 ) ) ;
#85248=ADVANCED_FACE ( 'NONE', ( #35037 ), #810, .F. ) ;
#85250=ORIENTED_EDGE ( 'NONE', *, *, #62348, .F. ) ;
#85251=CARTESIAN_POINT ( 'NONE',  ( 13.51540582558233794, -12.62708834333097663, 30.88030960425257021 ) ) ;
#85252=FACE_OUTER_BOUND ( 'NONE', #82592, .T. ) ;
#85253=VERTEX_POINT ( 'NONE', #49445 ) ;
#85254=ORIENTED_EDGE ( 'NONE', *, *, #55524, .F. ) ;
#85255=CARTESIAN_POINT ( 'NONE',  ( -6.000000000000121680, -12.70778746994576025, 30.41441678777401236 ) ) ;
#85256=CARTESIAN_POINT ( 'NONE',  ( -7.623374177175779920, -5.827830569534417471, 34.72679350104403539 ) ) ;
#85257=CARTESIAN_POINT ( 'NONE',  ( 6.065255571276025215, -11.48612834413965977, 32.76840700105972815 ) ) ;
#85258=CARTESIAN_POINT ( 'NONE',  ( -18.00000000000000000, -4.786620604624112651, 33.94971097300155094 ) ) ;
#85259=CARTESIAN_POINT ( 'NONE',  ( 10.39245839786846837, -4.186968288167450147, 33.49512374952580274 ) ) ;
#85260=EDGE_CURVE ( 'NONE', #53938, #40578, #81309, .T. ) ;
#85261=CARTESIAN_POINT ( 'NONE',  ( -8.769230769230890843, -11.94971097300221174, 32.03036669348237098 ) ) ;
#85262=VECTOR ( 'NONE', #63847, 1000.000000000000000 ) ;
#85263=CYLINDRICAL_SURFACE ( 'NONE', #50797, 0.2499999999999994726 ) ;
#85264=VERTEX_POINT ( 'NONE', #57522 ) ;
#85266=DIRECTION ( 'NONE',  ( -0.000000000000000000, -0.9848077530122085754, -0.1736481776669273613 ) ) ;
#85267=CARTESIAN_POINT ( 'NONE',  ( -9.561515884482902905, -11.18335022499818621, 33.13157742990016885 ) ) ;
#85268=CARTESIAN_POINT ( 'NONE',  ( -2.307692307692305711, -2.249999999999998668, 29.75000000000001776 ) ) ;
#85270=CARTESIAN_POINT ( 'NONE',  ( 7.623226887246997485, -2.308479472611653094, 30.53278059502174457 ) ) ;
#85271=AXIS2_PLACEMENT_3D ( 'NONE', #47255, #82388, #6715 ) ;
#85272=ADVANCED_FACE ( 'NONE', ( #23289 ), #66043, .F. ) ;
#85273=B_SPLINE_CURVE_WITH_KNOTS ( 'NONE', 3,
 ( #69109, #47939, #20913, #7855, #68661, #62772, #6961, #28572, #29024, #82639 ),
 .UNSPECIFIED., .F., .F.,
 ( 4, 2, 2, 2, 4 ),
 ( 0.000000000000000000, 0.0001954311564186876876, 0.0003908623128373753751, 0.0005862934692560630356, 0.0007817246256747507503 ),
 .UNSPECIFIED. ) ;
#85274=ORIENTED_EDGE ( 'NONE', *, *, #77286, .F. ) ;
#85275=CARTESIAN_POINT ( 'NONE',  ( 8.835298102580845025, -2.833524468853757750, 32.15551576947925838 ) ) ;
#85277=CARTESIAN_POINT ( 'NONE',  ( 6.250054419913455561, -12.65882529074907126, 30.72640787790839312 ) ) ;
#85278=ORIENTED_EDGE ( 'NONE', *, *, #59632, .T. ) ;
#85279=EDGE_CURVE ( 'NONE', #24019, #82116, #35120, .T. ) ;
#85280=CARTESIAN_POINT ( 'NONE',  ( 12.68455130563185662, -10.77377354290276124, 33.85451476688484718 ) ) ;
#85282=CARTESIAN_POINT ( 'NONE',  ( 14.30769230769231015, -8.318370150425687726, 35.83090037661290239 ) ) ;
#85283=CARTESIAN_POINT ( 'NONE',  ( -12.23852710992561299, -10.61302985866383963, 33.66295027996417843 ) ) ;
#85284=EDGE_CURVE ( 'NONE', #61132, #46109, #16981, .T. ) ;
#85285=VERTEX_POINT ( 'NONE', #85444 ) ;
#85286=CARTESIAN_POINT ( 'NONE',  ( -1.161835843346973096, -3.755027918224367767, 33.06320215134714857 ) ) ;
#85288=CARTESIAN_POINT ( 'NONE',  ( 10.61538461538461675, -2.249999999999998668, 29.75000000000001776 ) ) ;
#85291=DIRECTION ( 'NONE',  ( 0.000000000000000000, 0.3420201433256641055, -0.9396926207859100932 ) ) ;
#85293=FACE_OUTER_BOUND ( 'NONE', #13200, .T. ) ;
#85294=EDGE_CURVE ( 'NONE', #19286, #74960, #83379, .T. ) ;
#85295=AXIS2_PLACEMENT_3D ( 'NONE', #35204, #27565, #49157 ) ;
#85296=EDGE_LOOP ( 'NONE', ( #73707, #78899 ) ) ;
#85297=EDGE_LOOP ( 'NONE', ( #66383, #31563 ) ) ;
#85298=EDGE_CURVE ( 'NONE', #49865, #76544, #72804, .T. ) ;
#85300=EDGE_CURVE ( 'NONE', #85765, #50871, #43737, .T. ) ;
#85301=VERTEX_POINT ( 'NONE', #3897 ) ;
#85302=CARTESIAN_POINT ( 'NONE',  ( -1.253823576790598304, -3.062576670634119758, 32.05464942895959979 ) ) ;
#85303=CARTESIAN_POINT ( 'NONE',  ( 15.90386940979756858, -5.643011162660950042, 34.66104346484419096 ) ) ;
#85304=CARTESIAN_POINT ( 'NONE',  ( 16.15384615384615330, -10.51840700105979565, 33.73612834413961536 ) ) ;
#85305=CARTESIAN_POINT ( 'NONE',  ( -12.46153846153846168, -3.322132147404559976, 32.92929555188717927 ) ) ;
#85306=CARTESIAN_POINT ( 'NONE',  ( -13.13456107297706943, -5.728107161865378494, 34.42597550085002922 ) ) ;
#85307=CARTESIAN_POINT ( 'NONE',  ( -7.846153846153844924, -11.91647553114624181, 32.58852847137148245 ) ) ;
#85308=CARTESIAN_POINT ( 'NONE',  ( 6.000000000000001776, -11.69971097300155272, 32.46337939537588113 ) ) ;
#85309=CARTESIAN_POINT ( 'NONE',  ( -6.923076923076922462, -1.629998284177014645, 34.34916445242399163 ) ) ;
#85310=VERTEX_POINT ( 'NONE', #59294 ) ;
#85312=EDGE_LOOP ( 'NONE', ( #10624, #31723 ) ) ;
#85313=CARTESIAN_POINT ( 'NONE',  ( 0.3308478584281513979, -2.845849958028613624, 32.17971566917920967 ) ) ;
#85314=ORIENTED_EDGE ( 'NONE', *, *, #33706, .F. ) ;
#85315=AXIS2_PLACEMENT_3D ( 'NONE', #38856, #73077, #60445 ) ;
#85316=CYLINDRICAL_SURFACE ( 'NONE', #2847, 0.2500000000000009437 ) ;
#85317=CARTESIAN_POINT ( 'NONE',  ( 18.06519298829465825, -2.255955759149236073, 29.99999999999987921 ) ) ;
#85318=AXIS2_PLACEMENT_3D ( 'NONE', #76890, #2985, #42227 ) ;
#85319=CARTESIAN_POINT ( 'NONE',  ( 8.546404076751764833, -7.369208160676172348, 34.74850200257122879 ) ) ;
#85320=CARTESIAN_POINT ( 'NONE',  ( -11.40793610022789828, -9.503571793651731880, 34.60286762892837942 ) ) ;
#85321=ORIENTED_EDGE ( 'NONE', *, *, #71208, .F. ) ;
#85322=ORIENTED_EDGE ( 'NONE', *, *, #58703, .F. ) ;
#85323=CARTESIAN_POINT ( 'NONE',  ( -13.38461538461550582, -10.21337939537710326, 33.94971097300076224 ) ) ;
#85324=ORIENTED_EDGE ( 'NONE', *, *, #40372, .F. ) ;
#85325=FACE_BOUND ( 'NONE', #70412, .T. ) ;
#85326=B_SPLINE_CURVE_WITH_KNOTS ( 'NONE', 3,
 ( #47847, #20387, #49180, #8650, #83424, #69895, #8204, #62681, #21710, #82094 ),
 .UNSPECIFIED., .F., .F.,
 ( 4, 2, 2, 2, 4 ),
 ( 0.0007817359430256324996, 0.0009771253907249991422, 0.001172514838424365893, 0.001367904286123732428, 0.001563293733823099179 ),
 .UNSPECIFIED. ) ;
#85327=CARTESIAN_POINT ( 'NONE',  ( -6.130691466667557599, -8.999036380462719364, 34.52022231692819076 ) ) ;
#85328=CYLINDRICAL_SURFACE ( 'NONE', #75076, 0.2499999999999994726 ) ;
#85329=EDGE_LOOP ( 'NONE', ( #59927, #66013 ) ) ;
#85330=CARTESIAN_POINT ( 'NONE',  ( 16.21910172512217585, -11.48612834413965977, 32.76840700105972815 ) ) ;
#85331=CARTESIAN_POINT ( 'NONE',  ( 11.53846153846153832, -6.343179335718451384, 34.87096338111211935 ) ) ;
#85332=CARTESIAN_POINT ( 'NONE',  ( -4.153846153846152411, -8.120952969808772792, 34.71129190930000163 ) ) ;
#85333=ORIENTED_EDGE ( 'NONE', *, *, #9087, .T. ) ;
#85334=DIRECTION ( 'NONE',  ( -0.000000000000000000, -0.000000000000000000, -1.000000000000000000 ) ) ;
#85335=CARTESIAN_POINT ( 'NONE',  ( -17.07692307692307665, -2.538708090699994813, 30.37095296980875503 ) ) ;
#85336=ORIENTED_EDGE ( 'NONE', *, *, #16275, .F. ) ;
#85337=CARTESIAN_POINT ( 'NONE',  ( 7.912221179503922563, -11.35647404775217595, 33.31231777344666511 ) ) ;
#85338=CARTESIAN_POINT ( 'NONE',  ( -7.053224132515138578, -11.47017969459903952, 32.78971311882034456 ) ) ;
#85339=CARTESIAN_POINT ( 'NONE',  ( 3.230769230769231726, -4.098570777380720287, 33.41473453929634729 ) ) ;
#85340=CARTESIAN_POINT ( 'NONE',  ( 16.08857615328984281, -3.083524468853725775, 32.58852847137143272 ) ) ;
#85341=CARTESIAN_POINT ( 'NONE',  ( -10.48459280755982803, -5.582136614379148654, 34.36778462344220486 ) ) ;
#85342=DIRECTION ( 'NONE',  ( 0.000000000000000000, 0.6427876096865373645, -0.7660444431189797898 ) ) ;
#85343=CYLINDRICAL_SURFACE ( 'NONE', #30812, 5.000000000000000888 ) ;
#85344=CARTESIAN_POINT ( 'NONE',  ( 4.853996859406927378, -12.39988816332205701, 30.74660775122750778 ) ) ;
#85345=AXIS2_PLACEMENT_3D ( 'NONE', #55149, #48392, #74996 ) ;
#85346=CARTESIAN_POINT ( 'NONE',  ( 11.76142467272821257, -7.369474539155828730, 34.99858011523957657 ) ) ;
#85347=CARTESIAN_POINT ( 'NONE',  ( 1.449870955891410462, -11.48612834413965977, 32.76840700105972815 ) ) ;
#85348=DIRECTION ( 'NONE',  ( -0.000000000000000000, -0.000000000000000000, -1.000000000000000000 ) ) ;
#85349=CARTESIAN_POINT ( 'NONE',  ( -15.23076923076935074, -11.94971097300221174, 32.03036669348237098 ) ) ;
#85350=CARTESIAN_POINT ( 'NONE',  ( 13.63461538461680611, -7.500000000000154543, 35.00000000000007105 ) ) ;
#85356=AXIS2_PLACEMENT_3D ( 'NONE', #5552, #33023, #81216 ) ;
#85358=ORIENTED_EDGE ( 'NONE', *, *, #11177, .F. ) ;
#85359=CARTESIAN_POINT ( 'NONE',  ( -4.153846153846152411, -11.16473453929635440, 33.15142922261926373 ) ) ;
#85360=VERTEX_POINT ( 'NONE', #65597 ) ;
#85361=CARTESIAN_POINT ( 'NONE',  ( 5.999999999999878320, -11.06231777344772027, 33.60647404775119895 ) ) ;
#85363=DIRECTION ( 'NONE',  ( -0.000000000000000000, -0.8660254037844397068, -0.4999999999999978906 ) ) ;
#85364=DIRECTION ( 'NONE',  ( 0.000000000000000000, 0.8660254037844377084, -0.5000000000000015543 ) ) ;
#85365=CARTESIAN_POINT ( 'NONE',  ( 6.923076923076800782, -10.33852847137269571, 34.16647553114546554 ) ) ;
#85368=CARTESIAN_POINT ( 'NONE',  ( 11.40831432902332310, -2.882441371585227508, 31.66841991370172238 ) ) ;
#85369=CARTESIAN_POINT ( 'NONE',  ( -13.45069776397551742, -11.91647553114624181, 32.58852847137148245 ) ) ;
#85371=B_SPLINE_CURVE_WITH_KNOTS ( 'NONE', 3,
 ( #77769, #21494, #76894, #22822, #8437, #35012, #35460, #50280, #42231, #9326 ),
 .UNSPECIFIED., .F., .F.,
 ( 4, 2, 2, 2, 4 ),
 ( 0.000000000000000000, 0.0001954339857564054144, 0.0003908679715128108288, 0.0005863019572692162703, 0.0007817359430256216575 ),
 .UNSPECIFIED. ) ;
#85372=DIRECTION ( 'NONE',  ( 1.000000000000000000, 0.000000000000000000, 0.000000000000000000 ) ) ;
#85373=CARTESIAN_POINT ( 'NONE',  ( -15.10024352900566846, -2.619367082507849442, 30.83698974864643461 ) ) ;
#85374=CARTESIAN_POINT ( 'NONE',  ( 14.55763782604045176, -3.202959910592335646, 32.30730279482227019 ) ) ;
#85376=EDGE_CURVE ( 'NONE', #7293, #12053, #75864, .T. ) ;
#85377=ORIENTED_EDGE ( 'NONE', *, *, #45382, .F. ) ;
#85378=CARTESIAN_POINT ( 'NONE',  ( 14.37294787896833270, -5.219633306516380244, 34.19971097300157936 ) ) ;
#85380=CARTESIAN_POINT ( 'NONE',  ( 1.161688425708537142, -5.582147617184174848, 34.63737895849758530 ) ) ;
#85381=CARTESIAN_POINT ( 'NONE',  ( 5.207448778686639024, -2.882268652242224505, 31.66798894389554064 ) ) ;
#85382=CARTESIAN_POINT ( 'NONE',  ( 14.30769230769231015, -3.322132147404559976, 32.92929555188717927 ) ) ;
#85383=CARTESIAN_POINT ( 'NONE',  ( 9.442284455014730682, -11.37209801155882793, 32.91403422569033665 ) ) ;
#85384=VECTOR ( 'NONE', #47646, 1000.000000000000227 ) ;
#85385=EDGE_CURVE ( 'NONE', #88864, #88630, #55450, .T. ) ;
#85386=EDGE_LOOP ( 'NONE', ( #35679, #80868, #54168, #33659 ) ) ;
#85387=CARTESIAN_POINT ( 'NONE',  ( -6.923076923077044142, -10.21337939537710326, 33.94971097300076224 ) ) ;
#85388=ORIENTED_EDGE ( 'NONE', *, *, #83394, .F. ) ;
#85390=DIRECTION ( 'NONE',  ( 0.000000000000000000, 0.4999999999999960032, -0.8660254037844410391 ) ) ;
#85391=CARTESIAN_POINT ( 'NONE',  ( 5.299934428535925335, -11.76359900205217457, 32.36225158514719880 ) ) ;
#85392=CARTESIAN_POINT ( 'NONE',  ( 16.40379167219430201, -2.824170634883622633, 31.52227843825338738 ) ) ;
#85393=CARTESIAN_POINT ( 'NONE',  ( -13.38461538461550582, -9.442884908241554243, 34.35708131394783038 ) ) ;
#85394=CARTESIAN_POINT ( 'NONE',  ( 10.68145194873469173, -9.905515769479276145, 34.41647553114623292 ) ) ;
#85395=VERTEX_POINT ( 'NONE', #6578 ) ;
#85396=LINE ( 'NONE', #9733, #33466 ) ;
#85397=EDGE_LOOP ( 'NONE', ( #17812, #51949, #79072, #20284 ) ) ;
#85398=B_SPLINE_CURVE_WITH_KNOTS ( 'NONE', 3,
 ( #26371, #75442, #6103, #13737, #68679, #53837, #88537, #6979, #55160, #81325 ),
 .UNSPECIFIED., .F., .F.,
 ( 4, 2, 2, 2, 4 ),
 ( 0.0007817359430256365111, 0.0009771253907250045632, 0.001172514838424372399, 0.001367904286123740451, 0.001563293733823108503 ),
 .UNSPECIFIED. ) ;
#85401=ORIENTED_EDGE ( 'NONE', *, *, #10725, .T. ) ;
#85402=AXIS2_PLACEMENT_3D ( 'NONE', #58704, #17734, #3760 ) ;
#85403=CARTESIAN_POINT ( 'NONE',  ( 17.99999999999987566, -2.379036618888197729, 30.90682066428292885 ) ) ;
#85404=LINE ( 'NONE', #23687, #58915 ) ;
#85406=VECTOR ( 'NONE', #62433, 1000.000000000000000 ) ;
#85408=EDGE_CURVE ( 'NONE', #27810, #44478, #7216, .T. ) ;
#85409=CARTESIAN_POINT ( 'NONE',  ( -16.82697755857493149, -3.202959910592335202, 32.30730279482227019 ) ) ;
#85410=CARTESIAN_POINT ( 'NONE',  ( 18.00000000000000000, -1.509761064869970415, 31.06009739812519044 ) ) ;
#85411=ORIENTED_EDGE ( 'NONE', *, *, #59694, .T. ) ;
#85412=ORIENTED_EDGE ( 'NONE', *, *, #34476, .T. ) ;
#85414=ORIENTED_EDGE ( 'NONE', *, *, #34041, .F. ) ;
#85415=CARTESIAN_POINT ( 'NONE',  ( -5.777220458731589403, -3.236590943229499029, 32.36255958852954251 ) ) ;
#85417=DIRECTION ( 'NONE',  ( -0.000000000000000000, -0.1736481776669307198, -0.9848077530122080203 ) ) ;
#85418=DIRECTION ( 'NONE',  ( -1.000000000000000000, 0.000000000000000000, 0.000000000000000000 ) ) ;
#85419=CARTESIAN_POINT ( 'NONE',  ( 2.438482748659258625, -9.084667340241226796, 34.75534355489798344 ) ) ;
#85420=VERTEX_POINT ( 'NONE', #66951 ) ;
#85421=CARTESIAN_POINT ( 'NONE',  ( 5.076923076923391065, -2.255955759149395501, 30.00000000000324363 ) ) ;
#85422=ORIENTED_EDGE ( 'NONE', *, *, #70405, .T. ) ;
#85423=CARTESIAN_POINT ( 'NONE',  ( 6.000000000000001776, -9.058645607665452459, 34.76329471203371924 ) ) ;
#85424=CARTESIAN_POINT ( 'NONE',  ( 17.77651507543566112, -12.69144148231606017, 30.53333754910549303 ) ) ;
#85425=DIRECTION ( 'NONE',  ( -0.000000000000000000, 0.9396926207859093161, -0.3420201433256663259 ) ) ;
#85426=CARTESIAN_POINT ( 'NONE',  ( -6.857821351800898135, -12.46129190930001052, 30.37095296980870174 ) ) ;
#85427=CYLINDRICAL_SURFACE ( 'NONE', #87180, 0.2499999999999995559 ) ;
#85429=CARTESIAN_POINT ( 'NONE',  ( -0.3307480205715113697, -12.62708834333097663, 30.88030960425257021 ) ) ;
#85430=ORIENTED_EDGE ( 'NONE', *, *, #41539, .F. ) ;
#85431=B_SPLINE_CURVE_WITH_KNOTS ( 'NONE', 3,
 ( #53161, #80665, #5882, #88320, #18507, #26593, #32017, #45526, #47297, #18948 ),
 .UNSPECIFIED., .F., .F.,
 ( 4, 2, 2, 2, 4 ),
 ( 0.000000000000000000, 0.0001954339857564091278, 0.0003908679715128182556, 0.0005863019572692274375, 0.0007817359430256365111 ),
 .UNSPECIFIED. ) ;
#85432=CARTESIAN_POINT ( 'NONE',  ( -11.53846153846153655, -4.098570777380720287, 33.41473453929634729 ) ) ;
#85433=CARTESIAN_POINT ( 'NONE',  ( -17.07692307692307665, -1.242168528481310874, 33.36296068462461051 ) ) ;
#85434=ORIENTED_EDGE ( 'NONE', *, *, #24461, .F. ) ;
#85435=VECTOR ( 'NONE', #61267, 1000.000000000000000 ) ;
#85436=CARTESIAN_POINT ( 'NONE',  ( 11.53846153846141576, -12.16647553114689728, 32.15551576947799362 ) ) ;
#85438=CARTESIAN_POINT ( 'NONE',  ( -16.02332045208259359, -10.88167719472716399, 33.43325721877153711 ) ) ;
#85440=B_SPLINE_CURVE_WITH_KNOTS ( 'NONE', 3,
 ( #66079, #59775, #38620, #31418, #87273, #44918, #65190, #51662, #11600, #17464 ),
 .UNSPECIFIED., .F., .F.,
 ( 4, 2, 2, 2, 4 ),
 ( 0.000000000000000000, 0.0001954311564186863323, 0.0003908623128373726646, 0.0005862934692560590241, 0.0007817246256747453293 ),
 .UNSPECIFIED. ) ;
#85441=CARTESIAN_POINT ( 'NONE',  ( -13.31936024510254413, -11.67786785259547777, 32.92929555188713664 ) ) ;
#85442=FACE_OUTER_BOUND ( 'NONE', #43067, .T. ) ;
#85443=FACE_BOUND ( 'NONE', #51692, .T. ) ;
#85444=CARTESIAN_POINT ( 'NONE',  ( 5.999999999999878320, -3.643525952248796163, 33.31231777344771672 ) ) ;
#85445=DIRECTION ( 'NONE',  ( 0.000000000000000000, 1.000000000000000000, 0.000000000000000000 ) ) ;
#85446=CARTESIAN_POINT ( 'NONE',  ( -6.700297381808513641, -10.81320215134717344, 33.49497208177562868 ) ) ;
#85448=CARTESIAN_POINT ( 'NONE',  ( 0.4615384615384611200, -2.833524468853757305, 32.15551576947925838 ) ) ;
#85449=CARTESIAN_POINT ( 'NONE',  ( 1.384615384615386802, -2.833524468853757305, 32.15551576947925838 ) ) ;
#85450=CARTESIAN_POINT ( 'NONE',  ( 8.992242120843616959, -10.61302985866384141, 33.66295027996417843 ) ) ;
#85452=EDGE_LOOP ( 'NONE', ( #16635, #64255 ) ) ;
#85453=CARTESIAN_POINT ( 'NONE',  ( 0.4615384615384611200, -6.189225973068211317, 35.74407628777942847 ) ) ;
#85454=CARTESIAN_POINT ( 'NONE',  ( -4.403869391139119571, -3.202444869320336451, 32.30641848906366675 ) ) ;
#85455=CARTESIAN_POINT ( 'NONE',  ( 5.934729999443682402, -5.941354392334500467, 34.76329471203369792 ) ) ;
#85456=CARTESIAN_POINT ( 'NONE',  ( 16.94677510719138169, -8.630895178749536711, 34.87696386517710323 ) ) ;
#85457=CARTESIAN_POINT ( 'NONE',  ( 7.623227628637697428, -4.887634598454296153, 34.01352882383564946 ) ) ;
#85458=CARTESIAN_POINT ( 'NONE',  ( -17.07692307692319744, -8.656820664282941280, 34.87096338111179961 ) ) ;
#85461=CARTESIAN_POINT ( 'NONE',  ( -2.530619266599154482, -3.395401636524185474, 33.02366814457250399 ) ) ;
#85462=CARTESIAN_POINT ( 'NONE',  ( -2.057637887778853703, -6.523592122091589118, 34.90882529074906415 ) ) ;
#85463=CARTESIAN_POINT ( 'NONE',  ( 11.78846153846295763, -7.500000000000154543, 35.00000000000007105 ) ) ;
#85464=CARTESIAN_POINT ( 'NONE',  ( 17.99999999999987566, -8.656820664282941280, 34.87096338111179961 ) ) ;
#85465=CARTESIAN_POINT ( 'NONE',  ( 17.99999999999987566, -12.70778746994576025, 30.41441678777401236 ) ) ;
#85466=CARTESIAN_POINT ( 'NONE',  ( 10.83876055608279820, -2.501478030877322567, 29.88021232661721172 ) ) ;
#85468=DIRECTION ( 'NONE',  ( -0.000000000000000000, 0.7660444431189791237, -0.6427876096865379196 ) ) ;
#85469=CARTESIAN_POINT ( 'NONE',  ( 17.29970274590113632, -2.612705202774696200, 31.66806509827799943 ) ) ;
#85471=LINE ( 'NONE', #9376, #65756 ) ;
#85472=CYLINDRICAL_SURFACE ( 'NONE', #17268, 0.2500000000000002220 ) ;
#85474=AXIS2_PLACEMENT_3D ( 'NONE', #61126, #53930, #26910 ) ;
#85475=AXIS2_PLACEMENT_3D ( 'NONE', #59195, #53773, #47008 ) ;
#85476=EDGE_CURVE ( 'NONE', #84107, #20488, #32970, .T. ) ;
#85477=CARTESIAN_POINT ( 'NONE',  ( 6.923076923076924238, -4.661471528628507777, 34.16647553114623292 ) ) ;
#85478=CARTESIAN_POINT ( 'NONE',  ( 11.53846153846153832, -9.819645486525091727, 36.12317359536749706 ) ) ;
#85479=EDGE_LOOP ( 'NONE', ( #1810, #50714, #48064, #30580 ) ) ;
#85480=CARTESIAN_POINT ( 'NONE',  ( -18.06608341095587278, -8.973038597847269315, 34.52809138561120506 ) ) ;
#85481=CARTESIAN_POINT ( 'NONE',  ( -3.230769230769229949, -12.62096338111211580, 30.90682066428153263 ) ) ;
#85482=CARTESIAN_POINT ( 'NONE',  ( 4.087762742890272527, -5.557115091759785130, 34.35708131394839171 ) ) ;
#85483=VERTEX_POINT ( 'NONE', #47104 ) ;
#85484=CARTESIAN_POINT ( 'NONE',  ( 6.923076923076802558, -3.300289026999228881, 32.46337939537708905 ) ) ;
#85485=CYLINDRICAL_SURFACE ( 'NONE', #65607, 0.2499999999999995559 ) ;
#85486=EDGE_CURVE ( 'NONE', #78822, #31805, #59854, .T. ) ;
#85487=DIRECTION ( 'NONE',  ( -0.000000000000000000, -0.000000000000000000, -1.000000000000000000 ) ) ;
#85488=CARTESIAN_POINT ( 'NONE',  ( -13.45069879557126313, -3.050289026998445951, 32.03036669348365706 ) ) ;
#85489=ORIENTED_EDGE ( 'NONE', *, *, #22035, .F. ) ;
#85490=CARTESIAN_POINT ( 'NONE',  ( -11.78843826940389583, -4.236021600441997492, 33.53823185664189310 ) ) ;
#85491=CARTESIAN_POINT ( 'NONE',  ( -16.02305434602137169, -3.062576670634119758, 32.05464942895959979 ) ) ;
#85492=CYLINDRICAL_SURFACE ( 'NONE', #84452, 0.2500000000000008882 ) ;
#85493=EDGE_CURVE ( 'NONE', #20488, #57339, #19208, .T. ) ;
#85494=ORIENTED_EDGE ( 'NONE', *, *, #52329, .F. ) ;
#85495=VERTEX_POINT ( 'NONE', #12014 ) ;
#85496=B_SPLINE_CURVE_WITH_KNOTS ( 'NONE', 3,
 ( #18547, #65386, #78902, #85668, #3241, #86572, #24842, #17199, #52313, #25743 ),
 .UNSPECIFIED., .F., .F.,
 ( 4, 2, 2, 2, 4 ),
 ( 0.0007817246256747515092, 0.0009771112852218961399, 0.001172497944769040771, 0.001367884604316185401, 0.001563271263863330032 ),
 .UNSPECIFIED. ) ;
#85497=ORIENTED_EDGE ( 'NONE', *, *, #53146, .F. ) ;
#85498=EDGE_CURVE ( 'NONE', #38377, #29227, #76410, .T. ) ;
#85499=CARTESIAN_POINT ( 'NONE',  ( -5.142193077479396024, -9.528491918058357157, 34.59228464037090589 ) ) ;
#85500=CARTESIAN_POINT ( 'NONE',  ( -8.703975197954742171, -3.300289026998473041, 32.46337939537591666 ) ) ;
#85501=CARTESIAN_POINT ( 'NONE',  ( 11.53846153846141753, -10.90142922262034020, 33.41473453929536674 ) ) ;
#85502=VECTOR ( 'NONE', #68942, 1000.000000000000227 ) ;
#85503=CARTESIAN_POINT ( 'NONE',  ( 2.307692307692309264, -12.09954503811598769, 35.62045528018868623 ) ) ;
#85504=EDGE_CURVE ( 'NONE', #44924, #48096, #12543, .T. ) ;
#85506=ORIENTED_EDGE ( 'NONE', *, *, #40484, .T. ) ;
#85507=CARTESIAN_POINT ( 'NONE',  ( -1.319359813339359810, -5.219633306516380244, 34.19971097300157936 ) ) ;
#85508=EDGE_CURVE ( 'NONE', #63347, #87552, #28660, .T. ) ;
#85509=ORIENTED_EDGE ( 'NONE', *, *, #87272, .T. ) ;
#85510=CARTESIAN_POINT ( 'NONE',  ( -10.61538461538461320, -2.721908614388771852, 31.22303859784724978 ) ) ;
#85511=ADVANCED_FACE ( 'NONE', ( #15112 ), #28627, .F. ) ;
#85512=EDGE_CURVE ( 'NONE', #17756, #75262, #44742, .T. ) ;
#85513=CARTESIAN_POINT ( 'NONE',  ( 10.61538461538449596, -11.48612834414049644, 32.76840700105863391 ) ) ;
#85515=ORIENTED_EDGE ( 'NONE', *, *, #19569, .T. ) ;
#85516=EDGE_LOOP ( 'NONE', ( #33437, #1011, #21970, #60166 ) ) ;
#85517=CARTESIAN_POINT ( 'NONE',  ( -12.39547011053602432, -4.786620604624113540, 33.94971097300155805 ) ) ;
#85518=ORIENTED_EDGE ( 'NONE', *, *, #58401, .T. ) ;
#85519=CARTESIAN_POINT ( 'NONE',  ( -5.777220458731589403, -8.496831190052096971, 34.64984203495476578 ) ) ;
#85520=B_SPLINE_CURVE_WITH_KNOTS ( 'NONE', 3,
 ( #12355, #88047, #26308, #53776, #81262, #19548, #31286, #73166, #66405, #38493 ),
 .UNSPECIFIED., .F., .F.,
 ( 4, 2, 2, 2, 4 ),
 ( 0.000000000000000000, 0.0001954311564186860071, 0.0003908623128373720141, 0.0005862934692560580483, 0.0007817246256747440282 ),
 .UNSPECIFIED. ) ;
#85521=B_SPLINE_CURVE_WITH_KNOTS ( 'NONE', 3,
 ( #88646, #7087, #13399, #81874, #39567, #67023, #34114, #32789, #26035, #61580 ),
 .UNSPECIFIED., .F., .F.,
 ( 4, 2, 2, 2, 4 ),
 ( 0.0007817246256747503166, 0.0009771112852218946220, 0.001172497944769039036, 0.001367884604316183233, 0.001563271263863327647 ),
 .UNSPECIFIED. ) ;
#85522=CARTESIAN_POINT ( 'NONE',  ( 14.08420738312798015, -5.827078755546623690, 34.72654668319379567 ) ) ;
#85523=ORIENTED_EDGE ( 'NONE', *, *, #78163, .T. ) ;
#85524=CARTESIAN_POINT ( 'NONE',  ( 0.4615384615384611200, -2.499999999999998668, 29.75000000000001421 ) ) ;
#85525=B_SPLINE_CURVE_WITH_KNOTS ( 'NONE', 3,
 ( #19354, #8503, #76513, #43168, #61656, #70641, #82393, #54910, #15703, #27882 ),
 .UNSPECIFIED., .F., .F.,
 ( 4, 2, 2, 2, 4 ),
 ( 0.000000000000000000, 0.0001954311564186867389, 0.0003908623128373734778, 0.0005862934692560602167, 0.0007817246256747469556 ),
 .UNSPECIFIED. ) ;
#85526=CARTESIAN_POINT ( 'NONE',  ( 6.923076923076924238, -12.62096338111211580, 30.90682066428153263 ) ) ;
#85527=CARTESIAN_POINT ( 'NONE',  ( -2.307692307692427391, -11.48612834414049644, 32.76840700105863391 ) ) ;
#85528=FACE_BOUND ( 'NONE', #36999, .T. ) ;
#85531=CARTESIAN_POINT ( 'NONE',  ( 3.930361229281821966, -2.353723527008295680, 30.78948104536958752 ) ) ;
#85532=DIRECTION ( 'NONE',  ( -1.000000000000000000, 0.000000000000000000, 0.000000000000000000 ) ) ;
#85533=DIRECTION ( 'NONE',  ( 0.000000000000000000, 0.7660444431189807890, 0.6427876096865361433 ) ) ;
#85534=CARTESIAN_POINT ( 'NONE',  ( 6.699591979352975457, -11.89387501736622710, 32.13663884655806413 ) ) ;
#85535=CARTESIAN_POINT ( 'NONE',  ( 8.545745844666440050, -9.417330523894424488, 34.63758898049880486 ) ) ;
#85536=CARTESIAN_POINT ( 'NONE',  ( 1.515405825582335275, -2.295524264805589354, 30.44142389570982488 ) ) ;
#85538=CARTESIAN_POINT ( 'NONE',  ( 14.37283808702427557, -7.750023238201979581, 34.74374492549440419 ) ) ;
#85539=VERTEX_POINT ( 'NONE', #43022 ) ;
#85540=ORIENTED_EDGE ( 'NONE', *, *, #37093, .T. ) ;
#85541=DIRECTION ( 'NONE',  ( 0.000000000000000000, 0.7660444431189822323, -0.6427876096865344779 ) ) ;
#85542=CARTESIAN_POINT ( 'NONE',  ( 15.00728430620489995, -3.019605429927184392, 32.48692288466676814 ) ) ;
#85543=CARTESIAN_POINT ( 'NONE',  ( 2.373760658694747949, -2.538708090699994813, 30.37095296980875503 ) ) ;
#85545=DIRECTION ( 'NONE',  ( -0.000000000000000000, 0.6427876096865404731, -0.7660444431189770143 ) ) ;
#85546=DIRECTION ( 'NONE',  ( -0.000000000000000000, -0.9396926207859092051, -0.3420201433256662704 ) ) ;
#85547=EDGE_LOOP ( 'NONE', ( #65457, #24883, #73269, #15386 ) ) ;
#85548=ADVANCED_FACE ( 'NONE', ( #70493 ), #49338, .F. ) ;
#85549=FACE_OUTER_BOUND ( 'NONE', #28126, .T. ) ;
#85550=CARTESIAN_POINT ( 'NONE',  ( 15.23076923076923173, -10.67929555188718282, 33.92786785259544047 ) ) ;
#85551=FACE_OUTER_BOUND ( 'NONE', #18216, .T. ) ;
#85553=CARTESIAN_POINT ( 'NONE',  ( -16.94613263595612551, -2.494656445102014342, 31.33466734024120015 ) ) ;
#85554=EDGE_CURVE ( 'NONE', #5299, #2439, #34924, .T. ) ;
#85556=ORIENTED_EDGE ( 'NONE', *, *, #66184, .T. ) ;
#85557=ORIENTED_EDGE ( 'NONE', *, *, #81963, .F. ) ;
#85558=EDGE_CURVE ( 'NONE', #313, #61826, #2876, .T. ) ;
#85559=CARTESIAN_POINT ( 'NONE',  ( 14.05771556364371833, -12.41104346484419452, 31.60698883733904196 ) ) ;
#85560=ORIENTED_EDGE ( 'NONE', *, *, #88070, .T. ) ;
#85561=DIRECTION ( 'NONE',  ( -0.000000000000000000, -0.000000000000000000, -1.000000000000000000 ) ) ;
#85562=CARTESIAN_POINT ( 'NONE',  ( 9.757563263583717728, -10.21337939537593620, 33.94971097300152252 ) ) ;
#85563=CARTESIAN_POINT ( 'NONE',  ( -16.15384615384615330, -4.786620604624113540, 33.94971097300155094 ) ) ;
#85564=CYLINDRICAL_SURFACE ( 'NONE', #25780, 0.2499999999999973355 ) ;
#85566=EDGE_CURVE ( 'NONE', #85122, #42793, #62387, .T. ) ;
#85567=CARTESIAN_POINT ( 'NONE',  ( 14.17700170458200404, -6.369640206132551441, 34.87707690430378449 ) ) ;
#85568=VECTOR ( 'NONE', #24188, 1000.000000000000000 ) ;
#85569=ORIENTED_EDGE ( 'NONE', *, *, #8207, .F. ) ;
#85570=DIRECTION ( 'NONE',  ( -0.000000000000000000, 0.3420201433256694901, -0.9396926207859082059 ) ) ;
#85571=LINE ( 'NONE', #51297, #35293 ) ;
#85572=ORIENTED_EDGE ( 'NONE', *, *, #41605, .T. ) ;
#85573=DIRECTION ( 'NONE',  ( -0.000000000000000000, 0.5000000000000011102, -0.8660254037844381525 ) ) ;
#85574=CARTESIAN_POINT ( 'NONE',  ( 14.30769230769218758, -12.27809138561165270, 31.22303859784587132 ) ) ;
#85575=CARTESIAN_POINT ( 'NONE',  ( -3.099930812756466647, -7.277220443632450575, 34.74524770363009196 ) ) ;
#85576=CARTESIAN_POINT ( 'NONE',  ( 0.4615384615384611200, -2.721908614388771852, 31.22303859784724978 ) ) ;
#85577=CARTESIAN_POINT ( 'NONE',  ( -6.066083410955879884, -9.780366693483667717, 34.19971097300155805 ) ) ;
#85578=CARTESIAN_POINT ( 'NONE',  ( 7.715463243043537034, -3.338472653186243644, 32.95098750199972670 ) ) ;
#85579=FACE_OUTER_BOUND ( 'NONE', #38765, .T. ) ;
#85583=CARTESIAN_POINT ( 'NONE',  ( -13.25408994638174143, -10.31582465632705237, 34.18122507451815295 ) ) ;
#85584=CARTESIAN_POINT ( 'NONE',  ( -13.51530685128294351, -8.999036380462717588, 34.52022231692819076 ) ) ;
#85586=CARTESIAN_POINT ( 'NONE',  ( 0.2115617174898694053, -5.643011162660950042, 34.66104346484419096 ) ) ;
#85587=CARTESIAN_POINT ( 'NONE',  ( 15.93036122928181975, -4.988325925672468131, 34.36044203135681130 ) ) ;
#85588=ORIENTED_EDGE ( 'NONE', *, *, #39546, .F. ) ;
#85590=FACE_OUTER_BOUND ( 'NONE', #45857, .T. ) ;
#85591=EDGE_CURVE ( 'NONE', #43411, #57339, #8242, .T. ) ;
#85592=EDGE_LOOP ( 'NONE', ( #10344, #22297, #14312, #65959 ) ) ;
#85593=DIRECTION ( 'NONE',  ( 0.000000000000000000, 0.1736481776669267785, -0.9848077530122087975 ) ) ;
#85594=ORIENTED_EDGE ( 'NONE', *, *, #30633, .F. ) ;
#85595=CARTESIAN_POINT ( 'NONE',  ( 17.93472955403921887, -6.879047030191174805, 34.71129190930000163 ) ) ;
#85596=DIRECTION ( 'NONE',  ( -0.000000000000000000, -0.1736481776669307198, -0.9848077530122080203 ) ) ;
#85598=FACE_OUTER_BOUND ( 'NONE', #5883, .T. ) ;
#85599=EDGE_LOOP ( 'NONE', ( #87275, #47314, #47285, #86225 ) ) ;
#85600=CYLINDRICAL_SURFACE ( 'NONE', #73882, 0.2499999999999997502 ) ;
#85601=ORIENTED_EDGE ( 'NONE', *, *, #27109, .F. ) ;
#85604=CARTESIAN_POINT ( 'NONE',  ( 1.384615384615386802, -8.164416787775445883, 34.95778746994557906 ) ) ;
#85605=DIRECTION ( 'NONE',  ( 0.000000000000000000, 0.4999999999999985567, 0.8660254037844395958 ) ) ;
#85606=ORIENTED_EDGE ( 'NONE', *, *, #68391, .T. ) ;
#85608=CARTESIAN_POINT ( 'NONE',  ( -6.130147969731696733, -11.04286588640298561, 33.62463336215343901 ) ) ;
#85609=DIRECTION ( 'NONE',  ( -1.000000000000000000, 0.000000000000000000, 0.000000000000000000 ) ) ;
#85611=CARTESIAN_POINT ( 'NONE',  ( 4.946231610255517275, -8.999036380462719364, 34.52022231692819076 ) ) ;
#85612=CARTESIAN_POINT ( 'NONE',  ( -11.47320639894870276, -3.643525952247864463, 33.31231777344670064 ) ) ;
#85613=B_SPLINE_CURVE_WITH_KNOTS ( 'NONE', 3,
 ( #25662, #67538, #39189, #73860, #66650, #12155, #86034, #31528, #53569, #31978 ),
 .UNSPECIFIED., .F., .F.,
 ( 4, 2, 2, 2, 4 ),
 ( 0.0007817359430256288133, 0.0009771253907249948054, 0.001172514838424360689, 0.001367904286123726573, 0.001563293733823092457 ),
 .UNSPECIFIED. ) ;
#85615=EDGE_CURVE ( 'NONE', #1602, #54361, #38043, .T. ) ;
#85616=ORIENTED_EDGE ( 'NONE', *, *, #56694, .T. ) ;
#85617=ORIENTED_EDGE ( 'NONE', *, *, #59795, .F. ) ;
#85619=CARTESIAN_POINT ( 'NONE',  ( 3.296837581771669967, -3.513871655860379306, 32.76840700105978499 ) ) ;
#85621=EDGE_CURVE ( 'NONE', #5632, #33486, #76986, .T. ) ;
#85623=CYLINDRICAL_SURFACE ( 'NONE', #53591, 0.2500000000000002220 ) ;
#85625=ORIENTED_EDGE ( 'NONE', *, *, #35497, .F. ) ;
#85626=VERTEX_POINT ( 'NONE', #17325 ) ;
#85629=CARTESIAN_POINT ( 'NONE',  ( -1.449885830576160384, -11.94971097300153140, 32.03036669348370680 ) ) ;
#85630=ORIENTED_EDGE ( 'NONE', *, *, #24750, .F. ) ;
#85631=CARTESIAN_POINT ( 'NONE',  ( 11.53846153846153832, -11.16473453929635440, 33.15142922261926373 ) ) ;
#85632=B_SPLINE_CURVE_WITH_KNOTS ( 'NONE', 3,
 ( #79643, #38651, #39564, #5757, #33233, #18831, #53039, #73328, #66574, #72870 ),
 .UNSPECIFIED., .F., .F.,
 ( 4, 2, 2, 2, 4 ),
 ( 0.000000000000000000, 0.0001954311564186881484, 0.0003908623128373762967, 0.0005862934692560644451, 0.0007817246256747525934 ),
 .UNSPECIFIED. ) ;
#85633=DIRECTION ( 'NONE',  ( -0.000000000000000000, -0.7660444431189791237, -0.6427876096865379196 ) ) ;
#85634=B_SPLINE_CURVE_WITH_KNOTS ( 'NONE', 3,
 ( #88943, #62754, #74517, #82169, #19568, #40298, #47923, #67762, #55125, #33538 ),
 .UNSPECIFIED., .F., .F.,
 ( 4, 2, 2, 2, 4 ),
 ( 0.000000000000000000, 0.0001954311564186879857, 0.0003908623128373759715, 0.0005862934692560640114, 0.0007817246256747519429 ),
 .UNSPECIFIED. ) ;
#85636=CYLINDRICAL_SURFACE ( 'NONE', #79957, 0.2499999999999997502 ) ;
#85637=B_SPLINE_CURVE_WITH_KNOTS ( 'NONE', 3,
 ( #61390, #38582, #3891, #74480, #66037, #11106, #81690, #4348, #59288, #33930 ),
 .UNSPECIFIED., .F., .F.,
 ( 4, 2, 2, 2, 4 ),
 ( 0.0007817246256747434861, 0.0009771112852218859484, 0.001172497944769028411, 0.001367884604316171090, 0.001563271263863313552 ),
 .UNSPECIFIED. ) ;
#85638=FACE_BOUND ( 'NONE', #79813, .T. ) ;
#85639=VERTEX_POINT ( 'NONE', #65507 ) ;
#85640=CYLINDRICAL_SURFACE ( 'NONE', #84579, 0.2499999999999998890 ) ;
#85641=CARTESIAN_POINT ( 'NONE',  ( 4.219101725122177626, -8.613356846314928816, 34.62446782046653482 ) ) ;
#85642=EDGE_CURVE ( 'NONE', #41132, #16668, #45621, .T. ) ;
#85643=CARTESIAN_POINT ( 'NONE',  ( 2.057669083470851756, -8.475808217655753651, 34.90892951860618609 ) ) ;
#85644=FACE_OUTER_BOUND ( 'NONE', #42105, .T. ) ;
#85645=ORIENTED_EDGE ( 'NONE', *, *, #45640, .F. ) ;
#85646=CARTESIAN_POINT ( 'NONE',  ( -17.20761454359063691, -12.38065189839062263, 30.83690757178629482 ) ) ;
#85647=ORIENTED_EDGE ( 'NONE', *, *, #33860, .F. ) ;
#85648=VERTEX_POINT ( 'NONE', #58301 ) ;
#85650=FACE_OUTER_BOUND ( 'NONE', #18275, .T. ) ;
#85651=CARTESIAN_POINT ( 'NONE',  ( -0.4615384615384611200, -2.486705287966279876, 31.30864560766543647 ) ) ;
#85653=CARTESIAN_POINT ( 'NONE',  ( 7.715462379486289102, -12.38065189839062263, 30.83690757178629482 ) ) ;
#85654=CARTESIAN_POINT ( 'NONE',  ( -12.33101275977490019, -4.459921816937791661, 33.71989282347011851 ) ) ;
#85655=ORIENTED_EDGE ( 'NONE', *, *, #19717, .T. ) ;
#85656=ADVANCED_FACE ( 'NONE', ( #11020 ), #31285, .F. ) ;
#85657=VECTOR ( 'NONE', #57864, 1000.000000000000114 ) ;
#85659=CARTESIAN_POINT ( 'NONE',  ( 3.100621261037536325, -9.504002272028875709, 34.60269587691767867 ) ) ;
#85660=CARTESIAN_POINT ( 'NONE',  ( -17.20707028636129721, -11.93770438780619259, 32.05411857736982029 ) ) ;
#85661=CARTESIAN_POINT ( 'NONE',  ( 14.55774672760576571, -2.544122305571458575, 31.48381861865057729 ) ) ;
#85662=VERTEX_POINT ( 'NONE', #64161 ) ;
#85663=EDGE_CURVE ( 'NONE', #8169, #56983, #62834, .T. ) ;
#85664=ORIENTED_EDGE ( 'NONE', *, *, #40548, .T. ) ;
#85665=FACE_BOUND ( 'NONE', #51690, .T. ) ;
#85666=ORIENTED_EDGE ( 'NONE', *, *, #67392, .F. ) ;
#85667=CARTESIAN_POINT ( 'NONE',  ( -17.93129618099669997, -2.255932369308304875, 29.99950897402476713 ) ) ;
#85668=CARTESIAN_POINT ( 'NONE',  ( -1.161835715637317579, -2.353885683473779356, 30.79025554430704759 ) ) ;
#85670=CARTESIAN_POINT ( 'NONE',  ( 13.38461538461526601, -11.48612834414049644, 32.76840700105863391 ) ) ;
#85671=DIRECTION ( 'NONE',  ( -0.000000000000000000, 0.6427876096865404731, -0.7660444431189771253 ) ) ;
#85672=CARTESIAN_POINT ( 'NONE',  ( 5.010839665967195877, -2.721908614388772740, 31.22303859784724622 ) ) ;
#85673=CARTESIAN_POINT ( 'NONE',  ( -1.253824943648432777, -3.957578996910242619, 33.62503395064540257 ) ) ;
#85674=ORIENTED_EDGE ( 'NONE', *, *, #75333, .F. ) ;
#85675=EDGE_CURVE ( 'NONE', #25023, #67015, #38120, .T. ) ;
#85676=DIRECTION ( 'NONE',  ( 0.000000000000000000, 0.9848077530122072432, -0.1736481776669354937 ) ) ;
#85678=B_SPLINE_CURVE_WITH_KNOTS ( 'NONE', 3,
 ( #41363, #41813, #48542, #35488, #8020, #34602, #49000, #75579, #36378, #15224 ),
 .UNSPECIFIED., .F., .F.,
 ( 4, 2, 2, 2, 4 ),
 ( 0.000000000000000000, 0.0001954311564186881213, 0.0003908623128373762425, 0.0005862934692560643367, 0.0007817246256747524850 ),
 .UNSPECIFIED. ) ;
#85681=LINE ( 'NONE', #73506, #29667 ) ;
#85682=CARTESIAN_POINT ( 'NONE',  ( 3.930361210122205406, -6.760086850603068243, 34.69517049084099369 ) ) ;
#85683=DIRECTION ( 'NONE',  ( -0.000000000000000000, 0.7660444431189791237, -0.6427876096865379196 ) ) ;
#85684=CARTESIAN_POINT ( 'NONE',  ( -4.088590582570127197, -12.46129190930001052, 30.37095296980870174 ) ) ;
#85685=CARTESIAN_POINT ( 'NONE',  ( 13.51540719244017374, -5.582136614379148654, 34.36778462344220486 ) ) ;
#85686=EDGE_CURVE ( 'NONE', #58760, #43442, #9101, .T. ) ;
#85687=CARTESIAN_POINT ( 'NONE',  ( 5.207448778686639024, -12.45806712695776319, 30.39783852428763922 ) ) ;
#85689=ORIENTED_EDGE ( 'NONE', *, *, #37463, .T. ) ;
#85690=CARTESIAN_POINT ( 'NONE',  ( 4.153846153846154188, -9.819645486525091727, 36.12317359536749706 ) ) ;
#85691=CYLINDRICAL_SURFACE ( 'NONE', #69247, 0.2500000000000004996 ) ;
#85692=CARTESIAN_POINT ( 'NONE',  ( 6.223375940698185005, -2.501478030877322567, 29.88021232661720816 ) ) ;
#85693=AXIS2_PLACEMENT_3D ( 'NONE', #33738, #40070, #86935 ) ;
#85694=ORIENTED_EDGE ( 'NONE', *, *, #65978, .F. ) ;
#85695=EDGE_LOOP ( 'NONE', ( #85625, #58052 ) ) ;
#85696=CYLINDRICAL_SURFACE ( 'NONE', #68550, 0.2499999999999995559 ) ;
#85697=CARTESIAN_POINT ( 'NONE',  ( -14.24243716817947103, -2.657715359629131857, 31.77849191805844242 ) ) ;
#85698=EDGE_CURVE ( 'NONE', #60580, #62474, #36990, .T. ) ;
#85699=CARTESIAN_POINT ( 'NONE',  ( 5.999999999999880096, -11.48612834414049644, 32.76840700105863391 ) ) ;
#85700=VECTOR ( 'NONE', #52680, 1000.000000000000000 ) ;
#85701=CARTESIAN_POINT ( 'NONE',  ( 9.562160482869472844, -12.45813303252208648, 30.39737893381572675 ) ) ;
#85702=FACE_OUTER_BOUND ( 'NONE', #40775, .T. ) ;
#85704=CARTESIAN_POINT ( 'NONE',  ( -16.82697766754503377, -11.56426240980093567, 33.07394671870546432 ) ) ;
#85705=CARTESIAN_POINT ( 'NONE',  ( -14.98071481085577972, -8.346898887586323923, 34.93166121998716278 ) ) ;
#85706=ORIENTED_EDGE ( 'NONE', *, *, #19136, .F. ) ;
#85707=LINE ( 'NONE', #2383, #85140 ) ;
#85708=CARTESIAN_POINT ( 'NONE',  ( -17.01177729759111301, -7.750023238201980469, 34.74374492549440419 ) ) ;
#85709=CARTESIAN_POINT ( 'NONE',  ( 4.403846153847572609, -7.500000000000154543, 35.00000000000007105 ) ) ;
#85710=CARTESIAN_POINT ( 'NONE',  ( -18.00000000000000000, -13.85434399251292170, 33.13000708000598138 ) ) ;
#85711=VERTEX_POINT ( 'NONE', #39392 ) ;
#85714=EDGE_LOOP ( 'NONE', ( #23794, #80870, #5787, #32144 ) ) ;
#85715=CARTESIAN_POINT ( 'NONE',  ( -0.3962828902624376815, -2.892918686051626498, 31.69288490824025928 ) ) ;
#85717=CARTESIAN_POINT ( 'NONE',  ( 16.37722163961857547, -2.251407671071269601, 29.88021292934942963 ) ) ;
#85718=CARTESIAN_POINT ( 'NONE',  ( -8.769230769230768274, -1.509761064869970415, 31.06009739812519044 ) ) ;
#85719=EDGE_LOOP ( 'NONE', ( #19699, #49715 ) ) ;
#85720=CARTESIAN_POINT ( 'NONE',  ( -1.449885385171702845, -12.70778746994557551, 30.41441678777548319 ) ) ;
#85721=CYLINDRICAL_SURFACE ( 'NONE', #53781, 0.2499999999999994726 ) ;
#85722=LINE ( 'NONE', #85282, #55823 ) ;
#85723=B_SPLINE_CURVE_WITH_KNOTS ( 'NONE', 3,
 ( #1925, #50101, #9564, #49669, #2794, #78460, #16761, #71702, #57311, #17207 ),
 .UNSPECIFIED., .F., .F.,
 ( 4, 2, 2, 2, 4 ),
 ( 0.0007817359430256216575, 0.0009771253907249859150, 0.001172514838424350064, 0.001367904286123714213, 0.001563293733823078362 ),
 .UNSPECIFIED. ) ;
#85725=CARTESIAN_POINT ( 'NONE',  ( -4.854143407945011646, -10.97394488606064122, 33.68653795673694873 ) ) ;
#85727=EDGE_LOOP ( 'NONE', ( #56733, #75543, #85188, #26928 ) ) ;
#85728=CARTESIAN_POINT ( 'NONE',  ( 16.21910129335899597, -10.33852847137154107, 34.16647553114620450 ) ) ;
#85729=ORIENTED_EDGE ( 'NONE', *, *, #7213, .T. ) ;
#85730=CARTESIAN_POINT ( 'NONE',  ( -10.39200867468643175, -2.501478030877323455, 29.88021232661721172 ) ) ;
#85731=ADVANCED_FACE ( 'NONE', ( #26748 ), #87588, .F. ) ;
#85732=CARTESIAN_POINT ( 'NONE',  ( -16.37677237136229991, -11.24512374952581872, 33.06303171183252942 ) ) ;
#85734=EDGE_CURVE ( 'NONE', #59182, #84305, #70353, .T. ) ;
#85735=AXIS2_PLACEMENT_3D ( 'NONE', #12279, #58237, #78959 ) ;
#85736=CARTESIAN_POINT ( 'NONE',  ( -14.17716660592874156, -11.93748526763465279, 32.05452791011430946 ) ) ;
#85737=CARTESIAN_POINT ( 'NONE',  ( 9.442284455014730682, -8.432397168068783699, 34.66272746175022945 ) ) ;
#85738=ORIENTED_EDGE ( 'NONE', *, *, #9022, .F. ) ;
#85739=ORIENTED_EDGE ( 'NONE', *, *, #53365, .F. ) ;
#85740=EDGE_CURVE ( 'NONE', #46211, #45649, #30630, .T. ) ;
#85741=EDGE_LOOP ( 'NONE', ( #50971, #88291, #63922, #85489 ) ) ;
#85743=CARTESIAN_POINT ( 'NONE',  ( 12.46153846153846168, -11.69971097300155272, 32.46337939537588113 ) ) ;
#85744=CARTESIAN_POINT ( 'NONE',  ( -1.134669866267241867, -12.43552623307873972, 30.55307653245132826 ) ) ;
#85746=FACE_OUTER_BOUND ( 'NONE', #11629, .T. ) ;
#85747=CARTESIAN_POINT ( 'NONE',  ( -5.777220458731589403, -5.114059244376869984, 34.14424750095245287 ) ) ;
#85748=FACE_OUTER_BOUND ( 'NONE', #36097, .T. ) ;
#85749=CARTESIAN_POINT ( 'NONE',  ( 3.230769230769231726, -5.557115091759785130, 34.35708131394839171 ) ) ;
#85752=CARTESIAN_POINT ( 'NONE',  ( -17.75005448165186195, -10.05730279482229683, 34.04704008940765902 ) ) ;
#85753=CARTESIAN_POINT ( 'NONE',  ( -3.930834802233304170, -10.61302985866383963, 33.66295027996417843 ) ) ;
#85754=VERTEX_POINT ( 'NONE', #54209 ) ;
#85755=ORIENTED_EDGE ( 'NONE', *, *, #19034, .T. ) ;
#85756=VECTOR ( 'NONE', #59678, 1000.000000000000000 ) ;
#85757=VERTEX_POINT ( 'NONE', #67741 ) ;
#85759=CARTESIAN_POINT ( 'NONE',  ( 6.249945409378045547, -12.45601412856602863, 31.48342859153981621 ) ) ;
#85760=EDGE_LOOP ( 'NONE', ( #89054, #53392 ) ) ;
#85761=CARTESIAN_POINT ( 'NONE',  ( 8.899756470994333313, -8.586989748646452369, 34.63063291749215011 ) ) ;
#85762=CARTESIAN_POINT ( 'NONE',  ( -16.40382288478850725, -9.943427161483782584, 34.11278801902876978 ) ) ;
#85763=FACE_OUTER_BOUND ( 'NONE', #6126, .T. ) ;
#85764=CARTESIAN_POINT ( 'NONE',  ( -9.692307692307691624, -6.386643153685126251, 34.62446782046654192 ) ) ;
#85765=VERTEX_POINT ( 'NONE', #68184 ) ;
#85766=ORIENTED_EDGE ( 'NONE', *, *, #84563, .F. ) ;
#85767=CARTESIAN_POINT ( 'NONE',  ( -2.177647144857528527, -2.504778602574659896, 29.97347330155780298 ) ) ;
#85768=EDGE_CURVE ( 'NONE', #74753, #88347, #77844, .T. ) ;
#85769=ORIENTED_EDGE ( 'NONE', *, *, #32133, .F. ) ;
#85770=FACE_BOUND ( 'NONE', #17478, .T. ) ;
#85771=CARTESIAN_POINT ( 'NONE',  ( -6.223484943723947893, -9.331801661448606566, 34.40259984581193464 ) ) ;
#85772=B_SPLINE_CURVE_WITH_KNOTS ( 'NONE', 3,
 ( #725, #55659, #21885, #61976, #285, #27751, #82712, #49361, #48456, #42172 ),
 .UNSPECIFIED., .F., .F.,
 ( 4, 2, 2, 2, 4 ),
 ( 0.000000000000000000, 0.0001954339857564073659, 0.0003908679715128147319, 0.0005863019572692221250, 0.0007817359430256294638 ),
 .UNSPECIFIED. ) ;
#85773=DIRECTION ( 'NONE',  ( -0.000000000000000000, 0.3420201433256694901, -0.9396926207859082059 ) ) ;
#85775=CARTESIAN_POINT ( 'NONE',  ( -1.253824943648434109, -5.496552790871119143, 34.60292014791297532 ) ) ;
#85776=EDGE_CURVE ( 'NONE', #73779, #4699, #1603, .T. ) ;
#85777=CARTESIAN_POINT ( 'NONE',  ( 11.31553457955469000, -6.459968553980841577, 34.89616026154728701 ) ) ;
#85780=CARTESIAN_POINT ( 'NONE',  ( -11.60373153901785948, -5.094484230520674117, 34.41647553114621161 ) ) ;
#85781=CARTESIAN_POINT ( 'NONE',  ( 3.007284287045281168, -12.24155766932282496, 31.33739205006857986 ) ) ;
#85782=ORIENTED_EDGE ( 'NONE', *, *, #55315, .F. ) ;
#85783=DIRECTION ( 'NONE',  ( 0.000000000000000000, 0.4999999999999985567, 0.8660254037844395958 ) ) ;
#85784=FACE_OUTER_BOUND ( 'NONE', #624, .T. ) ;
#85785=EDGE_LOOP ( 'NONE', ( #47518, #1365, #33054, #51694 ) ) ;
#85786=CARTESIAN_POINT ( 'NONE',  ( 7.145856592054987466, -2.612705202774697533, 31.66806509827799943 ) ) ;
#85787=CYLINDRICAL_SURFACE ( 'NONE', #67014, 0.2500000000000002220 ) ;
#85788=CYLINDRICAL_SURFACE ( 'NONE', #75776, 0.2500000000000008882 ) ;
#85789=CARTESIAN_POINT ( 'NONE',  ( -8.638705067467206788, -9.417988943895561960, 34.36773134775777550 ) ) ;
#85790=LINE ( 'NONE', #24073, #2752 ) ;
#85791=VECTOR ( 'NONE', #69181, 1000.000000000000227 ) ;
#85792=CARTESIAN_POINT ( 'NONE',  ( 6.223011351612851350, -9.886259254753566594, 34.14407573483972413 ) ) ;
#85793=CARTESIAN_POINT ( 'NONE',  ( -13.38461538461538325, -3.937682226553329556, 33.60647404775216529 ) ) ;
#85795=EDGE_CURVE ( 'NONE', #82786, #65345, #61725, .T. ) ;
#85797=CARTESIAN_POINT ( 'NONE',  ( -0.2114840416250086119, -8.346898887586323923, 34.93166121998716278 ) ) ;
#85798=CARTESIAN_POINT ( 'NONE',  ( -15.29603967673000753, -11.94971097300153140, 32.03036669348370680 ) ) ;
#85799=CARTESIAN_POINT ( 'NONE',  ( -16.15384615384615330, -3.513871655860378418, 32.76840700105978499 ) ) ;
#85801=VERTEX_POINT ( 'NONE', #77153 ) ;
#85802=CARTESIAN_POINT ( 'NONE',  ( 0.4615384615384611200, -12.37446782046654192, 30.86335684631486131 ) ) ;
#85803=VERTEX_POINT ( 'NONE', #15015 ) ;
#85805=VERTEX_POINT ( 'NONE', #41595 ) ;
#85806=CARTESIAN_POINT ( 'NONE',  ( -13.38461538461538325, -2.292212530054420494, 30.41441678777542634 ) ) ;
#85807=ORIENTED_EDGE ( 'NONE', *, *, #70901, .F. ) ;
#85808=CARTESIAN_POINT ( 'NONE',  ( 18.06514577933196009, -7.750023238201980469, 34.74374492549440419 ) ) ;
#85810=CYLINDRICAL_SURFACE ( 'NONE', #40115, 0.2500000000000004996 ) ;
#85812=CARTESIAN_POINT ( 'NONE',  ( 6.857806477116147548, -11.48612834413959582, 32.76840700105983473 ) ) ;
#85813=CARTESIAN_POINT ( 'NONE',  ( -2.980714810855777053, -12.41089969410671223, 31.60739465890703670 ) ) ;
#85814=CARTESIAN_POINT ( 'NONE',  ( -14.53061926659915315, -10.77366814457252175, 33.85459836347579454 ) ) ;
#85815=CARTESIAN_POINT ( 'NONE',  ( -16.21911615440247090, -10.33852847137145048, 34.16647553114627556 ) ) ;
#85816=FACE_OUTER_BOUND ( 'NONE', #24589, .T. ) ;
#85817=LINE ( 'NONE', #24097, #22358 ) ;
#85819=EDGE_CURVE ( 'NONE', #25692, #10070, #13677, .T. ) ;
#85820=EDGE_CURVE ( 'NONE', #62030, #7735, #67171, .T. ) ;
#85821=CARTESIAN_POINT ( 'NONE',  ( 1.515141086378952506, -3.285477652293412820, 32.44071101563363158 ) ) ;
#85822=CARTESIAN_POINT ( 'NONE',  ( 13.16168842570853492, -3.395401636524185474, 33.02366814457250399 ) ) ;
#85823=B_SPLINE_CURVE_WITH_KNOTS ( 'NONE', 3,
 ( #24613, #18757, #11103, #31375, #85878, #80008, #4344, #87672, #52965, #32698 ),
 .UNSPECIFIED., .F., .F.,
 ( 4, 2, 2, 2, 4 ),
 ( 0.000000000000000000, 0.0001954339857564078809, 0.0003908679715128157619, 0.0005863019572692236428, 0.0007817359430256315238 ),
 .UNSPECIFIED. ) ;
#85824=CARTESIAN_POINT ( 'NONE',  ( -3.230769230768915534, -2.255955759149395501, 30.00000000000324363 ) ) ;
#85825=ADVANCED_FACE ( 'NONE', ( #35279 ), #34831, .F. ) ;
#85826=ORIENTED_EDGE ( 'NONE', *, *, #38756, .F. ) ;
#85827=CARTESIAN_POINT ( 'NONE',  ( 17.20744877868663991, -12.27024696741798770, 31.24895572276497546 ) ) ;
#85828=FACE_OUTER_BOUND ( 'NONE', #69021, .T. ) ;
#85829=CARTESIAN_POINT ( 'NONE',  ( 1.161688425708537808, -10.77366814457252175, 33.85459836347579454 ) ) ;
#85830=CARTESIAN_POINT ( 'NONE',  ( 16.02323649864207056, -7.722926974430166069, 34.99546784045485737 ) ) ;
#85831=CARTESIAN_POINT ( 'NONE',  ( -18.00000000000000000, -12.50000000000000000, 29.49999999999997868 ) ) ;
#85832=TOROIDAL_SURFACE ( 'NONE', #29694, 3.000000000000000888, 2.000000000000000000 ) ;
#85833=CARTESIAN_POINT ( 'NONE',  ( -9.019207500173124004, -8.303909089506435137, 34.68538101551103381 ) ) ;
#85834=ORIENTED_EDGE ( 'NONE', *, *, #24350, .T. ) ;
#85835=CARTESIAN_POINT ( 'NONE',  ( -1.161604033002533898, -9.886259254753564818, 34.14407573483972413 ) ) ;
#85837=EDGE_LOOP ( 'NONE', ( #76249, #9735 ) ) ;
#85838=CARTESIAN_POINT ( 'NONE',  ( 0.7114838709165037800, -12.45601412856602863, 31.48342859153981621 ) ) ;
#85839=CARTESIAN_POINT ( 'NONE',  ( -6.792551484843277976, -5.915461855592777596, 34.75538340440931506 ) ) ;
#85841=CARTESIAN_POINT ( 'NONE',  ( -6.130691466667560263, -3.062553014421049546, 32.05460306192773601 ) ) ;
#85842=CARTESIAN_POINT ( 'NONE',  ( 13.16113046005105858, -5.827078755546623690, 34.72654668319379567 ) ) ;
#85843=ORIENTED_EDGE ( 'NONE', *, *, #25303, .F. ) ;
#85845=B_SPLINE_CURVE_WITH_KNOTS ( 'NONE', 3,
 ( #8391, #49807, #43059, #64197, #56131, #29991, #50687, #2068, #21901, #15592 ),
 .UNSPECIFIED., .F., .F.,
 ( 4, 2, 2, 2, 4 ),
 ( 0.000000000000000000, 0.0001954339857564082604, 0.0003908679715128165208, 0.0005863019572692248355, 0.0007817359430256330417 ),
 .UNSPECIFIED. ) ;
#85847=CARTESIAN_POINT ( 'NONE',  ( -3.903900744468110418, -12.07971442181322352, 32.31769673815850297 ) ) ;
#85848=CARTESIAN_POINT ( 'NONE',  ( 16.21991450484859598, -12.37446782046654192, 30.86335684631486842 ) ) ;
#85849=AXIS2_PLACEMENT_3D ( 'NONE', #67564, #73876, #40975 ) ;
#85850=LINE ( 'NONE', #86310, #13518 ) ;
#85851=CARTESIAN_POINT ( 'NONE',  ( 10.39245765647776309, -4.762599654559228846, 34.23009711892697737 ) ) ;
#85852=CARTESIAN_POINT ( 'NONE',  ( 11.28843831424008215, -10.92453946501458795, 33.72985991061850086 ) ) ;
#85853=CARTESIAN_POINT ( 'NONE',  ( -18.00000000000000000, -11.69971097300155449, 32.46337939537587403 ) ) ;
#85854=EDGE_LOOP ( 'NONE', ( #27010, #88863, #76963, #42768 ) ) ;
#85855=VERTEX_POINT ( 'NONE', #611 ) ;
#85857=VERTEX_POINT ( 'NONE', #55106 ) ;
#85858=EDGE_CURVE ( 'NONE', #60430, #5967, #23133, .T. ) ;
#85859=DIRECTION ( 'NONE',  ( -0.000000000000000000, 0.5000000000000011102, -0.8660254037844381525 ) ) ;
#85860=EDGE_LOOP ( 'NONE', ( #60064, #9606 ) ) ;
#85861=CARTESIAN_POINT ( 'NONE',  ( 8.068933387422251968, -12.44528174975671853, 30.48912976160716681 ) ) ;
#85862=CARTESIAN_POINT ( 'NONE',  ( -2.057746898314262385, -4.176053281294514363, 33.81426240980091791 ) ) ;
#85864=ORIENTED_EDGE ( 'NONE', *, *, #84404, .F. ) ;
#85866=EDGE_LOOP ( 'NONE', ( #26251, #20817 ) ) ;
#85867=CARTESIAN_POINT ( 'NONE',  ( -8.834500769787091201, -5.094484230520674117, 34.41647553114621161 ) ) ;
#85868=LINE ( 'NONE', #16080, #55818 ) ;
#85869=CARTESIAN_POINT ( 'NONE',  ( -17.74994558008654622, -2.544122305571458575, 31.48381861865057729 ) ) ;
#85870=DIRECTION ( 'NONE',  ( 0.000000000000000000, 0.7660444431189807890, 0.6427876096865361433 ) ) ;
#85871=DIRECTION ( 'NONE',  ( -0.000000000000000000, -0.1736481776669307198, -0.9848077530122080203 ) ) ;
#85872=AXIS2_PLACEMENT_3D ( 'NONE', #69978, #88509, #35767 ) ;
#85873=CARTESIAN_POINT ( 'NONE',  ( 8.545745825506822158, -5.912607949931405926, 34.49155766932282319 ) ) ;
#85874=CARTESIAN_POINT ( 'NONE',  ( -10.86540785267757947, -10.76384336483936011, 33.53834819971076087 ) ) ;
#85875=ORIENTED_EDGE ( 'NONE', *, *, #5670, .T. ) ;
#85876=ADVANCED_FACE ( 'NONE', ( #50112 ), #30728, .F. ) ;
#85877=CARTESIAN_POINT ( 'NONE',  ( -10.68146802634049308, -9.780366693483667717, 34.19971097300155805 ) ) ;
#85878=CARTESIAN_POINT ( 'NONE',  ( 14.98079249982687777, -4.236021600441997492, 33.53823185664189310 ) ) ;
#85879=EDGE_LOOP ( 'NONE', ( #78497, #78880, #2040, #49687 ) ) ;
#85881=CARTESIAN_POINT ( 'NONE',  ( -12.33074802057151409, -3.338503747796866872, 32.95102852606553512 ) ) ;
#85882=LINE ( 'NONE', #85002, #28604 ) ;
#85885=CARTESIAN_POINT ( 'NONE',  ( 3.230769230769231726, -8.564572088678739092, 35.78748833219616898 ) ) ;
#85886=CARTESIAN_POINT ( 'NONE',  ( -8.769230769230890843, -6.026961402154118019, 34.52809138561165270 ) ) ;
#85887=FACE_BOUND ( 'NONE', #21151, .T. ) ;
#85888=CARTESIAN_POINT ( 'NONE',  ( 13.13459214732242408, -12.22074536777954989, 31.39888409691088356 ) ) ;
#85889=CARTESIAN_POINT ( 'NONE',  ( 17.99999999999987566, -11.06231777344772027, 33.60647404775119895 ) ) ;
#85891=CIRCLE ( 'NONE', #47047, 0.2500000000000002220 ) ;
#85892=DIRECTION ( 'NONE',  ( -1.000000000000000000, 0.000000000000000000, 0.000000000000000000 ) ) ;
#85893=CARTESIAN_POINT ( 'NONE',  ( 18.24994551834813805, -11.37275283266504111, 32.91324779482534524 ) ) ;
#85894=CARTESIAN_POINT ( 'NONE',  ( 9.757563263583719504, -4.481592998940250538, 33.73612834413965089 ) ) ;
#85895=CARTESIAN_POINT ( 'NONE',  ( -4.023320715612509701, -11.04252011169590020, 33.62494198852677130 ) ) ;
#85896=LINE ( 'NONE', #36813, #70645 ) ;
#85898=VERTEX_POINT ( 'NONE', #85246 ) ;
#85899=CYLINDRICAL_SURFACE ( 'NONE', #78051, 0.2500000000000009437 ) ;
#85900=CARTESIAN_POINT ( 'NONE',  ( -14.53117725141625627, -6.760086850603066466, 34.69517049084099369 ) ) ;
#85901=FACE_OUTER_BOUND ( 'NONE', #79640, .T. ) ;
#85903=CARTESIAN_POINT ( 'NONE',  ( 6.923076923076800782, -12.70778746994576025, 30.41441678777401236 ) ) ;
#85904=CARTESIAN_POINT ( 'NONE',  ( -3.296020220930472533, -2.506253911140460922, 30.00000000000013856 ) ) ;
#85906=CARTESIAN_POINT ( 'NONE',  ( -16.21911615440247090, -5.941354392334501355, 34.76329471203369792 ) ) ;
#85907=CARTESIAN_POINT ( 'NONE',  ( -2.307692307692428724, -6.835583212225970762, 34.95778746994575670 ) ) ;
#85908=CARTESIAN_POINT ( 'NONE',  ( 11.66850897371199203, -7.723484941389743952, 34.99544897038808955 ) ) ;
#85909=CARTESIAN_POINT ( 'NONE',  ( -18.00000000000000000, -7.500000000000001776, 35.00000000000000000 ) ) ;
#85910=CARTESIAN_POINT ( 'NONE',  ( -7.173100160369890510, -4.335965774309649134, 33.62209801155881905 ) ) ;
#85912=AXIS2_PLACEMENT_3D ( 'NONE', #80690, #87009, #25281 ) ;
#85914=EDGE_CURVE ( 'NONE', #35516, #20943, #18833, .T. ) ;
#85915=DIRECTION ( 'NONE',  ( -0.000000000000000000, -0.5000000000000009992, -0.8660254037844380415 ) ) ;
#85916=LINE ( 'NONE', #24199, #8272 ) ;
#85917=VERTEX_POINT ( 'NONE', #17673 ) ;
#85918=CARTESIAN_POINT ( 'NONE',  ( 14.98079248672064345, -11.47974371597207899, 33.17467449705390692 ) ) ;
#85922=CARTESIAN_POINT ( 'NONE',  ( 2.057715576749954867, -4.236021600441998380, 33.53823185664189310 ) ) ;
#85923=CYLINDRICAL_SURFACE ( 'NONE', #35446, 0.2500000000000008882 ) ;
#85925=CARTESIAN_POINT ( 'NONE',  ( 1.449870955891410462, -4.481592998940251427, 33.73612834413965089 ) ) ;
#85926=LINE ( 'NONE', #960, #30130 ) ;
#85927=DIRECTION ( 'NONE',  ( -0.000000000000000000, 1.000000000000000000, 3.491481338843133355E-15 ) ) ;
#85928=ORIENTED_EDGE ( 'NONE', *, *, #4863, .F. ) ;
#85930=CARTESIAN_POINT ( 'NONE',  ( -13.13466986626724342, -10.05730279482229683, 34.04704008940765902 ) ) ;
#85931=VECTOR ( 'NONE', #17902, 999.9999999999998863 ) ;
#85932=DIRECTION ( 'NONE',  ( 0.000000000000000000, 0.6427876096865368094, 0.7660444431189802339 ) ) ;
#85935=DIRECTION ( 'NONE',  ( -0.000000000000000000, 0.1736481776669307198, -0.9848077530122080203 ) ) ;
#85936=CARTESIAN_POINT ( 'NONE',  ( -14.30769230769230660, -10.89733346790207413, 36.13435417666054406 ) ) ;
#85937=CARTESIAN_POINT ( 'NONE',  ( 3.903869422903799347, -9.943427161483782584, 34.11278801902876978 ) ) ;
#85939=EDGE_LOOP ( 'NONE', ( #37195, #1448 ) ) ;
#85940=B_SPLINE_CURVE_WITH_KNOTS ( 'NONE', 3,
 ( #62584, #12644, #81997, #47304, #40569, #60822, #74795, #13084, #75236, #41003 ),
 .UNSPECIFIED., .F., .F.,
 ( 4, 2, 2, 2, 4 ),
 ( 0.0007817359430256288133, 0.0009771253907249948054, 0.001172514838424360689, 0.001367904286123726573, 0.001563293733823092457 ),
 .UNSPECIFIED. ) ;
#85941=B_SPLINE_CURVE_WITH_KNOTS ( 'NONE', 3,
 ( #40762, #20032, #25909, #39879, #73668, #68230, #13724, #40319, #27234, #5193 ),
 .UNSPECIFIED., .F., .F.,
 ( 4, 2, 2, 2, 4 ),
 ( 0.0007817359527651104954, 0.0009771254036996493593, 0.001172514854634188223, 0.001367904305568727087, 0.001563293756503265951 ),
 .UNSPECIFIED. ) ;
#85942=ORIENTED_EDGE ( 'NONE', *, *, #26553, .F. ) ;
#85944=CARTESIAN_POINT ( 'NONE',  ( -5.207071046654770718, -9.504002272028875709, 34.60269587691767867 ) ) ;
#85945=CARTESIAN_POINT ( 'NONE',  ( -3.100243792535588572, -3.068774925481847493, 32.56582465632704526 ) ) ;
#85946=CARTESIAN_POINT ( 'NONE',  ( 13.38461538461538680, -11.16473453929635440, 33.15142922261926373 ) ) ;
#85947=CARTESIAN_POINT ( 'NONE',  ( -10.54931626438217585, -3.050289026998446840, 32.03036669348366416 ) ) ;
#85948=ORIENTED_EDGE ( 'NONE', *, *, #6200, .F. ) ;
#85949=AXIS2_PLACEMENT_3D ( 'NONE', #80053, #46271, #68314 ) ;
#85950=VERTEX_POINT ( 'NONE', #38382 ) ;
#85951=CARTESIAN_POINT ( 'NONE',  ( 10.61538461538493117, -2.255955759149395501, 30.00000000000324363 ) ) ;
#85954=CARTESIAN_POINT ( 'NONE',  ( 9.758376043310132530, -12.37446782046654192, 30.86335684631486842 ) ) ;
#85955=CARTESIAN_POINT ( 'NONE',  ( -8.769230769230768274, -12.37446782046654192, 30.86335684631486131 ) ) ;
#85956=CARTESIAN_POINT ( 'NONE',  ( -17.07692307692307665, -2.708943851104267164, 35.45975837776705220 ) ) ;
#85958=EDGE_LOOP ( 'NONE', ( #21477, #7886, #47446, #55552 ) ) ;
#85959=EDGE_LOOP ( 'NONE', ( #70816, #23715 ) ) ;
#85960=CARTESIAN_POINT ( 'NONE',  ( 15.00784301325307979, -2.554751324335735152, 30.48935550225260727 ) ) ;
#85961=EDGE_LOOP ( 'NONE', ( #34901, #72674 ) ) ;
#85962=ADVANCED_FACE ( 'NONE', ( #56872 ), #64068, .F. ) ;
#85964=CARTESIAN_POINT ( 'NONE',  ( -5.076923076923075762, -6.189225973068211317, 35.74407628777942847 ) ) ;
#85965=VECTOR ( 'NONE', #31273, 999.9999999999998863 ) ;
#85966=CARTESIAN_POINT ( 'NONE',  ( -0.3307480205715123689, -4.684288915650983043, 34.18129842949671371 ) ) ;
#85967=EDGE_LOOP ( 'NONE', ( #31545, #45876, #42473, #48370 ) ) ;
#85968=FACE_OUTER_BOUND ( 'NONE', #57211, .T. ) ;
#85969=B_SPLINE_CURVE_WITH_KNOTS ( 'NONE', 3,
 ( #20209, #67066, #5364, #60296, #47674, #67512, #74718, #87806, #13005, #40923 ),
 .UNSPECIFIED., .F., .F.,
 ( 4, 2, 2, 2, 4 ),
 ( 0.0007817246256747463051, 0.0009771112852218896347, 0.001172497944769032747, 0.001367884604316176077, 0.001563271263863319407 ),
 .UNSPECIFIED. ) ;
#85970=CARTESIAN_POINT ( 'NONE',  ( -1.449885830576159496, -8.613356846314824011, 34.62446782046655613 ) ) ;
#85971=FACE_OUTER_BOUND ( 'NONE', #33851, .T. ) ;
#85972=FACE_BOUND ( 'NONE', #8246, .T. ) ;
#85973=CARTESIAN_POINT ( 'NONE',  ( 14.98079249982687955, -5.728515186090277211, 34.42611988154120439 ) ) ;
#85974=CARTESIAN_POINT ( 'NONE',  ( 2.372947878968332258, -8.613356846314928816, 34.62446782046653482 ) ) ;
#85975=EDGE_CURVE ( 'NONE', #55112, #87599, #72156, .T. ) ;
#85976=CARTESIAN_POINT ( 'NONE',  ( 8.639083559792549494, -2.619462340734462380, 30.83744416345203021 ) ) ;
#85977=CARTESIAN_POINT ( 'NONE',  ( 17.30029901762125988, -2.501478030877322567, 29.88021232661721172 ) ) ;
#85978=CARTESIAN_POINT ( 'NONE',  ( 9.915319043920543862, -3.105924265160262543, 32.13625925475356127 ) ) ;
#85979=CARTESIAN_POINT ( 'NONE',  ( 11.53846153846141753, -11.48612834414049644, 32.76840700105863391 ) ) ;
#85980=CARTESIAN_POINT ( 'NONE',  ( 14.30769230769231015, -3.937682226553329556, 33.60647404775216529 ) ) ;
#85981=ORIENTED_EDGE ( 'NONE', *, *, #33885, .F. ) ;
#85983=DIRECTION ( 'NONE',  ( -1.000000000000000000, 0.000000000000000000, 0.000000000000000000 ) ) ;
#85985=LINE ( 'NONE', #58943, #73858 ) ;
#85987=VERTEX_POINT ( 'NONE', #29856 ) ;
#85988=CARTESIAN_POINT ( 'NONE',  ( 5.776515056276054771, -6.760086850603068243, 34.69517049084099369 ) ) ;
#85989=CARTESIAN_POINT ( 'NONE',  ( 10.83839745947800992, -12.64618726649961289, 30.78989965857442712 ) ) ;
#85990=CARTESIAN_POINT ( 'NONE',  ( -6.792551221313360088, -6.852161475712352789, 34.70806712695775786 ) ) ;
#85992=CARTESIAN_POINT ( 'NONE',  ( 1.319344938654610111, -11.94971097300153140, 32.03036669348370680 ) ) ;
#85993=ORIENTED_EDGE ( 'NONE', *, *, #46916, .F. ) ;
#85995=CARTESIAN_POINT ( 'NONE',  ( -9.692307692307691624, -4.098570777380720287, 33.41473453929634729 ) ) ;
#85996=DIRECTION ( 'NONE',  ( 1.000000000000000000, 0.000000000000000000, 0.000000000000000000 ) ) ;
#85997=EDGE_CURVE ( 'NONE', #69454, #31211, #53117, .T. ) ;
#85998=CARTESIAN_POINT ( 'NONE',  ( 0.4615384615383382183, -3.643525952248795718, 33.31231777344771672 ) ) ;
#85999=CARTESIAN_POINT ( 'NONE',  ( -16.82686865700962642, -2.544122305571458575, 31.48381861865057729 ) ) ;
#86001=ORIENTED_EDGE ( 'NONE', *, *, #66755, .F. ) ;
#86002=ORIENTED_EDGE ( 'NONE', *, *, #84118, .T. ) ;
#86004=CARTESIAN_POINT ( 'NONE',  ( 14.17700170458200759, -12.35290016733513951, 31.75349464988449455 ) ) ;
#86005=ORIENTED_EDGE ( 'NONE', *, *, #48444, .F. ) ;
#86007=CARTESIAN_POINT ( 'NONE',  ( 17.86985203026830860, -11.66186481527757479, 32.95055677023626117 ) ) ;
#86008=CARTESIAN_POINT ( 'NONE',  ( 14.53070365930515706, -2.758310577978208666, 31.33698337089302299 ) ) ;
#86009=CARTESIAN_POINT ( 'NONE',  ( 5.749999999999976907, -2.249999999999999112, 29.81609741502488120 ) ) ;
#86011=CARTESIAN_POINT ( 'NONE',  ( -11.60373153901785948, -9.528491918058357157, 34.59228464037090589 ) ) ;
#86012=LINE ( 'NONE', #24293, #77664 ) ;
#86013=EDGE_LOOP ( 'NONE', ( #17984, #61669, #43794, #24240 ) ) ;
#86014=VECTOR ( 'NONE', #88000, 1000.000000000000114 ) ;
#86015=LINE ( 'NONE', #43688, #74570 ) ;
#86016=CARTESIAN_POINT ( 'NONE',  ( 4.153846153846154188, -12.78798330534103123, 29.99999999999997868 ) ) ;
#86017=ORIENTED_EDGE ( 'NONE', *, *, #70552, .T. ) ;
#86018=CARTESIAN_POINT ( 'NONE',  ( -9.442307692307753797, -7.565270000091922853, 34.99999999999999289 ) ) ;
#86019=CARTESIAN_POINT ( 'NONE',  ( 3.230769230769231726, -2.721908614388771852, 31.22303859784724978 ) ) ;
#86020=CARTESIAN_POINT ( 'NONE',  ( -12.68446542044531000, -8.282780595021769443, 34.94152052738834158 ) ) ;
#86021=DIRECTION ( 'NONE',  ( 0.000000000000000000, 0.4999999999999985567, 0.8660254037844395958 ) ) ;
#86022=EDGE_CURVE ( 'NONE', #60060, #83375, #64951, .T. ) ;
#86023=CARTESIAN_POINT ( 'NONE',  ( -5.777220331021932331, -4.989023458446560255, 34.36081565061822118 ) ) ;
#86024=CARTESIAN_POINT ( 'NONE',  ( 9.468822767743363400, -4.988325925672468131, 34.36044203135681130 ) ) ;
#86025=CARTESIAN_POINT ( 'NONE',  ( 15.23076923076911093, -11.48612834414049644, 32.76840700105863391 ) ) ;
#86026=EDGE_CURVE ( 'NONE', #71998, #74779, #2803, .T. ) ;
#86028=EDGE_LOOP ( 'NONE', ( #19263, #40148, #7174, #83021 ) ) ;
#86029=CARTESIAN_POINT ( 'NONE',  ( -4.377331097570100304, -5.113361153441932316, 34.14387501736621999 ) ) ;
#86030=CARTESIAN_POINT ( 'NONE',  ( -12.23811149967689360, -7.630147231320743018, 34.74852402298682819 ) ) ;
#86031=DIRECTION ( 'NONE',  ( -0.000000000000000000, -0.7660444431189791237, -0.6427876096865379196 ) ) ;
#86033=EDGE_CURVE ( 'NONE', #41851, #34671, #30368, .T. ) ;
#86034=CARTESIAN_POINT ( 'NONE',  ( 13.60762673622823726, -4.887748414852792322, 34.01359900205216746 ) ) ;
#86035=CARTESIAN_POINT ( 'NONE',  ( 2.438482748659257737, -11.93129842949671726, 32.56571108434900452 ) ) ;
#86036=EDGE_CURVE ( 'NONE', #37000, #77161, #49925, .T. ) ;
#86037=CARTESIAN_POINT ( 'NONE',  ( 12.39545505058258001, -10.51840700105979387, 33.73612834413961536 ) ) ;
#86038=ORIENTED_EDGE ( 'NONE', *, *, #63400, .T. ) ;
#86040=CARTESIAN_POINT ( 'NONE',  ( -1.134669975237340589, -12.45601412856602686, 31.48342859153981621 ) ) ;
#86041=VERTEX_POINT ( 'NONE', #38836 ) ;
#86042=CARTESIAN_POINT ( 'NONE',  ( -18.06527000055631760, -5.094484230520675894, 34.41647553114621161 ) ) ;
#86043=ORIENTED_EDGE ( 'NONE', *, *, #82314, .T. ) ;
#86044=CARTESIAN_POINT ( 'NONE',  ( -18.06608341095587278, -11.69971097300155272, 32.46337939537587403 ) ) ;
#86045=CARTESIAN_POINT ( 'NONE',  ( -15.23076923076922995, -2.833524468853757305, 32.15551576947925838 ) ) ;
#86046=CARTESIAN_POINT ( 'NONE',  ( -12.46153846153846168, -6.189225973068211317, 35.74407628777942847 ) ) ;
#86048=CARTESIAN_POINT ( 'NONE',  ( -0.6844047246015609876, -2.251424796025575770, 29.88072029997477586 ) ) ;
#86049=ORIENTED_EDGE ( 'NONE', *, *, #19152, .F. ) ;
#86050=CARTESIAN_POINT ( 'NONE',  ( 11.47237812750565666, -3.513871655860377086, 32.76840700105978499 ) ) ;
#86051=AXIS2_PLACEMENT_3D ( 'NONE', #45993, #10443, #58168 ) ;
#86052=ORIENTED_EDGE ( 'NONE', *, *, #49875, .F. ) ;
#86053=CARTESIAN_POINT ( 'NONE',  ( 13.45068373561782593, -11.69971097300155272, 32.46337939537588113 ) ) ;
#86055=EDGE_LOOP ( 'NONE', ( #75163, #9504 ) ) ;
#86058=CYLINDRICAL_SURFACE ( 'NONE', #76619, 0.2499999999999995559 ) ;
#86059=CARTESIAN_POINT ( 'NONE',  ( -11.53846153846153655, -2.833524468853757305, 32.15551576947925838 ) ) ;
#86060=CARTESIAN_POINT ( 'NONE',  ( 4.946775867484854317, -9.418419913701741919, 34.36755862841477693 ) ) ;
#86061=CARTESIAN_POINT ( 'NONE',  ( -8.069638770718176701, -12.69144148231606017, 30.53333754910549303 ) ) ;
#86062=B_SPLINE_CURVE_WITH_KNOTS ( 'NONE', 3,
 ( #86798, #32276, #66947, #74147, #12443, #67388, #47991, #21416, #62385, #75470 ),
 .UNSPECIFIED., .F., .F.,
 ( 4, 2, 2, 2, 4 ),
 ( 0.000000000000000000, 0.0001954339881912774883, 0.0003908679763825549766, 0.0005863019645738324920, 0.0007817359527651099533 ),
 .UNSPECIFIED. ) ;
#86063=ADVANCED_FACE ( 'NONE', ( #5936 ), #81597, .F. ) ;
#86064=ORIENTED_EDGE ( 'NONE', *, *, #14001, .T. ) ;
#86065=ORIENTED_EDGE ( 'NONE', *, *, #83880, .T. ) ;
#86067=CARTESIAN_POINT ( 'NONE',  ( 3.480714640147274608, -12.68172785388650681, 30.59649109432439218 ) ) ;
#86068=VERTEX_POINT ( 'NONE', #31626 ) ;
#86069=AXIS2_PLACEMENT_3D ( 'NONE', #46670, #26404, #33157 ) ;
#86070=CARTESIAN_POINT ( 'NONE',  ( -14.24162497434223162, -10.67929555188718282, 33.92786785259544757 ) ) ;
#86071=DIRECTION ( 'NONE',  ( -0.000000000000000000, 0.5000000000000011102, -0.8660254037844380415 ) ) ;
#86072=B_SPLINE_CURVE_WITH_KNOTS ( 'NONE', 3,
 ( #47820, #61764, #14931, #27553, #1407, #28896, #83842, #20788, #41510, #62217 ),
 .UNSPECIFIED., .F., .F.,
 ( 4, 2, 2, 2, 4 ),
 ( 0.000000000000000000, 0.0001954339857564073388, 0.0003908679715128146777, 0.0005863019572692220165, 0.0007817359430256293554 ),
 .UNSPECIFIED. ) ;
#86074=ORIENTED_EDGE ( 'NONE', *, *, #44718, .T. ) ;
#86075=EDGE_CURVE ( 'NONE', #60370, #22188, #57421, .T. ) ;
#86076=VECTOR ( 'NONE', #57577, 1000.000000000000227 ) ;
#86077=ORIENTED_EDGE ( 'NONE', *, *, #70539, .T. ) ;
#86078=CARTESIAN_POINT ( 'NONE',  ( -10.68146802634049486, -3.050289026998445951, 32.03036669348365706 ) ) ;
#86079=VERTEX_POINT ( 'NONE', #80723 ) ;
#86080=AXIS2_PLACEMENT_3D ( 'NONE', #3583, #63516, #36067 ) ;
#86083=CARTESIAN_POINT ( 'NONE',  ( 5.076923076922954969, -5.219633306517616589, 34.19971097300220464 ) ) ;
#86084=CARTESIAN_POINT ( 'NONE',  ( -2.307692307692305711, -9.058645607665452459, 34.76329471203371924 ) ) ;
#86085=FACE_BOUND ( 'NONE', #70565, .T. ) ;
#86086=VERTEX_POINT ( 'NONE', #59982 ) ;
#86088=CARTESIAN_POINT ( 'NONE',  ( 13.25392478150507891, -10.70098750199973203, 33.91152734681376302 ) ) ;
#86089=ADVANCED_FACE ( 'NONE', ( #53671 ), #86588, .F. ) ;
#86090=CARTESIAN_POINT ( 'NONE',  ( 4.284371855609716562, -8.586989748646452369, 34.63063291749215011 ) ) ;
#86091=CARTESIAN_POINT ( 'NONE',  ( -6.923076923076922462, -13.49023893513002648, 31.06009739812518688 ) ) ;
#86093=ORIENTED_EDGE ( 'NONE', *, *, #88787, .T. ) ;
#86095=EDGE_CURVE ( 'NONE', #21493, #63786, #73511, .T. ) ;
#86096=EDGE_LOOP ( 'NONE', ( #1508, #31630, #2447, #27966 ) ) ;
#86097=ORIENTED_EDGE ( 'NONE', *, *, #29147, .F. ) ;
#86098=CARTESIAN_POINT ( 'NONE',  ( 10.74591031714818357, -12.45806712695776319, 30.39783852428763922 ) ) ;
#86099=LINE ( 'NONE', #30696, #77922 ) ;
#86100=CARTESIAN_POINT ( 'NONE',  ( 6.923076923076924238, -6.386643153685126251, 34.62446782046654192 ) ) ;
#86102=CARTESIAN_POINT ( 'NONE',  ( 1.384615384615265343, -10.21337939537710326, 33.94971097300076224 ) ) ;
#86103=CARTESIAN_POINT ( 'NONE',  ( -15.45369618967607828, -3.395401636524185474, 33.02366814457250399 ) ) ;
#86104=ORIENTED_EDGE ( 'NONE', *, *, #84415, .F. ) ;
#86105=CYLINDRICAL_SURFACE ( 'NONE', #87485, 0.2499999999999995559 ) ;
#86106=CARTESIAN_POINT ( 'NONE',  ( -11.60373198442231590, -10.21337939537584383, 33.94971097300158647 ) ) ;
#86107=CARTESIAN_POINT ( 'NONE',  ( 2.372947447205147053, -12.70778746994558439, 30.41441678777536595 ) ) ;
#86108=EDGE_CURVE ( 'NONE', #603, #75030, #34932, .T. ) ;
#86109=CARTESIAN_POINT ( 'NONE',  ( 14.30769230769231015, -2.486705287966279876, 31.30864560766543647 ) ) ;
#86110=VERTEX_POINT ( 'NONE', #60871 ) ;
#86112=VERTEX_POINT ( 'NONE', #19884 ) ;
#86113=FACE_BOUND ( 'NONE', #33474, .T. ) ;
#86115=ORIENTED_EDGE ( 'NONE', *, *, #33892, .F. ) ;
#86116=EDGE_CURVE ( 'NONE', #67105, #37924, #15642, .T. ) ;
#86117=CARTESIAN_POINT ( 'NONE',  ( 11.76147438255493149, -12.38742843783360748, 31.66772728687926985 ) ) ;
#86118=CARTESIAN_POINT ( 'NONE',  ( 13.38461538461538680, -13.49023893513002648, 31.06009739812518688 ) ) ;
#86119=ORIENTED_EDGE ( 'NONE', *, *, #25044, .T. ) ;
#86120=EDGE_CURVE ( 'NONE', #17692, #42554, #66026, .T. ) ;
#86121=CARTESIAN_POINT ( 'NONE',  ( -16.40382289789473802, -11.47974371597207899, 33.17467449705390692 ) ) ;
#86122=CARTESIAN_POINT ( 'NONE',  ( -17.07692307692307665, -1.129524287112498415, 32.06866353760679544 ) ) ;
#86123=CARTESIAN_POINT ( 'NONE',  ( -8.096177083446809419, -11.86270091957321249, 32.19358267280087915 ) ) ;
#86124=CARTESIAN_POINT ( 'NONE',  ( 4.403791563224197070, -6.653508905675592722, 34.93172785388651391 ) ) ;
#86125=ORIENTED_EDGE ( 'NONE', *, *, #77950, .F. ) ;
#86126=CARTESIAN_POINT ( 'NONE',  ( -11.28840722682322273, -9.148310452688876993, 34.47095581063188519 ) ) ;
#86127=ORIENTED_EDGE ( 'NONE', *, *, #27895, .T. ) ;
#86128=CARTESIAN_POINT ( 'NONE',  ( 22.75000000000000000, -10.49999999999999822, 27.25000000000000000 ) ) ;
#86129=EDGE_LOOP ( 'NONE', ( #39459, #14830, #61062, #26951 ) ) ;
#86130=CARTESIAN_POINT ( 'NONE',  ( -8.769230769230768274, -13.53365097954675988, 30.81389545987213552 ) ) ;
#86132=CARTESIAN_POINT ( 'NONE',  ( -17.07692307692307665, -7.500000000000001776, 35.04278698407183867 ) ) ;
#86133=CARTESIAN_POINT ( 'NONE',  ( 10.39245765647776309, -12.38737895849757820, 31.66785238281580206 ) ) ;
#86135=EDGE_CURVE ( 'NONE', #83826, #46850, #59672, .T. ) ;
#86136=CARTESIAN_POINT ( 'NONE',  ( -9.942284436356281674, -12.01397095200674059, 32.43157075238190146 ) ) ;
#86138=ORIENTED_EDGE ( 'NONE', *, *, #4714, .T. ) ;
#86139=CARTESIAN_POINT ( 'NONE',  ( 10.61538461538461675, -13.78497067705608181, 32.30358669280327177 ) ) ;
#86140=CARTESIAN_POINT ( 'NONE',  ( 7.715544190949763070, -7.722926974430166069, 34.99546784045486447 ) ) ;
#86141=DIRECTION ( 'NONE',  ( 0.000000000000000000, 0.4999999999999985567, 0.8660254037844395958 ) ) ;
#86142=EDGE_CURVE ( 'NONE', #82006, #9304, #82927, .T. ) ;
#86144=ORIENTED_EDGE ( 'NONE', *, *, #87272, .F. ) ;
#86145=ADVANCED_FACE ( 'NONE', ( #27532 ), #22105, .F. ) ;
#86147=CARTESIAN_POINT ( 'NONE',  ( 9.692307692307570832, -3.643525952248795718, 33.31231777344771672 ) ) ;
#86148=CARTESIAN_POINT ( 'NONE',  ( 11.47237915910140771, -4.661471528628507777, 34.16647553114621871 ) ) ;
#86149=CARTESIAN_POINT ( 'NONE',  ( 17.32697749683652688, -3.435999193479609026, 33.07426656108011542 ) ) ;
#86150=VECTOR ( 'NONE', #49512, 1000.000000000000227 ) ;
#86151=CARTESIAN_POINT ( 'NONE',  ( -8.769230769230892619, -12.51329471203414379, 31.30864560766407578 ) ) ;
#86152=CARTESIAN_POINT ( 'NONE',  ( 13.16113046005105502, -3.019605429927184392, 32.48692288466676814 ) ) ;
#86153=CARTESIAN_POINT ( 'NONE',  ( 16.40379156322419973, -3.520799739797213501, 33.17531984108286025 ) ) ;
#86155=ORIENTED_EDGE ( 'NONE', *, *, #67025, .F. ) ;
#86156=CARTESIAN_POINT ( 'NONE',  ( -16.15384615384583711, -2.255955759149395501, 30.00000000000324363 ) ) ;
#86157=CARTESIAN_POINT ( 'NONE',  ( -17.20707028636130076, -12.27039167877662251, 31.24851455888617835 ) ) ;
#86158=AXIS2_PLACEMENT_3D ( 'NONE', #20084, #47097, #31834 ) ;
#86159=B_SPLINE_CURVE_WITH_KNOTS ( 'NONE', 3,
 ( #6460, #60947, #52854, #20415, #73598, #41130, #74922, #5123, #26722, #19960 ),
 .UNSPECIFIED., .F., .F.,
 ( 4, 2, 2, 2, 4 ),
 ( 0.000000000000000000, 0.0001954311564186879044, 0.0003908623128373758088, 0.0005862934692560636861, 0.0007817246256747516176 ),
 .UNSPECIFIED. ) ;
#86160=FACE_OUTER_BOUND ( 'NONE', #36539, .T. ) ;
#86161=EDGE_CURVE ( 'NONE', #55341, #49579, #49576, .T. ) ;
#86162=CARTESIAN_POINT ( 'NONE',  ( 16.94623161025551639, -8.999036380462719364, 34.52022231692819076 ) ) ;
#86163=B_SPLINE_CURVE_WITH_KNOTS ( 'NONE', 3,
 ( #27272, #32267, #80908, #34027, #20515, #19192 ),
 .UNSPECIFIED., .F., .F.,
 ( 4, 2, 4 ),
 ( 0.0003909569690057804843, 0.0005862646681846042955, 0.0007815723673634281067 ),
 .UNSPECIFIED. ) ;
#86164=ORIENTED_EDGE ( 'NONE', *, *, #55764, .F. ) ;
#86165=CARTESIAN_POINT ( 'NONE',  ( 16.02369818411445479, -12.50552854090298638, 31.33409797877408920 ) ) ;
#86166=B_SPLINE_CURVE_WITH_KNOTS ( 'NONE', 3,
 ( #38370, #72591, #31613, #9999, #66280, #31153, #43787, #86574, #65823, #18106 ),
 .UNSPECIFIED., .F., .F.,
 ( 4, 2, 2, 2, 4 ),
 ( 0.0007817359430256313069, 0.0009771253907249971907, 0.001172514838424363291, 0.001367904286123729175, 0.001563293733823095059 ),
 .UNSPECIFIED. ) ;
#86167=VERTEX_POINT ( 'NONE', #68511 ) ;
#86168=CARTESIAN_POINT ( 'NONE',  ( 9.019176178608812933, -2.986452184633680673, 32.43230066228895225 ) ) ;
#86169=LINE ( 'NONE', #45606, #67126 ) ;
#86170=EDGE_CURVE ( 'NONE', #68861, #23595, #42391, .T. ) ;
#86171=DIRECTION ( 'NONE',  ( -0.000000000000000000, 0.8660254037844397068, -0.4999999999999978906 ) ) ;
#86173=CARTESIAN_POINT ( 'NONE',  ( 8.703960323269994248, -10.90142922261923886, 33.41473453929638993 ) ) ;
#86174=DIRECTION ( 'NONE',  ( -0.000000000000000000, 1.000000000000000000, -0.000000000000000000 ) ) ;
#86176=CARTESIAN_POINT ( 'NONE',  ( -6.130690603110307002, -5.496505350115500121, 34.60290016733514307 ) ) ;
#86177=CARTESIAN_POINT ( 'NONE',  ( 3.230769230769108269, -3.083524468854526912, 32.58852847137268327 ) ) ;
#86178=EDGE_CURVE ( 'NONE', #7803, #51057, #68283, .T. ) ;
#86179=EDGE_LOOP ( 'NONE', ( #60666, #88974 ) ) ;
#86180=LINE ( 'NONE', #72645, #52949 ) ;
#86181=ORIENTED_EDGE ( 'NONE', *, *, #54312, .T. ) ;
#86182=CARTESIAN_POINT ( 'NONE',  ( -2.531177232256639709, -2.612411019501189813, 31.66733052389439962 ) ) ;
#86184=EDGE_CURVE ( 'NONE', #42382, #82187, #84409, .T. ) ;
#86185=DIRECTION ( 'NONE',  ( 0.000000000000000000, 0.9848077530122072432, -0.1736481776669354937 ) ) ;
#86186=ADVANCED_FACE ( 'NONE', ( #41051 ), #83822, .F. ) ;
#86187=CARTESIAN_POINT ( 'NONE',  ( -0.2387587925603970040, -2.612705202774697977, 31.66806509827799943 ) ) ;
#86188=CARTESIAN_POINT ( 'NONE',  ( 9.692307692307570832, -2.657715359629662544, 31.77849191805970364 ) ) ;
#86189=CARTESIAN_POINT ( 'NONE',  ( 7.053602624840485724, -10.19071101563364756, 33.96452234770658407 ) ) ;
#86190=CARTESIAN_POINT ( 'NONE',  ( 9.692307692307695177, -8.120952969808772792, 34.71129190930000163 ) ) ;
#86191=B_SPLINE_CURVE_WITH_KNOTS ( 'NONE', 3,
 ( #88464, #25853, #26734, #61839, #32601, #6471, #60069, #54195, #46563, #74046 ),
 .UNSPECIFIED., .F., .F.,
 ( 4, 2, 2, 2, 4 ),
 ( 0.0007817246256747434861, 0.0009771112852218861652, 0.001172497944769028844, 0.001367884604316171740, 0.001563271263863314419 ),
 .UNSPECIFIED. ) ;
#86192=ORIENTED_EDGE ( 'NONE', *, *, #84527, .T. ) ;
#86194=ORIENTED_EDGE ( 'NONE', *, *, #39214, .T. ) ;
#86195=B_SPLINE_CURVE_WITH_KNOTS ( 'NONE', 3,
 ( #50160, #42984, #51038, #1110, #77649, #64121, #63689, #78530, #7870, #15961 ),
 .UNSPECIFIED., .F., .F.,
 ( 4, 2, 2, 2, 4 ),
 ( 0.000000000000000000, 0.0001954311564186879857, 0.0003908623128373759715, 0.0005862934692560640114, 0.0007817246256747519429 ),
 .UNSPECIFIED. ) ;
#86197=B_SPLINE_CURVE_WITH_KNOTS ( 'NONE', 3,
 ( #37505, #64973, #30749, #41292, #7053, #38405, #58664, #73532, #17239, #85709 ),
 .UNSPECIFIED., .F., .F.,
 ( 4, 2, 2, 2, 4 ),
 ( 0.000000000000000000, 0.0001954311584214072923, 0.0003908623168428145846, 0.0005862934752642218498, 0.0007817246336856291692 ),
 .UNSPECIFIED. ) ;
#86200=CARTESIAN_POINT ( 'NONE',  ( -12.71153846153847233, -2.249999999999999556, 29.81609741502489541 ) ) ;
#86201=CARTESIAN_POINT ( 'NONE',  ( 16.15384615384615330, -12.10708131394839349, 31.69288490824020244 ) ) ;
#86202=CARTESIAN_POINT ( 'NONE',  ( 15.10062202133100939, -5.195881422630166391, 34.18770438780619259 ) ) ;
#86204=CARTESIAN_POINT ( 'NONE',  ( -13.63463860883683942, -3.520140089381495585, 33.17453946501458262 ) ) ;
#86205=CARTESIAN_POINT ( 'NONE',  ( 0.6845498131513101381, -4.887748414852792322, 34.01359900205216746 ) ) ;
#86207=CARTESIAN_POINT ( 'NONE',  ( -2.307692307692305711, -11.11383981884818262, 36.00935417666054406 ) ) ;
#86208=CARTESIAN_POINT ( 'NONE',  ( 9.442330948259101575, -10.06842814019191401, 34.32929386961144758 ) ) ;
#86209=DIRECTION ( 'NONE',  ( -0.000000000000000000, -0.9848077530122086864, -0.1736481776669273613 ) ) ;
#86210=ORIENTED_EDGE ( 'NONE', *, *, #31917, .F. ) ;
#86211=EDGE_CURVE ( 'NONE', #48549, #37467, #75767, .T. ) ;
#86212=EDGE_LOOP ( 'NONE', ( #37524, #68995, #24361, #20478 ) ) ;
#86213=ORIENTED_EDGE ( 'NONE', *, *, #43610, .T. ) ;
#86215=CARTESIAN_POINT ( 'NONE',  ( 0.3313904918067617777, -3.069018819979302926, 32.56621877034667278 ) ) ;
#86216=ORIENTED_EDGE ( 'NONE', *, *, #10056, .T. ) ;
#86217=CARTESIAN_POINT ( 'NONE',  ( 7.780070435197966816, -3.050289026998445951, 32.03036669348365706 ) ) ;
#86218=FACE_OUTER_BOUND ( 'NONE', #23908, .T. ) ;
#86219=VECTOR ( 'NONE', #49693, 999.9999999999998863 ) ;
#86220=CARTESIAN_POINT ( 'NONE',  ( -1.384615384615506484, -5.094484230521993062, 34.41647553114689373 ) ) ;
#86221=CARTESIAN_POINT ( 'NONE',  ( -14.37377571864818648, -9.780366693483667717, 34.19971097300155805 ) ) ;
#86222=ORIENTED_EDGE ( 'NONE', *, *, #41170, .F. ) ;
#86225=ORIENTED_EDGE ( 'NONE', *, *, #61538, .F. ) ;
#86226=FACE_BOUND ( 'NONE', #71992, .T. ) ;
#86227=B_SPLINE_CURVE_WITH_KNOTS ( 'NONE', 3,
 ( #45882, #81022, #74257, #53974, #67501, #6246, #75148, #11671, #46780, #39149 ),
 .UNSPECIFIED., .F., .F.,
 ( 4, 2, 2, 2, 4 ),
 ( 0.000000000000000000, 0.0001954311564186871184, 0.0003908623128373742367, 0.0005862934692560614093, 0.0007817246256747484735 ),
 .UNSPECIFIED. ) ;
#86228=CARTESIAN_POINT ( 'NONE',  ( 15.16549878480845770, -10.21337939537584383, 33.94971097300158647 ) ) ;
#86229=CARTESIAN_POINT ( 'NONE',  ( -0.4615384615384611200, -3.886160181151819604, 36.00935417666054406 ) ) ;
#86231=CARTESIAN_POINT ( 'NONE',  ( 14.17754509825408960, -2.882441371585227508, 31.66841991370172238 ) ) ;
#86232=CARTESIAN_POINT ( 'NONE',  ( 6.000000000000001776, -2.249999999999998668, 29.50000000000001421 ) ) ;
#86233=DIRECTION ( 'NONE',  ( -0.000000000000000000, -0.9396926207859092051, -0.3420201433256662704 ) ) ;
#86234=ORIENTED_EDGE ( 'NONE', *, *, #41630, .T. ) ;
#86235=CARTESIAN_POINT ( 'NONE',  ( -11.78848476268299628, -4.931416488878822335, 34.32920672191015399 ) ) ;
#86236=CARTESIAN_POINT ( 'NONE',  ( 20.99999999999999645, -4.249999999999998224, 29.75000000000000355 ) ) ;
#86238=CARTESIAN_POINT ( 'NONE',  ( -6.923076923076922462, -8.973038597847269315, 34.52809138561121927 ) ) ;
#86241=CARTESIAN_POINT ( 'NONE',  ( -12.71156168575991963, -5.765609946408404518, 34.70566812827425451 ) ) ;
#86242=CYLINDRICAL_SURFACE ( 'NONE', #22459, 0.2499999999999998890 ) ;
#86243=LINE ( 'NONE', #24962, #78477 ) ;
#86244=B_SPLINE_CURVE_WITH_KNOTS ( 'NONE', 3,
 ( #47667, #75152, #33713, #26960, #88683, #81913, #27398, #13437, #20633, #40915 ),
 .UNSPECIFIED., .F., .F.,
 ( 4, 2, 2, 2, 4 ),
 ( 0.0007817246256747507503, 0.0009771112852218957062, 0.001172497944769040771, 0.001367884604316185835, 0.001563271263863330682 ),
 .UNSPECIFIED. ) ;
#86245=LINE ( 'NONE', #39389, #45748 ) ;
#86246=DIRECTION ( 'NONE',  ( -0.000000000000000000, 0.1736481776669307198, -0.9848077530122080203 ) ) ;
#86247=CARTESIAN_POINT ( 'NONE',  ( 6.699591979352975457, -9.331801661448606566, 34.40259984581193464 ) ) ;
#86250=EDGE_CURVE ( 'NONE', #49638, #10, #87612, .T. ) ;
#86251=DIRECTION ( 'NONE',  ( -0.000000000000000000, 0.9396926207859093161, -0.3420201433256663259 ) ) ;
#86252=CARTESIAN_POINT ( 'NONE',  ( 3.165519298995146613, -2.255955759149247619, 30.00000000000013856 ) ) ;
#86253=DIRECTION ( 'NONE',  ( 0.000000000000000000, 0.9396926207859126468, 0.3420201433256571111 ) ) ;
#86254=AXIS2_PLACEMENT_3D ( 'NONE', #39277, #46015, #18111 ) ;
#86256=ORIENTED_EDGE ( 'NONE', *, *, #41024, .F. ) ;
#86257=CARTESIAN_POINT ( 'NONE',  ( 0.2115617305961065009, -12.41269422305637171, 30.68257228309993323 ) ) ;
#86258=VERTEX_POINT ( 'NONE', #1826 ) ;
#86259=EDGE_CURVE ( 'NONE', #36333, #29450, #14515, .T. ) ;
#86261=DIRECTION ( 'NONE',  ( -0.000000000000000000, 1.000000000000000000, 3.491481338843133355E-15 ) ) ;
#86263=ORIENTED_EDGE ( 'NONE', *, *, #8237, .T. ) ;
#86264=CARTESIAN_POINT ( 'NONE',  ( 14.30769230769231015, -4.661471528628507777, 34.16647553114623292 ) ) ;
#86266=CARTESIAN_POINT ( 'NONE',  ( -17.93393164899756087, -5.557115091759784242, 34.35708131394839882 ) ) ;
#86267=LINE ( 'NONE', #37162, #48171 ) ;
#86268=B_SPLINE_CURVE_WITH_KNOTS ( 'NONE', 3,
 ( #22738, #43903, #64602, #50199, #2900, #30392, #57861, #23629, #51080, #78574 ),
 .UNSPECIFIED., .F., .F.,
 ( 4, 2, 2, 2, 4 ),
 ( 0.0007817246256747439198, 0.0009771112852218863821, 0.001172497944769028844, 0.001367884604316171307, 0.001563271263863313769 ),
 .UNSPECIFIED. ) ;
#86269=CARTESIAN_POINT ( 'NONE',  ( -5.999999999999998224, -8.973038597847269315, 34.52809138561121927 ) ) ;
#86271=DIRECTION ( 'NONE',  ( -0.000000000000000000, -0.000000000000000000, -1.000000000000000000 ) ) ;
#86272=FACE_OUTER_BOUND ( 'NONE', #23487, .T. ) ;
#86273=LINE ( 'NONE', #45707, #33874 ) ;
#86274=ADVANCED_FACE ( 'NONE', ( #84265 ), #71163, .F. ) ;
#86276=CARTESIAN_POINT ( 'NONE',  ( -11.40767109749458541, -2.494656445102012565, 31.33466734024120015 ) ) ;
#86277=CARTESIAN_POINT ( 'NONE',  ( -2.307692307692428724, -12.16647553114689728, 32.15551576947799362 ) ) ;
#86279=CARTESIAN_POINT ( 'NONE',  ( 10.54930223602447903, -5.471508081941602875, 34.59228464037088457 ) ) ;
#86280=VECTOR ( 'NONE', #50311, 999.9999999999998863 ) ;
#86281=CIRCLE ( 'NONE', #74765, 0.2500000000000002220 ) ;
#86282=ORIENTED_EDGE ( 'NONE', *, *, #28924, .T. ) ;
#86283=ORIENTED_EDGE ( 'NONE', *, *, #24612, .T. ) ;
#86284=CARTESIAN_POINT ( 'NONE',  ( -17.07692307692307665, -9.058645607665452459, 34.76329471203371924 ) ) ;
#86285=DIRECTION ( 'NONE',  ( -0.000000000000000000, -0.9396926207859093161, -0.3420201433256663259 ) ) ;
#86286=PLANE ( 'NONE',  #71335 ) ;
#86288=VECTOR ( 'NONE', #66521, 1000.000000000000114 ) ;
#86289=CARTESIAN_POINT ( 'NONE',  ( 17.29970274590113632, -12.47679350104403007, 31.42216943046555855 ) ) ;
#86291=CIRCLE ( 'NONE', #10072, 0.2500000000000002220 ) ;
#86292=VERTEX_POINT ( 'NONE', #2255 ) ;
#86293=DIRECTION ( 'NONE',  ( -0.000000000000000000, -0.7660444431189791237, -0.6427876096865379196 ) ) ;
#86294=ORIENTED_EDGE ( 'NONE', *, *, #17173, .F. ) ;
#86295=EDGE_CURVE ( 'NONE', #61423, #14452, #39098, .T. ) ;
#86296=VERTEX_POINT ( 'NONE', #2695 ) ;
#86297=FACE_OUTER_BOUND ( 'NONE', #67107, .T. ) ;
#86298=CARTESIAN_POINT ( 'NONE',  ( 5.207714884747860928, -11.71459661697925903, 32.44059661609676937 ) ) ;
#86299=LINE ( 'NONE', #52036, #77514 ) ;
#86300=CARTESIAN_POINT ( 'NONE',  ( 6.130790440966952026, -8.191423895709842640, 34.95447573519442130 ) ) ;
#86301=CARTESIAN_POINT ( 'NONE',  ( 13.38461538461526423, -8.656820664282941280, 34.87096338111179961 ) ) ;
#86302=ORIENTED_EDGE ( 'NONE', *, *, #37848, .T. ) ;
#86303=EDGE_CURVE ( 'NONE', #1161, #77202, #9909, .T. ) ;
#86304=EDGE_LOOP ( 'NONE', ( #64912, #65299, #67372, #22276 ) ) ;
#86306=EDGE_CURVE ( 'NONE', #52068, #28470, #7376, .T. ) ;
#86307=CARTESIAN_POINT ( 'NONE',  ( -4.153846153846274980, -12.16647553114689728, 32.15551576947799362 ) ) ;
#86308=CARTESIAN_POINT ( 'NONE',  ( -0.3307480205715118693, -9.929761469519744921, 34.40412654351204225 ) ) ;
#86310=CARTESIAN_POINT ( 'NONE',  ( -14.30769230769230660, -2.517432740324522911, 35.29906147534542527 ) ) ;
#86311=B_SPLINE_CURVE_WITH_KNOTS ( 'NONE', 3,
 ( #62625, #83815, #82036, #27078, #497, #1378, #61290, #48671, #62190, #22098 ),
 .UNSPECIFIED., .F., .F.,
 ( 4, 2, 2, 2, 4 ),
 ( 0.0007817359430256303312, 0.0009771253907249965402, 0.001172514838424362641, 0.001367904286123728958, 0.001563293733823095059 ),
 .UNSPECIFIED. ) ;
#86312=CARTESIAN_POINT ( 'NONE',  ( 10.54930223602447903, -4.661471528628507777, 34.16647553114621871 ) ) ;
#86313=CARTESIAN_POINT ( 'NONE',  ( 11.40777093535123399, -10.70098750199973203, 33.91152734681376302 ) ) ;
#86314=DIRECTION ( 'NONE',  ( 0.000000000000000000, 0.7660444431189822323, -0.6427876096865344779 ) ) ;
#86316=ADVANCED_FACE ( 'NONE', ( #65293 ), #3590, .F. ) ;
#86319=ORIENTED_EDGE ( 'NONE', *, *, #69545, .F. ) ;
#86320=CARTESIAN_POINT ( 'NONE',  ( -16.15384615384627409, -8.656820664282941280, 34.87096338111179961 ) ) ;
#86321=VERTEX_POINT ( 'NONE', #24758 ) ;
#86322=CARTESIAN_POINT ( 'NONE',  ( -10.61538461538461320, -3.937682226553329556, 33.60647404775216529 ) ) ;
#86323=CARTESIAN_POINT ( 'NONE',  ( -9.942284423250045577, -11.79746400365624659, 32.30657167506340954 ) ) ;
#86324=EDGE_CURVE ( 'NONE', #30568, #69653, #59490, .T. ) ;
#86325=EDGE_CURVE ( 'NONE', #59481, #33850, #39628, .T. ) ;
#86327=ORIENTED_EDGE ( 'NONE', *, *, #31261, .F. ) ;
#86328=B_SPLINE_CURVE_WITH_KNOTS ( 'NONE', 3,
 ( #66396, #60076, #80372, #86694, #73620, #38486, #52872, #74489, #5143, #26301 ),
 .UNSPECIFIED., .F., .F.,
 ( 4, 2, 2, 2, 4 ),
 ( 0.000000000000000000, 0.0001954339857564073931, 0.0003908679715128147861, 0.0005863019572692222334, 0.0007817359430256295722 ),
 .UNSPECIFIED. ) ;
#86329=AXIS2_PLACEMENT_3D ( 'NONE', #14111, #83017, #36169 ) ;
#86330=CARTESIAN_POINT ( 'NONE',  ( 18.00000000000000000, -9.058645607665452459, 34.76329471203371924 ) ) ;
#86332=EDGE_CURVE ( 'NONE', #57709, #11427, #46584, .T. ) ;
#86334=CARTESIAN_POINT ( 'NONE',  ( 17.74997677577854205, -12.68155406624981119, 30.59749803192733708 ) ) ;
#86335=CARTESIAN_POINT ( 'NONE',  ( 7.846153846153846700, -3.937682226553329556, 33.60647404775216529 ) ) ;
#86336=DIRECTION ( 'NONE',  ( 1.000000000000000000, 0.000000000000000000, 0.000000000000000000 ) ) ;
#86337=VECTOR ( 'NONE', #26430, 1000.000000000000000 ) ;
#86340=CARTESIAN_POINT ( 'NONE',  ( -0.7115616857599191825, -12.45566812827425096, 31.48439005359158926 ) ) ;
#86342=VERTEX_POINT ( 'NONE', #46809 ) ;
#86343=CARTESIAN_POINT ( 'NONE',  ( 11.31553457955469000, -11.43668979543634734, 33.22377378376089752 ) ) ;
#86344=CARTESIAN_POINT ( 'NONE',  ( 8.769230769230647482, -6.879047030192662504, 34.71129190930017927 ) ) ;
#86345=AXIS2_PLACEMENT_3D ( 'NONE', #842, #42724, #43159 ) ;
#86347=VECTOR ( 'NONE', #52612, 1000.000000000000227 ) ;
#86348=CARTESIAN_POINT ( 'NONE',  ( 6.856993512121043466, -5.557115091759785130, 34.35708131394839171 ) ) ;
#86349=CARTESIAN_POINT ( 'NONE',  ( 10.39245839786846837, -6.503392248772476236, 34.64988816332204635 ) ) ;
#86350=CARTESIAN_POINT ( 'NONE',  ( -14.98071481085577972, -5.642605341092957971, 34.66089969410670335 ) ) ;
#86351=CARTESIAN_POINT ( 'NONE',  ( 7.846153846153846700, -3.937682226553329556, 33.60647404775216529 ) ) ;
#86353=FACE_BOUND ( 'NONE', #53395, .T. ) ;
#86354=CARTESIAN_POINT ( 'NONE',  ( 5.326977496836529546, -5.642605341092957083, 34.66089969410670335 ) ) ;
#86355=CYLINDRICAL_SURFACE ( 'NONE', #20101, 0.2500000000000009437 ) ;
#86356=CARTESIAN_POINT ( 'NONE',  ( 16.08776274289027342, -3.050289026998445951, 32.03036669348365706 ) ) ;
#86357=CARTESIAN_POINT ( 'NONE',  ( 1.253924781505078689, -12.62707690430377383, 30.88035979386743435 ) ) ;
#86358=CARTESIAN_POINT ( 'NONE',  ( 14.05766908347084865, -10.92453946501458795, 33.72985991061850086 ) ) ;
#86359=FACE_OUTER_BOUND ( 'NONE', #36250, .T. ) ;
#86360=DIRECTION ( 'NONE',  ( 0.000000000000000000, 0.9396926207859126468, 0.3420201433256571111 ) ) ;
#86363=ORIENTED_EDGE ( 'NONE', *, *, #5813, .T. ) ;
#86364=CARTESIAN_POINT ( 'NONE',  ( -7.846153846153844924, -11.16473453929635440, 33.15142922261926373 ) ) ;
#86365=DIRECTION ( 'NONE',  ( -0.000000000000000000, -0.8660254037844399289, -0.4999999999999980016 ) ) ;
#86366=CARTESIAN_POINT ( 'NONE',  ( 12.46153846153846168, -3.886160181151819604, 36.00935417666054406 ) ) ;
#86367=DIRECTION ( 'NONE',  ( -0.000000000000000000, 0.7660444431189791237, -0.6427876096865379196 ) ) ;
#86368=CARTESIAN_POINT ( 'NONE',  ( 6.699591998512592461, -12.69144148231606017, 30.53333754910549303 ) ) ;
#86369=LINE ( 'NONE', #72819, #13904 ) ;
#86371=CARTESIAN_POINT ( 'NONE',  ( -15.48074597481782178, -12.65889640711025521, 30.72598325615533454 ) ) ;
#86372=FACE_OUTER_BOUND ( 'NONE', #21934, .T. ) ;
#86373=CARTESIAN_POINT ( 'NONE',  ( -7.846153846153844924, -9.905515769479276145, 34.41647553114623292 ) ) ;
#86374=CARTESIAN_POINT ( 'NONE',  ( 5.326977496836529546, -12.65882529074907126, 30.72640787790839312 ) ) ;
#86377=ADVANCED_FACE ( 'NONE', ( #18010 ), #72496, .F. ) ;
#86378=CARTESIAN_POINT ( 'NONE',  ( -6.222926958906843886, -11.98009711892699691, 32.48740034544075428 ) ) ;
#86379=CARTESIAN_POINT ( 'NONE',  ( -11.28851602011339672, -10.76462480002816235, 33.53768742498949962 ) ) ;
#86380=ORIENTED_EDGE ( 'NONE', *, *, #45390, .F. ) ;
#86381=VECTOR ( 'NONE', #42834, 1000.000000000000114 ) ;
#86382=ADVANCED_FACE ( 'NONE', ( #12147 ), #32408, .F. ) ;
#86384=CARTESIAN_POINT ( 'NONE',  ( -14.30769230769242739, -3.835265460704628371, 33.15142922262033665 ) ) ;
#86386=DIRECTION ( 'NONE',  ( -0.000000000000000000, -0.7660444431189791237, -0.6427876096865379196 ) ) ;
#86387=DIRECTION ( 'NONE',  ( -0.000000000000000000, -0.9848077530122085754, -0.1736481776669273613 ) ) ;
#86388=VERTEX_POINT ( 'NONE', #59876 ) ;
#86389=CARTESIAN_POINT ( 'NONE',  ( -17.77698715590660328, -6.460100341425562220, 34.89618726649961644 ) ) ;
#86390=CARTESIAN_POINT ( 'NONE',  ( 11.53846153846141576, -6.835583212225970762, 34.95778746994575670 ) ) ;
#86393=CARTESIAN_POINT ( 'NONE',  ( -12.52680846209478283, -9.528491918058357157, 34.59228464037090589 ) ) ;
#86394=CARTESIAN_POINT ( 'NONE',  ( -11.53846153846153655, -3.886160181151819604, 36.00935417666054406 ) ) ;
#86395=CARTESIAN_POINT ( 'NONE',  ( -4.826868765284761054, -9.148310452688871663, 34.47095581063188519 ) ) ;
#86396=CARTESIAN_POINT ( 'NONE',  ( -12.46153846153858424, -5.094484230521993062, 34.41647553114689373 ) ) ;
#86397=EDGE_CURVE ( 'NONE', #31074, #38805, #19789, .T. ) ;
#86398=VERTEX_POINT ( 'NONE', #4028 ) ;
#86399=CARTESIAN_POINT ( 'NONE',  ( -2.307692307692305711, -8.564572088678739092, 35.78748833219616898 ) ) ;
#86400=CARTESIAN_POINT ( 'NONE',  ( -12.68446542044531000, -2.523278758544489797, 31.42238647778637528 ) ) ;
#86401=AXIS2_PLACEMENT_3D ( 'NONE', #37226, #37676, #71902 ) ;
#86402=CARTESIAN_POINT ( 'NONE',  ( -10.61538461538473399, -3.300289026999228881, 32.46337939537708905 ) ) ;
#86403=ORIENTED_EDGE ( 'NONE', *, *, #66045, .T. ) ;
#86404=VERTEX_POINT ( 'NONE', #26097 ) ;
#86405=EDGE_LOOP ( 'NONE', ( #48746, #34893 ) ) ;
#86406=B_SPLINE_CURVE_WITH_KNOTS ( 'NONE', 3,
 ( #88963, #27232, #66892, #32657, #56030, #29463, #14161, #41637, #62337, #49716 ),
 .UNSPECIFIED., .F., .F.,
 ( 4, 2, 2, 2, 4 ),
 ( 0.000000000000000000, 0.0001954339857564086670, 0.0003908679715128173340, 0.0005863019572692260281, 0.0007817359430256346680 ),
 .UNSPECIFIED. ) ;
#86409=DIRECTION ( 'NONE',  ( -0.000000000000000000, -0.8660254037844399289, -0.4999999999999980016 ) ) ;
#86410=CARTESIAN_POINT ( 'NONE',  ( 6.249945409378045547, -2.341251567377310217, 30.72681386836322659 ) ) ;
#86411=EDGE_CURVE ( 'NONE', #34578, #82613, #76737, .T. ) ;
#86412=EDGE_CURVE ( 'NONE', #88899, #5856, #60605, .T. ) ;
#86413=CARTESIAN_POINT ( 'NONE',  ( 2.557637826040450868, -5.852078868378310261, 34.47109172314383585 ) ) ;
#86415=AXIS2_PLACEMENT_3D ( 'NONE', #77342, #77783, #51167 ) ;
#86416=DIRECTION ( 'NONE',  ( -0.000000000000000000, 0.8660254037844397068, -0.4999999999999978906 ) ) ;
#86418=EDGE_CURVE ( 'NONE', #46856, #47638, #70186, .T. ) ;
#86420=EDGE_CURVE ( 'NONE', #18273, #57358, #29624, .T. ) ;
#86421=FACE_OUTER_BOUND ( 'NONE', #21595, .T. ) ;
#86422=ORIENTED_EDGE ( 'NONE', *, *, #55855, .T. ) ;
#86423=CARTESIAN_POINT ( 'NONE',  ( -5.326899820971665811, -2.544273027872574922, 31.48422191005632342 ) ) ;
#86425=DIRECTION ( 'NONE',  ( -0.000000000000000000, 0.8660254037844397068, -0.4999999999999978906 ) ) ;
#86426=CARTESIAN_POINT ( 'NONE',  ( -13.25408968285182354, -12.45806712695776319, 30.39783852428763922 ) ) ;
#86427=ORIENTED_EDGE ( 'NONE', *, *, #60408, .T. ) ;
#86428=ORIENTED_EDGE ( 'NONE', *, *, #4457, .T. ) ;
#86430=CARTESIAN_POINT ( 'NONE',  ( 14.98074599347626368, -2.587272538249754117, 30.68239716806877837 ) ) ;
#86431=ORIENTED_EDGE ( 'NONE', *, *, #43948, .F. ) ;
#86432=CARTESIAN_POINT ( 'NONE',  ( -10.86538461538461320, -2.249999999999998668, 29.75000000000000355 ) ) ;
#86433=ADVANCED_FACE ( 'NONE', ( #70603 ), #22413, .F. ) ;
#86434=CARTESIAN_POINT ( 'NONE',  ( -13.38461538461550582, -6.879047030192662504, 34.71129190930017927 ) ) ;
#86436=DIRECTION ( 'NONE',  ( 0.000000000000000000, 1.000000000000000000, 0.000000000000000000 ) ) ;
#86437=DIRECTION ( 'NONE',  ( -0.000000000000000000, 0.6427876096865404731, -0.7660444431189770143 ) ) ;
#86439=FACE_BOUND ( 'NONE', #59286, .T. ) ;
#86441=CARTESIAN_POINT ( 'NONE',  ( 9.442307692307693401, -7.500000000000001776, 34.75000000000000000 ) ) ;
#86442=LINE ( 'NONE', #24715, #43742 ) ;
#86444=CARTESIAN_POINT ( 'NONE',  ( -8.546451100252705047, -12.11081565061824250, 32.26097654155340422 ) ) ;
#86446=CARTESIAN_POINT ( 'NONE',  ( 1.450682717965462887, -2.292212530054420494, 30.41441678777542990 ) ) ;
#86447=EDGE_LOOP ( 'NONE', ( #82750, #61199, #75615, #22814 ) ) ;
#86448=CARTESIAN_POINT ( 'NONE',  ( 2.557637826040451312, -6.696923467548660192, 34.68552623307873972 ) ) ;
#86449=CARTESIAN_POINT ( 'NONE',  ( -13.38461538461550759, -4.320704448113951379, 33.92786785259630022 ) ) ;
#86450=ORIENTED_EDGE ( 'NONE', *, *, #49318, .F. ) ;
#86451=VERTEX_POINT ( 'NONE', #14781 ) ;
#86452=CARTESIAN_POINT ( 'NONE',  ( -6.923076923076922462, -8.120952969808772792, 34.71129190930000163 ) ) ;
#86453=CARTESIAN_POINT ( 'NONE',  ( 1.634560793993429684, -5.766571408460172243, 34.70601412856602508 ) ) ;
#86454=CARTESIAN_POINT ( 'NONE',  ( 16.40379156322419973, -6.653508905675593610, 34.93172785388651391 ) ) ;
#86455=CARTESIAN_POINT ( 'NONE',  ( 1.134592147322421196, -6.695914987888143877, 34.68535235679833306 ) ) ;
#86456=CARTESIAN_POINT ( 'NONE',  ( 17.07692307692307665, -11.11383981884818262, 36.00935417666054406 ) ) ;
#86457=ORIENTED_EDGE ( 'NONE', *, *, #41473, .F. ) ;
#86459=CARTESIAN_POINT ( 'NONE',  ( 4.219101293358991533, -5.094484230520773593, 34.41647553114626845 ) ) ;
#86460=CARTESIAN_POINT ( 'NONE',  ( 4.946775867484856093, -6.001485441113818986, 34.52039167877662607 ) ) ;
#86461=CARTESIAN_POINT ( 'NONE',  ( -9.942284423250047354, -4.236021600441997492, 33.53823185664189310 ) ) ;
#86463=CARTESIAN_POINT ( 'NONE',  ( 10.83839596699746721, -4.187068189119697692, 33.49521262558774026 ) ) ;
#86464=DIRECTION ( 'NONE',  ( -0.000000000000000000, 0.9396926207859093161, -0.3420201433256663259 ) ) ;
#86466=EDGE_LOOP ( 'NONE', ( #3849, #72095 ) ) ;
#86469=ORIENTED_EDGE ( 'NONE', *, *, #72828, .T. ) ;
#86470=CARTESIAN_POINT ( 'NONE',  ( -24.00000000000000000, -5.499999999999981348, 27.75000000000000000 ) ) ;
#86471=CARTESIAN_POINT ( 'NONE',  ( 0.4615384615383382183, -12.51329471203414379, 31.30864560766407578 ) ) ;
#86472=CARTESIAN_POINT ( 'NONE',  ( 18.22277954126840172, -5.913360116392396115, 34.49180327182771322 ) ) ;
#86473=CARTESIAN_POINT ( 'NONE',  ( 4.153846153846030731, -11.06231777344772027, 33.60647404775119895 ) ) ;
#86474=FACE_OUTER_BOUND ( 'NONE', #12184, .T. ) ;
#86477=CARTESIAN_POINT ( 'NONE',  ( 12.46153846153846168, -13.78497067705608181, 32.30358669280327177 ) ) ;
#86478=CARTESIAN_POINT ( 'NONE',  ( 16.15384615384615330, -13.95598074871891292, 31.83374038241031911 ) ) ;
#86479=CARTESIAN_POINT ( 'NONE',  ( -1.384615384615383471, -8.164416787775445883, 34.95778746994557906 ) ) ;
#86480=CARTESIAN_POINT ( 'NONE',  ( -6.249999999999997335, -2.499999999999998668, 29.75000000000000355 ) ) ;
#86481=DIRECTION ( 'NONE',  ( -0.000000000000000000, 0.8660254037844399289, -0.4999999999999980016 ) ) ;
#86482=CARTESIAN_POINT ( 'NONE',  ( -12.23852710992561299, -3.587049720035815348, 32.86302985866382897 ) ) ;
#86484=CARTESIAN_POINT ( 'NONE',  ( 7.173131342990377135, -2.318338780012835443, 30.59689888758630261 ) ) ;
#86485=DIRECTION ( 'NONE',  ( 0.000000000000000000, 1.000000000000000000, 0.000000000000000000 ) ) ;
#86486=CARTESIAN_POINT ( 'NONE',  ( 11.47237812750566022, -6.386643153685125363, 34.62446782046654903 ) ) ;
#86487=CARTESIAN_POINT ( 'NONE',  ( -15.36146069743678844, -8.147922237126337563, 34.70805685702651999 ) ) ;
#86488=ORIENTED_EDGE ( 'NONE', *, *, #14163, .F. ) ;
#86489=CARTESIAN_POINT ( 'NONE',  ( -16.15384615384615330, -6.343179335718451384, 34.87096338111211935 ) ) ;
#86490=CARTESIAN_POINT ( 'NONE',  ( 17.99999999999987566, -5.094484230521993062, 34.41647553114689373 ) ) ;
#86491=CARTESIAN_POINT ( 'NONE',  ( 17.99999999999987566, -10.21337939537710326, 33.94971097300076224 ) ) ;
#86493=CARTESIAN_POINT ( 'NONE',  ( 6.000000000000001776, -11.35647404775217417, 33.31231777344666511 ) ) ;
#86494=CARTESIAN_POINT ( 'NONE',  ( 16.02315555073584363, -4.684245665217972032, 34.18127051446801090 ) ) ;
#86495=DIRECTION ( 'NONE',  ( 0.000000000000000000, 0.6427876096865368094, 0.7660444431189802339 ) ) ;
#86496=ORIENTED_EDGE ( 'NONE', *, *, #32932, .T. ) ;
#86498=CARTESIAN_POINT ( 'NONE',  ( -1.634638621908349521, -10.05641848906368452, 34.04755513067966177 ) ) ;
#86499=VERTEX_POINT ( 'NONE', #77358 ) ;
#86500=CARTESIAN_POINT ( 'NONE',  ( 6.857806922520603976, -6.835583212224499938, 34.95778746994557906 ) ) ;
#86502=CARTESIAN_POINT ( 'NONE',  ( -7.623374177175779032, -6.717445702608402236, 34.94155399931962336 ) ) ;
#86504=CARTESIAN_POINT ( 'NONE',  ( 15.48071474911737511, -2.824170634883621744, 31.52227843825338738 ) ) ;
#86506=CARTESIAN_POINT ( 'NONE',  ( 11.53846153846153832, -11.91647553114624181, 32.58852847137148245 ) ) ;
#86508=FACE_OUTER_BOUND ( 'NONE', #26831, .T. ) ;
#86509=B_SPLINE_CURVE_WITH_KNOTS ( 'NONE', 3,
 ( #43797, #55541, #71259, #49673, #83024, #55985, #36606, #21757, #64064, #77149 ),
 .UNSPECIFIED., .F., .F.,
 ( 4, 2, 2, 2, 4 ),
 ( 0.0007817359430256400890, 0.0009771253907250091169, 0.001172514838424378253, 0.001367904286123747173, 0.001563293733823116309 ),
 .UNSPECIFIED. ) ;
#86510=B_SPLINE_CURVE_WITH_KNOTS ( 'NONE', 3,
 ( #1052, #62296, #19987, #20440, #76254, #54649, #82147, #82597, #41594, #20872 ),
 .UNSPECIFIED., .F., .F.,
 ( 4, 2, 2, 2, 4 ),
 ( 0.0007817359430256294638, 0.0009771253907249950223, 0.001172514838424360472, 0.001367904286123725922, 0.001563293733823091372 ),
 .UNSPECIFIED. ) ;
#86512=ORIENTED_EDGE ( 'NONE', *, *, #31181, .F. ) ;
#86513=CARTESIAN_POINT ( 'NONE',  ( 10.61538461538461675, -13.75783147151868846, 33.36296068462461051 ) ) ;
#86514=CARTESIAN_POINT ( 'NONE',  ( 12.71159277317677905, -12.17597550085003810, 31.52189283813460463 ) ) ;
#86515=ORIENTED_EDGE ( 'NONE', *, *, #2980, .F. ) ;
#86516=CARTESIAN_POINT ( 'NONE',  ( 9.692307692307695177, -8.973038597847269315, 34.52809138561121927 ) ) ;
#86517=CARTESIAN_POINT ( 'NONE',  ( 6.923076923076800782, -8.656820664282941280, 34.87096338111179961 ) ) ;
#86518=CARTESIAN_POINT ( 'NONE',  ( -1.253824943648433443, -10.70102852606553157, 33.91149625220312913 ) ) ;
#86519=CARTESIAN_POINT ( 'NONE',  ( -14.24162497434223162, -9.905515769479276145, 34.41647553114623292 ) ) ;
#86521=VERTEX_POINT ( 'NONE', #30061 ) ;
#86522=VERTEX_POINT ( 'NONE', #57525 ) ;
#86523=VECTOR ( 'NONE', #50978, 1000.000000000000000 ) ;
#86524=EDGE_CURVE ( 'NONE', #74762, #36504, #37964, .T. ) ;
#86525=ORIENTED_EDGE ( 'NONE', *, *, #32646, .F. ) ;
#86527=ORIENTED_EDGE ( 'NONE', *, *, #22754, .F. ) ;
#86528=AXIS2_PLACEMENT_3D ( 'NONE', #80787, #59156, #17287 ) ;
#86529=CARTESIAN_POINT ( 'NONE',  ( 10.36540788444226102, -4.943428324936578910, 34.04746400365624481 ) ) ;
#86530=CARTESIAN_POINT ( 'NONE',  ( 3.230769230769231726, -13.75783147151868846, 33.36296068462461051 ) ) ;
#86531=ORIENTED_EDGE ( 'NONE', *, *, #27443, .T. ) ;
#86532=ORIENTED_EDGE ( 'NONE', *, *, #39644, .F. ) ;
#86533=CARTESIAN_POINT ( 'NONE',  ( -10.83831083290076158, -3.105860786376062332, 32.13614157043599562 ) ) ;
#86534=ORIENTED_EDGE ( 'NONE', *, *, #31077, .T. ) ;
#86535=CARTESIAN_POINT ( 'NONE',  ( -9.692307692307377209, -2.255955759149395501, 30.00000000000324363 ) ) ;
#86536=B_SPLINE_CURVE_WITH_KNOTS ( 'NONE', 3,
 ( #78907, #59968, #52762, #11796, #65390, #50966, #16757, #71699, #3684, #54092 ),
 .UNSPECIFIED., .F., .F.,
 ( 4, 2, 2, 2, 4 ),
 ( 0.000000000000000000, 0.0001954339857564080165, 0.0003908679715128160329, 0.0005863019572692240765, 0.0007817359430256320659 ),
 .UNSPECIFIED. ) ;
#86537=ADVANCED_FACE ( 'NONE', ( #9782 ), #35940, .F. ) ;
#86538=CARTESIAN_POINT ( 'NONE',  ( 4.023698184114456566, -12.70455904226513866, 30.44083106164009322 ) ) ;
#86539=CARTESIAN_POINT ( 'NONE',  ( -11.31544869436814338, -11.98016756924215009, 32.48728574198911190 ) ) ;
#86540=FACE_BOUND ( 'NONE', #58839, .T. ) ;
#86541=EDGE_CURVE ( 'NONE', #10260, #10737, #33661, .T. ) ;
#86543=CYLINDRICAL_SURFACE ( 'NONE', #5318, 0.2499999999999995559 ) ;
#86544=CARTESIAN_POINT ( 'NONE',  ( -1.634615384615383027, -7.500000000000001776, 34.75000000000000000 ) ) ;
#86545=ADVANCED_FACE ( 'NONE', ( #31387 ), #38591, .F. ) ;
#86546=CARTESIAN_POINT ( 'NONE',  ( 4.946232473812766983, -3.338472653186242756, 32.95098750199972670 ) ) ;
#86547=CARTESIAN_POINT ( 'NONE',  ( -11.53846153846153655, -2.708943851104267164, 35.45975837776705220 ) ) ;
#86548=CARTESIAN_POINT ( 'NONE',  ( -1.634638621908348410, -2.587272538249755449, 30.68239716806877837 ) ) ;
#86549=ORIENTED_EDGE ( 'NONE', *, *, #40121, .T. ) ;
#86551=ORIENTED_EDGE ( 'NONE', *, *, #50335, .T. ) ;
#86552=EDGE_LOOP ( 'NONE', ( #62606, #50154, #71004, #63940 ) ) ;
#86553=CARTESIAN_POINT ( 'NONE',  ( -6.923076923077045919, -4.320704448113951379, 33.92786785259630022 ) ) ;
#86554=DIRECTION ( 'NONE',  ( -0.000000000000000000, -0.3420201433256694346, -0.9396926207859080948 ) ) ;
#86556=DIRECTION ( 'NONE',  ( 0.000000000000000000, -3.469446951953611033E-15, -1.000000000000000000 ) ) ;
#86559=CARTESIAN_POINT ( 'NONE',  ( -8.769230769230890843, -6.879047030192662504, 34.71129190930017927 ) ) ;
#86560=EDGE_LOOP ( 'NONE', ( #85254, #66642 ) ) ;
#86562=FACE_OUTER_BOUND ( 'NONE', #67978, .T. ) ;
#86563=CARTESIAN_POINT ( 'NONE',  ( 10.54930120442873687, -3.050289026998445951, 32.03036669348365706 ) ) ;
#86564=CARTESIAN_POINT ( 'NONE',  ( 13.13463865367303285, -12.41269422305637171, 30.68257228309993323 ) ) ;
#86565=AXIS2_PLACEMENT_3D ( 'NONE', #38402, #46493, #60002 ) ;
#86566=ORIENTED_EDGE ( 'NONE', *, *, #29680, .F. ) ;
#86567=ORIENTED_EDGE ( 'NONE', *, *, #5926, .T. ) ;
#86568=FACE_BOUND ( 'NONE', #78877, .T. ) ;
#86570=EDGE_LOOP ( 'NONE', ( #34713, #71990 ) ) ;
#86571=CARTESIAN_POINT ( 'NONE',  ( 7.780883400193070898, -2.892918686051582089, 31.69288490824015270 ) ) ;
#86572=CARTESIAN_POINT ( 'NONE',  ( -1.134560964701931463, -2.318338780012835443, 30.59689888758630261 ) ) ;
#86574=CARTESIAN_POINT ( 'NONE',  ( -7.715362038329057981, -4.118422570099827595, 33.43335022499816489 ) ) ;
#86575=CARTESIAN_POINT ( 'NONE',  ( 16.15384615384615330, -1.466349020453238561, 30.81389545987213907 ) ) ;
#86576=CARTESIAN_POINT ( 'NONE',  ( 0.5267940328144855577, -12.27809138561124591, 31.22303859784720359 ) ) ;
#86577=CARTESIAN_POINT ( 'NONE',  ( -6.923076923076922462, -1.242168528481310874, 33.36296068462461051 ) ) ;
#86578=DIRECTION ( 'NONE',  ( -0.000000000000000000, 1.000000000000000000, 3.491481338843133355E-15 ) ) ;
#86580=CARTESIAN_POINT ( 'NONE',  ( 0.3313912521002396194, -10.19110544564092002, 33.96427741523702792 ) ) ;
#86582=CARTESIAN_POINT ( 'NONE',  ( -7.780898274877819709, -9.442884908240271713, 34.35708131394835618 ) ) ;
#86583=CARTESIAN_POINT ( 'NONE',  ( 15.23076923076923173, -10.67929555188718282, 33.92786785259544047 ) ) ;
#86584=FACE_OUTER_BOUND ( 'NONE', #11408, .T. ) ;
#86585=B_SPLINE_CURVE_WITH_KNOTS ( 'NONE', 3,
 ( #39080, #66541, #73757, #12051, #20127, #27326 ),
 .UNSPECIFIED., .F., .F.,
 ( 4, 2, 4 ),
 ( 0.0003909512603273593376, 0.0005862562993131836733, 0.0007815613382990081173 ),
 .UNSPECIFIED. ) ;
#86586=EDGE_CURVE ( 'NONE', #30133, #28433, #83107, .T. ) ;
#86588=CYLINDRICAL_SURFACE ( 'NONE', #62005, 0.2500000000000009437 ) ;
#86589=CARTESIAN_POINT ( 'NONE',  ( 6.066068351002441794, -2.721908614388772296, 31.22303859784725333 ) ) ;
#86592=CARTESIAN_POINT ( 'NONE',  ( 14.30769230769218581, -2.379036618888197729, 30.90682066428292885 ) ) ;
#86593=CARTESIAN_POINT ( 'NONE',  ( 2.307692307692309264, -3.937682226553329556, 33.60647404775216529 ) ) ;
#86594=CYLINDRICAL_SURFACE ( 'NONE', #46734, 0.2499999999999986955 ) ;
#86595=AXIS2_PLACEMENT_3D ( 'NONE', #17760, #11001, #38473 ) ;
#86596=AXIS2_PLACEMENT_3D ( 'NONE', #19591, #81307, #88965 ) ;
#86598=EDGE_LOOP ( 'NONE', ( #30148, #59545 ) ) ;
#86599=LINE ( 'NONE', #31178, #34017 ) ;
#86600=CARTESIAN_POINT ( 'NONE',  ( 7.622668921589514923, -6.716662450894489211, 34.94144148231605840 ) ) ;
#86602=CIRCLE ( 'NONE', #77965, 0.2500000000000002220 ) ;
#86603=EDGE_CURVE ( 'NONE', #720, #45245, #69234, .T. ) ;
#86604=CARTESIAN_POINT ( 'NONE',  ( 10.48469314871706004, -4.118384482072086072, 33.43331474514187107 ) ) ;
#86605=CARTESIAN_POINT ( 'NONE',  ( 17.75002325595140817, -12.01397095200673881, 32.43157075238190146 ) ) ;
#86606=FACE_OUTER_BOUND ( 'NONE', #1222, .T. ) ;
#86607=ORIENTED_EDGE ( 'NONE', *, *, #57952, .F. ) ;
#86608=CARTESIAN_POINT ( 'NONE',  ( -2.980714810855778385, -12.65882529074907126, 30.72640787790839312 ) ) ;
#86609=LINE ( 'NONE', #55349, #57829 ) ;
#86610=DIRECTION ( 'NONE',  ( -0.000000000000000000, -0.3420201433256694901, -0.9396926207859082059 ) ) ;
#86611=B_SPLINE_CURVE_WITH_KNOTS ( 'NONE', 3,
 ( #58010, #1745, #71083, #84620, #1296, #69758, #8510, #49042, #43175, #56250 ),
 .UNSPECIFIED., .F., .F.,
 ( 4, 2, 2, 2, 4 ),
 ( 0.000000000000000000, 0.0001954311564186882568, 0.0003908623128373765136, 0.0005862934692560647703, 0.0007817246256747530271 ),
 .UNSPECIFIED. ) ;
#86612=CARTESIAN_POINT ( 'NONE',  ( 4.153846153846154188, -8.164416787775445883, 34.95778746994557906 ) ) ;
#86613=ORIENTED_EDGE ( 'NONE', *, *, #68753, .F. ) ;
#86614=CARTESIAN_POINT ( 'NONE',  ( 16.08776377448601735, -12.34228464037088280, 31.77849191805838558 ) ) ;
#86615=B_SPLINE_CURVE_WITH_KNOTS ( 'NONE', 3,
 ( #71446, #44405, #15195, #42666, #8432, #1670, #29157, #56616, #84103, #45760 ),
 .UNSPECIFIED., .F., .F.,
 ( 4, 2, 2, 2, 4 ),
 ( 0.0007817359430256361858, 0.0009771253907250041296, 0.001172514838424372182, 0.001367904286123740234, 0.001563293733823108286 ),
 .UNSPECIFIED. ) ;
#86617=ORIENTED_EDGE ( 'NONE', *, *, #32903, .F. ) ;
#86618=CARTESIAN_POINT ( 'NONE',  ( 1.607578288176872094, -7.369474270740069777, 34.74850911626239736 ) ) ;
#86620=CARTESIAN_POINT ( 'NONE',  ( -0.4615384615381466493, -2.255955759149395501, 30.00000000000324363 ) ) ;
#86621=VERTEX_POINT ( 'NONE', #58395 ) ;
#86622=EDGE_CURVE ( 'NONE', #67914, #28375, #48812, .T. ) ;
#86623=LINE ( 'NONE', #63772, #43468 ) ;
#86626=VECTOR ( 'NONE', #34715, 1000.000000000000114 ) ;
#86627=FACE_OUTER_BOUND ( 'NONE', #16643, .T. ) ;
#86628=CARTESIAN_POINT ( 'NONE',  ( -3.230769230769229949, -12.37446782046654192, 30.86335684631486131 ) ) ;
#86629=ORIENTED_EDGE ( 'NONE', *, *, #72392, .T. ) ;
#86630=EDGE_CURVE ( 'NONE', #79887, #45031, #12285, .T. ) ;
#86631=FACE_BOUND ( 'NONE', #9549, .T. ) ;
#86632=VERTEX_POINT ( 'NONE', #73263 ) ;
#86634=CARTESIAN_POINT ( 'NONE',  ( -2.372962308248625973, -2.657715359629089225, 31.77849191805834295 ) ) ;
#86635=B_SPLINE_CURVE_WITH_KNOTS ( 'NONE', 3,
 ( #13553, #68937, #32490, #59963, #80706, #41034, #68493, #81141, #60854, #88356 ),
 .UNSPECIFIED., .F., .F.,
 ( 4, 2, 2, 2, 4 ),
 ( 0.0007817359430256297891, 0.0009771253907249958896, 0.001172514838424361990, 0.001367904286123728091, 0.001563293733823094191 ),
 .UNSPECIFIED. ) ;
#86636=CARTESIAN_POINT ( 'NONE',  ( -9.469296340694841163, -12.15243808032446005, 31.58219941686247978 ) ) ;
#86637=EDGE_CURVE ( 'NONE', #83562, #29011, #10042, .T. ) ;
#86639=CARTESIAN_POINT ( 'NONE',  ( 15.23076923076910916, -9.528491918059723176, 34.59228464037033035 ) ) ;
#86640=EDGE_CURVE ( 'NONE', #6775, #58077, #71293, .T. ) ;
#86641=CARTESIAN_POINT ( 'NONE',  ( 4.826923076923065992, -2.499999999999999556, 29.81609845454692120 ) ) ;
#86642=DIRECTION ( 'NONE',  ( 0.000000000000000000, 0.4999999999999960032, -0.8660254037844410391 ) ) ;
#86644=EDGE_LOOP ( 'NONE', ( #46192, #4197 ) ) ;
#86645=ORIENTED_EDGE ( 'NONE', *, *, #45093, .T. ) ;
#86647=ORIENTED_EDGE ( 'NONE', *, *, #88565, .T. ) ;
#86648=ORIENTED_EDGE ( 'NONE', *, *, #51582, .T. ) ;
#86649=ADVANCED_FACE ( 'NONE', ( #12449 ), #53423, .F. ) ;
#86650=CARTESIAN_POINT ( 'NONE',  ( 12.52679403281448600, -11.94971097300157403, 32.03036669348361443 ) ) ;
#86651=CARTESIAN_POINT ( 'NONE',  ( 15.23076923076923173, -1.242168528481310874, 33.36296068462461051 ) ) ;
#86652=CARTESIAN_POINT ( 'NONE',  ( -2.557692307692305267, -7.500000000000001776, 34.75000000000000000 ) ) ;
#86653=CARTESIAN_POINT ( 'NONE',  ( -5.869474298236438514, -5.195472089885680766, 34.18748526763464923 ) ) ;
#86654=CARTESIAN_POINT ( 'NONE',  ( -16.37733109757010652, -2.599994579823202923, 30.74605699353653776 ) ) ;
#86655=AXIS2_PLACEMENT_3D ( 'NONE', #50852, #36912, #42365 ) ;
#86656=CARTESIAN_POINT ( 'NONE',  ( -6.223484924564332665, -3.019605429927184836, 32.48692288466676814 ) ) ;
#86657=VECTOR ( 'NONE', #78401, 1000.000000000000227 ) ;
#86658=ADVANCED_FACE ( 'NONE', ( #61074 ), #54310, .F. ) ;
#86659=CARTESIAN_POINT ( 'NONE',  ( 5.933916589044120116, -11.69971097300155272, 32.46337939537587403 ) ) ;
#86660=ADVANCED_FACE ( 'NONE', ( #87684 ), #80926, .F. ) ;
#86661=CARTESIAN_POINT ( 'NONE',  ( -7.715362038329058869, -3.062576670634119758, 32.05464942895959979 ) ) ;
#86662=CARTESIAN_POINT ( 'NONE',  ( 7.976679284387491187, -5.070358843744210198, 34.40418822224088302 ) ) ;
#86663=VERTEX_POINT ( 'NONE', #88581 ) ;
#86664=ORIENTED_EDGE ( 'NONE', *, *, #57704, .T. ) ;
#86666=EDGE_LOOP ( 'NONE', ( #74259, #71182 ) ) ;
#86667=CARTESIAN_POINT ( 'NONE',  ( 0.3962684609821409687, -3.083524468853724443, 32.58852847137143272 ) ) ;
#86668=ORIENTED_EDGE ( 'NONE', *, *, #76047, .T. ) ;
#86669=CARTESIAN_POINT ( 'NONE',  ( -15.90379184220783948, -6.567000820036036579, 34.66262288849541306 ) ) ;
#86670=CARTESIAN_POINT ( 'NONE',  ( 18.25000000000001776, -2.249999999999997780, 29.81603969181029257 ) ) ;
#86671=CARTESIAN_POINT ( 'NONE',  ( 1.515140822849030622, -5.070358843744210198, 34.40418822224088302 ) ) ;
#86672=CARTESIAN_POINT ( 'NONE',  ( 7.145856464345329506, -2.600157965045225339, 30.74683119005207743 ) ) ;
#86673=FACE_BOUND ( 'NONE', #37883, .T. ) ;
#86674=ORIENTED_EDGE ( 'NONE', *, *, #33229, .F. ) ;
#86675=B_SPLINE_CURVE_WITH_KNOTS ( 'NONE', 3,
 ( #39194, #81954, #66655, #12601, #40526, #33319, #86953, #54459, #18472, #40957 ),
 .UNSPECIFIED., .F., .F.,
 ( 4, 2, 2, 2, 4 ),
 ( 0.000000000000000000, 0.0001954339857564093717, 0.0003908679715128187434, 0.0005863019572692280881, 0.0007817359430256374869 ),
 .UNSPECIFIED. ) ;
#86676=VERTEX_POINT ( 'NONE', #69168 ) ;
#86677=CARTESIAN_POINT ( 'NONE',  ( 7.173076923076923350, -2.499999999999998668, 29.75000000000000355 ) ) ;
#86678=EDGE_LOOP ( 'NONE', ( #72539, #10342 ) ) ;
#86679=FACE_BOUND ( 'NONE', #7401, .T. ) ;
#86680=CARTESIAN_POINT ( 'NONE',  ( -10.86536135943320502, -2.920706130388546651, 32.31842814019191223 ) ) ;
#86682=ORIENTED_EDGE ( 'NONE', *, *, #29137, .F. ) ;
#86683=CARTESIAN_POINT ( 'NONE',  ( 2.242421861731533017, -8.613356846314824011, 34.62446782046655613 ) ) ;
#86684=CARTESIAN_POINT ( 'NONE',  ( 16.82692307692307665, -2.249999999999998668, 29.75000000000000355 ) ) ;
#86685=FACE_OUTER_BOUND ( 'NONE', #6516, .T. ) ;
#86686=ORIENTED_EDGE ( 'NONE', *, *, #39320, .T. ) ;
#86687=CARTESIAN_POINT ( 'NONE',  ( 17.07692307692307665, -3.050289026998446396, 32.03036669348365706 ) ) ;
#86688=CARTESIAN_POINT ( 'NONE',  ( -14.53061852520844965, -5.667676309546437530, 34.40238873228292249 ) ) ;
#86689=ORIENTED_EDGE ( 'NONE', *, *, #27866, .F. ) ;
#86690=CARTESIAN_POINT ( 'NONE',  ( -1.515306851282943068, -5.582088688514999397, 34.36776431015576350 ) ) ;
#86691=CARTESIAN_POINT ( 'NONE',  ( 7.053868730901711182, -10.54018710029568595, 33.71981072465678864 ) ) ;
#86692=AXIS2_PLACEMENT_3D ( 'NONE', #73273, #87249, #59754 ) ;
#86693=VERTEX_POINT ( 'NONE', #81804 ) ;
#86694=CARTESIAN_POINT ( 'NONE',  ( 0.2386122440223129304, -9.086856451489515152, 34.49173150075333183 ) ) ;
#86695=CARTESIAN_POINT ( 'NONE',  ( -10.48485891362105171, -5.195472089885680766, 34.18748526763464923 ) ) ;
#86696=CARTESIAN_POINT ( 'NONE',  ( 16.08776377448601025, -2.833524468853757305, 32.15551576947924417 ) ) ;
#86697=CARTESIAN_POINT ( 'NONE',  ( -8.519176457592452678, -9.148310452688876993, 34.47095581063188519 ) ) ;
#86698=CARTESIAN_POINT ( 'NONE',  ( -15.93106661257773560, -4.387253974876675677, 33.66317474335728832 ) ) ;
#86699=EDGE_CURVE ( 'NONE', #16511, #3680, #84246, .T. ) ;
#86700=LINE ( 'NONE', #59641, #27999 ) ;
#86701=CARTESIAN_POINT ( 'NONE',  ( 4.826899839630110378, -12.43535235679832596, 30.55408501211184813 ) ) ;
#86703=CARTESIAN_POINT ( 'NONE',  ( -16.08777780284371417, -11.69971097300155272, 32.46337939537588113 ) ) ;
#86704=DIRECTION ( 'NONE',  ( 0.000000000000000000, 0.000000000000000000, -1.000000000000000000 ) ) ;
#86705=DIRECTION ( 'NONE',  ( -0.000000000000000000, 0.9396926207859093161, -0.3420201433256663259 ) ) ;
#86706=EDGE_CURVE ( 'NONE', #81582, #63578, #79928, .T. ) ;
#86708=ORIENTED_EDGE ( 'NONE', *, *, #70860, .T. ) ;
#86710=CARTESIAN_POINT ( 'NONE',  ( 12.46153846153833911, -3.300289026999228881, 32.46337939537708905 ) ) ;
#86713=ORIENTED_EDGE ( 'NONE', *, *, #15095, .T. ) ;
#86714=CARTESIAN_POINT ( 'NONE',  ( -2.980823821391186623, -9.357781135181031829, 34.66075350412533851 ) ) ;
#86715=ORIENTED_EDGE ( 'NONE', *, *, #44175, .F. ) ;
#86716=CARTESIAN_POINT ( 'NONE',  ( -15.10024352900566846, -6.001044277235009439, 34.52024696741798948 ) ) ;
#86718=CARTESIAN_POINT ( 'NONE',  ( -13.16183571563731647, -5.827830569534417471, 34.72679350104403539 ) ) ;
#86719=CARTESIAN_POINT ( 'NONE',  ( -15.48074597481782178, -12.41104346484419452, 31.60698883733904196 ) ) ;
#86720=CARTESIAN_POINT ( 'NONE',  ( -3.230769230769229949, -1.242168528481310874, 33.36296068462461051 ) ) ;
#86722=EDGE_CURVE ( 'NONE', #43377, #16890, #1431, .T. ) ;
#86723=B_SPLINE_CURVE_WITH_KNOTS ( 'NONE', 3,
 ( #44842, #10629, #24582, #25026, #74114, #38549, #31796, #39892, #11975, #39451 ),
 .UNSPECIFIED., .F., .F.,
 ( 4, 2, 2, 2, 4 ),
 ( 0.0007817246256747505334, 0.0009771112852218954894, 0.001172497944769040554, 0.001367884604316185618, 0.001563271263863330682 ),
 .UNSPECIFIED. ) ;
#86724=CARTESIAN_POINT ( 'NONE',  ( -4.946132635956127288, -2.494656445102013453, 31.33466734024120015 ) ) ;
#86725=CARTESIAN_POINT ( 'NONE',  ( -10.83831083290076158, -4.186968288167449259, 33.49512374952580274 ) ) ;
#86726=CARTESIAN_POINT ( 'NONE',  ( -14.30769230769242739, -5.219633306517616589, 34.19971097300220464 ) ) ;
#86728=B_SPLINE_CURVE_WITH_KNOTS ( 'NONE', 3,
 ( #31335, #2077, #43513, #52483, #79528, #11514, #4304, #38995, #60129, #53376 ),
 .UNSPECIFIED., .F., .F.,
 ( 4, 2, 2, 2, 4 ),
 ( 0.0007817359527651090859, 0.0009771254036996478414, 0.001172514854634186489, 0.001367904305568725136, 0.001563293756503263783 ),
 .UNSPECIFIED. ) ;
#86729=CARTESIAN_POINT ( 'NONE',  ( -11.53846153846165912, -3.835265460704628371, 33.15142922262033665 ) ) ;
#86730=CYLINDRICAL_SURFACE ( 'NONE', #37642, 0.2499999999999994726 ) ;
#86732=AXIS2_PLACEMENT_3D ( 'NONE', #38496, #65953, #2907 ) ;
#86733=VECTOR ( 'NONE', #81987, 1000.000000000000000 ) ;
#86734=EDGE_LOOP ( 'NONE', ( #8630, #12599, #54095, #26394 ) ) ;
#86735=VERTEX_POINT ( 'NONE', #22309 ) ;
#86736=CARTESIAN_POINT ( 'NONE',  ( -9.469528151039277475, -3.755027918224367323, 33.06320215134714857 ) ) ;
#86737=DIRECTION ( 'NONE',  ( 0.000000000000000000, 0.4999999999999960032, -0.8660254037844410391 ) ) ;
#86738=CARTESIAN_POINT ( 'NONE',  ( -8.769230769230890843, -11.48612834414049644, 32.76840700105863391 ) ) ;
#86739=CARTESIAN_POINT ( 'NONE',  ( -6.989159302437058408, -5.471508081941601986, 34.59228464037088457 ) ) ;
#86740=EDGE_CURVE ( 'NONE', #88101, #79653, #35895, .T. ) ;
#86741=CARTESIAN_POINT ( 'NONE',  ( 8.703147358274888390, -11.69971097300155272, 32.46337939537587403 ) ) ;
#86742=CARTESIAN_POINT ( 'NONE',  ( -16.40386939113911779, -9.271318131107980420, 34.42618302367067429 ) ) ;
#86743=ORIENTED_EDGE ( 'NONE', *, *, #24273, .T. ) ;
#86744=FACE_OUTER_BOUND ( 'NONE', #21079, .T. ) ;
#86745=VERTEX_POINT ( 'NONE', #28630 ) ;
#86746=ORIENTED_EDGE ( 'NONE', *, *, #75319, .T. ) ;
#86747=CARTESIAN_POINT ( 'NONE',  ( 0.4615384615383382183, -12.51329471203414379, 31.30864560766407578 ) ) ;
#86748=CARTESIAN_POINT ( 'NONE',  ( 4.023698944407933631, -2.619462340734462380, 30.83744416345203021 ) ) ;
#86749=CARTESIAN_POINT ( 'NONE',  ( 11.53846153846141753, -10.90142922262034020, 33.41473453929536674 ) ) ;
#86750=CARTESIAN_POINT ( 'NONE',  ( 11.66925197942848769, -2.295524264805589354, 30.44142389570982488 ) ) ;
#86751=FACE_OUTER_BOUND ( 'NONE', #16345, .T. ) ;
#86752=ORIENTED_EDGE ( 'NONE', *, *, #8186, .F. ) ;
#86753=VECTOR ( 'NONE', #69971, 1000.000000000000000 ) ;
#86754=VERTEX_POINT ( 'NONE', #23195 ) ;
#86755=ORIENTED_EDGE ( 'NONE', *, *, #25418, .T. ) ;
#86756=EDGE_CURVE ( 'NONE', #83108, #21723, #88556, .T. ) ;
#86758=CARTESIAN_POINT ( 'NONE',  ( -4.088591014333314178, -12.16647553114626490, 32.15551576947920864 ) ) ;
#86759=CARTESIAN_POINT ( 'NONE',  ( -0.2114840416250090560, -10.06805714834173848, 34.32951233291982618 ) ) ;
#86760=CYLINDRICAL_SURFACE ( 'NONE', #23545, 0.2499999999999973355 ) ;
#86762=CARTESIAN_POINT ( 'NONE',  ( 1.254468175177164246, -3.817052484675422797, 33.13202310037935661 ) ) ;
#86763=CARTESIAN_POINT ( 'NONE',  ( -11.66915214157184444, -8.191372820521381826, 34.95448215188424967 ) ) ;
#86764=EDGE_CURVE ( 'NONE', #26836, #61826, #77249, .T. ) ;
#86765=CARTESIAN_POINT ( 'NONE',  ( 5.777073782483852504, -12.39988816332205701, 30.74660775122750778 ) ) ;
#86766=ORIENTED_EDGE ( 'NONE', *, *, #23539, .T. ) ;
#86769=VERTEX_POINT ( 'NONE', #2033 ) ;
#86770=CARTESIAN_POINT ( 'NONE',  ( 2.530471848960717640, -12.44528174975671853, 30.48912976160716681 ) ) ;
#86771=ORIENTED_EDGE ( 'NONE', *, *, #85111, .T. ) ;
#86772=EDGE_CURVE ( 'NONE', #58985, #34772, #28392, .T. ) ;
#86773=CARTESIAN_POINT ( 'NONE',  ( -9.942284436356285227, -10.06842814019191401, 34.32929386961144758 ) ) ;
#86774=CARTESIAN_POINT ( 'NONE',  ( -2.177166869458662113, -4.299079248970732792, 33.91157788607253565 ) ) ;
#86776=ORIENTED_EDGE ( 'NONE', *, *, #36758, .F. ) ;
#86777=EDGE_CURVE ( 'NONE', #59229, #40827, #83131, .T. ) ;
#86778=CARTESIAN_POINT ( 'NONE',  ( -13.51476259405360913, -12.27039167877662251, 31.24851455888617835 ) ) ;
#86779=ORIENTED_EDGE ( 'NONE', *, *, #77286, .T. ) ;
#86780=CARTESIAN_POINT ( 'NONE',  ( 2.373760658694747061, -8.973038597847269315, 34.52809138561122637 ) ) ;
#86781=CYLINDRICAL_SURFACE ( 'NONE', #12695, 0.2500000000000012212 ) ;
#86782=AXIS2_PLACEMENT_3D ( 'NONE', #5577, #47436, #68165 ) ;
#86783=FACE_BOUND ( 'NONE', #10418, .T. ) ;
#86784=CARTESIAN_POINT ( 'NONE',  ( -0.2115930521604184600, -11.56426240980093567, 33.07394671870546432 ) ) ;
#86785=CARTESIAN_POINT ( 'NONE',  ( 7.846153846153846700, -2.292212530054420494, 30.41441678777542634 ) ) ;
#86786=AXIS2_PLACEMENT_3D ( 'NONE', #12087, #33236, #18834 ) ;
#86787=CARTESIAN_POINT ( 'NONE',  ( -3.100243529005666687, -6.852161475712352789, 34.70806712695775786 ) ) ;
#86788=CYLINDRICAL_SURFACE ( 'NONE', #63550, 0.2500000000000008882 ) ;
#86790=ADVANCED_FACE ( 'NONE', ( #29085 ), #16439, .F. ) ;
#86791=CARTESIAN_POINT ( 'NONE',  ( 6.792929713638703682, -8.587444163452046197, 34.63053765926554206 ) ) ;
#86792=CARTESIAN_POINT ( 'NONE',  ( 9.692307692307695177, -2.249999999999998668, 29.75000000000001776 ) ) ;
#86793=VERTEX_POINT ( 'NONE', #56539 ) ;
#86797=CARTESIAN_POINT ( 'NONE',  ( -13.25382494364843389, -11.37503395064541678, 33.29242100308974273 ) ) ;
#86798=CARTESIAN_POINT ( 'NONE',  ( -0.7115384615384606759, -7.500000000000001776, 34.75000000000000000 ) ) ;
#86799=ADVANCED_FACE ( 'NONE', ( #70941 ), #64164, .F. ) ;
#86800=FACE_BOUND ( 'NONE', #27700, .T. ) ;
#86801=CARTESIAN_POINT ( 'NONE',  ( 13.25446741488368829, -2.373036134822904319, 30.88089517874952250 ) ) ;
#86803=CARTESIAN_POINT ( 'NONE',  ( -9.692307692307691624, -11.91647553114624181, 32.58852847137148245 ) ) ;
#86806=DIRECTION ( 'NONE',  ( -0.000000000000000000, -0.7660444431189791237, -0.6427876096865379196 ) ) ;
#86807=CARTESIAN_POINT ( 'NONE',  ( -8.519176457592452678, -3.627508038966690496, 32.91356715214248396 ) ) ;
#86810=B_SPLINE_CURVE_WITH_KNOTS ( 'NONE', 3,
 ( #25170, #60281, #87794, #52637, #32377, #59843, #74254, #5350, #5792, #80579 ),
 .UNSPECIFIED., .F., .F.,
 ( 4, 2, 2, 2, 4 ),
 ( 0.000000000000000000, 0.0001954339857564062817, 0.0003908679715128125635, 0.0005863019572692188723, 0.0007817359430256251270 ),
 .UNSPECIFIED. ) ;
#86811=LINE ( 'NONE', #32721, #82120 ) ;
#86812=EDGE_LOOP ( 'NONE', ( #77158, #54487 ) ) ;
#86813=B_SPLINE_CURVE_WITH_KNOTS ( 'NONE', 3,
 ( #72118, #23486, #24369, #59050, #50942, #78878, #70016, #10432, #62799, #35348 ),
 .UNSPECIFIED., .F., .F.,
 ( 4, 2, 2, 2, 4 ),
 ( 0.000000000000000000, 0.0001954339857564097512, 0.0003908679715128195024, 0.0005863019572692292807, 0.0007817359430256390048 ),
 .UNSPECIFIED. ) ;
#86815=CARTESIAN_POINT ( 'NONE',  ( 17.99999999999987566, -2.657715359629662544, 31.77849191805970364 ) ) ;
#86817=CARTESIAN_POINT ( 'NONE',  ( -9.822454901745912181, -10.88202310037935661, 33.43294751532457099 ) ) ;
#86818=CARTESIAN_POINT ( 'NONE',  ( -4.377331078410484189, -4.988325925672468131, 34.36044203135681130 ) ) ;
#86819=DIRECTION ( 'NONE',  ( 0.000000000000000000, 0.000000000000000000, -1.000000000000000000 ) ) ;
#86821=DIRECTION ( 'NONE',  ( 0.000000000000000000, 0.3420201433256610524, 0.9396926207859113145 ) ) ;
#86823=EDGE_CURVE ( 'NONE', #51516, #38794, #24520, .T. ) ;
#86824=AXIS2_PLACEMENT_3D ( 'NONE', #149, #54194, #27619 ) ;
#86825=CARTESIAN_POINT ( 'NONE',  ( 8.069165197766697162, -11.76359900205217635, 32.36225158514719880 ) ) ;
#86826=CARTESIAN_POINT ( 'NONE',  ( 9.561617089197383734, -3.957541250942358424, 33.62499894934981626 ) ) ;
#86827=CARTESIAN_POINT ( 'NONE',  ( 8.703960323269994248, -10.21337939537584383, 33.94971097300158647 ) ) ;
#86830=CARTESIAN_POINT ( 'NONE',  ( -2.242499319397651458, -2.255955759149235629, 29.99999999999988631 ) ) ;
#86831=EDGE_CURVE ( 'NONE', #32696, #79428, #54057, .T. ) ;
#86832=CARTESIAN_POINT ( 'NONE',  ( 17.29970274590113632, -8.540255544307068902, 34.89611431652622286 ) ) ;
#86833=EDGE_LOOP ( 'NONE', ( #60245, #73865, #60509, #19697 ) ) ;
#86834=DIRECTION ( 'NONE',  ( 0.000000000000000000, 0.1736481776669275834, 0.9848077530122086864 ) ) ;
#86835=CARTESIAN_POINT ( 'NONE',  ( 13.38461538461538680, -5.415277668671390821, 36.20867863119892149 ) ) ;
#86837=CARTESIAN_POINT ( 'NONE',  ( 6.066068351002440906, -4.098570777380720287, 33.41473453929635440 ) ) ;
#86838=CARTESIAN_POINT ( 'NONE',  ( -16.82697766754503377, -5.766571408460170467, 34.70601412856602508 ) ) ;
#86839=ORIENTED_EDGE ( 'NONE', *, *, #10809, .F. ) ;
#86840=CARTESIAN_POINT ( 'NONE',  ( -17.93393266664992325, -6.343179335718452272, 34.87096338111212646 ) ) ;
#86841=CARTESIAN_POINT ( 'NONE',  ( -16.85414340794500276, -9.418065098278011860, 34.63729479722530158 ) ) ;
#86842=CARTESIAN_POINT ( 'NONE',  ( 4.946775107191377252, -12.50552854090298993, 31.33409797877408920 ) ) ;
#86844=CARTESIAN_POINT ( 'NONE',  ( 18.00000000000000000, -2.900454961884010974, 35.62045528018868623 ) ) ;
#86845=CARTESIAN_POINT ( 'NONE',  ( 12.68431800280686694, -12.44528174975671853, 30.48912976160716681 ) ) ;
#86846=EDGE_CURVE ( 'NONE', #19730, #63457, #72712, .T. ) ;
#86847=DIRECTION ( 'NONE',  ( 0.000000000000000000, 0.9848077530122072432, 0.1736481776669354937 ) ) ;
#86848=CARTESIAN_POINT ( 'NONE',  ( -15.93088301957948083, -7.369474539155830506, 34.99858011523957657 ) ) ;
#86849=ADVANCED_FACE ( 'NONE', ( #44333 ), #37144, .F. ) ;
#86850=ORIENTED_EDGE ( 'NONE', *, *, #53367, .T. ) ;
#86851=FACE_OUTER_BOUND ( 'NONE', #12512, .T. ) ;
#86852=CARTESIAN_POINT ( 'NONE',  ( 10.86533002476265786, -4.176053281294518804, 33.81426240980091791 ) ) ;
#86853=VECTOR ( 'NONE', #87201, 1000.000000000000000 ) ;
#86855=ORIENTED_EDGE ( 'NONE', *, *, #12899, .F. ) ;
#86859=AXIS2_PLACEMENT_3D ( 'NONE', #74904, #12309, #26263 ) ;
#86860=CARTESIAN_POINT ( 'NONE',  ( 12.68431813051652846, -10.23759521482555357, 34.22997729860117033 ) ) ;
#86862=LINE ( 'NONE', #65653, #27998 ) ;
#86863=CARTESIAN_POINT ( 'NONE',  ( -1.384615384615383471, -11.35647404775217417, 33.31231777344666511 ) ) ;
#86864=EDGE_LOOP ( 'NONE', ( #87043, #33138, #1977, #71188 ) ) ;
#86865=VERTEX_POINT ( 'NONE', #10576 ) ;
#86866=CARTESIAN_POINT ( 'NONE',  ( 4.153846153846154188, -5.471508081941601098, 34.59228464037088457 ) ) ;
#86867=ORIENTED_EDGE ( 'NONE', *, *, #18518, .F. ) ;
#86869=FACE_OUTER_BOUND ( 'NONE', #10604, .T. ) ;
#86870=CARTESIAN_POINT ( 'NONE',  ( -9.692307692307812417, -9.442884908241554243, 34.35708131394783038 ) ) ;
#86871=CARTESIAN_POINT ( 'NONE',  ( -8.769230769230892619, -11.06231777344772027, 33.60647404775119895 ) ) ;
#86872=EDGE_CURVE ( 'NONE', #17114, #27570, #58355, .T. ) ;
#86873=ORIENTED_EDGE ( 'NONE', *, *, #51685, .T. ) ;
#86874=ORIENTED_EDGE ( 'NONE', *, *, #60289, .F. ) ;
#86875=B_SPLINE_CURVE_WITH_KNOTS ( 'NONE', 3,
 ( #3075, #10292, #3960, #32341, #58909, #30989, #80081, #38201, #18829, #53037 ),
 .UNSPECIFIED., .F., .F.,
 ( 4, 2, 2, 2, 4 ),
 ( 0.0007817359430256288133, 0.0009771253907249948054, 0.001172514838424360689, 0.001367904286123726573, 0.001563293733823092457 ),
 .UNSPECIFIED. ) ;
#86876=AXIS2_PLACEMENT_3D ( 'NONE', #41122, #20841, #33036 ) ;
#86878=FACE_OUTER_BOUND ( 'NONE', #65445, .T. ) ;
#86879=ORIENTED_EDGE ( 'NONE', *, *, #79177, .F. ) ;
#86880=EDGE_CURVE ( 'NONE', #1867, #38306, #24079, .T. ) ;
#86881=CARTESIAN_POINT ( 'NONE',  ( 2.307692307692309264, -2.486705287966279876, 31.30864560766543647 ) ) ;
#86882=CARTESIAN_POINT ( 'NONE',  ( -0.3954711281883858121, -4.661471528628508665, 34.16647553114624003 ) ) ;
#86884=CARTESIAN_POINT ( 'NONE',  ( 6.673076923076918021, -2.499999999999999556, 29.81609845454691765 ) ) ;
#86885=CARTESIAN_POINT ( 'NONE',  ( -13.38461538461538325, -6.435427911321262684, 35.78748833219616898 ) ) ;
#86886=EDGE_CURVE ( 'NONE', #16317, #75626, #74500, .T. ) ;
#86887=LINE ( 'NONE', #66595, #39661 ) ;
#86888=FACE_BOUND ( 'NONE', #80417, .T. ) ;
#86890=CARTESIAN_POINT ( 'NONE',  ( -1.384615384615383471, -11.69971097300155272, 32.46337939537588113 ) ) ;
#86891=CARTESIAN_POINT ( 'NONE',  ( 11.78840705680968171, -12.43552623307873972, 30.55307653245132826 ) ) ;
#86893=CARTESIAN_POINT ( 'NONE',  ( 14.37294744720514572, -3.083524468853784839, 32.58852847137153930 ) ) ;
#86894=CARTESIAN_POINT ( 'NONE',  ( -4.219599582159485607, -7.249945578846651806, 34.99404164642496795 ) ) ;
#86895=CARTESIAN_POINT ( 'NONE',  ( -16.37733109757010652, -8.496056993536548418, 34.65000542017679663 ) ) ;
#86896=ORIENTED_EDGE ( 'NONE', *, *, #77999, .F. ) ;
#86897=CARTESIAN_POINT ( 'NONE',  ( -15.90384615384608757, -7.434744429011174383, 34.75000000000000711 ) ) ;
#86898=CARTESIAN_POINT ( 'NONE',  ( -13.63459212866397685, -9.234221910056348293, 34.70572697212741531 ) ) ;
#86899=ORIENTED_EDGE ( 'NONE', *, *, #29442, .F. ) ;
#86900=VERTEX_POINT ( 'NONE', #51988 ) ;
#86901=CARTESIAN_POINT ( 'NONE',  ( -11.53846153846166089, -12.70778746994576025, 30.41441678777401236 ) ) ;
#86902=CARTESIAN_POINT ( 'NONE',  ( 0.5923289025054107038, -8.191423895709840863, 34.95447573519442130 ) ) ;
#86903=EDGE_CURVE ( 'NONE', #58570, #16922, #87271, .T. ) ;
#86904=CARTESIAN_POINT ( 'NONE',  ( 16.21991348719623360, -6.343179335718452272, 34.87096338111212646 ) ) ;
#86905=CARTESIAN_POINT ( 'NONE',  ( 15.90386940979756858, -2.318417181685854978, 30.59732222474233865 ) ) ;
#86906=CARTESIAN_POINT ( 'NONE',  ( -15.00780632720774932, -7.369474270740069777, 34.74850911626239736 ) ) ;
#86907=EDGE_LOOP ( 'NONE', ( #84797, #51115 ) ) ;
#86908=CARTESIAN_POINT ( 'NONE',  ( 14.30769230769218758, -9.442884908241554243, 34.35708131394783038 ) ) ;
#86909=CARTESIAN_POINT ( 'NONE',  ( 18.24994540937804643, -2.589246495874658827, 31.60778113518102828 ) ) ;
#86911=CARTESIAN_POINT ( 'NONE',  ( 4.946231610255516387, -5.582088688514999397, 34.36776431015576350 ) ) ;
#86913=CYLINDRICAL_SURFACE ( 'NONE', #11469, 0.2499999999999994726 ) ;
#86916=CARTESIAN_POINT ( 'NONE',  ( 15.23076923076911093, -3.300289026999228881, 32.46337939537708905 ) ) ;
#86917=B_SPLINE_CURVE_WITH_KNOTS ( 'NONE', 3,
 ( #30910, #30476, #79110, #58378, #63821, #77338, #44415, #51612, #22831, #70136 ),
 .UNSPECIFIED., .F., .F.,
 ( 4, 2, 2, 2, 4 ),
 ( 0.0007817359430256399806, 0.0009771253907250089001, 0.001172514838424378036, 0.001367904286123746956, 0.001563293733823115875 ),
 .UNSPECIFIED. ) ;
#86919=VERTEX_POINT ( 'NONE', #59199 ) ;
#86920=EDGE_CURVE ( 'NONE', #77395, #23595, #71820, .T. ) ;
#86921=AXIS2_PLACEMENT_3D ( 'NONE', #81631, #11387, #5529 ) ;
#86922=VERTEX_POINT ( 'NONE', #10125 ) ;
#86923=CARTESIAN_POINT ( 'NONE',  ( -14.55766905174090020, -4.818429247618089661, 34.26397095200675125 ) ) ;
#86924=EDGE_CURVE ( 'NONE', #58859, #18418, #72267, .T. ) ;
#86925=CARTESIAN_POINT ( 'NONE',  ( 12.23871176905946001, -7.369208160676172348, 34.74850200257122879 ) ) ;
#86926=CARTESIAN_POINT ( 'NONE',  ( 4.153846153846460609, -2.506253911140614576, 30.00000000000323297 ) ) ;
#86927=CARTESIAN_POINT ( 'NONE',  ( -13.38461538461538325, -1.129524287112498415, 32.06866353760679544 ) ) ;
#86928=B_SPLINE_CURVE_WITH_KNOTS ( 'NONE', 3,
 ( #65201, #37737, #79173, #71964, #9389, #71080 ),
 .UNSPECIFIED., .F., .F.,
 ( 4, 2, 4 ),
 ( 1.769077770938648657E-17, 0.0001954756301636885322, 0.0003909512603273593376 ),
 .UNSPECIFIED. ) ;
#86929=CARTESIAN_POINT ( 'NONE',  ( 2.057692307692309708, -7.500000000000001776, 34.75000000000000000 ) ) ;
#86931=CARTESIAN_POINT ( 'NONE',  ( -11.66915214157184622, -9.084618155246140248, 34.75535874321725771 ) ) ;
#86932=CARTESIAN_POINT ( 'NONE',  ( 1.515407192440172857, -4.809403383903225304, 33.96459661697924304 ) ) ;
#86933=CARTESIAN_POINT ( 'NONE',  ( -5.076923076923199218, -2.379036618888197729, 30.90682066428292885 ) ) ;
#86934=CARTESIAN_POINT ( 'NONE',  ( 13.31853300525525086, -9.905515769479276145, 34.41647553114623292 ) ) ;
#86935=DIRECTION ( 'NONE',  ( 0.000000000000000000, 0.3420201433256641055, -0.9396926207859100932 ) ) ;
#86937=CYLINDRICAL_SURFACE ( 'NONE', #26531, 0.2500000000000004996 ) ;
#86938=CARTESIAN_POINT ( 'NONE',  ( 7.173022332454967120, -2.341251567377310217, 30.72681386836322659 ) ) ;
#86939=CARTESIAN_POINT ( 'NONE',  ( 10.86533013373276013, -2.824170634883621744, 31.52227843825338738 ) ) ;
#86940=EDGE_CURVE ( 'NONE', #44583, #61593, #84073, .T. ) ;
#86941=CARTESIAN_POINT ( 'NONE',  ( -4.284537620513710010, -8.999036380462719364, 34.52022231692819076 ) ) ;
#86942=CARTESIAN_POINT ( 'NONE',  ( -7.623374304885435215, -12.44528174975671853, 30.48912976160716681 ) ) ;
#86943=VERTEX_POINT ( 'NONE', #55876 ) ;
#86945=CARTESIAN_POINT ( 'NONE',  ( -5.207398261998797295, -7.276987145209185215, 34.99546412871779211 ) ) ;
#86946=DIRECTION ( 'NONE',  ( -0.000000000000000000, -0.9396926207859094271, -0.3420201433256663814 ) ) ;
#86949=CARTESIAN_POINT ( 'NONE',  ( -17.14300648787895653, -2.538708090699995257, 30.37095296980875148 ) ) ;
#86950=DIRECTION ( 'NONE',  ( -0.000000000000000000, 1.000000000000000000, -0.000000000000000000 ) ) ;
#86951=ORIENTED_EDGE ( 'NONE', *, *, #26863, .T. ) ;
#86953=CARTESIAN_POINT ( 'NONE',  ( 17.77651505627605033, -3.754499324213721234, 33.06261337010820256 ) ) ;
#86954=EDGE_CURVE ( 'NONE', #54130, #46293, #86311, .T. ) ;
#86955=EDGE_LOOP ( 'NONE', ( #79669, #41463 ) ) ;
#86956=AXIS2_PLACEMENT_3D ( 'NONE', #74047, #37575, #44770 ) ;
#86957=CARTESIAN_POINT ( 'NONE',  ( 18.22277954126840172, -9.332535724633405749, 34.40230450496446224 ) ) ;
#86958=EDGE_LOOP ( 'NONE', ( #53802, #19830 ) ) ;
#86959=CARTESIAN_POINT ( 'NONE',  ( -18.25002323729296450, -11.86270091957321249, 32.19358267280088626 ) ) ;
#86960=EDGE_CURVE ( 'NONE', #15487, #85101, #52934, .T. ) ;
#86961=EDGE_CURVE ( 'NONE', #31770, #72596, #20328, .T. ) ;
#86962=CARTESIAN_POINT ( 'NONE',  ( -15.48074597481782178, -2.920706130388546651, 32.31842814019191223 ) ) ;
#86963=CARTESIAN_POINT ( 'NONE',  ( 15.36129493253279321, -2.882268652242222284, 31.66798894389554064 ) ) ;
#86964=ORIENTED_EDGE ( 'NONE', *, *, #29966, .T. ) ;
#86965=CARTESIAN_POINT ( 'NONE',  ( 0.2386115026316110443, -4.762599654559228846, 34.23009711892697737 ) ) ;
#86966=EDGE_LOOP ( 'NONE', ( #42187, #15725 ) ) ;
#86967=DIRECTION ( 'NONE',  ( -0.000000000000000000, -0.5000000000000009992, -0.8660254037844380415 ) ) ;
#86969=ADVANCED_FACE ( 'NONE', ( #47793 ), #75274, .F. ) ;
#86971=CARTESIAN_POINT ( 'NONE',  ( 13.63456090296352841, -11.86320923018887719, 32.19269448109604070 ) ) ;
#86972=CARTESIAN_POINT ( 'NONE',  ( 0.5267940328144851136, -11.48612834413965977, 32.76840700105972815 ) ) ;
#86973=FACE_OUTER_BOUND ( 'NONE', #22261, .T. ) ;
#86974=CARTESIAN_POINT ( 'NONE',  ( -4.153846153846152411, -12.29105614889573062, 35.45975837776705220 ) ) ;
#86975=CARTESIAN_POINT ( 'NONE',  ( 0.3962684609821414683, -2.379036618887870880, 30.90682066428147579 ) ) ;
#86976=DIRECTION ( 'NONE',  ( -0.000000000000000000, 0.1736481776669307198, -0.9848077530122080203 ) ) ;
#86977=ORIENTED_EDGE ( 'NONE', *, *, #1628, .T. ) ;
#86978=ORIENTED_EDGE ( 'NONE', *, *, #45390, .T. ) ;
#86979=ORIENTED_EDGE ( 'NONE', *, *, #86699, .T. ) ;
#86980=CARTESIAN_POINT ( 'NONE',  ( 3.453548899747295398, -12.69155399931963046, 30.53255429739157734 ) ) ;
#86981=ORIENTED_EDGE ( 'NONE', *, *, #63795, .F. ) ;
#86983=AXIS2_PLACEMENT_3D ( 'NONE', #2802, #10015, #83927 ) ;
#86984=CARTESIAN_POINT ( 'NONE',  ( -8.769230769230890843, -10.21337939537710326, 33.94971097300076224 ) ) ;
#86985=CARTESIAN_POINT ( 'NONE',  ( 9.442284468086237226, -5.765609946408404518, 34.70566812827425451 ) ) ;
#86986=ORIENTED_EDGE ( 'NONE', *, *, #27379, .F. ) ;
#86988=B_SPLINE_CURVE_WITH_KNOTS ( 'NONE', 3,
 ( #73045, #18994, #46460, #28864, #49118, #83812, #28401, #54990, #22095, #8587 ),
 .UNSPECIFIED., .F., .F.,
 ( 4, 2, 2, 2, 4 ),
 ( 0.0007817359430256338006, 0.0009771253907250062980, 0.001172514838424371531, 0.001367904286123736981, 0.001563293733823102431 ),
 .UNSPECIFIED. ) ;
#86989=ORIENTED_EDGE ( 'NONE', *, *, #14845, .T. ) ;
#86990=CARTESIAN_POINT ( 'NONE',  ( 17.07692307692307665, -9.058645607665452459, 34.76329471203371924 ) ) ;
#86992=CARTESIAN_POINT ( 'NONE',  ( -18.25002322422145440, -9.356822207818510151, 34.66110646841856635 ) ) ;
#86993=CARTESIAN_POINT ( 'NONE',  ( -11.53846153846165912, -3.835265460704628371, 33.15142922262033665 ) ) ;
#86994=CARTESIAN_POINT ( 'NONE',  ( 0.2386122440223127639, -4.887634598454295265, 34.01352882383564946 ) ) ;
#86995=FACE_BOUND ( 'NONE', #20689, .T. ) ;
#86996=CARTESIAN_POINT ( 'NONE',  ( 2.557692307692244871, -7.565270445406050648, 34.75000000000000000 ) ) ;
#86997=FACE_OUTER_BOUND ( 'NONE', #341, .T. ) ;
#86998=CARTESIAN_POINT ( 'NONE',  ( -1.384615384615506484, -2.379036618888197285, 30.90682066428292885 ) ) ;
#86999=CARTESIAN_POINT ( 'NONE',  ( -14.08468095607945969, -5.667800583137506010, 34.40243808032445827 ) ) ;
#87000=CARTESIAN_POINT ( 'NONE',  ( -4.826977667545033768, -4.176053281294514363, 33.81426240980091791 ) ) ;
#87001=CARTESIAN_POINT ( 'NONE',  ( -1.384615384615505151, -2.625532179533778709, 30.86335684631627174 ) ) ;
#87002=ORIENTED_EDGE ( 'NONE', *, *, #56978, .T. ) ;
#87003=CARTESIAN_POINT ( 'NONE',  ( -0.4615384615384611200, -1.242168528481310874, 33.36296068462461051 ) ) ;
#87004=EDGE_LOOP ( 'NONE', ( #49088, #28461, #40959, #51767 ) ) ;
#87005=VERTEX_POINT ( 'NONE', #83363 ) ;
#87006=VECTOR ( 'NONE', #82260, 1000.000000000000227 ) ;
#87007=CARTESIAN_POINT ( 'NONE',  ( 4.153846153846154188, -10.89733346790207413, 36.13435417666054406 ) ) ;
#87008=CARTESIAN_POINT ( 'NONE',  ( -1.384615384615383471, -5.471508081941601098, 34.59228464037088457 ) ) ;
#87009=DIRECTION ( 'NONE',  ( -0.000000000000000000, 0.1736481776669307198, -0.9848077530122080203 ) ) ;
#87010=CARTESIAN_POINT ( 'NONE',  ( -4.023320452082589149, -4.459921816937789885, 33.71989282347011851 ) ) ;
#87011=CARTESIAN_POINT ( 'NONE',  ( 17.07692307692307665, -8.120952969808772792, 34.71129190930000163 ) ) ;
#87012=CARTESIAN_POINT ( 'NONE',  ( -15.48074596171158746, -3.627789207965226748, 32.91389620160131102 ) ) ;
#87014=CARTESIAN_POINT ( 'NONE',  ( 16.94677586748485965, -6.001485441113818986, 34.52039167877662607 ) ) ;
#87015=CARTESIAN_POINT ( 'NONE',  ( 14.17700084102474989, -11.18331474514187995, 33.13161551792790505 ) ) ;
#87016=CARTESIAN_POINT ( 'NONE',  ( 10.36540787133602493, -2.920706130388546651, 32.31842814019191223 ) ) ;
#87017=CARTESIAN_POINT ( 'NONE',  ( 5.142068856255039400, -7.750023238201980469, 34.74374492549440419 ) ) ;
#87018=ORIENTED_EDGE ( 'NONE', *, *, #12855, .F. ) ;
#87019=ORIENTED_EDGE ( 'NONE', *, *, #57096, .T. ) ;
#87022=ORIENTED_EDGE ( 'NONE', *, *, #32423, .T. ) ;
#87023=CARTESIAN_POINT ( 'NONE',  ( 17.75000000000000000, -7.433931650972299465, 34.75000000000000711 ) ) ;
#87024=CARTESIAN_POINT ( 'NONE',  ( -7.623142494540996239, -4.887748414852790546, 34.01359900205216746 ) ) ;
#87025=VERTEX_POINT ( 'NONE', #75702 ) ;
#87026=CARTESIAN_POINT ( 'NONE',  ( -14.30769230769242917, -3.643525952248795718, 33.31231777344771672 ) ) ;
#87027=LINE ( 'NONE', #8584, #58639 ) ;
#87028=CARTESIAN_POINT ( 'NONE',  ( 5.076923076922954969, -2.892918686052165622, 31.69288490824153470 ) ) ;
#87029=CARTESIAN_POINT ( 'NONE',  ( 9.019176178608812933, -3.520799739797214389, 33.17531984108286025 ) ) ;
#87030=LINE ( 'NONE', #79361, #69070 ) ;
#87031=VERTEX_POINT ( 'NONE', #13126 ) ;
#87032=CARTESIAN_POINT ( 'NONE',  ( -0.3954711281883857565, -11.91647553114624358, 32.58852847137148245 ) ) ;
#87033=VERTEX_POINT ( 'NONE', #55434 ) ;
#87034=CARTESIAN_POINT ( 'NONE',  ( -17.07692307692307665, -3.886160181151819604, 36.00935417666054406 ) ) ;
#87035=CYLINDRICAL_SURFACE ( 'NONE', #6739, 0.2499999999999997502 ) ;
#87036=DIRECTION ( 'NONE',  ( 1.000000000000000000, 0.000000000000000000, 0.000000000000000000 ) ) ;
#87037=CARTESIAN_POINT ( 'NONE',  ( 15.45354877203763522, -12.44528174975671853, 30.48912976160716681 ) ) ;
#87038=CARTESIAN_POINT ( 'NONE',  ( -5.749999999999999112, -2.249999999999998668, 29.75000000000000355 ) ) ;
#87039=AXIS2_PLACEMENT_3D ( 'NONE', #69481, #28500, #84787 ) ;
#87040=EDGE_CURVE ( 'NONE', #1104, #5084, #16414, .T. ) ;
#87041=LINE ( 'NONE', #25315, #10451 ) ;
#87043=ORIENTED_EDGE ( 'NONE', *, *, #62332, .F. ) ;
#87044=CARTESIAN_POINT ( 'NONE',  ( 14.24160992833216888, -2.292212530054419606, 30.41441678777542634 ) ) ;
#87045=CARTESIAN_POINT ( 'NONE',  ( 18.00000000000000000, -3.937682226553329556, 33.60647404775216529 ) ) ;
#87046=DIRECTION ( 'NONE',  ( -0.000000000000000000, 0.8660254037844399289, -0.4999999999999980016 ) ) ;
#87047=ORIENTED_EDGE ( 'NONE', *, *, #27251, .F. ) ;
#87048=VERTEX_POINT ( 'NONE', #7706 ) ;
#87049=CARTESIAN_POINT ( 'NONE',  ( -5.749945580086545327, -12.65882529074907126, 30.72640787790839312 ) ) ;
#87050=CARTESIAN_POINT ( 'NONE',  ( 7.716005876422151744, -6.809168938359901446, 34.95455904226513866 ) ) ;
#87051=B_SPLINE_CURVE_WITH_KNOTS ( 'NONE', 3,
 ( #20250, #89168, #27449, #20685, #69324, #76068, #60783, #27890, #54918, #13925 ),
 .UNSPECIFIED., .F., .F.,
 ( 4, 2, 2, 2, 4 ),
 ( 0.000000000000000000, 0.0001954339857564097512, 0.0003908679715128195024, 0.0005863019572692292807, 0.0007817359430256390048 ),
 .UNSPECIFIED. ) ;
#87053=CARTESIAN_POINT ( 'NONE',  ( -0.4615384615385840772, -9.528491918059723176, 34.59228464037033035 ) ) ;
#87054=CARTESIAN_POINT ( 'NONE',  ( 15.90382292962469535, -10.18141759479407327, 34.26406193332782379 ) ) ;
#87055=B_SPLINE_CURVE_WITH_KNOTS ( 'NONE', 3,
 ( #9507, #1429, #78407, #28921, #36974, #16708, #71647, #64887, #3192, #22148 ),
 .UNSPECIFIED., .F., .F.,
 ( 4, 2, 2, 2, 4 ),
 ( 0.000000000000000000, 0.0001954311564186862781, 0.0003908623128373725562, 0.0005862934692560588072, 0.0007817246256747451124 ),
 .UNSPECIFIED. ) ;
#87056=CARTESIAN_POINT ( 'NONE',  ( 10.61538461538449596, -9.442884908241554243, 34.35708131394783038 ) ) ;
#87057=CYLINDRICAL_SURFACE ( 'NONE', #17789, 0.2499999999999994726 ) ;
#87058=ORIENTED_EDGE ( 'NONE', *, *, #15275, .T. ) ;
#87059=CARTESIAN_POINT ( 'NONE',  ( 5.933916589044120116, -3.513871655860377086, 32.76840700105978499 ) ) ;
#87060=EDGE_CURVE ( 'NONE', #8641, #2295, #36838, .T. ) ;
#87061=ADVANCED_FACE ( 'NONE', ( #21650 ), #49121, .F. ) ;
#87062=LINE ( 'NONE', #39751, #38345 ) ;
#87063=CARTESIAN_POINT ( 'NONE',  ( 16.85399685940691938, -9.086856451489516928, 34.49173150075333183 ) ) ;
#87064=ORIENTED_EDGE ( 'NONE', *, *, #2057, .T. ) ;
#87065=CARTESIAN_POINT ( 'NONE',  ( 15.90382292962469180, -12.45566812827425096, 31.48439005359158926 ) ) ;
#87066=VERTEX_POINT ( 'NONE', #63066 ) ;
#87068=DIRECTION ( 'NONE',  ( 0.000000000000000000, 0.7660444431189807890, 0.6427876096865361433 ) ) ;
#87070=CARTESIAN_POINT ( 'NONE',  ( -13.38461538461538325, -3.669653830205710676, 35.88435417666054406 ) ) ;
#87071=ORIENTED_EDGE ( 'NONE', *, *, #20823, .T. ) ;
#87072=CARTESIAN_POINT ( 'NONE',  ( 0.5267940328144853357, -4.481592998940251427, 33.73612834413965089 ) ) ;
#87073=CARTESIAN_POINT ( 'NONE',  ( 13.44987052412822059, -9.528491918058460186, 34.59228464037086326 ) ) ;
#87075=VECTOR ( 'NONE', #61192, 1000.000000000000227 ) ;
#87076=DIRECTION ( 'NONE',  ( -0.000000000000000000, -0.8660254037844399289, -0.4999999999999980016 ) ) ;
#87077=CARTESIAN_POINT ( 'NONE',  ( 3.361294669002873103, -3.068774925481847493, 32.56582465632704526 ) ) ;
#87079=CARTESIAN_POINT ( 'NONE',  ( -17.07692307692319744, -11.48612834414049644, 32.76840700105863391 ) ) ;
#87080=ORIENTED_EDGE ( 'NONE', *, *, #77256, .T. ) ;
#87081=CARTESIAN_POINT ( 'NONE',  ( 5.142990410273153401, -11.35647404775217595, 33.31231777344667222 ) ) ;
#87082=CARTESIAN_POINT ( 'NONE',  ( -13.38461538461538325, -1.422936976036506707, 30.56769352161908415 ) ) ;
#87083=CARTESIAN_POINT ( 'NONE',  ( -16.15384615384615330, -13.75783147151868846, 33.36296068462461051 ) ) ;
#87084=CARTESIAN_POINT ( 'NONE',  ( 18.00000000000000000, -12.62096338111211580, 30.90682066428153263 ) ) ;
#87085=DIRECTION ( 'NONE',  ( -0.000000000000000000, 0.1736481776669307198, -0.9848077530122080203 ) ) ;
#87086=CARTESIAN_POINT ( 'NONE',  ( 7.846153846153846700, -6.386643153685126251, 34.62446782046654192 ) ) ;
#87088=ORIENTED_EDGE ( 'NONE', *, *, #78257, .T. ) ;
#87089=VERTEX_POINT ( 'NONE', #31052 ) ;
#87090=VERTEX_POINT ( 'NONE', #16654 ) ;
#87091=EDGE_LOOP ( 'NONE', ( #29177, #57118 ) ) ;
#87093=CARTESIAN_POINT ( 'NONE',  ( -4.376772371362299907, -5.667676309546437530, 34.40238873228292249 ) ) ;
#87094=CARTESIAN_POINT ( 'NONE',  ( -2.176900499867521432, -3.062576670634119758, 32.05464942895959979 ) ) ;
#87095=CARTESIAN_POINT ( 'NONE',  ( -4.088590582570127197, -9.442884908240271713, 34.35708131394835618 ) ) ;
#87097=CARTESIAN_POINT ( 'NONE',  ( 13.31934493865461278, -8.613356846314824011, 34.62446782046655613 ) ) ;
#87098=CARTESIAN_POINT ( 'NONE',  ( 3.100077764101672795, -5.582088688514999397, 34.36776431015576350 ) ) ;
#87099=CARTESIAN_POINT ( 'NONE',  ( -5.326946314216042033, -8.432397168068783699, 34.66272746175022945 ) ) ;
#87100=CARTESIAN_POINT ( 'NONE',  ( 9.626225312947559232, -9.905515769479276145, 34.41647553114623292 ) ) ;
#87101=DIRECTION ( 'NONE',  ( -0.000000000000000000, 0.8660254037844397068, -0.4999999999999978906 ) ) ;
#87102=ORIENTED_EDGE ( 'NONE', *, *, #87743, .F. ) ;
#87103=VECTOR ( 'NONE', #84216, 1000.000000000000114 ) ;
#87105=EDGE_CURVE ( 'NONE', #52314, #50355, #27108, .T. ) ;
#87106=VERTEX_POINT ( 'NONE', #37365 ) ;
#87107=CARTESIAN_POINT ( 'NONE',  ( 18.00000000000000000, -1.129524287112498415, 32.06866353760679544 ) ) ;
#87108=VERTEX_POINT ( 'NONE', #77045 ) ;
#87109=CARTESIAN_POINT ( 'NONE',  ( 16.28463796167094202, -11.71459661697925903, 32.44059661609676937 ) ) ;
#87111=FACE_OUTER_BOUND ( 'NONE', #43511, .T. ) ;
#87112=DIRECTION ( 'NONE',  ( -0.000000000000000000, -0.9396926207859092051, -0.3420201433256662704 ) ) ;
#87113=FACE_BOUND ( 'NONE', #19165, .T. ) ;
#87114=ORIENTED_EDGE ( 'NONE', *, *, #4064, .F. ) ;
#87115=B_SPLINE_CURVE_WITH_KNOTS ( 'NONE', 3,
 ( #71468, #43560, #36805, #85005, #63834, #28734, #76914, #77790, #9776, #16530 ),
 .UNSPECIFIED., .F., .F.,
 ( 4, 2, 2, 2, 4 ),
 ( 0.0007817246256747442451, 0.0009771112852218865989, 0.001172497944769029061, 0.001367884604316171523, 0.001563271263863313986 ),
 .UNSPECIFIED. ) ;
#87117=CARTESIAN_POINT ( 'NONE',  ( -2.084316366994122482, -2.501478030877322567, 29.88021232661720816 ) ) ;
#87118=EDGE_LOOP ( 'NONE', ( #17866, #43866, #14024, #22397 ) ) ;
#87119=FACE_BOUND ( 'NONE', #4215, .T. ) ;
#87120=CARTESIAN_POINT ( 'NONE',  ( -10.86540783960607115, -2.985938066672154445, 32.43141759479405550 ) ) ;
#87121=EDGE_CURVE ( 'NONE', #50871, #46562, #30613, .T. ) ;
#87122=CARTESIAN_POINT ( 'NONE',  ( 7.911346834448499621, -2.255955759149235629, 29.99999999999988631 ) ) ;
#87123=ORIENTED_EDGE ( 'NONE', *, *, #84967, .T. ) ;
#87124=CARTESIAN_POINT ( 'NONE',  ( -15.10024352900566669, -12.27024696741798948, 31.24895572276497546 ) ) ;
#87126=CARTESIAN_POINT ( 'NONE',  ( -5.011778296203443617, -7.750023224968867197, 34.99404313364389907 ) ) ;
#87127=ORIENTED_EDGE ( 'NONE', *, *, #88082, .T. ) ;
#87128=EDGE_CURVE ( 'NONE', #74921, #47387, #77480, .T. ) ;
#87129=DIRECTION ( 'NONE',  ( 0.000000000000000000, 0.7660444431189807890, 0.6427876096865361433 ) ) ;
#87130=CARTESIAN_POINT ( 'NONE',  ( 6.923076923076924238, -5.471508081941601098, 34.59228464037088457 ) ) ;
#87131=CYLINDRICAL_SURFACE ( 'NONE', #46148, 0.2499999999999994726 ) ;
#87132=EDGE_LOOP ( 'NONE', ( #660, #2807, #19879, #72441 ) ) ;
#87133=DIRECTION ( 'NONE',  ( -0.000000000000000000, 0.5000000000000011102, -0.8660254037844380415 ) ) ;
#87134=DIRECTION ( 'NONE',  ( 0.000000000000000000, 0.4999999999999985567, 0.8660254037844395958 ) ) ;
#87135=ORIENTED_EDGE ( 'NONE', *, *, #88355, .F. ) ;
#87136=CARTESIAN_POINT ( 'NONE',  ( -17.32694630114453460, -12.68155406624981119, 30.59749803192733708 ) ) ;
#87137=CARTESIAN_POINT ( 'NONE',  ( 14.55774661933062575, -8.303483539816731707, 34.68545999027711702 ) ) ;
#87138=CARTESIAN_POINT ( 'NONE',  ( 1.384615384615264011, -12.16647553114689728, 32.15551576947799362 ) ) ;
#87139=CARTESIAN_POINT ( 'NONE',  ( 8.069116749715332659, -7.369474270740070665, 34.74850911626239025 ) ) ;
#87140=CYLINDRICAL_SURFACE ( 'NONE', #73240, 0.2499999999999995559 ) ;
#87141=CARTESIAN_POINT ( 'NONE',  ( 0.4615384615384611200, -12.10708131394839349, 31.69288490824020244 ) ) ;
#87144=EDGE_CURVE ( 'NONE', #24035, #13064, #86015, .T. ) ;
#87145=CARTESIAN_POINT ( 'NONE',  ( 8.769230769230768274, -2.486705287966279876, 31.30864560766543647 ) ) ;
#87146=DIRECTION ( 'NONE',  ( 0.000000000000000000, 0.9848077530122072432, 0.1736481776669354937 ) ) ;
#87149=FACE_OUTER_BOUND ( 'NONE', #58242, .T. ) ;
#87150=EDGE_LOOP ( 'NONE', ( #69995, #52489, #7545, #44920 ) ) ;
#87151=EDGE_CURVE ( 'NONE', #74998, #87392, #20724, .T. ) ;
#87153=CARTESIAN_POINT ( 'NONE',  ( -16.94639763868943660, -4.299079248970731015, 33.91157788607253565 ) ) ;
#87154=ORIENTED_EDGE ( 'NONE', *, *, #58857, .F. ) ;
#87155=CARTESIAN_POINT ( 'NONE',  ( 18.24999999999993250, -7.565270445406050648, 34.75000000000000000 ) ) ;
#87158=CARTESIAN_POINT ( 'NONE',  ( 10.74591005361825680, -2.647132371071621471, 31.75357179365171589 ) ) ;
#87159=DIRECTION ( 'NONE',  ( 0.000000000000000000, 0.4999999999999960032, -0.8660254037844410391 ) ) ;
#87160=CARTESIAN_POINT ( 'NONE',  ( -14.55766905174089665, -10.82459398097509329, 33.81372124010185587 ) ) ;
#87161=LINE ( 'NONE', #46160, #28865 ) ;
#87162=CARTESIAN_POINT ( 'NONE',  ( -8.769230769230768274, -12.29105614889573062, 35.45975837776705220 ) ) ;
#87163=CYLINDRICAL_SURFACE ( 'NONE', #48271, 0.2499999999999995837 ) ;
#87164=B_SPLINE_CURVE_WITH_KNOTS ( 'NONE', 3,
 ( #44044, #23336, #10722, #30975, #51224, #79626, #58441, #50793, #37293, #17030 ),
 .UNSPECIFIED., .F., .F.,
 ( 4, 2, 2, 2, 4 ),
 ( 0.0007817359430256285964, 0.0009771253907249943717, 0.001172514838424360255, 0.001367904286123726139, 0.001563293733823092023 ),
 .UNSPECIFIED. ) ;
#87167=CARTESIAN_POINT ( 'NONE',  ( 17.07692307692295586, -2.379036618888197729, 30.90682066428292885 ) ) ;
#87168=CARTESIAN_POINT ( 'NONE',  ( -10.36538461538461320, -2.249999999999998668, 29.75000000000000355 ) ) ;
#87169=EDGE_CURVE ( 'NONE', #17395, #29922, #50869, .T. ) ;
#87170=EDGE_CURVE ( 'NONE', #30322, #28929, #64390, .T. ) ;
#87171=LINE ( 'NONE', #25447, #69437 ) ;
#87172=ORIENTED_EDGE ( 'NONE', *, *, #56584, .T. ) ;
#87173=VERTEX_POINT ( 'NONE', #23843 ) ;
#87175=CARTESIAN_POINT ( 'NONE',  ( -11.31545018684868786, -5.667800583137506010, 34.40243808032445827 ) ) ;
#87176=CARTESIAN_POINT ( 'NONE',  ( 7.596130608860880429, -11.37209801155882971, 32.91403422569032955 ) ) ;
#87177=CARTESIAN_POINT ( 'NONE',  ( -2.438382910802614045, -2.295517848115769421, 30.44137282052137294 ) ) ;
#87178=FACE_OUTER_BOUND ( 'NONE', #43374, .T. ) ;
#87179=EDGE_CURVE ( 'NONE', #64886, #50355, #29309, .T. ) ;
#87180=AXIS2_PLACEMENT_3D ( 'NONE', #29172, #85871, #84556 ) ;
#87181=CARTESIAN_POINT ( 'NONE',  ( 8.703147358274888390, -4.098570777380720287, 33.41473453929634729 ) ) ;
#87182=CARTESIAN_POINT ( 'NONE',  ( 7.846153846153846700, -9.819645486525091727, 36.12317359536749706 ) ) ;
#87183=ORIENTED_EDGE ( 'NONE', *, *, #35859, .F. ) ;
#87184=CARTESIAN_POINT ( 'NONE',  ( -4.853911725310226188, -12.39991518177334129, 30.74647679643404530 ) ) ;
#87185=EDGE_LOOP ( 'NONE', ( #67002, #80555, #29733, #34119 ) ) ;
#87186=EDGE_LOOP ( 'NONE', ( #26221, #68561, #16846, #16749 ) ) ;
#87188=CARTESIAN_POINT ( 'NONE',  ( -14.30769230769242917, -6.835583212225970762, 34.95778746994575670 ) ) ;
#87190=CARTESIAN_POINT ( 'NONE',  ( -9.469296340694841163, -6.503523203565941380, 34.64991518177335195 ) ) ;
#87191=CARTESIAN_POINT ( 'NONE',  ( 6.000000000000001776, -8.164416787775445883, 34.95778746994557906 ) ) ;
#87192=CARTESIAN_POINT ( 'NONE',  ( -5.207613680033384540, -8.191372820521381826, 34.95448215188423546 ) ) ;
#87193=VECTOR ( 'NONE', #50139, 1000.000000000000227 ) ;
#87194=EDGE_LOOP ( 'NONE', ( #78284, #57513, #13378, #25694 ) ) ;
#87195=EDGE_LOOP ( 'NONE', ( #68457, #16600, #42425, #12227 ) ) ;
#87196=B_SPLINE_CURVE_WITH_KNOTS ( 'NONE', 3,
 ( #79917, #60971, #25416, #53772, #88477, #33062, #18221, #74493, #18672, #66401 ),
 .UNSPECIFIED., .F., .F.,
 ( 4, 2, 2, 2, 4 ),
 ( 0.0007817246336856291692, 0.0009771112958940103739, 0.001172497958102391470, 0.001367884620310772566, 0.001563271282519153879 ),
 .UNSPECIFIED. ) ;
#87198=VERTEX_POINT ( 'NONE', #56761 ) ;
#87199=CARTESIAN_POINT ( 'NONE',  ( 17.20744851515672025, -10.31582465632704704, 34.18122507451815295 ) ) ;
#87200=DIRECTION ( 'NONE',  ( 0.000000000000000000, 1.000000000000000000, 0.000000000000000000 ) ) ;
#87201=DIRECTION ( 'NONE',  ( -0.000000000000000000, 1.000000000000000000, 3.491481338843133355E-15 ) ) ;
#87203=DIRECTION ( 'NONE',  ( -0.000000000000000000, 0.1736481776669307198, -0.9848077530122080203 ) ) ;
#87204=FACE_OUTER_BOUND ( 'NONE', #14992, .T. ) ;
#87208=CARTESIAN_POINT ( 'NONE',  ( 0.6843180028068708287, -11.89424750095246175, 32.13594075562311758 ) ) ;
#87209=ADVANCED_FACE ( 'NONE', ( #65287 ), #57209, .F. ) ;
#87210=CARTESIAN_POINT ( 'NONE',  ( -12.71151519248081740, -11.28823185664190376, 33.01397839955799896 ) ) ;
#87212=DIRECTION ( 'NONE',  ( -0.000000000000000000, -0.5000000000000009992, -0.8660254037844380415 ) ) ;
#87213=CARTESIAN_POINT ( 'NONE',  ( -9.692307692307691624, -11.69971097300155272, 32.46337939537588113 ) ) ;
#87214=AXIS2_PLACEMENT_3D ( 'NONE', #87034, #25308, #4593 ) ;
#87216=ORIENTED_EDGE ( 'NONE', *, *, #60319, .T. ) ;
#87217=CARTESIAN_POINT ( 'NONE',  ( -14.30769230769242917, -12.51329471203414379, 31.30864560766407578 ) ) ;
#87218=ORIENTED_EDGE ( 'NONE', *, *, #30467, .F. ) ;
#87219=CARTESIAN_POINT ( 'NONE',  ( 2.557746619330623528, -9.148310452688873440, 34.47095581063188519 ) ) ;
#87220=CARTESIAN_POINT ( 'NONE',  ( 14.30769230769231015, -12.34228464037088635, 31.77849191805839268 ) ) ;
#87222=DIRECTION ( 'NONE',  ( -0.000000000000000000, 1.000000000000000000, 3.491481338843133355E-15 ) ) ;
#87223=CYLINDRICAL_SURFACE ( 'NONE', #18627, 0.2500000000000002220 ) ;
#87224=EDGE_CURVE ( 'NONE', #61379, #51951, #50002, .T. ) ;
#87226=ORIENTED_EDGE ( 'NONE', *, *, #70824, .F. ) ;
#87227=CARTESIAN_POINT ( 'NONE',  ( 11.40831356872984514, -11.66186481527757302, 32.95055677023626117 ) ) ;
#87228=VECTOR ( 'NONE', #57241, 1000.000000000000000 ) ;
#87229=CARTESIAN_POINT ( 'NONE',  ( -8.769230769230768274, -3.937682226553329556, 33.60647404775216529 ) ) ;
#87230=EDGE_CURVE ( 'NONE', #46109, #72161, #67958, .T. ) ;
#87231=CARTESIAN_POINT ( 'NONE',  ( -15.23076923076922995, -11.33034616979429110, 35.88435417666054406 ) ) ;
#87232=EDGE_LOOP ( 'NONE', ( #74007, #196, #16853, #19365 ) ) ;
#87233=CARTESIAN_POINT ( 'NONE',  ( -6.923076923076922462, -1.509761064869970415, 31.06009739812519044 ) ) ;
#87234=CARTESIAN_POINT ( 'NONE',  ( 14.55774672760575861, -10.06805714834173493, 34.32951233291982618 ) ) ;
#87235=CYLINDRICAL_SURFACE ( 'NONE', #84529, 0.2500000000000002220 ) ;
#87236=CARTESIAN_POINT ( 'NONE',  ( -3.230769230769229949, -3.937682226553329556, 33.60647404775216529 ) ) ;
#87237=FACE_BOUND ( 'NONE', #66728, .T. ) ;
#87238=CARTESIAN_POINT ( 'NONE',  ( -0.4615384615384611200, -2.499999999999998668, 29.75000000000001421 ) ) ;
#87239=CARTESIAN_POINT ( 'NONE',  ( -18.00000000000000000, -1.812984705146277520, 34.52197243641129631 ) ) ;
#87240=EDGE_CURVE ( 'NONE', #83195, #1868, #80887, .T. ) ;
#87241=CARTESIAN_POINT ( 'NONE',  ( 9.692307692308000711, -2.506253911140615021, 30.00000000000323297 ) ) ;
#87242=CARTESIAN_POINT ( 'NONE',  ( 18.22277954126840172, -11.41317474335729543, 32.86274602512330034 ) ) ;
#87243=CARTESIAN_POINT ( 'NONE',  ( -11.28851612908349722, -10.92531984108285670, 33.72920026020278073 ) ) ;
#87245=CARTESIAN_POINT ( 'NONE',  ( 6.222779668978065004, -4.989023458446560255, 34.36081565061822118 ) ) ;
#87247=CARTESIAN_POINT ( 'NONE',  ( -7.053224132515143907, -9.418419913701741919, 34.36755862841477693 ) ) ;
#87248=EDGE_LOOP ( 'NONE', ( #29093, #58745 ) ) ;
#87249=DIRECTION ( 'NONE',  ( 0.000000000000000000, 1.000000000000000000, 0.000000000000000000 ) ) ;
#87250=B_SPLINE_CURVE_WITH_KNOTS ( 'NONE', 3,
 ( #62619, #35610, #83357, #49562, #48222, #75696, #49115, #68941, #42375, #83809 ),
 .UNSPECIFIED., .F., .F.,
 ( 4, 2, 2, 2, 4 ),
 ( 0.000000000000000000, 0.0001954339857564078809, 0.0003908679715128157619, 0.0005863019572692236428, 0.0007817359430256315238 ),
 .UNSPECIFIED. ) ;
#87251=CARTESIAN_POINT ( 'NONE',  ( 2.057715563643717438, -2.318417181685854533, 30.59732222474233865 ) ) ;
#87252=LINE ( 'NONE', #80937, #20112 ) ;
#87254=CARTESIAN_POINT ( 'NONE',  ( -17.07692307692319744, -2.379036618888197285, 30.90682066428292885 ) ) ;
#87255=CARTESIAN_POINT ( 'NONE',  ( -11.66860950819323506, -4.299443229763728169, 33.91186481527756058 ) ) ;
#87257=CARTESIAN_POINT ( 'NONE',  ( 15.23076923076923173, -3.513871655860378418, 32.76840700105978499 ) ) ;
#87258=DIRECTION ( 'NONE',  ( 0.000000000000000000, 0.7660444431189822323, -0.6427876096865344779 ) ) ;
#87259=VECTOR ( 'NONE', #79744, 1000.000000000000114 ) ;
#87261=CARTESIAN_POINT ( 'NONE',  ( 4.946775107191381693, -9.504002272028875709, 34.60269587691767867 ) ) ;
#87262=CARTESIAN_POINT ( 'NONE',  ( 6.988332494352947677, -4.481592998940251427, 33.73612834413965089 ) ) ;
#87263=CYLINDRICAL_SURFACE ( 'NONE', #36819, 0.2500000000000009437 ) ;
#87264=CARTESIAN_POINT ( 'NONE',  ( 9.442307692307693401, -7.500000000000001776, 34.75000000000000000 ) ) ;
#87265=EDGE_CURVE ( 'NONE', #2304, #36412, #79260, .T. ) ;
#87266=CARTESIAN_POINT ( 'NONE',  ( 1.384615384615386802, -3.886160181151819604, 36.00935417666054406 ) ) ;
#87267=VERTEX_POINT ( 'NONE', #86479 ) ;
#87268=CARTESIAN_POINT ( 'NONE',  ( -10.61538461538473399, -12.46129190930018460, 30.37095296980731973 ) ) ;
#87271=B_SPLINE_CURVE_WITH_KNOTS ( 'NONE', 3,
 ( #79484, #45237, #44785, #65952, #16880, #65510 ),
 .UNSPECIFIED., .F., .F.,
 ( 4, 2, 4 ),
 ( 0.0003909569690057848211, 0.0005862646681846116680, 0.0007815723673634385150 ),
 .UNSPECIFIED. ) ;
#87272=EDGE_CURVE ( 'NONE', #88008, #77586, #60757, .T. ) ;
#87273=CARTESIAN_POINT ( 'NONE',  ( -10.86536135943320502, -10.06842814019191401, 34.32929386961144758 ) ) ;
#87274=CARTESIAN_POINT ( 'NONE',  ( -16.28453675695646652, -10.70098750199973203, 33.91152734681376302 ) ) ;
#87275=ORIENTED_EDGE ( 'NONE', *, *, #70790, .F. ) ;
#87276=DIRECTION ( 'NONE',  ( 0.000000000000000000, 0.4999999999999985567, 0.8660254037844395958 ) ) ;
#87277=CARTESIAN_POINT ( 'NONE',  ( 9.561617089197389063, -12.62707690430377383, 30.88035979386743435 ) ) ;
#87278=CARTESIAN_POINT ( 'NONE',  ( 7.911408985666682270, -2.657715359629132301, 31.77849191805844242 ) ) ;
#87279=ORIENTED_EDGE ( 'NONE', *, *, #26907, .F. ) ;
#87280=CARTESIAN_POINT ( 'NONE',  ( -13.31854703361294590, -11.16473453929635440, 33.15142922261926373 ) ) ;
#87281=CARTESIAN_POINT ( 'NONE',  ( -3.165513659493205179, -3.835265460703683349, 33.15142922261929925 ) ) ;
#87282=EDGE_CURVE ( 'NONE', #40851, #55169, #52662, .T. ) ;
#87283=CARTESIAN_POINT ( 'NONE',  ( -5.999999999999998224, -2.721908614388771852, 31.22303859784724978 ) ) ;
#87284=CARTESIAN_POINT ( 'NONE',  ( 11.53846153846141753, -9.442884908241554243, 34.35708131394783038 ) ) ;
#87285=ORIENTED_EDGE ( 'NONE', *, *, #396, .F. ) ;
#87287=CARTESIAN_POINT ( 'NONE',  ( -8.769230769230892619, -2.657715359629662544, 31.77849191805970364 ) ) ;
#87288=AXIS2_PLACEMENT_3D ( 'NONE', #14576, #42061, #69517 ) ;
#87289=LINE ( 'NONE', #73771, #22587 ) ;
#87291=VERTEX_POINT ( 'NONE', #18890 ) ;
#87293=ORIENTED_EDGE ( 'NONE', *, *, #77886, .T. ) ;
#87294=CARTESIAN_POINT ( 'NONE',  ( 0.2386122440223130969, -8.239355502252617924, 34.69524867566427417 ) ) ;
#87295=CARTESIAN_POINT ( 'NONE',  ( 11.53846153846141753, -11.94971097300221174, 32.03036669348237098 ) ) ;
#87296=EDGE_CURVE ( 'NONE', #80807, #57115, #87366, .T. ) ;
#87298=CARTESIAN_POINT ( 'NONE',  ( -12.68502340526241312, -3.754499324213721234, 33.06261337010820256 ) ) ;
#87299=CARTESIAN_POINT ( 'NONE',  ( 15.90386942290380290, -4.943428324936578910, 34.04746400365624481 ) ) ;
#87300=ORIENTED_EDGE ( 'NONE', *, *, #50083, .T. ) ;
#87301=ADVANCED_FACE ( 'NONE', ( #80150 ), #59427, .F. ) ;
#87302=ORIENTED_EDGE ( 'NONE', *, *, #45316, .F. ) ;
#87303=ORIENTED_EDGE ( 'NONE', *, *, #77878, .T. ) ;
#87307=ADVANCED_FACE ( 'NONE', ( #72490 ), #4023, .F. ) ;
#87308=CARTESIAN_POINT ( 'NONE',  ( 0.4615384615384611200, -8.120952969808772792, 34.71129190930000163 ) ) ;
#87309=EDGE_CURVE ( 'NONE', #41914, #42943, #65865, .T. ) ;
#87310=AXIS2_PLACEMENT_3D ( 'NONE', #37515, #44256, #56901 ) ;
#87311=CARTESIAN_POINT ( 'NONE',  ( 1.450683735617823933, -10.51840700105979565, 33.73612834413962247 ) ) ;
#87312=CARTESIAN_POINT ( 'NONE',  ( -2.307692307692305711, -6.386643153685126251, 34.62446782046654192 ) ) ;
#87315=EDGE_CURVE ( 'NONE', #51469, #57712, #60450, .T. ) ;
#87316=ORIENTED_EDGE ( 'NONE', *, *, #79566, .T. ) ;
#87317=CARTESIAN_POINT ( 'NONE',  ( -10.86536135943320502, -10.82459398097509329, 33.81372124010185587 ) ) ;
#87318=CARTESIAN_POINT ( 'NONE',  ( 5.207714884747860928, -4.809403383903225304, 33.96459661697924304 ) ) ;
#87319=VERTEX_POINT ( 'NONE', #7149 ) ;
#87320=CARTESIAN_POINT ( 'NONE',  ( 18.24994540937804643, -12.07971442181321997, 32.31769673815850297 ) ) ;
#87321=CARTESIAN_POINT ( 'NONE',  ( -0.2385256174450673672, -4.762714258010882773, 34.23016756924214832 ) ) ;
#87323=VECTOR ( 'NONE', #41730, 1000.000000000000227 ) ;
#87324=CARTESIAN_POINT ( 'NONE',  ( 16.37662569511456567, -8.496831190052089866, 34.64984203495476578 ) ) ;
#87326=CARTESIAN_POINT ( 'NONE',  ( -5.777220331021931443, -3.563462043263029955, 33.22394488606062879 ) ) ;
#87327=FACE_BOUND ( 'NONE', #81877, .T. ) ;
#87329=CARTESIAN_POINT ( 'NONE',  ( -12.46153846153846168, -8.973038597847269315, 34.52809138561121927 ) ) ;
#87330=FACE_OUTER_BOUND ( 'NONE', #71653, .T. ) ;
#87331=CARTESIAN_POINT ( 'NONE',  ( 0.3962684609821414128, -6.835583212224500826, 34.95778746994557906 ) ) ;
#87332=CARTESIAN_POINT ( 'NONE',  ( 6.923076923076800782, -11.06231777344772027, 33.60647404775119895 ) ) ;
#87335=ORIENTED_EDGE ( 'NONE', *, *, #86324, .F. ) ;
#87336=CARTESIAN_POINT ( 'NONE',  ( 2.373760658694747061, -6.386643153685127139, 34.62446782046654192 ) ) ;
#87337=DIRECTION ( 'NONE',  ( -0.000000000000000000, 0.5000000000000011102, -0.8660254037844381525 ) ) ;
#87338=ORIENTED_EDGE ( 'NONE', *, *, #13521, .F. ) ;
#87339=ADVANCED_FACE ( 'NONE', ( #21543 ), #34621, .F. ) ;
#87343=CARTESIAN_POINT ( 'NONE',  ( -3.230769230769229949, -8.120952969808772792, 34.71129190930000163 ) ) ;
#87344=EDGE_LOOP ( 'NONE', ( #59699, #4232 ) ) ;
#87346=DIRECTION ( 'NONE',  ( -0.000000000000000000, -0.7660444431189791237, -0.6427876096865379196 ) ) ;
#87347=FACE_OUTER_BOUND ( 'NONE', #4422, .T. ) ;
#87348=LINE ( 'NONE', #45440, #54728 ) ;
#87349=CARTESIAN_POINT ( 'NONE',  ( -5.076923076923075762, -7.500000000000001776, 35.04278698407183867 ) ) ;
#87350=CARTESIAN_POINT ( 'NONE',  ( -12.71156169883143150, -5.056417327199099532, 34.11270091957321426 ) ) ;
#87351=CARTESIAN_POINT ( 'NONE',  ( -8.769230769230768274, -9.780366693483667717, 34.19971097300155094 ) ) ;
#87352=DIRECTION ( 'NONE',  ( -0.000000000000000000, -0.6427876096865404731, -0.7660444431189770143 ) ) ;
#87353=AXIS2_PLACEMENT_3D ( 'NONE', #57363, #1982, #29029 ) ;
#87355=ORIENTED_EDGE ( 'NONE', *, *, #37629, .F. ) ;
#87356=ORIENTED_EDGE ( 'NONE', *, *, #87387, .F. ) ;
#87357=CARTESIAN_POINT ( 'NONE',  ( -9.942284436356281674, -2.544273027872575366, 31.48422191005632342 ) ) ;
#87358=VECTOR ( 'NONE', #76070, 1000.000000000000000 ) ;
#87359=CARTESIAN_POINT ( 'NONE',  ( -4.376772371362300795, -12.39988816332205701, 30.74660775122750778 ) ) ;
#87360=CARTESIAN_POINT ( 'NONE',  ( -5.999999999999998224, -10.67929555188718282, 33.92786785259544047 ) ) ;
#87361=CARTESIAN_POINT ( 'NONE',  ( 10.61538461538461675, -2.833524468853757305, 32.15551576947925838 ) ) ;
#87362=DIRECTION ( 'NONE',  ( 0.000000000000000000, 0.8660254037844377084, 0.5000000000000015543 ) ) ;
#87364=CARTESIAN_POINT ( 'NONE',  ( -7.715628144390283438, -8.586989748646452369, 34.63063291749215011 ) ) ;
#87366=LINE ( 'NONE', #73844, #5643 ) ;
#87367=CARTESIAN_POINT ( 'NONE',  ( -18.00000000000030553, -12.49374608885938542, 30.00000000000319744 ) ) ;
#87368=LINE ( 'NONE', #40509, #64123 ) ;
#87369=CARTESIAN_POINT ( 'NONE',  ( 13.13459214732242408, -4.335965774309649134, 33.62209801155881905 ) ) ;
#87370=CARTESIAN_POINT ( 'NONE',  ( -12.52762084089859584, -8.164416787775445883, 34.95778746994557906 ) ) ;
#87371=CARTESIAN_POINT ( 'NONE',  ( 8.096099255531889582, -8.476813868363244353, 34.90874843262270133 ) ) ;
#87372=CARTESIAN_POINT ( 'NONE',  ( 2.437739742942760746, -7.723484941389743952, 34.99544897038808955 ) ) ;
#87373=CARTESIAN_POINT ( 'NONE',  ( -15.29685264172511161, -9.780366693483667717, 34.19971097300155805 ) ) ;
#87374=ORIENTED_EDGE ( 'NONE', *, *, #81052, .T. ) ;
#87375=CARTESIAN_POINT ( 'NONE',  ( 8.769230769230645706, -5.094484230521993062, 34.41647553114689373 ) ) ;
#87376=CARTESIAN_POINT ( 'NONE',  ( -17.32694630114453105, -6.652501968072647820, 34.93155406624980941 ) ) ;
#87379=EDGE_CURVE ( 'NONE', #11510, #65002, #76561, .T. ) ;
#87380=CARTESIAN_POINT ( 'NONE',  ( -14.08491276642389423, -5.114059244376869984, 34.14424750095245287 ) ) ;
#87381=VECTOR ( 'NONE', #59828, 999.9999999999998863 ) ;
#87382=FACE_OUTER_BOUND ( 'NONE', #64341, .T. ) ;
#87383=DIRECTION ( 'NONE',  ( 0.000000000000000000, 0.7660444431189822323, -0.6427876096865344779 ) ) ;
#87384=ORIENTED_EDGE ( 'NONE', *, *, #55203, .T. ) ;
#87386=CYLINDRICAL_SURFACE ( 'NONE', #38309, 0.2499999999999986955 ) ;
#87387=EDGE_CURVE ( 'NONE', #20268, #14556, #55327, .T. ) ;
#87388=B_SPLINE_CURVE_WITH_KNOTS ( 'NONE', 3,
 ( #73990, #39322, #86176, #37976, #31663, #52365, #45614, #11389, #66334, #53253 ),
 .UNSPECIFIED., .F., .F.,
 ( 4, 2, 2, 2, 4 ),
 ( 0.000000000000000000, 0.0001954311564186864949, 0.0003908623128373729899, 0.0005862934692560594577, 0.0007817246256747459798 ),
 .UNSPECIFIED. ) ;
#87389=EDGE_LOOP ( 'NONE', ( #9452, #11530 ) ) ;
#87390=CARTESIAN_POINT ( 'NONE',  ( -7.173053667125512511, -11.47974371597207899, 33.17467449705390692 ) ) ;
#87391=ADVANCED_FACE ( 'NONE', ( #26983 ), #13019, .F. ) ;
#87392=VERTEX_POINT ( 'NONE', #398 ) ;
#87393=CARTESIAN_POINT ( 'NONE',  ( -7.715363405186896451, -6.369690395747424461, 34.87708834333098196 ) ) ;
#87394=CARTESIAN_POINT ( 'NONE',  ( -3.230769230769229949, -2.517432740324522911, 35.29906147534542527 ) ) ;
#87395=AXIS2_PLACEMENT_3D ( 'NONE', #6504, #61429, #82166 ) ;
#87396=DIRECTION ( 'NONE',  ( -1.000000000000000000, 0.000000000000000000, 0.000000000000000000 ) ) ;
#87398=DIRECTION ( 'NONE',  ( 0.000000000000000000, 0.1736481776669275834, 0.9848077530122086864 ) ) ;
#87399=VERTEX_POINT ( 'NONE', #61191 ) ;
#87400=EDGE_CURVE ( 'NONE', #12785, #7242, #28671, .T. ) ;
#87401=VERTEX_POINT ( 'NONE', #833 ) ;
#87402=CARTESIAN_POINT ( 'NONE',  ( 2.177544337960613863, -9.504002272028875709, 34.60269587691767867 ) ) ;
#87403=CARTESIAN_POINT ( 'NONE',  ( -0.2114841499001467451, -10.66356715214248396, 33.62249196103329751 ) ) ;
#87404=CARTESIAN_POINT ( 'NONE',  ( 10.61538461538461675, -1.215029322943914858, 32.30358669280327177 ) ) ;
#87405=CYLINDRICAL_SURFACE ( 'NONE', #1620, 0.2499999999999973355 ) ;
#87406=CARTESIAN_POINT ( 'NONE',  ( 7.145856592054988354, -8.540255544307065350, 34.89611431652622286 ) ) ;
#87407=CARTESIAN_POINT ( 'NONE',  ( -1.384615384615383471, -10.67929555188718282, 33.92786785259544047 ) ) ;
#87408=LINE ( 'NONE', #45509, #62140 ) ;
#87409=AXIS2_PLACEMENT_3D ( 'NONE', #28492, #1900, #55953 ) ;
#87410=ORIENTED_EDGE ( 'NONE', *, *, #70817, .F. ) ;
#87412=VERTEX_POINT ( 'NONE', #81491 ) ;
#87413=CARTESIAN_POINT ( 'NONE',  ( 3.230769230769110045, -3.835265460704628371, 33.15142922262033665 ) ) ;
#87414=EDGE_LOOP ( 'NONE', ( #88878, #28573 ) ) ;
#87415=VECTOR ( 'NONE', #38337, 1000.000000000000000 ) ;
#87416=EDGE_CURVE ( 'NONE', #12502, #53380, #12131, .T. ) ;
#87417=VECTOR ( 'NONE', #27867, 1000.000000000000114 ) ;
#87418=CARTESIAN_POINT ( 'NONE',  ( 10.54930120442873687, -4.786620604624113540, 33.94971097300155805 ) ) ;
#87419=DIRECTION ( 'NONE',  ( 0.000000000000000000, 0.4999999999999985567, 0.8660254037844395958 ) ) ;
#87420=ORIENTED_EDGE ( 'NONE', *, *, #42540, .F. ) ;
#87421=CARTESIAN_POINT ( 'NONE',  ( 14.37294744720514572, -12.16647553114626490, 32.15551576947920864 ) ) ;
#87422=EDGE_CURVE ( 'NONE', #66691, #50483, #28297, .T. ) ;
#87425=ORIENTED_EDGE ( 'NONE', *, *, #44490, .F. ) ;
#87426=DIRECTION ( 'NONE',  ( -0.000000000000000000, -0.5000000000000009992, -0.8660254037844380415 ) ) ;
#87428=EDGE_CURVE ( 'NONE', #67532, #64445, #64741, .T. ) ;
#87429=CARTESIAN_POINT ( 'NONE',  ( 4.087763774486018242, -12.62096338111211580, 30.90682066428152197 ) ) ;
#87430=CARTESIAN_POINT ( 'NONE',  ( 12.46153846153833911, -2.625532179533778709, 30.86335684631627174 ) ) ;
#87431=FACE_BOUND ( 'NONE', #17699, .T. ) ;
#87432=CARTESIAN_POINT ( 'NONE',  ( 2.437739913947992942, -7.723484964179500700, 34.74522123443823318 ) ) ;
#87433=CARTESIAN_POINT ( 'NONE',  ( 8.769230769230768274, -10.67929555188718282, 33.92786785259544047 ) ) ;
#87434=CARTESIAN_POINT ( 'NONE',  ( 5.750000000000002665, -2.499999999999998668, 29.75000000000000355 ) ) ;
#87435=CARTESIAN_POINT ( 'NONE',  ( 1.134592160393928628, -12.45566812827425096, 31.48439005359158926 ) ) ;
#87436=VECTOR ( 'NONE', #59171, 1000.000000000000000 ) ;
#87437=CARTESIAN_POINT ( 'NONE',  ( 20.99999999999998224, -2.249999999999999556, 27.25000000000000000 ) ) ;
#87438=CARTESIAN_POINT ( 'NONE',  ( 7.846153846153846700, -10.51840700105979565, 33.73612834413961536 ) ) ;
#87439=ORIENTED_EDGE ( 'NONE', *, *, #78781, .T. ) ;
#87440=CARTESIAN_POINT ( 'NONE',  ( -11.60454391782167249, -3.322132147404559532, 32.92929555188719348 ) ) ;
#87441=VERTEX_POINT ( 'NONE', #64286 ) ;
#87442=EDGE_CURVE ( 'NONE', #30965, #77971, #35957, .T. ) ;
#87443=VERTEX_POINT ( 'NONE', #77811 ) ;
#87444=AXIS2_PLACEMENT_3D ( 'NONE', #60752, #46353, #89138 ) ;
#87445=CARTESIAN_POINT ( 'NONE',  ( 5.749976775778542049, -12.07920672191015221, 32.31858351112116168 ) ) ;
#87447=CARTESIAN_POINT ( 'NONE',  ( 15.29602437028207085, -8.656820664281605460, 34.87096338111211224 ) ) ;
#87448=LINE ( 'NONE', #53186, #85435 ) ;
#87449=ADVANCED_FACE ( 'NONE', ( #36396 ), #84595, .F. ) ;
#87450=CARTESIAN_POINT ( 'NONE',  ( 8.899278204481223753, -7.723484941389743952, 34.99544897038808955 ) ) ;
#87451=CARTESIAN_POINT ( 'NONE',  ( 1.450682717965461332, -3.937682226553329556, 33.60647404775216529 ) ) ;
#87452=EDGE_CURVE ( 'NONE', #50071, #28639, #25029, .T. ) ;
#87453=EDGE_LOOP ( 'NONE', ( #57369, #49589, #46739, #39755 ) ) ;
#87454=CARTESIAN_POINT ( 'NONE',  ( -5.143005456283209931, -5.471508081941601986, 34.59228464037088457 ) ) ;
#87456=CARTESIAN_POINT ( 'NONE',  ( 11.47313752565723277, -7.749976730030849303, 34.74374725381503737 ) ) ;
#87457=CARTESIAN_POINT ( 'NONE',  ( -14.08431682191988621, -2.251407671071270489, 29.88021292934942963 ) ) ;
#87458=CARTESIAN_POINT ( 'NONE',  ( -16.02332071561251325, -4.299079248970731015, 33.91157788607253565 ) ) ;
#87459=EDGE_LOOP ( 'NONE', ( #9313, #52248, #49435, #2219 ) ) ;
#87460=EDGE_CURVE ( 'NONE', #47330, #12423, #73378, .T. ) ;
#87462=PRODUCT_CONTEXT ( 'NONE', #19322, 'mechanical' ) ;
#87463=EDGE_LOOP ( 'NONE', ( #84374, #47526, #9757, #44625 ) ) ;
#87464=CARTESIAN_POINT ( 'NONE',  ( 0.7115927731767753839, -10.66356715214248396, 33.62249196103329751 ) ) ;
#87465=CARTESIAN_POINT ( 'NONE',  ( 5.076923076922953193, -3.083524468854526912, 32.58852847137268327 ) ) ;
#87466=ORIENTED_EDGE ( 'NONE', *, *, #44206, .T. ) ;
#87467=LINE ( 'NONE', #68069, #45278 ) ;
#87468=CARTESIAN_POINT ( 'NONE',  ( 15.00728428704528561, -9.331801661448606566, 34.40259984581193464 ) ) ;
#87469=DIRECTION ( 'NONE',  ( -0.000000000000000000, 0.7660444431189791237, -0.6427876096865379196 ) ) ;
#87470=CARTESIAN_POINT ( 'NONE',  ( -2.531177251416255380, -8.496056993536548418, 34.65000542017679663 ) ) ;
#87472=ORIENTED_EDGE ( 'NONE', *, *, #58271, .T. ) ;
#87474=VERTEX_POINT ( 'NONE', #63411 ) ;
#87476=CARTESIAN_POINT ( 'NONE',  ( -16.15384615384627409, -10.90142922262034020, 33.41473453929536674 ) ) ;
#87477=CARTESIAN_POINT ( 'NONE',  ( -6.923076923076922462, -4.098570777380720287, 33.41473453929634729 ) ) ;
#87478=VECTOR ( 'NONE', #41037, 1000.000000000000227 ) ;
#87479=CARTESIAN_POINT ( 'NONE',  ( -3.930834802233302394, -12.39991518177334129, 30.74647679643404530 ) ) ;
#87480=CARTESIAN_POINT ( 'NONE',  ( -8.519285359852727169, -8.476813868363244353, 34.90874843262270133 ) ) ;
#87481=DIRECTION ( 'NONE',  ( 0.000000000000000000, 0.9848077530122072432, 0.1736481776669354937 ) ) ;
#87482=CARTESIAN_POINT ( 'NONE',  ( 9.692307692307572609, -6.879047030192662504, 34.71129190930017927 ) ) ;
#87484=ORIENTED_EDGE ( 'NONE', *, *, #33766, .T. ) ;
#87485=AXIS2_PLACEMENT_3D ( 'NONE', #64923, #45550, #39257 ) ;
#87487=CYLINDRICAL_SURFACE ( 'NONE', #23217, 0.2500000000000009437 ) ;
#87489=EDGE_LOOP ( 'NONE', ( #88794, #57243, #55537, #17729 ) ) ;
#87490=VECTOR ( 'NONE', #82843, 1000.000000000000227 ) ;
#87491=VERTEX_POINT ( 'NONE', #71056 ) ;
#87492=CARTESIAN_POINT ( 'NONE',  ( -5.933932666649924137, -12.62096338111211757, 30.90682066428152908 ) ) ;
#87493=CARTESIAN_POINT ( 'NONE',  ( -4.153846153846152411, -12.78798330534102945, 29.74999999999997868 ) ) ;
#87494=CARTESIAN_POINT ( 'NONE',  ( 13.16168916709923664, -3.586966769969701208, 32.86292498521069660 ) ) ;
#87495=CARTESIAN_POINT ( 'NONE',  ( 10.83839745947800992, -4.762714258010881885, 34.23016756924214832 ) ) ;
#87497=EDGE_CURVE ( 'NONE', #31340, #52889, #17002, .T. ) ;
#87498=B_SPLINE_CURVE_WITH_KNOTS ( 'NONE', 3,
 ( #1195, #9300, #1651, #77301, #9729, #56590, #43954, #50255, #70991, #28683 ),
 .UNSPECIFIED., .F., .F.,
 ( 4, 2, 2, 2, 4 ),
 ( 0.000000000000000000, 0.0001954311564186871184, 0.0003908623128373742367, 0.0005862934692560614093, 0.0007817246256747484735 ),
 .UNSPECIFIED. ) ;
#87500=ORIENTED_EDGE ( 'NONE', *, *, #2114, .F. ) ;
#87501=B_SPLINE_CURVE_WITH_KNOTS ( 'NONE', 3,
 ( #58045, #24252, #51717, #43648, #71117, #9426, #44969, #72448, #36890, #9863 ),
 .UNSPECIFIED., .F., .F.,
 ( 4, 2, 2, 2, 4 ),
 ( 0.000000000000000000, 0.0001954339857564081520, 0.0003908679715128163040, 0.0005863019572692244018, 0.0007817359430256326080 ),
 .UNSPECIFIED. ) ;
#87502=B_SPLINE_CURVE_WITH_KNOTS ( 'NONE', 3,
 ( #41270, #68734, #7030, #36189, #56878, #29430, #55216, #49683, #77160, #15469 ),
 .UNSPECIFIED., .F., .F.,
 ( 4, 2, 2, 2, 4 ),
 ( 0.0007817246256747463051, 0.0009771112852218896347, 0.001172497944769032747, 0.001367884604316176077, 0.001563271263863319407 ),
 .UNSPECIFIED. ) ;
#87505=CYLINDRICAL_SURFACE ( 'NONE', #39300, 0.2500000000000012212 ) ;
#87506=ORIENTED_EDGE ( 'NONE', *, *, #986, .F. ) ;
#87507=CARTESIAN_POINT ( 'NONE',  ( -7.596208327805703320, -3.712312575010499494, 33.01462480002815170 ) ) ;
#87508=EDGE_LOOP ( 'NONE', ( #45962, #82518, #34075, #83782 ) ) ;
#87509=AXIS2_PLACEMENT_3D ( 'NONE', #83478, #28525, #76252 ) ;
#87510=CARTESIAN_POINT ( 'NONE',  ( 13.51540719244017374, -3.530189275343204702, 32.79018710029569661 ) ) ;
#87512=DIRECTION ( 'NONE',  ( -0.000000000000000000, -0.000000000000000000, -1.000000000000000000 ) ) ;
#87514=EDGE_LOOP ( 'NONE', ( #70164, #8340, #3172, #18735 ) ) ;
#87515=CARTESIAN_POINT ( 'NONE',  ( 12.46153846153833911, -3.835265460704628371, 33.15142922262033665 ) ) ;
#87516=CARTESIAN_POINT ( 'NONE',  ( -6.223484924564330001, -2.353723527008295680, 30.78948104536958752 ) ) ;
#87517=LINE ( 'NONE', #53252, #14954 ) ;
#87519=EDGE_CURVE ( 'NONE', #1538, #85395, #31417, .T. ) ;
#87520=CARTESIAN_POINT ( 'NONE',  ( -7.780086512803769061, -4.661471528628508665, 34.16647553114624003 ) ) ;
#87521=FACE_OUTER_BOUND ( 'NONE', #15572, .T. ) ;
#87522=AXIS2_PLACEMENT_3D ( 'NONE', #28116, #15056, #55586 ) ;
#87523=VERTEX_POINT ( 'NONE', #56660 ) ;
#87524=FACE_BOUND ( 'NONE', #58253, .T. ) ;
#87526=CARTESIAN_POINT ( 'NONE',  ( -2.373774687052441212, -2.486705287966279876, 31.30864560766542937 ) ) ;
#87527=DIRECTION ( 'NONE',  ( -0.000000000000000000, 1.000000000000000000, -0.000000000000000000 ) ) ;
#87528=CARTESIAN_POINT ( 'NONE',  ( -3.296093243573539500, -7.749976730030849303, 34.74374725381503737 ) ) ;
#87529=CARTESIAN_POINT ( 'NONE',  ( 7.716005876422148191, -12.50552854090298638, 31.33409797877408920 ) ) ;
#87530=EDGE_CURVE ( 'NONE', #27912, #1531, #10996, .T. ) ;
#87531=CARTESIAN_POINT ( 'NONE',  ( 8.900022577055551665, -3.530189275343204702, 32.79018710029569661 ) ) ;
#87532=DIRECTION ( 'NONE',  ( -0.000000000000000000, 0.9396926207859092051, -0.3420201433256662704 ) ) ;
#87534=EDGE_CURVE ( 'NONE', #83971, #83905, #61381, .T. ) ;
#87535=ORIENTED_EDGE ( 'NONE', *, *, #78278, .F. ) ;
#87536=ORIENTED_EDGE ( 'NONE', *, *, #41216, .T. ) ;
#87537=ORIENTED_EDGE ( 'NONE', *, *, #72957, .T. ) ;
#87538=B_SPLINE_CURVE_WITH_KNOTS ( 'NONE', 3,
 ( #25320, #73517, #68, #74854, #7721, #47806, #83377, #47357, #48686, #21665 ),
 .UNSPECIFIED., .F., .F.,
 ( 4, 2, 2, 2, 4 ),
 ( 0.0007817246256747434861, 0.0009771112852218859484, 0.001172497944769028411, 0.001367884604316171090, 0.001563271263863313552 ),
 .UNSPECIFIED. ) ;
#87539=VERTEX_POINT ( 'NONE', #53444 ) ;
#87540=ADVANCED_FACE ( 'NONE', ( #3919 ), #32735, .F. ) ;
#87541=CARTESIAN_POINT ( 'NONE',  ( -10.48485891362105349, -11.46989282347013095, 32.79007818306219946 ) ) ;
#87542=CARTESIAN_POINT ( 'NONE',  ( -2.242436736416280940, -3.300289026998474817, 32.46337939537591666 ) ) ;
#87543=AXIS2_PLACEMENT_3D ( 'NONE', #89012, #42145, #27285 ) ;
#87544=CARTESIAN_POINT ( 'NONE',  ( -4.023054346021365468, -8.999086150933472084, 34.52020707165672064 ) ) ;
#87545=CARTESIAN_POINT ( 'NONE',  ( 4.088575707885377497, -3.300289026998414865, 32.46337939537583139 ) ) ;
#87546=CYLINDRICAL_SURFACE ( 'NONE', #58645, 0.2499999999999995559 ) ;
#87548=CARTESIAN_POINT ( 'NONE',  ( 17.86930853333243974, -2.541943142973489334, 30.39792223712631980 ) ) ;
#87549=CYLINDRICAL_SURFACE ( 'NONE', #86528, 0.2499999999999979738 ) ;
#87550=ORIENTED_EDGE ( 'NONE', *, *, #9547, .F. ) ;
#87552=VERTEX_POINT ( 'NONE', #45354 ) ;
#87553=CARTESIAN_POINT ( 'NONE',  ( -3.230769230769229949, -11.11383981884818262, 36.00935417666054406 ) ) ;
#87554=VERTEX_POINT ( 'NONE', #31405 ) ;
#87555=CARTESIAN_POINT ( 'NONE',  ( 7.596130608860880429, -3.202444869320336451, 32.30641848906366675 ) ) ;
#87556=CARTESIAN_POINT ( 'NONE',  ( -5.750054481651857508, -3.712312575010499494, 33.01462480002815170 ) ) ;
#87557=DIRECTION ( 'NONE',  ( -0.000000000000000000, -0.9396926207859092051, -0.3420201433256662704 ) ) ;
#87558=CARTESIAN_POINT ( 'NONE',  ( -8.835313148590904220, -6.343179335718451384, 34.87096338111212646 ) ) ;
#87560=FACE_BOUND ( 'NONE', #71355, .T. ) ;
#87561=EDGE_LOOP ( 'NONE', ( #27151, #62302, #71086, #74781, #75530, #59067 ) ) ;
#87562=ORIENTED_EDGE ( 'NONE', *, *, #44859, .F. ) ;
#87563=CARTESIAN_POINT ( 'NONE',  ( -5.076923076923197442, -6.879047030192662504, 34.71129190930017927 ) ) ;
#87564=ORIENTED_EDGE ( 'NONE', *, *, #36292, .F. ) ;
#87565=FACE_BOUND ( 'NONE', #58803, .T. ) ;
#87566=CARTESIAN_POINT ( 'NONE',  ( -9.469294848214296678, -2.308499170217967134, 30.53291367094873721 ) ) ;
#87567=AXIS2_PLACEMENT_3D ( 'NONE', #36071, #55881, #49574 ) ;
#87568=CARTESIAN_POINT ( 'NONE',  ( 18.22277954126840172, -5.114059244376869096, 34.14424750095245287 ) ) ;
#87570=CARTESIAN_POINT ( 'NONE',  ( -14.98071491913092146, -12.17597550085003633, 31.52189283813461884 ) ) ;
#87571=CARTESIAN_POINT ( 'NONE',  ( -6.673022503163469565, -2.318338780012835443, 30.59689888758630261 ) ) ;
#87573=VERTEX_POINT ( 'NONE', #18788 ) ;
#87574=CYLINDRICAL_SURFACE ( 'NONE', #47134, 0.2499999999999995559 ) ;
#87575=CARTESIAN_POINT ( 'NONE',  ( -14.55766903863466055, -5.728515186090277211, 34.42611988154120439 ) ) ;
#87576=CARTESIAN_POINT ( 'NONE',  ( 2.372947447205147942, -3.083524468853784839, 32.58852847137153930 ) ) ;
#87577=ORIENTED_EDGE ( 'NONE', *, *, #55175, .T. ) ;
#87578=CARTESIAN_POINT ( 'NONE',  ( -1.607541602131531855, -5.667676309546437530, 34.40238873228292249 ) ) ;
#87579=CARTESIAN_POINT ( 'NONE',  ( 7.146088274689772923, -10.61302985866383963, 33.66295027996417843 ) ) ;
#87580=VECTOR ( 'NONE', #85570, 999.9999999999998863 ) ;
#87581=VERTEX_POINT ( 'NONE', #66067 ) ;
#87582=CARTESIAN_POINT ( 'NONE',  ( 6.000000000000001776, -7.500000000000001776, 35.04278698407183867 ) ) ;
#87583=CYLINDRICAL_SURFACE ( 'NONE', #42583, 0.2499999999999979738 ) ;
#87584=CARTESIAN_POINT ( 'NONE',  ( -13.31935981333936425, -5.219633306516380244, 34.19971097300157936 ) ) ;
#87585=DIRECTION ( 'NONE',  ( -0.000000000000000000, -0.7660444431189791237, -0.6427876096865379196 ) ) ;
#87586=DIRECTION ( 'NONE',  ( -0.000000000000000000, 1.000000000000000000, -0.000000000000000000 ) ) ;
#87587=CARTESIAN_POINT ( 'NONE',  ( 7.846153846153846700, -12.48256725967547354, 35.29906147534542527 ) ) ;
#87588=CYLINDRICAL_SURFACE ( 'NONE', #51958, 0.2499999999999973355 ) ;
#87589=CARTESIAN_POINT ( 'NONE',  ( 9.692307692307570832, -5.094484230521993062, 34.41647553114689373 ) ) ;
#87590=DIRECTION ( 'NONE',  ( -0.000000000000000000, 0.5000000000000011102, -0.8660254037844380415 ) ) ;
#87591=DIRECTION ( 'NONE',  ( -0.000000000000000000, -0.1736481776669307198, -0.9848077530122080203 ) ) ;
#87593=ORIENTED_EDGE ( 'NONE', *, *, #47942, .F. ) ;
#87594=CARTESIAN_POINT ( 'NONE',  ( 10.61538461538461675, -1.129524287112498415, 32.06866353760679544 ) ) ;
#87595=ORIENTED_EDGE ( 'NONE', *, *, #4062, .T. ) ;
#87596=B_SPLINE_CURVE_WITH_KNOTS ( 'NONE', 3,
 ( #84760, #23036, #17626, #23909, #72108, #10420, #38329, #65787, #50499, #56817 ),
 .UNSPECIFIED., .F., .F.,
 ( 4, 2, 2, 2, 4 ),
 ( 0.0007817359430256294638, 0.0009771253907249948054, 0.001172514838424360255, 0.001367904286123725489, 0.001563293733823090939 ),
 .UNSPECIFIED. ) ;
#87597=ORIENTED_EDGE ( 'NONE', *, *, #42997, .T. ) ;
#87598=CARTESIAN_POINT ( 'NONE',  ( -17.07692307692307665, -3.937682226553329556, 33.60647404775216529 ) ) ;
#87599=VERTEX_POINT ( 'NONE', #12038 ) ;
#87600=CARTESIAN_POINT ( 'NONE',  ( -15.23076923076922995, -5.557115091759785130, 34.35708131394839171 ) ) ;
#87602=DIRECTION ( 'NONE',  ( 0.000000000000000000, -6.938893903907222067E-15, 1.000000000000000000 ) ) ;
#87603=CARTESIAN_POINT ( 'NONE',  ( -15.36145983387953606, -12.35290016733513951, 31.75349464988449455 ) ) ;
#87604=CARTESIAN_POINT ( 'NONE',  ( -3.007989689500820241, -9.332535724633405749, 34.40230450496446224 ) ) ;
#87605=CARTESIAN_POINT ( 'NONE',  ( -8.519176457592452678, -4.943051570960394159, 34.04725096376909477 ) ) ;
#87606=CARTESIAN_POINT ( 'NONE',  ( 0.4615384615383382183, -5.941354392335915335, 34.76329471203413846 ) ) ;
#87607=CARTESIAN_POINT ( 'NONE',  ( -3.230769230769351186, -4.481592998941358097, 33.73612834414048933 ) ) ;
#87609=CARTESIAN_POINT ( 'NONE',  ( 18.06606733335007675, -11.35647404775217595, 33.31231777344667222 ) ) ;
#87610=CARTESIAN_POINT ( 'NONE',  ( -17.77698715590659972, -2.308499170217966689, 30.53291367094874076 ) ) ;
#87611=DIRECTION ( 'NONE',  ( 0.000000000000000000, 0.9848077530122072432, 0.1736481776669354937 ) ) ;
#87612=B_SPLINE_CURVE_WITH_KNOTS ( 'NONE', 3,
 ( #57657, #63523, #22980, #71601, #85137, #70737, #29315, #17109, #23849, #37371 ),
 .UNSPECIFIED., .F., .F.,
 ( 4, 2, 2, 2, 4 ),
 ( 0.000000000000000000, 0.0001954311564186861155, 0.0003908623128373722310, 0.0005862934692560583735, 0.0007817246256747444619 ),
 .UNSPECIFIED. ) ;
#87613=VERTEX_POINT ( 'NONE', #31860 ) ;
#87614=ORIENTED_EDGE ( 'NONE', *, *, #39338, .F. ) ;
#87615=FACE_OUTER_BOUND ( 'NONE', #59092, .T. ) ;
#87617=CARTESIAN_POINT ( 'NONE',  ( 1.384615384615386802, -10.67929555188718282, 33.92786785259544047 ) ) ;
#87618=CARTESIAN_POINT ( 'NONE',  ( -16.02332045208259359, -12.45806712695776319, 30.39783852428763566 ) ) ;
#87619=CARTESIAN_POINT ( 'NONE',  ( -3.230769230769229949, -13.88283147151868846, 33.14645433367849847 ) ) ;
#87620=DIRECTION ( 'NONE',  ( -0.000000000000000000, -0.9848077530122085754, -0.1736481776669273613 ) ) ;
#87621=B_SPLINE_CURVE_WITH_KNOTS ( 'NONE', 3,
 ( #7490, #69183, #21883, #13791, #76836, #283, #14238, #34946, #15134, #62407 ),
 .UNSPECIFIED., .F., .F.,
 ( 4, 2, 2, 2, 4 ),
 ( 0.000000000000000000, 0.0001954339857564073659, 0.0003908679715128147319, 0.0005863019572692221250, 0.0007817359430256294638 ),
 .UNSPECIFIED. ) ;
#87622=B_SPLINE_CURVE_WITH_KNOTS ( 'NONE', 3,
 ( #37322, #69018, #7327, #34785, #43209, #64788, #3094, #8990, #63910, #30570 ),
 .UNSPECIFIED., .F., .F.,
 ( 4, 2, 2, 2, 4 ),
 ( 0.0007817246256747507503, 0.0009771112852218957062, 0.001172497944769040771, 0.001367884604316185835, 0.001563271263863330682 ),
 .UNSPECIFIED. ) ;
#87623=ORIENTED_EDGE ( 'NONE', *, *, #76096, .F. ) ;
#87624=B_SPLINE_CURVE_WITH_KNOTS ( 'NONE', 3,
 ( #23666, #43940, #78612, #85830, #64642, #38075, #77725, #15593, #22778, #58785 ),
 .UNSPECIFIED., .F., .F.,
 ( 4, 2, 2, 2, 4 ),
 ( 0.000000000000000000, 0.0001954311584214072381, 0.0003908623168428144762, 0.0005862934752642217414, 0.0007817246336856289524 ),
 .UNSPECIFIED. ) ;
#87625=CARTESIAN_POINT ( 'NONE',  ( 1.384615384615386802, -4.786620604624113540, 33.94971097300155094 ) ) ;
#87626=ORIENTED_EDGE ( 'NONE', *, *, #21189, .T. ) ;
#87627=ORIENTED_EDGE ( 'NONE', *, *, #32021, .T. ) ;
#87628=CARTESIAN_POINT ( 'NONE',  ( 17.93472955403921887, -3.300289026998414865, 32.46337939537583139 ) ) ;
#87629=EDGE_CURVE ( 'NONE', #29065, #15565, #24864, .T. ) ;
#87630=CIRCLE ( 'NONE', #48767, 5.000000000000000888 ) ;
#87631=CARTESIAN_POINT ( 'NONE',  ( -2.530619266599155370, -9.172386477786396597, 34.72672124145550043 ) ) ;
#87632=CARTESIAN_POINT ( 'NONE',  ( -17.07692307692307665, -11.69971097300155272, 32.46337939537588113 ) ) ;
#87633=DIRECTION ( 'NONE',  ( -0.000000000000000000, -0.1736481776669307198, -0.9848077530122080203 ) ) ;
#87634=CARTESIAN_POINT ( 'NONE',  ( -2.057637996053992335, -11.79725096376909654, 32.30694842903960762 ) ) ;
#87636=EDGE_LOOP ( 'NONE', ( #67128, #40841, #36662, #35331 ) ) ;
#87637=AXIS2_PLACEMENT_3D ( 'NONE', #44353, #17349, #3829 ) ;
#87639=ORIENTED_EDGE ( 'NONE', *, *, #48883, .F. ) ;
#87640=AXIS2_PLACEMENT_3D ( 'NONE', #61803, #70799, #55499 ) ;
#87641=EDGE_CURVE ( 'NONE', #62031, #71802, #46410, .T. ) ;
#87642=FACE_OUTER_BOUND ( 'NONE', #35620, .T. ) ;
#87643=CARTESIAN_POINT ( 'NONE',  ( 10.54930223602447903, -11.35647404775217595, 33.31231777344666511 ) ) ;
#87644=LINE ( 'NONE', #45291, #86853 ) ;
#87645=CARTESIAN_POINT ( 'NONE',  ( 10.55011461482829738, -5.094484230520674117, 34.41647553114621161 ) ) ;
#87646=CARTESIAN_POINT ( 'NONE',  ( 17.86985279056177944, -5.195881422630167279, 34.18770438780618548 ) ) ;
#87647=CARTESIAN_POINT ( 'NONE',  ( -15.29603923132555110, -2.657715359629089225, 31.77849191805832874 ) ) ;
#87648=VERTEX_POINT ( 'NONE', #66976 ) ;
#87651=B_SPLINE_CURVE_WITH_KNOTS ( 'NONE', 3,
 ( #32022, #87429, #25712, #9965, #78867, #23913, #52724, #86538, #51363, #3207 ),
 .UNSPECIFIED., .F., .F.,
 ( 4, 2, 2, 2, 4 ),
 ( 0.000000000000000000, 0.0001954311564186879315, 0.0003908623128373758630, 0.0005862934692560637946, 0.0007817246256747517261 ),
 .UNSPECIFIED. ) ;
#87652=DIRECTION ( 'NONE',  ( 0.000000000000000000, 0.9396926207859126468, 0.3420201433256571111 ) ) ;
#87653=VERTEX_POINT ( 'NONE', #60204 ) ;
#87654=CARTESIAN_POINT ( 'NONE',  ( 7.976679547917409963, -12.45806712695776319, 30.39783852428763922 ) ) ;
#87655=CARTESIAN_POINT ( 'NONE',  ( -9.915233909823841785, -11.76352882383564769, 32.36236540154569497 ) ) ;
#87657=EDGE_CURVE ( 'NONE', #48065, #37880, #4437, .T. ) ;
#87658=ORIENTED_EDGE ( 'NONE', *, *, #16056, .T. ) ;
#87659=ADVANCED_FACE ( 'NONE', ( #87708 ), #25980, .F. ) ;
#87660=DIRECTION ( 'NONE',  ( 0.000000000000000000, -1.000000000000000000, 0.000000000000000000 ) ) ;
#87662=ORIENTED_EDGE ( 'NONE', *, *, #10281, .T. ) ;
#87663=CARTESIAN_POINT ( 'NONE',  ( 13.44987052412822059, -11.06231777344671130, 33.60647404775212976 ) ) ;
#87664=CARTESIAN_POINT ( 'NONE',  ( 14.55774672760575861, -12.41089969410671223, 31.60739465890703670 ) ) ;
#87665=EDGE_CURVE ( 'NONE', #35354, #56825, #13070, .T. ) ;
#87666=FACE_BOUND ( 'NONE', #79006, .T. ) ;
#87667=CARTESIAN_POINT ( 'NONE',  ( -4.826868765284762830, -12.17597550085003633, 31.52189283813461884 ) ) ;
#87668=EDGE_CURVE ( 'NONE', #22650, #3401, #54777, .T. ) ;
#87669=DIRECTION ( 'NONE',  ( -0.000000000000000000, 0.8660254037844397068, -0.4999999999999978906 ) ) ;
#87670=ORIENTED_EDGE ( 'NONE', *, *, #28535, .F. ) ;
#87671=CYLINDRICAL_SURFACE ( 'NONE', #10148, 0.2500000000000008882 ) ;
#87672=CARTESIAN_POINT ( 'NONE',  ( 15.10062202133101295, -4.460286881179643004, 33.72017969459903242 ) ) ;
#87673=CARTESIAN_POINT ( 'NONE',  ( -14.08491276642389600, -2.847695495035523550, 31.58253572463339154 ) ) ;
#87674=ORIENTED_EDGE ( 'NONE', *, *, #60040, .F. ) ;
#87676=CARTESIAN_POINT ( 'NONE',  ( -5.999999999999998224, -10.51840700105979565, 33.73612834413961536 ) ) ;
#87677=CARTESIAN_POINT ( 'NONE',  ( -4.087778820496075660, -2.292212530054420494, 30.41441678777542990 ) ) ;
#87678=CARTESIAN_POINT ( 'NONE',  ( 11.47319109250076430, -6.026961402152685388, 34.52809138561120506 ) ) ;
#87679=CARTESIAN_POINT ( 'NONE',  ( 12.46153846153846168, -3.669653830205710676, 35.88435417666054406 ) ) ;
#87680=FACE_BOUND ( 'NONE', #2282, .T. ) ;
#87681=CARTESIAN_POINT ( 'NONE',  ( -7.173053667125515176, -12.41104346484419452, 31.60698883733904196 ) ) ;
#87682=DIRECTION ( 'NONE',  ( -0.000000000000000000, -0.6427876096865404731, -0.7660444431189770143 ) ) ;
#87683=CARTESIAN_POINT ( 'NONE',  ( 9.942307692307696954, -2.499999999999999556, 29.81604066197449754 ) ) ;
#87684=FACE_OUTER_BOUND ( 'NONE', #86212, .T. ) ;
#87685=CARTESIAN_POINT ( 'NONE',  ( -2.084679463598912097, -12.38742843783360748, 31.66772728687926985 ) ) ;
#87689=CARTESIAN_POINT ( 'NONE',  ( -8.546451227962355901, -5.913360116392397892, 34.49180327182771322 ) ) ;
#87690=ORIENTED_EDGE ( 'NONE', *, *, #47639, .F. ) ;
#87693=ORIENTED_EDGE ( 'NONE', *, *, #5799, .F. ) ;
#87694=B_SPLINE_CURVE_WITH_KNOTS ( 'NONE', 3,
 ( #21074, #14328, #8907, #76478, #7578, #14780, #35040, #62499, #35939, #15664 ),
 .UNSPECIFIED., .F., .F.,
 ( 4, 2, 2, 2, 4 ),
 ( 0.000000000000000000, 0.0001954339857564073659, 0.0003908679715128147319, 0.0005863019572692221250, 0.0007817359430256294638 ),
 .UNSPECIFIED. ) ;
#87695=CARTESIAN_POINT ( 'NONE',  ( -15.48076923076923350, -7.566083408709835645, 34.74999999999999289 ) ) ;
#87696=CARTESIAN_POINT ( 'NONE',  ( 13.38461538461538680, -9.584722331328613620, 36.20867863119891439 ) ) ;
#87697=CARTESIAN_POINT ( 'NONE',  ( -5.010855743573001675, -9.058645607665452459, 34.76329471203371924 ) ) ;
#87699=CARTESIAN_POINT ( 'NONE',  ( -16.37677237136229991, -2.554751324335733376, 30.48935550225260727 ) ) ;
#87700=CARTESIAN_POINT ( 'NONE',  ( -11.66915214157184622, -3.957541250942358424, 33.62499894934981626 ) ) ;
#87702=B_SPLINE_CURVE_WITH_KNOTS ( 'NONE', 3,
 ( #15456, #35272, #42930, #69062, #8701, #70399, #36177, #28524, #63629, #1933 ),
 .UNSPECIFIED., .F., .F.,
 ( 4, 2, 2, 2, 4 ),
 ( 0.000000000000000000, 0.0001954339857564081520, 0.0003908679715128163040, 0.0005863019572692244018, 0.0007817359430256326080 ),
 .UNSPECIFIED. ) ;
#87704=LINE ( 'NONE', #31857, #86337 ) ;
#87705=DIRECTION ( 'NONE',  ( -0.000000000000000000, -0.6427876096865404731, -0.7660444431189771253 ) ) ;
#87708=FACE_OUTER_BOUND ( 'NONE', #74395, .T. ) ;
#87709=CARTESIAN_POINT ( 'NONE',  ( 8.769230769230768274, -9.780366693483667717, 34.19971097300155094 ) ) ;
#87710=CARTESIAN_POINT ( 'NONE',  ( -11.40793583669797862, -10.19071101563364756, 33.96452234770658407 ) ) ;
#87711=VECTOR ( 'NONE', #11604, 1000.000000000000000 ) ;
#87713=B_SPLINE_CURVE_WITH_KNOTS ( 'NONE', 3,
 ( #23221, #14698, #35406, #49802, #28661, #9279, #8387, #50682, #56127, #43498 ),
 .UNSPECIFIED., .F., .F.,
 ( 4, 2, 2, 2, 4 ),
 ( 0.0007817359430256216575, 0.0009771253907249856981, 0.001172514838424349847, 0.001367904286123713779, 0.001563293733823077928 ),
 .UNSPECIFIED. ) ;
#87716=CARTESIAN_POINT ( 'NONE',  ( -1.134560964701930352, -12.01375889529407281, 32.43194544308182969 ) ) ;
#87717=ORIENTED_EDGE ( 'NONE', *, *, #54037, .F. ) ;
#87718=CARTESIAN_POINT ( 'NONE',  ( 17.32686859527122181, -2.824170634883622633, 31.52227843825338738 ) ) ;
#87719=CARTESIAN_POINT ( 'NONE',  ( 8.900022577055558770, -11.18335022499818621, 33.13157742990016885 ) ) ;
#87721=CARTESIAN_POINT ( 'NONE',  ( 2.307692307692309264, -4.098570777380720287, 33.41473453929634729 ) ) ;
#87722=CARTESIAN_POINT ( 'NONE',  ( 5.299702745901139878, -6.717445702608402236, 34.94155399931962336 ) ) ;
#87723=EDGE_LOOP ( 'NONE', ( #14930, #26366, #66587, #12480 ) ) ;
#87726=CARTESIAN_POINT ( 'NONE',  ( 11.31553457955469000, -2.889293201056495786, 32.26117774369186009 ) ) ;
#87727=VERTEX_POINT ( 'NONE', #62411 ) ;
#87728=CARTESIAN_POINT ( 'NONE',  ( -9.822455662039388358, -3.625366637846544116, 33.29286588640298561 ) ) ;
#87729=CARTESIAN_POINT ( 'NONE',  ( 4.088575707885377497, -8.613356846314824011, 34.62446782046655613 ) ) ;
#87730=CARTESIAN_POINT ( 'NONE',  ( 5.207761407409835286, -7.277220318596959281, 34.99547417642776992 ) ) ;
#87732=FACE_OUTER_BOUND ( 'NONE', #60584, .T. ) ;
#87733=ORIENTED_EDGE ( 'NONE', *, *, #22907, .T. ) ;
#87734=CARTESIAN_POINT ( 'NONE',  ( 7.173076923076937561, -2.249999999999999112, 29.81603969181031033 ) ) ;
#87735=CARTESIAN_POINT ( 'NONE',  ( 6.923076923076924238, -4.786620604624113540, 33.94971097300155094 ) ) ;
#87736=CARTESIAN_POINT ( 'NONE',  ( 1.134592160393929072, -2.985938066672154445, 32.43141759479405550 ) ) ;
#87737=ORIENTED_EDGE ( 'NONE', *, *, #24031, .T. ) ;
#87738=B_SPLINE_CURVE_WITH_KNOTS ( 'NONE', 3,
 ( #22229, #49696, #15481, #84832, #56890, #16355 ),
 .UNSPECIFIED., .F., .F.,
 ( 4, 2, 4 ),
 ( 0.0003909512603273853043, 0.0005862562993132091520, 0.0007815613382990329455 ),
 .UNSPECIFIED. ) ;
#87741=B_SPLINE_CURVE_WITH_KNOTS ( 'NONE', 3,
 ( #85764, #61823, #13642, #82567, #5563, #53743, #61372, #26275, #81229, #88445 ),
 .UNSPECIFIED., .F., .F.,
 ( 4, 2, 2, 2, 4 ),
 ( 0.000000000000000000, 0.0001954339857564074473, 0.0003908679715128148945, 0.0005863019572692223418, 0.0007817359430256297891 ),
 .UNSPECIFIED. ) ;
#87742=ORIENTED_EDGE ( 'NONE', *, *, #82010, .T. ) ;
#87743=EDGE_CURVE ( 'NONE', #45635, #73490, #34514, .T. ) ;
#87744=CARTESIAN_POINT ( 'NONE',  ( 5.076923076922954969, -12.27809138561165270, 31.22303859784587132 ) ) ;
#87745=CYLINDRICAL_SURFACE ( 'NONE', #27119, 0.2499999999999995559 ) ;
#87748=CARTESIAN_POINT ( 'NONE',  ( -17.74999999999856115, -7.500000000000155431, 34.75000000000007105 ) ) ;
#87749=ORIENTED_EDGE ( 'NONE', *, *, #59902, .F. ) ;
#87750=ORIENTED_EDGE ( 'NONE', *, *, #19822, .F. ) ;
#87751=EDGE_CURVE ( 'NONE', #84227, #53257, #72084, .T. ) ;
#87753=CARTESIAN_POINT ( 'NONE',  ( -8.069080063669991532, -4.887634598454294377, 34.01352882383564946 ) ) ;
#87754=ORIENTED_EDGE ( 'NONE', *, *, #15305, .F. ) ;
#87755=CARTESIAN_POINT ( 'NONE',  ( -6.857009589726848375, -3.937682226553329556, 33.60647404775216529 ) ) ;
#87756=B_SPLINE_CURVE_WITH_KNOTS ( 'NONE', 3,
 ( #62616, #927, #41924, #22525, #49559, #21194, #28395, #14898, #48662, #56752 ),
 .UNSPECIFIED., .F., .F.,
 ( 4, 2, 2, 2, 4 ),
 ( 0.000000000000000000, 0.0001954339857564079894, 0.0003908679715128159787, 0.0005863019572692239681, 0.0007817359430256319575 ),
 .UNSPECIFIED. ) ;
#87757=CARTESIAN_POINT ( 'NONE',  ( 9.692307692307695177, -11.11383981884818262, 36.00935417666054406 ) ) ;
#87759=AXIS2_PLACEMENT_3D ( 'NONE', #70238, #22930, #84214 ) ;
#87761=CARTESIAN_POINT ( 'NONE',  ( -12.23852710992561299, -12.15243808032446005, 31.58219941686247978 ) ) ;
#87762=CARTESIAN_POINT ( 'NONE',  ( 16.15384615384603251, -11.67786785259630911, 32.92929555188603530 ) ) ;
#87763=EDGE_CURVE ( 'NONE', #47735, #66615, #41279, .T. ) ;
#87764=ORIENTED_EDGE ( 'NONE', *, *, #37123, .T. ) ;
#87767=AXIS2_PLACEMENT_3D ( 'NONE', #67598, #12653, #80226 ) ;
#87768=ORIENTED_EDGE ( 'NONE', *, *, #64896, .T. ) ;
#87769=FACE_OUTER_BOUND ( 'NONE', #83749, .T. ) ;
#87771=VERTEX_POINT ( 'NONE', #33631 ) ;
#87772=VECTOR ( 'NONE', #32649, 1000.000000000000114 ) ;
#87773=CARTESIAN_POINT ( 'NONE',  ( 13.38461538461538680, -1.422936976036506707, 30.56769352161908415 ) ) ;
#87774=CARTESIAN_POINT ( 'NONE',  ( 2.057692307692309708, -7.500000000000001776, 35.00000000000000000 ) ) ;
#87775=EDGE_CURVE ( 'NONE', #87267, #22892, #81826, .T. ) ;
#87777=CARTESIAN_POINT ( 'NONE',  ( 9.942307692307712941, -2.249999999999999112, 29.81603969181029967 ) ) ;
#87778=DIRECTION ( 'NONE',  ( -0.000000000000000000, 1.000000000000000000, 3.491481338843133355E-15 ) ) ;
#87779=FACE_BOUND ( 'NONE', #68871, .T. ) ;
#87780=CARTESIAN_POINT ( 'NONE',  ( 15.16468581981335007, -5.557115091759785130, 34.35708131394839171 ) ) ;
#87781=CARTESIAN_POINT ( 'NONE',  ( -18.13069060311030967, -12.35290016733513951, 31.75349464988449455 ) ) ;
#87782=DIRECTION ( 'NONE',  ( 0.000000000000000000, 0.9396926207859126468, -0.3420201433256571111 ) ) ;
#87783=CARTESIAN_POINT ( 'NONE',  ( 0.3308478584281536183, -6.369640206132551441, 34.87707690430379159 ) ) ;
#87784=CARTESIAN_POINT ( 'NONE',  ( -5.326946314216043810, -3.202444869320336451, 32.30641848906366675 ) ) ;
#87785=EDGE_CURVE ( 'NONE', #34190, #70760, #726, .T. ) ;
#87786=CARTESIAN_POINT ( 'NONE',  ( -3.903846153846090239, -7.434744860731434812, 35.00000000000000711 ) ) ;
#87787=CARTESIAN_POINT ( 'NONE',  ( -20.99999999999999645, -10.75000000000000000, 29.75000000000000355 ) ) ;
#87788=ORIENTED_EDGE ( 'NONE', *, *, #10430, .T. ) ;
#87790=CARTESIAN_POINT ( 'NONE',  ( -16.40384615384615330, -7.433931650972299465, 34.75000000000000711 ) ) ;
#87791=CARTESIAN_POINT ( 'NONE',  ( -13.25382494364843389, -3.957578996910242619, 33.62503395064540257 ) ) ;
#87792=ORIENTED_EDGE ( 'NONE', *, *, #83227, .T. ) ;
#87794=CARTESIAN_POINT ( 'NONE',  ( -17.20761454359063691, -11.18331474514187995, 33.13161551792790505 ) ) ;
#87795=CARTESIAN_POINT ( 'NONE',  ( -15.36146069743679732, -2.541943142973491554, 30.39792223712631980 ) ) ;
#87796=CARTESIAN_POINT ( 'NONE',  ( 17.07692307692307665, -8.318370150425687726, 35.83090037661290239 ) ) ;
#87797=ORIENTED_EDGE ( 'NONE', *, *, #9445, .T. ) ;
#87798=CARTESIAN_POINT ( 'NONE',  ( 8.703960768674447124, -12.70778746994557551, 30.41441678777548319 ) ) ;
#87799=CARTESIAN_POINT ( 'NONE',  ( 6.673053698855465399, -8.475808217655753651, 34.90892951860618609 ) ) ;
#87801=CYLINDRICAL_SURFACE ( 'NONE', #24330, 0.2500000000000008882 ) ;
#87802=CARTESIAN_POINT ( 'NONE',  ( -13.38461538461538325, -2.292212530054420494, 30.41441678777542634 ) ) ;
#87803=B_SPLINE_CURVE_WITH_KNOTS ( 'NONE', 3,
 ( #80586, #12560, #88245, #40486, #34152, #68825, #26519, #61619, #26963, #7130 ),
 .UNSPECIFIED., .F., .F.,
 ( 4, 2, 2, 2, 4 ),
 ( 0.000000000000000000, 0.0001954339857564081249, 0.0003908679715128162498, 0.0005863019572692244018, 0.0007817359430256324996 ),
 .UNSPECIFIED. ) ;
#87804=CARTESIAN_POINT ( 'NONE',  ( 3.230769230769231726, -2.486705287966279876, 31.30864560766543647 ) ) ;
#87806=CARTESIAN_POINT ( 'NONE',  ( -10.48459417441766561, -11.37503395064541678, 33.29242100308974273 ) ) ;
#87807=VECTOR ( 'NONE', #39067, 1000.000000000000000 ) ;
#87809=EDGE_LOOP ( 'NONE', ( #60894, #82964 ) ) ;
#87810=ORIENTED_EDGE ( 'NONE', *, *, #46592, .F. ) ;
#87811=DIRECTION ( 'NONE',  ( -0.000000000000000000, 0.8660254037844399289, -0.4999999999999980016 ) ) ;
#87812=EDGE_CURVE ( 'NONE', #79197, #40179, #20118, .T. ) ;
#87813=CYLINDRICAL_SURFACE ( 'NONE', #42695, 0.2500000000000009437 ) ;
#87815=CARTESIAN_POINT ( 'NONE',  ( -12.46153846153858424, -12.16647553114689728, 32.15551576947799362 ) ) ;
#87816=CARTESIAN_POINT ( 'NONE',  ( 5.076923076923075762, -3.322132147404559976, 32.92929555188717927 ) ) ;
#87818=CARTESIAN_POINT ( 'NONE',  ( -1.449885385171702623, -4.320704448112771878, 33.92786785259540494 ) ) ;
#87819=CARTESIAN_POINT ( 'NONE',  ( 1.607394925883794734, -5.114059244376869984, 34.14424750095245287 ) ) ;
#87820=CARTESIAN_POINT ( 'NONE',  ( 16.94623161025551639, -12.11776431015576172, 31.66791131148498906 ) ) ;
#87821=CARTESIAN_POINT ( 'NONE',  ( -18.13004516283476519, -12.49522139742533966, 29.97347330155777811 ) ) ;
#87822=CARTESIAN_POINT ( 'NONE',  ( -9.915233909823838232, -11.24512374952581872, 33.06303171183252942 ) ) ;
#87823=CARTESIAN_POINT ( 'NONE',  ( 13.51514082284902862, -2.647132371071621471, 31.75357179365171589 ) ) ;
#87825=EDGE_CURVE ( 'NONE', #37311, #7100, #74333, .T. ) ;
#87826=CARTESIAN_POINT ( 'NONE',  ( 7.846153846153846700, -8.164416787775445883, 34.95778746994557906 ) ) ;
#87827=DIRECTION ( 'NONE',  ( -0.000000000000000000, 0.9396926207859093161, -0.3420201433256663259 ) ) ;
#87829=CARTESIAN_POINT ( 'NONE',  ( -15.48079246806219267, -10.05641848906368097, 34.04755513067966177 ) ) ;
#87830=ORIENTED_EDGE ( 'NONE', *, *, #14798, .T. ) ;
#87831=CARTESIAN_POINT ( 'NONE',  ( -5.076923076923075762, -11.69971097300155272, 32.46337939537588113 ) ) ;
#87833=CARTESIAN_POINT ( 'NONE',  ( -3.480745961711584791, -3.627789207965226748, 32.91389620160131102 ) ) ;
#87835=AXIS2_PLACEMENT_3D ( 'NONE', #57094, #71939, #17448 ) ;
#87836=VECTOR ( 'NONE', #51271, 1000.000000000000227 ) ;
#87837=EDGE_CURVE ( 'NONE', #84245, #34480, #52781, .T. ) ;
#87838=CARTESIAN_POINT ( 'NONE',  ( 5.207713517890025123, -9.929761469519744921, 34.40412654351204225 ) ) ;
#87839=CARTESIAN_POINT ( 'NONE',  ( 8.769230769230768274, -10.51840700105979565, 33.73612834413961536 ) ) ;
#87840=CARTESIAN_POINT ( 'NONE',  ( -11.28851612908349722, -4.932303261841489928, 34.32971442181322885 ) ) ;
#87841=CARTESIAN_POINT ( 'NONE',  ( -18.00000000000012079, -10.33852847137269926, 34.16647553114546554 ) ) ;
#87842=ORIENTED_EDGE ( 'NONE', *, *, #61769, .T. ) ;
#87844=DIRECTION ( 'NONE',  ( -0.000000000000000000, -0.5000000000000009992, -0.8660254037844380415 ) ) ;
#87846=ORIENTED_EDGE ( 'NONE', *, *, #64006, .F. ) ;
#87847=EDGE_CURVE ( 'NONE', #36328, #35073, #69626, .T. ) ;
#87848=B_SPLINE_CURVE_WITH_KNOTS ( 'NONE', 3,
 ( #66524, #79595, #4825, #52989, #32295, #33179, #38155, #80487, #25086, #3914 ),
 .UNSPECIFIED., .F., .F.,
 ( 4, 2, 2, 2, 4 ),
 ( 0.000000000000000000, 0.0001954311564186868744, 0.0003908623128373737488, 0.0005862934692560606504, 0.0007817246256747474977 ),
 .UNSPECIFIED. ) ;
#87850=COLOUR_RGB ( '', 0.31764706, 0.68627451, 0.89019608) ;
#87851=ORIENTED_EDGE ( 'NONE', *, *, #88186, .F. ) ;
#87853=CARTESIAN_POINT ( 'NONE',  ( -9.626239341305250719, -2.721908614388772296, 31.22303859784725333 ) ) ;
#87854=CARTESIAN_POINT ( 'NONE',  ( -7.976845312821408740, -3.530157926970578952, 32.79014554554150607 ) ) ;
#87855=ORIENTED_EDGE ( 'NONE', *, *, #30994, .F. ) ;
#87856=ORIENTED_EDGE ( 'NONE', *, *, #54312, .F. ) ;
#87857=ORIENTED_EDGE ( 'NONE', *, *, #10250, .T. ) ;
#87858=CARTESIAN_POINT ( 'NONE',  ( -16.15384615384615330, -2.292212530054420494, 30.41441678777542634 ) ) ;
#87859=CARTESIAN_POINT ( 'NONE',  ( 12.23861224402231151, -12.39988816332205701, 30.74660775122750778 ) ) ;
#87860=DIRECTION ( 'NONE',  ( -0.000000000000000000, -0.7660444431189791237, -0.6427876096865379196 ) ) ;
#87861=CARTESIAN_POINT ( 'NONE',  ( -10.74607608205217346, -2.541943142973491554, 30.39792223712631980 ) ) ;
#87862=CARTESIAN_POINT ( 'NONE',  ( -10.74553258511630638, -12.15440758774515473, 32.17923288041532004 ) ) ;
#87863=CARTESIAN_POINT ( 'NONE',  ( 6.989144256427000101, -8.164416787775445883, 34.95778746994558617 ) ) ;
#87864=ADVANCED_FACE ( 'NONE', ( #15137 ), #8379, .F. ) ;
#87865=CARTESIAN_POINT ( 'NONE',  ( 12.71148397988660150, -5.057305518903948638, 34.11320923018887896 ) ) ;
#87866=DIRECTION ( 'NONE',  ( -1.000000000000000000, 0.000000000000000000, 0.000000000000000000 ) ) ;
#87867=ORIENTED_EDGE ( 'NONE', *, *, #85498, .T. ) ;
#87868=VERTEX_POINT ( 'NONE', #2055 ) ;
#87869=EDGE_LOOP ( 'NONE', ( #84861, #29820 ) ) ;
#87870=CARTESIAN_POINT ( 'NONE',  ( -17.07692307692319744, -10.21337939537710326, 33.94971097300076224 ) ) ;
#87871=EDGE_LOOP ( 'NONE', ( #41325, #86527 ) ) ;
#87872=B_SPLINE_CURVE_WITH_KNOTS ( 'NONE', 3,
 ( #37456, #72131, #9987, #78891, #32046, #37009, #64472, #65376, #51848, #38807 ),
 .UNSPECIFIED., .F., .F.,
 ( 4, 2, 2, 2, 4 ),
 ( 0.0007817246256747443535, 0.0009771112852218868158, 0.001172497944769029278, 0.001367884604316171740, 0.001563271263863314203 ),
 .UNSPECIFIED. ) ;
#87873=VECTOR ( 'NONE', #37384, 1000.000000000000000 ) ;
#87874=B_SPLINE_CURVE_WITH_KNOTS ( 'NONE', 3,
 ( #47028, #73644, #52455, #38512, #33081, #25441, #74078, #52897, #11936, #19565 ),
 .UNSPECIFIED., .F., .F.,
 ( 4, 2, 2, 2, 4 ),
 ( 0.000000000000000000, 0.0001954311564186861155, 0.0003908623128373722310, 0.0005862934692560583735, 0.0007817246256747444619 ),
 .UNSPECIFIED. ) ;
#87875=B_SPLINE_CURVE_WITH_KNOTS ( 'NONE', 3,
 ( #6023, #59175, #19963, #40254, #86680, #87120, #66828, #53303, #24946, #53751 ),
 .UNSPECIFIED., .F., .F.,
 ( 4, 2, 2, 2, 4 ),
 ( 0.000000000000000000, 0.0001954311564186860613, 0.0003908623128373721225, 0.0005862934692560581567, 0.0007817246256747442451 ),
 .UNSPECIFIED. ) ;
#87876=CARTESIAN_POINT ( 'NONE',  ( -14.30769230769230660, -2.249999999999998668, 29.75000000000001776 ) ) ;
#87877=CARTESIAN_POINT ( 'NONE',  ( 9.468822748583747284, -5.113361153441934093, 34.14387501736622710 ) ) ;
#87878=B_SPLINE_CURVE_WITH_KNOTS ( 'NONE', 3,
 ( #81975, #26126, #81085, #5418, #75210, #13496, #6734, #34207, #33335, #74319 ),
 .UNSPECIFIED., .F., .F.,
 ( 4, 2, 2, 2, 4 ),
 ( 0.0007817359430256360774, 0.0009771253907250041296, 0.001172514838424371965, 0.001367904286123740017, 0.001563293733823108069 ),
 .UNSPECIFIED. ) ;
#87879=VERTEX_POINT ( 'NONE', #42610 ) ;
#87880=CARTESIAN_POINT ( 'NONE',  ( 15.23076923076910916, -9.528491918059723176, 34.59228464037033035 ) ) ;
#87884=CARTESIAN_POINT ( 'NONE',  ( -12.52686137703063984, -7.749976743299138882, 34.99404534957040624 ) ) ;
#87885=EDGE_CURVE ( 'NONE', #22173, #76098, #16257, .T. ) ;
#87886=CARTESIAN_POINT ( 'NONE',  ( 1.634560902963529072, -6.696923467548660192, 34.68552623307873972 ) ) ;
#87887=CARTESIAN_POINT ( 'NONE',  ( -16.15384615384615330, -10.67929555188718282, 33.92786785259544047 ) ) ;
#87888=FACE_BOUND ( 'NONE', #13997, .T. ) ;
#87889=CARTESIAN_POINT ( 'NONE',  ( 2.372838087024272458, -7.750023238201980469, 34.74374492549440419 ) ) ;
#87890=DIRECTION ( 'NONE',  ( 0.000000000000000000, 0.000000000000000000, 1.000000000000000000 ) ) ;
#87891=EDGE_CURVE ( 'NONE', #47764, #25506, #70071, .T. ) ;
#87892=VECTOR ( 'NONE', #24987, 1000.000000000000000 ) ;
#87894=FACE_OUTER_BOUND ( 'NONE', #8426, .T. ) ;
#87895=CARTESIAN_POINT ( 'NONE',  ( 3.453548899747296730, -4.989023458446561143, 34.36081565061822118 ) ) ;
#87896=CARTESIAN_POINT ( 'NONE',  ( -16.15384615384615330, -2.517432740324522911, 35.29906147534542527 ) ) ;
#87897=CARTESIAN_POINT ( 'NONE',  ( -13.38461538461538325, -1.367168528481310208, 33.57946703557072254 ) ) ;
#87898=ORIENTED_EDGE ( 'NONE', *, *, #54814, .F. ) ;
#87899=ADVANCED_FACE ( 'NONE', ( #56995 ), #28650, .F. ) ;
#87900=CARTESIAN_POINT ( 'NONE',  ( -13.31942140283202747, -2.506253911140448487, 29.99999999999988631 ) ) ;
#87901=ORIENTED_EDGE ( 'NONE', *, *, #72862, .T. ) ;
#87903=AXIS2_PLACEMENT_3D ( 'NONE', #85014, #16987, #10679 ) ;
#87904=CARTESIAN_POINT ( 'NONE',  ( 2.307692307692186251, -3.083524468854526912, 32.58852847137268327 ) ) ;
#87905=CYLINDRICAL_SURFACE ( 'NONE', #60615, 0.2499999999999994726 ) ;
#87906=EDGE_CURVE ( 'NONE', #68833, #21879, #8824, .T. ) ;
#87907=CARTESIAN_POINT ( 'NONE',  ( 15.23076923076923173, -12.62096338111211580, 30.90682066428153263 ) ) ;
#87908=DIRECTION ( 'NONE',  ( 0.000000000000000000, 0.9396926207859126468, -0.3420201433256571111 ) ) ;
#87909=DIRECTION ( 'NONE',  ( -0.000000000000000000, -0.9396926207859093161, -0.3420201433256663259 ) ) ;
#87910=CARTESIAN_POINT ( 'NONE',  ( 17.07692307692295586, -8.613356846316285953, 34.62446782046622218 ) ) ;
#87911=CARTESIAN_POINT ( 'NONE',  ( -2.176900499867522321, -2.729792928343269587, 31.24908615093345077 ) ) ;
#87912=ORIENTED_EDGE ( 'NONE', *, *, #56273, .T. ) ;
#87913=CARTESIAN_POINT ( 'NONE',  ( -11.53846153846153655, -12.10708131394839349, 31.69288490824020244 ) ) ;
#87916=CARTESIAN_POINT ( 'NONE',  ( -15.90379173393269596, -4.074993327901529128, 33.72946981652012255 ) ) ;
#87917=ORIENTED_EDGE ( 'NONE', *, *, #24063, .F. ) ;
#87918=EDGE_CURVE ( 'NONE', #51126, #20157, #64558, .T. ) ;
#87919=B_SPLINE_CURVE_WITH_KNOTS ( 'NONE', 3,
 ( #83056, #1075, #42075, #68645, #8284, #27217 ),
 .UNSPECIFIED., .F., .F.,
 ( 4, 2, 4 ),
 ( 0.0003909569690057831406, 0.0005862646681846083070, 0.0007815723673634335277 ),
 .UNSPECIFIED. ) ;
#87920=ORIENTED_EDGE ( 'NONE', *, *, #78629, .F. ) ;
#87923=CARTESIAN_POINT ( 'NONE',  ( 0.6845013650999459687, -7.369474270740072441, 34.74850911626239736 ) ) ;
#87925=CARTESIAN_POINT ( 'NONE',  ( -17.77698864838715309, -4.887748414852788770, 34.01359900205216746 ) ) ;
#87926=EDGE_LOOP ( 'NONE', ( #69477, #62102 ) ) ;
#87927=B_SPLINE_CURVE_WITH_KNOTS ( 'NONE', 3,
 ( #8376, #43486, #7491, #29103, #57433, #2052, #16457, #1166, #49360, #62846 ),
 .UNSPECIFIED., .F., .F.,
 ( 4, 2, 2, 2, 4 ),
 ( 0.000000000000000000, 0.0001954311564186869015, 0.0003908623128373738030, 0.0005862934692560607588, 0.0007817246256747476061 ),
 .UNSPECIFIED. ) ;
#87928=CARTESIAN_POINT ( 'NONE',  ( -15.90379184220783948, -4.943051570960395047, 34.04725096376909477 ) ) ;
#87929=CARTESIAN_POINT ( 'NONE',  ( -5.299849294439223257, -2.758268499246657957, 31.33685645148948140 ) ) ;
#87930=CARTESIAN_POINT ( 'NONE',  ( 3.453548899747296730, -10.23759521482555357, 34.22997729860117033 ) ) ;
#87931=CARTESIAN_POINT ( 'NONE',  ( 14.17721559957584709, -7.276988635370452485, 34.74523720219453793 ) ) ;
#87932=DIRECTION ( 'NONE',  ( -0.000000000000000000, -0.6427876096865404731, -0.7660444431189771253 ) ) ;
#87933=ORIENTED_EDGE ( 'NONE', *, *, #20753, .F. ) ;
#87934=CARTESIAN_POINT ( 'NONE',  ( -15.36091720050092846, -12.15440758774515473, 32.17923288041532004 ) ) ;
#87935=ORIENTED_EDGE ( 'NONE', *, *, #88552, .T. ) ;
#87936=LINE ( 'NONE', #88810, #71365 ) ;
#87937=CARTESIAN_POINT ( 'NONE',  ( -3.100243792535588572, -2.647132371071621471, 31.75357179365173010 ) ) ;
#87938=CARTESIAN_POINT ( 'NONE',  ( 1.134615384615387246, -7.500000000000001776, 34.75000000000000000 ) ) ;
#87939=CARTESIAN_POINT ( 'NONE',  ( 9.692307692307572609, -10.90142922262034020, 33.41473453929536674 ) ) ;
#87940=CARTESIAN_POINT ( 'NONE',  ( -16.15384615384615330, -13.53365097954675988, 30.81389545987213552 ) ) ;
#87941=CARTESIAN_POINT ( 'NONE',  ( -5.326946301144534601, -10.92453946501458439, 33.72985991061850086 ) ) ;
#87942=CARTESIAN_POINT ( 'NONE',  ( -0.7115616988314267255, -12.43535235679832596, 30.55408501211184813 ) ) ;
#87945=ORIENTED_EDGE ( 'NONE', *, *, #74213, .T. ) ;
#87946=EDGE_CURVE ( 'NONE', #43122, #11726, #33489, .T. ) ;
#87947=CARTESIAN_POINT ( 'NONE',  ( -6.988346923633244501, -11.06231777344662781, 33.60647404775220082 ) ) ;
#87948=CARTESIAN_POINT ( 'NONE',  ( -9.442253380669377805, -8.303483539816728154, 34.68545999027711702 ) ) ;
#87949=B_SPLINE_CURVE_WITH_KNOTS ( 'NONE', 3,
 ( #88548, #62364, #27262, #28143, #85207, #45539, #45091, #76786, #21838, #29055 ),
 .UNSPECIFIED., .F., .F.,
 ( 4, 2, 2, 2, 4 ),
 ( 0.0007817359430256293554, 0.0009771253907249952391, 0.001172514838424361123, 0.001367904286123727007, 0.001563293733823092890 ),
 .UNSPECIFIED. ) ;
#87950=ADVANCED_FACE ( 'NONE', ( #86272 ), #4275, .F. ) ;
#87952=EDGE_LOOP ( 'NONE', ( #19519, #56594 ) ) ;
#87953=CARTESIAN_POINT ( 'NONE',  ( 8.096208266067298709, -12.01375889529407637, 32.43194544308182969 ) ) ;
#87954=CARTESIAN_POINT ( 'NONE',  ( 11.47237915910140771, -12.62096338111211580, 30.90682066428152908 ) ) ;
#87955=CARTESIAN_POINT ( 'NONE',  ( 10.74617505635156789, -4.684288915650983043, 34.18129842949671371 ) ) ;
#87956=EDGE_CURVE ( 'NONE', #3816, #13509, #25442, .T. ) ;
#87957=DIRECTION ( 'NONE',  ( -0.000000000000000000, 0.7660444431189791237, -0.6427876096865379196 ) ) ;
#87958=CARTESIAN_POINT ( 'NONE',  ( 17.93472999944368240, -2.657715359629089669, 31.77849191805833584 ) ) ;
#87959=ORIENTED_EDGE ( 'NONE', *, *, #23165, .T. ) ;
#87961=ADVANCED_FACE ( 'NONE', ( #11485 ), #65970, .F. ) ;
#87962=AXIS2_PLACEMENT_3D ( 'NONE', #87238, #74150, #12446 ) ;
#87963=CARTESIAN_POINT ( 'NONE',  ( 17.20771488474786892, -5.582136614379148654, 34.36778462344220486 ) ) ;
#87964=CARTESIAN_POINT ( 'NONE',  ( 9.562159722575994891, -2.647304123082328875, 31.75400227202885972 ) ) ;
#87967=AXIS2_PLACEMENT_3D ( 'NONE', #2654, #30147, #49965 ) ;
#87968=EDGE_LOOP ( 'NONE', ( #62178, #23277 ) ) ;
#87969=LINE ( 'NONE', #24887, #12665 ) ;
#87971=CARTESIAN_POINT ( 'NONE',  ( -5.749945580086544439, -12.01375889529407281, 32.43194544308182969 ) ) ;
#87972=ORIENTED_EDGE ( 'NONE', *, *, #14812, .T. ) ;
#87974=DIRECTION ( 'NONE',  ( 0.000000000000000000, -6.938893903907222067E-15, 1.000000000000000000 ) ) ;
#87975=EDGE_CURVE ( 'NONE', #50820, #4743, #32363, .T. ) ;
#87976=CARTESIAN_POINT ( 'NONE',  ( -9.822454901745908629, -2.619462340734462380, 30.83744416345203021 ) ) ;
#87977=VECTOR ( 'NONE', #34332, 1000.000000000000227 ) ;
#87978=EDGE_CURVE ( 'NONE', #37947, #34931, #31308, .T. ) ;
#87979=CARTESIAN_POINT ( 'NONE',  ( 7.053867364043874488, -12.35292014791297710, 31.75344720912887198 ) ) ;
#87980=FACE_OUTER_BOUND ( 'NONE', #56432, .T. ) ;
#87981=EDGE_CURVE ( 'NONE', #65220, #22041, #66426, .T. ) ;
#87982=ORIENTED_EDGE ( 'NONE', *, *, #71289, .F. ) ;
#87983=FACE_BOUND ( 'NONE', #38291, .T. ) ;
#87984=ORIENTED_EDGE ( 'NONE', *, *, #66179, .F. ) ;
#87987=DIRECTION ( 'NONE',  ( 0.000000000000000000, 0.3420201433256641055, -0.9396926207859100932 ) ) ;
#87988=CARTESIAN_POINT ( 'NONE',  ( -6.857821351800896359, -6.026961402152789304, 34.52809138561124769 ) ) ;
#87989=DIRECTION ( 'NONE',  ( -0.000000000000000000, 0.7660444431189791237, -0.6427876096865379196 ) ) ;
#87990=VERTEX_POINT ( 'NONE', #39415 ) ;
#87991=VERTEX_POINT ( 'NONE', #31761 ) ;
#87992=ORIENTED_EDGE ( 'NONE', *, *, #55821, .T. ) ;
#87993=B_SPLINE_CURVE_WITH_KNOTS ( 'NONE', 3,
 ( #67732, #45674, #73155, #80368, #24957, #65937, #53315, #39821, #52425, #11452 ),
 .UNSPECIFIED., .F., .F.,
 ( 4, 2, 2, 2, 4 ),
 ( 0.000000000000000000, 0.0001954339857564065528, 0.0003908679715128131056, 0.0005863019572692196313, 0.0007817359430256262112 ),
 .UNSPECIFIED. ) ;
#87994=VECTOR ( 'NONE', #5463, 1000.000000000000000 ) ;
#87995=ORIENTED_EDGE ( 'NONE', *, *, #32870, .F. ) ;
#87996=CARTESIAN_POINT ( 'NONE',  ( 2.084766090176160880, -4.887634598454295265, 34.01352882383564946 ) ) ;
#87997=CARTESIAN_POINT ( 'NONE',  ( 16.15384615384603251, -11.06231777344772027, 33.60647404775119895 ) ) ;
#87998=AXIS2_PLACEMENT_3D ( 'NONE', #75389, #34395, #14569 ) ;
#87999=CARTESIAN_POINT ( 'NONE',  ( -15.48079246806219267, -10.76384336483936011, 33.53834819971076087 ) ) ;
#88000=DIRECTION ( 'NONE',  ( -0.000000000000000000, -0.3420201433256694346, -0.9396926207859080948 ) ) ;
#88003=CARTESIAN_POINT ( 'NONE',  ( 17.77707378248385339, -2.554751324335733376, 30.48935550225260727 ) ) ;
#88004=CARTESIAN_POINT ( 'NONE',  ( 17.14217864819909920, -2.625532179533470512, 30.86335684631491105 ) ) ;
#88005=EDGE_LOOP ( 'NONE', ( #570, #12268 ) ) ;
#88006=B_SPLINE_CURVE_WITH_KNOTS ( 'NONE', 3,
 ( #76184, #14487, #35203, #975, #61775, #14941, #6841, #15387, #47830, #55471 ),
 .UNSPECIFIED., .F., .F.,
 ( 4, 2, 2, 2, 4 ),
 ( 0.0007817246256747480398, 0.0009771112852218909357, 0.001172497944769034049, 0.001367884604316177161, 0.001563271263863320057 ),
 .UNSPECIFIED. ) ;
#88007=ORIENTED_EDGE ( 'NONE', *, *, #61330, .F. ) ;
#88008=VERTEX_POINT ( 'NONE', #18244 ) ;
#88009=CARTESIAN_POINT ( 'NONE',  ( 2.084207363968360927, -2.599994579823203367, 30.74605699353653776 ) ) ;
#88010=ORIENTED_EDGE ( 'NONE', *, *, #66417, .T. ) ;
#88011=CARTESIAN_POINT ( 'NONE',  ( 6.699591998512593349, -11.60425143139329940, 33.02411095842164457 ) ) ;
#88012=CARTESIAN_POINT ( 'NONE',  ( -10.61538461538461320, -12.62096338111211580, 30.90682066428153263 ) ) ;
#88013=EDGE_CURVE ( 'NONE', #3792, #58712, #28057, .T. ) ;
#88014=CARTESIAN_POINT ( 'NONE',  ( 15.90384615384615330, -7.566083408709835645, 34.74999999999999289 ) ) ;
#88015=CARTESIAN_POINT ( 'NONE',  ( -15.48074597481782178, -10.06842814019191401, 34.32929386961144758 ) ) ;
#88016=FACE_BOUND ( 'NONE', #87389, .T. ) ;
#88017=VERTEX_POINT ( 'NONE', #59664 ) ;
#88019=ADVANCED_FACE ( 'NONE', ( #38513 ), #30852, .F. ) ;
#88020=CARTESIAN_POINT ( 'NONE',  ( -8.704036787447412493, -2.506253911140448487, 29.99999999999988631 ) ) ;
#88021=EDGE_LOOP ( 'NONE', ( #35431, #39887, #20489, #73179 ) ) ;
#88022=FACE_BOUND ( 'NONE', #25487, .T. ) ;
#88023=CARTESIAN_POINT ( 'NONE',  ( 9.758375025657770152, -5.471508081941601098, 34.59228464037088457 ) ) ;
#88024=CIRCLE ( 'NONE', #72165, 0.2500000000000002220 ) ;
#88025=DIRECTION ( 'NONE',  ( 1.000000000000000000, 0.000000000000000000, 0.000000000000000000 ) ) ;
#88026=ORIENTED_EDGE ( 'NONE', *, *, #54802, .F. ) ;
#88027=CARTESIAN_POINT ( 'NONE',  ( -6.249999999999997335, -7.500000000000001776, 34.75000000000000000 ) ) ;
#88028=DIRECTION ( 'NONE',  ( 0.000000000000000000, 0.000000000000000000, 1.000000000000000000 ) ) ;
#88029=CARTESIAN_POINT ( 'NONE',  ( 1.319344938654610111, -3.300289026998414865, 32.46337939537583139 ) ) ;
#88030=EDGE_LOOP ( 'NONE', ( #13323, #29140 ) ) ;
#88031=CARTESIAN_POINT ( 'NONE',  ( -7.596208436775802930, -8.476813868363244353, 34.90874843262270133 ) ) ;
#88033=CARTESIAN_POINT ( 'NONE',  ( -17.93474486048716088, -12.70778746994558439, 30.41441678777537305 ) ) ;
#88034=ORIENTED_EDGE ( 'NONE', *, *, #49933, .T. ) ;
#88035=VECTOR ( 'NONE', #82841, 1000.000000000000114 ) ;
#88037=CYLINDRICAL_SURFACE ( 'NONE', #74742, 0.2499999999999995559 ) ;
#88038=CARTESIAN_POINT ( 'NONE',  ( 3.930919194939303196, -10.01117774369187252, 34.36070679894347535 ) ) ;
#88039=ORIENTED_EDGE ( 'NONE', *, *, #65277, .T. ) ;
#88040=DIRECTION ( 'NONE',  ( -1.000000000000000000, 0.000000000000000000, 0.000000000000000000 ) ) ;
#88041=CARTESIAN_POINT ( 'NONE',  ( -4.219116599806928214, -2.625532179533445198, 30.86335684631481513 ) ) ;
#88042=DIRECTION ( 'NONE',  ( 0.000000000000000000, 0.3420201433256610524, 0.9396926207859113145 ) ) ;
#88043=CARTESIAN_POINT ( 'NONE',  ( 16.37662582282421653, -12.11081565061823717, 32.26097654155341843 ) ) ;
#88044=CARTESIAN_POINT ( 'NONE',  ( 10.61538461538449418, -11.67786785259630911, 32.92929555188603530 ) ) ;
#88045=CARTESIAN_POINT ( 'NONE',  ( -5.326923076923075762, -2.249999999999998668, 29.75000000000000355 ) ) ;
#88046=CARTESIAN_POINT ( 'NONE',  ( -1.608100328339332474, -5.113361153441934093, 34.14387501736622710 ) ) ;
#88047=CARTESIAN_POINT ( 'NONE',  ( 8.703148389870632329, -2.833524468853757305, 32.15551576947924417 ) ) ;
#88048=CARTESIAN_POINT ( 'NONE',  ( 10.68063975489745232, -9.528491918058460186, 34.59228464037086326 ) ) ;
#88049=DIRECTION ( 'NONE',  ( 0.000000000000000000, 0.4999999999999985567, 0.8660254037844395958 ) ) ;
#88051=ORIENTED_EDGE ( 'NONE', *, *, #10358, .T. ) ;
#88052=ADVANCED_FACE ( 'NONE', ( #85816 ), #13696, .F. ) ;
#88053=CARTESIAN_POINT ( 'NONE',  ( 17.77707378248384629, -4.186968288167451036, 33.49512374952580274 ) ) ;
#88054=ORIENTED_EDGE ( 'NONE', *, *, #29996, .T. ) ;
#88055=VERTEX_POINT ( 'NONE', #53793 ) ;
#88056=EDGE_CURVE ( 'NONE', #87727, #20693, #7393, .T. ) ;
#88057=CARTESIAN_POINT ( 'NONE',  ( 17.07692307692307665, -12.78798330534102945, 29.74999999999997868 ) ) ;
#88058=ORIENTED_EDGE ( 'NONE', *, *, #12674, .T. ) ;
#88059=CARTESIAN_POINT ( 'NONE',  ( -5.299850035829924977, -11.43668979543635089, 33.22377378376089752 ) ) ;
#88061=CARTESIAN_POINT ( 'NONE',  ( 17.75002325595141173, -4.818429247618089661, 34.26397095200675125 ) ) ;
#88062=CARTESIAN_POINT ( 'NONE',  ( -9.019254006523732770, -3.202444869320336451, 32.30641848906366675 ) ) ;
#88063=CARTESIAN_POINT ( 'NONE',  ( 9.757562831820528970, -9.528491918058460186, 34.59228464037086326 ) ) ;
#88064=CARTESIAN_POINT ( 'NONE',  ( -4.826868657009621089, -2.544122305571457687, 31.48381861865059150 ) ) ;
#88068=CARTESIAN_POINT ( 'NONE',  ( -7.146561847641255127, -4.988325925672468131, 34.36044203135681130 ) ) ;
#88069=CARTESIAN_POINT ( 'NONE',  ( -0.4615384615384611200, -13.37000171582298513, 34.34916445242398453 ) ) ;
#88070=EDGE_CURVE ( 'NONE', #4121, #32754, #39877, .T. ) ;
#88072=CARTESIAN_POINT ( 'NONE',  ( 18.00000000000030553, -2.506253911140615021, 30.00000000000323297 ) ) ;
#88074=VERTEX_POINT ( 'NONE', #186 ) ;
#88075=CARTESIAN_POINT ( 'NONE',  ( -9.469296340694842939, -3.587049720035815348, 32.86302985866382897 ) ) ;
#88076=CARTESIAN_POINT ( 'NONE',  ( 15.29683656411930848, -11.91647553114624358, 32.58852847137148245 ) ) ;
#88077=CARTESIAN_POINT ( 'NONE',  ( -39.05038313613820122, -2.499999999999999556, 27.25000000000000000 ) ) ;
#88078=CARTESIAN_POINT ( 'NONE',  ( -6.000000000000119904, -3.835265460704628371, 33.15142922262033665 ) ) ;
#88079=CARTESIAN_POINT ( 'NONE',  ( 8.519254038288414321, -4.236021600441997492, 33.53823185664189310 ) ) ;
#88081=CARTESIAN_POINT ( 'NONE',  ( -0.7115151924808158501, -6.567427716900047230, 34.66269422305636283 ) ) ;
#88082=EDGE_CURVE ( 'NONE', #13990, #3335, #3316, .T. ) ;
#88084=ORIENTED_EDGE ( 'NONE', *, *, #25481, .F. ) ;
#88085=CARTESIAN_POINT ( 'NONE',  ( 1.254468175177166245, -5.195881422630166391, 34.18770438780619259 ) ) ;
#88086=EDGE_LOOP ( 'NONE', ( #42813, #37858 ) ) ;
#88087=B_SPLINE_CURVE_WITH_KNOTS ( 'NONE', 3,
 ( #43368, #64497, #9153, #16772, #52330, #2805, #79824, #72158, #86589, #10913 ),
 .UNSPECIFIED., .F., .F.,
 ( 4, 2, 2, 2, 4 ),
 ( 0.0007817359430256294638, 0.0009771253907249974075, 0.001172514838424365460, 0.001367904286123733295, 0.001563293733823094191 ),
 .UNSPECIFIED. ) ;
#88088=EDGE_CURVE ( 'NONE', #62746, #30988, #33964, .T. ) ;
#88089=VERTEX_POINT ( 'NONE', #74515 ) ;
#88091=CARTESIAN_POINT ( 'NONE',  ( 5.076923076923075762, -8.120952969808772792, 34.71129190930000163 ) ) ;
#88092=VECTOR ( 'NONE', #76977, 1000.000000000000000 ) ;
#88093=CARTESIAN_POINT ( 'NONE',  ( -2.531177232256636156, -9.417330523894424488, 34.63758898049880486 ) ) ;
#88094=CARTESIAN_POINT ( 'NONE',  ( -4.153846153846273204, -4.481592998941358097, 33.73612834414048933 ) ) ;
#88095=CARTESIAN_POINT ( 'NONE',  ( 11.76147438255493149, -2.308499170217967134, 30.53291367094873721 ) ) ;
#88099=VERTEX_POINT ( 'NONE', #12810 ) ;
#88100=ORIENTED_EDGE ( 'NONE', *, *, #61596, .T. ) ;
#88101=VERTEX_POINT ( 'NONE', #61430 ) ;
#88102=CARTESIAN_POINT ( 'NONE',  ( -17.07692307692319744, -11.94971097300221174, 32.03036669348237098 ) ) ;
#88103=FACE_OUTER_BOUND ( 'NONE', #84885, .T. ) ;
#88105=CARTESIAN_POINT ( 'NONE',  ( -15.29603967673000575, -11.48612834413959582, 32.76840700105983473 ) ) ;
#88106=CARTESIAN_POINT ( 'NONE',  ( -15.10024379253558635, -9.503571793651731880, 34.60286762892837942 ) ) ;
#88107=CARTESIAN_POINT ( 'NONE',  ( 14.08476609017615644, -12.39988816332205701, 30.74660775122750778 ) ) ;
#88108=ORIENTED_EDGE ( 'NONE', *, *, #87978, .T. ) ;
#88110=CARTESIAN_POINT ( 'NONE',  ( 17.07692307692307665, -12.37446782046654192, 30.86335684631486131 ) ) ;
#88111=ORIENTED_EDGE ( 'NONE', *, *, #4045, .T. ) ;
#88112=CARTESIAN_POINT ( 'NONE',  ( -9.915233909823838232, -4.887634598454295265, 34.01352882383564946 ) ) ;
#88113=FACE_OUTER_BOUND ( 'NONE', #30638, .T. ) ;
#88114=AXIS2_PLACEMENT_3D ( 'NONE', #62507, #8918, #62077 ) ;
#88116=VERTEX_POINT ( 'NONE', #67760 ) ;
#88117=CARTESIAN_POINT ( 'NONE',  ( 8.068933515131909928, -4.226511098958374291, 33.85474049983370293 ) ) ;
#88118=ORIENTED_EDGE ( 'NONE', *, *, #82772, .F. ) ;
#88120=CARTESIAN_POINT ( 'NONE',  ( 17.20744851515672025, -12.15418822224088657, 32.17964115625579069 ) ) ;
#88121=FACE_BOUND ( 'NONE', #10525, .T. ) ;
#88122=FACE_OUTER_BOUND ( 'NONE', #26441, .T. ) ;
#88125=CARTESIAN_POINT ( 'NONE',  ( -12.46153846153846168, -10.51840700105979565, 33.73612834413961536 ) ) ;
#88126=CARTESIAN_POINT ( 'NONE',  ( -14.30769230769242739, -2.625532179533778709, 30.86335684631627174 ) ) ;
#88127=CARTESIAN_POINT ( 'NONE',  ( 0.6843180028068693854, -12.44528174975671853, 30.48912976160716681 ) ) ;
#88129=CARTESIAN_POINT ( 'NONE',  ( -18.24997674404858827, -12.65889640711025521, 30.72598325615533454 ) ) ;
#88130=CARTESIAN_POINT ( 'NONE',  ( 14.30769230769231015, -9.905515769479276145, 34.41647553114623292 ) ) ;
#88131=CARTESIAN_POINT ( 'NONE',  ( -12.59222992820602371, -12.11776431015576172, 31.66791131148498906 ) ) ;
#88132=LINE ( 'NONE', #55193, #11233 ) ;
#88133=DIRECTION ( 'NONE',  ( 0.000000000000000000, 1.000000000000000000, 0.000000000000000000 ) ) ;
#88134=FACE_BOUND ( 'NONE', #77032, .T. ) ;
#88135=CARTESIAN_POINT ( 'NONE',  ( -6.988346923633242724, -12.51329471203370325, 31.30864560766548976 ) ) ;
#88136=DIRECTION ( 'NONE',  ( 0.000000000000000000, 0.6427876096865373645, -0.7660444431189797898 ) ) ;
#88137=CARTESIAN_POINT ( 'NONE',  ( -9.469294848214296678, -11.98016756924215009, 32.48728574198911190 ) ) ;
#88138=CARTESIAN_POINT ( 'NONE',  ( -18.25002322422145440, -2.341070481393819236, 30.72580821765574299 ) ) ;
#88139=CARTESIAN_POINT ( 'NONE',  ( -2.177166869458664777, -12.50538340440932217, 31.33453814440721885 ) ) ;
#88140=CARTESIAN_POINT ( 'NONE',  ( 13.31853300525524908, -2.486705287966279432, 31.30864560766542937 ) ) ;
#88142=ORIENTED_EDGE ( 'NONE', *, *, #40533, .F. ) ;
#88143=LINE ( 'NONE', #12024, #8762 ) ;
#88144=VERTEX_POINT ( 'NONE', #33536 ) ;
#88145=EDGE_CURVE ( 'NONE', #47721, #5191, #15145, .T. ) ;
#88146=AXIS2_PLACEMENT_3D ( 'NONE', #87876, #82868, #81541 ) ;
#88148=ORIENTED_EDGE ( 'NONE', *, *, #75261, .F. ) ;
#88149=CARTESIAN_POINT ( 'NONE',  ( -15.36137959039375644, -7.722926236386453702, 34.74524107206102030 ) ) ;
#88150=CARTESIAN_POINT ( 'NONE',  ( -1.384615384615505151, -10.90142922262034020, 33.41473453929536674 ) ) ;
#88151=CYLINDRICAL_SURFACE ( 'NONE', #12213, 0.2500000000000004996 ) ;
#88152=ORIENTED_EDGE ( 'NONE', *, *, #84655, .F. ) ;
#88153=LINE ( 'NONE', #53891, #55792 ) ;
#88154=CARTESIAN_POINT ( 'NONE',  ( 6.250054419913453785, -3.435999193479609914, 33.07426656108010832 ) ) ;
#88156=CARTESIAN_POINT ( 'NONE',  ( 4.403900465484467119, -10.66356715214248396, 33.62249196103329751 ) ) ;
#88157=CARTESIAN_POINT ( 'NONE',  ( 4.826899839630111266, -5.056417327199099532, 34.11270091957320716 ) ) ;
#88158=CARTESIAN_POINT ( 'NONE',  ( 8.068933387422253745, -11.89424750095246175, 32.13594075562310337 ) ) ;
#88159=CARTESIAN_POINT ( 'NONE',  ( 10.61538461538461675, -2.486705287966279876, 31.30864560766543647 ) ) ;
#88160=CARTESIAN_POINT ( 'NONE',  ( -12.23852561744506851, -8.282913670948747864, 34.94150082978203642 ) ) ;
#88161=CARTESIAN_POINT ( 'NONE',  ( 1.634560793993430350, -10.18230066228895758, 34.26354781536631577 ) ) ;
#88163=CARTESIAN_POINT ( 'NONE',  ( -4.403822897894744237, -2.920706130388546651, 32.31842814019191223 ) ) ;
#88164=ADVANCED_FACE ( 'NONE', ( #40738 ), #6505, .F. ) ;
#88165=CARTESIAN_POINT ( 'NONE',  ( -11.31545018684868964, -10.61302985866383963, 33.66295027996417843 ) ) ;
#88167=FACE_OUTER_BOUND ( 'NONE', #26269, .T. ) ;
#88168=CARTESIAN_POINT ( 'NONE',  ( 8.992242120843616959, -11.24521262558773493, 33.06293181088029343 ) ) ;
#88170=DIRECTION ( 'NONE',  ( 0.000000000000000000, 0.1736481776669275834, 0.9848077530122086864 ) ) ;
#88171=FACE_OUTER_BOUND ( 'NONE', #54638, .T. ) ;
#88172=EDGE_LOOP ( 'NONE', ( #24084, #52561 ) ) ;
#88173=DIRECTION ( 'NONE',  ( 0.000000000000000000, 0.9848077530122072432, -0.1736481776669354937 ) ) ;
#88174=CARTESIAN_POINT ( 'NONE',  ( 9.627037691751372250, -12.70778746994557551, 30.41441678777548319 ) ) ;
#88175=CARTESIAN_POINT ( 'NONE',  ( 11.40831356872984514, -3.069018819979302926, 32.56621877034667278 ) ) ;
#88177=FACE_OUTER_BOUND ( 'NONE', #12063, .T. ) ;
#88178=B_SPLINE_CURVE_WITH_KNOTS ( 'NONE', 3,
 ( #34460, #5657, #80894, #19176, #39903, #61921, #27699, #60595, #6109, #88110 ),
 .UNSPECIFIED., .F., .F.,
 ( 4, 2, 2, 2, 4 ),
 ( 0.0007817359430256323911, 0.0009771253907249991422, 0.001172514838424365893, 0.001367904286123732644, 0.001563293733823099396 ),
 .UNSPECIFIED. ) ;
#88179=CARTESIAN_POINT ( 'NONE',  ( -15.16470189741915675, -11.91647553114624358, 32.58852847137148245 ) ) ;
#88180=LINE ( 'NONE', #53016, #24120 ) ;
#88181=VECTOR ( 'NONE', #24996, 1000.000000000000114 ) ;
#88182=ORIENTED_EDGE ( 'NONE', *, *, #48592, .F. ) ;
#88183=CARTESIAN_POINT ( 'NONE',  ( 2.307692307692309264, -3.937682226553329556, 33.60647404775216529 ) ) ;
#88184=CARTESIAN_POINT ( 'NONE',  ( 6.700150705560774966, -4.887634598454295265, 34.01352882383564946 ) ) ;
#88185=EDGE_CURVE ( 'NONE', #26386, #55965, #48360, .T. ) ;
#88186=EDGE_CURVE ( 'NONE', #48079, #10580, #69083, .T. ) ;
#88187=CARTESIAN_POINT ( 'NONE',  ( -11.53846153846165912, -8.613356846316285953, 34.62446782046622218 ) ) ;
#88188=EDGE_LOOP ( 'NONE', ( #78406, #14620 ) ) ;
#88189=ORIENTED_EDGE ( 'NONE', *, *, #46379, .F. ) ;
#88191=EDGE_LOOP ( 'NONE', ( #6304, #80209 ) ) ;
#88192=CARTESIAN_POINT ( 'NONE',  ( 5.326977388561389581, -12.17597550085003633, 31.52189283813461884 ) ) ;
#88194=CARTESIAN_POINT ( 'NONE',  ( -16.28399412357784826, -3.069018819979305146, 32.56621877034667278 ) ) ;
#88195=CARTESIAN_POINT ( 'NONE',  ( -7.912236225513981758, -10.67929555188718460, 33.92786785259543336 ) ) ;
#88196=CARTESIAN_POINT ( 'NONE',  ( 5.207448778686637247, -6.001044277235011215, 34.52024696741798948 ) ) ;
#88198=ORIENTED_EDGE ( 'NONE', *, *, #42392, .T. ) ;
#88199=VERTEX_POINT ( 'NONE', #77167 ) ;
#88200=CARTESIAN_POINT ( 'NONE',  ( -8.096130577096200653, -4.943428324936579799, 34.04746400365624481 ) ) ;
#88201=ORIENTED_EDGE ( 'NONE', *, *, #80630, .F. ) ;
#88202=CARTESIAN_POINT ( 'NONE',  ( 11.53846153846153832, -8.564572088678739092, 35.78748833219616898 ) ) ;
#88203=B_SPLINE_CURVE_WITH_KNOTS ( 'NONE', 3,
 ( #1883, #64902, #16721, #57716, #28935, #56391, #63581, #71664, #56823, #50504 ),
 .UNSPECIFIED., .F., .F.,
 ( 4, 2, 2, 2, 4 ),
 ( 0.000000000000000000, 0.0001954311564186882026, 0.0003908623128373764051, 0.0005862934692560646619, 0.0007817246256747528103 ),
 .UNSPECIFIED. ) ;
#88204=B_SPLINE_CURVE_WITH_KNOTS ( 'NONE', 3,
 ( #65985, #2503, #51121, #79518, #17820, #71406, #16475, #23667, #79958, #38983 ),
 .UNSPECIFIED., .F., .F.,
 ( 4, 2, 2, 2, 4 ),
 ( 0.000000000000000000, 0.0001954311564186861155, 0.0003908623128373722310, 0.0005862934692560583735, 0.0007817246256747444619 ),
 .UNSPECIFIED. ) ;
#88205=CARTESIAN_POINT ( 'NONE',  ( -5.076923076923075762, -13.57706302396349152, 30.56769352161908060 ) ) ;
#88206=VECTOR ( 'NONE', #6644, 1000.000000000000114 ) ;
#88207=CARTESIAN_POINT ( 'NONE',  ( 10.61538461538449596, -6.879047030192662504, 34.71129190930017927 ) ) ;
#88208=CARTESIAN_POINT ( 'NONE',  ( -5.869208192175211281, -4.118422570099827595, 33.43335022499816489 ) ) ;
#88211=ORIENTED_EDGE ( 'NONE', *, *, #55001, .T. ) ;
#88212=ORIENTED_EDGE ( 'NONE', *, *, #23010, .T. ) ;
#88213=CARTESIAN_POINT ( 'NONE',  ( -5.326923076923075762, -7.500000000000001776, 34.75000000000000000 ) ) ;
#88214=DIRECTION ( 'NONE',  ( -0.000000000000000000, -0.5000000000000009992, -0.8660254037844380415 ) ) ;
#88215=ORIENTED_EDGE ( 'NONE', *, *, #83228, .T. ) ;
#88217=DIRECTION ( 'NONE',  ( -0.000000000000000000, -0.3420201433256694346, -0.9396926207859080948 ) ) ;
#88218=EDGE_LOOP ( 'NONE', ( #51165, #40524, #46305, #86256 ) ) ;
#88219=CARTESIAN_POINT ( 'NONE',  ( -11.47239420511146157, -3.937682226553329556, 33.60647404775216529 ) ) ;
#88220=CARTESIAN_POINT ( 'NONE',  ( 8.835299120233207404, -12.37446782046654192, 30.86335684631486842 ) ) ;
#88221=CARTESIAN_POINT ( 'NONE',  ( 12.68431813051652668, -9.418065098278013636, 34.63729479722530158 ) ) ;
#88222=FACE_BOUND ( 'NONE', #5189, .T. ) ;
#88224=CARTESIAN_POINT ( 'NONE',  ( -1.384615384615505151, -11.94971097300221174, 32.03036669348237098 ) ) ;
#88225=CARTESIAN_POINT ( 'NONE',  ( -10.48459417441766561, -10.70102852606553157, 33.91149625220312913 ) ) ;
#88227=CARTESIAN_POINT ( 'NONE',  ( 11.53846153846153832, -12.78798330534102945, 29.74999999999997868 ) ) ;
#88228=CARTESIAN_POINT ( 'NONE',  ( -39.05038313613820122, -2.499999999999999556, 29.75000000000000355 ) ) ;
#88229=LINE ( 'NONE', #19301, #28992 ) ;
#88230=VERTEX_POINT ( 'NONE', #9586 ) ;
#88231=CARTESIAN_POINT ( 'NONE',  ( -16.40384615384615330, -7.500000000000001776, 34.75000000000000000 ) ) ;
#88232=CARTESIAN_POINT ( 'NONE',  ( -10.61538461538473399, -2.625532179533778709, 30.86335684631627174 ) ) ;
#88233=ORIENTED_EDGE ( 'NONE', *, *, #39644, .T. ) ;
#88234=ORIENTED_EDGE ( 'NONE', *, *, #39768, .T. ) ;
#88235=EDGE_CURVE ( 'NONE', #28787, #47389, #58200, .T. ) ;
#88236=CARTESIAN_POINT ( 'NONE',  ( -3.230769230769229949, -13.20930481340135110, 34.54067556320372745 ) ) ;
#88239=CARTESIAN_POINT ( 'NONE',  ( -14.30769230769230660, -4.786620604624113540, 33.94971097300155094 ) ) ;
#88240=CARTESIAN_POINT ( 'NONE',  ( -15.48076923076922995, -7.500000000000001776, 34.75000000000000000 ) ) ;
#88241=EDGE_LOOP ( 'NONE', ( #50022, #69134 ) ) ;
#88242=CARTESIAN_POINT ( 'NONE',  ( -9.915792616872021625, -9.417330523894424488, 34.63758898049880486 ) ) ;
#88243=CARTESIAN_POINT ( 'NONE',  ( -7.146003140593070846, -9.886141570436013382, 34.14413921362392301 ) ) ;
#88244=FACE_BOUND ( 'NONE', #17824, .T. ) ;
#88245=CARTESIAN_POINT ( 'NONE',  ( -18.13069146666756026, -3.062553014421049991, 32.05460306192773601 ) ) ;
#88246=CARTESIAN_POINT ( 'NONE',  ( 6.000000000000001776, -6.343179335718451384, 34.87096338111211935 ) ) ;
#88247=CARTESIAN_POINT ( 'NONE',  ( -13.44988538517170440, -2.379036618887870436, 30.90682066428147934 ) ) ;
#88248=CARTESIAN_POINT ( 'NONE',  ( 3.480769230770650147, -7.500000000000154543, 35.00000000000007105 ) ) ;
#88250=CARTESIAN_POINT ( 'NONE',  ( -8.638438961405984884, -12.11778462344220841, 31.66786338562085135 ) ) ;
#88252=EDGE_LOOP ( 'NONE', ( #36556, #25731 ) ) ;
#88253=EDGE_LOOP ( 'NONE', ( #48214, #34108 ) ) ;
#88254=EDGE_CURVE ( 'NONE', #45693, #70825, #14582, .T. ) ;
#88255=CARTESIAN_POINT ( 'NONE',  ( -9.692307692307691624, -2.486705287966279876, 31.30864560766543647 ) ) ;
#88256=CARTESIAN_POINT ( 'NONE',  ( 15.23076923076923173, -13.87047571288749737, 32.06866353760679544 ) ) ;
#88257=DIRECTION ( 'NONE',  ( 0.000000000000000000, 0.3420201433256641055, -0.9396926207859100932 ) ) ;
#88258=CARTESIAN_POINT ( 'NONE',  ( 3.230769230769231726, -12.29105614889573062, 35.45975837776705220 ) ) ;
#88259=EDGE_CURVE ( 'NONE', #64445, #67532, #17371, .T. ) ;
#88260=CARTESIAN_POINT ( 'NONE',  ( 4.153846153846154188, -5.180354513474913603, 36.12317359536750416 ) ) ;
#88262=CARTESIAN_POINT ( 'NONE',  ( -8.899921372341079717, -9.929715669179220328, 34.40415004197138416 ) ) ;
#88263=CARTESIAN_POINT ( 'NONE',  ( -6.130690603110307002, -8.191372820521381826, 34.95448215188423546 ) ) ;
#88264=CARTESIAN_POINT ( 'NONE',  ( -5.010855743572999899, -2.292212530054420494, 30.41441678777542990 ) ) ;
#88266=CARTESIAN_POINT ( 'NONE',  ( -6.066083410955879884, -2.721908614388772740, 31.22303859784724622 ) ) ;
#88267=CARTESIAN_POINT ( 'NONE',  ( 13.38461538461538680, -13.87047571288749737, 32.06866353760679544 ) ) ;
#88268=DIRECTION ( 'NONE',  ( -0.000000000000000000, 1.000000000000000000, 3.491481338843133355E-15 ) ) ;
#88269=AXIS2_PLACEMENT_3D ( 'NONE', #75985, #40881, #54828 ) ;
#88270=CARTESIAN_POINT ( 'NONE',  ( 4.153846153846154188, -11.16473453929635440, 33.15142922261926373 ) ) ;
#88271=EDGE_CURVE ( 'NONE', #55035, #33529, #81835, .T. ) ;
#88272=CARTESIAN_POINT ( 'NONE',  ( 7.846153846153846700, -2.900454961884010974, 35.62045528018868623 ) ) ;
#88274=CARTESIAN_POINT ( 'NONE',  ( -3.230769230769229949, -12.10708131394839349, 31.69288490824020244 ) ) ;
#88275=CARTESIAN_POINT ( 'NONE',  ( 15.23076923076923173, -6.435427911321262684, 35.78748833219616898 ) ) ;
#88279=AXIS2_PLACEMENT_3D ( 'NONE', #71015, #49849, #7993 ) ;
#88280=CARTESIAN_POINT ( 'NONE',  ( -5.999999999999998224, -12.34228464037088635, 31.77849191805839268 ) ) ;
#88281=SURFACE_STYLE_FILL_AREA ( #38289 ) ;
#88282=DIRECTION ( 'NONE',  ( -0.000000000000000000, 0.8660254037844397068, -0.4999999999999978906 ) ) ;
#88283=CARTESIAN_POINT ( 'NONE',  ( 5.076923076922953193, -4.320704448113951379, 33.92786785259630022 ) ) ;
#88284=ORIENTED_EDGE ( 'NONE', *, *, #61851, .F. ) ;
#88286=CARTESIAN_POINT ( 'NONE',  ( 3.296836564119306701, -8.164416787775445883, 34.95778746994558617 ) ) ;
#88288=DIRECTION ( 'NONE',  ( 0.000000000000000000, 0.4999999999999985567, 0.8660254037844395958 ) ) ;
#88289=CARTESIAN_POINT ( 'NONE',  ( -14.30769230769242917, -11.06231777344772027, 33.60647404775119895 ) ) ;
#88290=B_SPLINE_CURVE_WITH_KNOTS ( 'NONE', 3,
 ( #69567, #76777, #7874, #35339, #42987, #62791, #15078, #71330, #49736, #55606 ),
 .UNSPECIFIED., .F., .F.,
 ( 4, 2, 2, 2, 4 ),
 ( 0.0007817359430256364027, 0.0009771253907250043464, 0.001172514838424372399, 0.001367904286123740234, 0.001563293733823108286 ),
 .UNSPECIFIED. ) ;
#88291=ORIENTED_EDGE ( 'NONE', *, *, #27684, .T. ) ;
#88292=B_SPLINE_CURVE_WITH_KNOTS ( 'NONE', 3,
 ( #14372, #28327, #70206, #55797, #83285, #21572, #43611, #14829, #49043, #76523 ),
 .UNSPECIFIED., .F., .F.,
 ( 4, 2, 2, 2, 4 ),
 ( 0.0007817246256747473893, 0.0009771112852218909357, 0.001172497944769034482, 0.001367884604316178246, 0.001563271263863321792 ),
 .UNSPECIFIED. ) ;
#88294=CARTESIAN_POINT ( 'NONE',  ( -15.93041919198458167, -7.630147231320743018, 34.74852402298682819 ) ) ;
#88295=ADVANCED_FACE ( 'NONE', ( #70863 ), #1068, .F. ) ;
#88296=CARTESIAN_POINT ( 'NONE',  ( 2.057669083470850424, -12.68155406624981119, 30.59749803192733708 ) ) ;
#88298=ADVANCED_FACE ( 'NONE', ( #15032 ), #42505, .F. ) ;
#88300=ORIENTED_EDGE ( 'NONE', *, *, #15790, .F. ) ;
#88301=CARTESIAN_POINT ( 'NONE',  ( -17.75005459062195712, -4.932303261841486375, 34.32971442181322885 ) ) ;
#88302=CARTESIAN_POINT ( 'NONE',  ( -0.3954701105360241553, -10.51840700105979565, 33.73612834413962247 ) ) ;
#88303=EDGE_CURVE ( 'NONE', #88905, #42352, #1515, .T. ) ;
#88304=CARTESIAN_POINT ( 'NONE',  ( 17.99999999999987566, -10.33852847137269571, 34.16647553114546554 ) ) ;
#88305=CARTESIAN_POINT ( 'NONE',  ( 2.307692307692309264, -1.242168528481310874, 33.36296068462461051 ) ) ;
#88306=EDGE_CURVE ( 'NONE', #69932, #15414, #22226, .T. ) ;
#88307=CARTESIAN_POINT ( 'NONE',  ( -12.46153846153858247, -6.026961402154118019, 34.52809138561165270 ) ) ;
#88308=CARTESIAN_POINT ( 'NONE',  ( 7.053602361310569613, -8.630441415882550871, 34.87705825610312615 ) ) ;
#88309=CARTESIAN_POINT ( 'NONE',  ( 0.3313904918067639982, -2.373036134822905208, 30.88089517874951540 ) ) ;
#88310=FACE_OUTER_BOUND ( 'NONE', #5233, .T. ) ;
#88312=ORIENTED_EDGE ( 'NONE', *, *, #12957, .T. ) ;
#88313=CARTESIAN_POINT ( 'NONE',  ( 7.146089767170319185, -12.64618726649961289, 30.78989965857442712 ) ) ;
#88314=EDGE_LOOP ( 'NONE', ( #26232, #18262, #5137, #15161 ) ) ;
#88315=CARTESIAN_POINT ( 'NONE',  ( 10.61538461538493117, -2.255955759149395501, 30.00000000000324363 ) ) ;
#88316=CARTESIAN_POINT ( 'NONE',  ( 12.68431800280686694, -3.236590943229499029, 32.36255958852954251 ) ) ;
#88317=VERTEX_POINT ( 'NONE', #36199 ) ;
#88318=CARTESIAN_POINT ( 'NONE',  ( 15.48082365068268018, -9.233818618650603938, 34.70587769442853698 ) ) ;
#88319=ORIENTED_EDGE ( 'NONE', *, *, #5993, .T. ) ;
#88320=CARTESIAN_POINT ( 'NONE',  ( 16.85399685940691938, -9.886141570436013382, 34.14413921362392301 ) ) ;
#88321=ORIENTED_EDGE ( 'NONE', *, *, #10368, .F. ) ;
#88322=CARTESIAN_POINT ( 'NONE',  ( -18.22348492456433178, -9.417330523894424488, 34.63758898049880486 ) ) ;
#88323=EDGE_CURVE ( 'NONE', #16148, #68002, #8603, .T. ) ;
#88324=VECTOR ( 'NONE', #79733, 1000.000000000000000 ) ;
#88325=CARTESIAN_POINT ( 'NONE',  ( -16.21911659980693443, -6.879047030191174805, 34.71129190930000163 ) ) ;
#88326=CARTESIAN_POINT ( 'NONE',  ( 7.846153846153846700, -10.51840700105979565, 33.73612834413961536 ) ) ;
#88327=FACE_BOUND ( 'NONE', #78404, .T. ) ;
#88328=AXIS2_PLACEMENT_3D ( 'NONE', #45613, #65874, #59570 ) ;
#88329=DIRECTION ( 'NONE',  ( -0.000000000000000000, -0.9396926207859093161, -0.3420201433256663259 ) ) ;
#88330=CARTESIAN_POINT ( 'NONE',  ( 1.254140199539667933, -7.276987145209184327, 34.99546412871779211 ) ) ;
#88331=EDGE_CURVE ( 'NONE', #28403, #71149, #37496, .T. ) ;
#88332=CARTESIAN_POINT ( 'NONE',  ( -1.607542343522232242, -2.308479472611653094, 30.53278059502174457 ) ) ;
#88335=CYLINDRICAL_SURFACE ( 'NONE', #23173, 0.2499999999999997502 ) ;
#88337=B_SPLINE_CURVE_WITH_KNOTS ( 'NONE', 3,
 ( #79392, #50132, #17237, #8726, #36204, #84834, #10492, #57340, #23112, #23543 ),
 .UNSPECIFIED., .F., .F.,
 ( 4, 2, 2, 2, 4 ),
 ( 0.000000000000000000, 0.0001954339857564076641, 0.0003908679715128153282, 0.0005863019572692229923, 0.0007817359430256306564 ),
 .UNSPECIFIED. ) ;
#88338=ORIENTED_EDGE ( 'NONE', *, *, #64036, .F. ) ;
#88339=ORIENTED_EDGE ( 'NONE', *, *, #11451, .T. ) ;
#88341=DIRECTION ( 'NONE',  ( -0.000000000000000000, 0.7660444431189791237, -0.6427876096865379196 ) ) ;
#88342=DIRECTION ( 'NONE',  ( -0.000000000000000000, -0.000000000000000000, -1.000000000000000000 ) ) ;
#88343=DIRECTION ( 'NONE',  ( -0.000000000000000000, 0.8660254037844397068, -0.4999999999999978906 ) ) ;
#88345=CARTESIAN_POINT ( 'NONE',  ( 14.30769230769231015, -3.513871655860378418, 32.76840700105978499 ) ) ;
#88346=CARTESIAN_POINT ( 'NONE',  ( 1.634669804528839476, -4.074993327901524687, 33.72946981652012255 ) ) ;
#88347=VERTEX_POINT ( 'NONE', #4614 ) ;
#88348=CYLINDRICAL_SURFACE ( 'NONE', #50089, 0.2499999999999998890 ) ;
#88349=CARTESIAN_POINT ( 'NONE',  ( -5.011667505647053211, -2.625532179533470512, 30.86335684631491105 ) ) ;
#88350=CARTESIAN_POINT ( 'NONE',  ( -8.992156986746916658, -12.15238873228292071, 31.58232369045353849 ) ) ;
#88351=DIRECTION ( 'NONE',  ( -0.000000000000000000, -0.9848077530122086864, -0.1736481776669273613 ) ) ;
#88352=ORIENTED_EDGE ( 'NONE', *, *, #8845, .F. ) ;
#88355=EDGE_CURVE ( 'NONE', #4784, #71827, #48293, .T. ) ;
#88356=CARTESIAN_POINT ( 'NONE',  ( 15.23076923076923173, -6.386643153685126251, 34.62446782046654192 ) ) ;
#88357=ORIENTED_EDGE ( 'NONE', *, *, #67325, .T. ) ;
#88359=CARTESIAN_POINT ( 'NONE',  ( 14.53047197667037516, -5.827830569534417471, 34.72679350104403539 ) ) ;
#88360=DIRECTION ( 'NONE',  ( 0.000000000000000000, 0.9396926207859126468, 0.3420201433256571111 ) ) ;
#88361=EDGE_CURVE ( 'NONE', #63342, #27014, #11785, .T. ) ;
#88362=CARTESIAN_POINT ( 'NONE',  ( 1.384615384615264011, -6.835583212225970762, 34.95778746994575670 ) ) ;
#88363=CARTESIAN_POINT ( 'NONE',  ( 9.757563263583717728, -6.026961402152789304, 34.52809138561124769 ) ) ;
#88366=CARTESIAN_POINT ( 'NONE',  ( -15.45369544828537833, -11.76352882383564769, 32.36236540154569497 ) ) ;
#88367=CARTESIAN_POINT ( 'NONE',  ( 0.4615384615383396616, -10.21337939537710326, 33.94971097300076224 ) ) ;
#88369=CARTESIAN_POINT ( 'NONE',  ( -15.48076923076922995, -2.499999999999998668, 29.75000000000000355 ) ) ;
#88370=CARTESIAN_POINT ( 'NONE',  ( -5.999999999999998224, -1.509761064869970415, 31.06009739812519044 ) ) ;
#88371=CARTESIAN_POINT ( 'NONE',  ( 5.076923076923075762, -1.044019251281081972, 31.83374038241031911 ) ) ;
#88372=CARTESIAN_POINT ( 'NONE',  ( 9.915319043920543862, -10.61302985866384141, 33.66295027996417843 ) ) ;
#88373=CARTESIAN_POINT ( 'NONE',  ( 2.307692307692186251, -2.657715359629662544, 31.77849191805970364 ) ) ;
#88374=CARTESIAN_POINT ( 'NONE',  ( -8.638440328263820689, -9.084667340241226796, 34.75534355489798344 ) ) ;
#88375=CARTESIAN_POINT ( 'NONE',  ( -0.6844646790546093928, -12.39988816332205701, 30.74660775122750778 ) ) ;
#88377=VERTEX_POINT ( 'NONE', #64515 ) ;
#88378=B_SPLINE_CURVE_WITH_KNOTS ( 'NONE', 3,
 ( #71543, #37762, #65228, #9850, #58461, #53044, #18390, #52155, #45852, #73333 ),
 .UNSPECIFIED., .F., .F.,
 ( 4, 2, 2, 2, 4 ),
 ( 0.0007817246256747452209, 0.0009771112852218887673, 0.001172497944769032531, 0.001367884604316176294, 0.001563271263863319840 ),
 .UNSPECIFIED. ) ;
#88380=CARTESIAN_POINT ( 'NONE',  ( 0.4615384615383396616, -3.300289026999228881, 32.46337939537708905 ) ) ;
#88381=EDGE_LOOP ( 'NONE', ( #22087, #68536, #74677, #60775 ) ) ;
#88382=CARTESIAN_POINT ( 'NONE',  ( -12.52762187249434156, -11.69971097300155272, 32.46337939537587403 ) ) ;
#88383=CARTESIAN_POINT ( 'NONE',  ( -3.165513659493206067, -6.026961402152789304, 34.52809138561124769 ) ) ;
#88384=CARTESIAN_POINT ( 'NONE',  ( -6.923076923076922462, -5.557115091759785130, 34.35708131394839171 ) ) ;
#88385=CARTESIAN_POINT ( 'NONE',  ( 0.4615384615383382183, -4.320704448113951379, 33.92786785259630022 ) ) ;
#88386=CARTESIAN_POINT ( 'NONE',  ( 0.6845513056318547340, -2.308499170217967134, 30.53291367094873721 ) ) ;
#88387=ORIENTED_EDGE ( 'NONE', *, *, #26088, .F. ) ;
#88388=DIRECTION ( 'NONE',  ( -0.000000000000000000, 1.000000000000000000, 3.491481338843133355E-15 ) ) ;
#88389=VECTOR ( 'NONE', #59260, 999.9999999999998863 ) ;
#88390=ADVANCED_FACE ( 'NONE', ( #85702 ), #2817, .F. ) ;
#88391=DIRECTION ( 'NONE',  ( -0.000000000000000000, -0.9848077530122086864, -0.1736481776669273613 ) ) ;
#88392=CARTESIAN_POINT ( 'NONE',  ( 18.22301284409339672, -12.38742843783360748, 31.66772728687926985 ) ) ;
#88393=VERTEX_POINT ( 'NONE', #58656 ) ;
#88394=CARTESIAN_POINT ( 'NONE',  ( -17.07692307692307665, -5.180354513474913603, 36.12317359536750416 ) ) ;
#88397=AXIS2_PLACEMENT_3D ( 'NONE', #11701, #80611, #18895 ) ;
#88398=ORIENTED_EDGE ( 'NONE', *, *, #59680, .T. ) ;
#88399=CARTESIAN_POINT ( 'NONE',  ( -5.076923076923075762, -1.242168528481310874, 33.36296068462461051 ) ) ;
#88400=CARTESIAN_POINT ( 'NONE',  ( 11.53846153846141576, -2.657715359629662544, 31.77849191805970364 ) ) ;
#88402=EDGE_CURVE ( 'NONE', #53125, #67703, #50530, .T. ) ;
#88403=CARTESIAN_POINT ( 'NONE',  ( -13.38461538461538325, -3.050289026998446396, 32.03036669348365706 ) ) ;
#88404=CARTESIAN_POINT ( 'NONE',  ( -16.15384615384615330, -13.95598074871891292, 31.83374038241031911 ) ) ;
#88405=CARTESIAN_POINT ( 'NONE',  ( -8.519230769229348965, -7.500000000000154543, 35.00000000000007105 ) ) ;
#88406=CYLINDRICAL_SURFACE ( 'NONE', #26344, 0.2500000000000012212 ) ;
#88407=CARTESIAN_POINT ( 'NONE',  ( -0.7115152055870521686, -11.47974371597208076, 33.17467449705390692 ) ) ;
#88408=ORIENTED_EDGE ( 'NONE', *, *, #75639, .F. ) ;
#88409=CARTESIAN_POINT ( 'NONE',  ( -4.023320715612507037, -12.50538340440932217, 31.33453814440721885 ) ) ;
#88410=EDGE_LOOP ( 'NONE', ( #51392, #51066 ) ) ;
#88411=DIRECTION ( 'NONE',  ( -0.000000000000000000, 0.6427876096865404731, -0.7660444431189770143 ) ) ;
#88412=EDGE_CURVE ( 'NONE', #80088, #21493, #63241, .T. ) ;
#88413=DIRECTION ( 'NONE',  ( -0.000000000000000000, -0.9848077530122086864, -0.1736481776669273613 ) ) ;
#88414=CARTESIAN_POINT ( 'NONE',  ( 6.130525701763565927, -9.417988943895561960, 34.36773134775778260 ) ) ;
#88415=EDGE_CURVE ( 'NONE', #54661, #69076, #30309, .T. ) ;
#88416=DIRECTION ( 'NONE',  ( -0.000000000000000000, -0.7660444431189791237, -0.6427876096865379196 ) ) ;
#88417=CARTESIAN_POINT ( 'NONE',  ( -6.250023237292966272, -12.22074536777954989, 31.39888409691088356 ) ) ;
#88418=VERTEX_POINT ( 'NONE', #72173 ) ;
#88420=EDGE_LOOP ( 'NONE', ( #12532, #80161, #64361, #12212 ) ) ;
#88421=ORIENTED_EDGE ( 'NONE', *, *, #82425, .F. ) ;
#88422=ORIENTED_EDGE ( 'NONE', *, *, #54590, .T. ) ;
#88423=EDGE_CURVE ( 'NONE', #78424, #21486, #10487, .T. ) ;
#88424=CARTESIAN_POINT ( 'NONE',  ( -4.153846153846152411, -5.557115091759785130, 34.35708131394839171 ) ) ;
#88425=CARTESIAN_POINT ( 'NONE',  ( 16.37662582282421653, -10.97394488606063589, 33.68653795673696294 ) ) ;
#88426=CARTESIAN_POINT ( 'NONE',  ( 2.307692307692309264, -9.819645486525091727, 36.12317359536749706 ) ) ;
#88427=EDGE_CURVE ( 'NONE', #14549, #19715, #6528, .T. ) ;
#88428=CARTESIAN_POINT ( 'NONE',  ( -8.069638770718176701, -3.562934362175800285, 33.22335522853832401 ) ) ;
#88429=DIRECTION ( 'NONE',  ( -0.000000000000000000, -0.000000000000000000, -1.000000000000000000 ) ) ;
#88430=DIRECTION ( 'NONE',  ( 0.000000000000000000, 1.000000000000000000, 0.000000000000000000 ) ) ;
#88431=CARTESIAN_POINT ( 'NONE',  ( 10.61538461538461675, -13.57706302396349152, 30.56769352161908060 ) ) ;
#88432=CARTESIAN_POINT ( 'NONE',  ( -5.076923076923075762, -11.35647404775217417, 33.31231777344666511 ) ) ;
#88433=ORIENTED_EDGE ( 'NONE', *, *, #71127, .T. ) ;
#88434=ORIENTED_EDGE ( 'NONE', *, *, #13640, .T. ) ;
#88435=B_SPLINE_CURVE_WITH_KNOTS ( 'NONE', 3,
 ( #83788, #22073, #27501, #82896, #34251, #47768, #13540, #41019, #76122, #36037 ),
 .UNSPECIFIED., .F., .F.,
 ( 4, 2, 2, 2, 4 ),
 ( 0.0007817359430256308733, 0.0009771253907249971907, 0.001172514838424363725, 0.001367904286123730259, 0.001563293733823096577 ),
 .UNSPECIFIED. ) ;
#88436=B_SPLINE_CURVE_WITH_KNOTS ( 'NONE', 3,
 ( #69476, #1903, #35702, #82570, #20408, #20843, #21282, #55074, #42017, #580 ),
 .UNSPECIFIED., .F., .F.,
 ( 4, 2, 2, 2, 4 ),
 ( 0.0007817359430256317406, 0.0009771253907249982749, 0.001172514838424365026, 0.001367904286123731560, 0.001563293733823098094 ),
 .UNSPECIFIED. ) ;
#88438=CARTESIAN_POINT ( 'NONE',  ( 2.057715576749954423, -2.564618984488975961, 30.55390908950641915 ) ) ;
#88439=EDGE_CURVE ( 'NONE', #68060, #33663, #61759, .T. ) ;
#88440=ORIENTED_EDGE ( 'NONE', *, *, #67323, .F. ) ;
#88441=CARTESIAN_POINT ( 'NONE',  ( -6.000000000000119904, -11.48612834414049644, 32.76840700105863391 ) ) ;
#88442=CARTESIAN_POINT ( 'NONE',  ( -9.942284436356281674, -4.075325502946081535, 33.72974371597206300 ) ) ;
#88443=B_SPLINE_CURVE_WITH_KNOTS ( 'NONE', 3,
 ( #47794, #75275, #13564, #30182, #37819, #44117, #1820, #23411, #16655, #36068 ),
 .UNSPECIFIED., .F., .F.,
 ( 4, 2, 2, 2, 4 ),
 ( 0.000000000000000000, 0.0001954339857564096157, 0.0003908679715128192313, 0.0005863019572692288470, 0.0007817359430256384627 ),
 .UNSPECIFIED. ) ;
#88444=CARTESIAN_POINT ( 'NONE',  ( -0.3962833220256232192, -2.379036618887895305, 30.90682066428159303 ) ) ;
#88445=CARTESIAN_POINT ( 'NONE',  ( -9.692307692307812417, -6.879047030192662504, 34.71129190930017927 ) ) ;
#88446=FACE_BOUND ( 'NONE', #37088, .T. ) ;
#88447=ORIENTED_EDGE ( 'NONE', *, *, #38823, .F. ) ;
#88448=ADVANCED_FACE ( 'NONE', ( #25773 ), #73966, .F. ) ;
#88449=CARTESIAN_POINT ( 'NONE',  ( -23.00000000000000000, -4.249999999999998224, 27.25000000000000000 ) ) ;
#88450=CARTESIAN_POINT ( 'NONE',  ( -3.230769230769229949, -6.386643153685126251, 34.62446782046654192 ) ) ;
#88451=ORIENTED_EDGE ( 'NONE', *, *, #69796, .F. ) ;
#88452=CARTESIAN_POINT ( 'NONE',  ( -8.639185606395990646, -2.504778602574660340, 29.97347330155780654 ) ) ;
#88453=ORIENTED_EDGE ( 'NONE', *, *, #50384, .F. ) ;
#88454=FACE_BOUND ( 'NONE', #22706, .T. ) ;
#88455=CARTESIAN_POINT ( 'NONE',  ( 7.780883400193069122, -11.94971097300153140, 32.03036669348370680 ) ) ;
#88456=AXIS2_PLACEMENT_3D ( 'NONE', #74829, #18990, #46457 ) ;
#88457=CARTESIAN_POINT ( 'NONE',  ( 18.06606835100243913, -4.786620604624113540, 33.94971097300155805 ) ) ;
#88458=ORIENTED_EDGE ( 'NONE', *, *, #57907, .F. ) ;
#88459=CARTESIAN_POINT ( 'NONE',  ( -12.39628289026243557, -8.613356846314928816, 34.62446782046653482 ) ) ;
#88460=CARTESIAN_POINT ( 'NONE',  ( -12.52680846209478460, -12.16647553114622049, 32.15551576947930812 ) ) ;
#88461=CARTESIAN_POINT ( 'NONE',  ( 1.134638653673033071, -3.137211980971221781, 32.19342716148376837 ) ) ;
#88462=VERTEX_POINT ( 'NONE', #75 ) ;
#88463=CARTESIAN_POINT ( 'NONE',  ( -4.153846153846152411, -13.87047571288749737, 32.06866353760679544 ) ) ;
#88464=CARTESIAN_POINT ( 'NONE',  ( 14.30769230769218581, -3.643525952248795718, 33.31231777344771672 ) ) ;
#88465=CARTESIAN_POINT ( 'NONE',  ( -3.296039676730005752, -2.892918686051582533, 31.69288490824015270 ) ) ;
#88466=EDGE_CURVE ( 'NONE', #33447, #68924, #17193, .T. ) ;
#88467=CARTESIAN_POINT ( 'NONE',  ( -18.00000000000012079, -12.70778746994576025, 30.41441678777401236 ) ) ;
#88468=ORIENTED_EDGE ( 'NONE', *, *, #20016, .T. ) ;
#88469=EDGE_CURVE ( 'NONE', #32972, #72998, #32521, .T. ) ;
#88470=CARTESIAN_POINT ( 'NONE',  ( -1.514762594053604250, -6.001485441113818986, 34.52039167877662607 ) ) ;
#88471=CARTESIAN_POINT ( 'NONE',  ( 2.372947447205146609, -3.643525952247864463, 33.31231777344670064 ) ) ;
#88472=VERTEX_POINT ( 'NONE', #33855 ) ;
#88473=CARTESIAN_POINT ( 'NONE',  ( 23.00000000000000000, -10.75000000000000000, 29.75000000000000355 ) ) ;
#88474=CARTESIAN_POINT ( 'NONE',  ( 9.561832507231976308, -7.276987145209184327, 34.99546412871779211 ) ) ;
#88475=CARTESIAN_POINT ( 'NONE',  ( 5.750023269057646935, -9.148715823498378086, 34.47080413974185120 ) ) ;
#88477=CARTESIAN_POINT ( 'NONE',  ( -6.856910316485284262, -7.250054591869668386, 34.99404684341514127 ) ) ;
#88478=CARTESIAN_POINT ( 'NONE',  ( 15.16549923021291058, -5.941354392334499579, 34.76329471203369792 ) ) ;
#88479=CARTESIAN_POINT ( 'NONE',  ( 6.066068351002441794, -11.69971097300155272, 32.46337939537588113 ) ) ;
#88480=CARTESIAN_POINT ( 'NONE',  ( -16.37677311275299985, -8.282780595021769443, 34.94152052738834158 ) ) ;
#88481=CYLINDRICAL_SURFACE ( 'NONE', #83829, 0.2499999999999998890 ) ;
#88483=ORIENTED_EDGE ( 'NONE', *, *, #19951, .T. ) ;
#88484=CARTESIAN_POINT ( 'NONE',  ( 4.946775107191380805, -6.809168938359898782, 34.95455904226513866 ) ) ;
#88485=VERTEX_POINT ( 'NONE', #39745 ) ;
#88486=B_SPLINE_CURVE_WITH_KNOTS ( 'NONE', 3,
 ( #18974, #19856, #81570, #20308, #81128, #47320, #87450, #74812, #32, #12218 ),
 .UNSPECIFIED., .F., .F.,
 ( 4, 2, 2, 2, 4 ),
 ( 0.000000000000000000, 0.0001954311584214072381, 0.0003908623168428144762, 0.0005862934752642217414, 0.0007817246336856289524 ),
 .UNSPECIFIED. ) ;
#88487=ORIENTED_EDGE ( 'NONE', *, *, #5655, .F. ) ;
#88488=CARTESIAN_POINT ( 'NONE',  ( 3.007284287045282944, -5.113361153441932316, 34.14387501736621999 ) ) ;
#88489=ORIENTED_EDGE ( 'NONE', *, *, #864, .T. ) ;
#88490=CARTESIAN_POINT ( 'NONE',  ( -4.219116154402471786, -2.657715359629089225, 31.77849191805834295 ) ) ;
#88492=CARTESIAN_POINT ( 'NONE',  ( 18.00000000000000000, -4.661471528628507777, 34.16647553114623292 ) ) ;
#88493=CARTESIAN_POINT ( 'NONE',  ( -8.899922235898330314, -3.062553014421049546, 32.05460306192773601 ) ) ;
#88495=VECTOR ( 'NONE', #81047, 1000.000000000000114 ) ;
#88496=CARTESIAN_POINT ( 'NONE',  ( -8.769230769230768274, -4.786620604624113540, 33.94971097300155094 ) ) ;
#88497=CARTESIAN_POINT ( 'NONE',  ( 9.692307692307570832, -12.51329471203414379, 31.30864560766407578 ) ) ;
#88498=CARTESIAN_POINT ( 'NONE',  ( -11.66860874789975888, -5.195881422630166391, 34.18770438780619259 ) ) ;
#88500=CARTESIAN_POINT ( 'NONE',  ( 17.20744851515672025, -2.372941743896878286, 30.88044141588253311 ) ) ;
#88502=DIRECTION ( 'NONE',  ( -0.000000000000000000, 0.1736481776669307198, -0.9848077530122080203 ) ) ;
#88504=ORIENTED_EDGE ( 'NONE', *, *, #63094, .T. ) ;
#88505=ORIENTED_EDGE ( 'NONE', *, *, #44718, .F. ) ;
#88506=CARTESIAN_POINT ( 'NONE',  ( -9.442253380669379581, -3.627508038966690496, 32.91356715214248396 ) ) ;
#88507=CARTESIAN_POINT ( 'NONE',  ( 15.36155967173618286, -11.93129842949671726, 32.56571108434900452 ) ) ;
#88508=DIRECTION ( 'NONE',  ( -0.000000000000000000, 0.7660444431189791237, -0.6427876096865379196 ) ) ;
#88509=DIRECTION ( 'NONE',  ( 0.000000000000000000, 1.000000000000000000, 0.000000000000000000 ) ) ;
#88511=CARTESIAN_POINT ( 'NONE',  ( -14.30769230769230660, -13.53365097954675988, 30.81389545987213552 ) ) ;
#88512=CARTESIAN_POINT ( 'NONE',  ( -6.066083410955879884, -8.120952969808774569, 34.71129190930000163 ) ) ;
#88513=EDGE_CURVE ( 'NONE', #77885, #25874, #54850, .T. ) ;
#88515=AXIS2_PLACEMENT_3D ( 'NONE', #67615, #54080, #81576 ) ;
#88516=ORIENTED_EDGE ( 'NONE', *, *, #77660, .T. ) ;
#88517=CARTESIAN_POINT ( 'NONE',  ( -4.854143535654666941, -12.44528174975671853, 30.48912976160716681 ) ) ;
#88519=EDGE_CURVE ( 'NONE', #40783, #16008, #26943, .T. ) ;
#88520=ORIENTED_EDGE ( 'NONE', *, *, #55268, .F. ) ;
#88521=CARTESIAN_POINT ( 'NONE',  ( -6.923076923076922462, -9.905515769479276145, 34.41647553114623292 ) ) ;
#88522=CARTESIAN_POINT ( 'NONE',  ( 4.088575707885377497, -2.625532179533445198, 30.86335684631481513 ) ) ;
#88523=EDGE_CURVE ( 'NONE', #15864, #64392, #41947, .T. ) ;
#88524=CARTESIAN_POINT ( 'NONE',  ( -0.3962828902624371818, -6.879047030191285828, 34.71129190930002295 ) ) ;
#88526=DIRECTION ( 'NONE',  ( 0.000000000000000000, 0.9848077530122072432, 0.1736481776669354937 ) ) ;
#88527=CARTESIAN_POINT ( 'NONE',  ( 5.934729554039225974, -2.892918686051582089, 31.69288490824015270 ) ) ;
#88528=ORIENTED_EDGE ( 'NONE', *, *, #84922, .F. ) ;
#88529=EDGE_CURVE ( 'NONE', #78341, #572, #5414, .T. ) ;
#88530=EDGE_LOOP ( 'NONE', ( #55188, #39973, #19832, #8238 ) ) ;
#88532=ORIENTED_EDGE ( 'NONE', *, *, #3160, .T. ) ;
#88533=CARTESIAN_POINT ( 'NONE',  ( 18.22301284409340028, -2.308499170217968022, 30.53291367094874076 ) ) ;
#88534=CARTESIAN_POINT ( 'NONE',  ( -2.437840277424001112, -10.31621877034669588, 34.18098118002070152 ) ) ;
#88535=EDGE_CURVE ( 'NONE', #35664, #62627, #78721, .T. ) ;
#88537=CARTESIAN_POINT ( 'NONE',  ( 16.37685750545900376, -9.886259254753566594, 34.14407573483972413 ) ) ;
#88538=CARTESIAN_POINT ( 'NONE',  ( -15.09997878980228059, -9.084667340241226796, 34.75534355489798344 ) ) ;
#88539=EDGE_CURVE ( 'NONE', #16148, #53666, #85926, .T. ) ;
#88540=CARTESIAN_POINT ( 'NONE',  ( -10.54931626438217762, -12.10708131394839882, 31.69288490824020954 ) ) ;
#88541=ORIENTED_EDGE ( 'NONE', *, *, #9648, .T. ) ;
#88542=ORIENTED_EDGE ( 'NONE', *, *, #52924, .T. ) ;
#88543=CIRCLE ( 'NONE', #65553, 0.2500000000000002220 ) ;
#88544=ORIENTED_EDGE ( 'NONE', *, *, #41888, .T. ) ;
#88545=DIRECTION ( 'NONE',  ( 0.000000000000000000, 0.6427876096865368094, 0.7660444431189802339 ) ) ;
#88546=VERTEX_POINT ( 'NONE', #23760 ) ;
#88547=CARTESIAN_POINT ( 'NONE',  ( 9.442284468086239002, -8.475808217655753651, 34.90892951860618609 ) ) ;
#88548=CARTESIAN_POINT ( 'NONE',  ( -2.307692307692427391, -9.442884908241554243, 34.35708131394783038 ) ) ;
#88552=EDGE_CURVE ( 'NONE', #18924, #38366, #14020, .T. ) ;
#88553=CARTESIAN_POINT ( 'NONE',  ( -1.253824943648431889, -11.37503395064541678, 33.29242100308974983 ) ) ;
#88554=VERTEX_POINT ( 'NONE', #34743 ) ;
#88555=DIRECTION ( 'NONE',  ( -0.000000000000000000, -0.1736481776669307198, -0.9848077530122080203 ) ) ;
#88556=B_SPLINE_CURVE_WITH_KNOTS ( 'NONE', 3,
 ( #71370, #56094, #29517, #76361, #8804, #76818, #28172, #50656, #83588, #43908 ),
 .UNSPECIFIED., .F., .F.,
 ( 4, 2, 2, 2, 4 ),
 ( 0.000000000000000000, 0.0001954311564186864949, 0.0003908623128373729899, 0.0005862934692560594577, 0.0007817246256747459798 ),
 .UNSPECIFIED. ) ;
#88557=FACE_BOUND ( 'NONE', #31088, .T. ) ;
#88558=CARTESIAN_POINT ( 'NONE',  ( -6.923076923077044142, -3.835265460704628371, 33.15142922262033665 ) ) ;
#88559=DIRECTION ( 'NONE',  ( 0.000000000000000000, 0.7660444431189822323, -0.6427876096865344779 ) ) ;
#88560=ORIENTED_EDGE ( 'NONE', *, *, #10389, .T. ) ;
#88563=CARTESIAN_POINT ( 'NONE',  ( -17.01166793741023042, -12.70778746994558439, 30.41441678777537305 ) ) ;
#88564=DIRECTION ( 'NONE',  ( 0.000000000000000000, 0.4999999999999960032, -0.8660254037844410391 ) ) ;
#88565=EDGE_CURVE ( 'NONE', #7242, #3517, #22621, .T. ) ;
#88566=VERTEX_POINT ( 'NONE', #51213 ) ;
#88567=B_SPLINE_CURVE_WITH_KNOTS ( 'NONE', 3,
 ( #47917, #63198, #61868, #83047, #74968, #62749, #41172, #48358, #7389, #88938 ),
 .UNSPECIFIED., .F., .F.,
 ( 4, 2, 2, 2, 4 ),
 ( 0.0007817359430256320659, 0.0009771253907249987086, 0.001172514838424365460, 0.001367904286123731994, 0.001563293733823098745 ),
 .UNSPECIFIED. ) ;
#88568=CARTESIAN_POINT ( 'NONE',  ( -9.561517251340744039, -4.684288915650983043, 34.18129842949671371 ) ) ;
#88569=CARTESIAN_POINT ( 'NONE',  ( -5.776987155906604166, -4.026326845037961455, 33.68677907613344047 ) ) ;
#88570=CARTESIAN_POINT ( 'NONE',  ( 17.29993442853592711, -9.886259254753566594, 34.14407573483972413 ) ) ;
#88571=CYLINDRICAL_SURFACE ( 'NONE', #15538, 0.2500000000000004996 ) ;
#88572=EDGE_CURVE ( 'NONE', #6380, #8424, #36516, .T. ) ;
#88573=DIRECTION ( 'NONE',  ( 0.000000000000000000, 0.8660254037844377084, 0.5000000000000015543 ) ) ;
#88574=EDGE_CURVE ( 'NONE', #31074, #8026, #76171, .T. ) ;
#88575=VECTOR ( 'NONE', #78200, 1000.000000000000227 ) ;
#88576=FACE_BOUND ( 'NONE', #12556, .T. ) ;
#88577=CARTESIAN_POINT ( 'NONE',  ( 5.777073041093149897, -4.762599654559228846, 34.23009711892697737 ) ) ;
#88578=LINE ( 'NONE', #81802, #63230 ) ;
#88579=B_SPLINE_CURVE_WITH_KNOTS ( 'NONE', 3,
 ( #38864, #25342, #4627, #68434, #22023, #69330, #15270, #27896, #55801, #76527 ),
 .UNSPECIFIED., .F., .F.,
 ( 4, 2, 2, 2, 4 ),
 ( 0.000000000000000000, 0.0001954311564186861697, 0.0003908623128373723394, 0.0005862934692560584820, 0.0007817246256747446788 ),
 .UNSPECIFIED. ) ;
#88580=CARTESIAN_POINT ( 'NONE',  ( 10.61538461538461675, -2.486705287966279876, 31.30864560766543647 ) ) ;
#88581=CARTESIAN_POINT ( 'NONE',  ( -18.25000000000000000, -2.499999999999999556, 29.75000000000000355 ) ) ;
#88582=CARTESIAN_POINT ( 'NONE',  ( -2.177166869458662557, -8.630441415882550871, 34.87705825610312615 ) ) ;
#88583=CARTESIAN_POINT ( 'NONE',  ( 15.23076923076923173, -8.120952969808772792, 34.71129190930000163 ) ) ;
#88586=EDGE_LOOP ( 'NONE', ( #1156, #73984 ) ) ;
#88588=VERTEX_POINT ( 'NONE', #1846 ) ;
#88589=CARTESIAN_POINT ( 'NONE',  ( -39.05038313613820122, -2.499999999999999556, 29.75000000000000355 ) ) ;
#88590=VERTEX_POINT ( 'NONE', #30529 ) ;
#88591=CARTESIAN_POINT ( 'NONE',  ( -11.53846153846153655, -6.343179335718451384, 34.87096338111211935 ) ) ;
#88592=CARTESIAN_POINT ( 'NONE',  ( 4.153846153846154188, -1.629998284177014645, 34.34916445242399163 ) ) ;
#88593=CARTESIAN_POINT ( 'NONE',  ( 15.16551824060798914, -2.506253911140460922, 30.00000000000013856 ) ) ;
#88594=VECTOR ( 'NONE', #54396, 1000.000000000000227 ) ;
#88595=VERTEX_POINT ( 'NONE', #85481 ) ;
#88596=CARTESIAN_POINT ( 'NONE',  ( -16.82686865700962642, -2.318338780012836775, 30.59689888758630616 ) ) ;
#88597=CARTESIAN_POINT ( 'NONE',  ( 13.38461538461526423, -12.70778746994576025, 30.41441678777401236 ) ) ;
#88599=CARTESIAN_POINT ( 'NONE',  ( 14.17700084102475522, -10.54014554554150607, 33.71984207302941883 ) ) ;
#88600=CYLINDRICAL_SURFACE ( 'NONE', #82068, 0.2499999999999986955 ) ;
#88601=CARTESIAN_POINT ( 'NONE',  ( -5.010855743573000787, -11.91647553114624358, 32.58852847137148245 ) ) ;
#88602=CARTESIAN_POINT ( 'NONE',  ( 1.161688425708536476, -4.762599654559228846, 34.23009711892697737 ) ) ;
#88603=CARTESIAN_POINT ( 'NONE',  ( -1.161835715637317357, -6.717445702608402236, 34.94155399931962336 ) ) ;
#88604=LINE ( 'NONE', #43814, #56932 ) ;
#88606=LINE ( 'NONE', #61099, #306 ) ;
#88607=CARTESIAN_POINT ( 'NONE',  ( -8.835313148590904220, -2.833524468853757305, 32.15551576947924417 ) ) ;
#88609=CARTESIAN_POINT ( 'NONE',  ( 2.307692307692309264, -13.53365097954675988, 30.81389545987213552 ) ) ;
#88611=EDGE_CURVE ( 'NONE', #73491, #37061, #20046, .T. ) ;
#88612=CARTESIAN_POINT ( 'NONE',  ( 17.07692307692307665, -13.53365097954675988, 30.81389545987213552 ) ) ;
#88614=ORIENTED_EDGE ( 'NONE', *, *, #36357, .T. ) ;
#88615=CARTESIAN_POINT ( 'NONE',  ( 0.4615384615384611200, -3.322132147404559976, 32.92929555188717927 ) ) ;
#88617=CARTESIAN_POINT ( 'NONE',  ( 2.241608896736428491, -2.721908614388772296, 31.22303859784724622 ) ) ;
#88618=ORIENTED_EDGE ( 'NONE', *, *, #37501, .F. ) ;
#88619=CARTESIAN_POINT ( 'NONE',  ( -2.177644872441854673, -7.723484941389743952, 34.99544897038808955 ) ) ;
#88620=LINE ( 'NONE', #34533, #82347 ) ;
#88622=CARTESIAN_POINT ( 'NONE',  ( 17.07692307692307665, -3.886160181151819604, 36.00935417666054406 ) ) ;
#88623=ORIENTED_EDGE ( 'NONE', *, *, #48386, .F. ) ;
#88624=B_SPLINE_CURVE_WITH_KNOTS ( 'NONE', 3,
 ( #53481, #10730, #31442, #58905, #86413, #32336, #4409, #46289, #65217, #38195 ),
 .UNSPECIFIED., .F., .F.,
 ( 4, 2, 2, 2, 4 ),
 ( 0.0007817359430256283796, 0.0009771253907249941549, 0.001172514838424359822, 0.001367904286123725489, 0.001563293733823091156 ),
 .UNSPECIFIED. ) ;
#88625=CARTESIAN_POINT ( 'NONE',  ( -9.627052552794857831, -2.657715359629131857, 31.77849191805844242 ) ) ;
#88626=CARTESIAN_POINT ( 'NONE',  ( -15.29603923132554932, -11.67786785259540849, 32.92929555188721480 ) ) ;
#88627=CARTESIAN_POINT ( 'NONE',  ( 8.769230769230645706, -3.643525952248795718, 33.31231777344771672 ) ) ;
#88629=VERTEX_POINT ( 'NONE', #44922 ) ;
#88630=VERTEX_POINT ( 'NONE', #80054 ) ;
#88631=VERTEX_POINT ( 'NONE', #4845 ) ;
#88632=CARTESIAN_POINT ( 'NONE',  ( 0.3313912521002396194, -8.587444163452046197, 34.63053765926554206 ) ) ;
#88633=CARTESIAN_POINT ( 'NONE',  ( 0.3962680155776845403, -2.625532179533445198, 30.86335684631481513 ) ) ;
#88634=CARTESIAN_POINT ( 'NONE',  ( -11.28840711854808632, -3.435999193479609914, 33.07426656108010832 ) ) ;
#88635=CARTESIAN_POINT ( 'NONE',  ( -15.48076923076922995, -7.500000000000001776, 34.75000000000000000 ) ) ;
#88636=EDGE_CURVE ( 'NONE', #83936, #68109, #38750, .T. ) ;
#88637=CARTESIAN_POINT ( 'NONE',  ( 15.90382291655318880, -5.056417327199097755, 34.11270091957320716 ) ) ;
#88638=ORIENTED_EDGE ( 'NONE', *, *, #80924, .F. ) ;
#88639=AXIS2_PLACEMENT_3D ( 'NONE', #66039, #79125, #5240 ) ;
#88640=ORIENTED_EDGE ( 'NONE', *, *, #82879, .F. ) ;
#88642=CARTESIAN_POINT ( 'NONE',  ( -3.230769230768923084, -2.506253911140615021, 30.00000000000323297 ) ) ;
#88643=ORIENTED_EDGE ( 'NONE', *, *, #62537, .F. ) ;
#88644=LINE ( 'NONE', #20592, #60346 ) ;
#88646=CARTESIAN_POINT ( 'NONE',  ( 6.923076923076800782, -5.094484230521993062, 34.41647553114689373 ) ) ;
#88648=CARTESIAN_POINT ( 'NONE',  ( 7.846153846153846700, -4.945431358278436385, 36.03766855953609394 ) ) ;
#88649=AXIS2_PLACEMENT_3D ( 'NONE', #55291, #76008, #68366 ) ;
#88651=ORIENTED_EDGE ( 'NONE', *, *, #66071, .F. ) ;
#88652=VERTEX_POINT ( 'NONE', #5285 ) ;
#88653=CARTESIAN_POINT ( 'NONE',  ( 14.53047197667037338, -10.97394488606064122, 33.68653795673694873 ) ) ;
#88654=FACE_OUTER_BOUND ( 'NONE', #6353, .T. ) ;
#88656=CARTESIAN_POINT ( 'NONE',  ( -11.28840711854808632, -12.65882529074907126, 30.72640787790839312 ) ) ;
#88657=CARTESIAN_POINT ( 'NONE',  ( -17.32694630114453105, -3.520140089381496473, 33.17453946501458262 ) ) ;
#88658=EDGE_LOOP ( 'NONE', ( #8665, #11188, #21680, #21215 ) ) ;
#88659=EDGE_CURVE ( 'NONE', #84061, #52397, #45818, .T. ) ;
#88660=FACE_OUTER_BOUND ( 'NONE', #68967, .T. ) ;
#88661=CARTESIAN_POINT ( 'NONE',  ( 16.21910172512217585, -3.835265460703683349, 33.15142922261929925 ) ) ;
#88662=LINE ( 'NONE', #26939, #88594 ) ;
#88663=FACE_BOUND ( 'NONE', #22034, .T. ) ;
#88664=CARTESIAN_POINT ( 'NONE',  ( -17.86920819217521483, -8.147973898785416225, 34.70805048591653730 ) ) ;
#88665=DIRECTION ( 'NONE',  ( 0.000000000000000000, 0.7660444431189822323, -0.6427876096865344779 ) ) ;
#88666=LINE ( 'NONE', #83672, #37966 ) ;
#88669=CARTESIAN_POINT ( 'NONE',  ( 6.923076923076924238, -1.509761064869970415, 31.06009739812519044 ) ) ;
#88670=CARTESIAN_POINT ( 'NONE',  ( -0.6850234052624116776, -3.754499324213721234, 33.06261337010820256 ) ) ;
#88671=ORIENTED_EDGE ( 'NONE', *, *, #40883, .T. ) ;
#88672=CARTESIAN_POINT ( 'NONE',  ( -16.15384615384615330, -6.343179335718451384, 34.87096338111211935 ) ) ;
#88675=VECTOR ( 'NONE', #63325, 1000.000000000000114 ) ;
#88676=CARTESIAN_POINT ( 'NONE',  ( -14.37296275365308418, -5.219633306516282545, 34.19971097300152962 ) ) ;
#88678=CARTESIAN_POINT ( 'NONE',  ( -12.46153846153846168, -4.786620604624113540, 33.94971097300155094 ) ) ;
#88679=ORIENTED_EDGE ( 'NONE', *, *, #29541, .T. ) ;
#88680=CYLINDRICAL_SURFACE ( 'NONE', #5452, 0.2499999999999994726 ) ;
#88681=EDGE_CURVE ( 'NONE', #37333, #75827, #74188, .T. ) ;
#88682=EDGE_CURVE ( 'NONE', #85803, #76443, #82777, .T. ) ;
#88683=CARTESIAN_POINT ( 'NONE',  ( -14.98082382139119062, -12.68172785388650681, 30.59649109432439218 ) ) ;
#88684=FACE_BOUND ( 'NONE', #13837, .T. ) ;
#88685=CARTESIAN_POINT ( 'NONE',  ( 17.07692307692295586, -5.941354392335915335, 34.76329471203413846 ) ) ;
#88686=DIRECTION ( 'NONE',  ( -0.000000000000000000, 0.9396926207859093161, -0.3420201433256663259 ) ) ;
#88687=CARTESIAN_POINT ( 'NONE',  ( 2.057715563643717882, -6.524016743844655686, 34.90889640711025521 ) ) ;
#88688=CYLINDRICAL_SURFACE ( 'NONE', #76978, 0.2499999999999986955 ) ;
#88690=CARTESIAN_POINT ( 'NONE',  ( 2.084765348785460048, -10.77366814457252175, 33.85459836347579454 ) ) ;
#88692=VERTEX_POINT ( 'NONE', #32752 ) ;
#88693=ORIENTED_EDGE ( 'NONE', *, *, #35952, .T. ) ;
#88694=CARTESIAN_POINT ( 'NONE',  ( -12.46153846153846168, -5.471508081941601098, 34.59228464037088457 ) ) ;
#88695=CARTESIAN_POINT ( 'NONE',  ( 7.145856464345333059, -12.24180327182771855, 31.33663988360758168 ) ) ;
#88696=DIRECTION ( 'NONE',  ( 0.000000000000000000, 0.9396926207859126468, 0.3420201433256571111 ) ) ;
#88697=FACE_OUTER_BOUND ( 'NONE', #15470, .T. ) ;
#88698=CARTESIAN_POINT ( 'NONE',  ( 10.61538461538461675, -12.10708131394839349, 31.69288490824020244 ) ) ;
#88701=DIRECTION ( 'NONE',  ( -0.000000000000000000, 0.3420201433256694346, -0.9396926207859080948 ) ) ;
#88702=CARTESIAN_POINT ( 'NONE',  ( 17.86985203026830504, -4.299443229763728169, 33.91186481527756058 ) ) ;
#88703=CARTESIAN_POINT ( 'NONE',  ( -1.515225039819465769, -7.722926974430166069, 34.99546784045485737 ) ) ;
#88704=CARTESIAN_POINT ( 'NONE',  ( -9.915792636031637741, -11.41268669641500466, 32.86336882939237825 ) ) ;
#88705=CARTESIAN_POINT ( 'NONE',  ( 13.60762822870878530, -2.523321265292115534, 31.42251411153756990 ) ) ;
#88706=CARTESIAN_POINT ( 'NONE',  ( -3.453696189676080053, -10.01117774369187252, 34.36070679894347535 ) ) ;
#88708=CARTESIAN_POINT ( 'NONE',  ( -8.546451100252703270, -11.60474049983371003, 33.02348890104160262 ) ) ;
#88709=CARTESIAN_POINT ( 'NONE',  ( -12.71153846153846345, -2.499999999999999556, 29.81609845454691765 ) ) ;
#88710=ORIENTED_EDGE ( 'NONE', *, *, #4095, .T. ) ;
#88711=CARTESIAN_POINT ( 'NONE',  ( 3.230769230769231726, -1.629998284177014645, 34.34916445242399163 ) ) ;
#88713=B_SPLINE_CURVE_WITH_KNOTS ( 'NONE', 3,
 ( #821, #14336, #55317, #56651, #62945, #34611, #48551, #49008, #387, #49886 ),
 .UNSPECIFIED., .F., .F.,
 ( 4, 2, 2, 2, 4 ),
 ( 0.000000000000000000, 0.0001954311564186876063, 0.0003908623128373752125, 0.0005862934692560628188, 0.0007817246256747504250 ),
 .UNSPECIFIED. ) ;
#88715=B_SPLINE_CURVE_WITH_KNOTS ( 'NONE', 3,
 ( #60407, #21979, #76028, #49451, #76923, #55311, #87925, #14331, #63396, #15227 ),
 .UNSPECIFIED., .F., .F.,
 ( 4, 2, 2, 2, 4 ),
 ( 0.0007817359430256285964, 0.0009771253907249941549, 0.001172514838424359822, 0.001367904286123725489, 0.001563293733823090939 ),
 .UNSPECIFIED. ) ;
#88717=CARTESIAN_POINT ( 'NONE',  ( -17.93474442872397034, -10.90142922261932235, 33.41473453929630466 ) ) ;
#88719=CARTESIAN_POINT ( 'NONE',  ( -9.627052121031665521, -5.219633306516380244, 34.19971097300157936 ) ) ;
#88720=EDGE_LOOP ( 'NONE', ( #81446, #4982 ) ) ;
#88722=CARTESIAN_POINT ( 'NONE',  ( -14.53061926659915315, -5.582147617184174848, 34.63737895849758530 ) ) ;
#88724=CARTESIAN_POINT ( 'NONE',  ( 8.638539302563209787, -8.147922237126337563, 34.70805685702651999 ) ) ;
#88725=DIRECTION ( 'NONE',  ( -0.000000000000000000, -0.7660444431189791237, -0.6427876096865379196 ) ) ;
#88726=ORIENTED_EDGE ( 'NONE', *, *, #61757, .T. ) ;
#88727=CARTESIAN_POINT ( 'NONE',  ( 7.780070435197965040, -4.098570777380720287, 33.41473453929634729 ) ) ;
#88728=CARTESIAN_POINT ( 'NONE',  ( -7.846153846153844924, -2.538708090699994813, 30.37095296980875503 ) ) ;
#88731=EDGE_LOOP ( 'NONE', ( #87742, #58571, #7541, #46225 ) ) ;
#88732=ORIENTED_EDGE ( 'NONE', *, *, #63108, .T. ) ;
#88733=CARTESIAN_POINT ( 'NONE',  ( -17.77722033102192967, -4.989023458446560255, 34.36081565061822118 ) ) ;
#88734=CARTESIAN_POINT ( 'NONE',  ( 18.00000000000000000, -4.098570777380720287, 33.41473453929634729 ) ) ;
#88735=FACE_OUTER_BOUND ( 'NONE', #44185, .T. ) ;
#88736=DIRECTION ( 'NONE',  ( -0.000000000000000000, -0.8660254037844399289, -0.4999999999999980016 ) ) ;
#88738=CARTESIAN_POINT ( 'NONE',  ( -4.283993363284373856, -6.852621066184267029, 34.70813303252209181 ) ) ;
#88740=AXIS2_PLACEMENT_3D ( 'NONE', #45500, #38308, #72087 ) ;
#88742=DIRECTION ( 'NONE',  ( -0.000000000000000000, -0.7660444431189791237, -0.6427876096865379196 ) ) ;
#88744=B_SPLINE_CURVE_WITH_KNOTS ( 'NONE', 3,
 ( #14565, #69507, #7813, #35280, #62738, #1054, #83483, #74496, #12793, #60975 ),
 .UNSPECIFIED., .F., .F.,
 ( 4, 2, 2, 2, 4 ),
 ( 0.0007817359430256296806, 0.0009771253907249958896, 0.001172514838424361990, 0.001367904286123728091, 0.001563293733823094408 ),
 .UNSPECIFIED. ) ;
#88745=ORIENTED_EDGE ( 'NONE', *, *, #39952, .F. ) ;
#88747=ORIENTED_EDGE ( 'NONE', *, *, #2709, .F. ) ;
#88748=DIRECTION ( 'NONE',  ( -0.000000000000000000, 1.000000000000000000, 3.491481338843133355E-15 ) ) ;
#88749=ORIENTED_EDGE ( 'NONE', *, *, #79750, .F. ) ;
#88750=B_SPLINE_CURVE_WITH_KNOTS ( 'NONE', 3,
 ( #26985, #88266, #81936, #59871, #81493, #60759, #18892, #11246, #26542, #54001 ),
 .UNSPECIFIED., .F., .F.,
 ( 4, 2, 2, 2, 4 ),
 ( 0.000000000000000000, 0.0001954339857564126514, 0.0003908679715128183098, 0.0005863019572692239681, 0.0007817359430256294638 ),
 .UNSPECIFIED. ) ;
#88751=ADVANCED_FACE ( 'NONE', ( #10710 ), #3934, .F. ) ;
#88752=CARTESIAN_POINT ( 'NONE',  ( 11.76124120743959978, -3.563462043263030399, 33.22394488606062879 ) ) ;
#88753=DIRECTION ( 'NONE',  ( -0.000000000000000000, -0.9396926207859093161, -0.3420201433256663259 ) ) ;
#88754=EDGE_CURVE ( 'NONE', #48201, #4579, #38174, .T. ) ;
#88755=ORIENTED_EDGE ( 'NONE', *, *, #54616, .T. ) ;
#88756=CARTESIAN_POINT ( 'NONE',  ( -12.46153846153846168, -11.35647404775217417, 33.31231777344666511 ) ) ;
#88757=ORIENTED_EDGE ( 'NONE', *, *, #52998, .F. ) ;
#88758=CARTESIAN_POINT ( 'NONE',  ( 17.20771351789002424, -9.084667340241228572, 34.75534355489798344 ) ) ;
#88759=ORIENTED_EDGE ( 'NONE', *, *, #8745, .F. ) ;
#88762=VERTEX_POINT ( 'NONE', #86390 ) ;
#88765=CARTESIAN_POINT ( 'NONE',  ( -4.376773112753000738, -6.459968553980839800, 34.89616026154728701 ) ) ;
#88767=FACE_BOUND ( 'NONE', #41370, .T. ) ;
#88768=DIRECTION ( 'NONE',  ( 0.000000000000000000, 0.9396926207859126468, 0.3420201433256571111 ) ) ;
#88769=DIRECTION ( 'NONE',  ( -0.000000000000000000, -0.8660254037844399289, -0.4999999999999980016 ) ) ;
#88770=CARTESIAN_POINT ( 'NONE',  ( 11.53846153846141576, -3.083524468854526912, 32.58852847137268327 ) ) ;
#88771=CARTESIAN_POINT ( 'NONE',  ( 1.134638640566795420, -12.41104346484419452, 31.60698883733904196 ) ) ;
#88772=CARTESIAN_POINT ( 'NONE',  ( 5.076923076923075762, -2.517432740324522911, 35.29906147534542527 ) ) ;
#88773=CARTESIAN_POINT ( 'NONE',  ( -7.846153846153967493, -9.528491918059723176, 34.59228464037033035 ) ) ;
#88775=FACE_OUTER_BOUND ( 'NONE', #64135, .T. ) ;
#88776=ORIENTED_EDGE ( 'NONE', *, *, #72873, .F. ) ;
#88777=EDGE_LOOP ( 'NONE', ( #68589, #61794 ) ) ;
#88778=B_SPLINE_CURVE_WITH_KNOTS ( 'NONE', 3,
 ( #6436, #61352, #88868, #27139, #54599, #50930, #35224, #14966, #21712, #77981 ),
 .UNSPECIFIED., .F., .F.,
 ( 4, 2, 2, 2, 4 ),
 ( 0.0007817359430256282712, 0.0009771253907249945886, 0.001172514838424360689, 0.001367904286123726790, 0.001563293733823093107 ),
 .UNSPECIFIED. ) ;
#88779=CARTESIAN_POINT ( 'NONE',  ( 2.084207383127975710, -3.019605429927184836, 32.48692288466676814 ) ) ;
#88780=CARTESIAN_POINT ( 'NONE',  ( -18.24997674404858827, -10.06842814019191934, 34.32929386961144758 ) ) ;
#88781=B_SPLINE_CURVE_WITH_KNOTS ( 'NONE', 3,
 ( #20265, #41869, #7638, #6738, #68881, #7191 ),
 .UNSPECIFIED., .F., .F.,
 ( 4, 2, 4 ),
 ( 4.228332872216503527E-17, 0.0001954756301637175617, 0.0003909512603273928395 ),
 .UNSPECIFIED. ) ;
#88782=CARTESIAN_POINT ( 'NONE',  ( 16.15384615384615330, -11.35647404775217417, 33.31231777344666511 ) ) ;
#88783=CARTESIAN_POINT ( 'NONE',  ( -4.153846153846274980, -9.528491918059723176, 34.59228464037033035 ) ) ;
#88785=CARTESIAN_POINT ( 'NONE',  ( 5.750000000000002665, -2.249999999999998668, 29.75000000000000355 ) ) ;
#88787=EDGE_CURVE ( 'NONE', #922, #43893, #45108, .T. ) ;
#88788=CARTESIAN_POINT ( 'NONE',  ( -11.66915300512910214, -12.11776431015576172, 31.66791131148498906 ) ) ;
#88789=CARTESIAN_POINT ( 'NONE',  ( 11.78846153846147438, -7.565270445406050648, 34.75000000000000000 ) ) ;
#88790=CARTESIAN_POINT ( 'NONE',  ( -3.454254155333562171, -11.60425143139329940, 33.02411095842164457 ) ) ;
#88793=ORIENTED_EDGE ( 'NONE', *, *, #20575, .F. ) ;
#88794=ORIENTED_EDGE ( 'NONE', *, *, #67465, .T. ) ;
#88795=ORIENTED_EDGE ( 'NONE', *, *, #64036, .T. ) ;
#88796=EDGE_CURVE ( 'NONE', #10299, #61398, #56913, .T. ) ;
#88798=DIRECTION ( 'NONE',  ( 0.000000000000000000, 0.6427876096865368094, 0.7660444431189802339 ) ) ;
#88799=EDGE_CURVE ( 'NONE', #51788, #53046, #16078, .T. ) ;
#88800=EDGE_LOOP ( 'NONE', ( #69871, #12858, #5754, #63162 ) ) ;
#88801=DIRECTION ( 'NONE',  ( -0.000000000000000000, -0.000000000000000000, -1.000000000000000000 ) ) ;
#88802=LINE ( 'NONE', #47788, #64414 ) ;
#88804=CARTESIAN_POINT ( 'NONE',  ( 14.05769230769230838, -7.433931650972300353, 34.75000000000000711 ) ) ;
#88805=FACE_OUTER_BOUND ( 'NONE', #56313, .T. ) ;
#88806=EDGE_LOOP ( 'NONE', ( #56813, #65314 ) ) ;
#88807=CARTESIAN_POINT ( 'NONE',  ( 11.28846153846153655, -2.499999999999999556, 29.81609845454691765 ) ) ;
#88808=CARTESIAN_POINT ( 'NONE',  ( -13.13456107297706588, -4.235687564193447052, 33.53795663066793509 ) ) ;
#88809=EDGE_LOOP ( 'NONE', ( #79157, #84748 ) ) ;
#88810=CARTESIAN_POINT ( 'NONE',  ( 18.00000000000000000, -9.584722331328613620, 36.20867863119891439 ) ) ;
#88811=CARTESIAN_POINT ( 'NONE',  ( -3.007989561791164945, -2.612705202774697533, 31.66806509827799943 ) ) ;
#88812=CARTESIAN_POINT ( 'NONE',  ( 1.608042346476957318, -7.630147231320743018, 34.74852402298682819 ) ) ;
#88813=CARTESIAN_POINT ( 'NONE',  ( 11.53846153846141576, -10.33852847137269571, 34.16647553114546554 ) ) ;
#88814=CARTESIAN_POINT ( 'NONE',  ( 22.75000000000000000, -2.249999999999999556, 27.25000000000000000 ) ) ;
#88815=CARTESIAN_POINT ( 'NONE',  ( -8.703163435880695076, -9.058645607665452459, 34.76329471203371924 ) ) ;
#88816=CARTESIAN_POINT ( 'NONE',  ( -0.6844654204453096691, -2.523278758544489353, 31.42238647778637528 ) ) ;
#88818=EDGE_LOOP ( 'NONE', ( #39549, #18526, #64664, #82294, #66413, #68864 ) ) ;
#88819=CARTESIAN_POINT ( 'NONE',  ( 15.23076923076923173, -8.120952969808772792, 34.71129190930000163 ) ) ;
#88820=CARTESIAN_POINT ( 'NONE',  ( 1.161130460051056579, -9.417330523894424488, 34.63758898049880486 ) ) ;
#88821=B_SPLINE_CURVE_WITH_KNOTS ( 'NONE', 3,
 ( #45265, #72737, #13267, #66438, #19140, #46611, #87175, #32648, #81735, #25000 ),
 .UNSPECIFIED., .F., .F.,
 ( 4, 2, 2, 2, 4 ),
 ( 0.0007817359430256297891, 0.0009771253907249961065, 0.001172514838424362424, 0.001367904286123728741, 0.001563293733823095059 ),
 .UNSPECIFIED. ) ;
#88822=FACE_OUTER_BOUND ( 'NONE', #57360, .T. ) ;
#88823=ORIENTED_EDGE ( 'NONE', *, *, #72427, .F. ) ;
#88824=ORIENTED_EDGE ( 'NONE', *, *, #65055, .F. ) ;
#88825=CARTESIAN_POINT ( 'NONE',  ( -16.40384615384615330, -7.500000000000001776, 34.75000000000000000 ) ) ;
#88826=CARTESIAN_POINT ( 'NONE',  ( -5.326899807865431491, -6.567427716900047230, 34.66269422305636283 ) ) ;
#88827=CARTESIAN_POINT ( 'NONE',  ( -10.86540783960607293, -2.341070481393819236, 30.72580821765574299 ) ) ;
#88828=CARTESIAN_POINT ( 'NONE',  ( -2.307692307692305711, -13.53365097954675988, 30.81389545987213552 ) ) ;
#88831=ADVANCED_FACE ( 'NONE', ( #69638 ), #34529, .F. ) ;
#88833=CARTESIAN_POINT ( 'NONE',  ( -12.46153846153846168, -8.973038597847269315, 34.52809138561121927 ) ) ;
#88834=DIRECTION ( 'NONE',  ( -0.000000000000000000, -0.3420201433256694901, -0.9396926207859082059 ) ) ;
#88835=CARTESIAN_POINT ( 'NONE',  ( 7.780070435197965040, -9.780366693483667717, 34.19971097300155805 ) ) ;
#88836=EDGE_LOOP ( 'NONE', ( #75119, #68939, #84877, #5907 ) ) ;
#88837=DIRECTION ( 'NONE',  ( 0.000000000000000000, 0.9396926207859126468, -0.3420201433256571111 ) ) ;
#88838=VECTOR ( 'NONE', #56916, 1000.000000000000227 ) ;
#88842=CARTESIAN_POINT ( 'NONE',  ( -5.869209559033048862, -11.93129842949671726, 32.56571108434900452 ) ) ;
#88843=EDGE_LOOP ( 'NONE', ( #53451, #84344 ) ) ;
#88844=AXIS2_PLACEMENT_3D ( 'NONE', #26218, #81173, #40191 ) ;
#88845=CARTESIAN_POINT ( 'NONE',  ( 10.61538461538449418, -11.67786785259630911, 32.92929555188603530 ) ) ;
#88846=CARTESIAN_POINT ( 'NONE',  ( -14.55769230769231370, -2.249999999999999556, 29.81609741502490252 ) ) ;
#88847=CARTESIAN_POINT ( 'NONE',  ( -10.86536134632696715, -5.728515186090277211, 34.42611988154120439 ) ) ;
#88849=DIRECTION ( 'NONE',  ( -0.000000000000000000, 0.8660254037844397068, -0.4999999999999978906 ) ) ;
#88850=CARTESIAN_POINT ( 'NONE',  ( -0.5922290646487697874, -11.37499894934982514, 33.29245874905763003 ) ) ;
#88851=B_SPLINE_CURVE_WITH_KNOTS ( 'NONE', 3,
 ( #64112, #43849, #8305, #51023, #1983, #37083, #76761, #23576, #35781, #64547 ),
 .UNSPECIFIED., .F., .F.,
 ( 4, 2, 2, 2, 4 ),
 ( 0.000000000000000000, 0.0001954339857564099951, 0.0003908679715128199903, 0.0005863019572692300396, 0.0007817359430256399806 ),
 .UNSPECIFIED. ) ;
#88852=VERTEX_POINT ( 'NONE', #68315 ) ;
#88853=FACE_BOUND ( 'NONE', #44138, .T. ) ;
#88855=LINE ( 'NONE', #19922, #11243 ) ;
#88856=B_SPLINE_CURVE_WITH_KNOTS ( 'NONE', 3,
 ( #56634, #9341, #22403, #71031, #77785, #51171, #71464, #78226, #78676, #16974 ),
 .UNSPECIFIED., .F., .F.,
 ( 4, 2, 2, 2, 4 ),
 ( 0.0007817359430256294638, 0.0009771253907249974075, 0.001172514838424365460, 0.001367904286123733295, 0.001563293733823094191 ),
 .UNSPECIFIED. ) ;
#88857=EDGE_CURVE ( 'NONE', #53843, #2122, #84854, .T. ) ;
#88858=CARTESIAN_POINT ( 'NONE',  ( -18.25002322422145085, -10.92453946501459328, 33.72985991061849376 ) ) ;
#88859=CARTESIAN_POINT ( 'NONE',  ( -1.384615384615383471, -3.050289026998446396, 32.03036669348365706 ) ) ;
#88860=CARTESIAN_POINT ( 'NONE',  ( 14.55763771707035303, -8.476813868363244353, 34.90874843262270133 ) ) ;
#88861=EDGE_CURVE ( 'NONE', #2497, #6435, #28851, .T. ) ;
#88862=ORIENTED_EDGE ( 'NONE', *, *, #60852, .T. ) ;
#88863=ORIENTED_EDGE ( 'NONE', *, *, #1475, .T. ) ;
#88864=VERTEX_POINT ( 'NONE', #62864 ) ;
#88865=ORIENTED_EDGE ( 'NONE', *, *, #62675, .T. ) ;
#88868=CARTESIAN_POINT ( 'NONE',  ( -4.946397375159514276, -5.195472089885680766, 34.18748526763464923 ) ) ;
#88869=CARTESIAN_POINT ( 'NONE',  ( -11.66915214157184977, -5.496505350115501010, 34.60290016733514307 ) ) ;
#88870=DIRECTION ( 'NONE',  ( -0.000000000000000000, 0.5000000000000011102, -0.8660254037844380415 ) ) ;
#88871=CARTESIAN_POINT ( 'NONE',  ( 18.00000000000000000, -9.780366693483667717, 34.19971097300155094 ) ) ;
#88873=CARTESIAN_POINT ( 'NONE',  ( -2.530618525208453651, -4.887634598454295265, 34.01352882383564946 ) ) ;
#88874=CYLINDRICAL_SURFACE ( 'NONE', #81177, 0.2499999999999997502 ) ;
#88875=CARTESIAN_POINT ( 'NONE',  ( -5.207614543590637801, -3.530157926970578508, 32.79014554554150607 ) ) ;
#88876=ORIENTED_EDGE ( 'NONE', *, *, #54134, .T. ) ;
#88877=EDGE_CURVE ( 'NONE', #43722, #39142, #2038, .T. ) ;
#88878=ORIENTED_EDGE ( 'NONE', *, *, #50367, .T. ) ;
#88880=CARTESIAN_POINT ( 'NONE',  ( -13.63459212866397685, -12.41104346484419452, 31.60698883733904196 ) ) ;
#88881=CARTESIAN_POINT ( 'NONE',  ( -1.607542343522231798, -2.523278758544489353, 31.42238647778637528 ) ) ;
#88882=CARTESIAN_POINT ( 'NONE',  ( -3.230769230769229949, -12.29105614889573062, 35.45975837776705220 ) ) ;
#88883=CARTESIAN_POINT ( 'NONE',  ( 16.21899193317811694, -7.750023238201980469, 34.74374492549440419 ) ) ;
#88884=AXIS2_PLACEMENT_3D ( 'NONE', #30382, #57851, #17312 ) ;
#88885=CARTESIAN_POINT ( 'NONE',  ( -8.899921372341079717, -6.369640206132551441, 34.87707690430378449 ) ) ;
#88886=FACE_BOUND ( 'NONE', #56047, .T. ) ;
#88887=VERTEX_POINT ( 'NONE', #84943 ) ;
#88888=ADVANCED_FACE ( 'NONE', ( #49373 ), #9282, .F. ) ;
#88889=CARTESIAN_POINT ( 'NONE',  ( -14.98076923076922462, -2.499999999999999556, 29.81604066197449754 ) ) ;
#88891=CARTESIAN_POINT ( 'NONE',  ( 15.23076923076923173, -11.69971097300155272, 32.46337939537588113 ) ) ;
#88892=ORIENTED_EDGE ( 'NONE', *, *, #19689, .T. ) ;
#88893=CARTESIAN_POINT ( 'NONE',  ( -8.519230769230768274, -2.499999999999998668, 29.75000000000000355 ) ) ;
#88894=AXIS2_PLACEMENT_3D ( 'NONE', #35228, #22166, #8211 ) ;
#88895=EDGE_LOOP ( 'NONE', ( #70410, #1027 ) ) ;
#88896=EDGE_CURVE ( 'NONE', #1750, #14097, #13839, .T. ) ;
#88897=FACE_BOUND ( 'NONE', #12432, .T. ) ;
#88898=CARTESIAN_POINT ( 'NONE',  ( -9.692307692307691624, -1.790695186598648903, 34.54067556320373455 ) ) ;
#88899=VERTEX_POINT ( 'NONE', #64640 ) ;
#88900=DIRECTION ( 'NONE',  ( -0.000000000000000000, 0.9848077530122085754, -0.1736481776669273613 ) ) ;
#88901=DIRECTION ( 'NONE',  ( 0.000000000000000000, 0.000000000000000000, 1.000000000000000000 ) ) ;
#88902=EDGE_CURVE ( 'NONE', #80080, #20644, #54677, .T. ) ;
#88903=AXIS2_PLACEMENT_3D ( 'NONE', #60226, #11157, #73306 ) ;
#88905=VERTEX_POINT ( 'NONE', #70083 ) ;
#88906=CARTESIAN_POINT ( 'NONE',  ( 6.792385456409365752, -9.804603061927743113, 34.18744698557895845 ) ) ;
#88907=DIRECTION ( 'NONE',  ( -0.000000000000000000, -0.9396926207859093161, -0.3420201433256663259 ) ) ;
#88909=CARTESIAN_POINT ( 'NONE',  ( 2.557746727605761272, -2.920487667080175154, 32.31805714834170828 ) ) ;
#88911=CARTESIAN_POINT ( 'NONE',  ( 13.16113044089144068, -5.912607949931405926, 34.49155766932282319 ) ) ;
#88912=CARTESIAN_POINT ( 'NONE',  ( 2.307692307692187583, -2.892918686052166066, 31.69288490824153470 ) ) ;
#88914=ORIENTED_EDGE ( 'NONE', *, *, #23073, .T. ) ;
#88915=CARTESIAN_POINT ( 'NONE',  ( -8.546451227962355901, -10.81320215134717344, 33.49497208177562868 ) ) ;
#88916=CARTESIAN_POINT ( 'NONE',  ( -4.376772371362300795, -2.554751324335733820, 30.48935550225260727 ) ) ;
#88917=CARTESIAN_POINT ( 'NONE',  ( -13.25408968285182354, -5.195472089885680766, 34.18748526763464923 ) ) ;
#88918=LINE ( 'NONE', #60079, #5520 ) ;
#88919=CARTESIAN_POINT ( 'NONE',  ( -10.39237326377176451, -2.554770724473667265, 30.48948780036025852 ) ) ;
#88920=LINE ( 'NONE', #7810, #32313 ) ;
#88921=CARTESIAN_POINT ( 'NONE',  ( 14.24244131753106757, -2.506253911140460922, 30.00000000000013856 ) ) ;
#88922=DIRECTION ( 'NONE',  ( -0.000000000000000000, 0.8660254037844399289, -0.4999999999999980016 ) ) ;
#88923=CARTESIAN_POINT ( 'NONE',  ( -0.4615384615385840772, -11.67786785259630911, 32.92929555188603530 ) ) ;
#88929=VECTOR ( 'NONE', #56869, 1000.000000000000227 ) ;
#88930=ADVANCED_FACE ( 'NONE', ( #2943 ), #70532, .F. ) ;
#88932=CARTESIAN_POINT ( 'NONE',  ( -11.31568186948346977, -2.353885683473779800, 30.79025554430704403 ) ) ;
#88933=ORIENTED_EDGE ( 'NONE', *, *, #42999, .T. ) ;
#88934=CARTESIAN_POINT ( 'NONE',  ( 1.515405825582335497, -11.93129842949671726, 32.56571108434900452 ) ) ;
#88937=DIRECTION ( 'NONE',  ( -0.000000000000000000, 0.9848077530122085754, -0.1736481776669273613 ) ) ;
#88938=CARTESIAN_POINT ( 'NONE',  ( 6.000000000000001776, -3.050289026998446396, 32.03036669348365706 ) ) ;
#88940=CARTESIAN_POINT ( 'NONE',  ( 1.318533005255251078, -2.486705287966279876, 31.30864560766542937 ) ) ;
#88941=CARTESIAN_POINT ( 'NONE',  ( 9.823098133274644539, -12.35292014791297710, 31.75344720912887198 ) ) ;
#88942=CARTESIAN_POINT ( 'NONE',  ( 2.057669070399343880, -10.05641848906368097, 34.04755513067966177 ) ) ;
#88943=CARTESIAN_POINT ( 'NONE',  ( 6.923076923076924238, -12.34228464037088635, 31.77849191805839268 ) ) ;
#88944=EDGE_CURVE ( 'NONE', #75182, #51245, #25659, .T. ) ;
#88946=CARTESIAN_POINT ( 'NONE',  ( 11.40831432902331954, -10.88202310037935661, 33.43294751532457099 ) ) ;
#88948=CARTESIAN_POINT ( 'NONE',  ( 14.30769230769218581, -12.16647553114689728, 32.15551576947799362 ) ) ;
#88949=EDGE_CURVE ( 'NONE', #44707, #34883, #29990, .T. ) ;
#88951=ORIENTED_EDGE ( 'NONE', *, *, #10684, .T. ) ;
#88952=ORIENTED_EDGE ( 'NONE', *, *, #4658, .T. ) ;
#88953=CARTESIAN_POINT ( 'NONE',  ( -15.10024352900566846, -8.586989748646452369, 34.63063291749215011 ) ) ;
#88954=CARTESIAN_POINT ( 'NONE',  ( 5.142991427925513115, -8.973038597847269315, 34.52809138561122637 ) ) ;
#88955=CARTESIAN_POINT ( 'NONE',  ( -6.700297254098857458, -12.11081565061823717, 32.26097654155341843 ) ) ;
#88956=LINE ( 'NONE', #62331, #71456 ) ;
#88957=B_SPLINE_CURVE_WITH_KNOTS ( 'NONE', 3,
 ( #75780, #46975, #74458, #40241, #88442, #82565, #13205, #20839, #27156, #40686 ),
 .UNSPECIFIED., .F., .F.,
 ( 4, 2, 2, 2, 4 ),
 ( 0.000000000000000000, 0.0001954311564186866305, 0.0003908623128373732609, 0.0005862934692560598914, 0.0007817246256747465219 ),
 .UNSPECIFIED. ) ;
#88958=CARTESIAN_POINT ( 'NONE',  ( 8.638539302563209787, -4.118384482072086072, 33.43331474514187107 ) ) ;
#88959=CARTESIAN_POINT ( 'NONE',  ( -9.561782254074051579, -11.04252011169590020, 33.62494198852677130 ) ) ;
#88960=EDGE_CURVE ( 'NONE', #74135, #25790, #66487, .T. ) ;
#88961=CARTESIAN_POINT ( 'NONE',  ( -2.307692307692305711, -8.164416787775445883, 34.95778746994557906 ) ) ;
#88962=ORIENTED_EDGE ( 'NONE', *, *, #79960, .T. ) ;
#88963=CARTESIAN_POINT ( 'NONE',  ( 16.15384615384615330, -2.721908614388771852, 31.22303859784724978 ) ) ;
#88964=ORIENTED_EDGE ( 'NONE', *, *, #68663, .F. ) ;
#88965=DIRECTION ( 'NONE',  ( 0.000000000000000000, 0.7660444431189807890, 0.6427876096865361433 ) ) ;
#88966=CARTESIAN_POINT ( 'NONE',  ( -18.22520792652322186, -12.74865929289141953, 29.87818027815293220 ) ) ;
#88967=CARTESIAN_POINT ( 'NONE',  ( -4.376772371362299019, -4.186968288167446595, 33.49512374952580274 ) ) ;
#88968=CARTESIAN_POINT ( 'NONE',  ( 3.230769230769231726, -8.164416787775445883, 34.95778746994557906 ) ) ;
#88969=LINE ( 'NONE', #27239, #58201 ) ;
#88970=EDGE_CURVE ( 'NONE', #79461, #2166, #24106, .T. ) ;
#88971=ORIENTED_EDGE ( 'NONE', *, *, #61443, .T. ) ;
#88972=VERTEX_POINT ( 'NONE', #72297 ) ;
#88974=ORIENTED_EDGE ( 'NONE', *, *, #69817, .T. ) ;
#88975=CARTESIAN_POINT ( 'NONE',  ( 17.32686848630112308, -10.18230066228895758, 34.26354781536631577 ) ) ;
#88976=CARTESIAN_POINT ( 'NONE',  ( -15.90390074446811042, -9.357781135181033605, 34.66075350412533851 ) ) ;
#88978=CARTESIAN_POINT ( 'NONE',  ( 14.55769230769372946, -7.500000000000154543, 35.00000000000007105 ) ) ;
#88979=CIRCLE ( 'NONE', #50120, 0.2500000000000002220 ) ;
#88981=CARTESIAN_POINT ( 'NONE',  ( 12.33084785842815378, -2.845849958028613624, 32.17971566917920967 ) ) ;
#88982=ORIENTED_EDGE ( 'NONE', *, *, #29907, .F. ) ;
#88984=ORIENTED_EDGE ( 'NONE', *, *, #71040, .F. ) ;
#88986=CARTESIAN_POINT ( 'NONE',  ( 11.28848480751918437, -9.148715823498378086, 34.47080413974185120 ) ) ;
#88987=ORIENTED_EDGE ( 'NONE', *, *, #4957, .T. ) ;
#88988=CARTESIAN_POINT ( 'NONE',  ( -9.822454901745912181, -5.195881422630166391, 34.18770438780619259 ) ) ;
#88989=CYLINDRICAL_SURFACE ( 'NONE', #27368, 0.2500000000000002220 ) ;
#88991=ORIENTED_EDGE ( 'NONE', *, *, #40164, .T. ) ;
#88992=ADVANCED_FACE ( 'NONE', ( #85828 ), #45718, .F. ) ;
#88993=CARTESIAN_POINT ( 'NONE',  ( -3.100243529005667575, -12.45806712695776319, 30.39783852428763922 ) ) ;
#88995=FACE_OUTER_BOUND ( 'NONE', #71081, .T. ) ;
#88996=ADVANCED_FACE ( 'NONE', ( #73200 ), #74091, .F. ) ;
#88997=FACE_BOUND ( 'NONE', #76893, .T. ) ;
#88998=CARTESIAN_POINT ( 'NONE',  ( 4.946775107191379028, -5.070767119584671079, 34.40440758774516183 ) ) ;
#88999=FACE_OUTER_BOUND ( 'NONE', #75719, .T. ) ;
#89000=VERTEX_POINT ( 'NONE', #51556 ) ;
#89001=DIRECTION ( 'NONE',  ( -0.000000000000000000, -0.000000000000000000, -1.000000000000000000 ) ) ;
#89003=CARTESIAN_POINT ( 'NONE',  ( -14.05774678934416499, -2.587454068350147018, 30.68340429815432202 ) ) ;
#89004=CARTESIAN_POINT ( 'NONE',  ( -16.94613263595612906, -12.62708834333097663, 30.88030960425256310 ) ) ;
#89005=CARTESIAN_POINT ( 'NONE',  ( 15.29683656411930848, -6.343179335718452272, 34.87096338111212646 ) ) ;
#89007=EDGE_CURVE ( 'NONE', #18413, #9576, #52022, .T. ) ;
#89008=CARTESIAN_POINT ( 'NONE',  ( -0.2115384615385247913, -7.565270000091922853, 34.99999999999999289 ) ) ;
#89009=CARTESIAN_POINT ( 'NONE',  ( 1.161688425708536254, -4.026226216239095379, 33.68668979543632958 ) ) ;
#89010=CARTESIAN_POINT ( 'NONE',  ( -10.54931728203453822, -2.292212530054420494, 30.41441678777542990 ) ) ;
#89011=LINE ( 'NONE', #74593, #57261 ) ;
#89012=CARTESIAN_POINT ( 'NONE',  ( -14.30769230769230660, -6.435427911321262684, 35.78748833219616898 ) ) ;
#89013=FACE_BOUND ( 'NONE', #55755, .T. ) ;
#89014=CARTESIAN_POINT ( 'NONE',  ( 5.869852030268305931, -5.070767119584671079, 34.40440758774516183 ) ) ;
#89015=CARTESIAN_POINT ( 'NONE',  ( -17.32694630114453460, -10.92453946501458439, 33.72985991061850086 ) ) ;
#89016=CARTESIAN_POINT ( 'NONE',  ( -14.53061926659915315, -3.395401636524185474, 33.02366814457250399 ) ) ;
#89017=CARTESIAN_POINT ( 'NONE',  ( -18.00000000000000000, -2.292212530054419606, 30.41441678777542990 ) ) ;
#89018=CARTESIAN_POINT ( 'NONE',  ( 15.45354877203763522, -10.11255958852956027, 34.01340905677048454 ) ) ;
#89020=CARTESIAN_POINT ( 'NONE',  ( -7.976844449264153702, -3.957541250942358424, 33.62499894934981626 ) ) ;
#89022=B_SPLINE_CURVE_WITH_KNOTS ( 'NONE', 3,
 ( #24431, #32985, #3723, #31194, #18139, #4621, #45598, #87964, #58666, #45152 ),
 .UNSPECIFIED., .F., .F.,
 ( 4, 2, 2, 2, 4 ),
 ( 0.000000000000000000, 0.0001954311564186861426, 0.0003908623128373722852, 0.0005862934692560583735, 0.0007817246256747445703 ),
 .UNSPECIFIED. ) ;
#89023=ORIENTED_EDGE ( 'NONE', *, *, #88323, .T. ) ;
#89024=CARTESIAN_POINT ( 'NONE',  ( 1.161130440891436466, -12.24155766932282496, 31.33739205006857986 ) ) ;
#89026=DIRECTION ( 'NONE',  ( -0.000000000000000000, -0.5000000000000009992, -0.8660254037844380415 ) ) ;
#89027=ORIENTED_EDGE ( 'NONE', *, *, #29966, .F. ) ;
#89028=CARTESIAN_POINT ( 'NONE',  ( -4.023054346021366356, -12.11778462344220841, 31.66786338562085135 ) ) ;
#89029=CARTESIAN_POINT ( 'NONE',  ( 17.07692307692295586, -10.90142922262034020, 33.41473453929536674 ) ) ;
#89030=CARTESIAN_POINT ( 'NONE',  ( -10.61538461538473577, -11.67786785259630911, 32.92929555188603530 ) ) ;
#89031=ORIENTED_EDGE ( 'NONE', *, *, #75644, .F. ) ;
#89032=CARTESIAN_POINT ( 'NONE',  ( -9.442307692306256328, -7.500000000000155431, 34.75000000000007105 ) ) ;
#89034=B_SPLINE_CURVE_WITH_KNOTS ( 'NONE', 3,
 ( #80944, #14240, #6156, #60645, #41716, #88157, #61528, #61091, #26431, #89036 ),
 .UNSPECIFIED., .F., .F.,
 ( 4, 2, 2, 2, 4 ),
 ( 0.000000000000000000, 0.0001954339857564070678, 0.0003908679715128141356, 0.0005863019572692211492, 0.0007817359430256282712 ),
 .UNSPECIFIED. ) ;
#89035=CARTESIAN_POINT ( 'NONE',  ( -0.4615384615384611200, -2.833524468853757305, 32.15551576947925838 ) ) ;
#89036=CARTESIAN_POINT ( 'NONE',  ( 5.076923076922954969, -5.219633306517616589, 34.19971097300220464 ) ) ;
#89038=CARTESIAN_POINT ( 'NONE',  ( 4.087762742890271639, -11.69971097300155272, 32.46337939537587403 ) ) ;
#89039=CARTESIAN_POINT ( 'NONE',  ( -12.21148404162501144, -8.346898887586323923, 34.93166121998716278 ) ) ;
#89040=CARTESIAN_POINT ( 'NONE',  ( 3.230769230769231726, -9.780366693483667717, 34.19971097300155094 ) ) ;
#89042=LINE ( 'NONE', #54782, #1672 ) ;
#89043=CARTESIAN_POINT ( 'NONE',  ( 5.076923076923075762, -2.486705287966279876, 31.30864560766543647 ) ) ;
#89044=ORIENTED_EDGE ( 'NONE', *, *, #75644, .T. ) ;
#89045=CARTESIAN_POINT ( 'NONE',  ( 13.38461538461538680, -4.661471528628507777, 34.16647553114623292 ) ) ;
#89047=EDGE_CURVE ( 'NONE', #1690, #48302, #80544, .T. ) ;
#89048=CARTESIAN_POINT ( 'NONE',  ( 2.057715563643716994, -4.818429247618089661, 34.26397095200675125 ) ) ;
#89049=CARTESIAN_POINT ( 'NONE',  ( 17.07692307692307665, -11.69971097300155272, 32.46337939537588113 ) ) ;
#89050=VERTEX_POINT ( 'NONE', #39865 ) ;
#89051=CARTESIAN_POINT ( 'NONE',  ( -5.999999999999998224, -12.09954503811598769, 35.62045528018868623 ) ) ;
#89052=CARTESIAN_POINT ( 'NONE',  ( -14.30769230769230660, -11.16473453929635440, 33.15142922261926373 ) ) ;
#89053=CARTESIAN_POINT ( 'NONE',  ( -17.32692307692307665, -7.500000000000001776, 34.75000000000000000 ) ) ;
#89054=ORIENTED_EDGE ( 'NONE', *, *, #5456, .F. ) ;
#89055=LINE ( 'NONE', #27333, #18179 ) ;
#89056=CARTESIAN_POINT ( 'NONE',  ( 15.48071464014727106, -5.766571408460171355, 34.70601412856602508 ) ) ;
#89057=CARTESIAN_POINT ( 'NONE',  ( -10.36533019547115941, -9.233818618650603938, 34.70587769442853698 ) ) ;
#89058=EDGE_CURVE ( 'NONE', #72792, #58923, #18158, .T. ) ;
#89059=B_SPLINE_CURVE_WITH_KNOTS ( 'NONE', 3,
 ( #21287, #48761, #42022, #28054, #76232, #55961, #71241, #1026, #9548, #1909 ),
 .UNSPECIFIED., .F., .F.,
 ( 4, 2, 2, 2, 4 ),
 ( 0.0007817246256747478229, 0.0009771112852218913694, 0.001172497944769034916, 0.001367884604316178679, 0.001563271263863322226 ),
 .UNSPECIFIED. ) ;
#89060=AXIS2_PLACEMENT_3D ( 'NONE', #49017, #89144, #27421 ) ;
#89061=CARTESIAN_POINT ( 'NONE',  ( -16.82686876528475750, -2.779044189368096607, 31.39831045268885035 ) ) ;
#89062=CARTESIAN_POINT ( 'NONE',  ( -18.22292621751614305, -12.15238873228291716, 31.58232369045353849 ) ) ;
#89064=EDGE_CURVE ( 'NONE', #85070, #60833, #25452, .T. ) ;
#89065=DIRECTION ( 'NONE',  ( -0.000000000000000000, -0.9848077530122086864, -0.1736481776669273613 ) ) ;
#89066=ORIENTED_EDGE ( 'NONE', *, *, #17809, .T. ) ;
#89067=VERTEX_POINT ( 'NONE', #46173 ) ;
#89068=ORIENTED_EDGE ( 'NONE', *, *, #66184, .F. ) ;
#89069=ORIENTED_EDGE ( 'NONE', *, *, #72290, .F. ) ;
#89071=CARTESIAN_POINT ( 'NONE',  ( 8.769230769230768274, -9.058645607665452459, 34.76329471203371924 ) ) ;
#89072=CARTESIAN_POINT ( 'NONE',  ( 9.915087233576098669, -5.114059244376869984, 34.14424750095245287 ) ) ;
#89073=CARTESIAN_POINT ( 'NONE',  ( 5.076923076923075762, -13.75783147151868846, 33.36296068462461051 ) ) ;
#89076=ORIENTED_EDGE ( 'NONE', *, *, #82653, .F. ) ;
#89077=EDGE_CURVE ( 'NONE', #69942, #45555, #26781, .T. ) ;
#89078=ADVANCED_FACE ( 'NONE', ( #61007 ), #75853, .F. ) ;
#89079=B_SPLINE_CURVE_WITH_KNOTS ( 'NONE', 3,
 ( #48496, #14277, #7076, #62885, #28685, #41759, #69661, #22793, #48945, #68779 ),
 .UNSPECIFIED., .F., .F.,
 ( 4, 2, 2, 2, 4 ),
 ( 0.0007817246256747489071, 0.0009771112852218922368, 0.001172497944769035350, 0.001367884604316178679, 0.001563271263863322009 ),
 .UNSPECIFIED. ) ;
#89080=VERTEX_POINT ( 'NONE', #61885 ) ;
#89081=VERTEX_POINT ( 'NONE', #67770 ) ;
#89082=DIRECTION ( 'NONE',  ( -0.000000000000000000, 0.9396926207859092051, -0.3420201433256662704 ) ) ;
#89083=ORIENTED_EDGE ( 'NONE', *, *, #715, .T. ) ;
#89084=CARTESIAN_POINT ( 'NONE',  ( -1.514763354347082869, -3.069018819979302926, 32.56621877034667278 ) ) ;
#89085=VECTOR ( 'NONE', #14989, 1000.000000000000000 ) ;
#89086=ADVANCED_FACE ( 'NONE', ( #47932 ), #27223, .F. ) ;
#89089=DIRECTION ( 'NONE',  ( 0.000000000000000000, 0.9396926207859126468, -0.3420201433256571111 ) ) ;
#89090=ORIENTED_EDGE ( 'NONE', *, *, #86120, .F. ) ;
#89091=ORIENTED_EDGE ( 'NONE', *, *, #48146, .F. ) ;
#89092=ORIENTED_EDGE ( 'NONE', *, *, #82470, .T. ) ;
#89093=CARTESIAN_POINT ( 'NONE',  ( -9.561781990544128362, -6.001044277235009439, 34.52024696741798948 ) ) ;
#89095=ORIENTED_EDGE ( 'NONE', *, *, #6820, .T. ) ;
#89096=B_SPLINE_CURVE_WITH_KNOTS ( 'NONE', 3,
 ( #18095, #59513, #17649, #66720, #87016, #72132, #52750, #10446, #44648, #73929 ),
 .UNSPECIFIED., .F., .F.,
 ( 4, 2, 2, 2, 4 ),
 ( 0.000000000000000000, 0.0001954311564186860071, 0.0003908623128373720141, 0.0005862934692560580483, 0.0007817246256747440282 ),
 .UNSPECIFIED. ) ;
#89097=CARTESIAN_POINT ( 'NONE',  ( -11.40793610022789828, -12.70449254468099198, 30.44128974285582956 ) ) ;
#89098=CARTESIAN_POINT ( 'NONE',  ( -14.55766903863466055, -2.564618984488975073, 30.55390908950641915 ) ) ;
#89099=ORIENTED_EDGE ( 'NONE', *, *, #504, .F. ) ;
#89100=CARTESIAN_POINT ( 'NONE',  ( -17.86920819217521483, -2.541949514083464479, 30.39797389878541267 ) ) ;
#89101=CARTESIAN_POINT ( 'NONE',  ( -1.384615384615383471, -1.044019251281081972, 31.83374038241031911 ) ) ;
#89102=FACE_BOUND ( 'NONE', #20936, .T. ) ;
#89103=CARTESIAN_POINT ( 'NONE',  ( -17.93474442872397034, -8.613356846314930593, 34.62446782046653482 ) ) ;
#89104=CARTESIAN_POINT ( 'NONE',  ( -18.13014796973170206, -12.50552854090298638, 31.33409797877408920 ) ) ;
#89105=EDGE_CURVE ( 'NONE', #87879, #88017, #46068, .T. ) ;
#89106=CARTESIAN_POINT ( 'NONE',  ( 3.230769230769110045, -9.442884908241554243, 34.35708131394783038 ) ) ;
#89108=CARTESIAN_POINT ( 'NONE',  ( 18.00000000000000000, -4.098570777380720287, 33.41473453929634729 ) ) ;
#89109=AXIS2_PLACEMENT_3D ( 'NONE', #9521, #15854, #16285 ) ;
#89111=CARTESIAN_POINT ( 'NONE',  ( -3.930833309752757021, -11.43677907613344757, 33.22367315496201456 ) ) ;
#89112=ORIENTED_EDGE ( 'NONE', *, *, #54167, .T. ) ;
#89113=DIRECTION ( 'NONE',  ( -0.000000000000000000, 0.7660444431189791237, -0.6427876096865379196 ) ) ;
#89114=DIRECTION ( 'NONE',  ( 0.000000000000000000, 0.6427876096865368094, 0.7660444431189802339 ) ) ;
#89116=ORIENTED_EDGE ( 'NONE', *, *, #69648, .F. ) ;
#89117=EDGE_CURVE ( 'NONE', #30707, #67360, #65356, .T. ) ;
#89118=CARTESIAN_POINT ( 'NONE',  ( 8.703960323269994248, -3.300289026998414865, 32.46337939537583139 ) ) ;
#89119=CARTESIAN_POINT ( 'NONE',  ( -4.153846153846152411, -3.322132147404559976, 32.92929555188717927 ) ) ;
#89121=DIRECTION ( 'NONE',  ( -0.000000000000000000, 0.6427876096865404731, -0.7660444431189770143 ) ) ;
#89122=FACE_OUTER_BOUND ( 'NONE', #44387, .T. ) ;
#89123=FACE_BOUND ( 'NONE', #47086, .T. ) ;
#89124=CARTESIAN_POINT ( 'NONE',  ( 13.38461538461538680, -1.117168528481311540, 33.14645433367849847 ) ) ;
#89126=CARTESIAN_POINT ( 'NONE',  ( -9.019207500173124004, -6.567427716900048118, 34.66269422305636283 ) ) ;
#89127=CARTESIAN_POINT ( 'NONE',  ( 2.307692307692187583, -5.219633306517616589, 34.19971097300220464 ) ) ;
#89129=CARTESIAN_POINT ( 'NONE',  ( -14.24254752697267712, -7.750023224968867197, 34.99404313364389907 ) ) ;
#89130=EDGE_CURVE ( 'NONE', #62909, #28968, #19579, .T. ) ;
#89133=EDGE_LOOP ( 'NONE', ( #73635, #27233 ) ) ;
#89134=CARTESIAN_POINT ( 'NONE',  ( -12.21159305216042057, -5.766571408460171355, 34.70601412856602508 ) ) ;
#89136=CYLINDRICAL_SURFACE ( 'NONE', #1400, 0.2499999999999995559 ) ;
#89137=CARTESIAN_POINT ( 'NONE',  ( -13.38461538461538325, -13.37000171582298513, 34.34916445242398453 ) ) ;
#89138=DIRECTION ( 'NONE',  ( 0.000000000000000000, 0.1736481776669267785, -0.9848077530122087975 ) ) ;
#89140=CARTESIAN_POINT ( 'NONE',  ( 0.5267936010512989098, -4.320704448112861584, 33.92786785259548310 ) ) ;
#89141=CARTESIAN_POINT ( 'NONE',  ( 5.999999999999878320, -3.083524468854526912, 32.58852847137268327 ) ) ;
#89142=EDGE_CURVE ( 'NONE', #48499, #51319, #31067, .T. ) ;
#89143=CARTESIAN_POINT ( 'NONE',  ( -17.14219352288385778, -5.219633306516282545, 34.19971097300152252 ) ) ;
#89144=DIRECTION ( 'NONE',  ( -0.000000000000000000, -0.6427876096865404731, -0.7660444431189770143 ) ) ;
#89145=CARTESIAN_POINT ( 'NONE',  ( -1.607494901352970018, -7.630690623152302621, 34.99857592706774057 ) ) ;
#89146=CARTESIAN_POINT ( 'NONE',  ( 7.846153846153846700, -11.33034616979429110, 35.88435417666054406 ) ) ;
#89147=CARTESIAN_POINT ( 'NONE',  ( 5.750023269057648712, -12.17611988154120972, 31.52148481390971213 ) ) ;
#89148=CARTESIAN_POINT ( 'NONE',  ( -6.792286482109968659, -3.338503747796866872, 32.95102852606553512 ) ) ;
#89149=DIRECTION ( 'NONE',  ( -0.000000000000000000, 0.9396926207859093161, -0.3420201433256663259 ) ) ;
#89150=ORIENTED_EDGE ( 'NONE', *, *, #12414, .F. ) ;
#89151=B_SPLINE_CURVE_WITH_KNOTS ( 'NONE', 3,
 ( #71016, #36350, #63812, #43538, #36786, #85421 ),
 .UNSPECIFIED., .F., .F.,
 ( 4, 2, 4 ),
 ( 4.220987180333913997E-17, 0.0001954756301637163962, 0.0003909512603273906169 ),
 .UNSPECIFIED. ) ;
#89152=VECTOR ( 'NONE', #11227, 1000.000000000000227 ) ;
#89153=CARTESIAN_POINT ( 'NONE',  ( 4.153846153846032507, -5.219633306517616589, 34.19971097300220464 ) ) ;
#89154=CARTESIAN_POINT ( 'NONE',  ( 10.83816428436267820, -5.827830569534417471, 34.72679350104403539 ) ) ;
#89156=ADVANCED_FACE ( 'NONE', ( #74528 ), #82179, .F. ) ;
#89158=CYLINDRICAL_SURFACE ( 'NONE', #12611, 0.2499999999999994726 ) ;
#89159=CARTESIAN_POINT ( 'NONE',  ( -1.384615384615383471, -4.098570777380720287, 33.41473453929634729 ) ) ;
#89160=ORIENTED_EDGE ( 'NONE', *, *, #16989, .F. ) ;
#89162=EDGE_CURVE ( 'NONE', #40515, #75886, #78283, .T. ) ;
#89163=CARTESIAN_POINT ( 'NONE',  ( 12.71148387091650278, -5.766571408460171355, 34.70601412856602508 ) ) ;
#89165=DIRECTION ( 'NONE',  ( -0.000000000000000000, -0.6427876096865404731, -0.7660444431189771253 ) ) ;
#89166=LINE ( 'NONE', #27447, #6899 ) ;
#89168=CARTESIAN_POINT ( 'NONE',  ( 14.24160889673642494, -2.538708090699994813, 30.37095296980875148 ) ) ;
#89169=CARTESIAN_POINT ( 'NONE',  ( -15.45359732840411482, -7.369209533119140509, 34.99857337881830688 ) ) ;
#89170=ADVANCED_FACE ( 'NONE', ( #84843 ), #23122, .F. ) ;
#89172=DIRECTION ( 'NONE',  ( -0.000000000000000000, -0.9396926207859092051, -0.3420201433256662704 ) ) ;
#89173=EDGE_CURVE ( 'NONE', #47774, #81622, #7846, .T. ) ;
#89174=VERTEX_POINT ( 'NONE', #56020 ) ;
#89175=ORIENTED_EDGE ( 'NONE', *, *, #7040, .T. ) ;
#89176=CARTESIAN_POINT ( 'NONE',  ( 15.23076923076910916, -5.094484230521993062, 34.41647553114689373 ) ) ;
#89177=EDGE_LOOP ( 'NONE', ( #84198, #54984 ) ) ;
#89178=VECTOR ( 'NONE', #82655, 1000.000000000000114 ) ;
#89179=CARTESIAN_POINT ( 'NONE',  ( -18.00000000000012079, -3.083524468854528244, 32.58852847137268327 ) ) ;
#89180=EDGE_LOOP ( 'NONE', ( #83664, #14420, #71966, #67456 ) ) ;
ENDSEC;
END-ISO-10303-21;
